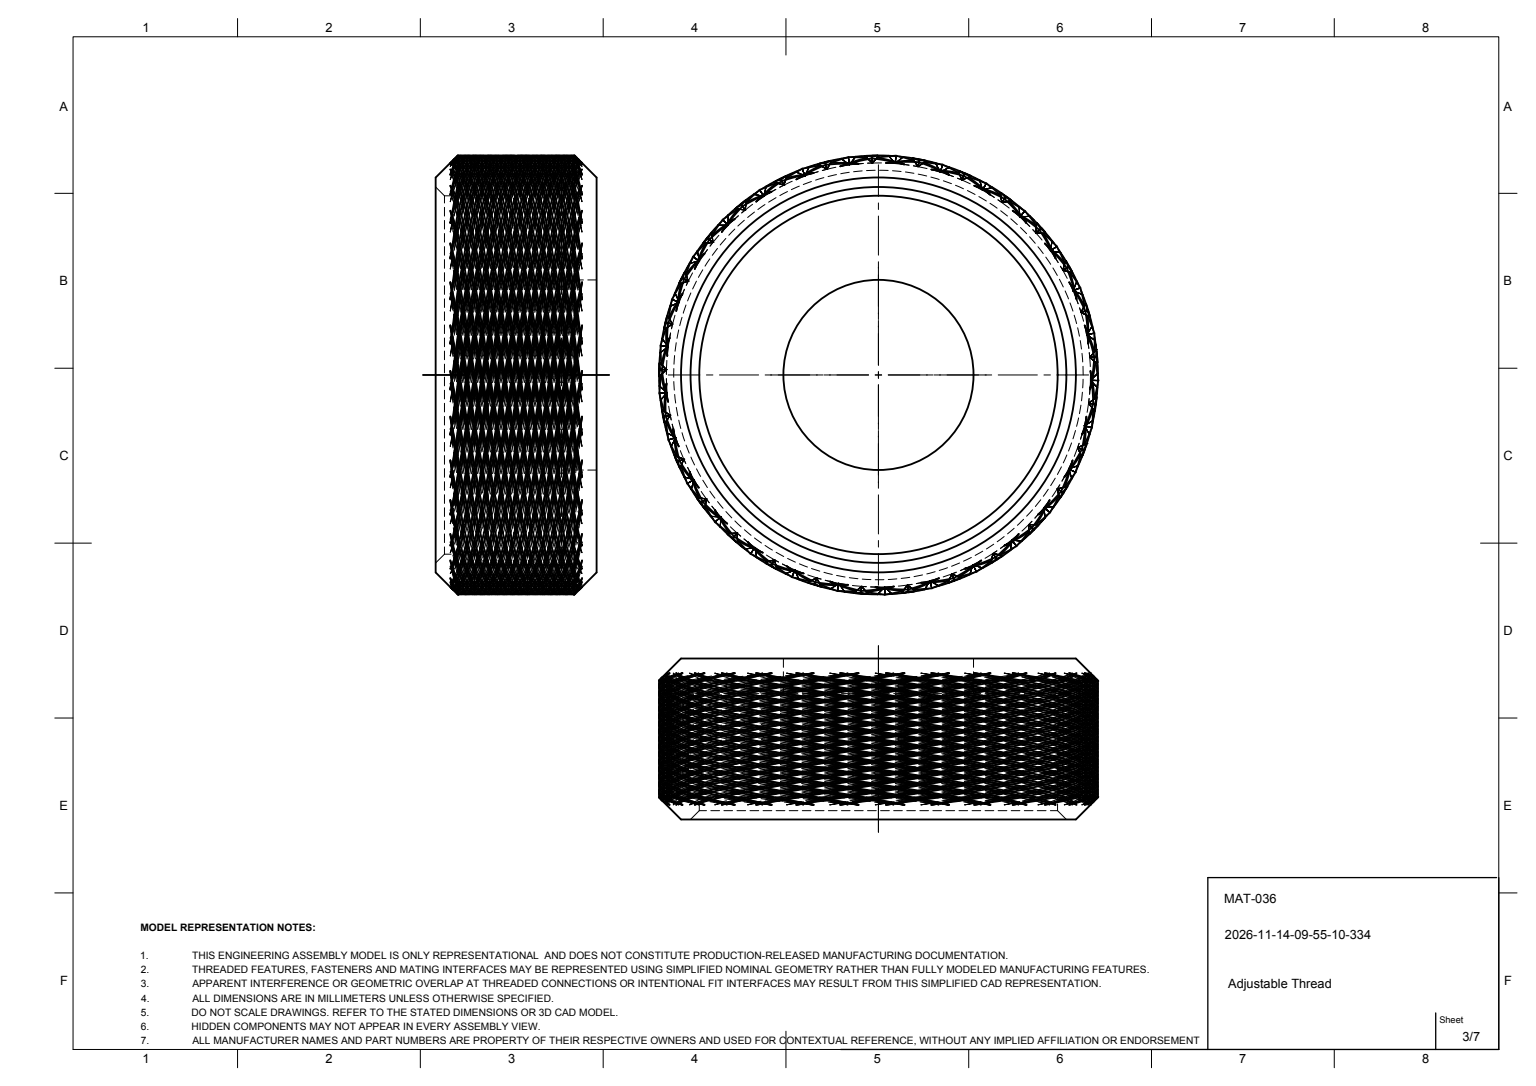
ISO-10303-21;
HEADER;
/* Generated by software containing ST-Developer
 * from STEP Tools, Inc. (www.steptools.com) 
 */

FILE_DESCRIPTION(
/* description */ (''),
/* implementation_level */ '2;1');

FILE_NAME(
/* name */ 'Adjustable Thread.step',
/* time_stamp */ '2026-11-14T09:55:16-08:00',
/* author */ (''),
/* organization */ (''),
/* preprocessor_version */ 'ST-DEVELOPER v20.2',
/* originating_system */ 'Autodesk Translation Framework v15.17.0.0',
/* authorisation */ '');

FILE_SCHEMA (('AUTOMOTIVE_DESIGN { 1 0 10303 214 3 1 1 }'));
ENDSEC;

DATA;
#10=MECHANICAL_DESIGN_GEOMETRIC_PRESENTATION_REPRESENTATION('',(#56),#170250);
#44=SHAPE_REPRESENTATION_RELATIONSHIP('SRR','None',#170276,#50);
#50=ADVANCED_BREP_SHAPE_REPRESENTATION('',(#64),#170244);
#56=STYLED_ITEM('',(#170315),#64);
#64=MANIFOLD_SOLID_BREP('Body1',#71398);
#70=FACE_BOUND('',#15472,.T.);
#71=FACE_BOUND('',#15675,.T.);
#72=FACE_BOUND('',#15851,.T.);
#73=FACE_BOUND('',#15853,.T.);
#86=PLANE('',#77414);
#87=PLANE('',#77609);
#88=PLANE('',#77639);
#89=PLANE('',#77640);
#112=ELLIPSE('',#76563,9.43047305119864,1.30240788908406);
#113=ELLIPSE('',#76566,9.43046793206525,1.30241506001113);
#114=ELLIPSE('',#76569,9.43050328768157,1.3024182004793);
#115=ELLIPSE('',#76572,9.43068708057878,1.30243363570333);
#116=ELLIPSE('',#76575,9.43006152330499,1.30236357371331);
#117=ELLIPSE('',#76578,9.4302777984402,1.30238875446472);
#118=ELLIPSE('',#76581,9.43072787174344,1.30243587534547);
#119=ELLIPSE('',#76584,9.43045773730215,1.30241075091437);
#120=ELLIPSE('',#76587,9.43030510916545,1.30239601642258);
#121=ELLIPSE('',#76590,9.43064494614307,1.30242369243536);
#122=ELLIPSE('',#76593,9.43056062900003,1.30242031583658);
#123=ELLIPSE('',#76596,9.43045585415815,1.30241175558088);
#124=ELLIPSE('',#76599,9.43046939213538,1.30240966255557);
#125=ELLIPSE('',#76602,9.43067088687587,1.30243579801834);
#126=ELLIPSE('',#76605,9.43040719667397,1.30240457641196);
#127=ELLIPSE('',#76608,9.42988108574405,1.30234497490862);
#128=ELLIPSE('',#76611,9.43068064311873,1.30243410507078);
#129=ELLIPSE('',#76614,9.43052303530734,1.30242084912571);
#130=ELLIPSE('',#76617,9.43038125328305,1.30240668645391);
#131=ELLIPSE('',#76620,9.43072128552616,1.30244009783621);
#132=ELLIPSE('',#76623,9.4305707477918,1.30242345770117);
#133=ELLIPSE('',#76626,9.43046465435441,1.30241113143356);
#134=ELLIPSE('',#76629,9.4308407271015,1.30245127577812);
#135=ELLIPSE('',#76632,9.43070104226015,1.30243878786344);
#136=ELLIPSE('',#76635,9.43055049151391,1.30242224667773);
#137=ELLIPSE('',#76638,9.43061695677763,1.30242474192035);
#138=ELLIPSE('',#76641,9.43035235935973,1.30239838521342);
#139=ELLIPSE('',#76644,9.4305559320503,1.30242196321693);
#140=ELLIPSE('',#76647,9.43068952357752,1.30243327777871);
#141=ELLIPSE('',#77415,9.431895379298,1.30254932670111);
#142=ELLIPSE('',#77418,15.3174410154795,1.90661239924035);
#143=ELLIPSE('',#77421,15.3157768747818,1.90647582479234);
#144=ELLIPSE('',#77424,15.3170696122663,1.90658252792732);
#145=ELLIPSE('',#77427,15.3167139940069,1.90655328959697);
#146=ELLIPSE('',#77430,15.3168209377553,1.90657168275161);
#147=ELLIPSE('',#77433,15.3160754936824,1.90650905813206);
#148=ELLIPSE('',#77436,15.3161208425833,1.90650426169268);
#149=ELLIPSE('',#77439,15.3159589603063,1.90649559716548);
#150=ELLIPSE('',#77442,15.3157944590339,1.9064768703695);
#151=ELLIPSE('',#77445,15.3172323469206,1.9066030234614);
#152=ELLIPSE('',#77448,15.3155039380165,1.9064570427492);
#153=ELLIPSE('',#77451,15.3159291529044,1.90649334528717);
#154=ELLIPSE('',#77454,15.3157700330761,1.90647081272421);
#155=ELLIPSE('',#77457,15.3160955154982,1.90650647722667);
#156=ELLIPSE('',#77460,15.3166693144536,1.90656216883429);
#157=ELLIPSE('',#77463,15.3166817133067,1.90655124693864);
#158=ELLIPSE('',#77466,15.31703730362,1.90657833462818);
#159=ELLIPSE('',#77469,15.3160164937855,1.90649874196003);
#160=ELLIPSE('',#77472,15.3158753484009,1.90648217113556);
#161=ELLIPSE('',#77475,15.3162380117898,1.90650822609983);
#162=ELLIPSE('',#77478,15.3156441463648,1.90646585124018);
#163=ELLIPSE('',#77481,15.317005919152,1.90658194664794);
#164=ELLIPSE('',#77484,15.3161739347467,1.90650429978856);
#165=ELLIPSE('',#77487,15.3153630258202,1.90644004375235);
#166=ELLIPSE('',#77490,15.3163094563979,1.90652013375223);
#167=ELLIPSE('',#77493,15.3167561122212,1.90656182181374);
#168=ELLIPSE('',#77496,15.3163730027201,1.90652953147296);
#169=ELLIPSE('',#77499,15.315903684448,1.90649008174056);
#170=ELLIPSE('',#77530,3.69853833711443,0.520053862149324);
#171=ELLIPSE('',#77535,3.6990050944682,0.520121997590068);
#172=ELLIPSE('',#77538,3.69740745136945,0.519884819312743);
#173=ELLIPSE('',#77541,3.6973850577443,0.519871926709589);
#174=ELLIPSE('',#77544,3.69880689749974,0.520100628836089);
#175=ELLIPSE('',#77547,3.69848799508326,0.520043846508826);
#176=ELLIPSE('',#77552,3.6988594244713,0.520105289468088);
#177=ELLIPSE('',#77555,3.6986202776342,0.520065731438254);
#178=ELLIPSE('',#77558,3.69735633553684,0.519872421748739);
#179=ELLIPSE('',#77561,3.69840385438922,0.520042143078421);
#180=ELLIPSE('',#77566,3.69753466975073,0.519893625210943);
#181=ELLIPSE('',#77569,3.69957450398795,0.520227606150056);
#182=ELLIPSE('',#77574,3.69928463265645,0.520166995452598);
#183=ELLIPSE('',#77579,3.69917885823403,0.520148170670083);
#184=ELLIPSE('',#77582,3.69767815300263,0.519919195910691);
#185=ELLIPSE('',#77589,3.69757944713663,0.519903285571644);
#186=ELLIPSE('',#77592,3.69653763812213,0.519733793607226);
#187=ELLIPSE('',#77595,3.69967418134432,0.520228182339355);
#188=ELLIPSE('',#77598,3.69741584633747,0.519874782638118);
#189=ELLIPSE('',#77601,3.69673411928317,0.519776228529677);
#190=ELLIPSE('',#77604,3.69979295210335,0.520255955848595);
#191=ELLIPSE('',#77607,3.69808486598988,0.51998245490985);
#194=(
BOUNDED_SURFACE()
B_SPLINE_SURFACE(1,2,((#95581,#95582,#95583),(#95584,#95585,#95586)),
 .UNSPECIFIED.,.F.,.F.,.F.)
B_SPLINE_SURFACE_WITH_KNOTS((2,2),(3,3),(0.,0.289681084359929),(0.331965345783649,
0.349369696259361),.UNSPECIFIED.)
GEOMETRIC_REPRESENTATION_ITEM()
RATIONAL_B_SPLINE_SURFACE(((0.988555124858681,0.99035748704491,0.99513694090229),
(0.988555124858681,0.99035748704491,0.99513694090229)))
REPRESENTATION_ITEM('')
SURFACE()
);
#195=(
BOUNDED_SURFACE()
B_SPLINE_SURFACE(1,2,((#95600,#95601,#95602,#95603,#95604),(#95605,#95606,
#95607,#95608,#95609),(#95610,#95611,#95612,#95613,#95614)),
 .UNSPECIFIED.,.F.,.F.,.F.)
B_SPLINE_SURFACE_WITH_KNOTS((2,1,2),(3,2,3),(-0.00289807040992861,0.,0.29039955403664),
(0.383340713896693,0.383933227114987,0.401145492974693),.UNSPECIFIED.)
GEOMETRIC_REPRESENTATION_ITEM()
RATIONAL_B_SPLINE_SURFACE(((0.988246641953811,0.988246641953811,0.988246641953811,
0.986737013496293,0.988139125479962),(0.988246641953811,0.988246641953811,
0.988246641953811,0.986737013496293,0.988139125479962),(0.988246641953811,
0.988246641953811,0.988246641953811,0.986737013496293,0.988139125479961)))
REPRESENTATION_ITEM('')
SURFACE()
);
#196=(
BOUNDED_SURFACE()
B_SPLINE_SURFACE(1,2,((#95639,#95640,#95641),(#95642,#95643,#95644)),
 .UNSPECIFIED.,.F.,.F.,.F.)
B_SPLINE_SURFACE_WITH_KNOTS((2,2),(3,3),(0.,0.289681084359919),(0.331965345783649,
0.349369696259361),.UNSPECIFIED.)
GEOMETRIC_REPRESENTATION_ITEM()
RATIONAL_B_SPLINE_SURFACE(((0.988555124858681,0.99035748704491,0.99513694090229),
(0.988555124858682,0.99035748704491,0.99513694090229)))
REPRESENTATION_ITEM('')
SURFACE()
);
#197=(
BOUNDED_SURFACE()
B_SPLINE_SURFACE(1,2,((#95648,#95649,#95650,#95651,#95652),(#95653,#95654,
#95655,#95656,#95657),(#95658,#95659,#95660,#95661,#95662)),
 .UNSPECIFIED.,.F.,.F.,.F.)
B_SPLINE_SURFACE_WITH_KNOTS((2,1,2),(3,2,3),(-0.00289807040992683,0.,0.290399554012505),
(0.38334071392065,0.383933227114987,0.401145492974695),.UNSPECIFIED.)
GEOMETRIC_REPRESENTATION_ITEM()
RATIONAL_B_SPLINE_SURFACE(((0.988246641953811,0.988246641953811,0.988246641953811,
0.986737013496293,0.988139125479962),(0.988246641953811,0.988246641953811,
0.988246641953811,0.986737013496293,0.988139125479962),(0.988246641953811,
0.988246641953811,0.988246641953811,0.986737013496293,0.988139125479962)))
REPRESENTATION_ITEM('')
SURFACE()
);
#198=(
BOUNDED_SURFACE()
B_SPLINE_SURFACE(1,2,((#95687,#95688,#95689),(#95690,#95691,#95692)),
 .UNSPECIFIED.,.F.,.F.,.F.)
B_SPLINE_SURFACE_WITH_KNOTS((2,2),(3,3),(0.,0.289681084359922),(0.331965345783648,
0.349369696259454),.UNSPECIFIED.)
GEOMETRIC_REPRESENTATION_ITEM()
RATIONAL_B_SPLINE_SURFACE(((0.988555124858681,0.99035748704492,0.995136940902341),
(0.988555124858682,0.99035748704492,0.995136940902341)))
REPRESENTATION_ITEM('')
SURFACE()
);
#199=(
BOUNDED_SURFACE()
B_SPLINE_SURFACE(1,2,((#95696,#95697,#95698,#95699,#95700),(#95701,#95702,
#95703,#95704,#95705),(#95706,#95707,#95708,#95709,#95710)),
 .UNSPECIFIED.,.F.,.F.,.F.)
B_SPLINE_SURFACE_WITH_KNOTS((2,1,2),(3,2,3),(-0.00289807040992654,0.,0.290399554026877),
(0.383340713906249,0.383933227114987,0.401145492974697),.UNSPECIFIED.)
GEOMETRIC_REPRESENTATION_ITEM()
RATIONAL_B_SPLINE_SURFACE(((0.988246641953811,0.988246641953811,0.988246641953811,
0.986737013496293,0.988139125479962),(0.988246641953811,0.988246641953811,
0.988246641953811,0.986737013496293,0.988139125479962),(0.988246641953811,
0.988246641953811,0.988246641953811,0.986737013496293,0.988139125479962)))
REPRESENTATION_ITEM('')
SURFACE()
);
#200=(
BOUNDED_SURFACE()
B_SPLINE_SURFACE(1,2,((#95735,#95736,#95737),(#95738,#95739,#95740)),
 .UNSPECIFIED.,.F.,.F.,.F.)
B_SPLINE_SURFACE_WITH_KNOTS((2,2),(3,3),(0.,0.289681084359918),(0.331965345783649,
0.349369696259361),.UNSPECIFIED.)
GEOMETRIC_REPRESENTATION_ITEM()
RATIONAL_B_SPLINE_SURFACE(((0.988555124858682,0.99035748704491,0.99513694090229),
(0.988555124858682,0.99035748704491,0.99513694090229)))
REPRESENTATION_ITEM('')
SURFACE()
);
#201=(
BOUNDED_SURFACE()
B_SPLINE_SURFACE(1,2,((#95744,#95745,#95746,#95747,#95748),(#95749,#95750,
#95751,#95752,#95753),(#95754,#95755,#95756,#95757,#95758)),
 .UNSPECIFIED.,.F.,.F.,.F.)
B_SPLINE_SURFACE_WITH_KNOTS((2,1,2),(3,2,3),(-0.00289807040992802,0.,0.29039955403663),
(0.383340713896644,0.383933227114987,0.401145492974693),.UNSPECIFIED.)
GEOMETRIC_REPRESENTATION_ITEM()
RATIONAL_B_SPLINE_SURFACE(((0.988246641953811,0.988246641953811,0.988246641953811,
0.986737013496293,0.988139125479962),(0.988246641953811,0.988246641953811,
0.988246641953811,0.986737013496293,0.988139125479962),(0.988246641953811,
0.988246641953811,0.988246641953811,0.986737013496293,0.988139125479962)))
REPRESENTATION_ITEM('')
SURFACE()
);
#202=(
BOUNDED_SURFACE()
B_SPLINE_SURFACE(1,2,((#95783,#95784,#95785),(#95786,#95787,#95788)),
 .UNSPECIFIED.,.F.,.F.,.F.)
B_SPLINE_SURFACE_WITH_KNOTS((2,2),(3,3),(0.,0.289681084359923),(0.331965345783649,
0.349369696259361),.UNSPECIFIED.)
GEOMETRIC_REPRESENTATION_ITEM()
RATIONAL_B_SPLINE_SURFACE(((0.988555124858681,0.99035748704491,0.99513694090229),
(0.988555124858682,0.99035748704491,0.99513694090229)))
REPRESENTATION_ITEM('')
SURFACE()
);
#203=(
BOUNDED_SURFACE()
B_SPLINE_SURFACE(1,2,((#95792,#95793,#95794,#95795,#95796),(#95797,#95798,
#95799,#95800,#95801),(#95802,#95803,#95804,#95805,#95806)),
 .UNSPECIFIED.,.F.,.F.,.F.)
B_SPLINE_SURFACE_WITH_KNOTS((2,1,2),(3,2,3),(-0.00289807040992325,0.,0.290399554035561),
(0.383340713897236,0.383933227114987,0.401145492974693),.UNSPECIFIED.)
GEOMETRIC_REPRESENTATION_ITEM()
RATIONAL_B_SPLINE_SURFACE(((0.988246641953811,0.988246641953811,0.988246641953811,
0.986737013496293,0.988139125479962),(0.988246641953811,0.988246641953811,
0.988246641953811,0.986737013496293,0.988139125479962),(0.988246641953811,
0.988246641953811,0.988246641953811,0.986737013496293,0.988139125479961)))
REPRESENTATION_ITEM('')
SURFACE()
);
#204=(
BOUNDED_SURFACE()
B_SPLINE_SURFACE(1,2,((#95831,#95832,#95833),(#95834,#95835,#95836)),
 .UNSPECIFIED.,.F.,.F.,.F.)
B_SPLINE_SURFACE_WITH_KNOTS((2,2),(3,3),(0.,0.289681084359924),(0.331965345783649,
0.349369696259361),.UNSPECIFIED.)
GEOMETRIC_REPRESENTATION_ITEM()
RATIONAL_B_SPLINE_SURFACE(((0.988555124858681,0.99035748704491,0.99513694090229),
(0.988555124858682,0.99035748704491,0.99513694090229)))
REPRESENTATION_ITEM('')
SURFACE()
);
#205=(
BOUNDED_SURFACE()
B_SPLINE_SURFACE(1,2,((#95840,#95841,#95842,#95843,#95844),(#95845,#95846,
#95847,#95848,#95849),(#95850,#95851,#95852,#95853,#95854)),
 .UNSPECIFIED.,.F.,.F.,.F.)
B_SPLINE_SURFACE_WITH_KNOTS((2,1,2),(3,2,3),(-0.00289807040992448,0.,0.290399554023854),
(0.383340713909065,0.383933227114976,0.401145492974693),.UNSPECIFIED.)
GEOMETRIC_REPRESENTATION_ITEM()
RATIONAL_B_SPLINE_SURFACE(((0.988246641953813,0.988246641953813,0.988246641953813,
0.986737013496292,0.988139125479961),(0.988246641953813,0.988246641953813,
0.988246641953813,0.986737013496292,0.988139125479961),(0.988246641953813,
0.988246641953813,0.988246641953813,0.986737013496292,0.988139125479961)))
REPRESENTATION_ITEM('')
SURFACE()
);
#206=(
BOUNDED_SURFACE()
B_SPLINE_SURFACE(1,2,((#95879,#95880,#95881),(#95882,#95883,#95884)),
 .UNSPECIFIED.,.F.,.F.,.F.)
B_SPLINE_SURFACE_WITH_KNOTS((2,2),(3,3),(0.,0.289681084359932),(0.331965345783649,
0.349369696259361),.UNSPECIFIED.)
GEOMETRIC_REPRESENTATION_ITEM()
RATIONAL_B_SPLINE_SURFACE(((0.988555124858682,0.99035748704491,0.99513694090229),
(0.988555124858682,0.99035748704491,0.99513694090229)))
REPRESENTATION_ITEM('')
SURFACE()
);
#207=(
BOUNDED_SURFACE()
B_SPLINE_SURFACE(1,2,((#95888,#95889,#95890,#95891,#95892),(#95893,#95894,
#95895,#95896,#95897),(#95898,#95899,#95900,#95901,#95902)),
 .UNSPECIFIED.,.F.,.F.,.F.)
B_SPLINE_SURFACE_WITH_KNOTS((2,1,2),(3,2,3),(-0.00289807040992691,0.,0.290399554024332),
(0.383340713908832,0.383933227114987,0.401145492974693),.UNSPECIFIED.)
GEOMETRIC_REPRESENTATION_ITEM()
RATIONAL_B_SPLINE_SURFACE(((0.988246641953811,0.988246641953811,0.988246641953811,
0.986737013496293,0.988139125479962),(0.988246641953811,0.988246641953811,
0.988246641953811,0.986737013496293,0.988139125479962),(0.988246641953811,
0.988246641953811,0.988246641953811,0.986737013496293,0.988139125479962)))
REPRESENTATION_ITEM('')
SURFACE()
);
#208=(
BOUNDED_SURFACE()
B_SPLINE_SURFACE(1,2,((#95912,#95913,#95914),(#95915,#95916,#95917)),
 .UNSPECIFIED.,.F.,.F.,.F.)
B_SPLINE_SURFACE_WITH_KNOTS((2,2),(3,3),(0.,0.289681084359925),(0.331965345783649,
0.349369696259361),.UNSPECIFIED.)
GEOMETRIC_REPRESENTATION_ITEM()
RATIONAL_B_SPLINE_SURFACE(((0.988555124858682,0.99035748704491,0.99513694090229),
(0.988555124858682,0.99035748704491,0.99513694090229)))
REPRESENTATION_ITEM('')
SURFACE()
);
#209=(
BOUNDED_SURFACE()
B_SPLINE_SURFACE(1,2,((#95921,#95922,#95923,#95924,#95925),(#95926,#95927,
#95928,#95929,#95930),(#95931,#95932,#95933,#95934,#95935)),
 .UNSPECIFIED.,.F.,.F.,.F.)
B_SPLINE_SURFACE_WITH_KNOTS((2,1,2),(3,2,3),(-0.00289807040992912,0.,0.290399554034495),
(0.383340713898888,0.383933227114987,0.401145492974693),.UNSPECIFIED.)
GEOMETRIC_REPRESENTATION_ITEM()
RATIONAL_B_SPLINE_SURFACE(((0.988246641953811,0.988246641953811,0.988246641953811,
0.986737013496293,0.988139125479962),(0.988246641953811,0.988246641953811,
0.988246641953811,0.986737013496293,0.988139125479962),(0.988246641953811,
0.988246641953811,0.988246641953811,0.986737013496293,0.988139125479962)))
REPRESENTATION_ITEM('')
SURFACE()
);
#210=(
BOUNDED_SURFACE()
B_SPLINE_SURFACE(1,2,((#95960,#95961,#95962),(#95963,#95964,#95965)),
 .UNSPECIFIED.,.F.,.F.,.F.)
B_SPLINE_SURFACE_WITH_KNOTS((2,2),(3,3),(0.,0.28968108435992),(0.331965345783649,
0.349369696259364),.UNSPECIFIED.)
GEOMETRIC_REPRESENTATION_ITEM()
RATIONAL_B_SPLINE_SURFACE(((0.988555124858682,0.990357487044911,0.995136940902291),
(0.988555124858682,0.990357487044911,0.995136940902291)))
REPRESENTATION_ITEM('')
SURFACE()
);
#211=(
BOUNDED_SURFACE()
B_SPLINE_SURFACE(1,2,((#95969,#95970,#95971,#95972,#95973),(#95974,#95975,
#95976,#95977,#95978),(#95979,#95980,#95981,#95982,#95983)),
 .UNSPECIFIED.,.F.,.F.,.F.)
B_SPLINE_SURFACE_WITH_KNOTS((2,1,2),(3,2,3),(-0.0028980704099176,0.,0.290399554034344),
(0.383340713897888,0.383933227114987,0.401145492974693),.UNSPECIFIED.)
GEOMETRIC_REPRESENTATION_ITEM()
RATIONAL_B_SPLINE_SURFACE(((0.988246641953811,0.988246641953811,0.988246641953811,
0.986737013496293,0.988139125479962),(0.988246641953811,0.988246641953811,
0.988246641953811,0.986737013496293,0.988139125479962),(0.988246641953811,
0.988246641953811,0.988246641953811,0.986737013496293,0.988139125479961)))
REPRESENTATION_ITEM('')
SURFACE()
);
#212=(
BOUNDED_SURFACE()
B_SPLINE_SURFACE(1,2,((#96008,#96009,#96010),(#96011,#96012,#96013)),
 .UNSPECIFIED.,.F.,.F.,.F.)
B_SPLINE_SURFACE_WITH_KNOTS((2,2),(3,3),(0.,0.289681084359917),(0.331965345783649,
0.349369696259361),.UNSPECIFIED.)
GEOMETRIC_REPRESENTATION_ITEM()
RATIONAL_B_SPLINE_SURFACE(((0.988555124858681,0.99035748704491,0.99513694090229),
(0.988555124858681,0.99035748704491,0.99513694090229)))
REPRESENTATION_ITEM('')
SURFACE()
);
#213=(
BOUNDED_SURFACE()
B_SPLINE_SURFACE(1,2,((#96017,#96018,#96019,#96020,#96021),(#96022,#96023,
#96024,#96025,#96026),(#96027,#96028,#96029,#96030,#96031)),
 .UNSPECIFIED.,.F.,.F.,.F.)
B_SPLINE_SURFACE_WITH_KNOTS((2,1,2),(3,2,3),(-0.00289807040991716,0.,0.29039955402085),
(0.383340713911338,0.383933227114987,0.401145492974693),.UNSPECIFIED.)
GEOMETRIC_REPRESENTATION_ITEM()
RATIONAL_B_SPLINE_SURFACE(((0.988246641953811,0.988246641953811,0.988246641953811,
0.986737013496293,0.988139125479962),(0.988246641953811,0.988246641953811,
0.988246641953811,0.986737013496293,0.988139125479962),(0.988246641953811,
0.988246641953811,0.988246641953811,0.986737013496293,0.988139125479962)))
REPRESENTATION_ITEM('')
SURFACE()
);
#214=(
BOUNDED_SURFACE()
B_SPLINE_SURFACE(1,2,((#96056,#96057,#96058),(#96059,#96060,#96061)),
 .UNSPECIFIED.,.F.,.F.,.F.)
B_SPLINE_SURFACE_WITH_KNOTS((2,2),(3,3),(0.,0.289681084359927),(0.331965345783649,
0.349369696259361),.UNSPECIFIED.)
GEOMETRIC_REPRESENTATION_ITEM()
RATIONAL_B_SPLINE_SURFACE(((0.988555124858681,0.99035748704491,0.99513694090229),
(0.988555124858682,0.99035748704491,0.99513694090229)))
REPRESENTATION_ITEM('')
SURFACE()
);
#215=(
BOUNDED_SURFACE()
B_SPLINE_SURFACE(1,2,((#96065,#96066,#96067,#96068,#96069),(#96070,#96071,
#96072,#96073,#96074),(#96075,#96076,#96077,#96078,#96079)),
 .UNSPECIFIED.,.F.,.F.,.F.)
B_SPLINE_SURFACE_WITH_KNOTS((2,1,2),(3,2,3),(-0.00289807040991567,0.,0.290399554021739),
(0.3833407139103,0.383933227114987,0.401145492974693),.UNSPECIFIED.)
GEOMETRIC_REPRESENTATION_ITEM()
RATIONAL_B_SPLINE_SURFACE(((0.988246641953811,0.988246641953811,0.988246641953811,
0.986737013496293,0.988139125479962),(0.988246641953811,0.988246641953811,
0.988246641953811,0.986737013496293,0.988139125479962),(0.988246641953811,
0.988246641953811,0.988246641953811,0.986737013496293,0.988139125479962)))
REPRESENTATION_ITEM('')
SURFACE()
);
#216=(
BOUNDED_SURFACE()
B_SPLINE_SURFACE(1,2,((#96104,#96105,#96106),(#96107,#96108,#96109)),
 .UNSPECIFIED.,.F.,.F.,.F.)
B_SPLINE_SURFACE_WITH_KNOTS((2,2),(3,3),(0.,0.289681084359927),(0.331965345783649,
0.349369696259361),.UNSPECIFIED.)
GEOMETRIC_REPRESENTATION_ITEM()
RATIONAL_B_SPLINE_SURFACE(((0.988555124858681,0.99035748704491,0.99513694090229),
(0.988555124858682,0.99035748704491,0.99513694090229)))
REPRESENTATION_ITEM('')
SURFACE()
);
#217=(
BOUNDED_SURFACE()
B_SPLINE_SURFACE(1,2,((#96113,#96114,#96115,#96116,#96117),(#96118,#96119,
#96120,#96121,#96122),(#96123,#96124,#96125,#96126,#96127)),
 .UNSPECIFIED.,.F.,.F.,.F.)
B_SPLINE_SURFACE_WITH_KNOTS((2,1,2),(3,2,3),(-0.00289807040991562,0.,0.290399554030109),
(0.383340713901925,0.383933227114987,0.401145492974693),.UNSPECIFIED.)
GEOMETRIC_REPRESENTATION_ITEM()
RATIONAL_B_SPLINE_SURFACE(((0.988246641953811,0.988246641953811,0.988246641953811,
0.986737013496293,0.988139125479962),(0.988246641953811,0.988246641953811,
0.988246641953811,0.986737013496293,0.988139125479962),(0.988246641953811,
0.988246641953811,0.988246641953811,0.986737013496293,0.988139125479962)))
REPRESENTATION_ITEM('')
SURFACE()
);
#218=(
BOUNDED_SURFACE()
B_SPLINE_SURFACE(1,2,((#96152,#96153,#96154),(#96155,#96156,#96157)),
 .UNSPECIFIED.,.F.,.F.,.F.)
B_SPLINE_SURFACE_WITH_KNOTS((2,2),(3,3),(0.,0.289681084359926),(0.331965345783649,
0.349369696259361),.UNSPECIFIED.)
GEOMETRIC_REPRESENTATION_ITEM()
RATIONAL_B_SPLINE_SURFACE(((0.988555124858682,0.99035748704491,0.99513694090229),
(0.988555124858682,0.99035748704491,0.99513694090229)))
REPRESENTATION_ITEM('')
SURFACE()
);
#219=(
BOUNDED_SURFACE()
B_SPLINE_SURFACE(1,2,((#96161,#96162,#96163,#96164,#96165),(#96166,#96167,
#96168,#96169,#96170),(#96171,#96172,#96173,#96174,#96175)),
 .UNSPECIFIED.,.F.,.F.,.F.)
B_SPLINE_SURFACE_WITH_KNOTS((2,1,2),(3,2,3),(-0.00289807040991561,0.,0.290399554022484),
(0.383340713909549,0.383933227114987,0.401145492974693),.UNSPECIFIED.)
GEOMETRIC_REPRESENTATION_ITEM()
RATIONAL_B_SPLINE_SURFACE(((0.988246641953811,0.988246641953811,0.988246641953811,
0.986737013496293,0.988139125479962),(0.988246641953811,0.988246641953811,
0.988246641953811,0.986737013496293,0.988139125479962),(0.988246641953811,
0.988246641953811,0.988246641953811,0.986737013496293,0.988139125479962)))
REPRESENTATION_ITEM('')
SURFACE()
);
#220=(
BOUNDED_SURFACE()
B_SPLINE_SURFACE(1,2,((#96200,#96201,#96202),(#96203,#96204,#96205)),
 .UNSPECIFIED.,.F.,.F.,.F.)
B_SPLINE_SURFACE_WITH_KNOTS((2,2),(3,3),(0.,0.289681084359927),(0.331965345783649,
0.349369696259361),.UNSPECIFIED.)
GEOMETRIC_REPRESENTATION_ITEM()
RATIONAL_B_SPLINE_SURFACE(((0.988555124858682,0.99035748704491,0.99513694090229),
(0.988555124858682,0.99035748704491,0.99513694090229)))
REPRESENTATION_ITEM('')
SURFACE()
);
#221=(
BOUNDED_SURFACE()
B_SPLINE_SURFACE(1,2,((#96209,#96210,#96211,#96212,#96213),(#96214,#96215,
#96216,#96217,#96218),(#96219,#96220,#96221,#96222,#96223)),
 .UNSPECIFIED.,.F.,.F.,.F.)
B_SPLINE_SURFACE_WITH_KNOTS((2,1,2),(3,2,3),(-0.00289807040991793,0.,0.290399554012505),
(0.38334071391976,0.383933227114987,0.401145492974693),.UNSPECIFIED.)
GEOMETRIC_REPRESENTATION_ITEM()
RATIONAL_B_SPLINE_SURFACE(((0.988246641953811,0.988246641953811,0.988246641953811,
0.986737013496293,0.988139125479962),(0.988246641953811,0.988246641953811,
0.988246641953811,0.986737013496293,0.988139125479962),(0.988246641953811,
0.988246641953811,0.988246641953811,0.986737013496293,0.988139125479962)))
REPRESENTATION_ITEM('')
SURFACE()
);
#222=(
BOUNDED_SURFACE()
B_SPLINE_SURFACE(1,2,((#96248,#96249,#96250),(#96251,#96252,#96253)),
 .UNSPECIFIED.,.F.,.F.,.F.)
B_SPLINE_SURFACE_WITH_KNOTS((2,2),(3,3),(0.,0.289681084359918),(0.331965345783649,
0.349369696259361),.UNSPECIFIED.)
GEOMETRIC_REPRESENTATION_ITEM()
RATIONAL_B_SPLINE_SURFACE(((0.988555124858682,0.99035748704491,0.99513694090229),
(0.988555124858682,0.99035748704491,0.99513694090229)))
REPRESENTATION_ITEM('')
SURFACE()
);
#223=(
BOUNDED_SURFACE()
B_SPLINE_SURFACE(1,2,((#96257,#96258,#96259,#96260,#96261),(#96262,#96263,
#96264,#96265,#96266),(#96267,#96268,#96269,#96270,#96271)),
 .UNSPECIFIED.,.F.,.F.,.F.)
B_SPLINE_SURFACE_WITH_KNOTS((2,1,2),(3,2,3),(-0.00289807040991568,0.,0.290399554034899),
(0.38334071389714,0.383933227114987,0.401145492974693),.UNSPECIFIED.)
GEOMETRIC_REPRESENTATION_ITEM()
RATIONAL_B_SPLINE_SURFACE(((0.988246641953811,0.988246641953811,0.988246641953811,
0.986737013496293,0.988139125479962),(0.988246641953811,0.988246641953811,
0.988246641953811,0.986737013496293,0.988139125479962),(0.988246641953811,
0.988246641953811,0.988246641953811,0.986737013496293,0.988139125479962)))
REPRESENTATION_ITEM('')
SURFACE()
);
#224=(
BOUNDED_SURFACE()
B_SPLINE_SURFACE(1,2,((#96296,#96297,#96298),(#96299,#96300,#96301)),
 .UNSPECIFIED.,.F.,.F.,.F.)
B_SPLINE_SURFACE_WITH_KNOTS((2,2),(3,3),(0.,0.289681084359924),(0.331965345783649,
0.349369696259361),.UNSPECIFIED.)
GEOMETRIC_REPRESENTATION_ITEM()
RATIONAL_B_SPLINE_SURFACE(((0.988555124858681,0.99035748704491,0.99513694090229),
(0.988555124858682,0.99035748704491,0.99513694090229)))
REPRESENTATION_ITEM('')
SURFACE()
);
#225=(
BOUNDED_SURFACE()
B_SPLINE_SURFACE(1,2,((#96305,#96306,#96307,#96308,#96309),(#96310,#96311,
#96312,#96313,#96314),(#96315,#96316,#96317,#96318,#96319)),
 .UNSPECIFIED.,.F.,.F.,.F.)
B_SPLINE_SURFACE_WITH_KNOTS((2,1,2),(3,2,3),(-0.0028980704099169,0.,0.290399554016211),
(0.383340713915951,0.383933227114987,0.401145492974693),.UNSPECIFIED.)
GEOMETRIC_REPRESENTATION_ITEM()
RATIONAL_B_SPLINE_SURFACE(((0.988246641953811,0.988246641953811,0.988246641953811,
0.986737013496293,0.988139125479962),(0.988246641953811,0.988246641953811,
0.988246641953811,0.986737013496293,0.988139125479962),(0.988246641953811,
0.988246641953811,0.988246641953811,0.986737013496293,0.988139125479962)))
REPRESENTATION_ITEM('')
SURFACE()
);
#226=(
BOUNDED_SURFACE()
B_SPLINE_SURFACE(1,2,((#96344,#96345,#96346),(#96347,#96348,#96349)),
 .UNSPECIFIED.,.F.,.F.,.F.)
B_SPLINE_SURFACE_WITH_KNOTS((2,2),(3,3),(0.,0.289681084359922),(0.331965345783649,
0.349369696259361),.UNSPECIFIED.)
GEOMETRIC_REPRESENTATION_ITEM()
RATIONAL_B_SPLINE_SURFACE(((0.988555124858682,0.99035748704491,0.99513694090229),
(0.988555124858682,0.99035748704491,0.99513694090229)))
REPRESENTATION_ITEM('')
SURFACE()
);
#227=(
BOUNDED_SURFACE()
B_SPLINE_SURFACE(1,2,((#96353,#96354,#96355,#96356,#96357),(#96358,#96359,
#96360,#96361,#96362),(#96363,#96364,#96365,#96366,#96367)),
 .UNSPECIFIED.,.F.,.F.,.F.)
B_SPLINE_SURFACE_WITH_KNOTS((2,1,2),(3,2,3),(-0.00289807040992971,0.,0.290399554009193),
(0.38334071392425,0.383933227114987,0.401145492974693),.UNSPECIFIED.)
GEOMETRIC_REPRESENTATION_ITEM()
RATIONAL_B_SPLINE_SURFACE(((0.988246641953811,0.988246641953811,0.988246641953811,
0.986737013496293,0.988139125479962),(0.988246641953811,0.988246641953811,
0.988246641953811,0.986737013496293,0.988139125479962),(0.988246641953811,
0.988246641953811,0.988246641953811,0.986737013496293,0.988139125479962)))
REPRESENTATION_ITEM('')
SURFACE()
);
#228=(
BOUNDED_SURFACE()
B_SPLINE_SURFACE(1,2,((#96392,#96393,#96394),(#96395,#96396,#96397)),
 .UNSPECIFIED.,.F.,.F.,.F.)
B_SPLINE_SURFACE_WITH_KNOTS((2,2),(3,3),(0.,0.28968108435992),(0.331965345783649,
0.349369696259361),.UNSPECIFIED.)
GEOMETRIC_REPRESENTATION_ITEM()
RATIONAL_B_SPLINE_SURFACE(((0.988555124858682,0.99035748704491,0.99513694090229),
(0.988555124858682,0.99035748704491,0.99513694090229)))
REPRESENTATION_ITEM('')
SURFACE()
);
#229=(
BOUNDED_SURFACE()
B_SPLINE_SURFACE(1,2,((#96401,#96402,#96403,#96404,#96405),(#96406,#96407,
#96408,#96409,#96410),(#96411,#96412,#96413,#96414,#96415)),
 .UNSPECIFIED.,.F.,.F.,.F.)
B_SPLINE_SURFACE_WITH_KNOTS((2,1,2),(3,2,3),(-0.00289807040991918,0.,0.290399554039631),
(0.383340713892758,0.383933227114987,0.401145492974693),.UNSPECIFIED.)
GEOMETRIC_REPRESENTATION_ITEM()
RATIONAL_B_SPLINE_SURFACE(((0.988246641953811,0.988246641953811,0.988246641953811,
0.986737013496293,0.988139125479962),(0.988246641953811,0.988246641953811,
0.988246641953811,0.986737013496293,0.988139125479962),(0.988246641953811,
0.988246641953811,0.988246641953811,0.986737013496293,0.988139125479962)))
REPRESENTATION_ITEM('')
SURFACE()
);
#230=(
BOUNDED_SURFACE()
B_SPLINE_SURFACE(1,2,((#96440,#96441,#96442),(#96443,#96444,#96445)),
 .UNSPECIFIED.,.F.,.F.,.F.)
B_SPLINE_SURFACE_WITH_KNOTS((2,2),(3,3),(0.,0.289681084359919),(0.331965345783649,
0.349369696259361),.UNSPECIFIED.)
GEOMETRIC_REPRESENTATION_ITEM()
RATIONAL_B_SPLINE_SURFACE(((0.988555124858682,0.99035748704491,0.99513694090229),
(0.988555124858682,0.99035748704491,0.99513694090229)))
REPRESENTATION_ITEM('')
SURFACE()
);
#231=(
BOUNDED_SURFACE()
B_SPLINE_SURFACE(1,2,((#96449,#96450,#96451,#96452,#96453),(#96454,#96455,
#96456,#96457,#96458),(#96459,#96460,#96461,#96462,#96463)),
 .UNSPECIFIED.,.F.,.F.,.F.)
B_SPLINE_SURFACE_WITH_KNOTS((2,1,2),(3,2,3),(-0.0028980704099156,0.,0.290399554016024),
(0.383340713916008,0.383933227114987,0.401145492974693),.UNSPECIFIED.)
GEOMETRIC_REPRESENTATION_ITEM()
RATIONAL_B_SPLINE_SURFACE(((0.988246641953811,0.988246641953811,0.988246641953811,
0.986737013496293,0.988139125479962),(0.988246641953811,0.988246641953811,
0.988246641953811,0.986737013496293,0.988139125479962),(0.988246641953811,
0.988246641953811,0.988246641953811,0.986737013496293,0.988139125479962)))
REPRESENTATION_ITEM('')
SURFACE()
);
#232=(
BOUNDED_SURFACE()
B_SPLINE_SURFACE(1,2,((#96488,#96489,#96490),(#96491,#96492,#96493)),
 .UNSPECIFIED.,.F.,.F.,.F.)
B_SPLINE_SURFACE_WITH_KNOTS((2,2),(3,3),(0.,0.289681084359922),(0.331965345783649,
0.349369696259361),.UNSPECIFIED.)
GEOMETRIC_REPRESENTATION_ITEM()
RATIONAL_B_SPLINE_SURFACE(((0.988555124858681,0.99035748704491,0.99513694090229),
(0.988555124858682,0.99035748704491,0.99513694090229)))
REPRESENTATION_ITEM('')
SURFACE()
);
#233=(
BOUNDED_SURFACE()
B_SPLINE_SURFACE(1,2,((#96497,#96498,#96499,#96500,#96501),(#96502,#96503,
#96504,#96505,#96506),(#96507,#96508,#96509,#96510,#96511)),
 .UNSPECIFIED.,.F.,.F.,.F.)
B_SPLINE_SURFACE_WITH_KNOTS((2,1,2),(3,2,3),(-0.00289807040991647,0.,0.290399554018306),
(0.383340713913812,0.383933227114987,0.401145492974693),.UNSPECIFIED.)
GEOMETRIC_REPRESENTATION_ITEM()
RATIONAL_B_SPLINE_SURFACE(((0.988246641953811,0.988246641953811,0.988246641953811,
0.986737013496293,0.988139125479962),(0.988246641953811,0.988246641953811,
0.988246641953811,0.986737013496293,0.988139125479962),(0.988246641953811,
0.988246641953811,0.988246641953811,0.986737013496293,0.988139125479962)))
REPRESENTATION_ITEM('')
SURFACE()
);
#234=(
BOUNDED_SURFACE()
B_SPLINE_SURFACE(1,2,((#96536,#96537,#96538),(#96539,#96540,#96541)),
 .UNSPECIFIED.,.F.,.F.,.F.)
B_SPLINE_SURFACE_WITH_KNOTS((2,2),(3,3),(0.,0.289681084359919),(0.331965345783649,
0.349369696259361),.UNSPECIFIED.)
GEOMETRIC_REPRESENTATION_ITEM()
RATIONAL_B_SPLINE_SURFACE(((0.988555124858681,0.99035748704491,0.99513694090229),
(0.988555124858681,0.99035748704491,0.99513694090229)))
REPRESENTATION_ITEM('')
SURFACE()
);
#235=(
BOUNDED_SURFACE()
B_SPLINE_SURFACE(1,2,((#96545,#96546,#96547,#96548,#96549),(#96550,#96551,
#96552,#96553,#96554),(#96555,#96556,#96557,#96558,#96559)),
 .UNSPECIFIED.,.F.,.F.,.F.)
B_SPLINE_SURFACE_WITH_KNOTS((2,1,2),(3,2,3),(-0.00289807040991561,0.,0.29039955400762),
(0.383340713924413,0.383933227114987,0.401145492974693),.UNSPECIFIED.)
GEOMETRIC_REPRESENTATION_ITEM()
RATIONAL_B_SPLINE_SURFACE(((0.988246641953811,0.988246641953811,0.988246641953811,
0.986737013496293,0.988139125479961),(0.988246641953811,0.988246641953811,
0.988246641953811,0.986737013496293,0.988139125479961),(0.988246641953811,
0.988246641953811,0.988246641953811,0.986737013496293,0.988139125479961)))
REPRESENTATION_ITEM('')
SURFACE()
);
#236=(
BOUNDED_SURFACE()
B_SPLINE_SURFACE(1,2,((#96584,#96585,#96586),(#96587,#96588,#96589)),
 .UNSPECIFIED.,.F.,.F.,.F.)
B_SPLINE_SURFACE_WITH_KNOTS((2,2),(3,3),(0.,0.289681084359919),(0.331965345783649,
0.349369696259361),.UNSPECIFIED.)
GEOMETRIC_REPRESENTATION_ITEM()
RATIONAL_B_SPLINE_SURFACE(((0.988555124858682,0.99035748704491,0.99513694090229),
(0.988555124858682,0.99035748704491,0.99513694090229)))
REPRESENTATION_ITEM('')
SURFACE()
);
#237=(
BOUNDED_SURFACE()
B_SPLINE_SURFACE(1,2,((#96593,#96594,#96595,#96596,#96597),(#96598,#96599,
#96600,#96601,#96602),(#96603,#96604,#96605,#96606,#96607)),
 .UNSPECIFIED.,.F.,.F.,.F.)
B_SPLINE_SURFACE_WITH_KNOTS((2,1,2),(3,2,3),(-0.00289807040991639,0.,0.290399554026997),
(0.383340713905114,0.383933227114987,0.401145492974693),.UNSPECIFIED.)
GEOMETRIC_REPRESENTATION_ITEM()
RATIONAL_B_SPLINE_SURFACE(((0.988246641953811,0.988246641953811,0.988246641953811,
0.986737013496293,0.988139125479962),(0.988246641953811,0.988246641953811,
0.988246641953811,0.986737013496293,0.988139125479962),(0.988246641953811,
0.988246641953811,0.988246641953811,0.986737013496293,0.988139125479962)))
REPRESENTATION_ITEM('')
SURFACE()
);
#238=(
BOUNDED_SURFACE()
B_SPLINE_SURFACE(1,2,((#96632,#96633,#96634),(#96635,#96636,#96637)),
 .UNSPECIFIED.,.F.,.F.,.F.)
B_SPLINE_SURFACE_WITH_KNOTS((2,2),(3,3),(0.,0.28968108435992),(0.331965345783649,
0.349369696259361),.UNSPECIFIED.)
GEOMETRIC_REPRESENTATION_ITEM()
RATIONAL_B_SPLINE_SURFACE(((0.988555124858682,0.99035748704491,0.99513694090229),
(0.988555124858682,0.99035748704491,0.99513694090229)))
REPRESENTATION_ITEM('')
SURFACE()
);
#239=(
BOUNDED_SURFACE()
B_SPLINE_SURFACE(1,2,((#96641,#96642,#96643,#96644,#96645),(#96646,#96647,
#96648,#96649,#96650),(#96651,#96652,#96653,#96654,#96655)),
 .UNSPECIFIED.,.F.,.F.,.F.)
B_SPLINE_SURFACE_WITH_KNOTS((2,1,2),(3,2,3),(-0.00289807040991643,0.,0.290399554033924),
(0.383340713898191,0.383933227114987,0.401145492974693),.UNSPECIFIED.)
GEOMETRIC_REPRESENTATION_ITEM()
RATIONAL_B_SPLINE_SURFACE(((0.988246641953811,0.988246641953811,0.988246641953811,
0.986737013496293,0.988139125479961),(0.988246641953811,0.988246641953811,
0.988246641953811,0.986737013496293,0.988139125479961),(0.988246641953811,
0.988246641953811,0.988246641953811,0.986737013496293,0.988139125479961)))
REPRESENTATION_ITEM('')
SURFACE()
);
#240=(
BOUNDED_SURFACE()
B_SPLINE_SURFACE(1,2,((#96680,#96681,#96682),(#96683,#96684,#96685)),
 .UNSPECIFIED.,.F.,.F.,.F.)
B_SPLINE_SURFACE_WITH_KNOTS((2,2),(3,3),(0.,0.289681084359918),(0.331965345783649,
0.349369696259361),.UNSPECIFIED.)
GEOMETRIC_REPRESENTATION_ITEM()
RATIONAL_B_SPLINE_SURFACE(((0.988555124858681,0.99035748704491,0.99513694090229),
(0.988555124858681,0.99035748704491,0.99513694090229)))
REPRESENTATION_ITEM('')
SURFACE()
);
#241=(
BOUNDED_SURFACE()
B_SPLINE_SURFACE(1,2,((#96689,#96690,#96691,#96692,#96693),(#96694,#96695,
#96696,#96697,#96698),(#96699,#96700,#96701,#96702,#96703)),
 .UNSPECIFIED.,.F.,.F.,.F.)
B_SPLINE_SURFACE_WITH_KNOTS((2,1,2),(3,2,3),(-0.00289807040991642,0.,0.290399554026227),
(0.383340713905887,0.383933227114987,0.401145492974693),.UNSPECIFIED.)
GEOMETRIC_REPRESENTATION_ITEM()
RATIONAL_B_SPLINE_SURFACE(((0.988246641953811,0.988246641953811,0.988246641953811,
0.986737013496293,0.988139125479962),(0.988246641953811,0.988246641953811,
0.988246641953811,0.986737013496293,0.988139125479962),(0.988246641953811,
0.988246641953811,0.988246641953811,0.986737013496293,0.988139125479961)))
REPRESENTATION_ITEM('')
SURFACE()
);
#242=(
BOUNDED_SURFACE()
B_SPLINE_SURFACE(1,2,((#96728,#96729,#96730),(#96731,#96732,#96733)),
 .UNSPECIFIED.,.F.,.F.,.F.)
B_SPLINE_SURFACE_WITH_KNOTS((2,2),(3,3),(0.,0.289681084359924),(0.331965345783649,
0.349369696259361),.UNSPECIFIED.)
GEOMETRIC_REPRESENTATION_ITEM()
RATIONAL_B_SPLINE_SURFACE(((0.988555124858681,0.99035748704491,0.99513694090229),
(0.988555124858681,0.99035748704491,0.99513694090229)))
REPRESENTATION_ITEM('')
SURFACE()
);
#243=(
BOUNDED_SURFACE()
B_SPLINE_SURFACE(1,2,((#96737,#96738,#96739,#96740,#96741),(#96742,#96743,
#96744,#96745,#96746),(#96747,#96748,#96749,#96750,#96751)),
 .UNSPECIFIED.,.F.,.F.,.F.)
B_SPLINE_SURFACE_WITH_KNOTS((2,1,2),(3,2,3),(-0.00289807040991638,0.,0.290399554027218),
(0.383340713904892,0.383933227114987,0.401145492974692),.UNSPECIFIED.)
GEOMETRIC_REPRESENTATION_ITEM()
RATIONAL_B_SPLINE_SURFACE(((0.988246641953811,0.988246641953811,0.988246641953811,
0.986737013496293,0.988139125479961),(0.988246641953811,0.988246641953811,
0.988246641953811,0.986737013496293,0.988139125479961),(0.988246641953811,
0.988246641953811,0.988246641953811,0.986737013496293,0.988139125479961)))
REPRESENTATION_ITEM('')
SURFACE()
);
#244=(
BOUNDED_SURFACE()
B_SPLINE_SURFACE(1,2,((#96764,#96765,#96766),(#96767,#96768,#96769)),
 .UNSPECIFIED.,.F.,.F.,.F.)
B_SPLINE_SURFACE_WITH_KNOTS((2,2),(3,3),(0.,0.289681084359914),(0.33196534578365,
0.349369696259362),.UNSPECIFIED.)
GEOMETRIC_REPRESENTATION_ITEM()
RATIONAL_B_SPLINE_SURFACE(((0.988555124858682,0.990357487044911,0.99513694090229),
(0.988555124858682,0.990357487044911,0.99513694090229)))
REPRESENTATION_ITEM('')
SURFACE()
);
#245=(
BOUNDED_SURFACE()
B_SPLINE_SURFACE(1,2,((#96785,#96786,#96787,#96788,#96789),(#96790,#96791,
#96792,#96793,#96794),(#96795,#96796,#96797,#96798,#96799)),
 .UNSPECIFIED.,.F.,.F.,.F.)
B_SPLINE_SURFACE_WITH_KNOTS((2,1,2),(3,2,3),(-0.00289807040991564,0.,0.290399554037147),
(0.383340713894887,0.383933227114985,0.401145492974692),.UNSPECIFIED.)
GEOMETRIC_REPRESENTATION_ITEM()
RATIONAL_B_SPLINE_SURFACE(((0.988246641953811,0.988246641953811,0.988246641953811,
0.986737013496293,0.988139125479961),(0.988246641953811,0.988246641953811,
0.988246641953811,0.986737013496293,0.988139125479961),(0.988246641953811,
0.988246641953811,0.988246641953811,0.986737013496293,0.988139125479961)))
REPRESENTATION_ITEM('')
SURFACE()
);
#246=(
BOUNDED_SURFACE()
B_SPLINE_SURFACE(1,2,((#96824,#96825,#96826),(#96827,#96828,#96829)),
 .UNSPECIFIED.,.F.,.F.,.F.)
B_SPLINE_SURFACE_WITH_KNOTS((2,2),(3,3),(0.,0.289681084359935),(0.33196534578365,
0.349369696259361),.UNSPECIFIED.)
GEOMETRIC_REPRESENTATION_ITEM()
RATIONAL_B_SPLINE_SURFACE(((0.988555124858682,0.990357487044911,0.99513694090229),
(0.988555124858682,0.990357487044911,0.99513694090229)))
REPRESENTATION_ITEM('')
SURFACE()
);
#247=(
BOUNDED_SURFACE()
B_SPLINE_SURFACE(1,2,((#96833,#96834,#96835,#96836,#96837),(#96838,#96839,
#96840,#96841,#96842),(#96843,#96844,#96845,#96846,#96847)),
 .UNSPECIFIED.,.F.,.F.,.F.)
B_SPLINE_SURFACE_WITH_KNOTS((2,1,2),(3,2,3),(-0.00289807040991981,0.,0.29039955402774),
(0.383340713904713,0.383933227114987,0.401145492974693),.UNSPECIFIED.)
GEOMETRIC_REPRESENTATION_ITEM()
RATIONAL_B_SPLINE_SURFACE(((0.988246641953811,0.988246641953811,0.988246641953811,
0.986737013496293,0.988139125479962),(0.988246641953811,0.988246641953811,
0.988246641953811,0.986737013496293,0.988139125479962),(0.988246641953811,
0.988246641953811,0.988246641953811,0.986737013496293,0.988139125479962)))
REPRESENTATION_ITEM('')
SURFACE()
);
#248=(
BOUNDED_SURFACE()
B_SPLINE_SURFACE(1,2,((#96872,#96873,#96874),(#96875,#96876,#96877)),
 .UNSPECIFIED.,.F.,.F.,.F.)
B_SPLINE_SURFACE_WITH_KNOTS((2,2),(3,3),(0.,0.289681084359928),(0.331965345783649,
0.349369696259361),.UNSPECIFIED.)
GEOMETRIC_REPRESENTATION_ITEM()
RATIONAL_B_SPLINE_SURFACE(((0.988555124858681,0.99035748704491,0.99513694090229),
(0.988555124858681,0.99035748704491,0.99513694090229)))
REPRESENTATION_ITEM('')
SURFACE()
);
#249=(
BOUNDED_SURFACE()
B_SPLINE_SURFACE(1,2,((#96881,#96882,#96883,#96884,#96885),(#96886,#96887,
#96888,#96889,#96890),(#96891,#96892,#96893,#96894,#96895)),
 .UNSPECIFIED.,.F.,.F.,.F.)
B_SPLINE_SURFACE_WITH_KNOTS((2,1,2),(3,2,3),(-0.00289807040991899,0.,0.290399554020957),
(0.383340713911414,0.383933227114987,0.401145492974693),.UNSPECIFIED.)
GEOMETRIC_REPRESENTATION_ITEM()
RATIONAL_B_SPLINE_SURFACE(((0.988246641953811,0.988246641953811,0.988246641953811,
0.986737013496293,0.988139125479962),(0.988246641953811,0.988246641953811,
0.988246641953811,0.986737013496293,0.988139125479962),(0.988246641953811,
0.988246641953811,0.988246641953811,0.986737013496293,0.988139125479962)))
REPRESENTATION_ITEM('')
SURFACE()
);
#250=(
BOUNDED_SURFACE()
B_SPLINE_SURFACE(1,2,((#96920,#96921,#96922),(#96923,#96924,#96925)),
 .UNSPECIFIED.,.F.,.F.,.F.)
B_SPLINE_SURFACE_WITH_KNOTS((2,2),(3,3),(0.,0.289681084359927),(0.331965345783649,
0.349369696259361),.UNSPECIFIED.)
GEOMETRIC_REPRESENTATION_ITEM()
RATIONAL_B_SPLINE_SURFACE(((0.988555124858681,0.99035748704491,0.99513694090229),
(0.988555124858681,0.99035748704491,0.99513694090229)))
REPRESENTATION_ITEM('')
SURFACE()
);
#251=(
BOUNDED_SURFACE()
B_SPLINE_SURFACE(1,2,((#96941,#96942,#96943,#96944,#96945),(#96946,#96947,
#96948,#96949,#96950),(#96951,#96952,#96953,#96954,#96955)),
 .UNSPECIFIED.,.F.,.F.,.F.)
B_SPLINE_SURFACE_WITH_KNOTS((2,1,2),(3,2,3),(-0.0028980704099201,0.,0.290399554036522),
(0.383340713895899,0.383933227114987,0.401145492974693),.UNSPECIFIED.)
GEOMETRIC_REPRESENTATION_ITEM()
RATIONAL_B_SPLINE_SURFACE(((0.988246641953811,0.988246641953811,0.988246641953811,
0.986737013496293,0.988139125479962),(0.988246641953811,0.988246641953811,
0.988246641953811,0.986737013496293,0.988139125479962),(0.988246641953811,
0.988246641953811,0.988246641953811,0.986737013496293,0.988139125479962)))
REPRESENTATION_ITEM('')
SURFACE()
);
#252=(
BOUNDED_SURFACE()
B_SPLINE_SURFACE(1,2,((#96958,#96959,#96960,#96961,#96962),(#96963,#96964,
#96965,#96966,#96967)),.UNSPECIFIED.,.F.,.F.,.F.)
B_SPLINE_SURFACE_WITH_KNOTS((2,2),(3,2,3),(0.709593954894314,1.),(0.331470144829386,
0.332069149066804,0.349473499542517),.UNSPECIFIED.)
GEOMETRIC_REPRESENTATION_ITEM()
RATIONAL_B_SPLINE_SURFACE(((0.988576730109495,0.988576730109495,0.988576730109495,
0.990396848309667,0.99519405818099),(0.988576730109495,0.988576730109495,
0.988576730109495,0.990396848309667,0.99519405818099)))
REPRESENTATION_ITEM('')
SURFACE()
);
#253=(
BOUNDED_SURFACE()
B_SPLINE_SURFACE(1,2,((#96978,#96979,#96980),(#96981,#96982,#96983),(#96984,
#96985,#96986)),.UNSPECIFIED.,.F.,.F.,.F.)
B_SPLINE_SURFACE_WITH_KNOTS((2,1,2),(3,3),(0.707422104796139,0.710318915639742,
1.),(0.383830569465724,0.401042835325431),.UNSPECIFIED.)
GEOMETRIC_REPRESENTATION_ITEM()
RATIONAL_B_SPLINE_SURFACE(((0.988264753026337,0.986737758323643,0.988122504062136),
(0.988264753026337,0.986737758323643,0.988122504062136),(0.988264753026337,
0.986737758323643,0.988122504062136)))
REPRESENTATION_ITEM('')
SURFACE()
);
#254=(
BOUNDED_SURFACE()
B_SPLINE_SURFACE(1,2,((#96997,#96998,#96999,#97000,#97001),(#97002,#97003,
#97004,#97005,#97006)),.UNSPECIFIED.,.F.,.F.,.F.)
B_SPLINE_SURFACE_WITH_KNOTS((2,2),(3,2,3),(0.709593954927603,1.),(0.331470144862805,
0.332069149066804,0.349473499542517),.UNSPECIFIED.)
GEOMETRIC_REPRESENTATION_ITEM()
RATIONAL_B_SPLINE_SURFACE(((0.988576730109495,0.988576730109495,0.988576730109495,
0.990396848309667,0.99519405818099),(0.988576730109495,0.988576730109495,
0.988576730109495,0.990396848309667,0.99519405818099)))
REPRESENTATION_ITEM('')
SURFACE()
);
#255=(
BOUNDED_SURFACE()
B_SPLINE_SURFACE(1,2,((#97014,#97015,#97016),(#97017,#97018,#97019),(#97020,
#97021,#97022)),.UNSPECIFIED.,.F.,.F.,.F.)
B_SPLINE_SURFACE_WITH_KNOTS((2,1,2),(3,3),(0.707422104796059,0.710318915639662,
1.),(0.383830569465724,0.401042835325431),.UNSPECIFIED.)
GEOMETRIC_REPRESENTATION_ITEM()
RATIONAL_B_SPLINE_SURFACE(((0.988264753026337,0.986737758323643,0.988122504062136),
(0.988264753026337,0.986737758323643,0.988122504062136),(0.988264753026337,
0.986737758323643,0.988122504062136)))
REPRESENTATION_ITEM('')
SURFACE()
);
#256=(
BOUNDED_SURFACE()
B_SPLINE_SURFACE(1,2,((#97033,#97034,#97035,#97036,#97037),(#97038,#97039,
#97040,#97041,#97042)),.UNSPECIFIED.,.F.,.F.,.F.)
B_SPLINE_SURFACE_WITH_KNOTS((2,2),(3,2,3),(0.70959395491761,1.),(0.33147014485254,
0.332069149066805,0.349473499542517),.UNSPECIFIED.)
GEOMETRIC_REPRESENTATION_ITEM()
RATIONAL_B_SPLINE_SURFACE(((0.988576730109495,0.988576730109495,0.988576730109495,
0.990396848309667,0.99519405818099),(0.988576730109495,0.988576730109495,
0.988576730109495,0.990396848309667,0.99519405818099)))
REPRESENTATION_ITEM('')
SURFACE()
);
#257=(
BOUNDED_SURFACE()
B_SPLINE_SURFACE(1,2,((#97050,#97051,#97052),(#97053,#97054,#97055),(#97056,
#97057,#97058)),.UNSPECIFIED.,.F.,.F.,.F.)
B_SPLINE_SURFACE_WITH_KNOTS((2,1,2),(3,3),(0.707422104796478,0.710318915640077,
1.),(0.383830569465723,0.40104283532543),.UNSPECIFIED.)
GEOMETRIC_REPRESENTATION_ITEM()
RATIONAL_B_SPLINE_SURFACE(((0.988264753026337,0.986737758323643,0.988122504062136),
(0.988264753026337,0.986737758323643,0.988122504062136),(0.988264753026337,
0.986737758323643,0.988122504062136)))
REPRESENTATION_ITEM('')
SURFACE()
);
#258=(
BOUNDED_SURFACE()
B_SPLINE_SURFACE(1,2,((#97069,#97070,#97071,#97072,#97073),(#97074,#97075,
#97076,#97077,#97078)),.UNSPECIFIED.,.F.,.F.,.F.)
B_SPLINE_SURFACE_WITH_KNOTS((2,2),(3,2,3),(0.709593954926867,1.),(0.331470144853475,
0.332069149066805,0.349473499542518),.UNSPECIFIED.)
GEOMETRIC_REPRESENTATION_ITEM()
RATIONAL_B_SPLINE_SURFACE(((0.988576730109495,0.988576730109495,0.988576730109495,
0.990396848309667,0.995194058180991),(0.988576730109495,0.988576730109495,
0.988576730109495,0.990396848309667,0.995194058180991)))
REPRESENTATION_ITEM('')
SURFACE()
);
#259=(
BOUNDED_SURFACE()
B_SPLINE_SURFACE(1,2,((#97086,#97087,#97088),(#97089,#97090,#97091),(#97092,
#97093,#97094)),.UNSPECIFIED.,.F.,.F.,.F.)
B_SPLINE_SURFACE_WITH_KNOTS((2,1,2),(3,3),(0.707422104796401,0.710318915640001,
1.),(0.383830569465724,0.40104283532543),.UNSPECIFIED.)
GEOMETRIC_REPRESENTATION_ITEM()
RATIONAL_B_SPLINE_SURFACE(((0.988264753026337,0.986737758323643,0.988122504062135),
(0.988264753026337,0.986737758323643,0.988122504062135),(0.988264753026337,
0.986737758323643,0.988122504062135)))
REPRESENTATION_ITEM('')
SURFACE()
);
#260=(
BOUNDED_SURFACE()
B_SPLINE_SURFACE(1,2,((#97105,#97106,#97107,#97108,#97109),(#97110,#97111,
#97112,#97113,#97114)),.UNSPECIFIED.,.F.,.F.,.F.)
B_SPLINE_SURFACE_WITH_KNOTS((2,2),(3,2,3),(0.709593954920529,1.),(0.331470144847347,
0.332069149066804,0.349473499542517),.UNSPECIFIED.)
GEOMETRIC_REPRESENTATION_ITEM()
RATIONAL_B_SPLINE_SURFACE(((0.988576730109495,0.988576730109495,0.988576730109495,
0.990396848309667,0.99519405818099),(0.988576730109495,0.988576730109495,
0.988576730109495,0.990396848309667,0.99519405818099)))
REPRESENTATION_ITEM('')
SURFACE()
);
#261=(
BOUNDED_SURFACE()
B_SPLINE_SURFACE(1,2,((#97122,#97123,#97124),(#97125,#97126,#97127),(#97128,
#97129,#97130)),.UNSPECIFIED.,.F.,.F.,.F.)
B_SPLINE_SURFACE_WITH_KNOTS((2,1,2),(3,3),(0.707422104796399,0.710318915639999,
1.),(0.383830569465724,0.401042835325431),.UNSPECIFIED.)
GEOMETRIC_REPRESENTATION_ITEM()
RATIONAL_B_SPLINE_SURFACE(((0.988264753026337,0.986737758323643,0.988122504062135),
(0.988264753026337,0.986737758323643,0.988122504062135),(0.988264753026337,
0.986737758323643,0.988122504062135)))
REPRESENTATION_ITEM('')
SURFACE()
);
#262=(
BOUNDED_SURFACE()
B_SPLINE_SURFACE(1,2,((#97141,#97142,#97143,#97144,#97145),(#97146,#97147,
#97148,#97149,#97150)),.UNSPECIFIED.,.F.,.F.,.F.)
B_SPLINE_SURFACE_WITH_KNOTS((2,2),(3,2,3),(0.709593954913145,1.),(0.331470144839669,
0.332069149066804,0.349473499542517),.UNSPECIFIED.)
GEOMETRIC_REPRESENTATION_ITEM()
RATIONAL_B_SPLINE_SURFACE(((0.988576730109495,0.988576730109495,0.988576730109495,
0.990396848309667,0.99519405818099),(0.988576730109495,0.988576730109495,
0.988576730109495,0.990396848309667,0.99519405818099)))
REPRESENTATION_ITEM('')
SURFACE()
);
#263=(
BOUNDED_SURFACE()
B_SPLINE_SURFACE(1,2,((#97158,#97159,#97160),(#97161,#97162,#97163),(#97164,
#97165,#97166)),.UNSPECIFIED.,.F.,.F.,.F.)
B_SPLINE_SURFACE_WITH_KNOTS((2,1,2),(3,3),(0.707422104796394,0.710318915639994,
1.),(0.383830569465724,0.401042835325431),.UNSPECIFIED.)
GEOMETRIC_REPRESENTATION_ITEM()
RATIONAL_B_SPLINE_SURFACE(((0.988264753026337,0.986737758323643,0.988122504062135),
(0.988264753026337,0.986737758323643,0.988122504062135),(0.988264753026337,
0.986737758323643,0.988122504062135)))
REPRESENTATION_ITEM('')
SURFACE()
);
#264=(
BOUNDED_SURFACE()
B_SPLINE_SURFACE(1,2,((#97177,#97178,#97179,#97180,#97181),(#97182,#97183,
#97184,#97185,#97186)),.UNSPECIFIED.,.F.,.F.,.F.)
B_SPLINE_SURFACE_WITH_KNOTS((2,2),(3,2,3),(0.709593954887389,1.),(0.331470144814559,
0.332069149066804,0.349473499542517),.UNSPECIFIED.)
GEOMETRIC_REPRESENTATION_ITEM()
RATIONAL_B_SPLINE_SURFACE(((0.988576730109495,0.988576730109495,0.988576730109495,
0.990396848309667,0.99519405818099),(0.988576730109495,0.988576730109495,
0.988576730109495,0.990396848309667,0.99519405818099)))
REPRESENTATION_ITEM('')
SURFACE()
);
#265=(
BOUNDED_SURFACE()
B_SPLINE_SURFACE(1,2,((#97194,#97195,#97196),(#97197,#97198,#97199),(#97200,
#97201,#97202)),.UNSPECIFIED.,.F.,.F.,.F.)
B_SPLINE_SURFACE_WITH_KNOTS((2,1,2),(3,3),(0.7074221047964,0.71031891564,
1.),(0.383830569465724,0.401042835325431),.UNSPECIFIED.)
GEOMETRIC_REPRESENTATION_ITEM()
RATIONAL_B_SPLINE_SURFACE(((0.988264753026337,0.986737758323643,0.988122504062136),
(0.988264753026337,0.986737758323643,0.988122504062136),(0.988264753026337,
0.986737758323643,0.988122504062136)))
REPRESENTATION_ITEM('')
SURFACE()
);
#266=(
BOUNDED_SURFACE()
B_SPLINE_SURFACE(1,2,((#97213,#97214,#97215,#97216,#97217),(#97218,#97219,
#97220,#97221,#97222)),.UNSPECIFIED.,.F.,.F.,.F.)
B_SPLINE_SURFACE_WITH_KNOTS((2,2),(3,2,3),(0.709593954900147,1.),(0.331470144834562,
0.332069149066804,0.349473499542517),.UNSPECIFIED.)
GEOMETRIC_REPRESENTATION_ITEM()
RATIONAL_B_SPLINE_SURFACE(((0.988576730109495,0.988576730109495,0.988576730109495,
0.990396848309667,0.99519405818099),(0.988576730109495,0.988576730109495,
0.988576730109495,0.990396848309667,0.99519405818099)))
REPRESENTATION_ITEM('')
SURFACE()
);
#267=(
BOUNDED_SURFACE()
B_SPLINE_SURFACE(1,2,((#97230,#97231,#97232),(#97233,#97234,#97235),(#97236,
#97237,#97238)),.UNSPECIFIED.,.F.,.F.,.F.)
B_SPLINE_SURFACE_WITH_KNOTS((2,1,2),(3,3),(0.70742210479648,0.710318915640079,
1.),(0.383830569465724,0.401042835325431),.UNSPECIFIED.)
GEOMETRIC_REPRESENTATION_ITEM()
RATIONAL_B_SPLINE_SURFACE(((0.988264753026337,0.986737758323643,0.988122504062135),
(0.988264753026337,0.986737758323643,0.988122504062135),(0.988264753026337,
0.986737758323643,0.988122504062135)))
REPRESENTATION_ITEM('')
SURFACE()
);
#268=(
BOUNDED_SURFACE()
B_SPLINE_SURFACE(1,2,((#97249,#97250,#97251,#97252,#97253),(#97254,#97255,
#97256,#97257,#97258)),.UNSPECIFIED.,.F.,.F.,.F.)
B_SPLINE_SURFACE_WITH_KNOTS((2,2),(3,2,3),(0.709593954911915,1.),(0.331470144846543,
0.332069149066804,0.349473499542517),.UNSPECIFIED.)
GEOMETRIC_REPRESENTATION_ITEM()
RATIONAL_B_SPLINE_SURFACE(((0.988576730109495,0.988576730109495,0.988576730109495,
0.990396848309667,0.99519405818099),(0.988576730109495,0.988576730109495,
0.988576730109495,0.990396848309667,0.99519405818099)))
REPRESENTATION_ITEM('')
SURFACE()
);
#269=(
BOUNDED_SURFACE()
B_SPLINE_SURFACE(1,2,((#97266,#97267,#97268),(#97269,#97270,#97271),(#97272,
#97273,#97274)),.UNSPECIFIED.,.F.,.F.,.F.)
B_SPLINE_SURFACE_WITH_KNOTS((2,1,2),(3,3),(0.707422104796394,0.710318915639994,
1.),(0.383830569465724,0.401042835325431),.UNSPECIFIED.)
GEOMETRIC_REPRESENTATION_ITEM()
RATIONAL_B_SPLINE_SURFACE(((0.988264753026337,0.986737758323643,0.988122504062135),
(0.988264753026337,0.986737758323643,0.988122504062135),(0.988264753026337,
0.986737758323643,0.988122504062135)))
REPRESENTATION_ITEM('')
SURFACE()
);
#270=(
BOUNDED_SURFACE()
B_SPLINE_SURFACE(1,2,((#97285,#97286,#97287,#97288,#97289),(#97290,#97291,
#97292,#97293,#97294)),.UNSPECIFIED.,.F.,.F.,.F.)
B_SPLINE_SURFACE_WITH_KNOTS((2,2),(3,2,3),(0.709593954893798,1.),(0.331470144828196,
0.332069149066804,0.349473499542517),.UNSPECIFIED.)
GEOMETRIC_REPRESENTATION_ITEM()
RATIONAL_B_SPLINE_SURFACE(((0.988576730109495,0.988576730109495,0.988576730109495,
0.990396848309667,0.99519405818099),(0.988576730109495,0.988576730109495,
0.988576730109495,0.990396848309667,0.99519405818099)))
REPRESENTATION_ITEM('')
SURFACE()
);
#271=(
BOUNDED_SURFACE()
B_SPLINE_SURFACE(1,2,((#97302,#97303,#97304),(#97305,#97306,#97307),(#97308,
#97309,#97310)),.UNSPECIFIED.,.F.,.F.,.F.)
B_SPLINE_SURFACE_WITH_KNOTS((2,1,2),(3,3),(0.707422104796478,0.710318915640077,
1.),(0.383830569465724,0.401042835325431),.UNSPECIFIED.)
GEOMETRIC_REPRESENTATION_ITEM()
RATIONAL_B_SPLINE_SURFACE(((0.988264753026337,0.986737758323643,0.988122504062136),
(0.988264753026337,0.986737758323643,0.988122504062136),(0.988264753026337,
0.986737758323643,0.988122504062136)))
REPRESENTATION_ITEM('')
SURFACE()
);
#272=(
BOUNDED_SURFACE()
B_SPLINE_SURFACE(1,2,((#97321,#97322,#97323,#97324,#97325),(#97326,#97327,
#97328,#97329,#97330)),.UNSPECIFIED.,.F.,.F.,.F.)
B_SPLINE_SURFACE_WITH_KNOTS((2,2),(3,2,3),(0.709593954913158,1.),(0.331470144847742,
0.332069149066804,0.349473499542517),.UNSPECIFIED.)
GEOMETRIC_REPRESENTATION_ITEM()
RATIONAL_B_SPLINE_SURFACE(((0.988576730109495,0.988576730109495,0.988576730109495,
0.990396848309667,0.99519405818099),(0.988576730109495,0.988576730109495,
0.988576730109495,0.990396848309667,0.99519405818099)))
REPRESENTATION_ITEM('')
SURFACE()
);
#273=(
BOUNDED_SURFACE()
B_SPLINE_SURFACE(1,2,((#97338,#97339,#97340),(#97341,#97342,#97343),(#97344,
#97345,#97346)),.UNSPECIFIED.,.F.,.F.,.F.)
B_SPLINE_SURFACE_WITH_KNOTS((2,1,2),(3,3),(0.707422104796117,0.71031891563972,
1.),(0.383830569465724,0.401042835325431),.UNSPECIFIED.)
GEOMETRIC_REPRESENTATION_ITEM()
RATIONAL_B_SPLINE_SURFACE(((0.988264753026337,0.986737758323643,0.988122504062136),
(0.988264753026337,0.986737758323643,0.988122504062136),(0.988264753026337,
0.986737758323643,0.988122504062136)))
REPRESENTATION_ITEM('')
SURFACE()
);
#274=(
BOUNDED_SURFACE()
B_SPLINE_SURFACE(1,2,((#97357,#97358,#97359,#97360,#97361),(#97362,#97363,
#97364,#97365,#97366)),.UNSPECIFIED.,.F.,.F.,.F.)
B_SPLINE_SURFACE_WITH_KNOTS((2,2),(3,2,3),(0.709593954916007,1.),(0.331470144842851,
0.332069149066804,0.349473499542517),.UNSPECIFIED.)
GEOMETRIC_REPRESENTATION_ITEM()
RATIONAL_B_SPLINE_SURFACE(((0.988576730109495,0.988576730109495,0.988576730109495,
0.990396848309667,0.99519405818099),(0.988576730109495,0.988576730109495,
0.988576730109495,0.990396848309667,0.99519405818099)))
REPRESENTATION_ITEM('')
SURFACE()
);
#275=(
BOUNDED_SURFACE()
B_SPLINE_SURFACE(1,2,((#97374,#97375,#97376),(#97377,#97378,#97379),(#97380,
#97381,#97382)),.UNSPECIFIED.,.F.,.F.,.F.)
B_SPLINE_SURFACE_WITH_KNOTS((2,1,2),(3,3),(0.707422104795055,0.710318915638668,
1.),(0.383830569465724,0.401042835325431),.UNSPECIFIED.)
GEOMETRIC_REPRESENTATION_ITEM()
RATIONAL_B_SPLINE_SURFACE(((0.988264753026337,0.986737758323643,0.988122504062136),
(0.988264753026337,0.986737758323643,0.988122504062136),(0.988264753026337,
0.986737758323643,0.988122504062136)))
REPRESENTATION_ITEM('')
SURFACE()
);
#276=(
BOUNDED_SURFACE()
B_SPLINE_SURFACE(1,2,((#97393,#97394,#97395,#97396,#97397),(#97398,#97399,
#97400,#97401,#97402)),.UNSPECIFIED.,.F.,.F.,.F.)
B_SPLINE_SURFACE_WITH_KNOTS((2,2),(3,2,3),(0.709593954907459,1.),(0.331470144835858,
0.332069149066804,0.349473499542517),.UNSPECIFIED.)
GEOMETRIC_REPRESENTATION_ITEM()
RATIONAL_B_SPLINE_SURFACE(((0.988576730109495,0.988576730109495,0.988576730109495,
0.990396848309667,0.99519405818099),(0.988576730109495,0.988576730109495,
0.988576730109495,0.990396848309667,0.99519405818099)))
REPRESENTATION_ITEM('')
SURFACE()
);
#277=(
BOUNDED_SURFACE()
B_SPLINE_SURFACE(1,2,((#97410,#97411,#97412),(#97413,#97414,#97415),(#97416,
#97417,#97418)),.UNSPECIFIED.,.F.,.F.,.F.)
B_SPLINE_SURFACE_WITH_KNOTS((2,1,2),(3,3),(0.707422104796353,0.710318915639953,
1.),(0.383830569465724,0.401042835325431),.UNSPECIFIED.)
GEOMETRIC_REPRESENTATION_ITEM()
RATIONAL_B_SPLINE_SURFACE(((0.988264753026337,0.986737758323643,0.988122504062136),
(0.988264753026337,0.986737758323643,0.988122504062136),(0.988264753026337,
0.986737758323643,0.988122504062136)))
REPRESENTATION_ITEM('')
SURFACE()
);
#278=(
BOUNDED_SURFACE()
B_SPLINE_SURFACE(1,2,((#97429,#97430,#97431,#97432,#97433),(#97434,#97435,
#97436,#97437,#97438)),.UNSPECIFIED.,.F.,.F.,.F.)
B_SPLINE_SURFACE_WITH_KNOTS((2,2),(3,2,3),(0.709593954923838,1.),(0.331470144850567,
0.332069149066804,0.349473499542517),.UNSPECIFIED.)
GEOMETRIC_REPRESENTATION_ITEM()
RATIONAL_B_SPLINE_SURFACE(((0.988576730109495,0.988576730109495,0.988576730109495,
0.990396848309667,0.99519405818099),(0.988576730109495,0.988576730109495,
0.988576730109495,0.990396848309667,0.99519405818099)))
REPRESENTATION_ITEM('')
SURFACE()
);
#279=(
BOUNDED_SURFACE()
B_SPLINE_SURFACE(1,2,((#97446,#97447,#97448),(#97449,#97450,#97451),(#97452,
#97453,#97454)),.UNSPECIFIED.,.F.,.F.,.F.)
B_SPLINE_SURFACE_WITH_KNOTS((2,1,2),(3,3),(0.707422104796472,0.710318915640071,
1.),(0.383830569465724,0.401042835325431),.UNSPECIFIED.)
GEOMETRIC_REPRESENTATION_ITEM()
RATIONAL_B_SPLINE_SURFACE(((0.988264753026337,0.986737758323643,0.988122504062136),
(0.988264753026337,0.986737758323643,0.988122504062136),(0.988264753026337,
0.986737758323643,0.988122504062136)))
REPRESENTATION_ITEM('')
SURFACE()
);
#280=(
BOUNDED_SURFACE()
B_SPLINE_SURFACE(1,2,((#97462,#97463,#97464,#97465,#97466),(#97467,#97468,
#97469,#97470,#97471)),.UNSPECIFIED.,.F.,.F.,.F.)
B_SPLINE_SURFACE_WITH_KNOTS((2,2),(3,2,3),(0.709961110188848,1.),(0.331837300123762,
0.332069149066804,0.349473499542517),.UNSPECIFIED.)
GEOMETRIC_REPRESENTATION_ITEM()
RATIONAL_B_SPLINE_SURFACE(((0.988576730109495,0.988576730109495,0.988576730109495,
0.990396848309667,0.99519405818099),(0.988576730109495,0.988576730109495,
0.988576730109495,0.990396848309667,0.99519405818099)))
REPRESENTATION_ITEM('')
SURFACE()
);
#281=(
BOUNDED_SURFACE()
B_SPLINE_SURFACE(1,2,((#97473,#97474,#97475),(#97476,#97477,#97478),(#97479,
#97480,#97481)),.UNSPECIFIED.,.F.,.F.,.F.)
B_SPLINE_SURFACE_WITH_KNOTS((2,1,2),(3,3),(0.707422104796241,0.710318915639843,
1.),(0.383830569465724,0.401042835325431),.UNSPECIFIED.)
GEOMETRIC_REPRESENTATION_ITEM()
RATIONAL_B_SPLINE_SURFACE(((0.988264753026337,0.986737758323643,0.988122504062135),
(0.988264753026337,0.986737758323643,0.988122504062135),(0.988264753026337,
0.986737758323643,0.988122504062135)))
REPRESENTATION_ITEM('')
SURFACE()
);
#282=(
BOUNDED_SURFACE()
B_SPLINE_SURFACE(1,2,((#97492,#97493,#97494,#97495,#97496),(#97497,#97498,
#97499,#97500,#97501)),.UNSPECIFIED.,.F.,.F.,.F.)
B_SPLINE_SURFACE_WITH_KNOTS((2,2),(3,2,3),(0.70959395489228,1.),(0.331470144827466,
0.332069149066804,0.349473499542517),.UNSPECIFIED.)
GEOMETRIC_REPRESENTATION_ITEM()
RATIONAL_B_SPLINE_SURFACE(((0.988576730109495,0.988576730109495,0.988576730109495,
0.990396848309667,0.99519405818099),(0.988576730109495,0.988576730109495,
0.988576730109495,0.990396848309667,0.99519405818099)))
REPRESENTATION_ITEM('')
SURFACE()
);
#283=(
BOUNDED_SURFACE()
B_SPLINE_SURFACE(1,2,((#97509,#97510,#97511),(#97512,#97513,#97514),(#97515,
#97516,#97517)),.UNSPECIFIED.,.F.,.F.,.F.)
B_SPLINE_SURFACE_WITH_KNOTS((2,1,2),(3,3),(0.707422104796478,0.710318915640077,
1.),(0.383830569465724,0.401042835325431),.UNSPECIFIED.)
GEOMETRIC_REPRESENTATION_ITEM()
RATIONAL_B_SPLINE_SURFACE(((0.988264753026337,0.986737758323643,0.988122504062136),
(0.988264753026337,0.986737758323643,0.988122504062136),(0.988264753026337,
0.986737758323643,0.988122504062136)))
REPRESENTATION_ITEM('')
SURFACE()
);
#284=(
BOUNDED_SURFACE()
B_SPLINE_SURFACE(1,2,((#97528,#97529,#97530,#97531,#97532),(#97533,#97534,
#97535,#97536,#97537)),.UNSPECIFIED.,.F.,.F.,.F.)
B_SPLINE_SURFACE_WITH_KNOTS((2,2),(3,2,3),(0.709593954915317,1.),(0.33147014485014,
0.332069149066804,0.349473499542517),.UNSPECIFIED.)
GEOMETRIC_REPRESENTATION_ITEM()
RATIONAL_B_SPLINE_SURFACE(((0.988576730109495,0.988576730109495,0.988576730109495,
0.990396848309667,0.99519405818099),(0.988576730109495,0.988576730109495,
0.988576730109495,0.990396848309667,0.99519405818099)))
REPRESENTATION_ITEM('')
SURFACE()
);
#285=(
BOUNDED_SURFACE()
B_SPLINE_SURFACE(1,2,((#97545,#97546,#97547),(#97548,#97549,#97550),(#97551,
#97552,#97553)),.UNSPECIFIED.,.F.,.F.,.F.)
B_SPLINE_SURFACE_WITH_KNOTS((2,1,2),(3,3),(0.707422104796476,0.710318915640075,
1.),(0.383830569465724,0.401042835325431),.UNSPECIFIED.)
GEOMETRIC_REPRESENTATION_ITEM()
RATIONAL_B_SPLINE_SURFACE(((0.988264753026337,0.986737758323643,0.988122504062135),
(0.988264753026337,0.986737758323643,0.988122504062135),(0.988264753026337,
0.986737758323643,0.988122504062135)))
REPRESENTATION_ITEM('')
SURFACE()
);
#286=(
BOUNDED_SURFACE()
B_SPLINE_SURFACE(1,2,((#97564,#97565,#97566,#97567,#97568),(#97569,#97570,
#97571,#97572,#97573)),.UNSPECIFIED.,.F.,.F.,.F.)
B_SPLINE_SURFACE_WITH_KNOTS((2,2),(3,2,3),(0.70959395491621,1.),(0.331470144850383,
0.332069149066804,0.349473499542517),.UNSPECIFIED.)
GEOMETRIC_REPRESENTATION_ITEM()
RATIONAL_B_SPLINE_SURFACE(((0.988576730109495,0.988576730109495,0.988576730109495,
0.990396848309667,0.99519405818099),(0.988576730109495,0.988576730109495,
0.988576730109495,0.990396848309667,0.99519405818099)))
REPRESENTATION_ITEM('')
SURFACE()
);
#287=(
BOUNDED_SURFACE()
B_SPLINE_SURFACE(1,2,((#97581,#97582,#97583),(#97584,#97585,#97586),(#97587,
#97588,#97589)),.UNSPECIFIED.,.F.,.F.,.F.)
B_SPLINE_SURFACE_WITH_KNOTS((2,1,2),(3,3),(0.707422104796473,0.710318915640072,
1.),(0.383830569465724,0.401042835325431),.UNSPECIFIED.)
GEOMETRIC_REPRESENTATION_ITEM()
RATIONAL_B_SPLINE_SURFACE(((0.988264753026337,0.986737758323643,0.988122504062135),
(0.988264753026337,0.986737758323643,0.988122504062135),(0.988264753026337,
0.986737758323643,0.988122504062135)))
REPRESENTATION_ITEM('')
SURFACE()
);
#288=(
BOUNDED_SURFACE()
B_SPLINE_SURFACE(1,2,((#97600,#97601,#97602,#97603,#97604),(#97605,#97606,
#97607,#97608,#97609)),.UNSPECIFIED.,.F.,.F.,.F.)
B_SPLINE_SURFACE_WITH_KNOTS((2,2),(3,2,3),(0.709593954915993,1.),(0.331470144842909,
0.332069149066804,0.349473499542517),.UNSPECIFIED.)
GEOMETRIC_REPRESENTATION_ITEM()
RATIONAL_B_SPLINE_SURFACE(((0.988576730109495,0.988576730109495,0.988576730109495,
0.990396848309667,0.99519405818099),(0.988576730109495,0.988576730109495,
0.988576730109495,0.990396848309667,0.99519405818099)))
REPRESENTATION_ITEM('')
SURFACE()
);
#289=(
BOUNDED_SURFACE()
B_SPLINE_SURFACE(1,2,((#97617,#97618,#97619),(#97620,#97621,#97622),(#97623,
#97624,#97625)),.UNSPECIFIED.,.F.,.F.,.F.)
B_SPLINE_SURFACE_WITH_KNOTS((2,1,2),(3,3),(0.707422104796323,0.710318915639924,
1.),(0.383830569465724,0.401042835325431),.UNSPECIFIED.)
GEOMETRIC_REPRESENTATION_ITEM()
RATIONAL_B_SPLINE_SURFACE(((0.988264753026337,0.986737758323643,0.988122504062136),
(0.988264753026337,0.986737758323643,0.988122504062136),(0.988264753026337,
0.986737758323643,0.988122504062136)))
REPRESENTATION_ITEM('')
SURFACE()
);
#290=(
BOUNDED_SURFACE()
B_SPLINE_SURFACE(1,2,((#97636,#97637,#97638,#97639,#97640),(#97641,#97642,
#97643,#97644,#97645)),.UNSPECIFIED.,.F.,.F.,.F.)
B_SPLINE_SURFACE_WITH_KNOTS((2,2),(3,2,3),(0.7095939549075,1.),(0.331470144834758,
0.332069149066804,0.349473499542517),.UNSPECIFIED.)
GEOMETRIC_REPRESENTATION_ITEM()
RATIONAL_B_SPLINE_SURFACE(((0.988576730109495,0.988576730109495,0.988576730109495,
0.990396848309667,0.99519405818099),(0.988576730109495,0.988576730109495,
0.988576730109495,0.990396848309667,0.99519405818099)))
REPRESENTATION_ITEM('')
SURFACE()
);
#291=(
BOUNDED_SURFACE()
B_SPLINE_SURFACE(1,2,((#97653,#97654,#97655),(#97656,#97657,#97658),(#97659,
#97660,#97661)),.UNSPECIFIED.,.F.,.F.,.F.)
B_SPLINE_SURFACE_WITH_KNOTS((2,1,2),(3,3),(0.707422104796278,0.710318915639879,
1.),(0.383830569465724,0.401042835325431),.UNSPECIFIED.)
GEOMETRIC_REPRESENTATION_ITEM()
RATIONAL_B_SPLINE_SURFACE(((0.988264753026337,0.986737758323643,0.988122504062136),
(0.988264753026337,0.986737758323643,0.988122504062136),(0.988264753026337,
0.986737758323643,0.988122504062136)))
REPRESENTATION_ITEM('')
SURFACE()
);
#292=(
BOUNDED_SURFACE()
B_SPLINE_SURFACE(1,2,((#97672,#97673,#97674,#97675,#97676),(#97677,#97678,
#97679,#97680,#97681)),.UNSPECIFIED.,.F.,.F.,.F.)
B_SPLINE_SURFACE_WITH_KNOTS((2,2),(3,2,3),(0.709593954908083,1.),(0.331470144835444,
0.332069149066804,0.349473499542517),.UNSPECIFIED.)
GEOMETRIC_REPRESENTATION_ITEM()
RATIONAL_B_SPLINE_SURFACE(((0.988576730109495,0.988576730109495,0.988576730109495,
0.990396848309667,0.99519405818099),(0.988576730109495,0.988576730109495,
0.988576730109495,0.990396848309667,0.99519405818099)))
REPRESENTATION_ITEM('')
SURFACE()
);
#293=(
BOUNDED_SURFACE()
B_SPLINE_SURFACE(1,2,((#97689,#97690,#97691),(#97692,#97693,#97694),(#97695,
#97696,#97697)),.UNSPECIFIED.,.F.,.F.,.F.)
B_SPLINE_SURFACE_WITH_KNOTS((2,1,2),(3,3),(0.707422104795113,0.710318915638726,
1.),(0.383830569465724,0.401042835325439),.UNSPECIFIED.)
GEOMETRIC_REPRESENTATION_ITEM()
RATIONAL_B_SPLINE_SURFACE(((0.988264753026337,0.986737758323642,0.988122504062137),
(0.988264753026337,0.986737758323642,0.988122504062137),(0.988264753026337,
0.986737758323642,0.988122504062137)))
REPRESENTATION_ITEM('')
SURFACE()
);
#294=(
BOUNDED_SURFACE()
B_SPLINE_SURFACE(1,2,((#97708,#97709,#97710,#97711,#97712),(#97713,#97714,
#97715,#97716,#97717)),.UNSPECIFIED.,.F.,.F.,.F.)
B_SPLINE_SURFACE_WITH_KNOTS((2,2),(3,2,3),(0.709593954917731,1.),(0.331470144846068,
0.332069149066804,0.349473499542517),.UNSPECIFIED.)
GEOMETRIC_REPRESENTATION_ITEM()
RATIONAL_B_SPLINE_SURFACE(((0.988576730109495,0.988576730109495,0.988576730109495,
0.990396848309667,0.99519405818099),(0.988576730109495,0.988576730109495,
0.988576730109495,0.990396848309667,0.99519405818099)))
REPRESENTATION_ITEM('')
SURFACE()
);
#295=(
BOUNDED_SURFACE()
B_SPLINE_SURFACE(1,2,((#97725,#97726,#97727),(#97728,#97729,#97730),(#97731,
#97732,#97733)),.UNSPECIFIED.,.F.,.F.,.F.)
B_SPLINE_SURFACE_WITH_KNOTS((2,1,2),(3,3),(0.707422104795338,0.710318915638948,
1.),(0.383830569465724,0.401042835325431),.UNSPECIFIED.)
GEOMETRIC_REPRESENTATION_ITEM()
RATIONAL_B_SPLINE_SURFACE(((0.988264753026337,0.986737758323643,0.988122504062136),
(0.988264753026337,0.986737758323643,0.988122504062136),(0.988264753026337,
0.986737758323643,0.988122504062136)))
REPRESENTATION_ITEM('')
SURFACE()
);
#296=(
BOUNDED_SURFACE()
B_SPLINE_SURFACE(1,2,((#97744,#97745,#97746,#97747,#97748),(#97749,#97750,
#97751,#97752,#97753)),.UNSPECIFIED.,.F.,.F.,.F.)
B_SPLINE_SURFACE_WITH_KNOTS((2,2),(3,2,3),(0.709593954917719,1.),(0.331470144853412,
0.332069149066804,0.349473499542517),.UNSPECIFIED.)
GEOMETRIC_REPRESENTATION_ITEM()
RATIONAL_B_SPLINE_SURFACE(((0.988576730109495,0.988576730109495,0.988576730109495,
0.990396848309667,0.99519405818099),(0.988576730109495,0.988576730109495,
0.988576730109495,0.990396848309667,0.99519405818099)))
REPRESENTATION_ITEM('')
SURFACE()
);
#297=(
BOUNDED_SURFACE()
B_SPLINE_SURFACE(1,2,((#97761,#97762,#97763),(#97764,#97765,#97766),(#97767,
#97768,#97769)),.UNSPECIFIED.,.F.,.F.,.F.)
B_SPLINE_SURFACE_WITH_KNOTS((2,1,2),(3,3),(0.707422104795584,0.710318915639192,
1.),(0.383830569465714,0.401042835325431),.UNSPECIFIED.)
GEOMETRIC_REPRESENTATION_ITEM()
RATIONAL_B_SPLINE_SURFACE(((0.988264753026339,0.986737758323642,0.988122504062136),
(0.988264753026339,0.986737758323642,0.988122504062136),(0.988264753026339,
0.986737758323642,0.988122504062136)))
REPRESENTATION_ITEM('')
SURFACE()
);
#298=(
BOUNDED_SURFACE()
B_SPLINE_SURFACE(1,2,((#97780,#97781,#97782,#97783,#97784),(#97785,#97786,
#97787,#97788,#97789)),.UNSPECIFIED.,.F.,.F.,.F.)
B_SPLINE_SURFACE_WITH_KNOTS((2,2),(3,2,3),(0.709593954893256,1.),(0.331470144829105,
0.332069149066804,0.349473499542517),.UNSPECIFIED.)
GEOMETRIC_REPRESENTATION_ITEM()
RATIONAL_B_SPLINE_SURFACE(((0.988576730109495,0.988576730109495,0.988576730109495,
0.990396848309667,0.99519405818099),(0.988576730109495,0.988576730109495,
0.988576730109495,0.990396848309667,0.99519405818099)))
REPRESENTATION_ITEM('')
SURFACE()
);
#299=(
BOUNDED_SURFACE()
B_SPLINE_SURFACE(1,2,((#97797,#97798,#97799),(#97800,#97801,#97802),(#97803,
#97804,#97805)),.UNSPECIFIED.,.F.,.F.,.F.)
B_SPLINE_SURFACE_WITH_KNOTS((2,1,2),(3,3),(0.707422104795713,0.71031891563932,
1.),(0.383830569465724,0.401042835325432),.UNSPECIFIED.)
GEOMETRIC_REPRESENTATION_ITEM()
RATIONAL_B_SPLINE_SURFACE(((0.988264753026337,0.986737758323643,0.988122504062136),
(0.988264753026337,0.986737758323643,0.988122504062136),(0.988264753026337,
0.986737758323643,0.988122504062136)))
REPRESENTATION_ITEM('')
SURFACE()
);
#300=(
BOUNDED_SURFACE()
B_SPLINE_SURFACE(1,2,((#97816,#97817,#97818,#97819,#97820),(#97821,#97822,
#97823,#97824,#97825)),.UNSPECIFIED.,.F.,.F.,.F.)
B_SPLINE_SURFACE_WITH_KNOTS((2,2),(3,2,3),(0.709593954897723,1.),(0.331470144833009,
0.332069149066804,0.349473499542517),.UNSPECIFIED.)
GEOMETRIC_REPRESENTATION_ITEM()
RATIONAL_B_SPLINE_SURFACE(((0.988576730109495,0.988576730109495,0.988576730109495,
0.990396848309667,0.99519405818099),(0.988576730109495,0.988576730109495,
0.988576730109495,0.990396848309667,0.99519405818099)))
REPRESENTATION_ITEM('')
SURFACE()
);
#301=(
BOUNDED_SURFACE()
B_SPLINE_SURFACE(1,2,((#97833,#97834,#97835),(#97836,#97837,#97838),(#97839,
#97840,#97841)),.UNSPECIFIED.,.F.,.F.,.F.)
B_SPLINE_SURFACE_WITH_KNOTS((2,1,2),(3,3),(0.707422104795225,0.710318915638837,
1.),(0.383830569465724,0.401042835325431),.UNSPECIFIED.)
GEOMETRIC_REPRESENTATION_ITEM()
RATIONAL_B_SPLINE_SURFACE(((0.988264753026337,0.986737758323643,0.988122504062136),
(0.988264753026337,0.986737758323643,0.988122504062136),(0.988264753026337,
0.986737758323643,0.988122504062136)))
REPRESENTATION_ITEM('')
SURFACE()
);
#302=(
BOUNDED_SURFACE()
B_SPLINE_SURFACE(1,2,((#97852,#97853,#97854,#97855,#97856),(#97857,#97858,
#97859,#97860,#97861)),.UNSPECIFIED.,.F.,.F.,.F.)
B_SPLINE_SURFACE_WITH_KNOTS((2,2),(3,2,3),(0.709593954907626,1.),(0.331470144835888,
0.332069149066804,0.349473499542517),.UNSPECIFIED.)
GEOMETRIC_REPRESENTATION_ITEM()
RATIONAL_B_SPLINE_SURFACE(((0.988576730109495,0.988576730109495,0.988576730109495,
0.990396848309667,0.99519405818099),(0.988576730109495,0.988576730109495,
0.988576730109495,0.990396848309667,0.99519405818099)))
REPRESENTATION_ITEM('')
SURFACE()
);
#303=(
BOUNDED_SURFACE()
B_SPLINE_SURFACE(1,2,((#97869,#97870,#97871),(#97872,#97873,#97874),(#97875,
#97876,#97877)),.UNSPECIFIED.,.F.,.F.,.F.)
B_SPLINE_SURFACE_WITH_KNOTS((2,1,2),(3,3),(0.707422104795377,0.710318915638987,
1.),(0.383830569465724,0.401042835325434),.UNSPECIFIED.)
GEOMETRIC_REPRESENTATION_ITEM()
RATIONAL_B_SPLINE_SURFACE(((0.988264753026337,0.986737758323643,0.988122504062136),
(0.988264753026337,0.986737758323643,0.988122504062136),(0.988264753026337,
0.986737758323643,0.988122504062136)))
REPRESENTATION_ITEM('')
SURFACE()
);
#304=(
BOUNDED_SURFACE()
B_SPLINE_SURFACE(1,2,((#97888,#97889,#97890,#97891,#97892),(#97893,#97894,
#97895,#97896,#97897)),.UNSPECIFIED.,.F.,.F.,.F.)
B_SPLINE_SURFACE_WITH_KNOTS((2,2),(3,2,3),(0.709593954929305,1.),(0.331470144857018,
0.332069149066804,0.349473499542517),.UNSPECIFIED.)
GEOMETRIC_REPRESENTATION_ITEM()
RATIONAL_B_SPLINE_SURFACE(((0.988576730109495,0.988576730109495,0.988576730109495,
0.990396848309667,0.99519405818099),(0.988576730109495,0.988576730109495,
0.988576730109495,0.990396848309667,0.99519405818099)))
REPRESENTATION_ITEM('')
SURFACE()
);
#305=(
BOUNDED_SURFACE()
B_SPLINE_SURFACE(1,2,((#97905,#97906,#97907),(#97908,#97909,#97910),(#97911,
#97912,#97913)),.UNSPECIFIED.,.F.,.F.,.F.)
B_SPLINE_SURFACE_WITH_KNOTS((2,1,2),(3,3),(0.707422104795348,0.710318915638958,
1.),(0.383830569465724,0.401042835325432),.UNSPECIFIED.)
GEOMETRIC_REPRESENTATION_ITEM()
RATIONAL_B_SPLINE_SURFACE(((0.988264753026337,0.986737758323643,0.988122504062136),
(0.988264753026337,0.986737758323643,0.988122504062136),(0.988264753026337,
0.986737758323643,0.988122504062136)))
REPRESENTATION_ITEM('')
SURFACE()
);
#306=(
BOUNDED_SURFACE()
B_SPLINE_SURFACE(1,2,((#97924,#97925,#97926,#97927,#97928),(#97929,#97930,
#97931,#97932,#97933)),.UNSPECIFIED.,.F.,.F.,.F.)
B_SPLINE_SURFACE_WITH_KNOTS((2,2),(3,2,3),(0.709593954903671,1.),(0.331470144831592,
0.332069149066804,0.349473499542517),.UNSPECIFIED.)
GEOMETRIC_REPRESENTATION_ITEM()
RATIONAL_B_SPLINE_SURFACE(((0.988576730109495,0.988576730109495,0.988576730109495,
0.990396848309667,0.99519405818099),(0.988576730109495,0.988576730109495,
0.988576730109495,0.990396848309667,0.99519405818099)))
REPRESENTATION_ITEM('')
SURFACE()
);
#307=(
BOUNDED_SURFACE()
B_SPLINE_SURFACE(1,2,((#97941,#97942,#97943),(#97944,#97945,#97946),(#97947,
#97948,#97949)),.UNSPECIFIED.,.F.,.F.,.F.)
B_SPLINE_SURFACE_WITH_KNOTS((2,1,2),(3,3),(0.707422104795167,0.710318915638779,
1.),(0.383830569465724,0.401042835325431),.UNSPECIFIED.)
GEOMETRIC_REPRESENTATION_ITEM()
RATIONAL_B_SPLINE_SURFACE(((0.988264753026337,0.986737758323643,0.988122504062136),
(0.988264753026337,0.986737758323643,0.988122504062136),(0.988264753026337,
0.986737758323643,0.988122504062136)))
REPRESENTATION_ITEM('')
SURFACE()
);
#308=(
BOUNDED_SURFACE()
B_SPLINE_SURFACE(1,2,((#97960,#97961,#97962,#97963,#97964),(#97965,#97966,
#97967,#97968,#97969)),.UNSPECIFIED.,.F.,.F.,.F.)
B_SPLINE_SURFACE_WITH_KNOTS((2,2),(3,2,3),(0.709593954891873,1.),(0.33147014482002,
0.332069149066804,0.349473499542517),.UNSPECIFIED.)
GEOMETRIC_REPRESENTATION_ITEM()
RATIONAL_B_SPLINE_SURFACE(((0.988576730109495,0.988576730109495,0.988576730109495,
0.990396848309667,0.99519405818099),(0.988576730109495,0.988576730109495,
0.988576730109495,0.990396848309667,0.99519405818099)))
REPRESENTATION_ITEM('')
SURFACE()
);
#309=(
BOUNDED_SURFACE()
B_SPLINE_SURFACE(1,2,((#97983,#97984,#97985),(#97986,#97987,#97988),(#97989,
#97990,#97991)),.UNSPECIFIED.,.F.,.F.,.F.)
B_SPLINE_SURFACE_WITH_KNOTS((2,1,2),(3,3),(0.707422104796028,0.710318915639632,
1.),(0.383830569465724,0.401042835325431),.UNSPECIFIED.)
GEOMETRIC_REPRESENTATION_ITEM()
RATIONAL_B_SPLINE_SURFACE(((0.988264753026337,0.986737758323643,0.988122504062135),
(0.988264753026337,0.986737758323643,0.988122504062135),(0.988264753026337,
0.986737758323643,0.988122504062135)))
REPRESENTATION_ITEM('')
SURFACE()
);
#310=(
BOUNDED_SURFACE()
B_SPLINE_SURFACE(1,2,((#97993,#97994,#97995),(#97996,#97997,#97998)),
 .UNSPECIFIED.,.F.,.F.,.F.)
B_SPLINE_SURFACE_WITH_KNOTS((2,2),(3,3),(0.710318915639632,1.),(0.366717817351065,
0.383933227114987),.UNSPECIFIED.)
GEOMETRIC_REPRESENTATION_ITEM()
RATIONAL_B_SPLINE_SURFACE(((0.994179254576316,0.989756546152321,0.988246641953811),
(0.994179254576316,0.989756546152321,0.988246641953811)))
REPRESENTATION_ITEM('')
SURFACE()
);
#311=(
BOUNDED_SURFACE()
B_SPLINE_SURFACE(1,2,((#98007,#98008,#98009,#98010,#98011,#98012,#98013),
(#98014,#98015,#98016,#98017,#98018,#98019,#98020)),.UNSPECIFIED.,.F.,.F.,
 .F.)
B_SPLINE_SURFACE_WITH_KNOTS((2,2),(3,2,2,3),(0.710192959007138,1.),(0.349194141236593,
0.349369696259361,0.357142857142857,0.366925198536205),.UNSPECIFIED.)
GEOMETRIC_REPRESENTATION_ITEM()
RATIONAL_B_SPLINE_SURFACE(((0.99513694090229,0.99513694090229,0.99513694090229,
0.997271548787858,1.,0.99656630788526,0.994073123128689),(0.99513694090229,
0.99513694090229,0.99513694090229,0.997271548787858,1.,0.99656630788526,
0.994073123128689)))
REPRESENTATION_ITEM('')
SURFACE()
);
#312=(
BOUNDED_SURFACE()
B_SPLINE_SURFACE(1,2,((#98033,#98034,#98035),(#98036,#98037,#98038)),
 .UNSPECIFIED.,.F.,.F.,.F.)
B_SPLINE_SURFACE_WITH_KNOTS((2,2),(3,3),(0.710318915638778,1.),(0.366717817351071,
0.383933227114987),.UNSPECIFIED.)
GEOMETRIC_REPRESENTATION_ITEM()
RATIONAL_B_SPLINE_SURFACE(((0.994179254576313,0.989756546152321,0.988246641953811),
(0.994179254576313,0.989756546152321,0.988246641953811)))
REPRESENTATION_ITEM('')
SURFACE()
);
#313=(
BOUNDED_SURFACE()
B_SPLINE_SURFACE(1,2,((#98040,#98041,#98042,#98043,#98044,#98045,#98046),
(#98047,#98048,#98049,#98050,#98051,#98052,#98053)),.UNSPECIFIED.,.F.,.F.,
 .F.)
B_SPLINE_SURFACE_WITH_KNOTS((2,2),(3,2,2,3),(0.710192959007322,1.),(0.349194141236593,
0.349369696259361,0.357142857142857,0.366925198536205),.UNSPECIFIED.)
GEOMETRIC_REPRESENTATION_ITEM()
RATIONAL_B_SPLINE_SURFACE(((0.99513694090229,0.99513694090229,0.99513694090229,
0.997271548787858,1.,0.99656630788526,0.99407312312869),(0.99513694090229,
0.99513694090229,0.99513694090229,0.997271548787858,1.,0.99656630788526,
0.99407312312869)))
REPRESENTATION_ITEM('')
SURFACE()
);
#314=(
BOUNDED_SURFACE()
B_SPLINE_SURFACE(1,2,((#98066,#98067,#98068),(#98069,#98070,#98071)),
 .UNSPECIFIED.,.F.,.F.,.F.)
B_SPLINE_SURFACE_WITH_KNOTS((2,2),(3,3),(0.710318915638965,1.),(0.366717817351071,
0.383933227115084),.UNSPECIFIED.)
GEOMETRIC_REPRESENTATION_ITEM()
RATIONAL_B_SPLINE_SURFACE(((0.994179254576314,0.989756546152296,0.988246641953794),
(0.994179254576314,0.989756546152296,0.988246641953794)))
REPRESENTATION_ITEM('')
SURFACE()
);
#315=(
BOUNDED_SURFACE()
B_SPLINE_SURFACE(1,2,((#98073,#98074,#98075,#98076,#98077,#98078,#98079),
(#98080,#98081,#98082,#98083,#98084,#98085,#98086)),.UNSPECIFIED.,.F.,.F.,
 .F.)
B_SPLINE_SURFACE_WITH_KNOTS((2,2),(3,2,2,3),(0.710192959007349,1.),(0.349194141236593,
0.349369696259361,0.357142857142857,0.366925198536205),.UNSPECIFIED.)
GEOMETRIC_REPRESENTATION_ITEM()
RATIONAL_B_SPLINE_SURFACE(((0.99513694090229,0.99513694090229,0.99513694090229,
0.997271548787858,1.,0.99656630788526,0.994073123128689),(0.99513694090229,
0.99513694090229,0.99513694090229,0.997271548787858,1.,0.99656630788526,
0.994073123128689)))
REPRESENTATION_ITEM('')
SURFACE()
);
#316=(
BOUNDED_SURFACE()
B_SPLINE_SURFACE(1,2,((#98099,#98100,#98101),(#98102,#98103,#98104)),
 .UNSPECIFIED.,.F.,.F.,.F.)
B_SPLINE_SURFACE_WITH_KNOTS((2,2),(3,3),(0.710318915638993,1.),(0.366717817351071,
0.383933227114987),.UNSPECIFIED.)
GEOMETRIC_REPRESENTATION_ITEM()
RATIONAL_B_SPLINE_SURFACE(((0.994179254576313,0.989756546152321,0.988246641953811),
(0.994179254576313,0.989756546152321,0.988246641953811)))
REPRESENTATION_ITEM('')
SURFACE()
);
#317=(
BOUNDED_SURFACE()
B_SPLINE_SURFACE(1,2,((#98106,#98107,#98108,#98109,#98110,#98111,#98112),
(#98113,#98114,#98115,#98116,#98117,#98118,#98119)),.UNSPECIFIED.,.F.,.F.,
 .F.)
B_SPLINE_SURFACE_WITH_KNOTS((2,2),(3,2,2,3),(0.710192959007199,1.),(0.349194141236593,
0.349369696259361,0.357142857142857,0.366925198536205),.UNSPECIFIED.)
GEOMETRIC_REPRESENTATION_ITEM()
RATIONAL_B_SPLINE_SURFACE(((0.99513694090229,0.99513694090229,0.99513694090229,
0.997271548787858,1.,0.99656630788526,0.994073123128689),(0.99513694090229,
0.99513694090229,0.99513694090229,0.997271548787858,1.,0.99656630788526,
0.994073123128689)))
REPRESENTATION_ITEM('')
SURFACE()
);
#318=(
BOUNDED_SURFACE()
B_SPLINE_SURFACE(1,2,((#98132,#98133,#98134),(#98135,#98136,#98137)),
 .UNSPECIFIED.,.F.,.F.,.F.)
B_SPLINE_SURFACE_WITH_KNOTS((2,2),(3,3),(0.710318915638838,1.),(0.366717817351071,
0.383933227114987),.UNSPECIFIED.)
GEOMETRIC_REPRESENTATION_ITEM()
RATIONAL_B_SPLINE_SURFACE(((0.994179254576313,0.98975654615232,0.988246641953811),
(0.994179254576313,0.989756546152321,0.988246641953811)))
REPRESENTATION_ITEM('')
SURFACE()
);
#319=(
BOUNDED_SURFACE()
B_SPLINE_SURFACE(1,2,((#98139,#98140,#98141,#98142,#98143,#98144,#98145),
(#98146,#98147,#98148,#98149,#98150,#98151,#98152)),.UNSPECIFIED.,.F.,.F.,
 .F.)
B_SPLINE_SURFACE_WITH_KNOTS((2,2),(3,2,2,3),(0.710192959007675,1.),(0.349194141236593,
0.349369696259361,0.357142857142857,0.366925198536205),.UNSPECIFIED.)
GEOMETRIC_REPRESENTATION_ITEM()
RATIONAL_B_SPLINE_SURFACE(((0.99513694090229,0.99513694090229,0.99513694090229,
0.997271548787858,1.,0.99656630788526,0.99407312312869),(0.99513694090229,
0.99513694090229,0.99513694090229,0.997271548787858,1.,0.99656630788526,
0.99407312312869)))
REPRESENTATION_ITEM('')
SURFACE()
);
#320=(
BOUNDED_SURFACE()
B_SPLINE_SURFACE(1,2,((#98165,#98166,#98167),(#98168,#98169,#98170)),
 .UNSPECIFIED.,.F.,.F.,.F.)
B_SPLINE_SURFACE_WITH_KNOTS((2,2),(3,3),(0.710318915639317,1.),(0.366717817351071,
0.383933227114987),.UNSPECIFIED.)
GEOMETRIC_REPRESENTATION_ITEM()
RATIONAL_B_SPLINE_SURFACE(((0.994179254576314,0.989756546152321,0.988246641953811),
(0.994179254576314,0.989756546152321,0.988246641953811)))
REPRESENTATION_ITEM('')
SURFACE()
);
#321=(
BOUNDED_SURFACE()
B_SPLINE_SURFACE(1,2,((#98172,#98173,#98174,#98175,#98176,#98177,#98178),
(#98179,#98180,#98181,#98182,#98183,#98184,#98185)),.UNSPECIFIED.,.F.,.F.,
 .F.)
B_SPLINE_SURFACE_WITH_KNOTS((2,2),(3,2,2,3),(0.71019295900755,1.),(0.349194141236582,
0.349369696259351,0.357142857142857,0.366925198536205),.UNSPECIFIED.)
GEOMETRIC_REPRESENTATION_ITEM()
RATIONAL_B_SPLINE_SURFACE(((0.995136940902284,0.995136940902284,0.995136940902284,
0.997271548787855,1.,0.99656630788526,0.99407312312869),(0.995136940902284,
0.995136940902284,0.995136940902284,0.997271548787855,1.,0.99656630788526,
0.99407312312869)))
REPRESENTATION_ITEM('')
SURFACE()
);
#322=(
BOUNDED_SURFACE()
B_SPLINE_SURFACE(1,2,((#98198,#98199,#98200),(#98201,#98202,#98203)),
 .UNSPECIFIED.,.F.,.F.,.F.)
B_SPLINE_SURFACE_WITH_KNOTS((2,2),(3,3),(0.710318915639189,1.),(0.366717817351071,
0.383933227114987),.UNSPECIFIED.)
GEOMETRIC_REPRESENTATION_ITEM()
RATIONAL_B_SPLINE_SURFACE(((0.994179254576313,0.98975654615232,0.988246641953811),
(0.994179254576313,0.989756546152321,0.988246641953811)))
REPRESENTATION_ITEM('')
SURFACE()
);
#323=(
BOUNDED_SURFACE()
B_SPLINE_SURFACE(1,2,((#98205,#98206,#98207,#98208,#98209,#98210,#98211),
(#98212,#98213,#98214,#98215,#98216,#98217,#98218)),.UNSPECIFIED.,.F.,.F.,
 .F.)
B_SPLINE_SURFACE_WITH_KNOTS((2,2),(3,2,2,3),(0.71019295900731,1.),(0.349194141236593,
0.349369696259361,0.357142857142857,0.366925198536205),.UNSPECIFIED.)
GEOMETRIC_REPRESENTATION_ITEM()
RATIONAL_B_SPLINE_SURFACE(((0.99513694090229,0.99513694090229,0.99513694090229,
0.997271548787858,1.,0.99656630788526,0.99407312312869),(0.99513694090229,
0.99513694090229,0.99513694090229,0.997271548787858,1.,0.99656630788526,
0.99407312312869)))
REPRESENTATION_ITEM('')
SURFACE()
);
#324=(
BOUNDED_SURFACE()
B_SPLINE_SURFACE(1,2,((#98231,#98232,#98233),(#98234,#98235,#98236)),
 .UNSPECIFIED.,.F.,.F.,.F.)
B_SPLINE_SURFACE_WITH_KNOTS((2,2),(3,3),(0.71031891563895,1.),(0.366717817351071,
0.383933227114987),.UNSPECIFIED.)
GEOMETRIC_REPRESENTATION_ITEM()
RATIONAL_B_SPLINE_SURFACE(((0.994179254576313,0.98975654615232,0.988246641953811),
(0.994179254576313,0.989756546152321,0.988246641953811)))
REPRESENTATION_ITEM('')
SURFACE()
);
#325=(
BOUNDED_SURFACE()
B_SPLINE_SURFACE(1,2,((#98238,#98239,#98240,#98241,#98242,#98243,#98244),
(#98245,#98246,#98247,#98248,#98249,#98250,#98251)),.UNSPECIFIED.,.F.,.F.,
 .F.)
B_SPLINE_SURFACE_WITH_KNOTS((2,2),(3,2,2,3),(0.710192959007093,1.),(0.349194141236593,
0.349369696259361,0.357142857142857,0.366925198536205),.UNSPECIFIED.)
GEOMETRIC_REPRESENTATION_ITEM()
RATIONAL_B_SPLINE_SURFACE(((0.99513694090229,0.99513694090229,0.99513694090229,
0.997271548787859,1.,0.99656630788526,0.994073123128689),(0.99513694090229,
0.99513694090229,0.99513694090229,0.997271548787859,1.,0.99656630788526,
0.994073123128689)))
REPRESENTATION_ITEM('')
SURFACE()
);
#326=(
BOUNDED_SURFACE()
B_SPLINE_SURFACE(1,2,((#98266,#98267,#98268),(#98269,#98270,#98271)),
 .UNSPECIFIED.,.F.,.F.,.F.)
B_SPLINE_SURFACE_WITH_KNOTS((2,2),(3,3),(0.710318915638735,1.),(0.366717817351071,
0.38393322711499),.UNSPECIFIED.)
GEOMETRIC_REPRESENTATION_ITEM()
RATIONAL_B_SPLINE_SURFACE(((0.994179254576314,0.98975654615232,0.988246641953811),
(0.994179254576314,0.98975654615232,0.988246641953811)))
REPRESENTATION_ITEM('')
SURFACE()
);
#327=(
BOUNDED_SURFACE()
B_SPLINE_SURFACE(1,2,((#98273,#98274,#98275,#98276,#98277,#98278,#98279),
(#98280,#98281,#98282,#98283,#98284,#98285,#98286)),.UNSPECIFIED.,.F.,.F.,
 .F.)
B_SPLINE_SURFACE_WITH_KNOTS((2,2),(3,2,2,3),(0.710192959008241,1.),(0.349194141236593,
0.349369696259361,0.357142857142857,0.366925198536205),.UNSPECIFIED.)
GEOMETRIC_REPRESENTATION_ITEM()
RATIONAL_B_SPLINE_SURFACE(((0.99513694090229,0.99513694090229,0.99513694090229,
0.997271548787858,1.,0.99656630788526,0.99407312312869),(0.99513694090229,
0.99513694090229,0.99513694090229,0.997271548787858,1.,0.99656630788526,
0.99407312312869)))
REPRESENTATION_ITEM('')
SURFACE()
);
#328=(
BOUNDED_SURFACE()
B_SPLINE_SURFACE(1,2,((#98299,#98300,#98301),(#98302,#98303,#98304)),
 .UNSPECIFIED.,.F.,.F.,.F.)
B_SPLINE_SURFACE_WITH_KNOTS((2,2),(3,3),(0.710318915639881,1.),(0.366717817351071,
0.383933227114987),.UNSPECIFIED.)
GEOMETRIC_REPRESENTATION_ITEM()
RATIONAL_B_SPLINE_SURFACE(((0.994179254576313,0.989756546152321,0.988246641953811),
(0.994179254576313,0.989756546152321,0.988246641953811)))
REPRESENTATION_ITEM('')
SURFACE()
);
#329=(
BOUNDED_SURFACE()
B_SPLINE_SURFACE(1,2,((#98306,#98307,#98308,#98309,#98310,#98311,#98312),
(#98313,#98314,#98315,#98316,#98317,#98318,#98319)),.UNSPECIFIED.,.F.,.F.,
 .F.)
B_SPLINE_SURFACE_WITH_KNOTS((2,2),(3,2,2,3),(0.710192959008286,1.),(0.349194141236593,
0.349369696259361,0.357142857142857,0.366925198536205),.UNSPECIFIED.)
GEOMETRIC_REPRESENTATION_ITEM()
RATIONAL_B_SPLINE_SURFACE(((0.99513694090229,0.99513694090229,0.99513694090229,
0.997271548787858,1.,0.99656630788526,0.994073123128689),(0.99513694090229,
0.99513694090229,0.99513694090229,0.997271548787858,1.,0.99656630788526,
0.994073123128689)))
REPRESENTATION_ITEM('')
SURFACE()
);
#330=(
BOUNDED_SURFACE()
B_SPLINE_SURFACE(1,2,((#98332,#98333,#98334),(#98335,#98336,#98337)),
 .UNSPECIFIED.,.F.,.F.,.F.)
B_SPLINE_SURFACE_WITH_KNOTS((2,2),(3,3),(0.710318915639926,1.),(0.366717817351071,
0.383933227114987),.UNSPECIFIED.)
GEOMETRIC_REPRESENTATION_ITEM()
RATIONAL_B_SPLINE_SURFACE(((0.994179254576313,0.989756546152321,0.988246641953811),
(0.994179254576313,0.989756546152321,0.988246641953811)))
REPRESENTATION_ITEM('')
SURFACE()
);
#331=(
BOUNDED_SURFACE()
B_SPLINE_SURFACE(1,2,((#98339,#98340,#98341,#98342,#98343,#98344,#98345),
(#98346,#98347,#98348,#98349,#98350,#98351,#98352)),.UNSPECIFIED.,.F.,.F.,
 .F.)
B_SPLINE_SURFACE_WITH_KNOTS((2,2),(3,2,2,3),(0.710192959008439,1.),(0.349194141236593,
0.349369696259361,0.357142857142857,0.366925198536205),.UNSPECIFIED.)
GEOMETRIC_REPRESENTATION_ITEM()
RATIONAL_B_SPLINE_SURFACE(((0.99513694090229,0.99513694090229,0.99513694090229,
0.997271548787858,1.,0.99656630788526,0.994073123128689),(0.99513694090229,
0.99513694090229,0.99513694090229,0.997271548787858,1.,0.99656630788526,
0.994073123128689)))
REPRESENTATION_ITEM('')
SURFACE()
);
#332=(
BOUNDED_SURFACE()
B_SPLINE_SURFACE(1,2,((#98365,#98366,#98367),(#98368,#98369,#98370)),
 .UNSPECIFIED.,.F.,.F.,.F.)
B_SPLINE_SURFACE_WITH_KNOTS((2,2),(3,3),(0.710318915640072,1.),(0.366717817351071,
0.383933227114987),.UNSPECIFIED.)
GEOMETRIC_REPRESENTATION_ITEM()
RATIONAL_B_SPLINE_SURFACE(((0.994179254576314,0.989756546152321,0.988246641953811),
(0.994179254576314,0.989756546152321,0.988246641953811)))
REPRESENTATION_ITEM('')
SURFACE()
);
#333=(
BOUNDED_SURFACE()
B_SPLINE_SURFACE(1,2,((#98372,#98373,#98374,#98375,#98376,#98377,#98378),
(#98379,#98380,#98381,#98382,#98383,#98384,#98385)),.UNSPECIFIED.,.F.,.F.,
 .F.)
B_SPLINE_SURFACE_WITH_KNOTS((2,2),(3,2,2,3),(0.710192959008445,1.),(0.349194141236593,
0.349369696259361,0.357142857142857,0.366925198536205),.UNSPECIFIED.)
GEOMETRIC_REPRESENTATION_ITEM()
RATIONAL_B_SPLINE_SURFACE(((0.99513694090229,0.99513694090229,0.99513694090229,
0.997271548787858,1.,0.99656630788526,0.99407312312869),(0.99513694090229,
0.99513694090229,0.99513694090229,0.997271548787858,1.,0.99656630788526,
0.99407312312869)))
REPRESENTATION_ITEM('')
SURFACE()
);
#334=(
BOUNDED_SURFACE()
B_SPLINE_SURFACE(1,2,((#98398,#98399,#98400),(#98401,#98402,#98403)),
 .UNSPECIFIED.,.F.,.F.,.F.)
B_SPLINE_SURFACE_WITH_KNOTS((2,2),(3,3),(0.710318915640078,1.),(0.36671781735104,
0.383933227114987),.UNSPECIFIED.)
GEOMETRIC_REPRESENTATION_ITEM()
RATIONAL_B_SPLINE_SURFACE(((0.994179254576329,0.989756546152323,0.988246641953811),
(0.994179254576329,0.989756546152323,0.988246641953811)))
REPRESENTATION_ITEM('')
SURFACE()
);
#335=(
BOUNDED_SURFACE()
B_SPLINE_SURFACE(1,2,((#98405,#98406,#98407,#98408,#98409,#98410,#98411),
(#98412,#98413,#98414,#98415,#98416,#98417,#98418)),.UNSPECIFIED.,.F.,.F.,
 .F.)
B_SPLINE_SURFACE_WITH_KNOTS((2,2),(3,2,2,3),(0.710192959008438,1.),(0.349194141236593,
0.349369696259361,0.357142857142857,0.366925198536205),.UNSPECIFIED.)
GEOMETRIC_REPRESENTATION_ITEM()
RATIONAL_B_SPLINE_SURFACE(((0.99513694090229,0.99513694090229,0.99513694090229,
0.997271548787858,1.,0.99656630788526,0.99407312312869),(0.99513694090229,
0.99513694090229,0.99513694090229,0.997271548787858,1.,0.99656630788526,
0.99407312312869)))
REPRESENTATION_ITEM('')
SURFACE()
);
#336=(
BOUNDED_SURFACE()
B_SPLINE_SURFACE(1,2,((#98433,#98434,#98435),(#98436,#98437,#98438)),
 .UNSPECIFIED.,.F.,.F.,.F.)
B_SPLINE_SURFACE_WITH_KNOTS((2,2),(3,3),(0.710318915640075,1.),(0.366717817351071,
0.383933227114987),.UNSPECIFIED.)
GEOMETRIC_REPRESENTATION_ITEM()
RATIONAL_B_SPLINE_SURFACE(((0.994179254576313,0.989756546152321,0.988246641953811),
(0.994179254576313,0.989756546152321,0.988246641953811)))
REPRESENTATION_ITEM('')
SURFACE()
);
#337=(
BOUNDED_SURFACE()
B_SPLINE_SURFACE(1,2,((#98440,#98441,#98442,#98443,#98444,#98445,#98446),
(#98447,#98448,#98449,#98450,#98451,#98452,#98453)),.UNSPECIFIED.,.F.,.F.,
 .F.)
B_SPLINE_SURFACE_WITH_KNOTS((2,2),(3,2,2,3),(0.710192959008205,1.),(0.349194141236593,
0.349369696259361,0.357142857142857,0.366925198536205),.UNSPECIFIED.)
GEOMETRIC_REPRESENTATION_ITEM()
RATIONAL_B_SPLINE_SURFACE(((0.99513694090229,0.99513694090229,0.99513694090229,
0.997271548787858,1.,0.99656630788526,0.99407312312869),(0.99513694090229,
0.99513694090229,0.99513694090229,0.997271548787858,1.,0.99656630788526,
0.99407312312869)))
REPRESENTATION_ITEM('')
SURFACE()
);
#338=(
BOUNDED_SURFACE()
B_SPLINE_SURFACE(1,2,((#98468,#98469,#98470),(#98471,#98472,#98473)),
 .UNSPECIFIED.,.F.,.F.,.F.)
B_SPLINE_SURFACE_WITH_KNOTS((2,2),(3,3),(0.710318915639842,1.),(0.366717817351071,
0.383933227114987),.UNSPECIFIED.)
GEOMETRIC_REPRESENTATION_ITEM()
RATIONAL_B_SPLINE_SURFACE(((0.994179254576314,0.989756546152321,0.988246641953811),
(0.994179254576314,0.989756546152321,0.988246641953811)))
REPRESENTATION_ITEM('')
SURFACE()
);
#339=(
BOUNDED_SURFACE()
B_SPLINE_SURFACE(1,2,((#98475,#98476,#98477,#98478,#98479,#98480,#98481),
(#98482,#98483,#98484,#98485,#98486,#98487,#98488)),.UNSPECIFIED.,.F.,.F.,
 .F.)
B_SPLINE_SURFACE_WITH_KNOTS((2,2),(3,2,2,3),(0.710192959008435,1.),(0.349194141236593,
0.349369696259361,0.357142857142857,0.366925198536205),.UNSPECIFIED.)
GEOMETRIC_REPRESENTATION_ITEM()
RATIONAL_B_SPLINE_SURFACE(((0.99513694090229,0.99513694090229,0.99513694090229,
0.997271548787858,1.,0.99656630788526,0.994073123128689),(0.99513694090229,
0.99513694090229,0.99513694090229,0.997271548787858,1.,0.99656630788526,
0.994073123128689)))
REPRESENTATION_ITEM('')
SURFACE()
);
#340=(
BOUNDED_SURFACE()
B_SPLINE_SURFACE(1,2,((#98501,#98502,#98503),(#98504,#98505,#98506)),
 .UNSPECIFIED.,.F.,.F.,.F.)
B_SPLINE_SURFACE_WITH_KNOTS((2,2),(3,3),(0.710318915640073,1.),(0.366717817351071,
0.383933227114987),.UNSPECIFIED.)
GEOMETRIC_REPRESENTATION_ITEM()
RATIONAL_B_SPLINE_SURFACE(((0.994179254576314,0.989756546152321,0.988246641953811),
(0.994179254576314,0.989756546152321,0.988246641953811)))
REPRESENTATION_ITEM('')
SURFACE()
);
#341=(
BOUNDED_SURFACE()
B_SPLINE_SURFACE(1,2,((#98508,#98509,#98510,#98511,#98512,#98513,#98514),
(#98515,#98516,#98517,#98518,#98519,#98520,#98521)),.UNSPECIFIED.,.F.,.F.,
 .F.)
B_SPLINE_SURFACE_WITH_KNOTS((2,2),(3,2,2,3),(0.71019295900831,1.),(0.349194141236593,
0.349369696259361,0.357142857142857,0.366925198536205),.UNSPECIFIED.)
GEOMETRIC_REPRESENTATION_ITEM()
RATIONAL_B_SPLINE_SURFACE(((0.99513694090229,0.99513694090229,0.99513694090229,
0.997271548787858,1.,0.99656630788526,0.99407312312869),(0.99513694090229,
0.99513694090229,0.99513694090229,0.997271548787858,1.,0.99656630788526,
0.99407312312869)))
REPRESENTATION_ITEM('')
SURFACE()
);
#342=(
BOUNDED_SURFACE()
B_SPLINE_SURFACE(1,2,((#98534,#98535,#98536),(#98537,#98538,#98539)),
 .UNSPECIFIED.,.F.,.F.,.F.)
B_SPLINE_SURFACE_WITH_KNOTS((2,2),(3,3),(0.71031891563995,1.),(0.366717817351071,
0.383933227114987),.UNSPECIFIED.)
GEOMETRIC_REPRESENTATION_ITEM()
RATIONAL_B_SPLINE_SURFACE(((0.994179254576314,0.989756546152321,0.988246641953811),
(0.994179254576314,0.989756546152321,0.988246641953811)))
REPRESENTATION_ITEM('')
SURFACE()
);
#343=(
BOUNDED_SURFACE()
B_SPLINE_SURFACE(1,2,((#98541,#98542,#98543,#98544,#98545,#98546,#98547),
(#98548,#98549,#98550,#98551,#98552,#98553,#98554)),.UNSPECIFIED.,.F.,.F.,
 .F.)
B_SPLINE_SURFACE_WITH_KNOTS((2,2),(3,2,2,3),(0.710192959007032,1.),(0.349194141236593,
0.349369696259361,0.357142857142857,0.366925198536205),.UNSPECIFIED.)
GEOMETRIC_REPRESENTATION_ITEM()
RATIONAL_B_SPLINE_SURFACE(((0.99513694090229,0.99513694090229,0.99513694090229,
0.997271548787858,1.,0.99656630788526,0.994073123128689),(0.99513694090229,
0.99513694090229,0.99513694090229,0.997271548787858,1.,0.99656630788526,
0.994073123128689)))
REPRESENTATION_ITEM('')
SURFACE()
);
#344=(
BOUNDED_SURFACE()
B_SPLINE_SURFACE(1,2,((#98569,#98570,#98571),(#98572,#98573,#98574)),
 .UNSPECIFIED.,.F.,.F.,.F.)
B_SPLINE_SURFACE_WITH_KNOTS((2,2),(3,3),(0.710318915638672,1.),(0.366717817351071,
0.383933227114987),.UNSPECIFIED.)
GEOMETRIC_REPRESENTATION_ITEM()
RATIONAL_B_SPLINE_SURFACE(((0.994179254576314,0.989756546152321,0.988246641953811),
(0.994179254576314,0.989756546152321,0.988246641953811)))
REPRESENTATION_ITEM('')
SURFACE()
);
#345=(
BOUNDED_SURFACE()
B_SPLINE_SURFACE(1,2,((#98576,#98577,#98578,#98579,#98580,#98581,#98582),
(#98583,#98584,#98585,#98586,#98587,#98588,#98589)),.UNSPECIFIED.,.F.,.F.,
 .F.)
B_SPLINE_SURFACE_WITH_KNOTS((2,2),(3,2,2,3),(0.710192959008083,1.),(0.349194141236593,
0.349369696259361,0.357142857142857,0.366925198536205),.UNSPECIFIED.)
GEOMETRIC_REPRESENTATION_ITEM()
RATIONAL_B_SPLINE_SURFACE(((0.99513694090229,0.99513694090229,0.99513694090229,
0.997271548787858,1.,0.99656630788526,0.99407312312869),(0.99513694090229,
0.99513694090229,0.99513694090229,0.997271548787858,1.,0.996566307885261,
0.99407312312869)))
REPRESENTATION_ITEM('')
SURFACE()
);
#346=(
BOUNDED_SURFACE()
B_SPLINE_SURFACE(1,2,((#98602,#98603,#98604),(#98605,#98606,#98607)),
 .UNSPECIFIED.,.F.,.F.,.F.)
B_SPLINE_SURFACE_WITH_KNOTS((2,2),(3,3),(0.71031891563972,1.),(0.36671781735083,
0.383933227114987),.UNSPECIFIED.)
GEOMETRIC_REPRESENTATION_ITEM()
RATIONAL_B_SPLINE_SURFACE(((0.994179254576438,0.989756546152342,0.988246641953811),
(0.994179254576438,0.989756546152342,0.988246641953811)))
REPRESENTATION_ITEM('')
SURFACE()
);
#347=(
BOUNDED_SURFACE()
B_SPLINE_SURFACE(1,2,((#98609,#98610,#98611,#98612,#98613,#98614,#98615),
(#98616,#98617,#98618,#98619,#98620,#98621,#98622)),.UNSPECIFIED.,.F.,.F.,
 .F.)
B_SPLINE_SURFACE_WITH_KNOTS((2,2),(3,2,2,3),(0.710192959008441,1.),(0.349194141236593,
0.349369696259361,0.357142857142857,0.366925198536205),.UNSPECIFIED.)
GEOMETRIC_REPRESENTATION_ITEM()
RATIONAL_B_SPLINE_SURFACE(((0.99513694090229,0.99513694090229,0.99513694090229,
0.997271548787858,1.,0.99656630788526,0.99407312312869),(0.99513694090229,
0.99513694090229,0.99513694090229,0.997271548787858,1.,0.99656630788526,
0.99407312312869)))
REPRESENTATION_ITEM('')
SURFACE()
);
#348=(
BOUNDED_SURFACE()
B_SPLINE_SURFACE(1,2,((#98635,#98636,#98637),(#98638,#98639,#98640)),
 .UNSPECIFIED.,.F.,.F.,.F.)
B_SPLINE_SURFACE_WITH_KNOTS((2,2),(3,3),(0.710318915640079,1.),(0.366717817350746,
0.383933227114987),.UNSPECIFIED.)
GEOMETRIC_REPRESENTATION_ITEM()
RATIONAL_B_SPLINE_SURFACE(((0.99417925457648,0.989756546152349,0.988246641953811),
(0.99417925457648,0.989756546152349,0.988246641953811)))
REPRESENTATION_ITEM('')
SURFACE()
);
#349=(
BOUNDED_SURFACE()
B_SPLINE_SURFACE(1,2,((#98642,#98643,#98644,#98645,#98646,#98647,#98648),
(#98649,#98650,#98651,#98652,#98653,#98654,#98655)),.UNSPECIFIED.,.F.,.F.,
 .F.)
B_SPLINE_SURFACE_WITH_KNOTS((2,2),(3,2,2,3),(0.710192959008353,1.),(0.349194141236593,
0.349369696259361,0.357142857142857,0.366925198536205),.UNSPECIFIED.)
GEOMETRIC_REPRESENTATION_ITEM()
RATIONAL_B_SPLINE_SURFACE(((0.99513694090229,0.99513694090229,0.99513694090229,
0.997271548787858,1.,0.99656630788526,0.994073123128689),(0.99513694090229,
0.99513694090229,0.99513694090229,0.997271548787858,1.,0.99656630788526,
0.994073123128689)))
REPRESENTATION_ITEM('')
SURFACE()
);
#350=(
BOUNDED_SURFACE()
B_SPLINE_SURFACE(1,2,((#98668,#98669,#98670),(#98671,#98672,#98673)),
 .UNSPECIFIED.,.F.,.F.,.F.)
B_SPLINE_SURFACE_WITH_KNOTS((2,2),(3,3),(0.710318915639995,1.),(0.366717817351071,
0.383933227114987),.UNSPECIFIED.)
GEOMETRIC_REPRESENTATION_ITEM()
RATIONAL_B_SPLINE_SURFACE(((0.994179254576314,0.989756546152321,0.988246641953811),
(0.994179254576314,0.989756546152321,0.988246641953811)))
REPRESENTATION_ITEM('')
SURFACE()
);
#351=(
BOUNDED_SURFACE()
B_SPLINE_SURFACE(1,2,((#98675,#98676,#98677,#98678,#98679,#98680,#98681),
(#98682,#98683,#98684,#98685,#98686,#98687,#98688)),.UNSPECIFIED.,.F.,.F.,
 .F.)
B_SPLINE_SURFACE_WITH_KNOTS((2,2),(3,2,2,3),(0.710192959008441,1.),(0.349194141236593,
0.349369696259361,0.357142857142857,0.366925198536205),.UNSPECIFIED.)
GEOMETRIC_REPRESENTATION_ITEM()
RATIONAL_B_SPLINE_SURFACE(((0.99513694090229,0.99513694090229,0.99513694090229,
0.997271548787858,1.,0.99656630788526,0.99407312312869),(0.99513694090229,
0.99513694090229,0.99513694090229,0.997271548787858,1.,0.99656630788526,
0.99407312312869)))
REPRESENTATION_ITEM('')
SURFACE()
);
#352=(
BOUNDED_SURFACE()
B_SPLINE_SURFACE(1,2,((#98701,#98702,#98703),(#98704,#98705,#98706)),
 .UNSPECIFIED.,.F.,.F.,.F.)
B_SPLINE_SURFACE_WITH_KNOTS((2,2),(3,3),(0.71031891564008,1.),(0.366717817351071,
0.383933227114987),.UNSPECIFIED.)
GEOMETRIC_REPRESENTATION_ITEM()
RATIONAL_B_SPLINE_SURFACE(((0.994179254576313,0.989756546152321,0.988246641953811),
(0.994179254576313,0.989756546152321,0.988246641953811)))
REPRESENTATION_ITEM('')
SURFACE()
);
#353=(
BOUNDED_SURFACE()
B_SPLINE_SURFACE(1,2,((#98708,#98709,#98710,#98711,#98712,#98713,#98714),
(#98715,#98716,#98717,#98718,#98719,#98720,#98721)),.UNSPECIFIED.,.F.,.F.,
 .F.)
B_SPLINE_SURFACE_WITH_KNOTS((2,2),(3,2,2,3),(0.710192959008357,1.),(0.349194141236593,
0.349369696259361,0.357142857142857,0.366925198536205),.UNSPECIFIED.)
GEOMETRIC_REPRESENTATION_ITEM()
RATIONAL_B_SPLINE_SURFACE(((0.99513694090229,0.99513694090229,0.99513694090229,
0.997271548787858,1.,0.99656630788526,0.99407312312869),(0.99513694090229,
0.99513694090229,0.99513694090229,0.997271548787858,1.,0.99656630788526,
0.99407312312869)))
REPRESENTATION_ITEM('')
SURFACE()
);
#354=(
BOUNDED_SURFACE()
B_SPLINE_SURFACE(1,2,((#98734,#98735,#98736),(#98737,#98738,#98739)),
 .UNSPECIFIED.,.F.,.F.,.F.)
B_SPLINE_SURFACE_WITH_KNOTS((2,2),(3,3),(0.710318915639997,1.),(0.366717817350691,
0.383933227114987),.UNSPECIFIED.)
GEOMETRIC_REPRESENTATION_ITEM()
RATIONAL_B_SPLINE_SURFACE(((0.994179254576509,0.989756546152354,0.988246641953811),
(0.994179254576509,0.989756546152354,0.988246641953811)))
REPRESENTATION_ITEM('')
SURFACE()
);
#355=(
BOUNDED_SURFACE()
B_SPLINE_SURFACE(1,2,((#98741,#98742,#98743,#98744,#98745,#98746,#98747),
(#98748,#98749,#98750,#98751,#98752,#98753,#98754)),.UNSPECIFIED.,.F.,.F.,
 .F.)
B_SPLINE_SURFACE_WITH_KNOTS((2,2),(3,2,2,3),(0.710192959008355,1.),(0.349194141236593,
0.349369696259361,0.357142857142857,0.366925198536205),.UNSPECIFIED.)
GEOMETRIC_REPRESENTATION_ITEM()
RATIONAL_B_SPLINE_SURFACE(((0.99513694090229,0.99513694090229,0.99513694090229,
0.997271548787858,1.,0.99656630788526,0.994073123128689),(0.99513694090229,
0.99513694090229,0.99513694090229,0.997271548787858,1.,0.99656630788526,
0.994073123128689)))
REPRESENTATION_ITEM('')
SURFACE()
);
#356=(
BOUNDED_SURFACE()
B_SPLINE_SURFACE(1,2,((#98769,#98770,#98771),(#98772,#98773,#98774)),
 .UNSPECIFIED.,.F.,.F.,.F.)
B_SPLINE_SURFACE_WITH_KNOTS((2,2),(3,3),(0.710318915639994,1.),(0.366717817351071,
0.383933227114987),.UNSPECIFIED.)
GEOMETRIC_REPRESENTATION_ITEM()
RATIONAL_B_SPLINE_SURFACE(((0.994179254576314,0.989756546152321,0.988246641953811),
(0.994179254576314,0.989756546152321,0.988246641953811)))
REPRESENTATION_ITEM('')
SURFACE()
);
#357=(
BOUNDED_SURFACE()
B_SPLINE_SURFACE(1,2,((#98776,#98777,#98778,#98779,#98780,#98781,#98782),
(#98783,#98784,#98785,#98786,#98787,#98788,#98789)),.UNSPECIFIED.,.F.,.F.,
 .F.)
B_SPLINE_SURFACE_WITH_KNOTS((2,2),(3,2,2,3),(0.710192959008362,1.),(0.349194141236593,
0.349369696259361,0.357142857142857,0.366925198536205),.UNSPECIFIED.)
GEOMETRIC_REPRESENTATION_ITEM()
RATIONAL_B_SPLINE_SURFACE(((0.99513694090229,0.99513694090229,0.99513694090229,
0.997271548787859,1.,0.99656630788526,0.99407312312869),(0.99513694090229,
0.99513694090229,0.99513694090229,0.997271548787859,1.,0.99656630788526,
0.99407312312869)))
REPRESENTATION_ITEM('')
SURFACE()
);
#358=(
BOUNDED_SURFACE()
B_SPLINE_SURFACE(1,2,((#98804,#98805,#98806),(#98807,#98808,#98809)),
 .UNSPECIFIED.,.F.,.F.,.F.)
B_SPLINE_SURFACE_WITH_KNOTS((2,2),(3,3),(0.710318915640001,1.),(0.366717817351071,
0.383933227114987),.UNSPECIFIED.)
GEOMETRIC_REPRESENTATION_ITEM()
RATIONAL_B_SPLINE_SURFACE(((0.994179254576314,0.989756546152321,0.988246641953811),
(0.994179254576314,0.989756546152321,0.988246641953811)))
REPRESENTATION_ITEM('')
SURFACE()
);
#359=(
BOUNDED_SURFACE()
B_SPLINE_SURFACE(1,2,((#98811,#98812,#98813,#98814,#98815,#98816,#98817),
(#98818,#98819,#98820,#98821,#98822,#98823,#98824)),.UNSPECIFIED.,.F.,.F.,
 .F.)
B_SPLINE_SURFACE_WITH_KNOTS((2,2),(3,2,2,3),(0.710192959008356,1.),(0.349194141236593,
0.349369696259361,0.357142857142857,0.366925198536205),.UNSPECIFIED.)
GEOMETRIC_REPRESENTATION_ITEM()
RATIONAL_B_SPLINE_SURFACE(((0.99513694090229,0.99513694090229,0.99513694090229,
0.997271548787858,1.,0.99656630788526,0.99407312312869),(0.99513694090229,
0.99513694090229,0.99513694090229,0.997271548787858,1.,0.99656630788526,
0.99407312312869)))
REPRESENTATION_ITEM('')
SURFACE()
);
#360=(
BOUNDED_SURFACE()
B_SPLINE_SURFACE(1,2,((#98839,#98840,#98841),(#98842,#98843,#98844)),
 .UNSPECIFIED.,.F.,.F.,.F.)
B_SPLINE_SURFACE_WITH_KNOTS((2,2),(3,3),(0.710318915639994,1.),(0.366717817351071,
0.383933227114986),.UNSPECIFIED.)
GEOMETRIC_REPRESENTATION_ITEM()
RATIONAL_B_SPLINE_SURFACE(((0.994179254576314,0.989756546152321,0.988246641953811),
(0.994179254576314,0.989756546152321,0.988246641953811)))
REPRESENTATION_ITEM('')
SURFACE()
);
#361=(
BOUNDED_SURFACE()
B_SPLINE_SURFACE(1,2,((#98846,#98847,#98848,#98849,#98850,#98851,#98852),
(#98853,#98854,#98855,#98856,#98857,#98858,#98859)),.UNSPECIFIED.,.F.,.F.,
 .F.)
B_SPLINE_SURFACE_WITH_KNOTS((2,2),(3,2,2,3),(0.710192959007468,1.),(0.349194141236594,
0.349369696259362,0.357142857142857,0.366925198536205),.UNSPECIFIED.)
GEOMETRIC_REPRESENTATION_ITEM()
RATIONAL_B_SPLINE_SURFACE(((0.99513694090229,0.99513694090229,0.99513694090229,
0.997271548787859,1.,0.996566307885261,0.99407312312869),(0.99513694090229,
0.99513694090229,0.99513694090229,0.997271548787859,1.,0.996566307885261,
0.99407312312869)))
REPRESENTATION_ITEM('')
SURFACE()
);
#362=(
BOUNDED_SURFACE()
B_SPLINE_SURFACE(1,2,((#98872,#98873,#98874),(#98875,#98876,#98877)),
 .UNSPECIFIED.,.F.,.F.,.F.)
B_SPLINE_SURFACE_WITH_KNOTS((2,2),(3,3),(0.710318915639108,1.),(0.366717817351052,
0.383933227114987),.UNSPECIFIED.)
GEOMETRIC_REPRESENTATION_ITEM()
RATIONAL_B_SPLINE_SURFACE(((0.994179254576324,0.989756546152323,0.988246641953811),
(0.994179254576324,0.989756546152322,0.988246641953811)))
REPRESENTATION_ITEM('')
SURFACE()
);
#363=(
BOUNDED_SURFACE()
B_SPLINE_SURFACE(1,2,((#98879,#98880,#98881,#98882,#98883,#98884,#98885),
(#98886,#98887,#98888,#98889,#98890,#98891,#98892)),.UNSPECIFIED.,.F.,.F.,
 .F.)
B_SPLINE_SURFACE_WITH_KNOTS((2,2),(3,2,2,3),(0.710192959008014,1.),(0.349194141236593,
0.349369696259361,0.357142857142857,0.366925198536205),.UNSPECIFIED.)
GEOMETRIC_REPRESENTATION_ITEM()
RATIONAL_B_SPLINE_SURFACE(((0.99513694090229,0.99513694090229,0.99513694090229,
0.997271548787858,1.,0.99656630788526,0.994073123128689),(0.99513694090229,
0.99513694090229,0.99513694090229,0.997271548787858,1.,0.99656630788526,
0.994073123128689)))
REPRESENTATION_ITEM('')
SURFACE()
);
#364=(
BOUNDED_SURFACE()
B_SPLINE_SURFACE(1,2,((#98905,#98906,#98907),(#98908,#98909,#98910)),
 .UNSPECIFIED.,.F.,.F.,.F.)
B_SPLINE_SURFACE_WITH_KNOTS((2,2),(3,3),(0.710318915639655,1.),(0.366717817351039,
0.383933227114987),.UNSPECIFIED.)
GEOMETRIC_REPRESENTATION_ITEM()
RATIONAL_B_SPLINE_SURFACE(((0.99417925457633,0.989756546152323,0.988246641953811),
(0.99417925457633,0.989756546152323,0.988246641953811)))
REPRESENTATION_ITEM('')
SURFACE()
);
#365=(
BOUNDED_SURFACE()
B_SPLINE_SURFACE(1,2,((#98912,#98913,#98914,#98915,#98916,#98917,#98918),
(#98919,#98920,#98921,#98922,#98923,#98924,#98925)),.UNSPECIFIED.,.F.,.F.,
 .F.)
B_SPLINE_SURFACE_WITH_KNOTS((2,2),(3,2,2,3),(0.710192959008103,1.),(0.349194141236593,
0.349369696259361,0.357142857142857,0.366925198536205),.UNSPECIFIED.)
GEOMETRIC_REPRESENTATION_ITEM()
RATIONAL_B_SPLINE_SURFACE(((0.99513694090229,0.99513694090229,0.99513694090229,
0.997271548787858,1.,0.99656630788526,0.99407312312869),(0.99513694090229,
0.99513694090229,0.99513694090229,0.997271548787858,1.,0.99656630788526,
0.99407312312869)))
REPRESENTATION_ITEM('')
SURFACE()
);
#366=(
BOUNDED_SURFACE()
B_SPLINE_SURFACE(1,2,((#98938,#98939,#98940),(#98941,#98942,#98943)),
 .UNSPECIFIED.,.F.,.F.,.F.)
B_SPLINE_SURFACE_WITH_KNOTS((2,2),(3,3),(0.710318915639745,1.),(0.366717817351071,
0.383933227114987),.UNSPECIFIED.)
GEOMETRIC_REPRESENTATION_ITEM()
RATIONAL_B_SPLINE_SURFACE(((0.994179254576314,0.989756546152321,0.988246641953811),
(0.994179254576314,0.989756546152321,0.988246641953811)))
REPRESENTATION_ITEM('')
SURFACE()
);
#367=(
BOUNDED_SURFACE()
B_SPLINE_SURFACE(1,2,((#98945,#98946,#98947,#98948,#98949,#98950,#98951),
(#98952,#98953,#98954,#98955,#98956,#98957,#98958)),.UNSPECIFIED.,.F.,.F.,
 .F.)
B_SPLINE_SURFACE_WITH_KNOTS((2,2),(3,2,2,3),(0.710192959007991,1.),(0.349194141236593,
0.349369696259361,0.357142857142857,0.366925198536206),.UNSPECIFIED.)
GEOMETRIC_REPRESENTATION_ITEM()
RATIONAL_B_SPLINE_SURFACE(((0.99513694090229,0.99513694090229,0.99513694090229,
0.997271548787859,1.,0.99656630788526,0.994073123128689),(0.99513694090229,
0.99513694090229,0.99513694090229,0.997271548787859,1.,0.99656630788526,
0.994073123128689)))
REPRESENTATION_ITEM('')
SURFACE()
);
#368=(
BOUNDED_SURFACE()
B_SPLINE_SURFACE(1,2,((#98966,#98967,#98968,#98969,#98970),(#98971,#98972,
#98973,#98974,#98975)),.UNSPECIFIED.,.F.,.F.,.F.)
B_SPLINE_SURFACE_WITH_KNOTS((2,2),(3,2,3),(0.,0.29040523113993),(0.40044464504831,
0.401042835325431,0.418415696246123),.UNSPECIFIED.)
GEOMETRIC_REPRESENTATION_ITEM()
RATIONAL_B_SPLINE_SURFACE(((0.988122504062136,0.988122504062136,0.988122504062136,
0.989520169850094,0.993884164197532),(0.988122504062135,0.988122504062135,
0.988122504062135,0.989520169850094,0.993884164197532)))
REPRESENTATION_ITEM('')
SURFACE()
);
#369=(
BOUNDED_SURFACE()
B_SPLINE_SURFACE(1,2,((#98984,#98985,#98986),(#98987,#98988,#98989)),
 .UNSPECIFIED.,.F.,.F.,.F.)
B_SPLINE_SURFACE_WITH_KNOTS((2,2),(3,3),(0.,0.289681084359929),(0.314840108491246,
0.332069149066805),.UNSPECIFIED.)
GEOMETRIC_REPRESENTATION_ITEM()
RATIONAL_B_SPLINE_SURFACE(((0.98789057959819,0.986774945528862,0.988576730109495),
(0.98789057959819,0.986774945528862,0.988576730109495)))
REPRESENTATION_ITEM('')
SURFACE()
);
#370=(
BOUNDED_SURFACE()
B_SPLINE_SURFACE(1,2,((#98998,#98999,#99000,#99001,#99002),(#99003,#99004,
#99005,#99006,#99007)),.UNSPECIFIED.,.F.,.F.,.F.)
B_SPLINE_SURFACE_WITH_KNOTS((2,2),(3,2,3),(0.,0.290405231173627),(0.400444645014739,
0.401042835325431,0.418415696246122),.UNSPECIFIED.)
GEOMETRIC_REPRESENTATION_ITEM()
RATIONAL_B_SPLINE_SURFACE(((0.988122504062135,0.988122504062135,0.988122504062135,
0.989520169850094,0.993884164197532),(0.988122504062135,0.988122504062135,
0.988122504062135,0.989520169850094,0.993884164197532)))
REPRESENTATION_ITEM('')
SURFACE()
);
#371=(
BOUNDED_SURFACE()
B_SPLINE_SURFACE(1,2,((#99009,#99010,#99011),(#99012,#99013,#99014)),
 .UNSPECIFIED.,.F.,.F.,.F.)
B_SPLINE_SURFACE_WITH_KNOTS((2,2),(3,3),(0.,0.28968108435993),(0.314840108491247,
0.332069149066804),.UNSPECIFIED.)
GEOMETRIC_REPRESENTATION_ITEM()
RATIONAL_B_SPLINE_SURFACE(((0.98789057959819,0.986774945528862,0.988576730109495),
(0.98789057959819,0.986774945528862,0.988576730109495)))
REPRESENTATION_ITEM('')
SURFACE()
);
#372=(
BOUNDED_SURFACE()
B_SPLINE_SURFACE(1,2,((#99023,#99024,#99025,#99026,#99027),(#99028,#99029,
#99030,#99031,#99032)),.UNSPECIFIED.,.F.,.F.,.F.)
B_SPLINE_SURFACE_WITH_KNOTS((2,2),(3,2,3),(0.,0.290405231161606),(0.400444645026067,
0.40104283532543,0.418415696246121),.UNSPECIFIED.)
GEOMETRIC_REPRESENTATION_ITEM()
RATIONAL_B_SPLINE_SURFACE(((0.988122504062135,0.988122504062135,0.988122504062135,
0.989520169850093,0.993884164197532),(0.988122504062135,0.988122504062135,
0.988122504062135,0.989520169850093,0.993884164197532)))
REPRESENTATION_ITEM('')
SURFACE()
);
#373=(
BOUNDED_SURFACE()
B_SPLINE_SURFACE(1,2,((#99034,#99035,#99036),(#99037,#99038,#99039)),
 .UNSPECIFIED.,.F.,.F.,.F.)
B_SPLINE_SURFACE_WITH_KNOTS((2,2),(3,3),(0.,0.289681084359922),(0.314840108491247,
0.332069149066805),.UNSPECIFIED.)
GEOMETRIC_REPRESENTATION_ITEM()
RATIONAL_B_SPLINE_SURFACE(((0.98789057959819,0.986774945528862,0.988576730109495),
(0.98789057959819,0.986774945528862,0.988576730109495)))
REPRESENTATION_ITEM('')
SURFACE()
);
#374=(
BOUNDED_SURFACE()
B_SPLINE_SURFACE(1,2,((#99048,#99049,#99050,#99051,#99052),(#99053,#99054,
#99055,#99056,#99057)),.UNSPECIFIED.,.F.,.F.,.F.)
B_SPLINE_SURFACE_WITH_KNOTS((2,2),(3,2,3),(0.,0.290405231142216),(0.400444645037561,
0.40104283532543,0.418415696246121),.UNSPECIFIED.)
GEOMETRIC_REPRESENTATION_ITEM()
RATIONAL_B_SPLINE_SURFACE(((0.988122504062135,0.988122504062135,0.988122504062135,
0.989520169850093,0.993884164197532),(0.988122504062135,0.988122504062135,
0.988122504062135,0.989520169850093,0.993884164197532)))
REPRESENTATION_ITEM('')
SURFACE()
);
#375=(
BOUNDED_SURFACE()
B_SPLINE_SURFACE(1,2,((#99059,#99060,#99061),(#99062,#99063,#99064)),
 .UNSPECIFIED.,.F.,.F.,.F.)
B_SPLINE_SURFACE_WITH_KNOTS((2,2),(3,3),(0.,0.289681084359915),(0.314840108491247,
0.332069149066805),.UNSPECIFIED.)
GEOMETRIC_REPRESENTATION_ITEM()
RATIONAL_B_SPLINE_SURFACE(((0.98789057959819,0.986774945528862,0.988576730109495),
(0.98789057959819,0.986774945528862,0.988576730109495)))
REPRESENTATION_ITEM('')
SURFACE()
);
#376=(
BOUNDED_SURFACE()
B_SPLINE_SURFACE(1,2,((#99073,#99074,#99075,#99076,#99077),(#99078,#99079,
#99080,#99081,#99082)),.UNSPECIFIED.,.F.,.F.,.F.)
B_SPLINE_SURFACE_WITH_KNOTS((2,2),(3,2,3),(0.,0.290405231151886),(0.400444645028098,
0.401042835325431,0.418415696246121),.UNSPECIFIED.)
GEOMETRIC_REPRESENTATION_ITEM()
RATIONAL_B_SPLINE_SURFACE(((0.988122504062136,0.988122504062136,0.988122504062136,
0.989520169850094,0.993884164197532),(0.988122504062136,0.988122504062136,
0.988122504062136,0.989520169850094,0.993884164197532)))
REPRESENTATION_ITEM('')
SURFACE()
);
#377=(
BOUNDED_SURFACE()
B_SPLINE_SURFACE(1,2,((#99084,#99085,#99086),(#99087,#99088,#99089)),
 .UNSPECIFIED.,.F.,.F.,.F.)
B_SPLINE_SURFACE_WITH_KNOTS((2,2),(3,3),(0.,0.289681084359921),(0.314840108491246,
0.332069149066804),.UNSPECIFIED.)
GEOMETRIC_REPRESENTATION_ITEM()
RATIONAL_B_SPLINE_SURFACE(((0.98789057959819,0.986774945528862,0.988576730109495),
(0.98789057959819,0.986774945528862,0.988576730109495)))
REPRESENTATION_ITEM('')
SURFACE()
);
#378=(
BOUNDED_SURFACE()
B_SPLINE_SURFACE(1,2,((#99098,#99099,#99100,#99101,#99102),(#99103,#99104,
#99105,#99106,#99107)),.UNSPECIFIED.,.F.,.F.,.F.)
B_SPLINE_SURFACE_WITH_KNOTS((2,2),(3,2,3),(0.,0.290405231115877),(0.400444645063817,
0.401042835325431,0.418415696246122),.UNSPECIFIED.)
GEOMETRIC_REPRESENTATION_ITEM()
RATIONAL_B_SPLINE_SURFACE(((0.988122504062135,0.988122504062135,0.988122504062135,
0.989520169850094,0.993884164197532),(0.988122504062136,0.988122504062136,
0.988122504062136,0.989520169850094,0.993884164197532)))
REPRESENTATION_ITEM('')
SURFACE()
);
#379=(
BOUNDED_SURFACE()
B_SPLINE_SURFACE(1,2,((#99109,#99110,#99111),(#99112,#99113,#99114)),
 .UNSPECIFIED.,.F.,.F.,.F.)
B_SPLINE_SURFACE_WITH_KNOTS((2,2),(3,3),(0.,0.289681084359917),(0.314840108491246,
0.332069149066804),.UNSPECIFIED.)
GEOMETRIC_REPRESENTATION_ITEM()
RATIONAL_B_SPLINE_SURFACE(((0.98789057959819,0.986774945528862,0.988576730109495),
(0.98789057959819,0.986774945528862,0.988576730109495)))
REPRESENTATION_ITEM('')
SURFACE()
);
#380=(
BOUNDED_SURFACE()
B_SPLINE_SURFACE(1,2,((#99123,#99124,#99125,#99126,#99127),(#99128,#99129,
#99130,#99131,#99132)),.UNSPECIFIED.,.F.,.F.,.F.)
B_SPLINE_SURFACE_WITH_KNOTS((2,2),(3,2,3),(0.,0.290405231151133),(0.400444645029202,
0.401042835325431,0.418415696246122),.UNSPECIFIED.)
GEOMETRIC_REPRESENTATION_ITEM()
RATIONAL_B_SPLINE_SURFACE(((0.988122504062136,0.988122504062136,0.988122504062136,
0.989520169850094,0.993884164197532),(0.988122504062135,0.988122504062135,
0.988122504062135,0.989520169850094,0.993884164197532)))
REPRESENTATION_ITEM('')
SURFACE()
);
#381=(
BOUNDED_SURFACE()
B_SPLINE_SURFACE(1,2,((#99134,#99135,#99136),(#99137,#99138,#99139)),
 .UNSPECIFIED.,.F.,.F.,.F.)
B_SPLINE_SURFACE_WITH_KNOTS((2,2),(3,3),(0.,0.289681084359922),(0.314840108491246,
0.332069149066804),.UNSPECIFIED.)
GEOMETRIC_REPRESENTATION_ITEM()
RATIONAL_B_SPLINE_SURFACE(((0.98789057959819,0.986774945528862,0.988576730109495),
(0.98789057959819,0.986774945528862,0.988576730109495)))
REPRESENTATION_ITEM('')
SURFACE()
);
#382=(
BOUNDED_SURFACE()
B_SPLINE_SURFACE(1,2,((#99148,#99149,#99150,#99151,#99152),(#99153,#99154,
#99155,#99156,#99157)),.UNSPECIFIED.,.F.,.F.,.F.)
B_SPLINE_SURFACE_WITH_KNOTS((2,2),(3,2,3),(0.,0.290405231117896),(0.400444645069685,
0.401042835325431,0.418415696246122),.UNSPECIFIED.)
GEOMETRIC_REPRESENTATION_ITEM()
RATIONAL_B_SPLINE_SURFACE(((0.988122504062136,0.988122504062136,0.988122504062136,
0.989520169850094,0.993884164197532),(0.988122504062135,0.988122504062135,
0.988122504062135,0.989520169850094,0.993884164197532)))
REPRESENTATION_ITEM('')
SURFACE()
);
#383=(
BOUNDED_SURFACE()
B_SPLINE_SURFACE(1,2,((#99159,#99160,#99161),(#99162,#99163,#99164)),
 .UNSPECIFIED.,.F.,.F.,.F.)
B_SPLINE_SURFACE_WITH_KNOTS((2,2),(3,3),(0.,0.289681084359918),(0.314840108491246,
0.332069149066804),.UNSPECIFIED.)
GEOMETRIC_REPRESENTATION_ITEM()
RATIONAL_B_SPLINE_SURFACE(((0.98789057959819,0.986774945528862,0.988576730109495),
(0.98789057959819,0.986774945528862,0.988576730109495)))
REPRESENTATION_ITEM('')
SURFACE()
);
#384=(
BOUNDED_SURFACE()
B_SPLINE_SURFACE(1,2,((#99173,#99174,#99175,#99176,#99177),(#99178,#99179,
#99180,#99181,#99182)),.UNSPECIFIED.,.F.,.F.,.F.)
B_SPLINE_SURFACE_WITH_KNOTS((2,2),(3,2,3),(0.,0.290405231125489),(0.400444645062306,
0.401042835325431,0.418415696246122),.UNSPECIFIED.)
GEOMETRIC_REPRESENTATION_ITEM()
RATIONAL_B_SPLINE_SURFACE(((0.988122504062135,0.988122504062135,0.988122504062135,
0.989520169850094,0.993884164197532),(0.988122504062136,0.988122504062136,
0.988122504062136,0.989520169850094,0.993884164197532)))
REPRESENTATION_ITEM('')
SURFACE()
);
#385=(
BOUNDED_SURFACE()
B_SPLINE_SURFACE(1,2,((#99184,#99185,#99186),(#99187,#99188,#99189)),
 .UNSPECIFIED.,.F.,.F.,.F.)
B_SPLINE_SURFACE_WITH_KNOTS((2,2),(3,3),(0.,0.289681084359918),(0.314840108491246,
0.332069149066804),.UNSPECIFIED.)
GEOMETRIC_REPRESENTATION_ITEM()
RATIONAL_B_SPLINE_SURFACE(((0.98789057959819,0.986774945528862,0.988576730109495),
(0.98789057959819,0.986774945528862,0.988576730109495)))
REPRESENTATION_ITEM('')
SURFACE()
);
#386=(
BOUNDED_SURFACE()
B_SPLINE_SURFACE(1,2,((#99198,#99199,#99200,#99201,#99202),(#99203,#99204,
#99205,#99206,#99207)),.UNSPECIFIED.,.F.,.F.,.F.)
B_SPLINE_SURFACE_WITH_KNOTS((2,2),(3,2,3),(0.,0.290405231155539),(0.400444645032021,
0.401042835325431,0.418415696246122),.UNSPECIFIED.)
GEOMETRIC_REPRESENTATION_ITEM()
RATIONAL_B_SPLINE_SURFACE(((0.988122504062136,0.988122504062136,0.988122504062136,
0.989520169850094,0.993884164197532),(0.988122504062136,0.988122504062136,
0.988122504062136,0.989520169850094,0.993884164197532)))
REPRESENTATION_ITEM('')
SURFACE()
);
#387=(
BOUNDED_SURFACE()
B_SPLINE_SURFACE(1,2,((#99209,#99210,#99211),(#99212,#99213,#99214)),
 .UNSPECIFIED.,.F.,.F.,.F.)
B_SPLINE_SURFACE_WITH_KNOTS((2,2),(3,3),(0.,0.289681084359924),(0.314840108491246,
0.332069149066804),.UNSPECIFIED.)
GEOMETRIC_REPRESENTATION_ITEM()
RATIONAL_B_SPLINE_SURFACE(((0.98789057959819,0.986774945528862,0.988576730109495),
(0.98789057959819,0.986774945528862,0.988576730109495)))
REPRESENTATION_ITEM('')
SURFACE()
);
#388=(
BOUNDED_SURFACE()
B_SPLINE_SURFACE(1,2,((#99223,#99224,#99225,#99226,#99227),(#99228,#99229,
#99230,#99231,#99232)),.UNSPECIFIED.,.F.,.F.,.F.)
B_SPLINE_SURFACE_WITH_KNOTS((2,2),(3,2,3),(0.,0.290405231152987),(0.400444645034762,
0.401042835325431,0.418415696246122),.UNSPECIFIED.)
GEOMETRIC_REPRESENTATION_ITEM()
RATIONAL_B_SPLINE_SURFACE(((0.988122504062136,0.988122504062136,0.988122504062136,
0.989520169850094,0.993884164197532),(0.988122504062136,0.988122504062136,
0.988122504062136,0.989520169850094,0.993884164197532)))
REPRESENTATION_ITEM('')
SURFACE()
);
#389=(
BOUNDED_SURFACE()
B_SPLINE_SURFACE(1,2,((#99234,#99235,#99236),(#99237,#99238,#99239)),
 .UNSPECIFIED.,.F.,.F.,.F.)
B_SPLINE_SURFACE_WITH_KNOTS((2,2),(3,3),(0.,0.289681084359924),(0.314840108491246,
0.332069149066804),.UNSPECIFIED.)
GEOMETRIC_REPRESENTATION_ITEM()
RATIONAL_B_SPLINE_SURFACE(((0.98789057959819,0.986774945528862,0.988576730109495),
(0.98789057959819,0.986774945528862,0.988576730109495)))
REPRESENTATION_ITEM('')
SURFACE()
);
#390=(
BOUNDED_SURFACE()
B_SPLINE_SURFACE(1,2,((#99248,#99249,#99250,#99251,#99252),(#99253,#99254,
#99255,#99256,#99257)),.UNSPECIFIED.,.F.,.F.,.F.)
B_SPLINE_SURFACE_WITH_KNOTS((2,2),(3,2,3),(0.,0.290405231142137),(0.400444645037875,
0.401042835325431,0.418415696246122),.UNSPECIFIED.)
GEOMETRIC_REPRESENTATION_ITEM()
RATIONAL_B_SPLINE_SURFACE(((0.988122504062136,0.988122504062136,0.988122504062136,
0.989520169850094,0.993884164197532),(0.988122504062136,0.988122504062136,
0.988122504062136,0.989520169850094,0.993884164197532)))
REPRESENTATION_ITEM('')
SURFACE()
);
#391=(
BOUNDED_SURFACE()
B_SPLINE_SURFACE(1,2,((#99259,#99260,#99261),(#99262,#99263,#99264)),
 .UNSPECIFIED.,.F.,.F.,.F.)
B_SPLINE_SURFACE_WITH_KNOTS((2,2),(3,3),(0.,0.28968108435992),(0.314840108491246,
0.332069149066804),.UNSPECIFIED.)
GEOMETRIC_REPRESENTATION_ITEM()
RATIONAL_B_SPLINE_SURFACE(((0.98789057959819,0.986774945528862,0.988576730109495),
(0.98789057959819,0.986774945528862,0.988576730109495)))
REPRESENTATION_ITEM('')
SURFACE()
);
#392=(
BOUNDED_SURFACE()
B_SPLINE_SURFACE(1,2,((#99273,#99274,#99275,#99276,#99277),(#99278,#99279,
#99280,#99281,#99282)),.UNSPECIFIED.,.F.,.F.,.F.)
B_SPLINE_SURFACE_WITH_KNOTS((2,2),(3,2,3),(0.,0.290405231138609),(0.400444645042956,
0.401042835325431,0.418415696246122),.UNSPECIFIED.)
GEOMETRIC_REPRESENTATION_ITEM()
RATIONAL_B_SPLINE_SURFACE(((0.988122504062136,0.988122504062136,0.988122504062136,
0.989520169850094,0.993884164197532),(0.988122504062136,0.988122504062136,
0.988122504062136,0.989520169850094,0.993884164197532)))
REPRESENTATION_ITEM('')
SURFACE()
);
#393=(
BOUNDED_SURFACE()
B_SPLINE_SURFACE(1,2,((#99284,#99285,#99286),(#99287,#99288,#99289)),
 .UNSPECIFIED.,.F.,.F.,.F.)
B_SPLINE_SURFACE_WITH_KNOTS((2,2),(3,3),(0.,0.289681084359919),(0.314840108491246,
0.332069149066804),.UNSPECIFIED.)
GEOMETRIC_REPRESENTATION_ITEM()
RATIONAL_B_SPLINE_SURFACE(((0.98789057959819,0.986774945528862,0.988576730109495),
(0.98789057959819,0.986774945528862,0.988576730109495)))
REPRESENTATION_ITEM('')
SURFACE()
);
#394=(
BOUNDED_SURFACE()
B_SPLINE_SURFACE(1,2,((#99298,#99299,#99300,#99301,#99302),(#99303,#99304,
#99305,#99306,#99307)),.UNSPECIFIED.,.F.,.F.,.F.)
B_SPLINE_SURFACE_WITH_KNOTS((2,2),(3,2,3),(0.,0.290405231111565),(0.400444645068332,
0.401042835325431,0.418415696246122),.UNSPECIFIED.)
GEOMETRIC_REPRESENTATION_ITEM()
RATIONAL_B_SPLINE_SURFACE(((0.988122504062136,0.988122504062136,0.988122504062136,
0.989520169850094,0.993884164197532),(0.988122504062135,0.988122504062135,
0.988122504062135,0.989520169850094,0.993884164197532)))
REPRESENTATION_ITEM('')
SURFACE()
);
#395=(
BOUNDED_SURFACE()
B_SPLINE_SURFACE(1,2,((#99309,#99310,#99311),(#99312,#99313,#99314)),
 .UNSPECIFIED.,.F.,.F.,.F.)
B_SPLINE_SURFACE_WITH_KNOTS((2,2),(3,3),(0.,0.289681084359928),(0.314840108491246,
0.332069149066804),.UNSPECIFIED.)
GEOMETRIC_REPRESENTATION_ITEM()
RATIONAL_B_SPLINE_SURFACE(((0.98789057959819,0.986774945528862,0.988576730109495),
(0.98789057959819,0.986774945528862,0.988576730109495)))
REPRESENTATION_ITEM('')
SURFACE()
);
#396=(
BOUNDED_SURFACE()
B_SPLINE_SURFACE(1,2,((#99323,#99324,#99325,#99326,#99327),(#99328,#99329,
#99330,#99331,#99332)),.UNSPECIFIED.,.F.,.F.,.F.)
B_SPLINE_SURFACE_WITH_KNOTS((2,2),(3,2,3),(0.,0.290038987984222),(0.400810888203859,
0.401042835325431,0.418415696246122),.UNSPECIFIED.)
GEOMETRIC_REPRESENTATION_ITEM()
RATIONAL_B_SPLINE_SURFACE(((0.988122504062136,0.988122504062136,0.988122504062136,
0.989520169850094,0.993884164197532),(0.988122504062136,0.988122504062136,
0.988122504062136,0.989520169850094,0.993884164197532)))
REPRESENTATION_ITEM('')
SURFACE()
);
#397=(
BOUNDED_SURFACE()
B_SPLINE_SURFACE(1,2,((#99334,#99335,#99336),(#99337,#99338,#99339)),
 .UNSPECIFIED.,.F.,.F.,.F.)
B_SPLINE_SURFACE_WITH_KNOTS((2,2),(3,3),(0.,0.289681084359918),(0.314840108491245,
0.332069149066804),.UNSPECIFIED.)
GEOMETRIC_REPRESENTATION_ITEM()
RATIONAL_B_SPLINE_SURFACE(((0.98789057959819,0.986774945528862,0.988576730109495),
(0.98789057959819,0.986774945528862,0.988576730109495)))
REPRESENTATION_ITEM('')
SURFACE()
);
#398=(
BOUNDED_SURFACE()
B_SPLINE_SURFACE(1,2,((#99348,#99349,#99350,#99351,#99352),(#99353,#99354,
#99355,#99356,#99357)),.UNSPECIFIED.,.F.,.F.,.F.)
B_SPLINE_SURFACE_WITH_KNOTS((2,2),(3,2,3),(0.,0.290405231165758),(0.400444645022587,
0.401042835325431,0.418415696246122),.UNSPECIFIED.)
GEOMETRIC_REPRESENTATION_ITEM()
RATIONAL_B_SPLINE_SURFACE(((0.988122504062135,0.988122504062135,0.988122504062135,
0.989520169850094,0.993884164197532),(0.988122504062135,0.988122504062135,
0.988122504062135,0.989520169850094,0.993884164197532)))
REPRESENTATION_ITEM('')
SURFACE()
);
#399=(
BOUNDED_SURFACE()
B_SPLINE_SURFACE(1,2,((#99359,#99360,#99361),(#99362,#99363,#99364)),
 .UNSPECIFIED.,.F.,.F.,.F.)
B_SPLINE_SURFACE_WITH_KNOTS((2,2),(3,3),(0.,0.289681084359926),(0.314840108491246,
0.332069149066804),.UNSPECIFIED.)
GEOMETRIC_REPRESENTATION_ITEM()
RATIONAL_B_SPLINE_SURFACE(((0.98789057959819,0.986774945528862,0.988576730109495),
(0.98789057959819,0.986774945528862,0.988576730109495)))
REPRESENTATION_ITEM('')
SURFACE()
);
#400=(
BOUNDED_SURFACE()
B_SPLINE_SURFACE(1,2,((#99373,#99374,#99375,#99376,#99377),(#99378,#99379,
#99380,#99381,#99382)),.UNSPECIFIED.,.F.,.F.,.F.)
B_SPLINE_SURFACE_WITH_KNOTS((2,2),(3,2,3),(0.,0.290405231142974),(0.40044464504501,
0.401042835325431,0.418415696246122),.UNSPECIFIED.)
GEOMETRIC_REPRESENTATION_ITEM()
RATIONAL_B_SPLINE_SURFACE(((0.988122504062136,0.988122504062136,0.988122504062136,
0.989520169850094,0.993884164197532),(0.988122504062136,0.988122504062136,
0.988122504062136,0.989520169850094,0.993884164197532)))
REPRESENTATION_ITEM('')
SURFACE()
);
#401=(
BOUNDED_SURFACE()
B_SPLINE_SURFACE(1,2,((#99384,#99385,#99386),(#99387,#99388,#99389)),
 .UNSPECIFIED.,.F.,.F.,.F.)
B_SPLINE_SURFACE_WITH_KNOTS((2,2),(3,3),(0.,0.289681084359927),(0.314840108491246,
0.332069149066804),.UNSPECIFIED.)
GEOMETRIC_REPRESENTATION_ITEM()
RATIONAL_B_SPLINE_SURFACE(((0.98789057959819,0.986774945528862,0.988576730109495),
(0.98789057959819,0.986774945528862,0.988576730109495)))
REPRESENTATION_ITEM('')
SURFACE()
);
#402=(
BOUNDED_SURFACE()
B_SPLINE_SURFACE(1,2,((#99398,#99399,#99400,#99401,#99402),(#99403,#99404,
#99405,#99406,#99407)),.UNSPECIFIED.,.F.,.F.,.F.)
B_SPLINE_SURFACE_WITH_KNOTS((2,2),(3,2,3),(0.,0.290405231138202),(0.400444645049142,
0.401042835325431,0.418415696246122),.UNSPECIFIED.)
GEOMETRIC_REPRESENTATION_ITEM()
RATIONAL_B_SPLINE_SURFACE(((0.988122504062135,0.988122504062135,0.988122504062135,
0.989520169850094,0.993884164197532),(0.988122504062135,0.988122504062135,
0.988122504062135,0.989520169850094,0.993884164197532)))
REPRESENTATION_ITEM('')
SURFACE()
);
#403=(
BOUNDED_SURFACE()
B_SPLINE_SURFACE(1,2,((#99409,#99410,#99411),(#99412,#99413,#99414)),
 .UNSPECIFIED.,.F.,.F.,.F.)
B_SPLINE_SURFACE_WITH_KNOTS((2,2),(3,3),(0.,0.289681084359929),(0.314840108491246,
0.332069149066804),.UNSPECIFIED.)
GEOMETRIC_REPRESENTATION_ITEM()
RATIONAL_B_SPLINE_SURFACE(((0.98789057959819,0.986774945528862,0.988576730109495),
(0.98789057959819,0.986774945528862,0.988576730109495)))
REPRESENTATION_ITEM('')
SURFACE()
);
#404=(
BOUNDED_SURFACE()
B_SPLINE_SURFACE(1,2,((#99423,#99424,#99425,#99426,#99427),(#99428,#99429,
#99430,#99431,#99432)),.UNSPECIFIED.,.F.,.F.,.F.)
B_SPLINE_SURFACE_WITH_KNOTS((2,2),(3,2,3),(0.,0.290405231155372),(0.400444645024719,
0.401042835325431,0.418415696246122),.UNSPECIFIED.)
GEOMETRIC_REPRESENTATION_ITEM()
RATIONAL_B_SPLINE_SURFACE(((0.988122504062136,0.988122504062136,0.988122504062136,
0.989520169850094,0.993884164197532),(0.988122504062136,0.988122504062136,
0.988122504062136,0.989520169850094,0.993884164197532)))
REPRESENTATION_ITEM('')
SURFACE()
);
#405=(
BOUNDED_SURFACE()
B_SPLINE_SURFACE(1,2,((#99434,#99435,#99436),(#99437,#99438,#99439)),
 .UNSPECIFIED.,.F.,.F.,.F.)
B_SPLINE_SURFACE_WITH_KNOTS((2,2),(3,3),(0.,0.289681084359924),(0.314840108491246,
0.332069149066804),.UNSPECIFIED.)
GEOMETRIC_REPRESENTATION_ITEM()
RATIONAL_B_SPLINE_SURFACE(((0.98789057959819,0.986774945528862,0.988576730109495),
(0.98789057959819,0.986774945528862,0.988576730109495)))
REPRESENTATION_ITEM('')
SURFACE()
);
#406=(
BOUNDED_SURFACE()
B_SPLINE_SURFACE(1,2,((#99448,#99449,#99450,#99451,#99452),(#99453,#99454,
#99455,#99456,#99457)),.UNSPECIFIED.,.F.,.F.,.F.)
B_SPLINE_SURFACE_WITH_KNOTS((2,2),(3,2,3),(0.,0.290405231151189),(0.40044464502924,
0.401042835325431,0.418415696246122),.UNSPECIFIED.)
GEOMETRIC_REPRESENTATION_ITEM()
RATIONAL_B_SPLINE_SURFACE(((0.988122504062136,0.988122504062136,0.988122504062136,
0.989520169850094,0.993884164197532),(0.988122504062136,0.988122504062136,
0.988122504062136,0.989520169850094,0.993884164197532)))
REPRESENTATION_ITEM('')
SURFACE()
);
#407=(
BOUNDED_SURFACE()
B_SPLINE_SURFACE(1,2,((#99459,#99460,#99461),(#99462,#99463,#99464)),
 .UNSPECIFIED.,.F.,.F.,.F.)
B_SPLINE_SURFACE_WITH_KNOTS((2,2),(3,3),(0.,0.289681084359917),(0.314840108491246,
0.332069149066804),.UNSPECIFIED.)
GEOMETRIC_REPRESENTATION_ITEM()
RATIONAL_B_SPLINE_SURFACE(((0.98789057959819,0.986774945528862,0.988576730109495),
(0.98789057959819,0.986774945528862,0.988576730109495)))
REPRESENTATION_ITEM('')
SURFACE()
);
#408=(
BOUNDED_SURFACE()
B_SPLINE_SURFACE(1,2,((#99473,#99474,#99475,#99476,#99477),(#99478,#99479,
#99480,#99481,#99482)),.UNSPECIFIED.,.F.,.F.,.F.)
B_SPLINE_SURFACE_WITH_KNOTS((2,2),(3,2,3),(0.,0.290405231148719),(0.400444645031816,
0.401042835325431,0.418415696246123),.UNSPECIFIED.)
GEOMETRIC_REPRESENTATION_ITEM()
RATIONAL_B_SPLINE_SURFACE(((0.988122504062136,0.988122504062136,0.988122504062136,
0.989520169850094,0.993884164197532),(0.988122504062136,0.988122504062136,
0.988122504062136,0.989520169850094,0.993884164197532)))
REPRESENTATION_ITEM('')
SURFACE()
);
#409=(
BOUNDED_SURFACE()
B_SPLINE_SURFACE(1,2,((#99484,#99485,#99486),(#99487,#99488,#99489)),
 .UNSPECIFIED.,.F.,.F.,.F.)
B_SPLINE_SURFACE_WITH_KNOTS((2,2),(3,3),(0.,0.289681084359925),(0.314840108491246,
0.332069149066812),.UNSPECIFIED.)
GEOMETRIC_REPRESENTATION_ITEM()
RATIONAL_B_SPLINE_SURFACE(((0.98789057959819,0.986774945528861,0.988576730109497),
(0.98789057959819,0.986774945528861,0.988576730109497)))
REPRESENTATION_ITEM('')
SURFACE()
);
#410=(
BOUNDED_SURFACE()
B_SPLINE_SURFACE(1,2,((#99498,#99499,#99500,#99501,#99502),(#99503,#99504,
#99505,#99506,#99507)),.UNSPECIFIED.,.F.,.F.,.F.)
B_SPLINE_SURFACE_WITH_KNOTS((2,2),(3,2,3),(0.,0.290405231137082),(0.400444645044425,
0.401042835325431,0.418415696246122),.UNSPECIFIED.)
GEOMETRIC_REPRESENTATION_ITEM()
RATIONAL_B_SPLINE_SURFACE(((0.988122504062135,0.988122504062135,0.988122504062135,
0.989520169850094,0.993884164197532),(0.988122504062135,0.988122504062135,
0.988122504062135,0.989520169850094,0.993884164197532)))
REPRESENTATION_ITEM('')
SURFACE()
);
#411=(
BOUNDED_SURFACE()
B_SPLINE_SURFACE(1,2,((#99509,#99510,#99511),(#99512,#99513,#99514)),
 .UNSPECIFIED.,.F.,.F.,.F.)
B_SPLINE_SURFACE_WITH_KNOTS((2,2),(3,3),(0.,0.289681084359928),(0.314840108491246,
0.332069149066804),.UNSPECIFIED.)
GEOMETRIC_REPRESENTATION_ITEM()
RATIONAL_B_SPLINE_SURFACE(((0.98789057959819,0.986774945528862,0.988576730109495),
(0.98789057959819,0.986774945528862,0.988576730109495)))
REPRESENTATION_ITEM('')
SURFACE()
);
#412=(
BOUNDED_SURFACE()
B_SPLINE_SURFACE(1,2,((#99523,#99524,#99525,#99526,#99527),(#99528,#99529,
#99530,#99531,#99532)),.UNSPECIFIED.,.F.,.F.,.F.)
B_SPLINE_SURFACE_WITH_KNOTS((2,2),(3,2,3),(0.,0.290405231145953),(0.400444645042899,
0.401042835325431,0.418415696246122),.UNSPECIFIED.)
GEOMETRIC_REPRESENTATION_ITEM()
RATIONAL_B_SPLINE_SURFACE(((0.988122504062136,0.988122504062136,0.988122504062136,
0.989520169850094,0.993884164197532),(0.988122504062135,0.988122504062135,
0.988122504062135,0.989520169850094,0.993884164197532)))
REPRESENTATION_ITEM('')
SURFACE()
);
#413=(
BOUNDED_SURFACE()
B_SPLINE_SURFACE(1,2,((#99534,#99535,#99536),(#99537,#99538,#99539)),
 .UNSPECIFIED.,.F.,.F.,.F.)
B_SPLINE_SURFACE_WITH_KNOTS((2,2),(3,3),(0.,0.289681084359932),(0.314840108491246,
0.332069149066804),.UNSPECIFIED.)
GEOMETRIC_REPRESENTATION_ITEM()
RATIONAL_B_SPLINE_SURFACE(((0.98789057959819,0.986774945528862,0.988576730109495),
(0.98789057959819,0.986774945528862,0.988576730109495)))
REPRESENTATION_ITEM('')
SURFACE()
);
#414=(
BOUNDED_SURFACE()
B_SPLINE_SURFACE(1,2,((#99548,#99549,#99550,#99551,#99552),(#99553,#99554,
#99555,#99556,#99557)),.UNSPECIFIED.,.F.,.F.,.F.)
B_SPLINE_SURFACE_WITH_KNOTS((2,2),(3,2,3),(0.,0.290405231150516),(0.400444645038493,
0.401042835325431,0.418415696246122),.UNSPECIFIED.)
GEOMETRIC_REPRESENTATION_ITEM()
RATIONAL_B_SPLINE_SURFACE(((0.988122504062136,0.988122504062136,0.988122504062136,
0.989520169850094,0.993884164197532),(0.988122504062135,0.988122504062135,
0.988122504062135,0.989520169850094,0.993884164197532)))
REPRESENTATION_ITEM('')
SURFACE()
);
#415=(
BOUNDED_SURFACE()
B_SPLINE_SURFACE(1,2,((#99559,#99560,#99561),(#99562,#99563,#99564)),
 .UNSPECIFIED.,.F.,.F.,.F.)
B_SPLINE_SURFACE_WITH_KNOTS((2,2),(3,3),(0.,0.289681084359926),(0.314840108491246,
0.332069149066806),.UNSPECIFIED.)
GEOMETRIC_REPRESENTATION_ITEM()
RATIONAL_B_SPLINE_SURFACE(((0.98789057959819,0.986774945528862,0.988576730109495),
(0.98789057959819,0.986774945528862,0.988576730109495)))
REPRESENTATION_ITEM('')
SURFACE()
);
#416=(
BOUNDED_SURFACE()
B_SPLINE_SURFACE(1,2,((#99573,#99574,#99575,#99576,#99577),(#99578,#99579,
#99580,#99581,#99582)),.UNSPECIFIED.,.F.,.F.,.F.)
B_SPLINE_SURFACE_WITH_KNOTS((2,2),(3,2,3),(0.,0.290405231145865),(0.400444645042583,
0.401042835325431,0.418415696246123),.UNSPECIFIED.)
GEOMETRIC_REPRESENTATION_ITEM()
RATIONAL_B_SPLINE_SURFACE(((0.988122504062135,0.988122504062135,0.988122504062135,
0.989520169850094,0.993884164197532),(0.988122504062136,0.988122504062136,
0.988122504062136,0.989520169850094,0.993884164197532)))
REPRESENTATION_ITEM('')
SURFACE()
);
#417=(
BOUNDED_SURFACE()
B_SPLINE_SURFACE(1,2,((#99584,#99585,#99586),(#99587,#99588,#99589)),
 .UNSPECIFIED.,.F.,.F.,.F.)
B_SPLINE_SURFACE_WITH_KNOTS((2,2),(3,3),(0.,0.289681084359922),(0.314840108491246,
0.332069149066804),.UNSPECIFIED.)
GEOMETRIC_REPRESENTATION_ITEM()
RATIONAL_B_SPLINE_SURFACE(((0.98789057959819,0.986774945528862,0.988576730109495),
(0.98789057959819,0.986774945528862,0.988576730109495)))
REPRESENTATION_ITEM('')
SURFACE()
);
#418=(
BOUNDED_SURFACE()
B_SPLINE_SURFACE(1,2,((#99598,#99599,#99600,#99601,#99602),(#99603,#99604,
#99605,#99606,#99607)),.UNSPECIFIED.,.F.,.F.,.F.)
B_SPLINE_SURFACE_WITH_KNOTS((2,2),(3,2,3),(0.,0.290405231151855),(0.400444645029575,
0.401042835325431,0.418415696246125),.UNSPECIFIED.)
GEOMETRIC_REPRESENTATION_ITEM()
RATIONAL_B_SPLINE_SURFACE(((0.988122504062136,0.988122504062136,0.988122504062136,
0.989520169850094,0.993884164197534),(0.988122504062136,0.988122504062136,
0.988122504062136,0.989520169850094,0.993884164197534)))
REPRESENTATION_ITEM('')
SURFACE()
);
#419=(
BOUNDED_SURFACE()
B_SPLINE_SURFACE(1,2,((#99609,#99610,#99611),(#99612,#99613,#99614)),
 .UNSPECIFIED.,.F.,.F.,.F.)
B_SPLINE_SURFACE_WITH_KNOTS((2,2),(3,3),(0.,0.289681084359918),(0.314840108491246,
0.332069149066807),.UNSPECIFIED.)
GEOMETRIC_REPRESENTATION_ITEM()
RATIONAL_B_SPLINE_SURFACE(((0.98789057959819,0.986774945528862,0.988576730109496),
(0.98789057959819,0.986774945528862,0.988576730109496)))
REPRESENTATION_ITEM('')
SURFACE()
);
#420=(
BOUNDED_SURFACE()
B_SPLINE_SURFACE(1,2,((#99623,#99624,#99625,#99626,#99627),(#99628,#99629,
#99630,#99631,#99632)),.UNSPECIFIED.,.F.,.F.,.F.)
B_SPLINE_SURFACE_WITH_KNOTS((2,2),(3,2,3),(0.,0.290405231144711),(0.400444645036177,
0.401042835325431,0.418415696246122),.UNSPECIFIED.)
GEOMETRIC_REPRESENTATION_ITEM()
RATIONAL_B_SPLINE_SURFACE(((0.988122504062135,0.988122504062135,0.988122504062135,
0.989520169850094,0.993884164197532),(0.988122504062135,0.988122504062135,
0.988122504062135,0.989520169850094,0.993884164197532)))
REPRESENTATION_ITEM('')
SURFACE()
);
#421=(
BOUNDED_SURFACE()
B_SPLINE_SURFACE(1,2,((#99634,#99635,#99636),(#99637,#99638,#99639)),
 .UNSPECIFIED.,.F.,.F.,.F.)
B_SPLINE_SURFACE_WITH_KNOTS((2,2),(3,3),(0.,0.289681084359923),(0.314840108491246,
0.332069149066806),.UNSPECIFIED.)
GEOMETRIC_REPRESENTATION_ITEM()
RATIONAL_B_SPLINE_SURFACE(((0.98789057959819,0.986774945528862,0.988576730109495),
(0.98789057959819,0.986774945528862,0.988576730109495)))
REPRESENTATION_ITEM('')
SURFACE()
);
#422=(
BOUNDED_SURFACE()
B_SPLINE_SURFACE(1,2,((#99648,#99649,#99650,#99651,#99652),(#99653,#99654,
#99655,#99656,#99657)),.UNSPECIFIED.,.F.,.F.,.F.)
B_SPLINE_SURFACE_WITH_KNOTS((2,2),(3,2,3),(0.,0.29040523112861),(0.400444645052479,
0.401042835325431,0.418415696246122),.UNSPECIFIED.)
GEOMETRIC_REPRESENTATION_ITEM()
RATIONAL_B_SPLINE_SURFACE(((0.988122504062135,0.988122504062135,0.988122504062135,
0.989520169850094,0.993884164197532),(0.988122504062135,0.988122504062135,
0.988122504062135,0.989520169850094,0.993884164197532)))
REPRESENTATION_ITEM('')
SURFACE()
);
#423=(
BOUNDED_SURFACE()
B_SPLINE_SURFACE(1,2,((#99659,#99660,#99661),(#99662,#99663,#99664)),
 .UNSPECIFIED.,.F.,.F.,.F.)
B_SPLINE_SURFACE_WITH_KNOTS((2,2),(3,3),(0.,0.289681084359918),(0.314840108491246,
0.332069149066804),.UNSPECIFIED.)
GEOMETRIC_REPRESENTATION_ITEM()
RATIONAL_B_SPLINE_SURFACE(((0.98789057959819,0.986774945528862,0.988576730109495),
(0.98789057959819,0.986774945528862,0.988576730109495)))
REPRESENTATION_ITEM('')
SURFACE()
);
#424=(
BOUNDED_SURFACE()
B_SPLINE_SURFACE(1,2,((#99673,#99674,#99675,#99676,#99677),(#99678,#99679,
#99680,#99681,#99682)),.UNSPECIFIED.,.F.,.F.,.F.)
B_SPLINE_SURFACE_WITH_KNOTS((2,2),(3,2,3),(0.,0.290405231116345),(0.400444645064969,
0.401042835325431,0.418415696246122),.UNSPECIFIED.)
GEOMETRIC_REPRESENTATION_ITEM()
RATIONAL_B_SPLINE_SURFACE(((0.988122504062136,0.988122504062136,0.988122504062136,
0.989520169850094,0.993884164197532),(0.988122504062136,0.988122504062136,
0.988122504062136,0.989520169850094,0.993884164197532)))
REPRESENTATION_ITEM('')
SURFACE()
);
#425=(
BOUNDED_SURFACE()
B_SPLINE_SURFACE(1,2,((#99684,#99685,#99686),(#99687,#99688,#99689)),
 .UNSPECIFIED.,.F.,.F.,.F.)
B_SPLINE_SURFACE_WITH_KNOTS((2,2),(3,3),(0.,0.289681084359931),(0.314840108491246,
0.332069149066804),.UNSPECIFIED.)
GEOMETRIC_REPRESENTATION_ITEM()
RATIONAL_B_SPLINE_SURFACE(((0.98789057959819,0.986774945528862,0.988576730109495),
(0.98789057959819,0.986774945528862,0.988576730109495)))
REPRESENTATION_ITEM('')
SURFACE()
);
#426=(
BOUNDED_SURFACE()
B_SPLINE_SURFACE(1,2,((#99691,#99692,#99693),(#99694,#99695,#99696)),
 .UNSPECIFIED.,.F.,.F.,.F.)
B_SPLINE_SURFACE_WITH_KNOTS((2,2),(3,3),(0.,0.289807040992008),(0.366820493751253,
0.384035903515169),.UNSPECIFIED.)
GEOMETRIC_REPRESENTATION_ITEM()
RATIONAL_B_SPLINE_SURFACE(((0.994126602224873,0.989721266390694,0.988228734781998),
(0.994126602224873,0.989721266390694,0.988228734781998)))
REPRESENTATION_ITEM('')
SURFACE()
);
#427=(
BOUNDED_SURFACE()
B_SPLINE_SURFACE(1,2,((#99725,#99726,#99727,#99728,#99729,#99730,#99731),
(#99732,#99733,#99734,#99735,#99736,#99737,#99738)),.UNSPECIFIED.,.F.,.F.,
 .F.)
B_SPLINE_SURFACE_WITH_KNOTS((2,2),(3,2,2,3),(0.,0.289681084359932),(0.34926499147441,
0.357142857142857,0.366820493751254,0.366996048774023),.UNSPECIFIED.)
GEOMETRIC_REPRESENTATION_ITEM()
RATIONAL_B_SPLINE_SURFACE(((0.995079542144874,0.997234796441972,1.,0.996603060231146,
0.994126602224873,0.994126602224873,0.994126602224873),(0.995079542144874,
0.997234796441972,1.,0.996603060231146,0.994126602224873,0.994126602224873,
0.994126602224873)))
REPRESENTATION_ITEM('')
SURFACE()
);
#428=(
BOUNDED_SURFACE()
B_SPLINE_SURFACE(1,2,((#99740,#99741,#99742),(#99743,#99744,#99745)),
 .UNSPECIFIED.,.F.,.F.,.F.)
B_SPLINE_SURFACE_WITH_KNOTS((2,2),(3,3),(0.,0.289807040992861),(0.366820493751253,
0.384035903515169),.UNSPECIFIED.)
GEOMETRIC_REPRESENTATION_ITEM()
RATIONAL_B_SPLINE_SURFACE(((0.994126602224873,0.989721266390694,0.988228734781998),
(0.994126602224873,0.989721266390694,0.988228734781998)))
REPRESENTATION_ITEM('')
SURFACE()
);
#429=(
BOUNDED_SURFACE()
B_SPLINE_SURFACE(1,2,((#99774,#99775,#99776,#99777,#99778,#99779,#99780),
(#99781,#99782,#99783,#99784,#99785,#99786,#99787)),.UNSPECIFIED.,.F.,.F.,
 .F.)
B_SPLINE_SURFACE_WITH_KNOTS((2,2),(3,2,2,3),(0.,0.289681084360137),(0.34926499147441,
0.357142857142857,0.366820493751255,0.366996048774024),.UNSPECIFIED.)
GEOMETRIC_REPRESENTATION_ITEM()
RATIONAL_B_SPLINE_SURFACE(((0.995079542144874,0.997234796441972,1.,0.996603060231146,
0.994126602224872,0.994126602224872,0.994126602224872),(0.995079542144874,
0.997234796441972,1.,0.996603060231146,0.994126602224872,0.994126602224872,
0.994126602224872)))
REPRESENTATION_ITEM('')
SURFACE()
);
#430=(
BOUNDED_SURFACE()
B_SPLINE_SURFACE(1,2,((#99789,#99790,#99791),(#99792,#99793,#99794)),
 .UNSPECIFIED.,.F.,.F.,.F.)
B_SPLINE_SURFACE_WITH_KNOTS((2,2),(3,3),(0.,0.289807040992678),(0.366820493751253,
0.384035903515169),.UNSPECIFIED.)
GEOMETRIC_REPRESENTATION_ITEM()
RATIONAL_B_SPLINE_SURFACE(((0.994126602224873,0.989721266390694,0.988228734781998),
(0.994126602224873,0.989721266390694,0.988228734781998)))
REPRESENTATION_ITEM('')
SURFACE()
);
#431=(
BOUNDED_SURFACE()
B_SPLINE_SURFACE(1,2,((#99823,#99824,#99825,#99826,#99827,#99828,#99829),
(#99830,#99831,#99832,#99833,#99834,#99835,#99836)),.UNSPECIFIED.,.F.,.F.,
 .F.)
B_SPLINE_SURFACE_WITH_KNOTS((2,2),(3,2,2,3),(0.,0.289681084360355),(0.34926499147441,
0.357142857142857,0.366820493751254,0.366996048774023),.UNSPECIFIED.)
GEOMETRIC_REPRESENTATION_ITEM()
RATIONAL_B_SPLINE_SURFACE(((0.995079542144874,0.997234796441972,1.,0.996603060231146,
0.994126602224873,0.994126602224873,0.994126602224873),(0.995079542144874,
0.997234796441972,1.,0.996603060231146,0.994126602224873,0.994126602224873,
0.994126602224873)))
REPRESENTATION_ITEM('')
SURFACE()
);
#432=(
BOUNDED_SURFACE()
B_SPLINE_SURFACE(1,2,((#99838,#99839,#99840),(#99841,#99842,#99843)),
 .UNSPECIFIED.,.F.,.F.,.F.)
B_SPLINE_SURFACE_WITH_KNOTS((2,2),(3,3),(0.,0.289807040992652),(0.366820493751253,
0.384035903515169),.UNSPECIFIED.)
GEOMETRIC_REPRESENTATION_ITEM()
RATIONAL_B_SPLINE_SURFACE(((0.994126602224873,0.989721266390694,0.988228734781998),
(0.994126602224873,0.989721266390694,0.988228734781998)))
REPRESENTATION_ITEM('')
SURFACE()
);
#433=(
BOUNDED_SURFACE()
B_SPLINE_SURFACE(1,2,((#99872,#99873,#99874,#99875,#99876,#99877,#99878),
(#99879,#99880,#99881,#99882,#99883,#99884,#99885)),.UNSPECIFIED.,.F.,.F.,
 .F.)
B_SPLINE_SURFACE_WITH_KNOTS((2,2),(3,2,2,3),(0.,0.289681084359916),(0.34926499147441,
0.357142857142857,0.366820493751254,0.366996048774023),.UNSPECIFIED.)
GEOMETRIC_REPRESENTATION_ITEM()
RATIONAL_B_SPLINE_SURFACE(((0.995079542144874,0.997234796441972,1.,0.996603060231146,
0.994126602224873,0.994126602224873,0.994126602224873),(0.995079542144874,
0.997234796441972,1.,0.996603060231146,0.994126602224873,0.994126602224873,
0.994126602224873)))
REPRESENTATION_ITEM('')
SURFACE()
);
#434=(
BOUNDED_SURFACE()
B_SPLINE_SURFACE(1,2,((#99887,#99888,#99889),(#99890,#99891,#99892)),
 .UNSPECIFIED.,.F.,.F.,.F.)
B_SPLINE_SURFACE_WITH_KNOTS((2,2),(3,3),(0.,0.289807040992801),(0.366820493751253,
0.384035903515169),.UNSPECIFIED.)
GEOMETRIC_REPRESENTATION_ITEM()
RATIONAL_B_SPLINE_SURFACE(((0.994126602224873,0.989721266390694,0.988228734781998),
(0.994126602224873,0.989721266390694,0.988228734781998)))
REPRESENTATION_ITEM('')
SURFACE()
);
#435=(
BOUNDED_SURFACE()
B_SPLINE_SURFACE(1,2,((#99921,#99922,#99923,#99924,#99925,#99926,#99927),
(#99928,#99929,#99930,#99931,#99932,#99933,#99934)),.UNSPECIFIED.,.F.,.F.,
 .F.)
B_SPLINE_SURFACE_WITH_KNOTS((2,2),(3,2,2,3),(0.,0.289681084359922),(0.34926499147441,
0.357142857142857,0.366820493751254,0.366996048774023),.UNSPECIFIED.)
GEOMETRIC_REPRESENTATION_ITEM()
RATIONAL_B_SPLINE_SURFACE(((0.995079542144874,0.997234796441972,1.,0.996603060231146,
0.994126602224873,0.994126602224873,0.994126602224873),(0.995079542144874,
0.997234796441972,1.,0.996603060231146,0.994126602224873,0.994126602224873,
0.994126602224873)))
REPRESENTATION_ITEM('')
SURFACE()
);
#436=(
BOUNDED_SURFACE()
B_SPLINE_SURFACE(1,2,((#99936,#99937,#99938),(#99939,#99940,#99941)),
 .UNSPECIFIED.,.F.,.F.,.F.)
B_SPLINE_SURFACE_WITH_KNOTS((2,2),(3,3),(0.,0.289807040992325),(0.366820493751253,
0.384035903515169),.UNSPECIFIED.)
GEOMETRIC_REPRESENTATION_ITEM()
RATIONAL_B_SPLINE_SURFACE(((0.994126602224873,0.989721266390694,0.988228734781998),
(0.994126602224873,0.989721266390694,0.988228734781998)))
REPRESENTATION_ITEM('')
SURFACE()
);
#437=(
BOUNDED_SURFACE()
B_SPLINE_SURFACE(1,2,((#99970,#99971,#99972,#99973,#99974,#99975,#99976),
(#99977,#99978,#99979,#99980,#99981,#99982,#99983)),.UNSPECIFIED.,.F.,.F.,
 .F.)
B_SPLINE_SURFACE_WITH_KNOTS((2,2),(3,2,2,3),(0.,0.289681084360531),(0.3492649914744,
0.357142857142857,0.366820493751254,0.366996048774023),.UNSPECIFIED.)
GEOMETRIC_REPRESENTATION_ITEM()
RATIONAL_B_SPLINE_SURFACE(((0.995079542144869,0.997234796441969,1.,0.996603060231146,
0.994126602224873,0.994126602224873,0.994126602224873),(0.995079542144869,
0.997234796441969,1.,0.996603060231146,0.994126602224873,0.994126602224873,
0.994126602224873)))
REPRESENTATION_ITEM('')
SURFACE()
);
#438=(
BOUNDED_SURFACE()
B_SPLINE_SURFACE(1,2,((#99985,#99986,#99987),(#99988,#99989,#99990)),
 .UNSPECIFIED.,.F.,.F.,.F.)
B_SPLINE_SURFACE_WITH_KNOTS((2,2),(3,3),(0.,0.289807040992452),(0.366820493751253,
0.384035903515169),.UNSPECIFIED.)
GEOMETRIC_REPRESENTATION_ITEM()
RATIONAL_B_SPLINE_SURFACE(((0.994126602224873,0.989721266390694,0.988228734781998),
(0.994126602224873,0.989721266390694,0.988228734781998)))
REPRESENTATION_ITEM('')
SURFACE()
);
#439=(
BOUNDED_SURFACE()
B_SPLINE_SURFACE(1,2,((#100019,#100020,#100021,#100022,#100023,#100024,
#100025),(#100026,#100027,#100028,#100029,#100030,#100031,#100032)),
 .UNSPECIFIED.,.F.,.F.,.F.)
B_SPLINE_SURFACE_WITH_KNOTS((2,2),(3,2,2,3),(0.,0.289681084359929),(0.34926499147441,
0.357142857142857,0.366820493751254,0.366996048774023),.UNSPECIFIED.)
GEOMETRIC_REPRESENTATION_ITEM()
RATIONAL_B_SPLINE_SURFACE(((0.995079542144874,0.997234796441972,1.,0.996603060231146,
0.994126602224873,0.994126602224873,0.994126602224873),(0.995079542144874,
0.997234796441972,1.,0.996603060231146,0.994126602224873,0.994126602224873,
0.994126602224873)))
REPRESENTATION_ITEM('')
SURFACE()
);
#440=(
BOUNDED_SURFACE()
B_SPLINE_SURFACE(1,2,((#100034,#100035,#100036),(#100037,#100038,#100039)),
 .UNSPECIFIED.,.F.,.F.,.F.)
B_SPLINE_SURFACE_WITH_KNOTS((2,2),(3,3),(0.,0.289807040992693),(0.366820493751253,
0.384035903515169),.UNSPECIFIED.)
GEOMETRIC_REPRESENTATION_ITEM()
RATIONAL_B_SPLINE_SURFACE(((0.994126602224873,0.989721266390694,0.988228734781998),
(0.994126602224873,0.989721266390694,0.988228734781998)))
REPRESENTATION_ITEM('')
SURFACE()
);
#441=(
BOUNDED_SURFACE()
B_SPLINE_SURFACE(1,2,((#100068,#100069,#100070,#100071,#100072,#100073,
#100074),(#100075,#100076,#100077,#100078,#100079,#100080,#100081)),
 .UNSPECIFIED.,.F.,.F.,.F.)
B_SPLINE_SURFACE_WITH_KNOTS((2,2),(3,2,2,3),(-0.000247526158567017,0.289681084359924),
(0.349122170180809,0.357142857142857,0.366820493751254,0.367068020353655),
 .UNSPECIFIED.)
GEOMETRIC_REPRESENTATION_ITEM()
RATIONAL_B_SPLINE_SURFACE(((0.995001595513646,0.997184664849756,1.,0.996603060231146,
0.994126602224873,0.994126602224873,0.994126602224873),(0.995001595513646,
0.997184664849755,1.,0.996603060231146,0.994126602224873,0.994126602224873,
0.994126602224873)))
REPRESENTATION_ITEM('')
SURFACE()
);
#442=(
BOUNDED_SURFACE()
B_SPLINE_SURFACE(1,2,((#100083,#100084,#100085),(#100086,#100087,#100088)),
 .UNSPECIFIED.,.F.,.F.,.F.)
B_SPLINE_SURFACE_WITH_KNOTS((2,2),(3,3),(0.,0.289807040992909),(0.366820493751253,
0.384035903515169),.UNSPECIFIED.)
GEOMETRIC_REPRESENTATION_ITEM()
RATIONAL_B_SPLINE_SURFACE(((0.994126602224873,0.989721266390694,0.988228734781998),
(0.994126602224873,0.989721266390694,0.988228734781998)))
REPRESENTATION_ITEM('')
SURFACE()
);
#443=(
BOUNDED_SURFACE()
B_SPLINE_SURFACE(1,2,((#100117,#100118,#100119,#100120,#100121,#100122,
#100123),(#100124,#100125,#100126,#100127,#100128,#100129,#100130)),
 .UNSPECIFIED.,.F.,.F.,.F.)
B_SPLINE_SURFACE_WITH_KNOTS((2,2),(3,2,2,3),(0.,0.28968108435992),(0.34926499147441,
0.357142857142857,0.366820493751254,0.366996048774023),.UNSPECIFIED.)
GEOMETRIC_REPRESENTATION_ITEM()
RATIONAL_B_SPLINE_SURFACE(((0.995079542144874,0.997234796441972,1.,0.996603060231146,
0.994126602224873,0.994126602224873,0.994126602224873),(0.995079542144874,
0.997234796441972,1.,0.996603060231146,0.994126602224873,0.994126602224873,
0.994126602224873)))
REPRESENTATION_ITEM('')
SURFACE()
);
#444=(
BOUNDED_SURFACE()
B_SPLINE_SURFACE(1,2,((#100132,#100133,#100134),(#100135,#100136,#100137)),
 .UNSPECIFIED.,.F.,.F.,.F.)
B_SPLINE_SURFACE_WITH_KNOTS((2,2),(3,3),(0.,0.28980704099176),(0.366820493751253,
0.384035903515169),.UNSPECIFIED.)
GEOMETRIC_REPRESENTATION_ITEM()
RATIONAL_B_SPLINE_SURFACE(((0.994126602224873,0.989721266390694,0.988228734781998),
(0.994126602224873,0.989721266390694,0.988228734781998)))
REPRESENTATION_ITEM('')
SURFACE()
);
#445=(
BOUNDED_SURFACE()
B_SPLINE_SURFACE(1,2,((#100166,#100167,#100168,#100169,#100170,#100171,
#100172),(#100173,#100174,#100175,#100176,#100177,#100178,#100179)),
 .UNSPECIFIED.,.F.,.F.,.F.)
B_SPLINE_SURFACE_WITH_KNOTS((2,2),(3,2,2,3),(0.,0.289681084359916),(0.34926499147441,
0.357142857142857,0.366820493751263,0.366996048774032),.UNSPECIFIED.)
GEOMETRIC_REPRESENTATION_ITEM()
RATIONAL_B_SPLINE_SURFACE(((0.995079542144874,0.997234796441972,1.,0.996603060231143,
0.994126602224868,0.994126602224868,0.994126602224868),(0.995079542144874,
0.997234796441972,1.,0.996603060231143,0.994126602224868,0.994126602224868,
0.994126602224868)))
REPRESENTATION_ITEM('')
SURFACE()
);
#446=(
BOUNDED_SURFACE()
B_SPLINE_SURFACE(1,2,((#100181,#100182,#100183),(#100184,#100185,#100186)),
 .UNSPECIFIED.,.F.,.F.,.F.)
B_SPLINE_SURFACE_WITH_KNOTS((2,2),(3,3),(0.,0.289807040991715),(0.366820493751253,
0.384035903515169),.UNSPECIFIED.)
GEOMETRIC_REPRESENTATION_ITEM()
RATIONAL_B_SPLINE_SURFACE(((0.994126602224873,0.989721266390694,0.988228734781998),
(0.994126602224873,0.989721266390694,0.988228734781998)))
REPRESENTATION_ITEM('')
SURFACE()
);
#447=(
BOUNDED_SURFACE()
B_SPLINE_SURFACE(1,2,((#100215,#100216,#100217,#100218,#100219,#100220,
#100221),(#100222,#100223,#100224,#100225,#100226,#100227,#100228)),
 .UNSPECIFIED.,.F.,.F.,.F.)
B_SPLINE_SURFACE_WITH_KNOTS((2,2),(3,2,2,3),(0.,0.289681084359924),(0.34926499147441,
0.357142857142857,0.366820493751263,0.366996048774032),.UNSPECIFIED.)
GEOMETRIC_REPRESENTATION_ITEM()
RATIONAL_B_SPLINE_SURFACE(((0.995079542144874,0.997234796441972,1.,0.996603060231143,
0.994126602224868,0.994126602224868,0.994126602224868),(0.995079542144874,
0.997234796441972,1.,0.996603060231143,0.994126602224868,0.994126602224868,
0.994126602224868)))
REPRESENTATION_ITEM('')
SURFACE()
);
#448=(
BOUNDED_SURFACE()
B_SPLINE_SURFACE(1,2,((#100230,#100231,#100232),(#100233,#100234,#100235)),
 .UNSPECIFIED.,.F.,.F.,.F.)
B_SPLINE_SURFACE_WITH_KNOTS((2,2),(3,3),(0.,0.289807040991572),(0.366820493751253,
0.384035903515169),.UNSPECIFIED.)
GEOMETRIC_REPRESENTATION_ITEM()
RATIONAL_B_SPLINE_SURFACE(((0.994126602224873,0.989721266390694,0.988228734781998),
(0.994126602224873,0.989721266390694,0.988228734781998)))
REPRESENTATION_ITEM('')
SURFACE()
);
#449=(
BOUNDED_SURFACE()
B_SPLINE_SURFACE(1,2,((#100264,#100265,#100266,#100267,#100268,#100269,
#100270),(#100271,#100272,#100273,#100274,#100275,#100276,#100277)),
 .UNSPECIFIED.,.F.,.F.,.F.)
B_SPLINE_SURFACE_WITH_KNOTS((2,2),(3,2,2,3),(0.,0.289681084360495),(0.34926499147441,
0.357142857142857,0.366820493751263,0.366996048774032),.UNSPECIFIED.)
GEOMETRIC_REPRESENTATION_ITEM()
RATIONAL_B_SPLINE_SURFACE(((0.995079542144874,0.997234796441972,1.,0.996603060231143,
0.994126602224868,0.994126602224868,0.994126602224868),(0.995079542144874,
0.997234796441972,1.,0.996603060231143,0.994126602224868,0.994126602224868,
0.994126602224868)))
REPRESENTATION_ITEM('')
SURFACE()
);
#450=(
BOUNDED_SURFACE()
B_SPLINE_SURFACE(1,2,((#100279,#100280,#100281),(#100282,#100283,#100284)),
 .UNSPECIFIED.,.F.,.F.,.F.)
B_SPLINE_SURFACE_WITH_KNOTS((2,2),(3,3),(0.,0.289807040991562),(0.366820493751253,
0.384035903515169),.UNSPECIFIED.)
GEOMETRIC_REPRESENTATION_ITEM()
RATIONAL_B_SPLINE_SURFACE(((0.994126602224873,0.989721266390694,0.988228734781998),
(0.994126602224873,0.989721266390694,0.988228734781998)))
REPRESENTATION_ITEM('')
SURFACE()
);
#451=(
BOUNDED_SURFACE()
B_SPLINE_SURFACE(1,2,((#100313,#100314,#100315,#100316,#100317,#100318,
#100319),(#100320,#100321,#100322,#100323,#100324,#100325,#100326)),
 .UNSPECIFIED.,.F.,.F.,.F.)
B_SPLINE_SURFACE_WITH_KNOTS((2,2),(3,2,2,3),(-0.000247526265803812,0.289681084359927),
(0.349122170275924,0.357142857142857,0.366820493751263,0.367068020291019),
 .UNSPECIFIED.)
GEOMETRIC_REPRESENTATION_ITEM()
RATIONAL_B_SPLINE_SURFACE(((0.995001595565422,0.997184664883142,1.,0.996603060231143,
0.994126602224868,0.994126602224868,0.994126602224868),(0.995001595565422,
0.997184664883142,1.,0.996603060231143,0.994126602224868,0.994126602224868,
0.994126602224868)))
REPRESENTATION_ITEM('')
SURFACE()
);
#452=(
BOUNDED_SURFACE()
B_SPLINE_SURFACE(1,2,((#100328,#100329,#100330),(#100331,#100332,#100333)),
 .UNSPECIFIED.,.F.,.F.,.F.)
B_SPLINE_SURFACE_WITH_KNOTS((2,2),(3,3),(0.,0.289807040991566),(0.366820493751253,
0.384035903515169),.UNSPECIFIED.)
GEOMETRIC_REPRESENTATION_ITEM()
RATIONAL_B_SPLINE_SURFACE(((0.994126602224873,0.989721266390694,0.988228734781998),
(0.994126602224873,0.989721266390694,0.988228734781998)))
REPRESENTATION_ITEM('')
SURFACE()
);
#453=(
BOUNDED_SURFACE()
B_SPLINE_SURFACE(1,2,((#100362,#100363,#100364,#100365,#100366,#100367,
#100368),(#100369,#100370,#100371,#100372,#100373,#100374,#100375)),
 .UNSPECIFIED.,.F.,.F.,.F.)
B_SPLINE_SURFACE_WITH_KNOTS((2,2),(3,2,2,3),(-0.000247526295446904,0.289681084359932),
(0.349122170227907,0.357142857142857,0.366820493751263,0.367068020309611),
 .UNSPECIFIED.)
GEOMETRIC_REPRESENTATION_ITEM()
RATIONAL_B_SPLINE_SURFACE(((0.995001595539283,0.997184664866287,1.,0.996603060231143,
0.994126602224868,0.994126602224868,0.994126602224868),(0.995001595539283,
0.997184664866287,1.,0.996603060231143,0.994126602224868,0.994126602224868,
0.994126602224868)))
REPRESENTATION_ITEM('')
SURFACE()
);
#454=(
BOUNDED_SURFACE()
B_SPLINE_SURFACE(1,2,((#100377,#100378,#100379),(#100380,#100381,#100382)),
 .UNSPECIFIED.,.F.,.F.,.F.)
B_SPLINE_SURFACE_WITH_KNOTS((2,2),(3,3),(0.,0.289807040991565),(0.366820493751253,
0.384035903515169),.UNSPECIFIED.)
GEOMETRIC_REPRESENTATION_ITEM()
RATIONAL_B_SPLINE_SURFACE(((0.994126602224873,0.989721266390694,0.988228734781998),
(0.994126602224873,0.989721266390694,0.988228734781998)))
REPRESENTATION_ITEM('')
SURFACE()
);
#455=(
BOUNDED_SURFACE()
B_SPLINE_SURFACE(1,2,((#100390,#100391,#100392,#100393,#100394,#100395,
#100396),(#100397,#100398,#100399,#100400,#100401,#100402,#100403)),
 .UNSPECIFIED.,.F.,.F.,.F.)
B_SPLINE_SURFACE_WITH_KNOTS((2,2),(3,2,2,3),(0.,0.289681084359918),(0.34926499147441,
0.357142857142857,0.366820493751263,0.366996048774032),.UNSPECIFIED.)
GEOMETRIC_REPRESENTATION_ITEM()
RATIONAL_B_SPLINE_SURFACE(((0.995079542144874,0.997234796441972,1.,0.996603060231143,
0.994126602224868,0.994126602224868,0.994126602224868),(0.995079542144874,
0.997234796441972,1.,0.996603060231143,0.994126602224868,0.994126602224868,
0.994126602224868)))
REPRESENTATION_ITEM('')
SURFACE()
);
#456=(
BOUNDED_SURFACE()
B_SPLINE_SURFACE(1,2,((#100405,#100406,#100407),(#100408,#100409,#100410)),
 .UNSPECIFIED.,.F.,.F.,.F.)
B_SPLINE_SURFACE_WITH_KNOTS((2,2),(3,3),(0.,0.289807040991565),(0.366820493751253,
0.384035903515169),.UNSPECIFIED.)
GEOMETRIC_REPRESENTATION_ITEM()
RATIONAL_B_SPLINE_SURFACE(((0.994126602224873,0.989721266390694,0.988228734781998),
(0.994126602224873,0.989721266390694,0.988228734781998)))
REPRESENTATION_ITEM('')
SURFACE()
);
#457=(
BOUNDED_SURFACE()
B_SPLINE_SURFACE(1,2,((#100439,#100440,#100441,#100442,#100443,#100444,
#100445),(#100446,#100447,#100448,#100449,#100450,#100451,#100452)),
 .UNSPECIFIED.,.F.,.F.,.F.)
B_SPLINE_SURFACE_WITH_KNOTS((2,2),(3,2,2,3),(0.,0.289681084359923),(0.34926499147441,
0.357142857142857,0.366820493751263,0.366996048774032),.UNSPECIFIED.)
GEOMETRIC_REPRESENTATION_ITEM()
RATIONAL_B_SPLINE_SURFACE(((0.995079542144874,0.997234796441972,1.,0.996603060231143,
0.994126602224868,0.994126602224868,0.994126602224868),(0.995079542144874,
0.997234796441972,1.,0.996603060231143,0.994126602224868,0.994126602224868,
0.994126602224868)))
REPRESENTATION_ITEM('')
SURFACE()
);
#458=(
BOUNDED_SURFACE()
B_SPLINE_SURFACE(1,2,((#100454,#100455,#100456),(#100457,#100458,#100459)),
 .UNSPECIFIED.,.F.,.F.,.F.)
B_SPLINE_SURFACE_WITH_KNOTS((2,2),(3,3),(0.,0.289807040991669),(0.366820493751253,
0.384035903515169),.UNSPECIFIED.)
GEOMETRIC_REPRESENTATION_ITEM()
RATIONAL_B_SPLINE_SURFACE(((0.994126602224873,0.989721266390694,0.988228734781998),
(0.994126602224873,0.989721266390694,0.988228734781998)))
REPRESENTATION_ITEM('')
SURFACE()
);
#459=(
BOUNDED_SURFACE()
B_SPLINE_SURFACE(1,2,((#100488,#100489,#100490,#100491,#100492,#100493,
#100494),(#100495,#100496,#100497,#100498,#100499,#100500,#100501)),
 .UNSPECIFIED.,.F.,.F.,.F.)
B_SPLINE_SURFACE_WITH_KNOTS((2,2),(3,2,2,3),(-0.00024752625948705,0.289681084359921),
(0.349122170220907,0.357142857142857,0.366820493751263,0.367068020290794),
 .UNSPECIFIED.)
GEOMETRIC_REPRESENTATION_ITEM()
RATIONAL_B_SPLINE_SURFACE(((0.995001595535473,0.99718466486383,1.,0.996603060231143,
0.994126602224868,0.994126602224868,0.994126602224868),(0.995001595535473,
0.99718466486383,1.,0.996603060231143,0.994126602224868,0.994126602224868,
0.994126602224868)))
REPRESENTATION_ITEM('')
SURFACE()
);
#460=(
BOUNDED_SURFACE()
B_SPLINE_SURFACE(1,2,((#100503,#100504,#100505),(#100506,#100507,#100508)),
 .UNSPECIFIED.,.F.,.F.,.F.)
B_SPLINE_SURFACE_WITH_KNOTS((2,2),(3,3),(0.,0.289807040992969),(0.366820493751253,
0.384035903515169),.UNSPECIFIED.)
GEOMETRIC_REPRESENTATION_ITEM()
RATIONAL_B_SPLINE_SURFACE(((0.994126602224873,0.989721266390694,0.988228734781998),
(0.994126602224873,0.989721266390694,0.988228734781998)))
REPRESENTATION_ITEM('')
SURFACE()
);
#461=(
BOUNDED_SURFACE()
B_SPLINE_SURFACE(1,2,((#100537,#100538,#100539,#100540,#100541,#100542,
#100543),(#100544,#100545,#100546,#100547,#100548,#100549,#100550)),
 .UNSPECIFIED.,.F.,.F.,.F.)
B_SPLINE_SURFACE_WITH_KNOTS((2,2),(3,2,2,3),(0.,0.28968108435992),(0.34926499147441,
0.357142857142857,0.366820493751263,0.366996048774032),.UNSPECIFIED.)
GEOMETRIC_REPRESENTATION_ITEM()
RATIONAL_B_SPLINE_SURFACE(((0.995079542144874,0.997234796441972,1.,0.996603060231143,
0.994126602224868,0.994126602224868,0.994126602224868),(0.995079542144874,
0.997234796441972,1.,0.996603060231143,0.994126602224868,0.994126602224868,
0.994126602224868)))
REPRESENTATION_ITEM('')
SURFACE()
);
#462=(
BOUNDED_SURFACE()
B_SPLINE_SURFACE(1,2,((#100552,#100553,#100554),(#100555,#100556,#100557)),
 .UNSPECIFIED.,.F.,.F.,.F.)
B_SPLINE_SURFACE_WITH_KNOTS((2,2),(3,3),(0.,0.289807040991813),(0.366820493751013,
0.384035903515171),.UNSPECIFIED.)
GEOMETRIC_REPRESENTATION_ITEM()
RATIONAL_B_SPLINE_SURFACE(((0.994126602224996,0.989721266390715,0.988228734781998),
(0.994126602224996,0.989721266390715,0.988228734781998)))
REPRESENTATION_ITEM('')
SURFACE()
);
#463=(
BOUNDED_SURFACE()
B_SPLINE_SURFACE(1,2,((#100586,#100587,#100588,#100589,#100590,#100591,
#100592),(#100593,#100594,#100595,#100596,#100597,#100598,#100599)),
 .UNSPECIFIED.,.F.,.F.,.F.)
B_SPLINE_SURFACE_WITH_KNOTS((2,2),(3,2,2,3),(0.,0.289681084359919),(0.34926499147441,
0.357142857142857,0.366820493751263,0.366996048774032),.UNSPECIFIED.)
GEOMETRIC_REPRESENTATION_ITEM()
RATIONAL_B_SPLINE_SURFACE(((0.995079542144874,0.997234796441972,1.,0.996603060231143,
0.994126602224868,0.994126602224868,0.994126602224868),(0.995079542144874,
0.997234796441972,1.,0.996603060231143,0.994126602224868,0.994126602224868,
0.994126602224868)))
REPRESENTATION_ITEM('')
SURFACE()
);
#464=(
BOUNDED_SURFACE()
B_SPLINE_SURFACE(1,2,((#100601,#100602,#100603),(#100604,#100605,#100606)),
 .UNSPECIFIED.,.F.,.F.,.F.)
B_SPLINE_SURFACE_WITH_KNOTS((2,2),(3,3),(0.,0.289807040991562),(0.366820493751253,
0.384035903515169),.UNSPECIFIED.)
GEOMETRIC_REPRESENTATION_ITEM()
RATIONAL_B_SPLINE_SURFACE(((0.994126602224873,0.989721266390694,0.988228734781998),
(0.994126602224873,0.989721266390694,0.988228734781998)))
REPRESENTATION_ITEM('')
SURFACE()
);
#465=(
BOUNDED_SURFACE()
B_SPLINE_SURFACE(1,2,((#100635,#100636,#100637,#100638,#100639,#100640,
#100641),(#100642,#100643,#100644,#100645,#100646,#100647,#100648)),
 .UNSPECIFIED.,.F.,.F.,.F.)
B_SPLINE_SURFACE_WITH_KNOTS((2,2),(3,2,2,3),(0.,0.289681084359922),(0.34926499147441,
0.357142857142857,0.366820493751263,0.366996048774032),.UNSPECIFIED.)
GEOMETRIC_REPRESENTATION_ITEM()
RATIONAL_B_SPLINE_SURFACE(((0.995079542144874,0.997234796441972,1.,0.996603060231143,
0.994126602224868,0.994126602224868,0.994126602224868),(0.995079542144874,
0.997234796441972,1.,0.996603060231143,0.994126602224868,0.994126602224868,
0.994126602224868)))
REPRESENTATION_ITEM('')
SURFACE()
);
#466=(
BOUNDED_SURFACE()
B_SPLINE_SURFACE(1,2,((#100650,#100651,#100652),(#100653,#100654,#100655)),
 .UNSPECIFIED.,.F.,.F.,.F.)
B_SPLINE_SURFACE_WITH_KNOTS((2,2),(3,3),(0.,0.289807040991559),(0.366820493751253,
0.384035903515169),.UNSPECIFIED.)
GEOMETRIC_REPRESENTATION_ITEM()
RATIONAL_B_SPLINE_SURFACE(((0.994126602224873,0.989721266390694,0.988228734781998),
(0.994126602224873,0.989721266390694,0.988228734781998)))
REPRESENTATION_ITEM('')
SURFACE()
);
#467=(
BOUNDED_SURFACE()
B_SPLINE_SURFACE(1,2,((#100684,#100685,#100686,#100687,#100688,#100689,
#100690),(#100691,#100692,#100693,#100694,#100695,#100696,#100697)),
 .UNSPECIFIED.,.F.,.F.,.F.)
B_SPLINE_SURFACE_WITH_KNOTS((2,2),(3,2,2,3),(0.,0.289681084359918),(0.34926499147441,
0.357142857142857,0.366820493751263,0.366996048774032),.UNSPECIFIED.)
GEOMETRIC_REPRESENTATION_ITEM()
RATIONAL_B_SPLINE_SURFACE(((0.995079542144874,0.997234796441972,1.,0.996603060231143,
0.994126602224868,0.994126602224868,0.994126602224868),(0.995079542144874,
0.997234796441972,1.,0.996603060231143,0.994126602224868,0.994126602224868,
0.994126602224868)))
REPRESENTATION_ITEM('')
SURFACE()
);
#468=(
BOUNDED_SURFACE()
B_SPLINE_SURFACE(1,2,((#100699,#100700,#100701),(#100702,#100703,#100704)),
 .UNSPECIFIED.,.F.,.F.,.F.)
B_SPLINE_SURFACE_WITH_KNOTS((2,2),(3,3),(0.,0.289807040991558),(0.366820493751253,
0.384035903515169),.UNSPECIFIED.)
GEOMETRIC_REPRESENTATION_ITEM()
RATIONAL_B_SPLINE_SURFACE(((0.994126602224873,0.989721266390694,0.988228734781998),
(0.994126602224873,0.989721266390694,0.988228734781998)))
REPRESENTATION_ITEM('')
SURFACE()
);
#469=(
BOUNDED_SURFACE()
B_SPLINE_SURFACE(1,2,((#100733,#100734,#100735,#100736,#100737,#100738,
#100739),(#100740,#100741,#100742,#100743,#100744,#100745,#100746)),
 .UNSPECIFIED.,.F.,.F.,.F.)
B_SPLINE_SURFACE_WITH_KNOTS((2,2),(3,2,2,3),(0.,0.289681084359919),(0.34926499147441,
0.357142857142857,0.366820493751263,0.366996048774032),.UNSPECIFIED.)
GEOMETRIC_REPRESENTATION_ITEM()
RATIONAL_B_SPLINE_SURFACE(((0.995079542144874,0.997234796441972,1.,0.996603060231143,
0.994126602224868,0.994126602224868,0.994126602224868),(0.995079542144874,
0.997234796441972,1.,0.996603060231143,0.994126602224868,0.994126602224868,
0.994126602224868)))
REPRESENTATION_ITEM('')
SURFACE()
);
#470=(
BOUNDED_SURFACE()
B_SPLINE_SURFACE(1,2,((#100748,#100749,#100750),(#100751,#100752,#100753)),
 .UNSPECIFIED.,.F.,.F.,.F.)
B_SPLINE_SURFACE_WITH_KNOTS((2,2),(3,3),(0.,0.289807040991561),(0.366820493751253,
0.384035903515169),.UNSPECIFIED.)
GEOMETRIC_REPRESENTATION_ITEM()
RATIONAL_B_SPLINE_SURFACE(((0.994126602224873,0.989721266390694,0.988228734781998),
(0.994126602224873,0.989721266390694,0.988228734781998)))
REPRESENTATION_ITEM('')
SURFACE()
);
#471=(
BOUNDED_SURFACE()
B_SPLINE_SURFACE(1,2,((#100782,#100783,#100784,#100785,#100786,#100787,
#100788),(#100789,#100790,#100791,#100792,#100793,#100794,#100795)),
 .UNSPECIFIED.,.F.,.F.,.F.)
B_SPLINE_SURFACE_WITH_KNOTS((2,2),(3,2,2,3),(-0.00024752608979232,0.289681084359921),
(0.349122170468145,0.357142857142857,0.366820493751263,0.367068020114749),
 .UNSPECIFIED.)
GEOMETRIC_REPRESENTATION_ITEM()
RATIONAL_B_SPLINE_SURFACE(((0.99500159567006,0.997184664950614,1.,0.996603060231143,
0.994126602224868,0.994126602224868,0.994126602224868),(0.99500159567006,
0.997184664950614,1.,0.996603060231143,0.994126602224868,0.994126602224868,
0.994126602224868)))
REPRESENTATION_ITEM('')
SURFACE()
);
#472=(
BOUNDED_SURFACE()
B_SPLINE_SURFACE(1,2,((#100797,#100798,#100799),(#100800,#100801,#100802)),
 .UNSPECIFIED.,.F.,.F.,.F.)
B_SPLINE_SURFACE_WITH_KNOTS((2,2),(3,3),(0.,0.289807040991564),(0.366820493751253,
0.384035903515169),.UNSPECIFIED.)
GEOMETRIC_REPRESENTATION_ITEM()
RATIONAL_B_SPLINE_SURFACE(((0.994126602224873,0.989721266390694,0.988228734781998),
(0.994126602224873,0.989721266390694,0.988228734781998)))
REPRESENTATION_ITEM('')
SURFACE()
);
#473=(
BOUNDED_SURFACE()
B_SPLINE_SURFACE(1,2,((#100831,#100832,#100833,#100834,#100835,#100836,
#100837),(#100838,#100839,#100840,#100841,#100842,#100843,#100844)),
 .UNSPECIFIED.,.F.,.F.,.F.)
B_SPLINE_SURFACE_WITH_KNOTS((2,2),(3,2,2,3),(-0.000247526153271754,0.289681084359918),
(0.349122170380219,0.357142857142857,0.366820493751264,0.367068020171335),
 .UNSPECIFIED.)
GEOMETRIC_REPRESENTATION_ITEM()
RATIONAL_B_SPLINE_SURFACE(((0.995001595622196,0.99718466491975,1.,0.996603060231143,
0.994126602224868,0.994126602224868,0.994126602224868),(0.995001595622196,
0.99718466491975,1.,0.996603060231143,0.994126602224868,0.994126602224868,
0.994126602224868)))
REPRESENTATION_ITEM('')
SURFACE()
);
#474=(
BOUNDED_SURFACE()
B_SPLINE_SURFACE(1,2,((#100846,#100847,#100848),(#100849,#100850,#100851)),
 .UNSPECIFIED.,.F.,.F.,.F.)
B_SPLINE_SURFACE_WITH_KNOTS((2,2),(3,3),(0.,0.289807040991555),(0.366820493751253,
0.384035903515169),.UNSPECIFIED.)
GEOMETRIC_REPRESENTATION_ITEM()
RATIONAL_B_SPLINE_SURFACE(((0.994126602224873,0.989721266390694,0.988228734781998),
(0.994126602224873,0.989721266390694,0.988228734781998)))
REPRESENTATION_ITEM('')
SURFACE()
);
#475=(
BOUNDED_SURFACE()
B_SPLINE_SURFACE(1,2,((#100862,#100863,#100864,#100865,#100866,#100867,
#100868),(#100869,#100870,#100871,#100872,#100873,#100874,#100875)),
 .UNSPECIFIED.,.F.,.F.,.F.)
B_SPLINE_SURFACE_WITH_KNOTS((2,2),(3,2,2,3),(-0.000247526181841607,0.289681084359921),
(0.349122170318008,0.357142857142857,0.366820493751254,0.367068020198209),
 .UNSPECIFIED.)
GEOMETRIC_REPRESENTATION_ITEM()
RATIONAL_B_SPLINE_SURFACE(((0.995001595588331,0.997184664897914,1.,0.996603060231146,
0.994126602224873,0.994126602224873,0.994126602224873),(0.995001595588331,
0.997184664897914,1.,0.996603060231146,0.994126602224873,0.994126602224873,
0.994126602224873)))
REPRESENTATION_ITEM('')
SURFACE()
);
#476=(
BOUNDED_SURFACE()
B_SPLINE_SURFACE(1,2,((#100895,#100896,#100897),(#100898,#100899,#100900)),
 .UNSPECIFIED.,.F.,.F.,.F.)
B_SPLINE_SURFACE_WITH_KNOTS((2,2),(3,3),(0.,0.289807040991564),(0.366820493751253,
0.384035903515168),.UNSPECIFIED.)
GEOMETRIC_REPRESENTATION_ITEM()
RATIONAL_B_SPLINE_SURFACE(((0.994126602224873,0.989721266390694,0.988228734781998),
(0.994126602224873,0.989721266390694,0.988228734781998)))
REPRESENTATION_ITEM('')
SURFACE()
);
#477=(
BOUNDED_SURFACE()
B_SPLINE_SURFACE(1,2,((#100929,#100930,#100931,#100932,#100933,#100934,
#100935),(#100936,#100937,#100938,#100939,#100940,#100941,#100942)),
 .UNSPECIFIED.,.F.,.F.,.F.)
B_SPLINE_SURFACE_WITH_KNOTS((2,2),(3,2,2,3),(0.,0.289681084360377),(0.349264991474411,
0.357142857142857,0.366820493751254,0.366996048774023),.UNSPECIFIED.)
GEOMETRIC_REPRESENTATION_ITEM()
RATIONAL_B_SPLINE_SURFACE(((0.995079542144875,0.997234796441973,1.,0.996603060231146,
0.994126602224873,0.994126602224873,0.994126602224873),(0.995079542144875,
0.997234796441973,1.,0.996603060231146,0.994126602224873,0.994126602224873,
0.994126602224873)))
REPRESENTATION_ITEM('')
SURFACE()
);
#478=(
BOUNDED_SURFACE()
B_SPLINE_SURFACE(1,2,((#100944,#100945,#100946),(#100947,#100948,#100949)),
 .UNSPECIFIED.,.F.,.F.,.F.)
B_SPLINE_SURFACE_WITH_KNOTS((2,2),(3,3),(0.,0.289807040992019),(0.366820493751234,
0.384035903515169),.UNSPECIFIED.)
GEOMETRIC_REPRESENTATION_ITEM()
RATIONAL_B_SPLINE_SURFACE(((0.994126602224883,0.989721266390696,0.988228734781998),
(0.994126602224883,0.989721266390696,0.988228734781998)))
REPRESENTATION_ITEM('')
SURFACE()
);
#479=(
BOUNDED_SURFACE()
B_SPLINE_SURFACE(1,2,((#100978,#100979,#100980,#100981,#100982,#100983,
#100984),(#100985,#100986,#100987,#100988,#100989,#100990,#100991)),
 .UNSPECIFIED.,.F.,.F.,.F.)
B_SPLINE_SURFACE_WITH_KNOTS((2,2),(3,2,2,3),(0.,0.289681084359932),(0.34926499147441,
0.357142857142857,0.366820493751254,0.366996048774023),.UNSPECIFIED.)
GEOMETRIC_REPRESENTATION_ITEM()
RATIONAL_B_SPLINE_SURFACE(((0.995079542144874,0.997234796441972,1.,0.996603060231146,
0.994126602224873,0.994126602224873,0.994126602224873),(0.995079542144874,
0.997234796441972,1.,0.996603060231146,0.994126602224873,0.994126602224873,
0.994126602224873)))
REPRESENTATION_ITEM('')
SURFACE()
);
#480=(
BOUNDED_SURFACE()
B_SPLINE_SURFACE(1,2,((#100993,#100994,#100995),(#100996,#100997,#100998)),
 .UNSPECIFIED.,.F.,.F.,.F.)
B_SPLINE_SURFACE_WITH_KNOTS((2,2),(3,3),(0.,0.289807040991983),(0.366820493751253,
0.384035903515169),.UNSPECIFIED.)
GEOMETRIC_REPRESENTATION_ITEM()
RATIONAL_B_SPLINE_SURFACE(((0.994126602224873,0.989721266390694,0.988228734781998),
(0.994126602224873,0.989721266390694,0.988228734781998)))
REPRESENTATION_ITEM('')
SURFACE()
);
#481=(
BOUNDED_SURFACE()
B_SPLINE_SURFACE(1,2,((#101027,#101028,#101029,#101030,#101031,#101032,
#101033),(#101034,#101035,#101036,#101037,#101038,#101039,#101040)),
 .UNSPECIFIED.,.F.,.F.,.F.)
B_SPLINE_SURFACE_WITH_KNOTS((2,2),(3,2,2,3),(0.,0.289681084359986),(0.34926499147441,
0.357142857142857,0.366820493751254,0.366996048774023),.UNSPECIFIED.)
GEOMETRIC_REPRESENTATION_ITEM()
RATIONAL_B_SPLINE_SURFACE(((0.995079542144874,0.997234796441972,1.,0.996603060231146,
0.994126602224873,0.994126602224873,0.994126602224873),(0.995079542144874,
0.997234796441972,1.,0.996603060231146,0.994126602224873,0.994126602224873,
0.994126602224873)))
REPRESENTATION_ITEM('')
SURFACE()
);
#482=(
BOUNDED_SURFACE()
B_SPLINE_SURFACE(1,2,((#101042,#101043,#101044),(#101045,#101046,#101047)),
 .UNSPECIFIED.,.F.,.F.,.F.)
B_SPLINE_SURFACE_WITH_KNOTS((2,2),(3,3),(0.,0.289807040991897),(0.366820493751253,
0.38403590351517),.UNSPECIFIED.)
GEOMETRIC_REPRESENTATION_ITEM()
RATIONAL_B_SPLINE_SURFACE(((0.994126602224873,0.989721266390694,0.988228734781998),
(0.994126602224873,0.989721266390694,0.988228734781998)))
REPRESENTATION_ITEM('')
SURFACE()
);
#483=(
BOUNDED_SURFACE()
B_SPLINE_SURFACE(1,2,((#101076,#101077,#101078,#101079,#101080,#101081,
#101082),(#101083,#101084,#101085,#101086,#101087,#101088,#101089)),
 .UNSPECIFIED.,.F.,.F.,.F.)
B_SPLINE_SURFACE_WITH_KNOTS((2,2),(3,2,2,3),(-0.00024752631999515,0.289681084359929),
(0.349122170227001,0.357142857142857,0.366820493751255,0.367068020367516),
 .UNSPECIFIED.)
GEOMETRIC_REPRESENTATION_ITEM()
RATIONAL_B_SPLINE_SURFACE(((0.995001595538792,0.99718466486597,1.,0.996603060231146,
0.994126602224872,0.994126602224872,0.994126602224872),(0.995001595538792,
0.99718466486597,1.,0.996603060231146,0.994126602224872,0.994126602224872,
0.994126602224872)))
REPRESENTATION_ITEM('')
SURFACE()
);
#484=(
BOUNDED_SURFACE()
B_SPLINE_SURFACE(1,2,((#101091,#101092,#101093,#101094,#101095),(#101096,
#101097,#101098,#101099,#101100)),.UNSPECIFIED.,.F.,.F.,.F.)
B_SPLINE_SURFACE_WITH_KNOTS((2,2),(3,2,3),(0.710318915639635,1.),(0.400939219852743,
0.418312080773435,0.418485809382642),.UNSPECIFIED.)
GEOMETRIC_REPRESENTATION_ITEM()
RATIONAL_B_SPLINE_SURFACE(((0.988105937622242,0.989485911589766,0.99383221411677,
0.99383221411677,0.99383221411677),(0.988105937622242,0.989485911589766,
0.99383221411677,0.99383221411677,0.99383221411677)))
REPRESENTATION_ITEM('')
SURFACE()
);
#485=(
BOUNDED_SURFACE()
B_SPLINE_SURFACE(1,2,((#101111,#101112,#101113,#101114,#101115),(#101116,
#101117,#101118,#101119,#101120)),.UNSPECIFIED.,.F.,.F.,.F.)
B_SPLINE_SURFACE_WITH_KNOTS((2,2),(3,2,3),(0.710192959005959,1.),(0.314770575782735,
0.314942866188491,0.332171906764074),.UNSPECIFIED.)
GEOMETRIC_REPRESENTATION_ITEM()
RATIONAL_B_SPLINE_SURFACE(((0.987877375613935,0.987877375613935,0.987877375613935,
0.986779141655833,0.988598326347701),(0.987877375613935,0.987877375613935,
0.987877375613935,0.986779141655833,0.988598326347701)))
REPRESENTATION_ITEM('')
SURFACE()
);
#486=(
BOUNDED_SURFACE()
B_SPLINE_SURFACE(1,2,((#101132,#101133,#101134,#101135,#101136),(#101137,
#101138,#101139,#101140,#101141)),.UNSPECIFIED.,.F.,.F.,.F.)
B_SPLINE_SURFACE_WITH_KNOTS((2,2),(3,2,3),(0.710318915639749,1.),(0.400939219852741,
0.418312080773612,0.41848580938282),.UNSPECIFIED.)
GEOMETRIC_REPRESENTATION_ITEM()
RATIONAL_B_SPLINE_SURFACE(((0.988105937622242,0.98948591158978,0.993832214116859,
0.993832214116859,0.993832214116859),(0.988105937622242,0.98948591158978,
0.993832214116859,0.993832214116859,0.993832214116859)))
REPRESENTATION_ITEM('')
SURFACE()
);
#487=(
BOUNDED_SURFACE()
B_SPLINE_SURFACE(1,2,((#101152,#101153,#101154,#101155,#101156),(#101157,
#101158,#101159,#101160,#101161)),.UNSPECIFIED.,.F.,.F.,.F.)
B_SPLINE_SURFACE_WITH_KNOTS((2,2),(3,2,3),(0.710192959006404,1.),(0.314770575782736,
0.314942866188492,0.332171906764074),.UNSPECIFIED.)
GEOMETRIC_REPRESENTATION_ITEM()
RATIONAL_B_SPLINE_SURFACE(((0.987877375613934,0.987877375613934,0.987877375613934,
0.986779141655833,0.988598326347701),(0.987877375613934,0.987877375613934,
0.987877375613934,0.986779141655833,0.988598326347701)))
REPRESENTATION_ITEM('')
SURFACE()
);
#488=(
BOUNDED_SURFACE()
B_SPLINE_SURFACE(1,2,((#101173,#101174,#101175,#101176,#101177),(#101178,
#101179,#101180,#101181,#101182)),.UNSPECIFIED.,.F.,.F.,.F.)
B_SPLINE_SURFACE_WITH_KNOTS((2,2),(3,2,3),(0.710318915640079,1.),(0.400939219852742,
0.418312080773433,0.41848580938264),.UNSPECIFIED.)
GEOMETRIC_REPRESENTATION_ITEM()
RATIONAL_B_SPLINE_SURFACE(((0.988105937622242,0.989485911589765,0.99383221411677,
0.99383221411677,0.99383221411677),(0.988105937622242,0.989485911589765,
0.99383221411677,0.99383221411677,0.99383221411677)))
REPRESENTATION_ITEM('')
SURFACE()
);
#489=(
BOUNDED_SURFACE()
B_SPLINE_SURFACE(1,2,((#101193,#101194,#101195,#101196,#101197),(#101198,
#101199,#101200,#101201,#101202)),.UNSPECIFIED.,.F.,.F.,.F.)
B_SPLINE_SURFACE_WITH_KNOTS((2,2),(3,2,3),(0.710192959008441,1.),(0.314770575782762,
0.314942866188517,0.332171906764075),.UNSPECIFIED.)
GEOMETRIC_REPRESENTATION_ITEM()
RATIONAL_B_SPLINE_SURFACE(((0.987877375613931,0.987877375613931,0.987877375613931,
0.986779141655835,0.988598326347701),(0.987877375613931,0.987877375613931,
0.987877375613931,0.986779141655835,0.988598326347701)))
REPRESENTATION_ITEM('')
SURFACE()
);
#490=(
BOUNDED_SURFACE()
B_SPLINE_SURFACE(1,2,((#101214,#101215,#101216,#101217,#101218),(#101219,
#101220,#101221,#101222,#101223)),.UNSPECIFIED.,.F.,.F.,.F.)
B_SPLINE_SURFACE_WITH_KNOTS((2,2),(3,2,3),(0.71031891564008,1.),(0.400939219852742,
0.418312080773433,0.41848580938264),.UNSPECIFIED.)
GEOMETRIC_REPRESENTATION_ITEM()
RATIONAL_B_SPLINE_SURFACE(((0.988105937622242,0.989485911589765,0.99383221411677,
0.99383221411677,0.99383221411677),(0.988105937622242,0.989485911589765,
0.99383221411677,0.99383221411677,0.99383221411677)))
REPRESENTATION_ITEM('')
SURFACE()
);
#491=(
BOUNDED_SURFACE()
B_SPLINE_SURFACE(1,2,((#101234,#101235,#101236,#101237,#101238),(#101239,
#101240,#101241,#101242,#101243)),.UNSPECIFIED.,.F.,.F.,.F.)
B_SPLINE_SURFACE_WITH_KNOTS((2,2),(3,2,3),(0.710192959006408,1.),(0.314770575782736,
0.314942866188492,0.332171906764075),.UNSPECIFIED.)
GEOMETRIC_REPRESENTATION_ITEM()
RATIONAL_B_SPLINE_SURFACE(((0.987877375613934,0.987877375613934,0.987877375613934,
0.986779141655833,0.988598326347701),(0.987877375613934,0.987877375613934,
0.987877375613934,0.986779141655833,0.988598326347701)))
REPRESENTATION_ITEM('')
SURFACE()
);
#492=(
BOUNDED_SURFACE()
B_SPLINE_SURFACE(1,2,((#101255,#101256,#101257,#101258,#101259),(#101260,
#101261,#101262,#101263,#101264)),.UNSPECIFIED.,.F.,.F.,.F.)
B_SPLINE_SURFACE_WITH_KNOTS((2,2),(3,2,3),(0.710318915639995,1.),(0.400939219852743,
0.418312080773433,0.41848580938264),.UNSPECIFIED.)
GEOMETRIC_REPRESENTATION_ITEM()
RATIONAL_B_SPLINE_SURFACE(((0.988105937622242,0.989485911589766,0.99383221411677,
0.99383221411677,0.99383221411677),(0.988105937622242,0.989485911589766,
0.99383221411677,0.99383221411677,0.99383221411677)))
REPRESENTATION_ITEM('')
SURFACE()
);
#493=(
BOUNDED_SURFACE()
B_SPLINE_SURFACE(1,2,((#101275,#101276,#101277,#101278,#101279),(#101280,
#101281,#101282,#101283,#101284)),.UNSPECIFIED.,.F.,.F.,.F.)
B_SPLINE_SURFACE_WITH_KNOTS((2,2),(3,2,3),(0.710192959008355,1.),(0.314770575782761,
0.314942866188516,0.332171906764074),.UNSPECIFIED.)
GEOMETRIC_REPRESENTATION_ITEM()
RATIONAL_B_SPLINE_SURFACE(((0.987877375613931,0.987877375613931,0.987877375613931,
0.986779141655835,0.988598326347701),(0.987877375613931,0.987877375613931,
0.987877375613931,0.986779141655835,0.988598326347701)))
REPRESENTATION_ITEM('')
SURFACE()
);
#494=(
BOUNDED_SURFACE()
B_SPLINE_SURFACE(1,2,((#101296,#101297,#101298,#101299,#101300),(#101301,
#101302,#101303,#101304,#101305)),.UNSPECIFIED.,.F.,.F.,.F.)
B_SPLINE_SURFACE_WITH_KNOTS((2,2),(3,2,3),(0.710318915640001,1.),(0.400939219852743,
0.418312080773434,0.418485809382641),.UNSPECIFIED.)
GEOMETRIC_REPRESENTATION_ITEM()
RATIONAL_B_SPLINE_SURFACE(((0.988105937622242,0.989485911589766,0.99383221411677,
0.99383221411677,0.99383221411677),(0.988105937622242,0.989485911589766,
0.99383221411677,0.99383221411677,0.99383221411677)))
REPRESENTATION_ITEM('')
SURFACE()
);
#495=(
BOUNDED_SURFACE()
B_SPLINE_SURFACE(1,2,((#101316,#101317,#101318,#101319,#101320),(#101321,
#101322,#101323,#101324,#101325)),.UNSPECIFIED.,.F.,.F.,.F.)
B_SPLINE_SURFACE_WITH_KNOTS((2,2),(3,2,3),(0.710192959006325,1.),(0.314770575782735,
0.314942866188491,0.332171906764074),.UNSPECIFIED.)
GEOMETRIC_REPRESENTATION_ITEM()
RATIONAL_B_SPLINE_SURFACE(((0.987877375613935,0.987877375613935,0.987877375613935,
0.986779141655833,0.988598326347701),(0.987877375613935,0.987877375613935,
0.987877375613935,0.986779141655833,0.988598326347701)))
REPRESENTATION_ITEM('')
SURFACE()
);
#496=(
BOUNDED_SURFACE()
B_SPLINE_SURFACE(1,2,((#101337,#101338,#101339,#101340,#101341),(#101342,
#101343,#101344,#101345,#101346)),.UNSPECIFIED.,.F.,.F.,.F.)
B_SPLINE_SURFACE_WITH_KNOTS((2,2),(3,2,3),(0.710318915639997,1.),(0.400939219852743,
0.418312080773434,0.418485809382641),.UNSPECIFIED.)
GEOMETRIC_REPRESENTATION_ITEM()
RATIONAL_B_SPLINE_SURFACE(((0.988105937622242,0.989485911589766,0.99383221411677,
0.99383221411677,0.99383221411677),(0.988105937622242,0.989485911589766,
0.99383221411677,0.99383221411677,0.99383221411677)))
REPRESENTATION_ITEM('')
SURFACE()
);
#497=(
BOUNDED_SURFACE()
B_SPLINE_SURFACE(1,2,((#101357,#101358,#101359,#101360,#101361),(#101362,
#101363,#101364,#101365,#101366)),.UNSPECIFIED.,.F.,.F.,.F.)
B_SPLINE_SURFACE_WITH_KNOTS((2,2),(3,2,3),(0.710192959008357,1.),(0.314770575782761,
0.314942866188516,0.332171906764074),.UNSPECIFIED.)
GEOMETRIC_REPRESENTATION_ITEM()
RATIONAL_B_SPLINE_SURFACE(((0.987877375613931,0.987877375613931,0.987877375613931,
0.986779141655835,0.988598326347701),(0.987877375613931,0.987877375613931,
0.987877375613931,0.986779141655835,0.988598326347701)))
REPRESENTATION_ITEM('')
SURFACE()
);
#498=(
BOUNDED_SURFACE()
B_SPLINE_SURFACE(1,2,((#101378,#101379,#101380,#101381,#101382),(#101383,
#101384,#101385,#101386,#101387)),.UNSPECIFIED.,.F.,.F.,.F.)
B_SPLINE_SURFACE_WITH_KNOTS((2,2),(3,2,3),(0.710318915639995,1.),(0.400939219852743,
0.418312080773434,0.418485809382641),.UNSPECIFIED.)
GEOMETRIC_REPRESENTATION_ITEM()
RATIONAL_B_SPLINE_SURFACE(((0.988105937622242,0.989485911589766,0.99383221411677,
0.99383221411677,0.99383221411677),(0.988105937622242,0.989485911589766,
0.99383221411677,0.99383221411677,0.99383221411677)))
REPRESENTATION_ITEM('')
SURFACE()
);
#499=(
BOUNDED_SURFACE()
B_SPLINE_SURFACE(1,2,((#101398,#101399,#101400,#101401,#101402),(#101403,
#101404,#101405,#101406,#101407)),.UNSPECIFIED.,.F.,.F.,.F.)
B_SPLINE_SURFACE_WITH_KNOTS((2,2),(3,2,3),(0.710192959006321,1.),(0.314770575782735,
0.314942866188491,0.332171906764074),.UNSPECIFIED.)
GEOMETRIC_REPRESENTATION_ITEM()
RATIONAL_B_SPLINE_SURFACE(((0.987877375613935,0.987877375613935,0.987877375613935,
0.986779141655833,0.988598326347701),(0.987877375613935,0.987877375613935,
0.987877375613935,0.986779141655833,0.988598326347701)))
REPRESENTATION_ITEM('')
SURFACE()
);
#500=(
BOUNDED_SURFACE()
B_SPLINE_SURFACE(1,2,((#101419,#101420,#101421,#101422,#101423),(#101424,
#101425,#101426,#101427,#101428)),.UNSPECIFIED.,.F.,.F.,.F.)
B_SPLINE_SURFACE_WITH_KNOTS((2,2),(3,2,3),(0.710318915640079,1.),(0.400939219852743,
0.418312080773434,0.418485809382641),.UNSPECIFIED.)
GEOMETRIC_REPRESENTATION_ITEM()
RATIONAL_B_SPLINE_SURFACE(((0.988105937622242,0.989485911589766,0.99383221411677,
0.99383221411677,0.99383221411677),(0.988105937622242,0.989485911589766,
0.99383221411677,0.99383221411677,0.99383221411677)))
REPRESENTATION_ITEM('')
SURFACE()
);
#501=(
BOUNDED_SURFACE()
B_SPLINE_SURFACE(1,2,((#101439,#101440,#101441,#101442,#101443),(#101444,
#101445,#101446,#101447,#101448)),.UNSPECIFIED.,.F.,.F.,.F.)
B_SPLINE_SURFACE_WITH_KNOTS((2,2),(3,2,3),(0.71019295900844,1.),(0.314770575782761,
0.314942866188516,0.332171906764074),.UNSPECIFIED.)
GEOMETRIC_REPRESENTATION_ITEM()
RATIONAL_B_SPLINE_SURFACE(((0.987877375613931,0.987877375613931,0.987877375613931,
0.986779141655835,0.988598326347701),(0.987877375613931,0.987877375613931,
0.987877375613931,0.986779141655835,0.988598326347701)))
REPRESENTATION_ITEM('')
SURFACE()
);
#502=(
BOUNDED_SURFACE()
B_SPLINE_SURFACE(1,2,((#101460,#101461,#101462,#101463,#101464),(#101465,
#101466,#101467,#101468,#101469)),.UNSPECIFIED.,.F.,.F.,.F.)
B_SPLINE_SURFACE_WITH_KNOTS((2,2),(3,2,3),(0.710318915639987,1.),(0.400939219852743,
0.418312080773434,0.418485809382641),.UNSPECIFIED.)
GEOMETRIC_REPRESENTATION_ITEM()
RATIONAL_B_SPLINE_SURFACE(((0.988105937622242,0.989485911589766,0.99383221411677,
0.99383221411677,0.99383221411677),(0.988105937622242,0.989485911589766,
0.99383221411677,0.99383221411677,0.99383221411677)))
REPRESENTATION_ITEM('')
SURFACE()
);
#503=(
BOUNDED_SURFACE()
B_SPLINE_SURFACE(1,2,((#101480,#101481,#101482,#101483,#101484),(#101485,
#101486,#101487,#101488,#101489)),.UNSPECIFIED.,.F.,.F.,.F.)
B_SPLINE_SURFACE_WITH_KNOTS((2,2),(3,2,3),(0.710192959008348,1.),(0.314770575782761,
0.314942866188516,0.332171906764074),.UNSPECIFIED.)
GEOMETRIC_REPRESENTATION_ITEM()
RATIONAL_B_SPLINE_SURFACE(((0.987877375613931,0.987877375613931,0.987877375613931,
0.986779141655835,0.988598326347701),(0.987877375613931,0.987877375613931,
0.987877375613931,0.986779141655835,0.988598326347701)))
REPRESENTATION_ITEM('')
SURFACE()
);
#504=(
BOUNDED_SURFACE()
B_SPLINE_SURFACE(1,2,((#101501,#101502,#101503,#101504,#101505),(#101506,
#101507,#101508,#101509,#101510)),.UNSPECIFIED.,.F.,.F.,.F.)
B_SPLINE_SURFACE_WITH_KNOTS((2,2),(3,2,3),(0.71031891564008,1.),(0.400939219852743,
0.418312080773434,0.418485809382641),.UNSPECIFIED.)
GEOMETRIC_REPRESENTATION_ITEM()
RATIONAL_B_SPLINE_SURFACE(((0.988105937622242,0.989485911589766,0.99383221411677,
0.99383221411677,0.99383221411677),(0.988105937622242,0.989485911589766,
0.99383221411677,0.99383221411677,0.99383221411677)))
REPRESENTATION_ITEM('')
SURFACE()
);
#505=(
BOUNDED_SURFACE()
B_SPLINE_SURFACE(1,2,((#101521,#101522,#101523,#101524,#101525),(#101526,
#101527,#101528,#101529,#101530)),.UNSPECIFIED.,.F.,.F.,.F.)
B_SPLINE_SURFACE_WITH_KNOTS((2,2),(3,2,3),(0.710192959008438,1.),(0.314770575782761,
0.314942866188516,0.332171906764074),.UNSPECIFIED.)
GEOMETRIC_REPRESENTATION_ITEM()
RATIONAL_B_SPLINE_SURFACE(((0.987877375613931,0.987877375613931,0.987877375613931,
0.986779141655835,0.988598326347701),(0.987877375613931,0.987877375613931,
0.987877375613931,0.986779141655835,0.988598326347701)))
REPRESENTATION_ITEM('')
SURFACE()
);
#506=(
BOUNDED_SURFACE()
B_SPLINE_SURFACE(1,2,((#101542,#101543,#101544,#101545,#101546),(#101547,
#101548,#101549,#101550,#101551)),.UNSPECIFIED.,.F.,.F.,.F.)
B_SPLINE_SURFACE_WITH_KNOTS((2,2),(3,2,3),(0.710318915639721,1.),(0.400939219852743,
0.418312080773435,0.418485809382642),.UNSPECIFIED.)
GEOMETRIC_REPRESENTATION_ITEM()
RATIONAL_B_SPLINE_SURFACE(((0.988105937622242,0.989485911589766,0.99383221411677,
0.99383221411677,0.99383221411677),(0.988105937622242,0.989485911589766,
0.99383221411677,0.99383221411677,0.99383221411677)))
REPRESENTATION_ITEM('')
SURFACE()
);
#507=(
BOUNDED_SURFACE()
B_SPLINE_SURFACE(1,2,((#101562,#101563,#101564,#101565,#101566),(#101567,
#101568,#101569,#101570,#101571)),.UNSPECIFIED.,.F.,.F.,.F.)
B_SPLINE_SURFACE_WITH_KNOTS((2,2),(3,2,3),(0.710192959006046,1.),(0.314770575782735,
0.314942866188491,0.332171906764074),.UNSPECIFIED.)
GEOMETRIC_REPRESENTATION_ITEM()
RATIONAL_B_SPLINE_SURFACE(((0.987877375613935,0.987877375613935,0.987877375613935,
0.986779141655833,0.988598326347701),(0.987877375613935,0.987877375613935,
0.987877375613935,0.986779141655833,0.988598326347701)))
REPRESENTATION_ITEM('')
SURFACE()
);
#508=(
BOUNDED_SURFACE()
B_SPLINE_SURFACE(1,2,((#101583,#101584,#101585,#101586,#101587),(#101588,
#101589,#101590,#101591,#101592)),.UNSPECIFIED.,.F.,.F.,.F.)
B_SPLINE_SURFACE_WITH_KNOTS((2,2),(3,2,3),(0.710318915638673,1.),(0.400939219852743,
0.418312080773434,0.418485809382641),.UNSPECIFIED.)
GEOMETRIC_REPRESENTATION_ITEM()
RATIONAL_B_SPLINE_SURFACE(((0.988105937622242,0.989485911589766,0.99383221411677,
0.99383221411677,0.99383221411677),(0.988105937622242,0.989485911589766,
0.99383221411677,0.99383221411677,0.99383221411677)))
REPRESENTATION_ITEM('')
SURFACE()
);
#509=(
BOUNDED_SURFACE()
B_SPLINE_SURFACE(1,2,((#101603,#101604,#101605,#101606,#101607),(#101608,
#101609,#101610,#101611,#101612)),.UNSPECIFIED.,.F.,.F.,.F.)
B_SPLINE_SURFACE_WITH_KNOTS((2,2),(3,2,3),(0.710192959007032,1.),(0.314770575782761,
0.314942866188516,0.332171906764074),.UNSPECIFIED.)
GEOMETRIC_REPRESENTATION_ITEM()
RATIONAL_B_SPLINE_SURFACE(((0.987877375613931,0.987877375613931,0.987877375613931,
0.986779141655835,0.988598326347701),(0.987877375613931,0.987877375613931,
0.987877375613931,0.986779141655835,0.988598326347701)))
REPRESENTATION_ITEM('')
SURFACE()
);
#510=(
BOUNDED_SURFACE()
B_SPLINE_SURFACE(1,2,((#101624,#101625,#101626,#101627,#101628),(#101629,
#101630,#101631,#101632,#101633)),.UNSPECIFIED.,.F.,.F.,.F.)
B_SPLINE_SURFACE_WITH_KNOTS((2,2),(3,2,3),(0.710318915639952,1.),(0.400939219852743,
0.418312080773434,0.418485809382641),.UNSPECIFIED.)
GEOMETRIC_REPRESENTATION_ITEM()
RATIONAL_B_SPLINE_SURFACE(((0.988105937622242,0.989485911589766,0.99383221411677,
0.99383221411677,0.99383221411677),(0.988105937622242,0.989485911589766,
0.99383221411677,0.99383221411677,0.99383221411677)))
REPRESENTATION_ITEM('')
SURFACE()
);
#511=(
BOUNDED_SURFACE()
B_SPLINE_SURFACE(1,2,((#101644,#101645,#101646,#101647,#101648),(#101649,
#101650,#101651,#101652,#101653)),.UNSPECIFIED.,.F.,.F.,.F.)
B_SPLINE_SURFACE_WITH_KNOTS((2,2),(3,2,3),(0.710192959006276,1.),(0.314770575782735,
0.314942866188491,0.332171906764074),.UNSPECIFIED.)
GEOMETRIC_REPRESENTATION_ITEM()
RATIONAL_B_SPLINE_SURFACE(((0.987877375613934,0.987877375613934,0.987877375613934,
0.986779141655832,0.988598326347701),(0.987877375613935,0.987877375613935,
0.987877375613935,0.986779141655832,0.988598326347701)))
REPRESENTATION_ITEM('')
SURFACE()
);
#512=(
BOUNDED_SURFACE()
B_SPLINE_SURFACE(1,2,((#101665,#101666,#101667,#101668,#101669),(#101670,
#101671,#101672,#101673,#101674)),.UNSPECIFIED.,.F.,.F.,.F.)
B_SPLINE_SURFACE_WITH_KNOTS((2,2),(3,2,3),(0.710318915640067,1.),(0.400939219852743,
0.418312080773434,0.418485809382641),.UNSPECIFIED.)
GEOMETRIC_REPRESENTATION_ITEM()
RATIONAL_B_SPLINE_SURFACE(((0.988105937622242,0.989485911589766,0.99383221411677,
0.99383221411677,0.99383221411677),(0.988105937622242,0.989485911589766,
0.99383221411677,0.99383221411677,0.99383221411677)))
REPRESENTATION_ITEM('')
SURFACE()
);
#513=(
BOUNDED_SURFACE()
B_SPLINE_SURFACE(1,2,((#101685,#101686,#101687,#101688,#101689),(#101690,
#101691,#101692,#101693,#101694)),.UNSPECIFIED.,.F.,.F.,.F.)
B_SPLINE_SURFACE_WITH_KNOTS((2,2),(3,2,3),(0.710192959008432,1.),(0.31477057578276,
0.314942866188515,0.332171906764074),.UNSPECIFIED.)
GEOMETRIC_REPRESENTATION_ITEM()
RATIONAL_B_SPLINE_SURFACE(((0.987877375613931,0.987877375613931,0.987877375613931,
0.986779141655835,0.988598326347701),(0.987877375613931,0.987877375613931,
0.987877375613931,0.986779141655835,0.988598326347701)))
REPRESENTATION_ITEM('')
SURFACE()
);
#514=(
BOUNDED_SURFACE()
B_SPLINE_SURFACE(1,2,((#101706,#101707,#101708,#101709,#101710),(#101711,
#101712,#101713,#101714,#101715)),.UNSPECIFIED.,.F.,.F.,.F.)
B_SPLINE_SURFACE_WITH_KNOTS((2,2),(3,2,3),(0.710318915639847,1.),(0.400939219852743,
0.418312080773434,0.418485809382641),.UNSPECIFIED.)
GEOMETRIC_REPRESENTATION_ITEM()
RATIONAL_B_SPLINE_SURFACE(((0.988105937622242,0.989485911589766,0.99383221411677,
0.99383221411677,0.99383221411677),(0.988105937622242,0.989485911589766,
0.99383221411677,0.99383221411677,0.99383221411677)))
REPRESENTATION_ITEM('')
SURFACE()
);
#515=(
BOUNDED_SURFACE()
B_SPLINE_SURFACE(1,2,((#101726,#101727,#101728,#101729,#101730),(#101731,
#101732,#101733,#101734,#101735)),.UNSPECIFIED.,.F.,.F.,.F.)
B_SPLINE_SURFACE_WITH_KNOTS((2,2),(3,2,3),(0.710192959006166,1.),(0.314770575782735,
0.314942866188491,0.332171906764074),.UNSPECIFIED.)
GEOMETRIC_REPRESENTATION_ITEM()
RATIONAL_B_SPLINE_SURFACE(((0.987877375613935,0.987877375613935,0.987877375613935,
0.986779141655833,0.988598326347701),(0.987877375613935,0.987877375613935,
0.987877375613935,0.986779141655833,0.988598326347701)))
REPRESENTATION_ITEM('')
SURFACE()
);
#516=(
BOUNDED_SURFACE()
B_SPLINE_SURFACE(1,2,((#101747,#101748,#101749,#101750,#101751),(#101752,
#101753,#101754,#101755,#101756)),.UNSPECIFIED.,.F.,.F.,.F.)
B_SPLINE_SURFACE_WITH_KNOTS((2,2),(3,2,3),(0.710318915640079,1.),(0.400939219852743,
0.418312080773434,0.418485809382641),.UNSPECIFIED.)
GEOMETRIC_REPRESENTATION_ITEM()
RATIONAL_B_SPLINE_SURFACE(((0.988105937622242,0.989485911589766,0.99383221411677,
0.99383221411677,0.99383221411677),(0.988105937622242,0.989485911589766,
0.99383221411677,0.99383221411677,0.99383221411677)))
REPRESENTATION_ITEM('')
SURFACE()
);
#517=(
BOUNDED_SURFACE()
B_SPLINE_SURFACE(1,2,((#101767,#101768,#101769,#101770,#101771),(#101772,
#101773,#101774,#101775,#101776)),.UNSPECIFIED.,.F.,.F.,.F.)
B_SPLINE_SURFACE_WITH_KNOTS((2,2),(3,2,3),(0.710192959008438,1.),(0.314770575782761,
0.314942866188516,0.332171906764074),.UNSPECIFIED.)
GEOMETRIC_REPRESENTATION_ITEM()
RATIONAL_B_SPLINE_SURFACE(((0.987877375613931,0.987877375613931,0.987877375613931,
0.986779141655835,0.988598326347701),(0.987877375613931,0.987877375613931,
0.987877375613931,0.986779141655835,0.988598326347701)))
REPRESENTATION_ITEM('')
SURFACE()
);
#518=(
BOUNDED_SURFACE()
B_SPLINE_SURFACE(1,2,((#101788,#101789,#101790,#101791,#101792),(#101793,
#101794,#101795,#101796,#101797)),.UNSPECIFIED.,.F.,.F.,.F.)
B_SPLINE_SURFACE_WITH_KNOTS((2,2),(3,2,3),(0.710318915638946,1.),(0.400939219852743,
0.418312080773434,0.418485809382641),.UNSPECIFIED.)
GEOMETRIC_REPRESENTATION_ITEM()
RATIONAL_B_SPLINE_SURFACE(((0.988105937622242,0.989485911589766,0.99383221411677,
0.99383221411677,0.99383221411677),(0.988105937622242,0.989485911589766,
0.99383221411677,0.99383221411677,0.99383221411677)))
REPRESENTATION_ITEM('')
SURFACE()
);
#519=(
BOUNDED_SURFACE()
B_SPLINE_SURFACE(1,2,((#101808,#101809,#101810,#101811,#101812),(#101813,
#101814,#101815,#101816,#101817)),.UNSPECIFIED.,.F.,.F.,.F.)
B_SPLINE_SURFACE_WITH_KNOTS((2,2),(3,2,3),(0.710192959005266,1.),(0.314770575782735,
0.314942866188491,0.332171906764074),.UNSPECIFIED.)
GEOMETRIC_REPRESENTATION_ITEM()
RATIONAL_B_SPLINE_SURFACE(((0.987877375613935,0.987877375613935,0.987877375613935,
0.986779141655833,0.988598326347701),(0.987877375613935,0.987877375613935,
0.987877375613935,0.986779141655833,0.988598326347701)))
REPRESENTATION_ITEM('')
SURFACE()
);
#520=(
BOUNDED_SURFACE()
B_SPLINE_SURFACE(1,2,((#101829,#101830,#101831,#101832,#101833),(#101834,
#101835,#101836,#101837,#101838)),.UNSPECIFIED.,.F.,.F.,.F.)
B_SPLINE_SURFACE_WITH_KNOTS((2,2),(3,2,3),(0.710318915639109,1.),(0.400939219852743,
0.418312080773434,0.418485809382641),.UNSPECIFIED.)
GEOMETRIC_REPRESENTATION_ITEM()
RATIONAL_B_SPLINE_SURFACE(((0.988105937622242,0.989485911589766,0.99383221411677,
0.99383221411677,0.99383221411677),(0.988105937622242,0.989485911589766,
0.99383221411677,0.99383221411677,0.99383221411677)))
REPRESENTATION_ITEM('')
SURFACE()
);
#521=(
BOUNDED_SURFACE()
B_SPLINE_SURFACE(1,2,((#101849,#101850,#101851,#101852,#101853),(#101854,
#101855,#101856,#101857,#101858)),.UNSPECIFIED.,.F.,.F.,.F.)
B_SPLINE_SURFACE_WITH_KNOTS((2,2),(3,2,3),(0.710192959007463,1.),(0.314770575782761,
0.314942866188516,0.332171906764074),.UNSPECIFIED.)
GEOMETRIC_REPRESENTATION_ITEM()
RATIONAL_B_SPLINE_SURFACE(((0.987877375613931,0.987877375613931,0.987877375613931,
0.986779141655835,0.988598326347701),(0.987877375613931,0.987877375613931,
0.987877375613931,0.986779141655835,0.988598326347701)))
REPRESENTATION_ITEM('')
SURFACE()
);
#522=(
BOUNDED_SURFACE()
B_SPLINE_SURFACE(1,2,((#101870,#101871,#101872,#101873,#101874),(#101875,
#101876,#101877,#101878,#101879)),.UNSPECIFIED.,.F.,.F.,.F.)
B_SPLINE_SURFACE_WITH_KNOTS((2,2),(3,2,3),(0.710318915638975,1.),(0.400939219852743,
0.418312080773434,0.418485809382641),.UNSPECIFIED.)
GEOMETRIC_REPRESENTATION_ITEM()
RATIONAL_B_SPLINE_SURFACE(((0.988105937622242,0.989485911589766,0.99383221411677,
0.99383221411677,0.99383221411677),(0.988105937622242,0.989485911589766,
0.99383221411677,0.99383221411677,0.99383221411677)))
REPRESENTATION_ITEM('')
SURFACE()
);
#523=(
BOUNDED_SURFACE()
B_SPLINE_SURFACE(1,2,((#101890,#101891,#101892,#101893,#101894),(#101895,
#101896,#101897,#101898,#101899)),.UNSPECIFIED.,.F.,.F.,.F.)
B_SPLINE_SURFACE_WITH_KNOTS((2,2),(3,2,3),(0.710192959005298,1.),(0.314770575782735,
0.314942866188491,0.332171906764074),.UNSPECIFIED.)
GEOMETRIC_REPRESENTATION_ITEM()
RATIONAL_B_SPLINE_SURFACE(((0.987877375613935,0.987877375613935,0.987877375613935,
0.986779141655833,0.988598326347701),(0.987877375613935,0.987877375613935,
0.987877375613935,0.986779141655833,0.988598326347701)))
REPRESENTATION_ITEM('')
SURFACE()
);
#524=(
BOUNDED_SURFACE()
B_SPLINE_SURFACE(1,2,((#101911,#101912,#101913,#101914,#101915),(#101916,
#101917,#101918,#101919,#101920)),.UNSPECIFIED.,.F.,.F.,.F.)
B_SPLINE_SURFACE_WITH_KNOTS((2,2),(3,2,3),(0.710318915639871,1.),(0.400939219852743,
0.418312080773435,0.418485809382642),.UNSPECIFIED.)
GEOMETRIC_REPRESENTATION_ITEM()
RATIONAL_B_SPLINE_SURFACE(((0.988105937622242,0.989485911589766,0.99383221411677,
0.99383221411677,0.99383221411677),(0.988105937622242,0.989485911589766,
0.99383221411677,0.99383221411677,0.99383221411677)))
REPRESENTATION_ITEM('')
SURFACE()
);
#525=(
BOUNDED_SURFACE()
B_SPLINE_SURFACE(1,2,((#101931,#101932,#101933,#101934,#101935),(#101936,
#101937,#101938,#101939,#101940)),.UNSPECIFIED.,.F.,.F.,.F.)
B_SPLINE_SURFACE_WITH_KNOTS((2,2),(3,2,3),(0.710192959008236,1.),(0.314770575782761,
0.314942866188516,0.332171906764074),.UNSPECIFIED.)
GEOMETRIC_REPRESENTATION_ITEM()
RATIONAL_B_SPLINE_SURFACE(((0.987877375613931,0.987877375613931,0.987877375613931,
0.986779141655835,0.988598326347701),(0.987877375613931,0.987877375613931,
0.987877375613931,0.986779141655835,0.988598326347701)))
REPRESENTATION_ITEM('')
SURFACE()
);
#526=(
BOUNDED_SURFACE()
B_SPLINE_SURFACE(1,2,((#101952,#101953,#101954,#101955,#101956),(#101957,
#101958,#101959,#101960,#101961)),.UNSPECIFIED.,.F.,.F.,.F.)
B_SPLINE_SURFACE_WITH_KNOTS((2,2),(3,2,3),(0.710318915638728,1.),(0.400939219852742,
0.418312080773556,0.418485809382764),.UNSPECIFIED.)
GEOMETRIC_REPRESENTATION_ITEM()
RATIONAL_B_SPLINE_SURFACE(((0.988105937622242,0.989485911589775,0.993832214116831,
0.993832214116831,0.993832214116831),(0.988105937622242,0.989485911589775,
0.993832214116831,0.993832214116831,0.993832214116831)))
REPRESENTATION_ITEM('')
SURFACE()
);
#527=(
BOUNDED_SURFACE()
B_SPLINE_SURFACE(1,2,((#101969,#101970,#101971,#101972,#101973),(#101974,
#101975,#101976,#101977,#101978)),.UNSPECIFIED.,.F.,.F.,.F.)
B_SPLINE_SURFACE_WITH_KNOTS((2,2),(3,2,3),(0.710192959005056,1.),(0.314770575782735,
0.314942866188491,0.332171906764074),.UNSPECIFIED.)
GEOMETRIC_REPRESENTATION_ITEM()
RATIONAL_B_SPLINE_SURFACE(((0.987877375613935,0.987877375613935,0.987877375613935,
0.986779141655833,0.988598326347701),(0.987877375613935,0.987877375613935,
0.987877375613935,0.986779141655833,0.988598326347701)))
REPRESENTATION_ITEM('')
SURFACE()
);
#528=(
BOUNDED_SURFACE()
B_SPLINE_SURFACE(1,2,((#101980,#101981,#101982,#101983,#101984),(#101985,
#101986,#101987,#101988,#101989)),.UNSPECIFIED.,.F.,.F.,.F.)
B_SPLINE_SURFACE_WITH_KNOTS((2,2),(3,2,3),(0.710318915638947,1.),(0.400939219852743,
0.418312080773435,0.418485809382642),.UNSPECIFIED.)
GEOMETRIC_REPRESENTATION_ITEM()
RATIONAL_B_SPLINE_SURFACE(((0.988105937622242,0.989485911589766,0.99383221411677,
0.99383221411677,0.99383221411677),(0.988105937622242,0.989485911589766,
0.99383221411677,0.99383221411677,0.99383221411677)))
REPRESENTATION_ITEM('')
SURFACE()
);
#529=(
BOUNDED_SURFACE()
B_SPLINE_SURFACE(1,2,((#102000,#102001,#102002,#102003,#102004),(#102005,
#102006,#102007,#102008,#102009)),.UNSPECIFIED.,.F.,.F.,.F.)
B_SPLINE_SURFACE_WITH_KNOTS((2,2),(3,2,3),(0.710192959007303,1.),(0.314770575782761,
0.314942866188516,0.332171906764074),.UNSPECIFIED.)
GEOMETRIC_REPRESENTATION_ITEM()
RATIONAL_B_SPLINE_SURFACE(((0.987877375613931,0.987877375613931,0.987877375613931,
0.986779141655835,0.988598326347701),(0.987877375613931,0.987877375613931,
0.987877375613931,0.986779141655835,0.988598326347701)))
REPRESENTATION_ITEM('')
SURFACE()
);
#530=(
BOUNDED_SURFACE()
B_SPLINE_SURFACE(1,2,((#102021,#102022,#102023,#102024,#102025),(#102026,
#102027,#102028,#102029,#102030)),.UNSPECIFIED.,.F.,.F.,.F.)
B_SPLINE_SURFACE_WITH_KNOTS((2,2),(3,2,3),(0.710318915639195,1.),(0.400939219852743,
0.418312080773434,0.418485809382641),.UNSPECIFIED.)
GEOMETRIC_REPRESENTATION_ITEM()
RATIONAL_B_SPLINE_SURFACE(((0.988105937622242,0.989485911589766,0.99383221411677,
0.99383221411677,0.99383221411677),(0.988105937622242,0.989485911589766,
0.99383221411677,0.99383221411677,0.99383221411677)))
REPRESENTATION_ITEM('')
SURFACE()
);
#531=(
BOUNDED_SURFACE()
B_SPLINE_SURFACE(1,2,((#102041,#102042,#102043,#102044,#102045),(#102046,
#102047,#102048,#102049,#102050)),.UNSPECIFIED.,.F.,.F.,.F.)
B_SPLINE_SURFACE_WITH_KNOTS((2,2),(3,2,3),(0.710192959005512,1.),(0.314770575782735,
0.314942866188491,0.332171906764074),.UNSPECIFIED.)
GEOMETRIC_REPRESENTATION_ITEM()
RATIONAL_B_SPLINE_SURFACE(((0.987877375613935,0.987877375613935,0.987877375613935,
0.986779141655833,0.988598326347701),(0.987877375613935,0.987877375613935,
0.987877375613935,0.986779141655833,0.988598326347701)))
REPRESENTATION_ITEM('')
SURFACE()
);
#532=(
BOUNDED_SURFACE()
B_SPLINE_SURFACE(1,2,((#102062,#102063,#102064,#102065,#102066),(#102067,
#102068,#102069,#102070,#102071)),.UNSPECIFIED.,.F.,.F.,.F.)
B_SPLINE_SURFACE_WITH_KNOTS((2,2),(3,2,3),(0.71031891563932,1.),(0.400939219852743,
0.418312080773435,0.418485809382642),.UNSPECIFIED.)
GEOMETRIC_REPRESENTATION_ITEM()
RATIONAL_B_SPLINE_SURFACE(((0.988105937622242,0.989485911589766,0.99383221411677,
0.99383221411677,0.99383221411677),(0.988105937622242,0.989485911589766,
0.99383221411677,0.99383221411677,0.99383221411677)))
REPRESENTATION_ITEM('')
SURFACE()
);
#533=(
BOUNDED_SURFACE()
B_SPLINE_SURFACE(1,2,((#102082,#102083,#102084,#102085,#102086),(#102087,
#102088,#102089,#102090,#102091)),.UNSPECIFIED.,.F.,.F.,.F.)
B_SPLINE_SURFACE_WITH_KNOTS((2,2),(3,2,3),(0.710192959007678,1.),(0.314770575782761,
0.314942866188516,0.332171906764074),.UNSPECIFIED.)
GEOMETRIC_REPRESENTATION_ITEM()
RATIONAL_B_SPLINE_SURFACE(((0.987877375613931,0.987877375613931,0.987877375613931,
0.986779141655835,0.988598326347701),(0.987877375613931,0.987877375613931,
0.987877375613931,0.986779141655835,0.988598326347701)))
REPRESENTATION_ITEM('')
SURFACE()
);
#534=(
BOUNDED_SURFACE()
B_SPLINE_SURFACE(1,2,((#102103,#102104,#102105,#102106,#102107),(#102108,
#102109,#102110,#102111,#102112)),.UNSPECIFIED.,.F.,.F.,.F.)
B_SPLINE_SURFACE_WITH_KNOTS((2,2),(3,2,3),(0.710318915638836,1.),(0.400939219852743,
0.418312080773437,0.418485809382644),.UNSPECIFIED.)
GEOMETRIC_REPRESENTATION_ITEM()
RATIONAL_B_SPLINE_SURFACE(((0.988105937622242,0.989485911589766,0.993832214116771,
0.993832214116771,0.993832214116771),(0.988105937622242,0.989485911589766,
0.993832214116771,0.993832214116771,0.993832214116771)))
REPRESENTATION_ITEM('')
SURFACE()
);
#535=(
BOUNDED_SURFACE()
B_SPLINE_SURFACE(1,2,((#102123,#102124,#102125,#102126,#102127),(#102128,
#102129,#102130,#102131,#102132)),.UNSPECIFIED.,.F.,.F.,.F.)
B_SPLINE_SURFACE_WITH_KNOTS((2,2),(3,2,3),(0.710192959005161,1.),(0.314770575782735,
0.314942866188491,0.332171906764077),.UNSPECIFIED.)
GEOMETRIC_REPRESENTATION_ITEM()
RATIONAL_B_SPLINE_SURFACE(((0.987877375613935,0.987877375613935,0.987877375613935,
0.986779141655832,0.988598326347702),(0.987877375613935,0.987877375613935,
0.987877375613935,0.986779141655832,0.988598326347702)))
REPRESENTATION_ITEM('')
SURFACE()
);
#536=(
BOUNDED_SURFACE()
B_SPLINE_SURFACE(1,2,((#102144,#102145,#102146,#102147,#102148),(#102149,
#102150,#102151,#102152,#102153)),.UNSPECIFIED.,.F.,.F.,.F.)
B_SPLINE_SURFACE_WITH_KNOTS((2,2),(3,2,3),(0.710318915638982,1.),(0.400939219852743,
0.418312080773434,0.418485809382641),.UNSPECIFIED.)
GEOMETRIC_REPRESENTATION_ITEM()
RATIONAL_B_SPLINE_SURFACE(((0.988105937622242,0.989485911589766,0.99383221411677,
0.99383221411677,0.99383221411677),(0.988105937622242,0.989485911589766,
0.99383221411677,0.99383221411677,0.99383221411677)))
REPRESENTATION_ITEM('')
SURFACE()
);
#537=(
BOUNDED_SURFACE()
B_SPLINE_SURFACE(1,2,((#102164,#102165,#102166,#102167,#102168),(#102169,
#102170,#102171,#102172,#102173)),.UNSPECIFIED.,.F.,.F.,.F.)
B_SPLINE_SURFACE_WITH_KNOTS((2,2),(3,2,3),(0.710192959007347,1.),(0.314770575782761,
0.314942866188516,0.332171906764075),.UNSPECIFIED.)
GEOMETRIC_REPRESENTATION_ITEM()
RATIONAL_B_SPLINE_SURFACE(((0.987877375613931,0.987877375613931,0.987877375613931,
0.986779141655835,0.988598326347701),(0.987877375613931,0.987877375613931,
0.987877375613931,0.986779141655835,0.988598326347701)))
REPRESENTATION_ITEM('')
SURFACE()
);
#538=(
BOUNDED_SURFACE()
B_SPLINE_SURFACE(1,2,((#102185,#102186,#102187,#102188,#102189),(#102190,
#102191,#102192,#102193,#102194)),.UNSPECIFIED.,.F.,.F.,.F.)
B_SPLINE_SURFACE_WITH_KNOTS((2,2),(3,2,3),(0.71031891563896,1.),(0.400939219852743,
0.418312080773435,0.418485809382642),.UNSPECIFIED.)
GEOMETRIC_REPRESENTATION_ITEM()
RATIONAL_B_SPLINE_SURFACE(((0.988105937622242,0.989485911589766,0.99383221411677,
0.99383221411677,0.99383221411677),(0.988105937622242,0.989485911589766,
0.99383221411677,0.99383221411677,0.99383221411677)))
REPRESENTATION_ITEM('')
SURFACE()
);
#539=(
BOUNDED_SURFACE()
B_SPLINE_SURFACE(1,2,((#102205,#102206,#102207,#102208,#102209),(#102210,
#102211,#102212,#102213,#102214)),.UNSPECIFIED.,.F.,.F.,.F.)
B_SPLINE_SURFACE_WITH_KNOTS((2,2),(3,2,3),(0.71019295900529,1.),(0.314770575782735,
0.314942866188491,0.332171906764074),.UNSPECIFIED.)
GEOMETRIC_REPRESENTATION_ITEM()
RATIONAL_B_SPLINE_SURFACE(((0.987877375613935,0.987877375613935,0.987877375613935,
0.986779141655833,0.988598326347701),(0.987877375613935,0.987877375613935,
0.987877375613935,0.986779141655833,0.988598326347701)))
REPRESENTATION_ITEM('')
SURFACE()
);
#540=(
BOUNDED_SURFACE()
B_SPLINE_SURFACE(1,2,((#102226,#102227,#102228,#102229,#102230),(#102231,
#102232,#102233,#102234,#102235)),.UNSPECIFIED.,.F.,.F.,.F.)
B_SPLINE_SURFACE_WITH_KNOTS((2,2),(3,2,3),(0.71031891563878,1.),(0.400939219852743,
0.418312080773434,0.418485809382641),.UNSPECIFIED.)
GEOMETRIC_REPRESENTATION_ITEM()
RATIONAL_B_SPLINE_SURFACE(((0.988105937622242,0.989485911589766,0.99383221411677,
0.99383221411677,0.99383221411677),(0.988105937622242,0.989485911589766,
0.99383221411677,0.99383221411677,0.99383221411677)))
REPRESENTATION_ITEM('')
SURFACE()
);
#541=(
BOUNDED_SURFACE()
B_SPLINE_SURFACE(1,2,((#102246,#102247,#102248,#102249,#102250),(#102251,
#102252,#102253,#102254,#102255)),.UNSPECIFIED.,.F.,.F.,.F.)
B_SPLINE_SURFACE_WITH_KNOTS((2,2),(3,2,3),(0.71019295900714,1.),(0.314770575782761,
0.314942866188516,0.332171906764074),.UNSPECIFIED.)
GEOMETRIC_REPRESENTATION_ITEM()
RATIONAL_B_SPLINE_SURFACE(((0.987877375613931,0.987877375613931,0.987877375613931,
0.986779141655835,0.988598326347701),(0.987877375613931,0.987877375613931,
0.987877375613931,0.986779141655835,0.988598326347701)))
REPRESENTATION_ITEM('')
SURFACE()
);
#542=(
BOUNDED_SURFACE()
B_SPLINE_SURFACE(1,2,((#102267,#102268,#102269),(#102270,#102271,#102272)),
 .UNSPECIFIED.,.F.,.F.,.F.)
B_SPLINE_SURFACE_WITH_KNOTS((2,2),(3,3),(0.710192959007992,1.),(0.366820493751253,
0.384035903515169),.UNSPECIFIED.)
GEOMETRIC_REPRESENTATION_ITEM()
RATIONAL_B_SPLINE_SURFACE(((0.994126602224873,0.989721266390694,0.988228734781998),
(0.994126602224873,0.989721266390694,0.988228734781998)))
REPRESENTATION_ITEM('')
SURFACE()
);
#543=(
BOUNDED_SURFACE()
B_SPLINE_SURFACE(1,2,((#102281,#102282,#102283,#102284,#102285,#102286,
#102287),(#102288,#102289,#102290,#102291,#102292,#102293,#102294)),
 .UNSPECIFIED.,.F.,.F.,.F.)
B_SPLINE_SURFACE_WITH_KNOTS((2,2),(3,2,2,3),(0.71031891563963,1.),(0.349264991474409,
0.357142857142857,0.366820493751254,0.366996048774023),.UNSPECIFIED.)
GEOMETRIC_REPRESENTATION_ITEM()
RATIONAL_B_SPLINE_SURFACE(((0.995079542144874,0.997234796441972,1.,0.996603060231146,
0.994126602224873,0.994126602224873,0.994126602224873),(0.995079542144874,
0.997234796441972,1.,0.996603060231146,0.994126602224873,0.994126602224873,
0.994126602224873)))
REPRESENTATION_ITEM('')
SURFACE()
);
#544=(
BOUNDED_SURFACE()
B_SPLINE_SURFACE(1,2,((#102302,#102303,#102304),(#102305,#102306,#102307)),
 .UNSPECIFIED.,.F.,.F.,.F.)
B_SPLINE_SURFACE_WITH_KNOTS((2,2),(3,3),(0.710192959007136,1.),(0.366820493751253,
0.384035903515172),.UNSPECIFIED.)
GEOMETRIC_REPRESENTATION_ITEM()
RATIONAL_B_SPLINE_SURFACE(((0.994126602224873,0.989721266390694,0.988228734781998),
(0.994126602224873,0.989721266390694,0.988228734781998)))
REPRESENTATION_ITEM('')
SURFACE()
);
#545=(
BOUNDED_SURFACE()
B_SPLINE_SURFACE(1,2,((#102316,#102317,#102318,#102319,#102320,#102321,
#102322),(#102323,#102324,#102325,#102326,#102327,#102328,#102329)),
 .UNSPECIFIED.,.F.,.F.,.F.)
B_SPLINE_SURFACE_WITH_KNOTS((2,2),(3,2,2,3),(0.710318915638783,1.),(0.349264991474413,
0.357142857142857,0.366820493751255,0.366996048774024),.UNSPECIFIED.)
GEOMETRIC_REPRESENTATION_ITEM()
RATIONAL_B_SPLINE_SURFACE(((0.995079542144876,0.997234796441973,1.,0.996603060231146,
0.994126602224872,0.994126602224872,0.994126602224872),(0.995079542144876,
0.997234796441973,1.,0.996603060231146,0.994126602224872,0.994126602224872,
0.994126602224872)))
REPRESENTATION_ITEM('')
SURFACE()
);
#546=(
BOUNDED_SURFACE()
B_SPLINE_SURFACE(1,2,((#102337,#102338,#102339),(#102340,#102341,#102342)),
 .UNSPECIFIED.,.F.,.F.,.F.)
B_SPLINE_SURFACE_WITH_KNOTS((2,2),(3,3),(0.710192959007322,1.),(0.366820493751253,
0.384035903515175),.UNSPECIFIED.)
GEOMETRIC_REPRESENTATION_ITEM()
RATIONAL_B_SPLINE_SURFACE(((0.994126602224873,0.989721266390693,0.988228734781997),
(0.994126602224873,0.989721266390693,0.988228734781997)))
REPRESENTATION_ITEM('')
SURFACE()
);
#547=(
BOUNDED_SURFACE()
B_SPLINE_SURFACE(1,2,((#102351,#102352,#102353,#102354,#102355,#102356,
#102357),(#102358,#102359,#102360,#102361,#102362,#102363,#102364)),
 .UNSPECIFIED.,.F.,.F.,.F.)
B_SPLINE_SURFACE_WITH_KNOTS((2,2),(3,2,2,3),(0.710318915638966,1.),(0.349264991474414,
0.357142857142857,0.366820493751254,0.366996048774023),.UNSPECIFIED.)
GEOMETRIC_REPRESENTATION_ITEM()
RATIONAL_B_SPLINE_SURFACE(((0.995079542144877,0.997234796441974,1.,0.996603060231146,
0.994126602224873,0.994126602224873,0.994126602224873),(0.995079542144877,
0.997234796441974,1.,0.996603060231146,0.994126602224873,0.994126602224873,
0.994126602224873)))
REPRESENTATION_ITEM('')
SURFACE()
);
#548=(
BOUNDED_SURFACE()
B_SPLINE_SURFACE(1,2,((#102372,#102373,#102374),(#102375,#102376,#102377)),
 .UNSPECIFIED.,.F.,.F.,.F.)
B_SPLINE_SURFACE_WITH_KNOTS((2,2),(3,3),(0.710192959007347,1.),(0.366820493751253,
0.384035903515169),.UNSPECIFIED.)
GEOMETRIC_REPRESENTATION_ITEM()
RATIONAL_B_SPLINE_SURFACE(((0.994126602224873,0.989721266390694,0.988228734781998),
(0.994126602224873,0.989721266390694,0.988228734781998)))
REPRESENTATION_ITEM('')
SURFACE()
);
#549=(
BOUNDED_SURFACE()
B_SPLINE_SURFACE(1,2,((#102386,#102387,#102388,#102389,#102390,#102391,
#102392),(#102393,#102394,#102395,#102396,#102397,#102398,#102399)),
 .UNSPECIFIED.,.F.,.F.,.F.)
B_SPLINE_SURFACE_WITH_KNOTS((2,2),(3,2,2,3),(0.710318915638992,1.),(0.349264991474409,
0.357142857142857,0.366820493751254,0.366996048774023),.UNSPECIFIED.)
GEOMETRIC_REPRESENTATION_ITEM()
RATIONAL_B_SPLINE_SURFACE(((0.995079542144874,0.997234796441972,1.,0.996603060231146,
0.994126602224873,0.994126602224873,0.994126602224873),(0.995079542144874,
0.997234796441972,1.,0.996603060231146,0.994126602224873,0.994126602224873,
0.994126602224873)))
REPRESENTATION_ITEM('')
SURFACE()
);
#550=(
BOUNDED_SURFACE()
B_SPLINE_SURFACE(1,2,((#102407,#102408,#102409),(#102410,#102411,#102412)),
 .UNSPECIFIED.,.F.,.F.,.F.)
B_SPLINE_SURFACE_WITH_KNOTS((2,2),(3,3),(0.710192959007198,1.),(0.366820493751253,
0.384035903515169),.UNSPECIFIED.)
GEOMETRIC_REPRESENTATION_ITEM()
RATIONAL_B_SPLINE_SURFACE(((0.994126602224873,0.989721266390694,0.988228734781998),
(0.994126602224873,0.989721266390694,0.988228734781998)))
REPRESENTATION_ITEM('')
SURFACE()
);
#551=(
BOUNDED_SURFACE()
B_SPLINE_SURFACE(1,2,((#102421,#102422,#102423,#102424,#102425,#102426,
#102427),(#102428,#102429,#102430,#102431,#102432,#102433,#102434)),
 .UNSPECIFIED.,.F.,.F.,.F.)
B_SPLINE_SURFACE_WITH_KNOTS((2,2),(3,2,2,3),(0.710318915638841,1.),(0.34926499147441,
0.357142857142857,0.366820493751254,0.366996048774023),.UNSPECIFIED.)
GEOMETRIC_REPRESENTATION_ITEM()
RATIONAL_B_SPLINE_SURFACE(((0.995079542144874,0.997234796441972,1.,0.996603060231146,
0.994126602224873,0.994126602224873,0.994126602224873),(0.995079542144874,
0.997234796441972,1.,0.996603060231146,0.994126602224873,0.994126602224873,
0.994126602224873)))
REPRESENTATION_ITEM('')
SURFACE()
);
#552=(
BOUNDED_SURFACE()
B_SPLINE_SURFACE(1,2,((#102442,#102443,#102444),(#102445,#102446,#102447)),
 .UNSPECIFIED.,.F.,.F.,.F.)
B_SPLINE_SURFACE_WITH_KNOTS((2,2),(3,3),(0.710192959007674,1.),(0.366820493751253,
0.384035903515168),.UNSPECIFIED.)
GEOMETRIC_REPRESENTATION_ITEM()
RATIONAL_B_SPLINE_SURFACE(((0.994126602224873,0.989721266390695,0.988228734781999),
(0.994126602224873,0.989721266390695,0.988228734781999)))
REPRESENTATION_ITEM('')
SURFACE()
);
#553=(
BOUNDED_SURFACE()
B_SPLINE_SURFACE(1,2,((#102456,#102457,#102458,#102459,#102460,#102461,
#102462),(#102463,#102464,#102465,#102466,#102467,#102468,#102469)),
 .UNSPECIFIED.,.F.,.F.,.F.)
B_SPLINE_SURFACE_WITH_KNOTS((2,2),(3,2,2,3),(0.71031891563931,1.),(0.349264991474391,
0.357142857142857,0.366820493751254,0.366996048774023),.UNSPECIFIED.)
GEOMETRIC_REPRESENTATION_ITEM()
RATIONAL_B_SPLINE_SURFACE(((0.995079542144864,0.997234796441966,1.,0.996603060231146,
0.994126602224873,0.994126602224873,0.994126602224873),(0.995079542144864,
0.997234796441966,1.,0.996603060231146,0.994126602224873,0.994126602224873,
0.994126602224873)))
REPRESENTATION_ITEM('')
SURFACE()
);
#554=(
BOUNDED_SURFACE()
B_SPLINE_SURFACE(1,2,((#102477,#102478,#102479),(#102480,#102481,#102482)),
 .UNSPECIFIED.,.F.,.F.,.F.)
B_SPLINE_SURFACE_WITH_KNOTS((2,2),(3,3),(0.710192959007547,1.),(0.366820493751253,
0.384035903515167),.UNSPECIFIED.)
GEOMETRIC_REPRESENTATION_ITEM()
RATIONAL_B_SPLINE_SURFACE(((0.994126602224873,0.989721266390695,0.988228734781999),
(0.994126602224873,0.989721266390695,0.988228734781999)))
REPRESENTATION_ITEM('')
SURFACE()
);
#555=(
BOUNDED_SURFACE()
B_SPLINE_SURFACE(1,2,((#102491,#102492,#102493,#102494,#102495,#102496,
#102497),(#102498,#102499,#102500,#102501,#102502,#102503,#102504)),
 .UNSPECIFIED.,.F.,.F.,.F.)
B_SPLINE_SURFACE_WITH_KNOTS((2,2),(3,2,2,3),(0.71031891563919,1.),(0.349264991474391,
0.357142857142857,0.366820493751254,0.366996048774023),.UNSPECIFIED.)
GEOMETRIC_REPRESENTATION_ITEM()
RATIONAL_B_SPLINE_SURFACE(((0.995079542144864,0.997234796441966,1.,0.996603060231146,
0.994126602224873,0.994126602224873,0.994126602224873),(0.995079542144864,
0.997234796441966,1.,0.996603060231146,0.994126602224873,0.994126602224873,
0.994126602224873)))
REPRESENTATION_ITEM('')
SURFACE()
);
#556=(
BOUNDED_SURFACE()
B_SPLINE_SURFACE(1,2,((#102512,#102513,#102514),(#102515,#102516,#102517)),
 .UNSPECIFIED.,.F.,.F.,.F.)
B_SPLINE_SURFACE_WITH_KNOTS((2,2),(3,3),(0.710192959007307,1.),(0.366820493751253,
0.384035903515168),.UNSPECIFIED.)
GEOMETRIC_REPRESENTATION_ITEM()
RATIONAL_B_SPLINE_SURFACE(((0.994126602224873,0.989721266390695,0.988228734781999),
(0.994126602224873,0.989721266390695,0.988228734781999)))
REPRESENTATION_ITEM('')
SURFACE()
);
#557=(
BOUNDED_SURFACE()
B_SPLINE_SURFACE(1,2,((#102526,#102527,#102528,#102529,#102530,#102531,
#102532),(#102533,#102534,#102535,#102536,#102537,#102538,#102539)),
 .UNSPECIFIED.,.F.,.F.,.F.)
B_SPLINE_SURFACE_WITH_KNOTS((2,2),(3,2,2,3),(0.710318915638953,1.),(0.349264991474392,
0.357142857142857,0.366820493751254,0.366996048774023),.UNSPECIFIED.)
GEOMETRIC_REPRESENTATION_ITEM()
RATIONAL_B_SPLINE_SURFACE(((0.995079542144865,0.997234796441966,1.,0.996603060231146,
0.994126602224873,0.994126602224873,0.994126602224873),(0.995079542144865,
0.997234796441966,1.,0.996603060231146,0.994126602224873,0.994126602224873,
0.994126602224873)))
REPRESENTATION_ITEM('')
SURFACE()
);
#558=(
BOUNDED_SURFACE()
B_SPLINE_SURFACE(1,2,((#102547,#102548,#102549),(#102550,#102551,#102552)),
 .UNSPECIFIED.,.F.,.F.,.F.)
B_SPLINE_SURFACE_WITH_KNOTS((2,2),(3,3),(0.710192959007092,1.),(0.366820493751253,
0.384035903515168),.UNSPECIFIED.)
GEOMETRIC_REPRESENTATION_ITEM()
RATIONAL_B_SPLINE_SURFACE(((0.994126602224873,0.989721266390695,0.988228734781998),
(0.994126602224873,0.989721266390695,0.988228734781998)))
REPRESENTATION_ITEM('')
SURFACE()
);
#559=(
BOUNDED_SURFACE()
B_SPLINE_SURFACE(1,2,((#102561,#102562,#102563,#102564,#102565,#102566,
#102567),(#102568,#102569,#102570,#102571,#102572,#102573,#102574)),
 .UNSPECIFIED.,.F.,.F.,.F.)
B_SPLINE_SURFACE_WITH_KNOTS((2,2),(3,2,2,3),(0.710318915638733,1.),(0.349264991474392,
0.357142857142857,0.366820493751254,0.366996048774023),.UNSPECIFIED.)
GEOMETRIC_REPRESENTATION_ITEM()
RATIONAL_B_SPLINE_SURFACE(((0.995079542144865,0.997234796441966,1.,0.996603060231146,
0.994126602224873,0.994126602224873,0.994126602224873),(0.995079542144865,
0.997234796441966,1.,0.996603060231146,0.994126602224873,0.994126602224873,
0.994126602224873)))
REPRESENTATION_ITEM('')
SURFACE()
);
#560=(
BOUNDED_SURFACE()
B_SPLINE_SURFACE(1,2,((#102582,#102583,#102584),(#102585,#102586,#102587)),
 .UNSPECIFIED.,.F.,.F.,.F.)
B_SPLINE_SURFACE_WITH_KNOTS((2,2),(3,3),(0.71019295900824,1.),(0.366820493751253,
0.384035903515169),.UNSPECIFIED.)
GEOMETRIC_REPRESENTATION_ITEM()
RATIONAL_B_SPLINE_SURFACE(((0.994126602224873,0.989721266390694,0.988228734781998),
(0.994126602224873,0.989721266390694,0.988228734781998)))
REPRESENTATION_ITEM('')
SURFACE()
);
#561=(
BOUNDED_SURFACE()
B_SPLINE_SURFACE(1,2,((#102596,#102597,#102598,#102599,#102600,#102601,
#102602),(#102603,#102604,#102605,#102606,#102607,#102608,#102609)),
 .UNSPECIFIED.,.F.,.F.,.F.)
B_SPLINE_SURFACE_WITH_KNOTS((2,2),(3,2,2,3),(0.710318915639881,1.),(0.349264991474409,
0.357142857142857,0.366820493751264,0.366996048774033),.UNSPECIFIED.)
GEOMETRIC_REPRESENTATION_ITEM()
RATIONAL_B_SPLINE_SURFACE(((0.995079542144874,0.997234796441972,1.,0.996603060231143,
0.994126602224868,0.994126602224868,0.994126602224868),(0.995079542144874,
0.997234796441972,1.,0.996603060231143,0.994126602224868,0.994126602224868,
0.994126602224868)))
REPRESENTATION_ITEM('')
SURFACE()
);
#562=(
BOUNDED_SURFACE()
B_SPLINE_SURFACE(1,2,((#102617,#102618,#102619),(#102620,#102621,#102622)),
 .UNSPECIFIED.,.F.,.F.,.F.)
B_SPLINE_SURFACE_WITH_KNOTS((2,2),(3,3),(0.710192959008287,1.),(0.366820493751253,
0.384035903515169),.UNSPECIFIED.)
GEOMETRIC_REPRESENTATION_ITEM()
RATIONAL_B_SPLINE_SURFACE(((0.994126602224873,0.989721266390694,0.988228734781998),
(0.994126602224873,0.989721266390694,0.988228734781998)))
REPRESENTATION_ITEM('')
SURFACE()
);
#563=(
BOUNDED_SURFACE()
B_SPLINE_SURFACE(1,2,((#102631,#102632,#102633,#102634,#102635,#102636,
#102637),(#102638,#102639,#102640,#102641,#102642,#102643,#102644)),
 .UNSPECIFIED.,.F.,.F.,.F.)
B_SPLINE_SURFACE_WITH_KNOTS((2,2),(3,2,2,3),(0.710318915639928,1.),(0.349264991474409,
0.357142857142857,0.366820493751264,0.366996048774033),.UNSPECIFIED.)
GEOMETRIC_REPRESENTATION_ITEM()
RATIONAL_B_SPLINE_SURFACE(((0.995079542144874,0.997234796441972,1.,0.996603060231143,
0.994126602224868,0.994126602224868,0.994126602224868),(0.995079542144874,
0.997234796441972,1.,0.996603060231143,0.994126602224868,0.994126602224868,
0.994126602224868)))
REPRESENTATION_ITEM('')
SURFACE()
);
#564=(
BOUNDED_SURFACE()
B_SPLINE_SURFACE(1,2,((#102652,#102653,#102654),(#102655,#102656,#102657)),
 .UNSPECIFIED.,.F.,.F.,.F.)
B_SPLINE_SURFACE_WITH_KNOTS((2,2),(3,3),(0.710192959008438,1.),(0.366820493751253,
0.384035903515169),.UNSPECIFIED.)
GEOMETRIC_REPRESENTATION_ITEM()
RATIONAL_B_SPLINE_SURFACE(((0.994126602224873,0.989721266390694,0.988228734781998),
(0.994126602224873,0.989721266390694,0.988228734781998)))
REPRESENTATION_ITEM('')
SURFACE()
);
#565=(
BOUNDED_SURFACE()
B_SPLINE_SURFACE(1,2,((#102666,#102667,#102668,#102669,#102670,#102671,
#102672),(#102673,#102674,#102675,#102676,#102677,#102678,#102679)),
 .UNSPECIFIED.,.F.,.F.,.F.)
B_SPLINE_SURFACE_WITH_KNOTS((2,2),(3,2,2,3),(0.710318915639478,1.),(0.349264991474409,
0.357142857142857,0.366820493751264,0.366996048774033),.UNSPECIFIED.)
GEOMETRIC_REPRESENTATION_ITEM()
RATIONAL_B_SPLINE_SURFACE(((0.995079542144874,0.997234796441972,1.,0.996603060231143,
0.994126602224868,0.994126602224868,0.994126602224868),(0.995079542144874,
0.997234796441972,1.,0.996603060231143,0.994126602224868,0.994126602224868,
0.994126602224868)))
REPRESENTATION_ITEM('')
SURFACE()
);
#566=(
BOUNDED_SURFACE()
B_SPLINE_SURFACE(1,2,((#102687,#102688,#102689),(#102690,#102691,#102692)),
 .UNSPECIFIED.,.F.,.F.,.F.)
B_SPLINE_SURFACE_WITH_KNOTS((2,2),(3,3),(0.710192959008445,1.),(0.366820493751253,
0.384035903515169),.UNSPECIFIED.)
GEOMETRIC_REPRESENTATION_ITEM()
RATIONAL_B_SPLINE_SURFACE(((0.994126602224873,0.989721266390694,0.988228734781998),
(0.994126602224873,0.989721266390694,0.988228734781998)))
REPRESENTATION_ITEM('')
SURFACE()
);
#567=(
BOUNDED_SURFACE()
B_SPLINE_SURFACE(1,2,((#102701,#102702,#102703,#102704,#102705,#102706,
#102707),(#102708,#102709,#102710,#102711,#102712,#102713,#102714)),
 .UNSPECIFIED.,.F.,.F.,.F.)
B_SPLINE_SURFACE_WITH_KNOTS((2,2),(3,2,2,3),(0.710318915640074,1.),(0.34926499147441,
0.357142857142857,0.366820493751264,0.366996048774033),.UNSPECIFIED.)
GEOMETRIC_REPRESENTATION_ITEM()
RATIONAL_B_SPLINE_SURFACE(((0.995079542144874,0.997234796441972,1.,0.996603060231143,
0.994126602224868,0.994126602224868,0.994126602224868),(0.995079542144874,
0.997234796441972,1.,0.996603060231143,0.994126602224868,0.994126602224868,
0.994126602224868)))
REPRESENTATION_ITEM('')
SURFACE()
);
#568=(
BOUNDED_SURFACE()
B_SPLINE_SURFACE(1,2,((#102722,#102723,#102724),(#102725,#102726,#102727)),
 .UNSPECIFIED.,.F.,.F.,.F.)
B_SPLINE_SURFACE_WITH_KNOTS((2,2),(3,3),(0.710192959008436,1.),(0.366820493751253,
0.384035903515169),.UNSPECIFIED.)
GEOMETRIC_REPRESENTATION_ITEM()
RATIONAL_B_SPLINE_SURFACE(((0.994126602224873,0.989721266390694,0.988228734781998),
(0.994126602224873,0.989721266390694,0.988228734781998)))
REPRESENTATION_ITEM('')
SURFACE()
);
#569=(
BOUNDED_SURFACE()
B_SPLINE_SURFACE(1,2,((#102736,#102737,#102738,#102739,#102740,#102741,
#102742),(#102743,#102744,#102745,#102746,#102747,#102748,#102749)),
 .UNSPECIFIED.,.F.,.F.,.F.)
B_SPLINE_SURFACE_WITH_KNOTS((2,2),(3,2,2,3),(0.710318915640068,1.),(0.349264991474409,
0.357142857142857,0.366820493751264,0.366996048774033),.UNSPECIFIED.)
GEOMETRIC_REPRESENTATION_ITEM()
RATIONAL_B_SPLINE_SURFACE(((0.995079542144874,0.997234796441972,1.,0.996603060231143,
0.994126602224868,0.994126602224868,0.994126602224868),(0.995079542144874,
0.997234796441972,1.,0.996603060231143,0.994126602224868,0.994126602224868,
0.994126602224868)))
REPRESENTATION_ITEM('')
SURFACE()
);
#570=(
BOUNDED_SURFACE()
B_SPLINE_SURFACE(1,2,((#102757,#102758,#102759),(#102760,#102761,#102762)),
 .UNSPECIFIED.,.F.,.F.,.F.)
B_SPLINE_SURFACE_WITH_KNOTS((2,2),(3,3),(0.710192959008435,1.),(0.366820493751253,
0.384035903515169),.UNSPECIFIED.)
GEOMETRIC_REPRESENTATION_ITEM()
RATIONAL_B_SPLINE_SURFACE(((0.994126602224873,0.989721266390694,0.988228734781998),
(0.994126602224873,0.989721266390694,0.988228734781998)))
REPRESENTATION_ITEM('')
SURFACE()
);
#571=(
BOUNDED_SURFACE()
B_SPLINE_SURFACE(1,2,((#102771,#102772,#102773,#102774,#102775,#102776,
#102777),(#102778,#102779,#102780,#102781,#102782,#102783,#102784)),
 .UNSPECIFIED.,.F.,.F.,.F.)
B_SPLINE_SURFACE_WITH_KNOTS((2,2),(3,2,2,3),(0.710318915640079,1.),(0.34926499147441,
0.357142857142857,0.366820493751264,0.366996048774033),.UNSPECIFIED.)
GEOMETRIC_REPRESENTATION_ITEM()
RATIONAL_B_SPLINE_SURFACE(((0.995079542144874,0.997234796441972,1.,0.996603060231143,
0.994126602224868,0.994126602224868,0.994126602224868),(0.995079542144874,
0.997234796441972,1.,0.996603060231143,0.994126602224868,0.994126602224868,
0.994126602224868)))
REPRESENTATION_ITEM('')
SURFACE()
);
#572=(
BOUNDED_SURFACE()
B_SPLINE_SURFACE(1,2,((#102792,#102793,#102794),(#102795,#102796,#102797)),
 .UNSPECIFIED.,.F.,.F.,.F.)
B_SPLINE_SURFACE_WITH_KNOTS((2,2),(3,3),(0.710192959008434,1.),(0.366820493751253,
0.384035903515169),.UNSPECIFIED.)
GEOMETRIC_REPRESENTATION_ITEM()
RATIONAL_B_SPLINE_SURFACE(((0.994126602224873,0.989721266390694,0.988228734781998),
(0.994126602224873,0.989721266390694,0.988228734781998)))
REPRESENTATION_ITEM('')
SURFACE()
);
#573=(
BOUNDED_SURFACE()
B_SPLINE_SURFACE(1,2,((#102806,#102807,#102808,#102809,#102810,#102811,
#102812),(#102813,#102814,#102815,#102816,#102817,#102818,#102819)),
 .UNSPECIFIED.,.F.,.F.,.F.)
B_SPLINE_SURFACE_WITH_KNOTS((2,2),(3,2,2,3),(0.710318915640073,1.),(0.349264991474409,
0.357142857142857,0.366820493751264,0.366996048774033),.UNSPECIFIED.)
GEOMETRIC_REPRESENTATION_ITEM()
RATIONAL_B_SPLINE_SURFACE(((0.995079542144874,0.997234796441972,1.,0.996603060231143,
0.994126602224868,0.994126602224868,0.994126602224868),(0.995079542144874,
0.997234796441972,1.,0.996603060231143,0.994126602224868,0.994126602224868,
0.994126602224868)))
REPRESENTATION_ITEM('')
SURFACE()
);
#574=(
BOUNDED_SURFACE()
B_SPLINE_SURFACE(1,2,((#102827,#102828,#102829),(#102830,#102831,#102832)),
 .UNSPECIFIED.,.F.,.F.,.F.)
B_SPLINE_SURFACE_WITH_KNOTS((2,2),(3,3),(0.71019295900833,1.),(0.366820493751253,
0.384035903515169),.UNSPECIFIED.)
GEOMETRIC_REPRESENTATION_ITEM()
RATIONAL_B_SPLINE_SURFACE(((0.994126602224873,0.989721266390694,0.988228734781998),
(0.994126602224873,0.989721266390694,0.988228734781998)))
REPRESENTATION_ITEM('')
SURFACE()
);
#575=(
BOUNDED_SURFACE()
B_SPLINE_SURFACE(1,2,((#102841,#102842,#102843,#102844,#102845,#102846,
#102847),(#102848,#102849,#102850,#102851,#102852,#102853,#102854)),
 .UNSPECIFIED.,.F.,.F.,.F.)
B_SPLINE_SURFACE_WITH_KNOTS((2,2),(3,2,2,3),(0.710318915639974,1.),(0.349264991474409,
0.357142857142857,0.366820493751264,0.366996048774033),.UNSPECIFIED.)
GEOMETRIC_REPRESENTATION_ITEM()
RATIONAL_B_SPLINE_SURFACE(((0.995079542144874,0.997234796441972,1.,0.996603060231143,
0.994126602224868,0.994126602224868,0.994126602224868),(0.995079542144874,
0.997234796441972,1.,0.996603060231143,0.994126602224868,0.994126602224868,
0.994126602224868)))
REPRESENTATION_ITEM('')
SURFACE()
);
#576=(
BOUNDED_SURFACE()
B_SPLINE_SURFACE(1,2,((#102862,#102863,#102864),(#102865,#102866,#102867)),
 .UNSPECIFIED.,.F.,.F.,.F.)
B_SPLINE_SURFACE_WITH_KNOTS((2,2),(3,3),(0.710192959007029,1.),(0.366820493751253,
0.384035903515169),.UNSPECIFIED.)
GEOMETRIC_REPRESENTATION_ITEM()
RATIONAL_B_SPLINE_SURFACE(((0.994126602224873,0.989721266390694,0.988228734781998),
(0.994126602224873,0.989721266390694,0.988228734781998)))
REPRESENTATION_ITEM('')
SURFACE()
);
#577=(
BOUNDED_SURFACE()
B_SPLINE_SURFACE(1,2,((#102876,#102877,#102878,#102879,#102880,#102881,
#102882),(#102883,#102884,#102885,#102886,#102887,#102888,#102889)),
 .UNSPECIFIED.,.F.,.F.,.F.)
B_SPLINE_SURFACE_WITH_KNOTS((2,2),(3,2,2,3),(0.71031891563867,1.),(0.34926499147441,
0.357142857142857,0.366820493751264,0.366996048774033),.UNSPECIFIED.)
GEOMETRIC_REPRESENTATION_ITEM()
RATIONAL_B_SPLINE_SURFACE(((0.995079542144874,0.997234796441972,1.,0.996603060231143,
0.994126602224868,0.994126602224868,0.994126602224868),(0.995079542144874,
0.997234796441972,1.,0.996603060231143,0.994126602224868,0.994126602224868,
0.994126602224868)))
REPRESENTATION_ITEM('')
SURFACE()
);
#578=(
BOUNDED_SURFACE()
B_SPLINE_SURFACE(1,2,((#102897,#102898,#102899),(#102900,#102901,#102902)),
 .UNSPECIFIED.,.F.,.F.,.F.)
B_SPLINE_SURFACE_WITH_KNOTS((2,2),(3,3),(0.710192959008187,1.),(0.366820493751026,
0.38403590351517),.UNSPECIFIED.)
GEOMETRIC_REPRESENTATION_ITEM()
RATIONAL_B_SPLINE_SURFACE(((0.994126602224989,0.989721266390714,0.988228734781998),
(0.994126602224989,0.989721266390714,0.988228734781998)))
REPRESENTATION_ITEM('')
SURFACE()
);
#579=(
BOUNDED_SURFACE()
B_SPLINE_SURFACE(1,2,((#102911,#102912,#102913,#102914,#102915,#102916,
#102917),(#102918,#102919,#102920,#102921,#102922,#102923,#102924)),
 .UNSPECIFIED.,.F.,.F.,.F.)
B_SPLINE_SURFACE_WITH_KNOTS((2,2),(3,2,2,3),(0.710318915639827,1.),(0.349264991474409,
0.357142857142857,0.366820493751264,0.366996048774033),.UNSPECIFIED.)
GEOMETRIC_REPRESENTATION_ITEM()
RATIONAL_B_SPLINE_SURFACE(((0.995079542144874,0.997234796441972,1.,0.996603060231143,
0.994126602224868,0.994126602224868,0.994126602224868),(0.995079542144874,
0.997234796441972,1.,0.996603060231143,0.994126602224868,0.994126602224868,
0.994126602224868)))
REPRESENTATION_ITEM('')
SURFACE()
);
#580=(
BOUNDED_SURFACE()
B_SPLINE_SURFACE(1,2,((#102932,#102933,#102934),(#102935,#102936,#102937)),
 .UNSPECIFIED.,.F.,.F.,.F.)
B_SPLINE_SURFACE_WITH_KNOTS((2,2),(3,3),(0.710192959008439,1.),(0.366820493751253,
0.384035903515169),.UNSPECIFIED.)
GEOMETRIC_REPRESENTATION_ITEM()
RATIONAL_B_SPLINE_SURFACE(((0.994126602224873,0.989721266390694,0.988228734781998),
(0.994126602224873,0.989721266390694,0.988228734781998)))
REPRESENTATION_ITEM('')
SURFACE()
);
#581=(
BOUNDED_SURFACE()
B_SPLINE_SURFACE(1,2,((#102946,#102947,#102948,#102949,#102950,#102951,
#102952),(#102953,#102954,#102955,#102956,#102957,#102958,#102959)),
 .UNSPECIFIED.,.F.,.F.,.F.)
B_SPLINE_SURFACE_WITH_KNOTS((2,2),(3,2,2,3),(0.710318915640079,1.),(0.349264991474409,
0.357142857142857,0.366820493751264,0.366996048774033),.UNSPECIFIED.)
GEOMETRIC_REPRESENTATION_ITEM()
RATIONAL_B_SPLINE_SURFACE(((0.995079542144874,0.997234796441972,1.,0.996603060231143,
0.994126602224868,0.994126602224868,0.994126602224868),(0.995079542144874,
0.997234796441972,1.,0.996603060231143,0.994126602224868,0.994126602224868,
0.994126602224868)))
REPRESENTATION_ITEM('')
SURFACE()
);
#582=(
BOUNDED_SURFACE()
B_SPLINE_SURFACE(1,2,((#102967,#102968,#102969),(#102970,#102971,#102972)),
 .UNSPECIFIED.,.F.,.F.,.F.)
B_SPLINE_SURFACE_WITH_KNOTS((2,2),(3,3),(0.710192959008441,1.),(0.366820493751253,
0.384035903515169),.UNSPECIFIED.)
GEOMETRIC_REPRESENTATION_ITEM()
RATIONAL_B_SPLINE_SURFACE(((0.994126602224873,0.989721266390694,0.988228734781998),
(0.994126602224873,0.989721266390694,0.988228734781998)))
REPRESENTATION_ITEM('')
SURFACE()
);
#583=(
BOUNDED_SURFACE()
B_SPLINE_SURFACE(1,2,((#102981,#102982,#102983,#102984,#102985,#102986,
#102987),(#102988,#102989,#102990,#102991,#102992,#102993,#102994)),
 .UNSPECIFIED.,.F.,.F.,.F.)
B_SPLINE_SURFACE_WITH_KNOTS((2,2),(3,2,2,3),(0.710318915640082,1.),(0.349264991474409,
0.357142857142857,0.366820493751264,0.366996048774033),.UNSPECIFIED.)
GEOMETRIC_REPRESENTATION_ITEM()
RATIONAL_B_SPLINE_SURFACE(((0.995079542144874,0.997234796441972,1.,0.996603060231143,
0.994126602224868,0.994126602224868,0.994126602224868),(0.995079542144874,
0.997234796441972,1.,0.996603060231143,0.994126602224868,0.994126602224868,
0.994126602224868)))
REPRESENTATION_ITEM('')
SURFACE()
);
#584=(
BOUNDED_SURFACE()
B_SPLINE_SURFACE(1,2,((#103002,#103003,#103004),(#103005,#103006,#103007)),
 .UNSPECIFIED.,.F.,.F.,.F.)
B_SPLINE_SURFACE_WITH_KNOTS((2,2),(3,3),(0.710192959008439,1.),(0.366820493751253,
0.384035903515169),.UNSPECIFIED.)
GEOMETRIC_REPRESENTATION_ITEM()
RATIONAL_B_SPLINE_SURFACE(((0.994126602224873,0.989721266390694,0.988228734781998),
(0.994126602224873,0.989721266390694,0.988228734781998)))
REPRESENTATION_ITEM('')
SURFACE()
);
#585=(
BOUNDED_SURFACE()
B_SPLINE_SURFACE(1,2,((#103016,#103017,#103018,#103019,#103020,#103021,
#103022),(#103023,#103024,#103025,#103026,#103027,#103028,#103029)),
 .UNSPECIFIED.,.F.,.F.,.F.)
B_SPLINE_SURFACE_WITH_KNOTS((2,2),(3,2,2,3),(0.710318915640079,1.),(0.349264991474409,
0.357142857142857,0.366820493751264,0.366996048774033),.UNSPECIFIED.)
GEOMETRIC_REPRESENTATION_ITEM()
RATIONAL_B_SPLINE_SURFACE(((0.995079542144874,0.997234796441972,1.,0.996603060231143,
0.994126602224868,0.994126602224868,0.994126602224868),(0.995079542144874,
0.997234796441972,1.,0.996603060231143,0.994126602224868,0.994126602224868,
0.994126602224868)))
REPRESENTATION_ITEM('')
SURFACE()
);
#586=(
BOUNDED_SURFACE()
B_SPLINE_SURFACE(1,2,((#103037,#103038,#103039),(#103040,#103041,#103042)),
 .UNSPECIFIED.,.F.,.F.,.F.)
B_SPLINE_SURFACE_WITH_KNOTS((2,2),(3,3),(0.710192959008439,1.),(0.366820493751253,
0.384035903515169),.UNSPECIFIED.)
GEOMETRIC_REPRESENTATION_ITEM()
RATIONAL_B_SPLINE_SURFACE(((0.994126602224873,0.989721266390694,0.988228734781998),
(0.994126602224873,0.989721266390694,0.988228734781998)))
REPRESENTATION_ITEM('')
SURFACE()
);
#587=(
BOUNDED_SURFACE()
B_SPLINE_SURFACE(1,2,((#103051,#103052,#103053,#103054,#103055,#103056,
#103057),(#103058,#103059,#103060,#103061,#103062,#103063,#103064)),
 .UNSPECIFIED.,.F.,.F.,.F.)
B_SPLINE_SURFACE_WITH_KNOTS((2,2),(3,2,2,3),(0.710318915640081,1.),(0.34926499147441,
0.357142857142857,0.366820493751264,0.366996048774033),.UNSPECIFIED.)
GEOMETRIC_REPRESENTATION_ITEM()
RATIONAL_B_SPLINE_SURFACE(((0.995079542144874,0.997234796441972,1.,0.996603060231143,
0.994126602224868,0.994126602224868,0.994126602224868),(0.995079542144874,
0.997234796441972,1.,0.996603060231143,0.994126602224868,0.994126602224868,
0.994126602224868)))
REPRESENTATION_ITEM('')
SURFACE()
);
#588=(
BOUNDED_SURFACE()
B_SPLINE_SURFACE(1,2,((#103072,#103073,#103074),(#103075,#103076,#103077)),
 .UNSPECIFIED.,.F.,.F.,.F.)
B_SPLINE_SURFACE_WITH_KNOTS((2,2),(3,3),(0.710192959008437,1.),(0.366820493751253,
0.384035903515169),.UNSPECIFIED.)
GEOMETRIC_REPRESENTATION_ITEM()
RATIONAL_B_SPLINE_SURFACE(((0.994126602224873,0.989721266390694,0.988228734781998),
(0.994126602224873,0.989721266390694,0.988228734781998)))
REPRESENTATION_ITEM('')
SURFACE()
);
#589=(
BOUNDED_SURFACE()
B_SPLINE_SURFACE(1,2,((#103086,#103087,#103088,#103089,#103090,#103091,
#103092),(#103093,#103094,#103095,#103096,#103097,#103098,#103099)),
 .UNSPECIFIED.,.F.,.F.,.F.)
B_SPLINE_SURFACE_WITH_KNOTS((2,2),(3,2,2,3),(0.710318915640083,1.),(0.349264991474409,
0.357142857142857,0.366820493751264,0.366996048774033),.UNSPECIFIED.)
GEOMETRIC_REPRESENTATION_ITEM()
RATIONAL_B_SPLINE_SURFACE(((0.995079542144874,0.997234796441972,1.,0.996603060231143,
0.994126602224867,0.994126602224867,0.994126602224867),(0.995079542144874,
0.997234796441972,1.,0.996603060231143,0.994126602224867,0.994126602224867,
0.994126602224867)))
REPRESENTATION_ITEM('')
SURFACE()
);
#590=(
BOUNDED_SURFACE()
B_SPLINE_SURFACE(1,2,((#103107,#103108,#103109),(#103110,#103111,#103112)),
 .UNSPECIFIED.,.F.,.F.,.F.)
B_SPLINE_SURFACE_WITH_KNOTS((2,2),(3,3),(0.710192959008444,1.),(0.366820493751253,
0.384035903515168),.UNSPECIFIED.)
GEOMETRIC_REPRESENTATION_ITEM()
RATIONAL_B_SPLINE_SURFACE(((0.994126602224873,0.989721266390695,0.988228734781999),
(0.994126602224873,0.989721266390695,0.988228734781999)))
REPRESENTATION_ITEM('')
SURFACE()
);
#591=(
BOUNDED_SURFACE()
B_SPLINE_SURFACE(1,2,((#103121,#103122,#103123,#103124,#103125,#103126,
#103127),(#103128,#103129,#103130,#103131,#103132,#103133,#103134)),
 .UNSPECIFIED.,.F.,.F.,.F.)
B_SPLINE_SURFACE_WITH_KNOTS((2,2),(3,2,2,3),(0.710318915640079,1.),(0.349264991474406,
0.357142857142857,0.366820493751254,0.366996048774023),.UNSPECIFIED.)
GEOMETRIC_REPRESENTATION_ITEM()
RATIONAL_B_SPLINE_SURFACE(((0.995079542144872,0.997234796441971,1.,0.996603060231146,
0.994126602224873,0.994126602224873,0.994126602224873),(0.995079542144872,
0.997234796441971,1.,0.996603060231146,0.994126602224873,0.994126602224873,
0.994126602224873)))
REPRESENTATION_ITEM('')
SURFACE()
);
#592=(
BOUNDED_SURFACE()
B_SPLINE_SURFACE(1,2,((#103142,#103143,#103144),(#103145,#103146,#103147)),
 .UNSPECIFIED.,.F.,.F.,.F.)
B_SPLINE_SURFACE_WITH_KNOTS((2,2),(3,3),(0.71019295900816,1.),(0.366820493751253,
0.384035903515168),.UNSPECIFIED.)
GEOMETRIC_REPRESENTATION_ITEM()
RATIONAL_B_SPLINE_SURFACE(((0.994126602224873,0.989721266390694,0.988228734781998),
(0.994126602224873,0.989721266390694,0.988228734781998)))
REPRESENTATION_ITEM('')
SURFACE()
);
#593=(
BOUNDED_SURFACE()
B_SPLINE_SURFACE(1,2,((#103156,#103157,#103158,#103159,#103160,#103161,
#103162),(#103163,#103164,#103165,#103166,#103167,#103168,#103169)),
 .UNSPECIFIED.,.F.,.F.,.F.)
B_SPLINE_SURFACE_WITH_KNOTS((2,2),(3,2,2,3),(0.710318915639601,1.),(0.349264991474411,
0.357142857142857,0.366820493751254,0.366996048774023),.UNSPECIFIED.)
GEOMETRIC_REPRESENTATION_ITEM()
RATIONAL_B_SPLINE_SURFACE(((0.995079542144875,0.997234796441973,1.,0.996603060231146,
0.994126602224873,0.994126602224873,0.994126602224873),(0.995079542144875,
0.997234796441973,1.,0.996603060231146,0.994126602224873,0.994126602224873,
0.994126602224873)))
REPRESENTATION_ITEM('')
SURFACE()
);
#594=(
BOUNDED_SURFACE()
B_SPLINE_SURFACE(1,2,((#103177,#103178,#103179),(#103180,#103181,#103182)),
 .UNSPECIFIED.,.F.,.F.,.F.)
B_SPLINE_SURFACE_WITH_KNOTS((2,2),(3,3),(0.710192959007978,1.),(0.366820493751235,
0.384035903515169),.UNSPECIFIED.)
GEOMETRIC_REPRESENTATION_ITEM()
RATIONAL_B_SPLINE_SURFACE(((0.994126602224882,0.989721266390696,0.988228734781998),
(0.994126602224882,0.989721266390696,0.988228734781998)))
REPRESENTATION_ITEM('')
SURFACE()
);
#595=(
BOUNDED_SURFACE()
B_SPLINE_SURFACE(1,2,((#103191,#103192,#103193,#103194,#103195,#103196,
#103197),(#103198,#103199,#103200,#103201,#103202,#103203,#103204)),
 .UNSPECIFIED.,.F.,.F.,.F.)
B_SPLINE_SURFACE_WITH_KNOTS((2,2),(3,2,2,3),(0.710318915639618,1.),(0.34926499147441,
0.357142857142857,0.366820493751254,0.366996048774023),.UNSPECIFIED.)
GEOMETRIC_REPRESENTATION_ITEM()
RATIONAL_B_SPLINE_SURFACE(((0.995079542144874,0.997234796441972,1.,0.996603060231146,
0.994126602224873,0.994126602224873,0.994126602224873),(0.995079542144874,
0.997234796441972,1.,0.996603060231146,0.994126602224873,0.994126602224873,
0.994126602224873)))
REPRESENTATION_ITEM('')
SURFACE()
);
#596=(
BOUNDED_SURFACE()
B_SPLINE_SURFACE(1,2,((#103212,#103213,#103214),(#103215,#103216,#103217)),
 .UNSPECIFIED.,.F.,.F.,.F.)
B_SPLINE_SURFACE_WITH_KNOTS((2,2),(3,3),(0.710192959008014,1.),(0.366820493751253,
0.384035903515169),.UNSPECIFIED.)
GEOMETRIC_REPRESENTATION_ITEM()
RATIONAL_B_SPLINE_SURFACE(((0.994126602224873,0.989721266390694,0.988228734781998),
(0.994126602224873,0.989721266390694,0.988228734781998)))
REPRESENTATION_ITEM('')
SURFACE()
);
#597=(
BOUNDED_SURFACE()
B_SPLINE_SURFACE(1,2,((#103226,#103227,#103228,#103229,#103230,#103231,
#103232),(#103233,#103234,#103235,#103236,#103237,#103238,#103239)),
 .UNSPECIFIED.,.F.,.F.,.F.)
B_SPLINE_SURFACE_WITH_KNOTS((2,2),(3,2,2,3),(0.710318915639658,1.),(0.34926499147441,
0.357142857142857,0.366820493751254,0.366996048774023),.UNSPECIFIED.)
GEOMETRIC_REPRESENTATION_ITEM()
RATIONAL_B_SPLINE_SURFACE(((0.995079542144874,0.997234796441972,1.,0.996603060231146,
0.994126602224873,0.994126602224873,0.994126602224873),(0.995079542144874,
0.997234796441972,1.,0.996603060231146,0.994126602224873,0.994126602224873,
0.994126602224873)))
REPRESENTATION_ITEM('')
SURFACE()
);
#598=(
BOUNDED_SURFACE()
B_SPLINE_SURFACE(1,2,((#103247,#103248,#103249),(#103250,#103251,#103252)),
 .UNSPECIFIED.,.F.,.F.,.F.)
B_SPLINE_SURFACE_WITH_KNOTS((2,2),(3,3),(0.710192959008105,1.),(0.366820493751253,
0.384035903515169),.UNSPECIFIED.)
GEOMETRIC_REPRESENTATION_ITEM()
RATIONAL_B_SPLINE_SURFACE(((0.994126602224873,0.989721266390694,0.988228734781998),
(0.994126602224873,0.989721266390694,0.988228734781998)))
REPRESENTATION_ITEM('')
SURFACE()
);
#599=(
BOUNDED_SURFACE()
B_SPLINE_SURFACE(1,2,((#103261,#103262,#103263,#103264,#103265,#103266,
#103267),(#103268,#103269,#103270,#103271,#103272,#103273,#103274)),
 .UNSPECIFIED.,.F.,.F.,.F.)
B_SPLINE_SURFACE_WITH_KNOTS((2,2),(3,2,2,3),(0.710318915639747,1.),(0.34926499147441,
0.357142857142857,0.366820493751255,0.366996048774024),.UNSPECIFIED.)
GEOMETRIC_REPRESENTATION_ITEM()
RATIONAL_B_SPLINE_SURFACE(((0.995079542144874,0.997234796441972,1.,0.996603060231146,
0.994126602224872,0.994126602224872,0.994126602224872),(0.995079542144874,
0.997234796441972,1.,0.996603060231146,0.994126602224872,0.994126602224872,
0.994126602224872)))
REPRESENTATION_ITEM('')
SURFACE()
);
#600=(
BOUNDED_SURFACE()
B_SPLINE_SURFACE(1,2,((#103282,#103283,#103284),(#103285,#103286,#103287)),
 .UNSPECIFIED.,.F.,.F.,.F.)
B_SPLINE_SURFACE_WITH_KNOTS((2,2),(3,3),(0.,0.289681084359928),(0.297753987024565,
0.314942866188516),.UNSPECIFIED.)
GEOMETRIC_REPRESENTATION_ITEM()
RATIONAL_B_SPLINE_SURFACE(((0.99297255681853,0.98897304955565,0.987877375613931),
(0.99297255681853,0.98897304955565,0.987877375613931)))
REPRESENTATION_ITEM('')
SURFACE()
);
#601=(
BOUNDED_SURFACE()
B_SPLINE_SURFACE(1,2,((#103296,#103297,#103298,#103299,#103300),(#103301,
#103302,#103303,#103304,#103305)),.UNSPECIFIED.,.F.,.F.,.F.)
B_SPLINE_SURFACE_WITH_KNOTS((2,2),(3,2,3),(0.,0.289807040992001),(0.418312080773434,
0.428571428571429,0.435879799328077),.UNSPECIFIED.)
GEOMETRIC_REPRESENTATION_ITEM()
RATIONAL_B_SPLINE_SURFACE(((0.99383221411677,0.99639887423472,1.,0.997434694412141,
0.995394338545807),(0.99383221411677,0.99639887423472,1.,0.997434694412141,
0.995394338545807)))
REPRESENTATION_ITEM('')
SURFACE()
);
#602=(
BOUNDED_SURFACE()
B_SPLINE_SURFACE(1,2,((#103313,#103314,#103315),(#103316,#103317,#103318)),
 .UNSPECIFIED.,.F.,.F.,.F.)
B_SPLINE_SURFACE_WITH_KNOTS((2,2),(3,3),(0.,0.289681084359927),(0.297753987024626,
0.314942866188684),.UNSPECIFIED.)
GEOMETRIC_REPRESENTATION_ITEM()
RATIONAL_B_SPLINE_SURFACE(((0.992972556818501,0.988973049555607,0.98787737561391),
(0.992972556818501,0.988973049555607,0.98787737561391)))
REPRESENTATION_ITEM('')
SURFACE()
);
#603=(
BOUNDED_SURFACE()
B_SPLINE_SURFACE(1,2,((#103327,#103328,#103329,#103330,#103331),(#103332,
#103333,#103334,#103335,#103336)),.UNSPECIFIED.,.F.,.F.,.F.)
B_SPLINE_SURFACE_WITH_KNOTS((2,2),(3,2,3),(0.,0.289807040991563),(0.418312080773433,
0.428571428571429,0.435879799328076),.UNSPECIFIED.)
GEOMETRIC_REPRESENTATION_ITEM()
RATIONAL_B_SPLINE_SURFACE(((0.993832214116769,0.99639887423472,1.,0.997434694412141,
0.995394338545808),(0.993832214116769,0.99639887423472,1.,0.997434694412141,
0.995394338545808)))
REPRESENTATION_ITEM('')
SURFACE()
);
#604=(
BOUNDED_SURFACE()
B_SPLINE_SURFACE(1,2,((#103344,#103345,#103346),(#103347,#103348,#103349)),
 .UNSPECIFIED.,.F.,.F.,.F.)
B_SPLINE_SURFACE_WITH_KNOTS((2,2),(3,3),(0.,0.289681084359919),(0.297753987024627,
0.314942866188517),.UNSPECIFIED.)
GEOMETRIC_REPRESENTATION_ITEM()
RATIONAL_B_SPLINE_SURFACE(((0.992972556818501,0.988973049555646,0.987877375613931),
(0.992972556818501,0.988973049555646,0.987877375613931)))
REPRESENTATION_ITEM('')
SURFACE()
);
#605=(
BOUNDED_SURFACE()
B_SPLINE_SURFACE(1,2,((#103358,#103359,#103360,#103361,#103362),(#103363,
#103364,#103365,#103366,#103367)),.UNSPECIFIED.,.F.,.F.,.F.)
B_SPLINE_SURFACE_WITH_KNOTS((2,2),(3,2,3),(0.,0.289807040991555),(0.418312080773433,
0.428571428571429,0.435879799328076),.UNSPECIFIED.)
GEOMETRIC_REPRESENTATION_ITEM()
RATIONAL_B_SPLINE_SURFACE(((0.993832214116769,0.99639887423472,1.,0.997434694412141,
0.995394338545808),(0.993832214116769,0.99639887423472,1.,0.997434694412141,
0.995394338545808)))
REPRESENTATION_ITEM('')
SURFACE()
);
#606=(
BOUNDED_SURFACE()
B_SPLINE_SURFACE(1,2,((#103375,#103376,#103377),(#103378,#103379,#103380)),
 .UNSPECIFIED.,.F.,.F.,.F.)
B_SPLINE_SURFACE_WITH_KNOTS((2,2),(3,3),(0.,0.289681084359924),(0.297753987024233,
0.314942866188517),.UNSPECIFIED.)
GEOMETRIC_REPRESENTATION_ITEM()
RATIONAL_B_SPLINE_SURFACE(((0.992972556818685,0.988973049555671,0.987877375613931),
(0.992972556818685,0.988973049555671,0.987877375613931)))
REPRESENTATION_ITEM('')
SURFACE()
);
#607=(
BOUNDED_SURFACE()
B_SPLINE_SURFACE(1,2,((#103389,#103390,#103391,#103392,#103393),(#103394,
#103395,#103396,#103397,#103398)),.UNSPECIFIED.,.F.,.F.,.F.)
B_SPLINE_SURFACE_WITH_KNOTS((2,2),(3,2,3),(0.,0.289807040991561),(0.418312080773433,
0.428571428571429,0.435879799328076),.UNSPECIFIED.)
GEOMETRIC_REPRESENTATION_ITEM()
RATIONAL_B_SPLINE_SURFACE(((0.993832214116769,0.99639887423472,1.,0.997434694412141,
0.995394338545808),(0.993832214116769,0.99639887423472,1.,0.997434694412141,
0.995394338545808)))
REPRESENTATION_ITEM('')
SURFACE()
);
#608=(
BOUNDED_SURFACE()
B_SPLINE_SURFACE(1,2,((#103406,#103407,#103408),(#103409,#103410,#103411)),
 .UNSPECIFIED.,.F.,.F.,.F.)
B_SPLINE_SURFACE_WITH_KNOTS((2,2),(3,3),(0.,0.28968108435992),(0.297753987024627,
0.314942866188517),.UNSPECIFIED.)
GEOMETRIC_REPRESENTATION_ITEM()
RATIONAL_B_SPLINE_SURFACE(((0.992972556818501,0.988973049555646,0.987877375613931),
(0.992972556818501,0.988973049555646,0.987877375613931)))
REPRESENTATION_ITEM('')
SURFACE()
);
#609=(
BOUNDED_SURFACE()
B_SPLINE_SURFACE(1,2,((#103420,#103421,#103422,#103423,#103424),(#103425,
#103426,#103427,#103428,#103429)),.UNSPECIFIED.,.F.,.F.,.F.)
B_SPLINE_SURFACE_WITH_KNOTS((2,2),(3,2,3),(0.,0.289807040991644),(0.418312080773434,
0.428571428571429,0.435879799328076),.UNSPECIFIED.)
GEOMETRIC_REPRESENTATION_ITEM()
RATIONAL_B_SPLINE_SURFACE(((0.99383221411677,0.99639887423472,1.,0.997434694412141,
0.995394338545808),(0.99383221411677,0.99639887423472,1.,0.997434694412141,
0.995394338545808)))
REPRESENTATION_ITEM('')
SURFACE()
);
#610=(
BOUNDED_SURFACE()
B_SPLINE_SURFACE(1,2,((#103437,#103438,#103439),(#103440,#103441,#103442)),
 .UNSPECIFIED.,.F.,.F.,.F.)
B_SPLINE_SURFACE_WITH_KNOTS((2,2),(3,3),(0.,0.289681084359923),(0.297753987024626,
0.314942866188516),.UNSPECIFIED.)
GEOMETRIC_REPRESENTATION_ITEM()
RATIONAL_B_SPLINE_SURFACE(((0.992972556818502,0.988973049555646,0.987877375613931),
(0.992972556818502,0.988973049555646,0.987877375613931)))
REPRESENTATION_ITEM('')
SURFACE()
);
#611=(
BOUNDED_SURFACE()
B_SPLINE_SURFACE(1,2,((#103451,#103452,#103453,#103454,#103455),(#103456,
#103457,#103458,#103459,#103460)),.UNSPECIFIED.,.F.,.F.,.F.)
B_SPLINE_SURFACE_WITH_KNOTS((2,2),(3,2,3),(0.,0.289807040991639),(0.418312080773434,
0.428571428571429,0.435879799328077),.UNSPECIFIED.)
GEOMETRIC_REPRESENTATION_ITEM()
RATIONAL_B_SPLINE_SURFACE(((0.99383221411677,0.996398874234721,1.,0.997434694412141,
0.995394338545807),(0.99383221411677,0.996398874234721,1.,0.997434694412141,
0.995394338545807)))
REPRESENTATION_ITEM('')
SURFACE()
);
#612=(
BOUNDED_SURFACE()
B_SPLINE_SURFACE(1,2,((#103468,#103469,#103470),(#103471,#103472,#103473)),
 .UNSPECIFIED.,.F.,.F.,.F.)
B_SPLINE_SURFACE_WITH_KNOTS((2,2),(3,3),(0.,0.289681084359918),(0.297753987024234,
0.314942866188516),.UNSPECIFIED.)
GEOMETRIC_REPRESENTATION_ITEM()
RATIONAL_B_SPLINE_SURFACE(((0.992972556818684,0.988973049555671,0.987877375613931),
(0.992972556818684,0.988973049555671,0.987877375613931)))
REPRESENTATION_ITEM('')
SURFACE()
);
#613=(
BOUNDED_SURFACE()
B_SPLINE_SURFACE(1,2,((#103482,#103483,#103484,#103485,#103486),(#103487,
#103488,#103489,#103490,#103491)),.UNSPECIFIED.,.F.,.F.,.F.)
B_SPLINE_SURFACE_WITH_KNOTS((2,2),(3,2,3),(0.,0.289807040991643),(0.418312080773434,
0.428571428571429,0.435879799328077),.UNSPECIFIED.)
GEOMETRIC_REPRESENTATION_ITEM()
RATIONAL_B_SPLINE_SURFACE(((0.99383221411677,0.99639887423472,1.,0.997434694412141,
0.995394338545807),(0.99383221411677,0.99639887423472,1.,0.997434694412141,
0.995394338545807)))
REPRESENTATION_ITEM('')
SURFACE()
);
#614=(
BOUNDED_SURFACE()
B_SPLINE_SURFACE(1,2,((#103499,#103500,#103501),(#103502,#103503,#103504)),
 .UNSPECIFIED.,.F.,.F.,.F.)
B_SPLINE_SURFACE_WITH_KNOTS((2,2),(3,3),(0.,0.289681084359921),(0.297753987024234,
0.314942866188516),.UNSPECIFIED.)
GEOMETRIC_REPRESENTATION_ITEM()
RATIONAL_B_SPLINE_SURFACE(((0.992972556818684,0.988973049555671,0.987877375613931),
(0.992972556818684,0.988973049555671,0.987877375613931)))
REPRESENTATION_ITEM('')
SURFACE()
);
#615=(
BOUNDED_SURFACE()
B_SPLINE_SURFACE(1,2,((#103513,#103514,#103515,#103516,#103517),(#103518,
#103519,#103520,#103521,#103522)),.UNSPECIFIED.,.F.,.F.,.F.)
B_SPLINE_SURFACE_WITH_KNOTS((2,2),(3,2,3),(0.,0.289807040991642),(0.418312080773434,
0.428571428571429,0.435879799328077),.UNSPECIFIED.)
GEOMETRIC_REPRESENTATION_ITEM()
RATIONAL_B_SPLINE_SURFACE(((0.99383221411677,0.996398874234721,1.,0.997434694412141,
0.995394338545807),(0.99383221411677,0.996398874234721,1.,0.997434694412141,
0.995394338545807)))
REPRESENTATION_ITEM('')
SURFACE()
);
#616=(
BOUNDED_SURFACE()
B_SPLINE_SURFACE(1,2,((#103530,#103531,#103532),(#103533,#103534,#103535)),
 .UNSPECIFIED.,.F.,.F.,.F.)
B_SPLINE_SURFACE_WITH_KNOTS((2,2),(3,3),(0.,0.289681084359921),(0.297753987024245,
0.314942866188516),.UNSPECIFIED.)
GEOMETRIC_REPRESENTATION_ITEM()
RATIONAL_B_SPLINE_SURFACE(((0.992972556818679,0.988973049555671,0.987877375613931),
(0.992972556818679,0.988973049555671,0.987877375613931)))
REPRESENTATION_ITEM('')
SURFACE()
);
#617=(
BOUNDED_SURFACE()
B_SPLINE_SURFACE(1,2,((#103544,#103545,#103546,#103547,#103548),(#103549,
#103550,#103551,#103552,#103553)),.UNSPECIFIED.,.F.,.F.,.F.)
B_SPLINE_SURFACE_WITH_KNOTS((2,2),(3,2,3),(0.,0.28980704099156),(0.418312080773434,
0.428571428571429,0.435879799328077),.UNSPECIFIED.)
GEOMETRIC_REPRESENTATION_ITEM()
RATIONAL_B_SPLINE_SURFACE(((0.99383221411677,0.996398874234721,1.,0.997434694412141,
0.995394338545807),(0.99383221411677,0.996398874234721,1.,0.997434694412141,
0.995394338545807)))
REPRESENTATION_ITEM('')
SURFACE()
);
#618=(
BOUNDED_SURFACE()
B_SPLINE_SURFACE(1,2,((#103561,#103562,#103563),(#103564,#103565,#103566)),
 .UNSPECIFIED.,.F.,.F.,.F.)
B_SPLINE_SURFACE_WITH_KNOTS((2,2),(3,3),(0.,0.289681084359924),(0.297753987024626,
0.314942866188516),.UNSPECIFIED.)
GEOMETRIC_REPRESENTATION_ITEM()
RATIONAL_B_SPLINE_SURFACE(((0.992972556818502,0.988973049555647,0.987877375613931),
(0.992972556818502,0.988973049555647,0.987877375613931)))
REPRESENTATION_ITEM('')
SURFACE()
);
#619=(
BOUNDED_SURFACE()
B_SPLINE_SURFACE(1,2,((#103575,#103576,#103577,#103578,#103579),(#103580,
#103581,#103582,#103583,#103584)),.UNSPECIFIED.,.F.,.F.,.F.)
B_SPLINE_SURFACE_WITH_KNOTS((2,2),(3,2,3),(0.,0.289807040991648),(0.418312080773434,
0.428571428571429,0.435879799328077),.UNSPECIFIED.)
GEOMETRIC_REPRESENTATION_ITEM()
RATIONAL_B_SPLINE_SURFACE(((0.99383221411677,0.996398874234721,1.,0.997434694412141,
0.995394338545807),(0.99383221411677,0.996398874234721,1.,0.997434694412141,
0.995394338545807)))
REPRESENTATION_ITEM('')
SURFACE()
);
#620=(
BOUNDED_SURFACE()
B_SPLINE_SURFACE(1,2,((#103592,#103593,#103594),(#103595,#103596,#103597)),
 .UNSPECIFIED.,.F.,.F.,.F.)
B_SPLINE_SURFACE_WITH_KNOTS((2,2),(3,3),(0.,0.289681084359922),(0.297753987024626,
0.314942866188516),.UNSPECIFIED.)
GEOMETRIC_REPRESENTATION_ITEM()
RATIONAL_B_SPLINE_SURFACE(((0.992972556818502,0.988973049555646,0.987877375613931),
(0.992972556818502,0.988973049555646,0.987877375613931)))
REPRESENTATION_ITEM('')
SURFACE()
);
#621=(
BOUNDED_SURFACE()
B_SPLINE_SURFACE(1,2,((#103606,#103607,#103608,#103609,#103610),(#103611,
#103612,#103613,#103614,#103615)),.UNSPECIFIED.,.F.,.F.,.F.)
B_SPLINE_SURFACE_WITH_KNOTS((2,2),(3,2,3),(0.,0.289807040991562),(0.418312080773434,
0.428571428571429,0.435879799328077),.UNSPECIFIED.)
GEOMETRIC_REPRESENTATION_ITEM()
RATIONAL_B_SPLINE_SURFACE(((0.99383221411677,0.99639887423472,1.,0.997434694412141,
0.995394338545807),(0.99383221411677,0.99639887423472,1.,0.997434694412141,
0.995394338545807)))
REPRESENTATION_ITEM('')
SURFACE()
);
#622=(
BOUNDED_SURFACE()
B_SPLINE_SURFACE(1,2,((#103623,#103624,#103625),(#103626,#103627,#103628)),
 .UNSPECIFIED.,.F.,.F.,.F.)
B_SPLINE_SURFACE_WITH_KNOTS((2,2),(3,3),(0.,0.289681084359921),(0.297753987024245,
0.314942866188516),.UNSPECIFIED.)
GEOMETRIC_REPRESENTATION_ITEM()
RATIONAL_B_SPLINE_SURFACE(((0.992972556818679,0.988973049555671,0.987877375613931),
(0.992972556818679,0.988973049555671,0.987877375613931)))
REPRESENTATION_ITEM('')
SURFACE()
);
#623=(
BOUNDED_SURFACE()
B_SPLINE_SURFACE(1,2,((#103637,#103638,#103639,#103640,#103641),(#103642,
#103643,#103644,#103645,#103646)),.UNSPECIFIED.,.F.,.F.,.F.)
B_SPLINE_SURFACE_WITH_KNOTS((2,2),(3,2,3),(0.,0.289807040991916),(0.418312080773434,
0.428571428571429,0.435879799328077),.UNSPECIFIED.)
GEOMETRIC_REPRESENTATION_ITEM()
RATIONAL_B_SPLINE_SURFACE(((0.99383221411677,0.996398874234721,1.,0.997434694412141,
0.995394338545807),(0.99383221411677,0.996398874234721,1.,0.997434694412141,
0.995394338545807)))
REPRESENTATION_ITEM('')
SURFACE()
);
#624=(
BOUNDED_SURFACE()
B_SPLINE_SURFACE(1,2,((#103654,#103655,#103656),(#103657,#103658,#103659)),
 .UNSPECIFIED.,.F.,.F.,.F.)
B_SPLINE_SURFACE_WITH_KNOTS((2,2),(3,3),(0.,0.28968108435992),(0.297753987024247,
0.314942866188516),.UNSPECIFIED.)
GEOMETRIC_REPRESENTATION_ITEM()
RATIONAL_B_SPLINE_SURFACE(((0.992972556818678,0.988973049555671,0.987877375613931),
(0.992972556818678,0.98897304955567,0.987877375613931)))
REPRESENTATION_ITEM('')
SURFACE()
);
#625=(
BOUNDED_SURFACE()
B_SPLINE_SURFACE(1,2,((#103668,#103669,#103670,#103671,#103672),(#103673,
#103674,#103675,#103676,#103677)),.UNSPECIFIED.,.F.,.F.,.F.)
B_SPLINE_SURFACE_WITH_KNOTS((2,2),(3,2,3),(0.,0.28980704099297),(0.418312080773434,
0.428571428571429,0.435879799328077),.UNSPECIFIED.)
GEOMETRIC_REPRESENTATION_ITEM()
RATIONAL_B_SPLINE_SURFACE(((0.99383221411677,0.996398874234721,1.,0.997434694412141,
0.995394338545807),(0.99383221411677,0.996398874234721,1.,0.997434694412141,
0.995394338545807)))
REPRESENTATION_ITEM('')
SURFACE()
);
#626=(
BOUNDED_SURFACE()
B_SPLINE_SURFACE(1,2,((#103685,#103686,#103687),(#103688,#103689,#103690)),
 .UNSPECIFIED.,.F.,.F.,.F.)
B_SPLINE_SURFACE_WITH_KNOTS((2,2),(3,3),(0.,0.28968108435992),(0.297753987024626,
0.314942866188516),.UNSPECIFIED.)
GEOMETRIC_REPRESENTATION_ITEM()
RATIONAL_B_SPLINE_SURFACE(((0.992972556818502,0.988973049555647,0.987877375613931),
(0.992972556818502,0.988973049555647,0.987877375613931)))
REPRESENTATION_ITEM('')
SURFACE()
);
#627=(
BOUNDED_SURFACE()
B_SPLINE_SURFACE(1,2,((#103699,#103700,#103701,#103702,#103703),(#103704,
#103705,#103706,#103707,#103708)),.UNSPECIFIED.,.F.,.F.,.F.)
B_SPLINE_SURFACE_WITH_KNOTS((2,2),(3,2,3),(0.,0.289807040991686),(0.418312080773434,
0.428571428571429,0.435879799328077),.UNSPECIFIED.)
GEOMETRIC_REPRESENTATION_ITEM()
RATIONAL_B_SPLINE_SURFACE(((0.99383221411677,0.99639887423472,1.,0.997434694412141,
0.995394338545807),(0.99383221411677,0.99639887423472,1.,0.997434694412141,
0.995394338545807)))
REPRESENTATION_ITEM('')
SURFACE()
);
#628=(
BOUNDED_SURFACE()
B_SPLINE_SURFACE(1,2,((#103716,#103717,#103718),(#103719,#103720,#103721)),
 .UNSPECIFIED.,.F.,.F.,.F.)
B_SPLINE_SURFACE_WITH_KNOTS((2,2),(3,3),(0.,0.289681084359925),(0.297753987024473,
0.314942866188516),.UNSPECIFIED.)
GEOMETRIC_REPRESENTATION_ITEM()
RATIONAL_B_SPLINE_SURFACE(((0.992972556818573,0.988973049555656,0.987877375613931),
(0.992972556818573,0.988973049555656,0.987877375613931)))
REPRESENTATION_ITEM('')
SURFACE()
);
#629=(
BOUNDED_SURFACE()
B_SPLINE_SURFACE(1,2,((#103730,#103731,#103732,#103733,#103734),(#103735,
#103736,#103737,#103738,#103739)),.UNSPECIFIED.,.F.,.F.,.F.)
B_SPLINE_SURFACE_WITH_KNOTS((2,2),(3,2,3),(0.,0.289807040991566),(0.418312080773433,
0.428571428571429,0.435879799328077),.UNSPECIFIED.)
GEOMETRIC_REPRESENTATION_ITEM()
RATIONAL_B_SPLINE_SURFACE(((0.99383221411677,0.99639887423472,1.,0.997434694412141,
0.995394338545807),(0.99383221411677,0.99639887423472,1.,0.997434694412141,
0.995394338545807)))
REPRESENTATION_ITEM('')
SURFACE()
);
#630=(
BOUNDED_SURFACE()
B_SPLINE_SURFACE(1,2,((#103747,#103748,#103749),(#103750,#103751,#103752)),
 .UNSPECIFIED.,.F.,.F.,.F.)
B_SPLINE_SURFACE_WITH_KNOTS((2,2),(3,3),(0.,0.289681084359922),(0.297753987024626,
0.314942866188516),.UNSPECIFIED.)
GEOMETRIC_REPRESENTATION_ITEM()
RATIONAL_B_SPLINE_SURFACE(((0.992972556818502,0.988973049555646,0.987877375613931),
(0.992972556818502,0.988973049555646,0.987877375613931)))
REPRESENTATION_ITEM('')
SURFACE()
);
#631=(
BOUNDED_SURFACE()
B_SPLINE_SURFACE(1,2,((#103761,#103762,#103763,#103764,#103765),(#103766,
#103767,#103768,#103769,#103770)),.UNSPECIFIED.,.F.,.F.,.F.)
B_SPLINE_SURFACE_WITH_KNOTS((2,2),(3,2,3),(0.,0.289807040991795),(0.418312080773434,
0.428571428571429,0.435879799328077),.UNSPECIFIED.)
GEOMETRIC_REPRESENTATION_ITEM()
RATIONAL_B_SPLINE_SURFACE(((0.99383221411677,0.996398874234721,1.,0.997434694412141,
0.995394338545807),(0.99383221411677,0.996398874234721,1.,0.997434694412141,
0.995394338545807)))
REPRESENTATION_ITEM('')
SURFACE()
);
#632=(
BOUNDED_SURFACE()
B_SPLINE_SURFACE(1,2,((#103778,#103779,#103780),(#103781,#103782,#103783)),
 .UNSPECIFIED.,.F.,.F.,.F.)
B_SPLINE_SURFACE_WITH_KNOTS((2,2),(3,3),(0.,0.289681084359927),(0.297753987024626,
0.314942866188516),.UNSPECIFIED.)
GEOMETRIC_REPRESENTATION_ITEM()
RATIONAL_B_SPLINE_SURFACE(((0.992972556818501,0.988973049555646,0.987877375613931),
(0.992972556818501,0.988973049555646,0.987877375613931)))
REPRESENTATION_ITEM('')
SURFACE()
);
#633=(
BOUNDED_SURFACE()
B_SPLINE_SURFACE(1,2,((#103792,#103793,#103794,#103795,#103796),(#103797,
#103798,#103799,#103800,#103801)),.UNSPECIFIED.,.F.,.F.,.F.)
B_SPLINE_SURFACE_WITH_KNOTS((2,2),(3,2,3),(0.,0.28980704099156),(0.418312080773434,
0.428571428571429,0.435879799328077),.UNSPECIFIED.)
GEOMETRIC_REPRESENTATION_ITEM()
RATIONAL_B_SPLINE_SURFACE(((0.99383221411677,0.996398874234721,1.,0.997434694412141,
0.995394338545807),(0.99383221411677,0.996398874234721,1.,0.997434694412141,
0.995394338545807)))
REPRESENTATION_ITEM('')
SURFACE()
);
#634=(
BOUNDED_SURFACE()
B_SPLINE_SURFACE(1,2,((#103809,#103810,#103811),(#103812,#103813,#103814)),
 .UNSPECIFIED.,.F.,.F.,.F.)
B_SPLINE_SURFACE_WITH_KNOTS((2,2),(3,3),(0.,0.289681084359927),(0.297753987024626,
0.314942866188516),.UNSPECIFIED.)
GEOMETRIC_REPRESENTATION_ITEM()
RATIONAL_B_SPLINE_SURFACE(((0.992972556818502,0.988973049555646,0.987877375613931),
(0.992972556818502,0.988973049555646,0.987877375613931)))
REPRESENTATION_ITEM('')
SURFACE()
);
#635=(
BOUNDED_SURFACE()
B_SPLINE_SURFACE(1,2,((#103823,#103824,#103825,#103826,#103827),(#103828,
#103829,#103830,#103831,#103832)),.UNSPECIFIED.,.F.,.F.,.F.)
B_SPLINE_SURFACE_WITH_KNOTS((2,2),(3,2,3),(0.,0.289807040992696),(0.418312080773434,
0.428571428571429,0.435879799328077),.UNSPECIFIED.)
GEOMETRIC_REPRESENTATION_ITEM()
RATIONAL_B_SPLINE_SURFACE(((0.99383221411677,0.996398874234721,1.,0.997434694412141,
0.995394338545807),(0.99383221411677,0.996398874234721,1.,0.997434694412141,
0.995394338545807)))
REPRESENTATION_ITEM('')
SURFACE()
);
#636=(
BOUNDED_SURFACE()
B_SPLINE_SURFACE(1,2,((#103840,#103841,#103842),(#103843,#103844,#103845)),
 .UNSPECIFIED.,.F.,.F.,.F.)
B_SPLINE_SURFACE_WITH_KNOTS((2,2),(3,3),(0.,0.289681084359927),(0.297753987024626,
0.314942866188516),.UNSPECIFIED.)
GEOMETRIC_REPRESENTATION_ITEM()
RATIONAL_B_SPLINE_SURFACE(((0.992972556818502,0.988973049555646,0.987877375613931),
(0.992972556818502,0.988973049555646,0.987877375613931)))
REPRESENTATION_ITEM('')
SURFACE()
);
#637=(
BOUNDED_SURFACE()
B_SPLINE_SURFACE(1,2,((#103854,#103855,#103856,#103857,#103858),(#103859,
#103860,#103861,#103862,#103863)),.UNSPECIFIED.,.F.,.F.,.F.)
B_SPLINE_SURFACE_WITH_KNOTS((2,2),(3,2,3),(0.,0.289807040992534),(0.418312080773434,
0.428571428571429,0.435879799328077),.UNSPECIFIED.)
GEOMETRIC_REPRESENTATION_ITEM()
RATIONAL_B_SPLINE_SURFACE(((0.99383221411677,0.996398874234721,1.,0.997434694412141,
0.995394338545807),(0.99383221411677,0.996398874234721,1.,0.997434694412141,
0.995394338545807)))
REPRESENTATION_ITEM('')
SURFACE()
);
#638=(
BOUNDED_SURFACE()
B_SPLINE_SURFACE(1,2,((#103871,#103872,#103873),(#103874,#103875,#103876)),
 .UNSPECIFIED.,.F.,.F.,.F.)
B_SPLINE_SURFACE_WITH_KNOTS((2,2),(3,3),(0.,0.289681084359924),(0.297753987024145,
0.314942866188516),.UNSPECIFIED.)
GEOMETRIC_REPRESENTATION_ITEM()
RATIONAL_B_SPLINE_SURFACE(((0.992972556818725,0.988973049555677,0.987877375613931),
(0.992972556818725,0.988973049555677,0.987877375613931)))
REPRESENTATION_ITEM('')
SURFACE()
);
#639=(
BOUNDED_SURFACE()
B_SPLINE_SURFACE(1,2,((#103885,#103886,#103887,#103888,#103889),(#103890,
#103891,#103892,#103893,#103894)),.UNSPECIFIED.,.F.,.F.,.F.)
B_SPLINE_SURFACE_WITH_KNOTS((2,2),(3,2,3),(0.,0.289807040992668),(0.418312080773434,
0.428571428571429,0.435879799328077),.UNSPECIFIED.)
GEOMETRIC_REPRESENTATION_ITEM()
RATIONAL_B_SPLINE_SURFACE(((0.99383221411677,0.996398874234721,1.,0.997434694412141,
0.995394338545807),(0.99383221411677,0.996398874234721,1.,0.997434694412141,
0.995394338545807)))
REPRESENTATION_ITEM('')
SURFACE()
);
#640=(
BOUNDED_SURFACE()
B_SPLINE_SURFACE(1,2,((#103902,#103903,#103904),(#103905,#103906,#103907)),
 .UNSPECIFIED.,.F.,.F.,.F.)
B_SPLINE_SURFACE_WITH_KNOTS((2,2),(3,3),(0.,0.28968108435992),(0.297753987024274,
0.314942866188516),.UNSPECIFIED.)
GEOMETRIC_REPRESENTATION_ITEM()
RATIONAL_B_SPLINE_SURFACE(((0.992972556818666,0.988973049555669,0.987877375613931),
(0.992972556818666,0.988973049555669,0.987877375613932)))
REPRESENTATION_ITEM('')
SURFACE()
);
#641=(
BOUNDED_SURFACE()
B_SPLINE_SURFACE(1,2,((#103916,#103917,#103918,#103919,#103920),(#103921,
#103922,#103923,#103924,#103925)),.UNSPECIFIED.,.F.,.F.,.F.)
B_SPLINE_SURFACE_WITH_KNOTS((2,2),(3,2,3),(0.,0.289807040991766),(0.418312080773434,
0.428571428571429,0.435879799328077),.UNSPECIFIED.)
GEOMETRIC_REPRESENTATION_ITEM()
RATIONAL_B_SPLINE_SURFACE(((0.99383221411677,0.996398874234721,1.,0.997434694412141,
0.995394338545807),(0.99383221411677,0.996398874234721,1.,0.997434694412141,
0.995394338545807)))
REPRESENTATION_ITEM('')
SURFACE()
);
#642=(
BOUNDED_SURFACE()
B_SPLINE_SURFACE(1,2,((#103933,#103934,#103935),(#103936,#103937,#103938)),
 .UNSPECIFIED.,.F.,.F.,.F.)
B_SPLINE_SURFACE_WITH_KNOTS((2,2),(3,3),(0.,0.289681084359923),(0.297753987024625,
0.314942866188631),.UNSPECIFIED.)
GEOMETRIC_REPRESENTATION_ITEM()
RATIONAL_B_SPLINE_SURFACE(((0.992972556818502,0.98897304955562,0.987877375613917),
(0.992972556818502,0.98897304955562,0.987877375613917)))
REPRESENTATION_ITEM('')
SURFACE()
);
#643=(
BOUNDED_SURFACE()
B_SPLINE_SURFACE(1,2,((#103947,#103948,#103949,#103950,#103951),(#103952,
#103953,#103954,#103955,#103956)),.UNSPECIFIED.,.F.,.F.,.F.)
B_SPLINE_SURFACE_WITH_KNOTS((2,2),(3,2,3),(0.,0.289807040992909),(0.418312080773434,
0.428571428571429,0.435879799328077),.UNSPECIFIED.)
GEOMETRIC_REPRESENTATION_ITEM()
RATIONAL_B_SPLINE_SURFACE(((0.99383221411677,0.996398874234721,1.,0.997434694412141,
0.995394338545807),(0.99383221411677,0.996398874234721,1.,0.997434694412141,
0.995394338545807)))
REPRESENTATION_ITEM('')
SURFACE()
);
#644=(
BOUNDED_SURFACE()
B_SPLINE_SURFACE(1,2,((#103964,#103965,#103966),(#103967,#103968,#103969)),
 .UNSPECIFIED.,.F.,.F.,.F.)
B_SPLINE_SURFACE_WITH_KNOTS((2,2),(3,3),(0.,0.289681084359929),(0.297753987024626,
0.314942866188516),.UNSPECIFIED.)
GEOMETRIC_REPRESENTATION_ITEM()
RATIONAL_B_SPLINE_SURFACE(((0.992972556818501,0.988973049555646,0.987877375613931),
(0.992972556818501,0.988973049555646,0.987877375613931)))
REPRESENTATION_ITEM('')
SURFACE()
);
#645=(
BOUNDED_SURFACE()
B_SPLINE_SURFACE(1,2,((#103978,#103979,#103980,#103981,#103982),(#103983,
#103984,#103985,#103986,#103987)),.UNSPECIFIED.,.F.,.F.,.F.)
B_SPLINE_SURFACE_WITH_KNOTS((2,2),(3,2,3),(0.,0.28980704099269),(0.418312080773434,
0.428571428571429,0.435879799328077),.UNSPECIFIED.)
GEOMETRIC_REPRESENTATION_ITEM()
RATIONAL_B_SPLINE_SURFACE(((0.99383221411677,0.99639887423472,1.,0.997434694412141,
0.995394338545807),(0.99383221411677,0.99639887423472,1.,0.997434694412141,
0.995394338545807)))
REPRESENTATION_ITEM('')
SURFACE()
);
#646=(
BOUNDED_SURFACE()
B_SPLINE_SURFACE(1,2,((#103995,#103996,#103997),(#103998,#103999,#104000)),
 .UNSPECIFIED.,.F.,.F.,.F.)
B_SPLINE_SURFACE_WITH_KNOTS((2,2),(3,3),(0.,0.289681084359937),(0.297753987024626,
0.314942866188516),.UNSPECIFIED.)
GEOMETRIC_REPRESENTATION_ITEM()
RATIONAL_B_SPLINE_SURFACE(((0.992972556818501,0.988973049555646,0.987877375613931),
(0.992972556818501,0.988973049555646,0.987877375613931)))
REPRESENTATION_ITEM('')
SURFACE()
);
#647=(
BOUNDED_SURFACE()
B_SPLINE_SURFACE(1,2,((#104009,#104010,#104011,#104012,#104013),(#104014,
#104015,#104016,#104017,#104018)),.UNSPECIFIED.,.F.,.F.,.F.)
B_SPLINE_SURFACE_WITH_KNOTS((2,2),(3,2,3),(0.,0.289807040992446),(0.418312080773434,
0.428571428571429,0.435879799328077),.UNSPECIFIED.)
GEOMETRIC_REPRESENTATION_ITEM()
RATIONAL_B_SPLINE_SURFACE(((0.99383221411677,0.996398874234721,1.,0.997434694412141,
0.995394338545807),(0.99383221411677,0.996398874234721,1.,0.997434694412141,
0.995394338545807)))
REPRESENTATION_ITEM('')
SURFACE()
);
#648=(
BOUNDED_SURFACE()
B_SPLINE_SURFACE(1,2,((#104026,#104027,#104028),(#104029,#104030,#104031)),
 .UNSPECIFIED.,.F.,.F.,.F.)
B_SPLINE_SURFACE_WITH_KNOTS((2,2),(3,3),(0.,0.289681084359928),(0.297753987024165,
0.314942866188516),.UNSPECIFIED.)
GEOMETRIC_REPRESENTATION_ITEM()
RATIONAL_B_SPLINE_SURFACE(((0.992972556818716,0.988973049555676,0.987877375613931),
(0.992972556818716,0.988973049555676,0.987877375613931)))
REPRESENTATION_ITEM('')
SURFACE()
);
#649=(
BOUNDED_SURFACE()
B_SPLINE_SURFACE(1,2,((#104040,#104041,#104042,#104043,#104044),(#104045,
#104046,#104047,#104048,#104049)),.UNSPECIFIED.,.F.,.F.,.F.)
B_SPLINE_SURFACE_WITH_KNOTS((2,2),(3,2,3),(0.,0.289807040992323),(0.418312080773434,
0.428571428571429,0.43587979932776),.UNSPECIFIED.)
GEOMETRIC_REPRESENTATION_ITEM()
RATIONAL_B_SPLINE_SURFACE(((0.99383221411677,0.996398874234721,1.,0.997434694412253,
0.995394338545984),(0.99383221411677,0.996398874234721,1.,0.997434694412253,
0.995394338545984)))
REPRESENTATION_ITEM('')
SURFACE()
);
#650=(
BOUNDED_SURFACE()
B_SPLINE_SURFACE(1,2,((#104057,#104058,#104059),(#104060,#104061,#104062)),
 .UNSPECIFIED.,.F.,.F.,.F.)
B_SPLINE_SURFACE_WITH_KNOTS((2,2),(3,3),(0.,0.289681084359923),(0.297753987024626,
0.314942866188518),.UNSPECIFIED.)
GEOMETRIC_REPRESENTATION_ITEM()
RATIONAL_B_SPLINE_SURFACE(((0.992972556818501,0.988973049555646,0.987877375613931),
(0.992972556818501,0.988973049555646,0.987877375613931)))
REPRESENTATION_ITEM('')
SURFACE()
);
#651=(
BOUNDED_SURFACE()
B_SPLINE_SURFACE(1,2,((#104071,#104072,#104073,#104074,#104075),(#104076,
#104077,#104078,#104079,#104080)),.UNSPECIFIED.,.F.,.F.,.F.)
B_SPLINE_SURFACE_WITH_KNOTS((2,2),(3,2,3),(0.,0.289807040992806),(0.418312080773434,
0.428571428571429,0.435879799328077),.UNSPECIFIED.)
GEOMETRIC_REPRESENTATION_ITEM()
RATIONAL_B_SPLINE_SURFACE(((0.99383221411677,0.99639887423472,1.,0.997434694412141,
0.995394338545807),(0.99383221411677,0.99639887423472,1.,0.997434694412141,
0.995394338545807)))
REPRESENTATION_ITEM('')
SURFACE()
);
#652=(
BOUNDED_SURFACE()
B_SPLINE_SURFACE(1,2,((#104088,#104089,#104090),(#104091,#104092,#104093)),
 .UNSPECIFIED.,.F.,.F.,.F.)
B_SPLINE_SURFACE_WITH_KNOTS((2,2),(3,3),(0.,0.289681084359917),(0.297753987024276,
0.314942866188516),.UNSPECIFIED.)
GEOMETRIC_REPRESENTATION_ITEM()
RATIONAL_B_SPLINE_SURFACE(((0.992972556818665,0.988973049555669,0.987877375613931),
(0.992972556818665,0.988973049555669,0.987877375613931)))
REPRESENTATION_ITEM('')
SURFACE()
);
#653=(
BOUNDED_SURFACE()
B_SPLINE_SURFACE(1,2,((#104102,#104103,#104104,#104105,#104106),(#104107,
#104108,#104109,#104110,#104111)),.UNSPECIFIED.,.F.,.F.,.F.)
B_SPLINE_SURFACE_WITH_KNOTS((2,2),(3,2,3),(0.,0.289807040992654),(0.418312080773434,
0.428571428571429,0.435879799328077),.UNSPECIFIED.)
GEOMETRIC_REPRESENTATION_ITEM()
RATIONAL_B_SPLINE_SURFACE(((0.99383221411677,0.996398874234721,1.,0.997434694412141,
0.995394338545807),(0.99383221411677,0.996398874234721,1.,0.997434694412141,
0.995394338545807)))
REPRESENTATION_ITEM('')
SURFACE()
);
#654=(
BOUNDED_SURFACE()
B_SPLINE_SURFACE(1,2,((#104119,#104120,#104121),(#104122,#104123,#104124)),
 .UNSPECIFIED.,.F.,.F.,.F.)
B_SPLINE_SURFACE_WITH_KNOTS((2,2),(3,3),(0.,0.289681084359925),(0.29775398702428,
0.314942866188516),.UNSPECIFIED.)
GEOMETRIC_REPRESENTATION_ITEM()
RATIONAL_B_SPLINE_SURFACE(((0.992972556818663,0.988973049555669,0.987877375613931),
(0.992972556818663,0.988973049555669,0.987877375613931)))
REPRESENTATION_ITEM('')
SURFACE()
);
#655=(
BOUNDED_SURFACE()
B_SPLINE_SURFACE(1,2,((#104133,#104134,#104135,#104136,#104137),(#104138,
#104139,#104140,#104141,#104142)),.UNSPECIFIED.,.F.,.F.,.F.)
B_SPLINE_SURFACE_WITH_KNOTS((2,2),(3,2,3),(0.,0.289807040992678),(0.418312080773434,
0.428571428571429,0.435879799327938),.UNSPECIFIED.)
GEOMETRIC_REPRESENTATION_ITEM()
RATIONAL_B_SPLINE_SURFACE(((0.99383221411677,0.99639887423472,1.,0.99743469441219,
0.995394338545885),(0.99383221411677,0.99639887423472,1.,0.99743469441219,
0.995394338545885)))
REPRESENTATION_ITEM('')
SURFACE()
);
#656=(
BOUNDED_SURFACE()
B_SPLINE_SURFACE(1,2,((#104150,#104151,#104152),(#104153,#104154,#104155)),
 .UNSPECIFIED.,.F.,.F.,.F.)
B_SPLINE_SURFACE_WITH_KNOTS((2,2),(3,3),(0.,0.289681084359921),(0.297753987024197,
0.314942866188516),.UNSPECIFIED.)
GEOMETRIC_REPRESENTATION_ITEM()
RATIONAL_B_SPLINE_SURFACE(((0.992972556818701,0.988973049555674,0.987877375613931),
(0.992972556818701,0.988973049555674,0.987877375613931)))
REPRESENTATION_ITEM('')
SURFACE()
);
#657=(
BOUNDED_SURFACE()
B_SPLINE_SURFACE(1,2,((#104164,#104165,#104166,#104167,#104168),(#104169,
#104170,#104171,#104172,#104173)),.UNSPECIFIED.,.F.,.F.,.F.)
B_SPLINE_SURFACE_WITH_KNOTS((2,2),(3,2,3),(0.,0.28980704099286),(0.418312080773434,
0.428571428571429,0.435879799328077),.UNSPECIFIED.)
GEOMETRIC_REPRESENTATION_ITEM()
RATIONAL_B_SPLINE_SURFACE(((0.99383221411677,0.996398874234721,1.,0.997434694412141,
0.995394338545807),(0.99383221411677,0.99639887423472,1.,0.997434694412141,
0.995394338545807)))
REPRESENTATION_ITEM('')
SURFACE()
);
#658=(
BOUNDED_SURFACE()
B_SPLINE_SURFACE(1,2,((#104181,#104182,#104183),(#104184,#104185,#104186)),
 .UNSPECIFIED.,.F.,.F.,.F.)
B_SPLINE_SURFACE_WITH_KNOTS((2,2),(3,3),(0.,0.289681084359929),(0.366717817351071,
0.383933227114987),.UNSPECIFIED.)
GEOMETRIC_REPRESENTATION_ITEM()
RATIONAL_B_SPLINE_SURFACE(((0.994179254576314,0.989756546152321,0.988246641953811),
(0.994179254576314,0.989756546152321,0.988246641953811)))
REPRESENTATION_ITEM('')
SURFACE()
);
#659=(
BOUNDED_SURFACE()
B_SPLINE_SURFACE(1,2,((#104197,#104198,#104199,#104200,#104201,#104202,
#104203),(#104204,#104205,#104206,#104207,#104208,#104209,#104210)),
 .UNSPECIFIED.,.F.,.F.,.F.)
B_SPLINE_SURFACE_WITH_KNOTS((2,2),(3,2,2,3),(-0.000384471073508479,0.289807040992007),
(0.348985225175754,0.349369696259361,0.357142857142857,0.367204964717613),
 .UNSPECIFIED.)
GEOMETRIC_REPRESENTATION_ITEM()
RATIONAL_B_SPLINE_SURFACE(((0.995136940902289,0.99513694090229,0.99513694090229,
0.997271548787858,1.,0.996468107373496,0.993931286686403),(0.99513694090229,
0.99513694090229,0.99513694090229,0.997271548787858,1.,0.996468107373496,
0.993931286686403)))
REPRESENTATION_ITEM('')
SURFACE()
);
#660=(
BOUNDED_SURFACE()
B_SPLINE_SURFACE(1,2,((#104233,#104234,#104235),(#104236,#104237,#104238)),
 .UNSPECIFIED.,.F.,.F.,.F.)
B_SPLINE_SURFACE_WITH_KNOTS((2,2),(3,3),(0.,0.289681084359933),(0.366717817351071,
0.383933227114989),.UNSPECIFIED.)
GEOMETRIC_REPRESENTATION_ITEM()
RATIONAL_B_SPLINE_SURFACE(((0.994179254576313,0.98975654615232,0.98824664195381),
(0.994179254576313,0.98975654615232,0.98824664195381)))
REPRESENTATION_ITEM('')
SURFACE()
);
#661=(
BOUNDED_SURFACE()
B_SPLINE_SURFACE(1,2,((#104240,#104241,#104242,#104243,#104244,#104245,
#104246),(#104247,#104248,#104249,#104250,#104251,#104252,#104253)),
 .UNSPECIFIED.,.F.,.F.,.F.)
B_SPLINE_SURFACE_WITH_KNOTS((2,2),(3,2,2,3),(-0.000384470876990202,0.289807040992908),
(0.348985225379442,0.349369696259359,0.357142857142857,0.3672049644935),
 .UNSPECIFIED.)
GEOMETRIC_REPRESENTATION_ITEM()
RATIONAL_B_SPLINE_SURFACE(((0.995136940902289,0.995136940902289,0.995136940902289,
0.997271548787858,1.,0.996468107452162,0.993931286799409),(0.995136940902289,
0.995136940902289,0.995136940902289,0.997271548787858,1.,0.996468107452162,
0.993931286799409)))
REPRESENTATION_ITEM('')
SURFACE()
);
#662=(
BOUNDED_SURFACE()
B_SPLINE_SURFACE(1,2,((#104276,#104277,#104278),(#104279,#104280,#104281)),
 .UNSPECIFIED.,.F.,.F.,.F.)
B_SPLINE_SURFACE_WITH_KNOTS((2,2),(3,3),(0.,0.289681084359918),(0.366717817351071,
0.383933227114993),.UNSPECIFIED.)
GEOMETRIC_REPRESENTATION_ITEM()
RATIONAL_B_SPLINE_SURFACE(((0.994179254576314,0.989756546152319,0.98824664195381),
(0.994179254576314,0.989756546152319,0.98824664195381)))
REPRESENTATION_ITEM('')
SURFACE()
);
#663=(
BOUNDED_SURFACE()
B_SPLINE_SURFACE(1,2,((#104283,#104284,#104285,#104286,#104287,#104288,
#104289),(#104290,#104291,#104292,#104293,#104294,#104295,#104296)),
 .UNSPECIFIED.,.F.,.F.,.F.)
B_SPLINE_SURFACE_WITH_KNOTS((2,2),(3,2,2,3),(-0.000384470989622132,0.289807040992866),
(0.348985225264237,0.349369696259357,0.357142857142857,0.367204964620462),
 .UNSPECIFIED.)
GEOMETRIC_REPRESENTATION_ITEM()
RATIONAL_B_SPLINE_SURFACE(((0.995136940902288,0.995136940902288,0.995136940902288,
0.997271548787857,1.,0.996468107407598,0.993931286735391),(0.995136940902287,
0.995136940902288,0.995136940902288,0.997271548787857,1.,0.996468107407597,
0.993931286735391)))
REPRESENTATION_ITEM('')
SURFACE()
);
#664=(
BOUNDED_SURFACE()
B_SPLINE_SURFACE(1,2,((#104319,#104320,#104321),(#104322,#104323,#104324)),
 .UNSPECIFIED.,.F.,.F.,.F.)
B_SPLINE_SURFACE_WITH_KNOTS((2,2),(3,3),(0.,0.289681084359924),(0.366717817351071,
0.383933227114987),.UNSPECIFIED.)
GEOMETRIC_REPRESENTATION_ITEM()
RATIONAL_B_SPLINE_SURFACE(((0.994179254576313,0.989756546152321,0.988246641953811),
(0.994179254576313,0.989756546152321,0.988246641953811)))
REPRESENTATION_ITEM('')
SURFACE()
);
#665=(
BOUNDED_SURFACE()
B_SPLINE_SURFACE(1,2,((#104326,#104327,#104328,#104329,#104330,#104331,
#104332),(#104333,#104334,#104335,#104336,#104337,#104338,#104339)),
 .UNSPECIFIED.,.F.,.F.,.F.)
B_SPLINE_SURFACE_WITH_KNOTS((2,2),(3,2,2,3),(-0.000384470951243084,0.289807040992824),
(0.348985225310178,0.349369696259357,0.357142857142857,0.367204964579277),
 .UNSPECIFIED.)
GEOMETRIC_REPRESENTATION_ITEM()
RATIONAL_B_SPLINE_SURFACE(((0.995136940902288,0.995136940902288,0.995136940902288,
0.997271548787857,1.,0.996468107422053,0.993931286756156),(0.995136940902288,
0.995136940902288,0.995136940902288,0.997271548787857,1.,0.996468107422054,
0.993931286756156)))
REPRESENTATION_ITEM('')
SURFACE()
);
#666=(
BOUNDED_SURFACE()
B_SPLINE_SURFACE(1,2,((#104362,#104363,#104364),(#104365,#104366,#104367)),
 .UNSPECIFIED.,.F.,.F.,.F.)
B_SPLINE_SURFACE_WITH_KNOTS((2,2),(3,3),(0.,0.289681084359916),(0.366717817351071,
0.383933227114987),.UNSPECIFIED.)
GEOMETRIC_REPRESENTATION_ITEM()
RATIONAL_B_SPLINE_SURFACE(((0.994179254576314,0.989756546152321,0.988246641953811),
(0.994179254576314,0.989756546152321,0.988246641953811)))
REPRESENTATION_ITEM('')
SURFACE()
);
#667=(
BOUNDED_SURFACE()
B_SPLINE_SURFACE(1,2,((#104369,#104370,#104371,#104372,#104373,#104374,
#104375),(#104376,#104377,#104378,#104379,#104380,#104381,#104382)),
 .UNSPECIFIED.,.F.,.F.,.F.)
B_SPLINE_SURFACE_WITH_KNOTS((2,2),(3,2,2,3),(-0.000384470777086583,0.289807040992855),
(0.348985225477453,0.349369696259359,0.357142857142857,0.367204964427647),
 .UNSPECIFIED.)
GEOMETRIC_REPRESENTATION_ITEM()
RATIONAL_B_SPLINE_SURFACE(((0.995136940902289,0.995136940902289,0.995136940902289,
0.997271548787858,1.,0.996468107475277,0.993931286832614),(0.995136940902289,
0.995136940902289,0.995136940902289,0.997271548787858,1.,0.996468107475277,
0.993931286832614)))
REPRESENTATION_ITEM('')
SURFACE()
);
#668=(
BOUNDED_SURFACE()
B_SPLINE_SURFACE(1,2,((#104405,#104406,#104407),(#104408,#104409,#104410)),
 .UNSPECIFIED.,.F.,.F.,.F.)
B_SPLINE_SURFACE_WITH_KNOTS((2,2),(3,3),(0.,0.289681084359922),(0.366717817351071,
0.383933227114987),.UNSPECIFIED.)
GEOMETRIC_REPRESENTATION_ITEM()
RATIONAL_B_SPLINE_SURFACE(((0.994179254576313,0.989756546152321,0.988246641953811),
(0.994179254576313,0.989756546152321,0.988246641953811)))
REPRESENTATION_ITEM('')
SURFACE()
);
#669=(
BOUNDED_SURFACE()
B_SPLINE_SURFACE(1,2,((#104412,#104413,#104414,#104415,#104416,#104417,
#104418),(#104419,#104420,#104421,#104422,#104423,#104424,#104425)),
 .UNSPECIFIED.,.F.,.F.,.F.)
B_SPLINE_SURFACE_WITH_KNOTS((2,2),(3,2,2,3),(-0.00038447093632129,0.289807040992328),
(0.348985225303722,0.349369696259343,0.357142857142857,0.367204964575977),
 .UNSPECIFIED.)
GEOMETRIC_REPRESENTATION_ITEM()
RATIONAL_B_SPLINE_SURFACE(((0.99513694090228,0.99513694090228,0.99513694090228,
0.997271548787852,1.,0.996468107423212,0.993931286757821),(0.99513694090228,
0.99513694090228,0.99513694090228,0.997271548787852,1.,0.996468107423212,
0.993931286757821)))
REPRESENTATION_ITEM('')
SURFACE()
);
#670=(
BOUNDED_SURFACE()
B_SPLINE_SURFACE(1,2,((#104448,#104449,#104450),(#104451,#104452,#104453)),
 .UNSPECIFIED.,.F.,.F.,.F.)
B_SPLINE_SURFACE_WITH_KNOTS((2,2),(3,3),(0.,0.28968108435993),(0.366717817351071,
0.383933227114987),.UNSPECIFIED.)
GEOMETRIC_REPRESENTATION_ITEM()
RATIONAL_B_SPLINE_SURFACE(((0.994179254576314,0.989756546152321,0.988246641953811),
(0.994179254576314,0.989756546152321,0.988246641953811)))
REPRESENTATION_ITEM('')
SURFACE()
);
#671=(
BOUNDED_SURFACE()
B_SPLINE_SURFACE(1,2,((#104455,#104456,#104457,#104458,#104459,#104460,
#104461),(#104462,#104463,#104464,#104465,#104466,#104467,#104468)),
 .UNSPECIFIED.,.F.,.F.,.F.)
B_SPLINE_SURFACE_WITH_KNOTS((2,2),(3,2,2,3),(-0.000384470852077006,0.289807040992451),
(0.348985225406444,0.349369696259343,0.357142857142857,0.367204964477797),
 .UNSPECIFIED.)
GEOMETRIC_REPRESENTATION_ITEM()
RATIONAL_B_SPLINE_SURFACE(((0.99513694090228,0.99513694090228,0.99513694090228,
0.997271548787852,1.,0.996468107457674,0.993931286807326),(0.99513694090228,
0.99513694090228,0.99513694090228,0.997271548787852,1.,0.996468107457674,
0.993931286807326)))
REPRESENTATION_ITEM('')
SURFACE()
);
#672=(
BOUNDED_SURFACE()
B_SPLINE_SURFACE(1,2,((#104476,#104477,#104478),(#104479,#104480,#104481)),
 .UNSPECIFIED.,.F.,.F.,.F.)
B_SPLINE_SURFACE_WITH_KNOTS((2,2),(3,3),(0.,0.289681084359928),(0.366717817351071,
0.383933227114987),.UNSPECIFIED.)
GEOMETRIC_REPRESENTATION_ITEM()
RATIONAL_B_SPLINE_SURFACE(((0.994179254576314,0.989756546152321,0.988246641953811),
(0.994179254576314,0.989756546152321,0.988246641953811)))
REPRESENTATION_ITEM('')
SURFACE()
);
#673=(
BOUNDED_SURFACE()
B_SPLINE_SURFACE(1,2,((#104483,#104484,#104485,#104486,#104487,#104488,
#104489),(#104490,#104491,#104492,#104493,#104494,#104495,#104496)),
 .UNSPECIFIED.,.F.,.F.,.F.)
B_SPLINE_SURFACE_WITH_KNOTS((2,2),(3,2,2,3),(-0.000384470769131978,0.289807040992686),
(0.348985225423804,0.349369696259343,0.357142857142857,0.367204964462875),
 .UNSPECIFIED.)
GEOMETRIC_REPRESENTATION_ITEM()
RATIONAL_B_SPLINE_SURFACE(((0.99513694090228,0.99513694090228,0.99513694090228,
0.997271548787852,1.,0.996468107462912,0.993931286814852),(0.99513694090228,
0.99513694090228,0.99513694090228,0.997271548787852,1.,0.996468107462912,
0.993931286814851)))
REPRESENTATION_ITEM('')
SURFACE()
);
#674=(
BOUNDED_SURFACE()
B_SPLINE_SURFACE(1,2,((#104519,#104520,#104521),(#104522,#104523,#104524)),
 .UNSPECIFIED.,.F.,.F.,.F.)
B_SPLINE_SURFACE_WITH_KNOTS((2,2),(3,3),(0.,0.289681084359927),(0.366717817351071,
0.383933227114987),.UNSPECIFIED.)
GEOMETRIC_REPRESENTATION_ITEM()
RATIONAL_B_SPLINE_SURFACE(((0.994179254576313,0.989756546152321,0.988246641953811),
(0.994179254576313,0.989756546152321,0.988246641953811)))
REPRESENTATION_ITEM('')
SURFACE()
);
#675=(
BOUNDED_SURFACE()
B_SPLINE_SURFACE(1,2,((#104526,#104527,#104528,#104529,#104530,#104531,
#104532),(#104533,#104534,#104535,#104536,#104537,#104538,#104539)),
 .UNSPECIFIED.,.F.,.F.,.F.)
B_SPLINE_SURFACE_WITH_KNOTS((2,2),(3,2,2,3),(-0.000384470922438091,0.289807040992906),
(0.348985225331245,0.349369696259343,0.357142857142857,0.367204964547758),
 .UNSPECIFIED.)
GEOMETRIC_REPRESENTATION_ITEM()
RATIONAL_B_SPLINE_SURFACE(((0.995136940902279,0.99513694090228,0.99513694090228,
0.997271548787852,1.,0.996468107433117,0.993931286772051),(0.99513694090228,
0.99513694090228,0.99513694090228,0.997271548787852,1.,0.996468107433117,
0.993931286772051)))
REPRESENTATION_ITEM('')
SURFACE()
);
#676=(
BOUNDED_SURFACE()
B_SPLINE_SURFACE(1,2,((#104562,#104563,#104564),(#104565,#104566,#104567)),
 .UNSPECIFIED.,.F.,.F.,.F.)
B_SPLINE_SURFACE_WITH_KNOTS((2,2),(3,3),(0.,0.28968108435992),(0.366717817350772,
0.383933227114987),.UNSPECIFIED.)
GEOMETRIC_REPRESENTATION_ITEM()
RATIONAL_B_SPLINE_SURFACE(((0.994179254576467,0.989756546152347,0.988246641953811),
(0.994179254576467,0.989756546152347,0.988246641953811)))
REPRESENTATION_ITEM('')
SURFACE()
);
#677=(
BOUNDED_SURFACE()
B_SPLINE_SURFACE(1,2,((#104569,#104570,#104571,#104572,#104573,#104574,
#104575),(#104576,#104577,#104578,#104579,#104580,#104581,#104582)),
 .UNSPECIFIED.,.F.,.F.,.F.)
B_SPLINE_SURFACE_WITH_KNOTS((2,2),(3,2,2,3),(-0.000384470727756695,0.289807040991758),
(0.348985225510703,0.349369696259361,0.357142857142857,0.367204964365651),
 .UNSPECIFIED.)
GEOMETRIC_REPRESENTATION_ITEM()
RATIONAL_B_SPLINE_SURFACE(((0.99513694090229,0.99513694090229,0.99513694090229,
0.997271548787858,1.,0.996468107497038,0.993931286863875),(0.99513694090229,
0.99513694090229,0.99513694090229,0.997271548787858,1.,0.996468107497038,
0.993931286863875)))
REPRESENTATION_ITEM('')
SURFACE()
);
#678=(
BOUNDED_SURFACE()
B_SPLINE_SURFACE(1,2,((#104605,#104606,#104607),(#104608,#104609,#104610)),
 .UNSPECIFIED.,.F.,.F.,.F.)
B_SPLINE_SURFACE_WITH_KNOTS((2,2),(3,3),(0.,0.28968108435992),(0.366717817350851,
0.383933227114987),.UNSPECIFIED.)
GEOMETRIC_REPRESENTATION_ITEM()
RATIONAL_B_SPLINE_SURFACE(((0.994179254576426,0.98975654615234,0.988246641953811),
(0.994179254576426,0.98975654615234,0.988246641953811)))
REPRESENTATION_ITEM('')
SURFACE()
);
#679=(
BOUNDED_SURFACE()
B_SPLINE_SURFACE(1,2,((#104612,#104613,#104614,#104615,#104616,#104617,
#104618),(#104619,#104620,#104621,#104622,#104623,#104624,#104625)),
 .UNSPECIFIED.,.F.,.F.,.F.)
B_SPLINE_SURFACE_WITH_KNOTS((2,2),(3,2,2,3),(-0.000384470761284522,0.289807040991714),
(0.348985225499164,0.349369696259361,0.357142857142857,0.36720496441584),
 .UNSPECIFIED.)
GEOMETRIC_REPRESENTATION_ITEM()
RATIONAL_B_SPLINE_SURFACE(((0.99513694090229,0.99513694090229,0.99513694090229,
0.997271548787858,1.,0.996468107479421,0.993931286838568),(0.99513694090229,
0.99513694090229,0.99513694090229,0.997271548787858,1.,0.996468107479422,
0.993931286838568)))
REPRESENTATION_ITEM('')
SURFACE()
);
#680=(
BOUNDED_SURFACE()
B_SPLINE_SURFACE(1,2,((#104648,#104649,#104650),(#104651,#104652,#104653)),
 .UNSPECIFIED.,.F.,.F.,.F.)
B_SPLINE_SURFACE_WITH_KNOTS((2,2),(3,3),(0.,0.289681084359927),(0.366717817351071,
0.383933227114987),.UNSPECIFIED.)
GEOMETRIC_REPRESENTATION_ITEM()
RATIONAL_B_SPLINE_SURFACE(((0.994179254576314,0.989756546152321,0.988246641953811),
(0.994179254576314,0.989756546152321,0.988246641953811)))
REPRESENTATION_ITEM('')
SURFACE()
);
#681=(
BOUNDED_SURFACE()
B_SPLINE_SURFACE(1,2,((#104655,#104656,#104657,#104658,#104659,#104660,
#104661),(#104662,#104663,#104664,#104665,#104666,#104667,#104668)),
 .UNSPECIFIED.,.F.,.F.,.F.)
B_SPLINE_SURFACE_WITH_KNOTS((2,2),(3,2,2,3),(-0.000384471191006712,0.289807040991564),
(0.348985225048002,0.349369696259361,0.357142857142857,0.367204964836913),
 .UNSPECIFIED.)
GEOMETRIC_REPRESENTATION_ITEM()
RATIONAL_B_SPLINE_SURFACE(((0.99513694090229,0.99513694090229,0.99513694090229,
0.997271548787858,1.,0.996468107331621,0.99393128662625),(0.99513694090229,
0.99513694090229,0.99513694090229,0.997271548787858,1.,0.996468107331621,
0.99393128662625)))
REPRESENTATION_ITEM('')
SURFACE()
);
#682=(
BOUNDED_SURFACE()
B_SPLINE_SURFACE(1,2,((#104691,#104692,#104693),(#104694,#104695,#104696)),
 .UNSPECIFIED.,.F.,.F.,.F.)
B_SPLINE_SURFACE_WITH_KNOTS((2,2),(3,3),(0.,0.289681084359927),(0.366717817351071,
0.383933227114987),.UNSPECIFIED.)
GEOMETRIC_REPRESENTATION_ITEM()
RATIONAL_B_SPLINE_SURFACE(((0.994179254576313,0.989756546152321,0.988246641953811),
(0.994179254576314,0.989756546152321,0.988246641953811)))
REPRESENTATION_ITEM('')
SURFACE()
);
#683=(
BOUNDED_SURFACE()
B_SPLINE_SURFACE(1,2,((#104698,#104699,#104700,#104701,#104702,#104703,
#104704),(#104705,#104706,#104707,#104708,#104709,#104710,#104711)),
 .UNSPECIFIED.,.F.,.F.,.F.)
B_SPLINE_SURFACE_WITH_KNOTS((2,2),(3,2,2,3),(-0.000384470750397015,0.289807040991566),
(0.348985225457864,0.349369696259361,0.357142857142857,0.367204964420445),
 .UNSPECIFIED.)
GEOMETRIC_REPRESENTATION_ITEM()
RATIONAL_B_SPLINE_SURFACE(((0.995136940902291,0.99513694090229,0.99513694090229,
0.997271548787858,1.,0.996468107477805,0.993931286836245),(0.995136940902291,
0.99513694090229,0.99513694090229,0.997271548787858,1.,0.996468107477805,
0.993931286836245)))
REPRESENTATION_ITEM('')
SURFACE()
);
#684=(
BOUNDED_SURFACE()
B_SPLINE_SURFACE(1,2,((#104734,#104735,#104736),(#104737,#104738,#104739)),
 .UNSPECIFIED.,.F.,.F.,.F.)
B_SPLINE_SURFACE_WITH_KNOTS((2,2),(3,3),(0.,0.289681084359929),(0.366717817350786,
0.383933227114987),.UNSPECIFIED.)
GEOMETRIC_REPRESENTATION_ITEM()
RATIONAL_B_SPLINE_SURFACE(((0.99417925457646,0.989756546152346,0.988246641953811),
(0.99417925457646,0.989756546152346,0.988246641953811)))
REPRESENTATION_ITEM('')
SURFACE()
);
#685=(
BOUNDED_SURFACE()
B_SPLINE_SURFACE(1,2,((#104741,#104742,#104743,#104744,#104745,#104746,
#104747),(#104748,#104749,#104750,#104751,#104752,#104753,#104754)),
 .UNSPECIFIED.,.F.,.F.,.F.)
B_SPLINE_SURFACE_WITH_KNOTS((2,2),(3,2,2,3),(-0.000384470913180565,0.289807040991567),
(0.3489852253338,0.349369696259361,0.357142857142857,0.367204964552289),
 .UNSPECIFIED.)
GEOMETRIC_REPRESENTATION_ITEM()
RATIONAL_B_SPLINE_SURFACE(((0.99513694090229,0.99513694090229,0.99513694090229,
0.997271548787858,1.,0.996468107431527,0.993931286769765),(0.99513694090229,
0.99513694090229,0.99513694090229,0.997271548787858,1.,0.996468107431527,
0.993931286769765)))
REPRESENTATION_ITEM('')
SURFACE()
);
#686=(
BOUNDED_SURFACE()
B_SPLINE_SURFACE(1,2,((#104777,#104778,#104779),(#104780,#104781,#104782)),
 .UNSPECIFIED.,.F.,.F.,.F.)
B_SPLINE_SURFACE_WITH_KNOTS((2,2),(3,3),(0.,0.289681084359931),(0.366717817351071,
0.383933227114987),.UNSPECIFIED.)
GEOMETRIC_REPRESENTATION_ITEM()
RATIONAL_B_SPLINE_SURFACE(((0.994179254576313,0.989756546152321,0.988246641953811),
(0.994179254576313,0.989756546152321,0.988246641953811)))
REPRESENTATION_ITEM('')
SURFACE()
);
#687=(
BOUNDED_SURFACE()
B_SPLINE_SURFACE(1,2,((#104784,#104785,#104786,#104787,#104788,#104789,
#104790),(#104791,#104792,#104793,#104794,#104795,#104796,#104797)),
 .UNSPECIFIED.,.F.,.F.,.F.)
B_SPLINE_SURFACE_WITH_KNOTS((2,2),(3,2,2,3),(-0.000384470870558051,0.289807040991559),
(0.348985225349386,0.349369696259361,0.357142857142857,0.367204964535364),
 .UNSPECIFIED.)
GEOMETRIC_REPRESENTATION_ITEM()
RATIONAL_B_SPLINE_SURFACE(((0.99513694090229,0.99513694090229,0.99513694090229,
0.997271548787858,1.,0.996468107437468,0.993931286778301),(0.99513694090229,
0.99513694090229,0.99513694090229,0.997271548787858,1.,0.996468107437468,
0.9939312867783)))
REPRESENTATION_ITEM('')
SURFACE()
);
#688=(
BOUNDED_SURFACE()
B_SPLINE_SURFACE(1,2,((#104820,#104821,#104822),(#104823,#104824,#104825)),
 .UNSPECIFIED.,.F.,.F.,.F.)
B_SPLINE_SURFACE_WITH_KNOTS((2,2),(3,3),(0.,0.28968108435992),(0.366717817351071,
0.383933227114987),.UNSPECIFIED.)
GEOMETRIC_REPRESENTATION_ITEM()
RATIONAL_B_SPLINE_SURFACE(((0.994179254576314,0.989756546152321,0.988246641953811),
(0.994179254576314,0.989756546152321,0.988246641953811)))
REPRESENTATION_ITEM('')
SURFACE()
);
#689=(
BOUNDED_SURFACE()
B_SPLINE_SURFACE(1,2,((#104827,#104828,#104829,#104830,#104831,#104832,
#104833),(#104834,#104835,#104836,#104837,#104838,#104839,#104840)),
 .UNSPECIFIED.,.F.,.F.,.F.)
B_SPLINE_SURFACE_WITH_KNOTS((2,2),(3,2,2,3),(-0.000384470880878568,0.289807040991565),
(0.348985225371886,0.349369696259361,0.357142857142857,0.367204964508579),
 .UNSPECIFIED.)
GEOMETRIC_REPRESENTATION_ITEM()
RATIONAL_B_SPLINE_SURFACE(((0.995136940902291,0.99513694090229,0.99513694090229,
0.997271548787858,1.,0.996468107446869,0.993931286791805),(0.995136940902291,
0.99513694090229,0.99513694090229,0.997271548787858,1.,0.996468107446869,
0.993931286791805)))
REPRESENTATION_ITEM('')
SURFACE()
);
#690=(
BOUNDED_SURFACE()
B_SPLINE_SURFACE(1,2,((#104863,#104864,#104865),(#104866,#104867,#104868)),
 .UNSPECIFIED.,.F.,.F.,.F.)
B_SPLINE_SURFACE_WITH_KNOTS((2,2),(3,3),(0.,0.289681084359924),(0.366717817351071,
0.383933227114987),.UNSPECIFIED.)
GEOMETRIC_REPRESENTATION_ITEM()
RATIONAL_B_SPLINE_SURFACE(((0.994179254576313,0.989756546152321,0.988246641953811),
(0.994179254576313,0.989756546152321,0.988246641953811)))
REPRESENTATION_ITEM('')
SURFACE()
);
#691=(
BOUNDED_SURFACE()
B_SPLINE_SURFACE(1,2,((#104870,#104871,#104872,#104873,#104874,#104875,
#104876),(#104877,#104878,#104879,#104880,#104881,#104882,#104883)),
 .UNSPECIFIED.,.F.,.F.,.F.)
B_SPLINE_SURFACE_WITH_KNOTS((2,2),(3,2,2,3),(-0.000384470963773044,0.289807040991667),
(0.348985225287661,0.349369696259361,0.357142857142857,0.367204964598757),
 .UNSPECIFIED.)
GEOMETRIC_REPRESENTATION_ITEM()
RATIONAL_B_SPLINE_SURFACE(((0.99513694090229,0.99513694090229,0.99513694090229,
0.997271548787858,1.,0.996468107415216,0.993931286746336),(0.99513694090229,
0.99513694090229,0.99513694090229,0.997271548787858,1.,0.996468107415216,
0.993931286746336)))
REPRESENTATION_ITEM('')
SURFACE()
);
#692=(
BOUNDED_SURFACE()
B_SPLINE_SURFACE(1,2,((#104906,#104907,#104908),(#104909,#104910,#104911)),
 .UNSPECIFIED.,.F.,.F.,.F.)
B_SPLINE_SURFACE_WITH_KNOTS((2,2),(3,3),(0.,0.289681084359924),(0.366717817351071,
0.383933227114987),.UNSPECIFIED.)
GEOMETRIC_REPRESENTATION_ITEM()
RATIONAL_B_SPLINE_SURFACE(((0.994179254576313,0.989756546152321,0.988246641953811),
(0.994179254576313,0.989756546152321,0.988246641953811)))
REPRESENTATION_ITEM('')
SURFACE()
);
#693=(
BOUNDED_SURFACE()
B_SPLINE_SURFACE(1,2,((#104913,#104914,#104915,#104916,#104917,#104918,
#104919),(#104920,#104921,#104922,#104923,#104924,#104925,#104926)),
 .UNSPECIFIED.,.F.,.F.,.F.)
B_SPLINE_SURFACE_WITH_KNOTS((2,2),(3,2,2,3),(-0.000384470506086084,0.289807040992968),
(0.348985225660948,0.349369696259361,0.357142857142857,0.367204964215901),
 .UNSPECIFIED.)
GEOMETRIC_REPRESENTATION_ITEM()
RATIONAL_B_SPLINE_SURFACE(((0.995136940902291,0.99513694090229,0.99513694090229,
0.997271548787858,1.,0.996468107549602,0.993931286939384),(0.995136940902291,
0.99513694090229,0.99513694090229,0.997271548787858,1.,0.996468107549602,
0.993931286939384)))
REPRESENTATION_ITEM('')
SURFACE()
);
#694=(
BOUNDED_SURFACE()
B_SPLINE_SURFACE(1,2,((#104949,#104950,#104951),(#104952,#104953,#104954)),
 .UNSPECIFIED.,.F.,.F.,.F.)
B_SPLINE_SURFACE_WITH_KNOTS((2,2),(3,3),(0.,0.289681084359921),(0.366717817350842,
0.383933227114987),.UNSPECIFIED.)
GEOMETRIC_REPRESENTATION_ITEM()
RATIONAL_B_SPLINE_SURFACE(((0.994179254576431,0.989756546152341,0.988246641953811),
(0.994179254576431,0.989756546152341,0.988246641953811)))
REPRESENTATION_ITEM('')
SURFACE()
);
#695=(
BOUNDED_SURFACE()
B_SPLINE_SURFACE(1,2,((#104956,#104957,#104958,#104959,#104960,#104961,
#104962),(#104963,#104964,#104965,#104966,#104967,#104968,#104969)),
 .UNSPECIFIED.,.F.,.F.,.F.)
B_SPLINE_SURFACE_WITH_KNOTS((2,2),(3,2,2,3),(-0.000384470883047098,0.289807040991813),
(0.34898522534491,0.349369696259361,0.357142857142857,0.367204964524695),
 .UNSPECIFIED.)
GEOMETRIC_REPRESENTATION_ITEM()
RATIONAL_B_SPLINE_SURFACE(((0.99513694090229,0.99513694090229,0.99513694090229,
0.997271548787858,1.,0.996468107441213,0.99393128678368),(0.99513694090229,
0.99513694090229,0.99513694090229,0.997271548787858,1.,0.996468107441213,
0.99393128678368)))
REPRESENTATION_ITEM('')
SURFACE()
);
#696=(
BOUNDED_SURFACE()
B_SPLINE_SURFACE(1,2,((#104992,#104993,#104994),(#104995,#104996,#104997)),
 .UNSPECIFIED.,.F.,.F.,.F.)
B_SPLINE_SURFACE_WITH_KNOTS((2,2),(3,3),(0.,0.289681084359923),(0.366717817351071,
0.383933227114987),.UNSPECIFIED.)
GEOMETRIC_REPRESENTATION_ITEM()
RATIONAL_B_SPLINE_SURFACE(((0.994179254576314,0.989756546152321,0.988246641953811),
(0.994179254576314,0.989756546152321,0.988246641953811)))
REPRESENTATION_ITEM('')
SURFACE()
);
#697=(
BOUNDED_SURFACE()
B_SPLINE_SURFACE(1,2,((#104999,#105000,#105001,#105002,#105003,#105004,
#105005),(#105006,#105007,#105008,#105009,#105010,#105011,#105012)),
 .UNSPECIFIED.,.F.,.F.,.F.)
B_SPLINE_SURFACE_WITH_KNOTS((2,2),(3,2,2,3),(-0.000384470884855509,0.289807040991563),
(0.348985225362649,0.349369696259361,0.357142857142857,0.367204964528156),
 .UNSPECIFIED.)
GEOMETRIC_REPRESENTATION_ITEM()
RATIONAL_B_SPLINE_SURFACE(((0.995136940902291,0.995136940902291,0.99513694090229,
0.997271548787858,1.,0.996468107439998,0.993931286781934),(0.995136940902291,
0.99513694090229,0.99513694090229,0.997271548787858,1.,0.996468107439998,
0.993931286781934)))
REPRESENTATION_ITEM('')
SURFACE()
);
#698=(
BOUNDED_SURFACE()
B_SPLINE_SURFACE(1,2,((#105035,#105036,#105037),(#105038,#105039,#105040)),
 .UNSPECIFIED.,.F.,.F.,.F.)
B_SPLINE_SURFACE_WITH_KNOTS((2,2),(3,3),(0.,0.289681084359921),(0.366717817351071,
0.383933227114987),.UNSPECIFIED.)
GEOMETRIC_REPRESENTATION_ITEM()
RATIONAL_B_SPLINE_SURFACE(((0.994179254576313,0.989756546152321,0.988246641953811),
(0.994179254576313,0.989756546152321,0.988246641953811)))
REPRESENTATION_ITEM('')
SURFACE()
);
#699=(
BOUNDED_SURFACE()
B_SPLINE_SURFACE(1,2,((#105042,#105043,#105044,#105045,#105046,#105047,
#105048),(#105049,#105050,#105051,#105052,#105053,#105054,#105055)),
 .UNSPECIFIED.,.F.,.F.,.F.)
B_SPLINE_SURFACE_WITH_KNOTS((2,2),(3,2,2,3),(-0.000384470797821128,0.289807040991558),
(0.348985225443547,0.349369696259361,0.357142857142857,0.367204964439945),
 .UNSPECIFIED.)
GEOMETRIC_REPRESENTATION_ITEM()
RATIONAL_B_SPLINE_SURFACE(((0.995136940902289,0.99513694090229,0.99513694090229,
0.997271548787858,1.,0.996468107470961,0.993931286826414),(0.99513694090229,
0.99513694090229,0.99513694090229,0.997271548787858,1.,0.996468107470961,
0.993931286826414)))
REPRESENTATION_ITEM('')
SURFACE()
);
#700=(
BOUNDED_SURFACE()
B_SPLINE_SURFACE(1,2,((#105078,#105079,#105080),(#105081,#105082,#105083)),
 .UNSPECIFIED.,.F.,.F.,.F.)
B_SPLINE_SURFACE_WITH_KNOTS((2,2),(3,3),(0.,0.289681084359919),(0.366717817351071,
0.383933227114987),.UNSPECIFIED.)
GEOMETRIC_REPRESENTATION_ITEM()
RATIONAL_B_SPLINE_SURFACE(((0.994179254576314,0.989756546152321,0.988246641953811),
(0.994179254576314,0.989756546152321,0.988246641953811)))
REPRESENTATION_ITEM('')
SURFACE()
);
#701=(
BOUNDED_SURFACE()
B_SPLINE_SURFACE(1,2,((#105085,#105086,#105087,#105088,#105089,#105090,
#105091),(#105092,#105093,#105094,#105095,#105096,#105097,#105098)),
 .UNSPECIFIED.,.F.,.F.,.F.)
B_SPLINE_SURFACE_WITH_KNOTS((2,2),(3,2,2,3),(-0.000384470745199549,0.28980704099156),
(0.348985225479933,0.349369696259361,0.357142857142857,0.367204964406885),
 .UNSPECIFIED.)
GEOMETRIC_REPRESENTATION_ITEM()
RATIONAL_B_SPLINE_SURFACE(((0.995136940902291,0.99513694090229,0.99513694090229,
0.997271548787858,1.,0.996468107482565,0.993931286843084),(0.995136940902291,
0.99513694090229,0.99513694090229,0.997271548787858,1.,0.996468107482565,
0.993931286843084)))
REPRESENTATION_ITEM('')
SURFACE()
);
#702=(
BOUNDED_SURFACE()
B_SPLINE_SURFACE(1,2,((#105121,#105122,#105123),(#105124,#105125,#105126)),
 .UNSPECIFIED.,.F.,.F.,.F.)
B_SPLINE_SURFACE_WITH_KNOTS((2,2),(3,3),(0.,0.289681084359919),(0.366717817351071,
0.383933227114987),.UNSPECIFIED.)
GEOMETRIC_REPRESENTATION_ITEM()
RATIONAL_B_SPLINE_SURFACE(((0.994179254576313,0.989756546152321,0.988246641953811),
(0.994179254576313,0.989756546152321,0.988246641953811)))
REPRESENTATION_ITEM('')
SURFACE()
);
#703=(
BOUNDED_SURFACE()
B_SPLINE_SURFACE(1,2,((#105128,#105129,#105130,#105131,#105132,#105133,
#105134),(#105135,#105136,#105137,#105138,#105139,#105140,#105141)),
 .UNSPECIFIED.,.F.,.F.,.F.)
B_SPLINE_SURFACE_WITH_KNOTS((2,2),(3,2,2,3),(-0.000384470876979244,0.289807040991562),
(0.348985225392862,0.349369696259361,0.357142857142857,0.36720496451606),
 .UNSPECIFIED.)
GEOMETRIC_REPRESENTATION_ITEM()
RATIONAL_B_SPLINE_SURFACE(((0.99513694090229,0.99513694090229,0.99513694090229,
0.997271548787858,1.,0.996468107444244,0.993931286788034),(0.99513694090229,
0.99513694090229,0.99513694090229,0.997271548787858,1.,0.996468107444244,
0.993931286788034)))
REPRESENTATION_ITEM('')
SURFACE()
);
#704=(
BOUNDED_SURFACE()
B_SPLINE_SURFACE(1,2,((#105164,#105165,#105166),(#105167,#105168,#105169)),
 .UNSPECIFIED.,.F.,.F.,.F.)
B_SPLINE_SURFACE_WITH_KNOTS((2,2),(3,3),(0.,0.289681084359922),(0.366717817351071,
0.383933227114987),.UNSPECIFIED.)
GEOMETRIC_REPRESENTATION_ITEM()
RATIONAL_B_SPLINE_SURFACE(((0.994179254576314,0.989756546152321,0.988246641953811),
(0.994179254576314,0.989756546152321,0.988246641953811)))
REPRESENTATION_ITEM('')
SURFACE()
);
#705=(
BOUNDED_SURFACE()
B_SPLINE_SURFACE(1,2,((#105171,#105172,#105173,#105174,#105175,#105176,
#105177),(#105178,#105179,#105180,#105181,#105182,#105183,#105184)),
 .UNSPECIFIED.,.F.,.F.,.F.)
B_SPLINE_SURFACE_WITH_KNOTS((2,2),(3,2,2,3),(-0.000384470896032662,0.289807040991558),
(0.348985225362887,0.349369696259361,0.357142857142857,0.367204964522724),
 .UNSPECIFIED.)
GEOMETRIC_REPRESENTATION_ITEM()
RATIONAL_B_SPLINE_SURFACE(((0.99513694090229,0.99513694090229,0.99513694090229,
0.997271548787858,1.,0.996468107441904,0.993931286784672),(0.99513694090229,
0.99513694090229,0.99513694090229,0.997271548787858,1.,0.996468107441904,
0.993931286784672)))
REPRESENTATION_ITEM('')
SURFACE()
);
#706=(
BOUNDED_SURFACE()
B_SPLINE_SURFACE(1,2,((#105201,#105202,#105203),(#105204,#105205,#105206)),
 .UNSPECIFIED.,.F.,.F.,.F.)
B_SPLINE_SURFACE_WITH_KNOTS((2,2),(3,3),(0.,0.289681084359918),(0.366717817351071,
0.383933227114987),.UNSPECIFIED.)
GEOMETRIC_REPRESENTATION_ITEM()
RATIONAL_B_SPLINE_SURFACE(((0.994179254576314,0.989756546152321,0.988246641953811),
(0.994179254576314,0.989756546152321,0.988246641953811)))
REPRESENTATION_ITEM('')
SURFACE()
);
#707=(
BOUNDED_SURFACE()
B_SPLINE_SURFACE(1,2,((#105214,#105215,#105216,#105217,#105218,#105219,
#105220),(#105221,#105222,#105223,#105224,#105225,#105226,#105227)),
 .UNSPECIFIED.,.F.,.F.,.F.)
B_SPLINE_SURFACE_WITH_KNOTS((2,2),(3,2,2,3),(-0.000384470919179307,0.28980704099156),
(0.348985225341793,0.349369696259357,0.357142857142857,0.367204964567339),
 .UNSPECIFIED.)
GEOMETRIC_REPRESENTATION_ITEM()
RATIONAL_B_SPLINE_SURFACE(((0.995136940902287,0.995136940902287,0.995136940902287,
0.997271548787857,1.,0.996468107426244,0.993931286762177),(0.995136940902288,
0.995136940902288,0.995136940902288,0.997271548787857,1.,0.996468107426244,
0.993931286762177)))
REPRESENTATION_ITEM('')
SURFACE()
);
#708=(
BOUNDED_SURFACE()
B_SPLINE_SURFACE(1,2,((#105250,#105251,#105252),(#105253,#105254,#105255)),
 .UNSPECIFIED.,.F.,.F.,.F.)
B_SPLINE_SURFACE_WITH_KNOTS((2,2),(3,3),(0.,0.289681084359925),(0.366717817350596,
0.383933227114986),.UNSPECIFIED.)
GEOMETRIC_REPRESENTATION_ITEM()
RATIONAL_B_SPLINE_SURFACE(((0.994179254576558,0.989756546152363,0.988246641953811),
(0.994179254576558,0.989756546152363,0.988246641953811)))
REPRESENTATION_ITEM('')
SURFACE()
);
#709=(
BOUNDED_SURFACE()
B_SPLINE_SURFACE(1,2,((#105257,#105258,#105259,#105260,#105261,#105262,
#105263),(#105264,#105265,#105266,#105267,#105268,#105269,#105270)),
 .UNSPECIFIED.,.F.,.F.,.F.)
B_SPLINE_SURFACE_WITH_KNOTS((2,2),(3,2,2,3),(-0.000384470951268838,0.289807040991836),
(0.348985225303333,0.349369696259362,0.357142857142857,0.367204964581818),
 .UNSPECIFIED.)
GEOMETRIC_REPRESENTATION_ITEM()
RATIONAL_B_SPLINE_SURFACE(((0.995136940902291,0.99513694090229,0.99513694090229,
0.997271548787859,1.,0.996468107421162,0.993931286754876),(0.995136940902291,
0.99513694090229,0.99513694090229,0.997271548787859,1.,0.996468107421162,
0.993931286754876)))
REPRESENTATION_ITEM('')
SURFACE()
);
#710=(
BOUNDED_SURFACE()
B_SPLINE_SURFACE(1,2,((#105293,#105294,#105295),(#105296,#105297,#105298)),
 .UNSPECIFIED.,.F.,.F.,.F.)
B_SPLINE_SURFACE_WITH_KNOTS((2,2),(3,3),(0.,0.289681084359919),(0.366717817351007,
0.383933227114987),.UNSPECIFIED.)
GEOMETRIC_REPRESENTATION_ITEM()
RATIONAL_B_SPLINE_SURFACE(((0.994179254576346,0.989756546152326,0.988246641953811),
(0.994179254576346,0.989756546152326,0.988246641953811)))
REPRESENTATION_ITEM('')
SURFACE()
);
#711=(
BOUNDED_SURFACE()
B_SPLINE_SURFACE(1,2,((#105300,#105301,#105302,#105303,#105304,#105305,
#105306),(#105307,#105308,#105309,#105310,#105311,#105312,#105313)),
 .UNSPECIFIED.,.F.,.F.,.F.)
B_SPLINE_SURFACE_WITH_KNOTS((2,2),(3,2,2,3),(-0.000384470793921457,0.289807040992022),
(0.348985225456814,0.349369696259361,0.357142857142857,0.367204964438393),
 .UNSPECIFIED.)
GEOMETRIC_REPRESENTATION_ITEM()
RATIONAL_B_SPLINE_SURFACE(((0.99513694090229,0.99513694090229,0.99513694090229,
0.997271548787858,1.,0.996468107471505,0.993931286827196),(0.99513694090229,
0.99513694090229,0.99513694090229,0.997271548787858,1.,0.996468107471505,
0.993931286827196)))
REPRESENTATION_ITEM('')
SURFACE()
);
#712=(
BOUNDED_SURFACE()
B_SPLINE_SURFACE(1,2,((#105336,#105337,#105338),(#105339,#105340,#105341)),
 .UNSPECIFIED.,.F.,.F.,.F.)
B_SPLINE_SURFACE_WITH_KNOTS((2,2),(3,3),(0.,0.289681084359933),(0.366717817351071,
0.383933227114987),.UNSPECIFIED.)
GEOMETRIC_REPRESENTATION_ITEM()
RATIONAL_B_SPLINE_SURFACE(((0.994179254576314,0.989756546152321,0.988246641953811),
(0.994179254576314,0.989756546152321,0.988246641953811)))
REPRESENTATION_ITEM('')
SURFACE()
);
#713=(
BOUNDED_SURFACE()
B_SPLINE_SURFACE(1,2,((#105343,#105344,#105345,#105346,#105347,#105348,
#105349),(#105350,#105351,#105352,#105353,#105354,#105355,#105356)),
 .UNSPECIFIED.,.F.,.F.,.F.)
B_SPLINE_SURFACE_WITH_KNOTS((2,2),(3,2,2,3),(-0.000384470853099693,0.289807040991983),
(0.34898522538828,0.349369696259361,0.357142857142857,0.367204964474479),
 .UNSPECIFIED.)
GEOMETRIC_REPRESENTATION_ITEM()
RATIONAL_B_SPLINE_SURFACE(((0.995136940902289,0.99513694090229,0.99513694090229,
0.997271548787858,1.,0.996468107458839,0.993931286808999),(0.995136940902289,
0.99513694090229,0.99513694090229,0.997271548787858,1.,0.996468107458839,
0.993931286808999)))
REPRESENTATION_ITEM('')
SURFACE()
);
#714=(
BOUNDED_SURFACE()
B_SPLINE_SURFACE(1,2,((#105379,#105380,#105381),(#105382,#105383,#105384)),
 .UNSPECIFIED.,.F.,.F.,.F.)
B_SPLINE_SURFACE_WITH_KNOTS((2,2),(3,3),(0.,0.289681084359926),(0.366717817351071,
0.383933227114987),.UNSPECIFIED.)
GEOMETRIC_REPRESENTATION_ITEM()
RATIONAL_B_SPLINE_SURFACE(((0.994179254576314,0.989756546152321,0.988246641953811),
(0.994179254576314,0.989756546152321,0.988246641953811)))
REPRESENTATION_ITEM('')
SURFACE()
);
#715=(
BOUNDED_SURFACE()
B_SPLINE_SURFACE(1,2,((#105398,#105399,#105400,#105401,#105402,#105403,
#105404),(#105405,#105406,#105407,#105408,#105409,#105410,#105411)),
 .UNSPECIFIED.,.F.,.F.,.F.)
B_SPLINE_SURFACE_WITH_KNOTS((2,2),(3,2,2,3),(-0.000384472577672092,0.289807040991895),
(0.348985223670602,0.349369696259361,0.357142857142857,0.367204966456659),
 .UNSPECIFIED.)
GEOMETRIC_REPRESENTATION_ITEM()
RATIONAL_B_SPLINE_SURFACE(((0.995136940902289,0.99513694090229,0.99513694090229,
0.997271548787858,1.,0.996468106763076,0.99393128580952),(0.99513694090229,
0.99513694090229,0.99513694090229,0.997271548787858,1.,0.996468106763076,
0.993931285809521)))
REPRESENTATION_ITEM('')
SURFACE()
);
#716=(
BOUNDED_SURFACE()
B_SPLINE_SURFACE(1,2,((#105413,#105414,#105415,#105416,#105417),(#105418,
#105419,#105420,#105421,#105422)),.UNSPECIFIED.,.F.,.F.,.F.)
B_SPLINE_SURFACE_WITH_KNOTS((2,2),(3,2,3),(0.710192959007142,1.),(0.297684616398914,
0.297856505190553,0.315045384354504),.UNSPECIFIED.)
GEOMETRIC_REPRESENTATION_ITEM()
RATIONAL_B_SPLINE_SURFACE(((0.99292495227316,0.99292495227316,0.99292495227316,
0.988942764095695,0.98786440923939),(0.99292495227316,0.99292495227316,
0.99292495227316,0.988942764095695,0.98786440923939)))
REPRESENTATION_ITEM('')
SURFACE()
);
#717=(
BOUNDED_SURFACE()
B_SPLINE_SURFACE(1,2,((#105433,#105434,#105435,#105436,#105437,#105438,
#105439),(#105440,#105441,#105442,#105443,#105444,#105445,#105446)),
 .UNSPECIFIED.,.F.,.F.,.F.)
B_SPLINE_SURFACE_WITH_KNOTS((2,2),(3,2,2,3),(0.710318915639639,1.),(0.418207303127979,
0.428571428571429,0.435775021682622,0.435950698868169),.UNSPECIFIED.)
GEOMETRIC_REPRESENTATION_ITEM()
RATIONAL_B_SPLINE_SURFACE(((0.993779895952495,0.996362096314125,1.,0.997471472332736,
0.995452950231063,0.995452950231063,0.995452950231063),(0.993779895952495,
0.996362096314125,1.,0.997471472332736,0.995452950231063,0.995452950231063,
0.995452950231063)))
REPRESENTATION_ITEM('')
SURFACE()
);
#718=(
BOUNDED_SURFACE()
B_SPLINE_SURFACE(1,2,((#105463,#105464,#105465,#105466,#105467),(#105468,
#105469,#105470,#105471,#105472)),.UNSPECIFIED.,.F.,.F.,.F.)
B_SPLINE_SURFACE_WITH_KNOTS((2,2),(3,2,3),(0.710192959007996,1.),(0.297684616398975,
0.297856505190614,0.315045384354503),.UNSPECIFIED.)
GEOMETRIC_REPRESENTATION_ITEM()
RATIONAL_B_SPLINE_SURFACE(((0.992924952273131,0.992924952273131,0.992924952273131,
0.988942764095691,0.98786440923939),(0.992924952273131,0.992924952273131,
0.992924952273131,0.988942764095691,0.98786440923939)))
REPRESENTATION_ITEM('')
SURFACE()
);
#719=(
BOUNDED_SURFACE()
B_SPLINE_SURFACE(1,2,((#105480,#105481,#105482,#105483,#105484,#105485,
#105486),(#105487,#105488,#105489,#105490,#105491,#105492,#105493)),
 .UNSPECIFIED.,.F.,.F.,.F.)
B_SPLINE_SURFACE_WITH_KNOTS((2,2),(3,2,2,3),(0.710318915640079,1.),(0.418207303127978,
0.428571428571429,0.435775021682621,0.435950698868168),.UNSPECIFIED.)
GEOMETRIC_REPRESENTATION_ITEM()
RATIONAL_B_SPLINE_SURFACE(((0.993779895952494,0.996362096314125,1.,0.997471472332737,
0.995452950231064,0.995452950231064,0.995452950231064),(0.993779895952495,
0.996362096314125,1.,0.997471472332737,0.995452950231064,0.995452950231064,
0.995452950231064)))
REPRESENTATION_ITEM('')
SURFACE()
);
#720=(
BOUNDED_SURFACE()
B_SPLINE_SURFACE(1,2,((#105510,#105511,#105512,#105513,#105514),(#105515,
#105516,#105517,#105518,#105519)),.UNSPECIFIED.,.F.,.F.,.F.)
B_SPLINE_SURFACE_WITH_KNOTS((2,2),(3,2,3),(0.710192959008438,1.),(0.297684616398975,
0.297856505190614,0.315045384354504),.UNSPECIFIED.)
GEOMETRIC_REPRESENTATION_ITEM()
RATIONAL_B_SPLINE_SURFACE(((0.992924952273132,0.992924952273132,0.992924952273132,
0.988942764095691,0.98786440923939),(0.992924952273132,0.992924952273132,
0.992924952273132,0.988942764095691,0.98786440923939)))
REPRESENTATION_ITEM('')
SURFACE()
);
#721=(
BOUNDED_SURFACE()
B_SPLINE_SURFACE(1,2,((#105527,#105528,#105529,#105530,#105531,#105532,
#105533),(#105534,#105535,#105536,#105537,#105538,#105539,#105540)),
 .UNSPECIFIED.,.F.,.F.,.F.)
B_SPLINE_SURFACE_WITH_KNOTS((2,2),(3,2,2,3),(0.710318915639646,1.),(0.418207303127977,
0.428571428571429,0.435775021682621,0.435950698868168),.UNSPECIFIED.)
GEOMETRIC_REPRESENTATION_ITEM()
RATIONAL_B_SPLINE_SURFACE(((0.993779895952494,0.996362096314125,1.,0.997471472332737,
0.995452950231064,0.995452950231064,0.995452950231064),(0.993779895952494,
0.996362096314125,1.,0.997471472332737,0.995452950231064,0.995452950231064,
0.995452950231064)))
REPRESENTATION_ITEM('')
SURFACE()
);
#722=(
BOUNDED_SURFACE()
B_SPLINE_SURFACE(1,2,((#105557,#105558,#105559,#105560,#105561),(#105562,
#105563,#105564,#105565,#105566)),.UNSPECIFIED.,.F.,.F.,.F.)
B_SPLINE_SURFACE_WITH_KNOTS((2,2),(3,2,3),(0.71019295900844,1.),(0.297684616398975,
0.297856505190614,0.315045384354504),.UNSPECIFIED.)
GEOMETRIC_REPRESENTATION_ITEM()
RATIONAL_B_SPLINE_SURFACE(((0.992924952273132,0.992924952273132,0.992924952273132,
0.988942764095691,0.98786440923939),(0.992924952273131,0.992924952273131,
0.992924952273131,0.988942764095691,0.98786440923939)))
REPRESENTATION_ITEM('')
SURFACE()
);
#723=(
BOUNDED_SURFACE()
B_SPLINE_SURFACE(1,2,((#105574,#105575,#105576,#105577,#105578,#105579,
#105580),(#105581,#105582,#105583,#105584,#105585,#105586,#105587)),
 .UNSPECIFIED.,.F.,.F.,.F.)
B_SPLINE_SURFACE_WITH_KNOTS((2,2),(3,2,2,3),(0.710318915640077,1.),(0.418207303127978,
0.428571428571429,0.435775021682621,0.435950698868168),.UNSPECIFIED.)
GEOMETRIC_REPRESENTATION_ITEM()
RATIONAL_B_SPLINE_SURFACE(((0.993779895952495,0.996362096314125,1.,0.997471472332737,
0.995452950231063,0.995452950231063,0.995452950231063),(0.993779895952495,
0.996362096314125,1.,0.997471472332737,0.995452950231063,0.995452950231063,
0.995452950231063)))
REPRESENTATION_ITEM('')
SURFACE()
);
#724=(
BOUNDED_SURFACE()
B_SPLINE_SURFACE(1,2,((#105604,#105605,#105606,#105607,#105608),(#105609,
#105610,#105611,#105612,#105613)),.UNSPECIFIED.,.F.,.F.,.F.)
B_SPLINE_SURFACE_WITH_KNOTS((2,2),(3,2,3),(0.710192959008444,1.),(0.297684616398975,
0.297856505190614,0.315045384354504),.UNSPECIFIED.)
GEOMETRIC_REPRESENTATION_ITEM()
RATIONAL_B_SPLINE_SURFACE(((0.992924952273132,0.992924952273132,0.992924952273132,
0.988942764095691,0.98786440923939),(0.992924952273131,0.992924952273131,
0.992924952273131,0.988942764095691,0.98786440923939)))
REPRESENTATION_ITEM('')
SURFACE()
);
#725=(
BOUNDED_SURFACE()
B_SPLINE_SURFACE(1,2,((#105621,#105622,#105623,#105624,#105625,#105626,
#105627),(#105628,#105629,#105630,#105631,#105632,#105633,#105634)),
 .UNSPECIFIED.,.F.,.F.,.F.)
B_SPLINE_SURFACE_WITH_KNOTS((2,2),(3,2,2,3),(0.710318915639999,1.),(0.418207303127979,
0.428571428571429,0.435775021682621,0.435950698868168),.UNSPECIFIED.)
GEOMETRIC_REPRESENTATION_ITEM()
RATIONAL_B_SPLINE_SURFACE(((0.993779895952495,0.996362096314125,1.,0.997471472332737,
0.995452950231064,0.995452950231064,0.995452950231064),(0.993779895952495,
0.996362096314125,1.,0.997471472332737,0.995452950231064,0.995452950231064,
0.995452950231064)))
REPRESENTATION_ITEM('')
SURFACE()
);
#726=(
BOUNDED_SURFACE()
B_SPLINE_SURFACE(1,2,((#105651,#105652,#105653,#105654,#105655),(#105656,
#105657,#105658,#105659,#105660)),.UNSPECIFIED.,.F.,.F.,.F.)
B_SPLINE_SURFACE_WITH_KNOTS((2,2),(3,2,3),(0.710192959008359,1.),(0.297684616398974,
0.297856505190613,0.315045384354503),.UNSPECIFIED.)
GEOMETRIC_REPRESENTATION_ITEM()
RATIONAL_B_SPLINE_SURFACE(((0.992924952273132,0.992924952273132,0.992924952273132,
0.988942764095691,0.98786440923939),(0.992924952273132,0.992924952273132,
0.992924952273132,0.988942764095691,0.98786440923939)))
REPRESENTATION_ITEM('')
SURFACE()
);
#727=(
BOUNDED_SURFACE()
B_SPLINE_SURFACE(1,2,((#105668,#105669,#105670,#105671,#105672,#105673,
#105674),(#105675,#105676,#105677,#105678,#105679,#105680,#105681)),
 .UNSPECIFIED.,.F.,.F.,.F.)
B_SPLINE_SURFACE_WITH_KNOTS((2,2),(3,2,2,3),(0.710318915639655,1.),(0.418207303127979,
0.428571428571429,0.435775021682622,0.435950698868169),.UNSPECIFIED.)
GEOMETRIC_REPRESENTATION_ITEM()
RATIONAL_B_SPLINE_SURFACE(((0.993779895952495,0.996362096314125,1.,0.997471472332736,
0.995452950231063,0.995452950231063,0.995452950231063),(0.993779895952495,
0.996362096314125,1.,0.997471472332736,0.995452950231063,0.995452950231063,
0.995452950231063)))
REPRESENTATION_ITEM('')
SURFACE()
);
#728=(
BOUNDED_SURFACE()
B_SPLINE_SURFACE(1,2,((#105698,#105699,#105700,#105701,#105702),(#105703,
#105704,#105705,#105706,#105707)),.UNSPECIFIED.,.F.,.F.,.F.)
B_SPLINE_SURFACE_WITH_KNOTS((2,2),(3,2,3),(0.710192959008363,1.),(0.297684616398974,
0.297856505190613,0.315045384354503),.UNSPECIFIED.)
GEOMETRIC_REPRESENTATION_ITEM()
RATIONAL_B_SPLINE_SURFACE(((0.992924952273132,0.992924952273132,0.992924952273132,
0.988942764095691,0.98786440923939),(0.992924952273132,0.992924952273132,
0.992924952273132,0.988942764095691,0.98786440923939)))
REPRESENTATION_ITEM('')
SURFACE()
);
#729=(
BOUNDED_SURFACE()
B_SPLINE_SURFACE(1,2,((#105715,#105716,#105717,#105718,#105719,#105720,
#105721),(#105722,#105723,#105724,#105725,#105726,#105727,#105728)),
 .UNSPECIFIED.,.F.,.F.,.F.)
B_SPLINE_SURFACE_WITH_KNOTS((2,2),(3,2,2,3),(0.71031891564,1.),(0.418207303127979,
0.428571428571429,0.435775021682622,0.435950698868169),.UNSPECIFIED.)
GEOMETRIC_REPRESENTATION_ITEM()
RATIONAL_B_SPLINE_SURFACE(((0.993779895952495,0.996362096314125,1.,0.997471472332736,
0.995452950231063,0.995452950231063,0.995452950231063),(0.993779895952495,
0.996362096314125,1.,0.997471472332736,0.995452950231063,0.995452950231063,
0.995452950231063)))
REPRESENTATION_ITEM('')
SURFACE()
);
#730=(
BOUNDED_SURFACE()
B_SPLINE_SURFACE(1,2,((#105745,#105746,#105747,#105748,#105749),(#105750,
#105751,#105752,#105753,#105754)),.UNSPECIFIED.,.F.,.F.,.F.)
B_SPLINE_SURFACE_WITH_KNOTS((2,2),(3,2,3),(0.710192959008359,1.),(0.297684616398974,
0.297856505190613,0.315045384354503),.UNSPECIFIED.)
GEOMETRIC_REPRESENTATION_ITEM()
RATIONAL_B_SPLINE_SURFACE(((0.992924952273132,0.992924952273132,0.992924952273132,
0.988942764095691,0.98786440923939),(0.992924952273132,0.992924952273132,
0.992924952273132,0.988942764095691,0.98786440923939)))
REPRESENTATION_ITEM('')
SURFACE()
);
#731=(
BOUNDED_SURFACE()
B_SPLINE_SURFACE(1,2,((#105762,#105763,#105764,#105765,#105766,#105767,
#105768),(#105769,#105770,#105771,#105772,#105773,#105774,#105775)),
 .UNSPECIFIED.,.F.,.F.,.F.)
B_SPLINE_SURFACE_WITH_KNOTS((2,2),(3,2,2,3),(0.710318915639998,1.),(0.418207303127979,
0.428571428571429,0.435775021682622,0.435950698868169),.UNSPECIFIED.)
GEOMETRIC_REPRESENTATION_ITEM()
RATIONAL_B_SPLINE_SURFACE(((0.993779895952495,0.996362096314125,1.,0.997471472332736,
0.995452950231063,0.995452950231063,0.995452950231063),(0.993779895952495,
0.996362096314125,1.,0.997471472332736,0.995452950231063,0.995452950231063,
0.995452950231063)))
REPRESENTATION_ITEM('')
SURFACE()
);
#732=(
BOUNDED_SURFACE()
B_SPLINE_SURFACE(1,2,((#105792,#105793,#105794,#105795,#105796),(#105797,
#105798,#105799,#105800,#105801)),.UNSPECIFIED.,.F.,.F.,.F.)
B_SPLINE_SURFACE_WITH_KNOTS((2,2),(3,2,3),(0.710192959008358,1.),(0.297684616398974,
0.297856505190613,0.315045384354503),.UNSPECIFIED.)
GEOMETRIC_REPRESENTATION_ITEM()
RATIONAL_B_SPLINE_SURFACE(((0.992924952273132,0.992924952273132,0.992924952273132,
0.988942764095691,0.98786440923939),(0.992924952273132,0.992924952273132,
0.992924952273132,0.988942764095691,0.98786440923939)))
REPRESENTATION_ITEM('')
SURFACE()
);
#733=(
BOUNDED_SURFACE()
B_SPLINE_SURFACE(1,2,((#105809,#105810,#105811,#105812,#105813,#105814,
#105815),(#105816,#105817,#105818,#105819,#105820,#105821,#105822)),
 .UNSPECIFIED.,.F.,.F.,.F.)
B_SPLINE_SURFACE_WITH_KNOTS((2,2),(3,2,2,3),(0.71031891563967,1.),(0.418207303127979,
0.428571428571429,0.435775021682622,0.435950698868169),.UNSPECIFIED.)
GEOMETRIC_REPRESENTATION_ITEM()
RATIONAL_B_SPLINE_SURFACE(((0.993779895952495,0.996362096314125,1.,0.997471472332736,
0.995452950231063,0.995452950231063,0.995452950231063),(0.993779895952495,
0.996362096314125,1.,0.997471472332736,0.995452950231063,0.995452950231063,
0.995452950231063)))
REPRESENTATION_ITEM('')
SURFACE()
);
#734=(
BOUNDED_SURFACE()
B_SPLINE_SURFACE(1,2,((#105839,#105840,#105841,#105842,#105843),(#105844,
#105845,#105846,#105847,#105848)),.UNSPECIFIED.,.F.,.F.,.F.)
B_SPLINE_SURFACE_WITH_KNOTS((2,2),(3,2,3),(0.71019295900844,1.),(0.297684616398974,
0.297856505190613,0.315045384354503),.UNSPECIFIED.)
GEOMETRIC_REPRESENTATION_ITEM()
RATIONAL_B_SPLINE_SURFACE(((0.992924952273132,0.992924952273132,0.992924952273132,
0.988942764095691,0.98786440923939),(0.992924952273132,0.992924952273132,
0.992924952273132,0.988942764095691,0.98786440923939)))
REPRESENTATION_ITEM('')
SURFACE()
);
#735=(
BOUNDED_SURFACE()
B_SPLINE_SURFACE(1,2,((#105856,#105857,#105858,#105859,#105860,#105861,
#105862),(#105863,#105864,#105865,#105866,#105867,#105868,#105869)),
 .UNSPECIFIED.,.F.,.F.,.F.)
B_SPLINE_SURFACE_WITH_KNOTS((2,2),(3,2,2,3),(0.710318915639991,1.),(0.418207303127979,
0.428571428571429,0.435775021682622,0.435950698868169),.UNSPECIFIED.)
GEOMETRIC_REPRESENTATION_ITEM()
RATIONAL_B_SPLINE_SURFACE(((0.993779895952495,0.996362096314125,1.,0.997471472332736,
0.995452950231063,0.995452950231063,0.995452950231063),(0.993779895952495,
0.996362096314125,1.,0.997471472332736,0.995452950231063,0.995452950231063,
0.995452950231063)))
REPRESENTATION_ITEM('')
SURFACE()
);
#736=(
BOUNDED_SURFACE()
B_SPLINE_SURFACE(1,2,((#105886,#105887,#105888,#105889,#105890),(#105891,
#105892,#105893,#105894,#105895)),.UNSPECIFIED.,.F.,.F.,.F.)
B_SPLINE_SURFACE_WITH_KNOTS((2,2),(3,2,3),(0.710192959008349,1.),(0.297684616398974,
0.297856505190613,0.315045384354503),.UNSPECIFIED.)
GEOMETRIC_REPRESENTATION_ITEM()
RATIONAL_B_SPLINE_SURFACE(((0.992924952273132,0.992924952273132,0.992924952273132,
0.988942764095691,0.98786440923939),(0.992924952273132,0.992924952273132,
0.992924952273132,0.988942764095691,0.98786440923939)))
REPRESENTATION_ITEM('')
SURFACE()
);
#737=(
BOUNDED_SURFACE()
B_SPLINE_SURFACE(1,2,((#105903,#105904,#105905,#105906,#105907,#105908,
#105909),(#105910,#105911,#105912,#105913,#105914,#105915,#105916)),
 .UNSPECIFIED.,.F.,.F.,.F.)
B_SPLINE_SURFACE_WITH_KNOTS((2,2),(3,2,2,3),(0.710318915640076,1.),(0.418207303127979,
0.428571428571429,0.435775021682622,0.435950698868169),.UNSPECIFIED.)
GEOMETRIC_REPRESENTATION_ITEM()
RATIONAL_B_SPLINE_SURFACE(((0.993779895952495,0.996362096314125,1.,0.997471472332736,
0.995452950231063,0.995452950231063,0.995452950231063),(0.993779895952495,
0.996362096314125,1.,0.997471472332736,0.995452950231063,0.995452950231063,
0.995452950231063)))
REPRESENTATION_ITEM('')
SURFACE()
);
#738=(
BOUNDED_SURFACE()
B_SPLINE_SURFACE(1,2,((#105933,#105934,#105935,#105936,#105937),(#105938,
#105939,#105940,#105941,#105942)),.UNSPECIFIED.,.F.,.F.,.F.)
B_SPLINE_SURFACE_WITH_KNOTS((2,2),(3,2,3),(0.710192959008437,1.),(0.297684616398974,
0.297856505190613,0.315045384354503),.UNSPECIFIED.)
GEOMETRIC_REPRESENTATION_ITEM()
RATIONAL_B_SPLINE_SURFACE(((0.992924952273132,0.992924952273132,0.992924952273132,
0.988942764095691,0.98786440923939),(0.992924952273132,0.992924952273132,
0.992924952273132,0.988942764095691,0.98786440923939)))
REPRESENTATION_ITEM('')
SURFACE()
);
#739=(
BOUNDED_SURFACE()
B_SPLINE_SURFACE(1,2,((#105950,#105951,#105952,#105953,#105954,#105955,
#105956),(#105957,#105958,#105959,#105960,#105961,#105962,#105963)),
 .UNSPECIFIED.,.F.,.F.,.F.)
B_SPLINE_SURFACE_WITH_KNOTS((2,2),(3,2,2,3),(0.710318915639662,1.),(0.418207303127979,
0.428571428571429,0.435775021682622,0.435950698868169),.UNSPECIFIED.)
GEOMETRIC_REPRESENTATION_ITEM()
RATIONAL_B_SPLINE_SURFACE(((0.993779895952495,0.996362096314125,1.,0.997471472332736,
0.995452950231063,0.995452950231063,0.995452950231063),(0.993779895952495,
0.996362096314125,1.,0.997471472332736,0.995452950231063,0.995452950231063,
0.995452950231063)))
REPRESENTATION_ITEM('')
SURFACE()
);
#740=(
BOUNDED_SURFACE()
B_SPLINE_SURFACE(1,2,((#105980,#105981,#105982,#105983,#105984),(#105985,
#105986,#105987,#105988,#105989)),.UNSPECIFIED.,.F.,.F.,.F.)
B_SPLINE_SURFACE_WITH_KNOTS((2,2),(3,2,3),(0.71019295900808,1.),(0.297684616398974,
0.297856505190613,0.315045384354503),.UNSPECIFIED.)
GEOMETRIC_REPRESENTATION_ITEM()
RATIONAL_B_SPLINE_SURFACE(((0.992924952273132,0.992924952273132,0.992924952273132,
0.988942764095691,0.98786440923939),(0.992924952273132,0.992924952273132,
0.992924952273132,0.988942764095691,0.98786440923939)))
REPRESENTATION_ITEM('')
SURFACE()
);
#741=(
BOUNDED_SURFACE()
B_SPLINE_SURFACE(1,2,((#105997,#105998,#105999,#106000,#106001,#106002,
#106003),(#106004,#106005,#106006,#106007,#106008,#106009,#106010)),
 .UNSPECIFIED.,.F.,.F.,.F.)
B_SPLINE_SURFACE_WITH_KNOTS((2,2),(3,2,2,3),(0.71031891563867,1.),(0.418207303127979,
0.428571428571429,0.435775021682622,0.435950698868169),.UNSPECIFIED.)
GEOMETRIC_REPRESENTATION_ITEM()
RATIONAL_B_SPLINE_SURFACE(((0.993779895952495,0.996362096314125,1.,0.997471472332736,
0.995452950231063,0.995452950231063,0.995452950231063),(0.993779895952495,
0.996362096314125,1.,0.997471472332736,0.995452950231063,0.995452950231063,
0.995452950231063)))
REPRESENTATION_ITEM('')
SURFACE()
);
#742=(
BOUNDED_SURFACE()
B_SPLINE_SURFACE(1,2,((#106027,#106028,#106029,#106030,#106031),(#106032,
#106033,#106034,#106035,#106036)),.UNSPECIFIED.,.F.,.F.,.F.)
B_SPLINE_SURFACE_WITH_KNOTS((2,2),(3,2,3),(0.710192959007034,1.),(0.297684616398974,
0.297856505190613,0.315045384354503),.UNSPECIFIED.)
GEOMETRIC_REPRESENTATION_ITEM()
RATIONAL_B_SPLINE_SURFACE(((0.992924952273132,0.992924952273132,0.992924952273132,
0.988942764095691,0.98786440923939),(0.992924952273132,0.992924952273132,
0.992924952273132,0.988942764095691,0.98786440923939)))
REPRESENTATION_ITEM('')
SURFACE()
);
#743=(
BOUNDED_SURFACE()
B_SPLINE_SURFACE(1,2,((#106044,#106045,#106046,#106047,#106048,#106049,
#106050),(#106051,#106052,#106053,#106054,#106055,#106056,#106057)),
 .UNSPECIFIED.,.F.,.F.,.F.)
B_SPLINE_SURFACE_WITH_KNOTS((2,2),(3,2,2,3),(0.710318915639954,1.),(0.418207303127979,
0.428571428571429,0.435775021682622,0.435950698868169),.UNSPECIFIED.)
GEOMETRIC_REPRESENTATION_ITEM()
RATIONAL_B_SPLINE_SURFACE(((0.993779895952495,0.996362096314125,1.,0.997471472332736,
0.995452950231063,0.995452950231063,0.995452950231063),(0.993779895952495,
0.996362096314125,1.,0.997471472332736,0.995452950231063,0.995452950231063,
0.995452950231063)))
REPRESENTATION_ITEM('')
SURFACE()
);
#744=(
BOUNDED_SURFACE()
B_SPLINE_SURFACE(1,2,((#106065,#106066,#106067,#106068,#106069),(#106070,
#106071,#106072,#106073,#106074)),.UNSPECIFIED.,.F.,.F.,.F.)
B_SPLINE_SURFACE_WITH_KNOTS((2,2),(3,2,3),(0.71019295900831,1.),(0.29768461639882,
0.297856505190461,0.315045384354504),.UNSPECIFIED.)
GEOMETRIC_REPRESENTATION_ITEM()
RATIONAL_B_SPLINE_SURFACE(((0.992924952273203,0.992924952273203,0.992924952273203,
0.988942764095701,0.98786440923939),(0.992924952273203,0.992924952273203,
0.992924952273203,0.988942764095701,0.98786440923939)))
REPRESENTATION_ITEM('')
SURFACE()
);
#745=(
BOUNDED_SURFACE()
B_SPLINE_SURFACE(1,2,((#106076,#106077,#106078,#106079,#106080,#106081,
#106082),(#106083,#106084,#106085,#106086,#106087,#106088,#106089)),
 .UNSPECIFIED.,.F.,.F.,.F.)
B_SPLINE_SURFACE_WITH_KNOTS((2,2),(3,2,2,3),(0.710318915640076,1.),(0.418207303127978,
0.428571428571429,0.435775021682622,0.435950698868169),.UNSPECIFIED.)
GEOMETRIC_REPRESENTATION_ITEM()
RATIONAL_B_SPLINE_SURFACE(((0.993779895952495,0.996362096314125,1.,0.997471472332736,
0.995452950231063,0.995452950231063,0.995452950231063),(0.993779895952495,
0.996362096314125,1.,0.997471472332736,0.995452950231063,0.995452950231063,
0.995452950231063)))
REPRESENTATION_ITEM('')
SURFACE()
);
#746=(
BOUNDED_SURFACE()
B_SPLINE_SURFACE(1,2,((#106106,#106107,#106108,#106109,#106110),(#106111,
#106112,#106113,#106114,#106115)),.UNSPECIFIED.,.F.,.F.,.F.)
B_SPLINE_SURFACE_WITH_KNOTS((2,2),(3,2,3),(0.710192959008433,1.),(0.297684616398974,
0.297856505190613,0.315045384354503),.UNSPECIFIED.)
GEOMETRIC_REPRESENTATION_ITEM()
RATIONAL_B_SPLINE_SURFACE(((0.992924952273132,0.992924952273132,0.992924952273132,
0.988942764095691,0.98786440923939),(0.992924952273132,0.992924952273132,
0.992924952273132,0.988942764095691,0.98786440923939)))
REPRESENTATION_ITEM('')
SURFACE()
);
#747=(
BOUNDED_SURFACE()
B_SPLINE_SURFACE(1,2,((#106123,#106124,#106125,#106126,#106127,#106128,
#106129),(#106130,#106131,#106132,#106133,#106134,#106135,#106136)),
 .UNSPECIFIED.,.F.,.F.,.F.)
B_SPLINE_SURFACE_WITH_KNOTS((2,2),(3,2,2,3),(0.71031891563985,1.),(0.418207303127979,
0.428571428571429,0.435775021682622,0.435950698868169),.UNSPECIFIED.)
GEOMETRIC_REPRESENTATION_ITEM()
RATIONAL_B_SPLINE_SURFACE(((0.993779895952495,0.996362096314125,1.,0.997471472332736,
0.995452950231063,0.995452950231063,0.995452950231063),(0.993779895952495,
0.996362096314125,1.,0.997471472332736,0.995452950231063,0.995452950231063,
0.995452950231063)))
REPRESENTATION_ITEM('')
SURFACE()
);
#748=(
BOUNDED_SURFACE()
B_SPLINE_SURFACE(1,2,((#106153,#106154,#106155,#106156,#106157),(#106158,
#106159,#106160,#106161,#106162)),.UNSPECIFIED.,.F.,.F.,.F.)
B_SPLINE_SURFACE_WITH_KNOTS((2,2),(3,2,3),(0.710192959008205,1.),(0.297684616398974,
0.297856505190613,0.315045384354503),.UNSPECIFIED.)
GEOMETRIC_REPRESENTATION_ITEM()
RATIONAL_B_SPLINE_SURFACE(((0.992924952273132,0.992924952273132,0.992924952273132,
0.988942764095691,0.987864409239391),(0.992924952273132,0.992924952273132,
0.992924952273132,0.988942764095691,0.98786440923939)))
REPRESENTATION_ITEM('')
SURFACE()
);
#749=(
BOUNDED_SURFACE()
B_SPLINE_SURFACE(1,2,((#106170,#106171,#106172,#106173,#106174,#106175,
#106176),(#106177,#106178,#106179,#106180,#106181,#106182,#106183)),
 .UNSPECIFIED.,.F.,.F.,.F.)
B_SPLINE_SURFACE_WITH_KNOTS((2,2),(3,2,2,3),(0.71031891564008,1.),(0.418207303127979,
0.428571428571429,0.435775021682622,0.435950698868169),.UNSPECIFIED.)
GEOMETRIC_REPRESENTATION_ITEM()
RATIONAL_B_SPLINE_SURFACE(((0.993779895952495,0.996362096314125,1.,0.997471472332736,
0.995452950231063,0.995452950231063,0.995452950231063),(0.993779895952495,
0.996362096314125,1.,0.997471472332736,0.995452950231063,0.995452950231063,
0.995452950231063)))
REPRESENTATION_ITEM('')
SURFACE()
);
#750=(
BOUNDED_SURFACE()
B_SPLINE_SURFACE(1,2,((#106200,#106201,#106202,#106203,#106204),(#106205,
#106206,#106207,#106208,#106209)),.UNSPECIFIED.,.F.,.F.,.F.)
B_SPLINE_SURFACE_WITH_KNOTS((2,2),(3,2,3),(0.71019295900844,1.),(0.297684616398974,
0.297856505190613,0.315045384354503),.UNSPECIFIED.)
GEOMETRIC_REPRESENTATION_ITEM()
RATIONAL_B_SPLINE_SURFACE(((0.992924952273132,0.992924952273132,0.992924952273132,
0.988942764095691,0.98786440923939),(0.992924952273132,0.992924952273132,
0.992924952273132,0.988942764095691,0.98786440923939)))
REPRESENTATION_ITEM('')
SURFACE()
);
#751=(
BOUNDED_SURFACE()
B_SPLINE_SURFACE(1,2,((#106217,#106218,#106219,#106220,#106221,#106222,
#106223),(#106224,#106225,#106226,#106227,#106228,#106229,#106230)),
 .UNSPECIFIED.,.F.,.F.,.F.)
B_SPLINE_SURFACE_WITH_KNOTS((2,2),(3,2,2,3),(0.710318915638946,1.),(0.418207303127979,
0.428571428571429,0.435775021682622,0.435950698868169),.UNSPECIFIED.)
GEOMETRIC_REPRESENTATION_ITEM()
RATIONAL_B_SPLINE_SURFACE(((0.993779895952495,0.996362096314125,1.,0.997471472332736,
0.995452950231063,0.995452950231063,0.995452950231063),(0.993779895952495,
0.996362096314125,1.,0.997471472332736,0.995452950231063,0.995452950231063,
0.995452950231063)))
REPRESENTATION_ITEM('')
SURFACE()
);
#752=(
BOUNDED_SURFACE()
B_SPLINE_SURFACE(1,2,((#106247,#106248,#106249,#106250,#106251),(#106252,
#106253,#106254,#106255,#106256)),.UNSPECIFIED.,.F.,.F.,.F.)
B_SPLINE_SURFACE_WITH_KNOTS((2,2),(3,2,3),(0.710192959007305,1.),(0.297684616398974,
0.297856505190613,0.315045384354503),.UNSPECIFIED.)
GEOMETRIC_REPRESENTATION_ITEM()
RATIONAL_B_SPLINE_SURFACE(((0.992924952273132,0.992924952273132,0.992924952273132,
0.988942764095691,0.98786440923939),(0.992924952273132,0.992924952273132,
0.992924952273132,0.988942764095691,0.98786440923939)))
REPRESENTATION_ITEM('')
SURFACE()
);
#753=(
BOUNDED_SURFACE()
B_SPLINE_SURFACE(1,2,((#106264,#106265,#106266,#106267,#106268,#106269,
#106270),(#106271,#106272,#106273,#106274,#106275,#106276,#106277)),
 .UNSPECIFIED.,.F.,.F.,.F.)
B_SPLINE_SURFACE_WITH_KNOTS((2,2),(3,2,2,3),(0.710318915639109,1.),(0.418207303127979,
0.428571428571429,0.435775021682622,0.435950698868169),.UNSPECIFIED.)
GEOMETRIC_REPRESENTATION_ITEM()
RATIONAL_B_SPLINE_SURFACE(((0.993779895952495,0.996362096314125,1.,0.997471472332736,
0.995452950231063,0.995452950231063,0.995452950231063),(0.993779895952495,
0.996362096314125,1.,0.997471472332736,0.995452950231063,0.995452950231063,
0.995452950231063)))
REPRESENTATION_ITEM('')
SURFACE()
);
#754=(
BOUNDED_SURFACE()
B_SPLINE_SURFACE(1,2,((#106294,#106295,#106296,#106297,#106298),(#106299,
#106300,#106301,#106302,#106303)),.UNSPECIFIED.,.F.,.F.,.F.)
B_SPLINE_SURFACE_WITH_KNOTS((2,2),(3,2,3),(0.710192959007464,1.),(0.297684616398492,
0.297856505190135,0.315045384354506),.UNSPECIFIED.)
GEOMETRIC_REPRESENTATION_ITEM()
RATIONAL_B_SPLINE_SURFACE(((0.992924952273353,0.992924952273353,0.992924952273353,
0.98894276409572,0.98786440923939),(0.992924952273353,0.992924952273353,
0.992924952273353,0.98894276409572,0.98786440923939)))
REPRESENTATION_ITEM('')
SURFACE()
);
#755=(
BOUNDED_SURFACE()
B_SPLINE_SURFACE(1,2,((#106311,#106312,#106313,#106314,#106315,#106316,
#106317),(#106318,#106319,#106320,#106321,#106322,#106323,#106324)),
 .UNSPECIFIED.,.F.,.F.,.F.)
B_SPLINE_SURFACE_WITH_KNOTS((2,2),(3,2,2,3),(0.710318915638971,1.),(0.418207303127979,
0.428571428571429,0.435775021682622,0.435950698868169),.UNSPECIFIED.)
GEOMETRIC_REPRESENTATION_ITEM()
RATIONAL_B_SPLINE_SURFACE(((0.993779895952495,0.996362096314125,1.,0.997471472332736,
0.995452950231063,0.995452950231063,0.995452950231063),(0.993779895952495,
0.996362096314125,1.,0.997471472332736,0.995452950231063,0.995452950231063,
0.995452950231063)))
REPRESENTATION_ITEM('')
SURFACE()
);
#756=(
BOUNDED_SURFACE()
B_SPLINE_SURFACE(1,2,((#106341,#106342,#106343,#106344,#106345),(#106346,
#106347,#106348,#106349,#106350)),.UNSPECIFIED.,.F.,.F.,.F.)
B_SPLINE_SURFACE_WITH_KNOTS((2,2),(3,2,3),(0.710192959007334,1.),(0.297684616398621,
0.297856505190263,0.315045384354506),.UNSPECIFIED.)
GEOMETRIC_REPRESENTATION_ITEM()
RATIONAL_B_SPLINE_SURFACE(((0.992924952273294,0.992924952273294,0.992924952273294,
0.988942764095713,0.98786440923939),(0.992924952273294,0.992924952273294,
0.992924952273294,0.988942764095713,0.98786440923939)))
REPRESENTATION_ITEM('')
SURFACE()
);
#757=(
BOUNDED_SURFACE()
B_SPLINE_SURFACE(1,2,((#106358,#106359,#106360,#106361,#106362,#106363,
#106364),(#106365,#106366,#106367,#106368,#106369,#106370,#106371)),
 .UNSPECIFIED.,.F.,.F.,.F.)
B_SPLINE_SURFACE_WITH_KNOTS((2,2),(3,2,2,3),(0.710318915639849,1.),(0.418207303127979,
0.428571428571429,0.435775021682622,0.435950698868169),.UNSPECIFIED.)
GEOMETRIC_REPRESENTATION_ITEM()
RATIONAL_B_SPLINE_SURFACE(((0.993779895952495,0.996362096314125,1.,0.997471472332736,
0.995452950231063,0.995452950231063,0.995452950231063),(0.993779895952495,
0.996362096314125,1.,0.997471472332736,0.995452950231063,0.995452950231063,
0.995452950231063)))
REPRESENTATION_ITEM('')
SURFACE()
);
#758=(
BOUNDED_SURFACE()
B_SPLINE_SURFACE(1,2,((#106388,#106389,#106390,#106391,#106392),(#106393,
#106394,#106395,#106396,#106397)),.UNSPECIFIED.,.F.,.F.,.F.)
B_SPLINE_SURFACE_WITH_KNOTS((2,2),(3,2,3),(0.710192959008238,1.),(0.297684616398974,
0.297856505190613,0.315045384354504),.UNSPECIFIED.)
GEOMETRIC_REPRESENTATION_ITEM()
RATIONAL_B_SPLINE_SURFACE(((0.992924952273132,0.992924952273132,0.992924952273132,
0.988942764095691,0.98786440923939),(0.992924952273132,0.992924952273132,
0.992924952273132,0.988942764095691,0.98786440923939)))
REPRESENTATION_ITEM('')
SURFACE()
);
#759=(
BOUNDED_SURFACE()
B_SPLINE_SURFACE(1,2,((#106405,#106406,#106407,#106408,#106409,#106410,
#106411),(#106412,#106413,#106414,#106415,#106416,#106417,#106418)),
 .UNSPECIFIED.,.F.,.F.,.F.)
B_SPLINE_SURFACE_WITH_KNOTS((2,2),(3,2,2,3),(0.710318915638589,1.),(0.418207303127979,
0.428571428571429,0.435775021682622,0.435950698868169),.UNSPECIFIED.)
GEOMETRIC_REPRESENTATION_ITEM()
RATIONAL_B_SPLINE_SURFACE(((0.993779895952495,0.996362096314125,1.,0.997471472332736,
0.995452950231063,0.995452950231063,0.995452950231063),(0.993779895952495,
0.996362096314125,1.,0.997471472332736,0.995452950231063,0.995452950231063,
0.995452950231063)))
REPRESENTATION_ITEM('')
SURFACE()
);
#760=(
BOUNDED_SURFACE()
B_SPLINE_SURFACE(1,2,((#106435,#106436,#106437,#106438,#106439),(#106440,
#106441,#106442,#106443,#106444)),.UNSPECIFIED.,.F.,.F.,.F.)
B_SPLINE_SURFACE_WITH_KNOTS((2,2),(3,2,3),(0.710192959006948,1.),(0.297684616398974,
0.297856505190613,0.315045384354503),.UNSPECIFIED.)
GEOMETRIC_REPRESENTATION_ITEM()
RATIONAL_B_SPLINE_SURFACE(((0.992924952273132,0.992924952273132,0.992924952273132,
0.988942764095691,0.98786440923939),(0.992924952273132,0.992924952273132,
0.992924952273132,0.988942764095691,0.98786440923939)))
REPRESENTATION_ITEM('')
SURFACE()
);
#761=(
BOUNDED_SURFACE()
B_SPLINE_SURFACE(1,2,((#106452,#106453,#106454,#106455,#106456,#106457,
#106458),(#106459,#106460,#106461,#106462,#106463,#106464,#106465)),
 .UNSPECIFIED.,.F.,.F.,.F.)
B_SPLINE_SURFACE_WITH_KNOTS((2,2),(3,2,2,3),(0.710318915638846,1.),(0.418207303127979,
0.428571428571429,0.435775021682622,0.435950698868169),.UNSPECIFIED.)
GEOMETRIC_REPRESENTATION_ITEM()
RATIONAL_B_SPLINE_SURFACE(((0.993779895952495,0.996362096314125,1.,0.997471472332736,
0.995452950231063,0.995452950231063,0.995452950231063),(0.993779895952495,
0.996362096314125,1.,0.997471472332736,0.995452950231063,0.995452950231063,
0.995452950231063)))
REPRESENTATION_ITEM('')
SURFACE()
);
#762=(
BOUNDED_SURFACE()
B_SPLINE_SURFACE(1,2,((#106482,#106483,#106484,#106485,#106486),(#106487,
#106488,#106489,#106490,#106491)),.UNSPECIFIED.,.F.,.F.,.F.)
B_SPLINE_SURFACE_WITH_KNOTS((2,2),(3,2,3),(0.710192959007198,1.),(0.297684616398974,
0.297856505190613,0.315045384354504),.UNSPECIFIED.)
GEOMETRIC_REPRESENTATION_ITEM()
RATIONAL_B_SPLINE_SURFACE(((0.992924952273132,0.992924952273132,0.992924952273132,
0.988942764095691,0.98786440923939),(0.992924952273132,0.992924952273132,
0.992924952273132,0.988942764095691,0.98786440923939)))
REPRESENTATION_ITEM('')
SURFACE()
);
#763=(
BOUNDED_SURFACE()
B_SPLINE_SURFACE(1,2,((#106499,#106500,#106501,#106502,#106503,#106504,
#106505),(#106506,#106507,#106508,#106509,#106510,#106511,#106512)),
 .UNSPECIFIED.,.F.,.F.,.F.)
B_SPLINE_SURFACE_WITH_KNOTS((2,2),(3,2,2,3),(0.710318915639085,1.),(0.418207303127979,
0.428571428571429,0.435775021682622,0.435950698868169),.UNSPECIFIED.)
GEOMETRIC_REPRESENTATION_ITEM()
RATIONAL_B_SPLINE_SURFACE(((0.993779895952495,0.996362096314125,1.,0.997471472332736,
0.995452950231063,0.995452950231063,0.995452950231063),(0.993779895952495,
0.996362096314125,1.,0.997471472332736,0.995452950231063,0.995452950231063,
0.995452950231063)))
REPRESENTATION_ITEM('')
SURFACE()
);
#764=(
BOUNDED_SURFACE()
B_SPLINE_SURFACE(1,2,((#106529,#106530,#106531,#106532,#106533),(#106534,
#106535,#106536,#106537,#106538)),.UNSPECIFIED.,.F.,.F.,.F.)
B_SPLINE_SURFACE_WITH_KNOTS((2,2),(3,2,3),(0.710192959007439,1.),(0.297684616398674,
0.297856505190316,0.315045384354505),.UNSPECIFIED.)
GEOMETRIC_REPRESENTATION_ITEM()
RATIONAL_B_SPLINE_SURFACE(((0.99292495227327,0.99292495227327,0.99292495227327,
0.98894276409571,0.98786440923939),(0.99292495227327,0.99292495227327,0.99292495227327,
0.988942764095709,0.98786440923939)))
REPRESENTATION_ITEM('')
SURFACE()
);
#765=(
BOUNDED_SURFACE()
B_SPLINE_SURFACE(1,2,((#106546,#106547,#106548,#106549,#106550,#106551,
#106552),(#106553,#106554,#106555,#106556,#106557,#106558,#106559)),
 .UNSPECIFIED.,.F.,.F.,.F.)
B_SPLINE_SURFACE_WITH_KNOTS((2,2),(3,2,2,3),(0.710318915639157,1.),(0.418207303127979,
0.428571428571429,0.435775021682622,0.435950698868169),.UNSPECIFIED.)
GEOMETRIC_REPRESENTATION_ITEM()
RATIONAL_B_SPLINE_SURFACE(((0.993779895952495,0.996362096314125,1.,0.997471472332736,
0.995452950231063,0.995452950231063,0.995452950231063),(0.993779895952495,
0.996362096314125,1.,0.997471472332736,0.995452950231063,0.995452950231063,
0.995452950231063)))
REPRESENTATION_ITEM('')
SURFACE()
);
#766=(
BOUNDED_SURFACE()
B_SPLINE_SURFACE(1,2,((#106576,#106577,#106578,#106579,#106580),(#106581,
#106582,#106583,#106584,#106585)),.UNSPECIFIED.,.F.,.F.,.F.)
B_SPLINE_SURFACE_WITH_KNOTS((2,2),(3,2,3),(0.710192959007517,1.),(0.297684616398974,
0.297856505190613,0.315045384354506),.UNSPECIFIED.)
GEOMETRIC_REPRESENTATION_ITEM()
RATIONAL_B_SPLINE_SURFACE(((0.992924952273132,0.992924952273132,0.992924952273132,
0.98894276409569,0.98786440923939),(0.992924952273132,0.992924952273132,
0.992924952273132,0.98894276409569,0.98786440923939)))
REPRESENTATION_ITEM('')
SURFACE()
);
#767=(
BOUNDED_SURFACE()
B_SPLINE_SURFACE(1,2,((#106593,#106594,#106595,#106596,#106597,#106598,
#106599),(#106600,#106601,#106602,#106603,#106604,#106605,#106606)),
 .UNSPECIFIED.,.F.,.F.,.F.)
B_SPLINE_SURFACE_WITH_KNOTS((2,2),(3,2,2,3),(0.710318915638831,1.),(0.418207303127979,
0.428571428571429,0.435775021682622,0.435950698868169),.UNSPECIFIED.)
GEOMETRIC_REPRESENTATION_ITEM()
RATIONAL_B_SPLINE_SURFACE(((0.993779895952495,0.996362096314125,1.,0.997471472332736,
0.995452950231063,0.995452950231063,0.995452950231063),(0.993779895952495,
0.996362096314125,1.,0.997471472332736,0.995452950231063,0.995452950231063,
0.995452950231063)))
REPRESENTATION_ITEM('')
SURFACE()
);
#768=(
BOUNDED_SURFACE()
B_SPLINE_SURFACE(1,2,((#106623,#106624,#106625,#106626,#106627),(#106628,
#106629,#106630,#106631,#106632)),.UNSPECIFIED.,.F.,.F.,.F.)
B_SPLINE_SURFACE_WITH_KNOTS((2,2),(3,2,3),(0.710192959007199,1.),(0.297684616398623,
0.297856505190265,0.315045384354506),.UNSPECIFIED.)
GEOMETRIC_REPRESENTATION_ITEM()
RATIONAL_B_SPLINE_SURFACE(((0.992924952273293,0.992924952273293,0.992924952273293,
0.988942764095713,0.98786440923939),(0.992924952273293,0.992924952273293,
0.992924952273293,0.988942764095713,0.98786440923939)))
REPRESENTATION_ITEM('')
SURFACE()
);
#769=(
BOUNDED_SURFACE()
B_SPLINE_SURFACE(1,2,((#106640,#106641,#106642,#106643,#106644,#106645,
#106646),(#106647,#106648,#106649,#106650,#106651,#106652,#106653)),
 .UNSPECIFIED.,.F.,.F.,.F.)
B_SPLINE_SURFACE_WITH_KNOTS((2,2),(3,2,2,3),(0.710318915638982,1.),(0.418207303127979,
0.428571428571429,0.435775021682622,0.435950698868169),.UNSPECIFIED.)
GEOMETRIC_REPRESENTATION_ITEM()
RATIONAL_B_SPLINE_SURFACE(((0.993779895952495,0.996362096314125,1.,0.997471472332736,
0.995452950231063,0.995452950231063,0.995452950231063),(0.993779895952495,
0.996362096314125,1.,0.997471472332736,0.995452950231063,0.995452950231063,
0.995452950231063)))
REPRESENTATION_ITEM('')
SURFACE()
);
#770=(
BOUNDED_SURFACE()
B_SPLINE_SURFACE(1,2,((#106670,#106671,#106672,#106673,#106674),(#106675,
#106676,#106677,#106678,#106679)),.UNSPECIFIED.,.F.,.F.,.F.)
B_SPLINE_SURFACE_WITH_KNOTS((2,2),(3,2,3),(0.710192959007344,1.),(0.297684616398843,
0.297856505190483,0.315045384354504),.UNSPECIFIED.)
GEOMETRIC_REPRESENTATION_ITEM()
RATIONAL_B_SPLINE_SURFACE(((0.992924952273192,0.992924952273192,0.992924952273192,
0.988942764095699,0.98786440923939),(0.992924952273192,0.992924952273192,
0.992924952273192,0.988942764095699,0.98786440923939)))
REPRESENTATION_ITEM('')
SURFACE()
);
#771=(
BOUNDED_SURFACE()
B_SPLINE_SURFACE(1,2,((#106687,#106688,#106689,#106690,#106691,#106692,
#106693),(#106694,#106695,#106696,#106697,#106698,#106699,#106700)),
 .UNSPECIFIED.,.F.,.F.,.F.)
B_SPLINE_SURFACE_WITH_KNOTS((2,2),(3,2,2,3),(0.710318915638968,1.),(0.418207303127979,
0.428571428571429,0.435775021682622,0.435950698868169),.UNSPECIFIED.)
GEOMETRIC_REPRESENTATION_ITEM()
RATIONAL_B_SPLINE_SURFACE(((0.993779895952495,0.996362096314125,1.,0.997471472332736,
0.995452950231063,0.995452950231063,0.995452950231063),(0.993779895952495,
0.996362096314125,1.,0.997471472332736,0.995452950231063,0.995452950231063,
0.995452950231063)))
REPRESENTATION_ITEM('')
SURFACE()
);
#772=(
BOUNDED_SURFACE()
B_SPLINE_SURFACE(1,2,((#106717,#106718,#106719,#106720,#106721),(#106722,
#106723,#106724,#106725,#106726)),.UNSPECIFIED.,.F.,.F.,.F.)
B_SPLINE_SURFACE_WITH_KNOTS((2,2),(3,2,3),(0.710192959007328,1.),(0.297684616398544,
0.297856505190187,0.315045384354506),.UNSPECIFIED.)
GEOMETRIC_REPRESENTATION_ITEM()
RATIONAL_B_SPLINE_SURFACE(((0.99292495227333,0.99292495227333,0.99292495227333,
0.988942764095718,0.98786440923939),(0.99292495227333,0.99292495227333,
0.99292495227333,0.988942764095718,0.98786440923939)))
REPRESENTATION_ITEM('')
SURFACE()
);
#773=(
BOUNDED_SURFACE()
B_SPLINE_SURFACE(1,2,((#106746,#106747,#106748,#106749,#106750,#106751,
#106752),(#106753,#106754,#106755,#106756,#106757,#106758,#106759)),
 .UNSPECIFIED.,.F.,.F.,.F.)
B_SPLINE_SURFACE_WITH_KNOTS((2,2),(3,2,2,3),(0.710318915638782,1.),(0.418207303127979,
0.428571428571429,0.435775021682622,0.435950698868169),.UNSPECIFIED.)
GEOMETRIC_REPRESENTATION_ITEM()
RATIONAL_B_SPLINE_SURFACE(((0.993779895952495,0.996362096314125,1.,0.997471472332736,
0.995452950231063,0.995452950231063,0.995452950231063),(0.993779895952495,
0.996362096314125,1.,0.997471472332736,0.995452950231063,0.995452950231063,
0.995452950231063)))
REPRESENTATION_ITEM('')
SURFACE()
);
#774=(
BOUNDED_SURFACE()
B_SPLINE_SURFACE(1,2,((#106761,#106762,#106763),(#106764,#106765,#106766)),
 .UNSPECIFIED.,.F.,.F.,.F.)
B_SPLINE_SURFACE_WITH_KNOTS((2,2),(3,3),(0.710318915639741,1.),(0.331965345783649,
0.349369696259361),.UNSPECIFIED.)
GEOMETRIC_REPRESENTATION_ITEM()
RATIONAL_B_SPLINE_SURFACE(((0.988555124858682,0.99035748704491,0.99513694090229),
(0.988555124858682,0.99035748704491,0.99513694090229)))
REPRESENTATION_ITEM('')
SURFACE()
);
#775=(
BOUNDED_SURFACE()
B_SPLINE_SURFACE(1,2,((#106775,#106776,#106777,#106778,#106779),(#106780,
#106781,#106782,#106783,#106784),(#106785,#106786,#106787,#106788,#106789)),
 .UNSPECIFIED.,.F.,.F.,.F.)
B_SPLINE_SURFACE_WITH_KNOTS((2,1,2),(3,2,3),(0.709600445964224,1.,1.00289807040992),
(0.383340713896642,0.383933227114987,0.401145492974693),.UNSPECIFIED.)
GEOMETRIC_REPRESENTATION_ITEM()
RATIONAL_B_SPLINE_SURFACE(((0.988246641953811,0.988246641953811,0.988246641953811,
0.986737013496293,0.988139125479961),(0.988246641953811,0.988246641953811,
0.988246641953811,0.986737013496293,0.988139125479961),(0.988246641953811,
0.988246641953811,0.988246641953811,0.986737013496293,0.988139125479961)))
REPRESENTATION_ITEM('')
SURFACE()
);
#776=(
BOUNDED_SURFACE()
B_SPLINE_SURFACE(1,2,((#106798,#106799,#106800),(#106801,#106802,#106803)),
 .UNSPECIFIED.,.F.,.F.,.F.)
B_SPLINE_SURFACE_WITH_KNOTS((2,2),(3,3),(0.710318915639637,1.),(0.331965345783649,
0.349369696259364),.UNSPECIFIED.)
GEOMETRIC_REPRESENTATION_ITEM()
RATIONAL_B_SPLINE_SURFACE(((0.988555124858682,0.990357487044911,0.995136940902291),
(0.988555124858682,0.990357487044911,0.995136940902291)))
REPRESENTATION_ITEM('')
SURFACE()
);
#777=(
BOUNDED_SURFACE()
B_SPLINE_SURFACE(1,2,((#106805,#106806,#106807,#106808,#106809),(#106810,
#106811,#106812,#106813,#106814),(#106815,#106816,#106817,#106818,#106819)),
 .UNSPECIFIED.,.F.,.F.,.F.)
B_SPLINE_SURFACE_WITH_KNOTS((2,1,2),(3,2,3),(0.709600445987324,1.,1.00289807040993),
(0.383340713920641,0.383933227114984,0.401145492974693),.UNSPECIFIED.)
GEOMETRIC_REPRESENTATION_ITEM()
RATIONAL_B_SPLINE_SURFACE(((0.988246641953811,0.988246641953811,0.988246641953811,
0.986737013496293,0.988139125479962),(0.988246641953811,0.988246641953811,
0.988246641953811,0.986737013496293,0.988139125479962),(0.988246641953811,
0.988246641953811,0.988246641953811,0.986737013496293,0.988139125479962)))
REPRESENTATION_ITEM('')
SURFACE()
);
#778=(
BOUNDED_SURFACE()
B_SPLINE_SURFACE(1,2,((#106828,#106829,#106830),(#106831,#106832,#106833)),
 .UNSPECIFIED.,.F.,.F.,.F.)
B_SPLINE_SURFACE_WITH_KNOTS((2,2),(3,3),(0.710318915638942,1.),(0.331965345783649,
0.349369696259367),.UNSPECIFIED.)
GEOMETRIC_REPRESENTATION_ITEM()
RATIONAL_B_SPLINE_SURFACE(((0.988555124858681,0.990357487044911,0.995136940902293),
(0.988555124858681,0.990357487044911,0.995136940902293)))
REPRESENTATION_ITEM('')
SURFACE()
);
#779=(
BOUNDED_SURFACE()
B_SPLINE_SURFACE(1,2,((#106835,#106836,#106837,#106838,#106839),(#106840,
#106841,#106842,#106843,#106844),(#106845,#106846,#106847,#106848,#106849)),
 .UNSPECIFIED.,.F.,.F.,.F.)
B_SPLINE_SURFACE_WITH_KNOTS((2,1,2),(3,2,3),(0.709600445972972,1.,1.00289807040993),
(0.383340713906237,0.383933227114983,0.401145492974693),.UNSPECIFIED.)
GEOMETRIC_REPRESENTATION_ITEM()
RATIONAL_B_SPLINE_SURFACE(((0.988246641953811,0.988246641953811,0.988246641953811,
0.986737013496293,0.988139125479961),(0.988246641953811,0.988246641953811,
0.988246641953811,0.986737013496293,0.988139125479961),(0.988246641953811,
0.988246641953811,0.988246641953811,0.986737013496293,0.988139125479961)))
REPRESENTATION_ITEM('')
SURFACE()
);
#780=(
BOUNDED_SURFACE()
B_SPLINE_SURFACE(1,2,((#106858,#106859,#106860),(#106861,#106862,#106863)),
 .UNSPECIFIED.,.F.,.F.,.F.)
B_SPLINE_SURFACE_WITH_KNOTS((2,2),(3,3),(0.710318915639095,1.),(0.331965345783647,
0.349369696259361),.UNSPECIFIED.)
GEOMETRIC_REPRESENTATION_ITEM()
RATIONAL_B_SPLINE_SURFACE(((0.988555124858681,0.99035748704491,0.99513694090229),
(0.988555124858681,0.99035748704491,0.99513694090229)))
REPRESENTATION_ITEM('')
SURFACE()
);
#781=(
BOUNDED_SURFACE()
B_SPLINE_SURFACE(1,2,((#106865,#106866,#106867,#106868,#106869),(#106870,
#106871,#106872,#106873,#106874),(#106875,#106876,#106877,#106878,#106879)),
 .UNSPECIFIED.,.F.,.F.,.F.)
B_SPLINE_SURFACE_WITH_KNOTS((2,1,2),(3,2,3),(0.7096004459634,1.,1.00289807040993),
(0.383340713896623,0.383933227114983,0.401145492974693),.UNSPECIFIED.)
GEOMETRIC_REPRESENTATION_ITEM()
RATIONAL_B_SPLINE_SURFACE(((0.988246641953811,0.988246641953811,0.988246641953811,
0.986737013496292,0.988139125479961),(0.988246641953811,0.988246641953811,
0.988246641953811,0.986737013496293,0.988139125479961),(0.988246641953811,
0.988246641953811,0.988246641953811,0.986737013496293,0.988139125479961)))
REPRESENTATION_ITEM('')
SURFACE()
);
#782=(
BOUNDED_SURFACE()
B_SPLINE_SURFACE(1,2,((#106888,#106889,#106890),(#106891,#106892,#106893)),
 .UNSPECIFIED.,.F.,.F.,.F.)
B_SPLINE_SURFACE_WITH_KNOTS((2,2),(3,3),(0.710318915639123,1.),(0.331965345783649,
0.349369696259361),.UNSPECIFIED.)
GEOMETRIC_REPRESENTATION_ITEM()
RATIONAL_B_SPLINE_SURFACE(((0.988555124858681,0.99035748704491,0.99513694090229),
(0.988555124858681,0.99035748704491,0.99513694090229)))
REPRESENTATION_ITEM('')
SURFACE()
);
#783=(
BOUNDED_SURFACE()
B_SPLINE_SURFACE(1,2,((#106895,#106896,#106897,#106898,#106899),(#106900,
#106901,#106902,#106903,#106904),(#106905,#106906,#106907,#106908,#106909)),
 .UNSPECIFIED.,.F.,.F.,.F.)
B_SPLINE_SURFACE_WITH_KNOTS((2,1,2),(3,2,3),(0.709600445963976,1.,1.00289807040993),
(0.383340713897237,0.383933227114985,0.401145492974693),.UNSPECIFIED.)
GEOMETRIC_REPRESENTATION_ITEM()
RATIONAL_B_SPLINE_SURFACE(((0.988246641953811,0.988246641953811,0.988246641953811,
0.986737013496293,0.988139125479962),(0.988246641953811,0.988246641953811,
0.988246641953811,0.986737013496293,0.988139125479962),(0.988246641953811,
0.988246641953811,0.988246641953811,0.986737013496293,0.988139125479962)))
REPRESENTATION_ITEM('')
SURFACE()
);
#784=(
BOUNDED_SURFACE()
B_SPLINE_SURFACE(1,2,((#106918,#106919,#106920),(#106921,#106922,#106923)),
 .UNSPECIFIED.,.F.,.F.,.F.)
B_SPLINE_SURFACE_WITH_KNOTS((2,2),(3,3),(0.710318915638953,1.),(0.331965345783649,
0.349369696259361),.UNSPECIFIED.)
GEOMETRIC_REPRESENTATION_ITEM()
RATIONAL_B_SPLINE_SURFACE(((0.988555124858682,0.99035748704491,0.99513694090229),
(0.988555124858681,0.99035748704491,0.99513694090229)))
REPRESENTATION_ITEM('')
SURFACE()
);
#785=(
BOUNDED_SURFACE()
B_SPLINE_SURFACE(1,2,((#106925,#106926,#106927,#106928,#106929),(#106930,
#106931,#106932,#106933,#106934),(#106935,#106936,#106937,#106938,#106939)),
 .UNSPECIFIED.,.F.,.F.,.F.)
B_SPLINE_SURFACE_WITH_KNOTS((2,1,2),(3,2,3),(0.709600445977375,1.,1.00289807040992),
(0.383340713910112,0.38393322711497,0.401145492974693),.UNSPECIFIED.)
GEOMETRIC_REPRESENTATION_ITEM()
RATIONAL_B_SPLINE_SURFACE(((0.988246641953814,0.988246641953814,0.988246641953814,
0.986737013496291,0.988139125479961),(0.988246641953814,0.988246641953814,
0.988246641953814,0.986737013496291,0.988139125479961),(0.988246641953814,
0.988246641953814,0.988246641953814,0.986737013496291,0.988139125479961)))
REPRESENTATION_ITEM('')
SURFACE()
);
#786=(
BOUNDED_SURFACE()
B_SPLINE_SURFACE(1,2,((#106948,#106949,#106950),(#106951,#106952,#106953)),
 .UNSPECIFIED.,.F.,.F.,.F.)
B_SPLINE_SURFACE_WITH_KNOTS((2,2),(3,3),(0.710318915639313,1.),(0.331965345783649,
0.349369696259361),.UNSPECIFIED.)
GEOMETRIC_REPRESENTATION_ITEM()
RATIONAL_B_SPLINE_SURFACE(((0.988555124858681,0.99035748704491,0.99513694090229),
(0.988555124858681,0.99035748704491,0.99513694090229)))
REPRESENTATION_ITEM('')
SURFACE()
);
#787=(
BOUNDED_SURFACE()
B_SPLINE_SURFACE(1,2,((#106955,#106956,#106957,#106958,#106959),(#106960,
#106961,#106962,#106963,#106964),(#106965,#106966,#106967,#106968,#106969)),
 .UNSPECIFIED.,.F.,.F.,.F.)
B_SPLINE_SURFACE_WITH_KNOTS((2,1,2),(3,2,3),(0.709600445975744,1.,1.00289807040992),
(0.383340713908609,0.383933227114969,0.401145492974693),.UNSPECIFIED.)
GEOMETRIC_REPRESENTATION_ITEM()
RATIONAL_B_SPLINE_SURFACE(((0.988246641953814,0.988246641953814,0.988246641953814,
0.986737013496292,0.988139125479962),(0.988246641953814,0.988246641953814,
0.988246641953814,0.986737013496292,0.988139125479962),(0.988246641953814,
0.988246641953814,0.988246641953814,0.986737013496292,0.988139125479962)))
REPRESENTATION_ITEM('')
SURFACE()
);
#788=(
BOUNDED_SURFACE()
B_SPLINE_SURFACE(1,2,((#106978,#106979,#106980),(#106981,#106982,#106983)),
 .UNSPECIFIED.,.F.,.F.,.F.)
B_SPLINE_SURFACE_WITH_KNOTS((2,2),(3,3),(0.710318915639192,1.),(0.331965345783646,
0.349369696259361),.UNSPECIFIED.)
GEOMETRIC_REPRESENTATION_ITEM()
RATIONAL_B_SPLINE_SURFACE(((0.988555124858681,0.99035748704491,0.99513694090229),
(0.988555124858681,0.99035748704491,0.99513694090229)))
REPRESENTATION_ITEM('')
SURFACE()
);
#789=(
BOUNDED_SURFACE()
B_SPLINE_SURFACE(1,2,((#106985,#106986,#106987,#106988,#106989),(#106990,
#106991,#106992,#106993,#106994),(#106995,#106996,#106997,#106998,#106999)),
 .UNSPECIFIED.,.F.,.F.,.F.)
B_SPLINE_SURFACE_WITH_KNOTS((2,1,2),(3,2,3),(0.709600445963145,1.,1.00289807040993),
(0.383340713896254,0.38393322711497,0.401145492974693),.UNSPECIFIED.)
GEOMETRIC_REPRESENTATION_ITEM()
RATIONAL_B_SPLINE_SURFACE(((0.988246641953814,0.988246641953814,0.988246641953814,
0.986737013496292,0.988139125479962),(0.988246641953814,0.988246641953814,
0.988246641953814,0.986737013496292,0.988139125479962),(0.988246641953814,
0.988246641953814,0.988246641953814,0.986737013496292,0.988139125479962)))
REPRESENTATION_ITEM('')
SURFACE()
);
#790=(
BOUNDED_SURFACE()
B_SPLINE_SURFACE(1,2,((#107008,#107009,#107010),(#107011,#107012,#107013)),
 .UNSPECIFIED.,.F.,.F.,.F.)
B_SPLINE_SURFACE_WITH_KNOTS((2,2),(3,3),(0.710318915638951,1.),(0.331965345783647,
0.349369696259361),.UNSPECIFIED.)
GEOMETRIC_REPRESENTATION_ITEM()
RATIONAL_B_SPLINE_SURFACE(((0.988555124858681,0.99035748704491,0.99513694090229),
(0.988555124858681,0.99035748704491,0.99513694090229)))
REPRESENTATION_ITEM('')
SURFACE()
);
#791=(
BOUNDED_SURFACE()
B_SPLINE_SURFACE(1,2,((#107015,#107016,#107017,#107018,#107019),(#107020,
#107021,#107022,#107023,#107024),(#107025,#107026,#107027,#107028,#107029)),
 .UNSPECIFIED.,.F.,.F.,.F.)
B_SPLINE_SURFACE_WITH_KNOTS((2,1,2),(3,2,3),(0.709600445963726,1.,1.00289807040993),
(0.383340713897051,0.38393322711497,0.401145492974693),.UNSPECIFIED.)
GEOMETRIC_REPRESENTATION_ITEM()
RATIONAL_B_SPLINE_SURFACE(((0.988246641953814,0.988246641953814,0.988246641953814,
0.986737013496292,0.988139125479961),(0.988246641953814,0.988246641953814,
0.988246641953814,0.986737013496292,0.988139125479961),(0.988246641953814,
0.988246641953814,0.988246641953814,0.986737013496292,0.988139125479961)))
REPRESENTATION_ITEM('')
SURFACE()
);
#792=(
BOUNDED_SURFACE()
B_SPLINE_SURFACE(1,2,((#107038,#107039,#107040),(#107041,#107042,#107043)),
 .UNSPECIFIED.,.F.,.F.,.F.)
B_SPLINE_SURFACE_WITH_KNOTS((2,2),(3,3),(0.710318915638733,1.),(0.331965345783646,
0.349369696259361),.UNSPECIFIED.)
GEOMETRIC_REPRESENTATION_ITEM()
RATIONAL_B_SPLINE_SURFACE(((0.988555124858681,0.99035748704491,0.99513694090229),
(0.988555124858681,0.99035748704491,0.99513694090229)))
REPRESENTATION_ITEM('')
SURFACE()
);
#793=(
BOUNDED_SURFACE()
B_SPLINE_SURFACE(1,2,((#107045,#107046,#107047,#107048,#107049),(#107050,
#107051,#107052,#107053,#107054),(#107055,#107056,#107057,#107058,#107059)),
 .UNSPECIFIED.,.F.,.F.,.F.)
B_SPLINE_SURFACE_WITH_KNOTS((2,1,2),(3,2,3),(0.709600445979167,1.,1.00289807040992),
(0.383340713911332,0.383933227114987,0.401145492974693),.UNSPECIFIED.)
GEOMETRIC_REPRESENTATION_ITEM()
RATIONAL_B_SPLINE_SURFACE(((0.988246641953811,0.988246641953811,0.988246641953811,
0.986737013496293,0.988139125479962),(0.988246641953811,0.988246641953811,
0.988246641953811,0.986737013496293,0.988139125479962),(0.988246641953811,
0.988246641953811,0.988246641953811,0.986737013496293,0.988139125479962)))
REPRESENTATION_ITEM('')
SURFACE()
);
#794=(
BOUNDED_SURFACE()
B_SPLINE_SURFACE(1,2,((#107068,#107069,#107070),(#107071,#107072,#107073)),
 .UNSPECIFIED.,.F.,.F.,.F.)
B_SPLINE_SURFACE_WITH_KNOTS((2,2),(3,3),(0.710318915639885,1.),(0.331965345783647,
0.349369696259361),.UNSPECIFIED.)
GEOMETRIC_REPRESENTATION_ITEM()
RATIONAL_B_SPLINE_SURFACE(((0.988555124858681,0.99035748704491,0.99513694090229),
(0.988555124858681,0.99035748704491,0.99513694090229)))
REPRESENTATION_ITEM('')
SURFACE()
);
#795=(
BOUNDED_SURFACE()
B_SPLINE_SURFACE(1,2,((#107075,#107076,#107077,#107078,#107079),(#107080,
#107081,#107082,#107083,#107084),(#107085,#107086,#107087,#107088,#107089)),
 .UNSPECIFIED.,.F.,.F.,.F.)
B_SPLINE_SURFACE_WITH_KNOTS((2,1,2),(3,2,3),(0.709600445978175,1.,1.00289807040992),
(0.383340713910296,0.383933227114987,0.401145492974693),.UNSPECIFIED.)
GEOMETRIC_REPRESENTATION_ITEM()
RATIONAL_B_SPLINE_SURFACE(((0.988246641953811,0.988246641953811,0.988246641953811,
0.986737013496293,0.988139125479961),(0.988246641953811,0.988246641953811,
0.988246641953811,0.986737013496293,0.988139125479961),(0.988246641953811,
0.988246641953811,0.988246641953811,0.986737013496293,0.988139125479961)))
REPRESENTATION_ITEM('')
SURFACE()
);
#796=(
BOUNDED_SURFACE()
B_SPLINE_SURFACE(1,2,((#107098,#107099,#107100),(#107101,#107102,#107103)),
 .UNSPECIFIED.,.F.,.F.,.F.)
B_SPLINE_SURFACE_WITH_KNOTS((2,2),(3,3),(0.71031891563993,1.),(0.331965345783646,
0.349369696259361),.UNSPECIFIED.)
GEOMETRIC_REPRESENTATION_ITEM()
RATIONAL_B_SPLINE_SURFACE(((0.988555124858681,0.99035748704491,0.99513694090229),
(0.988555124858681,0.99035748704491,0.99513694090229)))
REPRESENTATION_ITEM('')
SURFACE()
);
#797=(
BOUNDED_SURFACE()
B_SPLINE_SURFACE(1,2,((#107105,#107106,#107107,#107108,#107109),(#107110,
#107111,#107112,#107113,#107114),(#107115,#107116,#107117,#107118,#107119)),
 .UNSPECIFIED.,.F.,.F.,.F.)
B_SPLINE_SURFACE_WITH_KNOTS((2,1,2),(3,2,3),(0.709600445969953,1.,1.00289807040992),
(0.383340713901921,0.383933227114987,0.401145492974693),.UNSPECIFIED.)
GEOMETRIC_REPRESENTATION_ITEM()
RATIONAL_B_SPLINE_SURFACE(((0.988246641953811,0.988246641953811,0.988246641953811,
0.986737013496293,0.988139125479962),(0.988246641953811,0.988246641953811,
0.988246641953811,0.986737013496293,0.988139125479962),(0.988246641953811,
0.988246641953811,0.988246641953811,0.986737013496293,0.988139125479962)))
REPRESENTATION_ITEM('')
SURFACE()
);
#798=(
BOUNDED_SURFACE()
B_SPLINE_SURFACE(1,2,((#107128,#107129,#107130),(#107131,#107132,#107133)),
 .UNSPECIFIED.,.F.,.F.,.F.)
B_SPLINE_SURFACE_WITH_KNOTS((2,2),(3,3),(0.710318915640068,1.),(0.331965345783649,
0.349369696259361),.UNSPECIFIED.)
GEOMETRIC_REPRESENTATION_ITEM()
RATIONAL_B_SPLINE_SURFACE(((0.988555124858682,0.99035748704491,0.99513694090229),
(0.988555124858682,0.99035748704491,0.99513694090229)))
REPRESENTATION_ITEM('')
SURFACE()
);
#799=(
BOUNDED_SURFACE()
B_SPLINE_SURFACE(1,2,((#107135,#107136,#107137,#107138,#107139),(#107140,
#107141,#107142,#107143,#107144),(#107145,#107146,#107147,#107148,#107149)),
 .UNSPECIFIED.,.F.,.F.,.F.)
B_SPLINE_SURFACE_WITH_KNOTS((2,1,2),(3,2,3),(0.70960044597758,1.,1.00289807040992),
(0.383340713909544,0.383933227114987,0.401145492974693),.UNSPECIFIED.)
GEOMETRIC_REPRESENTATION_ITEM()
RATIONAL_B_SPLINE_SURFACE(((0.988246641953811,0.988246641953811,0.988246641953811,
0.986737013496293,0.988139125479962),(0.988246641953811,0.988246641953811,
0.988246641953811,0.986737013496293,0.988139125479962),(0.988246641953811,
0.988246641953811,0.988246641953811,0.986737013496293,0.988139125479962)))
REPRESENTATION_ITEM('')
SURFACE()
);
#800=(
BOUNDED_SURFACE()
B_SPLINE_SURFACE(1,2,((#107158,#107159,#107160),(#107161,#107162,#107163)),
 .UNSPECIFIED.,.F.,.F.,.F.)
B_SPLINE_SURFACE_WITH_KNOTS((2,2),(3,3),(0.71031891564007,1.),(0.331965345783649,
0.349369696259361),.UNSPECIFIED.)
GEOMETRIC_REPRESENTATION_ITEM()
RATIONAL_B_SPLINE_SURFACE(((0.988555124858681,0.99035748704491,0.99513694090229),
(0.988555124858681,0.99035748704491,0.99513694090229)))
REPRESENTATION_ITEM('')
SURFACE()
);
#801=(
BOUNDED_SURFACE()
B_SPLINE_SURFACE(1,2,((#107165,#107166,#107167,#107168,#107169),(#107170,
#107171,#107172,#107173,#107174),(#107175,#107176,#107177,#107178,#107179)),
 .UNSPECIFIED.,.F.,.F.,.F.)
B_SPLINE_SURFACE_WITH_KNOTS((2,1,2),(3,2,3),(0.709600445987776,1.,1.00289807040992),
(0.383340713919749,0.383933227114986,0.401145492974693),.UNSPECIFIED.)
GEOMETRIC_REPRESENTATION_ITEM()
RATIONAL_B_SPLINE_SURFACE(((0.988246641953811,0.988246641953811,0.988246641953811,
0.986737013496293,0.988139125479962),(0.988246641953811,0.988246641953811,
0.988246641953811,0.986737013496293,0.988139125479962),(0.988246641953811,
0.988246641953811,0.988246641953811,0.986737013496293,0.988139125479962)))
REPRESENTATION_ITEM('')
SURFACE()
);
#802=(
BOUNDED_SURFACE()
B_SPLINE_SURFACE(1,2,((#107188,#107189,#107190),(#107191,#107192,#107193)),
 .UNSPECIFIED.,.F.,.F.,.F.)
B_SPLINE_SURFACE_WITH_KNOTS((2,2),(3,3),(0.710318915640073,1.),(0.331965345783649,
0.349369696259361),.UNSPECIFIED.)
GEOMETRIC_REPRESENTATION_ITEM()
RATIONAL_B_SPLINE_SURFACE(((0.988555124858682,0.99035748704491,0.99513694090229),
(0.988555124858681,0.99035748704491,0.99513694090229)))
REPRESENTATION_ITEM('')
SURFACE()
);
#803=(
BOUNDED_SURFACE()
B_SPLINE_SURFACE(1,2,((#107195,#107196,#107197,#107198,#107199),(#107200,
#107201,#107202,#107203,#107204),(#107205,#107206,#107207,#107208,#107209)),
 .UNSPECIFIED.,.F.,.F.,.F.)
B_SPLINE_SURFACE_WITH_KNOTS((2,1,2),(3,2,3),(0.709600445965168,1.,1.00289807040992),
(0.383340713897137,0.383933227114987,0.401145492974693),.UNSPECIFIED.)
GEOMETRIC_REPRESENTATION_ITEM()
RATIONAL_B_SPLINE_SURFACE(((0.988246641953811,0.988246641953811,0.988246641953811,
0.986737013496293,0.988139125479962),(0.988246641953811,0.988246641953811,
0.988246641953811,0.986737013496293,0.988139125479962),(0.988246641953811,
0.988246641953811,0.988246641953811,0.986737013496293,0.988139125479962)))
REPRESENTATION_ITEM('')
SURFACE()
);
#804=(
BOUNDED_SURFACE()
B_SPLINE_SURFACE(1,2,((#107218,#107219,#107220),(#107221,#107222,#107223)),
 .UNSPECIFIED.,.F.,.F.,.F.)
B_SPLINE_SURFACE_WITH_KNOTS((2,2),(3,3),(0.71031891564008,1.),(0.331965345783649,
0.349369696259361),.UNSPECIFIED.)
GEOMETRIC_REPRESENTATION_ITEM()
RATIONAL_B_SPLINE_SURFACE(((0.988555124858681,0.99035748704491,0.99513694090229),
(0.988555124858681,0.99035748704491,0.99513694090229)))
REPRESENTATION_ITEM('')
SURFACE()
);
#805=(
BOUNDED_SURFACE()
B_SPLINE_SURFACE(1,2,((#107225,#107226,#107227,#107228,#107229),(#107230,
#107231,#107232,#107233,#107234),(#107235,#107236,#107237,#107238,#107239)),
 .UNSPECIFIED.,.F.,.F.,.F.)
B_SPLINE_SURFACE_WITH_KNOTS((2,1,2),(3,2,3),(0.709600445983969,1.,1.00289807040992),
(0.383340713915941,0.383933227114987,0.401145492974693),.UNSPECIFIED.)
GEOMETRIC_REPRESENTATION_ITEM()
RATIONAL_B_SPLINE_SURFACE(((0.988246641953811,0.988246641953811,0.988246641953811,
0.986737013496293,0.988139125479962),(0.988246641953811,0.988246641953811,
0.988246641953811,0.986737013496293,0.988139125479962),(0.988246641953811,
0.988246641953811,0.988246641953811,0.986737013496293,0.988139125479962)))
REPRESENTATION_ITEM('')
SURFACE()
);
#806=(
BOUNDED_SURFACE()
B_SPLINE_SURFACE(1,2,((#107248,#107249,#107250),(#107251,#107252,#107253)),
 .UNSPECIFIED.,.F.,.F.,.F.)
B_SPLINE_SURFACE_WITH_KNOTS((2,2),(3,3),(0.710318915640075,1.),(0.331965345783649,
0.349369696259361),.UNSPECIFIED.)
GEOMETRIC_REPRESENTATION_ITEM()
RATIONAL_B_SPLINE_SURFACE(((0.988555124858682,0.99035748704491,0.99513694090229),
(0.988555124858682,0.99035748704491,0.99513694090229)))
REPRESENTATION_ITEM('')
SURFACE()
);
#807=(
BOUNDED_SURFACE()
B_SPLINE_SURFACE(1,2,((#107255,#107256,#107257,#107258,#107259),(#107260,
#107261,#107262,#107263,#107264),(#107265,#107266,#107267,#107268,#107269)),
 .UNSPECIFIED.,.F.,.F.,.F.)
B_SPLINE_SURFACE_WITH_KNOTS((2,1,2),(3,2,3),(0.70960044599214,1.,1.00289807040992),
(0.383340713924216,0.383933227114986,0.401145492974693),.UNSPECIFIED.)
GEOMETRIC_REPRESENTATION_ITEM()
RATIONAL_B_SPLINE_SURFACE(((0.988246641953811,0.988246641953811,0.988246641953811,
0.986737013496293,0.988139125479961),(0.988246641953811,0.988246641953811,
0.988246641953811,0.986737013496293,0.988139125479961),(0.988246641953811,
0.988246641953811,0.988246641953811,0.986737013496293,0.988139125479961)))
REPRESENTATION_ITEM('')
SURFACE()
);
#808=(
BOUNDED_SURFACE()
B_SPLINE_SURFACE(1,2,((#107278,#107279,#107280),(#107281,#107282,#107283)),
 .UNSPECIFIED.,.F.,.F.,.F.)
B_SPLINE_SURFACE_WITH_KNOTS((2,2),(3,3),(0.710318915639971,1.),(0.331965345783649,
0.349369696259361),.UNSPECIFIED.)
GEOMETRIC_REPRESENTATION_ITEM()
RATIONAL_B_SPLINE_SURFACE(((0.988555124858682,0.99035748704491,0.99513694090229),
(0.988555124858682,0.99035748704491,0.99513694090229)))
REPRESENTATION_ITEM('')
SURFACE()
);
#809=(
BOUNDED_SURFACE()
B_SPLINE_SURFACE(1,2,((#107285,#107286,#107287,#107288,#107289),(#107290,
#107291,#107292,#107293,#107294),(#107295,#107296,#107297,#107298,#107299)),
 .UNSPECIFIED.,.F.,.F.,.F.)
B_SPLINE_SURFACE_WITH_KNOTS((2,1,2),(3,2,3),(0.709600445959392,1.,1.00289807040993),
(0.38334071389278,0.383933227114987,0.401145492974693),.UNSPECIFIED.)
GEOMETRIC_REPRESENTATION_ITEM()
RATIONAL_B_SPLINE_SURFACE(((0.988246641953811,0.988246641953811,0.988246641953811,
0.986737013496293,0.988139125479962),(0.988246641953811,0.988246641953811,
0.988246641953811,0.986737013496293,0.988139125479962),(0.988246641953811,
0.988246641953811,0.988246641953811,0.986737013496293,0.988139125479962)))
REPRESENTATION_ITEM('')
SURFACE()
);
#810=(
BOUNDED_SURFACE()
B_SPLINE_SURFACE(1,2,((#107308,#107309,#107310),(#107311,#107312,#107313)),
 .UNSPECIFIED.,.F.,.F.,.F.)
B_SPLINE_SURFACE_WITH_KNOTS((2,2),(3,3),(0.710318915638668,1.),(0.331965345783647,
0.349369696259361),.UNSPECIFIED.)
GEOMETRIC_REPRESENTATION_ITEM()
RATIONAL_B_SPLINE_SURFACE(((0.988555124858681,0.99035748704491,0.99513694090229),
(0.988555124858681,0.99035748704491,0.99513694090229)))
REPRESENTATION_ITEM('')
SURFACE()
);
#811=(
BOUNDED_SURFACE()
B_SPLINE_SURFACE(1,2,((#107315,#107316,#107317,#107318,#107319),(#107320,
#107321,#107322,#107323,#107324),(#107325,#107326,#107327,#107328,#107329)),
 .UNSPECIFIED.,.F.,.F.,.F.)
B_SPLINE_SURFACE_WITH_KNOTS((2,1,2),(3,2,3),(0.70960044598379,1.,1.00289807040992),
(0.383340713916011,0.383933227114987,0.401145492974693),.UNSPECIFIED.)
GEOMETRIC_REPRESENTATION_ITEM()
RATIONAL_B_SPLINE_SURFACE(((0.988246641953811,0.988246641953811,0.988246641953811,
0.986737013496293,0.988139125479961),(0.988246641953811,0.988246641953811,
0.988246641953811,0.986737013496293,0.988139125479962),(0.988246641953811,
0.988246641953811,0.988246641953811,0.986737013496293,0.988139125479962)))
REPRESENTATION_ITEM('')
SURFACE()
);
#812=(
BOUNDED_SURFACE()
B_SPLINE_SURFACE(1,2,((#107338,#107339,#107340),(#107341,#107342,#107343)),
 .UNSPECIFIED.,.F.,.F.,.F.)
B_SPLINE_SURFACE_WITH_KNOTS((2,2),(3,3),(0.710318915639827,1.),(0.331965345783647,
0.349369696259361),.UNSPECIFIED.)
GEOMETRIC_REPRESENTATION_ITEM()
RATIONAL_B_SPLINE_SURFACE(((0.988555124858681,0.99035748704491,0.99513694090229),
(0.988555124858681,0.99035748704491,0.99513694090229)))
REPRESENTATION_ITEM('')
SURFACE()
);
#813=(
BOUNDED_SURFACE()
B_SPLINE_SURFACE(1,2,((#107345,#107346,#107347,#107348,#107349),(#107350,
#107351,#107352,#107353,#107354),(#107355,#107356,#107357,#107358,#107359)),
 .UNSPECIFIED.,.F.,.F.,.F.)
B_SPLINE_SURFACE_WITH_KNOTS((2,1,2),(3,2,3),(0.709600445981835,1.,1.00289807040992),
(0.383340713913804,0.383933227114986,0.401145492974693),.UNSPECIFIED.)
GEOMETRIC_REPRESENTATION_ITEM()
RATIONAL_B_SPLINE_SURFACE(((0.988246641953811,0.988246641953811,0.988246641953811,
0.986737013496293,0.988139125479961),(0.988246641953811,0.988246641953811,
0.988246641953811,0.986737013496293,0.988139125479961),(0.988246641953811,
0.988246641953811,0.988246641953811,0.986737013496293,0.988139125479961)))
REPRESENTATION_ITEM('')
SURFACE()
);
#814=(
BOUNDED_SURFACE()
B_SPLINE_SURFACE(1,2,((#107368,#107369,#107370),(#107371,#107372,#107373)),
 .UNSPECIFIED.,.F.,.F.,.F.)
B_SPLINE_SURFACE_WITH_KNOTS((2,2),(3,3),(0.710318915640078,1.),(0.331965345783649,
0.349369696259361),.UNSPECIFIED.)
GEOMETRIC_REPRESENTATION_ITEM()
RATIONAL_B_SPLINE_SURFACE(((0.988555124858682,0.99035748704491,0.99513694090229),
(0.988555124858681,0.99035748704491,0.99513694090229)))
REPRESENTATION_ITEM('')
SURFACE()
);
#815=(
BOUNDED_SURFACE()
B_SPLINE_SURFACE(1,2,((#107375,#107376,#107377,#107378,#107379),(#107380,
#107381,#107382,#107383,#107384),(#107385,#107386,#107387,#107388,#107389)),
 .UNSPECIFIED.,.F.,.F.,.F.)
B_SPLINE_SURFACE_WITH_KNOTS((2,1,2),(3,2,3),(0.70960044599244,1.,1.00289807040992),
(0.383340713924407,0.383933227114987,0.401145492974693),.UNSPECIFIED.)
GEOMETRIC_REPRESENTATION_ITEM()
RATIONAL_B_SPLINE_SURFACE(((0.988246641953811,0.988246641953811,0.988246641953811,
0.986737013496293,0.988139125479962),(0.988246641953811,0.988246641953811,
0.988246641953811,0.986737013496293,0.988139125479962),(0.988246641953811,
0.988246641953811,0.988246641953811,0.986737013496293,0.988139125479962)))
REPRESENTATION_ITEM('')
SURFACE()
);
#816=(
BOUNDED_SURFACE()
B_SPLINE_SURFACE(1,2,((#107398,#107399,#107400),(#107401,#107402,#107403)),
 .UNSPECIFIED.,.F.,.F.,.F.)
B_SPLINE_SURFACE_WITH_KNOTS((2,2),(3,3),(0.71031891564008,1.),(0.331965345783647,
0.349369696259361),.UNSPECIFIED.)
GEOMETRIC_REPRESENTATION_ITEM()
RATIONAL_B_SPLINE_SURFACE(((0.988555124858681,0.99035748704491,0.99513694090229),
(0.988555124858681,0.99035748704491,0.99513694090229)))
REPRESENTATION_ITEM('')
SURFACE()
);
#817=(
BOUNDED_SURFACE()
B_SPLINE_SURFACE(1,2,((#107405,#107406,#107407,#107408,#107409),(#107410,
#107411,#107412,#107413,#107414),(#107415,#107416,#107417,#107418,#107419)),
 .UNSPECIFIED.,.F.,.F.,.F.)
B_SPLINE_SURFACE_WITH_KNOTS((2,1,2),(3,2,3),(0.709600445973141,1.,1.00289807040992),
(0.383340713905106,0.383933227114987,0.401145492974693),.UNSPECIFIED.)
GEOMETRIC_REPRESENTATION_ITEM()
RATIONAL_B_SPLINE_SURFACE(((0.988246641953811,0.988246641953811,0.988246641953811,
0.986737013496293,0.988139125479961),(0.988246641953811,0.988246641953811,
0.988246641953811,0.986737013496293,0.988139125479961),(0.988246641953811,
0.988246641953811,0.988246641953811,0.986737013496293,0.988139125479961)))
REPRESENTATION_ITEM('')
SURFACE()
);
#818=(
BOUNDED_SURFACE()
B_SPLINE_SURFACE(1,2,((#107428,#107429,#107430),(#107431,#107432,#107433)),
 .UNSPECIFIED.,.F.,.F.,.F.)
B_SPLINE_SURFACE_WITH_KNOTS((2,2),(3,3),(0.710318915640081,1.),(0.331965345783647,
0.349369696259361),.UNSPECIFIED.)
GEOMETRIC_REPRESENTATION_ITEM()
RATIONAL_B_SPLINE_SURFACE(((0.988555124858681,0.99035748704491,0.99513694090229),
(0.988555124858681,0.99035748704491,0.99513694090229)))
REPRESENTATION_ITEM('')
SURFACE()
);
#819=(
BOUNDED_SURFACE()
B_SPLINE_SURFACE(1,2,((#107435,#107436,#107437,#107438,#107439),(#107440,
#107441,#107442,#107443,#107444),(#107445,#107446,#107447,#107448,#107449)),
 .UNSPECIFIED.,.F.,.F.,.F.)
B_SPLINE_SURFACE_WITH_KNOTS((2,1,2),(3,2,3),(0.709600445966216,1.,1.00289807040992),
(0.383340713898184,0.383933227114987,0.401145492974693),.UNSPECIFIED.)
GEOMETRIC_REPRESENTATION_ITEM()
RATIONAL_B_SPLINE_SURFACE(((0.988246641953811,0.988246641953811,0.988246641953811,
0.986737013496293,0.988139125479962),(0.988246641953811,0.988246641953811,
0.988246641953811,0.986737013496293,0.988139125479962),(0.988246641953811,
0.988246641953811,0.988246641953811,0.986737013496293,0.988139125479962)))
REPRESENTATION_ITEM('')
SURFACE()
);
#820=(
BOUNDED_SURFACE()
B_SPLINE_SURFACE(1,2,((#107458,#107459,#107460),(#107461,#107462,#107463)),
 .UNSPECIFIED.,.F.,.F.,.F.)
B_SPLINE_SURFACE_WITH_KNOTS((2,2),(3,3),(0.710318915640083,1.),(0.331965345783647,
0.349369696259361),.UNSPECIFIED.)
GEOMETRIC_REPRESENTATION_ITEM()
RATIONAL_B_SPLINE_SURFACE(((0.988555124858681,0.99035748704491,0.99513694090229),
(0.988555124858681,0.99035748704491,0.99513694090229)))
REPRESENTATION_ITEM('')
SURFACE()
);
#821=(
BOUNDED_SURFACE()
B_SPLINE_SURFACE(1,2,((#107465,#107466,#107467,#107468,#107469),(#107470,
#107471,#107472,#107473,#107474),(#107475,#107476,#107477,#107478,#107479)),
 .UNSPECIFIED.,.F.,.F.,.F.)
B_SPLINE_SURFACE_WITH_KNOTS((2,1,2),(3,2,3),(0.70960044597391,1.,1.00289807040992),
(0.383340713905879,0.383933227114987,0.401145492974693),.UNSPECIFIED.)
GEOMETRIC_REPRESENTATION_ITEM()
RATIONAL_B_SPLINE_SURFACE(((0.988246641953811,0.988246641953811,0.988246641953811,
0.986737013496293,0.988139125479962),(0.988246641953811,0.988246641953811,
0.988246641953811,0.986737013496293,0.988139125479962),(0.988246641953811,
0.988246641953811,0.988246641953811,0.986737013496293,0.988139125479962)))
REPRESENTATION_ITEM('')
SURFACE()
);
#822=(
BOUNDED_SURFACE()
B_SPLINE_SURFACE(1,2,((#107488,#107489,#107490),(#107491,#107492,#107493)),
 .UNSPECIFIED.,.F.,.F.,.F.)
B_SPLINE_SURFACE_WITH_KNOTS((2,2),(3,3),(0.710318915640079,1.),(0.331965345783649,
0.349369696259361),.UNSPECIFIED.)
GEOMETRIC_REPRESENTATION_ITEM()
RATIONAL_B_SPLINE_SURFACE(((0.988555124858681,0.99035748704491,0.99513694090229),
(0.988555124858681,0.99035748704491,0.99513694090229)))
REPRESENTATION_ITEM('')
SURFACE()
);
#823=(
BOUNDED_SURFACE()
B_SPLINE_SURFACE(1,2,((#107495,#107496,#107497,#107498,#107499),(#107500,
#107501,#107502,#107503,#107504),(#107505,#107506,#107507,#107508,#107509)),
 .UNSPECIFIED.,.F.,.F.,.F.)
B_SPLINE_SURFACE_WITH_KNOTS((2,1,2),(3,2,3),(0.709600445962162,1.,1.00289807040992),
(0.383340713894442,0.383933227114983,0.401145492974692),.UNSPECIFIED.)
GEOMETRIC_REPRESENTATION_ITEM()
RATIONAL_B_SPLINE_SURFACE(((0.988246641953811,0.988246641953811,0.988246641953811,
0.986737013496293,0.988139125479961),(0.988246641953811,0.988246641953811,
0.988246641953811,0.986737013496293,0.988139125479961),(0.988246641953811,
0.988246641953811,0.988246641953811,0.986737013496293,0.988139125479961)))
REPRESENTATION_ITEM('')
SURFACE()
);
#824=(
BOUNDED_SURFACE()
B_SPLINE_SURFACE(1,2,((#107518,#107519,#107520),(#107521,#107522,#107523)),
 .UNSPECIFIED.,.F.,.F.,.F.)
B_SPLINE_SURFACE_WITH_KNOTS((2,2),(3,3),(0.710318915639765,1.),(0.331965345783648,
0.349369696259362),.UNSPECIFIED.)
GEOMETRIC_REPRESENTATION_ITEM()
RATIONAL_B_SPLINE_SURFACE(((0.988555124858681,0.99035748704491,0.99513694090229),
(0.988555124858681,0.99035748704491,0.995136940902291)))
REPRESENTATION_ITEM('')
SURFACE()
);
#825=(
BOUNDED_SURFACE()
B_SPLINE_SURFACE(1,2,((#107525,#107526,#107527,#107528,#107529),(#107530,
#107531,#107532,#107533,#107534),(#107535,#107536,#107537,#107538,#107539)),
 .UNSPECIFIED.,.F.,.F.,.F.)
B_SPLINE_SURFACE_WITH_KNOTS((2,1,2),(3,2,3),(0.709600445962641,1.,1.00289807040992),
(0.383340713894891,0.383933227114985,0.401145492974692),.UNSPECIFIED.)
GEOMETRIC_REPRESENTATION_ITEM()
RATIONAL_B_SPLINE_SURFACE(((0.988246641953811,0.988246641953811,0.988246641953811,
0.986737013496293,0.988139125479961),(0.988246641953811,0.988246641953811,
0.988246641953811,0.986737013496293,0.988139125479961),(0.988246641953811,
0.988246641953811,0.988246641953811,0.986737013496293,0.988139125479961)))
REPRESENTATION_ITEM('')
SURFACE()
);
#826=(
BOUNDED_SURFACE()
B_SPLINE_SURFACE(1,2,((#107548,#107549,#107550),(#107551,#107552,#107553)),
 .UNSPECIFIED.,.F.,.F.,.F.)
B_SPLINE_SURFACE_WITH_KNOTS((2,2),(3,3),(0.7103189156398,1.),(0.331965345783649,
0.349369696259361),.UNSPECIFIED.)
GEOMETRIC_REPRESENTATION_ITEM()
RATIONAL_B_SPLINE_SURFACE(((0.988555124858681,0.99035748704491,0.99513694090229),
(0.988555124858682,0.990357487044911,0.99513694090229)))
REPRESENTATION_ITEM('')
SURFACE()
);
#827=(
BOUNDED_SURFACE()
B_SPLINE_SURFACE(1,2,((#107555,#107556,#107557,#107558,#107559),(#107560,
#107561,#107562,#107563,#107564),(#107565,#107566,#107567,#107568,#107569)),
 .UNSPECIFIED.,.F.,.F.,.F.)
B_SPLINE_SURFACE_WITH_KNOTS((2,1,2),(3,2,3),(0.709600445972273,1.,1.00289807040992),
(0.383340713904703,0.383933227114987,0.401145492974693),.UNSPECIFIED.)
GEOMETRIC_REPRESENTATION_ITEM()
RATIONAL_B_SPLINE_SURFACE(((0.988246641953811,0.988246641953811,0.988246641953811,
0.986737013496293,0.988139125479962),(0.988246641953811,0.988246641953811,
0.988246641953811,0.986737013496293,0.988139125479962),(0.988246641953811,
0.988246641953811,0.988246641953811,0.986737013496293,0.988139125479962)))
REPRESENTATION_ITEM('')
SURFACE()
);
#828=(
BOUNDED_SURFACE()
B_SPLINE_SURFACE(1,2,((#107578,#107579,#107580),(#107581,#107582,#107583)),
 .UNSPECIFIED.,.F.,.F.,.F.)
B_SPLINE_SURFACE_WITH_KNOTS((2,2),(3,3),(0.710318915639619,1.),(0.331965345783649,
0.349369696259361),.UNSPECIFIED.)
GEOMETRIC_REPRESENTATION_ITEM()
RATIONAL_B_SPLINE_SURFACE(((0.988555124858681,0.99035748704491,0.99513694090229),
(0.988555124858681,0.99035748704491,0.99513694090229)))
REPRESENTATION_ITEM('')
SURFACE()
);
#829=(
BOUNDED_SURFACE()
B_SPLINE_SURFACE(1,2,((#107585,#107586,#107587,#107588,#107589),(#107590,
#107591,#107592,#107593,#107594),(#107595,#107596,#107597,#107598,#107599)),
 .UNSPECIFIED.,.F.,.F.,.F.)
B_SPLINE_SURFACE_WITH_KNOTS((2,1,2),(3,2,3),(0.709600445979013,1.,1.00289807040992),
(0.383340713911408,0.383933227114987,0.401145492974693),.UNSPECIFIED.)
GEOMETRIC_REPRESENTATION_ITEM()
RATIONAL_B_SPLINE_SURFACE(((0.988246641953811,0.988246641953811,0.988246641953811,
0.986737013496293,0.988139125479962),(0.988246641953811,0.988246641953811,
0.988246641953811,0.986737013496293,0.988139125479962),(0.988246641953811,
0.988246641953811,0.988246641953811,0.986737013496293,0.988139125479962)))
REPRESENTATION_ITEM('')
SURFACE()
);
#830=(
BOUNDED_SURFACE()
B_SPLINE_SURFACE(1,2,((#107608,#107609,#107610),(#107611,#107612,#107613)),
 .UNSPECIFIED.,.F.,.F.,.F.)
B_SPLINE_SURFACE_WITH_KNOTS((2,2),(3,3),(0.71031891563966,1.),(0.331965345783649,
0.349369696259361),.UNSPECIFIED.)
GEOMETRIC_REPRESENTATION_ITEM()
RATIONAL_B_SPLINE_SURFACE(((0.988555124858681,0.99035748704491,0.99513694090229),
(0.988555124858681,0.99035748704491,0.99513694090229)))
REPRESENTATION_ITEM('')
SURFACE()
);
#831=(
BOUNDED_SURFACE()
B_SPLINE_SURFACE(1,2,((#107615,#107616,#107617,#107618,#107619),(#107620,
#107621,#107622,#107623,#107624),(#107625,#107626,#107627,#107628,#107629)),
 .UNSPECIFIED.,.F.,.F.,.F.)
B_SPLINE_SURFACE_WITH_KNOTS((2,1,2),(3,2,3),(0.709600445963461,1.,1.00289807040992),
(0.383340713895831,0.383933227114987,0.401145492974693),.UNSPECIFIED.)
GEOMETRIC_REPRESENTATION_ITEM()
RATIONAL_B_SPLINE_SURFACE(((0.988246641953811,0.988246641953811,0.988246641953811,
0.986737013496293,0.988139125479962),(0.988246641953811,0.988246641953811,
0.988246641953811,0.986737013496293,0.988139125479962),(0.988246641953811,
0.988246641953811,0.988246641953811,0.986737013496293,0.988139125479962)))
REPRESENTATION_ITEM('')
SURFACE()
);
#832=(
BOUNDED_SURFACE()
B_SPLINE_SURFACE(1,2,((#107631,#107632,#107633),(#107634,#107635,#107636)),
 .UNSPECIFIED.,.F.,.F.,.F.)
B_SPLINE_SURFACE_WITH_KNOTS((2,2),(3,3),(0.,0.289807040992854),(0.435775021682558,
0.453027768259469),.UNSPECIFIED.)
GEOMETRIC_REPRESENTATION_ITEM()
RATIONAL_B_SPLINE_SURFACE(((0.995452950231099,0.990618550266721,0.988709602819327),
(0.995452950231099,0.990618550266721,0.988709602819327)))
REPRESENTATION_ITEM('')
SURFACE()
);
#833=(
BOUNDED_SURFACE()
B_SPLINE_SURFACE(1,2,((#107645,#107646,#107647,#107648,#107649),(#107650,
#107651,#107652,#107653,#107654)),.UNSPECIFIED.,.F.,.F.,.F.)
B_SPLINE_SURFACE_WITH_KNOTS((2,2),(3,2,3),(0.,0.289681084360052),(0.280328542633766,
0.285714285714286,0.297856505190614),.UNSPECIFIED.)
GEOMETRIC_REPRESENTATION_ITEM()
RATIONAL_B_SPLINE_SURFACE(((0.996504189652447,0.998109554471267,1.,0.995737968897747,
0.992924952273132),(0.996504189652447,0.998109554471267,1.,0.995737968897747,
0.992924952273132)))
REPRESENTATION_ITEM('')
SURFACE()
);
#834=(
BOUNDED_SURFACE()
B_SPLINE_SURFACE(1,2,((#107672,#107673,#107674),(#107675,#107676,#107677)),
 .UNSPECIFIED.,.F.,.F.,.F.)
B_SPLINE_SURFACE_WITH_KNOTS((2,2),(3,3),(0.,0.289807040991561),(0.435775021682621,
0.453027768259468),.UNSPECIFIED.)
GEOMETRIC_REPRESENTATION_ITEM()
RATIONAL_B_SPLINE_SURFACE(((0.995452950231064,0.990618550266715,0.988709602819327),
(0.995452950231064,0.990618550266715,0.988709602819327)))
REPRESENTATION_ITEM('')
SURFACE()
);
#835=(
BOUNDED_SURFACE()
B_SPLINE_SURFACE(1,2,((#107679,#107680,#107681,#107682,#107683),(#107684,
#107685,#107686,#107687,#107688)),.UNSPECIFIED.,.F.,.F.,.F.)
B_SPLINE_SURFACE_WITH_KNOTS((2,2),(3,2,3),(0.,0.289681084359918),(0.280328542633766,
0.285714285714286,0.297856505190615),.UNSPECIFIED.)
GEOMETRIC_REPRESENTATION_ITEM()
RATIONAL_B_SPLINE_SURFACE(((0.996504189652447,0.998109554471267,1.,0.995737968897747,
0.992924952273131),(0.996504189652447,0.998109554471267,1.,0.995737968897747,
0.992924952273131)))
REPRESENTATION_ITEM('')
SURFACE()
);
#836=(
BOUNDED_SURFACE()
B_SPLINE_SURFACE(1,2,((#107706,#107707,#107708),(#107709,#107710,#107711)),
 .UNSPECIFIED.,.F.,.F.,.F.)
B_SPLINE_SURFACE_WITH_KNOTS((2,2),(3,3),(0.,0.289807040991557),(0.435775021682621,
0.453027768259468),.UNSPECIFIED.)
GEOMETRIC_REPRESENTATION_ITEM()
RATIONAL_B_SPLINE_SURFACE(((0.995452950231064,0.990618550266715,0.988709602819327),
(0.995452950231064,0.990618550266715,0.988709602819327)))
REPRESENTATION_ITEM('')
SURFACE()
);
#837=(
BOUNDED_SURFACE()
B_SPLINE_SURFACE(1,2,((#107713,#107714,#107715,#107716,#107717),(#107718,
#107719,#107720,#107721,#107722)),.UNSPECIFIED.,.F.,.F.,.F.)
B_SPLINE_SURFACE_WITH_KNOTS((2,2),(3,2,3),(0.,0.289681084360338),(0.280328542633766,
0.285714285714286,0.297856505190615),.UNSPECIFIED.)
GEOMETRIC_REPRESENTATION_ITEM()
RATIONAL_B_SPLINE_SURFACE(((0.996504189652447,0.998109554471267,1.,0.995737968897747,
0.992924952273132),(0.996504189652447,0.998109554471267,1.,0.995737968897747,
0.992924952273132)))
REPRESENTATION_ITEM('')
SURFACE()
);
#838=(
BOUNDED_SURFACE()
B_SPLINE_SURFACE(1,2,((#107740,#107741,#107742),(#107743,#107744,#107745)),
 .UNSPECIFIED.,.F.,.F.,.F.)
B_SPLINE_SURFACE_WITH_KNOTS((2,2),(3,3),(0.,0.28980704099156),(0.435775021682621,
0.453027768259468),.UNSPECIFIED.)
GEOMETRIC_REPRESENTATION_ITEM()
RATIONAL_B_SPLINE_SURFACE(((0.995452950231064,0.990618550266715,0.988709602819327),
(0.995452950231064,0.990618550266715,0.988709602819327)))
REPRESENTATION_ITEM('')
SURFACE()
);
#839=(
BOUNDED_SURFACE()
B_SPLINE_SURFACE(1,2,((#107747,#107748,#107749,#107750,#107751),(#107752,
#107753,#107754,#107755,#107756)),.UNSPECIFIED.,.F.,.F.,.F.)
B_SPLINE_SURFACE_WITH_KNOTS((2,2),(3,2,3),(0.,0.289681084359927),(0.280328542633766,
0.285714285714286,0.297856505190615),.UNSPECIFIED.)
GEOMETRIC_REPRESENTATION_ITEM()
RATIONAL_B_SPLINE_SURFACE(((0.996504189652447,0.998109554471267,1.,0.995737968897747,
0.992924952273131),(0.996504189652447,0.998109554471267,1.,0.995737968897747,
0.992924952273131)))
REPRESENTATION_ITEM('')
SURFACE()
);
#840=(
BOUNDED_SURFACE()
B_SPLINE_SURFACE(1,2,((#107774,#107775,#107776),(#107777,#107778,#107779)),
 .UNSPECIFIED.,.F.,.F.,.F.)
B_SPLINE_SURFACE_WITH_KNOTS((2,2),(3,3),(0.,0.289807040991564),(0.435775021682621,
0.453027768259468),.UNSPECIFIED.)
GEOMETRIC_REPRESENTATION_ITEM()
RATIONAL_B_SPLINE_SURFACE(((0.995452950231064,0.990618550266715,0.988709602819327),
(0.995452950231064,0.990618550266715,0.988709602819327)))
REPRESENTATION_ITEM('')
SURFACE()
);
#841=(
BOUNDED_SURFACE()
B_SPLINE_SURFACE(1,2,((#107781,#107782,#107783,#107784,#107785),(#107786,
#107787,#107788,#107789,#107790)),.UNSPECIFIED.,.F.,.F.,.F.)
B_SPLINE_SURFACE_WITH_KNOTS((2,2),(3,2,3),(0.,0.289681084359916),(0.280328542633766,
0.285714285714286,0.297856505190615),.UNSPECIFIED.)
GEOMETRIC_REPRESENTATION_ITEM()
RATIONAL_B_SPLINE_SURFACE(((0.996504189652447,0.998109554471267,1.,0.995737968897747,
0.992924952273131),(0.996504189652447,0.998109554471267,1.,0.995737968897747,
0.992924952273131)))
REPRESENTATION_ITEM('')
SURFACE()
);
#842=(
BOUNDED_SURFACE()
B_SPLINE_SURFACE(1,2,((#107808,#107809,#107810),(#107811,#107812,#107813)),
 .UNSPECIFIED.,.F.,.F.,.F.)
B_SPLINE_SURFACE_WITH_KNOTS((2,2),(3,3),(0.,0.289807040991642),(0.435775021682622,
0.453027768259468),.UNSPECIFIED.)
GEOMETRIC_REPRESENTATION_ITEM()
RATIONAL_B_SPLINE_SURFACE(((0.995452950231063,0.990618550266715,0.988709602819327),
(0.995452950231063,0.990618550266715,0.988709602819327)))
REPRESENTATION_ITEM('')
SURFACE()
);
#843=(
BOUNDED_SURFACE()
B_SPLINE_SURFACE(1,2,((#107815,#107816,#107817,#107818,#107819),(#107820,
#107821,#107822,#107823,#107824)),.UNSPECIFIED.,.F.,.F.,.F.)
B_SPLINE_SURFACE_WITH_KNOTS((2,2),(3,2,3),(0.,0.28968108436033),(0.280328542633765,
0.285714285714286,0.297856505190614),.UNSPECIFIED.)
GEOMETRIC_REPRESENTATION_ITEM()
RATIONAL_B_SPLINE_SURFACE(((0.996504189652447,0.998109554471267,1.,0.995737968897747,
0.992924952273132),(0.996504189652447,0.998109554471267,1.,0.995737968897747,
0.992924952273132)))
REPRESENTATION_ITEM('')
SURFACE()
);
#844=(
BOUNDED_SURFACE()
B_SPLINE_SURFACE(1,2,((#107842,#107843,#107844),(#107845,#107846,#107847)),
 .UNSPECIFIED.,.F.,.F.,.F.)
B_SPLINE_SURFACE_WITH_KNOTS((2,2),(3,3),(0.,0.289807040991638),(0.435775021682622,
0.453027768259469),.UNSPECIFIED.)
GEOMETRIC_REPRESENTATION_ITEM()
RATIONAL_B_SPLINE_SURFACE(((0.995452950231063,0.990618550266714,0.988709602819327),
(0.995452950231063,0.990618550266714,0.988709602819327)))
REPRESENTATION_ITEM('')
SURFACE()
);
#845=(
BOUNDED_SURFACE()
B_SPLINE_SURFACE(1,2,((#107849,#107850,#107851,#107852,#107853),(#107854,
#107855,#107856,#107857,#107858)),.UNSPECIFIED.,.F.,.F.,.F.)
B_SPLINE_SURFACE_WITH_KNOTS((2,2),(3,2,3),(0.,0.289681084359919),(0.280328542633765,
0.285714285714286,0.297856505190614),.UNSPECIFIED.)
GEOMETRIC_REPRESENTATION_ITEM()
RATIONAL_B_SPLINE_SURFACE(((0.996504189652447,0.998109554471267,1.,0.995737968897747,
0.992924952273132),(0.996504189652447,0.998109554471267,1.,0.995737968897747,
0.992924952273132)))
REPRESENTATION_ITEM('')
SURFACE()
);
#846=(
BOUNDED_SURFACE()
B_SPLINE_SURFACE(1,2,((#107876,#107877,#107878),(#107879,#107880,#107881)),
 .UNSPECIFIED.,.F.,.F.,.F.)
B_SPLINE_SURFACE_WITH_KNOTS((2,2),(3,3),(0.,0.28980704099164),(0.435775021682622,
0.453027768259469),.UNSPECIFIED.)
GEOMETRIC_REPRESENTATION_ITEM()
RATIONAL_B_SPLINE_SURFACE(((0.995452950231063,0.990618550266714,0.988709602819327),
(0.995452950231063,0.990618550266714,0.988709602819327)))
REPRESENTATION_ITEM('')
SURFACE()
);
#847=(
BOUNDED_SURFACE()
B_SPLINE_SURFACE(1,2,((#107883,#107884,#107885,#107886,#107887),(#107888,
#107889,#107890,#107891,#107892)),.UNSPECIFIED.,.F.,.F.,.F.)
B_SPLINE_SURFACE_WITH_KNOTS((2,2),(3,2,3),(0.,0.289681084359922),(0.280328542633765,
0.285714285714286,0.297856505190614),.UNSPECIFIED.)
GEOMETRIC_REPRESENTATION_ITEM()
RATIONAL_B_SPLINE_SURFACE(((0.996504189652447,0.998109554471267,1.,0.995737968897747,
0.992924952273132),(0.996504189652447,0.998109554471267,1.,0.995737968897747,
0.992924952273132)))
REPRESENTATION_ITEM('')
SURFACE()
);
#848=(
BOUNDED_SURFACE()
B_SPLINE_SURFACE(1,2,((#107910,#107911,#107912),(#107913,#107914,#107915)),
 .UNSPECIFIED.,.F.,.F.,.F.)
B_SPLINE_SURFACE_WITH_KNOTS((2,2),(3,3),(0.,0.289807040991643),(0.435775021682622,
0.453027768259469),.UNSPECIFIED.)
GEOMETRIC_REPRESENTATION_ITEM()
RATIONAL_B_SPLINE_SURFACE(((0.995452950231063,0.990618550266714,0.988709602819327),
(0.995452950231063,0.990618550266714,0.988709602819327)))
REPRESENTATION_ITEM('')
SURFACE()
);
#849=(
BOUNDED_SURFACE()
B_SPLINE_SURFACE(1,2,((#107917,#107918,#107919,#107920,#107921),(#107922,
#107923,#107924,#107925,#107926)),.UNSPECIFIED.,.F.,.F.,.F.)
B_SPLINE_SURFACE_WITH_KNOTS((2,2),(3,2,3),(0.,0.289681084360311),(0.280328542633765,
0.285714285714286,0.297856505190614),.UNSPECIFIED.)
GEOMETRIC_REPRESENTATION_ITEM()
RATIONAL_B_SPLINE_SURFACE(((0.996504189652447,0.998109554471267,1.,0.995737968897747,
0.992924952273132),(0.996504189652447,0.998109554471267,1.,0.995737968897747,
0.992924952273132)))
REPRESENTATION_ITEM('')
SURFACE()
);
#850=(
BOUNDED_SURFACE()
B_SPLINE_SURFACE(1,2,((#107944,#107945,#107946),(#107947,#107948,#107949)),
 .UNSPECIFIED.,.F.,.F.,.F.)
B_SPLINE_SURFACE_WITH_KNOTS((2,2),(3,3),(0.,0.289807040991563),(0.435775021682622,
0.453027768259469),.UNSPECIFIED.)
GEOMETRIC_REPRESENTATION_ITEM()
RATIONAL_B_SPLINE_SURFACE(((0.995452950231063,0.990618550266714,0.988709602819327),
(0.995452950231063,0.990618550266714,0.988709602819327)))
REPRESENTATION_ITEM('')
SURFACE()
);
#851=(
BOUNDED_SURFACE()
B_SPLINE_SURFACE(1,2,((#107951,#107952,#107953,#107954,#107955),(#107956,
#107957,#107958,#107959,#107960)),.UNSPECIFIED.,.F.,.F.,.F.)
B_SPLINE_SURFACE_WITH_KNOTS((2,2),(3,2,3),(0.,0.289681084359919),(0.280328542633765,
0.285714285714286,0.297856505190614),.UNSPECIFIED.)
GEOMETRIC_REPRESENTATION_ITEM()
RATIONAL_B_SPLINE_SURFACE(((0.996504189652447,0.998109554471267,1.,0.995737968897747,
0.992924952273132),(0.996504189652447,0.998109554471267,1.,0.995737968897747,
0.992924952273132)))
REPRESENTATION_ITEM('')
SURFACE()
);
#852=(
BOUNDED_SURFACE()
B_SPLINE_SURFACE(1,2,((#107978,#107979,#107980),(#107981,#107982,#107983)),
 .UNSPECIFIED.,.F.,.F.,.F.)
B_SPLINE_SURFACE_WITH_KNOTS((2,2),(3,3),(0.,0.289807040991651),(0.435775021682622,
0.453027768259469),.UNSPECIFIED.)
GEOMETRIC_REPRESENTATION_ITEM()
RATIONAL_B_SPLINE_SURFACE(((0.995452950231063,0.990618550266714,0.988709602819327),
(0.995452950231063,0.990618550266714,0.988709602819327)))
REPRESENTATION_ITEM('')
SURFACE()
);
#853=(
BOUNDED_SURFACE()
B_SPLINE_SURFACE(1,2,((#107985,#107986,#107987,#107988,#107989),(#107990,
#107991,#107992,#107993,#107994)),.UNSPECIFIED.,.F.,.F.,.F.)
B_SPLINE_SURFACE_WITH_KNOTS((2,2),(3,2,3),(0.,0.289681084359921),(0.280328542633765,
0.285714285714286,0.297856505190614),.UNSPECIFIED.)
GEOMETRIC_REPRESENTATION_ITEM()
RATIONAL_B_SPLINE_SURFACE(((0.996504189652447,0.998109554471267,1.,0.995737968897747,
0.992924952273132),(0.996504189652447,0.998109554471267,1.,0.995737968897747,
0.992924952273132)))
REPRESENTATION_ITEM('')
SURFACE()
);
#854=(
BOUNDED_SURFACE()
B_SPLINE_SURFACE(1,2,((#108012,#108013,#108014),(#108015,#108016,#108017)),
 .UNSPECIFIED.,.F.,.F.,.F.)
B_SPLINE_SURFACE_WITH_KNOTS((2,2),(3,3),(0.,0.28980704099156),(0.435775021682622,
0.453027768259469),.UNSPECIFIED.)
GEOMETRIC_REPRESENTATION_ITEM()
RATIONAL_B_SPLINE_SURFACE(((0.995452950231063,0.990618550266714,0.988709602819327),
(0.995452950231063,0.990618550266714,0.988709602819327)))
REPRESENTATION_ITEM('')
SURFACE()
);
#855=(
BOUNDED_SURFACE()
B_SPLINE_SURFACE(1,2,((#108019,#108020,#108021,#108022,#108023),(#108024,
#108025,#108026,#108027,#108028)),.UNSPECIFIED.,.F.,.F.,.F.)
B_SPLINE_SURFACE_WITH_KNOTS((2,2),(3,2,3),(0.,0.289681084360324),(0.280328542633765,
0.285714285714286,0.297856505190614),.UNSPECIFIED.)
GEOMETRIC_REPRESENTATION_ITEM()
RATIONAL_B_SPLINE_SURFACE(((0.996504189652447,0.998109554471267,1.,0.995737968897747,
0.992924952273132),(0.996504189652447,0.998109554471267,1.,0.995737968897747,
0.992924952273132)))
REPRESENTATION_ITEM('')
SURFACE()
);
#856=(
BOUNDED_SURFACE()
B_SPLINE_SURFACE(1,2,((#108046,#108047,#108048),(#108049,#108050,#108051)),
 .UNSPECIFIED.,.F.,.F.,.F.)
B_SPLINE_SURFACE_WITH_KNOTS((2,2),(3,3),(0.,0.289807040991919),(0.435775021682622,
0.453027768259469),.UNSPECIFIED.)
GEOMETRIC_REPRESENTATION_ITEM()
RATIONAL_B_SPLINE_SURFACE(((0.995452950231063,0.990618550266714,0.988709602819327),
(0.995452950231063,0.990618550266714,0.988709602819327)))
REPRESENTATION_ITEM('')
SURFACE()
);
#857=(
BOUNDED_SURFACE()
B_SPLINE_SURFACE(1,2,((#108053,#108054,#108055,#108056,#108057),(#108058,
#108059,#108060,#108061,#108062)),.UNSPECIFIED.,.F.,.F.,.F.)
B_SPLINE_SURFACE_WITH_KNOTS((2,2),(3,2,3),(0.,0.289681084359923),(0.280328542633765,
0.285714285714286,0.297856505190614),.UNSPECIFIED.)
GEOMETRIC_REPRESENTATION_ITEM()
RATIONAL_B_SPLINE_SURFACE(((0.996504189652447,0.998109554471267,1.,0.995737968897747,
0.992924952273132),(0.996504189652447,0.998109554471267,1.,0.995737968897747,
0.992924952273132)))
REPRESENTATION_ITEM('')
SURFACE()
);
#858=(
BOUNDED_SURFACE()
B_SPLINE_SURFACE(1,2,((#108080,#108081,#108082),(#108083,#108084,#108085)),
 .UNSPECIFIED.,.F.,.F.,.F.)
B_SPLINE_SURFACE_WITH_KNOTS((2,2),(3,3),(0.,0.289807040992968),(0.435775021682622,
0.453027768259469),.UNSPECIFIED.)
GEOMETRIC_REPRESENTATION_ITEM()
RATIONAL_B_SPLINE_SURFACE(((0.995452950231063,0.990618550266714,0.988709602819327),
(0.995452950231063,0.990618550266714,0.988709602819327)))
REPRESENTATION_ITEM('')
SURFACE()
);
#859=(
BOUNDED_SURFACE()
B_SPLINE_SURFACE(1,2,((#108087,#108088,#108089,#108090,#108091),(#108092,
#108093,#108094,#108095,#108096)),.UNSPECIFIED.,.F.,.F.,.F.)
B_SPLINE_SURFACE_WITH_KNOTS((2,2),(3,2,3),(0.,0.289681084359921),(0.280328542633765,
0.285714285714286,0.297856505190614),.UNSPECIFIED.)
GEOMETRIC_REPRESENTATION_ITEM()
RATIONAL_B_SPLINE_SURFACE(((0.996504189652447,0.998109554471267,1.,0.995737968897747,
0.992924952273132),(0.996504189652447,0.998109554471267,1.,0.995737968897747,
0.992924952273132)))
REPRESENTATION_ITEM('')
SURFACE()
);
#860=(
BOUNDED_SURFACE()
B_SPLINE_SURFACE(1,2,((#108114,#108115,#108116),(#108117,#108118,#108119)),
 .UNSPECIFIED.,.F.,.F.,.F.)
B_SPLINE_SURFACE_WITH_KNOTS((2,2),(3,3),(0.,0.289807040991685),(0.435775021682461,
0.45302776825947),.UNSPECIFIED.)
GEOMETRIC_REPRESENTATION_ITEM()
RATIONAL_B_SPLINE_SURFACE(((0.995452950231154,0.990618550266732,0.988709602819327),
(0.995452950231154,0.990618550266732,0.988709602819327)))
REPRESENTATION_ITEM('')
SURFACE()
);
#861=(
BOUNDED_SURFACE()
B_SPLINE_SURFACE(1,2,((#108121,#108122,#108123,#108124,#108125),(#108126,
#108127,#108128,#108129,#108130)),.UNSPECIFIED.,.F.,.F.,.F.)
B_SPLINE_SURFACE_WITH_KNOTS((2,2),(3,2,3),(0.,0.289681084359926),(0.280328542633765,
0.285714285714286,0.297856505190614),.UNSPECIFIED.)
GEOMETRIC_REPRESENTATION_ITEM()
RATIONAL_B_SPLINE_SURFACE(((0.996504189652447,0.998109554471267,1.,0.995737968897747,
0.992924952273132),(0.996504189652447,0.998109554471267,1.,0.995737968897747,
0.992924952273132)))
REPRESENTATION_ITEM('')
SURFACE()
);
#862=(
BOUNDED_SURFACE()
B_SPLINE_SURFACE(1,2,((#108148,#108149,#108150),(#108151,#108152,#108153)),
 .UNSPECIFIED.,.F.,.F.,.F.)
B_SPLINE_SURFACE_WITH_KNOTS((2,2),(3,3),(0.,0.289807040991565),(0.435775021682622,
0.453027768259469),.UNSPECIFIED.)
GEOMETRIC_REPRESENTATION_ITEM()
RATIONAL_B_SPLINE_SURFACE(((0.995452950231063,0.990618550266714,0.988709602819327),
(0.995452950231063,0.990618550266714,0.988709602819327)))
REPRESENTATION_ITEM('')
SURFACE()
);
#863=(
BOUNDED_SURFACE()
B_SPLINE_SURFACE(1,2,((#108155,#108156,#108157,#108158,#108159),(#108160,
#108161,#108162,#108163,#108164)),.UNSPECIFIED.,.F.,.F.,.F.)
B_SPLINE_SURFACE_WITH_KNOTS((2,2),(3,2,3),(0.,0.289681084360124),(0.280328542633765,
0.285714285714286,0.297856505190614),.UNSPECIFIED.)
GEOMETRIC_REPRESENTATION_ITEM()
RATIONAL_B_SPLINE_SURFACE(((0.996504189652447,0.998109554471267,1.,0.995737968897747,
0.992924952273132),(0.996504189652447,0.998109554471267,1.,0.995737968897747,
0.992924952273132)))
REPRESENTATION_ITEM('')
SURFACE()
);
#864=(
BOUNDED_SURFACE()
B_SPLINE_SURFACE(1,2,((#108182,#108183,#108184),(#108185,#108186,#108187)),
 .UNSPECIFIED.,.F.,.F.,.F.)
B_SPLINE_SURFACE_WITH_KNOTS((2,2),(3,3),(0.,0.289807040991792),(0.435775021682622,
0.453027768259469),.UNSPECIFIED.)
GEOMETRIC_REPRESENTATION_ITEM()
RATIONAL_B_SPLINE_SURFACE(((0.995452950231063,0.990618550266714,0.988709602819327),
(0.995452950231063,0.990618550266714,0.988709602819327)))
REPRESENTATION_ITEM('')
SURFACE()
);
#865=(
BOUNDED_SURFACE()
B_SPLINE_SURFACE(1,2,((#108189,#108190,#108191,#108192,#108193),(#108194,
#108195,#108196,#108197,#108198)),.UNSPECIFIED.,.F.,.F.,.F.)
B_SPLINE_SURFACE_WITH_KNOTS((2,2),(3,2,3),(0.,0.289681084359926),(0.280328542633765,
0.285714285714286,0.297856505190614),.UNSPECIFIED.)
GEOMETRIC_REPRESENTATION_ITEM()
RATIONAL_B_SPLINE_SURFACE(((0.996504189652447,0.998109554471267,1.,0.995737968897747,
0.992924952273132),(0.996504189652447,0.998109554471267,1.,0.995737968897747,
0.992924952273132)))
REPRESENTATION_ITEM('')
SURFACE()
);
#866=(
BOUNDED_SURFACE()
B_SPLINE_SURFACE(1,2,((#108216,#108217,#108218),(#108219,#108220,#108221)),
 .UNSPECIFIED.,.F.,.F.,.F.)
B_SPLINE_SURFACE_WITH_KNOTS((2,2),(3,3),(0.,0.289807040991559),(0.435775021682622,
0.453027768259469),.UNSPECIFIED.)
GEOMETRIC_REPRESENTATION_ITEM()
RATIONAL_B_SPLINE_SURFACE(((0.995452950231063,0.990618550266714,0.988709602819327),
(0.995452950231063,0.990618550266714,0.988709602819327)))
REPRESENTATION_ITEM('')
SURFACE()
);
#867=(
BOUNDED_SURFACE()
B_SPLINE_SURFACE(1,2,((#108223,#108224,#108225,#108226,#108227),(#108228,
#108229,#108230,#108231,#108232)),.UNSPECIFIED.,.F.,.F.,.F.)
B_SPLINE_SURFACE_WITH_KNOTS((2,2),(3,2,3),(0.,0.289681084359928),(0.280328542633765,
0.285714285714286,0.297856505190614),.UNSPECIFIED.)
GEOMETRIC_REPRESENTATION_ITEM()
RATIONAL_B_SPLINE_SURFACE(((0.996504189652446,0.998109554471267,1.,0.995737968897747,
0.992924952273132),(0.996504189652446,0.998109554471267,1.,0.995737968897747,
0.992924952273132)))
REPRESENTATION_ITEM('')
SURFACE()
);
#868=(
BOUNDED_SURFACE()
B_SPLINE_SURFACE(1,2,((#108250,#108251,#108252),(#108253,#108254,#108255)),
 .UNSPECIFIED.,.F.,.F.,.F.)
B_SPLINE_SURFACE_WITH_KNOTS((2,2),(3,3),(0.,0.289807040992696),(0.435775021682622,
0.453027768259469),.UNSPECIFIED.)
GEOMETRIC_REPRESENTATION_ITEM()
RATIONAL_B_SPLINE_SURFACE(((0.995452950231063,0.990618550266714,0.988709602819327),
(0.995452950231063,0.990618550266714,0.988709602819327)))
REPRESENTATION_ITEM('')
SURFACE()
);
#869=(
BOUNDED_SURFACE()
B_SPLINE_SURFACE(1,2,((#108257,#108258,#108259,#108260,#108261),(#108262,
#108263,#108264,#108265,#108266)),.UNSPECIFIED.,.F.,.F.,.F.)
B_SPLINE_SURFACE_WITH_KNOTS((2,2),(3,2,3),(0.,0.289681084360402),(0.280328542633765,
0.285714285714286,0.297856505190614),.UNSPECIFIED.)
GEOMETRIC_REPRESENTATION_ITEM()
RATIONAL_B_SPLINE_SURFACE(((0.996504189652447,0.998109554471267,1.,0.995737968897747,
0.992924952273132),(0.996504189652447,0.998109554471267,1.,0.995737968897747,
0.992924952273132)))
REPRESENTATION_ITEM('')
SURFACE()
);
#870=(
BOUNDED_SURFACE()
B_SPLINE_SURFACE(1,2,((#108284,#108285,#108286),(#108287,#108288,#108289)),
 .UNSPECIFIED.,.F.,.F.,.F.)
B_SPLINE_SURFACE_WITH_KNOTS((2,2),(3,3),(0.,0.289807040992538),(0.435775021682116,
0.453027768259472),.UNSPECIFIED.)
GEOMETRIC_REPRESENTATION_ITEM()
RATIONAL_B_SPLINE_SURFACE(((0.995452950231347,0.990618550266769,0.988709602819326),
(0.995452950231347,0.990618550266769,0.988709602819326)))
REPRESENTATION_ITEM('')
SURFACE()
);
#871=(
BOUNDED_SURFACE()
B_SPLINE_SURFACE(1,2,((#108291,#108292,#108293,#108294,#108295),(#108296,
#108297,#108298,#108299,#108300)),.UNSPECIFIED.,.F.,.F.,.F.)
B_SPLINE_SURFACE_WITH_KNOTS((2,2),(3,2,3),(0.,0.289681084359924),(0.280328542633765,
0.285714285714286,0.297856505190614),.UNSPECIFIED.)
GEOMETRIC_REPRESENTATION_ITEM()
RATIONAL_B_SPLINE_SURFACE(((0.996504189652447,0.998109554471267,1.,0.995737968897747,
0.992924952273132),(0.996504189652447,0.998109554471267,1.,0.995737968897747,
0.992924952273132)))
REPRESENTATION_ITEM('')
SURFACE()
);
#872=(
BOUNDED_SURFACE()
B_SPLINE_SURFACE(1,2,((#108318,#108319,#108320),(#108321,#108322,#108323)),
 .UNSPECIFIED.,.F.,.F.,.F.)
B_SPLINE_SURFACE_WITH_KNOTS((2,2),(3,3),(0.,0.289807040992669),(0.435775021682251,
0.453027768259471),.UNSPECIFIED.)
GEOMETRIC_REPRESENTATION_ITEM()
RATIONAL_B_SPLINE_SURFACE(((0.995452950231271,0.990618550266755,0.988709602819326),
(0.995452950231271,0.990618550266755,0.988709602819326)))
REPRESENTATION_ITEM('')
SURFACE()
);
#873=(
BOUNDED_SURFACE()
B_SPLINE_SURFACE(1,2,((#108325,#108326,#108327,#108328,#108329),(#108330,
#108331,#108332,#108333,#108334)),.UNSPECIFIED.,.F.,.F.,.F.)
B_SPLINE_SURFACE_WITH_KNOTS((2,2),(3,2,3),(0.,0.289681084360136),(0.280328542633765,
0.285714285714286,0.297856505190614),.UNSPECIFIED.)
GEOMETRIC_REPRESENTATION_ITEM()
RATIONAL_B_SPLINE_SURFACE(((0.996504189652447,0.998109554471267,1.,0.995737968897747,
0.992924952273132),(0.996504189652447,0.998109554471267,1.,0.995737968897747,
0.992924952273132)))
REPRESENTATION_ITEM('')
SURFACE()
);
#874=(
BOUNDED_SURFACE()
B_SPLINE_SURFACE(1,2,((#108352,#108353,#108354),(#108355,#108356,#108357)),
 .UNSPECIFIED.,.F.,.F.,.F.)
B_SPLINE_SURFACE_WITH_KNOTS((2,2),(3,3),(0.,0.289807040991763),(0.435775021682622,
0.453027768259469),.UNSPECIFIED.)
GEOMETRIC_REPRESENTATION_ITEM()
RATIONAL_B_SPLINE_SURFACE(((0.995452950231063,0.990618550266714,0.988709602819327),
(0.995452950231063,0.990618550266714,0.988709602819327)))
REPRESENTATION_ITEM('')
SURFACE()
);
#875=(
BOUNDED_SURFACE()
B_SPLINE_SURFACE(1,2,((#108359,#108360,#108361,#108362,#108363),(#108364,
#108365,#108366,#108367,#108368)),.UNSPECIFIED.,.F.,.F.,.F.)
B_SPLINE_SURFACE_WITH_KNOTS((2,2),(3,2,3),(0.,0.289681084359923),(0.280328542633765,
0.285714285714286,0.297856505190614),.UNSPECIFIED.)
GEOMETRIC_REPRESENTATION_ITEM()
RATIONAL_B_SPLINE_SURFACE(((0.996504189652446,0.998109554471267,1.,0.995737968897747,
0.992924952273132),(0.996504189652446,0.998109554471267,1.,0.995737968897747,
0.992924952273132)))
REPRESENTATION_ITEM('')
SURFACE()
);
#876=(
BOUNDED_SURFACE()
B_SPLINE_SURFACE(1,2,((#108386,#108387,#108388),(#108389,#108390,#108391)),
 .UNSPECIFIED.,.F.,.F.,.F.)
B_SPLINE_SURFACE_WITH_KNOTS((2,2),(3,3),(0.,0.289807040993048),(0.435775021682622,
0.453027768259469),.UNSPECIFIED.)
GEOMETRIC_REPRESENTATION_ITEM()
RATIONAL_B_SPLINE_SURFACE(((0.995452950231063,0.990618550266714,0.988709602819327),
(0.995452950231063,0.990618550266714,0.988709602819327)))
REPRESENTATION_ITEM('')
SURFACE()
);
#877=(
BOUNDED_SURFACE()
B_SPLINE_SURFACE(1,2,((#108393,#108394,#108395,#108396,#108397),(#108398,
#108399,#108400,#108401,#108402)),.UNSPECIFIED.,.F.,.F.,.F.)
B_SPLINE_SURFACE_WITH_KNOTS((2,2),(3,2,3),(0.,0.289681084359929),(0.280328542633765,
0.285714285714286,0.297856505190614),.UNSPECIFIED.)
GEOMETRIC_REPRESENTATION_ITEM()
RATIONAL_B_SPLINE_SURFACE(((0.996504189652446,0.998109554471267,1.,0.995737968897747,
0.992924952273132),(0.996504189652446,0.998109554471267,1.,0.995737968897747,
0.992924952273132)))
REPRESENTATION_ITEM('')
SURFACE()
);
#878=(
BOUNDED_SURFACE()
B_SPLINE_SURFACE(1,2,((#108420,#108421,#108422),(#108423,#108424,#108425)),
 .UNSPECIFIED.,.F.,.F.,.F.)
B_SPLINE_SURFACE_WITH_KNOTS((2,2),(3,3),(0.,0.289807040992795),(0.435775021682622,
0.453027768259469),.UNSPECIFIED.)
GEOMETRIC_REPRESENTATION_ITEM()
RATIONAL_B_SPLINE_SURFACE(((0.995452950231063,0.990618550266714,0.988709602819327),
(0.995452950231063,0.990618550266714,0.988709602819327)))
REPRESENTATION_ITEM('')
SURFACE()
);
#879=(
BOUNDED_SURFACE()
B_SPLINE_SURFACE(1,2,((#108427,#108428,#108429,#108430,#108431),(#108432,
#108433,#108434,#108435,#108436)),.UNSPECIFIED.,.F.,.F.,.F.)
B_SPLINE_SURFACE_WITH_KNOTS((2,2),(3,2,3),(0.,0.289681084360214),(0.280328542633765,
0.285714285714286,0.297856505190614),.UNSPECIFIED.)
GEOMETRIC_REPRESENTATION_ITEM()
RATIONAL_B_SPLINE_SURFACE(((0.996504189652446,0.998109554471267,1.,0.995737968897747,
0.992924952273132),(0.996504189652446,0.998109554471267,1.,0.995737968897747,
0.992924952273132)))
REPRESENTATION_ITEM('')
SURFACE()
);
#880=(
BOUNDED_SURFACE()
B_SPLINE_SURFACE(1,2,((#108454,#108455,#108456),(#108457,#108458,#108459)),
 .UNSPECIFIED.,.F.,.F.,.F.)
B_SPLINE_SURFACE_WITH_KNOTS((2,2),(3,3),(0.,0.289807040992557),(0.435775021682307,
0.453027768259471),.UNSPECIFIED.)
GEOMETRIC_REPRESENTATION_ITEM()
RATIONAL_B_SPLINE_SURFACE(((0.99545295023124,0.990618550266749,0.988709602819327),
(0.99545295023124,0.990618550266749,0.988709602819327)))
REPRESENTATION_ITEM('')
SURFACE()
);
#881=(
BOUNDED_SURFACE()
B_SPLINE_SURFACE(1,2,((#108461,#108462,#108463,#108464,#108465),(#108466,
#108467,#108468,#108469,#108470)),.UNSPECIFIED.,.F.,.F.,.F.)
B_SPLINE_SURFACE_WITH_KNOTS((2,2),(3,2,3),(0.,0.289681084360026),(0.280328542633765,
0.285714285714286,0.297856505190614),.UNSPECIFIED.)
GEOMETRIC_REPRESENTATION_ITEM()
RATIONAL_B_SPLINE_SURFACE(((0.996504189652447,0.998109554471267,1.,0.995737968897747,
0.992924952273132),(0.996504189652447,0.998109554471267,1.,0.995737968897747,
0.992924952273132)))
REPRESENTATION_ITEM('')
SURFACE()
);
#882=(
BOUNDED_SURFACE()
B_SPLINE_SURFACE(1,2,((#108488,#108489,#108490),(#108491,#108492,#108493)),
 .UNSPECIFIED.,.F.,.F.,.F.)
B_SPLINE_SURFACE_WITH_KNOTS((2,2),(3,3),(0.,0.289807040992487),(0.435775021682621,
0.453027768259469),.UNSPECIFIED.)
GEOMETRIC_REPRESENTATION_ITEM()
RATIONAL_B_SPLINE_SURFACE(((0.995452950231063,0.990618550266714,0.988709602819327),
(0.995452950231063,0.990618550266714,0.988709602819327)))
REPRESENTATION_ITEM('')
SURFACE()
);
#883=(
BOUNDED_SURFACE()
B_SPLINE_SURFACE(1,2,((#108495,#108496,#108497,#108498,#108499),(#108500,
#108501,#108502,#108503,#108504)),.UNSPECIFIED.,.F.,.F.,.F.)
B_SPLINE_SURFACE_WITH_KNOTS((2,2),(3,2,3),(0.,0.28968108436023),(0.280328542633765,
0.285714285714286,0.297856505190614),.UNSPECIFIED.)
GEOMETRIC_REPRESENTATION_ITEM()
RATIONAL_B_SPLINE_SURFACE(((0.996504189652447,0.998109554471267,1.,0.995737968897747,
0.992924952273132),(0.996504189652447,0.998109554471267,1.,0.995737968897747,
0.992924952273132)))
REPRESENTATION_ITEM('')
SURFACE()
);
#884=(
BOUNDED_SURFACE()
B_SPLINE_SURFACE(1,2,((#108522,#108523,#108524),(#108525,#108526,#108527)),
 .UNSPECIFIED.,.F.,.F.,.F.)
B_SPLINE_SURFACE_WITH_KNOTS((2,2),(3,3),(0.,0.289807040992805),(0.435775021682253,
0.453027768259471),.UNSPECIFIED.)
GEOMETRIC_REPRESENTATION_ITEM()
RATIONAL_B_SPLINE_SURFACE(((0.99545295023127,0.990618550266755,0.988709602819327),
(0.99545295023127,0.990618550266755,0.988709602819327)))
REPRESENTATION_ITEM('')
SURFACE()
);
#885=(
BOUNDED_SURFACE()
B_SPLINE_SURFACE(1,2,((#108529,#108530,#108531,#108532,#108533),(#108534,
#108535,#108536,#108537,#108538)),.UNSPECIFIED.,.F.,.F.,.F.)
B_SPLINE_SURFACE_WITH_KNOTS((2,2),(3,2,3),(0.,0.28968108435992),(0.280328542633765,
0.285714285714286,0.297856505190614),.UNSPECIFIED.)
GEOMETRIC_REPRESENTATION_ITEM()
RATIONAL_B_SPLINE_SURFACE(((0.996504189652447,0.998109554471267,1.,0.995737968897747,
0.992924952273132),(0.996504189652447,0.998109554471267,1.,0.995737968897747,
0.992924952273132)))
REPRESENTATION_ITEM('')
SURFACE()
);
#886=(
BOUNDED_SURFACE()
B_SPLINE_SURFACE(1,2,((#108556,#108557,#108558),(#108559,#108560,#108561)),
 .UNSPECIFIED.,.F.,.F.,.F.)
B_SPLINE_SURFACE_WITH_KNOTS((2,2),(3,3),(0.,0.28980704099266),(0.435775021682484,
0.45302776825947),.UNSPECIFIED.)
GEOMETRIC_REPRESENTATION_ITEM()
RATIONAL_B_SPLINE_SURFACE(((0.99545295023114,0.990618550266729,0.988709602819327),
(0.99545295023114,0.990618550266729,0.988709602819327)))
REPRESENTATION_ITEM('')
SURFACE()
);
#887=(
BOUNDED_SURFACE()
B_SPLINE_SURFACE(1,2,((#108563,#108564,#108565,#108566,#108567),(#108568,
#108569,#108570,#108571,#108572)),.UNSPECIFIED.,.F.,.F.,.F.)
B_SPLINE_SURFACE_WITH_KNOTS((2,2),(3,2,3),(0.,0.289681084359924),(0.280328542633765,
0.285714285714286,0.297856505190614),.UNSPECIFIED.)
GEOMETRIC_REPRESENTATION_ITEM()
RATIONAL_B_SPLINE_SURFACE(((0.996504189652446,0.998109554471267,1.,0.995737968897747,
0.992924952273132),(0.996504189652446,0.998109554471267,1.,0.995737968897747,
0.992924952273132)))
REPRESENTATION_ITEM('')
SURFACE()
);
#888=(
BOUNDED_SURFACE()
B_SPLINE_SURFACE(1,2,((#108590,#108591,#108592),(#108593,#108594,#108595)),
 .UNSPECIFIED.,.F.,.F.,.F.)
B_SPLINE_SURFACE_WITH_KNOTS((2,2),(3,3),(0.,0.289807040992677),(0.43577502168217,
0.453027768259471),.UNSPECIFIED.)
GEOMETRIC_REPRESENTATION_ITEM()
RATIONAL_B_SPLINE_SURFACE(((0.995452950231316,0.990618550266764,0.988709602819327),
(0.995452950231316,0.990618550266764,0.988709602819327)))
REPRESENTATION_ITEM('')
SURFACE()
);
#889=(
BOUNDED_SURFACE()
B_SPLINE_SURFACE(1,2,((#108597,#108598,#108599,#108600,#108601),(#108602,
#108603,#108604,#108605,#108606)),.UNSPECIFIED.,.F.,.F.,.F.)
B_SPLINE_SURFACE_WITH_KNOTS((2,2),(3,2,3),(0.,0.289681084359919),(0.280328542633765,
0.285714285714286,0.297856505190614),.UNSPECIFIED.)
GEOMETRIC_REPRESENTATION_ITEM()
RATIONAL_B_SPLINE_SURFACE(((0.996504189652446,0.998109554471267,1.,0.995737968897747,
0.992924952273132),(0.996504189652446,0.998109554471267,1.,0.995737968897747,
0.992924952273132)))
REPRESENTATION_ITEM('')
SURFACE()
);
#890=(
BOUNDED_SURFACE()
B_SPLINE_SURFACE(1,2,((#108612,#108613,#108614,#108615,#108616),(#108617,
#108618,#108619,#108620,#108621)),.UNSPECIFIED.,.F.,.F.,.F.)
B_SPLINE_SURFACE_WITH_KNOTS((2,2),(3,2,3),(0.,0.290406045058907),(0.331470144818563,
0.332069149066804,0.349473499542517),.UNSPECIFIED.)
GEOMETRIC_REPRESENTATION_ITEM()
RATIONAL_B_SPLINE_SURFACE(((0.988576730109495,0.988576730109495,0.988576730109495,
0.990396848309667,0.99519405818099),(0.988576730109495,0.988576730109495,
0.988576730109495,0.990396848309667,0.99519405818099)))
REPRESENTATION_ITEM('')
SURFACE()
);
#891=(
BOUNDED_SURFACE()
B_SPLINE_SURFACE(1,2,((#108638,#108639,#108640),(#108641,#108642,#108643),
(#108644,#108645,#108646)),.UNSPECIFIED.,.F.,.F.,.F.)
B_SPLINE_SURFACE_WITH_KNOTS((2,1,2),(3,3),(0.,0.289681084359929,0.292577895203529),
(0.383830569465723,0.401042835325579),.UNSPECIFIED.)
GEOMETRIC_REPRESENTATION_ITEM()
RATIONAL_B_SPLINE_SURFACE(((0.988264753026337,0.98673775832363,0.988122504062159),
(0.988264753026337,0.98673775832363,0.988122504062159),(0.988264753026337,
0.98673775832363,0.988122504062159)))
REPRESENTATION_ITEM('')
SURFACE()
);
#892=(
BOUNDED_SURFACE()
B_SPLINE_SURFACE(1,2,((#108648,#108649,#108650,#108651,#108652),(#108653,
#108654,#108655,#108656,#108657)),.UNSPECIFIED.,.F.,.F.,.F.)
B_SPLINE_SURFACE_WITH_KNOTS((2,2),(3,2,3),(0.,0.290406045025257),(0.331470144821685,
0.332069149066804,0.349473499542519),.UNSPECIFIED.)
GEOMETRIC_REPRESENTATION_ITEM()
RATIONAL_B_SPLINE_SURFACE(((0.988576730109495,0.988576730109495,0.988576730109495,
0.990396848309667,0.995194058180991),(0.988576730109495,0.988576730109495,
0.988576730109495,0.990396848309667,0.995194058180991)))
REPRESENTATION_ITEM('')
SURFACE()
);
#893=(
BOUNDED_SURFACE()
B_SPLINE_SURFACE(1,2,((#108674,#108675,#108676),(#108677,#108678,#108679),
(#108680,#108681,#108682)),.UNSPECIFIED.,.F.,.F.,.F.)
B_SPLINE_SURFACE_WITH_KNOTS((2,1,2),(3,3),(0.,0.289681084359929,0.292577895203529),
(0.383830569465724,0.401042835325431),.UNSPECIFIED.)
GEOMETRIC_REPRESENTATION_ITEM()
RATIONAL_B_SPLINE_SURFACE(((0.988264753026337,0.986737758323643,0.988122504062135),
(0.988264753026337,0.986737758323643,0.988122504062135),(0.988264753026337,
0.986737758323643,0.988122504062135)))
REPRESENTATION_ITEM('')
SURFACE()
);
#894=(
BOUNDED_SURFACE()
B_SPLINE_SURFACE(1,2,((#108684,#108685,#108686,#108687,#108688),(#108689,
#108690,#108691,#108692,#108693)),.UNSPECIFIED.,.F.,.F.,.F.)
B_SPLINE_SURFACE_WITH_KNOTS((2,2),(3,2,3),(0.,0.290406045000865),(0.331470144846541,
0.332069149066804,0.349473499542523),.UNSPECIFIED.)
GEOMETRIC_REPRESENTATION_ITEM()
RATIONAL_B_SPLINE_SURFACE(((0.988576730109495,0.988576730109495,0.988576730109495,
0.990396848309668,0.995194058180993),(0.988576730109495,0.988576730109495,
0.988576730109495,0.990396848309668,0.995194058180993)))
REPRESENTATION_ITEM('')
SURFACE()
);
#895=(
BOUNDED_SURFACE()
B_SPLINE_SURFACE(1,2,((#108710,#108711,#108712),(#108713,#108714,#108715),
(#108716,#108717,#108718)),.UNSPECIFIED.,.F.,.F.,.F.)
B_SPLINE_SURFACE_WITH_KNOTS((2,1,2),(3,3),(0.,0.289681084359919,0.292577895203518),
(0.383830569465724,0.401042835325431),.UNSPECIFIED.)
GEOMETRIC_REPRESENTATION_ITEM()
RATIONAL_B_SPLINE_SURFACE(((0.988264753026337,0.986737758323643,0.988122504062135),
(0.988264753026337,0.986737758323643,0.988122504062135),(0.988264753026337,
0.986737758323643,0.988122504062135)))
REPRESENTATION_ITEM('')
SURFACE()
);
#896=(
BOUNDED_SURFACE()
B_SPLINE_SURFACE(1,2,((#108720,#108721,#108722,#108723,#108724),(#108725,
#108726,#108727,#108728,#108729)),.UNSPECIFIED.,.F.,.F.,.F.)
B_SPLINE_SURFACE_WITH_KNOTS((2,2),(3,2,3),(0.,0.290406045022049),(0.331470144825657,
0.332069149066802,0.349473499542516),.UNSPECIFIED.)
GEOMETRIC_REPRESENTATION_ITEM()
RATIONAL_B_SPLINE_SURFACE(((0.988576730109495,0.988576730109495,0.988576730109495,
0.990396848309667,0.99519405818099),(0.988576730109495,0.988576730109495,
0.988576730109495,0.990396848309667,0.99519405818099)))
REPRESENTATION_ITEM('')
SURFACE()
);
#897=(
BOUNDED_SURFACE()
B_SPLINE_SURFACE(1,2,((#108746,#108747,#108748),(#108749,#108750,#108751),
(#108752,#108753,#108754)),.UNSPECIFIED.,.F.,.F.,.F.)
B_SPLINE_SURFACE_WITH_KNOTS((2,1,2),(3,3),(0.,0.289681084359923,0.292577895203522),
(0.383830569465724,0.401042835325431),.UNSPECIFIED.)
GEOMETRIC_REPRESENTATION_ITEM()
RATIONAL_B_SPLINE_SURFACE(((0.988264753026337,0.986737758323643,0.988122504062135),
(0.988264753026337,0.986737758323643,0.988122504062135),(0.988264753026337,
0.986737758323643,0.988122504062135)))
REPRESENTATION_ITEM('')
SURFACE()
);
#898=(
BOUNDED_SURFACE()
B_SPLINE_SURFACE(1,2,((#108756,#108757,#108758,#108759,#108760),(#108761,
#108762,#108763,#108764,#108765)),.UNSPECIFIED.,.F.,.F.,.F.)
B_SPLINE_SURFACE_WITH_KNOTS((2,2),(3,2,3),(0.,0.290406045027367),(0.331470144820027,
0.332069149066804,0.349473499542516),.UNSPECIFIED.)
GEOMETRIC_REPRESENTATION_ITEM()
RATIONAL_B_SPLINE_SURFACE(((0.988576730109495,0.988576730109495,0.988576730109495,
0.990396848309667,0.99519405818099),(0.988576730109495,0.988576730109495,
0.988576730109495,0.990396848309667,0.99519405818099)))
REPRESENTATION_ITEM('')
SURFACE()
);
#899=(
BOUNDED_SURFACE()
B_SPLINE_SURFACE(1,2,((#108782,#108783,#108784),(#108785,#108786,#108787),
(#108788,#108789,#108790)),.UNSPECIFIED.,.F.,.F.,.F.)
B_SPLINE_SURFACE_WITH_KNOTS((2,1,2),(3,3),(0.,0.289681084359917,0.292577895203516),
(0.383830569465724,0.401042835325431),.UNSPECIFIED.)
GEOMETRIC_REPRESENTATION_ITEM()
RATIONAL_B_SPLINE_SURFACE(((0.988264753026337,0.986737758323643,0.988122504062135),
(0.988264753026337,0.986737758323643,0.988122504062135),(0.988264753026337,
0.986737758323643,0.988122504062135)))
REPRESENTATION_ITEM('')
SURFACE()
);
#900=(
BOUNDED_SURFACE()
B_SPLINE_SURFACE(1,2,((#108792,#108793,#108794,#108795,#108796),(#108797,
#108798,#108799,#108800,#108801)),.UNSPECIFIED.,.F.,.F.,.F.)
B_SPLINE_SURFACE_WITH_KNOTS((2,2),(3,2,3),(0.,0.290406045052955),(0.331470144825287,
0.332069149066804,0.349473499542498),.UNSPECIFIED.)
GEOMETRIC_REPRESENTATION_ITEM()
RATIONAL_B_SPLINE_SURFACE(((0.988576730109495,0.988576730109495,0.988576730109495,
0.990396848309665,0.99519405818098),(0.988576730109495,0.988576730109495,
0.988576730109495,0.990396848309665,0.99519405818098)))
REPRESENTATION_ITEM('')
SURFACE()
);
#901=(
BOUNDED_SURFACE()
B_SPLINE_SURFACE(1,2,((#108818,#108819,#108820),(#108821,#108822,#108823),
(#108824,#108825,#108826)),.UNSPECIFIED.,.F.,.F.,.F.)
B_SPLINE_SURFACE_WITH_KNOTS((2,1,2),(3,3),(0.,0.289681084359922,0.292577895203521),
(0.383830569465707,0.401042835325431),.UNSPECIFIED.)
GEOMETRIC_REPRESENTATION_ITEM()
RATIONAL_B_SPLINE_SURFACE(((0.98826475302634,0.986737758323642,0.988122504062136),
(0.98826475302634,0.986737758323642,0.988122504062136),(0.98826475302634,
0.986737758323642,0.988122504062136)))
REPRESENTATION_ITEM('')
SURFACE()
);
#902=(
BOUNDED_SURFACE()
B_SPLINE_SURFACE(1,2,((#108828,#108829,#108830,#108831,#108832),(#108833,
#108834,#108835,#108836,#108837)),.UNSPECIFIED.,.F.,.F.,.F.)
B_SPLINE_SURFACE_WITH_KNOTS((2,2),(3,2,3),(0.,0.290406045005485),(0.331470144841198,
0.332069149066804,0.349473499542501),.UNSPECIFIED.)
GEOMETRIC_REPRESENTATION_ITEM()
RATIONAL_B_SPLINE_SURFACE(((0.988576730109495,0.988576730109495,0.988576730109495,
0.990396848309665,0.995194058180981),(0.988576730109495,0.988576730109495,
0.988576730109495,0.990396848309665,0.995194058180981)))
REPRESENTATION_ITEM('')
SURFACE()
);
#903=(
BOUNDED_SURFACE()
B_SPLINE_SURFACE(1,2,((#108854,#108855,#108856),(#108857,#108858,#108859),
(#108860,#108861,#108862)),.UNSPECIFIED.,.F.,.F.,.F.)
B_SPLINE_SURFACE_WITH_KNOTS((2,1,2),(3,3),(0.,0.289681084359922,0.292577895203521),
(0.383830569465707,0.401042835325431),.UNSPECIFIED.)
GEOMETRIC_REPRESENTATION_ITEM()
RATIONAL_B_SPLINE_SURFACE(((0.98826475302634,0.986737758323642,0.988122504062136),
(0.98826475302634,0.986737758323642,0.988122504062136),(0.98826475302634,
0.986737758323642,0.988122504062136)))
REPRESENTATION_ITEM('')
SURFACE()
);
#904=(
BOUNDED_SURFACE()
B_SPLINE_SURFACE(1,2,((#108864,#108865,#108866,#108867,#108868),(#108869,
#108870,#108871,#108872,#108873)),.UNSPECIFIED.,.F.,.F.,.F.)
B_SPLINE_SURFACE_WITH_KNOTS((2,2),(3,2,3),(0.,0.290406045032764),(0.331470144844551,
0.332069149066802,0.349473499542498),.UNSPECIFIED.)
GEOMETRIC_REPRESENTATION_ITEM()
RATIONAL_B_SPLINE_SURFACE(((0.988576730109495,0.988576730109495,0.988576730109495,
0.990396848309664,0.99519405818098),(0.988576730109495,0.988576730109495,
0.988576730109495,0.990396848309664,0.99519405818098)))
REPRESENTATION_ITEM('')
SURFACE()
);
#905=(
BOUNDED_SURFACE()
B_SPLINE_SURFACE(1,2,((#108890,#108891,#108892),(#108893,#108894,#108895),
(#108896,#108897,#108898)),.UNSPECIFIED.,.F.,.F.,.F.)
B_SPLINE_SURFACE_WITH_KNOTS((2,1,2),(3,3),(0.,0.289681084359926,0.292577895203525),
(0.383830569465707,0.401042835325431),.UNSPECIFIED.)
GEOMETRIC_REPRESENTATION_ITEM()
RATIONAL_B_SPLINE_SURFACE(((0.98826475302634,0.986737758323642,0.988122504062136),
(0.98826475302634,0.986737758323642,0.988122504062136),(0.98826475302634,
0.986737758323642,0.988122504062136)))
REPRESENTATION_ITEM('')
SURFACE()
);
#906=(
BOUNDED_SURFACE()
B_SPLINE_SURFACE(1,2,((#108900,#108901,#108902,#108903,#108904),(#108905,
#108906,#108907,#108908,#108909)),.UNSPECIFIED.,.F.,.F.,.F.)
B_SPLINE_SURFACE_WITH_KNOTS((2,2),(3,2,3),(0.,0.290406045042011),(0.331470144835407,
0.332069149066802,0.349473499542498),.UNSPECIFIED.)
GEOMETRIC_REPRESENTATION_ITEM()
RATIONAL_B_SPLINE_SURFACE(((0.988576730109495,0.988576730109495,0.988576730109495,
0.990396848309665,0.99519405818098),(0.988576730109495,0.988576730109495,
0.988576730109495,0.990396848309665,0.99519405818098)))
REPRESENTATION_ITEM('')
SURFACE()
);
#907=(
BOUNDED_SURFACE()
B_SPLINE_SURFACE(1,2,((#108926,#108927,#108928),(#108929,#108930,#108931),
(#108932,#108933,#108934)),.UNSPECIFIED.,.F.,.F.,.F.)
B_SPLINE_SURFACE_WITH_KNOTS((2,1,2),(3,3),(0.,0.289681084359927,0.292577895203526),
(0.383830569465707,0.401042835325431),.UNSPECIFIED.)
GEOMETRIC_REPRESENTATION_ITEM()
RATIONAL_B_SPLINE_SURFACE(((0.98826475302634,0.986737758323642,0.988122504062136),
(0.98826475302634,0.986737758323642,0.988122504062136),(0.98826475302634,
0.986737758323642,0.988122504062136)))
REPRESENTATION_ITEM('')
SURFACE()
);
#908=(
BOUNDED_SURFACE()
B_SPLINE_SURFACE(1,2,((#108936,#108937,#108938,#108939,#108940),(#108941,
#108942,#108943,#108944,#108945)),.UNSPECIFIED.,.F.,.F.,.F.)
B_SPLINE_SURFACE_WITH_KNOTS((2,2),(3,2,3),(0.,0.290406045022594),(0.331470144824454,
0.332069149066802,0.349473499542517),.UNSPECIFIED.)
GEOMETRIC_REPRESENTATION_ITEM()
RATIONAL_B_SPLINE_SURFACE(((0.988576730109495,0.988576730109495,0.988576730109495,
0.990396848309666,0.99519405818099),(0.988576730109495,0.988576730109495,
0.988576730109495,0.990396848309666,0.99519405818099)))
REPRESENTATION_ITEM('')
SURFACE()
);
#909=(
BOUNDED_SURFACE()
B_SPLINE_SURFACE(1,2,((#108962,#108963,#108964),(#108965,#108966,#108967),
(#108968,#108969,#108970)),.UNSPECIFIED.,.F.,.F.,.F.)
B_SPLINE_SURFACE_WITH_KNOTS((2,1,2),(3,3),(0.,0.289681084359921,0.29257789520352),
(0.383830569465723,0.401042835325579),.UNSPECIFIED.)
GEOMETRIC_REPRESENTATION_ITEM()
RATIONAL_B_SPLINE_SURFACE(((0.988264753026337,0.98673775832363,0.98812250406216),
(0.988264753026337,0.98673775832363,0.98812250406216),(0.988264753026337,
0.98673775832363,0.98812250406216)))
REPRESENTATION_ITEM('')
SURFACE()
);
#910=(
BOUNDED_SURFACE()
B_SPLINE_SURFACE(1,2,((#108972,#108973,#108974,#108975,#108976),(#108977,
#108978,#108979,#108980,#108981)),.UNSPECIFIED.,.F.,.F.,.F.)
B_SPLINE_SURFACE_WITH_KNOTS((2,2),(3,2,3),(0.,0.290406045013778),(0.33147014483302,
0.332069149066802,0.349473499542517),.UNSPECIFIED.)
GEOMETRIC_REPRESENTATION_ITEM()
RATIONAL_B_SPLINE_SURFACE(((0.988576730109495,0.988576730109495,0.988576730109495,
0.990396848309666,0.99519405818099),(0.988576730109495,0.988576730109495,
0.988576730109495,0.990396848309666,0.99519405818099)))
REPRESENTATION_ITEM('')
SURFACE()
);
#911=(
BOUNDED_SURFACE()
B_SPLINE_SURFACE(1,2,((#108998,#108999,#109000),(#109001,#109002,#109003),
(#109004,#109005,#109006)),.UNSPECIFIED.,.F.,.F.,.F.)
B_SPLINE_SURFACE_WITH_KNOTS((2,1,2),(3,3),(0.,0.289681084359917,0.292577895203516),
(0.383830569465724,0.401042835325432),.UNSPECIFIED.)
GEOMETRIC_REPRESENTATION_ITEM()
RATIONAL_B_SPLINE_SURFACE(((0.988264753026337,0.986737758323643,0.988122504062136),
(0.988264753026337,0.986737758323643,0.988122504062136),(0.988264753026337,
0.986737758323643,0.988122504062136)))
REPRESENTATION_ITEM('')
SURFACE()
);
#912=(
BOUNDED_SURFACE()
B_SPLINE_SURFACE(1,2,((#109008,#109009,#109010,#109011,#109012),(#109013,
#109014,#109015,#109016,#109017)),.UNSPECIFIED.,.F.,.F.,.F.)
B_SPLINE_SURFACE_WITH_KNOTS((2,2),(3,2,3),(0.,0.290406045030811),(0.33147014484647,
0.332069149066802,0.349473499542517),.UNSPECIFIED.)
GEOMETRIC_REPRESENTATION_ITEM()
RATIONAL_B_SPLINE_SURFACE(((0.988576730109495,0.988576730109495,0.988576730109495,
0.990396848309666,0.99519405818099),(0.988576730109495,0.988576730109495,
0.988576730109495,0.990396848309667,0.99519405818099)))
REPRESENTATION_ITEM('')
SURFACE()
);
#913=(
BOUNDED_SURFACE()
B_SPLINE_SURFACE(1,2,((#109034,#109035,#109036),(#109037,#109038,#109039),
(#109040,#109041,#109042)),.UNSPECIFIED.,.F.,.F.,.F.)
B_SPLINE_SURFACE_WITH_KNOTS((2,1,2),(3,3),(0.,0.289681084359925,0.292577895203524),
(0.383830569465724,0.401042835325431),.UNSPECIFIED.)
GEOMETRIC_REPRESENTATION_ITEM()
RATIONAL_B_SPLINE_SURFACE(((0.988264753026337,0.986737758323643,0.988122504062136),
(0.988264753026337,0.986737758323643,0.988122504062135),(0.988264753026337,
0.986737758323643,0.988122504062135)))
REPRESENTATION_ITEM('')
SURFACE()
);
#914=(
BOUNDED_SURFACE()
B_SPLINE_SURFACE(1,2,((#109044,#109045,#109046,#109047,#109048),(#109049,
#109050,#109051,#109052,#109053)),.UNSPECIFIED.,.F.,.F.,.F.)
B_SPLINE_SURFACE_WITH_KNOTS((2,2),(3,2,3),(0.,0.290406045030277),(0.331470144846858,
0.332069149066804,0.349473499542517),.UNSPECIFIED.)
GEOMETRIC_REPRESENTATION_ITEM()
RATIONAL_B_SPLINE_SURFACE(((0.988576730109495,0.988576730109495,0.988576730109495,
0.990396848309667,0.99519405818099),(0.988576730109495,0.988576730109495,
0.988576730109495,0.990396848309667,0.99519405818099)))
REPRESENTATION_ITEM('')
SURFACE()
);
#915=(
BOUNDED_SURFACE()
B_SPLINE_SURFACE(1,2,((#109070,#109071,#109072),(#109073,#109074,#109075),
(#109076,#109077,#109078)),.UNSPECIFIED.,.F.,.F.,.F.)
B_SPLINE_SURFACE_WITH_KNOTS((2,1,2),(3,3),(0.,0.289681084359927,0.292577895203526),
(0.383830569465724,0.401042835325431),.UNSPECIFIED.)
GEOMETRIC_REPRESENTATION_ITEM()
RATIONAL_B_SPLINE_SURFACE(((0.988264753026337,0.986737758323643,0.988122504062136),
(0.988264753026337,0.986737758323643,0.988122504062136),(0.988264753026337,
0.986737758323643,0.988122504062136)))
REPRESENTATION_ITEM('')
SURFACE()
);
#916=(
BOUNDED_SURFACE()
B_SPLINE_SURFACE(1,2,((#109080,#109081,#109082,#109083,#109084),(#109085,
#109086,#109087,#109088,#109089)),.UNSPECIFIED.,.F.,.F.,.F.)
B_SPLINE_SURFACE_WITH_KNOTS((2,2),(3,2,3),(0.,0.290406045030895),(0.331470144814642,
0.332069149066804,0.349473499542517),.UNSPECIFIED.)
GEOMETRIC_REPRESENTATION_ITEM()
RATIONAL_B_SPLINE_SURFACE(((0.988576730109495,0.988576730109495,0.988576730109495,
0.990396848309667,0.99519405818099),(0.988576730109495,0.988576730109495,
0.988576730109495,0.990396848309667,0.99519405818099)))
REPRESENTATION_ITEM('')
SURFACE()
);
#917=(
BOUNDED_SURFACE()
B_SPLINE_SURFACE(1,2,((#109106,#109107,#109108),(#109109,#109110,#109111),
(#109112,#109113,#109114)),.UNSPECIFIED.,.F.,.F.,.F.)
B_SPLINE_SURFACE_WITH_KNOTS((2,1,2),(3,3),(0.,0.289681084359927,0.292577895203526),
(0.383830569465724,0.401042835325431),.UNSPECIFIED.)
GEOMETRIC_REPRESENTATION_ITEM()
RATIONAL_B_SPLINE_SURFACE(((0.988264753026337,0.986737758323643,0.988122504062136),
(0.988264753026337,0.986737758323643,0.988122504062136),(0.988264753026337,
0.986737758323643,0.988122504062136)))
REPRESENTATION_ITEM('')
SURFACE()
);
#918=(
BOUNDED_SURFACE()
B_SPLINE_SURFACE(1,2,((#109116,#109117,#109118,#109119,#109120),(#109121,
#109122,#109123,#109124,#109125)),.UNSPECIFIED.,.F.,.F.,.F.)
B_SPLINE_SURFACE_WITH_KNOTS((2,2),(3,2,3),(0.,0.290038889744793),(0.331837300100696,
0.332069149066804,0.349473499542517),.UNSPECIFIED.)
GEOMETRIC_REPRESENTATION_ITEM()
RATIONAL_B_SPLINE_SURFACE(((0.988576730109495,0.988576730109495,0.988576730109495,
0.990396848309667,0.99519405818099),(0.988576730109495,0.988576730109495,
0.988576730109495,0.990396848309667,0.99519405818099)))
REPRESENTATION_ITEM('')
SURFACE()
);
#919=(
BOUNDED_SURFACE()
B_SPLINE_SURFACE(1,2,((#109133,#109134,#109135),(#109136,#109137,#109138),
(#109139,#109140,#109141)),.UNSPECIFIED.,.F.,.F.,.F.)
B_SPLINE_SURFACE_WITH_KNOTS((2,1,2),(3,3),(0.,0.289681084359933,0.292577895203533),
(0.383830569465724,0.401042835325431),.UNSPECIFIED.)
GEOMETRIC_REPRESENTATION_ITEM()
RATIONAL_B_SPLINE_SURFACE(((0.988264753026337,0.986737758323643,0.988122504062136),
(0.988264753026337,0.986737758323643,0.988122504062136),(0.988264753026337,
0.986737758323643,0.988122504062136)))
REPRESENTATION_ITEM('')
SURFACE()
);
#920=(
BOUNDED_SURFACE()
B_SPLINE_SURFACE(1,2,((#109143,#109144,#109145,#109146,#109147),(#109148,
#109149,#109150,#109151,#109152)),.UNSPECIFIED.,.F.,.F.,.F.)
B_SPLINE_SURFACE_WITH_KNOTS((2,2),(3,2,3),(0.,0.290406045005544),(0.331470144840714,
0.332069149066804,0.349473499542517),.UNSPECIFIED.)
GEOMETRIC_REPRESENTATION_ITEM()
RATIONAL_B_SPLINE_SURFACE(((0.988576730109495,0.988576730109495,0.988576730109495,
0.990396848309667,0.99519405818099),(0.988576730109495,0.988576730109495,
0.988576730109495,0.990396848309667,0.99519405818099)))
REPRESENTATION_ITEM('')
SURFACE()
);
#921=(
BOUNDED_SURFACE()
B_SPLINE_SURFACE(1,2,((#109169,#109170,#109171),(#109172,#109173,#109174),
(#109175,#109176,#109177)),.UNSPECIFIED.,.F.,.F.,.F.)
B_SPLINE_SURFACE_WITH_KNOTS((2,1,2),(3,3),(0.,0.289681084359918,0.292577895203517),
(0.383830569465724,0.401042835325432),.UNSPECIFIED.)
GEOMETRIC_REPRESENTATION_ITEM()
RATIONAL_B_SPLINE_SURFACE(((0.988264753026337,0.986737758323643,0.988122504062136),
(0.988264753026337,0.986737758323643,0.988122504062136),(0.988264753026337,
0.986737758323643,0.988122504062136)))
REPRESENTATION_ITEM('')
SURFACE()
);
#922=(
BOUNDED_SURFACE()
B_SPLINE_SURFACE(1,2,((#109179,#109180,#109181,#109182,#109183),(#109184,
#109185,#109186,#109187,#109188)),.UNSPECIFIED.,.F.,.F.,.F.)
B_SPLINE_SURFACE_WITH_KNOTS((2,2),(3,2,3),(0.,0.29040604502067),(0.331470144826036,
0.332069149066804,0.349473499542517),.UNSPECIFIED.)
GEOMETRIC_REPRESENTATION_ITEM()
RATIONAL_B_SPLINE_SURFACE(((0.988576730109495,0.988576730109495,0.988576730109495,
0.990396848309667,0.99519405818099),(0.988576730109495,0.988576730109495,
0.988576730109495,0.990396848309667,0.99519405818099)))
REPRESENTATION_ITEM('')
SURFACE()
);
#923=(
BOUNDED_SURFACE()
B_SPLINE_SURFACE(1,2,((#109205,#109206,#109207),(#109208,#109209,#109210),
(#109211,#109212,#109213)),.UNSPECIFIED.,.F.,.F.,.F.)
B_SPLINE_SURFACE_WITH_KNOTS((2,1,2),(3,3),(0.,0.289681084359923,0.292577895203522),
(0.383830569465724,0.401042835325432),.UNSPECIFIED.)
GEOMETRIC_REPRESENTATION_ITEM()
RATIONAL_B_SPLINE_SURFACE(((0.988264753026337,0.986737758323643,0.988122504062136),
(0.988264753026337,0.986737758323643,0.988122504062136),(0.988264753026337,
0.986737758323643,0.988122504062136)))
REPRESENTATION_ITEM('')
SURFACE()
);
#924=(
BOUNDED_SURFACE()
B_SPLINE_SURFACE(1,2,((#109215,#109216,#109217,#109218,#109219),(#109220,
#109221,#109222,#109223,#109224)),.UNSPECIFIED.,.F.,.F.,.F.)
B_SPLINE_SURFACE_WITH_KNOTS((2,2),(3,2,3),(0.,0.290406045013821),(0.331470144832401,
0.332069149066804,0.349473499542517),.UNSPECIFIED.)
GEOMETRIC_REPRESENTATION_ITEM()
RATIONAL_B_SPLINE_SURFACE(((0.988576730109495,0.988576730109495,0.988576730109495,
0.990396848309667,0.99519405818099),(0.988576730109495,0.988576730109495,
0.988576730109495,0.990396848309667,0.99519405818099)))
REPRESENTATION_ITEM('')
SURFACE()
);
#925=(
BOUNDED_SURFACE()
B_SPLINE_SURFACE(1,2,((#109241,#109242,#109243),(#109244,#109245,#109246),
(#109247,#109248,#109249)),.UNSPECIFIED.,.F.,.F.,.F.)
B_SPLINE_SURFACE_WITH_KNOTS((2,1,2),(3,3),(0.,0.289681084359923,0.292577895203522),
(0.383830569465724,0.401042835325432),.UNSPECIFIED.)
GEOMETRIC_REPRESENTATION_ITEM()
RATIONAL_B_SPLINE_SURFACE(((0.988264753026337,0.986737758323643,0.988122504062136),
(0.988264753026337,0.986737758323643,0.988122504062136),(0.988264753026337,
0.986737758323643,0.988122504062136)))
REPRESENTATION_ITEM('')
SURFACE()
);
#926=(
BOUNDED_SURFACE()
B_SPLINE_SURFACE(1,2,((#109251,#109252,#109253,#109254,#109255),(#109256,
#109257,#109258,#109259,#109260)),.UNSPECIFIED.,.F.,.F.,.F.)
B_SPLINE_SURFACE_WITH_KNOTS((2,2),(3,2,3),(0.,0.2904060450347),(0.331470144843839,
0.332069149066802,0.349473499542517),.UNSPECIFIED.)
GEOMETRIC_REPRESENTATION_ITEM()
RATIONAL_B_SPLINE_SURFACE(((0.988576730109495,0.988576730109495,0.988576730109495,
0.990396848309667,0.99519405818099),(0.988576730109495,0.988576730109495,
0.988576730109495,0.990396848309667,0.99519405818099)))
REPRESENTATION_ITEM('')
SURFACE()
);
#927=(
BOUNDED_SURFACE()
B_SPLINE_SURFACE(1,2,((#109277,#109278,#109279),(#109280,#109281,#109282),
(#109283,#109284,#109285)),.UNSPECIFIED.,.F.,.F.,.F.)
B_SPLINE_SURFACE_WITH_KNOTS((2,1,2),(3,3),(0.,0.289681084359922,0.292577895203521),
(0.383830569465724,0.401042835325431),.UNSPECIFIED.)
GEOMETRIC_REPRESENTATION_ITEM()
RATIONAL_B_SPLINE_SURFACE(((0.988264753026337,0.986737758323643,0.988122504062136),
(0.988264753026337,0.986737758323643,0.988122504062136),(0.988264753026337,
0.986737758323643,0.988122504062136)))
REPRESENTATION_ITEM('')
SURFACE()
);
#928=(
BOUNDED_SURFACE()
B_SPLINE_SURFACE(1,2,((#109287,#109288,#109289,#109290,#109291),(#109292,
#109293,#109294,#109295,#109296)),.UNSPECIFIED.,.F.,.F.,.F.)
B_SPLINE_SURFACE_WITH_KNOTS((2,2),(3,2,3),(0.,0.290406045030005),(0.331470144816454,
0.332069149066802,0.349473499542517),.UNSPECIFIED.)
GEOMETRIC_REPRESENTATION_ITEM()
RATIONAL_B_SPLINE_SURFACE(((0.988576730109495,0.988576730109495,0.988576730109495,
0.990396848309667,0.99519405818099),(0.988576730109495,0.988576730109495,
0.988576730109495,0.990396848309667,0.99519405818099)))
REPRESENTATION_ITEM('')
SURFACE()
);
#929=(
BOUNDED_SURFACE()
B_SPLINE_SURFACE(1,2,((#109313,#109314,#109315),(#109316,#109317,#109318),
(#109319,#109320,#109321)),.UNSPECIFIED.,.F.,.F.,.F.)
B_SPLINE_SURFACE_WITH_KNOTS((2,1,2),(3,3),(0.,0.289681084359921,0.29257789520352),
(0.383830569465724,0.401042835325431),.UNSPECIFIED.)
GEOMETRIC_REPRESENTATION_ITEM()
RATIONAL_B_SPLINE_SURFACE(((0.988264753026337,0.986737758323643,0.988122504062136),
(0.988264753026337,0.986737758323643,0.988122504062136),(0.988264753026337,
0.986737758323643,0.988122504062136)))
REPRESENTATION_ITEM('')
SURFACE()
);
#930=(
BOUNDED_SURFACE()
B_SPLINE_SURFACE(1,2,((#109323,#109324,#109325,#109326,#109327),(#109328,
#109329,#109330,#109331,#109332)),.UNSPECIFIED.,.F.,.F.,.F.)
B_SPLINE_SURFACE_WITH_KNOTS((2,2),(3,2,3),(0.,0.290406045012658),(0.331470144833921,
0.332069149066804,0.349473499542517),.UNSPECIFIED.)
GEOMETRIC_REPRESENTATION_ITEM()
RATIONAL_B_SPLINE_SURFACE(((0.988576730109495,0.988576730109495,0.988576730109495,
0.990396848309667,0.99519405818099),(0.988576730109495,0.988576730109495,
0.988576730109495,0.990396848309667,0.99519405818099)))
REPRESENTATION_ITEM('')
SURFACE()
);
#931=(
BOUNDED_SURFACE()
B_SPLINE_SURFACE(1,2,((#109349,#109350,#109351),(#109352,#109353,#109354),
(#109355,#109356,#109357)),.UNSPECIFIED.,.F.,.F.,.F.)
B_SPLINE_SURFACE_WITH_KNOTS((2,1,2),(3,3),(0.,0.289681084359924,0.292577895203523),
(0.383830569465724,0.401042835325431),.UNSPECIFIED.)
GEOMETRIC_REPRESENTATION_ITEM()
RATIONAL_B_SPLINE_SURFACE(((0.988264753026337,0.986737758323643,0.988122504062136),
(0.988264753026337,0.986737758323643,0.988122504062135),(0.988264753026337,
0.986737758323643,0.988122504062135)))
REPRESENTATION_ITEM('')
SURFACE()
);
#932=(
BOUNDED_SURFACE()
B_SPLINE_SURFACE(1,2,((#109359,#109360,#109361,#109362,#109363),(#109364,
#109365,#109366,#109367,#109368)),.UNSPECIFIED.,.F.,.F.,.F.)
B_SPLINE_SURFACE_WITH_KNOTS((2,2),(3,2,3),(0.,0.29040604502366),(0.331470144822577,
0.332069149066802,0.349473499542517),.UNSPECIFIED.)
GEOMETRIC_REPRESENTATION_ITEM()
RATIONAL_B_SPLINE_SURFACE(((0.988576730109495,0.988576730109495,0.988576730109495,
0.990396848309667,0.99519405818099),(0.988576730109495,0.988576730109495,
0.988576730109495,0.990396848309667,0.99519405818099)))
REPRESENTATION_ITEM('')
SURFACE()
);
#933=(
BOUNDED_SURFACE()
B_SPLINE_SURFACE(1,2,((#109385,#109386,#109387),(#109388,#109389,#109390),
(#109391,#109392,#109393)),.UNSPECIFIED.,.F.,.F.,.F.)
B_SPLINE_SURFACE_WITH_KNOTS((2,1,2),(3,3),(0.,0.289681084359919,0.292577895203518),
(0.383830569465724,0.401042835325431),.UNSPECIFIED.)
GEOMETRIC_REPRESENTATION_ITEM()
RATIONAL_B_SPLINE_SURFACE(((0.988264753026337,0.986737758323643,0.988122504062136),
(0.988264753026337,0.986737758323643,0.988122504062135),(0.988264753026337,
0.986737758323643,0.988122504062135)))
REPRESENTATION_ITEM('')
SURFACE()
);
#934=(
BOUNDED_SURFACE()
B_SPLINE_SURFACE(1,2,((#109395,#109396,#109397,#109398,#109399),(#109400,
#109401,#109402,#109403,#109404)),.UNSPECIFIED.,.F.,.F.,.F.)
B_SPLINE_SURFACE_WITH_KNOTS((2,2),(3,2,3),(0.,0.290406045042354),(0.33147014480446,
0.332069149066802,0.349473499542517),.UNSPECIFIED.)
GEOMETRIC_REPRESENTATION_ITEM()
RATIONAL_B_SPLINE_SURFACE(((0.988576730109495,0.988576730109495,0.988576730109495,
0.990396848309667,0.99519405818099),(0.988576730109495,0.988576730109495,
0.988576730109495,0.990396848309666,0.99519405818099)))
REPRESENTATION_ITEM('')
SURFACE()
);
#935=(
BOUNDED_SURFACE()
B_SPLINE_SURFACE(1,2,((#109421,#109422,#109423),(#109424,#109425,#109426),
(#109427,#109428,#109429)),.UNSPECIFIED.,.F.,.F.,.F.)
B_SPLINE_SURFACE_WITH_KNOTS((2,1,2),(3,3),(0.,0.289681084359919,0.292577895203518),
(0.383830569465724,0.401042835325431),.UNSPECIFIED.)
GEOMETRIC_REPRESENTATION_ITEM()
RATIONAL_B_SPLINE_SURFACE(((0.988264753026337,0.986737758323643,0.988122504062136),
(0.988264753026337,0.986737758323643,0.988122504062136),(0.988264753026337,
0.986737758323643,0.988122504062136)))
REPRESENTATION_ITEM('')
SURFACE()
);
#936=(
BOUNDED_SURFACE()
B_SPLINE_SURFACE(1,2,((#109431,#109432,#109433,#109434,#109435),(#109436,
#109437,#109438,#109439,#109440)),.UNSPECIFIED.,.F.,.F.,.F.)
B_SPLINE_SURFACE_WITH_KNOTS((2,2),(3,2,3),(0.,0.290406045004334),(0.331470144841729,
0.332069149066802,0.349473499542517),.UNSPECIFIED.)
GEOMETRIC_REPRESENTATION_ITEM()
RATIONAL_B_SPLINE_SURFACE(((0.988576730109495,0.988576730109495,0.988576730109495,
0.990396848309667,0.99519405818099),(0.988576730109495,0.988576730109495,
0.988576730109495,0.990396848309666,0.99519405818099)))
REPRESENTATION_ITEM('')
SURFACE()
);
#937=(
BOUNDED_SURFACE()
B_SPLINE_SURFACE(1,2,((#109451,#109452,#109453),(#109454,#109455,#109456),
(#109457,#109458,#109459)),.UNSPECIFIED.,.F.,.F.,.F.)
B_SPLINE_SURFACE_WITH_KNOTS((2,1,2),(3,3),(0.,0.289681084359924,0.292577895203523),
(0.383830569465724,0.401042835325431),.UNSPECIFIED.)
GEOMETRIC_REPRESENTATION_ITEM()
RATIONAL_B_SPLINE_SURFACE(((0.988264753026337,0.986737758323643,0.988122504062136),
(0.988264753026337,0.986737758323643,0.988122504062136),(0.988264753026337,
0.986737758323643,0.988122504062136)))
REPRESENTATION_ITEM('')
SURFACE()
);
#938=(
BOUNDED_SURFACE()
B_SPLINE_SURFACE(1,2,((#109467,#109468,#109469,#109470,#109471),(#109472,
#109473,#109474,#109475,#109476)),.UNSPECIFIED.,.F.,.F.,.F.)
B_SPLINE_SURFACE_WITH_KNOTS((2,2),(3,2,3),(0.,0.290406045008831),(0.331470144837565,
0.332069149066804,0.349473499542517),.UNSPECIFIED.)
GEOMETRIC_REPRESENTATION_ITEM()
RATIONAL_B_SPLINE_SURFACE(((0.988576730109495,0.988576730109495,0.988576730109495,
0.990396848309667,0.99519405818099),(0.988576730109495,0.988576730109495,
0.988576730109495,0.990396848309667,0.99519405818099)))
REPRESENTATION_ITEM('')
SURFACE()
);
#939=(
BOUNDED_SURFACE()
B_SPLINE_SURFACE(1,2,((#109493,#109494,#109495),(#109496,#109497,#109498),
(#109499,#109500,#109501)),.UNSPECIFIED.,.F.,.F.,.F.)
B_SPLINE_SURFACE_WITH_KNOTS((2,1,2),(3,3),(0.,0.289681084359917,0.292577895203516),
(0.38383056946572,0.401042835325487),.UNSPECIFIED.)
GEOMETRIC_REPRESENTATION_ITEM()
RATIONAL_B_SPLINE_SURFACE(((0.988264753026338,0.986737758323638,0.988122504062145),
(0.988264753026338,0.986737758323638,0.988122504062145),(0.988264753026338,
0.986737758323638,0.988122504062145)))
REPRESENTATION_ITEM('')
SURFACE()
);
#940=(
BOUNDED_SURFACE()
B_SPLINE_SURFACE(1,2,((#109503,#109504,#109505,#109506,#109507),(#109508,
#109509,#109510,#109511,#109512)),.UNSPECIFIED.,.F.,.F.,.F.)
B_SPLINE_SURFACE_WITH_KNOTS((2,2),(3,2,3),(0.,0.290406045002945),(0.331470144843635,
0.332069149066803,0.349473499542518),.UNSPECIFIED.)
GEOMETRIC_REPRESENTATION_ITEM()
RATIONAL_B_SPLINE_SURFACE(((0.988576730109495,0.988576730109495,0.988576730109495,
0.990396848309667,0.995194058180991),(0.988576730109495,0.988576730109495,
0.988576730109495,0.990396848309667,0.995194058180991)))
REPRESENTATION_ITEM('')
SURFACE()
);
#941=(
BOUNDED_SURFACE()
B_SPLINE_SURFACE(1,2,((#109529,#109530,#109531),(#109532,#109533,#109534),
(#109535,#109536,#109537)),.UNSPECIFIED.,.F.,.F.,.F.)
B_SPLINE_SURFACE_WITH_KNOTS((2,1,2),(3,3),(0.,0.289681084359926,0.292577895203525),
(0.383830569465722,0.40104283532548),.UNSPECIFIED.)
GEOMETRIC_REPRESENTATION_ITEM()
RATIONAL_B_SPLINE_SURFACE(((0.988264753026337,0.986737758323638,0.988122504062143),
(0.988264753026337,0.986737758323638,0.988122504062143),(0.988264753026337,
0.986737758323638,0.988122504062143)))
REPRESENTATION_ITEM('')
SURFACE()
);
#942=(
BOUNDED_SURFACE()
B_SPLINE_SURFACE(1,2,((#109539,#109540,#109541,#109542,#109543),(#109544,
#109545,#109546,#109547,#109548)),.UNSPECIFIED.,.F.,.F.,.F.)
B_SPLINE_SURFACE_WITH_KNOTS((2,2),(3,2,3),(0.,0.290406045028382),(0.331470144849026,
0.332069149066805,0.349473499542517),.UNSPECIFIED.)
GEOMETRIC_REPRESENTATION_ITEM()
RATIONAL_B_SPLINE_SURFACE(((0.988576730109495,0.988576730109495,0.988576730109495,
0.990396848309667,0.99519405818099),(0.988576730109495,0.988576730109495,
0.988576730109495,0.990396848309667,0.99519405818099)))
REPRESENTATION_ITEM('')
SURFACE()
);
#943=(
BOUNDED_SURFACE()
B_SPLINE_SURFACE(1,2,((#109565,#109566,#109567),(#109568,#109569,#109570),
(#109571,#109572,#109573)),.UNSPECIFIED.,.F.,.F.,.F.)
B_SPLINE_SURFACE_WITH_KNOTS((2,1,2),(3,3),(0.,0.289681084359917,0.292577895203516),
(0.383830569465723,0.40104283532558),.UNSPECIFIED.)
GEOMETRIC_REPRESENTATION_ITEM()
RATIONAL_B_SPLINE_SURFACE(((0.988264753026337,0.98673775832363,0.98812250406216),
(0.988264753026337,0.98673775832363,0.98812250406216),(0.988264753026337,
0.98673775832363,0.98812250406216)))
REPRESENTATION_ITEM('')
SURFACE()
);
#944=(
BOUNDED_SURFACE()
B_SPLINE_SURFACE(1,2,((#109575,#109576,#109577,#109578,#109579),(#109580,
#109581,#109582,#109583,#109584)),.UNSPECIFIED.,.F.,.F.,.F.)
B_SPLINE_SURFACE_WITH_KNOTS((2,2),(3,2,3),(0.,0.290406045018038),(0.331470144859553,
0.332069149066804,0.349473499542517),.UNSPECIFIED.)
GEOMETRIC_REPRESENTATION_ITEM()
RATIONAL_B_SPLINE_SURFACE(((0.988576730109495,0.988576730109495,0.988576730109495,
0.990396848309667,0.99519405818099),(0.988576730109495,0.988576730109495,
0.988576730109495,0.990396848309667,0.99519405818099)))
REPRESENTATION_ITEM('')
SURFACE()
);
#945=(
BOUNDED_SURFACE()
B_SPLINE_SURFACE(1,2,((#109601,#109602,#109603),(#109604,#109605,#109606),
(#109607,#109608,#109609)),.UNSPECIFIED.,.F.,.F.,.F.)
B_SPLINE_SURFACE_WITH_KNOTS((2,1,2),(3,3),(0.,0.289681084359936,0.292577895203535),
(0.383830569465723,0.40104283532558),.UNSPECIFIED.)
GEOMETRIC_REPRESENTATION_ITEM()
RATIONAL_B_SPLINE_SURFACE(((0.988264753026337,0.986737758323629,0.988122504062159),
(0.988264753026337,0.986737758323629,0.988122504062159),(0.988264753026337,
0.986737758323629,0.988122504062159)))
REPRESENTATION_ITEM('')
SURFACE()
);
#946=(
BOUNDED_SURFACE()
B_SPLINE_SURFACE(1,2,((#109611,#109612,#109613,#109614,#109615),(#109616,
#109617,#109618,#109619,#109620)),.UNSPECIFIED.,.F.,.F.,.F.)
B_SPLINE_SURFACE_WITH_KNOTS((2,2),(3,2,3),(0.,0.290406045046641),(0.331470144830908,
0.332069149066804,0.349473499542517),.UNSPECIFIED.)
GEOMETRIC_REPRESENTATION_ITEM()
RATIONAL_B_SPLINE_SURFACE(((0.988576730109495,0.988576730109495,0.988576730109495,
0.990396848309667,0.99519405818099),(0.988576730109495,0.988576730109495,
0.988576730109495,0.990396848309667,0.99519405818099)))
REPRESENTATION_ITEM('')
SURFACE()
);
#947=(
BOUNDED_SURFACE()
B_SPLINE_SURFACE(1,2,((#109637,#109638,#109639),(#109640,#109641,#109642),
(#109643,#109644,#109645)),.UNSPECIFIED.,.F.,.F.,.F.)
B_SPLINE_SURFACE_WITH_KNOTS((2,1,2),(3,3),(0.,0.289681084359927,0.292577895203526),
(0.383830569465723,0.401042835325579),.UNSPECIFIED.)
GEOMETRIC_REPRESENTATION_ITEM()
RATIONAL_B_SPLINE_SURFACE(((0.988264753026337,0.98673775832363,0.988122504062159),
(0.988264753026337,0.98673775832363,0.988122504062159),(0.988264753026337,
0.98673775832363,0.988122504062159)))
REPRESENTATION_ITEM('')
SURFACE()
);
#948=(
BOUNDED_SURFACE()
B_SPLINE_SURFACE(1,2,((#109647,#109648,#109649),(#109650,#109651,#109652)),
 .UNSPECIFIED.,.F.,.F.,.F.)
B_SPLINE_SURFACE_WITH_KNOTS((2,2),(3,3),(0.710318915638199,1.),(0.435672122597606,
0.452924869174518),.UNSPECIFIED.)
GEOMETRIC_REPRESENTATION_ITEM()
RATIONAL_B_SPLINE_SURFACE(((0.995510721093658,0.99065887310234,0.988732477628005),
(0.995510721093658,0.99065887310234,0.988732477628005)))
REPRESENTATION_ITEM('')
SURFACE()
);
#949=(
BOUNDED_SURFACE()
B_SPLINE_SURFACE(1,2,((#109663,#109664,#109665,#109666,#109667,#109668,
#109669),(#109670,#109671,#109672,#109673,#109674,#109675,#109676)),
 .UNSPECIFIED.,.F.,.F.,.F.)
B_SPLINE_SURFACE_WITH_KNOTS((2,2),(3,2,2,3),(0.710192959006552,1.),(0.280257803540346,
0.280433083165914,0.285714285714286,0.297961045722742),.UNSPECIFIED.)
GEOMETRIC_REPRESENTATION_ITEM()
RATIONAL_B_SPLINE_SURFACE(((0.996566619267864,0.996566619267864,0.996566619267864,
0.998146249162903,1.,0.995701274206118,0.992876621380151),(0.996566619267864,
0.996566619267864,0.996566619267864,0.998146249162903,1.,0.995701274206118,
0.992876621380151)))
REPRESENTATION_ITEM('')
SURFACE()
);
#950=(
BOUNDED_SURFACE()
B_SPLINE_SURFACE(1,2,((#109690,#109691,#109692),(#109693,#109694,#109695)),
 .UNSPECIFIED.,.F.,.F.,.F.)
B_SPLINE_SURFACE_WITH_KNOTS((2,2),(3,3),(0.710318915640079,1.),(0.43567212259767,
0.452924869174517),.UNSPECIFIED.)
GEOMETRIC_REPRESENTATION_ITEM()
RATIONAL_B_SPLINE_SURFACE(((0.995510721093622,0.990658873102333,0.988732477628005),
(0.995510721093622,0.990658873102333,0.988732477628005)))
REPRESENTATION_ITEM('')
SURFACE()
);
#951=(
BOUNDED_SURFACE()
B_SPLINE_SURFACE(1,2,((#109706,#109707,#109708,#109709,#109710,#109711,
#109712),(#109713,#109714,#109715,#109716,#109717,#109718,#109719)),
 .UNSPECIFIED.,.F.,.F.,.F.)
B_SPLINE_SURFACE_WITH_KNOTS((2,2),(3,2,2,3),(0.710192959008442,1.),(0.280257803540343,
0.280433083165911,0.285714285714286,0.297961045722763),.UNSPECIFIED.)
GEOMETRIC_REPRESENTATION_ITEM()
RATIONAL_B_SPLINE_SURFACE(((0.996566619267862,0.996566619267862,0.996566619267862,
0.998146249162902,1.,0.995701274206111,0.992876621380142),(0.996566619267862,
0.996566619267862,0.996566619267862,0.998146249162902,1.,0.995701274206111,
0.992876621380142)))
REPRESENTATION_ITEM('')
SURFACE()
);
#952=(
BOUNDED_SURFACE()
B_SPLINE_SURFACE(1,2,((#109733,#109734,#109735),(#109736,#109737,#109738)),
 .UNSPECIFIED.,.F.,.F.,.F.)
B_SPLINE_SURFACE_WITH_KNOTS((2,2),(3,3),(0.710318915639502,1.),(0.43567212259767,
0.452924869174517),.UNSPECIFIED.)
GEOMETRIC_REPRESENTATION_ITEM()
RATIONAL_B_SPLINE_SURFACE(((0.995510721093622,0.990658873102333,0.988732477628006),
(0.995510721093622,0.990658873102333,0.988732477628006)))
REPRESENTATION_ITEM('')
SURFACE()
);
#953=(
BOUNDED_SURFACE()
B_SPLINE_SURFACE(1,2,((#109749,#109750,#109751,#109752,#109753,#109754,
#109755),(#109756,#109757,#109758,#109759,#109760,#109761,#109762)),
 .UNSPECIFIED.,.F.,.F.,.F.)
B_SPLINE_SURFACE_WITH_KNOTS((2,2),(3,2,2,3),(0.710192959007859,1.),(0.280257803540345,
0.280433083165913,0.285714285714286,0.297961045722763),.UNSPECIFIED.)
GEOMETRIC_REPRESENTATION_ITEM()
RATIONAL_B_SPLINE_SURFACE(((0.996566619267863,0.996566619267863,0.996566619267863,
0.998146249162903,1.,0.995701274206111,0.992876621380141),(0.996566619267863,
0.996566619267863,0.996566619267863,0.998146249162903,1.,0.995701274206111,
0.992876621380141)))
REPRESENTATION_ITEM('')
SURFACE()
);
#954=(
BOUNDED_SURFACE()
B_SPLINE_SURFACE(1,2,((#109776,#109777,#109778),(#109779,#109780,#109781)),
 .UNSPECIFIED.,.F.,.F.,.F.)
B_SPLINE_SURFACE_WITH_KNOTS((2,2),(3,3),(0.710318915640078,1.),(0.43567212259767,
0.452924869174517),.UNSPECIFIED.)
GEOMETRIC_REPRESENTATION_ITEM()
RATIONAL_B_SPLINE_SURFACE(((0.995510721093622,0.990658873102333,0.988732477628005),
(0.995510721093622,0.990658873102333,0.988732477628005)))
REPRESENTATION_ITEM('')
SURFACE()
);
#955=(
BOUNDED_SURFACE()
B_SPLINE_SURFACE(1,2,((#109792,#109793,#109794,#109795,#109796,#109797,
#109798),(#109799,#109800,#109801,#109802,#109803,#109804,#109805)),
 .UNSPECIFIED.,.F.,.F.,.F.)
B_SPLINE_SURFACE_WITH_KNOTS((2,2),(3,2,2,3),(0.710192959008441,1.),(0.280257803540345,
0.280433083165913,0.285714285714286,0.297961045722763),.UNSPECIFIED.)
GEOMETRIC_REPRESENTATION_ITEM()
RATIONAL_B_SPLINE_SURFACE(((0.996566619267863,0.996566619267863,0.996566619267863,
0.998146249162903,1.,0.995701274206111,0.992876621380142),(0.996566619267863,
0.996566619267863,0.996566619267863,0.998146249162903,1.,0.995701274206111,
0.992876621380142)))
REPRESENTATION_ITEM('')
SURFACE()
);
#956=(
BOUNDED_SURFACE()
B_SPLINE_SURFACE(1,2,((#109819,#109820,#109821),(#109822,#109823,#109824)),
 .UNSPECIFIED.,.F.,.F.,.F.)
B_SPLINE_SURFACE_WITH_KNOTS((2,2),(3,3),(0.710318915639499,1.),(0.43567212259767,
0.452924869174517),.UNSPECIFIED.)
GEOMETRIC_REPRESENTATION_ITEM()
RATIONAL_B_SPLINE_SURFACE(((0.995510721093622,0.990658873102333,0.988732477628005),
(0.995510721093622,0.990658873102333,0.988732477628005)))
REPRESENTATION_ITEM('')
SURFACE()
);
#957=(
BOUNDED_SURFACE()
B_SPLINE_SURFACE(1,2,((#109835,#109836,#109837,#109838,#109839,#109840,
#109841),(#109842,#109843,#109844,#109845,#109846,#109847,#109848)),
 .UNSPECIFIED.,.F.,.F.,.F.)
B_SPLINE_SURFACE_WITH_KNOTS((2,2),(3,2,2,3),(0.710192959007862,1.),(0.280257803540345,
0.280433083165913,0.285714285714286,0.297961045722763),.UNSPECIFIED.)
GEOMETRIC_REPRESENTATION_ITEM()
RATIONAL_B_SPLINE_SURFACE(((0.996566619267863,0.996566619267863,0.996566619267863,
0.998146249162903,1.,0.995701274206111,0.992876621380142),(0.996566619267863,
0.996566619267863,0.996566619267863,0.998146249162903,1.,0.995701274206111,
0.992876621380142)))
REPRESENTATION_ITEM('')
SURFACE()
);
#958=(
BOUNDED_SURFACE()
B_SPLINE_SURFACE(1,2,((#109862,#109863,#109864),(#109865,#109866,#109867)),
 .UNSPECIFIED.,.F.,.F.,.F.)
B_SPLINE_SURFACE_WITH_KNOTS((2,2),(3,3),(0.710318915640002,1.),(0.435672122597671,
0.452924869174517),.UNSPECIFIED.)
GEOMETRIC_REPRESENTATION_ITEM()
RATIONAL_B_SPLINE_SURFACE(((0.995510721093621,0.990658873102333,0.988732477628005),
(0.995510721093621,0.990658873102333,0.988732477628005)))
REPRESENTATION_ITEM('')
SURFACE()
);
#959=(
BOUNDED_SURFACE()
B_SPLINE_SURFACE(1,2,((#109878,#109879,#109880,#109881,#109882,#109883,
#109884),(#109885,#109886,#109887,#109888,#109889,#109890,#109891)),
 .UNSPECIFIED.,.F.,.F.,.F.)
B_SPLINE_SURFACE_WITH_KNOTS((2,2),(3,2,2,3),(0.710192959008361,1.),(0.280257803540343,
0.280433083165911,0.285714285714286,0.297961045722762),.UNSPECIFIED.)
GEOMETRIC_REPRESENTATION_ITEM()
RATIONAL_B_SPLINE_SURFACE(((0.996566619267862,0.996566619267862,0.996566619267862,
0.998146249162902,1.,0.995701274206111,0.992876621380142),(0.996566619267862,
0.996566619267862,0.996566619267862,0.998146249162902,1.,0.995701274206111,
0.992876621380142)))
REPRESENTATION_ITEM('')
SURFACE()
);
#960=(
BOUNDED_SURFACE()
B_SPLINE_SURFACE(1,2,((#109905,#109906,#109907),(#109908,#109909,#109910)),
 .UNSPECIFIED.,.F.,.F.,.F.)
B_SPLINE_SURFACE_WITH_KNOTS((2,2),(3,3),(0.710318915640002,1.),(0.435672122597671,
0.452924869174518),.UNSPECIFIED.)
GEOMETRIC_REPRESENTATION_ITEM()
RATIONAL_B_SPLINE_SURFACE(((0.995510721093621,0.990658873102333,0.988732477628005),
(0.995510721093621,0.990658873102333,0.988732477628005)))
REPRESENTATION_ITEM('')
SURFACE()
);
#961=(
BOUNDED_SURFACE()
B_SPLINE_SURFACE(1,2,((#109921,#109922,#109923,#109924,#109925,#109926,
#109927),(#109928,#109929,#109930,#109931,#109932,#109933,#109934)),
 .UNSPECIFIED.,.F.,.F.,.F.)
B_SPLINE_SURFACE_WITH_KNOTS((2,2),(3,2,2,3),(0.710192959008365,1.),(0.280257803540344,
0.280433083165912,0.285714285714286,0.297961045722762),.UNSPECIFIED.)
GEOMETRIC_REPRESENTATION_ITEM()
RATIONAL_B_SPLINE_SURFACE(((0.996566619267863,0.996566619267863,0.996566619267863,
0.998146249162903,1.,0.995701274206111,0.992876621380142),(0.996566619267863,
0.996566619267863,0.996566619267863,0.998146249162903,1.,0.995701274206111,
0.992876621380142)))
REPRESENTATION_ITEM('')
SURFACE()
);
#962=(
BOUNDED_SURFACE()
B_SPLINE_SURFACE(1,2,((#109948,#109949,#109950),(#109951,#109952,#109953)),
 .UNSPECIFIED.,.F.,.F.,.F.)
B_SPLINE_SURFACE_WITH_KNOTS((2,2),(3,3),(0.71031891563941,1.),(0.435672122597671,
0.452924869174518),.UNSPECIFIED.)
GEOMETRIC_REPRESENTATION_ITEM()
RATIONAL_B_SPLINE_SURFACE(((0.995510721093621,0.990658873102333,0.988732477628005),
(0.995510721093621,0.990658873102333,0.988732477628005)))
REPRESENTATION_ITEM('')
SURFACE()
);
#963=(
BOUNDED_SURFACE()
B_SPLINE_SURFACE(1,2,((#109964,#109965,#109966,#109967,#109968,#109969,
#109970),(#109971,#109972,#109973,#109974,#109975,#109976,#109977)),
 .UNSPECIFIED.,.F.,.F.,.F.)
B_SPLINE_SURFACE_WITH_KNOTS((2,2),(3,2,2,3),(0.71019295900777,1.),(0.280257803540344,
0.280433083165912,0.285714285714286,0.297961045722762),.UNSPECIFIED.)
GEOMETRIC_REPRESENTATION_ITEM()
RATIONAL_B_SPLINE_SURFACE(((0.996566619267863,0.996566619267863,0.996566619267863,
0.998146249162903,1.,0.995701274206111,0.992876621380142),(0.996566619267863,
0.996566619267863,0.996566619267863,0.998146249162903,1.,0.995701274206111,
0.992876621380142)))
REPRESENTATION_ITEM('')
SURFACE()
);
#964=(
BOUNDED_SURFACE()
B_SPLINE_SURFACE(1,2,((#109991,#109992,#109993),(#109994,#109995,#109996)),
 .UNSPECIFIED.,.F.,.F.,.F.)
B_SPLINE_SURFACE_WITH_KNOTS((2,2),(3,3),(0.710318915639997,1.),(0.435672122597671,
0.452924869174518),.UNSPECIFIED.)
GEOMETRIC_REPRESENTATION_ITEM()
RATIONAL_B_SPLINE_SURFACE(((0.995510721093621,0.990658873102333,0.988732477628005),
(0.995510721093621,0.990658873102333,0.988732477628005)))
REPRESENTATION_ITEM('')
SURFACE()
);
#965=(
BOUNDED_SURFACE()
B_SPLINE_SURFACE(1,2,((#110007,#110008,#110009,#110010,#110011,#110012,
#110013),(#110014,#110015,#110016,#110017,#110018,#110019,#110020)),
 .UNSPECIFIED.,.F.,.F.,.F.)
B_SPLINE_SURFACE_WITH_KNOTS((2,2),(3,2,2,3),(0.710192959008358,1.),(0.280257803540343,
0.280433083165911,0.285714285714286,0.297961045722762),.UNSPECIFIED.)
GEOMETRIC_REPRESENTATION_ITEM()
RATIONAL_B_SPLINE_SURFACE(((0.996566619267862,0.996566619267862,0.996566619267862,
0.998146249162902,1.,0.995701274206111,0.992876621380142),(0.996566619267862,
0.996566619267862,0.996566619267862,0.998146249162902,1.,0.995701274206111,
0.992876621380142)))
REPRESENTATION_ITEM('')
SURFACE()
);
#966=(
BOUNDED_SURFACE()
B_SPLINE_SURFACE(1,2,((#110034,#110035,#110036),(#110037,#110038,#110039)),
 .UNSPECIFIED.,.F.,.F.,.F.)
B_SPLINE_SURFACE_WITH_KNOTS((2,2),(3,3),(0.710318915639496,1.),(0.435672122597671,
0.452924869174518),.UNSPECIFIED.)
GEOMETRIC_REPRESENTATION_ITEM()
RATIONAL_B_SPLINE_SURFACE(((0.995510721093621,0.990658873102333,0.988732477628005),
(0.995510721093621,0.990658873102333,0.988732477628005)))
REPRESENTATION_ITEM('')
SURFACE()
);
#967=(
BOUNDED_SURFACE()
B_SPLINE_SURFACE(1,2,((#110050,#110051,#110052,#110053,#110054,#110055,
#110056),(#110057,#110058,#110059,#110060,#110061,#110062,#110063)),
 .UNSPECIFIED.,.F.,.F.,.F.)
B_SPLINE_SURFACE_WITH_KNOTS((2,2),(3,2,2,3),(0.710192959007859,1.),(0.280257803540344,
0.280433083165912,0.285714285714286,0.297961045722762),.UNSPECIFIED.)
GEOMETRIC_REPRESENTATION_ITEM()
RATIONAL_B_SPLINE_SURFACE(((0.996566619267862,0.996566619267862,0.996566619267862,
0.998146249162902,1.,0.995701274206111,0.992876621380142),(0.996566619267862,
0.996566619267862,0.996566619267862,0.998146249162902,1.,0.995701274206111,
0.992876621380142)))
REPRESENTATION_ITEM('')
SURFACE()
);
#968=(
BOUNDED_SURFACE()
B_SPLINE_SURFACE(1,2,((#110077,#110078,#110079),(#110080,#110081,#110082)),
 .UNSPECIFIED.,.F.,.F.,.F.)
B_SPLINE_SURFACE_WITH_KNOTS((2,2),(3,3),(0.71031891563999,1.),(0.435672122597671,
0.452924869174518),.UNSPECIFIED.)
GEOMETRIC_REPRESENTATION_ITEM()
RATIONAL_B_SPLINE_SURFACE(((0.995510721093621,0.990658873102333,0.988732477628005),
(0.995510721093621,0.990658873102333,0.988732477628005)))
REPRESENTATION_ITEM('')
SURFACE()
);
#969=(
BOUNDED_SURFACE()
B_SPLINE_SURFACE(1,2,((#110093,#110094,#110095,#110096,#110097,#110098,
#110099),(#110100,#110101,#110102,#110103,#110104,#110105,#110106)),
 .UNSPECIFIED.,.F.,.F.,.F.)
B_SPLINE_SURFACE_WITH_KNOTS((2,2),(3,2,2,3),(0.710192959008352,1.),(0.280257803540344,
0.280433083165912,0.285714285714286,0.297961045722762),.UNSPECIFIED.)
GEOMETRIC_REPRESENTATION_ITEM()
RATIONAL_B_SPLINE_SURFACE(((0.996566619267863,0.996566619267863,0.996566619267863,
0.998146249162902,1.,0.995701274206111,0.992876621380142),(0.996566619267863,
0.996566619267863,0.996566619267863,0.998146249162902,1.,0.995701274206111,
0.992876621380142)))
REPRESENTATION_ITEM('')
SURFACE()
);
#970=(
BOUNDED_SURFACE()
B_SPLINE_SURFACE(1,2,((#110120,#110121,#110122),(#110123,#110124,#110125)),
 .UNSPECIFIED.,.F.,.F.,.F.)
B_SPLINE_SURFACE_WITH_KNOTS((2,2),(3,3),(0.710318915639497,1.),(0.435672122597671,
0.452924869174518),.UNSPECIFIED.)
GEOMETRIC_REPRESENTATION_ITEM()
RATIONAL_B_SPLINE_SURFACE(((0.995510721093621,0.990658873102333,0.988732477628005),
(0.995510721093621,0.990658873102333,0.988732477628005)))
REPRESENTATION_ITEM('')
SURFACE()
);
#971=(
BOUNDED_SURFACE()
B_SPLINE_SURFACE(1,2,((#110136,#110137,#110138,#110139,#110140,#110141,
#110142),(#110143,#110144,#110145,#110146,#110147,#110148,#110149)),
 .UNSPECIFIED.,.F.,.F.,.F.)
B_SPLINE_SURFACE_WITH_KNOTS((2,2),(3,2,2,3),(0.710192959007853,1.),(0.280257803540344,
0.280433083165912,0.285714285714286,0.297961045722762),.UNSPECIFIED.)
GEOMETRIC_REPRESENTATION_ITEM()
RATIONAL_B_SPLINE_SURFACE(((0.996566619267863,0.996566619267863,0.996566619267863,
0.998146249162902,1.,0.995701274206111,0.992876621380142),(0.996566619267863,
0.996566619267863,0.996566619267863,0.998146249162902,1.,0.995701274206111,
0.992876621380142)))
REPRESENTATION_ITEM('')
SURFACE()
);
#972=(
BOUNDED_SURFACE()
B_SPLINE_SURFACE(1,2,((#110163,#110164,#110165),(#110166,#110167,#110168)),
 .UNSPECIFIED.,.F.,.F.,.F.)
B_SPLINE_SURFACE_WITH_KNOTS((2,2),(3,3),(0.710318915639716,1.),(0.435672122597671,
0.452924869174518),.UNSPECIFIED.)
GEOMETRIC_REPRESENTATION_ITEM()
RATIONAL_B_SPLINE_SURFACE(((0.995510721093621,0.990658873102333,0.988732477628005),
(0.995510721093621,0.990658873102333,0.988732477628005)))
REPRESENTATION_ITEM('')
SURFACE()
);
#973=(
BOUNDED_SURFACE()
B_SPLINE_SURFACE(1,2,((#110179,#110180,#110181,#110182,#110183,#110184,
#110185),(#110186,#110187,#110188,#110189,#110190,#110191,#110192)),
 .UNSPECIFIED.,.F.,.F.,.F.)
B_SPLINE_SURFACE_WITH_KNOTS((2,2),(3,2,2,3),(0.71019295900808,1.),(0.280257803540343,
0.280433083165911,0.285714285714286,0.297961045722762),.UNSPECIFIED.)
GEOMETRIC_REPRESENTATION_ITEM()
RATIONAL_B_SPLINE_SURFACE(((0.996566619267862,0.996566619267862,0.996566619267862,
0.998146249162902,1.,0.995701274206111,0.992876621380142),(0.996566619267862,
0.996566619267862,0.996566619267862,0.998146249162902,1.,0.995701274206111,
0.992876621380142)))
REPRESENTATION_ITEM('')
SURFACE()
);
#974=(
BOUNDED_SURFACE()
B_SPLINE_SURFACE(1,2,((#110206,#110207,#110208),(#110209,#110210,#110211)),
 .UNSPECIFIED.,.F.,.F.,.F.)
B_SPLINE_SURFACE_WITH_KNOTS((2,2),(3,3),(0.710318915638671,1.),(0.435672122597671,
0.452924869174518),.UNSPECIFIED.)
GEOMETRIC_REPRESENTATION_ITEM()
RATIONAL_B_SPLINE_SURFACE(((0.995510721093621,0.990658873102333,0.988732477628005),
(0.995510721093621,0.990658873102333,0.988732477628005)))
REPRESENTATION_ITEM('')
SURFACE()
);
#975=(
BOUNDED_SURFACE()
B_SPLINE_SURFACE(1,2,((#110222,#110223,#110224,#110225,#110226,#110227,
#110228),(#110229,#110230,#110231,#110232,#110233,#110234,#110235)),
 .UNSPECIFIED.,.F.,.F.,.F.)
B_SPLINE_SURFACE_WITH_KNOTS((2,2),(3,2,2,3),(0.710192959007032,1.),(0.280257803540344,
0.280433083165912,0.285714285714286,0.297961045722762),.UNSPECIFIED.)
GEOMETRIC_REPRESENTATION_ITEM()
RATIONAL_B_SPLINE_SURFACE(((0.996566619267863,0.996566619267863,0.996566619267863,
0.998146249162902,1.,0.995701274206111,0.992876621380142),(0.996566619267863,
0.996566619267863,0.996566619267863,0.998146249162902,1.,0.995701274206111,
0.992876621380142)))
REPRESENTATION_ITEM('')
SURFACE()
);
#976=(
BOUNDED_SURFACE()
B_SPLINE_SURFACE(1,2,((#110249,#110250,#110251),(#110252,#110253,#110254)),
 .UNSPECIFIED.,.F.,.F.,.F.)
B_SPLINE_SURFACE_WITH_KNOTS((2,2),(3,3),(0.710318915639955,1.),(0.435672122597508,
0.452924869174518),.UNSPECIFIED.)
GEOMETRIC_REPRESENTATION_ITEM()
RATIONAL_B_SPLINE_SURFACE(((0.995510721093713,0.990658873102351,0.988732477628005),
(0.995510721093713,0.990658873102351,0.988732477628005)))
REPRESENTATION_ITEM('')
SURFACE()
);
#977=(
BOUNDED_SURFACE()
B_SPLINE_SURFACE(1,2,((#110265,#110266,#110267,#110268,#110269,#110270,
#110271),(#110272,#110273,#110274,#110275,#110276,#110277,#110278)),
 .UNSPECIFIED.,.F.,.F.,.F.)
B_SPLINE_SURFACE_WITH_KNOTS((2,2),(3,2,2,3),(0.710192959008314,1.),(0.280257803540344,
0.280433083165912,0.285714285714286,0.29796104572276),.UNSPECIFIED.)
GEOMETRIC_REPRESENTATION_ITEM()
RATIONAL_B_SPLINE_SURFACE(((0.996566619267863,0.996566619267863,0.996566619267863,
0.998146249162903,1.,0.995701274206112,0.992876621380143),(0.996566619267863,
0.996566619267863,0.996566619267863,0.998146249162903,1.,0.995701274206112,
0.992876621380143)))
REPRESENTATION_ITEM('')
SURFACE()
);
#978=(
BOUNDED_SURFACE()
B_SPLINE_SURFACE(1,2,((#110292,#110293,#110294),(#110295,#110296,#110297)),
 .UNSPECIFIED.,.F.,.F.,.F.)
B_SPLINE_SURFACE_WITH_KNOTS((2,2),(3,3),(0.710318915640075,1.),(0.435672122597671,
0.452924869174518),.UNSPECIFIED.)
GEOMETRIC_REPRESENTATION_ITEM()
RATIONAL_B_SPLINE_SURFACE(((0.995510721093621,0.990658873102333,0.988732477628005),
(0.995510721093621,0.990658873102333,0.988732477628005)))
REPRESENTATION_ITEM('')
SURFACE()
);
#979=(
BOUNDED_SURFACE()
B_SPLINE_SURFACE(1,2,((#110308,#110309,#110310,#110311,#110312,#110313,
#110314),(#110315,#110316,#110317,#110318,#110319,#110320,#110321)),
 .UNSPECIFIED.,.F.,.F.,.F.)
B_SPLINE_SURFACE_WITH_KNOTS((2,2),(3,2,2,3),(0.710192959008435,1.),(0.280257803540343,
0.280433083165911,0.285714285714286,0.297961045722762),.UNSPECIFIED.)
GEOMETRIC_REPRESENTATION_ITEM()
RATIONAL_B_SPLINE_SURFACE(((0.996566619267862,0.996566619267862,0.996566619267862,
0.998146249162902,1.,0.995701274206111,0.992876621380142),(0.996566619267862,
0.996566619267862,0.996566619267862,0.998146249162902,1.,0.995701274206111,
0.992876621380142)))
REPRESENTATION_ITEM('')
SURFACE()
);
#980=(
BOUNDED_SURFACE()
B_SPLINE_SURFACE(1,2,((#110335,#110336,#110337),(#110338,#110339,#110340)),
 .UNSPECIFIED.,.F.,.F.,.F.)
B_SPLINE_SURFACE_WITH_KNOTS((2,2),(3,3),(0.710318915639446,1.),(0.4356721225975,
0.452924869174518),.UNSPECIFIED.)
GEOMETRIC_REPRESENTATION_ITEM()
RATIONAL_B_SPLINE_SURFACE(((0.995510721093717,0.990658873102352,0.988732477628005),
(0.995510721093717,0.990658873102352,0.988732477628005)))
REPRESENTATION_ITEM('')
SURFACE()
);
#981=(
BOUNDED_SURFACE()
B_SPLINE_SURFACE(1,2,((#110351,#110352,#110353,#110354,#110355,#110356,
#110357),(#110358,#110359,#110360,#110361,#110362,#110363,#110364)),
 .UNSPECIFIED.,.F.,.F.,.F.)
B_SPLINE_SURFACE_WITH_KNOTS((2,2),(3,2,2,3),(0.710192959007802,1.),(0.280257803540344,
0.280433083165912,0.285714285714286,0.297961045722762),.UNSPECIFIED.)
GEOMETRIC_REPRESENTATION_ITEM()
RATIONAL_B_SPLINE_SURFACE(((0.996566619267863,0.996566619267863,0.996566619267863,
0.998146249162902,1.,0.995701274206111,0.992876621380142),(0.996566619267863,
0.996566619267863,0.996566619267863,0.998146249162902,1.,0.995701274206111,
0.992876621380142)))
REPRESENTATION_ITEM('')
SURFACE()
);
#982=(
BOUNDED_SURFACE()
B_SPLINE_SURFACE(1,2,((#110378,#110379,#110380),(#110381,#110382,#110383)),
 .UNSPECIFIED.,.F.,.F.,.F.)
B_SPLINE_SURFACE_WITH_KNOTS((2,2),(3,3),(0.71031891564008,1.),(0.435672122597573,
0.452924869174518),.UNSPECIFIED.)
GEOMETRIC_REPRESENTATION_ITEM()
RATIONAL_B_SPLINE_SURFACE(((0.995510721093677,0.990658873102344,0.988732477628005),
(0.995510721093677,0.990658873102344,0.988732477628005)))
REPRESENTATION_ITEM('')
SURFACE()
);
#983=(
BOUNDED_SURFACE()
B_SPLINE_SURFACE(1,2,((#110394,#110395,#110396,#110397,#110398,#110399,
#110400),(#110401,#110402,#110403,#110404,#110405,#110406,#110407)),
 .UNSPECIFIED.,.F.,.F.,.F.)
B_SPLINE_SURFACE_WITH_KNOTS((2,2),(3,2,2,3),(0.710192959008442,1.),(0.280257803540345,
0.280433083165913,0.285714285714286,0.297961045722762),.UNSPECIFIED.)
GEOMETRIC_REPRESENTATION_ITEM()
RATIONAL_B_SPLINE_SURFACE(((0.996566619267863,0.996566619267863,0.996566619267863,
0.998146249162903,1.,0.995701274206111,0.992876621380142),(0.996566619267863,
0.996566619267863,0.996566619267863,0.998146249162903,1.,0.995701274206111,
0.992876621380142)))
REPRESENTATION_ITEM('')
SURFACE()
);
#984=(
BOUNDED_SURFACE()
B_SPLINE_SURFACE(1,2,((#110421,#110422,#110423),(#110424,#110425,#110426)),
 .UNSPECIFIED.,.F.,.F.,.F.)
B_SPLINE_SURFACE_WITH_KNOTS((2,2),(3,3),(0.710318915638947,1.),(0.435672122597671,
0.452924869174518),.UNSPECIFIED.)
GEOMETRIC_REPRESENTATION_ITEM()
RATIONAL_B_SPLINE_SURFACE(((0.995510721093621,0.990658873102333,0.988732477628005),
(0.995510721093621,0.990658873102333,0.988732477628005)))
REPRESENTATION_ITEM('')
SURFACE()
);
#985=(
BOUNDED_SURFACE()
B_SPLINE_SURFACE(1,2,((#110437,#110438,#110439,#110440,#110441,#110442,
#110443),(#110444,#110445,#110446,#110447,#110448,#110449,#110450)),
 .UNSPECIFIED.,.F.,.F.,.F.)
B_SPLINE_SURFACE_WITH_KNOTS((2,2),(3,2,2,3),(0.710192959007306,1.),(0.280257803540345,
0.280433083165913,0.285714285714286,0.297961045722762),.UNSPECIFIED.)
GEOMETRIC_REPRESENTATION_ITEM()
RATIONAL_B_SPLINE_SURFACE(((0.996566619267863,0.996566619267863,0.996566619267863,
0.998146249162903,1.,0.995701274206111,0.992876621380142),(0.996566619267863,
0.996566619267863,0.996566619267863,0.998146249162903,1.,0.995701274206111,
0.992876621380142)))
REPRESENTATION_ITEM('')
SURFACE()
);
#986=(
BOUNDED_SURFACE()
B_SPLINE_SURFACE(1,2,((#110464,#110465,#110466),(#110467,#110468,#110469)),
 .UNSPECIFIED.,.F.,.F.,.F.)
B_SPLINE_SURFACE_WITH_KNOTS((2,2),(3,3),(0.710318915639103,1.),(0.435672122597161,
0.452924869174518),.UNSPECIFIED.)
GEOMETRIC_REPRESENTATION_ITEM()
RATIONAL_B_SPLINE_SURFACE(((0.995510721093908,0.99065887310239,0.988732477628006),
(0.995510721093908,0.99065887310239,0.988732477628006)))
REPRESENTATION_ITEM('')
SURFACE()
);
#987=(
BOUNDED_SURFACE()
B_SPLINE_SURFACE(1,2,((#110480,#110481,#110482,#110483,#110484,#110485,
#110486),(#110487,#110488,#110489,#110490,#110491,#110492,#110493)),
 .UNSPECIFIED.,.F.,.F.,.F.)
B_SPLINE_SURFACE_WITH_KNOTS((2,2),(3,2,2,3),(0.710192959007465,1.),(0.280257803540345,
0.280433083165913,0.285714285714286,0.29796104572276),.UNSPECIFIED.)
GEOMETRIC_REPRESENTATION_ITEM()
RATIONAL_B_SPLINE_SURFACE(((0.996566619267863,0.996566619267863,0.996566619267863,
0.998146249162903,1.,0.995701274206112,0.992876621380143),(0.996566619267863,
0.996566619267863,0.996566619267863,0.998146249162903,1.,0.995701274206112,
0.992876621380143)))
REPRESENTATION_ITEM('')
SURFACE()
);
#988=(
BOUNDED_SURFACE()
B_SPLINE_SURFACE(1,2,((#110507,#110508,#110509),(#110510,#110511,#110512)),
 .UNSPECIFIED.,.F.,.F.,.F.)
B_SPLINE_SURFACE_WITH_KNOTS((2,2),(3,3),(0.710318915638374,1.),(0.435672122597297,
0.452924869174625),.UNSPECIFIED.)
GEOMETRIC_REPRESENTATION_ITEM()
RATIONAL_B_SPLINE_SURFACE(((0.995510721093831,0.990658873102344,0.988732477627981),
(0.995510721093832,0.990658873102344,0.988732477627981)))
REPRESENTATION_ITEM('')
SURFACE()
);
#989=(
BOUNDED_SURFACE()
B_SPLINE_SURFACE(1,2,((#110523,#110524,#110525,#110526,#110527,#110528,
#110529),(#110530,#110531,#110532,#110533,#110534,#110535,#110536)),
 .UNSPECIFIED.,.F.,.F.,.F.)
B_SPLINE_SURFACE_WITH_KNOTS((2,2),(3,2,2,3),(0.710192959006739,1.),(0.280257803540345,
0.280433083165913,0.285714285714286,0.29796104572276),.UNSPECIFIED.)
GEOMETRIC_REPRESENTATION_ITEM()
RATIONAL_B_SPLINE_SURFACE(((0.996566619267863,0.996566619267863,0.996566619267863,
0.998146249162903,1.,0.995701274206112,0.992876621380143),(0.996566619267863,
0.996566619267863,0.996566619267863,0.998146249162903,1.,0.995701274206112,
0.992876621380143)))
REPRESENTATION_ITEM('')
SURFACE()
);
#990=(
BOUNDED_SURFACE()
B_SPLINE_SURFACE(1,2,((#110550,#110551,#110552),(#110553,#110554,#110555)),
 .UNSPECIFIED.,.F.,.F.,.F.)
B_SPLINE_SURFACE_WITH_KNOTS((2,2),(3,3),(0.710318915639878,1.),(0.435672122597669,
0.452924869174794),.UNSPECIFIED.)
GEOMETRIC_REPRESENTATION_ITEM()
RATIONAL_B_SPLINE_SURFACE(((0.995510721093622,0.990658873102255,0.988732477627944),
(0.995510721093622,0.990658873102255,0.988732477627944)))
REPRESENTATION_ITEM('')
SURFACE()
);
#991=(
BOUNDED_SURFACE()
B_SPLINE_SURFACE(1,2,((#110566,#110567,#110568,#110569,#110570,#110571,
#110572),(#110573,#110574,#110575,#110576,#110577,#110578,#110579)),
 .UNSPECIFIED.,.F.,.F.,.F.)
B_SPLINE_SURFACE_WITH_KNOTS((2,2),(3,2,2,3),(0.710192959008237,1.),(0.280257803540345,
0.280433083165913,0.285714285714286,0.297961045722762),.UNSPECIFIED.)
GEOMETRIC_REPRESENTATION_ITEM()
RATIONAL_B_SPLINE_SURFACE(((0.996566619267863,0.996566619267863,0.996566619267863,
0.998146249162903,1.,0.995701274206111,0.992876621380142),(0.996566619267863,
0.996566619267863,0.996566619267863,0.998146249162903,1.,0.995701274206111,
0.992876621380142)))
REPRESENTATION_ITEM('')
SURFACE()
);
#992=(
BOUNDED_SURFACE()
B_SPLINE_SURFACE(1,2,((#110593,#110594,#110595),(#110596,#110597,#110598)),
 .UNSPECIFIED.,.F.,.F.,.F.)
B_SPLINE_SURFACE_WITH_KNOTS((2,2),(3,3),(0.710318915638592,1.),(0.435672122597671,
0.452924869174518),.UNSPECIFIED.)
GEOMETRIC_REPRESENTATION_ITEM()
RATIONAL_B_SPLINE_SURFACE(((0.995510721093621,0.990658873102333,0.988732477628005),
(0.995510721093621,0.990658873102333,0.988732477628005)))
REPRESENTATION_ITEM('')
SURFACE()
);
#993=(
BOUNDED_SURFACE()
B_SPLINE_SURFACE(1,2,((#110609,#110610,#110611,#110612,#110613,#110614,
#110615),(#110616,#110617,#110618,#110619,#110620,#110621,#110622)),
 .UNSPECIFIED.,.F.,.F.,.F.)
B_SPLINE_SURFACE_WITH_KNOTS((2,2),(3,2,2,3),(0.710192959006951,1.),(0.280257803540345,
0.280433083165913,0.285714285714286,0.297961045722762),.UNSPECIFIED.)
GEOMETRIC_REPRESENTATION_ITEM()
RATIONAL_B_SPLINE_SURFACE(((0.996566619267863,0.996566619267863,0.996566619267863,
0.998146249162903,1.,0.995701274206111,0.992876621380142),(0.996566619267863,
0.996566619267863,0.996566619267863,0.998146249162903,1.,0.995701274206111,
0.992876621380142)))
REPRESENTATION_ITEM('')
SURFACE()
);
#994=(
BOUNDED_SURFACE()
B_SPLINE_SURFACE(1,2,((#110636,#110637,#110638),(#110639,#110640,#110641)),
 .UNSPECIFIED.,.F.,.F.,.F.)
B_SPLINE_SURFACE_WITH_KNOTS((2,2),(3,3),(0.710318915638846,1.),(0.435672122597539,
0.452924869174518),.UNSPECIFIED.)
GEOMETRIC_REPRESENTATION_ITEM()
RATIONAL_B_SPLINE_SURFACE(((0.995510721093696,0.990658873102347,0.988732477628005),
(0.995510721093696,0.990658873102347,0.988732477628005)))
REPRESENTATION_ITEM('')
SURFACE()
);
#995=(
BOUNDED_SURFACE()
B_SPLINE_SURFACE(1,2,((#110652,#110653,#110654,#110655,#110656,#110657,
#110658),(#110659,#110660,#110661,#110662,#110663,#110664,#110665)),
 .UNSPECIFIED.,.F.,.F.,.F.)
B_SPLINE_SURFACE_WITH_KNOTS((2,2),(3,2,2,3),(0.710192959007199,1.),(0.280257803540345,
0.280433083165913,0.285714285714286,0.297961045722762),.UNSPECIFIED.)
GEOMETRIC_REPRESENTATION_ITEM()
RATIONAL_B_SPLINE_SURFACE(((0.996566619267863,0.996566619267863,0.996566619267863,
0.998146249162903,1.,0.995701274206111,0.992876621380142),(0.996566619267863,
0.996566619267863,0.996566619267863,0.998146249162903,1.,0.995701274206111,
0.992876621380142)))
REPRESENTATION_ITEM('')
SURFACE()
);
#996=(
BOUNDED_SURFACE()
B_SPLINE_SURFACE(1,2,((#110679,#110680,#110681),(#110682,#110683,#110684)),
 .UNSPECIFIED.,.F.,.F.,.F.)
B_SPLINE_SURFACE_WITH_KNOTS((2,2),(3,3),(0.710318915639085,1.),(0.435672122597353,
0.452924869174518),.UNSPECIFIED.)
GEOMETRIC_REPRESENTATION_ITEM()
RATIONAL_B_SPLINE_SURFACE(((0.9955107210938,0.990658873102368,0.988732477628005),
(0.9955107210938,0.990658873102368,0.988732477628005)))
REPRESENTATION_ITEM('')
SURFACE()
);
#997=(
BOUNDED_SURFACE()
B_SPLINE_SURFACE(1,2,((#110695,#110696,#110697,#110698,#110699,#110700,
#110701),(#110702,#110703,#110704,#110705,#110706,#110707,#110708)),
 .UNSPECIFIED.,.F.,.F.,.F.)
B_SPLINE_SURFACE_WITH_KNOTS((2,2),(3,2,2,3),(0.71019295900744,1.),(0.280257803540346,
0.280433083165913,0.285714285714286,0.297961045722604),.UNSPECIFIED.)
GEOMETRIC_REPRESENTATION_ITEM()
RATIONAL_B_SPLINE_SURFACE(((0.996566619267863,0.996566619267863,0.996566619267863,
0.998146249162903,1.,0.995701274206166,0.992876621380215),(0.996566619267863,
0.996566619267863,0.996566619267863,0.998146249162903,1.,0.995701274206166,
0.992876621380215)))
REPRESENTATION_ITEM('')
SURFACE()
);
#998=(
BOUNDED_SURFACE()
B_SPLINE_SURFACE(1,2,((#110722,#110723,#110724),(#110725,#110726,#110727)),
 .UNSPECIFIED.,.F.,.F.,.F.)
B_SPLINE_SURFACE_WITH_KNOTS((2,2),(3,3),(0.710318915639152,1.),(0.435672122597622,
0.452924869174518),.UNSPECIFIED.)
GEOMETRIC_REPRESENTATION_ITEM()
RATIONAL_B_SPLINE_SURFACE(((0.995510721093649,0.990658873102338,0.988732477628005),
(0.995510721093649,0.990658873102338,0.988732477628005)))
REPRESENTATION_ITEM('')
SURFACE()
);
#999=(
BOUNDED_SURFACE()
B_SPLINE_SURFACE(1,2,((#110738,#110739,#110740,#110741,#110742,#110743,
#110744),(#110745,#110746,#110747,#110748,#110749,#110750,#110751)),
 .UNSPECIFIED.,.F.,.F.,.F.)
B_SPLINE_SURFACE_WITH_KNOTS((2,2),(3,2,2,3),(0.710192959007518,1.),(0.280257803540345,
0.280433083165913,0.285714285714286,0.297961045722762),.UNSPECIFIED.)
GEOMETRIC_REPRESENTATION_ITEM()
RATIONAL_B_SPLINE_SURFACE(((0.996566619267863,0.996566619267863,0.996566619267863,
0.998146249162903,1.,0.995701274206111,0.992876621380142),(0.996566619267863,
0.996566619267863,0.996566619267863,0.998146249162903,1.,0.995701274206111,
0.992876621380142)))
REPRESENTATION_ITEM('')
SURFACE()
);
#1000=(
BOUNDED_SURFACE()
B_SPLINE_SURFACE(1,2,((#110765,#110766,#110767),(#110768,#110769,#110770)),
 .UNSPECIFIED.,.F.,.F.,.F.)
B_SPLINE_SURFACE_WITH_KNOTS((2,2),(3,3),(0.710318915638835,1.),(0.4356721225973,
0.452924869174518),.UNSPECIFIED.)
GEOMETRIC_REPRESENTATION_ITEM()
RATIONAL_B_SPLINE_SURFACE(((0.99551072109383,0.990658873102374,0.988732477628005),
(0.99551072109383,0.990658873102374,0.988732477628005)))
REPRESENTATION_ITEM('')
SURFACE()
);
#1001=(
BOUNDED_SURFACE()
B_SPLINE_SURFACE(1,2,((#110781,#110782,#110783,#110784,#110785,#110786,
#110787),(#110788,#110789,#110790,#110791,#110792,#110793,#110794)),
 .UNSPECIFIED.,.F.,.F.,.F.)
B_SPLINE_SURFACE_WITH_KNOTS((2,2),(3,2,2,3),(0.710192959006289,1.),(0.280257803540335,
0.280433083165902,0.285714285714286,0.297961045722673),.UNSPECIFIED.)
GEOMETRIC_REPRESENTATION_ITEM()
RATIONAL_B_SPLINE_SURFACE(((0.996566619267857,0.996566619267857,0.996566619267857,
0.998146249162899,1.,0.995701274206142,0.992876621380183),(0.996566619267857,
0.996566619267857,0.996566619267857,0.998146249162899,1.,0.995701274206142,
0.992876621380183)))
REPRESENTATION_ITEM('')
SURFACE()
);
#1002=(
BOUNDED_SURFACE()
B_SPLINE_SURFACE(1,2,((#110808,#110809,#110810),(#110811,#110812,#110813)),
 .UNSPECIFIED.,.F.,.F.,.F.)
B_SPLINE_SURFACE_WITH_KNOTS((2,2),(3,3),(0.710318915638985,1.),(0.435672122597532,
0.452924869174518),.UNSPECIFIED.)
GEOMETRIC_REPRESENTATION_ITEM()
RATIONAL_B_SPLINE_SURFACE(((0.9955107210937,0.990658873102348,0.988732477628005),
(0.9955107210937,0.990658873102348,0.988732477628005)))
REPRESENTATION_ITEM('')
SURFACE()
);
#1003=(
BOUNDED_SURFACE()
B_SPLINE_SURFACE(1,2,((#110824,#110825,#110826,#110827,#110828,#110829,
#110830),(#110831,#110832,#110833,#110834,#110835,#110836,#110837)),
 .UNSPECIFIED.,.F.,.F.,.F.)
B_SPLINE_SURFACE_WITH_KNOTS((2,2),(3,2,2,3),(0.710192959007348,1.),(0.280257803540345,
0.280433083165913,0.285714285714286,0.29796104572276),.UNSPECIFIED.)
GEOMETRIC_REPRESENTATION_ITEM()
RATIONAL_B_SPLINE_SURFACE(((0.996566619267863,0.996566619267863,0.996566619267863,
0.998146249162903,1.,0.995701274206112,0.992876621380143),(0.996566619267863,
0.996566619267863,0.996566619267863,0.998146249162903,1.,0.995701274206112,
0.992876621380143)))
REPRESENTATION_ITEM('')
SURFACE()
);
#1004=(
BOUNDED_SURFACE()
B_SPLINE_SURFACE(1,2,((#110851,#110852,#110853),(#110854,#110855,#110856)),
 .UNSPECIFIED.,.F.,.F.,.F.)
B_SPLINE_SURFACE_WITH_KNOTS((2,2),(3,3),(0.710318915638962,1.),(0.435672122597216,
0.452924869174518),.UNSPECIFIED.)
GEOMETRIC_REPRESENTATION_ITEM()
RATIONAL_B_SPLINE_SURFACE(((0.995510721093877,0.990658873102383,0.988732477628005),
(0.995510721093877,0.990658873102383,0.988732477628005)))
REPRESENTATION_ITEM('')
SURFACE()
);
#1005=(
BOUNDED_SURFACE()
B_SPLINE_SURFACE(1,2,((#110867,#110868,#110869,#110870,#110871,#110872,
#110873),(#110874,#110875,#110876,#110877,#110878,#110879,#110880)),
 .UNSPECIFIED.,.F.,.F.,.F.)
B_SPLINE_SURFACE_WITH_KNOTS((2,2),(3,2,2,3),(0.710192959007327,1.),(0.280257803540346,
0.280433083165913,0.285714285714286,0.297961045722661),.UNSPECIFIED.)
GEOMETRIC_REPRESENTATION_ITEM()
RATIONAL_B_SPLINE_SURFACE(((0.996566619267863,0.996566619267863,0.996566619267863,
0.998146249162903,1.,0.995701274206146,0.992876621380189),(0.996566619267863,
0.996566619267863,0.996566619267863,0.998146249162903,1.,0.995701274206146,
0.992876621380189)))
REPRESENTATION_ITEM('')
SURFACE()
);
#1006=(
BOUNDED_SURFACE()
B_SPLINE_SURFACE(1,2,((#110894,#110895,#110896,#110897,#110898),(#110899,
#110900,#110901,#110902,#110903)),.UNSPECIFIED.,.F.,.F.,.F.)
B_SPLINE_SURFACE_WITH_KNOTS((2,2),(3,2,3),(0.709594768913623,1.),(0.40044464506204,
0.401042835325431,0.418415696246127),.UNSPECIFIED.)
GEOMETRIC_REPRESENTATION_ITEM()
RATIONAL_B_SPLINE_SURFACE(((0.988122504062136,0.988122504062136,0.988122504062136,
0.989520169850094,0.993884164197535),(0.988122504062136,0.988122504062136,
0.988122504062136,0.989520169850094,0.993884164197535)))
REPRESENTATION_ITEM('')
SURFACE()
);
#1007=(
BOUNDED_SURFACE()
B_SPLINE_SURFACE(1,2,((#110912,#110913,#110914),(#110915,#110916,#110917)),
 .UNSPECIFIED.,.F.,.F.,.F.)
B_SPLINE_SURFACE_WITH_KNOTS((2,2),(3,3),(0.710318915639747,1.),(0.314840108491245,
0.332069149066961),.UNSPECIFIED.)
GEOMETRIC_REPRESENTATION_ITEM()
RATIONAL_B_SPLINE_SURFACE(((0.98789057959819,0.986774945528852,0.988576730109528),
(0.98789057959819,0.986774945528852,0.988576730109528)))
REPRESENTATION_ITEM('')
SURFACE()
);
#1008=(
BOUNDED_SURFACE()
B_SPLINE_SURFACE(1,2,((#110919,#110920,#110921,#110922,#110923),(#110924,
#110925,#110926,#110927,#110928)),.UNSPECIFIED.,.F.,.F.,.F.)
B_SPLINE_SURFACE_WITH_KNOTS((2,2),(3,2,3),(0.709594768940214,1.),(0.400444645034863,
0.401042835325431,0.418415696246122),.UNSPECIFIED.)
GEOMETRIC_REPRESENTATION_ITEM()
RATIONAL_B_SPLINE_SURFACE(((0.988122504062136,0.988122504062136,0.988122504062136,
0.989520169850094,0.993884164197532),(0.988122504062136,0.988122504062136,
0.988122504062136,0.989520169850094,0.993884164197532)))
REPRESENTATION_ITEM('')
SURFACE()
);
#1009=(
BOUNDED_SURFACE()
B_SPLINE_SURFACE(1,2,((#110937,#110938,#110939),(#110940,#110941,#110942)),
 .UNSPECIFIED.,.F.,.F.,.F.)
B_SPLINE_SURFACE_WITH_KNOTS((2,2),(3,3),(0.710318915639637,1.),(0.314840108491246,
0.332069149066804),.UNSPECIFIED.)
GEOMETRIC_REPRESENTATION_ITEM()
RATIONAL_B_SPLINE_SURFACE(((0.98789057959819,0.986774945528862,0.988576730109495),
(0.98789057959819,0.986774945528862,0.988576730109495)))
REPRESENTATION_ITEM('')
SURFACE()
);
#1010=(
BOUNDED_SURFACE()
B_SPLINE_SURFACE(1,2,((#110944,#110945,#110946,#110947,#110948),(#110949,
#110950,#110951,#110952,#110953)),.UNSPECIFIED.,.F.,.F.,.F.)
B_SPLINE_SURFACE_WITH_KNOTS((2,2),(3,2,3),(0.709594768922229,1.),(0.400444645017343,
0.40104283532543,0.418415696246122),.UNSPECIFIED.)
GEOMETRIC_REPRESENTATION_ITEM()
RATIONAL_B_SPLINE_SURFACE(((0.988122504062135,0.988122504062135,0.988122504062135,
0.989520169850094,0.993884164197532),(0.988122504062135,0.988122504062135,
0.988122504062135,0.989520169850094,0.993884164197532)))
REPRESENTATION_ITEM('')
SURFACE()
);
#1011=(
BOUNDED_SURFACE()
B_SPLINE_SURFACE(1,2,((#110962,#110963,#110964),(#110965,#110966,#110967)),
 .UNSPECIFIED.,.F.,.F.,.F.)
B_SPLINE_SURFACE_WITH_KNOTS((2,2),(3,3),(0.710318915638961,1.),(0.314840108491246,
0.332069149066804),.UNSPECIFIED.)
GEOMETRIC_REPRESENTATION_ITEM()
RATIONAL_B_SPLINE_SURFACE(((0.98789057959819,0.986774945528862,0.988576730109495),
(0.98789057959819,0.986774945528862,0.988576730109495)))
REPRESENTATION_ITEM('')
SURFACE()
);
#1012=(
BOUNDED_SURFACE()
B_SPLINE_SURFACE(1,2,((#110969,#110970,#110971,#110972,#110973),(#110974,
#110975,#110976,#110977,#110978)),.UNSPECIFIED.,.F.,.F.,.F.)
B_SPLINE_SURFACE_WITH_KNOTS((2,2),(3,2,3),(0.709594768914856,1.),(0.400444645010268,
0.401042835325429,0.418415696246123),.UNSPECIFIED.)
GEOMETRIC_REPRESENTATION_ITEM()
RATIONAL_B_SPLINE_SURFACE(((0.988122504062135,0.988122504062135,0.988122504062135,
0.989520169850093,0.993884164197532),(0.988122504062135,0.988122504062135,
0.988122504062135,0.989520169850093,0.993884164197532)))
REPRESENTATION_ITEM('')
SURFACE()
);
#1013=(
BOUNDED_SURFACE()
B_SPLINE_SURFACE(1,2,((#110987,#110988,#110989),(#110990,#110991,#110992)),
 .UNSPECIFIED.,.F.,.F.,.F.)
B_SPLINE_SURFACE_WITH_KNOTS((2,2),(3,3),(0.710318915639114,1.),(0.314840108491246,
0.332069149066804),.UNSPECIFIED.)
GEOMETRIC_REPRESENTATION_ITEM()
RATIONAL_B_SPLINE_SURFACE(((0.98789057959819,0.986774945528862,0.988576730109495),
(0.98789057959819,0.986774945528862,0.988576730109495)))
REPRESENTATION_ITEM('')
SURFACE()
);
#1014=(
BOUNDED_SURFACE()
B_SPLINE_SURFACE(1,2,((#110994,#110995,#110996,#110997,#110998),(#110999,
#111000,#111001,#111002,#111003)),.UNSPECIFIED.,.F.,.F.,.F.)
B_SPLINE_SURFACE_WITH_KNOTS((2,2),(3,2,3),(0.70959476892646,1.),(0.40044464502156,
0.40104283532543,0.418415696246148),.UNSPECIFIED.)
GEOMETRIC_REPRESENTATION_ITEM()
RATIONAL_B_SPLINE_SURFACE(((0.988122504062136,0.988122504062136,0.988122504062136,
0.989520169850096,0.993884164197545),(0.988122504062135,0.988122504062135,
0.988122504062135,0.989520169850095,0.993884164197545)))
REPRESENTATION_ITEM('')
SURFACE()
);
#1015=(
BOUNDED_SURFACE()
B_SPLINE_SURFACE(1,2,((#111012,#111013,#111014),(#111015,#111016,#111017)),
 .UNSPECIFIED.,.F.,.F.,.F.)
B_SPLINE_SURFACE_WITH_KNOTS((2,2),(3,3),(0.710318915639138,1.),(0.314840108491246,
0.332069149066804),.UNSPECIFIED.)
GEOMETRIC_REPRESENTATION_ITEM()
RATIONAL_B_SPLINE_SURFACE(((0.98789057959819,0.986774945528862,0.988576730109495),
(0.98789057959819,0.986774945528862,0.988576730109495)))
REPRESENTATION_ITEM('')
SURFACE()
);
#1016=(
BOUNDED_SURFACE()
B_SPLINE_SURFACE(1,2,((#111019,#111020,#111021,#111022,#111023),(#111024,
#111025,#111026,#111027,#111028)),.UNSPECIFIED.,.F.,.F.,.F.)
B_SPLINE_SURFACE_WITH_KNOTS((2,2),(3,2,3),(0.709594768882625,1.),(0.400444645032233,
0.401042835325431,0.418415696246122),.UNSPECIFIED.)
GEOMETRIC_REPRESENTATION_ITEM()
RATIONAL_B_SPLINE_SURFACE(((0.988122504062136,0.988122504062136,0.988122504062136,
0.989520169850094,0.993884164197532),(0.988122504062136,0.988122504062136,
0.988122504062136,0.989520169850094,0.993884164197532)))
REPRESENTATION_ITEM('')
SURFACE()
);
#1017=(
BOUNDED_SURFACE()
B_SPLINE_SURFACE(1,2,((#111037,#111038,#111039),(#111040,#111041,#111042)),
 .UNSPECIFIED.,.F.,.F.,.F.)
B_SPLINE_SURFACE_WITH_KNOTS((2,2),(3,3),(0.710318915638967,1.),(0.314840108491246,
0.332069149066804),.UNSPECIFIED.)
GEOMETRIC_REPRESENTATION_ITEM()
RATIONAL_B_SPLINE_SURFACE(((0.98789057959819,0.986774945528862,0.988576730109495),
(0.98789057959819,0.986774945528862,0.988576730109495)))
REPRESENTATION_ITEM('')
SURFACE()
);
#1018=(
BOUNDED_SURFACE()
B_SPLINE_SURFACE(1,2,((#111044,#111045,#111046,#111047,#111048),(#111049,
#111050,#111051,#111052,#111053)),.UNSPECIFIED.,.F.,.F.,.F.)
B_SPLINE_SURFACE_WITH_KNOTS((2,2),(3,2,3),(0.709594768927658,1.),(0.40044464502204,
0.401042835325431,0.418415696246123),.UNSPECIFIED.)
GEOMETRIC_REPRESENTATION_ITEM()
RATIONAL_B_SPLINE_SURFACE(((0.988122504062135,0.988122504062135,0.988122504062135,
0.989520169850094,0.993884164197532),(0.988122504062136,0.988122504062136,
0.988122504062136,0.989520169850094,0.993884164197532)))
REPRESENTATION_ITEM('')
SURFACE()
);
#1019=(
BOUNDED_SURFACE()
B_SPLINE_SURFACE(1,2,((#111062,#111063,#111064),(#111065,#111066,#111067)),
 .UNSPECIFIED.,.F.,.F.,.F.)
B_SPLINE_SURFACE_WITH_KNOTS((2,2),(3,3),(0.710318915639904,1.),(0.314840108491246,
0.332069149066804),.UNSPECIFIED.)
GEOMETRIC_REPRESENTATION_ITEM()
RATIONAL_B_SPLINE_SURFACE(((0.98789057959819,0.986774945528862,0.988576730109495),
(0.98789057959819,0.986774945528862,0.988576730109495)))
REPRESENTATION_ITEM('')
SURFACE()
);
#1020=(
BOUNDED_SURFACE()
B_SPLINE_SURFACE(1,2,((#111069,#111070,#111071,#111072,#111073),(#111074,
#111075,#111076,#111077,#111078)),.UNSPECIFIED.,.F.,.F.,.F.)
B_SPLINE_SURFACE_WITH_KNOTS((2,2),(3,2,3),(0.709594768892998,1.),(0.400444645041438,
0.401042835325428,0.418415696246122),.UNSPECIFIED.)
GEOMETRIC_REPRESENTATION_ITEM()
RATIONAL_B_SPLINE_SURFACE(((0.988122504062135,0.988122504062135,0.988122504062135,
0.989520169850093,0.993884164197532),(0.988122504062135,0.988122504062135,
0.988122504062135,0.989520169850093,0.993884164197532)))
REPRESENTATION_ITEM('')
SURFACE()
);
#1021=(
BOUNDED_SURFACE()
B_SPLINE_SURFACE(1,2,((#111087,#111088,#111089),(#111090,#111091,#111092)),
 .UNSPECIFIED.,.F.,.F.,.F.)
B_SPLINE_SURFACE_WITH_KNOTS((2,2),(3,3),(0.710318915639899,1.),(0.314840108491246,
0.332069149066804),.UNSPECIFIED.)
GEOMETRIC_REPRESENTATION_ITEM()
RATIONAL_B_SPLINE_SURFACE(((0.98789057959819,0.986774945528862,0.988576730109495),
(0.98789057959819,0.986774945528862,0.988576730109495)))
REPRESENTATION_ITEM('')
SURFACE()
);
#1022=(
BOUNDED_SURFACE()
B_SPLINE_SURFACE(1,2,((#111094,#111095,#111096,#111097,#111098),(#111099,
#111100,#111101,#111102,#111103)),.UNSPECIFIED.,.F.,.F.,.F.)
B_SPLINE_SURFACE_WITH_KNOTS((2,2),(3,2,3),(0.709594768879046,1.),(0.400444645027766,
0.401042835325429,0.418415696246122),.UNSPECIFIED.)
GEOMETRIC_REPRESENTATION_ITEM()
RATIONAL_B_SPLINE_SURFACE(((0.988122504062135,0.988122504062135,0.988122504062135,
0.989520169850093,0.993884164197532),(0.988122504062135,0.988122504062135,
0.988122504062135,0.989520169850093,0.993884164197532)))
REPRESENTATION_ITEM('')
SURFACE()
);
#1023=(
BOUNDED_SURFACE()
B_SPLINE_SURFACE(1,2,((#111112,#111113,#111114),(#111115,#111116,#111117)),
 .UNSPECIFIED.,.F.,.F.,.F.)
B_SPLINE_SURFACE_WITH_KNOTS((2,2),(3,3),(0.710318915639792,1.),(0.314840108491246,
0.332069149066804),.UNSPECIFIED.)
GEOMETRIC_REPRESENTATION_ITEM()
RATIONAL_B_SPLINE_SURFACE(((0.98789057959819,0.986774945528862,0.988576730109495),
(0.98789057959819,0.986774945528862,0.988576730109495)))
REPRESENTATION_ITEM('')
SURFACE()
);
#1024=(
BOUNDED_SURFACE()
B_SPLINE_SURFACE(1,2,((#111119,#111120,#111121,#111122,#111123),(#111124,
#111125,#111126,#111127,#111128)),.UNSPECIFIED.,.F.,.F.,.F.)
B_SPLINE_SURFACE_WITH_KNOTS((2,2),(3,2,3),(0.709594768914364,1.),(0.400444645009116,
0.401042835325428,0.418415696246123),.UNSPECIFIED.)
GEOMETRIC_REPRESENTATION_ITEM()
RATIONAL_B_SPLINE_SURFACE(((0.988122504062135,0.988122504062135,0.988122504062135,
0.989520169850093,0.993884164197532),(0.988122504062135,0.988122504062135,
0.988122504062135,0.989520169850093,0.993884164197532)))
REPRESENTATION_ITEM('')
SURFACE()
);
#1025=(
BOUNDED_SURFACE()
B_SPLINE_SURFACE(1,2,((#111137,#111138,#111139),(#111140,#111141,#111142)),
 .UNSPECIFIED.,.F.,.F.,.F.)
B_SPLINE_SURFACE_WITH_KNOTS((2,2),(3,3),(0.710318915639852,1.),(0.314840108491245,
0.332069149066961),.UNSPECIFIED.)
GEOMETRIC_REPRESENTATION_ITEM()
RATIONAL_B_SPLINE_SURFACE(((0.98789057959819,0.986774945528852,0.988576730109528),
(0.98789057959819,0.986774945528852,0.988576730109528)))
REPRESENTATION_ITEM('')
SURFACE()
);
#1026=(
BOUNDED_SURFACE()
B_SPLINE_SURFACE(1,2,((#111144,#111145,#111146,#111147,#111148),(#111149,
#111150,#111151,#111152,#111153)),.UNSPECIFIED.,.F.,.F.,.F.)
B_SPLINE_SURFACE_WITH_KNOTS((2,2),(3,2,3),(0.709594768913958,1.),(0.40044464500846,
0.401042835325429,0.418415696246123),.UNSPECIFIED.)
GEOMETRIC_REPRESENTATION_ITEM()
RATIONAL_B_SPLINE_SURFACE(((0.988122504062135,0.988122504062135,0.988122504062135,
0.989520169850093,0.993884164197532),(0.988122504062135,0.988122504062135,
0.988122504062135,0.989520169850093,0.993884164197532)))
REPRESENTATION_ITEM('')
SURFACE()
);
#1027=(
BOUNDED_SURFACE()
B_SPLINE_SURFACE(1,2,((#111162,#111163,#111164),(#111165,#111166,#111167)),
 .UNSPECIFIED.,.F.,.F.,.F.)
B_SPLINE_SURFACE_WITH_KNOTS((2,2),(3,3),(0.710318915639882,1.),(0.314840108491246,
0.332069149066805),.UNSPECIFIED.)
GEOMETRIC_REPRESENTATION_ITEM()
RATIONAL_B_SPLINE_SURFACE(((0.98789057959819,0.986774945528862,0.988576730109495),
(0.98789057959819,0.986774945528862,0.988576730109495)))
REPRESENTATION_ITEM('')
SURFACE()
);
#1028=(
BOUNDED_SURFACE()
B_SPLINE_SURFACE(1,2,((#111169,#111170,#111171,#111172,#111173),(#111174,
#111175,#111176,#111177,#111178)),.UNSPECIFIED.,.F.,.F.,.F.)
B_SPLINE_SURFACE_WITH_KNOTS((2,2),(3,2,3),(0.709594768896135,1.),(0.400444645043879,
0.401042835325428,0.418415696246123),.UNSPECIFIED.)
GEOMETRIC_REPRESENTATION_ITEM()
RATIONAL_B_SPLINE_SURFACE(((0.988122504062135,0.988122504062135,0.988122504062135,
0.989520169850093,0.993884164197532),(0.988122504062135,0.988122504062135,
0.988122504062135,0.989520169850093,0.993884164197532)))
REPRESENTATION_ITEM('')
SURFACE()
);
#1029=(
BOUNDED_SURFACE()
B_SPLINE_SURFACE(1,2,((#111187,#111188,#111189),(#111190,#111191,#111192)),
 .UNSPECIFIED.,.F.,.F.,.F.)
B_SPLINE_SURFACE_WITH_KNOTS((2,2),(3,3),(0.710318915639927,1.),(0.314840108491246,
0.332069149066805),.UNSPECIFIED.)
GEOMETRIC_REPRESENTATION_ITEM()
RATIONAL_B_SPLINE_SURFACE(((0.98789057959819,0.986774945528862,0.988576730109495),
(0.98789057959819,0.986774945528862,0.988576730109495)))
REPRESENTATION_ITEM('')
SURFACE()
);
#1030=(
BOUNDED_SURFACE()
B_SPLINE_SURFACE(1,2,((#111194,#111195,#111196,#111197,#111198),(#111199,
#111200,#111201,#111202,#111203)),.UNSPECIFIED.,.F.,.F.,.F.)
B_SPLINE_SURFACE_WITH_KNOTS((2,2),(3,2,3),(0.709594768891415,1.),(0.400444645039748,
0.401042835325431,0.418415696246122),.UNSPECIFIED.)
GEOMETRIC_REPRESENTATION_ITEM()
RATIONAL_B_SPLINE_SURFACE(((0.988122504062136,0.988122504062136,0.988122504062136,
0.989520169850094,0.993884164197532),(0.988122504062136,0.988122504062136,
0.988122504062136,0.989520169850094,0.993884164197532)))
REPRESENTATION_ITEM('')
SURFACE()
);
#1031=(
BOUNDED_SURFACE()
B_SPLINE_SURFACE(1,2,((#111212,#111213,#111214),(#111215,#111216,#111217)),
 .UNSPECIFIED.,.F.,.F.,.F.)
B_SPLINE_SURFACE_WITH_KNOTS((2,2),(3,3),(0.710318915640067,1.),(0.314840108491246,
0.332069149066804),.UNSPECIFIED.)
GEOMETRIC_REPRESENTATION_ITEM()
RATIONAL_B_SPLINE_SURFACE(((0.98789057959819,0.986774945528862,0.988576730109495),
(0.98789057959819,0.986774945528862,0.988576730109495)))
REPRESENTATION_ITEM('')
SURFACE()
);
#1032=(
BOUNDED_SURFACE()
B_SPLINE_SURFACE(1,2,((#111219,#111220,#111221,#111222,#111223),(#111224,
#111225,#111226,#111227,#111228)),.UNSPECIFIED.,.F.,.F.,.F.)
B_SPLINE_SURFACE_WITH_KNOTS((2,2),(3,2,3),(0.709594768879615,1.),(0.400444644973927,
0.40104283532543,0.418415696246122),.UNSPECIFIED.)
GEOMETRIC_REPRESENTATION_ITEM()
RATIONAL_B_SPLINE_SURFACE(((0.988122504062136,0.988122504062136,0.988122504062136,
0.989520169850094,0.993884164197532),(0.988122504062135,0.988122504062135,
0.988122504062135,0.989520169850094,0.993884164197532)))
REPRESENTATION_ITEM('')
SURFACE()
);
#1033=(
BOUNDED_SURFACE()
B_SPLINE_SURFACE(1,2,((#111237,#111238,#111239),(#111240,#111241,#111242)),
 .UNSPECIFIED.,.F.,.F.,.F.)
B_SPLINE_SURFACE_WITH_KNOTS((2,2),(3,3),(0.710318915640078,1.),(0.314840108491246,
0.332069149066804),.UNSPECIFIED.)
GEOMETRIC_REPRESENTATION_ITEM()
RATIONAL_B_SPLINE_SURFACE(((0.98789057959819,0.986774945528862,0.988576730109495),
(0.98789057959819,0.986774945528862,0.988576730109495)))
REPRESENTATION_ITEM('')
SURFACE()
);
#1034=(
BOUNDED_SURFACE()
B_SPLINE_SURFACE(1,2,((#111244,#111245,#111246,#111247,#111248),(#111249,
#111250,#111251,#111252,#111253)),.UNSPECIFIED.,.F.,.F.,.F.)
B_SPLINE_SURFACE_WITH_KNOTS((2,2),(3,2,3),(0.709961012046059,1.),(0.400810888140328,
0.401042835325431,0.418415696246122),.UNSPECIFIED.)
GEOMETRIC_REPRESENTATION_ITEM()
RATIONAL_B_SPLINE_SURFACE(((0.988122504062135,0.988122504062135,0.988122504062135,
0.989520169850094,0.993884164197532),(0.988122504062135,0.988122504062135,
0.988122504062135,0.989520169850094,0.993884164197532)))
REPRESENTATION_ITEM('')
SURFACE()
);
#1035=(
BOUNDED_SURFACE()
B_SPLINE_SURFACE(1,2,((#111262,#111263,#111264),(#111265,#111266,#111267)),
 .UNSPECIFIED.,.F.,.F.,.F.)
B_SPLINE_SURFACE_WITH_KNOTS((2,2),(3,3),(0.710318915640071,1.),(0.314840108491246,
0.332069149066804),.UNSPECIFIED.)
GEOMETRIC_REPRESENTATION_ITEM()
RATIONAL_B_SPLINE_SURFACE(((0.98789057959819,0.986774945528862,0.988576730109495),
(0.98789057959819,0.986774945528862,0.988576730109495)))
REPRESENTATION_ITEM('')
SURFACE()
);
#1036=(
BOUNDED_SURFACE()
B_SPLINE_SURFACE(1,2,((#111269,#111270,#111271,#111272,#111273),(#111274,
#111275,#111276,#111277,#111278)),.UNSPECIFIED.,.F.,.F.,.F.)
B_SPLINE_SURFACE_WITH_KNOTS((2,2),(3,2,3),(0.709594768954711,1.),(0.400444645048674,
0.401042835325431,0.418415696246122),.UNSPECIFIED.)
GEOMETRIC_REPRESENTATION_ITEM()
RATIONAL_B_SPLINE_SURFACE(((0.988122504062136,0.988122504062136,0.988122504062136,
0.989520169850094,0.993884164197532),(0.988122504062135,0.988122504062135,
0.988122504062135,0.989520169850094,0.993884164197532)))
REPRESENTATION_ITEM('')
SURFACE()
);
#1037=(
BOUNDED_SURFACE()
B_SPLINE_SURFACE(1,2,((#111287,#111288,#111289),(#111290,#111291,#111292)),
 .UNSPECIFIED.,.F.,.F.,.F.)
B_SPLINE_SURFACE_WITH_KNOTS((2,2),(3,3),(0.71031891564008,1.),(0.314840108491246,
0.332069149066805),.UNSPECIFIED.)
GEOMETRIC_REPRESENTATION_ITEM()
RATIONAL_B_SPLINE_SURFACE(((0.98789057959819,0.986774945528862,0.988576730109495),
(0.98789057959819,0.986774945528862,0.988576730109495)))
REPRESENTATION_ITEM('')
SURFACE()
);
#1038=(
BOUNDED_SURFACE()
B_SPLINE_SURFACE(1,2,((#111294,#111295,#111296,#111297,#111298),(#111299,
#111300,#111301,#111302,#111303)),.UNSPECIFIED.,.F.,.F.,.F.)
B_SPLINE_SURFACE_WITH_KNOTS((2,2),(3,2,3),(0.709594768929927,1.),(0.400444645024341,
0.401042835325431,0.418415696246123),.UNSPECIFIED.)
GEOMETRIC_REPRESENTATION_ITEM()
RATIONAL_B_SPLINE_SURFACE(((0.988122504062136,0.988122504062136,0.988122504062136,
0.989520169850094,0.993884164197532),(0.988122504062136,0.988122504062136,
0.988122504062136,0.989520169850094,0.993884164197532)))
REPRESENTATION_ITEM('')
SURFACE()
);
#1039=(
BOUNDED_SURFACE()
B_SPLINE_SURFACE(1,2,((#111312,#111313,#111314),(#111315,#111316,#111317)),
 .UNSPECIFIED.,.F.,.F.,.F.)
B_SPLINE_SURFACE_WITH_KNOTS((2,2),(3,3),(0.710318915640074,1.),(0.314840108491246,
0.332069149066805),.UNSPECIFIED.)
GEOMETRIC_REPRESENTATION_ITEM()
RATIONAL_B_SPLINE_SURFACE(((0.98789057959819,0.986774945528862,0.988576730109495),
(0.98789057959819,0.986774945528862,0.988576730109495)))
REPRESENTATION_ITEM('')
SURFACE()
);
#1040=(
BOUNDED_SURFACE()
B_SPLINE_SURFACE(1,2,((#111319,#111320,#111321,#111322,#111323),(#111324,
#111325,#111326,#111327,#111328)),.UNSPECIFIED.,.F.,.F.,.F.)
B_SPLINE_SURFACE_WITH_KNOTS((2,2),(3,2,3),(0.709594768925206,1.),(0.400444645019135,
0.401042835325431,0.418415696246122),.UNSPECIFIED.)
GEOMETRIC_REPRESENTATION_ITEM()
RATIONAL_B_SPLINE_SURFACE(((0.988122504062136,0.988122504062136,0.988122504062136,
0.989520169850094,0.993884164197532),(0.988122504062136,0.988122504062136,
0.988122504062136,0.989520169850094,0.993884164197532)))
REPRESENTATION_ITEM('')
SURFACE()
);
#1041=(
BOUNDED_SURFACE()
B_SPLINE_SURFACE(1,2,((#111337,#111338,#111339),(#111340,#111341,#111342)),
 .UNSPECIFIED.,.F.,.F.,.F.)
B_SPLINE_SURFACE_WITH_KNOTS((2,2),(3,3),(0.71031891563997,1.),(0.314840108491246,
0.332069149066805),.UNSPECIFIED.)
GEOMETRIC_REPRESENTATION_ITEM()
RATIONAL_B_SPLINE_SURFACE(((0.98789057959819,0.986774945528862,0.988576730109495),
(0.98789057959819,0.986774945528862,0.988576730109495)))
REPRESENTATION_ITEM('')
SURFACE()
);
#1042=(
BOUNDED_SURFACE()
B_SPLINE_SURFACE(1,2,((#111344,#111345,#111346,#111347,#111348),(#111349,
#111350,#111351,#111352,#111353)),.UNSPECIFIED.,.F.,.F.,.F.)
B_SPLINE_SURFACE_WITH_KNOTS((2,2),(3,2,3),(0.70959476887014,1.),(0.40044464501961,
0.401042835325428,0.418415696246123),.UNSPECIFIED.)
GEOMETRIC_REPRESENTATION_ITEM()
RATIONAL_B_SPLINE_SURFACE(((0.988122504062135,0.988122504062135,0.988122504062135,
0.989520169850093,0.993884164197532),(0.988122504062135,0.988122504062135,
0.988122504062135,0.989520169850093,0.993884164197532)))
REPRESENTATION_ITEM('')
SURFACE()
);
#1043=(
BOUNDED_SURFACE()
B_SPLINE_SURFACE(1,2,((#111362,#111363,#111364),(#111365,#111366,#111367)),
 .UNSPECIFIED.,.F.,.F.,.F.)
B_SPLINE_SURFACE_WITH_KNOTS((2,2),(3,3),(0.710318915638668,1.),(0.314840108491246,
0.332069149066805),.UNSPECIFIED.)
GEOMETRIC_REPRESENTATION_ITEM()
RATIONAL_B_SPLINE_SURFACE(((0.98789057959819,0.986774945528862,0.988576730109495),
(0.98789057959819,0.986774945528862,0.988576730109495)))
REPRESENTATION_ITEM('')
SURFACE()
);
#1044=(
BOUNDED_SURFACE()
B_SPLINE_SURFACE(1,2,((#111369,#111370,#111371,#111372,#111373),(#111374,
#111375,#111376,#111377,#111378)),.UNSPECIFIED.,.F.,.F.,.F.)
B_SPLINE_SURFACE_WITH_KNOTS((2,2),(3,2,3),(0.709594768915212,1.),(0.400444645009376,
0.401042835325429,0.418415696246122),.UNSPECIFIED.)
GEOMETRIC_REPRESENTATION_ITEM()
RATIONAL_B_SPLINE_SURFACE(((0.988122504062135,0.988122504062135,0.988122504062135,
0.989520169850093,0.993884164197532),(0.988122504062135,0.988122504062135,
0.988122504062135,0.989520169850093,0.993884164197532)))
REPRESENTATION_ITEM('')
SURFACE()
);
#1045=(
BOUNDED_SURFACE()
B_SPLINE_SURFACE(1,2,((#111387,#111388,#111389),(#111390,#111391,#111392)),
 .UNSPECIFIED.,.F.,.F.,.F.)
B_SPLINE_SURFACE_WITH_KNOTS((2,2),(3,3),(0.710318915639828,1.),(0.314840108491246,
0.332069149066805),.UNSPECIFIED.)
GEOMETRIC_REPRESENTATION_ITEM()
RATIONAL_B_SPLINE_SURFACE(((0.98789057959819,0.986774945528862,0.988576730109495),
(0.98789057959819,0.986774945528862,0.988576730109495)))
REPRESENTATION_ITEM('')
SURFACE()
);
#1046=(
BOUNDED_SURFACE()
B_SPLINE_SURFACE(1,2,((#111394,#111395,#111396,#111397,#111398),(#111399,
#111400,#111401,#111402,#111403)),.UNSPECIFIED.,.F.,.F.,.F.)
B_SPLINE_SURFACE_WITH_KNOTS((2,2),(3,2,3),(0.709594768950057,1.),(0.400444645044343,
0.401042835325431,0.418415696246123),.UNSPECIFIED.)
GEOMETRIC_REPRESENTATION_ITEM()
RATIONAL_B_SPLINE_SURFACE(((0.988122504062135,0.988122504062135,0.988122504062135,
0.989520169850094,0.993884164197532),(0.988122504062135,0.988122504062135,
0.988122504062135,0.989520169850094,0.993884164197532)))
REPRESENTATION_ITEM('')
SURFACE()
);
#1047=(
BOUNDED_SURFACE()
B_SPLINE_SURFACE(1,2,((#111412,#111413,#111414),(#111415,#111416,#111417)),
 .UNSPECIFIED.,.F.,.F.,.F.)
B_SPLINE_SURFACE_WITH_KNOTS((2,2),(3,3),(0.710318915640079,1.),(0.314840108491246,
0.332069149066805),.UNSPECIFIED.)
GEOMETRIC_REPRESENTATION_ITEM()
RATIONAL_B_SPLINE_SURFACE(((0.98789057959819,0.986774945528862,0.988576730109495),
(0.98789057959819,0.986774945528862,0.988576730109495)))
REPRESENTATION_ITEM('')
SURFACE()
);
#1048=(
BOUNDED_SURFACE()
B_SPLINE_SURFACE(1,2,((#111419,#111420,#111421,#111422,#111423),(#111424,
#111425,#111426,#111427,#111428)),.UNSPECIFIED.,.F.,.F.,.F.)
B_SPLINE_SURFACE_WITH_KNOTS((2,2),(3,2,3),(0.709594768954782,1.),(0.400444645048726,
0.401042835325429,0.418415696246123),.UNSPECIFIED.)
GEOMETRIC_REPRESENTATION_ITEM()
RATIONAL_B_SPLINE_SURFACE(((0.988122504062135,0.988122504062135,0.988122504062135,
0.989520169850093,0.993884164197532),(0.988122504062135,0.988122504062135,
0.988122504062135,0.989520169850093,0.993884164197532)))
REPRESENTATION_ITEM('')
SURFACE()
);
#1049=(
BOUNDED_SURFACE()
B_SPLINE_SURFACE(1,2,((#111437,#111438,#111439),(#111440,#111441,#111442)),
 .UNSPECIFIED.,.F.,.F.,.F.)
B_SPLINE_SURFACE_WITH_KNOTS((2,2),(3,3),(0.710318915640079,1.),(0.314840108491246,
0.332069149066805),.UNSPECIFIED.)
GEOMETRIC_REPRESENTATION_ITEM()
RATIONAL_B_SPLINE_SURFACE(((0.98789057959819,0.986774945528862,0.988576730109495),
(0.98789057959819,0.986774945528862,0.988576730109495)))
REPRESENTATION_ITEM('')
SURFACE()
);
#1050=(
BOUNDED_SURFACE()
B_SPLINE_SURFACE(1,2,((#111444,#111445,#111446,#111447,#111448),(#111449,
#111450,#111451,#111452,#111453)),.UNSPECIFIED.,.F.,.F.,.F.)
B_SPLINE_SURFACE_WITH_KNOTS((2,2),(3,2,3),(0.709594768915967,1.),(0.400444645010483,
0.401042835325429,0.418415696246123),.UNSPECIFIED.)
GEOMETRIC_REPRESENTATION_ITEM()
RATIONAL_B_SPLINE_SURFACE(((0.988122504062135,0.988122504062135,0.988122504062135,
0.989520169850093,0.993884164197532),(0.988122504062135,0.988122504062135,
0.988122504062135,0.989520169850093,0.993884164197532)))
REPRESENTATION_ITEM('')
SURFACE()
);
#1051=(
BOUNDED_SURFACE()
B_SPLINE_SURFACE(1,2,((#111462,#111463,#111464),(#111465,#111466,#111467)),
 .UNSPECIFIED.,.F.,.F.,.F.)
B_SPLINE_SURFACE_WITH_KNOTS((2,2),(3,3),(0.71031891564008,1.),(0.314840108491246,
0.332069149066805),.UNSPECIFIED.)
GEOMETRIC_REPRESENTATION_ITEM()
RATIONAL_B_SPLINE_SURFACE(((0.98789057959819,0.986774945528862,0.988576730109495),
(0.98789057959819,0.986774945528862,0.988576730109495)))
REPRESENTATION_ITEM('')
SURFACE()
);
#1052=(
BOUNDED_SURFACE()
B_SPLINE_SURFACE(1,2,((#111469,#111470,#111471,#111472,#111473),(#111474,
#111475,#111476,#111477,#111478)),.UNSPECIFIED.,.F.,.F.,.F.)
B_SPLINE_SURFACE_WITH_KNOTS((2,2),(3,2,3),(0.709594768949808,1.),(0.400444645043581,
0.401042835325428,0.418415696246123),.UNSPECIFIED.)
GEOMETRIC_REPRESENTATION_ITEM()
RATIONAL_B_SPLINE_SURFACE(((0.988122504062135,0.988122504062135,0.988122504062135,
0.989520169850093,0.993884164197532),(0.988122504062135,0.988122504062135,
0.988122504062135,0.989520169850093,0.993884164197532)))
REPRESENTATION_ITEM('')
SURFACE()
);
#1053=(
BOUNDED_SURFACE()
B_SPLINE_SURFACE(1,2,((#111487,#111488,#111489),(#111490,#111491,#111492)),
 .UNSPECIFIED.,.F.,.F.,.F.)
B_SPLINE_SURFACE_WITH_KNOTS((2,2),(3,3),(0.710318915640075,1.),(0.314840108491246,
0.332069149066804),.UNSPECIFIED.)
GEOMETRIC_REPRESENTATION_ITEM()
RATIONAL_B_SPLINE_SURFACE(((0.98789057959819,0.986774945528862,0.988576730109495),
(0.98789057959819,0.986774945528862,0.988576730109495)))
REPRESENTATION_ITEM('')
SURFACE()
);
#1054=(
BOUNDED_SURFACE()
B_SPLINE_SURFACE(1,2,((#111494,#111495,#111496,#111497,#111498),(#111499,
#111500,#111501,#111502,#111503)),.UNSPECIFIED.,.F.,.F.,.F.)
B_SPLINE_SURFACE_WITH_KNOTS((2,2),(3,2,3),(0.709594768917399,1.),(0.400444645011763,
0.401042835325431,0.418415696246121),.UNSPECIFIED.)
GEOMETRIC_REPRESENTATION_ITEM()
RATIONAL_B_SPLINE_SURFACE(((0.988122504062135,0.988122504062135,0.988122504062135,
0.989520169850093,0.993884164197532),(0.988122504062135,0.988122504062135,
0.988122504062135,0.989520169850093,0.993884164197532)))
REPRESENTATION_ITEM('')
SURFACE()
);
#1055=(
BOUNDED_SURFACE()
B_SPLINE_SURFACE(1,2,((#111512,#111513,#111514),(#111515,#111516,#111517)),
 .UNSPECIFIED.,.F.,.F.,.F.)
B_SPLINE_SURFACE_WITH_KNOTS((2,2),(3,3),(0.710318915639816,1.),(0.314840108491247,
0.332069149066865),.UNSPECIFIED.)
GEOMETRIC_REPRESENTATION_ITEM()
RATIONAL_B_SPLINE_SURFACE(((0.98789057959819,0.986774945528858,0.988576730109508),
(0.98789057959819,0.986774945528858,0.988576730109508)))
REPRESENTATION_ITEM('')
SURFACE()
);
#1056=(
BOUNDED_SURFACE()
B_SPLINE_SURFACE(1,2,((#111519,#111520,#111521,#111522,#111523),(#111524,
#111525,#111526,#111527,#111528)),.UNSPECIFIED.,.F.,.F.,.F.)
B_SPLINE_SURFACE_WITH_KNOTS((2,2),(3,2,3),(0.709594768924498,1.),(0.400444645018782,
0.401042835325428,0.418415696246121),.UNSPECIFIED.)
GEOMETRIC_REPRESENTATION_ITEM()
RATIONAL_B_SPLINE_SURFACE(((0.988122504062135,0.988122504062135,0.988122504062135,
0.989520169850093,0.993884164197532),(0.988122504062135,0.988122504062135,
0.988122504062135,0.989520169850093,0.993884164197532)))
REPRESENTATION_ITEM('')
SURFACE()
);
#1057=(
BOUNDED_SURFACE()
B_SPLINE_SURFACE(1,2,((#111537,#111538,#111539),(#111540,#111541,#111542)),
 .UNSPECIFIED.,.F.,.F.,.F.)
B_SPLINE_SURFACE_WITH_KNOTS((2,2),(3,3),(0.71031891563976,1.),(0.314840108491247,
0.332069149066858),.UNSPECIFIED.)
GEOMETRIC_REPRESENTATION_ITEM()
RATIONAL_B_SPLINE_SURFACE(((0.98789057959819,0.986774945528858,0.988576730109506),
(0.98789057959819,0.986774945528858,0.988576730109506)))
REPRESENTATION_ITEM('')
SURFACE()
);
#1058=(
BOUNDED_SURFACE()
B_SPLINE_SURFACE(1,2,((#111544,#111545,#111546,#111547,#111548),(#111549,
#111550,#111551,#111552,#111553)),.UNSPECIFIED.,.F.,.F.,.F.)
B_SPLINE_SURFACE_WITH_KNOTS((2,2),(3,2,3),(0.709594768872521,1.),(0.400444645020776,
0.401042835325429,0.418415696246121),.UNSPECIFIED.)
GEOMETRIC_REPRESENTATION_ITEM()
RATIONAL_B_SPLINE_SURFACE(((0.988122504062135,0.988122504062135,0.988122504062135,
0.989520169850093,0.993884164197532),(0.988122504062135,0.988122504062135,
0.988122504062135,0.989520169850093,0.993884164197532)))
REPRESENTATION_ITEM('')
SURFACE()
);
#1059=(
BOUNDED_SURFACE()
B_SPLINE_SURFACE(1,2,((#111562,#111563,#111564),(#111565,#111566,#111567)),
 .UNSPECIFIED.,.F.,.F.,.F.)
B_SPLINE_SURFACE_WITH_KNOTS((2,2),(3,3),(0.710318915639801,1.),(0.314840108491246,
0.332069149066961),.UNSPECIFIED.)
GEOMETRIC_REPRESENTATION_ITEM()
RATIONAL_B_SPLINE_SURFACE(((0.98789057959819,0.986774945528852,0.988576730109528),
(0.98789057959819,0.986774945528852,0.988576730109528)))
REPRESENTATION_ITEM('')
SURFACE()
);
#1060=(
BOUNDED_SURFACE()
B_SPLINE_SURFACE(1,2,((#111569,#111570,#111571,#111572,#111573),(#111574,
#111575,#111576,#111577,#111578)),.UNSPECIFIED.,.F.,.F.,.F.)
B_SPLINE_SURFACE_WITH_KNOTS((2,2),(3,2,3),(0.709594768860568,1.),(0.400444645009416,
0.40104283532543,0.418415696246122),.UNSPECIFIED.)
GEOMETRIC_REPRESENTATION_ITEM()
RATIONAL_B_SPLINE_SURFACE(((0.988122504062135,0.988122504062135,0.988122504062135,
0.989520169850094,0.993884164197532),(0.988122504062135,0.988122504062135,
0.988122504062135,0.989520169850094,0.993884164197532)))
REPRESENTATION_ITEM('')
SURFACE()
);
#1061=(
BOUNDED_SURFACE()
B_SPLINE_SURFACE(1,2,((#111587,#111588,#111589),(#111590,#111591,#111592)),
 .UNSPECIFIED.,.F.,.F.,.F.)
B_SPLINE_SURFACE_WITH_KNOTS((2,2),(3,3),(0.710318915639618,1.),(0.314840108491245,
0.332069149066961),.UNSPECIFIED.)
GEOMETRIC_REPRESENTATION_ITEM()
RATIONAL_B_SPLINE_SURFACE(((0.98789057959819,0.986774945528851,0.988576730109528),
(0.98789057959819,0.986774945528852,0.988576730109528)))
REPRESENTATION_ITEM('')
SURFACE()
);
#1062=(
BOUNDED_SURFACE()
B_SPLINE_SURFACE(1,2,((#111594,#111595,#111596,#111597,#111598),(#111599,
#111600,#111601,#111602,#111603)),.UNSPECIFIED.,.F.,.F.,.F.)
B_SPLINE_SURFACE_WITH_KNOTS((2,2),(3,2,3),(0.709594768894549,1.),(0.400444645043085,
0.401042835325431,0.418415696246122),.UNSPECIFIED.)
GEOMETRIC_REPRESENTATION_ITEM()
RATIONAL_B_SPLINE_SURFACE(((0.988122504062135,0.988122504062135,0.988122504062135,
0.989520169850094,0.993884164197532),(0.988122504062135,0.988122504062135,
0.988122504062135,0.989520169850094,0.993884164197532)))
REPRESENTATION_ITEM('')
SURFACE()
);
#1063=(
BOUNDED_SURFACE()
B_SPLINE_SURFACE(1,2,((#111612,#111613,#111614),(#111615,#111616,#111617)),
 .UNSPECIFIED.,.F.,.F.,.F.)
B_SPLINE_SURFACE_WITH_KNOTS((2,2),(3,3),(0.71031891563966,1.),(0.314840108491245,
0.332069149066961),.UNSPECIFIED.)
GEOMETRIC_REPRESENTATION_ITEM()
RATIONAL_B_SPLINE_SURFACE(((0.98789057959819,0.986774945528852,0.988576730109528),
(0.98789057959819,0.986774945528852,0.988576730109528)))
REPRESENTATION_ITEM('')
SURFACE()
);
#1064=(
BOUNDED_SURFACE()
B_SPLINE_SURFACE(1,2,((#111619,#111620,#111621),(#111622,#111623,#111624)),
 .UNSPECIFIED.,.F.,.F.,.F.)
B_SPLINE_SURFACE_WITH_KNOTS((2,2),(3,3),(0.,0.28968108435992),(0.262994994770444,
0.280433083165913),.UNSPECIFIED.)
GEOMETRIC_REPRESENTATION_ITEM()
RATIONAL_B_SPLINE_SURFACE(((0.989123653000983,0.991350813683904,0.996566619267863),
(0.989123653000983,0.991350813683904,0.996566619267863)))
REPRESENTATION_ITEM('')
SURFACE()
);
#1065=(
BOUNDED_SURFACE()
B_SPLINE_SURFACE(1,2,((#111633,#111634,#111635,#111636,#111637),(#111638,
#111639,#111640,#111641,#111642)),.UNSPECIFIED.,.F.,.F.,.F.)
B_SPLINE_SURFACE_WITH_KNOTS((2,2),(3,2,3),(0.,0.29039866515125),(0.452333244852708,
0.452924869174517,0.470122329512317),.UNSPECIFIED.)
GEOMETRIC_REPRESENTATION_ITEM()
RATIONAL_B_SPLINE_SURFACE(((0.988732477628006,0.988732477628006,0.988732477628006,
0.986812255267055,0.987798766302166),(0.988732477628006,0.988732477628006,
0.988732477628006,0.986812255267055,0.987798766302166)))
REPRESENTATION_ITEM('')
SURFACE()
);
#1066=(
BOUNDED_SURFACE()
B_SPLINE_SURFACE(1,2,((#111644,#111645,#111646),(#111647,#111648,#111649)),
 .UNSPECIFIED.,.F.,.F.,.F.)
B_SPLINE_SURFACE_WITH_KNOTS((2,2),(3,3),(0.,0.289681084359921),(0.262994994770445,
0.280433083165915),.UNSPECIFIED.)
GEOMETRIC_REPRESENTATION_ITEM()
RATIONAL_B_SPLINE_SURFACE(((0.989123653000983,0.991350813683905,0.996566619267864),
(0.989123653000983,0.991350813683905,0.996566619267864)))
REPRESENTATION_ITEM('')
SURFACE()
);
#1067=(
BOUNDED_SURFACE()
B_SPLINE_SURFACE(1,2,((#111658,#111659,#111660,#111661,#111662),(#111663,
#111664,#111665,#111666,#111667)),.UNSPECIFIED.,.F.,.F.,.F.)
B_SPLINE_SURFACE_WITH_KNOTS((2,2),(3,2,3),(0.,0.290398665170194),(0.452333244833745,
0.452924869174514,0.470122329512317),.UNSPECIFIED.)
GEOMETRIC_REPRESENTATION_ITEM()
RATIONAL_B_SPLINE_SURFACE(((0.988732477628006,0.988732477628006,0.988732477628006,
0.986812255267055,0.987798766302166),(0.988732477628006,0.988732477628006,
0.988732477628006,0.986812255267055,0.987798766302166)))
REPRESENTATION_ITEM('')
SURFACE()
);
#1068=(
BOUNDED_SURFACE()
B_SPLINE_SURFACE(1,2,((#111669,#111670,#111671),(#111672,#111673,#111674)),
 .UNSPECIFIED.,.F.,.F.,.F.)
B_SPLINE_SURFACE_WITH_KNOTS((2,2),(3,3),(0.,0.289681084359918),(0.262994994770445,
0.280433083165914),.UNSPECIFIED.)
GEOMETRIC_REPRESENTATION_ITEM()
RATIONAL_B_SPLINE_SURFACE(((0.989123653000983,0.991350813683905,0.996566619267864),
(0.989123653000983,0.991350813683905,0.996566619267864)))
REPRESENTATION_ITEM('')
SURFACE()
);
#1069=(
BOUNDED_SURFACE()
B_SPLINE_SURFACE(1,2,((#111683,#111684,#111685,#111686,#111687),(#111688,
#111689,#111690,#111691,#111692)),.UNSPECIFIED.,.F.,.F.,.F.)
B_SPLINE_SURFACE_WITH_KNOTS((2,2),(3,2,3),(0.,0.290398665162971),(0.452333244841549,
0.452924869174515,0.470122329512317),.UNSPECIFIED.)
GEOMETRIC_REPRESENTATION_ITEM()
RATIONAL_B_SPLINE_SURFACE(((0.988732477628006,0.988732477628006,0.988732477628006,
0.986812255267055,0.987798766302166),(0.988732477628006,0.988732477628006,
0.988732477628006,0.986812255267055,0.987798766302166)))
REPRESENTATION_ITEM('')
SURFACE()
);
#1070=(
BOUNDED_SURFACE()
B_SPLINE_SURFACE(1,2,((#111694,#111695,#111696),(#111697,#111698,#111699)),
 .UNSPECIFIED.,.F.,.F.,.F.)
B_SPLINE_SURFACE_WITH_KNOTS((2,2),(3,3),(0.,0.289681084359921),(0.262994994770445,
0.280433083165914),.UNSPECIFIED.)
GEOMETRIC_REPRESENTATION_ITEM()
RATIONAL_B_SPLINE_SURFACE(((0.989123653000983,0.991350813683905,0.996566619267864),
(0.989123653000983,0.991350813683905,0.996566619267864)))
REPRESENTATION_ITEM('')
SURFACE()
);
#1071=(
BOUNDED_SURFACE()
B_SPLINE_SURFACE(1,2,((#111708,#111709,#111710,#111711,#111712),(#111713,
#111714,#111715,#111716,#111717)),.UNSPECIFIED.,.F.,.F.,.F.)
B_SPLINE_SURFACE_WITH_KNOTS((2,2),(3,2,3),(0.,0.290398665157545),(0.452333244846396,
0.452924869174515,0.470122329512317),.UNSPECIFIED.)
GEOMETRIC_REPRESENTATION_ITEM()
RATIONAL_B_SPLINE_SURFACE(((0.988732477628006,0.988732477628006,0.988732477628006,
0.986812255267055,0.987798766302166),(0.988732477628006,0.988732477628006,
0.988732477628006,0.986812255267055,0.987798766302166)))
REPRESENTATION_ITEM('')
SURFACE()
);
#1072=(
BOUNDED_SURFACE()
B_SPLINE_SURFACE(1,2,((#111719,#111720,#111721),(#111722,#111723,#111724)),
 .UNSPECIFIED.,.F.,.F.,.F.)
B_SPLINE_SURFACE_WITH_KNOTS((2,2),(3,3),(0.,0.289681084359921),(0.262994994770445,
0.280433083165914),.UNSPECIFIED.)
GEOMETRIC_REPRESENTATION_ITEM()
RATIONAL_B_SPLINE_SURFACE(((0.989123653000983,0.991350813683905,0.996566619267864),
(0.989123653000983,0.991350813683905,0.996566619267864)))
REPRESENTATION_ITEM('')
SURFACE()
);
#1073=(
BOUNDED_SURFACE()
B_SPLINE_SURFACE(1,2,((#111733,#111734,#111735,#111736,#111737),(#111738,
#111739,#111740,#111741,#111742)),.UNSPECIFIED.,.F.,.F.,.F.)
B_SPLINE_SURFACE_WITH_KNOTS((2,2),(3,2,3),(0.,0.29039866515236),(0.452333244852162,
0.452924869174515,0.470122329512317),.UNSPECIFIED.)
GEOMETRIC_REPRESENTATION_ITEM()
RATIONAL_B_SPLINE_SURFACE(((0.988732477628006,0.988732477628006,0.988732477628006,
0.986812255267055,0.987798766302166),(0.988732477628006,0.988732477628006,
0.988732477628006,0.986812255267055,0.987798766302166)))
REPRESENTATION_ITEM('')
SURFACE()
);
#1074=(
BOUNDED_SURFACE()
B_SPLINE_SURFACE(1,2,((#111744,#111745,#111746),(#111747,#111748,#111749)),
 .UNSPECIFIED.,.F.,.F.,.F.)
B_SPLINE_SURFACE_WITH_KNOTS((2,2),(3,3),(0.,0.289681084359916),(0.262994994770445,
0.280433083165914),.UNSPECIFIED.)
GEOMETRIC_REPRESENTATION_ITEM()
RATIONAL_B_SPLINE_SURFACE(((0.989123653000983,0.991350813683905,0.996566619267864),
(0.989123653000983,0.991350813683905,0.996566619267864)))
REPRESENTATION_ITEM('')
SURFACE()
);
#1075=(
BOUNDED_SURFACE()
B_SPLINE_SURFACE(1,2,((#111758,#111759,#111760,#111761,#111762),(#111763,
#111764,#111765,#111766,#111767)),.UNSPECIFIED.,.F.,.F.,.F.)
B_SPLINE_SURFACE_WITH_KNOTS((2,2),(3,2,3),(0.,0.290398665167829),(0.452333244836186,
0.452924869174516,0.470122329512317),.UNSPECIFIED.)
GEOMETRIC_REPRESENTATION_ITEM()
RATIONAL_B_SPLINE_SURFACE(((0.988732477628006,0.988732477628006,0.988732477628006,
0.986812255267055,0.987798766302166),(0.988732477628006,0.988732477628006,
0.988732477628006,0.986812255267055,0.987798766302166)))
REPRESENTATION_ITEM('')
SURFACE()
);
#1076=(
BOUNDED_SURFACE()
B_SPLINE_SURFACE(1,2,((#111769,#111770,#111771),(#111772,#111773,#111774)),
 .UNSPECIFIED.,.F.,.F.,.F.)
B_SPLINE_SURFACE_WITH_KNOTS((2,2),(3,3),(0.,0.289681084359922),(0.262994994770443,
0.280433083165913),.UNSPECIFIED.)
GEOMETRIC_REPRESENTATION_ITEM()
RATIONAL_B_SPLINE_SURFACE(((0.989123653000983,0.991350813683904,0.996566619267864),
(0.989123653000983,0.991350813683904,0.996566619267864)))
REPRESENTATION_ITEM('')
SURFACE()
);
#1077=(
BOUNDED_SURFACE()
B_SPLINE_SURFACE(1,2,((#111783,#111784,#111785,#111786,#111787),(#111788,
#111789,#111790,#111791,#111792)),.UNSPECIFIED.,.F.,.F.,.F.)
B_SPLINE_SURFACE_WITH_KNOTS((2,2),(3,2,3),(0.,0.290398665157212),(0.452333244846804,
0.452924869174517,0.470122329512318),.UNSPECIFIED.)
GEOMETRIC_REPRESENTATION_ITEM()
RATIONAL_B_SPLINE_SURFACE(((0.988732477628006,0.988732477628006,0.988732477628006,
0.986812255267055,0.987798766302167),(0.988732477628006,0.988732477628006,
0.988732477628006,0.986812255267055,0.987798766302167)))
REPRESENTATION_ITEM('')
SURFACE()
);
#1078=(
BOUNDED_SURFACE()
B_SPLINE_SURFACE(1,2,((#111794,#111795,#111796),(#111797,#111798,#111799)),
 .UNSPECIFIED.,.F.,.F.,.F.)
B_SPLINE_SURFACE_WITH_KNOTS((2,2),(3,3),(0.,0.289681084359917),(0.262994994770443,
0.280433083165913),.UNSPECIFIED.)
GEOMETRIC_REPRESENTATION_ITEM()
RATIONAL_B_SPLINE_SURFACE(((0.989123653000983,0.991350813683904,0.996566619267863),
(0.989123653000983,0.991350813683904,0.996566619267863)))
REPRESENTATION_ITEM('')
SURFACE()
);
#1079=(
BOUNDED_SURFACE()
B_SPLINE_SURFACE(1,2,((#111808,#111809,#111810,#111811,#111812),(#111813,
#111814,#111815,#111816,#111817)),.UNSPECIFIED.,.F.,.F.,.F.)
B_SPLINE_SURFACE_WITH_KNOTS((2,2),(3,2,3),(0.,0.290398665177456),(0.45233324482716,
0.452924869174517,0.470122329512318),.UNSPECIFIED.)
GEOMETRIC_REPRESENTATION_ITEM()
RATIONAL_B_SPLINE_SURFACE(((0.988732477628005,0.988732477628005,0.988732477628005,
0.986812255267055,0.987798766302166),(0.988732477628005,0.988732477628005,
0.988732477628005,0.986812255267055,0.987798766302166)))
REPRESENTATION_ITEM('')
SURFACE()
);
#1080=(
BOUNDED_SURFACE()
B_SPLINE_SURFACE(1,2,((#111819,#111820,#111821),(#111822,#111823,#111824)),
 .UNSPECIFIED.,.F.,.F.,.F.)
B_SPLINE_SURFACE_WITH_KNOTS((2,2),(3,3),(0.,0.289681084359919),(0.262994994770443,
0.280433083165913),.UNSPECIFIED.)
GEOMETRIC_REPRESENTATION_ITEM()
RATIONAL_B_SPLINE_SURFACE(((0.989123653000983,0.991350813683904,0.996566619267864),
(0.989123653000983,0.991350813683904,0.996566619267864)))
REPRESENTATION_ITEM('')
SURFACE()
);
#1081=(
BOUNDED_SURFACE()
B_SPLINE_SURFACE(1,2,((#111833,#111834,#111835,#111836,#111837),(#111838,
#111839,#111840,#111841,#111842)),.UNSPECIFIED.,.F.,.F.,.F.)
B_SPLINE_SURFACE_WITH_KNOTS((2,2),(3,2,3),(0.,0.290398665175405),(0.452333244828615,
0.452924869174516,0.470122329512318),.UNSPECIFIED.)
GEOMETRIC_REPRESENTATION_ITEM()
RATIONAL_B_SPLINE_SURFACE(((0.988732477628006,0.988732477628006,0.988732477628006,
0.986812255267055,0.987798766302166),(0.988732477628006,0.988732477628006,
0.988732477628006,0.986812255267055,0.987798766302166)))
REPRESENTATION_ITEM('')
SURFACE()
);
#1082=(
BOUNDED_SURFACE()
B_SPLINE_SURFACE(1,2,((#111844,#111845,#111846),(#111847,#111848,#111849)),
 .UNSPECIFIED.,.F.,.F.,.F.)
B_SPLINE_SURFACE_WITH_KNOTS((2,2),(3,3),(0.,0.289681084359922),(0.262994994770443,
0.280433083165913),.UNSPECIFIED.)
GEOMETRIC_REPRESENTATION_ITEM()
RATIONAL_B_SPLINE_SURFACE(((0.989123653000983,0.991350813683904,0.996566619267863),
(0.989123653000983,0.991350813683904,0.996566619267863)))
REPRESENTATION_ITEM('')
SURFACE()
);
#1083=(
BOUNDED_SURFACE()
B_SPLINE_SURFACE(1,2,((#111858,#111859,#111860,#111861,#111862),(#111863,
#111864,#111865,#111866,#111867)),.UNSPECIFIED.,.F.,.F.,.F.)
B_SPLINE_SURFACE_WITH_KNOTS((2,2),(3,2,3),(0.,0.290398665173023),(0.452333244831502,
0.452924869174516,0.470122329512318),.UNSPECIFIED.)
GEOMETRIC_REPRESENTATION_ITEM()
RATIONAL_B_SPLINE_SURFACE(((0.988732477628006,0.988732477628006,0.988732477628006,
0.986812255267055,0.987798766302167),(0.988732477628006,0.988732477628006,
0.988732477628006,0.986812255267055,0.987798766302167)))
REPRESENTATION_ITEM('')
SURFACE()
);
#1084=(
BOUNDED_SURFACE()
B_SPLINE_SURFACE(1,2,((#111869,#111870,#111871),(#111872,#111873,#111874)),
 .UNSPECIFIED.,.F.,.F.,.F.)
B_SPLINE_SURFACE_WITH_KNOTS((2,2),(3,3),(0.,0.289681084359919),(0.262994994770443,
0.280433083165913),.UNSPECIFIED.)
GEOMETRIC_REPRESENTATION_ITEM()
RATIONAL_B_SPLINE_SURFACE(((0.989123653000983,0.991350813683904,0.996566619267864),
(0.989123653000983,0.991350813683904,0.996566619267864)))
REPRESENTATION_ITEM('')
SURFACE()
);
#1085=(
BOUNDED_SURFACE()
B_SPLINE_SURFACE(1,2,((#111883,#111884,#111885,#111886,#111887),(#111888,
#111889,#111890,#111891,#111892)),.UNSPECIFIED.,.F.,.F.,.F.)
B_SPLINE_SURFACE_WITH_KNOTS((2,2),(3,2,3),(0.,0.290398665142381),(0.452333244861645,
0.452924869174517,0.470122329512318),.UNSPECIFIED.)
GEOMETRIC_REPRESENTATION_ITEM()
RATIONAL_B_SPLINE_SURFACE(((0.988732477628006,0.988732477628006,0.988732477628006,
0.986812255267055,0.987798766302167),(0.988732477628006,0.988732477628006,
0.988732477628006,0.986812255267055,0.987798766302167)))
REPRESENTATION_ITEM('')
SURFACE()
);
#1086=(
BOUNDED_SURFACE()
B_SPLINE_SURFACE(1,2,((#111894,#111895,#111896),(#111897,#111898,#111899)),
 .UNSPECIFIED.,.F.,.F.,.F.)
B_SPLINE_SURFACE_WITH_KNOTS((2,2),(3,3),(0.,0.289681084359921),(0.262994994770443,
0.280433083165913),.UNSPECIFIED.)
GEOMETRIC_REPRESENTATION_ITEM()
RATIONAL_B_SPLINE_SURFACE(((0.989123653000983,0.991350813683904,0.996566619267864),
(0.989123653000983,0.991350813683904,0.996566619267864)))
REPRESENTATION_ITEM('')
SURFACE()
);
#1087=(
BOUNDED_SURFACE()
B_SPLINE_SURFACE(1,2,((#111908,#111909,#111910,#111911,#111912),(#111913,
#111914,#111915,#111916,#111917)),.UNSPECIFIED.,.F.,.F.,.F.)
B_SPLINE_SURFACE_WITH_KNOTS((2,2),(3,2,3),(0.,0.290398665147505),(0.452333244857022,
0.452924869174516,0.470122329512318),.UNSPECIFIED.)
GEOMETRIC_REPRESENTATION_ITEM()
RATIONAL_B_SPLINE_SURFACE(((0.988732477628006,0.988732477628006,0.988732477628006,
0.986812255267055,0.987798766302166),(0.988732477628006,0.988732477628006,
0.988732477628006,0.986812255267055,0.987798766302166)))
REPRESENTATION_ITEM('')
SURFACE()
);
#1088=(
BOUNDED_SURFACE()
B_SPLINE_SURFACE(1,2,((#111919,#111920,#111921),(#111922,#111923,#111924)),
 .UNSPECIFIED.,.F.,.F.,.F.)
B_SPLINE_SURFACE_WITH_KNOTS((2,2),(3,3),(0.,0.289681084359921),(0.262994994770444,
0.280433083165913),.UNSPECIFIED.)
GEOMETRIC_REPRESENTATION_ITEM()
RATIONAL_B_SPLINE_SURFACE(((0.989123653000983,0.991350813683904,0.996566619267863),
(0.989123653000983,0.991350813683904,0.996566619267863)))
REPRESENTATION_ITEM('')
SURFACE()
);
#1089=(
BOUNDED_SURFACE()
B_SPLINE_SURFACE(1,2,((#111933,#111934,#111935,#111936,#111937),(#111938,
#111939,#111940,#111941,#111942)),.UNSPECIFIED.,.F.,.F.,.F.)
B_SPLINE_SURFACE_WITH_KNOTS((2,2),(3,2,3),(0.,0.290398665150954),(0.452333244853345,
0.452924869174516,0.470122329512318),.UNSPECIFIED.)
GEOMETRIC_REPRESENTATION_ITEM()
RATIONAL_B_SPLINE_SURFACE(((0.988732477628006,0.988732477628006,0.988732477628006,
0.986812255267055,0.987798766302166),(0.988732477628006,0.988732477628006,
0.988732477628006,0.986812255267055,0.987798766302166)))
REPRESENTATION_ITEM('')
SURFACE()
);
#1090=(
BOUNDED_SURFACE()
B_SPLINE_SURFACE(1,2,((#111944,#111945,#111946),(#111947,#111948,#111949)),
 .UNSPECIFIED.,.F.,.F.,.F.)
B_SPLINE_SURFACE_WITH_KNOTS((2,2),(3,3),(0.,0.289681084359921),(0.262994994770444,
0.280433083165913),.UNSPECIFIED.)
GEOMETRIC_REPRESENTATION_ITEM()
RATIONAL_B_SPLINE_SURFACE(((0.989123653000983,0.991350813683904,0.996566619267864),
(0.989123653000983,0.991350813683904,0.996566619267864)))
REPRESENTATION_ITEM('')
SURFACE()
);
#1091=(
BOUNDED_SURFACE()
B_SPLINE_SURFACE(1,2,((#111958,#111959,#111960,#111961,#111962),(#111963,
#111964,#111965,#111966,#111967)),.UNSPECIFIED.,.F.,.F.,.F.)
B_SPLINE_SURFACE_WITH_KNOTS((2,2),(3,2,3),(0.,0.290398665158173),(0.45233324484718,
0.452924869174516,0.470122329512318),.UNSPECIFIED.)
GEOMETRIC_REPRESENTATION_ITEM()
RATIONAL_B_SPLINE_SURFACE(((0.988732477628006,0.988732477628006,0.988732477628006,
0.986812255267055,0.987798766302167),(0.988732477628006,0.988732477628006,
0.988732477628006,0.986812255267055,0.987798766302166)))
REPRESENTATION_ITEM('')
SURFACE()
);
#1092=(
BOUNDED_SURFACE()
B_SPLINE_SURFACE(1,2,((#111969,#111970,#111971),(#111972,#111973,#111974)),
 .UNSPECIFIED.,.F.,.F.,.F.)
B_SPLINE_SURFACE_WITH_KNOTS((2,2),(3,3),(0.,0.289681084359921),(0.262994994770444,
0.280433083165913),.UNSPECIFIED.)
GEOMETRIC_REPRESENTATION_ITEM()
RATIONAL_B_SPLINE_SURFACE(((0.989123653000983,0.991350813683904,0.996566619267864),
(0.989123653000983,0.991350813683904,0.996566619267864)))
REPRESENTATION_ITEM('')
SURFACE()
);
#1093=(
BOUNDED_SURFACE()
B_SPLINE_SURFACE(1,2,((#111983,#111984,#111985,#111986,#111987),(#111988,
#111989,#111990,#111991,#111992)),.UNSPECIFIED.,.F.,.F.,.F.)
B_SPLINE_SURFACE_WITH_KNOTS((2,2),(3,2,3),(0.,0.290398665174958),(0.452333244829107,
0.452924869174517,0.470122329512318),.UNSPECIFIED.)
GEOMETRIC_REPRESENTATION_ITEM()
RATIONAL_B_SPLINE_SURFACE(((0.988732477628005,0.988732477628005,0.988732477628005,
0.986812255267055,0.987798766302167),(0.988732477628005,0.988732477628005,
0.988732477628005,0.986812255267055,0.987798766302167)))
REPRESENTATION_ITEM('')
SURFACE()
);
#1094=(
BOUNDED_SURFACE()
B_SPLINE_SURFACE(1,2,((#111994,#111995,#111996),(#111997,#111998,#111999)),
 .UNSPECIFIED.,.F.,.F.,.F.)
B_SPLINE_SURFACE_WITH_KNOTS((2,2),(3,3),(0.,0.28968108435993),(0.262994994770444,
0.280433083165913),.UNSPECIFIED.)
GEOMETRIC_REPRESENTATION_ITEM()
RATIONAL_B_SPLINE_SURFACE(((0.989123653000983,0.991350813683904,0.996566619267864),
(0.989123653000983,0.991350813683904,0.996566619267864)))
REPRESENTATION_ITEM('')
SURFACE()
);
#1095=(
BOUNDED_SURFACE()
B_SPLINE_SURFACE(1,2,((#112008,#112009,#112010,#112011,#112012),(#112013,
#112014,#112015,#112016,#112017)),.UNSPECIFIED.,.F.,.F.,.F.)
B_SPLINE_SURFACE_WITH_KNOTS((2,2),(3,2,3),(0.,0.290398665152165),(0.452333244851786,
0.452924869174515,0.470122329512318),.UNSPECIFIED.)
GEOMETRIC_REPRESENTATION_ITEM()
RATIONAL_B_SPLINE_SURFACE(((0.988732477628006,0.988732477628006,0.988732477628006,
0.986812255267055,0.987798766302166),(0.988732477628006,0.988732477628006,
0.988732477628006,0.986812255267055,0.987798766302166)))
REPRESENTATION_ITEM('')
SURFACE()
);
#1096=(
BOUNDED_SURFACE()
B_SPLINE_SURFACE(1,2,((#112019,#112020,#112021),(#112022,#112023,#112024)),
 .UNSPECIFIED.,.F.,.F.,.F.)
B_SPLINE_SURFACE_WITH_KNOTS((2,2),(3,3),(0.,0.289681084359921),(0.262994994770443,
0.280433083165913),.UNSPECIFIED.)
GEOMETRIC_REPRESENTATION_ITEM()
RATIONAL_B_SPLINE_SURFACE(((0.989123653000983,0.991350813683904,0.996566619267863),
(0.989123653000983,0.991350813683904,0.996566619267863)))
REPRESENTATION_ITEM('')
SURFACE()
);
#1097=(
BOUNDED_SURFACE()
B_SPLINE_SURFACE(1,2,((#112033,#112034,#112035,#112036,#112037),(#112038,
#112039,#112040,#112041,#112042)),.UNSPECIFIED.,.F.,.F.,.F.)
B_SPLINE_SURFACE_WITH_KNOTS((2,2),(3,2,3),(0.,0.290398665180164),(0.452333244824412,
0.452924869174517,0.470122329512318),.UNSPECIFIED.)
GEOMETRIC_REPRESENTATION_ITEM()
RATIONAL_B_SPLINE_SURFACE(((0.988732477628006,0.988732477628006,0.988732477628006,
0.986812255267055,0.987798766302167),(0.988732477628006,0.988732477628006,
0.988732477628006,0.986812255267055,0.987798766302167)))
REPRESENTATION_ITEM('')
SURFACE()
);
#1098=(
BOUNDED_SURFACE()
B_SPLINE_SURFACE(1,2,((#112044,#112045,#112046),(#112047,#112048,#112049)),
 .UNSPECIFIED.,.F.,.F.,.F.)
B_SPLINE_SURFACE_WITH_KNOTS((2,2),(3,3),(0.,0.289681084359926),(0.262994994770443,
0.280433083165913),.UNSPECIFIED.)
GEOMETRIC_REPRESENTATION_ITEM()
RATIONAL_B_SPLINE_SURFACE(((0.989123653000983,0.991350813683904,0.996566619267863),
(0.989123653000983,0.991350813683904,0.996566619267863)))
REPRESENTATION_ITEM('')
SURFACE()
);
#1099=(
BOUNDED_SURFACE()
B_SPLINE_SURFACE(1,2,((#112058,#112059,#112060,#112061,#112062),(#112063,
#112064,#112065,#112066,#112067)),.UNSPECIFIED.,.F.,.F.,.F.)
B_SPLINE_SURFACE_WITH_KNOTS((2,2),(3,2,3),(0.,0.290398665174101),(0.45233324482984,
0.452924869174517,0.470122329512318),.UNSPECIFIED.)
GEOMETRIC_REPRESENTATION_ITEM()
RATIONAL_B_SPLINE_SURFACE(((0.988732477628005,0.988732477628005,0.988732477628005,
0.986812255267055,0.987798766302166),(0.988732477628005,0.988732477628005,
0.988732477628005,0.986812255267055,0.987798766302166)))
REPRESENTATION_ITEM('')
SURFACE()
);
#1100=(
BOUNDED_SURFACE()
B_SPLINE_SURFACE(1,2,((#112069,#112070,#112071),(#112072,#112073,#112074)),
 .UNSPECIFIED.,.F.,.F.,.F.)
B_SPLINE_SURFACE_WITH_KNOTS((2,2),(3,3),(0.,0.289681084359926),(0.262994994770443,
0.280433083165913),.UNSPECIFIED.)
GEOMETRIC_REPRESENTATION_ITEM()
RATIONAL_B_SPLINE_SURFACE(((0.989123653000983,0.991350813683904,0.996566619267864),
(0.989123653000983,0.991350813683904,0.996566619267864)))
REPRESENTATION_ITEM('')
SURFACE()
);
#1101=(
BOUNDED_SURFACE()
B_SPLINE_SURFACE(1,2,((#112083,#112084,#112085,#112086,#112087),(#112088,
#112089,#112090,#112091,#112092)),.UNSPECIFIED.,.F.,.F.,.F.)
B_SPLINE_SURFACE_WITH_KNOTS((2,2),(3,2,3),(0.,0.29039866517598),(0.452333244829113,
0.452924869174518,0.470122329512318),.UNSPECIFIED.)
GEOMETRIC_REPRESENTATION_ITEM()
RATIONAL_B_SPLINE_SURFACE(((0.988732477628005,0.988732477628005,0.988732477628005,
0.986812255267055,0.987798766302166),(0.988732477628005,0.988732477628005,
0.988732477628005,0.986812255267055,0.987798766302166)))
REPRESENTATION_ITEM('')
SURFACE()
);
#1102=(
BOUNDED_SURFACE()
B_SPLINE_SURFACE(1,2,((#112094,#112095,#112096),(#112097,#112098,#112099)),
 .UNSPECIFIED.,.F.,.F.,.F.)
B_SPLINE_SURFACE_WITH_KNOTS((2,2),(3,3),(0.,0.289681084359929),(0.262994994770443,
0.280433083165913),.UNSPECIFIED.)
GEOMETRIC_REPRESENTATION_ITEM()
RATIONAL_B_SPLINE_SURFACE(((0.989123653000983,0.991350813683904,0.996566619267863),
(0.989123653000983,0.991350813683904,0.996566619267863)))
REPRESENTATION_ITEM('')
SURFACE()
);
#1103=(
BOUNDED_SURFACE()
B_SPLINE_SURFACE(1,2,((#112108,#112109,#112110,#112111,#112112),(#112113,
#112114,#112115,#112116,#112117)),.UNSPECIFIED.,.F.,.F.,.F.)
B_SPLINE_SURFACE_WITH_KNOTS((2,2),(3,2,3),(0.,0.290398665149643),(0.452333244855286,
0.452924869174518,0.470122329512318),.UNSPECIFIED.)
GEOMETRIC_REPRESENTATION_ITEM()
RATIONAL_B_SPLINE_SURFACE(((0.988732477628005,0.988732477628005,0.988732477628005,
0.986812255267055,0.987798766302167),(0.988732477628005,0.988732477628005,
0.988732477628005,0.986812255267055,0.987798766302167)))
REPRESENTATION_ITEM('')
SURFACE()
);
#1104=(
BOUNDED_SURFACE()
B_SPLINE_SURFACE(1,2,((#112119,#112120,#112121),(#112122,#112123,#112124)),
 .UNSPECIFIED.,.F.,.F.,.F.)
B_SPLINE_SURFACE_WITH_KNOTS((2,2),(3,3),(0.,0.289681084359926),(0.262994994770443,
0.280433083166016),.UNSPECIFIED.)
GEOMETRIC_REPRESENTATION_ITEM()
RATIONAL_B_SPLINE_SURFACE(((0.989123653000982,0.991350813683917,0.996566619267925),
(0.989123653000982,0.991350813683917,0.996566619267925)))
REPRESENTATION_ITEM('')
SURFACE()
);
#1105=(
BOUNDED_SURFACE()
B_SPLINE_SURFACE(1,2,((#112133,#112134,#112135,#112136,#112137),(#112138,
#112139,#112140,#112141,#112142)),.UNSPECIFIED.,.F.,.F.,.F.)
B_SPLINE_SURFACE_WITH_KNOTS((2,2),(3,2,3),(0.,0.290398665156825),(0.452333244848833,
0.452924869174518,0.470122329512318),.UNSPECIFIED.)
GEOMETRIC_REPRESENTATION_ITEM()
RATIONAL_B_SPLINE_SURFACE(((0.988732477628005,0.988732477628005,0.988732477628005,
0.986812255267055,0.987798766302166),(0.988732477628005,0.988732477628005,
0.988732477628005,0.986812255267055,0.987798766302166)))
REPRESENTATION_ITEM('')
SURFACE()
);
#1106=(
BOUNDED_SURFACE()
B_SPLINE_SURFACE(1,2,((#112144,#112145,#112146),(#112147,#112148,#112149)),
 .UNSPECIFIED.,.F.,.F.,.F.)
B_SPLINE_SURFACE_WITH_KNOTS((2,2),(3,3),(0.,0.289681084359918),(0.262994994770442,
0.280433083166178),.UNSPECIFIED.)
GEOMETRIC_REPRESENTATION_ITEM()
RATIONAL_B_SPLINE_SURFACE(((0.989123653000982,0.991350813683937,0.996566619268022),
(0.989123653000982,0.991350813683937,0.996566619268022)))
REPRESENTATION_ITEM('')
SURFACE()
);
#1107=(
BOUNDED_SURFACE()
B_SPLINE_SURFACE(1,2,((#112158,#112159,#112160,#112161,#112162),(#112163,
#112164,#112165,#112166,#112167)),.UNSPECIFIED.,.F.,.F.,.F.)
B_SPLINE_SURFACE_WITH_KNOTS((2,2),(3,2,3),(0.,0.290398665150478),(0.45233324485367,
0.452924869174517,0.470122329512318),.UNSPECIFIED.)
GEOMETRIC_REPRESENTATION_ITEM()
RATIONAL_B_SPLINE_SURFACE(((0.988732477628005,0.988732477628005,0.988732477628005,
0.986812255267055,0.987798766302167),(0.988732477628005,0.988732477628005,
0.988732477628005,0.986812255267055,0.987798766302167)))
REPRESENTATION_ITEM('')
SURFACE()
);
#1108=(
BOUNDED_SURFACE()
B_SPLINE_SURFACE(1,2,((#112169,#112170,#112171),(#112172,#112173,#112174)),
 .UNSPECIFIED.,.F.,.F.,.F.)
B_SPLINE_SURFACE_WITH_KNOTS((2,2),(3,3),(0.,0.289681084359922),(0.262994994770443,
0.280433083165913),.UNSPECIFIED.)
GEOMETRIC_REPRESENTATION_ITEM()
RATIONAL_B_SPLINE_SURFACE(((0.989123653000983,0.991350813683904,0.996566619267863),
(0.989123653000983,0.991350813683904,0.996566619267863)))
REPRESENTATION_ITEM('')
SURFACE()
);
#1109=(
BOUNDED_SURFACE()
B_SPLINE_SURFACE(1,2,((#112183,#112184,#112185,#112186,#112187),(#112188,
#112189,#112190,#112191,#112192)),.UNSPECIFIED.,.F.,.F.,.F.)
B_SPLINE_SURFACE_WITH_KNOTS((2,2),(3,2,3),(0.,0.290398665153931),(0.452333244851512,
0.452924869174518,0.470122329512318),.UNSPECIFIED.)
GEOMETRIC_REPRESENTATION_ITEM()
RATIONAL_B_SPLINE_SURFACE(((0.988732477628005,0.988732477628005,0.988732477628005,
0.986812255267055,0.987798766302167),(0.988732477628005,0.988732477628005,
0.988732477628005,0.986812255267055,0.987798766302167)))
REPRESENTATION_ITEM('')
SURFACE()
);
#1110=(
BOUNDED_SURFACE()
B_SPLINE_SURFACE(1,2,((#112194,#112195,#112196),(#112197,#112198,#112199)),
 .UNSPECIFIED.,.F.,.F.,.F.)
B_SPLINE_SURFACE_WITH_KNOTS((2,2),(3,3),(0.,0.289681084359929),(0.262994994770444,
0.280433083165913),.UNSPECIFIED.)
GEOMETRIC_REPRESENTATION_ITEM()
RATIONAL_B_SPLINE_SURFACE(((0.989123653000983,0.991350813683904,0.996566619267863),
(0.989123653000983,0.991350813683904,0.996566619267863)))
REPRESENTATION_ITEM('')
SURFACE()
);
#1111=(
BOUNDED_SURFACE()
B_SPLINE_SURFACE(1,2,((#112208,#112209,#112210,#112211,#112212),(#112213,
#112214,#112215,#112216,#112217)),.UNSPECIFIED.,.F.,.F.,.F.)
B_SPLINE_SURFACE_WITH_KNOTS((2,2),(3,2,3),(0.,0.290398665157378),(0.452333244847814,
0.452924869174518,0.470122329512321),.UNSPECIFIED.)
GEOMETRIC_REPRESENTATION_ITEM()
RATIONAL_B_SPLINE_SURFACE(((0.988732477628005,0.988732477628005,0.988732477628005,
0.986812255267055,0.987798766302167),(0.988732477628005,0.988732477628005,
0.988732477628005,0.986812255267055,0.987798766302167)))
REPRESENTATION_ITEM('')
SURFACE()
);
#1112=(
BOUNDED_SURFACE()
B_SPLINE_SURFACE(1,2,((#112219,#112220,#112221),(#112222,#112223,#112224)),
 .UNSPECIFIED.,.F.,.F.,.F.)
B_SPLINE_SURFACE_WITH_KNOTS((2,2),(3,3),(0.,0.289681084359937),(0.262994994770443,
0.280433083165913),.UNSPECIFIED.)
GEOMETRIC_REPRESENTATION_ITEM()
RATIONAL_B_SPLINE_SURFACE(((0.989123653000983,0.991350813683904,0.996566619267863),
(0.989123653000983,0.991350813683904,0.996566619267863)))
REPRESENTATION_ITEM('')
SURFACE()
);
#1113=(
BOUNDED_SURFACE()
B_SPLINE_SURFACE(1,2,((#112233,#112234,#112235,#112236,#112237),(#112238,
#112239,#112240,#112241,#112242)),.UNSPECIFIED.,.F.,.F.,.F.)
B_SPLINE_SURFACE_WITH_KNOTS((2,2),(3,2,3),(0.,0.290398665156934),(0.452333244848014,
0.452924869174518,0.470122329512319),.UNSPECIFIED.)
GEOMETRIC_REPRESENTATION_ITEM()
RATIONAL_B_SPLINE_SURFACE(((0.988732477628005,0.988732477628005,0.988732477628005,
0.986812255267055,0.987798766302166),(0.988732477628005,0.988732477628005,
0.988732477628005,0.986812255267055,0.987798766302166)))
REPRESENTATION_ITEM('')
SURFACE()
);
#1114=(
BOUNDED_SURFACE()
B_SPLINE_SURFACE(1,2,((#112244,#112245,#112246),(#112247,#112248,#112249)),
 .UNSPECIFIED.,.F.,.F.,.F.)
B_SPLINE_SURFACE_WITH_KNOTS((2,2),(3,3),(0.,0.289681084359929),(0.262994994770443,
0.280433083165913),.UNSPECIFIED.)
GEOMETRIC_REPRESENTATION_ITEM()
RATIONAL_B_SPLINE_SURFACE(((0.989123653000983,0.991350813683904,0.996566619267863),
(0.989123653000983,0.991350813683904,0.996566619267863)))
REPRESENTATION_ITEM('')
SURFACE()
);
#1115=(
BOUNDED_SURFACE()
B_SPLINE_SURFACE(1,2,((#112258,#112259,#112260,#112261,#112262),(#112263,
#112264,#112265,#112266,#112267)),.UNSPECIFIED.,.F.,.F.,.F.)
B_SPLINE_SURFACE_WITH_KNOTS((2,2),(3,2,3),(0.,0.29039866515975),(0.452333244845127,
0.452924869174518,0.470122329512318),.UNSPECIFIED.)
GEOMETRIC_REPRESENTATION_ITEM()
RATIONAL_B_SPLINE_SURFACE(((0.988732477628005,0.988732477628005,0.988732477628005,
0.986812255267055,0.987798766302166),(0.988732477628005,0.988732477628005,
0.988732477628005,0.986812255267055,0.987798766302167)))
REPRESENTATION_ITEM('')
SURFACE()
);
#1116=(
BOUNDED_SURFACE()
B_SPLINE_SURFACE(1,2,((#112269,#112270,#112271),(#112272,#112273,#112274)),
 .UNSPECIFIED.,.F.,.F.,.F.)
B_SPLINE_SURFACE_WITH_KNOTS((2,2),(3,3),(0.,0.289681084359923),(0.262994994770443,
0.280433083165913),.UNSPECIFIED.)
GEOMETRIC_REPRESENTATION_ITEM()
RATIONAL_B_SPLINE_SURFACE(((0.989123653000983,0.991350813683904,0.996566619267863),
(0.989123653000983,0.991350813683904,0.996566619267863)))
REPRESENTATION_ITEM('')
SURFACE()
);
#1117=(
BOUNDED_SURFACE()
B_SPLINE_SURFACE(1,2,((#112283,#112284,#112285,#112286,#112287),(#112288,
#112289,#112290,#112291,#112292)),.UNSPECIFIED.,.F.,.F.,.F.)
B_SPLINE_SURFACE_WITH_KNOTS((2,2),(3,2,3),(0.,0.29039866518354),(0.452333244822635,
0.452924869174506,0.470122329512318),.UNSPECIFIED.)
GEOMETRIC_REPRESENTATION_ITEM()
RATIONAL_B_SPLINE_SURFACE(((0.988732477628008,0.988732477628008,0.988732477628008,
0.986812255267055,0.987798766302166),(0.988732477628008,0.988732477628008,
0.988732477628008,0.986812255267054,0.987798766302166)))
REPRESENTATION_ITEM('')
SURFACE()
);
#1118=(
BOUNDED_SURFACE()
B_SPLINE_SURFACE(1,2,((#112294,#112295,#112296),(#112297,#112298,#112299)),
 .UNSPECIFIED.,.F.,.F.,.F.)
B_SPLINE_SURFACE_WITH_KNOTS((2,2),(3,3),(0.,0.289681084359921),(0.262994994770443,
0.280433083165913),.UNSPECIFIED.)
GEOMETRIC_REPRESENTATION_ITEM()
RATIONAL_B_SPLINE_SURFACE(((0.989123653000983,0.991350813683904,0.996566619267864),
(0.989123653000983,0.991350813683904,0.996566619267864)))
REPRESENTATION_ITEM('')
SURFACE()
);
#1119=(
BOUNDED_SURFACE()
B_SPLINE_SURFACE(1,2,((#112308,#112309,#112310,#112311,#112312),(#112313,
#112314,#112315,#112316,#112317)),.UNSPECIFIED.,.F.,.F.,.F.)
B_SPLINE_SURFACE_WITH_KNOTS((2,2),(3,2,3),(0.,0.290398665168458),(0.452333244836591,
0.452924869174517,0.470122329512318),.UNSPECIFIED.)
GEOMETRIC_REPRESENTATION_ITEM()
RATIONAL_B_SPLINE_SURFACE(((0.988732477628005,0.988732477628005,0.988732477628005,
0.986812255267055,0.987798766302167),(0.988732477628005,0.988732477628005,
0.988732477628005,0.986812255267055,0.987798766302167)))
REPRESENTATION_ITEM('')
SURFACE()
);
#1120=(
BOUNDED_SURFACE()
B_SPLINE_SURFACE(1,2,((#112319,#112320,#112321),(#112322,#112323,#112324)),
 .UNSPECIFIED.,.F.,.F.,.F.)
B_SPLINE_SURFACE_WITH_KNOTS((2,2),(3,3),(0.,0.289681084359922),(0.262994994770443,
0.280433083165913),.UNSPECIFIED.)
GEOMETRIC_REPRESENTATION_ITEM()
RATIONAL_B_SPLINE_SURFACE(((0.989123653000983,0.991350813683904,0.996566619267863),
(0.989123653000983,0.991350813683904,0.996566619267863)))
REPRESENTATION_ITEM('')
SURFACE()
);
#1121=(
BOUNDED_SURFACE()
B_SPLINE_SURFACE(1,2,((#112333,#112334,#112335,#112336,#112337),(#112338,
#112339,#112340,#112341,#112342)),.UNSPECIFIED.,.F.,.F.,.F.)
B_SPLINE_SURFACE_WITH_KNOTS((2,2),(3,2,3),(0.,0.290398665166776),(0.452333244838288,
0.452924869174517,0.470122329512318),.UNSPECIFIED.)
GEOMETRIC_REPRESENTATION_ITEM()
RATIONAL_B_SPLINE_SURFACE(((0.988732477628005,0.988732477628005,0.988732477628005,
0.986812255267055,0.987798766302166),(0.988732477628005,0.988732477628005,
0.988732477628005,0.986812255267055,0.987798766302166)))
REPRESENTATION_ITEM('')
SURFACE()
);
#1122=(
BOUNDED_SURFACE()
B_SPLINE_SURFACE(1,2,((#112344,#112345,#112346,#112347,#112348),(#112349,
#112350,#112351,#112352,#112353)),.UNSPECIFIED.,.F.,.F.,.F.)
B_SPLINE_SURFACE_WITH_KNOTS((2,2),(3,2,3),(0.,0.289681084359925),(0.400939219852743,
0.418312080773439,0.418485809382646),.UNSPECIFIED.)
GEOMETRIC_REPRESENTATION_ITEM()
RATIONAL_B_SPLINE_SURFACE(((0.988105937622242,0.989485911589766,0.993832214116773,
0.993832214116773,0.993832214116773),(0.988105937622242,0.989485911589766,
0.993832214116773,0.993832214116773,0.993832214116773)))
REPRESENTATION_ITEM('')
SURFACE()
);
#1123=(
BOUNDED_SURFACE()
B_SPLINE_SURFACE(1,2,((#112364,#112365,#112366,#112367,#112368),(#112369,
#112370,#112371,#112372,#112373)),.UNSPECIFIED.,.F.,.F.,.F.)
B_SPLINE_SURFACE_WITH_KNOTS((2,2),(3,2,3),(0.,0.289807040991894),(0.314770575782761,
0.314942866188516,0.332171906764074),.UNSPECIFIED.)
GEOMETRIC_REPRESENTATION_ITEM()
RATIONAL_B_SPLINE_SURFACE(((0.987877375613931,0.987877375613931,0.987877375613931,
0.986779141655835,0.988598326347701),(0.987877375613931,0.987877375613931,
0.987877375613931,0.986779141655835,0.988598326347701)))
REPRESENTATION_ITEM('')
SURFACE()
);
#1124=(
BOUNDED_SURFACE()
B_SPLINE_SURFACE(1,2,((#112399,#112400,#112401,#112402,#112403),(#112404,
#112405,#112406,#112407,#112408)),.UNSPECIFIED.,.F.,.F.,.F.)
B_SPLINE_SURFACE_WITH_KNOTS((2,2),(3,2,3),(0.,0.289681084359929),(0.400939219852743,
0.418312080773434,0.418485809382641),.UNSPECIFIED.)
GEOMETRIC_REPRESENTATION_ITEM()
RATIONAL_B_SPLINE_SURFACE(((0.988105937622242,0.989485911589766,0.99383221411677,
0.99383221411677,0.99383221411677),(0.988105937622242,0.989485911589766,
0.99383221411677,0.99383221411677,0.99383221411677)))
REPRESENTATION_ITEM('')
SURFACE()
);
#1125=(
BOUNDED_SURFACE()
B_SPLINE_SURFACE(1,2,((#112410,#112411,#112412,#112413,#112414),(#112415,
#112416,#112417,#112418,#112419)),.UNSPECIFIED.,.F.,.F.,.F.)
B_SPLINE_SURFACE_WITH_KNOTS((2,2),(3,2,3),(0.,0.289807040992009),(0.314770575782761,
0.314942866188516,0.332171906764074),.UNSPECIFIED.)
GEOMETRIC_REPRESENTATION_ITEM()
RATIONAL_B_SPLINE_SURFACE(((0.987877375613931,0.987877375613931,0.987877375613931,
0.986779141655835,0.988598326347701),(0.987877375613931,0.987877375613931,
0.987877375613931,0.986779141655835,0.988598326347701)))
REPRESENTATION_ITEM('')
SURFACE()
);
#1126=(
BOUNDED_SURFACE()
B_SPLINE_SURFACE(1,2,((#112445,#112446,#112447,#112448,#112449),(#112450,
#112451,#112452,#112453,#112454)),.UNSPECIFIED.,.F.,.F.,.F.)
B_SPLINE_SURFACE_WITH_KNOTS((2,2),(3,2,3),(0.,0.289681084359929),(0.400939219852742,
0.418312080773434,0.418485809382641),.UNSPECIFIED.)
GEOMETRIC_REPRESENTATION_ITEM()
RATIONAL_B_SPLINE_SURFACE(((0.988105937622242,0.989485911589766,0.99383221411677,
0.99383221411677,0.99383221411677),(0.988105937622242,0.989485911589766,
0.99383221411677,0.99383221411677,0.99383221411677)))
REPRESENTATION_ITEM('')
SURFACE()
);
#1127=(
BOUNDED_SURFACE()
B_SPLINE_SURFACE(1,2,((#112456,#112457,#112458,#112459,#112460),(#112461,
#112462,#112463,#112464,#112465)),.UNSPECIFIED.,.F.,.F.,.F.)
B_SPLINE_SURFACE_WITH_KNOTS((2,2),(3,2,3),(0.,0.289807040993042),(0.314770575782756,
0.314942866188511,0.332171906764072),.UNSPECIFIED.)
GEOMETRIC_REPRESENTATION_ITEM()
RATIONAL_B_SPLINE_SURFACE(((0.987877375613932,0.987877375613932,0.987877375613932,
0.986779141655835,0.988598326347701),(0.987877375613932,0.987877375613932,
0.987877375613932,0.986779141655835,0.988598326347701)))
REPRESENTATION_ITEM('')
SURFACE()
);
#1128=(
BOUNDED_SURFACE()
B_SPLINE_SURFACE(1,2,((#112491,#112492,#112493,#112494,#112495),(#112496,
#112497,#112498,#112499,#112500)),.UNSPECIFIED.,.F.,.F.,.F.)
B_SPLINE_SURFACE_WITH_KNOTS((2,2),(3,2,3),(0.,0.289681084359915),(0.40093921985274,
0.418312080773435,0.418485809382642),.UNSPECIFIED.)
GEOMETRIC_REPRESENTATION_ITEM()
RATIONAL_B_SPLINE_SURFACE(((0.988105937622242,0.989485911589765,0.99383221411677,
0.99383221411677,0.99383221411677),(0.988105937622242,0.989485911589765,
0.99383221411677,0.99383221411677,0.99383221411677)))
REPRESENTATION_ITEM('')
SURFACE()
);
#1129=(
BOUNDED_SURFACE()
B_SPLINE_SURFACE(1,2,((#112502,#112503,#112504,#112505,#112506),(#112507,
#112508,#112509,#112510,#112511)),.UNSPECIFIED.,.F.,.F.,.F.)
B_SPLINE_SURFACE_WITH_KNOTS((2,2),(3,2,3),(0.,0.289807040992772),(0.314770575782758,
0.314942866188513,0.332171906764074),.UNSPECIFIED.)
GEOMETRIC_REPRESENTATION_ITEM()
RATIONAL_B_SPLINE_SURFACE(((0.987877375613932,0.987877375613932,0.987877375613932,
0.986779141655835,0.988598326347701),(0.987877375613932,0.987877375613932,
0.987877375613932,0.986779141655835,0.988598326347701)))
REPRESENTATION_ITEM('')
SURFACE()
);
#1130=(
BOUNDED_SURFACE()
B_SPLINE_SURFACE(1,2,((#112537,#112538,#112539,#112540,#112541),(#112542,
#112543,#112544,#112545,#112546)),.UNSPECIFIED.,.F.,.F.,.F.)
B_SPLINE_SURFACE_WITH_KNOTS((2,2),(3,2,3),(0.,0.289681084359922),(0.400939219852742,
0.41831208077346,0.418485809382667),.UNSPECIFIED.)
GEOMETRIC_REPRESENTATION_ITEM()
RATIONAL_B_SPLINE_SURFACE(((0.988105937622242,0.989485911589768,0.993832214116783,
0.993832214116783,0.993832214116783),(0.988105937622242,0.989485911589768,
0.993832214116783,0.993832214116783,0.993832214116783)))
REPRESENTATION_ITEM('')
SURFACE()
);
#1131=(
BOUNDED_SURFACE()
B_SPLINE_SURFACE(1,2,((#112548,#112549,#112550,#112551,#112552),(#112553,
#112554,#112555,#112556,#112557)),.UNSPECIFIED.,.F.,.F.,.F.)
B_SPLINE_SURFACE_WITH_KNOTS((2,2),(3,2,3),(0.,0.2898070409925),(0.314770575782761,
0.314942866188516,0.332171906764074),.UNSPECIFIED.)
GEOMETRIC_REPRESENTATION_ITEM()
RATIONAL_B_SPLINE_SURFACE(((0.987877375613931,0.987877375613931,0.987877375613931,
0.986779141655835,0.988598326347701),(0.987877375613931,0.987877375613931,
0.987877375613931,0.986779141655835,0.988598326347701)))
REPRESENTATION_ITEM('')
SURFACE()
);
#1132=(
BOUNDED_SURFACE()
B_SPLINE_SURFACE(1,2,((#112583,#112584,#112585,#112586,#112587),(#112588,
#112589,#112590,#112591,#112592)),.UNSPECIFIED.,.F.,.F.,.F.)
B_SPLINE_SURFACE_WITH_KNOTS((2,2),(3,2,3),(0.,0.289681084359915),(0.400939219852743,
0.418312080773434,0.418485809382641),.UNSPECIFIED.)
GEOMETRIC_REPRESENTATION_ITEM()
RATIONAL_B_SPLINE_SURFACE(((0.988105937622242,0.989485911589766,0.99383221411677,
0.99383221411677,0.99383221411677),(0.988105937622242,0.989485911589766,
0.99383221411677,0.99383221411677,0.99383221411677)))
REPRESENTATION_ITEM('')
SURFACE()
);
#1133=(
BOUNDED_SURFACE()
B_SPLINE_SURFACE(1,2,((#112594,#112595,#112596,#112597,#112598),(#112599,
#112600,#112601,#112602,#112603)),.UNSPECIFIED.,.F.,.F.,.F.)
B_SPLINE_SURFACE_WITH_KNOTS((2,2),(3,2,3),(0.,0.289807040992675),(0.314770575782761,
0.314942866188516,0.332171906764074),.UNSPECIFIED.)
GEOMETRIC_REPRESENTATION_ITEM()
RATIONAL_B_SPLINE_SURFACE(((0.987877375613931,0.987877375613931,0.987877375613931,
0.986779141655835,0.988598326347701),(0.987877375613931,0.987877375613931,
0.987877375613931,0.986779141655835,0.988598326347701)))
REPRESENTATION_ITEM('')
SURFACE()
);
#1134=(
BOUNDED_SURFACE()
B_SPLINE_SURFACE(1,2,((#112629,#112630,#112631,#112632,#112633),(#112634,
#112635,#112636,#112637,#112638)),.UNSPECIFIED.,.F.,.F.,.F.)
B_SPLINE_SURFACE_WITH_KNOTS((2,2),(3,2,3),(0.,0.289681084359923),(0.400939219852743,
0.418312080773434,0.418485809382641),.UNSPECIFIED.)
GEOMETRIC_REPRESENTATION_ITEM()
RATIONAL_B_SPLINE_SURFACE(((0.988105937622242,0.989485911589766,0.99383221411677,
0.99383221411677,0.99383221411677),(0.988105937622242,0.989485911589766,
0.99383221411677,0.99383221411677,0.99383221411677)))
REPRESENTATION_ITEM('')
SURFACE()
);
#1135=(
BOUNDED_SURFACE()
B_SPLINE_SURFACE(1,2,((#112640,#112641,#112642,#112643,#112644),(#112645,
#112646,#112647,#112648,#112649)),.UNSPECIFIED.,.F.,.F.,.F.)
B_SPLINE_SURFACE_WITH_KNOTS((2,2),(3,2,3),(0.,0.289807040991735),(0.314770575782761,
0.314942866188516,0.332171906764071),.UNSPECIFIED.)
GEOMETRIC_REPRESENTATION_ITEM()
RATIONAL_B_SPLINE_SURFACE(((0.987877375613931,0.987877375613931,0.987877375613931,
0.986779141655835,0.9885983263477),(0.987877375613931,0.987877375613931,
0.987877375613931,0.986779141655835,0.9885983263477)))
REPRESENTATION_ITEM('')
SURFACE()
);
#1136=(
BOUNDED_SURFACE()
B_SPLINE_SURFACE(1,2,((#112657,#112658,#112659,#112660,#112661),(#112662,
#112663,#112664,#112665,#112666)),.UNSPECIFIED.,.F.,.F.,.F.)
B_SPLINE_SURFACE_WITH_KNOTS((2,2),(3,2,3),(0.,0.289681084359923),(0.40093921985274,
0.418312080773434,0.418485809382641),.UNSPECIFIED.)
GEOMETRIC_REPRESENTATION_ITEM()
RATIONAL_B_SPLINE_SURFACE(((0.988105937622241,0.989485911589765,0.99383221411677,
0.99383221411677,0.99383221411677),(0.988105937622241,0.989485911589765,
0.99383221411677,0.99383221411677,0.99383221411677)))
REPRESENTATION_ITEM('')
SURFACE()
);
#1137=(
BOUNDED_SURFACE()
B_SPLINE_SURFACE(1,2,((#112668,#112669,#112670,#112671,#112672),(#112673,
#112674,#112675,#112676,#112677)),.UNSPECIFIED.,.F.,.F.,.F.)
B_SPLINE_SURFACE_WITH_KNOTS((2,2),(3,2,3),(0.,0.289807040991743),(0.314770575782761,
0.314942866188516,0.332171906764072),.UNSPECIFIED.)
GEOMETRIC_REPRESENTATION_ITEM()
RATIONAL_B_SPLINE_SURFACE(((0.987877375613931,0.987877375613931,0.987877375613931,
0.986779141655835,0.9885983263477),(0.987877375613931,0.987877375613931,
0.987877375613931,0.986779141655835,0.9885983263477)))
REPRESENTATION_ITEM('')
SURFACE()
);
#1138=(
BOUNDED_SURFACE()
B_SPLINE_SURFACE(1,2,((#112703,#112704,#112705,#112706,#112707),(#112708,
#112709,#112710,#112711,#112712)),.UNSPECIFIED.,.F.,.F.,.F.)
B_SPLINE_SURFACE_WITH_KNOTS((2,2),(3,2,3),(0.,0.289681084359925),(0.40093921985274,
0.418312080773435,0.418485809382642),.UNSPECIFIED.)
GEOMETRIC_REPRESENTATION_ITEM()
RATIONAL_B_SPLINE_SURFACE(((0.988105937622242,0.989485911589765,0.99383221411677,
0.99383221411677,0.99383221411677),(0.988105937622242,0.989485911589765,
0.99383221411677,0.99383221411677,0.99383221411677)))
REPRESENTATION_ITEM('')
SURFACE()
);
#1139=(
BOUNDED_SURFACE()
B_SPLINE_SURFACE(1,2,((#112714,#112715,#112716,#112717,#112718),(#112719,
#112720,#112721,#112722,#112723)),.UNSPECIFIED.,.F.,.F.,.F.)
B_SPLINE_SURFACE_WITH_KNOTS((2,2),(3,2,3),(0.,0.289807040991848),(0.314770575782761,
0.314942866188516,0.332171906764071),.UNSPECIFIED.)
GEOMETRIC_REPRESENTATION_ITEM()
RATIONAL_B_SPLINE_SURFACE(((0.987877375613931,0.987877375613931,0.987877375613931,
0.986779141655835,0.9885983263477),(0.987877375613931,0.987877375613931,
0.987877375613931,0.986779141655835,0.9885983263477)))
REPRESENTATION_ITEM('')
SURFACE()
);
#1140=(
BOUNDED_SURFACE()
B_SPLINE_SURFACE(1,2,((#112749,#112750,#112751,#112752,#112753),(#112754,
#112755,#112756,#112757,#112758)),.UNSPECIFIED.,.F.,.F.,.F.)
B_SPLINE_SURFACE_WITH_KNOTS((2,2),(3,2,3),(0.,0.28968108435993),(0.40093921985274,
0.418312080773434,0.418485809382641),.UNSPECIFIED.)
GEOMETRIC_REPRESENTATION_ITEM()
RATIONAL_B_SPLINE_SURFACE(((0.988105937622242,0.989485911589765,0.99383221411677,
0.99383221411677,0.99383221411677),(0.988105937622241,0.989485911589765,
0.99383221411677,0.99383221411677,0.99383221411677)))
REPRESENTATION_ITEM('')
SURFACE()
);
#1141=(
BOUNDED_SURFACE()
B_SPLINE_SURFACE(1,2,((#112760,#112761,#112762,#112763,#112764),(#112765,
#112766,#112767,#112768,#112769)),.UNSPECIFIED.,.F.,.F.,.F.)
B_SPLINE_SURFACE_WITH_KNOTS((2,2),(3,2,3),(0.,0.289807040991791),(0.314770575782761,
0.314942866188516,0.332171906764072),.UNSPECIFIED.)
GEOMETRIC_REPRESENTATION_ITEM()
RATIONAL_B_SPLINE_SURFACE(((0.987877375613931,0.987877375613931,0.987877375613931,
0.986779141655835,0.988598326347701),(0.987877375613931,0.987877375613931,
0.987877375613931,0.986779141655836,0.988598326347701)))
REPRESENTATION_ITEM('')
SURFACE()
);
#1142=(
BOUNDED_SURFACE()
B_SPLINE_SURFACE(1,2,((#112795,#112796,#112797,#112798,#112799),(#112800,
#112801,#112802,#112803,#112804)),.UNSPECIFIED.,.F.,.F.,.F.)
B_SPLINE_SURFACE_WITH_KNOTS((2,2),(3,2,3),(0.,0.289681084359921),(0.400939219852741,
0.418312080773434,0.418485809382641),.UNSPECIFIED.)
GEOMETRIC_REPRESENTATION_ITEM()
RATIONAL_B_SPLINE_SURFACE(((0.988105937622242,0.989485911589765,0.99383221411677,
0.99383221411677,0.99383221411677),(0.988105937622242,0.989485911589765,
0.99383221411677,0.99383221411677,0.99383221411677)))
REPRESENTATION_ITEM('')
SURFACE()
);
#1143=(
BOUNDED_SURFACE()
B_SPLINE_SURFACE(1,2,((#112806,#112807,#112808,#112809,#112810),(#112811,
#112812,#112813,#112814,#112815)),.UNSPECIFIED.,.F.,.F.,.F.)
B_SPLINE_SURFACE_WITH_KNOTS((2,2),(3,2,3),(0.,0.289807040991756),(0.314770575782761,
0.314942866188516,0.332171906764071),.UNSPECIFIED.)
GEOMETRIC_REPRESENTATION_ITEM()
RATIONAL_B_SPLINE_SURFACE(((0.987877375613931,0.987877375613931,0.987877375613931,
0.986779141655835,0.9885983263477),(0.987877375613931,0.987877375613931,
0.987877375613931,0.986779141655835,0.9885983263477)))
REPRESENTATION_ITEM('')
SURFACE()
);
#1144=(
BOUNDED_SURFACE()
B_SPLINE_SURFACE(1,2,((#112841,#112842,#112843,#112844,#112845),(#112846,
#112847,#112848,#112849,#112850)),.UNSPECIFIED.,.F.,.F.,.F.)
B_SPLINE_SURFACE_WITH_KNOTS((2,2),(3,2,3),(0.,0.289681084359919),(0.40093921985274,
0.418312080773434,0.418485809382641),.UNSPECIFIED.)
GEOMETRIC_REPRESENTATION_ITEM()
RATIONAL_B_SPLINE_SURFACE(((0.988105937622242,0.989485911589765,0.99383221411677,
0.99383221411677,0.99383221411677),(0.988105937622241,0.989485911589765,
0.99383221411677,0.99383221411677,0.99383221411677)))
REPRESENTATION_ITEM('')
SURFACE()
);
#1145=(
BOUNDED_SURFACE()
B_SPLINE_SURFACE(1,2,((#112852,#112853,#112854,#112855,#112856),(#112857,
#112858,#112859,#112860,#112861)),.UNSPECIFIED.,.F.,.F.,.F.)
B_SPLINE_SURFACE_WITH_KNOTS((2,2),(3,2,3),(0.,0.289807040991712),(0.314770575782761,
0.314942866188516,0.332171906764074),.UNSPECIFIED.)
GEOMETRIC_REPRESENTATION_ITEM()
RATIONAL_B_SPLINE_SURFACE(((0.987877375613931,0.987877375613931,0.987877375613931,
0.986779141655835,0.988598326347701),(0.987877375613931,0.987877375613931,
0.987877375613931,0.986779141655835,0.988598326347701)))
REPRESENTATION_ITEM('')
SURFACE()
);
#1146=(
BOUNDED_SURFACE()
B_SPLINE_SURFACE(1,2,((#112887,#112888,#112889,#112890,#112891),(#112892,
#112893,#112894,#112895,#112896)),.UNSPECIFIED.,.F.,.F.,.F.)
B_SPLINE_SURFACE_WITH_KNOTS((2,2),(3,2,3),(0.,0.289681084359925),(0.400939219852743,
0.418312080773434,0.418485809382641),.UNSPECIFIED.)
GEOMETRIC_REPRESENTATION_ITEM()
RATIONAL_B_SPLINE_SURFACE(((0.988105937622242,0.989485911589766,0.99383221411677,
0.99383221411677,0.99383221411677),(0.988105937622242,0.989485911589766,
0.99383221411677,0.99383221411677,0.99383221411677)))
REPRESENTATION_ITEM('')
SURFACE()
);
#1147=(
BOUNDED_SURFACE()
B_SPLINE_SURFACE(1,2,((#112898,#112899,#112900,#112901,#112902),(#112903,
#112904,#112905,#112906,#112907)),.UNSPECIFIED.,.F.,.F.,.F.)
B_SPLINE_SURFACE_WITH_KNOTS((2,2),(3,2,3),(0.,0.289807040991569),(0.314770575782761,
0.314942866188516,0.332171906764074),.UNSPECIFIED.)
GEOMETRIC_REPRESENTATION_ITEM()
RATIONAL_B_SPLINE_SURFACE(((0.987877375613931,0.987877375613931,0.987877375613931,
0.986779141655835,0.988598326347701),(0.987877375613931,0.987877375613931,
0.987877375613931,0.986779141655835,0.988598326347701)))
REPRESENTATION_ITEM('')
SURFACE()
);
#1148=(
BOUNDED_SURFACE()
B_SPLINE_SURFACE(1,2,((#112933,#112934,#112935,#112936,#112937),(#112938,
#112939,#112940,#112941,#112942)),.UNSPECIFIED.,.F.,.F.,.F.)
B_SPLINE_SURFACE_WITH_KNOTS((2,2),(3,2,3),(0.,0.289681084359925),(0.400939219852742,
0.418312080773434,0.418485809382641),.UNSPECIFIED.)
GEOMETRIC_REPRESENTATION_ITEM()
RATIONAL_B_SPLINE_SURFACE(((0.988105937622242,0.989485911589766,0.99383221411677,
0.99383221411677,0.99383221411677),(0.988105937622242,0.989485911589766,
0.99383221411677,0.99383221411677,0.99383221411677)))
REPRESENTATION_ITEM('')
SURFACE()
);
#1149=(
BOUNDED_SURFACE()
B_SPLINE_SURFACE(1,2,((#112944,#112945,#112946,#112947,#112948),(#112949,
#112950,#112951,#112952,#112953)),.UNSPECIFIED.,.F.,.F.,.F.)
B_SPLINE_SURFACE_WITH_KNOTS((2,2),(3,2,3),(0.,0.289807040991565),(0.314770575782761,
0.314942866188516,0.332171906764074),.UNSPECIFIED.)
GEOMETRIC_REPRESENTATION_ITEM()
RATIONAL_B_SPLINE_SURFACE(((0.987877375613931,0.987877375613931,0.987877375613931,
0.986779141655835,0.988598326347701),(0.987877375613931,0.987877375613931,
0.987877375613931,0.986779141655835,0.988598326347701)))
REPRESENTATION_ITEM('')
SURFACE()
);
#1150=(
BOUNDED_SURFACE()
B_SPLINE_SURFACE(1,2,((#112979,#112980,#112981,#112982,#112983),(#112984,
#112985,#112986,#112987,#112988)),.UNSPECIFIED.,.F.,.F.,.F.)
B_SPLINE_SURFACE_WITH_KNOTS((2,2),(3,2,3),(0.,0.289681084359926),(0.400939219852743,
0.418312080773434,0.418485809382641),.UNSPECIFIED.)
GEOMETRIC_REPRESENTATION_ITEM()
RATIONAL_B_SPLINE_SURFACE(((0.988105937622242,0.989485911589766,0.99383221411677,
0.99383221411677,0.99383221411677),(0.988105937622242,0.989485911589766,
0.99383221411677,0.99383221411677,0.99383221411677)))
REPRESENTATION_ITEM('')
SURFACE()
);
#1151=(
BOUNDED_SURFACE()
B_SPLINE_SURFACE(1,2,((#112990,#112991,#112992,#112993,#112994),(#112995,
#112996,#112997,#112998,#112999)),.UNSPECIFIED.,.F.,.F.,.F.)
B_SPLINE_SURFACE_WITH_KNOTS((2,2),(3,2,3),(0.,0.289807040991566),(0.314770575782761,
0.314942866188516,0.332171906764074),.UNSPECIFIED.)
GEOMETRIC_REPRESENTATION_ITEM()
RATIONAL_B_SPLINE_SURFACE(((0.987877375613931,0.987877375613931,0.987877375613931,
0.986779141655835,0.988598326347701),(0.987877375613931,0.987877375613931,
0.987877375613931,0.986779141655835,0.988598326347701)))
REPRESENTATION_ITEM('')
SURFACE()
);
#1152=(
BOUNDED_SURFACE()
B_SPLINE_SURFACE(1,2,((#113025,#113026,#113027,#113028,#113029),(#113030,
#113031,#113032,#113033,#113034)),.UNSPECIFIED.,.F.,.F.,.F.)
B_SPLINE_SURFACE_WITH_KNOTS((2,2),(3,2,3),(0.,0.289681084359931),(0.400939219852743,
0.418312080773435,0.418485809382642),.UNSPECIFIED.)
GEOMETRIC_REPRESENTATION_ITEM()
RATIONAL_B_SPLINE_SURFACE(((0.988105937622242,0.989485911589766,0.993832214116771,
0.993832214116771,0.993832214116771),(0.988105937622242,0.989485911589766,
0.993832214116771,0.993832214116771,0.993832214116771)))
REPRESENTATION_ITEM('')
SURFACE()
);
#1153=(
BOUNDED_SURFACE()
B_SPLINE_SURFACE(1,2,((#113036,#113037,#113038,#113039,#113040),(#113041,
#113042,#113043,#113044,#113045)),.UNSPECIFIED.,.F.,.F.,.F.)
B_SPLINE_SURFACE_WITH_KNOTS((2,2),(3,2,3),(0.,0.289807040991562),(0.314770575782761,
0.314942866188516,0.332171906764074),.UNSPECIFIED.)
GEOMETRIC_REPRESENTATION_ITEM()
RATIONAL_B_SPLINE_SURFACE(((0.987877375613931,0.987877375613931,0.987877375613931,
0.986779141655835,0.988598326347701),(0.987877375613931,0.987877375613931,
0.987877375613931,0.986779141655835,0.988598326347701)))
REPRESENTATION_ITEM('')
SURFACE()
);
#1154=(
BOUNDED_SURFACE()
B_SPLINE_SURFACE(1,2,((#113071,#113072,#113073,#113074,#113075),(#113076,
#113077,#113078,#113079,#113080)),.UNSPECIFIED.,.F.,.F.,.F.)
B_SPLINE_SURFACE_WITH_KNOTS((2,2),(3,2,3),(0.,0.289681084359919),(0.400939219852743,
0.418312080773434,0.418485809382641),.UNSPECIFIED.)
GEOMETRIC_REPRESENTATION_ITEM()
RATIONAL_B_SPLINE_SURFACE(((0.988105937622242,0.989485911589766,0.99383221411677,
0.99383221411677,0.99383221411677),(0.988105937622242,0.989485911589766,
0.99383221411677,0.99383221411677,0.99383221411677)))
REPRESENTATION_ITEM('')
SURFACE()
);
#1155=(
BOUNDED_SURFACE()
B_SPLINE_SURFACE(1,2,((#113082,#113083,#113084,#113085,#113086),(#113087,
#113088,#113089,#113090,#113091)),.UNSPECIFIED.,.F.,.F.,.F.)
B_SPLINE_SURFACE_WITH_KNOTS((2,2),(3,2,3),(0.,0.289807040991562),(0.314770575782761,
0.314942866188516,0.332171906764074),.UNSPECIFIED.)
GEOMETRIC_REPRESENTATION_ITEM()
RATIONAL_B_SPLINE_SURFACE(((0.987877375613931,0.987877375613931,0.987877375613931,
0.986779141655835,0.988598326347701),(0.987877375613931,0.987877375613931,
0.987877375613931,0.986779141655835,0.988598326347701)))
REPRESENTATION_ITEM('')
SURFACE()
);
#1156=(
BOUNDED_SURFACE()
B_SPLINE_SURFACE(1,2,((#113117,#113118,#113119,#113120,#113121),(#113122,
#113123,#113124,#113125,#113126)),.UNSPECIFIED.,.F.,.F.,.F.)
B_SPLINE_SURFACE_WITH_KNOTS((2,2),(3,2,3),(0.,0.28968108435992),(0.400939219852743,
0.418312080773434,0.418485809382641),.UNSPECIFIED.)
GEOMETRIC_REPRESENTATION_ITEM()
RATIONAL_B_SPLINE_SURFACE(((0.988105937622242,0.989485911589766,0.99383221411677,
0.99383221411677,0.99383221411677),(0.988105937622242,0.989485911589766,
0.99383221411677,0.99383221411677,0.99383221411677)))
REPRESENTATION_ITEM('')
SURFACE()
);
#1157=(
BOUNDED_SURFACE()
B_SPLINE_SURFACE(1,2,((#113128,#113129,#113130,#113131,#113132),(#113133,
#113134,#113135,#113136,#113137)),.UNSPECIFIED.,.F.,.F.,.F.)
B_SPLINE_SURFACE_WITH_KNOTS((2,2),(3,2,3),(0.,0.289807040991671),(0.314770575782761,
0.314942866188516,0.332171906764072),.UNSPECIFIED.)
GEOMETRIC_REPRESENTATION_ITEM()
RATIONAL_B_SPLINE_SURFACE(((0.987877375613931,0.987877375613931,0.987877375613931,
0.986779141655835,0.9885983263477),(0.987877375613931,0.987877375613931,
0.987877375613931,0.986779141655836,0.988598326347701)))
REPRESENTATION_ITEM('')
SURFACE()
);
#1158=(
BOUNDED_SURFACE()
B_SPLINE_SURFACE(1,2,((#113163,#113164,#113165,#113166,#113167),(#113168,
#113169,#113170,#113171,#113172)),.UNSPECIFIED.,.F.,.F.,.F.)
B_SPLINE_SURFACE_WITH_KNOTS((2,2),(3,2,3),(0.,0.289681084359922),(0.40093921985274,
0.418312080773434,0.418485809382641),.UNSPECIFIED.)
GEOMETRIC_REPRESENTATION_ITEM()
RATIONAL_B_SPLINE_SURFACE(((0.988105937622242,0.989485911589765,0.99383221411677,
0.99383221411677,0.99383221411677),(0.988105937622242,0.989485911589765,
0.99383221411677,0.99383221411677,0.99383221411677)))
REPRESENTATION_ITEM('')
SURFACE()
);
#1159=(
BOUNDED_SURFACE()
B_SPLINE_SURFACE(1,2,((#113174,#113175,#113176,#113177,#113178),(#113179,
#113180,#113181,#113182,#113183)),.UNSPECIFIED.,.F.,.F.,.F.)
B_SPLINE_SURFACE_WITH_KNOTS((2,2),(3,2,3),(0.,0.289807040992971),(0.314770575782761,
0.314942866188516,0.332171906764072),.UNSPECIFIED.)
GEOMETRIC_REPRESENTATION_ITEM()
RATIONAL_B_SPLINE_SURFACE(((0.987877375613931,0.987877375613931,0.987877375613931,
0.986779141655835,0.9885983263477),(0.987877375613931,0.987877375613931,
0.987877375613931,0.986779141655835,0.9885983263477)))
REPRESENTATION_ITEM('')
SURFACE()
);
#1160=(
BOUNDED_SURFACE()
B_SPLINE_SURFACE(1,2,((#113209,#113210,#113211,#113212,#113213),(#113214,
#113215,#113216,#113217,#113218)),.UNSPECIFIED.,.F.,.F.,.F.)
B_SPLINE_SURFACE_WITH_KNOTS((2,2),(3,2,3),(0.,0.28968108435992),(0.40093921985274,
0.418312080773434,0.418485809382641),.UNSPECIFIED.)
GEOMETRIC_REPRESENTATION_ITEM()
RATIONAL_B_SPLINE_SURFACE(((0.988105937622242,0.989485911589765,0.99383221411677,
0.99383221411677,0.99383221411677),(0.988105937622242,0.989485911589765,
0.99383221411677,0.99383221411677,0.99383221411677)))
REPRESENTATION_ITEM('')
SURFACE()
);
#1161=(
BOUNDED_SURFACE()
B_SPLINE_SURFACE(1,2,((#113220,#113221,#113222,#113223,#113224),(#113225,
#113226,#113227,#113228,#113229)),.UNSPECIFIED.,.F.,.F.,.F.)
B_SPLINE_SURFACE_WITH_KNOTS((2,2),(3,2,3),(0.,0.289807040991813),(0.314770575782761,
0.314942866188516,0.332171906764074),.UNSPECIFIED.)
GEOMETRIC_REPRESENTATION_ITEM()
RATIONAL_B_SPLINE_SURFACE(((0.987877375613931,0.987877375613931,0.987877375613931,
0.986779141655835,0.988598326347701),(0.987877375613931,0.987877375613931,
0.987877375613931,0.986779141655835,0.988598326347701)))
REPRESENTATION_ITEM('')
SURFACE()
);
#1162=(
BOUNDED_SURFACE()
B_SPLINE_SURFACE(1,2,((#113255,#113256,#113257,#113258,#113259),(#113260,
#113261,#113262,#113263,#113264)),.UNSPECIFIED.,.F.,.F.,.F.)
B_SPLINE_SURFACE_WITH_KNOTS((2,2),(3,2,3),(0.,0.289681084359921),(0.400939219852743,
0.418312080773434,0.418485809382641),.UNSPECIFIED.)
GEOMETRIC_REPRESENTATION_ITEM()
RATIONAL_B_SPLINE_SURFACE(((0.988105937622242,0.989485911589766,0.99383221411677,
0.99383221411677,0.99383221411677),(0.988105937622242,0.989485911589766,
0.99383221411677,0.99383221411677,0.99383221411677)))
REPRESENTATION_ITEM('')
SURFACE()
);
#1163=(
BOUNDED_SURFACE()
B_SPLINE_SURFACE(1,2,((#113266,#113267,#113268,#113269,#113270),(#113271,
#113272,#113273,#113274,#113275)),.UNSPECIFIED.,.F.,.F.,.F.)
B_SPLINE_SURFACE_WITH_KNOTS((2,2),(3,2,3),(0.,0.28980704099156),(0.314770575782761,
0.314942866188516,0.332171906764072),.UNSPECIFIED.)
GEOMETRIC_REPRESENTATION_ITEM()
RATIONAL_B_SPLINE_SURFACE(((0.987877375613931,0.987877375613931,0.987877375613931,
0.986779141655835,0.9885983263477),(0.987877375613931,0.987877375613931,
0.987877375613931,0.986779141655835,0.9885983263477)))
REPRESENTATION_ITEM('')
SURFACE()
);
#1164=(
BOUNDED_SURFACE()
B_SPLINE_SURFACE(1,2,((#113301,#113302,#113303,#113304,#113305),(#113306,
#113307,#113308,#113309,#113310)),.UNSPECIFIED.,.F.,.F.,.F.)
B_SPLINE_SURFACE_WITH_KNOTS((2,2),(3,2,3),(0.,0.289681084359923),(0.400939219852741,
0.418312080773434,0.418485809382641),.UNSPECIFIED.)
GEOMETRIC_REPRESENTATION_ITEM()
RATIONAL_B_SPLINE_SURFACE(((0.988105937622242,0.989485911589765,0.99383221411677,
0.99383221411677,0.99383221411677),(0.988105937622242,0.989485911589765,
0.99383221411677,0.99383221411677,0.99383221411677)))
REPRESENTATION_ITEM('')
SURFACE()
);
#1165=(
BOUNDED_SURFACE()
B_SPLINE_SURFACE(1,2,((#113312,#113313,#113314,#113315,#113316),(#113317,
#113318,#113319,#113320,#113321)),.UNSPECIFIED.,.F.,.F.,.F.)
B_SPLINE_SURFACE_WITH_KNOTS((2,2),(3,2,3),(0.,0.28980704099156),(0.314770575782761,
0.314942866188516,0.332171906764072),.UNSPECIFIED.)
GEOMETRIC_REPRESENTATION_ITEM()
RATIONAL_B_SPLINE_SURFACE(((0.987877375613931,0.987877375613931,0.987877375613931,
0.986779141655835,0.988598326347701),(0.987877375613931,0.987877375613931,
0.987877375613931,0.986779141655836,0.988598326347701)))
REPRESENTATION_ITEM('')
SURFACE()
);
#1166=(
BOUNDED_SURFACE()
B_SPLINE_SURFACE(1,2,((#113347,#113348,#113349,#113350,#113351),(#113352,
#113353,#113354,#113355,#113356)),.UNSPECIFIED.,.F.,.F.,.F.)
B_SPLINE_SURFACE_WITH_KNOTS((2,2),(3,2,3),(0.,0.289681084359917),(0.40093921985274,
0.418312080773434,0.418485809382641),.UNSPECIFIED.)
GEOMETRIC_REPRESENTATION_ITEM()
RATIONAL_B_SPLINE_SURFACE(((0.988105937622242,0.989485911589765,0.99383221411677,
0.99383221411677,0.99383221411677),(0.988105937622242,0.989485911589765,
0.99383221411677,0.99383221411677,0.99383221411677)))
REPRESENTATION_ITEM('')
SURFACE()
);
#1167=(
BOUNDED_SURFACE()
B_SPLINE_SURFACE(1,2,((#113358,#113359,#113360,#113361,#113362),(#113363,
#113364,#113365,#113366,#113367)),.UNSPECIFIED.,.F.,.F.,.F.)
B_SPLINE_SURFACE_WITH_KNOTS((2,2),(3,2,3),(0.,0.289807040991559),(0.314770575782761,
0.314942866188516,0.332171906764072),.UNSPECIFIED.)
GEOMETRIC_REPRESENTATION_ITEM()
RATIONAL_B_SPLINE_SURFACE(((0.987877375613931,0.987877375613931,0.987877375613931,
0.986779141655835,0.9885983263477),(0.987877375613931,0.987877375613931,
0.987877375613931,0.986779141655835,0.9885983263477)))
REPRESENTATION_ITEM('')
SURFACE()
);
#1168=(
BOUNDED_SURFACE()
B_SPLINE_SURFACE(1,2,((#113378,#113379,#113380,#113381,#113382),(#113383,
#113384,#113385,#113386,#113387)),.UNSPECIFIED.,.F.,.F.,.F.)
B_SPLINE_SURFACE_WITH_KNOTS((2,2),(3,2,3),(0.,0.289681084359918),(0.40093921985274,
0.418312080773435,0.418485809382642),.UNSPECIFIED.)
GEOMETRIC_REPRESENTATION_ITEM()
RATIONAL_B_SPLINE_SURFACE(((0.988105937622242,0.989485911589765,0.99383221411677,
0.99383221411677,0.99383221411677),(0.988105937622242,0.989485911589765,
0.99383221411677,0.99383221411677,0.99383221411677)))
REPRESENTATION_ITEM('')
SURFACE()
);
#1169=(
BOUNDED_SURFACE()
B_SPLINE_SURFACE(1,2,((#113404,#113405,#113406,#113407,#113408),(#113409,
#113410,#113411,#113412,#113413)),.UNSPECIFIED.,.F.,.F.,.F.)
B_SPLINE_SURFACE_WITH_KNOTS((2,2),(3,2,3),(0.,0.28980704099156),(0.314770575782761,
0.314942866188516,0.332171906764074),.UNSPECIFIED.)
GEOMETRIC_REPRESENTATION_ITEM()
RATIONAL_B_SPLINE_SURFACE(((0.987877375613931,0.987877375613931,0.987877375613931,
0.986779141655835,0.988598326347701),(0.987877375613931,0.987877375613931,
0.987877375613931,0.986779141655835,0.988598326347701)))
REPRESENTATION_ITEM('')
SURFACE()
);
#1170=(
BOUNDED_SURFACE()
B_SPLINE_SURFACE(1,2,((#113439,#113440,#113441,#113442,#113443),(#113444,
#113445,#113446,#113447,#113448)),.UNSPECIFIED.,.F.,.F.,.F.)
B_SPLINE_SURFACE_WITH_KNOTS((2,2),(3,2,3),(0.,0.289681084359927),(0.400939219852743,
0.418312080773433,0.41848580938264),.UNSPECIFIED.)
GEOMETRIC_REPRESENTATION_ITEM()
RATIONAL_B_SPLINE_SURFACE(((0.988105937622242,0.989485911589766,0.99383221411677,
0.99383221411677,0.99383221411677),(0.988105937622242,0.989485911589766,
0.99383221411677,0.99383221411677,0.99383221411677)))
REPRESENTATION_ITEM('')
SURFACE()
);
#1171=(
BOUNDED_SURFACE()
B_SPLINE_SURFACE(1,2,((#113450,#113451,#113452,#113453,#113454),(#113455,
#113456,#113457,#113458,#113459)),.UNSPECIFIED.,.F.,.F.,.F.)
B_SPLINE_SURFACE_WITH_KNOTS((2,2),(3,2,3),(0.,0.289807040991823),(0.314770575782762,
0.314942866188517,0.332171906764075),.UNSPECIFIED.)
GEOMETRIC_REPRESENTATION_ITEM()
RATIONAL_B_SPLINE_SURFACE(((0.987877375613931,0.987877375613931,0.987877375613931,
0.986779141655835,0.988598326347701),(0.987877375613931,0.987877375613931,
0.987877375613931,0.986779141655835,0.988598326347701)))
REPRESENTATION_ITEM('')
SURFACE()
);
#1172=(
BOUNDED_SURFACE()
B_SPLINE_SURFACE(1,2,((#113485,#113486,#113487,#113488,#113489),(#113490,
#113491,#113492,#113493,#113494)),.UNSPECIFIED.,.F.,.F.,.F.)
B_SPLINE_SURFACE_WITH_KNOTS((2,2),(3,2,3),(0.,0.289681084359918),(0.400939219852739,
0.418312080773433,0.41848580938264),.UNSPECIFIED.)
GEOMETRIC_REPRESENTATION_ITEM()
RATIONAL_B_SPLINE_SURFACE(((0.988105937622241,0.989485911589765,0.99383221411677,
0.99383221411677,0.99383221411677),(0.988105937622241,0.989485911589765,
0.99383221411677,0.99383221411677,0.99383221411677)))
REPRESENTATION_ITEM('')
SURFACE()
);
#1173=(
BOUNDED_SURFACE()
B_SPLINE_SURFACE(1,2,((#113496,#113497,#113498,#113499,#113500),(#113501,
#113502,#113503,#113504,#113505)),.UNSPECIFIED.,.F.,.F.,.F.)
B_SPLINE_SURFACE_WITH_KNOTS((2,2),(3,2,3),(0.,0.289807040991884),(0.314770575782762,
0.314942866188517,0.332171906764075),.UNSPECIFIED.)
GEOMETRIC_REPRESENTATION_ITEM()
RATIONAL_B_SPLINE_SURFACE(((0.987877375613931,0.987877375613931,0.987877375613931,
0.986779141655835,0.988598326347701),(0.987877375613931,0.987877375613931,
0.987877375613931,0.986779141655835,0.988598326347701)))
REPRESENTATION_ITEM('')
SURFACE()
);
#1174=(
BOUNDED_SURFACE()
B_SPLINE_SURFACE(1,2,((#113531,#113532,#113533,#113534,#113535),(#113536,
#113537,#113538,#113539,#113540)),.UNSPECIFIED.,.F.,.F.,.F.)
B_SPLINE_SURFACE_WITH_KNOTS((2,2),(3,2,3),(0.,0.289681084359927),(0.400939219852741,
0.418312080773433,0.41848580938264),.UNSPECIFIED.)
GEOMETRIC_REPRESENTATION_ITEM()
RATIONAL_B_SPLINE_SURFACE(((0.988105937622242,0.989485911589765,0.99383221411677,
0.99383221411677,0.99383221411677),(0.988105937622242,0.989485911589765,
0.99383221411677,0.99383221411677,0.99383221411677)))
REPRESENTATION_ITEM('')
SURFACE()
);
#1175=(
BOUNDED_SURFACE()
B_SPLINE_SURFACE(1,2,((#113542,#113543,#113544,#113545,#113546),(#113547,
#113548,#113549,#113550,#113551)),.UNSPECIFIED.,.F.,.F.,.F.)
B_SPLINE_SURFACE_WITH_KNOTS((2,2),(3,2,3),(0.,0.289807040991838),(0.314770575782762,
0.314942866188517,0.332171906764074),.UNSPECIFIED.)
GEOMETRIC_REPRESENTATION_ITEM()
RATIONAL_B_SPLINE_SURFACE(((0.987877375613931,0.987877375613931,0.987877375613931,
0.986779141655835,0.988598326347701),(0.987877375613931,0.987877375613931,
0.987877375613931,0.986779141655835,0.988598326347701)))
REPRESENTATION_ITEM('')
SURFACE()
);
#1176=(
BOUNDED_SURFACE()
B_SPLINE_SURFACE(1,2,((#113577,#113578,#113579,#113580,#113581),(#113582,
#113583,#113584,#113585,#113586)),.UNSPECIFIED.,.F.,.F.,.F.)
B_SPLINE_SURFACE_WITH_KNOTS((2,2),(3,2,3),(0.,0.289681084359916),(0.400939219852742,
0.418312080773434,0.418485809382641),.UNSPECIFIED.)
GEOMETRIC_REPRESENTATION_ITEM()
RATIONAL_B_SPLINE_SURFACE(((0.988105937622242,0.989485911589766,0.99383221411677,
0.99383221411677,0.99383221411677),(0.988105937622242,0.989485911589766,
0.99383221411677,0.99383221411677,0.99383221411677)))
REPRESENTATION_ITEM('')
SURFACE()
);
#1177=(
BOUNDED_SURFACE()
B_SPLINE_SURFACE(1,2,((#113588,#113589,#113590,#113591,#113592),(#113593,
#113594,#113595,#113596,#113597)),.UNSPECIFIED.,.F.,.F.,.F.)
B_SPLINE_SURFACE_WITH_KNOTS((2,2),(3,2,3),(0.,0.289807040992021),(0.314770575782761,
0.314942866188516,0.332171906764074),.UNSPECIFIED.)
GEOMETRIC_REPRESENTATION_ITEM()
RATIONAL_B_SPLINE_SURFACE(((0.987877375613931,0.987877375613931,0.987877375613931,
0.986779141655835,0.988598326347701),(0.987877375613931,0.987877375613931,
0.987877375613931,0.986779141655835,0.988598326347701)))
REPRESENTATION_ITEM('')
SURFACE()
);
#1178=(
BOUNDED_SURFACE()
B_SPLINE_SURFACE(1,2,((#113623,#113624,#113625,#113626,#113627),(#113628,
#113629,#113630,#113631,#113632)),.UNSPECIFIED.,.F.,.F.,.F.)
B_SPLINE_SURFACE_WITH_KNOTS((2,2),(3,2,3),(0.,0.289681084359935),(0.400939219852743,
0.418312080773434,0.418485809382641),.UNSPECIFIED.)
GEOMETRIC_REPRESENTATION_ITEM()
RATIONAL_B_SPLINE_SURFACE(((0.988105937622242,0.989485911589766,0.99383221411677,
0.99383221411677,0.99383221411677),(0.988105937622242,0.989485911589766,
0.99383221411677,0.99383221411677,0.99383221411677)))
REPRESENTATION_ITEM('')
SURFACE()
);
#1179=(
BOUNDED_SURFACE()
B_SPLINE_SURFACE(1,2,((#113649,#113650,#113651,#113652,#113653),(#113654,
#113655,#113656,#113657,#113658)),.UNSPECIFIED.,.F.,.F.,.F.)
B_SPLINE_SURFACE_WITH_KNOTS((2,2),(3,2,3),(0.,0.289807040991979),(0.314770575782761,
0.314942866188516,0.332171906764074),.UNSPECIFIED.)
GEOMETRIC_REPRESENTATION_ITEM()
RATIONAL_B_SPLINE_SURFACE(((0.987877375613931,0.987877375613931,0.987877375613931,
0.986779141655835,0.988598326347701),(0.987877375613931,0.987877375613931,
0.987877375613931,0.986779141655835,0.988598326347701)))
REPRESENTATION_ITEM('')
SURFACE()
);
#1180=(
BOUNDED_SURFACE()
B_SPLINE_SURFACE(1,2,((#113660,#113661,#113662,#113663,#113664),(#113665,
#113666,#113667,#113668,#113669)),.UNSPECIFIED.,.F.,.F.,.F.)
B_SPLINE_SURFACE_WITH_KNOTS((2,2),(3,2,3),(0.710192959007329,1.),(0.262924618389842,
0.263098999273797,0.280537087669266),.UNSPECIFIED.)
GEOMETRIC_REPRESENTATION_ITEM()
RATIONAL_B_SPLINE_SURFACE(((0.989150325841653,0.989150325841653,0.989150325841653,
0.991395311444462,0.996628941948308),(0.989150325841653,0.989150325841653,
0.989150325841653,0.991395311444462,0.996628941948308)))
REPRESENTATION_ITEM('')
SURFACE()
);
#1181=(
BOUNDED_SURFACE()
B_SPLINE_SURFACE(1,2,((#113680,#113681,#113682),(#113683,#113684,#113685)),
 .UNSPECIFIED.,.F.,.F.,.F.)
B_SPLINE_SURFACE_WITH_KNOTS((2,2),(3,3),(0.710318915640079,1.),(0.452822299828563,
0.470019760166384),.UNSPECIFIED.)
GEOMETRIC_REPRESENTATION_ITEM()
RATIONAL_B_SPLINE_SURFACE(((0.988755486262821,0.986817927519784,0.987787102172816),
(0.988755486262821,0.986817927519784,0.987787102172816)))
REPRESENTATION_ITEM('')
SURFACE()
);
#1182=(
BOUNDED_SURFACE()
B_SPLINE_SURFACE(1,2,((#113696,#113697,#113698,#113699,#113700),(#113701,
#113702,#113703,#113704,#113705)),.UNSPECIFIED.,.F.,.F.,.F.)
B_SPLINE_SURFACE_WITH_KNOTS((2,2),(3,2,3),(0.710192959008441,1.),(0.262924618389842,
0.263098999273797,0.280537087669267),.UNSPECIFIED.)
GEOMETRIC_REPRESENTATION_ITEM()
RATIONAL_B_SPLINE_SURFACE(((0.989150325841653,0.989150325841653,0.989150325841653,
0.991395311444462,0.996628941948308),(0.989150325841653,0.989150325841653,
0.989150325841653,0.991395311444462,0.996628941948308)))
REPRESENTATION_ITEM('')
SURFACE()
);
#1183=(
BOUNDED_SURFACE()
B_SPLINE_SURFACE(1,2,((#113713,#113714,#113715),(#113716,#113717,#113718)),
 .UNSPECIFIED.,.F.,.F.,.F.)
B_SPLINE_SURFACE_WITH_KNOTS((2,2),(3,3),(0.710318915640082,1.),(0.452822299828565,
0.470019760166366),.UNSPECIFIED.)
GEOMETRIC_REPRESENTATION_ITEM()
RATIONAL_B_SPLINE_SURFACE(((0.988755486262821,0.986817927519786,0.987787102172814),
(0.988755486262821,0.986817927519786,0.987787102172814)))
REPRESENTATION_ITEM('')
SURFACE()
);
#1184=(
BOUNDED_SURFACE()
B_SPLINE_SURFACE(1,2,((#113729,#113730,#113731,#113732,#113733),(#113734,
#113735,#113736,#113737,#113738)),.UNSPECIFIED.,.F.,.F.,.F.)
B_SPLINE_SURFACE_WITH_KNOTS((2,2),(3,2,3),(0.710192959008439,1.),(0.262924618389842,
0.263098999273797,0.280537087669267),.UNSPECIFIED.)
GEOMETRIC_REPRESENTATION_ITEM()
RATIONAL_B_SPLINE_SURFACE(((0.989150325841653,0.989150325841653,0.989150325841653,
0.991395311444462,0.996628941948308),(0.989150325841653,0.989150325841653,
0.989150325841653,0.991395311444462,0.996628941948308)))
REPRESENTATION_ITEM('')
SURFACE()
);
#1185=(
BOUNDED_SURFACE()
B_SPLINE_SURFACE(1,2,((#113746,#113747,#113748),(#113749,#113750,#113751)),
 .UNSPECIFIED.,.F.,.F.,.F.)
B_SPLINE_SURFACE_WITH_KNOTS((2,2),(3,3),(0.710318915639499,1.),(0.452822299828566,
0.470019760166366),.UNSPECIFIED.)
GEOMETRIC_REPRESENTATION_ITEM()
RATIONAL_B_SPLINE_SURFACE(((0.98875548626282,0.986817927519786,0.987787102172814),
(0.98875548626282,0.986817927519786,0.987787102172814)))
REPRESENTATION_ITEM('')
SURFACE()
);
#1186=(
BOUNDED_SURFACE()
B_SPLINE_SURFACE(1,2,((#113762,#113763,#113764,#113765,#113766),(#113767,
#113768,#113769,#113770,#113771)),.UNSPECIFIED.,.F.,.F.,.F.)
B_SPLINE_SURFACE_WITH_KNOTS((2,2),(3,2,3),(0.709593130080989,1.),(0.26249917015916,
0.263098999273797,0.280537087669267),.UNSPECIFIED.)
GEOMETRIC_REPRESENTATION_ITEM()
RATIONAL_B_SPLINE_SURFACE(((0.989150325841653,0.989150325841653,0.989150325841653,
0.991395311444462,0.996628941948308),(0.989150325841653,0.989150325841653,
0.989150325841653,0.991395311444462,0.996628941948308)))
REPRESENTATION_ITEM('')
SURFACE()
);
#1187=(
BOUNDED_SURFACE()
B_SPLINE_SURFACE(1,2,((#113779,#113780,#113781),(#113782,#113783,#113784)),
 .UNSPECIFIED.,.F.,.F.,.F.)
B_SPLINE_SURFACE_WITH_KNOTS((2,2),(3,3),(0.710318915640079,1.),(0.452822299828565,
0.470019760166366),.UNSPECIFIED.)
GEOMETRIC_REPRESENTATION_ITEM()
RATIONAL_B_SPLINE_SURFACE(((0.98875548626282,0.986817927519786,0.987787102172814),
(0.988755486262821,0.986817927519786,0.987787102172814)))
REPRESENTATION_ITEM('')
SURFACE()
);
#1188=(
BOUNDED_SURFACE()
B_SPLINE_SURFACE(1,2,((#113795,#113796,#113797,#113798,#113799),(#113800,
#113801,#113802,#113803,#113804)),.UNSPECIFIED.,.F.,.F.,.F.)
B_SPLINE_SURFACE_WITH_KNOTS((2,2),(3,2,3),(0.709593130109806,1.),(0.262499170175398,
0.263098999273797,0.280537087669267),.UNSPECIFIED.)
GEOMETRIC_REPRESENTATION_ITEM()
RATIONAL_B_SPLINE_SURFACE(((0.989150325841653,0.989150325841653,0.989150325841653,
0.991395311444462,0.996628941948309),(0.989150325841653,0.989150325841653,
0.989150325841653,0.991395311444462,0.996628941948308)))
REPRESENTATION_ITEM('')
SURFACE()
);
#1189=(
BOUNDED_SURFACE()
B_SPLINE_SURFACE(1,2,((#113812,#113813,#113814),(#113815,#113816,#113817)),
 .UNSPECIFIED.,.F.,.F.,.F.)
B_SPLINE_SURFACE_WITH_KNOTS((2,2),(3,3),(0.710318915639495,1.),(0.452822299828565,
0.470019760166366),.UNSPECIFIED.)
GEOMETRIC_REPRESENTATION_ITEM()
RATIONAL_B_SPLINE_SURFACE(((0.98875548626282,0.986817927519786,0.987787102172814),
(0.988755486262821,0.986817927519786,0.987787102172814)))
REPRESENTATION_ITEM('')
SURFACE()
);
#1190=(
BOUNDED_SURFACE()
B_SPLINE_SURFACE(1,2,((#113828,#113829,#113830,#113831,#113832),(#113833,
#113834,#113835,#113836,#113837)),.UNSPECIFIED.,.F.,.F.,.F.)
B_SPLINE_SURFACE_WITH_KNOTS((2,2),(3,2,3),(0.709593130090909,1.),(0.262499170157079,
0.263098999273797,0.280537087669267),.UNSPECIFIED.)
GEOMETRIC_REPRESENTATION_ITEM()
RATIONAL_B_SPLINE_SURFACE(((0.989150325841653,0.989150325841653,0.989150325841653,
0.991395311444462,0.996628941948308),(0.989150325841653,0.989150325841653,
0.989150325841653,0.991395311444462,0.996628941948308)))
REPRESENTATION_ITEM('')
SURFACE()
);
#1191=(
BOUNDED_SURFACE()
B_SPLINE_SURFACE(1,2,((#113845,#113846,#113847),(#113848,#113849,#113850)),
 .UNSPECIFIED.,.F.,.F.,.F.)
B_SPLINE_SURFACE_WITH_KNOTS((2,2),(3,3),(0.710318915639997,1.),(0.452822299828567,
0.470019760166366),.UNSPECIFIED.)
GEOMETRIC_REPRESENTATION_ITEM()
RATIONAL_B_SPLINE_SURFACE(((0.98875548626282,0.986817927519786,0.987787102172814),
(0.98875548626282,0.986817927519786,0.987787102172814)))
REPRESENTATION_ITEM('')
SURFACE()
);
#1192=(
BOUNDED_SURFACE()
B_SPLINE_SURFACE(1,2,((#113861,#113862,#113863,#113864,#113865),(#113866,
#113867,#113868,#113869,#113870)),.UNSPECIFIED.,.F.,.F.,.F.)
B_SPLINE_SURFACE_WITH_KNOTS((2,2),(3,2,3),(0.709593130119578,1.),(0.262499170185248,
0.263098999273796,0.280537087669266),.UNSPECIFIED.)
GEOMETRIC_REPRESENTATION_ITEM()
RATIONAL_B_SPLINE_SURFACE(((0.989150325841653,0.989150325841653,0.989150325841653,
0.991395311444461,0.996628941948308),(0.989150325841653,0.989150325841653,
0.989150325841653,0.991395311444461,0.996628941948308)))
REPRESENTATION_ITEM('')
SURFACE()
);
#1193=(
BOUNDED_SURFACE()
B_SPLINE_SURFACE(1,2,((#113878,#113879,#113880),(#113881,#113882,#113883)),
 .UNSPECIFIED.,.F.,.F.,.F.)
B_SPLINE_SURFACE_WITH_KNOTS((2,2),(3,3),(0.710318915640003,1.),(0.452822299828567,
0.470019760166367),.UNSPECIFIED.)
GEOMETRIC_REPRESENTATION_ITEM()
RATIONAL_B_SPLINE_SURFACE(((0.98875548626282,0.986817927519786,0.987787102172814),
(0.98875548626282,0.986817927519786,0.987787102172814)))
REPRESENTATION_ITEM('')
SURFACE()
);
#1194=(
BOUNDED_SURFACE()
B_SPLINE_SURFACE(1,2,((#113894,#113895,#113896,#113897,#113898),(#113899,
#113900,#113901,#113902,#113903)),.UNSPECIFIED.,.F.,.F.,.F.)
B_SPLINE_SURFACE_WITH_KNOTS((2,2),(3,2,3),(0.710192959008368,1.),(0.262924618389841,
0.263098999273796,0.280537087669266),.UNSPECIFIED.)
GEOMETRIC_REPRESENTATION_ITEM()
RATIONAL_B_SPLINE_SURFACE(((0.989150325841653,0.989150325841653,0.989150325841653,
0.991395311444461,0.996628941948308),(0.989150325841653,0.989150325841653,
0.989150325841653,0.991395311444461,0.996628941948308)))
REPRESENTATION_ITEM('')
SURFACE()
);
#1195=(
BOUNDED_SURFACE()
B_SPLINE_SURFACE(1,2,((#113911,#113912,#113913),(#113914,#113915,#113916)),
 .UNSPECIFIED.,.F.,.F.,.F.)
B_SPLINE_SURFACE_WITH_KNOTS((2,2),(3,3),(0.710318915639408,1.),(0.452822299828567,
0.470019760166367),.UNSPECIFIED.)
GEOMETRIC_REPRESENTATION_ITEM()
RATIONAL_B_SPLINE_SURFACE(((0.98875548626282,0.986817927519786,0.987787102172814),
(0.98875548626282,0.986817927519786,0.987787102172814)))
REPRESENTATION_ITEM('')
SURFACE()
);
#1196=(
BOUNDED_SURFACE()
B_SPLINE_SURFACE(1,2,((#113927,#113928,#113929,#113930,#113931),(#113932,
#113933,#113934,#113935,#113936)),.UNSPECIFIED.,.F.,.F.,.F.)
B_SPLINE_SURFACE_WITH_KNOTS((2,2),(3,2,3),(0.710192959007765,1.),(0.262924618389841,
0.263098999273796,0.280537087669266),.UNSPECIFIED.)
GEOMETRIC_REPRESENTATION_ITEM()
RATIONAL_B_SPLINE_SURFACE(((0.989150325841653,0.989150325841653,0.989150325841653,
0.991395311444461,0.996628941948308),(0.989150325841653,0.989150325841653,
0.989150325841653,0.991395311444461,0.996628941948308)))
REPRESENTATION_ITEM('')
SURFACE()
);
#1197=(
BOUNDED_SURFACE()
B_SPLINE_SURFACE(1,2,((#113944,#113945,#113946),(#113947,#113948,#113949)),
 .UNSPECIFIED.,.F.,.F.,.F.)
B_SPLINE_SURFACE_WITH_KNOTS((2,2),(3,3),(0.710318915639996,1.),(0.452822299828567,
0.470019760166367),.UNSPECIFIED.)
GEOMETRIC_REPRESENTATION_ITEM()
RATIONAL_B_SPLINE_SURFACE(((0.98875548626282,0.986817927519786,0.987787102172814),
(0.98875548626282,0.986817927519786,0.987787102172814)))
REPRESENTATION_ITEM('')
SURFACE()
);
#1198=(
BOUNDED_SURFACE()
B_SPLINE_SURFACE(1,2,((#113960,#113961,#113962,#113963,#113964),(#113965,
#113966,#113967,#113968,#113969)),.UNSPECIFIED.,.F.,.F.,.F.)
B_SPLINE_SURFACE_WITH_KNOTS((2,2),(3,2,3),(0.710192959008356,1.),(0.262924618389841,
0.263098999273796,0.280537087669266),.UNSPECIFIED.)
GEOMETRIC_REPRESENTATION_ITEM()
RATIONAL_B_SPLINE_SURFACE(((0.989150325841653,0.989150325841653,0.989150325841653,
0.991395311444461,0.996628941948308),(0.989150325841653,0.989150325841653,
0.989150325841653,0.991395311444461,0.996628941948308)))
REPRESENTATION_ITEM('')
SURFACE()
);
#1199=(
BOUNDED_SURFACE()
B_SPLINE_SURFACE(1,2,((#113977,#113978,#113979),(#113980,#113981,#113982)),
 .UNSPECIFIED.,.F.,.F.,.F.)
B_SPLINE_SURFACE_WITH_KNOTS((2,2),(3,3),(0.710318915639494,1.),(0.452822299828567,
0.470019760166367),.UNSPECIFIED.)
GEOMETRIC_REPRESENTATION_ITEM()
RATIONAL_B_SPLINE_SURFACE(((0.98875548626282,0.986817927519786,0.987787102172814),
(0.98875548626282,0.986817927519786,0.987787102172814)))
REPRESENTATION_ITEM('')
SURFACE()
);
#1200=(
BOUNDED_SURFACE()
B_SPLINE_SURFACE(1,2,((#113993,#113994,#113995,#113996,#113997),(#113998,
#113999,#114000,#114001,#114002)),.UNSPECIFIED.,.F.,.F.,.F.)
B_SPLINE_SURFACE_WITH_KNOTS((2,2),(3,2,3),(0.710192959007858,1.),(0.262924618389841,
0.263098999273796,0.280537087669266),.UNSPECIFIED.)
GEOMETRIC_REPRESENTATION_ITEM()
RATIONAL_B_SPLINE_SURFACE(((0.989150325841653,0.989150325841653,0.989150325841653,
0.991395311444461,0.996628941948308),(0.989150325841653,0.989150325841653,
0.989150325841653,0.991395311444461,0.996628941948308)))
REPRESENTATION_ITEM('')
SURFACE()
);
#1201=(
BOUNDED_SURFACE()
B_SPLINE_SURFACE(1,2,((#114010,#114011,#114012),(#114013,#114014,#114015)),
 .UNSPECIFIED.,.F.,.F.,.F.)
B_SPLINE_SURFACE_WITH_KNOTS((2,2),(3,3),(0.710318915639993,1.),(0.452822299828567,
0.470019760166367),.UNSPECIFIED.)
GEOMETRIC_REPRESENTATION_ITEM()
RATIONAL_B_SPLINE_SURFACE(((0.98875548626282,0.986817927519786,0.987787102172814),
(0.98875548626282,0.986817927519786,0.987787102172814)))
REPRESENTATION_ITEM('')
SURFACE()
);
#1202=(
BOUNDED_SURFACE()
B_SPLINE_SURFACE(1,2,((#114026,#114027,#114028,#114029,#114030),(#114031,
#114032,#114033,#114034,#114035)),.UNSPECIFIED.,.F.,.F.,.F.)
B_SPLINE_SURFACE_WITH_KNOTS((2,2),(3,2,3),(0.709593130089926,1.),(0.262499170167511,
0.263098999273796,0.280537087669266),.UNSPECIFIED.)
GEOMETRIC_REPRESENTATION_ITEM()
RATIONAL_B_SPLINE_SURFACE(((0.989150325841653,0.989150325841653,0.989150325841653,
0.991395311444461,0.996628941948308),(0.989150325841653,0.989150325841653,
0.989150325841653,0.991395311444461,0.996628941948308)))
REPRESENTATION_ITEM('')
SURFACE()
);
#1203=(
BOUNDED_SURFACE()
B_SPLINE_SURFACE(1,2,((#114043,#114044,#114045),(#114046,#114047,#114048)),
 .UNSPECIFIED.,.F.,.F.,.F.)
B_SPLINE_SURFACE_WITH_KNOTS((2,2),(3,3),(0.710318915639495,1.),(0.452822299828567,
0.470019760166367),.UNSPECIFIED.)
GEOMETRIC_REPRESENTATION_ITEM()
RATIONAL_B_SPLINE_SURFACE(((0.98875548626282,0.986817927519786,0.987787102172814),
(0.98875548626282,0.986817927519786,0.987787102172814)))
REPRESENTATION_ITEM('')
SURFACE()
);
#1204=(
BOUNDED_SURFACE()
B_SPLINE_SURFACE(1,2,((#114059,#114060,#114061,#114062,#114063),(#114064,
#114065,#114066,#114067,#114068)),.UNSPECIFIED.,.F.,.F.,.F.)
B_SPLINE_SURFACE_WITH_KNOTS((2,2),(3,2,3),(0.709593130096317,1.),(0.262499170174355,
0.263098999273796,0.280537087669266),.UNSPECIFIED.)
GEOMETRIC_REPRESENTATION_ITEM()
RATIONAL_B_SPLINE_SURFACE(((0.989150325841653,0.989150325841653,0.989150325841653,
0.991395311444461,0.996628941948308),(0.989150325841653,0.989150325841653,
0.989150325841653,0.991395311444461,0.996628941948308)))
REPRESENTATION_ITEM('')
SURFACE()
);
#1205=(
BOUNDED_SURFACE()
B_SPLINE_SURFACE(1,2,((#114076,#114077,#114078),(#114079,#114080,#114081)),
 .UNSPECIFIED.,.F.,.F.,.F.)
B_SPLINE_SURFACE_WITH_KNOTS((2,2),(3,3),(0.710318915639721,1.),(0.452822299828567,
0.470019760166367),.UNSPECIFIED.)
GEOMETRIC_REPRESENTATION_ITEM()
RATIONAL_B_SPLINE_SURFACE(((0.98875548626282,0.986817927519786,0.987787102172814),
(0.98875548626282,0.986817927519786,0.987787102172814)))
REPRESENTATION_ITEM('')
SURFACE()
);
#1206=(
BOUNDED_SURFACE()
B_SPLINE_SURFACE(1,2,((#114092,#114093,#114094,#114095,#114096),(#114097,
#114098,#114099,#114100,#114101)),.UNSPECIFIED.,.F.,.F.,.F.)
B_SPLINE_SURFACE_WITH_KNOTS((2,2),(3,2,3),(0.709593130099464,1.),(0.262499170165416,
0.263098999273796,0.280537087669266),.UNSPECIFIED.)
GEOMETRIC_REPRESENTATION_ITEM()
RATIONAL_B_SPLINE_SURFACE(((0.989150325841653,0.989150325841653,0.989150325841653,
0.991395311444461,0.996628941948308),(0.989150325841653,0.989150325841653,
0.989150325841653,0.991395311444461,0.996628941948308)))
REPRESENTATION_ITEM('')
SURFACE()
);
#1207=(
BOUNDED_SURFACE()
B_SPLINE_SURFACE(1,2,((#114109,#114110,#114111),(#114112,#114113,#114114)),
 .UNSPECIFIED.,.F.,.F.,.F.)
B_SPLINE_SURFACE_WITH_KNOTS((2,2),(3,3),(0.710318915638678,1.),(0.452822299828567,
0.470019760166367),.UNSPECIFIED.)
GEOMETRIC_REPRESENTATION_ITEM()
RATIONAL_B_SPLINE_SURFACE(((0.98875548626282,0.986817927519786,0.987787102172814),
(0.98875548626282,0.986817927519786,0.987787102172814)))
REPRESENTATION_ITEM('')
SURFACE()
);
#1208=(
BOUNDED_SURFACE()
B_SPLINE_SURFACE(1,2,((#114122,#114123,#114124,#114125,#114126),(#114127,
#114128,#114129,#114130,#114131)),.UNSPECIFIED.,.F.,.F.,.F.)
B_SPLINE_SURFACE_WITH_KNOTS((2,2),(3,2,3),(0.71019295900703,1.),(0.262924618389841,
0.263098999273796,0.280537087669266),.UNSPECIFIED.)
GEOMETRIC_REPRESENTATION_ITEM()
RATIONAL_B_SPLINE_SURFACE(((0.989150325841653,0.989150325841653,0.989150325841653,
0.991395311444461,0.996628941948308),(0.989150325841653,0.989150325841653,
0.989150325841653,0.991395311444461,0.996628941948308)))
REPRESENTATION_ITEM('')
SURFACE()
);
#1209=(
BOUNDED_SURFACE()
B_SPLINE_SURFACE(1,2,((#114133,#114134,#114135),(#114136,#114137,#114138)),
 .UNSPECIFIED.,.F.,.F.,.F.)
B_SPLINE_SURFACE_WITH_KNOTS((2,2),(3,3),(0.710318915639959,1.),(0.452822299828567,
0.470019760166367),.UNSPECIFIED.)
GEOMETRIC_REPRESENTATION_ITEM()
RATIONAL_B_SPLINE_SURFACE(((0.98875548626282,0.986817927519786,0.987787102172814),
(0.98875548626282,0.986817927519786,0.987787102172814)))
REPRESENTATION_ITEM('')
SURFACE()
);
#1210=(
BOUNDED_SURFACE()
B_SPLINE_SURFACE(1,2,((#114149,#114150,#114151,#114152,#114153),(#114154,
#114155,#114156,#114157,#114158)),.UNSPECIFIED.,.F.,.F.,.F.)
B_SPLINE_SURFACE_WITH_KNOTS((2,2),(3,2,3),(0.710192959008315,1.),(0.262924618389841,
0.263098999273796,0.280537087669266),.UNSPECIFIED.)
GEOMETRIC_REPRESENTATION_ITEM()
RATIONAL_B_SPLINE_SURFACE(((0.989150325841653,0.989150325841653,0.989150325841653,
0.991395311444461,0.996628941948308),(0.989150325841653,0.989150325841653,
0.989150325841653,0.991395311444461,0.996628941948308)))
REPRESENTATION_ITEM('')
SURFACE()
);
#1211=(
BOUNDED_SURFACE()
B_SPLINE_SURFACE(1,2,((#114166,#114167,#114168),(#114169,#114170,#114171)),
 .UNSPECIFIED.,.F.,.F.,.F.)
B_SPLINE_SURFACE_WITH_KNOTS((2,2),(3,3),(0.710318915640075,1.),(0.452822299828567,
0.470019760166367),.UNSPECIFIED.)
GEOMETRIC_REPRESENTATION_ITEM()
RATIONAL_B_SPLINE_SURFACE(((0.98875548626282,0.986817927519786,0.987787102172814),
(0.98875548626282,0.986817927519786,0.987787102172814)))
REPRESENTATION_ITEM('')
SURFACE()
);
#1212=(
BOUNDED_SURFACE()
B_SPLINE_SURFACE(1,2,((#114182,#114183,#114184,#114185,#114186),(#114187,
#114188,#114189,#114190,#114191)),.UNSPECIFIED.,.F.,.F.,.F.)
B_SPLINE_SURFACE_WITH_KNOTS((2,2),(3,2,3),(0.710192959008434,1.),(0.262924618389841,
0.263098999273796,0.280537087669266),.UNSPECIFIED.)
GEOMETRIC_REPRESENTATION_ITEM()
RATIONAL_B_SPLINE_SURFACE(((0.989150325841653,0.989150325841653,0.989150325841653,
0.991395311444461,0.996628941948308),(0.989150325841653,0.989150325841653,
0.989150325841653,0.991395311444461,0.996628941948308)))
REPRESENTATION_ITEM('')
SURFACE()
);
#1213=(
BOUNDED_SURFACE()
B_SPLINE_SURFACE(1,2,((#114199,#114200,#114201),(#114202,#114203,#114204)),
 .UNSPECIFIED.,.F.,.F.,.F.)
B_SPLINE_SURFACE_WITH_KNOTS((2,2),(3,3),(0.710318915639447,1.),(0.452822299828566,
0.470019760166367),.UNSPECIFIED.)
GEOMETRIC_REPRESENTATION_ITEM()
RATIONAL_B_SPLINE_SURFACE(((0.98875548626282,0.986817927519786,0.987787102172814),
(0.98875548626282,0.986817927519786,0.987787102172814)))
REPRESENTATION_ITEM('')
SURFACE()
);
#1214=(
BOUNDED_SURFACE()
B_SPLINE_SURFACE(1,2,((#114215,#114216,#114217,#114218,#114219),(#114220,
#114221,#114222,#114223,#114224)),.UNSPECIFIED.,.F.,.F.,.F.)
B_SPLINE_SURFACE_WITH_KNOTS((2,2),(3,2,3),(0.710192959007799,1.),(0.262924618389841,
0.263098999273796,0.280537087669266),.UNSPECIFIED.)
GEOMETRIC_REPRESENTATION_ITEM()
RATIONAL_B_SPLINE_SURFACE(((0.989150325841653,0.989150325841653,0.989150325841653,
0.991395311444461,0.996628941948308),(0.989150325841653,0.989150325841653,
0.989150325841653,0.991395311444461,0.996628941948308)))
REPRESENTATION_ITEM('')
SURFACE()
);
#1215=(
BOUNDED_SURFACE()
B_SPLINE_SURFACE(1,2,((#114232,#114233,#114234),(#114235,#114236,#114237)),
 .UNSPECIFIED.,.F.,.F.,.F.)
B_SPLINE_SURFACE_WITH_KNOTS((2,2),(3,3),(0.71031891564008,1.),(0.452822299828566,
0.470019760166367),.UNSPECIFIED.)
GEOMETRIC_REPRESENTATION_ITEM()
RATIONAL_B_SPLINE_SURFACE(((0.98875548626282,0.986817927519786,0.987787102172814),
(0.98875548626282,0.986817927519786,0.987787102172814)))
REPRESENTATION_ITEM('')
SURFACE()
);
#1216=(
BOUNDED_SURFACE()
B_SPLINE_SURFACE(1,2,((#114248,#114249,#114250,#114251,#114252),(#114253,
#114254,#114255,#114256,#114257)),.UNSPECIFIED.,.F.,.F.,.F.)
B_SPLINE_SURFACE_WITH_KNOTS((2,2),(3,2,3),(0.709593130092405,1.),(0.262499170169975,
0.263098999273796,0.280537087669266),.UNSPECIFIED.)
GEOMETRIC_REPRESENTATION_ITEM()
RATIONAL_B_SPLINE_SURFACE(((0.989150325841653,0.989150325841653,0.989150325841653,
0.991395311444461,0.996628941948308),(0.989150325841653,0.989150325841653,
0.989150325841653,0.991395311444461,0.996628941948308)))
REPRESENTATION_ITEM('')
SURFACE()
);
#1217=(
BOUNDED_SURFACE()
B_SPLINE_SURFACE(1,2,((#114265,#114266,#114267),(#114268,#114269,#114270)),
 .UNSPECIFIED.,.F.,.F.,.F.)
B_SPLINE_SURFACE_WITH_KNOTS((2,2),(3,3),(0.710318915638944,1.),(0.452822299828567,
0.470019760166367),.UNSPECIFIED.)
GEOMETRIC_REPRESENTATION_ITEM()
RATIONAL_B_SPLINE_SURFACE(((0.98875548626282,0.986817927519786,0.987787102172814),
(0.98875548626282,0.986817927519786,0.987787102172814)))
REPRESENTATION_ITEM('')
SURFACE()
);
#1218=(
BOUNDED_SURFACE()
B_SPLINE_SURFACE(1,2,((#114281,#114282,#114283,#114284,#114285),(#114286,
#114287,#114288,#114289,#114290)),.UNSPECIFIED.,.F.,.F.,.F.)
B_SPLINE_SURFACE_WITH_KNOTS((2,2),(3,2,3),(0.70959313010765,1.),(0.262499170174373,
0.263098999273796,0.280537087669266),.UNSPECIFIED.)
GEOMETRIC_REPRESENTATION_ITEM()
RATIONAL_B_SPLINE_SURFACE(((0.989150325841653,0.989150325841653,0.989150325841653,
0.991395311444461,0.996628941948308),(0.989150325841653,0.989150325841653,
0.989150325841653,0.991395311444461,0.996628941948308)))
REPRESENTATION_ITEM('')
SURFACE()
);
#1219=(
BOUNDED_SURFACE()
B_SPLINE_SURFACE(1,2,((#114298,#114299,#114300),(#114301,#114302,#114303)),
 .UNSPECIFIED.,.F.,.F.,.F.)
B_SPLINE_SURFACE_WITH_KNOTS((2,2),(3,3),(0.710318915639103,1.),(0.452822299828567,
0.470019760166367),.UNSPECIFIED.)
GEOMETRIC_REPRESENTATION_ITEM()
RATIONAL_B_SPLINE_SURFACE(((0.98875548626282,0.986817927519786,0.987787102172814),
(0.98875548626282,0.986817927519786,0.987787102172814)))
REPRESENTATION_ITEM('')
SURFACE()
);
#1220=(
BOUNDED_SURFACE()
B_SPLINE_SURFACE(1,2,((#114314,#114315,#114316,#114317,#114318),(#114319,
#114320,#114321,#114322,#114323)),.UNSPECIFIED.,.F.,.F.,.F.)
B_SPLINE_SURFACE_WITH_KNOTS((2,2),(3,2,3),(0.709593130086774,1.),(0.262499170165146,
0.263098999273796,0.280537087669266),.UNSPECIFIED.)
GEOMETRIC_REPRESENTATION_ITEM()
RATIONAL_B_SPLINE_SURFACE(((0.989150325841653,0.989150325841653,0.989150325841653,
0.991395311444461,0.996628941948308),(0.989150325841653,0.989150325841653,
0.989150325841653,0.991395311444461,0.996628941948308)))
REPRESENTATION_ITEM('')
SURFACE()
);
#1221=(
BOUNDED_SURFACE()
B_SPLINE_SURFACE(1,2,((#114331,#114332,#114333),(#114334,#114335,#114336)),
 .UNSPECIFIED.,.F.,.F.,.F.)
B_SPLINE_SURFACE_WITH_KNOTS((2,2),(3,3),(0.710318915638382,1.),(0.452822299828567,
0.470019760166367),.UNSPECIFIED.)
GEOMETRIC_REPRESENTATION_ITEM()
RATIONAL_B_SPLINE_SURFACE(((0.98875548626282,0.986817927519786,0.987787102172814),
(0.98875548626282,0.986817927519786,0.987787102172814)))
REPRESENTATION_ITEM('')
SURFACE()
);
#1222=(
BOUNDED_SURFACE()
B_SPLINE_SURFACE(1,2,((#114347,#114348,#114349,#114350,#114351),(#114352,
#114353,#114354,#114355,#114356)),.UNSPECIFIED.,.F.,.F.,.F.)
B_SPLINE_SURFACE_WITH_KNOTS((2,2),(3,2,3),(0.709593130097478,1.),(0.262499170176673,
0.263098999273796,0.280537087669266),.UNSPECIFIED.)
GEOMETRIC_REPRESENTATION_ITEM()
RATIONAL_B_SPLINE_SURFACE(((0.989150325841653,0.989150325841653,0.989150325841653,
0.991395311444461,0.996628941948308),(0.989150325841653,0.989150325841653,
0.989150325841653,0.991395311444461,0.996628941948308)))
REPRESENTATION_ITEM('')
SURFACE()
);
#1223=(
BOUNDED_SURFACE()
B_SPLINE_SURFACE(1,2,((#114364,#114365,#114366),(#114367,#114368,#114369)),
 .UNSPECIFIED.,.F.,.F.,.F.)
B_SPLINE_SURFACE_WITH_KNOTS((2,2),(3,3),(0.71031891563988,1.),(0.452822299828566,
0.470019760166367),.UNSPECIFIED.)
GEOMETRIC_REPRESENTATION_ITEM()
RATIONAL_B_SPLINE_SURFACE(((0.98875548626282,0.986817927519786,0.987787102172814),
(0.98875548626282,0.986817927519786,0.987787102172814)))
REPRESENTATION_ITEM('')
SURFACE()
);
#1224=(
BOUNDED_SURFACE()
B_SPLINE_SURFACE(1,2,((#114380,#114381,#114382,#114383,#114384),(#114385,
#114386,#114387,#114388,#114389)),.UNSPECIFIED.,.F.,.F.,.F.)
B_SPLINE_SURFACE_WITH_KNOTS((2,2),(3,2,3),(0.710192959008239,1.),(0.262924618389841,
0.263098999273796,0.280537087669266),.UNSPECIFIED.)
GEOMETRIC_REPRESENTATION_ITEM()
RATIONAL_B_SPLINE_SURFACE(((0.989150325841653,0.989150325841653,0.989150325841653,
0.991395311444461,0.996628941948308),(0.989150325841653,0.989150325841653,
0.989150325841653,0.991395311444461,0.996628941948308)))
REPRESENTATION_ITEM('')
SURFACE()
);
#1225=(
BOUNDED_SURFACE()
B_SPLINE_SURFACE(1,2,((#114397,#114398,#114399),(#114400,#114401,#114402)),
 .UNSPECIFIED.,.F.,.F.,.F.)
B_SPLINE_SURFACE_WITH_KNOTS((2,2),(3,3),(0.710318915638594,1.),(0.452822299828566,
0.470019760166367),.UNSPECIFIED.)
GEOMETRIC_REPRESENTATION_ITEM()
RATIONAL_B_SPLINE_SURFACE(((0.98875548626282,0.986817927519787,0.987787102172814),
(0.98875548626282,0.986817927519786,0.987787102172814)))
REPRESENTATION_ITEM('')
SURFACE()
);
#1226=(
BOUNDED_SURFACE()
B_SPLINE_SURFACE(1,2,((#114413,#114414,#114415,#114416,#114417),(#114418,
#114419,#114420,#114421,#114422)),.UNSPECIFIED.,.F.,.F.,.F.)
B_SPLINE_SURFACE_WITH_KNOTS((2,2),(3,2,3),(0.710192959006949,1.),(0.262924618389841,
0.263098999273796,0.280537087669266),.UNSPECIFIED.)
GEOMETRIC_REPRESENTATION_ITEM()
RATIONAL_B_SPLINE_SURFACE(((0.989150325841653,0.989150325841653,0.989150325841653,
0.991395311444461,0.996628941948308),(0.989150325841653,0.989150325841653,
0.989150325841653,0.991395311444461,0.996628941948308)))
REPRESENTATION_ITEM('')
SURFACE()
);
#1227=(
BOUNDED_SURFACE()
B_SPLINE_SURFACE(1,2,((#114430,#114431,#114432),(#114433,#114434,#114435)),
 .UNSPECIFIED.,.F.,.F.,.F.)
B_SPLINE_SURFACE_WITH_KNOTS((2,2),(3,3),(0.710318915638842,1.),(0.452822299828566,
0.47001976016637),.UNSPECIFIED.)
GEOMETRIC_REPRESENTATION_ITEM()
RATIONAL_B_SPLINE_SURFACE(((0.98875548626282,0.986817927519786,0.987787102172814),
(0.98875548626282,0.986817927519786,0.987787102172814)))
REPRESENTATION_ITEM('')
SURFACE()
);
#1228=(
BOUNDED_SURFACE()
B_SPLINE_SURFACE(1,2,((#114446,#114447,#114448,#114449,#114450),(#114451,
#114452,#114453,#114454,#114455)),.UNSPECIFIED.,.F.,.F.,.F.)
B_SPLINE_SURFACE_WITH_KNOTS((2,2),(3,2,3),(0.710192959007197,1.),(0.262924618389841,
0.263098999273796,0.280537087669266),.UNSPECIFIED.)
GEOMETRIC_REPRESENTATION_ITEM()
RATIONAL_B_SPLINE_SURFACE(((0.989150325841653,0.989150325841653,0.989150325841653,
0.991395311444461,0.996628941948308),(0.989150325841653,0.989150325841653,
0.989150325841653,0.991395311444461,0.996628941948308)))
REPRESENTATION_ITEM('')
SURFACE()
);
#1229=(
BOUNDED_SURFACE()
B_SPLINE_SURFACE(1,2,((#114463,#114464,#114465),(#114466,#114467,#114468)),
 .UNSPECIFIED.,.F.,.F.,.F.)
B_SPLINE_SURFACE_WITH_KNOTS((2,2),(3,3),(0.71031891563908,1.),(0.452822299828567,
0.470019760166368),.UNSPECIFIED.)
GEOMETRIC_REPRESENTATION_ITEM()
RATIONAL_B_SPLINE_SURFACE(((0.98875548626282,0.986817927519786,0.987787102172814),
(0.98875548626282,0.986817927519786,0.987787102172814)))
REPRESENTATION_ITEM('')
SURFACE()
);
#1230=(
BOUNDED_SURFACE()
B_SPLINE_SURFACE(1,2,((#114479,#114480,#114481,#114482,#114483),(#114484,
#114485,#114486,#114487,#114488)),.UNSPECIFIED.,.F.,.F.,.F.)
B_SPLINE_SURFACE_WITH_KNOTS((2,2),(3,2,3),(0.709593130094452,1.),(0.262499170161042,
0.263098999273796,0.280537087669266),.UNSPECIFIED.)
GEOMETRIC_REPRESENTATION_ITEM()
RATIONAL_B_SPLINE_SURFACE(((0.989150325841653,0.989150325841653,0.989150325841653,
0.991395311444461,0.996628941948308),(0.989150325841653,0.989150325841653,
0.989150325841653,0.991395311444461,0.996628941948308)))
REPRESENTATION_ITEM('')
SURFACE()
);
#1231=(
BOUNDED_SURFACE()
B_SPLINE_SURFACE(1,2,((#114496,#114497,#114498),(#114499,#114500,#114501)),
 .UNSPECIFIED.,.F.,.F.,.F.)
B_SPLINE_SURFACE_WITH_KNOTS((2,2),(3,3),(0.710318915639153,1.),(0.452822299828566,
0.470019760166367),.UNSPECIFIED.)
GEOMETRIC_REPRESENTATION_ITEM()
RATIONAL_B_SPLINE_SURFACE(((0.98875548626282,0.986817927519786,0.987787102172814),
(0.98875548626282,0.986817927519786,0.987787102172814)))
REPRESENTATION_ITEM('')
SURFACE()
);
#1232=(
BOUNDED_SURFACE()
B_SPLINE_SURFACE(1,2,((#114512,#114513,#114514,#114515,#114516),(#114517,
#114518,#114519,#114520,#114521)),.UNSPECIFIED.,.F.,.F.,.F.)
B_SPLINE_SURFACE_WITH_KNOTS((2,2),(3,2,3),(0.70959313010617,1.),(0.262499170172683,
0.263098999273796,0.280537087669266),.UNSPECIFIED.)
GEOMETRIC_REPRESENTATION_ITEM()
RATIONAL_B_SPLINE_SURFACE(((0.989150325841653,0.989150325841653,0.989150325841653,
0.991395311444461,0.996628941948308),(0.989150325841653,0.989150325841653,
0.989150325841653,0.991395311444461,0.996628941948308)))
REPRESENTATION_ITEM('')
SURFACE()
);
#1233=(
BOUNDED_SURFACE()
B_SPLINE_SURFACE(1,2,((#114529,#114530,#114531),(#114532,#114533,#114534)),
 .UNSPECIFIED.,.F.,.F.,.F.)
B_SPLINE_SURFACE_WITH_KNOTS((2,2),(3,3),(0.710318915638837,1.),(0.452822299828566,
0.470019760166367),.UNSPECIFIED.)
GEOMETRIC_REPRESENTATION_ITEM()
RATIONAL_B_SPLINE_SURFACE(((0.98875548626282,0.986817927519786,0.987787102172814),
(0.98875548626282,0.986817927519786,0.987787102172814)))
REPRESENTATION_ITEM('')
SURFACE()
);
#1234=(
BOUNDED_SURFACE()
B_SPLINE_SURFACE(1,2,((#114545,#114546,#114547,#114548,#114549),(#114550,
#114551,#114552,#114553,#114554)),.UNSPECIFIED.,.F.,.F.,.F.)
B_SPLINE_SURFACE_WITH_KNOTS((2,2),(3,2,3),(0.709593130114102,1.),(0.262499170180933,
0.263098999273796,0.280537087669266),.UNSPECIFIED.)
GEOMETRIC_REPRESENTATION_ITEM()
RATIONAL_B_SPLINE_SURFACE(((0.989150325841653,0.989150325841653,0.989150325841653,
0.991395311444461,0.996628941948308),(0.989150325841653,0.989150325841653,
0.989150325841653,0.991395311444461,0.996628941948308)))
REPRESENTATION_ITEM('')
SURFACE()
);
#1235=(
BOUNDED_SURFACE()
B_SPLINE_SURFACE(1,2,((#114562,#114563,#114564),(#114565,#114566,#114567)),
 .UNSPECIFIED.,.F.,.F.,.F.)
B_SPLINE_SURFACE_WITH_KNOTS((2,2),(3,3),(0.710318915638982,1.),(0.452822299828566,
0.470019760166367),.UNSPECIFIED.)
GEOMETRIC_REPRESENTATION_ITEM()
RATIONAL_B_SPLINE_SURFACE(((0.98875548626282,0.986817927519786,0.987787102172814),
(0.98875548626282,0.986817927519786,0.987787102172814)))
REPRESENTATION_ITEM('')
SURFACE()
);
#1236=(
BOUNDED_SURFACE()
B_SPLINE_SURFACE(1,2,((#114578,#114579,#114580,#114581,#114582),(#114583,
#114584,#114585,#114586,#114587)),.UNSPECIFIED.,.F.,.F.,.F.)
B_SPLINE_SURFACE_WITH_KNOTS((2,2),(3,2,3),(0.709593130112758,1.),(0.262499170191214,
0.263098999273796,0.280537087669266),.UNSPECIFIED.)
GEOMETRIC_REPRESENTATION_ITEM()
RATIONAL_B_SPLINE_SURFACE(((0.989150325841653,0.989150325841653,0.989150325841653,
0.991395311444461,0.996628941948308),(0.989150325841653,0.989150325841653,
0.989150325841653,0.991395311444461,0.996628941948308)))
REPRESENTATION_ITEM('')
SURFACE()
);
#1237=(
BOUNDED_SURFACE()
B_SPLINE_SURFACE(1,2,((#114601,#114602,#114603),(#114604,#114605,#114606)),
 .UNSPECIFIED.,.F.,.F.,.F.)
B_SPLINE_SURFACE_WITH_KNOTS((2,2),(3,3),(0.710318915638967,1.),(0.452822299828566,
0.470019760166367),.UNSPECIFIED.)
GEOMETRIC_REPRESENTATION_ITEM()
RATIONAL_B_SPLINE_SURFACE(((0.98875548626282,0.986817927519786,0.987787102172814),
(0.98875548626282,0.986817927519786,0.987787102172814)))
REPRESENTATION_ITEM('')
SURFACE()
);
#1238=(
BOUNDED_SURFACE()
B_SPLINE_SURFACE(1,2,((#114608,#114609,#114610),(#114611,#114612,#114613)),
 .UNSPECIFIED.,.F.,.F.,.F.)
B_SPLINE_SURFACE_WITH_KNOTS((2,2),(3,3),(0.710318915639666,1.),(0.297753987024626,
0.314942866188521),.UNSPECIFIED.)
GEOMETRIC_REPRESENTATION_ITEM()
RATIONAL_B_SPLINE_SURFACE(((0.992972556818501,0.988973049555645,0.987877375613931),
(0.992972556818501,0.988973049555645,0.987877375613931)))
REPRESENTATION_ITEM('')
SURFACE()
);
#1239=(
BOUNDED_SURFACE()
B_SPLINE_SURFACE(1,2,((#114622,#114623,#114624,#114625,#114626),(#114627,
#114628,#114629,#114630,#114631)),.UNSPECIFIED.,.F.,.F.,.F.)
B_SPLINE_SURFACE_WITH_KNOTS((2,2),(3,2,3),(0.710192959008103,1.),(0.418312080773434,
0.428571428571429,0.435879799328077),.UNSPECIFIED.)
GEOMETRIC_REPRESENTATION_ITEM()
RATIONAL_B_SPLINE_SURFACE(((0.99383221411677,0.996398874234721,1.,0.997434694412141,
0.995394338545807),(0.99383221411677,0.996398874234721,1.,0.997434694412141,
0.995394338545807)))
REPRESENTATION_ITEM('')
SURFACE()
);
#1240=(
BOUNDED_SURFACE()
B_SPLINE_SURFACE(1,2,((#114646,#114647,#114648),(#114649,#114650,#114651)),
 .UNSPECIFIED.,.F.,.F.,.F.)
B_SPLINE_SURFACE_WITH_KNOTS((2,2),(3,3),(0.710318915639748,1.),(0.297753987024626,
0.314942866188516),.UNSPECIFIED.)
GEOMETRIC_REPRESENTATION_ITEM()
RATIONAL_B_SPLINE_SURFACE(((0.992972556818501,0.988973049555646,0.987877375613931),
(0.992972556818501,0.988973049555646,0.987877375613931)))
REPRESENTATION_ITEM('')
SURFACE()
);
#1241=(
BOUNDED_SURFACE()
B_SPLINE_SURFACE(1,2,((#114653,#114654,#114655,#114656,#114657),(#114658,
#114659,#114660,#114661,#114662)),.UNSPECIFIED.,.F.,.F.,.F.)
B_SPLINE_SURFACE_WITH_KNOTS((2,2),(3,2,3),(0.710192959007989,1.),(0.418312080773434,
0.428571428571429,0.435879799327622),.UNSPECIFIED.)
GEOMETRIC_REPRESENTATION_ITEM()
RATIONAL_B_SPLINE_SURFACE(((0.99383221411677,0.996398874234721,1.,0.997434694412301,
0.995394338546061),(0.99383221411677,0.996398874234721,1.,0.997434694412301,
0.995394338546061)))
REPRESENTATION_ITEM('')
SURFACE()
);
#1242=(
BOUNDED_SURFACE()
B_SPLINE_SURFACE(1,2,((#114677,#114678,#114679),(#114680,#114681,#114682)),
 .UNSPECIFIED.,.F.,.F.,.F.)
B_SPLINE_SURFACE_WITH_KNOTS((2,2),(3,3),(0.710318915639632,1.),(0.297753987024127,
0.314942866188516),.UNSPECIFIED.)
GEOMETRIC_REPRESENTATION_ITEM()
RATIONAL_B_SPLINE_SURFACE(((0.992972556818734,0.988973049555678,0.987877375613931),
(0.992972556818734,0.988973049555678,0.987877375613931)))
REPRESENTATION_ITEM('')
SURFACE()
);
#1243=(
BOUNDED_SURFACE()
B_SPLINE_SURFACE(1,2,((#114684,#114685,#114686,#114687,#114688),(#114689,
#114690,#114691,#114692,#114693)),.UNSPECIFIED.,.F.,.F.,.F.)
B_SPLINE_SURFACE_WITH_KNOTS((2,2),(3,2,3),(0.710192959006973,1.),(0.41831208077343,
0.428571428571429,0.435879799328077),.UNSPECIFIED.)
GEOMETRIC_REPRESENTATION_ITEM()
RATIONAL_B_SPLINE_SURFACE(((0.993832214116768,0.996398874234719,1.,0.997434694412141,
0.995394338545807),(0.993832214116768,0.996398874234719,1.,0.997434694412141,
0.995394338545807)))
REPRESENTATION_ITEM('')
SURFACE()
);
#1244=(
BOUNDED_SURFACE()
B_SPLINE_SURFACE(1,2,((#114708,#114709,#114710),(#114711,#114712,#114713)),
 .UNSPECIFIED.,.F.,.F.,.F.)
B_SPLINE_SURFACE_WITH_KNOTS((2,2),(3,3),(0.71031891563896,1.),(0.297753987024626,
0.314942866188516),.UNSPECIFIED.)
GEOMETRIC_REPRESENTATION_ITEM()
RATIONAL_B_SPLINE_SURFACE(((0.992972556818501,0.988973049555646,0.987877375613931),
(0.992972556818501,0.988973049555646,0.987877375613931)))
REPRESENTATION_ITEM('')
SURFACE()
);
#1245=(
BOUNDED_SURFACE()
B_SPLINE_SURFACE(1,2,((#114715,#114716,#114717,#114718,#114719),(#114720,
#114721,#114722,#114723,#114724)),.UNSPECIFIED.,.F.,.F.,.F.)
B_SPLINE_SURFACE_WITH_KNOTS((2,2),(3,2,3),(0.710192959007242,1.),(0.418312080773432,
0.428571428571429,0.435879799328077),.UNSPECIFIED.)
GEOMETRIC_REPRESENTATION_ITEM()
RATIONAL_B_SPLINE_SURFACE(((0.993832214116769,0.99639887423472,1.,0.997434694412141,
0.995394338545807),(0.993832214116769,0.99639887423472,1.,0.997434694412141,
0.995394338545807)))
REPRESENTATION_ITEM('')
SURFACE()
);
#1246=(
BOUNDED_SURFACE()
B_SPLINE_SURFACE(1,2,((#114739,#114740,#114741),(#114742,#114743,#114744)),
 .UNSPECIFIED.,.F.,.F.,.F.)
B_SPLINE_SURFACE_WITH_KNOTS((2,2),(3,3),(0.710318915639108,1.),(0.297753987024626,
0.314942866188543),.UNSPECIFIED.)
GEOMETRIC_REPRESENTATION_ITEM()
RATIONAL_B_SPLINE_SURFACE(((0.992972556818502,0.98897304955564,0.987877375613928),
(0.992972556818501,0.98897304955564,0.987877375613928)))
REPRESENTATION_ITEM('')
SURFACE()
);
#1247=(
BOUNDED_SURFACE()
B_SPLINE_SURFACE(1,2,((#114746,#114747,#114748,#114749,#114750),(#114751,
#114752,#114753,#114754,#114755)),.UNSPECIFIED.,.F.,.F.,.F.)
B_SPLINE_SURFACE_WITH_KNOTS((2,2),(3,2,3),(0.710192959007502,1.),(0.418312080773435,
0.428571428571429,0.435879799328077),.UNSPECIFIED.)
GEOMETRIC_REPRESENTATION_ITEM()
RATIONAL_B_SPLINE_SURFACE(((0.99383221411677,0.996398874234721,1.,0.997434694412141,
0.995394338545807),(0.99383221411677,0.996398874234721,1.,0.997434694412141,
0.995394338545807)))
REPRESENTATION_ITEM('')
SURFACE()
);
#1248=(
BOUNDED_SURFACE()
B_SPLINE_SURFACE(1,2,((#114770,#114771,#114772),(#114773,#114774,#114775)),
 .UNSPECIFIED.,.F.,.F.,.F.)
B_SPLINE_SURFACE_WITH_KNOTS((2,2),(3,3),(0.710318915639139,1.),(0.297753987024626,
0.314942866188516),.UNSPECIFIED.)
GEOMETRIC_REPRESENTATION_ITEM()
RATIONAL_B_SPLINE_SURFACE(((0.992972556818501,0.988973049555646,0.987877375613931),
(0.992972556818501,0.988973049555646,0.987877375613931)))
REPRESENTATION_ITEM('')
SURFACE()
);
#1249=(
BOUNDED_SURFACE()
B_SPLINE_SURFACE(1,2,((#114777,#114778,#114779,#114780,#114781),(#114782,
#114783,#114784,#114785,#114786)),.UNSPECIFIED.,.F.,.F.,.F.)
B_SPLINE_SURFACE_WITH_KNOTS((2,2),(3,2,3),(0.710192959007329,1.),(0.418312080773434,
0.428571428571429,0.435879799328077),.UNSPECIFIED.)
GEOMETRIC_REPRESENTATION_ITEM()
RATIONAL_B_SPLINE_SURFACE(((0.99383221411677,0.996398874234721,1.,0.997434694412141,
0.995394338545807),(0.99383221411677,0.996398874234721,1.,0.997434694412141,
0.995394338545807)))
REPRESENTATION_ITEM('')
SURFACE()
);
#1250=(
BOUNDED_SURFACE()
B_SPLINE_SURFACE(1,2,((#114801,#114802,#114803),(#114804,#114805,#114806)),
 .UNSPECIFIED.,.F.,.F.,.F.)
B_SPLINE_SURFACE_WITH_KNOTS((2,2),(3,3),(0.710318915638972,1.),(0.297753987024626,
0.314942866188516),.UNSPECIFIED.)
GEOMETRIC_REPRESENTATION_ITEM()
RATIONAL_B_SPLINE_SURFACE(((0.992972556818502,0.988973049555647,0.987877375613931),
(0.992972556818502,0.988973049555647,0.987877375613931)))
REPRESENTATION_ITEM('')
SURFACE()
);
#1251=(
BOUNDED_SURFACE()
B_SPLINE_SURFACE(1,2,((#114808,#114809,#114810,#114811,#114812),(#114813,
#114814,#114815,#114816,#114817)),.UNSPECIFIED.,.F.,.F.,.F.)
B_SPLINE_SURFACE_WITH_KNOTS((2,2),(3,2,3),(0.710192959008261,1.),(0.418312080773434,
0.428571428571429,0.435879799328077),.UNSPECIFIED.)
GEOMETRIC_REPRESENTATION_ITEM()
RATIONAL_B_SPLINE_SURFACE(((0.99383221411677,0.996398874234721,1.,0.997434694412141,
0.995394338545807),(0.99383221411677,0.996398874234721,1.,0.997434694412141,
0.995394338545807)))
REPRESENTATION_ITEM('')
SURFACE()
);
#1252=(
BOUNDED_SURFACE()
B_SPLINE_SURFACE(1,2,((#114832,#114833,#114834),(#114835,#114836,#114837)),
 .UNSPECIFIED.,.F.,.F.,.F.)
B_SPLINE_SURFACE_WITH_KNOTS((2,2),(3,3),(0.710318915639903,1.),(0.297753987024626,
0.314942866188516),.UNSPECIFIED.)
GEOMETRIC_REPRESENTATION_ITEM()
RATIONAL_B_SPLINE_SURFACE(((0.992972556818501,0.988973049555646,0.987877375613931),
(0.992972556818501,0.988973049555646,0.987877375613931)))
REPRESENTATION_ITEM('')
SURFACE()
);
#1253=(
BOUNDED_SURFACE()
B_SPLINE_SURFACE(1,2,((#114839,#114840,#114841,#114842,#114843),(#114844,
#114845,#114846,#114847,#114848)),.UNSPECIFIED.,.F.,.F.,.F.)
B_SPLINE_SURFACE_WITH_KNOTS((2,2),(3,2,3),(0.71019295900825,1.),(0.418312080773434,
0.428571428571429,0.435879799328077),.UNSPECIFIED.)
GEOMETRIC_REPRESENTATION_ITEM()
RATIONAL_B_SPLINE_SURFACE(((0.99383221411677,0.996398874234721,1.,0.997434694412141,
0.995394338545807),(0.99383221411677,0.996398874234721,1.,0.997434694412141,
0.995394338545807)))
REPRESENTATION_ITEM('')
SURFACE()
);
#1254=(
BOUNDED_SURFACE()
B_SPLINE_SURFACE(1,2,((#114863,#114864,#114865),(#114866,#114867,#114868)),
 .UNSPECIFIED.,.F.,.F.,.F.)
B_SPLINE_SURFACE_WITH_KNOTS((2,2),(3,3),(0.710318915639894,1.),(0.297753987024626,
0.314942866188516),.UNSPECIFIED.)
GEOMETRIC_REPRESENTATION_ITEM()
RATIONAL_B_SPLINE_SURFACE(((0.992972556818502,0.988973049555647,0.987877375613931),
(0.992972556818502,0.988973049555647,0.987877375613931)))
REPRESENTATION_ITEM('')
SURFACE()
);
#1255=(
BOUNDED_SURFACE()
B_SPLINE_SURFACE(1,2,((#114870,#114871,#114872,#114873,#114874),(#114875,
#114876,#114877,#114878,#114879)),.UNSPECIFIED.,.F.,.F.,.F.)
B_SPLINE_SURFACE_WITH_KNOTS((2,2),(3,2,3),(0.710192959008146,1.),(0.418312080773434,
0.428571428571429,0.435879799328077),.UNSPECIFIED.)
GEOMETRIC_REPRESENTATION_ITEM()
RATIONAL_B_SPLINE_SURFACE(((0.99383221411677,0.996398874234721,1.,0.997434694412141,
0.995394338545807),(0.99383221411677,0.996398874234721,1.,0.997434694412141,
0.995394338545807)))
REPRESENTATION_ITEM('')
SURFACE()
);
#1256=(
BOUNDED_SURFACE()
B_SPLINE_SURFACE(1,2,((#114894,#114895,#114896),(#114897,#114898,#114899)),
 .UNSPECIFIED.,.F.,.F.,.F.)
B_SPLINE_SURFACE_WITH_KNOTS((2,2),(3,3),(0.710318915639792,1.),(0.29775398702454,
0.314942866188516),.UNSPECIFIED.)
GEOMETRIC_REPRESENTATION_ITEM()
RATIONAL_B_SPLINE_SURFACE(((0.992972556818541,0.988973049555652,0.987877375613931),
(0.992972556818541,0.988973049555652,0.987877375613931)))
REPRESENTATION_ITEM('')
SURFACE()
);
#1257=(
BOUNDED_SURFACE()
B_SPLINE_SURFACE(1,2,((#114901,#114902,#114903,#114904,#114905),(#114906,
#114907,#114908,#114909,#114910)),.UNSPECIFIED.,.F.,.F.,.F.)
B_SPLINE_SURFACE_WITH_KNOTS((2,2),(3,2,3),(0.710192959008211,1.),(0.418312080773434,
0.428571428571429,0.435879799328077),.UNSPECIFIED.)
GEOMETRIC_REPRESENTATION_ITEM()
RATIONAL_B_SPLINE_SURFACE(((0.99383221411677,0.996398874234721,1.,0.997434694412141,
0.995394338545807),(0.99383221411677,0.996398874234721,1.,0.997434694412141,
0.995394338545807)))
REPRESENTATION_ITEM('')
SURFACE()
);
#1258=(
BOUNDED_SURFACE()
B_SPLINE_SURFACE(1,2,((#114925,#114926,#114927),(#114928,#114929,#114930)),
 .UNSPECIFIED.,.F.,.F.,.F.)
B_SPLINE_SURFACE_WITH_KNOTS((2,2),(3,3),(0.710318915639852,1.),(0.297753987024605,
0.314942866188516),.UNSPECIFIED.)
GEOMETRIC_REPRESENTATION_ITEM()
RATIONAL_B_SPLINE_SURFACE(((0.992972556818511,0.988973049555648,0.987877375613931),
(0.992972556818511,0.988973049555648,0.987877375613931)))
REPRESENTATION_ITEM('')
SURFACE()
);
#1259=(
BOUNDED_SURFACE()
B_SPLINE_SURFACE(1,2,((#114932,#114933,#114934,#114935,#114936),(#114937,
#114938,#114939,#114940,#114941)),.UNSPECIFIED.,.F.,.F.,.F.)
B_SPLINE_SURFACE_WITH_KNOTS((2,2),(3,2,3),(0.710192959008243,1.),(0.418312080773434,
0.428571428571429,0.435879799328077),.UNSPECIFIED.)
GEOMETRIC_REPRESENTATION_ITEM()
RATIONAL_B_SPLINE_SURFACE(((0.99383221411677,0.996398874234721,1.,0.997434694412141,
0.995394338545807),(0.99383221411677,0.996398874234721,1.,0.997434694412141,
0.995394338545807)))
REPRESENTATION_ITEM('')
SURFACE()
);
#1260=(
BOUNDED_SURFACE()
B_SPLINE_SURFACE(1,2,((#114956,#114957,#114958),(#114959,#114960,#114961)),
 .UNSPECIFIED.,.F.,.F.,.F.)
B_SPLINE_SURFACE_WITH_KNOTS((2,2),(3,3),(0.71031891563988,1.),(0.297753987024518,
0.314942866188516),.UNSPECIFIED.)
GEOMETRIC_REPRESENTATION_ITEM()
RATIONAL_B_SPLINE_SURFACE(((0.992972556818552,0.988973049555653,0.987877375613931),
(0.992972556818552,0.988973049555653,0.987877375613931)))
REPRESENTATION_ITEM('')
SURFACE()
);
#1261=(
BOUNDED_SURFACE()
B_SPLINE_SURFACE(1,2,((#114963,#114964,#114965,#114966,#114967),(#114968,
#114969,#114970,#114971,#114972)),.UNSPECIFIED.,.F.,.F.,.F.)
B_SPLINE_SURFACE_WITH_KNOTS((2,2),(3,2,3),(0.71019295900829,1.),(0.418312080773434,
0.428571428571429,0.435879799328077),.UNSPECIFIED.)
GEOMETRIC_REPRESENTATION_ITEM()
RATIONAL_B_SPLINE_SURFACE(((0.99383221411677,0.996398874234721,1.,0.997434694412141,
0.995394338545807),(0.99383221411677,0.996398874234721,1.,0.997434694412141,
0.995394338545807)))
REPRESENTATION_ITEM('')
SURFACE()
);
#1262=(
BOUNDED_SURFACE()
B_SPLINE_SURFACE(1,2,((#114987,#114988,#114989),(#114990,#114991,#114992)),
 .UNSPECIFIED.,.F.,.F.,.F.)
B_SPLINE_SURFACE_WITH_KNOTS((2,2),(3,3),(0.710318915639924,1.),(0.297753987024626,
0.314942866188516),.UNSPECIFIED.)
GEOMETRIC_REPRESENTATION_ITEM()
RATIONAL_B_SPLINE_SURFACE(((0.992972556818502,0.988973049555646,0.987877375613931),
(0.992972556818502,0.988973049555646,0.987877375613931)))
REPRESENTATION_ITEM('')
SURFACE()
);
#1263=(
BOUNDED_SURFACE()
B_SPLINE_SURFACE(1,2,((#114994,#114995,#114996,#114997,#114998),(#114999,
#115000,#115001,#115002,#115003)),.UNSPECIFIED.,.F.,.F.,.F.)
B_SPLINE_SURFACE_WITH_KNOTS((2,2),(3,2,3),(0.710192959008442,1.),(0.418312080773434,
0.428571428571429,0.435879799328077),.UNSPECIFIED.)
GEOMETRIC_REPRESENTATION_ITEM()
RATIONAL_B_SPLINE_SURFACE(((0.99383221411677,0.996398874234721,1.,0.997434694412141,
0.995394338545807),(0.99383221411677,0.996398874234721,1.,0.997434694412141,
0.995394338545807)))
REPRESENTATION_ITEM('')
SURFACE()
);
#1264=(
BOUNDED_SURFACE()
B_SPLINE_SURFACE(1,2,((#115018,#115019,#115020),(#115021,#115022,#115023)),
 .UNSPECIFIED.,.F.,.F.,.F.)
B_SPLINE_SURFACE_WITH_KNOTS((2,2),(3,3),(0.710318915640075,1.),(0.297753987024626,
0.314942866188516),.UNSPECIFIED.)
GEOMETRIC_REPRESENTATION_ITEM()
RATIONAL_B_SPLINE_SURFACE(((0.992972556818502,0.988973049555646,0.987877375613931),
(0.992972556818502,0.988973049555646,0.987877375613931)))
REPRESENTATION_ITEM('')
SURFACE()
);
#1265=(
BOUNDED_SURFACE()
B_SPLINE_SURFACE(1,2,((#115025,#115026,#115027,#115028,#115029),(#115030,
#115031,#115032,#115033,#115034)),.UNSPECIFIED.,.F.,.F.,.F.)
B_SPLINE_SURFACE_WITH_KNOTS((2,2),(3,2,3),(0.710192959008442,1.),(0.418312080773434,
0.428571428571429,0.435879799328077),.UNSPECIFIED.)
GEOMETRIC_REPRESENTATION_ITEM()
RATIONAL_B_SPLINE_SURFACE(((0.99383221411677,0.996398874234721,1.,0.997434694412141,
0.995394338545807),(0.99383221411677,0.996398874234721,1.,0.997434694412141,
0.995394338545807)))
REPRESENTATION_ITEM('')
SURFACE()
);
#1266=(
BOUNDED_SURFACE()
B_SPLINE_SURFACE(1,2,((#115049,#115050,#115051),(#115052,#115053,#115054)),
 .UNSPECIFIED.,.F.,.F.,.F.)
B_SPLINE_SURFACE_WITH_KNOTS((2,2),(3,3),(0.710318915640075,1.),(0.297753987024626,
0.314942866188516),.UNSPECIFIED.)
GEOMETRIC_REPRESENTATION_ITEM()
RATIONAL_B_SPLINE_SURFACE(((0.992972556818501,0.988973049555646,0.987877375613931),
(0.992972556818501,0.988973049555646,0.987877375613931)))
REPRESENTATION_ITEM('')
SURFACE()
);
#1267=(
BOUNDED_SURFACE()
B_SPLINE_SURFACE(1,2,((#115056,#115057,#115058,#115059,#115060),(#115061,
#115062,#115063,#115064,#115065)),.UNSPECIFIED.,.F.,.F.,.F.)
B_SPLINE_SURFACE_WITH_KNOTS((2,2),(3,2,3),(0.710192959008435,1.),(0.418312080773434,
0.428571428571429,0.435879799328077),.UNSPECIFIED.)
GEOMETRIC_REPRESENTATION_ITEM()
RATIONAL_B_SPLINE_SURFACE(((0.99383221411677,0.996398874234721,1.,0.997434694412141,
0.995394338545807),(0.99383221411677,0.996398874234721,1.,0.997434694412141,
0.995394338545807)))
REPRESENTATION_ITEM('')
SURFACE()
);
#1268=(
BOUNDED_SURFACE()
B_SPLINE_SURFACE(1,2,((#115080,#115081,#115082),(#115083,#115084,#115085)),
 .UNSPECIFIED.,.F.,.F.,.F.)
B_SPLINE_SURFACE_WITH_KNOTS((2,2),(3,3),(0.710318915640074,1.),(0.297753987024626,
0.314942866188517),.UNSPECIFIED.)
GEOMETRIC_REPRESENTATION_ITEM()
RATIONAL_B_SPLINE_SURFACE(((0.992972556818502,0.988973049555646,0.987877375613931),
(0.992972556818502,0.988973049555646,0.987877375613931)))
REPRESENTATION_ITEM('')
SURFACE()
);
#1269=(
BOUNDED_SURFACE()
B_SPLINE_SURFACE(1,2,((#115087,#115088,#115089,#115090,#115091),(#115092,
#115093,#115094,#115095,#115096)),.UNSPECIFIED.,.F.,.F.,.F.)
B_SPLINE_SURFACE_WITH_KNOTS((2,2),(3,2,3),(0.710192959008438,1.),(0.418312080773434,
0.428571428571429,0.435879799328077),.UNSPECIFIED.)
GEOMETRIC_REPRESENTATION_ITEM()
RATIONAL_B_SPLINE_SURFACE(((0.99383221411677,0.996398874234721,1.,0.997434694412141,
0.995394338545807),(0.99383221411677,0.996398874234721,1.,0.997434694412141,
0.995394338545807)))
REPRESENTATION_ITEM('')
SURFACE()
);
#1270=(
BOUNDED_SURFACE()
B_SPLINE_SURFACE(1,2,((#115111,#115112,#115113),(#115114,#115115,#115116)),
 .UNSPECIFIED.,.F.,.F.,.F.)
B_SPLINE_SURFACE_WITH_KNOTS((2,2),(3,3),(0.710318915640078,1.),(0.297753987024626,
0.314942866188516),.UNSPECIFIED.)
GEOMETRIC_REPRESENTATION_ITEM()
RATIONAL_B_SPLINE_SURFACE(((0.992972556818502,0.988973049555647,0.987877375613931),
(0.992972556818502,0.988973049555646,0.987877375613931)))
REPRESENTATION_ITEM('')
SURFACE()
);
#1271=(
BOUNDED_SURFACE()
B_SPLINE_SURFACE(1,2,((#115118,#115119,#115120,#115121,#115122),(#115123,
#115124,#115125,#115126,#115127)),.UNSPECIFIED.,.F.,.F.,.F.)
B_SPLINE_SURFACE_WITH_KNOTS((2,2),(3,2,3),(0.710192959008439,1.),(0.418312080773434,
0.428571428571429,0.435879799328077),.UNSPECIFIED.)
GEOMETRIC_REPRESENTATION_ITEM()
RATIONAL_B_SPLINE_SURFACE(((0.99383221411677,0.996398874234721,1.,0.997434694412141,
0.995394338545807),(0.99383221411677,0.996398874234721,1.,0.997434694412141,
0.995394338545807)))
REPRESENTATION_ITEM('')
SURFACE()
);
#1272=(
BOUNDED_SURFACE()
B_SPLINE_SURFACE(1,2,((#115142,#115143,#115144),(#115145,#115146,#115147)),
 .UNSPECIFIED.,.F.,.F.,.F.)
B_SPLINE_SURFACE_WITH_KNOTS((2,2),(3,3),(0.710318915640077,1.),(0.297753987024626,
0.314942866188516),.UNSPECIFIED.)
GEOMETRIC_REPRESENTATION_ITEM()
RATIONAL_B_SPLINE_SURFACE(((0.992972556818502,0.988973049555646,0.987877375613931),
(0.992972556818502,0.988973049555646,0.987877375613931)))
REPRESENTATION_ITEM('')
SURFACE()
);
#1273=(
BOUNDED_SURFACE()
B_SPLINE_SURFACE(1,2,((#115149,#115150,#115151,#115152,#115153),(#115154,
#115155,#115156,#115157,#115158)),.UNSPECIFIED.,.F.,.F.,.F.)
B_SPLINE_SURFACE_WITH_KNOTS((2,2),(3,2,3),(0.710192959008327,1.),(0.418312080773434,
0.428571428571429,0.435879799328077),.UNSPECIFIED.)
GEOMETRIC_REPRESENTATION_ITEM()
RATIONAL_B_SPLINE_SURFACE(((0.99383221411677,0.996398874234721,1.,0.997434694412141,
0.995394338545807),(0.99383221411677,0.996398874234721,1.,0.997434694412141,
0.995394338545807)))
REPRESENTATION_ITEM('')
SURFACE()
);
#1274=(
BOUNDED_SURFACE()
B_SPLINE_SURFACE(1,2,((#115173,#115174,#115175),(#115176,#115177,#115178)),
 .UNSPECIFIED.,.F.,.F.,.F.)
B_SPLINE_SURFACE_WITH_KNOTS((2,2),(3,3),(0.710318915639967,1.),(0.297753987024626,
0.314942866188516),.UNSPECIFIED.)
GEOMETRIC_REPRESENTATION_ITEM()
RATIONAL_B_SPLINE_SURFACE(((0.992972556818502,0.988973049555646,0.987877375613931),
(0.992972556818502,0.988973049555646,0.987877375613931)))
REPRESENTATION_ITEM('')
SURFACE()
);
#1275=(
BOUNDED_SURFACE()
B_SPLINE_SURFACE(1,2,((#115180,#115181,#115182,#115183,#115184),(#115185,
#115186,#115187,#115188,#115189)),.UNSPECIFIED.,.F.,.F.,.F.)
B_SPLINE_SURFACE_WITH_KNOTS((2,2),(3,2,3),(0.71019295900703,1.),(0.418312080773434,
0.428571428571429,0.435879799328077),.UNSPECIFIED.)
GEOMETRIC_REPRESENTATION_ITEM()
RATIONAL_B_SPLINE_SURFACE(((0.99383221411677,0.996398874234721,1.,0.997434694412141,
0.995394338545807),(0.99383221411677,0.996398874234721,1.,0.997434694412141,
0.995394338545807)))
REPRESENTATION_ITEM('')
SURFACE()
);
#1276=(
BOUNDED_SURFACE()
B_SPLINE_SURFACE(1,2,((#115204,#115205,#115206),(#115207,#115208,#115209)),
 .UNSPECIFIED.,.F.,.F.,.F.)
B_SPLINE_SURFACE_WITH_KNOTS((2,2),(3,3),(0.71031891563867,1.),(0.297753987024626,
0.314942866188516),.UNSPECIFIED.)
GEOMETRIC_REPRESENTATION_ITEM()
RATIONAL_B_SPLINE_SURFACE(((0.992972556818502,0.988973049555647,0.987877375613931),
(0.992972556818502,0.988973049555647,0.987877375613931)))
REPRESENTATION_ITEM('')
SURFACE()
);
#1277=(
BOUNDED_SURFACE()
B_SPLINE_SURFACE(1,2,((#115211,#115212,#115213,#115214,#115215),(#115216,
#115217,#115218,#115219,#115220)),.UNSPECIFIED.,.F.,.F.,.F.)
B_SPLINE_SURFACE_WITH_KNOTS((2,2),(3,2,3),(0.710192959008186,1.),(0.418312080773434,
0.428571428571429,0.435879799328077),.UNSPECIFIED.)
GEOMETRIC_REPRESENTATION_ITEM()
RATIONAL_B_SPLINE_SURFACE(((0.99383221411677,0.996398874234721,1.,0.997434694412141,
0.995394338545807),(0.99383221411677,0.996398874234721,1.,0.997434694412141,
0.995394338545807)))
REPRESENTATION_ITEM('')
SURFACE()
);
#1278=(
BOUNDED_SURFACE()
B_SPLINE_SURFACE(1,2,((#115235,#115236,#115237),(#115238,#115239,#115240)),
 .UNSPECIFIED.,.F.,.F.,.F.)
B_SPLINE_SURFACE_WITH_KNOTS((2,2),(3,3),(0.710318915639825,1.),(0.297753987024626,
0.314942866188516),.UNSPECIFIED.)
GEOMETRIC_REPRESENTATION_ITEM()
RATIONAL_B_SPLINE_SURFACE(((0.992972556818502,0.988973049555647,0.987877375613931),
(0.992972556818502,0.988973049555647,0.987877375613931)))
REPRESENTATION_ITEM('')
SURFACE()
);
#1279=(
BOUNDED_SURFACE()
B_SPLINE_SURFACE(1,2,((#115242,#115243,#115244,#115245,#115246),(#115247,
#115248,#115249,#115250,#115251)),.UNSPECIFIED.,.F.,.F.,.F.)
B_SPLINE_SURFACE_WITH_KNOTS((2,2),(3,2,3),(0.710192959008442,1.),(0.418312080773434,
0.428571428571429,0.435879799328077),.UNSPECIFIED.)
GEOMETRIC_REPRESENTATION_ITEM()
RATIONAL_B_SPLINE_SURFACE(((0.99383221411677,0.996398874234721,1.,0.997434694412141,
0.995394338545807),(0.99383221411677,0.996398874234721,1.,0.997434694412141,
0.995394338545807)))
REPRESENTATION_ITEM('')
SURFACE()
);
#1280=(
BOUNDED_SURFACE()
B_SPLINE_SURFACE(1,2,((#115266,#115267,#115268),(#115269,#115270,#115271)),
 .UNSPECIFIED.,.F.,.F.,.F.)
B_SPLINE_SURFACE_WITH_KNOTS((2,2),(3,3),(0.710318915640081,1.),(0.297753987024626,
0.314942866188516),.UNSPECIFIED.)
GEOMETRIC_REPRESENTATION_ITEM()
RATIONAL_B_SPLINE_SURFACE(((0.992972556818501,0.988973049555646,0.987877375613931),
(0.992972556818501,0.988973049555646,0.987877375613931)))
REPRESENTATION_ITEM('')
SURFACE()
);
#1281=(
BOUNDED_SURFACE()
B_SPLINE_SURFACE(1,2,((#115273,#115274,#115275,#115276,#115277),(#115278,
#115279,#115280,#115281,#115282)),.UNSPECIFIED.,.F.,.F.,.F.)
B_SPLINE_SURFACE_WITH_KNOTS((2,2),(3,2,3),(0.71019295900844,1.),(0.418312080773434,
0.428571428571429,0.435879799328077),.UNSPECIFIED.)
GEOMETRIC_REPRESENTATION_ITEM()
RATIONAL_B_SPLINE_SURFACE(((0.99383221411677,0.996398874234721,1.,0.997434694412141,
0.995394338545807),(0.99383221411677,0.996398874234721,1.,0.997434694412141,
0.995394338545807)))
REPRESENTATION_ITEM('')
SURFACE()
);
#1282=(
BOUNDED_SURFACE()
B_SPLINE_SURFACE(1,2,((#115297,#115298,#115299),(#115300,#115301,#115302)),
 .UNSPECIFIED.,.F.,.F.,.F.)
B_SPLINE_SURFACE_WITH_KNOTS((2,2),(3,3),(0.710318915640086,1.),(0.297753987024626,
0.314942866188516),.UNSPECIFIED.)
GEOMETRIC_REPRESENTATION_ITEM()
RATIONAL_B_SPLINE_SURFACE(((0.992972556818502,0.988973049555646,0.987877375613931),
(0.992972556818502,0.988973049555646,0.987877375613931)))
REPRESENTATION_ITEM('')
SURFACE()
);
#1283=(
BOUNDED_SURFACE()
B_SPLINE_SURFACE(1,2,((#115304,#115305,#115306,#115307,#115308),(#115309,
#115310,#115311,#115312,#115313)),.UNSPECIFIED.,.F.,.F.,.F.)
B_SPLINE_SURFACE_WITH_KNOTS((2,2),(3,2,3),(0.710192959008441,1.),(0.418312080773434,
0.428571428571429,0.435879799328077),.UNSPECIFIED.)
GEOMETRIC_REPRESENTATION_ITEM()
RATIONAL_B_SPLINE_SURFACE(((0.99383221411677,0.996398874234721,1.,0.997434694412141,
0.995394338545807),(0.99383221411677,0.996398874234721,1.,0.997434694412141,
0.995394338545807)))
REPRESENTATION_ITEM('')
SURFACE()
);
#1284=(
BOUNDED_SURFACE()
B_SPLINE_SURFACE(1,2,((#115328,#115329,#115330),(#115331,#115332,#115333)),
 .UNSPECIFIED.,.F.,.F.,.F.)
B_SPLINE_SURFACE_WITH_KNOTS((2,2),(3,3),(0.710318915640077,1.),(0.297753987024626,
0.314942866188516),.UNSPECIFIED.)
GEOMETRIC_REPRESENTATION_ITEM()
RATIONAL_B_SPLINE_SURFACE(((0.992972556818502,0.988973049555646,0.987877375613931),
(0.992972556818502,0.988973049555646,0.987877375613931)))
REPRESENTATION_ITEM('')
SURFACE()
);
#1285=(
BOUNDED_SURFACE()
B_SPLINE_SURFACE(1,2,((#115335,#115336,#115337,#115338,#115339),(#115340,
#115341,#115342,#115343,#115344)),.UNSPECIFIED.,.F.,.F.,.F.)
B_SPLINE_SURFACE_WITH_KNOTS((2,2),(3,2,3),(0.71019295900772,1.),(0.418312080773434,
0.428571428571429,0.435879799328076),.UNSPECIFIED.)
GEOMETRIC_REPRESENTATION_ITEM()
RATIONAL_B_SPLINE_SURFACE(((0.99383221411677,0.996398874234721,1.,0.997434694412141,
0.995394338545808),(0.99383221411677,0.996398874234721,1.,0.997434694412141,
0.995394338545808)))
REPRESENTATION_ITEM('')
SURFACE()
);
#1286=(
BOUNDED_SURFACE()
B_SPLINE_SURFACE(1,2,((#115359,#115360,#115361),(#115362,#115363,#115364)),
 .UNSPECIFIED.,.F.,.F.,.F.)
B_SPLINE_SURFACE_WITH_KNOTS((2,2),(3,3),(0.710318915639364,1.),(0.297753987024627,
0.314942866188517),.UNSPECIFIED.)
GEOMETRIC_REPRESENTATION_ITEM()
RATIONAL_B_SPLINE_SURFACE(((0.992972556818501,0.988973049555646,0.987877375613931),
(0.992972556818501,0.988973049555646,0.987877375613931)))
REPRESENTATION_ITEM('')
SURFACE()
);
#1287=(
BOUNDED_SURFACE()
B_SPLINE_SURFACE(1,2,((#115366,#115367,#115368,#115369,#115370),(#115371,
#115372,#115373,#115374,#115375)),.UNSPECIFIED.,.F.,.F.,.F.)
B_SPLINE_SURFACE_WITH_KNOTS((2,2),(3,2,3),(0.710192959008172,1.),(0.418312080773433,
0.428571428571429,0.435879799328076),.UNSPECIFIED.)
GEOMETRIC_REPRESENTATION_ITEM()
RATIONAL_B_SPLINE_SURFACE(((0.993832214116769,0.99639887423472,1.,0.997434694412141,
0.995394338545808),(0.993832214116769,0.99639887423472,1.,0.997434694412141,
0.995394338545808)))
REPRESENTATION_ITEM('')
SURFACE()
);
#1288=(
BOUNDED_SURFACE()
B_SPLINE_SURFACE(1,2,((#115390,#115391,#115392),(#115393,#115394,#115395)),
 .UNSPECIFIED.,.F.,.F.,.F.)
B_SPLINE_SURFACE_WITH_KNOTS((2,2),(3,3),(0.710318915639813,1.),(0.297753987024418,
0.314942866188517),.UNSPECIFIED.)
GEOMETRIC_REPRESENTATION_ITEM()
RATIONAL_B_SPLINE_SURFACE(((0.992972556818598,0.988973049555659,0.987877375613931),
(0.992972556818598,0.988973049555659,0.987877375613931)))
REPRESENTATION_ITEM('')
SURFACE()
);
#1289=(
BOUNDED_SURFACE()
B_SPLINE_SURFACE(1,2,((#115397,#115398,#115399,#115400,#115401),(#115402,
#115403,#115404,#115405,#115406)),.UNSPECIFIED.,.F.,.F.,.F.)
B_SPLINE_SURFACE_WITH_KNOTS((2,2),(3,2,3),(0.710192959008117,1.),(0.418312080773433,
0.428571428571429,0.435879799328042),.UNSPECIFIED.)
GEOMETRIC_REPRESENTATION_ITEM()
RATIONAL_B_SPLINE_SURFACE(((0.99383221411677,0.99639887423472,1.,0.997434694412154,
0.995394338545827),(0.99383221411677,0.99639887423472,1.,0.997434694412154,
0.995394338545827)))
REPRESENTATION_ITEM('')
SURFACE()
);
#1290=(
BOUNDED_SURFACE()
B_SPLINE_SURFACE(1,2,((#115421,#115422,#115423),(#115424,#115425,#115426)),
 .UNSPECIFIED.,.F.,.F.,.F.)
B_SPLINE_SURFACE_WITH_KNOTS((2,2),(3,3),(0.710318915639757,1.),(0.297753987024401,
0.314942866188517),.UNSPECIFIED.)
GEOMETRIC_REPRESENTATION_ITEM()
RATIONAL_B_SPLINE_SURFACE(((0.992972556818606,0.98897304955566,0.987877375613931),
(0.992972556818606,0.98897304955566,0.987877375613931)))
REPRESENTATION_ITEM('')
SURFACE()
);
#1291=(
BOUNDED_SURFACE()
B_SPLINE_SURFACE(1,2,((#115428,#115429,#115430,#115431,#115432),(#115433,
#115434,#115435,#115436,#115437)),.UNSPECIFIED.,.F.,.F.,.F.)
B_SPLINE_SURFACE_WITH_KNOTS((2,2),(3,2,3),(0.710192959008159,1.),(0.418312080773433,
0.428571428571429,0.435879799328077),.UNSPECIFIED.)
GEOMETRIC_REPRESENTATION_ITEM()
RATIONAL_B_SPLINE_SURFACE(((0.993832214116769,0.99639887423472,1.,0.997434694412141,
0.995394338545807),(0.993832214116769,0.99639887423472,1.,0.997434694412141,
0.995394338545807)))
REPRESENTATION_ITEM('')
SURFACE()
);
#1292=(
BOUNDED_SURFACE()
B_SPLINE_SURFACE(1,2,((#115452,#115453,#115454),(#115455,#115456,#115457)),
 .UNSPECIFIED.,.F.,.F.,.F.)
B_SPLINE_SURFACE_WITH_KNOTS((2,2),(3,3),(0.710318915639801,1.),(0.297753987024479,
0.314942866188516),.UNSPECIFIED.)
GEOMETRIC_REPRESENTATION_ITEM()
RATIONAL_B_SPLINE_SURFACE(((0.99297255681857,0.988973049555656,0.987877375613931),
(0.99297255681857,0.988973049555656,0.987877375613931)))
REPRESENTATION_ITEM('')
SURFACE()
);
#1293=(
BOUNDED_SURFACE()
B_SPLINE_SURFACE(1,2,((#115459,#115460,#115461,#115462,#115463),(#115464,
#115465,#115466,#115467,#115468)),.UNSPECIFIED.,.F.,.F.,.F.)
B_SPLINE_SURFACE_WITH_KNOTS((2,2),(3,2,3),(0.71019295900798,1.),(0.418312080773434,
0.428571428571429,0.435879799328079),.UNSPECIFIED.)
GEOMETRIC_REPRESENTATION_ITEM()
RATIONAL_B_SPLINE_SURFACE(((0.99383221411677,0.996398874234721,1.,0.997434694412141,
0.995394338545806),(0.99383221411677,0.996398874234721,1.,0.997434694412141,
0.995394338545806)))
REPRESENTATION_ITEM('')
SURFACE()
);
#1294=(
BOUNDED_SURFACE()
B_SPLINE_SURFACE(1,2,((#115483,#115484,#115485),(#115486,#115487,#115488)),
 .UNSPECIFIED.,.F.,.F.,.F.)
B_SPLINE_SURFACE_WITH_KNOTS((2,2),(3,3),(0.710318915639618,1.),(0.297753987024626,
0.314942866188516),.UNSPECIFIED.)
GEOMETRIC_REPRESENTATION_ITEM()
RATIONAL_B_SPLINE_SURFACE(((0.992972556818502,0.988973049555647,0.987877375613931),
(0.992972556818502,0.988973049555647,0.987877375613931)))
REPRESENTATION_ITEM('')
SURFACE()
);
#1295=(
BOUNDED_SURFACE()
B_SPLINE_SURFACE(1,2,((#115490,#115491,#115492,#115493,#115494),(#115495,
#115496,#115497,#115498,#115499)),.UNSPECIFIED.,.F.,.F.,.F.)
B_SPLINE_SURFACE_WITH_KNOTS((2,2),(3,2,3),(0.710192959008018,1.),(0.418312080773434,
0.428571428571429,0.435879799328077),.UNSPECIFIED.)
GEOMETRIC_REPRESENTATION_ITEM()
RATIONAL_B_SPLINE_SURFACE(((0.99383221411677,0.996398874234721,1.,0.997434694412141,
0.995394338545807),(0.99383221411677,0.996398874234721,1.,0.997434694412141,
0.995394338545807)))
REPRESENTATION_ITEM('')
SURFACE()
);
#1296=(
BOUNDED_SURFACE()
B_SPLINE_SURFACE(1,2,((#115507,#115508,#115509,#115510,#115511),(#115512,
#115513,#115514,#115515,#115516)),.UNSPECIFIED.,.F.,.F.,.F.)
B_SPLINE_SURFACE_WITH_KNOTS((2,2),(3,2,3),(0.,0.28980704099156),(0.469846324360764,
0.470019760166365,0.487363340726489),.UNSPECIFIED.)
GEOMETRIC_REPRESENTATION_ITEM()
RATIONAL_B_SPLINE_SURFACE(((0.987787102172814,0.987787102172814,0.987787102172814,
0.988764511531024,0.992698258926487),(0.987787102172814,0.987787102172814,
0.987787102172814,0.988764511531024,0.992698258926487)))
REPRESENTATION_ITEM('')
SURFACE()
);
#1297=(
BOUNDED_SURFACE()
B_SPLINE_SURFACE(1,2,((#115525,#115526,#115527),(#115528,#115529,#115530)),
 .UNSPECIFIED.,.F.,.F.,.F.)
B_SPLINE_SURFACE_WITH_KNOTS((2,2),(3,3),(0.,0.289681084359914),(0.245851183393691,
0.263098999273814),.UNSPECIFIED.)
GEOMETRIC_REPRESENTATION_ITEM()
RATIONAL_B_SPLINE_SURFACE(((0.987633126750593,0.986929835989061,0.989150325841658),
(0.987633126750593,0.986929835989061,0.989150325841658)))
REPRESENTATION_ITEM('')
SURFACE()
);
#1298=(
BOUNDED_SURFACE()
B_SPLINE_SURFACE(1,2,((#115539,#115540,#115541,#115542,#115543),(#115544,
#115545,#115546,#115547,#115548)),.UNSPECIFIED.,.F.,.F.,.F.)
B_SPLINE_SURFACE_WITH_KNOTS((2,2),(3,2,3),(0.,0.289807040991555),(0.469846324360765,
0.470019760166366,0.487363340726489),.UNSPECIFIED.)
GEOMETRIC_REPRESENTATION_ITEM()
RATIONAL_B_SPLINE_SURFACE(((0.987787102172814,0.987787102172814,0.987787102172814,
0.988764511531023,0.992698258926487),(0.987787102172814,0.987787102172814,
0.987787102172814,0.988764511531023,0.992698258926487)))
REPRESENTATION_ITEM('')
SURFACE()
);
#1299=(
BOUNDED_SURFACE()
B_SPLINE_SURFACE(1,2,((#115550,#115551,#115552),(#115553,#115554,#115555)),
 .UNSPECIFIED.,.F.,.F.,.F.)
B_SPLINE_SURFACE_WITH_KNOTS((2,2),(3,3),(0.,0.289681084359923),(0.245851183393691,
0.263098999273798),.UNSPECIFIED.)
GEOMETRIC_REPRESENTATION_ITEM()
RATIONAL_B_SPLINE_SURFACE(((0.987633126750593,0.986929835989062,0.989150325841653),
(0.987633126750593,0.986929835989062,0.989150325841653)))
REPRESENTATION_ITEM('')
SURFACE()
);
#1300=(
BOUNDED_SURFACE()
B_SPLINE_SURFACE(1,2,((#115564,#115565,#115566,#115567,#115568),(#115569,
#115570,#115571,#115572,#115573)),.UNSPECIFIED.,.F.,.F.,.F.)
B_SPLINE_SURFACE_WITH_KNOTS((2,2),(3,2,3),(0.,0.289807040991561),(0.469846324360764,
0.470019760166365,0.487363340726489),.UNSPECIFIED.)
GEOMETRIC_REPRESENTATION_ITEM()
RATIONAL_B_SPLINE_SURFACE(((0.987787102172814,0.987787102172814,0.987787102172814,
0.988764511531024,0.992698258926487),(0.987787102172814,0.987787102172814,
0.987787102172814,0.988764511531024,0.992698258926487)))
REPRESENTATION_ITEM('')
SURFACE()
);
#1301=(
BOUNDED_SURFACE()
B_SPLINE_SURFACE(1,2,((#115575,#115576,#115577),(#115578,#115579,#115580)),
 .UNSPECIFIED.,.F.,.F.,.F.)
B_SPLINE_SURFACE_WITH_KNOTS((2,2),(3,3),(0.,0.289681084359918),(0.245851183393691,
0.263098999273798),.UNSPECIFIED.)
GEOMETRIC_REPRESENTATION_ITEM()
RATIONAL_B_SPLINE_SURFACE(((0.987633126750594,0.986929835989062,0.989150325841653),
(0.987633126750594,0.986929835989062,0.989150325841653)))
REPRESENTATION_ITEM('')
SURFACE()
);
#1302=(
BOUNDED_SURFACE()
B_SPLINE_SURFACE(1,2,((#115589,#115590,#115591,#115592,#115593),(#115594,
#115595,#115596,#115597,#115598)),.UNSPECIFIED.,.F.,.F.,.F.)
B_SPLINE_SURFACE_WITH_KNOTS((2,2),(3,2,3),(0.,0.290404426476257),(0.469422374491981,
0.470019760166365,0.487363340726489),.UNSPECIFIED.)
GEOMETRIC_REPRESENTATION_ITEM()
RATIONAL_B_SPLINE_SURFACE(((0.987787102172814,0.987787102172814,0.987787102172814,
0.988764511531023,0.992698258926487),(0.987787102172814,0.987787102172814,
0.987787102172814,0.988764511531023,0.992698258926487)))
REPRESENTATION_ITEM('')
SURFACE()
);
#1303=(
BOUNDED_SURFACE()
B_SPLINE_SURFACE(1,2,((#115600,#115601,#115602),(#115603,#115604,#115605)),
 .UNSPECIFIED.,.F.,.F.,.F.)
B_SPLINE_SURFACE_WITH_KNOTS((2,2),(3,3),(0.,0.289681084359921),(0.245851183393691,
0.263098999273798),.UNSPECIFIED.)
GEOMETRIC_REPRESENTATION_ITEM()
RATIONAL_B_SPLINE_SURFACE(((0.987633126750593,0.986929835989062,0.989150325841653),
(0.987633126750593,0.986929835989062,0.989150325841653)))
REPRESENTATION_ITEM('')
SURFACE()
);
#1304=(
BOUNDED_SURFACE()
B_SPLINE_SURFACE(1,2,((#115614,#115615,#115616,#115617,#115618),(#115619,
#115620,#115621,#115622,#115623)),.UNSPECIFIED.,.F.,.F.,.F.)
B_SPLINE_SURFACE_WITH_KNOTS((2,2),(3,2,3),(0.,0.290404426466868),(0.469422374491797,
0.470019760166365,0.487363340726489),.UNSPECIFIED.)
GEOMETRIC_REPRESENTATION_ITEM()
RATIONAL_B_SPLINE_SURFACE(((0.987787102172814,0.987787102172814,0.987787102172814,
0.988764511531023,0.992698258926487),(0.987787102172814,0.987787102172814,
0.987787102172814,0.988764511531023,0.992698258926487)))
REPRESENTATION_ITEM('')
SURFACE()
);
#1305=(
BOUNDED_SURFACE()
B_SPLINE_SURFACE(1,2,((#115625,#115626,#115627),(#115628,#115629,#115630)),
 .UNSPECIFIED.,.F.,.F.,.F.)
B_SPLINE_SURFACE_WITH_KNOTS((2,2),(3,3),(0.,0.289681084359923),(0.245851183393691,
0.263098999273798),.UNSPECIFIED.)
GEOMETRIC_REPRESENTATION_ITEM()
RATIONAL_B_SPLINE_SURFACE(((0.987633126750594,0.986929835989062,0.989150325841653),
(0.987633126750594,0.986929835989062,0.989150325841653)))
REPRESENTATION_ITEM('')
SURFACE()
);
#1306=(
BOUNDED_SURFACE()
B_SPLINE_SURFACE(1,2,((#115639,#115640,#115641,#115642,#115643),(#115644,
#115645,#115646,#115647,#115648)),.UNSPECIFIED.,.F.,.F.,.F.)
B_SPLINE_SURFACE_WITH_KNOTS((2,2),(3,2,3),(0.,0.290404426468995),(0.469422374490255,
0.470019760166365,0.487363340726489),.UNSPECIFIED.)
GEOMETRIC_REPRESENTATION_ITEM()
RATIONAL_B_SPLINE_SURFACE(((0.987787102172814,0.987787102172814,0.987787102172814,
0.988764511531023,0.992698258926487),(0.987787102172814,0.987787102172814,
0.987787102172814,0.988764511531023,0.992698258926487)))
REPRESENTATION_ITEM('')
SURFACE()
);
#1307=(
BOUNDED_SURFACE()
B_SPLINE_SURFACE(1,2,((#115650,#115651,#115652),(#115653,#115654,#115655)),
 .UNSPECIFIED.,.F.,.F.,.F.)
B_SPLINE_SURFACE_WITH_KNOTS((2,2),(3,3),(0.,0.289681084359914),(0.245851183393691,
0.263098999273798),.UNSPECIFIED.)
GEOMETRIC_REPRESENTATION_ITEM()
RATIONAL_B_SPLINE_SURFACE(((0.987633126750593,0.986929835989062,0.989150325841653),
(0.987633126750593,0.986929835989062,0.989150325841653)))
REPRESENTATION_ITEM('')
SURFACE()
);
#1308=(
BOUNDED_SURFACE()
B_SPLINE_SURFACE(1,2,((#115664,#115665,#115666,#115667,#115668),(#115669,
#115670,#115671,#115672,#115673)),.UNSPECIFIED.,.F.,.F.,.F.)
B_SPLINE_SURFACE_WITH_KNOTS((2,2),(3,2,3),(0.,0.290404426439913),(0.469422374518831,
0.470019760166367,0.487363340726489),.UNSPECIFIED.)
GEOMETRIC_REPRESENTATION_ITEM()
RATIONAL_B_SPLINE_SURFACE(((0.987787102172814,0.987787102172814,0.987787102172814,
0.988764511531024,0.992698258926487),(0.987787102172814,0.987787102172814,
0.987787102172814,0.988764511531024,0.992698258926487)))
REPRESENTATION_ITEM('')
SURFACE()
);
#1309=(
BOUNDED_SURFACE()
B_SPLINE_SURFACE(1,2,((#115675,#115676,#115677),(#115678,#115679,#115680)),
 .UNSPECIFIED.,.F.,.F.,.F.)
B_SPLINE_SURFACE_WITH_KNOTS((2,2),(3,3),(0.,0.289681084359922),(0.24585118339369,
0.263098999273797),.UNSPECIFIED.)
GEOMETRIC_REPRESENTATION_ITEM()
RATIONAL_B_SPLINE_SURFACE(((0.987633126750593,0.986929835989062,0.989150325841653),
(0.987633126750593,0.986929835989062,0.989150325841653)))
REPRESENTATION_ITEM('')
SURFACE()
);
#1310=(
BOUNDED_SURFACE()
B_SPLINE_SURFACE(1,2,((#115689,#115690,#115691,#115692,#115693),(#115694,
#115695,#115696,#115697,#115698)),.UNSPECIFIED.,.F.,.F.,.F.)
B_SPLINE_SURFACE_WITH_KNOTS((2,2),(3,2,3),(0.,0.289807040991635),(0.469846324360766,
0.470019760166367,0.48736334072649),.UNSPECIFIED.)
GEOMETRIC_REPRESENTATION_ITEM()
RATIONAL_B_SPLINE_SURFACE(((0.987787102172814,0.987787102172814,0.987787102172814,
0.988764511531024,0.992698258926488),(0.987787102172814,0.987787102172814,
0.987787102172814,0.988764511531024,0.992698258926488)))
REPRESENTATION_ITEM('')
SURFACE()
);
#1311=(
BOUNDED_SURFACE()
B_SPLINE_SURFACE(1,2,((#115700,#115701,#115702),(#115703,#115704,#115705)),
 .UNSPECIFIED.,.F.,.F.,.F.)
B_SPLINE_SURFACE_WITH_KNOTS((2,2),(3,3),(0.,0.289681084359916),(0.24585118339369,
0.263098999273797),.UNSPECIFIED.)
GEOMETRIC_REPRESENTATION_ITEM()
RATIONAL_B_SPLINE_SURFACE(((0.987633126750594,0.986929835989062,0.989150325841653),
(0.987633126750594,0.986929835989062,0.989150325841653)))
REPRESENTATION_ITEM('')
SURFACE()
);
#1312=(
BOUNDED_SURFACE()
B_SPLINE_SURFACE(1,2,((#115714,#115715,#115716,#115717,#115718),(#115719,
#115720,#115721,#115722,#115723)),.UNSPECIFIED.,.F.,.F.,.F.)
B_SPLINE_SURFACE_WITH_KNOTS((2,2),(3,2,3),(0.,0.289807040992233),(0.469846324360766,
0.470019760166367,0.48736334072649),.UNSPECIFIED.)
GEOMETRIC_REPRESENTATION_ITEM()
RATIONAL_B_SPLINE_SURFACE(((0.987787102172814,0.987787102172814,0.987787102172814,
0.988764511531024,0.992698258926488),(0.987787102172814,0.987787102172814,
0.987787102172814,0.988764511531024,0.992698258926488)))
REPRESENTATION_ITEM('')
SURFACE()
);
#1313=(
BOUNDED_SURFACE()
B_SPLINE_SURFACE(1,2,((#115725,#115726,#115727),(#115728,#115729,#115730)),
 .UNSPECIFIED.,.F.,.F.,.F.)
B_SPLINE_SURFACE_WITH_KNOTS((2,2),(3,3),(0.,0.289681084359921),(0.24585118339369,
0.263098999273797),.UNSPECIFIED.)
GEOMETRIC_REPRESENTATION_ITEM()
RATIONAL_B_SPLINE_SURFACE(((0.987633126750594,0.986929835989062,0.989150325841653),
(0.987633126750594,0.986929835989062,0.989150325841653)))
REPRESENTATION_ITEM('')
SURFACE()
);
#1314=(
BOUNDED_SURFACE()
B_SPLINE_SURFACE(1,2,((#115739,#115740,#115741,#115742,#115743),(#115744,
#115745,#115746,#115747,#115748)),.UNSPECIFIED.,.F.,.F.,.F.)
B_SPLINE_SURFACE_WITH_KNOTS((2,2),(3,2,3),(0.,0.289807040991645),(0.469846324360766,
0.470019760166367,0.48736334072649),.UNSPECIFIED.)
GEOMETRIC_REPRESENTATION_ITEM()
RATIONAL_B_SPLINE_SURFACE(((0.987787102172814,0.987787102172814,0.987787102172814,
0.988764511531024,0.992698258926488),(0.987787102172814,0.987787102172814,
0.987787102172814,0.988764511531024,0.992698258926488)))
REPRESENTATION_ITEM('')
SURFACE()
);
#1315=(
BOUNDED_SURFACE()
B_SPLINE_SURFACE(1,2,((#115750,#115751,#115752),(#115753,#115754,#115755)),
 .UNSPECIFIED.,.F.,.F.,.F.)
B_SPLINE_SURFACE_WITH_KNOTS((2,2),(3,3),(0.,0.28968108435992),(0.24585118339369,
0.263098999273797),.UNSPECIFIED.)
GEOMETRIC_REPRESENTATION_ITEM()
RATIONAL_B_SPLINE_SURFACE(((0.987633126750594,0.986929835989062,0.989150325841653),
(0.987633126750594,0.986929835989062,0.989150325841653)))
REPRESENTATION_ITEM('')
SURFACE()
);
#1316=(
BOUNDED_SURFACE()
B_SPLINE_SURFACE(1,2,((#115764,#115765,#115766,#115767,#115768),(#115769,
#115770,#115771,#115772,#115773)),.UNSPECIFIED.,.F.,.F.,.F.)
B_SPLINE_SURFACE_WITH_KNOTS((2,2),(3,2,3),(0.,0.289807040992142),(0.469846324360766,
0.470019760166367,0.48736334072649),.UNSPECIFIED.)
GEOMETRIC_REPRESENTATION_ITEM()
RATIONAL_B_SPLINE_SURFACE(((0.987787102172814,0.987787102172814,0.987787102172814,
0.988764511531024,0.992698258926488),(0.987787102172814,0.987787102172814,
0.987787102172814,0.988764511531024,0.992698258926488)))
REPRESENTATION_ITEM('')
SURFACE()
);
#1317=(
BOUNDED_SURFACE()
B_SPLINE_SURFACE(1,2,((#115775,#115776,#115777),(#115778,#115779,#115780)),
 .UNSPECIFIED.,.F.,.F.,.F.)
B_SPLINE_SURFACE_WITH_KNOTS((2,2),(3,3),(0.,0.28968108435992),(0.24585118339369,
0.263098999273797),.UNSPECIFIED.)
GEOMETRIC_REPRESENTATION_ITEM()
RATIONAL_B_SPLINE_SURFACE(((0.987633126750594,0.986929835989062,0.989150325841653),
(0.987633126750594,0.986929835989062,0.989150325841653)))
REPRESENTATION_ITEM('')
SURFACE()
);
#1318=(
BOUNDED_SURFACE()
B_SPLINE_SURFACE(1,2,((#115789,#115790,#115791,#115792,#115793),(#115794,
#115795,#115796,#115797,#115798)),.UNSPECIFIED.,.F.,.F.,.F.)
B_SPLINE_SURFACE_WITH_KNOTS((2,2),(3,2,3),(0.,0.290404426498244),(0.469422374469413,
0.470019760166367,0.48736334072649),.UNSPECIFIED.)
GEOMETRIC_REPRESENTATION_ITEM()
RATIONAL_B_SPLINE_SURFACE(((0.987787102172814,0.987787102172814,0.987787102172814,
0.988764511531024,0.992698258926488),(0.987787102172814,0.987787102172814,
0.987787102172814,0.988764511531024,0.992698258926488)))
REPRESENTATION_ITEM('')
SURFACE()
);
#1319=(
BOUNDED_SURFACE()
B_SPLINE_SURFACE(1,2,((#115800,#115801,#115802),(#115803,#115804,#115805)),
 .UNSPECIFIED.,.F.,.F.,.F.)
B_SPLINE_SURFACE_WITH_KNOTS((2,2),(3,3),(0.,0.289681084359923),(0.24585118339369,
0.263098999273797),.UNSPECIFIED.)
GEOMETRIC_REPRESENTATION_ITEM()
RATIONAL_B_SPLINE_SURFACE(((0.987633126750594,0.986929835989062,0.989150325841653),
(0.987633126750594,0.986929835989062,0.989150325841653)))
REPRESENTATION_ITEM('')
SURFACE()
);
#1320=(
BOUNDED_SURFACE()
B_SPLINE_SURFACE(1,2,((#115814,#115815,#115816,#115817,#115818),(#115819,
#115820,#115821,#115822,#115823)),.UNSPECIFIED.,.F.,.F.,.F.)
B_SPLINE_SURFACE_WITH_KNOTS((2,2),(3,2,3),(0.,0.290404426464598),(0.469422374503515,
0.470019760166367,0.48736334072649),.UNSPECIFIED.)
GEOMETRIC_REPRESENTATION_ITEM()
RATIONAL_B_SPLINE_SURFACE(((0.987787102172814,0.987787102172814,0.987787102172814,
0.988764511531024,0.992698258926488),(0.987787102172814,0.987787102172814,
0.987787102172814,0.988764511531024,0.992698258926488)))
REPRESENTATION_ITEM('')
SURFACE()
);
#1321=(
BOUNDED_SURFACE()
B_SPLINE_SURFACE(1,2,((#115825,#115826,#115827),(#115828,#115829,#115830)),
 .UNSPECIFIED.,.F.,.F.,.F.)
B_SPLINE_SURFACE_WITH_KNOTS((2,2),(3,3),(0.,0.289681084359922),(0.24585118339369,
0.263098999273797),.UNSPECIFIED.)
GEOMETRIC_REPRESENTATION_ITEM()
RATIONAL_B_SPLINE_SURFACE(((0.987633126750594,0.986929835989062,0.989150325841653),
(0.987633126750594,0.986929835989062,0.989150325841653)))
REPRESENTATION_ITEM('')
SURFACE()
);
#1322=(
BOUNDED_SURFACE()
B_SPLINE_SURFACE(1,2,((#115839,#115840,#115841,#115842,#115843),(#115844,
#115845,#115846,#115847,#115848)),.UNSPECIFIED.,.F.,.F.,.F.)
B_SPLINE_SURFACE_WITH_KNOTS((2,2),(3,2,3),(0.,0.290404426443499),(0.469422374515526,
0.470019760166367,0.48736334072649),.UNSPECIFIED.)
GEOMETRIC_REPRESENTATION_ITEM()
RATIONAL_B_SPLINE_SURFACE(((0.987787102172814,0.987787102172814,0.987787102172814,
0.988764511531024,0.992698258926488),(0.987787102172814,0.987787102172814,
0.987787102172814,0.988764511531024,0.992698258926488)))
REPRESENTATION_ITEM('')
SURFACE()
);
#1323=(
BOUNDED_SURFACE()
B_SPLINE_SURFACE(1,2,((#115850,#115851,#115852),(#115853,#115854,#115855)),
 .UNSPECIFIED.,.F.,.F.,.F.)
B_SPLINE_SURFACE_WITH_KNOTS((2,2),(3,3),(0.,0.289681084359924),(0.24585118339369,
0.263098999273797),.UNSPECIFIED.)
GEOMETRIC_REPRESENTATION_ITEM()
RATIONAL_B_SPLINE_SURFACE(((0.987633126750593,0.986929835989062,0.989150325841653),
(0.987633126750593,0.986929835989062,0.989150325841653)))
REPRESENTATION_ITEM('')
SURFACE()
);
#1324=(
BOUNDED_SURFACE()
B_SPLINE_SURFACE(1,2,((#115864,#115865,#115866,#115867,#115868),(#115869,
#115870,#115871,#115872,#115873)),.UNSPECIFIED.,.F.,.F.,.F.)
B_SPLINE_SURFACE_WITH_KNOTS((2,2),(3,2,3),(0.,0.289807040992967),(0.469846324360766,
0.470019760166367,0.48736334072649),.UNSPECIFIED.)
GEOMETRIC_REPRESENTATION_ITEM()
RATIONAL_B_SPLINE_SURFACE(((0.987787102172814,0.987787102172814,0.987787102172814,
0.988764511531024,0.992698258926488),(0.987787102172814,0.987787102172814,
0.987787102172814,0.988764511531024,0.992698258926488)))
REPRESENTATION_ITEM('')
SURFACE()
);
#1325=(
BOUNDED_SURFACE()
B_SPLINE_SURFACE(1,2,((#115875,#115876,#115877),(#115878,#115879,#115880)),
 .UNSPECIFIED.,.F.,.F.,.F.)
B_SPLINE_SURFACE_WITH_KNOTS((2,2),(3,3),(0.,0.289681084359922),(0.24585118339369,
0.263098999273797),.UNSPECIFIED.)
GEOMETRIC_REPRESENTATION_ITEM()
RATIONAL_B_SPLINE_SURFACE(((0.987633126750594,0.986929835989062,0.989150325841653),
(0.987633126750594,0.986929835989062,0.989150325841653)))
REPRESENTATION_ITEM('')
SURFACE()
);
#1326=(
BOUNDED_SURFACE()
B_SPLINE_SURFACE(1,2,((#115889,#115890,#115891,#115892,#115893),(#115894,
#115895,#115896,#115897,#115898)),.UNSPECIFIED.,.F.,.F.,.F.)
B_SPLINE_SURFACE_WITH_KNOTS((2,2),(3,2,3),(0.,0.289807040991681),(0.469846324360766,
0.470019760166367,0.48736334072649),.UNSPECIFIED.)
GEOMETRIC_REPRESENTATION_ITEM()
RATIONAL_B_SPLINE_SURFACE(((0.987787102172814,0.987787102172814,0.987787102172814,
0.988764511531024,0.992698258926488),(0.987787102172814,0.987787102172814,
0.987787102172814,0.988764511531024,0.992698258926488)))
REPRESENTATION_ITEM('')
SURFACE()
);
#1327=(
BOUNDED_SURFACE()
B_SPLINE_SURFACE(1,2,((#115900,#115901,#115902),(#115903,#115904,#115905)),
 .UNSPECIFIED.,.F.,.F.,.F.)
B_SPLINE_SURFACE_WITH_KNOTS((2,2),(3,3),(0.,0.289681084359928),(0.24585118339369,
0.263098999273797),.UNSPECIFIED.)
GEOMETRIC_REPRESENTATION_ITEM()
RATIONAL_B_SPLINE_SURFACE(((0.987633126750594,0.986929835989062,0.989150325841653),
(0.987633126750594,0.986929835989062,0.989150325841653)))
REPRESENTATION_ITEM('')
SURFACE()
);
#1328=(
BOUNDED_SURFACE()
B_SPLINE_SURFACE(1,2,((#115914,#115915,#115916,#115917,#115918),(#115919,
#115920,#115921,#115922,#115923)),.UNSPECIFIED.,.F.,.F.,.F.)
B_SPLINE_SURFACE_WITH_KNOTS((2,2),(3,2,3),(0.,0.289807040991564),(0.469846324360766,
0.470019760166367,0.48736334072649),.UNSPECIFIED.)
GEOMETRIC_REPRESENTATION_ITEM()
RATIONAL_B_SPLINE_SURFACE(((0.987787102172814,0.987787102172814,0.987787102172814,
0.988764511531024,0.992698258926488),(0.987787102172814,0.987787102172814,
0.987787102172814,0.988764511531024,0.992698258926488)))
REPRESENTATION_ITEM('')
SURFACE()
);
#1329=(
BOUNDED_SURFACE()
B_SPLINE_SURFACE(1,2,((#115925,#115926,#115927),(#115928,#115929,#115930)),
 .UNSPECIFIED.,.F.,.F.,.F.)
B_SPLINE_SURFACE_WITH_KNOTS((2,2),(3,3),(0.,0.289681084359921),(0.24585118339369,
0.263098999273796),.UNSPECIFIED.)
GEOMETRIC_REPRESENTATION_ITEM()
RATIONAL_B_SPLINE_SURFACE(((0.987633126750594,0.986929835989062,0.989150325841653),
(0.987633126750594,0.986929835989062,0.989150325841653)))
REPRESENTATION_ITEM('')
SURFACE()
);
#1330=(
BOUNDED_SURFACE()
B_SPLINE_SURFACE(1,2,((#115939,#115940,#115941,#115942,#115943),(#115944,
#115945,#115946,#115947,#115948)),.UNSPECIFIED.,.F.,.F.,.F.)
B_SPLINE_SURFACE_WITH_KNOTS((2,2),(3,2,3),(0.,0.289807040992195),(0.469846324360765,
0.470019760166366,0.48736334072649),.UNSPECIFIED.)
GEOMETRIC_REPRESENTATION_ITEM()
RATIONAL_B_SPLINE_SURFACE(((0.987787102172814,0.987787102172814,0.987787102172814,
0.988764511531024,0.992698258926488),(0.987787102172814,0.987787102172814,
0.987787102172814,0.988764511531024,0.992698258926488)))
REPRESENTATION_ITEM('')
SURFACE()
);
#1331=(
BOUNDED_SURFACE()
B_SPLINE_SURFACE(1,2,((#115950,#115951,#115952),(#115953,#115954,#115955)),
 .UNSPECIFIED.,.F.,.F.,.F.)
B_SPLINE_SURFACE_WITH_KNOTS((2,2),(3,3),(0.,0.289681084359926),(0.24585118339369,
0.263098999273796),.UNSPECIFIED.)
GEOMETRIC_REPRESENTATION_ITEM()
RATIONAL_B_SPLINE_SURFACE(((0.987633126750594,0.986929835989062,0.989150325841653),
(0.987633126750594,0.986929835989062,0.989150325841653)))
REPRESENTATION_ITEM('')
SURFACE()
);
#1332=(
BOUNDED_SURFACE()
B_SPLINE_SURFACE(1,2,((#115964,#115965,#115966,#115967,#115968),(#115969,
#115970,#115971,#115972,#115973)),.UNSPECIFIED.,.F.,.F.,.F.)
B_SPLINE_SURFACE_WITH_KNOTS((2,2),(3,2,3),(0.,0.290404426475224),(0.469422374492427,
0.470019760166367,0.48736334072649),.UNSPECIFIED.)
GEOMETRIC_REPRESENTATION_ITEM()
RATIONAL_B_SPLINE_SURFACE(((0.987787102172814,0.987787102172814,0.987787102172814,
0.988764511531024,0.992698258926488),(0.987787102172814,0.987787102172814,
0.987787102172814,0.988764511531024,0.992698258926488)))
REPRESENTATION_ITEM('')
SURFACE()
);
#1333=(
BOUNDED_SURFACE()
B_SPLINE_SURFACE(1,2,((#115975,#115976,#115977),(#115978,#115979,#115980)),
 .UNSPECIFIED.,.F.,.F.,.F.)
B_SPLINE_SURFACE_WITH_KNOTS((2,2),(3,3),(0.,0.289681084359927),(0.24585118339369,
0.263098999273796),.UNSPECIFIED.)
GEOMETRIC_REPRESENTATION_ITEM()
RATIONAL_B_SPLINE_SURFACE(((0.987633126750594,0.986929835989062,0.989150325841653),
(0.987633126750594,0.986929835989062,0.989150325841653)))
REPRESENTATION_ITEM('')
SURFACE()
);
#1334=(
BOUNDED_SURFACE()
B_SPLINE_SURFACE(1,2,((#115989,#115990,#115991,#115992,#115993),(#115994,
#115995,#115996,#115997,#115998)),.UNSPECIFIED.,.F.,.F.,.F.)
B_SPLINE_SURFACE_WITH_KNOTS((2,2),(3,2,3),(0.,0.290404426435714),(0.469422374524091,
0.470019760166367,0.48736334072649),.UNSPECIFIED.)
GEOMETRIC_REPRESENTATION_ITEM()
RATIONAL_B_SPLINE_SURFACE(((0.987787102172814,0.987787102172814,0.987787102172814,
0.988764511531024,0.992698258926488),(0.987787102172814,0.987787102172814,
0.987787102172814,0.988764511531024,0.992698258926488)))
REPRESENTATION_ITEM('')
SURFACE()
);
#1335=(
BOUNDED_SURFACE()
B_SPLINE_SURFACE(1,2,((#116000,#116001,#116002),(#116003,#116004,#116005)),
 .UNSPECIFIED.,.F.,.F.,.F.)
B_SPLINE_SURFACE_WITH_KNOTS((2,2),(3,3),(0.,0.289681084359928),(0.24585118339369,
0.263098999273796),.UNSPECIFIED.)
GEOMETRIC_REPRESENTATION_ITEM()
RATIONAL_B_SPLINE_SURFACE(((0.987633126750594,0.986929835989062,0.989150325841653),
(0.987633126750594,0.986929835989062,0.989150325841653)))
REPRESENTATION_ITEM('')
SURFACE()
);
#1336=(
BOUNDED_SURFACE()
B_SPLINE_SURFACE(1,2,((#116014,#116015,#116016,#116017,#116018),(#116019,
#116020,#116021,#116022,#116023)),.UNSPECIFIED.,.F.,.F.,.F.)
B_SPLINE_SURFACE_WITH_KNOTS((2,2),(3,2,3),(0.,0.290404426476923),(0.469422374491519,
0.470019760166367,0.48736334072649),.UNSPECIFIED.)
GEOMETRIC_REPRESENTATION_ITEM()
RATIONAL_B_SPLINE_SURFACE(((0.987787102172814,0.987787102172814,0.987787102172814,
0.988764511531024,0.992698258926488),(0.987787102172814,0.987787102172814,
0.987787102172814,0.988764511531024,0.992698258926488)))
REPRESENTATION_ITEM('')
SURFACE()
);
#1337=(
BOUNDED_SURFACE()
B_SPLINE_SURFACE(1,2,((#116025,#116026,#116027),(#116028,#116029,#116030)),
 .UNSPECIFIED.,.F.,.F.,.F.)
B_SPLINE_SURFACE_WITH_KNOTS((2,2),(3,3),(0.,0.289681084359926),(0.24585118339369,
0.263098999273796),.UNSPECIFIED.)
GEOMETRIC_REPRESENTATION_ITEM()
RATIONAL_B_SPLINE_SURFACE(((0.987633126750594,0.986929835989062,0.989150325841653),
(0.987633126750594,0.986929835989062,0.989150325841653)))
REPRESENTATION_ITEM('')
SURFACE()
);
#1338=(
BOUNDED_SURFACE()
B_SPLINE_SURFACE(1,2,((#116039,#116040,#116041,#116042,#116043),(#116044,
#116045,#116046,#116047,#116048)),.UNSPECIFIED.,.F.,.F.,.F.)
B_SPLINE_SURFACE_WITH_KNOTS((2,2),(3,2,3),(0.,0.290404426447106),(0.469422374522161,
0.470019760166367,0.48736334072649),.UNSPECIFIED.)
GEOMETRIC_REPRESENTATION_ITEM()
RATIONAL_B_SPLINE_SURFACE(((0.987787102172814,0.987787102172814,0.987787102172814,
0.988764511531024,0.992698258926488),(0.987787102172814,0.987787102172814,
0.987787102172814,0.988764511531024,0.992698258926488)))
REPRESENTATION_ITEM('')
SURFACE()
);
#1339=(
BOUNDED_SURFACE()
B_SPLINE_SURFACE(1,2,((#116050,#116051,#116052),(#116053,#116054,#116055)),
 .UNSPECIFIED.,.F.,.F.,.F.)
B_SPLINE_SURFACE_WITH_KNOTS((2,2),(3,3),(0.,0.28968108435992),(0.24585118339369,
0.263098999273796),.UNSPECIFIED.)
GEOMETRIC_REPRESENTATION_ITEM()
RATIONAL_B_SPLINE_SURFACE(((0.987633126750594,0.986929835989062,0.989150325841653),
(0.987633126750594,0.986929835989062,0.989150325841653)))
REPRESENTATION_ITEM('')
SURFACE()
);
#1340=(
BOUNDED_SURFACE()
B_SPLINE_SURFACE(1,2,((#116064,#116065,#116066,#116067,#116068),(#116069,
#116070,#116071,#116072,#116073)),.UNSPECIFIED.,.F.,.F.,.F.)
B_SPLINE_SURFACE_WITH_KNOTS((2,2),(3,2,3),(0.,0.28980704099176),(0.469846324360766,
0.470019760166367,0.48736334072649),.UNSPECIFIED.)
GEOMETRIC_REPRESENTATION_ITEM()
RATIONAL_B_SPLINE_SURFACE(((0.987787102172814,0.987787102172814,0.987787102172814,
0.988764511531024,0.992698258926488),(0.987787102172814,0.987787102172814,
0.987787102172814,0.988764511531024,0.992698258926488)))
REPRESENTATION_ITEM('')
SURFACE()
);
#1341=(
BOUNDED_SURFACE()
B_SPLINE_SURFACE(1,2,((#116075,#116076,#116077),(#116078,#116079,#116080)),
 .UNSPECIFIED.,.F.,.F.,.F.)
B_SPLINE_SURFACE_WITH_KNOTS((2,2),(3,3),(0.,0.289681084359922),(0.24585118339369,
0.263098999273796),.UNSPECIFIED.)
GEOMETRIC_REPRESENTATION_ITEM()
RATIONAL_B_SPLINE_SURFACE(((0.987633126750594,0.986929835989062,0.989150325841653),
(0.987633126750594,0.986929835989062,0.989150325841653)))
REPRESENTATION_ITEM('')
SURFACE()
);
#1342=(
BOUNDED_SURFACE()
B_SPLINE_SURFACE(1,2,((#116089,#116090,#116091,#116092,#116093),(#116094,
#116095,#116096,#116097,#116098)),.UNSPECIFIED.,.F.,.F.,.F.)
B_SPLINE_SURFACE_WITH_KNOTS((2,2),(3,2,3),(0.,0.289807040993049),(0.469846324360766,
0.470019760166367,0.48736334072649),.UNSPECIFIED.)
GEOMETRIC_REPRESENTATION_ITEM()
RATIONAL_B_SPLINE_SURFACE(((0.987787102172814,0.987787102172814,0.987787102172814,
0.988764511531024,0.992698258926488),(0.987787102172814,0.987787102172814,
0.987787102172814,0.988764511531024,0.992698258926488)))
REPRESENTATION_ITEM('')
SURFACE()
);
#1343=(
BOUNDED_SURFACE()
B_SPLINE_SURFACE(1,2,((#116100,#116101,#116102),(#116103,#116104,#116105)),
 .UNSPECIFIED.,.F.,.F.,.F.)
B_SPLINE_SURFACE_WITH_KNOTS((2,2),(3,3),(0.,0.289681084359929),(0.24585118339369,
0.2630989992738),.UNSPECIFIED.)
GEOMETRIC_REPRESENTATION_ITEM()
RATIONAL_B_SPLINE_SURFACE(((0.987633126750594,0.986929835989062,0.989150325841654),
(0.987633126750594,0.986929835989062,0.989150325841654)))
REPRESENTATION_ITEM('')
SURFACE()
);
#1344=(
BOUNDED_SURFACE()
B_SPLINE_SURFACE(1,2,((#116114,#116115,#116116,#116117,#116118),(#116119,
#116120,#116121,#116122,#116123)),.UNSPECIFIED.,.F.,.F.,.F.)
B_SPLINE_SURFACE_WITH_KNOTS((2,2),(3,2,3),(0.,0.289807040992803),(0.469846324360765,
0.470019760166366,0.48736334072649),.UNSPECIFIED.)
GEOMETRIC_REPRESENTATION_ITEM()
RATIONAL_B_SPLINE_SURFACE(((0.987787102172814,0.987787102172814,0.987787102172814,
0.988764511531024,0.992698258926488),(0.987787102172814,0.987787102172814,
0.987787102172814,0.988764511531024,0.992698258926488)))
REPRESENTATION_ITEM('')
SURFACE()
);
#1345=(
BOUNDED_SURFACE()
B_SPLINE_SURFACE(1,2,((#116125,#116126,#116127),(#116128,#116129,#116130)),
 .UNSPECIFIED.,.F.,.F.,.F.)
B_SPLINE_SURFACE_WITH_KNOTS((2,2),(3,3),(0.,0.289681084359935),(0.24585118339369,
0.263098999273798),.UNSPECIFIED.)
GEOMETRIC_REPRESENTATION_ITEM()
RATIONAL_B_SPLINE_SURFACE(((0.987633126750594,0.986929835989062,0.989150325841653),
(0.987633126750594,0.986929835989062,0.989150325841653)))
REPRESENTATION_ITEM('')
SURFACE()
);
#1346=(
BOUNDED_SURFACE()
B_SPLINE_SURFACE(1,2,((#116139,#116140,#116141,#116142,#116143),(#116144,
#116145,#116146,#116147,#116148)),.UNSPECIFIED.,.F.,.F.,.F.)
B_SPLINE_SURFACE_WITH_KNOTS((2,2),(3,2,3),(0.,0.290404426453367),(0.469422374506297,
0.470019760166367,0.48736334072649),.UNSPECIFIED.)
GEOMETRIC_REPRESENTATION_ITEM()
RATIONAL_B_SPLINE_SURFACE(((0.987787102172814,0.987787102172814,0.987787102172814,
0.988764511531024,0.992698258926488),(0.987787102172814,0.987787102172814,
0.987787102172814,0.988764511531024,0.992698258926488)))
REPRESENTATION_ITEM('')
SURFACE()
);
#1347=(
BOUNDED_SURFACE()
B_SPLINE_SURFACE(1,2,((#116150,#116151,#116152),(#116153,#116154,#116155)),
 .UNSPECIFIED.,.F.,.F.,.F.)
B_SPLINE_SURFACE_WITH_KNOTS((2,2),(3,3),(0.,0.289681084359929),(0.24585118339369,
0.263098999273796),.UNSPECIFIED.)
GEOMETRIC_REPRESENTATION_ITEM()
RATIONAL_B_SPLINE_SURFACE(((0.987633126750594,0.986929835989062,0.989150325841653),
(0.987633126750594,0.986929835989062,0.989150325841653)))
REPRESENTATION_ITEM('')
SURFACE()
);
#1348=(
BOUNDED_SURFACE()
B_SPLINE_SURFACE(1,2,((#116164,#116165,#116166,#116167,#116168),(#116169,
#116170,#116171,#116172,#116173)),.UNSPECIFIED.,.F.,.F.,.F.)
B_SPLINE_SURFACE_WITH_KNOTS((2,2),(3,2,3),(0.,0.290404426459532),(0.46942237450006,
0.470019760166366,0.48736334072649),.UNSPECIFIED.)
GEOMETRIC_REPRESENTATION_ITEM()
RATIONAL_B_SPLINE_SURFACE(((0.987787102172814,0.987787102172814,0.987787102172814,
0.988764511531024,0.992698258926488),(0.987787102172814,0.987787102172814,
0.987787102172814,0.988764511531024,0.992698258926488)))
REPRESENTATION_ITEM('')
SURFACE()
);
#1349=(
BOUNDED_SURFACE()
B_SPLINE_SURFACE(1,2,((#116175,#116176,#116177),(#116178,#116179,#116180)),
 .UNSPECIFIED.,.F.,.F.,.F.)
B_SPLINE_SURFACE_WITH_KNOTS((2,2),(3,3),(0.,0.289681084359924),(0.24585118339369,
0.263098999273796),.UNSPECIFIED.)
GEOMETRIC_REPRESENTATION_ITEM()
RATIONAL_B_SPLINE_SURFACE(((0.987633126750594,0.986929835989062,0.989150325841653),
(0.987633126750594,0.986929835989062,0.989150325841653)))
REPRESENTATION_ITEM('')
SURFACE()
);
#1350=(
BOUNDED_SURFACE()
B_SPLINE_SURFACE(1,2,((#116189,#116190,#116191,#116192,#116193),(#116194,
#116195,#116196,#116197,#116198)),.UNSPECIFIED.,.F.,.F.,.F.)
B_SPLINE_SURFACE_WITH_KNOTS((2,2),(3,2,3),(0.,0.290404426466932),(0.469422374492982,
0.470019760166367,0.487363340726492),.UNSPECIFIED.)
GEOMETRIC_REPRESENTATION_ITEM()
RATIONAL_B_SPLINE_SURFACE(((0.987787102172814,0.987787102172814,0.987787102172814,
0.988764511531024,0.992698258926488),(0.987787102172814,0.987787102172814,
0.987787102172814,0.988764511531024,0.992698258926488)))
REPRESENTATION_ITEM('')
SURFACE()
);
#1351=(
BOUNDED_SURFACE()
B_SPLINE_SURFACE(1,2,((#116200,#116201,#116202),(#116203,#116204,#116205)),
 .UNSPECIFIED.,.F.,.F.,.F.)
B_SPLINE_SURFACE_WITH_KNOTS((2,2),(3,3),(0.,0.289681084359922),(0.245851183393682,
0.263098999273796),.UNSPECIFIED.)
GEOMETRIC_REPRESENTATION_ITEM()
RATIONAL_B_SPLINE_SURFACE(((0.987633126750594,0.986929835989061,0.989150325841653),
(0.987633126750594,0.986929835989061,0.989150325841653)))
REPRESENTATION_ITEM('')
SURFACE()
);
#1352=(
BOUNDED_SURFACE()
B_SPLINE_SURFACE(1,2,((#116214,#116215,#116216,#116217,#116218),(#116219,
#116220,#116221,#116222,#116223)),.UNSPECIFIED.,.F.,.F.,.F.)
B_SPLINE_SURFACE_WITH_KNOTS((2,2),(3,2,3),(0.,0.290404426475473),(0.469422374493052,
0.470019760166366,0.48736334072649),.UNSPECIFIED.)
GEOMETRIC_REPRESENTATION_ITEM()
RATIONAL_B_SPLINE_SURFACE(((0.987787102172814,0.987787102172814,0.987787102172814,
0.988764511531024,0.992698258926488),(0.987787102172814,0.987787102172814,
0.987787102172814,0.988764511531024,0.992698258926488)))
REPRESENTATION_ITEM('')
SURFACE()
);
#1353=(
BOUNDED_SURFACE()
B_SPLINE_SURFACE(1,2,((#116225,#116226,#116227),(#116228,#116229,#116230)),
 .UNSPECIFIED.,.F.,.F.,.F.)
B_SPLINE_SURFACE_WITH_KNOTS((2,2),(3,3),(0.,0.289681084359924),(0.245851183393691,
0.263098999273796),.UNSPECIFIED.)
GEOMETRIC_REPRESENTATION_ITEM()
RATIONAL_B_SPLINE_SURFACE(((0.987633126750594,0.986929835989062,0.989150325841653),
(0.987633126750594,0.986929835989062,0.989150325841653)))
REPRESENTATION_ITEM('')
SURFACE()
);
#1354=(
BOUNDED_SURFACE()
B_SPLINE_SURFACE(1,2,((#116232,#116233,#116234,#116235,#116236),(#116237,
#116238,#116239,#116240,#116241)),.UNSPECIFIED.,.F.,.F.,.F.)
B_SPLINE_SURFACE_WITH_KNOTS((2,2),(3,2,3),(0.,0.289807040991971),(0.297684616398974,
0.297856505190613,0.315045384354509),.UNSPECIFIED.)
GEOMETRIC_REPRESENTATION_ITEM()
RATIONAL_B_SPLINE_SURFACE(((0.992924952273132,0.992924952273132,0.992924952273132,
0.98894276409569,0.98786440923939),(0.992924952273132,0.992924952273132,
0.992924952273132,0.98894276409569,0.98786440923939)))
REPRESENTATION_ITEM('')
SURFACE()
);
#1355=(
BOUNDED_SURFACE()
B_SPLINE_SURFACE(1,2,((#116264,#116265,#116266,#116267,#116268,#116269,
#116270),(#116271,#116272,#116273,#116274,#116275,#116276,#116277)),
 .UNSPECIFIED.,.F.,.F.,.F.)
B_SPLINE_SURFACE_WITH_KNOTS((2,2),(3,2,2,3),(0.,0.289681084359924),(0.418207303127979,
0.428571428571429,0.435775021682622,0.435950698868169),.UNSPECIFIED.)
GEOMETRIC_REPRESENTATION_ITEM()
RATIONAL_B_SPLINE_SURFACE(((0.993779895952495,0.996362096314125,1.,0.997471472332736,
0.995452950231063,0.995452950231063,0.995452950231063),(0.993779895952495,
0.996362096314125,1.,0.997471472332736,0.995452950231063,0.995452950231063,
0.995452950231063)))
REPRESENTATION_ITEM('')
SURFACE()
);
#1356=(
BOUNDED_SURFACE()
B_SPLINE_SURFACE(1,2,((#116279,#116280,#116281,#116282,#116283),(#116284,
#116285,#116286,#116287,#116288)),.UNSPECIFIED.,.F.,.F.,.F.)
B_SPLINE_SURFACE_WITH_KNOTS((2,2),(3,2,3),(0.,0.289807040991893),(0.297684616398974,
0.297856505190613,0.315045384354503),.UNSPECIFIED.)
GEOMETRIC_REPRESENTATION_ITEM()
RATIONAL_B_SPLINE_SURFACE(((0.992924952273132,0.992924952273132,0.992924952273132,
0.988942764095691,0.987864409239391),(0.992924952273132,0.992924952273132,
0.992924952273132,0.988942764095691,0.987864409239391)))
REPRESENTATION_ITEM('')
SURFACE()
);
#1357=(
BOUNDED_SURFACE()
B_SPLINE_SURFACE(1,2,((#116311,#116312,#116313,#116314,#116315,#116316,
#116317),(#116318,#116319,#116320,#116321,#116322,#116323,#116324)),
 .UNSPECIFIED.,.F.,.F.,.F.)
B_SPLINE_SURFACE_WITH_KNOTS((2,2),(3,2,2,3),(0.,0.289681084359928),(0.418207303127979,
0.428571428571429,0.435775021682622,0.435950698868169),.UNSPECIFIED.)
GEOMETRIC_REPRESENTATION_ITEM()
RATIONAL_B_SPLINE_SURFACE(((0.993779895952495,0.996362096314125,1.,0.997471472332736,
0.995452950231063,0.995452950231063,0.995452950231063),(0.993779895952495,
0.996362096314125,1.,0.997471472332736,0.995452950231063,0.995452950231063,
0.995452950231063)))
REPRESENTATION_ITEM('')
SURFACE()
);
#1358=(
BOUNDED_SURFACE()
B_SPLINE_SURFACE(1,2,((#116326,#116327,#116328,#116329,#116330),(#116331,
#116332,#116333,#116334,#116335)),.UNSPECIFIED.,.F.,.F.,.F.)
B_SPLINE_SURFACE_WITH_KNOTS((2,2),(3,2,3),(0.,0.289807040992008),(0.297684616398473,
0.297856505190117,0.315045384354506),.UNSPECIFIED.)
GEOMETRIC_REPRESENTATION_ITEM()
RATIONAL_B_SPLINE_SURFACE(((0.992924952273362,0.992924952273362,0.992924952273362,
0.988942764095722,0.98786440923939),(0.992924952273362,0.992924952273362,
0.992924952273362,0.988942764095722,0.98786440923939)))
REPRESENTATION_ITEM('')
SURFACE()
);
#1359=(
BOUNDED_SURFACE()
B_SPLINE_SURFACE(1,2,((#116358,#116359,#116360,#116361,#116362,#116363,
#116364),(#116365,#116366,#116367,#116368,#116369,#116370,#116371)),
 .UNSPECIFIED.,.F.,.F.,.F.)
B_SPLINE_SURFACE_WITH_KNOTS((2,2),(3,2,2,3),(0.,0.289681084359928),(0.418207303127979,
0.428571428571429,0.435775021682622,0.435950698868169),.UNSPECIFIED.)
GEOMETRIC_REPRESENTATION_ITEM()
RATIONAL_B_SPLINE_SURFACE(((0.993779895952495,0.996362096314125,1.,0.997471472332736,
0.995452950231063,0.995452950231063,0.995452950231063),(0.993779895952495,
0.996362096314125,1.,0.997471472332736,0.995452950231063,0.995452950231063,
0.995452950231063)))
REPRESENTATION_ITEM('')
SURFACE()
);
#1360=(
BOUNDED_SURFACE()
B_SPLINE_SURFACE(1,2,((#116373,#116374,#116375,#116376,#116377),(#116378,
#116379,#116380,#116381,#116382)),.UNSPECIFIED.,.F.,.F.,.F.)
B_SPLINE_SURFACE_WITH_KNOTS((2,2),(3,2,3),(0.,0.289807040992683),(0.297684616398974,
0.297856505190613,0.315045384354503),.UNSPECIFIED.)
GEOMETRIC_REPRESENTATION_ITEM()
RATIONAL_B_SPLINE_SURFACE(((0.992924952273132,0.992924952273132,0.992924952273132,
0.988942764095691,0.98786440923939),(0.992924952273132,0.992924952273132,
0.992924952273132,0.988942764095691,0.98786440923939)))
REPRESENTATION_ITEM('')
SURFACE()
);
#1361=(
BOUNDED_SURFACE()
B_SPLINE_SURFACE(1,2,((#116405,#116406,#116407,#116408,#116409,#116410,
#116411),(#116412,#116413,#116414,#116415,#116416,#116417,#116418)),
 .UNSPECIFIED.,.F.,.F.,.F.)
B_SPLINE_SURFACE_WITH_KNOTS((2,2),(3,2,2,3),(0.,0.289681084360555),(0.418207303127979,
0.428571428571429,0.435775021682622,0.435950698868169),.UNSPECIFIED.)
GEOMETRIC_REPRESENTATION_ITEM()
RATIONAL_B_SPLINE_SURFACE(((0.993779895952495,0.996362096314125,1.,0.997471472332736,
0.995452950231063,0.995452950231063,0.995452950231063),(0.993779895952495,
0.996362096314125,1.,0.997471472332736,0.995452950231063,0.995452950231063,
0.995452950231063)))
REPRESENTATION_ITEM('')
SURFACE()
);
#1362=(
BOUNDED_SURFACE()
B_SPLINE_SURFACE(1,2,((#116420,#116421,#116422,#116423,#116424),(#116425,
#116426,#116427,#116428,#116429)),.UNSPECIFIED.,.F.,.F.,.F.)
B_SPLINE_SURFACE_WITH_KNOTS((2,2),(3,2,3),(0.,0.289807040992536),(0.297684616398974,
0.297856505190613,0.31504538435453),.UNSPECIFIED.)
GEOMETRIC_REPRESENTATION_ITEM()
RATIONAL_B_SPLINE_SURFACE(((0.992924952273132,0.992924952273132,0.992924952273132,
0.988942764095685,0.987864409239387),(0.992924952273132,0.992924952273132,
0.992924952273132,0.988942764095685,0.987864409239387)))
REPRESENTATION_ITEM('')
SURFACE()
);
#1363=(
BOUNDED_SURFACE()
B_SPLINE_SURFACE(1,2,((#116452,#116453,#116454,#116455,#116456,#116457,
#116458),(#116459,#116460,#116461,#116462,#116463,#116464,#116465)),
 .UNSPECIFIED.,.F.,.F.,.F.)
B_SPLINE_SURFACE_WITH_KNOTS((2,2),(3,2,2,3),(0.,0.289681084360345),(0.41820730312798,
0.428571428571429,0.435775021682622,0.435950698868169),.UNSPECIFIED.)
GEOMETRIC_REPRESENTATION_ITEM()
RATIONAL_B_SPLINE_SURFACE(((0.993779895952495,0.996362096314126,1.,0.997471472332736,
0.995452950231063,0.995452950231063,0.995452950231063),(0.993779895952495,
0.996362096314126,1.,0.997471472332736,0.995452950231063,0.995452950231063,
0.995452950231063)))
REPRESENTATION_ITEM('')
SURFACE()
);
#1364=(
BOUNDED_SURFACE()
B_SPLINE_SURFACE(1,2,((#116467,#116468,#116469,#116470,#116471),(#116472,
#116473,#116474,#116475,#116476)),.UNSPECIFIED.,.F.,.F.,.F.)
B_SPLINE_SURFACE_WITH_KNOTS((2,2),(3,2,3),(0.,0.289807040992501),(0.297684616398974,
0.297856505190613,0.315045384354503),.UNSPECIFIED.)
GEOMETRIC_REPRESENTATION_ITEM()
RATIONAL_B_SPLINE_SURFACE(((0.992924952273132,0.992924952273132,0.992924952273132,
0.988942764095691,0.98786440923939),(0.992924952273132,0.992924952273132,
0.992924952273132,0.988942764095691,0.987864409239391)))
REPRESENTATION_ITEM('')
SURFACE()
);
#1365=(
BOUNDED_SURFACE()
B_SPLINE_SURFACE(1,2,((#116499,#116500,#116501,#116502,#116503,#116504,
#116505),(#116506,#116507,#116508,#116509,#116510,#116511,#116512)),
 .UNSPECIFIED.,.F.,.F.,.F.)
B_SPLINE_SURFACE_WITH_KNOTS((2,2),(3,2,2,3),(0.,0.289681084359914),(0.418207303127979,
0.428571428571429,0.435775021682622,0.435950698868169),.UNSPECIFIED.)
GEOMETRIC_REPRESENTATION_ITEM()
RATIONAL_B_SPLINE_SURFACE(((0.993779895952495,0.996362096314125,1.,0.997471472332736,
0.995452950231063,0.995452950231063,0.995452950231063),(0.993779895952495,
0.996362096314125,1.,0.997471472332736,0.995452950231063,0.995452950231063,
0.995452950231063)))
REPRESENTATION_ITEM('')
SURFACE()
);
#1366=(
BOUNDED_SURFACE()
B_SPLINE_SURFACE(1,2,((#116514,#116515,#116516,#116517,#116518),(#116519,
#116520,#116521,#116522,#116523)),.UNSPECIFIED.,.F.,.F.,.F.)
B_SPLINE_SURFACE_WITH_KNOTS((2,2),(3,2,3),(0.,0.289807040992673),(0.297684616398974,
0.297856505190613,0.315045384354503),.UNSPECIFIED.)
GEOMETRIC_REPRESENTATION_ITEM()
RATIONAL_B_SPLINE_SURFACE(((0.992924952273132,0.992924952273132,0.992924952273132,
0.988942764095691,0.98786440923939),(0.992924952273132,0.992924952273132,
0.992924952273132,0.988942764095691,0.98786440923939)))
REPRESENTATION_ITEM('')
SURFACE()
);
#1367=(
BOUNDED_SURFACE()
B_SPLINE_SURFACE(1,2,((#116546,#116547,#116548,#116549,#116550,#116551,
#116552),(#116553,#116554,#116555,#116556,#116557,#116558,#116559)),
 .UNSPECIFIED.,.F.,.F.,.F.)
B_SPLINE_SURFACE_WITH_KNOTS((2,2),(3,2,2,3),(0.,0.28968108435992),(0.418207303127979,
0.428571428571429,0.435775021682622,0.435950698868169),.UNSPECIFIED.)
GEOMETRIC_REPRESENTATION_ITEM()
RATIONAL_B_SPLINE_SURFACE(((0.993779895952495,0.996362096314125,1.,0.997471472332736,
0.995452950231063,0.995452950231063,0.995452950231063),(0.993779895952495,
0.996362096314125,1.,0.997471472332736,0.995452950231063,0.995452950231063,
0.995452950231063)))
REPRESENTATION_ITEM('')
SURFACE()
);
#1368=(
BOUNDED_SURFACE()
B_SPLINE_SURFACE(1,2,((#116561,#116562,#116563,#116564,#116565),(#116566,
#116567,#116568,#116569,#116570)),.UNSPECIFIED.,.F.,.F.,.F.)
B_SPLINE_SURFACE_WITH_KNOTS((2,2),(3,2,3),(0.,0.289807040991738),(0.297684616398974,
0.297856505190613,0.315045384354503),.UNSPECIFIED.)
GEOMETRIC_REPRESENTATION_ITEM()
RATIONAL_B_SPLINE_SURFACE(((0.992924952273132,0.992924952273132,0.992924952273132,
0.988942764095691,0.98786440923939),(0.992924952273132,0.992924952273132,
0.992924952273132,0.988942764095691,0.98786440923939)))
REPRESENTATION_ITEM('')
SURFACE()
);
#1369=(
BOUNDED_SURFACE()
B_SPLINE_SURFACE(1,2,((#116593,#116594,#116595,#116596,#116597,#116598,
#116599),(#116600,#116601,#116602,#116603,#116604,#116605,#116606)),
 .UNSPECIFIED.,.F.,.F.,.F.)
B_SPLINE_SURFACE_WITH_KNOTS((2,2),(3,2,2,3),(0.,0.289681084359925),(0.418207303127979,
0.428571428571429,0.435775021682622,0.435950698868169),.UNSPECIFIED.)
GEOMETRIC_REPRESENTATION_ITEM()
RATIONAL_B_SPLINE_SURFACE(((0.993779895952495,0.996362096314125,1.,0.997471472332736,
0.995452950231063,0.995452950231063,0.995452950231063),(0.993779895952495,
0.996362096314125,1.,0.997471472332736,0.995452950231063,0.995452950231063,
0.995452950231063)))
REPRESENTATION_ITEM('')
SURFACE()
);
#1370=(
BOUNDED_SURFACE()
B_SPLINE_SURFACE(1,2,((#116608,#116609,#116610,#116611,#116612),(#116613,
#116614,#116615,#116616,#116617)),.UNSPECIFIED.,.F.,.F.,.F.)
B_SPLINE_SURFACE_WITH_KNOTS((2,2),(3,2,3),(0.,0.289807040991744),(0.297684616398974,
0.297856505190613,0.315045384354503),.UNSPECIFIED.)
GEOMETRIC_REPRESENTATION_ITEM()
RATIONAL_B_SPLINE_SURFACE(((0.992924952273132,0.992924952273132,0.992924952273132,
0.988942764095691,0.98786440923939),(0.992924952273132,0.992924952273132,
0.992924952273132,0.988942764095691,0.98786440923939)))
REPRESENTATION_ITEM('')
SURFACE()
);
#1371=(
BOUNDED_SURFACE()
B_SPLINE_SURFACE(1,2,((#116640,#116641,#116642,#116643,#116644,#116645,
#116646),(#116647,#116648,#116649,#116650,#116651,#116652,#116653)),
 .UNSPECIFIED.,.F.,.F.,.F.)
B_SPLINE_SURFACE_WITH_KNOTS((2,2),(3,2,2,3),(0.,0.289681084359988),(0.418207303127979,
0.428571428571429,0.435775021682622,0.435950698868169),.UNSPECIFIED.)
GEOMETRIC_REPRESENTATION_ITEM()
RATIONAL_B_SPLINE_SURFACE(((0.993779895952495,0.996362096314125,1.,0.997471472332736,
0.995452950231063,0.995452950231063,0.995452950231063),(0.993779895952495,
0.996362096314125,1.,0.997471472332736,0.995452950231063,0.995452950231063,
0.995452950231063)))
REPRESENTATION_ITEM('')
SURFACE()
);
#1372=(
BOUNDED_SURFACE()
B_SPLINE_SURFACE(1,2,((#116655,#116656,#116657,#116658,#116659),(#116660,
#116661,#116662,#116663,#116664)),.UNSPECIFIED.,.F.,.F.,.F.)
B_SPLINE_SURFACE_WITH_KNOTS((2,2),(3,2,3),(0.,0.289807040991851),(0.297684616398974,
0.297856505190613,0.315045384354503),.UNSPECIFIED.)
GEOMETRIC_REPRESENTATION_ITEM()
RATIONAL_B_SPLINE_SURFACE(((0.992924952273132,0.992924952273132,0.992924952273132,
0.988942764095691,0.98786440923939),(0.992924952273132,0.992924952273132,
0.992924952273132,0.988942764095691,0.98786440923939)))
REPRESENTATION_ITEM('')
SURFACE()
);
#1373=(
BOUNDED_SURFACE()
B_SPLINE_SURFACE(1,2,((#116687,#116688,#116689,#116690,#116691,#116692,
#116693),(#116694,#116695,#116696,#116697,#116698,#116699,#116700)),
 .UNSPECIFIED.,.F.,.F.,.F.)
B_SPLINE_SURFACE_WITH_KNOTS((2,2),(3,2,2,3),(0.,0.289681084360646),(0.418207303127979,
0.428571428571429,0.435775021682622,0.435950698868169),.UNSPECIFIED.)
GEOMETRIC_REPRESENTATION_ITEM()
RATIONAL_B_SPLINE_SURFACE(((0.993779895952495,0.996362096314125,1.,0.997471472332736,
0.995452950231063,0.995452950231063,0.995452950231063),(0.993779895952495,
0.996362096314125,1.,0.997471472332736,0.995452950231063,0.995452950231063,
0.995452950231063)))
REPRESENTATION_ITEM('')
SURFACE()
);
#1374=(
BOUNDED_SURFACE()
B_SPLINE_SURFACE(1,2,((#116702,#116703,#116704,#116705,#116706),(#116707,
#116708,#116709,#116710,#116711)),.UNSPECIFIED.,.F.,.F.,.F.)
B_SPLINE_SURFACE_WITH_KNOTS((2,2),(3,2,3),(0.,0.289807040991787),(0.297684616398974,
0.297856505190613,0.315045384354503),.UNSPECIFIED.)
GEOMETRIC_REPRESENTATION_ITEM()
RATIONAL_B_SPLINE_SURFACE(((0.992924952273132,0.992924952273132,0.992924952273132,
0.988942764095691,0.98786440923939),(0.992924952273132,0.992924952273132,
0.992924952273132,0.988942764095691,0.98786440923939)))
REPRESENTATION_ITEM('')
SURFACE()
);
#1375=(
BOUNDED_SURFACE()
B_SPLINE_SURFACE(1,2,((#116734,#116735,#116736,#116737,#116738,#116739,
#116740),(#116741,#116742,#116743,#116744,#116745,#116746,#116747)),
 .UNSPECIFIED.,.F.,.F.,.F.)
B_SPLINE_SURFACE_WITH_KNOTS((2,2),(3,2,2,3),(0.,0.289681084359924),(0.418207303127979,
0.428571428571429,0.435775021682622,0.435950698868169),.UNSPECIFIED.)
GEOMETRIC_REPRESENTATION_ITEM()
RATIONAL_B_SPLINE_SURFACE(((0.993779895952495,0.996362096314125,1.,0.997471472332736,
0.995452950231063,0.995452950231063,0.995452950231063),(0.993779895952495,
0.996362096314125,1.,0.997471472332736,0.995452950231063,0.995452950231063,
0.995452950231063)))
REPRESENTATION_ITEM('')
SURFACE()
);
#1376=(
BOUNDED_SURFACE()
B_SPLINE_SURFACE(1,2,((#116749,#116750,#116751,#116752,#116753),(#116754,
#116755,#116756,#116757,#116758)),.UNSPECIFIED.,.F.,.F.,.F.)
B_SPLINE_SURFACE_WITH_KNOTS((2,2),(3,2,3),(0.,0.289807040991759),(0.297684616398974,
0.297856505190613,0.315045384354503),.UNSPECIFIED.)
GEOMETRIC_REPRESENTATION_ITEM()
RATIONAL_B_SPLINE_SURFACE(((0.992924952273132,0.992924952273132,0.992924952273132,
0.988942764095691,0.98786440923939),(0.992924952273132,0.992924952273132,
0.992924952273132,0.988942764095691,0.98786440923939)))
REPRESENTATION_ITEM('')
SURFACE()
);
#1377=(
BOUNDED_SURFACE()
B_SPLINE_SURFACE(1,2,((#116781,#116782,#116783,#116784,#116785,#116786,
#116787),(#116788,#116789,#116790,#116791,#116792,#116793,#116794)),
 .UNSPECIFIED.,.F.,.F.,.F.)
B_SPLINE_SURFACE_WITH_KNOTS((2,2),(3,2,2,3),(0.,0.289681084359918),(0.418207303127979,
0.428571428571429,0.435775021682622,0.435950698868169),.UNSPECIFIED.)
GEOMETRIC_REPRESENTATION_ITEM()
RATIONAL_B_SPLINE_SURFACE(((0.993779895952495,0.996362096314125,1.,0.997471472332736,
0.995452950231063,0.995452950231063,0.995452950231063),(0.993779895952495,
0.996362096314125,1.,0.997471472332736,0.995452950231063,0.995452950231063,
0.995452950231063)))
REPRESENTATION_ITEM('')
SURFACE()
);
#1378=(
BOUNDED_SURFACE()
B_SPLINE_SURFACE(1,2,((#116796,#116797,#116798,#116799,#116800),(#116801,
#116802,#116803,#116804,#116805)),.UNSPECIFIED.,.F.,.F.,.F.)
B_SPLINE_SURFACE_WITH_KNOTS((2,2),(3,2,3),(0.,0.289807040991714),(0.297684616398974,
0.297856505190613,0.315045384354503),.UNSPECIFIED.)
GEOMETRIC_REPRESENTATION_ITEM()
RATIONAL_B_SPLINE_SURFACE(((0.992924952273132,0.992924952273132,0.992924952273132,
0.988942764095691,0.98786440923939),(0.992924952273132,0.992924952273132,
0.992924952273132,0.988942764095691,0.98786440923939)))
REPRESENTATION_ITEM('')
SURFACE()
);
#1379=(
BOUNDED_SURFACE()
B_SPLINE_SURFACE(1,2,((#116828,#116829,#116830,#116831,#116832,#116833,
#116834),(#116835,#116836,#116837,#116838,#116839,#116840,#116841)),
 .UNSPECIFIED.,.F.,.F.,.F.)
B_SPLINE_SURFACE_WITH_KNOTS((2,2),(3,2,2,3),(0.,0.289681084359924),(0.418207303127979,
0.428571428571429,0.435775021682622,0.435950698868169),.UNSPECIFIED.)
GEOMETRIC_REPRESENTATION_ITEM()
RATIONAL_B_SPLINE_SURFACE(((0.993779895952495,0.996362096314125,1.,0.997471472332736,
0.995452950231063,0.995452950231063,0.995452950231063),(0.993779895952495,
0.996362096314125,1.,0.997471472332736,0.995452950231063,0.995452950231063,
0.995452950231063)))
REPRESENTATION_ITEM('')
SURFACE()
);
#1380=(
BOUNDED_SURFACE()
B_SPLINE_SURFACE(1,2,((#116843,#116844,#116845,#116846,#116847),(#116848,
#116849,#116850,#116851,#116852)),.UNSPECIFIED.,.F.,.F.,.F.)
B_SPLINE_SURFACE_WITH_KNOTS((2,2),(3,2,3),(0.,0.289807040991564),(0.297684616398974,
0.297856505190613,0.315045384354503),.UNSPECIFIED.)
GEOMETRIC_REPRESENTATION_ITEM()
RATIONAL_B_SPLINE_SURFACE(((0.992924952273132,0.992924952273132,0.992924952273132,
0.988942764095691,0.98786440923939),(0.992924952273132,0.992924952273132,
0.992924952273132,0.988942764095691,0.98786440923939)))
REPRESENTATION_ITEM('')
SURFACE()
);
#1381=(
BOUNDED_SURFACE()
B_SPLINE_SURFACE(1,2,((#116875,#116876,#116877,#116878,#116879,#116880,
#116881),(#116882,#116883,#116884,#116885,#116886,#116887,#116888)),
 .UNSPECIFIED.,.F.,.F.,.F.)
B_SPLINE_SURFACE_WITH_KNOTS((2,2),(3,2,2,3),(0.,0.289681084359924),(0.418207303127979,
0.428571428571429,0.435775021682622,0.435950698868169),.UNSPECIFIED.)
GEOMETRIC_REPRESENTATION_ITEM()
RATIONAL_B_SPLINE_SURFACE(((0.993779895952495,0.996362096314125,1.,0.997471472332736,
0.995452950231063,0.995452950231063,0.995452950231063),(0.993779895952495,
0.996362096314125,1.,0.997471472332736,0.995452950231063,0.995452950231063,
0.995452950231063)))
REPRESENTATION_ITEM('')
SURFACE()
);
#1382=(
BOUNDED_SURFACE()
B_SPLINE_SURFACE(1,2,((#116890,#116891,#116892,#116893,#116894),(#116895,
#116896,#116897,#116898,#116899)),.UNSPECIFIED.,.F.,.F.,.F.)
B_SPLINE_SURFACE_WITH_KNOTS((2,2),(3,2,3),(0.,0.289807040991565),(0.297684616398974,
0.297856505190613,0.315045384354503),.UNSPECIFIED.)
GEOMETRIC_REPRESENTATION_ITEM()
RATIONAL_B_SPLINE_SURFACE(((0.992924952273132,0.992924952273132,0.992924952273132,
0.988942764095691,0.98786440923939),(0.992924952273132,0.992924952273132,
0.992924952273132,0.988942764095691,0.98786440923939)))
REPRESENTATION_ITEM('')
SURFACE()
);
#1383=(
BOUNDED_SURFACE()
B_SPLINE_SURFACE(1,2,((#116907,#116908,#116909,#116910,#116911,#116912,
#116913),(#116914,#116915,#116916,#116917,#116918,#116919,#116920)),
 .UNSPECIFIED.,.F.,.F.,.F.)
B_SPLINE_SURFACE_WITH_KNOTS((2,2),(3,2,2,3),(0.,0.289681084359926),(0.418207303127979,
0.428571428571429,0.435775021682622,0.435950698868169),.UNSPECIFIED.)
GEOMETRIC_REPRESENTATION_ITEM()
RATIONAL_B_SPLINE_SURFACE(((0.993779895952495,0.996362096314125,1.,0.997471472332736,
0.995452950231063,0.995452950231063,0.995452950231063),(0.993779895952495,
0.996362096314125,1.,0.997471472332736,0.995452950231063,0.995452950231063,
0.995452950231063)))
REPRESENTATION_ITEM('')
SURFACE()
);
#1384=(
BOUNDED_SURFACE()
B_SPLINE_SURFACE(1,2,((#116922,#116923,#116924,#116925,#116926),(#116927,
#116928,#116929,#116930,#116931)),.UNSPECIFIED.,.F.,.F.,.F.)
B_SPLINE_SURFACE_WITH_KNOTS((2,2),(3,2,3),(0.,0.289807040991568),(0.297684616398974,
0.297856505190613,0.315045384354503),.UNSPECIFIED.)
GEOMETRIC_REPRESENTATION_ITEM()
RATIONAL_B_SPLINE_SURFACE(((0.992924952273132,0.992924952273132,0.992924952273132,
0.988942764095691,0.98786440923939),(0.992924952273132,0.992924952273132,
0.992924952273132,0.988942764095691,0.98786440923939)))
REPRESENTATION_ITEM('')
SURFACE()
);
#1385=(
BOUNDED_SURFACE()
B_SPLINE_SURFACE(1,2,((#116954,#116955,#116956,#116957,#116958,#116959,
#116960),(#116961,#116962,#116963,#116964,#116965,#116966,#116967)),
 .UNSPECIFIED.,.F.,.F.,.F.)
B_SPLINE_SURFACE_WITH_KNOTS((2,2),(3,2,2,3),(0.,0.289681084359931),(0.418207303127979,
0.428571428571429,0.435775021682622,0.435950698868169),.UNSPECIFIED.)
GEOMETRIC_REPRESENTATION_ITEM()
RATIONAL_B_SPLINE_SURFACE(((0.993779895952495,0.996362096314125,1.,0.997471472332736,
0.995452950231063,0.995452950231063,0.995452950231063),(0.993779895952495,
0.996362096314125,1.,0.997471472332736,0.995452950231063,0.995452950231063,
0.995452950231063)))
REPRESENTATION_ITEM('')
SURFACE()
);
#1386=(
BOUNDED_SURFACE()
B_SPLINE_SURFACE(1,2,((#116969,#116970,#116971,#116972,#116973),(#116974,
#116975,#116976,#116977,#116978)),.UNSPECIFIED.,.F.,.F.,.F.)
B_SPLINE_SURFACE_WITH_KNOTS((2,2),(3,2,3),(0.,0.289807040991561),(0.297684616398974,
0.297856505190613,0.315045384354503),.UNSPECIFIED.)
GEOMETRIC_REPRESENTATION_ITEM()
RATIONAL_B_SPLINE_SURFACE(((0.992924952273132,0.992924952273132,0.992924952273132,
0.988942764095691,0.98786440923939),(0.992924952273132,0.992924952273132,
0.992924952273132,0.988942764095691,0.98786440923939)))
REPRESENTATION_ITEM('')
SURFACE()
);
#1387=(
BOUNDED_SURFACE()
B_SPLINE_SURFACE(1,2,((#117001,#117002,#117003,#117004,#117005,#117006,
#117007),(#117008,#117009,#117010,#117011,#117012,#117013,#117014)),
 .UNSPECIFIED.,.F.,.F.,.F.)
B_SPLINE_SURFACE_WITH_KNOTS((2,2),(3,2,2,3),(0.,0.289681084359919),(0.418207303127979,
0.428571428571429,0.435775021682622,0.435950698868169),.UNSPECIFIED.)
GEOMETRIC_REPRESENTATION_ITEM()
RATIONAL_B_SPLINE_SURFACE(((0.993779895952495,0.996362096314125,1.,0.997471472332736,
0.995452950231063,0.995452950231063,0.995452950231063),(0.993779895952495,
0.996362096314125,1.,0.997471472332736,0.995452950231063,0.995452950231063,
0.995452950231063)))
REPRESENTATION_ITEM('')
SURFACE()
);
#1388=(
BOUNDED_SURFACE()
B_SPLINE_SURFACE(1,2,((#117016,#117017,#117018,#117019,#117020),(#117021,
#117022,#117023,#117024,#117025)),.UNSPECIFIED.,.F.,.F.,.F.)
B_SPLINE_SURFACE_WITH_KNOTS((2,2),(3,2,3),(0.,0.289807040991558),(0.297684616398974,
0.297856505190613,0.315045384354503),.UNSPECIFIED.)
GEOMETRIC_REPRESENTATION_ITEM()
RATIONAL_B_SPLINE_SURFACE(((0.992924952273132,0.992924952273132,0.992924952273132,
0.988942764095691,0.98786440923939),(0.992924952273132,0.992924952273132,
0.992924952273132,0.988942764095691,0.98786440923939)))
REPRESENTATION_ITEM('')
SURFACE()
);
#1389=(
BOUNDED_SURFACE()
B_SPLINE_SURFACE(1,2,((#117048,#117049,#117050,#117051,#117052,#117053,
#117054),(#117055,#117056,#117057,#117058,#117059,#117060,#117061)),
 .UNSPECIFIED.,.F.,.F.,.F.)
B_SPLINE_SURFACE_WITH_KNOTS((2,2),(3,2,2,3),(0.,0.289681084359921),(0.418207303127979,
0.428571428571429,0.435775021682622,0.435950698868169),.UNSPECIFIED.)
GEOMETRIC_REPRESENTATION_ITEM()
RATIONAL_B_SPLINE_SURFACE(((0.993779895952495,0.996362096314125,1.,0.997471472332736,
0.995452950231063,0.995452950231063,0.995452950231063),(0.993779895952495,
0.996362096314125,1.,0.997471472332736,0.995452950231063,0.995452950231063,
0.995452950231063)))
REPRESENTATION_ITEM('')
SURFACE()
);
#1390=(
BOUNDED_SURFACE()
B_SPLINE_SURFACE(1,2,((#117063,#117064,#117065,#117066,#117067),(#117068,
#117069,#117070,#117071,#117072)),.UNSPECIFIED.,.F.,.F.,.F.)
B_SPLINE_SURFACE_WITH_KNOTS((2,2),(3,2,3),(0.,0.289807040991672),(0.297684616398974,
0.297856505190613,0.315045384354503),.UNSPECIFIED.)
GEOMETRIC_REPRESENTATION_ITEM()
RATIONAL_B_SPLINE_SURFACE(((0.992924952273132,0.992924952273132,0.992924952273132,
0.988942764095691,0.98786440923939),(0.992924952273132,0.992924952273132,
0.992924952273132,0.988942764095691,0.98786440923939)))
REPRESENTATION_ITEM('')
SURFACE()
);
#1391=(
BOUNDED_SURFACE()
B_SPLINE_SURFACE(1,2,((#117095,#117096,#117097,#117098,#117099,#117100,
#117101),(#117102,#117103,#117104,#117105,#117106,#117107,#117108)),
 .UNSPECIFIED.,.F.,.F.,.F.)
B_SPLINE_SURFACE_WITH_KNOTS((2,2),(3,2,2,3),(0.,0.289681084359923),(0.418207303127979,
0.428571428571429,0.435775021682622,0.435950698868169),.UNSPECIFIED.)
GEOMETRIC_REPRESENTATION_ITEM()
RATIONAL_B_SPLINE_SURFACE(((0.993779895952495,0.996362096314125,1.,0.997471472332736,
0.995452950231063,0.995452950231063,0.995452950231063),(0.993779895952495,
0.996362096314125,1.,0.997471472332736,0.995452950231063,0.995452950231063,
0.995452950231063)))
REPRESENTATION_ITEM('')
SURFACE()
);
#1392=(
BOUNDED_SURFACE()
B_SPLINE_SURFACE(1,2,((#117110,#117111,#117112,#117113,#117114),(#117115,
#117116,#117117,#117118,#117119)),.UNSPECIFIED.,.F.,.F.,.F.)
B_SPLINE_SURFACE_WITH_KNOTS((2,2),(3,2,3),(0.,0.289807040992966),(0.297684616398974,
0.297856505190613,0.315045384354503),.UNSPECIFIED.)
GEOMETRIC_REPRESENTATION_ITEM()
RATIONAL_B_SPLINE_SURFACE(((0.992924952273132,0.992924952273132,0.992924952273132,
0.988942764095691,0.98786440923939),(0.992924952273132,0.992924952273132,
0.992924952273132,0.988942764095691,0.98786440923939)))
REPRESENTATION_ITEM('')
SURFACE()
);
#1393=(
BOUNDED_SURFACE()
B_SPLINE_SURFACE(1,2,((#117142,#117143,#117144,#117145,#117146,#117147,
#117148),(#117149,#117150,#117151,#117152,#117153,#117154,#117155)),
 .UNSPECIFIED.,.F.,.F.,.F.)
B_SPLINE_SURFACE_WITH_KNOTS((2,2),(3,2,2,3),(0.,0.28968108435992),(0.418207303127979,
0.428571428571429,0.435775021682622,0.435950698868169),.UNSPECIFIED.)
GEOMETRIC_REPRESENTATION_ITEM()
RATIONAL_B_SPLINE_SURFACE(((0.993779895952495,0.996362096314125,1.,0.997471472332736,
0.995452950231063,0.995452950231063,0.995452950231063),(0.993779895952495,
0.996362096314125,1.,0.997471472332736,0.995452950231063,0.995452950231063,
0.995452950231063)))
REPRESENTATION_ITEM('')
SURFACE()
);
#1394=(
BOUNDED_SURFACE()
B_SPLINE_SURFACE(1,2,((#117157,#117158,#117159,#117160,#117161),(#117162,
#117163,#117164,#117165,#117166)),.UNSPECIFIED.,.F.,.F.,.F.)
B_SPLINE_SURFACE_WITH_KNOTS((2,2),(3,2,3),(0.,0.289807040991817),(0.297684616398974,
0.297856505190613,0.315045384354503),.UNSPECIFIED.)
GEOMETRIC_REPRESENTATION_ITEM()
RATIONAL_B_SPLINE_SURFACE(((0.992924952273132,0.992924952273132,0.992924952273132,
0.988942764095691,0.98786440923939),(0.992924952273132,0.992924952273132,
0.992924952273132,0.988942764095691,0.987864409239391)))
REPRESENTATION_ITEM('')
SURFACE()
);
#1395=(
BOUNDED_SURFACE()
B_SPLINE_SURFACE(1,2,((#117189,#117190,#117191,#117192,#117193,#117194,
#117195),(#117196,#117197,#117198,#117199,#117200,#117201,#117202)),
 .UNSPECIFIED.,.F.,.F.,.F.)
B_SPLINE_SURFACE_WITH_KNOTS((2,2),(3,2,2,3),(0.,0.28968108435992),(0.418207303127979,
0.428571428571429,0.435775021682622,0.435950698868169),.UNSPECIFIED.)
GEOMETRIC_REPRESENTATION_ITEM()
RATIONAL_B_SPLINE_SURFACE(((0.993779895952495,0.996362096314125,1.,0.997471472332736,
0.995452950231063,0.995452950231063,0.995452950231063),(0.993779895952495,
0.996362096314125,1.,0.997471472332736,0.995452950231063,0.995452950231063,
0.995452950231063)))
REPRESENTATION_ITEM('')
SURFACE()
);
#1396=(
BOUNDED_SURFACE()
B_SPLINE_SURFACE(1,2,((#117204,#117205,#117206,#117207,#117208),(#117209,
#117210,#117211,#117212,#117213)),.UNSPECIFIED.,.F.,.F.,.F.)
B_SPLINE_SURFACE_WITH_KNOTS((2,2),(3,2,3),(0.,0.28980704099156),(0.297684616398974,
0.297856505190613,0.315045384354503),.UNSPECIFIED.)
GEOMETRIC_REPRESENTATION_ITEM()
RATIONAL_B_SPLINE_SURFACE(((0.992924952273132,0.992924952273132,0.992924952273132,
0.988942764095691,0.98786440923939),(0.992924952273132,0.992924952273132,
0.992924952273132,0.988942764095691,0.98786440923939)))
REPRESENTATION_ITEM('')
SURFACE()
);
#1397=(
BOUNDED_SURFACE()
B_SPLINE_SURFACE(1,2,((#117236,#117237,#117238,#117239,#117240,#117241,
#117242),(#117243,#117244,#117245,#117246,#117247,#117248,#117249)),
 .UNSPECIFIED.,.F.,.F.,.F.)
B_SPLINE_SURFACE_WITH_KNOTS((2,2),(3,2,2,3),(0.,0.28968108435992),(0.418207303127979,
0.428571428571429,0.435775021682622,0.435950698868169),.UNSPECIFIED.)
GEOMETRIC_REPRESENTATION_ITEM()
RATIONAL_B_SPLINE_SURFACE(((0.993779895952495,0.996362096314125,1.,0.997471472332736,
0.995452950231063,0.995452950231063,0.995452950231063),(0.993779895952495,
0.996362096314125,1.,0.997471472332736,0.995452950231063,0.995452950231063,
0.995452950231063)))
REPRESENTATION_ITEM('')
SURFACE()
);
#1398=(
BOUNDED_SURFACE()
B_SPLINE_SURFACE(1,2,((#117251,#117252,#117253,#117254,#117255),(#117256,
#117257,#117258,#117259,#117260)),.UNSPECIFIED.,.F.,.F.,.F.)
B_SPLINE_SURFACE_WITH_KNOTS((2,2),(3,2,3),(0.,0.289807040991555),(0.297684616398974,
0.297856505190613,0.315045384354503),.UNSPECIFIED.)
GEOMETRIC_REPRESENTATION_ITEM()
RATIONAL_B_SPLINE_SURFACE(((0.992924952273132,0.992924952273132,0.992924952273132,
0.988942764095691,0.98786440923939),(0.992924952273132,0.992924952273132,
0.992924952273132,0.988942764095691,0.98786440923939)))
REPRESENTATION_ITEM('')
SURFACE()
);
#1399=(
BOUNDED_SURFACE()
B_SPLINE_SURFACE(1,2,((#117271,#117272,#117273,#117274,#117275,#117276,
#117277),(#117278,#117279,#117280,#117281,#117282,#117283,#117284)),
 .UNSPECIFIED.,.F.,.F.,.F.)
B_SPLINE_SURFACE_WITH_KNOTS((2,2),(3,2,2,3),(0.,0.289681084359917),(0.418207303127979,
0.428571428571429,0.435775021682622,0.435950698868169),.UNSPECIFIED.)
GEOMETRIC_REPRESENTATION_ITEM()
RATIONAL_B_SPLINE_SURFACE(((0.993779895952495,0.996362096314125,1.,0.997471472332736,
0.995452950231063,0.995452950231063,0.995452950231063),(0.993779895952495,
0.996362096314125,1.,0.997471472332736,0.995452950231063,0.995452950231063,
0.995452950231063)))
REPRESENTATION_ITEM('')
SURFACE()
);
#1400=(
BOUNDED_SURFACE()
B_SPLINE_SURFACE(1,2,((#117298,#117299,#117300,#117301,#117302),(#117303,
#117304,#117305,#117306,#117307)),.UNSPECIFIED.,.F.,.F.,.F.)
B_SPLINE_SURFACE_WITH_KNOTS((2,2),(3,2,3),(0.,0.289807040991562),(0.297684616398974,
0.297856505190613,0.315045384354503),.UNSPECIFIED.)
GEOMETRIC_REPRESENTATION_ITEM()
RATIONAL_B_SPLINE_SURFACE(((0.992924952273132,0.992924952273132,0.992924952273132,
0.988942764095691,0.98786440923939),(0.992924952273132,0.992924952273132,
0.992924952273132,0.988942764095691,0.98786440923939)))
REPRESENTATION_ITEM('')
SURFACE()
);
#1401=(
BOUNDED_SURFACE()
B_SPLINE_SURFACE(1,2,((#117330,#117331,#117332,#117333,#117334,#117335,
#117336),(#117337,#117338,#117339,#117340,#117341,#117342,#117343)),
 .UNSPECIFIED.,.F.,.F.,.F.)
B_SPLINE_SURFACE_WITH_KNOTS((2,2),(3,2,2,3),(0.,0.289681084359921),(0.418207303127979,
0.428571428571429,0.435775021682621,0.435950698868168),.UNSPECIFIED.)
GEOMETRIC_REPRESENTATION_ITEM()
RATIONAL_B_SPLINE_SURFACE(((0.993779895952495,0.996362096314125,1.,0.997471472332737,
0.995452950231064,0.995452950231064,0.995452950231064),(0.993779895952495,
0.996362096314125,1.,0.997471472332737,0.995452950231063,0.995452950231063,
0.995452950231063)))
REPRESENTATION_ITEM('')
SURFACE()
);
#1402=(
BOUNDED_SURFACE()
B_SPLINE_SURFACE(1,2,((#117345,#117346,#117347,#117348,#117349),(#117350,
#117351,#117352,#117353,#117354)),.UNSPECIFIED.,.F.,.F.,.F.)
B_SPLINE_SURFACE_WITH_KNOTS((2,2),(3,2,3),(0.,0.289807040991634),(0.297684616398489,
0.297856505190132,0.315045384354507),.UNSPECIFIED.)
GEOMETRIC_REPRESENTATION_ITEM()
RATIONAL_B_SPLINE_SURFACE(((0.992924952273355,0.992924952273355,0.992924952273355,
0.988942764095721,0.98786440923939),(0.992924952273355,0.992924952273355,
0.992924952273355,0.988942764095721,0.98786440923939)))
REPRESENTATION_ITEM('')
SURFACE()
);
#1403=(
BOUNDED_SURFACE()
B_SPLINE_SURFACE(1,2,((#117377,#117378,#117379,#117380,#117381,#117382,
#117383),(#117384,#117385,#117386,#117387,#117388,#117389,#117390)),
 .UNSPECIFIED.,.F.,.F.,.F.)
B_SPLINE_SURFACE_WITH_KNOTS((2,2),(3,2,2,3),(0.,0.289681084359999),(0.418207303127978,
0.428571428571429,0.435775021682621,0.435950698868168),.UNSPECIFIED.)
GEOMETRIC_REPRESENTATION_ITEM()
RATIONAL_B_SPLINE_SURFACE(((0.993779895952495,0.996362096314125,1.,0.997471472332737,
0.995452950231063,0.995452950231063,0.995452950231063),(0.993779895952495,
0.996362096314125,1.,0.997471472332737,0.995452950231063,0.995452950231063,
0.995452950231063)))
REPRESENTATION_ITEM('')
SURFACE()
);
#1404=(
BOUNDED_SURFACE()
B_SPLINE_SURFACE(1,2,((#117392,#117393,#117394,#117395,#117396),(#117397,
#117398,#117399,#117400,#117401)),.UNSPECIFIED.,.F.,.F.,.F.)
B_SPLINE_SURFACE_WITH_KNOTS((2,2),(3,2,3),(0.,0.289807040991643),(0.297684616398975,
0.297856505190614,0.315045384354505),.UNSPECIFIED.)
GEOMETRIC_REPRESENTATION_ITEM()
RATIONAL_B_SPLINE_SURFACE(((0.992924952273132,0.992924952273132,0.992924952273132,
0.988942764095691,0.98786440923939),(0.992924952273132,0.992924952273132,
0.992924952273132,0.988942764095691,0.98786440923939)))
REPRESENTATION_ITEM('')
SURFACE()
);
#1405=(
BOUNDED_SURFACE()
B_SPLINE_SURFACE(1,2,((#117424,#117425,#117426,#117427,#117428,#117429,
#117430),(#117431,#117432,#117433,#117434,#117435,#117436,#117437)),
 .UNSPECIFIED.,.F.,.F.,.F.)
B_SPLINE_SURFACE_WITH_KNOTS((2,2),(3,2,2,3),(0.,0.28968108436),(0.418207303127978,
0.428571428571429,0.435775021682621,0.435950698868168),.UNSPECIFIED.)
GEOMETRIC_REPRESENTATION_ITEM()
RATIONAL_B_SPLINE_SURFACE(((0.993779895952495,0.996362096314125,1.,0.997471472332737,
0.995452950231063,0.995452950231063,0.995452950231063),(0.993779895952495,
0.996362096314125,1.,0.997471472332737,0.995452950231063,0.995452950231063,
0.995452950231063)))
REPRESENTATION_ITEM('')
SURFACE()
);
#1406=(
BOUNDED_SURFACE()
B_SPLINE_SURFACE(1,2,((#117439,#117440,#117441,#117442,#117443),(#117444,
#117445,#117446,#117447,#117448)),.UNSPECIFIED.,.F.,.F.,.F.)
B_SPLINE_SURFACE_WITH_KNOTS((2,2),(3,2,3),(0.,0.289807040991662),(0.29768461639894,
0.297856505190579,0.315045384354505),.UNSPECIFIED.)
GEOMETRIC_REPRESENTATION_ITEM()
RATIONAL_B_SPLINE_SURFACE(((0.992924952273148,0.992924952273148,0.992924952273148,
0.988942764095693,0.98786440923939),(0.992924952273148,0.992924952273148,
0.992924952273148,0.988942764095693,0.98786440923939)))
REPRESENTATION_ITEM('')
SURFACE()
);
#1407=(
BOUNDED_SURFACE()
B_SPLINE_SURFACE(1,2,((#117471,#117472,#117473,#117474,#117475,#117476,
#117477),(#117478,#117479,#117480,#117481,#117482,#117483,#117484)),
 .UNSPECIFIED.,.F.,.F.,.F.)
B_SPLINE_SURFACE_WITH_KNOTS((2,2),(3,2,2,3),(0.,0.289681084360011),(0.418207303127978,
0.428571428571429,0.435775021682622,0.435950698868169),.UNSPECIFIED.)
GEOMETRIC_REPRESENTATION_ITEM()
RATIONAL_B_SPLINE_SURFACE(((0.993779895952495,0.996362096314125,1.,0.997471472332736,
0.995452950231063,0.995452950231063,0.995452950231063),(0.993779895952495,
0.996362096314125,1.,0.997471472332736,0.995452950231063,0.995452950231063,
0.995452950231063)))
REPRESENTATION_ITEM('')
SURFACE()
);
#1408=(
BOUNDED_SURFACE()
B_SPLINE_SURFACE(1,2,((#117486,#117487,#117488,#117489,#117490),(#117491,
#117492,#117493,#117494,#117495)),.UNSPECIFIED.,.F.,.F.,.F.)
B_SPLINE_SURFACE_WITH_KNOTS((2,2),(3,2,3),(0.,0.289807040991655),(0.297684616398975,
0.297856505190614,0.315045384354503),.UNSPECIFIED.)
GEOMETRIC_REPRESENTATION_ITEM()
RATIONAL_B_SPLINE_SURFACE(((0.992924952273132,0.992924952273132,0.992924952273132,
0.988942764095691,0.98786440923939),(0.992924952273132,0.992924952273132,
0.992924952273132,0.988942764095691,0.98786440923939)))
REPRESENTATION_ITEM('')
SURFACE()
);
#1409=(
BOUNDED_SURFACE()
B_SPLINE_SURFACE(1,2,((#117518,#117519,#117520,#117521,#117522,#117523,
#117524),(#117525,#117526,#117527,#117528,#117529,#117530,#117531)),
 .UNSPECIFIED.,.F.,.F.,.F.)
B_SPLINE_SURFACE_WITH_KNOTS((2,2),(3,2,2,3),(0.,0.289681084359918),(0.418207303127979,
0.428571428571429,0.435775021682624,0.435950698868171),.UNSPECIFIED.)
GEOMETRIC_REPRESENTATION_ITEM()
RATIONAL_B_SPLINE_SURFACE(((0.993779895952495,0.996362096314125,1.,0.997471472332736,
0.995452950231062,0.995452950231062,0.995452950231062),(0.993779895952495,
0.996362096314125,1.,0.997471472332736,0.995452950231062,0.995452950231062,
0.995452950231062)))
REPRESENTATION_ITEM('')
SURFACE()
);
#1410=(
BOUNDED_SURFACE()
B_SPLINE_SURFACE(1,2,((#117533,#117534,#117535,#117536,#117537),(#117538,
#117539,#117540,#117541,#117542)),.UNSPECIFIED.,.F.,.F.,.F.)
B_SPLINE_SURFACE_WITH_KNOTS((2,2),(3,2,3),(0.,0.289807040992022),(0.297684616398974,
0.297856505190613,0.315045384354503),.UNSPECIFIED.)
GEOMETRIC_REPRESENTATION_ITEM()
RATIONAL_B_SPLINE_SURFACE(((0.992924952273132,0.992924952273132,0.992924952273132,
0.988942764095691,0.98786440923939),(0.992924952273132,0.992924952273132,
0.992924952273132,0.988942764095691,0.98786440923939)))
REPRESENTATION_ITEM('')
SURFACE()
);
#1411=(
BOUNDED_SURFACE()
B_SPLINE_SURFACE(1,2,((#117565,#117566,#117567,#117568,#117569,#117570,
#117571),(#117572,#117573,#117574,#117575,#117576,#117577,#117578)),
 .UNSPECIFIED.,.F.,.F.,.F.)
B_SPLINE_SURFACE_WITH_KNOTS((2,2),(3,2,2,3),(0.,0.289681084359936),(0.418207303127979,
0.428571428571429,0.435775021682622,0.435950698868169),.UNSPECIFIED.)
GEOMETRIC_REPRESENTATION_ITEM()
RATIONAL_B_SPLINE_SURFACE(((0.993779895952495,0.996362096314125,1.,0.997471472332736,
0.995452950231063,0.995452950231063,0.995452950231063),(0.993779895952495,
0.996362096314125,1.,0.997471472332736,0.995452950231063,0.995452950231063,
0.995452950231063)))
REPRESENTATION_ITEM('')
SURFACE()
);
#1412=(
BOUNDED_SURFACE()
B_SPLINE_SURFACE(1,2,((#117580,#117581,#117582,#117583,#117584),(#117585,
#117586,#117587,#117588,#117589)),.UNSPECIFIED.,.F.,.F.,.F.)
B_SPLINE_SURFACE_WITH_KNOTS((2,2),(3,2,3),(0.710318915640079,1.),(0.469916319328035,
0.487259899888158,0.487433335693759),.UNSPECIFIED.)
GEOMETRIC_REPRESENTATION_ITEM()
RATIONAL_B_SPLINE_SURFACE(((0.987775548376701,0.988735325500096,0.992651440660745,
0.992651440660745,0.992651440660745),(0.987775548376701,0.988735325500096,
0.992651440660745,0.992651440660745,0.992651440660745)))
REPRESENTATION_ITEM('')
SURFACE()
);
#1413=(
BOUNDED_SURFACE()
B_SPLINE_SURFACE(1,2,((#117600,#117601,#117602,#117603,#117604),(#117605,
#117606,#117607,#117608,#117609)),.UNSPECIFIED.,.F.,.F.,.F.)
B_SPLINE_SURFACE_WITH_KNOTS((2,2),(3,2,3),(0.709598828809336,1.),(0.245359920965979,
0.245954053070908,0.263201868951015),.UNSPECIFIED.)
GEOMETRIC_REPRESENTATION_ITEM()
RATIONAL_B_SPLINE_SURFACE(((0.987624841600687,0.987624841600687,0.987624841600687,
0.986938988894507,0.989176916802452),(0.987624841600687,0.987624841600687,
0.987624841600687,0.986938988894507,0.989176916802452)))
REPRESENTATION_ITEM('')
SURFACE()
);
#1414=(
BOUNDED_SURFACE()
B_SPLINE_SURFACE(1,2,((#117617,#117618,#117619,#117620,#117621),(#117622,
#117623,#117624,#117625,#117626)),.UNSPECIFIED.,.F.,.F.,.F.)
B_SPLINE_SURFACE_WITH_KNOTS((2,2),(3,2,3),(0.710318915640086,1.),(0.469916319328035,
0.487259899888158,0.487433335693759),.UNSPECIFIED.)
GEOMETRIC_REPRESENTATION_ITEM()
RATIONAL_B_SPLINE_SURFACE(((0.987775548376701,0.988735325500096,0.992651440660745,
0.992651440660745,0.992651440660745),(0.987775548376701,0.988735325500096,
0.992651440660745,0.992651440660745,0.992651440660745)))
REPRESENTATION_ITEM('')
SURFACE()
);
#1415=(
BOUNDED_SURFACE()
B_SPLINE_SURFACE(1,2,((#117637,#117638,#117639,#117640,#117641),(#117642,
#117643,#117644,#117645,#117646)),.UNSPECIFIED.,.F.,.F.,.F.)
B_SPLINE_SURFACE_WITH_KNOTS((2,2),(3,2,3),(0.709598828760674,1.),(0.245359920917525,
0.245954053070909,0.263201868951015),.UNSPECIFIED.)
GEOMETRIC_REPRESENTATION_ITEM()
RATIONAL_B_SPLINE_SURFACE(((0.987624841600687,0.987624841600687,0.987624841600687,
0.986938988894508,0.989176916802452),(0.987624841600687,0.987624841600687,
0.987624841600687,0.986938988894508,0.989176916802452)))
REPRESENTATION_ITEM('')
SURFACE()
);
#1416=(
BOUNDED_SURFACE()
B_SPLINE_SURFACE(1,2,((#117654,#117655,#117656,#117657,#117658),(#117659,
#117660,#117661,#117662,#117663)),.UNSPECIFIED.,.F.,.F.,.F.)
B_SPLINE_SURFACE_WITH_KNOTS((2,2),(3,2,3),(0.710318915640078,1.),(0.469916319328035,
0.487259899888158,0.487433335693759),.UNSPECIFIED.)
GEOMETRIC_REPRESENTATION_ITEM()
RATIONAL_B_SPLINE_SURFACE(((0.987775548376701,0.988735325500096,0.992651440660745,
0.992651440660745,0.992651440660745),(0.987775548376701,0.988735325500096,
0.992651440660745,0.992651440660745,0.992651440660745)))
REPRESENTATION_ITEM('')
SURFACE()
);
#1417=(
BOUNDED_SURFACE()
B_SPLINE_SURFACE(1,2,((#117674,#117675,#117676,#117677,#117678),(#117679,
#117680,#117681,#117682,#117683)),.UNSPECIFIED.,.F.,.F.,.F.)
B_SPLINE_SURFACE_WITH_KNOTS((2,2),(3,2,3),(0.709598828789182,1.),(0.245359920945796,
0.245954053070908,0.263201868951015),.UNSPECIFIED.)
GEOMETRIC_REPRESENTATION_ITEM()
RATIONAL_B_SPLINE_SURFACE(((0.987624841600687,0.987624841600687,0.987624841600687,
0.986938988894507,0.989176916802452),(0.987624841600687,0.987624841600687,
0.987624841600687,0.986938988894508,0.989176916802452)))
REPRESENTATION_ITEM('')
SURFACE()
);
#1418=(
BOUNDED_SURFACE()
B_SPLINE_SURFACE(1,2,((#117691,#117692,#117693,#117694,#117695),(#117696,
#117697,#117698,#117699,#117700)),.UNSPECIFIED.,.F.,.F.,.F.)
B_SPLINE_SURFACE_WITH_KNOTS((2,2),(3,2,3),(0.710318915639496,1.),(0.469916319328035,
0.487259899888158,0.487433335693759),.UNSPECIFIED.)
GEOMETRIC_REPRESENTATION_ITEM()
RATIONAL_B_SPLINE_SURFACE(((0.987775548376701,0.988735325500096,0.992651440660745,
0.992651440660745,0.992651440660745),(0.987775548376701,0.988735325500096,
0.992651440660745,0.992651440660745,0.992651440660745)))
REPRESENTATION_ITEM('')
SURFACE()
);
#1419=(
BOUNDED_SURFACE()
B_SPLINE_SURFACE(1,2,((#117711,#117712,#117713,#117714,#117715),(#117716,
#117717,#117718,#117719,#117720)),.UNSPECIFIED.,.F.,.F.,.F.)
B_SPLINE_SURFACE_WITH_KNOTS((2,2),(3,2,3),(0.709598828802843,1.),(0.245359920959965,
0.245954053070909,0.263201868951015),.UNSPECIFIED.)
GEOMETRIC_REPRESENTATION_ITEM()
RATIONAL_B_SPLINE_SURFACE(((0.987624841600687,0.987624841600687,0.987624841600687,
0.986938988894508,0.989176916802452),(0.987624841600687,0.987624841600687,
0.987624841600687,0.986938988894508,0.989176916802452)))
REPRESENTATION_ITEM('')
SURFACE()
);
#1420=(
BOUNDED_SURFACE()
B_SPLINE_SURFACE(1,2,((#117728,#117729,#117730,#117731,#117732),(#117733,
#117734,#117735,#117736,#117737)),.UNSPECIFIED.,.F.,.F.,.F.)
B_SPLINE_SURFACE_WITH_KNOTS((2,2),(3,2,3),(0.710318915640075,1.),(0.469916319328035,
0.487259899888158,0.487433335693759),.UNSPECIFIED.)
GEOMETRIC_REPRESENTATION_ITEM()
RATIONAL_B_SPLINE_SURFACE(((0.987775548376701,0.988735325500096,0.992651440660745,
0.992651440660745,0.992651440660745),(0.987775548376701,0.988735325500096,
0.992651440660745,0.992651440660745,0.992651440660745)))
REPRESENTATION_ITEM('')
SURFACE()
);
#1421=(
BOUNDED_SURFACE()
B_SPLINE_SURFACE(1,2,((#117748,#117749,#117750,#117751,#117752),(#117753,
#117754,#117755,#117756,#117757)),.UNSPECIFIED.,.F.,.F.,.F.)
B_SPLINE_SURFACE_WITH_KNOTS((2,2),(3,2,3),(0.709598828791051,1.),(0.245359920947667,
0.245954053070909,0.263201868951015),.UNSPECIFIED.)
GEOMETRIC_REPRESENTATION_ITEM()
RATIONAL_B_SPLINE_SURFACE(((0.987624841600687,0.987624841600687,0.987624841600687,
0.986938988894508,0.989176916802452),(0.987624841600687,0.987624841600687,
0.987624841600687,0.986938988894508,0.989176916802452)))
REPRESENTATION_ITEM('')
SURFACE()
);
#1422=(
BOUNDED_SURFACE()
B_SPLINE_SURFACE(1,2,((#117765,#117766,#117767,#117768,#117769),(#117770,
#117771,#117772,#117773,#117774)),.UNSPECIFIED.,.F.,.F.,.F.)
B_SPLINE_SURFACE_WITH_KNOTS((2,2),(3,2,3),(0.710318915639492,1.),(0.469916319328035,
0.487259899888158,0.487433335693759),.UNSPECIFIED.)
GEOMETRIC_REPRESENTATION_ITEM()
RATIONAL_B_SPLINE_SURFACE(((0.987775548376701,0.988735325500096,0.992651440660745,
0.992651440660745,0.992651440660745),(0.987775548376701,0.988735325500096,
0.992651440660745,0.992651440660745,0.992651440660745)))
REPRESENTATION_ITEM('')
SURFACE()
);
#1423=(
BOUNDED_SURFACE()
B_SPLINE_SURFACE(1,2,((#117785,#117786,#117787,#117788,#117789),(#117790,
#117791,#117792,#117793,#117794)),.UNSPECIFIED.,.F.,.F.,.F.)
B_SPLINE_SURFACE_WITH_KNOTS((2,2),(3,2,3),(0.709598828800151,1.),(0.245359920957343,
0.245954053070909,0.263201868951015),.UNSPECIFIED.)
GEOMETRIC_REPRESENTATION_ITEM()
RATIONAL_B_SPLINE_SURFACE(((0.987624841600687,0.987624841600687,0.987624841600687,
0.986938988894508,0.989176916802452),(0.987624841600687,0.987624841600687,
0.987624841600687,0.986938988894508,0.989176916802452)))
REPRESENTATION_ITEM('')
SURFACE()
);
#1424=(
BOUNDED_SURFACE()
B_SPLINE_SURFACE(1,2,((#117802,#117803,#117804,#117805,#117806),(#117807,
#117808,#117809,#117810,#117811)),.UNSPECIFIED.,.F.,.F.,.F.)
B_SPLINE_SURFACE_WITH_KNOTS((2,2),(3,2,3),(0.710318915640001,1.),(0.469916319328036,
0.487259899888158,0.487433335693759),.UNSPECIFIED.)
GEOMETRIC_REPRESENTATION_ITEM()
RATIONAL_B_SPLINE_SURFACE(((0.987775548376701,0.988735325500096,0.992651440660745,
0.992651440660745,0.992651440660745),(0.987775548376701,0.988735325500096,
0.992651440660745,0.992651440660745,0.992651440660745)))
REPRESENTATION_ITEM('')
SURFACE()
);
#1425=(
BOUNDED_SURFACE()
B_SPLINE_SURFACE(1,2,((#117822,#117823,#117824,#117825,#117826),(#117827,
#117828,#117829,#117830,#117831)),.UNSPECIFIED.,.F.,.F.,.F.)
B_SPLINE_SURFACE_WITH_KNOTS((2,2),(3,2,3),(0.709598828766692,1.),(0.245359920923563,
0.245954053070907,0.263201868951014),.UNSPECIFIED.)
GEOMETRIC_REPRESENTATION_ITEM()
RATIONAL_B_SPLINE_SURFACE(((0.987624841600687,0.987624841600687,0.987624841600687,
0.986938988894508,0.989176916802452),(0.987624841600687,0.987624841600687,
0.987624841600687,0.986938988894508,0.989176916802452)))
REPRESENTATION_ITEM('')
SURFACE()
);
#1426=(
BOUNDED_SURFACE()
B_SPLINE_SURFACE(1,2,((#117839,#117840,#117841,#117842,#117843),(#117844,
#117845,#117846,#117847,#117848)),.UNSPECIFIED.,.F.,.F.,.F.)
B_SPLINE_SURFACE_WITH_KNOTS((2,2),(3,2,3),(0.710318915640006,1.),(0.469916319328036,
0.487259899888159,0.48743333569376),.UNSPECIFIED.)
GEOMETRIC_REPRESENTATION_ITEM()
RATIONAL_B_SPLINE_SURFACE(((0.987775548376701,0.988735325500096,0.992651440660746,
0.992651440660746,0.992651440660746),(0.987775548376701,0.988735325500096,
0.992651440660746,0.992651440660746,0.992651440660746)))
REPRESENTATION_ITEM('')
SURFACE()
);
#1427=(
BOUNDED_SURFACE()
B_SPLINE_SURFACE(1,2,((#117859,#117860,#117861,#117862,#117863),(#117864,
#117865,#117866,#117867,#117868)),.UNSPECIFIED.,.F.,.F.,.F.)
B_SPLINE_SURFACE_WITH_KNOTS((2,2),(3,2,3),(0.70959882880507,1.),(0.245359920961868,
0.245954053070908,0.263201868951014),.UNSPECIFIED.)
GEOMETRIC_REPRESENTATION_ITEM()
RATIONAL_B_SPLINE_SURFACE(((0.987624841600687,0.987624841600687,0.987624841600687,
0.986938988894508,0.989176916802451),(0.987624841600687,0.987624841600687,
0.987624841600687,0.986938988894508,0.989176916802451)))
REPRESENTATION_ITEM('')
SURFACE()
);
#1428=(
BOUNDED_SURFACE()
B_SPLINE_SURFACE(1,2,((#117876,#117877,#117878,#117879,#117880),(#117881,
#117882,#117883,#117884,#117885)),.UNSPECIFIED.,.F.,.F.,.F.)
B_SPLINE_SURFACE_WITH_KNOTS((2,2),(3,2,3),(0.710318915639408,1.),(0.469916319328036,
0.487259899888159,0.48743333569376),.UNSPECIFIED.)
GEOMETRIC_REPRESENTATION_ITEM()
RATIONAL_B_SPLINE_SURFACE(((0.987775548376701,0.988735325500096,0.992651440660746,
0.992651440660746,0.992651440660746),(0.987775548376701,0.988735325500096,
0.992651440660746,0.992651440660746,0.992651440660746)))
REPRESENTATION_ITEM('')
SURFACE()
);
#1429=(
BOUNDED_SURFACE()
B_SPLINE_SURFACE(1,2,((#117896,#117897,#117898,#117899,#117900),(#117901,
#117902,#117903,#117904,#117905)),.UNSPECIFIED.,.F.,.F.,.F.)
B_SPLINE_SURFACE_WITH_KNOTS((2,2),(3,2,3),(0.709598828765639,1.),(0.245359920923153,
0.245954053070907,0.263201868951014),.UNSPECIFIED.)
GEOMETRIC_REPRESENTATION_ITEM()
RATIONAL_B_SPLINE_SURFACE(((0.987624841600687,0.987624841600687,0.987624841600687,
0.986938988894508,0.989176916802452),(0.987624841600687,0.987624841600687,
0.987624841600687,0.986938988894508,0.989176916802452)))
REPRESENTATION_ITEM('')
SURFACE()
);
#1430=(
BOUNDED_SURFACE()
B_SPLINE_SURFACE(1,2,((#117913,#117914,#117915,#117916,#117917),(#117918,
#117919,#117920,#117921,#117922)),.UNSPECIFIED.,.F.,.F.,.F.)
B_SPLINE_SURFACE_WITH_KNOTS((2,2),(3,2,3),(0.710318915639994,1.),(0.469916319328036,
0.487259899888159,0.48743333569376),.UNSPECIFIED.)
GEOMETRIC_REPRESENTATION_ITEM()
RATIONAL_B_SPLINE_SURFACE(((0.987775548376701,0.988735325500096,0.992651440660746,
0.992651440660746,0.992651440660746),(0.987775548376701,0.988735325500096,
0.992651440660746,0.992651440660746,0.992651440660746)))
REPRESENTATION_ITEM('')
SURFACE()
);
#1431=(
BOUNDED_SURFACE()
B_SPLINE_SURFACE(1,2,((#117933,#117934,#117935,#117936,#117937),(#117938,
#117939,#117940,#117941,#117942)),.UNSPECIFIED.,.F.,.F.,.F.)
B_SPLINE_SURFACE_WITH_KNOTS((2,2),(3,2,3),(0.709598828795369,1.),(0.245359920952099,
0.245954053070907,0.263201868951014),.UNSPECIFIED.)
GEOMETRIC_REPRESENTATION_ITEM()
RATIONAL_B_SPLINE_SURFACE(((0.987624841600687,0.987624841600687,0.987624841600687,
0.986938988894507,0.989176916802451),(0.987624841600687,0.987624841600687,
0.987624841600687,0.986938988894507,0.989176916802451)))
REPRESENTATION_ITEM('')
SURFACE()
);
#1432=(
BOUNDED_SURFACE()
B_SPLINE_SURFACE(1,2,((#117950,#117951,#117952,#117953,#117954),(#117955,
#117956,#117957,#117958,#117959)),.UNSPECIFIED.,.F.,.F.,.F.)
B_SPLINE_SURFACE_WITH_KNOTS((2,2),(3,2,3),(0.710318915639496,1.),(0.469916319328036,
0.487259899888159,0.48743333569376),.UNSPECIFIED.)
GEOMETRIC_REPRESENTATION_ITEM()
RATIONAL_B_SPLINE_SURFACE(((0.987775548376701,0.988735325500096,0.992651440660745,
0.992651440660745,0.992651440660745),(0.987775548376701,0.988735325500096,
0.992651440660745,0.992651440660745,0.992651440660745)))
REPRESENTATION_ITEM('')
SURFACE()
);
#1433=(
BOUNDED_SURFACE()
B_SPLINE_SURFACE(1,2,((#117970,#117971,#117972,#117973,#117974),(#117975,
#117976,#117977,#117978,#117979)),.UNSPECIFIED.,.F.,.F.,.F.)
B_SPLINE_SURFACE_WITH_KNOTS((2,2),(3,2,3),(0.709598828793834,1.),(0.245359920950977,
0.245954053070907,0.263201868951014),.UNSPECIFIED.)
GEOMETRIC_REPRESENTATION_ITEM()
RATIONAL_B_SPLINE_SURFACE(((0.987624841600687,0.987624841600687,0.987624841600687,
0.986938988894507,0.989176916802451),(0.987624841600687,0.987624841600687,
0.987624841600687,0.986938988894507,0.989176916802451)))
REPRESENTATION_ITEM('')
SURFACE()
);
#1434=(
BOUNDED_SURFACE()
B_SPLINE_SURFACE(1,2,((#117987,#117988,#117989,#117990,#117991),(#117992,
#117993,#117994,#117995,#117996)),.UNSPECIFIED.,.F.,.F.,.F.)
B_SPLINE_SURFACE_WITH_KNOTS((2,2),(3,2,3),(0.71031891563999,1.),(0.469916319328036,
0.48725989988816,0.487433335693761),.UNSPECIFIED.)
GEOMETRIC_REPRESENTATION_ITEM()
RATIONAL_B_SPLINE_SURFACE(((0.987775548376701,0.988735325500096,0.992651440660746,
0.992651440660746,0.992651440660746),(0.987775548376701,0.988735325500096,
0.992651440660746,0.992651440660746,0.992651440660746)))
REPRESENTATION_ITEM('')
SURFACE()
);
#1435=(
BOUNDED_SURFACE()
B_SPLINE_SURFACE(1,2,((#118007,#118008,#118009,#118010,#118011),(#118012,
#118013,#118014,#118015,#118016)),.UNSPECIFIED.,.F.,.F.,.F.)
B_SPLINE_SURFACE_WITH_KNOTS((2,2),(3,2,3),(0.709598828771055,1.),(0.245359920927963,
0.245954053070907,0.263201868951014),.UNSPECIFIED.)
GEOMETRIC_REPRESENTATION_ITEM()
RATIONAL_B_SPLINE_SURFACE(((0.987624841600687,0.987624841600687,0.987624841600687,
0.986938988894508,0.989176916802452),(0.987624841600687,0.987624841600687,
0.987624841600687,0.986938988894508,0.989176916802452)))
REPRESENTATION_ITEM('')
SURFACE()
);
#1436=(
BOUNDED_SURFACE()
B_SPLINE_SURFACE(1,2,((#118024,#118025,#118026,#118027,#118028),(#118029,
#118030,#118031,#118032,#118033)),.UNSPECIFIED.,.F.,.F.,.F.)
B_SPLINE_SURFACE_WITH_KNOTS((2,2),(3,2,3),(0.710318915639492,1.),(0.469916319328036,
0.487259899888159,0.48743333569376),.UNSPECIFIED.)
GEOMETRIC_REPRESENTATION_ITEM()
RATIONAL_B_SPLINE_SURFACE(((0.987775548376701,0.988735325500096,0.992651440660745,
0.992651440660745,0.992651440660745),(0.987775548376701,0.988735325500096,
0.992651440660745,0.992651440660745,0.992651440660745)))
REPRESENTATION_ITEM('')
SURFACE()
);
#1437=(
BOUNDED_SURFACE()
B_SPLINE_SURFACE(1,2,((#118044,#118045,#118046,#118047,#118048),(#118049,
#118050,#118051,#118052,#118053)),.UNSPECIFIED.,.F.,.F.,.F.)
B_SPLINE_SURFACE_WITH_KNOTS((2,2),(3,2,3),(0.709598828793346,1.),(0.2453599209506,
0.245954053070908,0.263201868951014),.UNSPECIFIED.)
GEOMETRIC_REPRESENTATION_ITEM()
RATIONAL_B_SPLINE_SURFACE(((0.987624841600687,0.987624841600687,0.987624841600687,
0.986938988894507,0.989176916802451),(0.987624841600687,0.987624841600687,
0.987624841600687,0.986938988894507,0.989176916802451)))
REPRESENTATION_ITEM('')
SURFACE()
);
#1438=(
BOUNDED_SURFACE()
B_SPLINE_SURFACE(1,2,((#118061,#118062,#118063,#118064,#118065),(#118066,
#118067,#118068,#118069,#118070)),.UNSPECIFIED.,.F.,.F.,.F.)
B_SPLINE_SURFACE_WITH_KNOTS((2,2),(3,2,3),(0.71031891563972,1.),(0.469916319328036,
0.487259899888159,0.48743333569376),.UNSPECIFIED.)
GEOMETRIC_REPRESENTATION_ITEM()
RATIONAL_B_SPLINE_SURFACE(((0.987775548376701,0.988735325500096,0.992651440660746,
0.992651440660746,0.992651440660746),(0.987775548376701,0.988735325500096,
0.992651440660746,0.992651440660746,0.992651440660746)))
REPRESENTATION_ITEM('')
SURFACE()
);
#1439=(
BOUNDED_SURFACE()
B_SPLINE_SURFACE(1,2,((#118081,#118082,#118083,#118084,#118085),(#118086,
#118087,#118088,#118089,#118090)),.UNSPECIFIED.,.F.,.F.,.F.)
B_SPLINE_SURFACE_WITH_KNOTS((2,2),(3,2,3),(0.709598828778751,1.),(0.24535992093593,
0.245954053070907,0.263201868951014),.UNSPECIFIED.)
GEOMETRIC_REPRESENTATION_ITEM()
RATIONAL_B_SPLINE_SURFACE(((0.987624841600687,0.987624841600687,0.987624841600687,
0.986938988894508,0.989176916802452),(0.987624841600687,0.987624841600687,
0.987624841600687,0.986938988894508,0.989176916802452)))
REPRESENTATION_ITEM('')
SURFACE()
);
#1440=(
BOUNDED_SURFACE()
B_SPLINE_SURFACE(1,2,((#118098,#118099,#118100,#118101,#118102),(#118103,
#118104,#118105,#118106,#118107)),.UNSPECIFIED.,.F.,.F.,.F.)
B_SPLINE_SURFACE_WITH_KNOTS((2,2),(3,2,3),(0.710318915638677,1.),(0.469916319328036,
0.487259899888159,0.48743333569376),.UNSPECIFIED.)
GEOMETRIC_REPRESENTATION_ITEM()
RATIONAL_B_SPLINE_SURFACE(((0.987775548376701,0.988735325500096,0.992651440660746,
0.992651440660746,0.992651440660746),(0.987775548376701,0.988735325500096,
0.992651440660746,0.992651440660746,0.992651440660746)))
REPRESENTATION_ITEM('')
SURFACE()
);
#1441=(
BOUNDED_SURFACE()
B_SPLINE_SURFACE(1,2,((#118118,#118119,#118120,#118121,#118122),(#118123,
#118124,#118125,#118126,#118127)),.UNSPECIFIED.,.F.,.F.,.F.)
B_SPLINE_SURFACE_WITH_KNOTS((2,2),(3,2,3),(0.709598828786485,1.),(0.245359920944462,
0.245954053070907,0.263201868951014),.UNSPECIFIED.)
GEOMETRIC_REPRESENTATION_ITEM()
RATIONAL_B_SPLINE_SURFACE(((0.987624841600687,0.987624841600687,0.987624841600687,
0.986938988894508,0.989176916802452),(0.987624841600687,0.987624841600687,
0.987624841600687,0.986938988894507,0.989176916802451)))
REPRESENTATION_ITEM('')
SURFACE()
);
#1442=(
BOUNDED_SURFACE()
B_SPLINE_SURFACE(1,2,((#118135,#118136,#118137,#118138,#118139),(#118140,
#118141,#118142,#118143,#118144)),.UNSPECIFIED.,.F.,.F.,.F.)
B_SPLINE_SURFACE_WITH_KNOTS((2,2),(3,2,3),(0.710318915639962,1.),(0.469916319328036,
0.487259899888159,0.48743333569376),.UNSPECIFIED.)
GEOMETRIC_REPRESENTATION_ITEM()
RATIONAL_B_SPLINE_SURFACE(((0.987775548376701,0.988735325500096,0.992651440660746,
0.992651440660746,0.992651440660746),(0.987775548376701,0.988735325500096,
0.992651440660746,0.992651440660746,0.992651440660746)))
REPRESENTATION_ITEM('')
SURFACE()
);
#1443=(
BOUNDED_SURFACE()
B_SPLINE_SURFACE(1,2,((#118155,#118156,#118157,#118158,#118159),(#118160,
#118161,#118162,#118163,#118164)),.UNSPECIFIED.,.F.,.F.,.F.)
B_SPLINE_SURFACE_WITH_KNOTS((2,2),(3,2,3),(0.709598828781523,1.),(0.245359920938325,
0.245954053070907,0.263201868951014),.UNSPECIFIED.)
GEOMETRIC_REPRESENTATION_ITEM()
RATIONAL_B_SPLINE_SURFACE(((0.987624841600687,0.987624841600687,0.987624841600687,
0.986938988894508,0.989176916802452),(0.987624841600687,0.987624841600687,
0.987624841600687,0.986938988894508,0.989176916802452)))
REPRESENTATION_ITEM('')
SURFACE()
);
#1444=(
BOUNDED_SURFACE()
B_SPLINE_SURFACE(1,2,((#118172,#118173,#118174,#118175,#118176),(#118177,
#118178,#118179,#118180,#118181)),.UNSPECIFIED.,.F.,.F.,.F.)
B_SPLINE_SURFACE_WITH_KNOTS((2,2),(3,2,3),(0.710318915640078,1.),(0.469916319328036,
0.487259899888159,0.48743333569376),.UNSPECIFIED.)
GEOMETRIC_REPRESENTATION_ITEM()
RATIONAL_B_SPLINE_SURFACE(((0.987775548376701,0.988735325500096,0.992651440660746,
0.992651440660746,0.992651440660746),(0.987775548376701,0.988735325500096,
0.992651440660746,0.992651440660746,0.992651440660746)))
REPRESENTATION_ITEM('')
SURFACE()
);
#1445=(
BOUNDED_SURFACE()
B_SPLINE_SURFACE(1,2,((#118192,#118193,#118194,#118195,#118196),(#118197,
#118198,#118199,#118200,#118201)),.UNSPECIFIED.,.F.,.F.,.F.)
B_SPLINE_SURFACE_WITH_KNOTS((2,2),(3,2,3),(0.70959882878374,1.),(0.245359920940315,
0.245954053070907,0.263201868951014),.UNSPECIFIED.)
GEOMETRIC_REPRESENTATION_ITEM()
RATIONAL_B_SPLINE_SURFACE(((0.987624841600687,0.987624841600687,0.987624841600687,
0.986938988894507,0.989176916802451),(0.987624841600687,0.987624841600687,
0.987624841600687,0.986938988894507,0.989176916802451)))
REPRESENTATION_ITEM('')
SURFACE()
);
#1446=(
BOUNDED_SURFACE()
B_SPLINE_SURFACE(1,2,((#118209,#118210,#118211,#118212,#118213),(#118214,
#118215,#118216,#118217,#118218)),.UNSPECIFIED.,.F.,.F.,.F.)
B_SPLINE_SURFACE_WITH_KNOTS((2,2),(3,2,3),(0.710318915639442,1.),(0.469916319328036,
0.487259899888159,0.48743333569376),.UNSPECIFIED.)
GEOMETRIC_REPRESENTATION_ITEM()
RATIONAL_B_SPLINE_SURFACE(((0.987775548376701,0.988735325500096,0.992651440660746,
0.992651440660746,0.992651440660746),(0.987775548376701,0.988735325500096,
0.992651440660746,0.992651440660746,0.992651440660746)))
REPRESENTATION_ITEM('')
SURFACE()
);
#1447=(
BOUNDED_SURFACE()
B_SPLINE_SURFACE(1,2,((#118229,#118230,#118231,#118232,#118233),(#118234,
#118235,#118236,#118237,#118238)),.UNSPECIFIED.,.F.,.F.,.F.)
B_SPLINE_SURFACE_WITH_KNOTS((2,2),(3,2,3),(0.70959882881485,1.),(0.245359920972021,
0.245954053070907,0.263201868951014),.UNSPECIFIED.)
GEOMETRIC_REPRESENTATION_ITEM()
RATIONAL_B_SPLINE_SURFACE(((0.987624841600687,0.987624841600687,0.987624841600687,
0.986938988894507,0.989176916802451),(0.987624841600687,0.987624841600687,
0.987624841600687,0.986938988894507,0.989176916802451)))
REPRESENTATION_ITEM('')
SURFACE()
);
#1448=(
BOUNDED_SURFACE()
B_SPLINE_SURFACE(1,2,((#118246,#118247,#118248,#118249,#118250),(#118251,
#118252,#118253,#118254,#118255)),.UNSPECIFIED.,.F.,.F.,.F.)
B_SPLINE_SURFACE_WITH_KNOTS((2,2),(3,2,3),(0.710318915640074,1.),(0.469916319328036,
0.487259899888159,0.48743333569376),.UNSPECIFIED.)
GEOMETRIC_REPRESENTATION_ITEM()
RATIONAL_B_SPLINE_SURFACE(((0.987775548376701,0.988735325500096,0.992651440660746,
0.992651440660746,0.992651440660746),(0.987775548376701,0.988735325500096,
0.992651440660746,0.992651440660746,0.992651440660746)))
REPRESENTATION_ITEM('')
SURFACE()
);
#1449=(
BOUNDED_SURFACE()
B_SPLINE_SURFACE(1,2,((#118266,#118267,#118268,#118269,#118270),(#118271,
#118272,#118273,#118274,#118275)),.UNSPECIFIED.,.F.,.F.,.F.)
B_SPLINE_SURFACE_WITH_KNOTS((2,2),(3,2,3),(0.709598828775925,1.),(0.245359920932689,
0.245954053070907,0.263201868951013),.UNSPECIFIED.)
GEOMETRIC_REPRESENTATION_ITEM()
RATIONAL_B_SPLINE_SURFACE(((0.987624841600687,0.987624841600687,0.987624841600687,
0.986938988894507,0.989176916802451),(0.987624841600687,0.987624841600687,
0.987624841600687,0.986938988894507,0.989176916802451)))
REPRESENTATION_ITEM('')
SURFACE()
);
#1450=(
BOUNDED_SURFACE()
B_SPLINE_SURFACE(1,2,((#118283,#118284,#118285,#118286,#118287),(#118288,
#118289,#118290,#118291,#118292)),.UNSPECIFIED.,.F.,.F.,.F.)
B_SPLINE_SURFACE_WITH_KNOTS((2,2),(3,2,3),(0.710318915638945,1.),(0.469916319328036,
0.487259899888159,0.48743333569376),.UNSPECIFIED.)
GEOMETRIC_REPRESENTATION_ITEM()
RATIONAL_B_SPLINE_SURFACE(((0.987775548376701,0.988735325500096,0.992651440660746,
0.992651440660746,0.992651440660746),(0.987775548376701,0.988735325500096,
0.992651440660746,0.992651440660746,0.992651440660746)))
REPRESENTATION_ITEM('')
SURFACE()
);
#1451=(
BOUNDED_SURFACE()
B_SPLINE_SURFACE(1,2,((#118303,#118304,#118305,#118306,#118307),(#118308,
#118309,#118310,#118311,#118312)),.UNSPECIFIED.,.F.,.F.,.F.)
B_SPLINE_SURFACE_WITH_KNOTS((2,2),(3,2,3),(0.709598828783652,1.),(0.245359920941388,
0.245954053070907,0.263201868951014),.UNSPECIFIED.)
GEOMETRIC_REPRESENTATION_ITEM()
RATIONAL_B_SPLINE_SURFACE(((0.987624841600687,0.987624841600687,0.987624841600687,
0.986938988894507,0.989176916802451),(0.987624841600687,0.987624841600687,
0.987624841600687,0.986938988894507,0.989176916802451)))
REPRESENTATION_ITEM('')
SURFACE()
);
#1452=(
BOUNDED_SURFACE()
B_SPLINE_SURFACE(1,2,((#118320,#118321,#118322,#118323,#118324),(#118325,
#118326,#118327,#118328,#118329)),.UNSPECIFIED.,.F.,.F.,.F.)
B_SPLINE_SURFACE_WITH_KNOTS((2,2),(3,2,3),(0.710318915639109,1.),(0.469916319328036,
0.487259899888159,0.48743333569376),.UNSPECIFIED.)
GEOMETRIC_REPRESENTATION_ITEM()
RATIONAL_B_SPLINE_SURFACE(((0.987775548376701,0.988735325500096,0.992651440660746,
0.992651440660746,0.992651440660746),(0.987775548376701,0.988735325500096,
0.992651440660746,0.992651440660746,0.992651440660746)))
REPRESENTATION_ITEM('')
SURFACE()
);
#1453=(
BOUNDED_SURFACE()
B_SPLINE_SURFACE(1,2,((#118340,#118341,#118342,#118343,#118344),(#118345,
#118346,#118347,#118348,#118349)),.UNSPECIFIED.,.F.,.F.,.F.)
B_SPLINE_SURFACE_WITH_KNOTS((2,2),(3,2,3),(0.709598828772429,1.),(0.245359920930035,
0.245954053070907,0.263201868951013),.UNSPECIFIED.)
GEOMETRIC_REPRESENTATION_ITEM()
RATIONAL_B_SPLINE_SURFACE(((0.987624841600687,0.987624841600687,0.987624841600687,
0.986938988894508,0.989176916802452),(0.987624841600687,0.987624841600687,
0.987624841600687,0.986938988894508,0.989176916802452)))
REPRESENTATION_ITEM('')
SURFACE()
);
#1454=(
BOUNDED_SURFACE()
B_SPLINE_SURFACE(1,2,((#118357,#118358,#118359,#118360,#118361),(#118362,
#118363,#118364,#118365,#118366)),.UNSPECIFIED.,.F.,.F.,.F.)
B_SPLINE_SURFACE_WITH_KNOTS((2,2),(3,2,3),(0.710318915638385,1.),(0.469916319328036,
0.487259899888159,0.48743333569376),.UNSPECIFIED.)
GEOMETRIC_REPRESENTATION_ITEM()
RATIONAL_B_SPLINE_SURFACE(((0.987775548376701,0.988735325500096,0.992651440660746,
0.992651440660746,0.992651440660746),(0.987775548376701,0.988735325500096,
0.992651440660746,0.992651440660746,0.992651440660746)))
REPRESENTATION_ITEM('')
SURFACE()
);
#1455=(
BOUNDED_SURFACE()
B_SPLINE_SURFACE(1,2,((#118374,#118375,#118376,#118377,#118378),(#118379,
#118380,#118381,#118382,#118383)),.UNSPECIFIED.,.F.,.F.,.F.)
B_SPLINE_SURFACE_WITH_KNOTS((2,2),(3,2,3),(0.709598828798267,1.),(0.245359920956622,
0.245954053070907,0.263201868951013),.UNSPECIFIED.)
GEOMETRIC_REPRESENTATION_ITEM()
RATIONAL_B_SPLINE_SURFACE(((0.987624841600687,0.987624841600687,0.987624841600687,
0.986938988894507,0.989176916802451),(0.987624841600687,0.987624841600687,
0.987624841600687,0.986938988894507,0.989176916802451)))
REPRESENTATION_ITEM('')
SURFACE()
);
#1456=(
BOUNDED_SURFACE()
B_SPLINE_SURFACE(1,2,((#118385,#118386,#118387,#118388,#118389),(#118390,
#118391,#118392,#118393,#118394)),.UNSPECIFIED.,.F.,.F.,.F.)
B_SPLINE_SURFACE_WITH_KNOTS((2,2),(3,2,3),(0.71031891563988,1.),(0.469916319328036,
0.487259899888159,0.48743333569376),.UNSPECIFIED.)
GEOMETRIC_REPRESENTATION_ITEM()
RATIONAL_B_SPLINE_SURFACE(((0.987775548376701,0.988735325500096,0.992651440660746,
0.992651440660746,0.992651440660746),(0.987775548376701,0.988735325500096,
0.992651440660746,0.992651440660746,0.992651440660746)))
REPRESENTATION_ITEM('')
SURFACE()
);
#1457=(
BOUNDED_SURFACE()
B_SPLINE_SURFACE(1,2,((#118405,#118406,#118407,#118408,#118409),(#118410,
#118411,#118412,#118413,#118414)),.UNSPECIFIED.,.F.,.F.,.F.)
B_SPLINE_SURFACE_WITH_KNOTS((2,2),(3,2,3),(0.70959882880242,1.),(0.245359920959295,
0.245954053070907,0.263201868951013),.UNSPECIFIED.)
GEOMETRIC_REPRESENTATION_ITEM()
RATIONAL_B_SPLINE_SURFACE(((0.987624841600687,0.987624841600687,0.987624841600687,
0.986938988894507,0.989176916802451),(0.987624841600687,0.987624841600687,
0.987624841600687,0.986938988894507,0.989176916802451)))
REPRESENTATION_ITEM('')
SURFACE()
);
#1458=(
BOUNDED_SURFACE()
B_SPLINE_SURFACE(1,2,((#118422,#118423,#118424,#118425,#118426),(#118427,
#118428,#118429,#118430,#118431)),.UNSPECIFIED.,.F.,.F.,.F.)
B_SPLINE_SURFACE_WITH_KNOTS((2,2),(3,2,3),(0.710318915638591,1.),(0.469916319328036,
0.487259899888159,0.48743333569376),.UNSPECIFIED.)
GEOMETRIC_REPRESENTATION_ITEM()
RATIONAL_B_SPLINE_SURFACE(((0.987775548376701,0.988735325500096,0.992651440660746,
0.992651440660746,0.992651440660746),(0.987775548376701,0.988735325500096,
0.992651440660746,0.992651440660746,0.992651440660746)))
REPRESENTATION_ITEM('')
SURFACE()
);
#1459=(
BOUNDED_SURFACE()
B_SPLINE_SURFACE(1,2,((#118442,#118443,#118444,#118445,#118446),(#118447,
#118448,#118449,#118450,#118451)),.UNSPECIFIED.,.F.,.F.,.F.)
B_SPLINE_SURFACE_WITH_KNOTS((2,2),(3,2,3),(0.709598828781214,1.),(0.245359920939413,
0.245954053070907,0.263201868951017),.UNSPECIFIED.)
GEOMETRIC_REPRESENTATION_ITEM()
RATIONAL_B_SPLINE_SURFACE(((0.987624841600687,0.987624841600687,0.987624841600687,
0.986938988894507,0.989176916802452),(0.987624841600687,0.987624841600687,
0.987624841600687,0.986938988894507,0.989176916802452)))
REPRESENTATION_ITEM('')
SURFACE()
);
#1460=(
BOUNDED_SURFACE()
B_SPLINE_SURFACE(1,2,((#118459,#118460,#118461,#118462,#118463),(#118464,
#118465,#118466,#118467,#118468)),.UNSPECIFIED.,.F.,.F.,.F.)
B_SPLINE_SURFACE_WITH_KNOTS((2,2),(3,2,3),(0.710318915638836,1.),(0.469916319328036,
0.487259899888159,0.48743333569376),.UNSPECIFIED.)
GEOMETRIC_REPRESENTATION_ITEM()
RATIONAL_B_SPLINE_SURFACE(((0.987775548376701,0.988735325500096,0.992651440660746,
0.992651440660746,0.992651440660746),(0.987775548376701,0.988735325500096,
0.992651440660746,0.992651440660746,0.992651440660746)))
REPRESENTATION_ITEM('')
SURFACE()
);
#1461=(
BOUNDED_SURFACE()
B_SPLINE_SURFACE(1,2,((#118479,#118480,#118481,#118482,#118483),(#118484,
#118485,#118486,#118487,#118488)),.UNSPECIFIED.,.F.,.F.,.F.)
B_SPLINE_SURFACE_WITH_KNOTS((2,2),(3,2,3),(0.709598828784904,1.),(0.245359920942991,
0.245954053070907,0.263201868951015),.UNSPECIFIED.)
GEOMETRIC_REPRESENTATION_ITEM()
RATIONAL_B_SPLINE_SURFACE(((0.987624841600687,0.987624841600687,0.987624841600687,
0.986938988894507,0.989176916802452),(0.987624841600687,0.987624841600687,
0.987624841600687,0.986938988894507,0.989176916802452)))
REPRESENTATION_ITEM('')
SURFACE()
);
#1462=(
BOUNDED_SURFACE()
B_SPLINE_SURFACE(1,2,((#118496,#118497,#118498,#118499,#118500),(#118501,
#118502,#118503,#118504,#118505)),.UNSPECIFIED.,.F.,.F.,.F.)
B_SPLINE_SURFACE_WITH_KNOTS((2,2),(3,2,3),(0.710318915639086,1.),(0.469916319328036,
0.487259899888159,0.48743333569376),.UNSPECIFIED.)
GEOMETRIC_REPRESENTATION_ITEM()
RATIONAL_B_SPLINE_SURFACE(((0.987775548376701,0.988735325500096,0.992651440660746,
0.992651440660746,0.992651440660746),(0.987775548376701,0.988735325500096,
0.992651440660746,0.992651440660746,0.992651440660746)))
REPRESENTATION_ITEM('')
SURFACE()
);
#1463=(
BOUNDED_SURFACE()
B_SPLINE_SURFACE(1,2,((#118516,#118517,#118518,#118519,#118520),(#118521,
#118522,#118523,#118524,#118525)),.UNSPECIFIED.,.F.,.F.,.F.)
B_SPLINE_SURFACE_WITH_KNOTS((2,2),(3,2,3),(0.709598828779162,1.),(0.245359920936906,
0.245954053070907,0.263201868951013),.UNSPECIFIED.)
GEOMETRIC_REPRESENTATION_ITEM()
RATIONAL_B_SPLINE_SURFACE(((0.987624841600687,0.987624841600687,0.987624841600687,
0.986938988894507,0.989176916802451),(0.987624841600687,0.987624841600687,
0.987624841600687,0.986938988894507,0.989176916802451)))
REPRESENTATION_ITEM('')
SURFACE()
);
#1464=(
BOUNDED_SURFACE()
B_SPLINE_SURFACE(1,2,((#118533,#118534,#118535,#118536,#118537),(#118538,
#118539,#118540,#118541,#118542)),.UNSPECIFIED.,.F.,.F.,.F.)
B_SPLINE_SURFACE_WITH_KNOTS((2,2),(3,2,3),(0.710318915639156,1.),(0.469916319328036,
0.487259899888159,0.48743333569376),.UNSPECIFIED.)
GEOMETRIC_REPRESENTATION_ITEM()
RATIONAL_B_SPLINE_SURFACE(((0.987775548376701,0.988735325500096,0.992651440660746,
0.992651440660746,0.992651440660746),(0.987775548376701,0.988735325500096,
0.992651440660746,0.992651440660746,0.992651440660746)))
REPRESENTATION_ITEM('')
SURFACE()
);
#1465=(
BOUNDED_SURFACE()
B_SPLINE_SURFACE(1,2,((#118553,#118554,#118555,#118556,#118557),(#118558,
#118559,#118560,#118561,#118562)),.UNSPECIFIED.,.F.,.F.,.F.)
B_SPLINE_SURFACE_WITH_KNOTS((2,2),(3,2,3),(0.709598828805424,1.),(0.245359920963013,
0.245954053070908,0.263201868951014),.UNSPECIFIED.)
GEOMETRIC_REPRESENTATION_ITEM()
RATIONAL_B_SPLINE_SURFACE(((0.987624841600687,0.987624841600687,0.987624841600687,
0.986938988894508,0.989176916802451),(0.987624841600687,0.987624841600687,
0.987624841600687,0.986938988894508,0.989176916802451)))
REPRESENTATION_ITEM('')
SURFACE()
);
#1466=(
BOUNDED_SURFACE()
B_SPLINE_SURFACE(1,2,((#118570,#118571,#118572,#118573,#118574),(#118575,
#118576,#118577,#118578,#118579)),.UNSPECIFIED.,.F.,.F.,.F.)
B_SPLINE_SURFACE_WITH_KNOTS((2,2),(3,2,3),(0.71031891563883,1.),(0.469916319328036,
0.487259899888161,0.487433335693762),.UNSPECIFIED.)
GEOMETRIC_REPRESENTATION_ITEM()
RATIONAL_B_SPLINE_SURFACE(((0.987775548376701,0.988735325500096,0.992651440660746,
0.992651440660746,0.992651440660746),(0.987775548376701,0.988735325500096,
0.992651440660746,0.992651440660746,0.992651440660746)))
REPRESENTATION_ITEM('')
SURFACE()
);
#1467=(
BOUNDED_SURFACE()
B_SPLINE_SURFACE(1,2,((#118590,#118591,#118592,#118593,#118594),(#118595,
#118596,#118597,#118598,#118599)),.UNSPECIFIED.,.F.,.F.,.F.)
B_SPLINE_SURFACE_WITH_KNOTS((2,2),(3,2,3),(0.709598828788555,1.),(0.24535992094641,
0.245954053070899,0.263201868951014),.UNSPECIFIED.)
GEOMETRIC_REPRESENTATION_ITEM()
RATIONAL_B_SPLINE_SURFACE(((0.987624841600687,0.987624841600687,0.987624841600687,
0.986938988894506,0.989176916802451),(0.987624841600687,0.987624841600687,
0.987624841600687,0.986938988894506,0.989176916802451)))
REPRESENTATION_ITEM('')
SURFACE()
);
#1468=(
BOUNDED_SURFACE()
B_SPLINE_SURFACE(1,2,((#118607,#118608,#118609,#118610,#118611),(#118612,
#118613,#118614,#118615,#118616)),.UNSPECIFIED.,.F.,.F.,.F.)
B_SPLINE_SURFACE_WITH_KNOTS((2,2),(3,2,3),(0.710318915638989,1.),(0.469916319328036,
0.487259899888159,0.48743333569376),.UNSPECIFIED.)
GEOMETRIC_REPRESENTATION_ITEM()
RATIONAL_B_SPLINE_SURFACE(((0.987775548376701,0.988735325500096,0.992651440660746,
0.992651440660746,0.992651440660746),(0.987775548376701,0.988735325500096,
0.992651440660746,0.992651440660746,0.992651440660746)))
REPRESENTATION_ITEM('')
SURFACE()
);
#1469=(
BOUNDED_SURFACE()
B_SPLINE_SURFACE(1,2,((#118627,#118628,#118629,#118630,#118631),(#118632,
#118633,#118634,#118635,#118636)),.UNSPECIFIED.,.F.,.F.,.F.)
B_SPLINE_SURFACE_WITH_KNOTS((2,2),(3,2,3),(0.709598828800189,1.),(0.24535992095796,
0.245954053070909,0.263201868951013),.UNSPECIFIED.)
GEOMETRIC_REPRESENTATION_ITEM()
RATIONAL_B_SPLINE_SURFACE(((0.987624841600687,0.987624841600687,0.987624841600687,
0.986938988894508,0.989176916802452),(0.987624841600687,0.987624841600687,
0.987624841600687,0.986938988894508,0.989176916802452)))
REPRESENTATION_ITEM('')
SURFACE()
);
#1470=(
BOUNDED_SURFACE()
B_SPLINE_SURFACE(1,2,((#118644,#118645,#118646),(#118647,#118648,#118649)),
 .UNSPECIFIED.,.F.,.F.,.F.)
B_SPLINE_SURFACE_WITH_KNOTS((2,2),(3,3),(0.710192959008021,1.),(0.435775021682622,
0.453027768259469),.UNSPECIFIED.)
GEOMETRIC_REPRESENTATION_ITEM()
RATIONAL_B_SPLINE_SURFACE(((0.995452950231063,0.990618550266714,0.988709602819327),
(0.995452950231063,0.990618550266714,0.988709602819327)))
REPRESENTATION_ITEM('')
SURFACE()
);
#1471=(
BOUNDED_SURFACE()
B_SPLINE_SURFACE(1,2,((#118658,#118659,#118660,#118661,#118662),(#118663,
#118664,#118665,#118666,#118667)),.UNSPECIFIED.,.F.,.F.,.F.)
B_SPLINE_SURFACE_WITH_KNOTS((2,2),(3,2,3),(0.710318915639671,1.),(0.280328542633765,
0.285714285714286,0.297856505190614),.UNSPECIFIED.)
GEOMETRIC_REPRESENTATION_ITEM()
RATIONAL_B_SPLINE_SURFACE(((0.996504189652446,0.998109554471267,1.,0.995737968897747,
0.992924952273132),(0.996504189652447,0.998109554471267,1.,0.995737968897747,
0.992924952273132)))
REPRESENTATION_ITEM('')
SURFACE()
);
#1472=(
BOUNDED_SURFACE()
B_SPLINE_SURFACE(1,2,((#118678,#118679,#118680),(#118681,#118682,#118683)),
 .UNSPECIFIED.,.F.,.F.,.F.)
B_SPLINE_SURFACE_WITH_KNOTS((2,2),(3,3),(0.710192959008101,1.),(0.435775021682622,
0.453027768259469),.UNSPECIFIED.)
GEOMETRIC_REPRESENTATION_ITEM()
RATIONAL_B_SPLINE_SURFACE(((0.995452950231063,0.990618550266714,0.988709602819327),
(0.995452950231063,0.990618550266714,0.988709602819327)))
REPRESENTATION_ITEM('')
SURFACE()
);
#1473=(
BOUNDED_SURFACE()
B_SPLINE_SURFACE(1,2,((#118692,#118693,#118694,#118695,#118696),(#118697,
#118698,#118699,#118700,#118701)),.UNSPECIFIED.,.F.,.F.,.F.)
B_SPLINE_SURFACE_WITH_KNOTS((2,2),(3,2,3),(0.710318915639747,1.),(0.280328542633765,
0.285714285714286,0.297856505190613),.UNSPECIFIED.)
GEOMETRIC_REPRESENTATION_ITEM()
RATIONAL_B_SPLINE_SURFACE(((0.996504189652446,0.998109554471267,1.,0.995737968897747,
0.992924952273132),(0.996504189652447,0.998109554471267,1.,0.995737968897747,
0.992924952273132)))
REPRESENTATION_ITEM('')
SURFACE()
);
#1474=(
BOUNDED_SURFACE()
B_SPLINE_SURFACE(1,2,((#118712,#118713,#118714),(#118715,#118716,#118717)),
 .UNSPECIFIED.,.F.,.F.,.F.)
B_SPLINE_SURFACE_WITH_KNOTS((2,2),(3,3),(0.71019295900799,1.),(0.43577502168215,
0.453027768259472),.UNSPECIFIED.)
GEOMETRIC_REPRESENTATION_ITEM()
RATIONAL_B_SPLINE_SURFACE(((0.995452950231328,0.990618550266766,0.988709602819326),
(0.995452950231328,0.990618550266766,0.988709602819326)))
REPRESENTATION_ITEM('')
SURFACE()
);
#1475=(
BOUNDED_SURFACE()
B_SPLINE_SURFACE(1,2,((#118726,#118727,#118728,#118729,#118730),(#118731,
#118732,#118733,#118734,#118735)),.UNSPECIFIED.,.F.,.F.,.F.)
B_SPLINE_SURFACE_WITH_KNOTS((2,2),(3,2,3),(0.710318915639631,1.),(0.280328542633765,
0.285714285714286,0.297856505190614),.UNSPECIFIED.)
GEOMETRIC_REPRESENTATION_ITEM()
RATIONAL_B_SPLINE_SURFACE(((0.996504189652446,0.998109554471267,1.,0.995737968897747,
0.992924952273132),(0.996504189652446,0.998109554471267,1.,0.995737968897747,
0.992924952273132)))
REPRESENTATION_ITEM('')
SURFACE()
);
#1476=(
BOUNDED_SURFACE()
B_SPLINE_SURFACE(1,2,((#118746,#118747,#118748),(#118749,#118750,#118751)),
 .UNSPECIFIED.,.F.,.F.,.F.)
B_SPLINE_SURFACE_WITH_KNOTS((2,2),(3,3),(0.710192959007314,1.),(0.435775021682621,
0.453027768259469),.UNSPECIFIED.)
GEOMETRIC_REPRESENTATION_ITEM()
RATIONAL_B_SPLINE_SURFACE(((0.995452950231063,0.990618550266714,0.988709602819327),
(0.995452950231063,0.990618550266714,0.988709602819327)))
REPRESENTATION_ITEM('')
SURFACE()
);
#1477=(
BOUNDED_SURFACE()
B_SPLINE_SURFACE(1,2,((#118760,#118761,#118762,#118763,#118764),(#118765,
#118766,#118767,#118768,#118769)),.UNSPECIFIED.,.F.,.F.,.F.)
B_SPLINE_SURFACE_WITH_KNOTS((2,2),(3,2,3),(0.710318915638957,1.),(0.280328542633765,
0.285714285714286,0.297856505190614),.UNSPECIFIED.)
GEOMETRIC_REPRESENTATION_ITEM()
RATIONAL_B_SPLINE_SURFACE(((0.996504189652447,0.998109554471267,1.,0.995737968897747,
0.992924952273132),(0.996504189652447,0.998109554471267,1.,0.995737968897747,
0.992924952273132)))
REPRESENTATION_ITEM('')
SURFACE()
);
#1478=(
BOUNDED_SURFACE()
B_SPLINE_SURFACE(1,2,((#118780,#118781,#118782),(#118783,#118784,#118785)),
 .UNSPECIFIED.,.F.,.F.,.F.)
B_SPLINE_SURFACE_WITH_KNOTS((2,2),(3,3),(0.710192959007467,1.),(0.435775021682622,
0.453027768259469),.UNSPECIFIED.)
GEOMETRIC_REPRESENTATION_ITEM()
RATIONAL_B_SPLINE_SURFACE(((0.995452950231063,0.990618550266714,0.988709602819327),
(0.995452950231063,0.990618550266714,0.988709602819327)))
REPRESENTATION_ITEM('')
SURFACE()
);
#1479=(
BOUNDED_SURFACE()
B_SPLINE_SURFACE(1,2,((#118794,#118795,#118796,#118797,#118798),(#118799,
#118800,#118801,#118802,#118803)),.UNSPECIFIED.,.F.,.F.,.F.)
B_SPLINE_SURFACE_WITH_KNOTS((2,2),(3,2,3),(0.710318915639107,1.),(0.280328542633765,
0.285714285714286,0.297856505190614),.UNSPECIFIED.)
GEOMETRIC_REPRESENTATION_ITEM()
RATIONAL_B_SPLINE_SURFACE(((0.996504189652447,0.998109554471267,1.,0.995737968897747,
0.992924952273132),(0.996504189652447,0.998109554471267,1.,0.995737968897747,
0.992924952273132)))
REPRESENTATION_ITEM('')
SURFACE()
);
#1480=(
BOUNDED_SURFACE()
B_SPLINE_SURFACE(1,2,((#118814,#118815,#118816),(#118817,#118818,#118819)),
 .UNSPECIFIED.,.F.,.F.,.F.)
B_SPLINE_SURFACE_WITH_KNOTS((2,2),(3,3),(0.710192959007502,1.),(0.435775021682622,
0.453027768259469),.UNSPECIFIED.)
GEOMETRIC_REPRESENTATION_ITEM()
RATIONAL_B_SPLINE_SURFACE(((0.995452950231063,0.990618550266714,0.988709602819327),
(0.995452950231063,0.990618550266714,0.988709602819327)))
REPRESENTATION_ITEM('')
SURFACE()
);
#1481=(
BOUNDED_SURFACE()
B_SPLINE_SURFACE(1,2,((#118828,#118829,#118830,#118831,#118832),(#118833,
#118834,#118835,#118836,#118837)),.UNSPECIFIED.,.F.,.F.,.F.)
B_SPLINE_SURFACE_WITH_KNOTS((2,2),(3,2,3),(0.710318915639146,1.),(0.280328542633765,
0.285714285714286,0.297856505190614),.UNSPECIFIED.)
GEOMETRIC_REPRESENTATION_ITEM()
RATIONAL_B_SPLINE_SURFACE(((0.996504189652446,0.998109554471267,1.,0.995737968897747,
0.992924952273132),(0.996504189652446,0.998109554471267,1.,0.995737968897747,
0.992924952273132)))
REPRESENTATION_ITEM('')
SURFACE()
);
#1482=(
BOUNDED_SURFACE()
B_SPLINE_SURFACE(1,2,((#118848,#118849,#118850),(#118851,#118852,#118853)),
 .UNSPECIFIED.,.F.,.F.,.F.)
B_SPLINE_SURFACE_WITH_KNOTS((2,2),(3,3),(0.710192959007325,1.),(0.435775021682622,
0.453027768259469),.UNSPECIFIED.)
GEOMETRIC_REPRESENTATION_ITEM()
RATIONAL_B_SPLINE_SURFACE(((0.995452950231063,0.990618550266714,0.988709602819327),
(0.995452950231063,0.990618550266714,0.988709602819327)))
REPRESENTATION_ITEM('')
SURFACE()
);
#1483=(
BOUNDED_SURFACE()
B_SPLINE_SURFACE(1,2,((#118862,#118863,#118864,#118865,#118866),(#118867,
#118868,#118869,#118870,#118871)),.UNSPECIFIED.,.F.,.F.,.F.)
B_SPLINE_SURFACE_WITH_KNOTS((2,2),(3,2,3),(0.710318915638968,1.),(0.280328542633765,
0.285714285714286,0.297856505190614),.UNSPECIFIED.)
GEOMETRIC_REPRESENTATION_ITEM()
RATIONAL_B_SPLINE_SURFACE(((0.996504189652446,0.998109554471267,1.,0.995737968897747,
0.992924952273132),(0.996504189652446,0.998109554471267,1.,0.995737968897747,
0.992924952273132)))
REPRESENTATION_ITEM('')
SURFACE()
);
#1484=(
BOUNDED_SURFACE()
B_SPLINE_SURFACE(1,2,((#118882,#118883,#118884),(#118885,#118886,#118887)),
 .UNSPECIFIED.,.F.,.F.,.F.)
B_SPLINE_SURFACE_WITH_KNOTS((2,2),(3,3),(0.710192959008261,1.),(0.435775021682622,
0.453027768259469),.UNSPECIFIED.)
GEOMETRIC_REPRESENTATION_ITEM()
RATIONAL_B_SPLINE_SURFACE(((0.995452950231063,0.990618550266714,0.988709602819327),
(0.995452950231063,0.990618550266714,0.988709602819327)))
REPRESENTATION_ITEM('')
SURFACE()
);
#1485=(
BOUNDED_SURFACE()
B_SPLINE_SURFACE(1,2,((#118896,#118897,#118898,#118899,#118900),(#118901,
#118902,#118903,#118904,#118905)),.UNSPECIFIED.,.F.,.F.,.F.)
B_SPLINE_SURFACE_WITH_KNOTS((2,2),(3,2,3),(0.7103189156399,1.),(0.280328542633765,
0.285714285714286,0.297856505190614),.UNSPECIFIED.)
GEOMETRIC_REPRESENTATION_ITEM()
RATIONAL_B_SPLINE_SURFACE(((0.996504189652446,0.998109554471267,1.,0.995737968897747,
0.992924952273132),(0.996504189652446,0.998109554471267,1.,0.995737968897747,
0.992924952273132)))
REPRESENTATION_ITEM('')
SURFACE()
);
#1486=(
BOUNDED_SURFACE()
B_SPLINE_SURFACE(1,2,((#118916,#118917,#118918),(#118919,#118920,#118921)),
 .UNSPECIFIED.,.F.,.F.,.F.)
B_SPLINE_SURFACE_WITH_KNOTS((2,2),(3,3),(0.710192959008251,1.),(0.435775021682622,
0.453027768259469),.UNSPECIFIED.)
GEOMETRIC_REPRESENTATION_ITEM()
RATIONAL_B_SPLINE_SURFACE(((0.995452950231063,0.990618550266714,0.988709602819327),
(0.995452950231063,0.990618550266714,0.988709602819327)))
REPRESENTATION_ITEM('')
SURFACE()
);
#1487=(
BOUNDED_SURFACE()
B_SPLINE_SURFACE(1,2,((#118930,#118931,#118932,#118933,#118934),(#118935,
#118936,#118937,#118938,#118939)),.UNSPECIFIED.,.F.,.F.,.F.)
B_SPLINE_SURFACE_WITH_KNOTS((2,2),(3,2,3),(0.710318915639895,1.),(0.280328542633765,
0.285714285714286,0.297856505190614),.UNSPECIFIED.)
GEOMETRIC_REPRESENTATION_ITEM()
RATIONAL_B_SPLINE_SURFACE(((0.996504189652446,0.998109554471267,1.,0.995737968897747,
0.992924952273132),(0.996504189652446,0.998109554471267,1.,0.995737968897747,
0.992924952273132)))
REPRESENTATION_ITEM('')
SURFACE()
);
#1488=(
BOUNDED_SURFACE()
B_SPLINE_SURFACE(1,2,((#118950,#118951,#118952),(#118953,#118954,#118955)),
 .UNSPECIFIED.,.F.,.F.,.F.)
B_SPLINE_SURFACE_WITH_KNOTS((2,2),(3,3),(0.710192959008144,1.),(0.435775021682622,
0.453027768259469),.UNSPECIFIED.)
GEOMETRIC_REPRESENTATION_ITEM()
RATIONAL_B_SPLINE_SURFACE(((0.995452950231063,0.990618550266714,0.988709602819327),
(0.995452950231063,0.990618550266714,0.988709602819327)))
REPRESENTATION_ITEM('')
SURFACE()
);
#1489=(
BOUNDED_SURFACE()
B_SPLINE_SURFACE(1,2,((#118964,#118965,#118966,#118967,#118968),(#118969,
#118970,#118971,#118972,#118973)),.UNSPECIFIED.,.F.,.F.,.F.)
B_SPLINE_SURFACE_WITH_KNOTS((2,2),(3,2,3),(0.710318915639317,1.),(0.280328542633765,
0.285714285714286,0.297856505190614),.UNSPECIFIED.)
GEOMETRIC_REPRESENTATION_ITEM()
RATIONAL_B_SPLINE_SURFACE(((0.996504189652446,0.998109554471267,1.,0.995737968897747,
0.992924952273132),(0.996504189652446,0.998109554471267,1.,0.995737968897747,
0.992924952273132)))
REPRESENTATION_ITEM('')
SURFACE()
);
#1490=(
BOUNDED_SURFACE()
B_SPLINE_SURFACE(1,2,((#118984,#118985,#118986),(#118987,#118988,#118989)),
 .UNSPECIFIED.,.F.,.F.,.F.)
B_SPLINE_SURFACE_WITH_KNOTS((2,2),(3,3),(0.710192959008211,1.),(0.435775021682622,
0.453027768259469),.UNSPECIFIED.)
GEOMETRIC_REPRESENTATION_ITEM()
RATIONAL_B_SPLINE_SURFACE(((0.995452950231063,0.990618550266714,0.988709602819327),
(0.995452950231063,0.990618550266714,0.988709602819327)))
REPRESENTATION_ITEM('')
SURFACE()
);
#1491=(
BOUNDED_SURFACE()
B_SPLINE_SURFACE(1,2,((#118998,#118999,#119000,#119001,#119002),(#119003,
#119004,#119005,#119006,#119007)),.UNSPECIFIED.,.F.,.F.,.F.)
B_SPLINE_SURFACE_WITH_KNOTS((2,2),(3,2,3),(0.710318915639847,1.),(0.280328542633765,
0.285714285714286,0.297856505190614),.UNSPECIFIED.)
GEOMETRIC_REPRESENTATION_ITEM()
RATIONAL_B_SPLINE_SURFACE(((0.996504189652446,0.998109554471267,1.,0.995737968897747,
0.992924952273132),(0.996504189652446,0.998109554471267,1.,0.995737968897747,
0.992924952273132)))
REPRESENTATION_ITEM('')
SURFACE()
);
#1492=(
BOUNDED_SURFACE()
B_SPLINE_SURFACE(1,2,((#119018,#119019,#119020),(#119021,#119022,#119023)),
 .UNSPECIFIED.,.F.,.F.,.F.)
B_SPLINE_SURFACE_WITH_KNOTS((2,2),(3,3),(0.710192959008243,1.),(0.435775021682622,
0.453027768259469),.UNSPECIFIED.)
GEOMETRIC_REPRESENTATION_ITEM()
RATIONAL_B_SPLINE_SURFACE(((0.995452950231063,0.990618550266714,0.988709602819327),
(0.995452950231063,0.990618550266714,0.988709602819327)))
REPRESENTATION_ITEM('')
SURFACE()
);
#1493=(
BOUNDED_SURFACE()
B_SPLINE_SURFACE(1,2,((#119032,#119033,#119034,#119035,#119036),(#119037,
#119038,#119039,#119040,#119041)),.UNSPECIFIED.,.F.,.F.,.F.)
B_SPLINE_SURFACE_WITH_KNOTS((2,2),(3,2,3),(0.710318915639875,1.),(0.280328542633765,
0.285714285714286,0.297856505190614),.UNSPECIFIED.)
GEOMETRIC_REPRESENTATION_ITEM()
RATIONAL_B_SPLINE_SURFACE(((0.996504189652446,0.998109554471267,1.,0.995737968897747,
0.992924952273132),(0.996504189652446,0.998109554471267,1.,0.995737968897747,
0.992924952273132)))
REPRESENTATION_ITEM('')
SURFACE()
);
#1494=(
BOUNDED_SURFACE()
B_SPLINE_SURFACE(1,2,((#119052,#119053,#119054),(#119055,#119056,#119057)),
 .UNSPECIFIED.,.F.,.F.,.F.)
B_SPLINE_SURFACE_WITH_KNOTS((2,2),(3,3),(0.71019295900829,1.),(0.435775021682622,
0.453027768259469),.UNSPECIFIED.)
GEOMETRIC_REPRESENTATION_ITEM()
RATIONAL_B_SPLINE_SURFACE(((0.995452950231063,0.990618550266714,0.988709602819327),
(0.995452950231063,0.990618550266714,0.988709602819327)))
REPRESENTATION_ITEM('')
SURFACE()
);
#1495=(
BOUNDED_SURFACE()
B_SPLINE_SURFACE(1,2,((#119066,#119067,#119068,#119069,#119070),(#119071,
#119072,#119073,#119074,#119075)),.UNSPECIFIED.,.F.,.F.,.F.)
B_SPLINE_SURFACE_WITH_KNOTS((2,2),(3,2,3),(0.710318915639929,1.),(0.280328542633765,
0.285714285714286,0.297856505190614),.UNSPECIFIED.)
GEOMETRIC_REPRESENTATION_ITEM()
RATIONAL_B_SPLINE_SURFACE(((0.996504189652446,0.998109554471267,1.,0.995737968897747,
0.992924952273132),(0.996504189652447,0.998109554471267,1.,0.995737968897747,
0.992924952273132)))
REPRESENTATION_ITEM('')
SURFACE()
);
#1496=(
BOUNDED_SURFACE()
B_SPLINE_SURFACE(1,2,((#119086,#119087,#119088),(#119089,#119090,#119091)),
 .UNSPECIFIED.,.F.,.F.,.F.)
B_SPLINE_SURFACE_WITH_KNOTS((2,2),(3,3),(0.710192959008439,1.),(0.435775021682622,
0.453027768259469),.UNSPECIFIED.)
GEOMETRIC_REPRESENTATION_ITEM()
RATIONAL_B_SPLINE_SURFACE(((0.995452950231063,0.990618550266714,0.988709602819327),
(0.995452950231063,0.990618550266714,0.988709602819327)))
REPRESENTATION_ITEM('')
SURFACE()
);
#1497=(
BOUNDED_SURFACE()
B_SPLINE_SURFACE(1,2,((#119100,#119101,#119102,#119103,#119104),(#119105,
#119106,#119107,#119108,#119109)),.UNSPECIFIED.,.F.,.F.,.F.)
B_SPLINE_SURFACE_WITH_KNOTS((2,2),(3,2,3),(0.710318915640072,1.),(0.280328542633765,
0.285714285714286,0.297856505190614),.UNSPECIFIED.)
GEOMETRIC_REPRESENTATION_ITEM()
RATIONAL_B_SPLINE_SURFACE(((0.996504189652447,0.998109554471267,1.,0.995737968897747,
0.992924952273132),(0.996504189652447,0.998109554471267,1.,0.995737968897747,
0.992924952273132)))
REPRESENTATION_ITEM('')
SURFACE()
);
#1498=(
BOUNDED_SURFACE()
B_SPLINE_SURFACE(1,2,((#119120,#119121,#119122),(#119123,#119124,#119125)),
 .UNSPECIFIED.,.F.,.F.,.F.)
B_SPLINE_SURFACE_WITH_KNOTS((2,2),(3,3),(0.710192959008441,1.),(0.435775021682622,
0.453027768259469),.UNSPECIFIED.)
GEOMETRIC_REPRESENTATION_ITEM()
RATIONAL_B_SPLINE_SURFACE(((0.995452950231063,0.990618550266714,0.988709602819327),
(0.995452950231063,0.990618550266714,0.988709602819327)))
REPRESENTATION_ITEM('')
SURFACE()
);
#1499=(
BOUNDED_SURFACE()
B_SPLINE_SURFACE(1,2,((#119134,#119135,#119136,#119137,#119138),(#119139,
#119140,#119141,#119142,#119143)),.UNSPECIFIED.,.F.,.F.,.F.)
B_SPLINE_SURFACE_WITH_KNOTS((2,2),(3,2,3),(0.710318915640079,1.),(0.280328542633765,
0.285714285714286,0.297856505190614),.UNSPECIFIED.)
GEOMETRIC_REPRESENTATION_ITEM()
RATIONAL_B_SPLINE_SURFACE(((0.996504189652446,0.998109554471267,1.,0.995737968897747,
0.992924952273132),(0.996504189652447,0.998109554471267,1.,0.995737968897747,
0.992924952273132)))
REPRESENTATION_ITEM('')
SURFACE()
);
#1500=(
BOUNDED_SURFACE()
B_SPLINE_SURFACE(1,2,((#119154,#119155,#119156),(#119157,#119158,#119159)),
 .UNSPECIFIED.,.F.,.F.,.F.)
B_SPLINE_SURFACE_WITH_KNOTS((2,2),(3,3),(0.710192959008438,1.),(0.435775021682622,
0.453027768259469),.UNSPECIFIED.)
GEOMETRIC_REPRESENTATION_ITEM()
RATIONAL_B_SPLINE_SURFACE(((0.995452950231063,0.990618550266714,0.988709602819327),
(0.995452950231063,0.990618550266714,0.988709602819327)))
REPRESENTATION_ITEM('')
SURFACE()
);
#1501=(
BOUNDED_SURFACE()
B_SPLINE_SURFACE(1,2,((#119168,#119169,#119170,#119171,#119172),(#119173,
#119174,#119175,#119176,#119177)),.UNSPECIFIED.,.F.,.F.,.F.)
B_SPLINE_SURFACE_WITH_KNOTS((2,2),(3,2,3),(0.710318915640069,1.),(0.280328542633765,
0.285714285714286,0.297856505190614),.UNSPECIFIED.)
GEOMETRIC_REPRESENTATION_ITEM()
RATIONAL_B_SPLINE_SURFACE(((0.996504189652446,0.998109554471267,1.,0.995737968897747,
0.992924952273132),(0.996504189652446,0.998109554471267,1.,0.995737968897747,
0.992924952273132)))
REPRESENTATION_ITEM('')
SURFACE()
);
#1502=(
BOUNDED_SURFACE()
B_SPLINE_SURFACE(1,2,((#119188,#119189,#119190),(#119191,#119192,#119193)),
 .UNSPECIFIED.,.F.,.F.,.F.)
B_SPLINE_SURFACE_WITH_KNOTS((2,2),(3,3),(0.710192959008439,1.),(0.435775021682622,
0.453027768259469),.UNSPECIFIED.)
GEOMETRIC_REPRESENTATION_ITEM()
RATIONAL_B_SPLINE_SURFACE(((0.995452950231063,0.990618550266714,0.988709602819327),
(0.995452950231063,0.990618550266714,0.988709602819327)))
REPRESENTATION_ITEM('')
SURFACE()
);
#1503=(
BOUNDED_SURFACE()
B_SPLINE_SURFACE(1,2,((#119202,#119203,#119204,#119205,#119206),(#119207,
#119208,#119209,#119210,#119211)),.UNSPECIFIED.,.F.,.F.,.F.)
B_SPLINE_SURFACE_WITH_KNOTS((2,2),(3,2,3),(0.710318915640078,1.),(0.280328542633765,
0.285714285714286,0.297856505190614),.UNSPECIFIED.)
GEOMETRIC_REPRESENTATION_ITEM()
RATIONAL_B_SPLINE_SURFACE(((0.996504189652446,0.998109554471267,1.,0.995737968897747,
0.992924952273132),(0.996504189652446,0.998109554471267,1.,0.995737968897747,
0.992924952273132)))
REPRESENTATION_ITEM('')
SURFACE()
);
#1504=(
BOUNDED_SURFACE()
B_SPLINE_SURFACE(1,2,((#119222,#119223,#119224),(#119225,#119226,#119227)),
 .UNSPECIFIED.,.F.,.F.,.F.)
B_SPLINE_SURFACE_WITH_KNOTS((2,2),(3,3),(0.710192959008441,1.),(0.435775021682622,
0.453027768259469),.UNSPECIFIED.)
GEOMETRIC_REPRESENTATION_ITEM()
RATIONAL_B_SPLINE_SURFACE(((0.995452950231063,0.990618550266714,0.988709602819327),
(0.995452950231063,0.990618550266714,0.988709602819327)))
REPRESENTATION_ITEM('')
SURFACE()
);
#1505=(
BOUNDED_SURFACE()
B_SPLINE_SURFACE(1,2,((#119236,#119237,#119238,#119239,#119240),(#119241,
#119242,#119243,#119244,#119245)),.UNSPECIFIED.,.F.,.F.,.F.)
B_SPLINE_SURFACE_WITH_KNOTS((2,2),(3,2,3),(0.710318915640079,1.),(0.280328542633765,
0.285714285714286,0.297856505190614),.UNSPECIFIED.)
GEOMETRIC_REPRESENTATION_ITEM()
RATIONAL_B_SPLINE_SURFACE(((0.996504189652446,0.998109554471267,1.,0.995737968897747,
0.992924952273132),(0.996504189652447,0.998109554471267,1.,0.995737968897747,
0.992924952273132)))
REPRESENTATION_ITEM('')
SURFACE()
);
#1506=(
BOUNDED_SURFACE()
B_SPLINE_SURFACE(1,2,((#119256,#119257,#119258),(#119259,#119260,#119261)),
 .UNSPECIFIED.,.F.,.F.,.F.)
B_SPLINE_SURFACE_WITH_KNOTS((2,2),(3,3),(0.710192959008329,1.),(0.435775021682622,
0.453027768259469),.UNSPECIFIED.)
GEOMETRIC_REPRESENTATION_ITEM()
RATIONAL_B_SPLINE_SURFACE(((0.995452950231063,0.990618550266714,0.988709602819327),
(0.995452950231063,0.990618550266714,0.988709602819327)))
REPRESENTATION_ITEM('')
SURFACE()
);
#1507=(
BOUNDED_SURFACE()
B_SPLINE_SURFACE(1,2,((#119270,#119271,#119272,#119273,#119274),(#119275,
#119276,#119277,#119278,#119279)),.UNSPECIFIED.,.F.,.F.,.F.)
B_SPLINE_SURFACE_WITH_KNOTS((2,2),(3,2,3),(0.710318915639972,1.),(0.280328542633765,
0.285714285714286,0.297856505190614),.UNSPECIFIED.)
GEOMETRIC_REPRESENTATION_ITEM()
RATIONAL_B_SPLINE_SURFACE(((0.996504189652447,0.998109554471267,1.,0.995737968897747,
0.992924952273132),(0.996504189652447,0.998109554471267,1.,0.995737968897747,
0.992924952273132)))
REPRESENTATION_ITEM('')
SURFACE()
);
#1508=(
BOUNDED_SURFACE()
B_SPLINE_SURFACE(1,2,((#119290,#119291,#119292),(#119293,#119294,#119295)),
 .UNSPECIFIED.,.F.,.F.,.F.)
B_SPLINE_SURFACE_WITH_KNOTS((2,2),(3,3),(0.710192959007031,1.),(0.435775021682622,
0.453027768259469),.UNSPECIFIED.)
GEOMETRIC_REPRESENTATION_ITEM()
RATIONAL_B_SPLINE_SURFACE(((0.995452950231063,0.990618550266714,0.988709602819327),
(0.995452950231063,0.990618550266714,0.988709602819327)))
REPRESENTATION_ITEM('')
SURFACE()
);
#1509=(
BOUNDED_SURFACE()
B_SPLINE_SURFACE(1,2,((#119304,#119305,#119306,#119307,#119308),(#119309,
#119310,#119311,#119312,#119313)),.UNSPECIFIED.,.F.,.F.,.F.)
B_SPLINE_SURFACE_WITH_KNOTS((2,2),(3,2,3),(0.710318915638671,1.),(0.280328542633765,
0.285714285714286,0.297856505190614),.UNSPECIFIED.)
GEOMETRIC_REPRESENTATION_ITEM()
RATIONAL_B_SPLINE_SURFACE(((0.996504189652446,0.998109554471267,1.,0.995737968897747,
0.992924952273132),(0.996504189652446,0.998109554471267,1.,0.995737968897747,
0.992924952273132)))
REPRESENTATION_ITEM('')
SURFACE()
);
#1510=(
BOUNDED_SURFACE()
B_SPLINE_SURFACE(1,2,((#119324,#119325,#119326),(#119327,#119328,#119329)),
 .UNSPECIFIED.,.F.,.F.,.F.)
B_SPLINE_SURFACE_WITH_KNOTS((2,2),(3,3),(0.710192959008183,1.),(0.435775021682622,
0.453027768259469),.UNSPECIFIED.)
GEOMETRIC_REPRESENTATION_ITEM()
RATIONAL_B_SPLINE_SURFACE(((0.995452950231063,0.990618550266714,0.988709602819327),
(0.995452950231063,0.990618550266714,0.988709602819327)))
REPRESENTATION_ITEM('')
SURFACE()
);
#1511=(
BOUNDED_SURFACE()
B_SPLINE_SURFACE(1,2,((#119338,#119339,#119340,#119341,#119342),(#119343,
#119344,#119345,#119346,#119347)),.UNSPECIFIED.,.F.,.F.,.F.)
B_SPLINE_SURFACE_WITH_KNOTS((2,2),(3,2,3),(0.710318915639824,1.),(0.280328542633765,
0.285714285714286,0.297856505190614),.UNSPECIFIED.)
GEOMETRIC_REPRESENTATION_ITEM()
RATIONAL_B_SPLINE_SURFACE(((0.996504189652447,0.998109554471267,1.,0.995737968897747,
0.992924952273132),(0.996504189652447,0.998109554471267,1.,0.995737968897747,
0.992924952273132)))
REPRESENTATION_ITEM('')
SURFACE()
);
#1512=(
BOUNDED_SURFACE()
B_SPLINE_SURFACE(1,2,((#119358,#119359,#119360),(#119361,#119362,#119363)),
 .UNSPECIFIED.,.F.,.F.,.F.)
B_SPLINE_SURFACE_WITH_KNOTS((2,2),(3,3),(0.710192959008437,1.),(0.435775021682622,
0.453027768259469),.UNSPECIFIED.)
GEOMETRIC_REPRESENTATION_ITEM()
RATIONAL_B_SPLINE_SURFACE(((0.995452950231063,0.990618550266714,0.988709602819327),
(0.995452950231063,0.990618550266714,0.988709602819327)))
REPRESENTATION_ITEM('')
SURFACE()
);
#1513=(
BOUNDED_SURFACE()
B_SPLINE_SURFACE(1,2,((#119372,#119373,#119374,#119375,#119376),(#119377,
#119378,#119379,#119380,#119381)),.UNSPECIFIED.,.F.,.F.,.F.)
B_SPLINE_SURFACE_WITH_KNOTS((2,2),(3,2,3),(0.710318915640082,1.),(0.280328542633765,
0.285714285714286,0.297856505190614),.UNSPECIFIED.)
GEOMETRIC_REPRESENTATION_ITEM()
RATIONAL_B_SPLINE_SURFACE(((0.996504189652447,0.998109554471267,1.,0.995737968897747,
0.992924952273132),(0.996504189652447,0.998109554471267,1.,0.995737968897747,
0.992924952273132)))
REPRESENTATION_ITEM('')
SURFACE()
);
#1514=(
BOUNDED_SURFACE()
B_SPLINE_SURFACE(1,2,((#119392,#119393,#119394),(#119395,#119396,#119397)),
 .UNSPECIFIED.,.F.,.F.,.F.)
B_SPLINE_SURFACE_WITH_KNOTS((2,2),(3,3),(0.71019295900844,1.),(0.435775021682622,
0.453027768259469),.UNSPECIFIED.)
GEOMETRIC_REPRESENTATION_ITEM()
RATIONAL_B_SPLINE_SURFACE(((0.995452950231063,0.990618550266714,0.988709602819327),
(0.995452950231063,0.990618550266714,0.988709602819327)))
REPRESENTATION_ITEM('')
SURFACE()
);
#1515=(
BOUNDED_SURFACE()
B_SPLINE_SURFACE(1,2,((#119406,#119407,#119408,#119409,#119410),(#119411,
#119412,#119413,#119414,#119415)),.UNSPECIFIED.,.F.,.F.,.F.)
B_SPLINE_SURFACE_WITH_KNOTS((2,2),(3,2,3),(0.710318915640079,1.),(0.280328542633765,
0.285714285714286,0.297856505190614),.UNSPECIFIED.)
GEOMETRIC_REPRESENTATION_ITEM()
RATIONAL_B_SPLINE_SURFACE(((0.996504189652446,0.998109554471267,1.,0.995737968897747,
0.992924952273132),(0.996504189652447,0.998109554471267,1.,0.995737968897747,
0.992924952273132)))
REPRESENTATION_ITEM('')
SURFACE()
);
#1516=(
BOUNDED_SURFACE()
B_SPLINE_SURFACE(1,2,((#119426,#119427,#119428),(#119429,#119430,#119431)),
 .UNSPECIFIED.,.F.,.F.,.F.)
B_SPLINE_SURFACE_WITH_KNOTS((2,2),(3,3),(0.710192959008364,1.),(0.435775021682622,
0.453027768259468),.UNSPECIFIED.)
GEOMETRIC_REPRESENTATION_ITEM()
RATIONAL_B_SPLINE_SURFACE(((0.995452950231063,0.990618550266715,0.988709602819327),
(0.995452950231063,0.990618550266715,0.988709602819327)))
REPRESENTATION_ITEM('')
SURFACE()
);
#1517=(
BOUNDED_SURFACE()
B_SPLINE_SURFACE(1,2,((#119440,#119441,#119442,#119443,#119444),(#119445,
#119446,#119447,#119448,#119449)),.UNSPECIFIED.,.F.,.F.,.F.)
B_SPLINE_SURFACE_WITH_KNOTS((2,2),(3,2,3),(0.710318915640008,1.),(0.280328542633766,
0.285714285714286,0.297856505190615),.UNSPECIFIED.)
GEOMETRIC_REPRESENTATION_ITEM()
RATIONAL_B_SPLINE_SURFACE(((0.996504189652447,0.998109554471267,1.,0.995737968897747,
0.992924952273131),(0.996504189652447,0.998109554471267,1.,0.995737968897747,
0.992924952273131)))
REPRESENTATION_ITEM('')
SURFACE()
);
#1518=(
BOUNDED_SURFACE()
B_SPLINE_SURFACE(1,2,((#119460,#119461,#119462),(#119463,#119464,#119465)),
 .UNSPECIFIED.,.F.,.F.,.F.)
B_SPLINE_SURFACE_WITH_KNOTS((2,2),(3,3),(0.710192959007759,1.),(0.435775021682136,
0.453027768259471),.UNSPECIFIED.)
GEOMETRIC_REPRESENTATION_ITEM()
RATIONAL_B_SPLINE_SURFACE(((0.995452950231336,0.990618550266768,0.988709602819327),
(0.995452950231336,0.990618550266768,0.988709602819327)))
REPRESENTATION_ITEM('')
SURFACE()
);
#1519=(
BOUNDED_SURFACE()
B_SPLINE_SURFACE(1,2,((#119474,#119475,#119476,#119477,#119478),(#119479,
#119480,#119481,#119482,#119483)),.UNSPECIFIED.,.F.,.F.,.F.)
B_SPLINE_SURFACE_WITH_KNOTS((2,2),(3,2,3),(0.710318915639399,1.),(0.280328542633766,
0.285714285714286,0.297856505190615),.UNSPECIFIED.)
GEOMETRIC_REPRESENTATION_ITEM()
RATIONAL_B_SPLINE_SURFACE(((0.996504189652447,0.998109554471267,1.,0.995737968897747,
0.992924952273131),(0.996504189652447,0.998109554471267,1.,0.995737968897747,
0.992924952273131)))
REPRESENTATION_ITEM('')
SURFACE()
);
#1520=(
BOUNDED_SURFACE()
B_SPLINE_SURFACE(1,2,((#119494,#119495,#119496),(#119497,#119498,#119499)),
 .UNSPECIFIED.,.F.,.F.,.F.)
B_SPLINE_SURFACE_WITH_KNOTS((2,2),(3,3),(0.710192959008366,1.),(0.435775021682621,
0.453027768259468),.UNSPECIFIED.)
GEOMETRIC_REPRESENTATION_ITEM()
RATIONAL_B_SPLINE_SURFACE(((0.995452950231064,0.990618550266715,0.988709602819327),
(0.995452950231064,0.990618550266715,0.988709602819327)))
REPRESENTATION_ITEM('')
SURFACE()
);
#1521=(
BOUNDED_SURFACE()
B_SPLINE_SURFACE(1,2,((#119508,#119509,#119510,#119511,#119512),(#119513,
#119514,#119515,#119516,#119517)),.UNSPECIFIED.,.F.,.F.,.F.)
B_SPLINE_SURFACE_WITH_KNOTS((2,2),(3,2,3),(0.710318915640004,1.),(0.280328542633766,
0.285714285714286,0.297856505190615),.UNSPECIFIED.)
GEOMETRIC_REPRESENTATION_ITEM()
RATIONAL_B_SPLINE_SURFACE(((0.996504189652447,0.998109554471267,1.,0.995737968897746,
0.992924952273131),(0.996504189652447,0.998109554471267,1.,0.995737968897746,
0.992924952273131)))
REPRESENTATION_ITEM('')
SURFACE()
);
#1522=(
BOUNDED_SURFACE()
B_SPLINE_SURFACE(1,2,((#119528,#119529,#119530),(#119531,#119532,#119533)),
 .UNSPECIFIED.,.F.,.F.,.F.)
B_SPLINE_SURFACE_WITH_KNOTS((2,2),(3,3),(0.710192959008342,1.),(0.435775021682587,
0.453027768259468),.UNSPECIFIED.)
GEOMETRIC_REPRESENTATION_ITEM()
RATIONAL_B_SPLINE_SURFACE(((0.995452950231083,0.990618550266718,0.988709602819327),
(0.995452950231083,0.990618550266718,0.988709602819327)))
REPRESENTATION_ITEM('')
SURFACE()
);
#1523=(
BOUNDED_SURFACE()
B_SPLINE_SURFACE(1,2,((#119542,#119543,#119544,#119545,#119546),(#119547,
#119548,#119549,#119550,#119551)),.UNSPECIFIED.,.F.,.F.,.F.)
B_SPLINE_SURFACE_WITH_KNOTS((2,2),(3,2,3),(0.710318915639979,1.),(0.280328542633766,
0.285714285714286,0.297856505190616),.UNSPECIFIED.)
GEOMETRIC_REPRESENTATION_ITEM()
RATIONAL_B_SPLINE_SURFACE(((0.996504189652447,0.998109554471267,1.,0.995737968897746,
0.992924952273131),(0.996504189652447,0.998109554471267,1.,0.995737968897746,
0.992924952273131)))
REPRESENTATION_ITEM('')
SURFACE()
);
#1524=(
BOUNDED_SURFACE()
B_SPLINE_SURFACE(1,2,((#119562,#119563,#119564),(#119565,#119566,#119567)),
 .UNSPECIFIED.,.F.,.F.,.F.)
B_SPLINE_SURFACE_WITH_KNOTS((2,2),(3,3),(0.710192959008342,1.),(0.435775021682621,
0.453027768259468),.UNSPECIFIED.)
GEOMETRIC_REPRESENTATION_ITEM()
RATIONAL_B_SPLINE_SURFACE(((0.995452950231064,0.990618550266715,0.988709602819327),
(0.995452950231064,0.990618550266715,0.988709602819327)))
REPRESENTATION_ITEM('')
SURFACE()
);
#1525=(
BOUNDED_SURFACE()
B_SPLINE_SURFACE(1,2,((#119576,#119577,#119578,#119579,#119580),(#119581,
#119582,#119583,#119584,#119585)),.UNSPECIFIED.,.F.,.F.,.F.)
B_SPLINE_SURFACE_WITH_KNOTS((2,2),(3,2,3),(0.710318915639981,1.),(0.280328542633766,
0.285714285714286,0.297856505190615),.UNSPECIFIED.)
GEOMETRIC_REPRESENTATION_ITEM()
RATIONAL_B_SPLINE_SURFACE(((0.996504189652447,0.998109554471267,1.,0.995737968897746,
0.992924952273131),(0.996504189652447,0.998109554471267,1.,0.995737968897746,
0.992924952273131)))
REPRESENTATION_ITEM('')
SURFACE()
);
#1526=(
BOUNDED_SURFACE()
B_SPLINE_SURFACE(1,2,((#119596,#119597,#119598),(#119599,#119600,#119601)),
 .UNSPECIFIED.,.F.,.F.,.F.)
B_SPLINE_SURFACE_WITH_KNOTS((2,2),(3,3),(0.710192959007979,1.),(0.435775021682622,
0.453027768259469),.UNSPECIFIED.)
GEOMETRIC_REPRESENTATION_ITEM()
RATIONAL_B_SPLINE_SURFACE(((0.995452950231063,0.990618550266714,0.988709602819327),
(0.995452950231063,0.990618550266714,0.988709602819327)))
REPRESENTATION_ITEM('')
SURFACE()
);
#1527=(
BOUNDED_SURFACE()
B_SPLINE_SURFACE(1,2,((#119610,#119611,#119612,#119613,#119614),(#119615,
#119616,#119617,#119618,#119619)),.UNSPECIFIED.,.F.,.F.,.F.)
B_SPLINE_SURFACE_WITH_KNOTS((2,2),(3,2,3),(0.710318915639623,1.),(0.280328542633765,
0.285714285714286,0.297856505190614),.UNSPECIFIED.)
GEOMETRIC_REPRESENTATION_ITEM()
RATIONAL_B_SPLINE_SURFACE(((0.996504189652446,0.998109554471267,1.,0.995737968897747,
0.992924952273132),(0.996504189652446,0.998109554471267,1.,0.995737968897747,
0.992924952273132)))
REPRESENTATION_ITEM('')
SURFACE()
);
#1528=(
BOUNDED_SURFACE()
B_SPLINE_SURFACE(1,2,((#119630,#119631,#119632),(#119633,#119634,#119635)),
 .UNSPECIFIED.,.F.,.F.,.F.)
B_SPLINE_SURFACE_WITH_KNOTS((2,2),(3,3),(0.,0.289681084359915),(0.228780950825311,
0.245954053070909),.UNSPECIFIED.)
GEOMETRIC_REPRESENTATION_ITEM()
RATIONAL_B_SPLINE_SURFACE(((0.991889110260683,0.988307723348179,0.987624841600687),
(0.991889110260683,0.988307723348179,0.987624841600687)))
REPRESENTATION_ITEM('')
SURFACE()
);
#1529=(
BOUNDED_SURFACE()
B_SPLINE_SURFACE(1,2,((#119648,#119649,#119650,#119651,#119652),(#119653,
#119654,#119655,#119656,#119657)),.UNSPECIFIED.,.F.,.F.,.F.)
B_SPLINE_SURFACE_WITH_KNOTS((2,2),(3,2,3),(0.,0.289807040991556),(0.487259899888157,
0.5,0.504824515313955),.UNSPECIFIED.)
GEOMETRIC_REPRESENTATION_ITEM()
RATIONAL_B_SPLINE_SURFACE(((0.992651440660745,0.995528107276569,1.,0.998306550597157,
0.996841863226483),(0.992651440660745,0.995528107276569,1.,0.998306550597157,
0.996841863226483)))
REPRESENTATION_ITEM('')
SURFACE()
);
#1530=(
BOUNDED_SURFACE()
B_SPLINE_SURFACE(1,2,((#119668,#119669,#119670),(#119671,#119672,#119673)),
 .UNSPECIFIED.,.F.,.F.,.F.)
B_SPLINE_SURFACE_WITH_KNOTS((2,2),(3,3),(0.,0.289681084359919),(0.228780950825311,
0.245954053070909),.UNSPECIFIED.)
GEOMETRIC_REPRESENTATION_ITEM()
RATIONAL_B_SPLINE_SURFACE(((0.991889110260684,0.988307723348179,0.987624841600686),
(0.991889110260683,0.988307723348179,0.987624841600686)))
REPRESENTATION_ITEM('')
SURFACE()
);
#1531=(
BOUNDED_SURFACE()
B_SPLINE_SURFACE(1,2,((#119686,#119687,#119688,#119689,#119690),(#119691,
#119692,#119693,#119694,#119695)),.UNSPECIFIED.,.F.,.F.,.F.)
B_SPLINE_SURFACE_WITH_KNOTS((2,2),(3,2,3),(0.,0.289807040991562),(0.487259899888158,
0.5,0.504824515313955),.UNSPECIFIED.)
GEOMETRIC_REPRESENTATION_ITEM()
RATIONAL_B_SPLINE_SURFACE(((0.992651440660745,0.995528107276569,1.,0.998306550597157,
0.996841863226483),(0.992651440660745,0.995528107276569,1.,0.998306550597157,
0.996841863226483)))
REPRESENTATION_ITEM('')
SURFACE()
);
#1532=(
BOUNDED_SURFACE()
B_SPLINE_SURFACE(1,2,((#119706,#119707,#119708),(#119709,#119710,#119711)),
 .UNSPECIFIED.,.F.,.F.,.F.)
B_SPLINE_SURFACE_WITH_KNOTS((2,2),(3,3),(0.,0.289681084359922),(0.228780950825753,
0.245954053070909),.UNSPECIFIED.)
GEOMETRIC_REPRESENTATION_ITEM()
RATIONAL_B_SPLINE_SURFACE(((0.991889110260499,0.988307723348161,0.987624841600687),
(0.991889110260499,0.988307723348161,0.987624841600687)))
REPRESENTATION_ITEM('')
SURFACE()
);
#1533=(
BOUNDED_SURFACE()
B_SPLINE_SURFACE(1,2,((#119724,#119725,#119726,#119727,#119728),(#119729,
#119730,#119731,#119732,#119733)),.UNSPECIFIED.,.F.,.F.,.F.)
B_SPLINE_SURFACE_WITH_KNOTS((2,2),(3,2,3),(0.,0.289807040991561),(0.487259899888157,
0.5,0.504824515313955),.UNSPECIFIED.)
GEOMETRIC_REPRESENTATION_ITEM()
RATIONAL_B_SPLINE_SURFACE(((0.992651440660745,0.995528107276569,1.,0.998306550597157,
0.996841863226483),(0.992651440660745,0.995528107276569,1.,0.998306550597157,
0.996841863226483)))
REPRESENTATION_ITEM('')
SURFACE()
);
#1534=(
BOUNDED_SURFACE()
B_SPLINE_SURFACE(1,2,((#119744,#119745,#119746),(#119747,#119748,#119749)),
 .UNSPECIFIED.,.F.,.F.,.F.)
B_SPLINE_SURFACE_WITH_KNOTS((2,2),(3,3),(0.,0.289681084359919),(0.228780950825753,
0.245954053070909),.UNSPECIFIED.)
GEOMETRIC_REPRESENTATION_ITEM()
RATIONAL_B_SPLINE_SURFACE(((0.991889110260499,0.988307723348161,0.987624841600687),
(0.991889110260499,0.988307723348161,0.987624841600687)))
REPRESENTATION_ITEM('')
SURFACE()
);
#1535=(
BOUNDED_SURFACE()
B_SPLINE_SURFACE(1,2,((#119762,#119763,#119764,#119765,#119766),(#119767,
#119768,#119769,#119770,#119771)),.UNSPECIFIED.,.F.,.F.,.F.)
B_SPLINE_SURFACE_WITH_KNOTS((2,2),(3,2,3),(0.,0.289807040992138),(0.487259899888158,
0.5,0.504824515313955),.UNSPECIFIED.)
GEOMETRIC_REPRESENTATION_ITEM()
RATIONAL_B_SPLINE_SURFACE(((0.992651440660745,0.995528107276569,1.,0.998306550597157,
0.996841863226483),(0.992651440660745,0.995528107276569,1.,0.998306550597157,
0.996841863226483)))
REPRESENTATION_ITEM('')
SURFACE()
);
#1536=(
BOUNDED_SURFACE()
B_SPLINE_SURFACE(1,2,((#119782,#119783,#119784),(#119785,#119786,#119787)),
 .UNSPECIFIED.,.F.,.F.,.F.)
B_SPLINE_SURFACE_WITH_KNOTS((2,2),(3,3),(0.,0.289681084359922),(0.228780950825753,
0.245954053070909),.UNSPECIFIED.)
GEOMETRIC_REPRESENTATION_ITEM()
RATIONAL_B_SPLINE_SURFACE(((0.991889110260499,0.988307723348161,0.987624841600687),
(0.991889110260499,0.988307723348161,0.987624841600687)))
REPRESENTATION_ITEM('')
SURFACE()
);
#1537=(
BOUNDED_SURFACE()
B_SPLINE_SURFACE(1,2,((#119800,#119801,#119802,#119803,#119804),(#119805,
#119806,#119807,#119808,#119809)),.UNSPECIFIED.,.F.,.F.,.F.)
B_SPLINE_SURFACE_WITH_KNOTS((2,2),(3,2,3),(0.,0.28980704099156),(0.487259899888158,
0.5,0.504824515313955),.UNSPECIFIED.)
GEOMETRIC_REPRESENTATION_ITEM()
RATIONAL_B_SPLINE_SURFACE(((0.992651440660745,0.995528107276569,1.,0.998306550597157,
0.996841863226483),(0.992651440660745,0.995528107276569,1.,0.998306550597157,
0.996841863226483)))
REPRESENTATION_ITEM('')
SURFACE()
);
#1538=(
BOUNDED_SURFACE()
B_SPLINE_SURFACE(1,2,((#119820,#119821,#119822),(#119823,#119824,#119825)),
 .UNSPECIFIED.,.F.,.F.,.F.)
B_SPLINE_SURFACE_WITH_KNOTS((2,2),(3,3),(0.,0.289681084359924),(0.228780950825753,
0.245954053070909),.UNSPECIFIED.)
GEOMETRIC_REPRESENTATION_ITEM()
RATIONAL_B_SPLINE_SURFACE(((0.991889110260499,0.988307723348161,0.987624841600687),
(0.991889110260499,0.988307723348161,0.987624841600687)))
REPRESENTATION_ITEM('')
SURFACE()
);
#1539=(
BOUNDED_SURFACE()
B_SPLINE_SURFACE(1,2,((#119838,#119839,#119840,#119841,#119842),(#119843,
#119844,#119845,#119846,#119847)),.UNSPECIFIED.,.F.,.F.,.F.)
B_SPLINE_SURFACE_WITH_KNOTS((2,2),(3,2,3),(0.,0.289807040992146),(0.487259899888158,
0.5,0.504824515313955),.UNSPECIFIED.)
GEOMETRIC_REPRESENTATION_ITEM()
RATIONAL_B_SPLINE_SURFACE(((0.992651440660745,0.995528107276569,1.,0.998306550597157,
0.996841863226483),(0.992651440660745,0.995528107276569,1.,0.998306550597157,
0.996841863226483)))
REPRESENTATION_ITEM('')
SURFACE()
);
#1540=(
BOUNDED_SURFACE()
B_SPLINE_SURFACE(1,2,((#119858,#119859,#119860),(#119861,#119862,#119863)),
 .UNSPECIFIED.,.F.,.F.,.F.)
B_SPLINE_SURFACE_WITH_KNOTS((2,2),(3,3),(0.,0.289681084359919),(0.228780950825753,
0.245954053070909),.UNSPECIFIED.)
GEOMETRIC_REPRESENTATION_ITEM()
RATIONAL_B_SPLINE_SURFACE(((0.991889110260499,0.988307723348161,0.987624841600687),
(0.991889110260499,0.988307723348161,0.987624841600687)))
REPRESENTATION_ITEM('')
SURFACE()
);
#1541=(
BOUNDED_SURFACE()
B_SPLINE_SURFACE(1,2,((#119876,#119877,#119878,#119879,#119880),(#119881,
#119882,#119883,#119884,#119885)),.UNSPECIFIED.,.F.,.F.,.F.)
B_SPLINE_SURFACE_WITH_KNOTS((2,2),(3,2,3),(0.,0.28980704099164),(0.487259899888159,
0.5,0.504824515313955),.UNSPECIFIED.)
GEOMETRIC_REPRESENTATION_ITEM()
RATIONAL_B_SPLINE_SURFACE(((0.992651440660745,0.99552810727657,1.,0.998306550597157,
0.996841863226483),(0.992651440660745,0.99552810727657,1.,0.998306550597157,
0.996841863226483)))
REPRESENTATION_ITEM('')
SURFACE()
);
#1542=(
BOUNDED_SURFACE()
B_SPLINE_SURFACE(1,2,((#119896,#119897,#119898),(#119899,#119900,#119901)),
 .UNSPECIFIED.,.F.,.F.,.F.)
B_SPLINE_SURFACE_WITH_KNOTS((2,2),(3,3),(0.,0.289681084359925),(0.228780950825752,
0.245954053070908),.UNSPECIFIED.)
GEOMETRIC_REPRESENTATION_ITEM()
RATIONAL_B_SPLINE_SURFACE(((0.991889110260499,0.988307723348161,0.987624841600687),
(0.991889110260499,0.988307723348161,0.987624841600687)))
REPRESENTATION_ITEM('')
SURFACE()
);
#1543=(
BOUNDED_SURFACE()
B_SPLINE_SURFACE(1,2,((#119914,#119915,#119916,#119917,#119918),(#119919,
#119920,#119921,#119922,#119923)),.UNSPECIFIED.,.F.,.F.,.F.)
B_SPLINE_SURFACE_WITH_KNOTS((2,2),(3,2,3),(0.,0.289807040991634),(0.487259899888159,
0.5,0.504824515313956),.UNSPECIFIED.)
GEOMETRIC_REPRESENTATION_ITEM()
RATIONAL_B_SPLINE_SURFACE(((0.992651440660745,0.99552810727657,1.,0.998306550597157,
0.996841863226482),(0.992651440660745,0.99552810727657,1.,0.998306550597157,
0.996841863226482)))
REPRESENTATION_ITEM('')
SURFACE()
);
#1544=(
BOUNDED_SURFACE()
B_SPLINE_SURFACE(1,2,((#119934,#119935,#119936),(#119937,#119938,#119939)),
 .UNSPECIFIED.,.F.,.F.,.F.)
B_SPLINE_SURFACE_WITH_KNOTS((2,2),(3,3),(0.,0.289681084361937),(0.22878095082531,
0.245954053070933),.UNSPECIFIED.)
GEOMETRIC_REPRESENTATION_ITEM()
RATIONAL_B_SPLINE_SURFACE(((0.991889110260684,0.988307723348174,0.987624841600685),
(0.991889110260684,0.988307723348174,0.987624841600685)))
REPRESENTATION_ITEM('')
SURFACE()
);
#1545=(
BOUNDED_SURFACE()
B_SPLINE_SURFACE(1,2,((#119952,#119953,#119954,#119955,#119956),(#119957,
#119958,#119959,#119960,#119961)),.UNSPECIFIED.,.F.,.F.,.F.)
B_SPLINE_SURFACE_WITH_KNOTS((2,2),(3,2,3),(0.,0.289807040992233),(0.487259899888159,
0.5,0.504824515313956),.UNSPECIFIED.)
GEOMETRIC_REPRESENTATION_ITEM()
RATIONAL_B_SPLINE_SURFACE(((0.992651440660745,0.99552810727657,1.,0.998306550597157,
0.996841863226482),(0.992651440660745,0.99552810727657,1.,0.998306550597157,
0.996841863226482)))
REPRESENTATION_ITEM('')
SURFACE()
);
#1546=(
BOUNDED_SURFACE()
B_SPLINE_SURFACE(1,2,((#119972,#119973,#119974),(#119975,#119976,#119977)),
 .UNSPECIFIED.,.F.,.F.,.F.)
B_SPLINE_SURFACE_WITH_KNOTS((2,2),(3,3),(0.,0.289681084359923),(0.228780950825308,
0.245954053070908),.UNSPECIFIED.)
GEOMETRIC_REPRESENTATION_ITEM()
RATIONAL_B_SPLINE_SURFACE(((0.991889110260685,0.988307723348179,0.987624841600687),
(0.991889110260685,0.988307723348179,0.987624841600687)))
REPRESENTATION_ITEM('')
SURFACE()
);
#1547=(
BOUNDED_SURFACE()
B_SPLINE_SURFACE(1,2,((#119990,#119991,#119992,#119993,#119994),(#119995,
#119996,#119997,#119998,#119999)),.UNSPECIFIED.,.F.,.F.,.F.)
B_SPLINE_SURFACE_WITH_KNOTS((2,2),(3,2,3),(0.,0.289807040991645),(0.487259899888159,
0.5,0.504824515313956),.UNSPECIFIED.)
GEOMETRIC_REPRESENTATION_ITEM()
RATIONAL_B_SPLINE_SURFACE(((0.992651440660745,0.99552810727657,1.,0.998306550597157,
0.996841863226482),(0.992651440660745,0.99552810727657,1.,0.998306550597157,
0.996841863226482)))
REPRESENTATION_ITEM('')
SURFACE()
);
#1548=(
BOUNDED_SURFACE()
B_SPLINE_SURFACE(1,2,((#120010,#120011,#120012),(#120013,#120014,#120015)),
 .UNSPECIFIED.,.F.,.F.,.F.)
B_SPLINE_SURFACE_WITH_KNOTS((2,2),(3,3),(0.,0.289681084359923),(0.228780950825302,
0.245954053070908),.UNSPECIFIED.)
GEOMETRIC_REPRESENTATION_ITEM()
RATIONAL_B_SPLINE_SURFACE(((0.991889110260687,0.98830772334818,0.987624841600687),
(0.991889110260687,0.98830772334818,0.987624841600687)))
REPRESENTATION_ITEM('')
SURFACE()
);
#1549=(
BOUNDED_SURFACE()
B_SPLINE_SURFACE(1,2,((#120028,#120029,#120030,#120031,#120032),(#120033,
#120034,#120035,#120036,#120037)),.UNSPECIFIED.,.F.,.F.,.F.)
B_SPLINE_SURFACE_WITH_KNOTS((2,2),(3,2,3),(0.,0.289807040992145),(0.487259899888159,
0.5,0.504824515313956),.UNSPECIFIED.)
GEOMETRIC_REPRESENTATION_ITEM()
RATIONAL_B_SPLINE_SURFACE(((0.992651440660745,0.99552810727657,1.,0.998306550597157,
0.996841863226482),(0.992651440660745,0.99552810727657,1.,0.998306550597157,
0.996841863226482)))
REPRESENTATION_ITEM('')
SURFACE()
);
#1550=(
BOUNDED_SURFACE()
B_SPLINE_SURFACE(1,2,((#120048,#120049,#120050),(#120051,#120052,#120053)),
 .UNSPECIFIED.,.F.,.F.,.F.)
B_SPLINE_SURFACE_WITH_KNOTS((2,2),(3,3),(0.,0.289681084359918),(0.228780950825752,
0.245954053070908),.UNSPECIFIED.)
GEOMETRIC_REPRESENTATION_ITEM()
RATIONAL_B_SPLINE_SURFACE(((0.991889110260499,0.988307723348161,0.987624841600687),
(0.991889110260499,0.988307723348162,0.987624841600687)))
REPRESENTATION_ITEM('')
SURFACE()
);
#1551=(
BOUNDED_SURFACE()
B_SPLINE_SURFACE(1,2,((#120066,#120067,#120068,#120069,#120070),(#120071,
#120072,#120073,#120074,#120075)),.UNSPECIFIED.,.F.,.F.,.F.)
B_SPLINE_SURFACE_WITH_KNOTS((2,2),(3,2,3),(0.,0.289807040991646),(0.487259899888158,
0.5,0.504824515313956),.UNSPECIFIED.)
GEOMETRIC_REPRESENTATION_ITEM()
RATIONAL_B_SPLINE_SURFACE(((0.992651440660745,0.99552810727657,1.,0.998306550597157,
0.996841863226482),(0.992651440660745,0.99552810727657,1.,0.998306550597157,
0.996841863226482)))
REPRESENTATION_ITEM('')
SURFACE()
);
#1552=(
BOUNDED_SURFACE()
B_SPLINE_SURFACE(1,2,((#120086,#120087,#120088),(#120089,#120090,#120091)),
 .UNSPECIFIED.,.F.,.F.,.F.)
B_SPLINE_SURFACE_WITH_KNOTS((2,2),(3,3),(0.,0.289681084359922),(0.228780950825302,
0.245954053070908),.UNSPECIFIED.)
GEOMETRIC_REPRESENTATION_ITEM()
RATIONAL_B_SPLINE_SURFACE(((0.991889110260687,0.98830772334818,0.987624841600687),
(0.991889110260687,0.98830772334818,0.987624841600687)))
REPRESENTATION_ITEM('')
SURFACE()
);
#1553=(
BOUNDED_SURFACE()
B_SPLINE_SURFACE(1,2,((#120104,#120105,#120106,#120107,#120108),(#120109,
#120110,#120111,#120112,#120113)),.UNSPECIFIED.,.F.,.F.,.F.)
B_SPLINE_SURFACE_WITH_KNOTS((2,2),(3,2,3),(0.,0.289807040992144),(0.487259899888159,
0.5,0.504824515313956),.UNSPECIFIED.)
GEOMETRIC_REPRESENTATION_ITEM()
RATIONAL_B_SPLINE_SURFACE(((0.992651440660745,0.99552810727657,1.,0.998306550597157,
0.996841863226482),(0.992651440660745,0.99552810727657,1.,0.998306550597157,
0.996841863226482)))
REPRESENTATION_ITEM('')
SURFACE()
);
#1554=(
BOUNDED_SURFACE()
B_SPLINE_SURFACE(1,2,((#120124,#120125,#120126),(#120127,#120128,#120129)),
 .UNSPECIFIED.,.F.,.F.,.F.)
B_SPLINE_SURFACE_WITH_KNOTS((2,2),(3,3),(0.,0.289681084359919),(0.228780950825305,
0.245954053070908),.UNSPECIFIED.)
GEOMETRIC_REPRESENTATION_ITEM()
RATIONAL_B_SPLINE_SURFACE(((0.991889110260686,0.988307723348179,0.987624841600687),
(0.991889110260686,0.988307723348179,0.987624841600687)))
REPRESENTATION_ITEM('')
SURFACE()
);
#1555=(
BOUNDED_SURFACE()
B_SPLINE_SURFACE(1,2,((#120142,#120143,#120144,#120145,#120146),(#120147,
#120148,#120149,#120150,#120151)),.UNSPECIFIED.,.F.,.F.,.F.)
B_SPLINE_SURFACE_WITH_KNOTS((2,2),(3,2,3),(0.,0.289807040991922),(0.487259899888159,
0.5,0.504824515313956),.UNSPECIFIED.)
GEOMETRIC_REPRESENTATION_ITEM()
RATIONAL_B_SPLINE_SURFACE(((0.992651440660745,0.99552810727657,1.,0.998306550597157,
0.996841863226482),(0.992651440660745,0.99552810727657,1.,0.998306550597157,
0.996841863226482)))
REPRESENTATION_ITEM('')
SURFACE()
);
#1556=(
BOUNDED_SURFACE()
B_SPLINE_SURFACE(1,2,((#120162,#120163,#120164),(#120165,#120166,#120167)),
 .UNSPECIFIED.,.F.,.F.,.F.)
B_SPLINE_SURFACE_WITH_KNOTS((2,2),(3,3),(0.,0.28968108435992),(0.228780950825309,
0.245954053070908),.UNSPECIFIED.)
GEOMETRIC_REPRESENTATION_ITEM()
RATIONAL_B_SPLINE_SURFACE(((0.991889110260684,0.988307723348179,0.987624841600687),
(0.991889110260684,0.988307723348179,0.987624841600687)))
REPRESENTATION_ITEM('')
SURFACE()
);
#1557=(
BOUNDED_SURFACE()
B_SPLINE_SURFACE(1,2,((#120180,#120181,#120182,#120183,#120184),(#120185,
#120186,#120187,#120188,#120189)),.UNSPECIFIED.,.F.,.F.,.F.)
B_SPLINE_SURFACE_WITH_KNOTS((2,2),(3,2,3),(0.,0.289807040992964),(0.487259899888159,
0.5,0.504824515313956),.UNSPECIFIED.)
GEOMETRIC_REPRESENTATION_ITEM()
RATIONAL_B_SPLINE_SURFACE(((0.992651440660745,0.99552810727657,1.,0.998306550597157,
0.996841863226482),(0.992651440660745,0.99552810727657,1.,0.998306550597157,
0.996841863226482)))
REPRESENTATION_ITEM('')
SURFACE()
);
#1558=(
BOUNDED_SURFACE()
B_SPLINE_SURFACE(1,2,((#120200,#120201,#120202),(#120203,#120204,#120205)),
 .UNSPECIFIED.,.F.,.F.,.F.)
B_SPLINE_SURFACE_WITH_KNOTS((2,2),(3,3),(0.,0.289681084359923),(0.228780950825313,
0.245954053070908),.UNSPECIFIED.)
GEOMETRIC_REPRESENTATION_ITEM()
RATIONAL_B_SPLINE_SURFACE(((0.991889110260683,0.988307723348179,0.987624841600687),
(0.991889110260683,0.988307723348179,0.987624841600687)))
REPRESENTATION_ITEM('')
SURFACE()
);
#1559=(
BOUNDED_SURFACE()
B_SPLINE_SURFACE(1,2,((#120218,#120219,#120220,#120221,#120222),(#120223,
#120224,#120225,#120226,#120227)),.UNSPECIFIED.,.F.,.F.,.F.)
B_SPLINE_SURFACE_WITH_KNOTS((2,2),(3,2,3),(0.,0.289807040991679),(0.487259899888159,
0.5,0.504824515313956),.UNSPECIFIED.)
GEOMETRIC_REPRESENTATION_ITEM()
RATIONAL_B_SPLINE_SURFACE(((0.992651440660745,0.99552810727657,1.,0.998306550597157,
0.996841863226482),(0.992651440660745,0.99552810727657,1.,0.998306550597157,
0.996841863226482)))
REPRESENTATION_ITEM('')
SURFACE()
);
#1560=(
BOUNDED_SURFACE()
B_SPLINE_SURFACE(1,2,((#120238,#120239,#120240),(#120241,#120242,#120243)),
 .UNSPECIFIED.,.F.,.F.,.F.)
B_SPLINE_SURFACE_WITH_KNOTS((2,2),(3,3),(0.,0.289681084359926),(0.228780950825752,
0.245954053070908),.UNSPECIFIED.)
GEOMETRIC_REPRESENTATION_ITEM()
RATIONAL_B_SPLINE_SURFACE(((0.991889110260499,0.988307723348161,0.987624841600687),
(0.991889110260499,0.988307723348161,0.987624841600687)))
REPRESENTATION_ITEM('')
SURFACE()
);
#1561=(
BOUNDED_SURFACE()
B_SPLINE_SURFACE(1,2,((#120256,#120257,#120258,#120259,#120260),(#120261,
#120262,#120263,#120264,#120265)),.UNSPECIFIED.,.F.,.F.,.F.)
B_SPLINE_SURFACE_WITH_KNOTS((2,2),(3,2,3),(0.,0.289807040991562),(0.487259899888159,
0.5,0.504824515313956),.UNSPECIFIED.)
GEOMETRIC_REPRESENTATION_ITEM()
RATIONAL_B_SPLINE_SURFACE(((0.992651440660745,0.99552810727657,1.,0.998306550597157,
0.996841863226482),(0.992651440660745,0.99552810727657,1.,0.998306550597157,
0.996841863226482)))
REPRESENTATION_ITEM('')
SURFACE()
);
#1562=(
BOUNDED_SURFACE()
B_SPLINE_SURFACE(1,2,((#120276,#120277,#120278),(#120279,#120280,#120281)),
 .UNSPECIFIED.,.F.,.F.,.F.)
B_SPLINE_SURFACE_WITH_KNOTS((2,2),(3,3),(0.,0.289681084359922),(0.22878095082551,
0.245954053070908),.UNSPECIFIED.)
GEOMETRIC_REPRESENTATION_ITEM()
RATIONAL_B_SPLINE_SURFACE(((0.9918891102606,0.988307723348171,0.987624841600687),
(0.9918891102606,0.988307723348171,0.987624841600687)))
REPRESENTATION_ITEM('')
SURFACE()
);
#1563=(
BOUNDED_SURFACE()
B_SPLINE_SURFACE(1,2,((#120294,#120295,#120296,#120297,#120298),(#120299,
#120300,#120301,#120302,#120303)),.UNSPECIFIED.,.F.,.F.,.F.)
B_SPLINE_SURFACE_WITH_KNOTS((2,2),(3,2,3),(0.,0.289807040992201),(0.487259899888159,
0.5,0.504824515313956),.UNSPECIFIED.)
GEOMETRIC_REPRESENTATION_ITEM()
RATIONAL_B_SPLINE_SURFACE(((0.992651440660745,0.99552810727657,1.,0.998306550597157,
0.996841863226482),(0.992651440660745,0.99552810727657,1.,0.998306550597157,
0.996841863226482)))
REPRESENTATION_ITEM('')
SURFACE()
);
#1564=(
BOUNDED_SURFACE()
B_SPLINE_SURFACE(1,2,((#120314,#120315,#120316),(#120317,#120318,#120319)),
 .UNSPECIFIED.,.F.,.F.,.F.)
B_SPLINE_SURFACE_WITH_KNOTS((2,2),(3,3),(0.,0.289681084359927),(0.22878095082532,
0.245954053070908),.UNSPECIFIED.)
GEOMETRIC_REPRESENTATION_ITEM()
RATIONAL_B_SPLINE_SURFACE(((0.99188911026068,0.988307723348179,0.987624841600687),
(0.99188911026068,0.988307723348179,0.987624841600687)))
REPRESENTATION_ITEM('')
SURFACE()
);
#1565=(
BOUNDED_SURFACE()
B_SPLINE_SURFACE(1,2,((#120332,#120333,#120334,#120335,#120336),(#120337,
#120338,#120339,#120340,#120341)),.UNSPECIFIED.,.F.,.F.,.F.)
B_SPLINE_SURFACE_WITH_KNOTS((2,2),(3,2,3),(0.,0.289807040991564),(0.487259899888159,
0.5,0.504824515313681),.UNSPECIFIED.)
GEOMETRIC_REPRESENTATION_ITEM()
RATIONAL_B_SPLINE_SURFACE(((0.992651440660745,0.99552810727657,1.,0.998306550597253,
0.996841863226649),(0.992651440660745,0.99552810727657,1.,0.998306550597253,
0.996841863226649)))
REPRESENTATION_ITEM('')
SURFACE()
);
#1566=(
BOUNDED_SURFACE()
B_SPLINE_SURFACE(1,2,((#120352,#120353,#120354),(#120355,#120356,#120357)),
 .UNSPECIFIED.,.F.,.F.,.F.)
B_SPLINE_SURFACE_WITH_KNOTS((2,2),(3,3),(0.,0.289681084359927),(0.228780950825606,
0.245954053070908),.UNSPECIFIED.)
GEOMETRIC_REPRESENTATION_ITEM()
RATIONAL_B_SPLINE_SURFACE(((0.991889110260561,0.988307723348167,0.987624841600687),
(0.991889110260561,0.988307723348168,0.987624841600687)))
REPRESENTATION_ITEM('')
SURFACE()
);
#1567=(
BOUNDED_SURFACE()
B_SPLINE_SURFACE(1,2,((#120370,#120371,#120372,#120373,#120374),(#120375,
#120376,#120377,#120378,#120379)),.UNSPECIFIED.,.F.,.F.,.F.)
B_SPLINE_SURFACE_WITH_KNOTS((2,2),(3,2,3),(0.,0.289807040992693),(0.487259899888159,
0.5,0.504824515313956),.UNSPECIFIED.)
GEOMETRIC_REPRESENTATION_ITEM()
RATIONAL_B_SPLINE_SURFACE(((0.992651440660745,0.99552810727657,1.,0.998306550597157,
0.996841863226482),(0.992651440660745,0.99552810727657,1.,0.998306550597157,
0.996841863226482)))
REPRESENTATION_ITEM('')
SURFACE()
);
#1568=(
BOUNDED_SURFACE()
B_SPLINE_SURFACE(1,2,((#120390,#120391,#120392),(#120393,#120394,#120395)),
 .UNSPECIFIED.,.F.,.F.,.F.)
B_SPLINE_SURFACE_WITH_KNOTS((2,2),(3,3),(0.,0.289681084359929),(0.228780950825752,
0.245954053070908),.UNSPECIFIED.)
GEOMETRIC_REPRESENTATION_ITEM()
RATIONAL_B_SPLINE_SURFACE(((0.991889110260499,0.988307723348162,0.987624841600687),
(0.991889110260499,0.988307723348162,0.987624841600687)))
REPRESENTATION_ITEM('')
SURFACE()
);
#1569=(
BOUNDED_SURFACE()
B_SPLINE_SURFACE(1,2,((#120408,#120409,#120410,#120411,#120412),(#120413,
#120414,#120415,#120416,#120417)),.UNSPECIFIED.,.F.,.F.,.F.)
B_SPLINE_SURFACE_WITH_KNOTS((2,2),(3,2,3),(0.,0.289807040992531),(0.487259899888159,
0.5,0.504824515313956),.UNSPECIFIED.)
GEOMETRIC_REPRESENTATION_ITEM()
RATIONAL_B_SPLINE_SURFACE(((0.992651440660745,0.99552810727657,1.,0.998306550597157,
0.996841863226482),(0.992651440660745,0.99552810727657,1.,0.998306550597157,
0.996841863226482)))
REPRESENTATION_ITEM('')
SURFACE()
);
#1570=(
BOUNDED_SURFACE()
B_SPLINE_SURFACE(1,2,((#120428,#120429,#120430),(#120431,#120432,#120433)),
 .UNSPECIFIED.,.F.,.F.,.F.)
B_SPLINE_SURFACE_WITH_KNOTS((2,2),(3,3),(0.,0.289681084359926),(0.228780950825465,
0.245954053070908),.UNSPECIFIED.)
GEOMETRIC_REPRESENTATION_ITEM()
RATIONAL_B_SPLINE_SURFACE(((0.991889110260619,0.988307723348173,0.987624841600687),
(0.991889110260619,0.988307723348173,0.987624841600687)))
REPRESENTATION_ITEM('')
SURFACE()
);
#1571=(
BOUNDED_SURFACE()
B_SPLINE_SURFACE(1,2,((#120446,#120447,#120448,#120449,#120450),(#120451,
#120452,#120453,#120454,#120455)),.UNSPECIFIED.,.F.,.F.,.F.)
B_SPLINE_SURFACE_WITH_KNOTS((2,2),(3,2,3),(0.,0.289807040993255),(0.487259899888159,
0.5,0.504824515313827),.UNSPECIFIED.)
GEOMETRIC_REPRESENTATION_ITEM()
RATIONAL_B_SPLINE_SURFACE(((0.992651440660745,0.99552810727657,1.,0.998306550597202,
0.99684186322656),(0.992651440660745,0.99552810727657,1.,0.998306550597202,
0.99684186322656)))
REPRESENTATION_ITEM('')
SURFACE()
);
#1572=(
BOUNDED_SURFACE()
B_SPLINE_SURFACE(1,2,((#120466,#120467,#120468),(#120469,#120470,#120471)),
 .UNSPECIFIED.,.F.,.F.,.F.)
B_SPLINE_SURFACE_WITH_KNOTS((2,2),(3,3),(0.,0.289681084359919),(0.228780950825422,
0.245954053070908),.UNSPECIFIED.)
GEOMETRIC_REPRESENTATION_ITEM()
RATIONAL_B_SPLINE_SURFACE(((0.991889110260637,0.988307723348175,0.987624841600687),
(0.991889110260637,0.988307723348175,0.987624841600687)))
REPRESENTATION_ITEM('')
SURFACE()
);
#1573=(
BOUNDED_SURFACE()
B_SPLINE_SURFACE(1,2,((#120484,#120485,#120486,#120487,#120488),(#120489,
#120490,#120491,#120492,#120493)),.UNSPECIFIED.,.F.,.F.,.F.)
B_SPLINE_SURFACE_WITH_KNOTS((2,2),(3,2,3),(0.,0.289807040991761),(0.487259899888159,
0.5,0.504824515313794),.UNSPECIFIED.)
GEOMETRIC_REPRESENTATION_ITEM()
RATIONAL_B_SPLINE_SURFACE(((0.992651440660745,0.99552810727657,1.,0.998306550597214,
0.99684186322658),(0.992651440660745,0.99552810727657,1.,0.998306550597214,
0.99684186322658)))
REPRESENTATION_ITEM('')
SURFACE()
);
#1574=(
BOUNDED_SURFACE()
B_SPLINE_SURFACE(1,2,((#120504,#120505,#120506),(#120507,#120508,#120509)),
 .UNSPECIFIED.,.F.,.F.,.F.)
B_SPLINE_SURFACE_WITH_KNOTS((2,2),(3,3),(0.,0.28968108435992),(0.228780950825549,
0.245954053070908),.UNSPECIFIED.)
GEOMETRIC_REPRESENTATION_ITEM()
RATIONAL_B_SPLINE_SURFACE(((0.991889110260584,0.98830772334817,0.987624841600687),
(0.991889110260584,0.98830772334817,0.987624841600687)))
REPRESENTATION_ITEM('')
SURFACE()
);
#1575=(
BOUNDED_SURFACE()
B_SPLINE_SURFACE(1,2,((#120522,#120523,#120524,#120525,#120526),(#120527,
#120528,#120529,#120530,#120531)),.UNSPECIFIED.,.F.,.F.,.F.)
B_SPLINE_SURFACE_WITH_KNOTS((2,2),(3,2,3),(0.,0.289807040993054),(0.487259899888159,
0.5,0.504824515313847),.UNSPECIFIED.)
GEOMETRIC_REPRESENTATION_ITEM()
RATIONAL_B_SPLINE_SURFACE(((0.992651440660745,0.99552810727657,1.,0.998306550597195,
0.996841863226548),(0.992651440660745,0.99552810727657,1.,0.998306550597195,
0.996841863226548)))
REPRESENTATION_ITEM('')
SURFACE()
);
#1576=(
BOUNDED_SURFACE()
B_SPLINE_SURFACE(1,2,((#120542,#120543,#120544),(#120545,#120546,#120547)),
 .UNSPECIFIED.,.F.,.F.,.F.)
B_SPLINE_SURFACE_WITH_KNOTS((2,2),(3,3),(0.,0.289681084359929),(0.228780950825689,
0.245954053070908),.UNSPECIFIED.)
GEOMETRIC_REPRESENTATION_ITEM()
RATIONAL_B_SPLINE_SURFACE(((0.991889110260526,0.988307723348164,0.987624841600687),
(0.991889110260526,0.988307723348164,0.987624841600687)))
REPRESENTATION_ITEM('')
SURFACE()
);
#1577=(
BOUNDED_SURFACE()
B_SPLINE_SURFACE(1,2,((#120560,#120561,#120562,#120563,#120564),(#120565,
#120566,#120567,#120568,#120569)),.UNSPECIFIED.,.F.,.F.,.F.)
B_SPLINE_SURFACE_WITH_KNOTS((2,2),(3,2,3),(0.,0.289807040992802),(0.487259899888159,
0.5,0.504824515313924),.UNSPECIFIED.)
GEOMETRIC_REPRESENTATION_ITEM()
RATIONAL_B_SPLINE_SURFACE(((0.992651440660745,0.99552810727657,1.,0.998306550597168,
0.996841863226501),(0.992651440660745,0.99552810727657,1.,0.998306550597168,
0.996841863226501)))
REPRESENTATION_ITEM('')
SURFACE()
);
#1578=(
BOUNDED_SURFACE()
B_SPLINE_SURFACE(1,2,((#120580,#120581,#120582),(#120583,#120584,#120585)),
 .UNSPECIFIED.,.F.,.F.,.F.)
B_SPLINE_SURFACE_WITH_KNOTS((2,2),(3,3),(0.,0.289681084359935),(0.228780950825721,
0.245954053070908),.UNSPECIFIED.)
GEOMETRIC_REPRESENTATION_ITEM()
RATIONAL_B_SPLINE_SURFACE(((0.991889110260513,0.988307723348163,0.987624841600687),
(0.991889110260513,0.988307723348163,0.987624841600687)))
REPRESENTATION_ITEM('')
SURFACE()
);
#1579=(
BOUNDED_SURFACE()
B_SPLINE_SURFACE(1,2,((#120598,#120599,#120600,#120601,#120602),(#120603,
#120604,#120605,#120606,#120607)),.UNSPECIFIED.,.F.,.F.,.F.)
B_SPLINE_SURFACE_WITH_KNOTS((2,2),(3,2,3),(0.,0.289807040992555),(0.487259899888159,
0.5,0.50482451531395),.UNSPECIFIED.)
GEOMETRIC_REPRESENTATION_ITEM()
RATIONAL_B_SPLINE_SURFACE(((0.992651440660745,0.99552810727657,1.,0.998306550597159,
0.996841863226485),(0.992651440660745,0.99552810727657,1.,0.998306550597159,
0.996841863226485)))
REPRESENTATION_ITEM('')
SURFACE()
);
#1580=(
BOUNDED_SURFACE()
B_SPLINE_SURFACE(1,2,((#120618,#120619,#120620),(#120621,#120622,#120623)),
 .UNSPECIFIED.,.F.,.F.,.F.)
B_SPLINE_SURFACE_WITH_KNOTS((2,2),(3,3),(0.,0.289681084359928),(0.228780950825752,
0.245954053070908),.UNSPECIFIED.)
GEOMETRIC_REPRESENTATION_ITEM()
RATIONAL_B_SPLINE_SURFACE(((0.9918891102605,0.988307723348162,0.987624841600687),
(0.9918891102605,0.988307723348162,0.987624841600687)))
REPRESENTATION_ITEM('')
SURFACE()
);
#1581=(
BOUNDED_SURFACE()
B_SPLINE_SURFACE(1,2,((#120636,#120637,#120638,#120639,#120640),(#120641,
#120642,#120643,#120644,#120645)),.UNSPECIFIED.,.F.,.F.,.F.)
B_SPLINE_SURFACE_WITH_KNOTS((2,2),(3,2,3),(0.,0.289807040992489),(0.487259899888159,
0.5,0.504824515313956),.UNSPECIFIED.)
GEOMETRIC_REPRESENTATION_ITEM()
RATIONAL_B_SPLINE_SURFACE(((0.992651440660745,0.99552810727657,1.,0.998306550597157,
0.996841863226482),(0.992651440660745,0.99552810727657,1.,0.998306550597157,
0.996841863226482)))
REPRESENTATION_ITEM('')
SURFACE()
);
#1582=(
BOUNDED_SURFACE()
B_SPLINE_SURFACE(1,2,((#120656,#120657,#120658),(#120659,#120660,#120661)),
 .UNSPECIFIED.,.F.,.F.,.F.)
B_SPLINE_SURFACE_WITH_KNOTS((2,2),(3,3),(0.,0.289681084359923),(0.228780950825752,
0.245954053070909),.UNSPECIFIED.)
GEOMETRIC_REPRESENTATION_ITEM()
RATIONAL_B_SPLINE_SURFACE(((0.9918891102605,0.988307723348161,0.987624841600687),
(0.9918891102605,0.988307723348161,0.987624841600687)))
REPRESENTATION_ITEM('')
SURFACE()
);
#1583=(
BOUNDED_SURFACE()
B_SPLINE_SURFACE(1,2,((#120674,#120675,#120676,#120677,#120678),(#120679,
#120680,#120681,#120682,#120683)),.UNSPECIFIED.,.F.,.F.,.F.)
B_SPLINE_SURFACE_WITH_KNOTS((2,2),(3,2,3),(0.,0.289807040992803),(0.48725989988815,
0.5,0.504824515313956),.UNSPECIFIED.)
GEOMETRIC_REPRESENTATION_ITEM()
RATIONAL_B_SPLINE_SURFACE(((0.992651440660741,0.995528107276567,1.,0.998306550597157,
0.996841863226482),(0.992651440660741,0.995528107276567,1.,0.998306550597157,
0.996841863226482)))
REPRESENTATION_ITEM('')
SURFACE()
);
#1584=(
BOUNDED_SURFACE()
B_SPLINE_SURFACE(1,2,((#120694,#120695,#120696),(#120697,#120698,#120699)),
 .UNSPECIFIED.,.F.,.F.,.F.)
B_SPLINE_SURFACE_WITH_KNOTS((2,2),(3,3),(0.,0.289681084359922),(0.228780950825753,
0.245954053070908),.UNSPECIFIED.)
GEOMETRIC_REPRESENTATION_ITEM()
RATIONAL_B_SPLINE_SURFACE(((0.991889110260499,0.988307723348161,0.987624841600687),
(0.991889110260499,0.988307723348161,0.987624841600687)))
REPRESENTATION_ITEM('')
SURFACE()
);
#1585=(
BOUNDED_SURFACE()
B_SPLINE_SURFACE(1,2,((#120712,#120713,#120714,#120715,#120716),(#120717,
#120718,#120719,#120720,#120721)),.UNSPECIFIED.,.F.,.F.,.F.)
B_SPLINE_SURFACE_WITH_KNOTS((2,2),(3,2,3),(0.,0.28980704099156),(0.487259899888158,
0.5,0.504824515313955),.UNSPECIFIED.)
GEOMETRIC_REPRESENTATION_ITEM()
RATIONAL_B_SPLINE_SURFACE(((0.992651440660745,0.995528107276569,1.,0.998306550597157,
0.996841863226483),(0.992651440660745,0.995528107276569,1.,0.998306550597157,
0.996841863226483)))
REPRESENTATION_ITEM('')
SURFACE()
);
#1586=(
BOUNDED_SURFACE()
B_SPLINE_SURFACE(1,2,((#120732,#120733,#120734),(#120735,#120736,#120737)),
 .UNSPECIFIED.,.F.,.F.,.F.)
B_SPLINE_SURFACE_WITH_KNOTS((2,2),(3,3),(0.,0.289681084359934),(0.43567212259767,
0.452924869174518),.UNSPECIFIED.)
GEOMETRIC_REPRESENTATION_ITEM()
RATIONAL_B_SPLINE_SURFACE(((0.995510721093622,0.990658873102333,0.988732477628005),
(0.995510721093622,0.990658873102333,0.988732477628005)))
REPRESENTATION_ITEM('')
SURFACE()
);
#1587=(
BOUNDED_SURFACE()
B_SPLINE_SURFACE(1,2,((#120748,#120749,#120750,#120751,#120752,#120753,
#120754),(#120755,#120756,#120757,#120758,#120759,#120760,#120761)),
 .UNSPECIFIED.,.F.,.F.,.F.)
B_SPLINE_SURFACE_WITH_KNOTS((2,2),(3,2,2,3),(0.,0.289807040991593),(0.280257803540345,
0.280433083165913,0.285714285714286,0.297961045722762),.UNSPECIFIED.)
GEOMETRIC_REPRESENTATION_ITEM()
RATIONAL_B_SPLINE_SURFACE(((0.996566619267863,0.996566619267863,0.996566619267863,
0.998146249162903,1.,0.995701274206111,0.992876621380142),(0.996566619267863,
0.996566619267863,0.996566619267863,0.998146249162903,1.,0.995701274206111,
0.992876621380142)))
REPRESENTATION_ITEM('')
SURFACE()
);
#1588=(
BOUNDED_SURFACE()
B_SPLINE_SURFACE(1,2,((#120784,#120785,#120786),(#120787,#120788,#120789)),
 .UNSPECIFIED.,.F.,.F.,.F.)
B_SPLINE_SURFACE_WITH_KNOTS((2,2),(3,3),(0.,0.289681084359924),(0.43567212259767,
0.452924869174518),.UNSPECIFIED.)
GEOMETRIC_REPRESENTATION_ITEM()
RATIONAL_B_SPLINE_SURFACE(((0.995510721093622,0.990658873102333,0.988732477628005),
(0.995510721093622,0.990658873102333,0.988732477628005)))
REPRESENTATION_ITEM('')
SURFACE()
);
#1589=(
BOUNDED_SURFACE()
B_SPLINE_SURFACE(1,2,((#120791,#120792,#120793,#120794,#120795,#120796,
#120797),(#120798,#120799,#120800,#120801,#120802,#120803,#120804)),
 .UNSPECIFIED.,.F.,.F.,.F.)
B_SPLINE_SURFACE_WITH_KNOTS((2,2),(3,2,2,3),(0.,0.289807040991598),(0.280257803540345,
0.280433083165913,0.285714285714286,0.297961045722761),.UNSPECIFIED.)
GEOMETRIC_REPRESENTATION_ITEM()
RATIONAL_B_SPLINE_SURFACE(((0.996566619267863,0.996566619267863,0.996566619267863,
0.998146249162903,1.,0.995701274206111,0.992876621380142),(0.996566619267863,
0.996566619267863,0.996566619267863,0.998146249162903,1.,0.995701274206111,
0.992876621380142)))
REPRESENTATION_ITEM('')
SURFACE()
);
#1590=(
BOUNDED_SURFACE()
B_SPLINE_SURFACE(1,2,((#120827,#120828,#120829),(#120830,#120831,#120832)),
 .UNSPECIFIED.,.F.,.F.,.F.)
B_SPLINE_SURFACE_WITH_KNOTS((2,2),(3,3),(0.,0.289681084359926),(0.435672122597196,
0.452924869174518),.UNSPECIFIED.)
GEOMETRIC_REPRESENTATION_ITEM()
RATIONAL_B_SPLINE_SURFACE(((0.995510721093888,0.990658873102386,0.988732477628005),
(0.995510721093888,0.990658873102386,0.988732477628005)))
REPRESENTATION_ITEM('')
SURFACE()
);
#1591=(
BOUNDED_SURFACE()
B_SPLINE_SURFACE(1,2,((#120834,#120835,#120836,#120837,#120838,#120839,
#120840),(#120841,#120842,#120843,#120844,#120845,#120846,#120847)),
 .UNSPECIFIED.,.F.,.F.,.F.)
B_SPLINE_SURFACE_WITH_KNOTS((2,2),(3,2,2,3),(0.,0.289807040991589),(0.280257803540345,
0.280433083165913,0.285714285714286,0.297961045722762),.UNSPECIFIED.)
GEOMETRIC_REPRESENTATION_ITEM()
RATIONAL_B_SPLINE_SURFACE(((0.996566619267863,0.996566619267863,0.996566619267863,
0.998146249162903,1.,0.995701274206111,0.992876621380142),(0.996566619267863,
0.996566619267863,0.996566619267863,0.998146249162903,1.,0.995701274206111,
0.992876621380142)))
REPRESENTATION_ITEM('')
SURFACE()
);
#1592=(
BOUNDED_SURFACE()
B_SPLINE_SURFACE(1,2,((#120870,#120871,#120872),(#120873,#120874,#120875)),
 .UNSPECIFIED.,.F.,.F.,.F.)
B_SPLINE_SURFACE_WITH_KNOTS((2,2),(3,3),(0.,0.289681084359925),(0.43567212259767,
0.452924869174518),.UNSPECIFIED.)
GEOMETRIC_REPRESENTATION_ITEM()
RATIONAL_B_SPLINE_SURFACE(((0.995510721093622,0.990658873102333,0.988732477628005),
(0.995510721093622,0.990658873102333,0.988732477628005)))
REPRESENTATION_ITEM('')
SURFACE()
);
#1593=(
BOUNDED_SURFACE()
B_SPLINE_SURFACE(1,2,((#120877,#120878,#120879,#120880,#120881,#120882,
#120883),(#120884,#120885,#120886,#120887,#120888,#120889,#120890)),
 .UNSPECIFIED.,.F.,.F.,.F.)
B_SPLINE_SURFACE_WITH_KNOTS((2,2),(3,2,2,3),(0.,0.289807040992543),(0.280257803540345,
0.280433083165913,0.285714285714286,0.297961045722762),.UNSPECIFIED.)
GEOMETRIC_REPRESENTATION_ITEM()
RATIONAL_B_SPLINE_SURFACE(((0.996566619267863,0.996566619267863,0.996566619267863,
0.998146249162903,1.,0.995701274206111,0.992876621380142),(0.996566619267863,
0.996566619267863,0.996566619267863,0.998146249162903,1.,0.995701274206111,
0.992876621380142)))
REPRESENTATION_ITEM('')
SURFACE()
);
#1594=(
BOUNDED_SURFACE()
B_SPLINE_SURFACE(1,2,((#120913,#120914,#120915),(#120916,#120917,#120918)),
 .UNSPECIFIED.,.F.,.F.,.F.)
B_SPLINE_SURFACE_WITH_KNOTS((2,2),(3,3),(0.,0.289681084359917),(0.43567212259767,
0.452924869174518),.UNSPECIFIED.)
GEOMETRIC_REPRESENTATION_ITEM()
RATIONAL_B_SPLINE_SURFACE(((0.995510721093622,0.990658873102333,0.988732477628005),
(0.995510721093622,0.990658873102333,0.988732477628005)))
REPRESENTATION_ITEM('')
SURFACE()
);
#1595=(
BOUNDED_SURFACE()
B_SPLINE_SURFACE(1,2,((#120920,#120921,#120922,#120923,#120924,#120925,
#120926),(#120927,#120928,#120929,#120930,#120931,#120932,#120933)),
 .UNSPECIFIED.,.F.,.F.,.F.)
B_SPLINE_SURFACE_WITH_KNOTS((2,2),(3,2,2,3),(0.,0.289807040992539),(0.280257803540345,
0.280433083165913,0.285714285714286,0.297961045722762),.UNSPECIFIED.)
GEOMETRIC_REPRESENTATION_ITEM()
RATIONAL_B_SPLINE_SURFACE(((0.996566619267863,0.996566619267863,0.996566619267863,
0.998146249162903,1.,0.995701274206111,0.992876621380142),(0.996566619267863,
0.996566619267863,0.996566619267863,0.998146249162903,1.,0.995701274206111,
0.992876621380142)))
REPRESENTATION_ITEM('')
SURFACE()
);
#1596=(
BOUNDED_SURFACE()
B_SPLINE_SURFACE(1,2,((#120956,#120957,#120958),(#120959,#120960,#120961)),
 .UNSPECIFIED.,.F.,.F.,.F.)
B_SPLINE_SURFACE_WITH_KNOTS((2,2),(3,3),(0.,0.289681084359922),(0.435672122597671,
0.452924869174518),.UNSPECIFIED.)
GEOMETRIC_REPRESENTATION_ITEM()
RATIONAL_B_SPLINE_SURFACE(((0.995510721093621,0.990658873102333,0.988732477628005),
(0.995510721093622,0.990658873102333,0.988732477628005)))
REPRESENTATION_ITEM('')
SURFACE()
);
#1597=(
BOUNDED_SURFACE()
B_SPLINE_SURFACE(1,2,((#120963,#120964,#120965,#120966,#120967,#120968,
#120969),(#120970,#120971,#120972,#120973,#120974,#120975,#120976)),
 .UNSPECIFIED.,.F.,.F.,.F.)
B_SPLINE_SURFACE_WITH_KNOTS((2,2),(3,2,2,3),(0.,0.289807040992498),(0.280257803540345,
0.280433083165913,0.285714285714286,0.297961045722762),.UNSPECIFIED.)
GEOMETRIC_REPRESENTATION_ITEM()
RATIONAL_B_SPLINE_SURFACE(((0.996566619267863,0.996566619267863,0.996566619267863,
0.998146249162903,1.,0.995701274206111,0.992876621380142),(0.996566619267863,
0.996566619267863,0.996566619267863,0.998146249162903,1.,0.995701274206111,
0.992876621380142)))
REPRESENTATION_ITEM('')
SURFACE()
);
#1598=(
BOUNDED_SURFACE()
B_SPLINE_SURFACE(1,2,((#120999,#121000,#121001),(#121002,#121003,#121004)),
 .UNSPECIFIED.,.F.,.F.,.F.)
B_SPLINE_SURFACE_WITH_KNOTS((2,2),(3,3),(0.,0.289681084359914),(0.43567212259767,
0.452924869174518),.UNSPECIFIED.)
GEOMETRIC_REPRESENTATION_ITEM()
RATIONAL_B_SPLINE_SURFACE(((0.995510721093622,0.990658873102333,0.988732477628005),
(0.995510721093622,0.990658873102333,0.988732477628005)))
REPRESENTATION_ITEM('')
SURFACE()
);
#1599=(
BOUNDED_SURFACE()
B_SPLINE_SURFACE(1,2,((#121006,#121007,#121008,#121009,#121010,#121011,
#121012),(#121013,#121014,#121015,#121016,#121017,#121018,#121019)),
 .UNSPECIFIED.,.F.,.F.,.F.)
B_SPLINE_SURFACE_WITH_KNOTS((2,2),(3,2,2,3),(0.,0.289807040992513),(0.280257803540345,
0.280433083165913,0.285714285714286,0.297961045722762),.UNSPECIFIED.)
GEOMETRIC_REPRESENTATION_ITEM()
RATIONAL_B_SPLINE_SURFACE(((0.996566619267863,0.996566619267863,0.996566619267863,
0.998146249162903,1.,0.995701274206111,0.992876621380142),(0.996566619267863,
0.996566619267863,0.996566619267863,0.998146249162903,1.,0.995701274206111,
0.992876621380142)))
REPRESENTATION_ITEM('')
SURFACE()
);
#1600=(
BOUNDED_SURFACE()
B_SPLINE_SURFACE(1,2,((#121027,#121028,#121029),(#121030,#121031,#121032)),
 .UNSPECIFIED.,.F.,.F.,.F.)
B_SPLINE_SURFACE_WITH_KNOTS((2,2),(3,3),(0.,0.289681084359923),(0.43567212259767,
0.452924869174518),.UNSPECIFIED.)
GEOMETRIC_REPRESENTATION_ITEM()
RATIONAL_B_SPLINE_SURFACE(((0.995510721093622,0.990658873102333,0.988732477628005),
(0.995510721093622,0.990658873102333,0.988732477628005)))
REPRESENTATION_ITEM('')
SURFACE()
);
#1601=(
BOUNDED_SURFACE()
B_SPLINE_SURFACE(1,2,((#121034,#121035,#121036,#121037,#121038,#121039,
#121040),(#121041,#121042,#121043,#121044,#121045,#121046,#121047)),
 .UNSPECIFIED.,.F.,.F.,.F.)
B_SPLINE_SURFACE_WITH_KNOTS((2,2),(3,2,2,3),(0.,0.289807040991561),(0.280257803540345,
0.280433083165913,0.285714285714286,0.297961045722762),.UNSPECIFIED.)
GEOMETRIC_REPRESENTATION_ITEM()
RATIONAL_B_SPLINE_SURFACE(((0.996566619267863,0.996566619267863,0.996566619267863,
0.998146249162903,1.,0.995701274206111,0.992876621380142),(0.996566619267863,
0.996566619267863,0.996566619267863,0.998146249162903,1.,0.995701274206111,
0.992876621380142)))
REPRESENTATION_ITEM('')
SURFACE()
);
#1602=(
BOUNDED_SURFACE()
B_SPLINE_SURFACE(1,2,((#121070,#121071,#121072),(#121073,#121074,#121075)),
 .UNSPECIFIED.,.F.,.F.,.F.)
B_SPLINE_SURFACE_WITH_KNOTS((2,2),(3,3),(0.,0.289681084359924),(0.43567212259767,
0.452924869174518),.UNSPECIFIED.)
GEOMETRIC_REPRESENTATION_ITEM()
RATIONAL_B_SPLINE_SURFACE(((0.995510721093622,0.990658873102333,0.988732477628005),
(0.995510721093622,0.990658873102333,0.988732477628005)))
REPRESENTATION_ITEM('')
SURFACE()
);
#1603=(
BOUNDED_SURFACE()
B_SPLINE_SURFACE(1,2,((#121077,#121078,#121079,#121080,#121081,#121082,
#121083),(#121084,#121085,#121086,#121087,#121088,#121089,#121090)),
 .UNSPECIFIED.,.F.,.F.,.F.)
B_SPLINE_SURFACE_WITH_KNOTS((2,2),(3,2,2,3),(0.,0.289807040991563),(0.280257803540345,
0.280433083165913,0.285714285714286,0.297961045722762),.UNSPECIFIED.)
GEOMETRIC_REPRESENTATION_ITEM()
RATIONAL_B_SPLINE_SURFACE(((0.996566619267863,0.996566619267863,0.996566619267863,
0.998146249162903,1.,0.995701274206111,0.992876621380142),(0.996566619267863,
0.996566619267863,0.996566619267863,0.998146249162903,1.,0.995701274206111,
0.992876621380142)))
REPRESENTATION_ITEM('')
SURFACE()
);
#1604=(
BOUNDED_SURFACE()
B_SPLINE_SURFACE(1,2,((#121113,#121114,#121115),(#121116,#121117,#121118)),
 .UNSPECIFIED.,.F.,.F.,.F.)
B_SPLINE_SURFACE_WITH_KNOTS((2,2),(3,3),(0.,0.289681084359924),(0.43567212259767,
0.452924869174518),.UNSPECIFIED.)
GEOMETRIC_REPRESENTATION_ITEM()
RATIONAL_B_SPLINE_SURFACE(((0.995510721093622,0.990658873102333,0.988732477628005),
(0.995510721093622,0.990658873102333,0.988732477628005)))
REPRESENTATION_ITEM('')
SURFACE()
);
#1605=(
BOUNDED_SURFACE()
B_SPLINE_SURFACE(1,2,((#121120,#121121,#121122,#121123,#121124,#121125,
#121126),(#121127,#121128,#121129,#121130,#121131,#121132,#121133)),
 .UNSPECIFIED.,.F.,.F.,.F.)
B_SPLINE_SURFACE_WITH_KNOTS((2,2),(3,2,2,3),(0.,0.289807040991564),(0.280257803540345,
0.280433083165913,0.285714285714286,0.297961045722762),.UNSPECIFIED.)
GEOMETRIC_REPRESENTATION_ITEM()
RATIONAL_B_SPLINE_SURFACE(((0.996566619267863,0.996566619267863,0.996566619267863,
0.998146249162903,1.,0.995701274206111,0.992876621380142),(0.996566619267863,
0.996566619267863,0.996566619267863,0.998146249162903,1.,0.995701274206111,
0.992876621380142)))
REPRESENTATION_ITEM('')
SURFACE()
);
#1606=(
BOUNDED_SURFACE()
B_SPLINE_SURFACE(1,2,((#121156,#121157,#121158),(#121159,#121160,#121161)),
 .UNSPECIFIED.,.F.,.F.,.F.)
B_SPLINE_SURFACE_WITH_KNOTS((2,2),(3,3),(0.,0.289681084359998),(0.43567212259767,
0.452924869174518),.UNSPECIFIED.)
GEOMETRIC_REPRESENTATION_ITEM()
RATIONAL_B_SPLINE_SURFACE(((0.995510721093622,0.990658873102333,0.988732477628005),
(0.995510721093622,0.990658873102333,0.988732477628005)))
REPRESENTATION_ITEM('')
SURFACE()
);
#1607=(
BOUNDED_SURFACE()
B_SPLINE_SURFACE(1,2,((#121163,#121164,#121165,#121166,#121167,#121168,
#121169),(#121170,#121171,#121172,#121173,#121174,#121175,#121176)),
 .UNSPECIFIED.,.F.,.F.,.F.)
B_SPLINE_SURFACE_WITH_KNOTS((2,2),(3,2,2,3),(0.,0.289807040991565),(0.280257803540345,
0.280433083165913,0.285714285714286,0.297961045722762),.UNSPECIFIED.)
GEOMETRIC_REPRESENTATION_ITEM()
RATIONAL_B_SPLINE_SURFACE(((0.996566619267863,0.996566619267863,0.996566619267863,
0.998146249162903,1.,0.995701274206111,0.992876621380142),(0.996566619267863,
0.996566619267863,0.996566619267863,0.998146249162903,1.,0.995701274206111,
0.992876621380142)))
REPRESENTATION_ITEM('')
SURFACE()
);
#1608=(
BOUNDED_SURFACE()
B_SPLINE_SURFACE(1,2,((#121199,#121200,#121201),(#121202,#121203,#121204)),
 .UNSPECIFIED.,.F.,.F.,.F.)
B_SPLINE_SURFACE_WITH_KNOTS((2,2),(3,3),(0.,0.28968108435992),(0.43567212259767,
0.452924869174518),.UNSPECIFIED.)
GEOMETRIC_REPRESENTATION_ITEM()
RATIONAL_B_SPLINE_SURFACE(((0.995510721093622,0.990658873102333,0.988732477628006),
(0.995510721093622,0.990658873102333,0.988732477628006)))
REPRESENTATION_ITEM('')
SURFACE()
);
#1609=(
BOUNDED_SURFACE()
B_SPLINE_SURFACE(1,2,((#121206,#121207,#121208,#121209,#121210,#121211,
#121212),(#121213,#121214,#121215,#121216,#121217,#121218,#121219)),
 .UNSPECIFIED.,.F.,.F.,.F.)
B_SPLINE_SURFACE_WITH_KNOTS((2,2),(3,2,2,3),(0.,0.289807040991563),(0.280257803540345,
0.280433083165913,0.285714285714286,0.297961045722762),.UNSPECIFIED.)
GEOMETRIC_REPRESENTATION_ITEM()
RATIONAL_B_SPLINE_SURFACE(((0.996566619267863,0.996566619267863,0.996566619267863,
0.998146249162903,1.,0.995701274206111,0.992876621380142),(0.996566619267863,
0.996566619267863,0.996566619267863,0.998146249162903,1.,0.995701274206111,
0.992876621380142)))
REPRESENTATION_ITEM('')
SURFACE()
);
#1610=(
BOUNDED_SURFACE()
B_SPLINE_SURFACE(1,2,((#121242,#121243,#121244),(#121245,#121246,#121247)),
 .UNSPECIFIED.,.F.,.F.,.F.)
B_SPLINE_SURFACE_WITH_KNOTS((2,2),(3,3),(0.,0.289681084359918),(0.43567212259767,
0.452924869174518),.UNSPECIFIED.)
GEOMETRIC_REPRESENTATION_ITEM()
RATIONAL_B_SPLINE_SURFACE(((0.995510721093622,0.990658873102333,0.988732477628005),
(0.995510721093622,0.990658873102333,0.988732477628005)))
REPRESENTATION_ITEM('')
SURFACE()
);
#1611=(
BOUNDED_SURFACE()
B_SPLINE_SURFACE(1,2,((#121249,#121250,#121251,#121252,#121253,#121254,
#121255),(#121256,#121257,#121258,#121259,#121260,#121261,#121262)),
 .UNSPECIFIED.,.F.,.F.,.F.)
B_SPLINE_SURFACE_WITH_KNOTS((2,2),(3,2,2,3),(0.,0.289807040991569),(0.280257803540345,
0.280433083165913,0.285714285714286,0.297961045722762),.UNSPECIFIED.)
GEOMETRIC_REPRESENTATION_ITEM()
RATIONAL_B_SPLINE_SURFACE(((0.996566619267863,0.996566619267863,0.996566619267863,
0.998146249162903,1.,0.995701274206111,0.992876621380142),(0.996566619267863,
0.996566619267863,0.996566619267863,0.998146249162903,1.,0.995701274206111,
0.992876621380142)))
REPRESENTATION_ITEM('')
SURFACE()
);
#1612=(
BOUNDED_SURFACE()
B_SPLINE_SURFACE(1,2,((#121285,#121286,#121287),(#121288,#121289,#121290)),
 .UNSPECIFIED.,.F.,.F.,.F.)
B_SPLINE_SURFACE_WITH_KNOTS((2,2),(3,3),(0.,0.289681084359925),(0.43567212259767,
0.452924869174518),.UNSPECIFIED.)
GEOMETRIC_REPRESENTATION_ITEM()
RATIONAL_B_SPLINE_SURFACE(((0.995510721093622,0.990658873102333,0.988732477628005),
(0.995510721093622,0.990658873102333,0.988732477628005)))
REPRESENTATION_ITEM('')
SURFACE()
);
#1613=(
BOUNDED_SURFACE()
B_SPLINE_SURFACE(1,2,((#121292,#121293,#121294,#121295,#121296,#121297,
#121298),(#121299,#121300,#121301,#121302,#121303,#121304,#121305)),
 .UNSPECIFIED.,.F.,.F.,.F.)
B_SPLINE_SURFACE_WITH_KNOTS((2,2),(3,2,2,3),(0.,0.289807040991567),(0.280257803540345,
0.280433083165913,0.285714285714286,0.297961045722762),.UNSPECIFIED.)
GEOMETRIC_REPRESENTATION_ITEM()
RATIONAL_B_SPLINE_SURFACE(((0.996566619267863,0.996566619267863,0.996566619267863,
0.998146249162903,1.,0.995701274206111,0.992876621380142),(0.996566619267863,
0.996566619267863,0.996566619267863,0.998146249162903,1.,0.995701274206111,
0.992876621380142)))
REPRESENTATION_ITEM('')
SURFACE()
);
#1614=(
BOUNDED_SURFACE()
B_SPLINE_SURFACE(1,2,((#121328,#121329,#121330),(#121331,#121332,#121333)),
 .UNSPECIFIED.,.F.,.F.,.F.)
B_SPLINE_SURFACE_WITH_KNOTS((2,2),(3,3),(0.,0.289681084359924),(0.43567212259767,
0.452924869174518),.UNSPECIFIED.)
GEOMETRIC_REPRESENTATION_ITEM()
RATIONAL_B_SPLINE_SURFACE(((0.995510721093622,0.990658873102333,0.988732477628005),
(0.995510721093622,0.990658873102333,0.988732477628005)))
REPRESENTATION_ITEM('')
SURFACE()
);
#1615=(
BOUNDED_SURFACE()
B_SPLINE_SURFACE(1,2,((#121335,#121336,#121337,#121338,#121339,#121340,
#121341),(#121342,#121343,#121344,#121345,#121346,#121347,#121348)),
 .UNSPECIFIED.,.F.,.F.,.F.)
B_SPLINE_SURFACE_WITH_KNOTS((2,2),(3,2,2,3),(0.,0.289807040991561),(0.280257803540345,
0.280433083165913,0.285714285714286,0.297961045722762),.UNSPECIFIED.)
GEOMETRIC_REPRESENTATION_ITEM()
RATIONAL_B_SPLINE_SURFACE(((0.996566619267863,0.996566619267863,0.996566619267863,
0.998146249162903,1.,0.995701274206111,0.992876621380142),(0.996566619267863,
0.996566619267863,0.996566619267863,0.998146249162903,1.,0.995701274206111,
0.992876621380142)))
REPRESENTATION_ITEM('')
SURFACE()
);
#1616=(
BOUNDED_SURFACE()
B_SPLINE_SURFACE(1,2,((#121371,#121372,#121373),(#121374,#121375,#121376)),
 .UNSPECIFIED.,.F.,.F.,.F.)
B_SPLINE_SURFACE_WITH_KNOTS((2,2),(3,3),(0.,0.289681084359921),(0.43567212259767,
0.452924869174518),.UNSPECIFIED.)
GEOMETRIC_REPRESENTATION_ITEM()
RATIONAL_B_SPLINE_SURFACE(((0.995510721093622,0.990658873102333,0.988732477628005),
(0.995510721093622,0.990658873102333,0.988732477628005)))
REPRESENTATION_ITEM('')
SURFACE()
);
#1617=(
BOUNDED_SURFACE()
B_SPLINE_SURFACE(1,2,((#121378,#121379,#121380,#121381,#121382,#121383,
#121384),(#121385,#121386,#121387,#121388,#121389,#121390,#121391)),
 .UNSPECIFIED.,.F.,.F.,.F.)
B_SPLINE_SURFACE_WITH_KNOTS((2,2),(3,2,2,3),(0.,0.289807040991566),(0.280257803540345,
0.280433083165913,0.285714285714286,0.297961045722762),.UNSPECIFIED.)
GEOMETRIC_REPRESENTATION_ITEM()
RATIONAL_B_SPLINE_SURFACE(((0.996566619267863,0.996566619267863,0.996566619267863,
0.998146249162903,1.,0.995701274206111,0.992876621380142),(0.996566619267863,
0.996566619267863,0.996566619267863,0.998146249162903,1.,0.995701274206111,
0.992876621380142)))
REPRESENTATION_ITEM('')
SURFACE()
);
#1618=(
BOUNDED_SURFACE()
B_SPLINE_SURFACE(1,2,((#121414,#121415,#121416),(#121417,#121418,#121419)),
 .UNSPECIFIED.,.F.,.F.,.F.)
B_SPLINE_SURFACE_WITH_KNOTS((2,2),(3,3),(0.,0.289681084359929),(0.43567212259767,
0.452924869174518),.UNSPECIFIED.)
GEOMETRIC_REPRESENTATION_ITEM()
RATIONAL_B_SPLINE_SURFACE(((0.995510721093622,0.990658873102333,0.988732477628005),
(0.995510721093622,0.990658873102333,0.988732477628005)))
REPRESENTATION_ITEM('')
SURFACE()
);
#1619=(
BOUNDED_SURFACE()
B_SPLINE_SURFACE(1,2,((#121421,#121422,#121423,#121424,#121425,#121426,
#121427),(#121428,#121429,#121430,#121431,#121432,#121433,#121434)),
 .UNSPECIFIED.,.F.,.F.,.F.)
B_SPLINE_SURFACE_WITH_KNOTS((2,2),(3,2,2,3),(0.,0.289807040991562),(0.280257803540345,
0.280433083165913,0.285714285714286,0.297961045722762),.UNSPECIFIED.)
GEOMETRIC_REPRESENTATION_ITEM()
RATIONAL_B_SPLINE_SURFACE(((0.996566619267863,0.996566619267863,0.996566619267863,
0.998146249162903,1.,0.995701274206111,0.992876621380142),(0.996566619267863,
0.996566619267863,0.996566619267863,0.998146249162903,1.,0.995701274206111,
0.992876621380142)))
REPRESENTATION_ITEM('')
SURFACE()
);
#1620=(
BOUNDED_SURFACE()
B_SPLINE_SURFACE(1,2,((#121457,#121458,#121459),(#121460,#121461,#121462)),
 .UNSPECIFIED.,.F.,.F.,.F.)
B_SPLINE_SURFACE_WITH_KNOTS((2,2),(3,3),(0.,0.289681084359919),(0.43567212259767,
0.452924869174518),.UNSPECIFIED.)
GEOMETRIC_REPRESENTATION_ITEM()
RATIONAL_B_SPLINE_SURFACE(((0.995510721093622,0.990658873102333,0.988732477628005),
(0.995510721093622,0.990658873102333,0.988732477628005)))
REPRESENTATION_ITEM('')
SURFACE()
);
#1621=(
BOUNDED_SURFACE()
B_SPLINE_SURFACE(1,2,((#121464,#121465,#121466,#121467,#121468,#121469,
#121470),(#121471,#121472,#121473,#121474,#121475,#121476,#121477)),
 .UNSPECIFIED.,.F.,.F.,.F.)
B_SPLINE_SURFACE_WITH_KNOTS((2,2),(3,2,2,3),(0.,0.289807040991561),(0.280257803540345,
0.280433083165913,0.285714285714286,0.297961045722762),.UNSPECIFIED.)
GEOMETRIC_REPRESENTATION_ITEM()
RATIONAL_B_SPLINE_SURFACE(((0.996566619267863,0.996566619267863,0.996566619267863,
0.998146249162903,1.,0.995701274206111,0.992876621380142),(0.996566619267863,
0.996566619267863,0.996566619267863,0.998146249162903,1.,0.995701274206111,
0.992876621380142)))
REPRESENTATION_ITEM('')
SURFACE()
);
#1622=(
BOUNDED_SURFACE()
B_SPLINE_SURFACE(1,2,((#121500,#121501,#121502),(#121503,#121504,#121505)),
 .UNSPECIFIED.,.F.,.F.,.F.)
B_SPLINE_SURFACE_WITH_KNOTS((2,2),(3,3),(0.,0.289681084359921),(0.43567212259767,
0.452924869174518),.UNSPECIFIED.)
GEOMETRIC_REPRESENTATION_ITEM()
RATIONAL_B_SPLINE_SURFACE(((0.995510721093622,0.990658873102333,0.988732477628005),
(0.995510721093622,0.990658873102333,0.988732477628005)))
REPRESENTATION_ITEM('')
SURFACE()
);
#1623=(
BOUNDED_SURFACE()
B_SPLINE_SURFACE(1,2,((#121507,#121508,#121509,#121510,#121511,#121512,
#121513),(#121514,#121515,#121516,#121517,#121518,#121519,#121520)),
 .UNSPECIFIED.,.F.,.F.,.F.)
B_SPLINE_SURFACE_WITH_KNOTS((2,2),(3,2,2,3),(0.,0.28980704099156),(0.280257803540345,
0.280433083165913,0.285714285714286,0.297961045722762),.UNSPECIFIED.)
GEOMETRIC_REPRESENTATION_ITEM()
RATIONAL_B_SPLINE_SURFACE(((0.996566619267863,0.996566619267863,0.996566619267863,
0.998146249162903,1.,0.995701274206111,0.992876621380142),(0.996566619267863,
0.996566619267863,0.996566619267863,0.998146249162903,1.,0.995701274206111,
0.992876621380142)))
REPRESENTATION_ITEM('')
SURFACE()
);
#1624=(
BOUNDED_SURFACE()
B_SPLINE_SURFACE(1,2,((#121543,#121544,#121545),(#121546,#121547,#121548)),
 .UNSPECIFIED.,.F.,.F.,.F.)
B_SPLINE_SURFACE_WITH_KNOTS((2,2),(3,3),(0.,0.289681084359922),(0.43567212259767,
0.452924869174518),.UNSPECIFIED.)
GEOMETRIC_REPRESENTATION_ITEM()
RATIONAL_B_SPLINE_SURFACE(((0.995510721093622,0.990658873102333,0.988732477628005),
(0.995510721093622,0.990658873102333,0.988732477628005)))
REPRESENTATION_ITEM('')
SURFACE()
);
#1625=(
BOUNDED_SURFACE()
B_SPLINE_SURFACE(1,2,((#121550,#121551,#121552,#121553,#121554,#121555,
#121556),(#121557,#121558,#121559,#121560,#121561,#121562,#121563)),
 .UNSPECIFIED.,.F.,.F.,.F.)
B_SPLINE_SURFACE_WITH_KNOTS((2,2),(3,2,2,3),(0.,0.289807040992967),(0.280257803540345,
0.280433083165913,0.285714285714286,0.297961045722762),.UNSPECIFIED.)
GEOMETRIC_REPRESENTATION_ITEM()
RATIONAL_B_SPLINE_SURFACE(((0.996566619267863,0.996566619267863,0.996566619267863,
0.998146249162903,1.,0.995701274206111,0.992876621380142),(0.996566619267863,
0.996566619267863,0.996566619267863,0.998146249162903,1.,0.995701274206111,
0.992876621380142)))
REPRESENTATION_ITEM('')
SURFACE()
);
#1626=(
BOUNDED_SURFACE()
B_SPLINE_SURFACE(1,2,((#121586,#121587,#121588),(#121589,#121590,#121591)),
 .UNSPECIFIED.,.F.,.F.,.F.)
B_SPLINE_SURFACE_WITH_KNOTS((2,2),(3,3),(0.,0.289681084359923),(0.43567212259767,
0.452924869174518),.UNSPECIFIED.)
GEOMETRIC_REPRESENTATION_ITEM()
RATIONAL_B_SPLINE_SURFACE(((0.995510721093622,0.990658873102333,0.988732477628005),
(0.995510721093622,0.990658873102333,0.988732477628005)))
REPRESENTATION_ITEM('')
SURFACE()
);
#1627=(
BOUNDED_SURFACE()
B_SPLINE_SURFACE(1,2,((#121593,#121594,#121595,#121596,#121597,#121598,
#121599),(#121600,#121601,#121602,#121603,#121604,#121605,#121606)),
 .UNSPECIFIED.,.F.,.F.,.F.)
B_SPLINE_SURFACE_WITH_KNOTS((2,2),(3,2,2,3),(0.,0.289807040991561),(0.280257803540345,
0.280433083165913,0.285714285714286,0.297961045722762),.UNSPECIFIED.)
GEOMETRIC_REPRESENTATION_ITEM()
RATIONAL_B_SPLINE_SURFACE(((0.996566619267863,0.996566619267863,0.996566619267863,
0.998146249162903,1.,0.995701274206111,0.992876621380142),(0.996566619267863,
0.996566619267863,0.996566619267863,0.998146249162903,1.,0.995701274206111,
0.992876621380142)))
REPRESENTATION_ITEM('')
SURFACE()
);
#1628=(
BOUNDED_SURFACE()
B_SPLINE_SURFACE(1,2,((#121629,#121630,#121631),(#121632,#121633,#121634)),
 .UNSPECIFIED.,.F.,.F.,.F.)
B_SPLINE_SURFACE_WITH_KNOTS((2,2),(3,3),(0.,0.289681084359924),(0.43567212259767,
0.452924869174518),.UNSPECIFIED.)
GEOMETRIC_REPRESENTATION_ITEM()
RATIONAL_B_SPLINE_SURFACE(((0.995510721093622,0.990658873102333,0.988732477628005),
(0.995510721093622,0.990658873102333,0.988732477628005)))
REPRESENTATION_ITEM('')
SURFACE()
);
#1629=(
BOUNDED_SURFACE()
B_SPLINE_SURFACE(1,2,((#121636,#121637,#121638,#121639,#121640,#121641,
#121642),(#121643,#121644,#121645,#121646,#121647,#121648,#121649)),
 .UNSPECIFIED.,.F.,.F.,.F.)
B_SPLINE_SURFACE_WITH_KNOTS((2,2),(3,2,2,3),(0.,0.289807040991556),(0.280257803540345,
0.280433083165913,0.285714285714286,0.297961045722762),.UNSPECIFIED.)
GEOMETRIC_REPRESENTATION_ITEM()
RATIONAL_B_SPLINE_SURFACE(((0.996566619267863,0.996566619267863,0.996566619267863,
0.998146249162903,1.,0.995701274206111,0.992876621380142),(0.996566619267863,
0.996566619267863,0.996566619267863,0.998146249162903,1.,0.995701274206111,
0.992876621380142)))
REPRESENTATION_ITEM('')
SURFACE()
);
#1630=(
BOUNDED_SURFACE()
B_SPLINE_SURFACE(1,2,((#121666,#121667,#121668),(#121669,#121670,#121671)),
 .UNSPECIFIED.,.F.,.F.,.F.)
B_SPLINE_SURFACE_WITH_KNOTS((2,2),(3,3),(0.,0.28968108435992),(0.43567212259767,
0.452924869174518),.UNSPECIFIED.)
GEOMETRIC_REPRESENTATION_ITEM()
RATIONAL_B_SPLINE_SURFACE(((0.995510721093622,0.990658873102333,0.988732477628005),
(0.995510721093622,0.990658873102333,0.988732477628005)))
REPRESENTATION_ITEM('')
SURFACE()
);
#1631=(
BOUNDED_SURFACE()
B_SPLINE_SURFACE(1,2,((#121679,#121680,#121681,#121682,#121683,#121684,
#121685),(#121686,#121687,#121688,#121689,#121690,#121691,#121692)),
 .UNSPECIFIED.,.F.,.F.,.F.)
B_SPLINE_SURFACE_WITH_KNOTS((2,2),(3,2,2,3),(0.,0.28980704099156),(0.280257803540344,
0.280433083165912,0.285714285714286,0.297961045722762),.UNSPECIFIED.)
GEOMETRIC_REPRESENTATION_ITEM()
RATIONAL_B_SPLINE_SURFACE(((0.996566619267863,0.996566619267863,0.996566619267863,
0.998146249162903,1.,0.995701274206111,0.992876621380142),(0.996566619267863,
0.996566619267863,0.996566619267863,0.998146249162903,1.,0.995701274206111,
0.992876621380142)))
REPRESENTATION_ITEM('')
SURFACE()
);
#1632=(
BOUNDED_SURFACE()
B_SPLINE_SURFACE(1,2,((#121715,#121716,#121717),(#121718,#121719,#121720)),
 .UNSPECIFIED.,.F.,.F.,.F.)
B_SPLINE_SURFACE_WITH_KNOTS((2,2),(3,3),(0.,0.289681084359921),(0.43567212259767,
0.452924869174517),.UNSPECIFIED.)
GEOMETRIC_REPRESENTATION_ITEM()
RATIONAL_B_SPLINE_SURFACE(((0.995510721093622,0.990658873102333,0.988732477628006),
(0.995510721093622,0.990658873102333,0.988732477628006)))
REPRESENTATION_ITEM('')
SURFACE()
);
#1633=(
BOUNDED_SURFACE()
B_SPLINE_SURFACE(1,2,((#121722,#121723,#121724,#121725,#121726,#121727,
#121728),(#121729,#121730,#121731,#121732,#121733,#121734,#121735)),
 .UNSPECIFIED.,.F.,.F.,.F.)
B_SPLINE_SURFACE_WITH_KNOTS((2,2),(3,2,2,3),(0.,0.289807040991633),(0.280257803540346,
0.280433083165914,0.285714285714286,0.297961045722763),.UNSPECIFIED.)
GEOMETRIC_REPRESENTATION_ITEM()
RATIONAL_B_SPLINE_SURFACE(((0.996566619267864,0.996566619267864,0.996566619267864,
0.998146249162903,1.,0.99570127420611,0.992876621380141),(0.996566619267864,
0.996566619267864,0.996566619267864,0.998146249162903,1.,0.995701274206111,
0.992876621380141)))
REPRESENTATION_ITEM('')
SURFACE()
);
#1634=(
BOUNDED_SURFACE()
B_SPLINE_SURFACE(1,2,((#121758,#121759,#121760),(#121761,#121762,#121763)),
 .UNSPECIFIED.,.F.,.F.,.F.)
B_SPLINE_SURFACE_WITH_KNOTS((2,2),(3,3),(0.,0.28968108435992),(0.435672122597669,
0.452924869174531),.UNSPECIFIED.)
GEOMETRIC_REPRESENTATION_ITEM()
RATIONAL_B_SPLINE_SURFACE(((0.995510721093622,0.990658873102329,0.988732477628002),
(0.995510721093622,0.990658873102329,0.988732477628002)))
REPRESENTATION_ITEM('')
SURFACE()
);
#1635=(
BOUNDED_SURFACE()
B_SPLINE_SURFACE(1,2,((#121765,#121766,#121767,#121768,#121769,#121770,
#121771),(#121772,#121773,#121774,#121775,#121776,#121777,#121778)),
 .UNSPECIFIED.,.F.,.F.,.F.)
B_SPLINE_SURFACE_WITH_KNOTS((2,2),(3,2,2,3),(0.,0.289807040992762),(0.28025780354034,
0.280433083165908,0.285714285714286,0.297961045722763),.UNSPECIFIED.)
GEOMETRIC_REPRESENTATION_ITEM()
RATIONAL_B_SPLINE_SURFACE(((0.99656661926786,0.99656661926786,0.99656661926786,
0.998146249162901,1.,0.995701274206111,0.992876621380141),(0.99656661926786,
0.99656661926786,0.99656661926786,0.998146249162901,1.,0.995701274206111,
0.992876621380141)))
REPRESENTATION_ITEM('')
SURFACE()
);
#1636=(
BOUNDED_SURFACE()
B_SPLINE_SURFACE(1,2,((#121801,#121802,#121803),(#121804,#121805,#121806)),
 .UNSPECIFIED.,.F.,.F.,.F.)
B_SPLINE_SURFACE_WITH_KNOTS((2,2),(3,3),(0.,0.289681084359927),(0.435672122597218,
0.452924869174574),.UNSPECIFIED.)
GEOMETRIC_REPRESENTATION_ITEM()
RATIONAL_B_SPLINE_SURFACE(((0.995510721093876,0.990658873102367,0.988732477627993),
(0.995510721093876,0.990658873102368,0.988732477627993)))
REPRESENTATION_ITEM('')
SURFACE()
);
#1637=(
BOUNDED_SURFACE()
B_SPLINE_SURFACE(1,2,((#121808,#121809,#121810,#121811,#121812,#121813,
#121814),(#121815,#121816,#121817,#121818,#121819,#121820,#121821)),
 .UNSPECIFIED.,.F.,.F.,.F.)
B_SPLINE_SURFACE_WITH_KNOTS((2,2),(3,2,2,3),(0.,0.289807040992469),(0.280257803540335,
0.280433083165903,0.285714285714286,0.297961045722763),.UNSPECIFIED.)
GEOMETRIC_REPRESENTATION_ITEM()
RATIONAL_B_SPLINE_SURFACE(((0.996566619267858,0.996566619267858,0.996566619267858,
0.998146249162899,1.,0.995701274206111,0.992876621380142),(0.996566619267858,
0.996566619267858,0.996566619267858,0.998146249162899,1.,0.995701274206111,
0.992876621380142)))
REPRESENTATION_ITEM('')
SURFACE()
);
#1638=(
BOUNDED_SURFACE()
B_SPLINE_SURFACE(1,2,((#121844,#121845,#121846),(#121847,#121848,#121849)),
 .UNSPECIFIED.,.F.,.F.,.F.)
B_SPLINE_SURFACE_WITH_KNOTS((2,2),(3,3),(0.,0.289681084359916),(0.435672122597635,
0.452924869174517),.UNSPECIFIED.)
GEOMETRIC_REPRESENTATION_ITEM()
RATIONAL_B_SPLINE_SURFACE(((0.995510721093642,0.990658873102337,0.988732477628006),
(0.995510721093642,0.990658873102337,0.988732477628006)))
REPRESENTATION_ITEM('')
SURFACE()
);
#1639=(
BOUNDED_SURFACE()
B_SPLINE_SURFACE(1,2,((#121851,#121852,#121853,#121854,#121855,#121856,
#121857),(#121858,#121859,#121860,#121861,#121862,#121863,#121864)),
 .UNSPECIFIED.,.F.,.F.,.F.)
B_SPLINE_SURFACE_WITH_KNOTS((2,2),(3,2,2,3),(0.,0.289807040992393),(0.280257803540336,
0.280433083165904,0.285714285714286,0.297961045722764),.UNSPECIFIED.)
GEOMETRIC_REPRESENTATION_ITEM()
RATIONAL_B_SPLINE_SURFACE(((0.996566619267858,0.996566619267858,0.996566619267858,
0.9981462491629,1.,0.99570127420611,0.992876621380141),(0.996566619267858,
0.996566619267858,0.996566619267858,0.9981462491629,1.,0.99570127420611,
0.992876621380141)))
REPRESENTATION_ITEM('')
SURFACE()
);
#1640=(
BOUNDED_SURFACE()
B_SPLINE_SURFACE(1,2,((#121887,#121888,#121889),(#121890,#121891,#121892)),
 .UNSPECIFIED.,.F.,.F.,.F.)
B_SPLINE_SURFACE_WITH_KNOTS((2,2),(3,3),(0.,0.289681084359926),(0.435672122597471,
0.452924869174526),.UNSPECIFIED.)
GEOMETRIC_REPRESENTATION_ITEM()
RATIONAL_B_SPLINE_SURFACE(((0.995510721093734,0.990658873102352,0.988732477628003),
(0.995510721093734,0.990658873102352,0.988732477628003)))
REPRESENTATION_ITEM('')
SURFACE()
);
#1641=(
BOUNDED_SURFACE()
B_SPLINE_SURFACE(1,2,((#121894,#121895,#121896,#121897,#121898,#121899,
#121900),(#121901,#121902,#121903,#121904,#121905,#121906,#121907)),
 .UNSPECIFIED.,.F.,.F.,.F.)
B_SPLINE_SURFACE_WITH_KNOTS((2,2),(3,2,2,3),(0.,0.289807040992293),(0.280257803540338,
0.280433083165906,0.285714285714286,0.297961045722764),.UNSPECIFIED.)
GEOMETRIC_REPRESENTATION_ITEM()
RATIONAL_B_SPLINE_SURFACE(((0.996566619267859,0.996566619267859,0.996566619267859,
0.9981462491629,1.,0.99570127420611,0.992876621380141),(0.996566619267859,
0.996566619267859,0.996566619267859,0.9981462491629,1.,0.99570127420611,
0.992876621380141)))
REPRESENTATION_ITEM('')
SURFACE()
);
#1642=(
BOUNDED_SURFACE()
B_SPLINE_SURFACE(1,2,((#121930,#121931,#121932),(#121933,#121934,#121935)),
 .UNSPECIFIED.,.F.,.F.,.F.)
B_SPLINE_SURFACE_WITH_KNOTS((2,2),(3,3),(0.,0.289681084359918),(0.43567212259767,
0.452924869174518),.UNSPECIFIED.)
GEOMETRIC_REPRESENTATION_ITEM()
RATIONAL_B_SPLINE_SURFACE(((0.995510721093622,0.990658873102333,0.988732477628005),
(0.995510721093622,0.990658873102333,0.988732477628005)))
REPRESENTATION_ITEM('')
SURFACE()
);
#1643=(
BOUNDED_SURFACE()
B_SPLINE_SURFACE(1,2,((#121949,#121950,#121951,#121952,#121953,#121954,
#121955),(#121956,#121957,#121958,#121959,#121960,#121961,#121962)),
 .UNSPECIFIED.,.F.,.F.,.F.)
B_SPLINE_SURFACE_WITH_KNOTS((2,2),(3,2,2,3),(0.,0.289807040991589),(0.280257803540345,
0.280433083165913,0.285714285714286,0.297961045722762),.UNSPECIFIED.)
GEOMETRIC_REPRESENTATION_ITEM()
RATIONAL_B_SPLINE_SURFACE(((0.996566619267863,0.996566619267863,0.996566619267863,
0.998146249162903,1.,0.995701274206111,0.992876621380142),(0.996566619267863,
0.996566619267863,0.996566619267863,0.998146249162903,1.,0.995701274206111,
0.992876621380142)))
REPRESENTATION_ITEM('')
SURFACE()
);
#1644=(
BOUNDED_SURFACE()
B_SPLINE_SURFACE(1,2,((#121964,#121965,#121966),(#121967,#121968,#121969)),
 .UNSPECIFIED.,.F.,.F.,.F.)
B_SPLINE_SURFACE_WITH_KNOTS((2,2),(3,3),(0.710192959008446,1.),(0.22888337489481,
0.246056477139965),.UNSPECIFIED.)
GEOMETRIC_REPRESENTATION_ITEM()
RATIONAL_B_SPLINE_SURFACE(((0.991846493044689,0.988282393439497,0.987616798999169),
(0.991846493044689,0.988282393439497,0.987616798999169)))
REPRESENTATION_ITEM('')
SURFACE()
);
#1645=(
BOUNDED_SURFACE()
B_SPLINE_SURFACE(1,2,((#121980,#121981,#121982,#121983,#121984),(#121985,
#121986,#121987,#121988,#121989)),.UNSPECIFIED.,.F.,.F.,.F.)
B_SPLINE_SURFACE_WITH_KNOTS((2,2),(3,2,3),(0.710318915639153,1.),(0.487155140750429,
0.5,0.504719756176226),.UNSPECIFIED.)
GEOMETRIC_REPRESENTATION_ITEM()
RATIONAL_B_SPLINE_SURFACE(((0.992604240083356,0.995491335852357,1.,0.99834332202137,
0.996905579294146),(0.992604240083356,0.995491335852357,1.,0.99834332202137,
0.996905579294146)))
REPRESENTATION_ITEM('')
SURFACE()
);
#1646=(
BOUNDED_SURFACE()
B_SPLINE_SURFACE(1,2,((#122006,#122007,#122008),(#122009,#122010,#122011)),
 .UNSPECIFIED.,.F.,.F.,.F.)
B_SPLINE_SURFACE_WITH_KNOTS((2,2),(3,3),(0.710192959007513,1.),(0.22888337489481,
0.246056477139965),.UNSPECIFIED.)
GEOMETRIC_REPRESENTATION_ITEM()
RATIONAL_B_SPLINE_SURFACE(((0.991846493044689,0.988282393439497,0.987616798999169),
(0.991846493044689,0.988282393439497,0.987616798999169)))
REPRESENTATION_ITEM('')
SURFACE()
);
#1647=(
BOUNDED_SURFACE()
B_SPLINE_SURFACE(1,2,((#122019,#122020,#122021,#122022,#122023),(#122024,
#122025,#122026,#122027,#122028)),.UNSPECIFIED.,.F.,.F.,.F.)
B_SPLINE_SURFACE_WITH_KNOTS((2,2),(3,2,3),(0.710318915639152,1.),(0.487155140750429,
0.5,0.504719756176227),.UNSPECIFIED.)
GEOMETRIC_REPRESENTATION_ITEM()
RATIONAL_B_SPLINE_SURFACE(((0.992604240083356,0.995491335852357,1.,0.99834332202137,
0.996905579294146),(0.992604240083356,0.995491335852357,1.,0.99834332202137,
0.996905579294146)))
REPRESENTATION_ITEM('')
SURFACE()
);
#1648=(
BOUNDED_SURFACE()
B_SPLINE_SURFACE(1,2,((#122045,#122046,#122047),(#122048,#122049,#122050)),
 .UNSPECIFIED.,.F.,.F.,.F.)
B_SPLINE_SURFACE_WITH_KNOTS((2,2),(3,3),(0.710192959007511,1.),(0.22888337489481,
0.246056477139965),.UNSPECIFIED.)
GEOMETRIC_REPRESENTATION_ITEM()
RATIONAL_B_SPLINE_SURFACE(((0.991846493044689,0.988282393439497,0.987616798999169),
(0.991846493044689,0.988282393439497,0.987616798999169)))
REPRESENTATION_ITEM('')
SURFACE()
);
#1649=(
BOUNDED_SURFACE()
B_SPLINE_SURFACE(1,2,((#122058,#122059,#122060,#122061,#122062),(#122063,
#122064,#122065,#122066,#122067)),.UNSPECIFIED.,.F.,.F.,.F.)
B_SPLINE_SURFACE_WITH_KNOTS((2,2),(3,2,3),(0.710318915639148,1.),(0.487155140750429,
0.5,0.504719756176227),.UNSPECIFIED.)
GEOMETRIC_REPRESENTATION_ITEM()
RATIONAL_B_SPLINE_SURFACE(((0.992604240083356,0.995491335852357,1.,0.99834332202137,
0.996905579294146),(0.992604240083356,0.995491335852357,1.,0.99834332202137,
0.996905579294146)))
REPRESENTATION_ITEM('')
SURFACE()
);
#1650=(
BOUNDED_SURFACE()
B_SPLINE_SURFACE(1,2,((#122084,#122085,#122086),(#122087,#122088,#122089)),
 .UNSPECIFIED.,.F.,.F.,.F.)
B_SPLINE_SURFACE_WITH_KNOTS((2,2),(3,3),(0.71019295900751,1.),(0.22888337489481,
0.246056477139966),.UNSPECIFIED.)
GEOMETRIC_REPRESENTATION_ITEM()
RATIONAL_B_SPLINE_SURFACE(((0.991846493044689,0.988282393439497,0.987616798999169),
(0.991846493044689,0.988282393439497,0.987616798999169)))
REPRESENTATION_ITEM('')
SURFACE()
);
#1651=(
BOUNDED_SURFACE()
B_SPLINE_SURFACE(1,2,((#122097,#122098,#122099,#122100,#122101),(#122102,
#122103,#122104,#122105,#122106)),.UNSPECIFIED.,.F.,.F.,.F.)
B_SPLINE_SURFACE_WITH_KNOTS((2,2),(3,2,3),(0.710318915638565,1.),(0.487155140750429,
0.5,0.504719756176227),.UNSPECIFIED.)
GEOMETRIC_REPRESENTATION_ITEM()
RATIONAL_B_SPLINE_SURFACE(((0.992604240083356,0.995491335852357,1.,0.99834332202137,
0.996905579294146),(0.992604240083356,0.995491335852357,1.,0.99834332202137,
0.996905579294146)))
REPRESENTATION_ITEM('')
SURFACE()
);
#1652=(
BOUNDED_SURFACE()
B_SPLINE_SURFACE(1,2,((#122123,#122124,#122125),(#122126,#122127,#122128)),
 .UNSPECIFIED.,.F.,.F.,.F.)
B_SPLINE_SURFACE_WITH_KNOTS((2,2),(3,3),(0.710192959006924,1.),(0.22888337489481,
0.246056477139965),.UNSPECIFIED.)
GEOMETRIC_REPRESENTATION_ITEM()
RATIONAL_B_SPLINE_SURFACE(((0.991846493044689,0.988282393439497,0.987616798999169),
(0.991846493044689,0.988282393439497,0.987616798999169)))
REPRESENTATION_ITEM('')
SURFACE()
);
#1653=(
BOUNDED_SURFACE()
B_SPLINE_SURFACE(1,2,((#122136,#122137,#122138,#122139,#122140),(#122141,
#122142,#122143,#122144,#122145)),.UNSPECIFIED.,.F.,.F.,.F.)
B_SPLINE_SURFACE_WITH_KNOTS((2,2),(3,2,3),(0.710318915639151,1.),(0.487155140750429,
0.5,0.504719756176227),.UNSPECIFIED.)
GEOMETRIC_REPRESENTATION_ITEM()
RATIONAL_B_SPLINE_SURFACE(((0.992604240083356,0.995491335852357,1.,0.99834332202137,
0.996905579294146),(0.992604240083356,0.995491335852357,1.,0.99834332202137,
0.996905579294146)))
REPRESENTATION_ITEM('')
SURFACE()
);
#1654=(
BOUNDED_SURFACE()
B_SPLINE_SURFACE(1,2,((#122162,#122163,#122164),(#122165,#122166,#122167)),
 .UNSPECIFIED.,.F.,.F.,.F.)
B_SPLINE_SURFACE_WITH_KNOTS((2,2),(3,3),(0.710192959007512,1.),(0.22888337489481,
0.246056477139966),.UNSPECIFIED.)
GEOMETRIC_REPRESENTATION_ITEM()
RATIONAL_B_SPLINE_SURFACE(((0.991846493044689,0.988282393439497,0.987616798999169),
(0.991846493044689,0.988282393439497,0.987616798999169)))
REPRESENTATION_ITEM('')
SURFACE()
);
#1655=(
BOUNDED_SURFACE()
B_SPLINE_SURFACE(1,2,((#122175,#122176,#122177,#122178,#122179),(#122180,
#122181,#122182,#122183,#122184)),.UNSPECIFIED.,.F.,.F.,.F.)
B_SPLINE_SURFACE_WITH_KNOTS((2,2),(3,2,3),(0.710318915638566,1.),(0.487155140750429,
0.5,0.504719756176226),.UNSPECIFIED.)
GEOMETRIC_REPRESENTATION_ITEM()
RATIONAL_B_SPLINE_SURFACE(((0.992604240083356,0.995491335852357,1.,0.99834332202137,
0.996905579294146),(0.992604240083356,0.995491335852357,1.,0.99834332202137,
0.996905579294146)))
REPRESENTATION_ITEM('')
SURFACE()
);
#1656=(
BOUNDED_SURFACE()
B_SPLINE_SURFACE(1,2,((#122201,#122202,#122203),(#122204,#122205,#122206)),
 .UNSPECIFIED.,.F.,.F.,.F.)
B_SPLINE_SURFACE_WITH_KNOTS((2,2),(3,3),(0.710192959006926,1.),(0.22888337489481,
0.246056477139965),.UNSPECIFIED.)
GEOMETRIC_REPRESENTATION_ITEM()
RATIONAL_B_SPLINE_SURFACE(((0.991846493044689,0.988282393439497,0.987616798999169),
(0.991846493044689,0.988282393439497,0.987616798999169)))
REPRESENTATION_ITEM('')
SURFACE()
);
#1657=(
BOUNDED_SURFACE()
B_SPLINE_SURFACE(1,2,((#122214,#122215,#122216,#122217,#122218),(#122219,
#122220,#122221,#122222,#122223)),.UNSPECIFIED.,.F.,.F.,.F.)
B_SPLINE_SURFACE_WITH_KNOTS((2,2),(3,2,3),(0.710318915639068,1.),(0.48715514075043,
0.5,0.504719756176227),.UNSPECIFIED.)
GEOMETRIC_REPRESENTATION_ITEM()
RATIONAL_B_SPLINE_SURFACE(((0.992604240083356,0.995491335852357,1.,0.99834332202137,
0.996905579294146),(0.992604240083356,0.995491335852357,1.,0.99834332202137,
0.996905579294146)))
REPRESENTATION_ITEM('')
SURFACE()
);
#1658=(
BOUNDED_SURFACE()
B_SPLINE_SURFACE(1,2,((#122240,#122241,#122242),(#122243,#122244,#122245)),
 .UNSPECIFIED.,.F.,.F.,.F.)
B_SPLINE_SURFACE_WITH_KNOTS((2,2),(3,3),(0.71019295900743,1.),(0.228883374894809,
0.246056477139964),.UNSPECIFIED.)
GEOMETRIC_REPRESENTATION_ITEM()
RATIONAL_B_SPLINE_SURFACE(((0.991846493044689,0.988282393439498,0.987616798999169),
(0.991846493044689,0.988282393439498,0.987616798999169)))
REPRESENTATION_ITEM('')
SURFACE()
);
#1659=(
BOUNDED_SURFACE()
B_SPLINE_SURFACE(1,2,((#122253,#122254,#122255,#122256,#122257),(#122258,
#122259,#122260,#122261,#122262)),.UNSPECIFIED.,.F.,.F.,.F.)
B_SPLINE_SURFACE_WITH_KNOTS((2,2),(3,2,3),(0.710318915639073,1.),(0.48715514075043,
0.5,0.504719756176228),.UNSPECIFIED.)
GEOMETRIC_REPRESENTATION_ITEM()
RATIONAL_B_SPLINE_SURFACE(((0.992604240083356,0.995491335852357,1.,0.998343322021369,
0.996905579294145),(0.992604240083356,0.995491335852357,1.,0.998343322021369,
0.996905579294145)))
REPRESENTATION_ITEM('')
SURFACE()
);
#1660=(
BOUNDED_SURFACE()
B_SPLINE_SURFACE(1,2,((#122279,#122280,#122281),(#122282,#122283,#122284)),
 .UNSPECIFIED.,.F.,.F.,.F.)
B_SPLINE_SURFACE_WITH_KNOTS((2,2),(3,3),(0.710192959007434,1.),(0.228883374894809,
0.246056477139964),.UNSPECIFIED.)
GEOMETRIC_REPRESENTATION_ITEM()
RATIONAL_B_SPLINE_SURFACE(((0.991846493044689,0.988282393439498,0.987616798999169),
(0.991846493044689,0.988282393439498,0.987616798999169)))
REPRESENTATION_ITEM('')
SURFACE()
);
#1661=(
BOUNDED_SURFACE()
B_SPLINE_SURFACE(1,2,((#122292,#122293,#122294,#122295,#122296),(#122297,
#122298,#122299,#122300,#122301)),.UNSPECIFIED.,.F.,.F.,.F.)
B_SPLINE_SURFACE_WITH_KNOTS((2,2),(3,2,3),(0.710318915638474,1.),(0.48715514075043,
0.5,0.504719756176228),.UNSPECIFIED.)
GEOMETRIC_REPRESENTATION_ITEM()
RATIONAL_B_SPLINE_SURFACE(((0.992604240083356,0.995491335852357,1.,0.998343322021369,
0.996905579294145),(0.992604240083356,0.995491335852357,1.,0.998343322021369,
0.996905579294145)))
REPRESENTATION_ITEM('')
SURFACE()
);
#1662=(
BOUNDED_SURFACE()
B_SPLINE_SURFACE(1,2,((#122318,#122319,#122320),(#122321,#122322,#122323)),
 .UNSPECIFIED.,.F.,.F.,.F.)
B_SPLINE_SURFACE_WITH_KNOTS((2,2),(3,3),(0.710192959006835,1.),(0.228883374894809,
0.246056477139964),.UNSPECIFIED.)
GEOMETRIC_REPRESENTATION_ITEM()
RATIONAL_B_SPLINE_SURFACE(((0.991846493044689,0.988282393439498,0.987616798999169),
(0.991846493044689,0.988282393439498,0.987616798999169)))
REPRESENTATION_ITEM('')
SURFACE()
);
#1663=(
BOUNDED_SURFACE()
B_SPLINE_SURFACE(1,2,((#122331,#122332,#122333,#122334,#122335),(#122336,
#122337,#122338,#122339,#122340)),.UNSPECIFIED.,.F.,.F.,.F.)
B_SPLINE_SURFACE_WITH_KNOTS((2,2),(3,2,3),(0.710318915639067,1.),(0.48715514075043,
0.5,0.504719756176228),.UNSPECIFIED.)
GEOMETRIC_REPRESENTATION_ITEM()
RATIONAL_B_SPLINE_SURFACE(((0.992604240083356,0.995491335852357,1.,0.998343322021369,
0.996905579294145),(0.992604240083356,0.995491335852357,1.,0.998343322021369,
0.996905579294145)))
REPRESENTATION_ITEM('')
SURFACE()
);
#1664=(
BOUNDED_SURFACE()
B_SPLINE_SURFACE(1,2,((#122357,#122358,#122359),(#122360,#122361,#122362)),
 .UNSPECIFIED.,.F.,.F.,.F.)
B_SPLINE_SURFACE_WITH_KNOTS((2,2),(3,3),(0.710192959007425,1.),(0.228883374894809,
0.246056477139964),.UNSPECIFIED.)
GEOMETRIC_REPRESENTATION_ITEM()
RATIONAL_B_SPLINE_SURFACE(((0.991846493044689,0.988282393439498,0.987616798999169),
(0.991846493044689,0.988282393439498,0.987616798999169)))
REPRESENTATION_ITEM('')
SURFACE()
);
#1665=(
BOUNDED_SURFACE()
B_SPLINE_SURFACE(1,2,((#122370,#122371,#122372,#122373,#122374),(#122375,
#122376,#122377,#122378,#122379)),.UNSPECIFIED.,.F.,.F.,.F.)
B_SPLINE_SURFACE_WITH_KNOTS((2,2),(3,2,3),(0.710318915638563,1.),(0.48715514075043,
0.5,0.504719756176228),.UNSPECIFIED.)
GEOMETRIC_REPRESENTATION_ITEM()
RATIONAL_B_SPLINE_SURFACE(((0.992604240083356,0.995491335852357,1.,0.998343322021369,
0.996905579294145),(0.992604240083356,0.995491335852357,1.,0.998343322021369,
0.996905579294145)))
REPRESENTATION_ITEM('')
SURFACE()
);
#1666=(
BOUNDED_SURFACE()
B_SPLINE_SURFACE(1,2,((#122396,#122397,#122398),(#122399,#122400,#122401)),
 .UNSPECIFIED.,.F.,.F.,.F.)
B_SPLINE_SURFACE_WITH_KNOTS((2,2),(3,3),(0.710192959006925,1.),(0.228883374894809,
0.246056477139964),.UNSPECIFIED.)
GEOMETRIC_REPRESENTATION_ITEM()
RATIONAL_B_SPLINE_SURFACE(((0.991846493044689,0.988282393439498,0.987616798999169),
(0.991846493044689,0.988282393439498,0.987616798999169)))
REPRESENTATION_ITEM('')
SURFACE()
);
#1667=(
BOUNDED_SURFACE()
B_SPLINE_SURFACE(1,2,((#122409,#122410,#122411,#122412,#122413),(#122414,
#122415,#122416,#122417,#122418)),.UNSPECIFIED.,.F.,.F.,.F.)
B_SPLINE_SURFACE_WITH_KNOTS((2,2),(3,2,3),(0.71031891563906,1.),(0.48715514075043,
0.5,0.504719756176228),.UNSPECIFIED.)
GEOMETRIC_REPRESENTATION_ITEM()
RATIONAL_B_SPLINE_SURFACE(((0.992604240083356,0.995491335852357,1.,0.998343322021369,
0.996905579294145),(0.992604240083356,0.995491335852357,1.,0.998343322021369,
0.996905579294145)))
REPRESENTATION_ITEM('')
SURFACE()
);
#1668=(
BOUNDED_SURFACE()
B_SPLINE_SURFACE(1,2,((#122435,#122436,#122437),(#122438,#122439,#122440)),
 .UNSPECIFIED.,.F.,.F.,.F.)
B_SPLINE_SURFACE_WITH_KNOTS((2,2),(3,3),(0.710192959007421,1.),(0.228883374894809,
0.246056477139964),.UNSPECIFIED.)
GEOMETRIC_REPRESENTATION_ITEM()
RATIONAL_B_SPLINE_SURFACE(((0.991846493044689,0.988282393439498,0.987616798999169),
(0.991846493044689,0.988282393439498,0.987616798999169)))
REPRESENTATION_ITEM('')
SURFACE()
);
#1669=(
BOUNDED_SURFACE()
B_SPLINE_SURFACE(1,2,((#122448,#122449,#122450,#122451,#122452),(#122453,
#122454,#122455,#122456,#122457)),.UNSPECIFIED.,.F.,.F.,.F.)
B_SPLINE_SURFACE_WITH_KNOTS((2,2),(3,2,3),(0.710318915638562,1.),(0.48715514075043,
0.5,0.504719756176228),.UNSPECIFIED.)
GEOMETRIC_REPRESENTATION_ITEM()
RATIONAL_B_SPLINE_SURFACE(((0.992604240083356,0.995491335852357,1.,0.998343322021369,
0.996905579294145),(0.992604240083356,0.995491335852357,1.,0.998343322021369,
0.996905579294145)))
REPRESENTATION_ITEM('')
SURFACE()
);
#1670=(
BOUNDED_SURFACE()
B_SPLINE_SURFACE(1,2,((#122474,#122475,#122476),(#122477,#122478,#122479)),
 .UNSPECIFIED.,.F.,.F.,.F.)
B_SPLINE_SURFACE_WITH_KNOTS((2,2),(3,3),(0.710192959006918,1.),(0.228883374894809,
0.246056477139964),.UNSPECIFIED.)
GEOMETRIC_REPRESENTATION_ITEM()
RATIONAL_B_SPLINE_SURFACE(((0.991846493044689,0.988282393439498,0.987616798999169),
(0.991846493044689,0.988282393439498,0.987616798999169)))
REPRESENTATION_ITEM('')
SURFACE()
);
#1671=(
BOUNDED_SURFACE()
B_SPLINE_SURFACE(1,2,((#122487,#122488,#122489,#122490,#122491),(#122492,
#122493,#122494,#122495,#122496)),.UNSPECIFIED.,.F.,.F.,.F.)
B_SPLINE_SURFACE_WITH_KNOTS((2,2),(3,2,3),(0.710318915638789,1.),(0.48715514075043,
0.5,0.504719756176228),.UNSPECIFIED.)
GEOMETRIC_REPRESENTATION_ITEM()
RATIONAL_B_SPLINE_SURFACE(((0.992604240083356,0.995491335852357,1.,0.998343322021369,
0.996905579294145),(0.992604240083356,0.995491335852357,1.,0.998343322021369,
0.996905579294145)))
REPRESENTATION_ITEM('')
SURFACE()
);
#1672=(
BOUNDED_SURFACE()
B_SPLINE_SURFACE(1,2,((#122504,#122505,#122506),(#122507,#122508,#122509)),
 .UNSPECIFIED.,.F.,.F.,.F.)
B_SPLINE_SURFACE_WITH_KNOTS((2,2),(3,3),(0.710192959007146,1.),(0.228883374894809,
0.246056477139964),.UNSPECIFIED.)
GEOMETRIC_REPRESENTATION_ITEM()
RATIONAL_B_SPLINE_SURFACE(((0.991846493044689,0.988282393439498,0.987616798999169),
(0.991846493044689,0.988282393439498,0.987616798999169)))
REPRESENTATION_ITEM('')
SURFACE()
);
#1673=(
BOUNDED_SURFACE()
B_SPLINE_SURFACE(1,2,((#122511,#122512,#122513,#122514,#122515),(#122516,
#122517,#122518,#122519,#122520)),.UNSPECIFIED.,.F.,.F.,.F.)
B_SPLINE_SURFACE_WITH_KNOTS((2,2),(3,2,3),(0.710318915637747,1.),(0.48715514075043,
0.5,0.504719756176228),.UNSPECIFIED.)
GEOMETRIC_REPRESENTATION_ITEM()
RATIONAL_B_SPLINE_SURFACE(((0.992604240083356,0.995491335852357,1.,0.998343322021369,
0.996905579294145),(0.992604240083356,0.995491335852357,1.,0.998343322021369,
0.996905579294145)))
REPRESENTATION_ITEM('')
SURFACE()
);
#1674=(
BOUNDED_SURFACE()
B_SPLINE_SURFACE(1,2,((#122537,#122538,#122539),(#122540,#122541,#122542)),
 .UNSPECIFIED.,.F.,.F.,.F.)
B_SPLINE_SURFACE_WITH_KNOTS((2,2),(3,3),(0.710192959006102,1.),(0.228883374894809,
0.246056477139964),.UNSPECIFIED.)
GEOMETRIC_REPRESENTATION_ITEM()
RATIONAL_B_SPLINE_SURFACE(((0.991846493044689,0.988282393439498,0.987616798999169),
(0.991846493044689,0.988282393439498,0.987616798999169)))
REPRESENTATION_ITEM('')
SURFACE()
);
#1675=(
BOUNDED_SURFACE()
B_SPLINE_SURFACE(1,2,((#122550,#122551,#122552,#122553,#122554),(#122555,
#122556,#122557,#122558,#122559)),.UNSPECIFIED.,.F.,.F.,.F.)
B_SPLINE_SURFACE_WITH_KNOTS((2,2),(3,2,3),(0.710318915639029,1.),(0.48715514075043,
0.5,0.50471975617623),.UNSPECIFIED.)
GEOMETRIC_REPRESENTATION_ITEM()
RATIONAL_B_SPLINE_SURFACE(((0.992604240083356,0.995491335852357,1.,0.998343322021369,
0.996905579294144),(0.992604240083356,0.995491335852357,1.,0.998343322021369,
0.996905579294144)))
REPRESENTATION_ITEM('')
SURFACE()
);
#1676=(
BOUNDED_SURFACE()
B_SPLINE_SURFACE(1,2,((#122576,#122577,#122578),(#122579,#122580,#122581)),
 .UNSPECIFIED.,.F.,.F.,.F.)
B_SPLINE_SURFACE_WITH_KNOTS((2,2),(3,3),(0.710192959007385,1.),(0.228883374894809,
0.246056477139964),.UNSPECIFIED.)
GEOMETRIC_REPRESENTATION_ITEM()
RATIONAL_B_SPLINE_SURFACE(((0.991846493044689,0.988282393439498,0.987616798999169),
(0.991846493044689,0.988282393439498,0.987616798999169)))
REPRESENTATION_ITEM('')
SURFACE()
);
#1677=(
BOUNDED_SURFACE()
B_SPLINE_SURFACE(1,2,((#122589,#122590,#122591,#122592,#122593),(#122594,
#122595,#122596,#122597,#122598)),.UNSPECIFIED.,.F.,.F.,.F.)
B_SPLINE_SURFACE_WITH_KNOTS((2,2),(3,2,3),(0.710318915639146,1.),(0.48715514075043,
0.5,0.504719756176228),.UNSPECIFIED.)
GEOMETRIC_REPRESENTATION_ITEM()
RATIONAL_B_SPLINE_SURFACE(((0.992604240083356,0.995491335852357,1.,0.998343322021369,
0.996905579294145),(0.992604240083356,0.995491335852357,1.,0.998343322021369,
0.996905579294145)))
REPRESENTATION_ITEM('')
SURFACE()
);
#1678=(
BOUNDED_SURFACE()
B_SPLINE_SURFACE(1,2,((#122615,#122616,#122617),(#122618,#122619,#122620)),
 .UNSPECIFIED.,.F.,.F.,.F.)
B_SPLINE_SURFACE_WITH_KNOTS((2,2),(3,3),(0.710192959007501,1.),(0.228883374894809,
0.246056477139964),.UNSPECIFIED.)
GEOMETRIC_REPRESENTATION_ITEM()
RATIONAL_B_SPLINE_SURFACE(((0.991846493044689,0.988282393439498,0.987616798999169),
(0.991846493044689,0.988282393439498,0.987616798999169)))
REPRESENTATION_ITEM('')
SURFACE()
);
#1679=(
BOUNDED_SURFACE()
B_SPLINE_SURFACE(1,2,((#122628,#122629,#122630,#122631,#122632),(#122633,
#122634,#122635,#122636,#122637)),.UNSPECIFIED.,.F.,.F.,.F.)
B_SPLINE_SURFACE_WITH_KNOTS((2,2),(3,2,3),(0.710318915638505,1.),(0.48715514075043,
0.5,0.504719756176228),.UNSPECIFIED.)
GEOMETRIC_REPRESENTATION_ITEM()
RATIONAL_B_SPLINE_SURFACE(((0.992604240083356,0.995491335852357,1.,0.998343322021369,
0.996905579294145),(0.992604240083356,0.995491335852357,1.,0.998343322021369,
0.996905579294145)))
REPRESENTATION_ITEM('')
SURFACE()
);
#1680=(
BOUNDED_SURFACE()
B_SPLINE_SURFACE(1,2,((#122654,#122655,#122656),(#122657,#122658,#122659)),
 .UNSPECIFIED.,.F.,.F.,.F.)
B_SPLINE_SURFACE_WITH_KNOTS((2,2),(3,3),(0.710192959006866,1.),(0.228883374894552,
0.246056477139966),.UNSPECIFIED.)
GEOMETRIC_REPRESENTATION_ITEM()
RATIONAL_B_SPLINE_SURFACE(((0.991846493044796,0.988282393439507,0.987616798999169),
(0.991846493044796,0.988282393439507,0.987616798999169)))
REPRESENTATION_ITEM('')
SURFACE()
);
#1681=(
BOUNDED_SURFACE()
B_SPLINE_SURFACE(1,2,((#122667,#122668,#122669,#122670,#122671),(#122672,
#122673,#122674,#122675,#122676)),.UNSPECIFIED.,.F.,.F.,.F.)
B_SPLINE_SURFACE_WITH_KNOTS((2,2),(3,2,3),(0.710318915639913,1.),(0.48715514075043,
0.5,0.504719756176227),.UNSPECIFIED.)
GEOMETRIC_REPRESENTATION_ITEM()
RATIONAL_B_SPLINE_SURFACE(((0.992604240083356,0.995491335852357,1.,0.998343322021369,
0.996905579294145),(0.992604240083356,0.995491335852357,1.,0.998343322021369,
0.996905579294145)))
REPRESENTATION_ITEM('')
SURFACE()
);
#1682=(
BOUNDED_SURFACE()
B_SPLINE_SURFACE(1,2,((#122693,#122694,#122695),(#122696,#122697,#122698)),
 .UNSPECIFIED.,.F.,.F.,.F.)
B_SPLINE_SURFACE_WITH_KNOTS((2,2),(3,3),(0.710192959008272,1.),(0.228883374894663,
0.246056477139965),.UNSPECIFIED.)
GEOMETRIC_REPRESENTATION_ITEM()
RATIONAL_B_SPLINE_SURFACE(((0.99184649304475,0.988282393439503,0.987616798999169),
(0.99184649304475,0.988282393439503,0.987616798999169)))
REPRESENTATION_ITEM('')
SURFACE()
);
#1683=(
BOUNDED_SURFACE()
B_SPLINE_SURFACE(1,2,((#122706,#122707,#122708,#122709,#122710),(#122711,
#122712,#122713,#122714,#122715)),.UNSPECIFIED.,.F.,.F.,.F.)
B_SPLINE_SURFACE_WITH_KNOTS((2,2),(3,2,3),(0.710318915638763,1.),(0.48715514075043,
0.5,0.504719756176228),.UNSPECIFIED.)
GEOMETRIC_REPRESENTATION_ITEM()
RATIONAL_B_SPLINE_SURFACE(((0.992604240083356,0.995491335852357,1.,0.998343322021369,
0.996905579294145),(0.992604240083356,0.995491335852357,1.,0.998343322021369,
0.996905579294145)))
REPRESENTATION_ITEM('')
SURFACE()
);
#1684=(
BOUNDED_SURFACE()
B_SPLINE_SURFACE(1,2,((#122732,#122733,#122734),(#122735,#122736,#122737)),
 .UNSPECIFIED.,.F.,.F.,.F.)
B_SPLINE_SURFACE_WITH_KNOTS((2,2),(3,3),(0.710192959007122,1.),(0.228883374894809,
0.246056477139964),.UNSPECIFIED.)
GEOMETRIC_REPRESENTATION_ITEM()
RATIONAL_B_SPLINE_SURFACE(((0.991846493044689,0.988282393439497,0.987616798999169),
(0.991846493044689,0.988282393439497,0.987616798999169)))
REPRESENTATION_ITEM('')
SURFACE()
);
#1685=(
BOUNDED_SURFACE()
B_SPLINE_SURFACE(1,2,((#122745,#122746,#122747,#122748,#122749),(#122750,
#122751,#122752,#122753,#122754)),.UNSPECIFIED.,.F.,.F.,.F.)
B_SPLINE_SURFACE_WITH_KNOTS((2,2),(3,2,3),(0.710318915638795,1.),(0.48715514075043,
0.5,0.504719756176228),.UNSPECIFIED.)
GEOMETRIC_REPRESENTATION_ITEM()
RATIONAL_B_SPLINE_SURFACE(((0.992604240083356,0.995491335852357,1.,0.998343322021369,
0.996905579294145),(0.992604240083356,0.995491335852357,1.,0.998343322021369,
0.996905579294145)))
REPRESENTATION_ITEM('')
SURFACE()
);
#1686=(
BOUNDED_SURFACE()
B_SPLINE_SURFACE(1,2,((#122771,#122772,#122773),(#122774,#122775,#122776)),
 .UNSPECIFIED.,.F.,.F.,.F.)
B_SPLINE_SURFACE_WITH_KNOTS((2,2),(3,3),(0.710192959007302,1.),(0.228883374894523,
0.246056477139966),.UNSPECIFIED.)
GEOMETRIC_REPRESENTATION_ITEM()
RATIONAL_B_SPLINE_SURFACE(((0.991846493044808,0.988282393439508,0.987616798999169),
(0.991846493044808,0.988282393439508,0.987616798999169)))
REPRESENTATION_ITEM('')
SURFACE()
);
#1687=(
BOUNDED_SURFACE()
B_SPLINE_SURFACE(1,2,((#122784,#122785,#122786,#122787,#122788),(#122789,
#122790,#122791,#122792,#122793)),.UNSPECIFIED.,.F.,.F.,.F.)
B_SPLINE_SURFACE_WITH_KNOTS((2,2),(3,2,3),(0.710318915638241,1.),(0.48715514075043,
0.5,0.504719756176228),.UNSPECIFIED.)
GEOMETRIC_REPRESENTATION_ITEM()
RATIONAL_B_SPLINE_SURFACE(((0.992604240083356,0.995491335852357,1.,0.998343322021369,
0.996905579294145),(0.992604240083356,0.995491335852357,1.,0.998343322021369,
0.996905579294145)))
REPRESENTATION_ITEM('')
SURFACE()
);
#1688=(
BOUNDED_SURFACE()
B_SPLINE_SURFACE(1,2,((#122810,#122811,#122812),(#122813,#122814,#122815)),
 .UNSPECIFIED.,.F.,.F.,.F.)
B_SPLINE_SURFACE_WITH_KNOTS((2,2),(3,3),(0.710192959006596,1.),(0.228883374894657,
0.246056477139965),.UNSPECIFIED.)
GEOMETRIC_REPRESENTATION_ITEM()
RATIONAL_B_SPLINE_SURFACE(((0.991846493044752,0.988282393439503,0.987616798999169),
(0.991846493044752,0.988282393439503,0.987616798999169)))
REPRESENTATION_ITEM('')
SURFACE()
);
#1689=(
BOUNDED_SURFACE()
B_SPLINE_SURFACE(1,2,((#122823,#122824,#122825,#122826,#122827),(#122828,
#122829,#122830,#122831,#122832)),.UNSPECIFIED.,.F.,.F.,.F.)
B_SPLINE_SURFACE_WITH_KNOTS((2,2),(3,2,3),(0.710318915639737,1.),(0.48715514075043,
0.5,0.504719756176228),.UNSPECIFIED.)
GEOMETRIC_REPRESENTATION_ITEM()
RATIONAL_B_SPLINE_SURFACE(((0.992604240083356,0.995491335852357,1.,0.998343322021369,
0.996905579294145),(0.992604240083356,0.995491335852357,1.,0.998343322021369,
0.996905579294145)))
REPRESENTATION_ITEM('')
SURFACE()
);
#1690=(
BOUNDED_SURFACE()
B_SPLINE_SURFACE(1,2,((#122849,#122850,#122851),(#122852,#122853,#122854)),
 .UNSPECIFIED.,.F.,.F.,.F.)
B_SPLINE_SURFACE_WITH_KNOTS((2,2),(3,3),(0.710192959008097,1.),(0.228883374894707,
0.246056477139965),.UNSPECIFIED.)
GEOMETRIC_REPRESENTATION_ITEM()
RATIONAL_B_SPLINE_SURFACE(((0.991846493044731,0.988282393439501,0.987616798999169),
(0.991846493044731,0.988282393439501,0.987616798999169)))
REPRESENTATION_ITEM('')
SURFACE()
);
#1691=(
BOUNDED_SURFACE()
B_SPLINE_SURFACE(1,2,((#122862,#122863,#122864,#122865,#122866),(#122867,
#122868,#122869,#122870,#122871)),.UNSPECIFIED.,.F.,.F.,.F.)
B_SPLINE_SURFACE_WITH_KNOTS((2,2),(3,2,3),(0.710318915638587,1.),(0.48715514075043,
0.5,0.50471975617627),.UNSPECIFIED.)
GEOMETRIC_REPRESENTATION_ITEM()
RATIONAL_B_SPLINE_SURFACE(((0.992604240083356,0.995491335852357,1.,0.998343322021354,
0.996905579294119),(0.992604240083356,0.995491335852357,1.,0.998343322021354,
0.996905579294119)))
REPRESENTATION_ITEM('')
SURFACE()
);
#1692=(
BOUNDED_SURFACE()
B_SPLINE_SURFACE(1,2,((#122888,#122889,#122890),(#122891,#122892,#122893)),
 .UNSPECIFIED.,.F.,.F.,.F.)
B_SPLINE_SURFACE_WITH_KNOTS((2,2),(3,3),(0.710192959006951,1.),(0.22888337489478,
0.246056477139965),.UNSPECIFIED.)
GEOMETRIC_REPRESENTATION_ITEM()
RATIONAL_B_SPLINE_SURFACE(((0.991846493044701,0.988282393439499,0.987616798999169),
(0.991846493044701,0.988282393439499,0.987616798999169)))
REPRESENTATION_ITEM('')
SURFACE()
);
#1693=(
BOUNDED_SURFACE()
B_SPLINE_SURFACE(1,2,((#122901,#122902,#122903,#122904,#122905),(#122906,
#122907,#122908,#122909,#122910)),.UNSPECIFIED.,.F.,.F.,.F.)
B_SPLINE_SURFACE_WITH_KNOTS((2,2),(3,2,3),(0.710318915638838,1.),(0.48715514075043,
0.5,0.504719756176235),.UNSPECIFIED.)
GEOMETRIC_REPRESENTATION_ITEM()
RATIONAL_B_SPLINE_SURFACE(((0.992604240083356,0.995491335852357,1.,0.998343322021367,
0.996905579294141),(0.992604240083356,0.995491335852357,1.,0.998343322021367,
0.996905579294141)))
REPRESENTATION_ITEM('')
SURFACE()
);
#1694=(
BOUNDED_SURFACE()
B_SPLINE_SURFACE(1,2,((#122927,#122928,#122929),(#122930,#122931,#122932)),
 .UNSPECIFIED.,.F.,.F.,.F.)
B_SPLINE_SURFACE_WITH_KNOTS((2,2),(3,3),(0.710192959007197,1.),(0.228883374894804,
0.246056477139964),.UNSPECIFIED.)
GEOMETRIC_REPRESENTATION_ITEM()
RATIONAL_B_SPLINE_SURFACE(((0.991846493044691,0.988282393439498,0.987616798999169),
(0.991846493044691,0.988282393439498,0.987616798999169)))
REPRESENTATION_ITEM('')
SURFACE()
);
#1695=(
BOUNDED_SURFACE()
B_SPLINE_SURFACE(1,2,((#122940,#122941,#122942,#122943,#122944),(#122945,
#122946,#122947,#122948,#122949)),.UNSPECIFIED.,.F.,.F.,.F.)
B_SPLINE_SURFACE_WITH_KNOTS((2,2),(3,2,3),(0.710318915639088,1.),(0.48715514075043,
0.5,0.504719756176228),.UNSPECIFIED.)
GEOMETRIC_REPRESENTATION_ITEM()
RATIONAL_B_SPLINE_SURFACE(((0.992604240083356,0.995491335852357,1.,0.998343322021369,
0.996905579294145),(0.992604240083356,0.995491335852357,1.,0.998343322021369,
0.996905579294145)))
REPRESENTATION_ITEM('')
SURFACE()
);
#1696=(
BOUNDED_SURFACE()
B_SPLINE_SURFACE(1,2,((#122966,#122967,#122968),(#122969,#122970,#122971)),
 .UNSPECIFIED.,.F.,.F.,.F.)
B_SPLINE_SURFACE_WITH_KNOTS((2,2),(3,3),(0.710192959007447,1.),(0.228883374894809,
0.246056477139964),.UNSPECIFIED.)
GEOMETRIC_REPRESENTATION_ITEM()
RATIONAL_B_SPLINE_SURFACE(((0.991846493044689,0.988282393439498,0.987616798999169),
(0.991846493044689,0.988282393439498,0.987616798999169)))
REPRESENTATION_ITEM('')
SURFACE()
);
#1697=(
BOUNDED_SURFACE()
B_SPLINE_SURFACE(1,2,((#122979,#122980,#122981,#122982,#122983),(#122984,
#122985,#122986,#122987,#122988)),.UNSPECIFIED.,.F.,.F.,.F.)
B_SPLINE_SURFACE_WITH_KNOTS((2,2),(3,2,3),(0.710318915639149,1.),(0.48715514075043,
0.5,0.504719756176302),.UNSPECIFIED.)
GEOMETRIC_REPRESENTATION_ITEM()
RATIONAL_B_SPLINE_SURFACE(((0.992604240083356,0.995491335852357,1.,0.998343322021343,
0.9969055792941),(0.992604240083356,0.995491335852357,1.,0.998343322021343,
0.9969055792941)))
REPRESENTATION_ITEM('')
SURFACE()
);
#1698=(
BOUNDED_SURFACE()
B_SPLINE_SURFACE(1,2,((#123005,#123006,#123007),(#123008,#123009,#123010)),
 .UNSPECIFIED.,.F.,.F.,.F.)
B_SPLINE_SURFACE_WITH_KNOTS((2,2),(3,3),(0.710192959007517,1.),(0.228883374894809,
0.246056477139966),.UNSPECIFIED.)
GEOMETRIC_REPRESENTATION_ITEM()
RATIONAL_B_SPLINE_SURFACE(((0.991846493044689,0.988282393439497,0.987616798999169),
(0.991846493044689,0.988282393439497,0.987616798999169)))
REPRESENTATION_ITEM('')
SURFACE()
);
#1699=(
BOUNDED_SURFACE()
B_SPLINE_SURFACE(1,2,((#123018,#123019,#123020,#123021,#123022),(#123023,
#123024,#123025,#123026,#123027)),.UNSPECIFIED.,.F.,.F.,.F.)
B_SPLINE_SURFACE_WITH_KNOTS((2,2),(3,2,3),(0.710318915637906,1.),(0.487155140750422,
0.5,0.504719756176228),.UNSPECIFIED.)
GEOMETRIC_REPRESENTATION_ITEM()
RATIONAL_B_SPLINE_SURFACE(((0.992604240083352,0.995491335852354,1.,0.998343322021369,
0.996905579294145),(0.992604240083352,0.995491335852354,1.,0.998343322021369,
0.996905579294145)))
REPRESENTATION_ITEM('')
SURFACE()
);
#1700=(
BOUNDED_SURFACE()
B_SPLINE_SURFACE(1,2,((#123044,#123045,#123046),(#123047,#123048,#123049)),
 .UNSPECIFIED.,.F.,.F.,.F.)
B_SPLINE_SURFACE_WITH_KNOTS((2,2),(3,3),(0.710192959006267,1.),(0.22888337489481,
0.246056477139964),.UNSPECIFIED.)
GEOMETRIC_REPRESENTATION_ITEM()
RATIONAL_B_SPLINE_SURFACE(((0.991846493044689,0.988282393439498,0.987616798999169),
(0.991846493044689,0.988282393439498,0.987616798999169)))
REPRESENTATION_ITEM('')
SURFACE()
);
#1701=(
BOUNDED_SURFACE()
B_SPLINE_SURFACE(1,2,((#123069,#123070,#123071,#123072,#123073),(#123074,
#123075,#123076,#123077,#123078)),.UNSPECIFIED.,.F.,.F.,.F.)
B_SPLINE_SURFACE_WITH_KNOTS((2,2),(3,2,3),(0.710318915640079,1.),(0.487155140750429,
0.5,0.504719756176227),.UNSPECIFIED.)
GEOMETRIC_REPRESENTATION_ITEM()
RATIONAL_B_SPLINE_SURFACE(((0.992604240083356,0.995491335852357,1.,0.99834332202137,
0.996905579294146),(0.992604240083356,0.995491335852357,1.,0.99834332202137,
0.996905579294146)))
REPRESENTATION_ITEM('')
SURFACE()
);
#1702=(
BOUNDED_SURFACE()
B_SPLINE_SURFACE(1,2,((#123080,#123081,#123082),(#123083,#123084,#123085)),
 .UNSPECIFIED.,.F.,.F.,.F.)
B_SPLINE_SURFACE_WITH_KNOTS((2,2),(3,3),(0.710318915640052,1.),(0.262994994770441,
0.280433083165913),.UNSPECIFIED.)
GEOMETRIC_REPRESENTATION_ITEM()
RATIONAL_B_SPLINE_SURFACE(((0.989123653000982,0.991350813683903,0.996566619267863),
(0.989123653000982,0.991350813683903,0.996566619267863)))
REPRESENTATION_ITEM('')
SURFACE()
);
#1703=(
BOUNDED_SURFACE()
B_SPLINE_SURFACE(1,2,((#123094,#123095,#123096,#123097,#123098),(#123099,
#123100,#123101,#123102,#123103)),.UNSPECIFIED.,.F.,.F.,.F.)
B_SPLINE_SURFACE_WITH_KNOTS((2,2),(3,2,3),(0.709601334832402,1.),(0.452333244836385,
0.452924869174518,0.470122329512318),.UNSPECIFIED.)
GEOMETRIC_REPRESENTATION_ITEM()
RATIONAL_B_SPLINE_SURFACE(((0.988732477628005,0.988732477628005,0.988732477628005,
0.986812255267055,0.987798766302166),(0.988732477628005,0.988732477628005,
0.988732477628005,0.986812255267055,0.987798766302166)))
REPRESENTATION_ITEM('')
SURFACE()
);
#1704=(
BOUNDED_SURFACE()
B_SPLINE_SURFACE(1,2,((#123112,#123113,#123114),(#123115,#123116,#123117)),
 .UNSPECIFIED.,.F.,.F.,.F.)
B_SPLINE_SURFACE_WITH_KNOTS((2,2),(3,3),(0.710318915640047,1.),(0.262994994770441,
0.280433083165913),.UNSPECIFIED.)
GEOMETRIC_REPRESENTATION_ITEM()
RATIONAL_B_SPLINE_SURFACE(((0.989123653000982,0.991350813683903,0.996566619267863),
(0.989123653000982,0.991350813683903,0.996566619267863)))
REPRESENTATION_ITEM('')
SURFACE()
);
#1705=(
BOUNDED_SURFACE()
B_SPLINE_SURFACE(1,2,((#123119,#123120,#123121,#123122,#123123),(#123124,
#123125,#123126,#123127,#123128)),.UNSPECIFIED.,.F.,.F.,.F.)
B_SPLINE_SURFACE_WITH_KNOTS((2,2),(3,2,3),(0.709601334818244,1.),(0.452333244822231,
0.452924869174517,0.470122329512318),.UNSPECIFIED.)
GEOMETRIC_REPRESENTATION_ITEM()
RATIONAL_B_SPLINE_SURFACE(((0.988732477628005,0.988732477628005,0.988732477628005,
0.986812255267055,0.987798766302166),(0.988732477628005,0.988732477628005,
0.988732477628005,0.986812255267055,0.987798766302167)))
REPRESENTATION_ITEM('')
SURFACE()
);
#1706=(
BOUNDED_SURFACE()
B_SPLINE_SURFACE(1,2,((#123137,#123138,#123139),(#123140,#123141,#123142)),
 .UNSPECIFIED.,.F.,.F.,.F.)
B_SPLINE_SURFACE_WITH_KNOTS((2,2),(3,3),(0.71031891564004,1.),(0.262994994770441,
0.280433083165913),.UNSPECIFIED.)
GEOMETRIC_REPRESENTATION_ITEM()
RATIONAL_B_SPLINE_SURFACE(((0.989123653000982,0.991350813683903,0.996566619267863),
(0.989123653000982,0.991350813683903,0.996566619267863)))
REPRESENTATION_ITEM('')
SURFACE()
);
#1707=(
BOUNDED_SURFACE()
B_SPLINE_SURFACE(1,2,((#123144,#123145,#123146,#123147,#123148),(#123149,
#123150,#123151,#123152,#123153)),.UNSPECIFIED.,.F.,.F.,.F.)
B_SPLINE_SURFACE_WITH_KNOTS((2,2),(3,2,3),(0.70960133484095,1.),(0.452333244844927,
0.452924869174518,0.470122329512318),.UNSPECIFIED.)
GEOMETRIC_REPRESENTATION_ITEM()
RATIONAL_B_SPLINE_SURFACE(((0.988732477628005,0.988732477628005,0.988732477628005,
0.986812255267055,0.987798766302166),(0.988732477628005,0.988732477628005,
0.988732477628005,0.986812255267055,0.987798766302166)))
REPRESENTATION_ITEM('')
SURFACE()
);
#1708=(
BOUNDED_SURFACE()
B_SPLINE_SURFACE(1,2,((#123162,#123163,#123164),(#123165,#123166,#123167)),
 .UNSPECIFIED.,.F.,.F.,.F.)
B_SPLINE_SURFACE_WITH_KNOTS((2,2),(3,3),(0.710318915640049,1.),(0.262994994770441,
0.280433083165913),.UNSPECIFIED.)
GEOMETRIC_REPRESENTATION_ITEM()
RATIONAL_B_SPLINE_SURFACE(((0.989123653000982,0.991350813683903,0.996566619267863),
(0.989123653000982,0.991350813683903,0.996566619267863)))
REPRESENTATION_ITEM('')
SURFACE()
);
#1709=(
BOUNDED_SURFACE()
B_SPLINE_SURFACE(1,2,((#123169,#123170,#123171,#123172,#123173),(#123174,
#123175,#123176,#123177,#123178)),.UNSPECIFIED.,.F.,.F.,.F.)
B_SPLINE_SURFACE_WITH_KNOTS((2,2),(3,2,3),(0.709601334842905,1.),(0.452333244847841,
0.452924869174518,0.470122329512318),.UNSPECIFIED.)
GEOMETRIC_REPRESENTATION_ITEM()
RATIONAL_B_SPLINE_SURFACE(((0.988732477628005,0.988732477628005,0.988732477628005,
0.986812255267055,0.987798766302166),(0.988732477628005,0.988732477628005,
0.988732477628005,0.986812255267055,0.987798766302166)))
REPRESENTATION_ITEM('')
SURFACE()
);
#1710=(
BOUNDED_SURFACE()
B_SPLINE_SURFACE(1,2,((#123187,#123188,#123189),(#123190,#123191,#123192)),
 .UNSPECIFIED.,.F.,.F.,.F.)
B_SPLINE_SURFACE_WITH_KNOTS((2,2),(3,3),(0.710318915639097,1.),(0.262994994770441,
0.280433083165913),.UNSPECIFIED.)
GEOMETRIC_REPRESENTATION_ITEM()
RATIONAL_B_SPLINE_SURFACE(((0.989123653000982,0.991350813683903,0.996566619267863),
(0.989123653000982,0.991350813683903,0.996566619267863)))
REPRESENTATION_ITEM('')
SURFACE()
);
#1711=(
BOUNDED_SURFACE()
B_SPLINE_SURFACE(1,2,((#123194,#123195,#123196,#123197,#123198),(#123199,
#123200,#123201,#123202,#123203)),.UNSPECIFIED.,.F.,.F.,.F.)
B_SPLINE_SURFACE_WITH_KNOTS((2,2),(3,2,3),(0.709601334842701,1.),(0.452333244847627,
0.452924869174518,0.470122329512318),.UNSPECIFIED.)
GEOMETRIC_REPRESENTATION_ITEM()
RATIONAL_B_SPLINE_SURFACE(((0.988732477628005,0.988732477628005,0.988732477628005,
0.986812255267055,0.987798766302167),(0.988732477628005,0.988732477628005,
0.988732477628005,0.986812255267055,0.987798766302166)))
REPRESENTATION_ITEM('')
SURFACE()
);
#1712=(
BOUNDED_SURFACE()
B_SPLINE_SURFACE(1,2,((#123212,#123213,#123214),(#123215,#123216,#123217)),
 .UNSPECIFIED.,.F.,.F.,.F.)
B_SPLINE_SURFACE_WITH_KNOTS((2,2),(3,3),(0.710318915639107,1.),(0.262994994770441,
0.280433083165913),.UNSPECIFIED.)
GEOMETRIC_REPRESENTATION_ITEM()
RATIONAL_B_SPLINE_SURFACE(((0.989123653000982,0.991350813683903,0.996566619267863),
(0.989123653000982,0.991350813683903,0.996566619267863)))
REPRESENTATION_ITEM('')
SURFACE()
);
#1713=(
BOUNDED_SURFACE()
B_SPLINE_SURFACE(1,2,((#123219,#123220,#123221,#123222,#123223),(#123224,
#123225,#123226,#123227,#123228)),.UNSPECIFIED.,.F.,.F.,.F.)
B_SPLINE_SURFACE_WITH_KNOTS((2,2),(3,2,3),(0.709601334846431,1.),(0.45233324485132,
0.452924869174518,0.470122329512318),.UNSPECIFIED.)
GEOMETRIC_REPRESENTATION_ITEM()
RATIONAL_B_SPLINE_SURFACE(((0.988732477628005,0.988732477628005,0.988732477628005,
0.986812255267055,0.987798766302166),(0.988732477628005,0.988732477628005,
0.988732477628005,0.986812255267055,0.987798766302166)))
REPRESENTATION_ITEM('')
SURFACE()
);
#1714=(
BOUNDED_SURFACE()
B_SPLINE_SURFACE(1,2,((#123237,#123238,#123239),(#123240,#123241,#123242)),
 .UNSPECIFIED.,.F.,.F.,.F.)
B_SPLINE_SURFACE_WITH_KNOTS((2,2),(3,3),(0.710318915639146,1.),(0.262994994770441,
0.280433083165913),.UNSPECIFIED.)
GEOMETRIC_REPRESENTATION_ITEM()
RATIONAL_B_SPLINE_SURFACE(((0.989123653000982,0.991350813683903,0.996566619267863),
(0.989123653000982,0.991350813683903,0.996566619267863)))
REPRESENTATION_ITEM('')
SURFACE()
);
#1715=(
BOUNDED_SURFACE()
B_SPLINE_SURFACE(1,2,((#123244,#123245,#123246,#123247,#123248),(#123249,
#123250,#123251,#123252,#123253)),.UNSPECIFIED.,.F.,.F.,.F.)
B_SPLINE_SURFACE_WITH_KNOTS((2,2),(3,2,3),(0.70960133484861,1.),(0.452333244853516,
0.452924869174518,0.470122329512318),.UNSPECIFIED.)
GEOMETRIC_REPRESENTATION_ITEM()
RATIONAL_B_SPLINE_SURFACE(((0.988732477628005,0.988732477628005,0.988732477628005,
0.986812255267055,0.987798766302166),(0.988732477628005,0.988732477628005,
0.988732477628005,0.986812255267055,0.987798766302166)))
REPRESENTATION_ITEM('')
SURFACE()
);
#1716=(
BOUNDED_SURFACE()
B_SPLINE_SURFACE(1,2,((#123262,#123263,#123264),(#123265,#123266,#123267)),
 .UNSPECIFIED.,.F.,.F.,.F.)
B_SPLINE_SURFACE_WITH_KNOTS((2,2),(3,3),(0.710318915639129,1.),(0.262994994770441,
0.280433083165913),.UNSPECIFIED.)
GEOMETRIC_REPRESENTATION_ITEM()
RATIONAL_B_SPLINE_SURFACE(((0.989123653000982,0.991350813683903,0.996566619267863),
(0.989123653000982,0.991350813683903,0.996566619267863)))
REPRESENTATION_ITEM('')
SURFACE()
);
#1717=(
BOUNDED_SURFACE()
B_SPLINE_SURFACE(1,2,((#123269,#123270,#123271,#123272,#123273),(#123274,
#123275,#123276,#123277,#123278)),.UNSPECIFIED.,.F.,.F.,.F.)
B_SPLINE_SURFACE_WITH_KNOTS((2,2),(3,2,3),(0.709601334844663,1.),(0.452333244848607,
0.452924869174518,0.470122329512318),.UNSPECIFIED.)
GEOMETRIC_REPRESENTATION_ITEM()
RATIONAL_B_SPLINE_SURFACE(((0.988732477628005,0.988732477628005,0.988732477628005,
0.986812255267055,0.987798766302166),(0.988732477628005,0.988732477628005,
0.988732477628005,0.986812255267055,0.987798766302166)))
REPRESENTATION_ITEM('')
SURFACE()
);
#1718=(
BOUNDED_SURFACE()
B_SPLINE_SURFACE(1,2,((#123287,#123288,#123289),(#123290,#123291,#123292)),
 .UNSPECIFIED.,.F.,.F.,.F.)
B_SPLINE_SURFACE_WITH_KNOTS((2,2),(3,3),(0.710318915640079,1.),(0.262994994770441,
0.280433083165913),.UNSPECIFIED.)
GEOMETRIC_REPRESENTATION_ITEM()
RATIONAL_B_SPLINE_SURFACE(((0.989123653000982,0.991350813683903,0.996566619267863),
(0.989123653000982,0.991350813683903,0.996566619267863)))
REPRESENTATION_ITEM('')
SURFACE()
);
#1719=(
BOUNDED_SURFACE()
B_SPLINE_SURFACE(1,2,((#123294,#123295,#123296,#123297,#123298),(#123299,
#123300,#123301,#123302,#123303)),.UNSPECIFIED.,.F.,.F.,.F.)
B_SPLINE_SURFACE_WITH_KNOTS((2,2),(3,2,3),(0.709601334851136,1.),(0.452333244855082,
0.452924869174517,0.470122329512318),.UNSPECIFIED.)
GEOMETRIC_REPRESENTATION_ITEM()
RATIONAL_B_SPLINE_SURFACE(((0.988732477628005,0.988732477628005,0.988732477628005,
0.986812255267055,0.987798766302167),(0.988732477628005,0.988732477628005,
0.988732477628005,0.986812255267055,0.987798766302167)))
REPRESENTATION_ITEM('')
SURFACE()
);
#1720=(
BOUNDED_SURFACE()
B_SPLINE_SURFACE(1,2,((#123312,#123313,#123314),(#123315,#123316,#123317)),
 .UNSPECIFIED.,.F.,.F.,.F.)
B_SPLINE_SURFACE_WITH_KNOTS((2,2),(3,3),(0.71031891564008,1.),(0.262994994770441,
0.280433083165913),.UNSPECIFIED.)
GEOMETRIC_REPRESENTATION_ITEM()
RATIONAL_B_SPLINE_SURFACE(((0.989123653000982,0.991350813683903,0.996566619267863),
(0.989123653000982,0.991350813683903,0.996566619267863)))
REPRESENTATION_ITEM('')
SURFACE()
);
#1721=(
BOUNDED_SURFACE()
B_SPLINE_SURFACE(1,2,((#123319,#123320,#123321,#123322,#123323),(#123324,
#123325,#123326,#123327,#123328)),.UNSPECIFIED.,.F.,.F.,.F.)
B_SPLINE_SURFACE_WITH_KNOTS((2,2),(3,2,3),(0.709601334824955,1.),(0.452333244828901,
0.452924869174518,0.47012232951232),.UNSPECIFIED.)
GEOMETRIC_REPRESENTATION_ITEM()
RATIONAL_B_SPLINE_SURFACE(((0.988732477628005,0.988732477628005,0.988732477628005,
0.986812255267055,0.987798766302167),(0.988732477628005,0.988732477628005,
0.988732477628005,0.986812255267055,0.987798766302167)))
REPRESENTATION_ITEM('')
SURFACE()
);
#1722=(
BOUNDED_SURFACE()
B_SPLINE_SURFACE(1,2,((#123337,#123338,#123339),(#123340,#123341,#123342)),
 .UNSPECIFIED.,.F.,.F.,.F.)
B_SPLINE_SURFACE_WITH_KNOTS((2,2),(3,3),(0.710318915639993,1.),(0.262994994770443,
0.280433083165914),.UNSPECIFIED.)
GEOMETRIC_REPRESENTATION_ITEM()
RATIONAL_B_SPLINE_SURFACE(((0.989123653000983,0.991350813683904,0.996566619267864),
(0.989123653000983,0.991350813683904,0.996566619267864)))
REPRESENTATION_ITEM('')
SURFACE()
);
#1723=(
BOUNDED_SURFACE()
B_SPLINE_SURFACE(1,2,((#123344,#123345,#123346,#123347,#123348),(#123349,
#123350,#123351,#123352,#123353)),.UNSPECIFIED.,.F.,.F.,.F.)
B_SPLINE_SURFACE_WITH_KNOTS((2,2),(3,2,3),(0.709601334825716,1.),(0.452333244829658,
0.452924869174518,0.470122329512318),.UNSPECIFIED.)
GEOMETRIC_REPRESENTATION_ITEM()
RATIONAL_B_SPLINE_SURFACE(((0.988732477628005,0.988732477628005,0.988732477628005,
0.986812255267055,0.987798766302166),(0.988732477628005,0.988732477628005,
0.988732477628005,0.986812255267055,0.987798766302166)))
REPRESENTATION_ITEM('')
SURFACE()
);
#1724=(
BOUNDED_SURFACE()
B_SPLINE_SURFACE(1,2,((#123362,#123363,#123364),(#123365,#123366,#123367)),
 .UNSPECIFIED.,.F.,.F.,.F.)
B_SPLINE_SURFACE_WITH_KNOTS((2,2),(3,3),(0.710318915640073,1.),(0.262994994770443,
0.280433083165913),.UNSPECIFIED.)
GEOMETRIC_REPRESENTATION_ITEM()
RATIONAL_B_SPLINE_SURFACE(((0.989123653000983,0.991350813683904,0.996566619267863),
(0.989123653000983,0.991350813683904,0.996566619267863)))
REPRESENTATION_ITEM('')
SURFACE()
);
#1725=(
BOUNDED_SURFACE()
B_SPLINE_SURFACE(1,2,((#123369,#123370,#123371,#123372,#123373),(#123374,
#123375,#123376,#123377,#123378)),.UNSPECIFIED.,.F.,.F.,.F.)
B_SPLINE_SURFACE_WITH_KNOTS((2,2),(3,2,3),(0.709601334819264,1.),(0.452333244823207,
0.452924869174518,0.470122329512318),.UNSPECIFIED.)
GEOMETRIC_REPRESENTATION_ITEM()
RATIONAL_B_SPLINE_SURFACE(((0.988732477628005,0.988732477628005,0.988732477628005,
0.986812255267055,0.987798766302166),(0.988732477628005,0.988732477628005,
0.988732477628005,0.986812255267055,0.987798766302166)))
REPRESENTATION_ITEM('')
SURFACE()
);
#1726=(
BOUNDED_SURFACE()
B_SPLINE_SURFACE(1,2,((#123387,#123388,#123389),(#123390,#123391,#123392)),
 .UNSPECIFIED.,.F.,.F.,.F.)
B_SPLINE_SURFACE_WITH_KNOTS((2,2),(3,3),(0.710318915640082,1.),(0.262994994770441,
0.280433083165913),.UNSPECIFIED.)
GEOMETRIC_REPRESENTATION_ITEM()
RATIONAL_B_SPLINE_SURFACE(((0.989123653000982,0.991350813683903,0.996566619267863),
(0.989123653000982,0.991350813683903,0.996566619267863)))
REPRESENTATION_ITEM('')
SURFACE()
);
#1727=(
BOUNDED_SURFACE()
B_SPLINE_SURFACE(1,2,((#123394,#123395,#123396,#123397,#123398),(#123399,
#123400,#123401,#123402,#123403)),.UNSPECIFIED.,.F.,.F.,.F.)
B_SPLINE_SURFACE_WITH_KNOTS((2,2),(3,2,3),(0.709601334846308,1.),(0.452333244850251,
0.452924869174518,0.470122329512318),.UNSPECIFIED.)
GEOMETRIC_REPRESENTATION_ITEM()
RATIONAL_B_SPLINE_SURFACE(((0.988732477628005,0.988732477628005,0.988732477628005,
0.986812255267055,0.987798766302166),(0.988732477628005,0.988732477628005,
0.988732477628005,0.986812255267055,0.987798766302166)))
REPRESENTATION_ITEM('')
SURFACE()
);
#1728=(
BOUNDED_SURFACE()
B_SPLINE_SURFACE(1,2,((#123412,#123413,#123414),(#123415,#123416,#123417)),
 .UNSPECIFIED.,.F.,.F.,.F.)
B_SPLINE_SURFACE_WITH_KNOTS((2,2),(3,3),(0.710318915640072,1.),(0.262994994770441,
0.280433083165913),.UNSPECIFIED.)
GEOMETRIC_REPRESENTATION_ITEM()
RATIONAL_B_SPLINE_SURFACE(((0.989123653000982,0.991350813683903,0.996566619267863),
(0.989123653000982,0.991350813683903,0.996566619267863)))
REPRESENTATION_ITEM('')
SURFACE()
);
#1729=(
BOUNDED_SURFACE()
B_SPLINE_SURFACE(1,2,((#123419,#123420,#123421,#123422,#123423),(#123424,
#123425,#123426,#123427,#123428)),.UNSPECIFIED.,.F.,.F.,.F.)
B_SPLINE_SURFACE_WITH_KNOTS((2,2),(3,2,3),(0.70960133482498,1.),(0.452333244828929,
0.452924869174518,0.470122329512318),.UNSPECIFIED.)
GEOMETRIC_REPRESENTATION_ITEM()
RATIONAL_B_SPLINE_SURFACE(((0.988732477628005,0.988732477628005,0.988732477628005,
0.986812255267055,0.987798766302166),(0.988732477628005,0.988732477628005,
0.988732477628005,0.986812255267055,0.987798766302166)))
REPRESENTATION_ITEM('')
SURFACE()
);
#1730=(
BOUNDED_SURFACE()
B_SPLINE_SURFACE(1,2,((#123437,#123438,#123439),(#123440,#123441,#123442)),
 .UNSPECIFIED.,.F.,.F.,.F.)
B_SPLINE_SURFACE_WITH_KNOTS((2,2),(3,3),(0.710318915640073,1.),(0.262994994770441,
0.280433083165913),.UNSPECIFIED.)
GEOMETRIC_REPRESENTATION_ITEM()
RATIONAL_B_SPLINE_SURFACE(((0.989123653000982,0.991350813683903,0.996566619267864),
(0.989123653000982,0.991350813683903,0.996566619267864)))
REPRESENTATION_ITEM('')
SURFACE()
);
#1731=(
BOUNDED_SURFACE()
B_SPLINE_SURFACE(1,2,((#123444,#123445,#123446,#123447,#123448),(#123449,
#123450,#123451,#123452,#123453)),.UNSPECIFIED.,.F.,.F.,.F.)
B_SPLINE_SURFACE_WITH_KNOTS((2,2),(3,2,3),(0.709601334843721,1.),(0.452333244847661,
0.452924869174518,0.470122329512318),.UNSPECIFIED.)
GEOMETRIC_REPRESENTATION_ITEM()
RATIONAL_B_SPLINE_SURFACE(((0.988732477628005,0.988732477628005,0.988732477628005,
0.986812255267055,0.987798766302166),(0.988732477628005,0.988732477628005,
0.988732477628005,0.986812255267055,0.987798766302166)))
REPRESENTATION_ITEM('')
SURFACE()
);
#1732=(
BOUNDED_SURFACE()
B_SPLINE_SURFACE(1,2,((#123462,#123463,#123464),(#123465,#123466,#123467)),
 .UNSPECIFIED.,.F.,.F.,.F.)
B_SPLINE_SURFACE_WITH_KNOTS((2,2),(3,3),(0.710318915640077,1.),(0.262994994770441,
0.280433083165913),.UNSPECIFIED.)
GEOMETRIC_REPRESENTATION_ITEM()
RATIONAL_B_SPLINE_SURFACE(((0.989123653000982,0.991350813683903,0.996566619267863),
(0.989123653000982,0.991350813683903,0.996566619267863)))
REPRESENTATION_ITEM('')
SURFACE()
);
#1733=(
BOUNDED_SURFACE()
B_SPLINE_SURFACE(1,2,((#123469,#123470,#123471,#123472,#123473),(#123474,
#123475,#123476,#123477,#123478)),.UNSPECIFIED.,.F.,.F.,.F.)
B_SPLINE_SURFACE_WITH_KNOTS((2,2),(3,2,3),(0.709601334848688,1.),(0.452333244852634,
0.452924869174518,0.470122329512318),.UNSPECIFIED.)
GEOMETRIC_REPRESENTATION_ITEM()
RATIONAL_B_SPLINE_SURFACE(((0.988732477628005,0.988732477628005,0.988732477628005,
0.986812255267055,0.987798766302167),(0.988732477628005,0.988732477628005,
0.988732477628005,0.986812255267055,0.987798766302167)))
REPRESENTATION_ITEM('')
SURFACE()
);
#1734=(
BOUNDED_SURFACE()
B_SPLINE_SURFACE(1,2,((#123487,#123488,#123489),(#123490,#123491,#123492)),
 .UNSPECIFIED.,.F.,.F.,.F.)
B_SPLINE_SURFACE_WITH_KNOTS((2,2),(3,3),(0.710318915640071,1.),(0.262994994770441,
0.280433083165913),.UNSPECIFIED.)
GEOMETRIC_REPRESENTATION_ITEM()
RATIONAL_B_SPLINE_SURFACE(((0.989123653000982,0.991350813683903,0.996566619267863),
(0.989123653000982,0.991350813683903,0.996566619267863)))
REPRESENTATION_ITEM('')
SURFACE()
);
#1735=(
BOUNDED_SURFACE()
B_SPLINE_SURFACE(1,2,((#123494,#123495,#123496,#123497,#123498),(#123499,
#123500,#123501,#123502,#123503)),.UNSPECIFIED.,.F.,.F.,.F.)
B_SPLINE_SURFACE_WITH_KNOTS((2,2),(3,2,3),(0.709601334852901,1.),(0.452333244856846,
0.452924869174518,0.470122329512318),.UNSPECIFIED.)
GEOMETRIC_REPRESENTATION_ITEM()
RATIONAL_B_SPLINE_SURFACE(((0.988732477628005,0.988732477628005,0.988732477628005,
0.986812255267055,0.987798766302167),(0.988732477628005,0.988732477628005,
0.988732477628005,0.986812255267055,0.987798766302167)))
REPRESENTATION_ITEM('')
SURFACE()
);
#1736=(
BOUNDED_SURFACE()
B_SPLINE_SURFACE(1,2,((#123512,#123513,#123514),(#123515,#123516,#123517)),
 .UNSPECIFIED.,.F.,.F.,.F.)
B_SPLINE_SURFACE_WITH_KNOTS((2,2),(3,3),(0.710318915640077,1.),(0.262994994770441,
0.280433083165913),.UNSPECIFIED.)
GEOMETRIC_REPRESENTATION_ITEM()
RATIONAL_B_SPLINE_SURFACE(((0.989123653000982,0.991350813683903,0.996566619267863),
(0.989123653000982,0.991350813683903,0.996566619267863)))
REPRESENTATION_ITEM('')
SURFACE()
);
#1737=(
BOUNDED_SURFACE()
B_SPLINE_SURFACE(1,2,((#123519,#123520,#123521,#123522,#123523),(#123524,
#123525,#123526,#123527,#123528)),.UNSPECIFIED.,.F.,.F.,.F.)
B_SPLINE_SURFACE_WITH_KNOTS((2,2),(3,2,3),(0.70960133485792,1.),(0.452333244861864,
0.452924869174518,0.470122329512318),.UNSPECIFIED.)
GEOMETRIC_REPRESENTATION_ITEM()
RATIONAL_B_SPLINE_SURFACE(((0.988732477628005,0.988732477628005,0.988732477628005,
0.986812255267055,0.987798766302166),(0.988732477628005,0.988732477628005,
0.988732477628005,0.986812255267055,0.987798766302166)))
REPRESENTATION_ITEM('')
SURFACE()
);
#1738=(
BOUNDED_SURFACE()
B_SPLINE_SURFACE(1,2,((#123537,#123538,#123539),(#123540,#123541,#123542)),
 .UNSPECIFIED.,.F.,.F.,.F.)
B_SPLINE_SURFACE_WITH_KNOTS((2,2),(3,3),(0.710318915640081,1.),(0.262994994770441,
0.280433083165913),.UNSPECIFIED.)
GEOMETRIC_REPRESENTATION_ITEM()
RATIONAL_B_SPLINE_SURFACE(((0.989123653000982,0.991350813683903,0.996566619267863),
(0.989123653000982,0.991350813683903,0.996566619267863)))
REPRESENTATION_ITEM('')
SURFACE()
);
#1739=(
BOUNDED_SURFACE()
B_SPLINE_SURFACE(1,2,((#123544,#123545,#123546,#123547,#123548),(#123549,
#123550,#123551,#123552,#123553)),.UNSPECIFIED.,.F.,.F.,.F.)
B_SPLINE_SURFACE_WITH_KNOTS((2,2),(3,2,3),(0.709601334827665,1.),(0.45233324483161,
0.452924869174518,0.470122329512318),.UNSPECIFIED.)
GEOMETRIC_REPRESENTATION_ITEM()
RATIONAL_B_SPLINE_SURFACE(((0.988732477628005,0.988732477628005,0.988732477628005,
0.986812255267055,0.987798766302166),(0.988732477628005,0.988732477628005,
0.988732477628005,0.986812255267055,0.987798766302166)))
REPRESENTATION_ITEM('')
SURFACE()
);
#1740=(
BOUNDED_SURFACE()
B_SPLINE_SURFACE(1,2,((#123562,#123563,#123564),(#123565,#123566,#123567)),
 .UNSPECIFIED.,.F.,.F.,.F.)
B_SPLINE_SURFACE_WITH_KNOTS((2,2),(3,3),(0.710318915640078,1.),(0.262994994770441,
0.280433083165913),.UNSPECIFIED.)
GEOMETRIC_REPRESENTATION_ITEM()
RATIONAL_B_SPLINE_SURFACE(((0.989123653000982,0.991350813683903,0.996566619267863),
(0.989123653000982,0.991350813683903,0.996566619267863)))
REPRESENTATION_ITEM('')
SURFACE()
);
#1741=(
BOUNDED_SURFACE()
B_SPLINE_SURFACE(1,2,((#123569,#123570,#123571,#123572,#123573),(#123574,
#123575,#123576,#123577,#123578)),.UNSPECIFIED.,.F.,.F.,.F.)
B_SPLINE_SURFACE_WITH_KNOTS((2,2),(3,2,3),(0.70960133482239,1.),(0.452333244827756,
0.452924869174518,0.470122329512318),.UNSPECIFIED.)
GEOMETRIC_REPRESENTATION_ITEM()
RATIONAL_B_SPLINE_SURFACE(((0.988732477628005,0.988732477628005,0.988732477628005,
0.986812255267055,0.987798766302166),(0.988732477628005,0.988732477628005,
0.988732477628005,0.986812255267055,0.987798766302166)))
REPRESENTATION_ITEM('')
SURFACE()
);
#1742=(
BOUNDED_SURFACE()
B_SPLINE_SURFACE(1,2,((#123587,#123588,#123589),(#123590,#123591,#123592)),
 .UNSPECIFIED.,.F.,.F.,.F.)
B_SPLINE_SURFACE_WITH_KNOTS((2,2),(3,3),(0.710318915638669,1.),(0.262994994770441,
0.280433083165913),.UNSPECIFIED.)
GEOMETRIC_REPRESENTATION_ITEM()
RATIONAL_B_SPLINE_SURFACE(((0.989123653000982,0.991350813683903,0.996566619267863),
(0.989123653000982,0.991350813683903,0.996566619267863)))
REPRESENTATION_ITEM('')
SURFACE()
);
#1743=(
BOUNDED_SURFACE()
B_SPLINE_SURFACE(1,2,((#123594,#123595,#123596,#123597,#123598),(#123599,
#123600,#123601,#123602,#123603)),.UNSPECIFIED.,.F.,.F.,.F.)
B_SPLINE_SURFACE_WITH_KNOTS((2,2),(3,2,3),(0.709601334823023,1.),(0.452333244826969,
0.452924869174518,0.470122329512318),.UNSPECIFIED.)
GEOMETRIC_REPRESENTATION_ITEM()
RATIONAL_B_SPLINE_SURFACE(((0.988732477628005,0.988732477628005,0.988732477628005,
0.986812255267055,0.987798766302166),(0.988732477628005,0.988732477628005,
0.988732477628005,0.986812255267055,0.987798766302166)))
REPRESENTATION_ITEM('')
SURFACE()
);
#1744=(
BOUNDED_SURFACE()
B_SPLINE_SURFACE(1,2,((#123612,#123613,#123614),(#123615,#123616,#123617)),
 .UNSPECIFIED.,.F.,.F.,.F.)
B_SPLINE_SURFACE_WITH_KNOTS((2,2),(3,3),(0.710318915640086,1.),(0.262994994770441,
0.280433083165913),.UNSPECIFIED.)
GEOMETRIC_REPRESENTATION_ITEM()
RATIONAL_B_SPLINE_SURFACE(((0.989123653000982,0.991350813683903,0.996566619267863),
(0.989123653000982,0.991350813683903,0.996566619267863)))
REPRESENTATION_ITEM('')
SURFACE()
);
#1745=(
BOUNDED_SURFACE()
B_SPLINE_SURFACE(1,2,((#123619,#123620,#123621,#123622,#123623),(#123624,
#123625,#123626,#123627,#123628)),.UNSPECIFIED.,.F.,.F.,.F.)
B_SPLINE_SURFACE_WITH_KNOTS((2,2),(3,2,3),(0.709601334842211,1.),(0.452333244846155,
0.452924869174518,0.47012232951232),.UNSPECIFIED.)
GEOMETRIC_REPRESENTATION_ITEM()
RATIONAL_B_SPLINE_SURFACE(((0.988732477628005,0.988732477628005,0.988732477628005,
0.986812255267055,0.987798766302167),(0.988732477628005,0.988732477628005,
0.988732477628005,0.986812255267055,0.987798766302167)))
REPRESENTATION_ITEM('')
SURFACE()
);
#1746=(
BOUNDED_SURFACE()
B_SPLINE_SURFACE(1,2,((#123637,#123638,#123639),(#123640,#123641,#123642)),
 .UNSPECIFIED.,.F.,.F.,.F.)
B_SPLINE_SURFACE_WITH_KNOTS((2,2),(3,3),(0.710318915640079,1.),(0.262994994770444,
0.280433083165913),.UNSPECIFIED.)
GEOMETRIC_REPRESENTATION_ITEM()
RATIONAL_B_SPLINE_SURFACE(((0.989123653000983,0.991350813683904,0.996566619267863),
(0.989123653000983,0.991350813683904,0.996566619267863)))
REPRESENTATION_ITEM('')
SURFACE()
);
#1747=(
BOUNDED_SURFACE()
B_SPLINE_SURFACE(1,2,((#123644,#123645,#123646,#123647,#123648),(#123649,
#123650,#123651,#123652,#123653)),.UNSPECIFIED.,.F.,.F.,.F.)
B_SPLINE_SURFACE_WITH_KNOTS((2,2),(3,2,3),(0.709601334832975,1.),(0.452333244836997,
0.452924869174517,0.470122329512317),.UNSPECIFIED.)
GEOMETRIC_REPRESENTATION_ITEM()
RATIONAL_B_SPLINE_SURFACE(((0.988732477628005,0.988732477628005,0.988732477628005,
0.986812255267055,0.987798766302166),(0.988732477628005,0.988732477628005,
0.988732477628005,0.986812255267055,0.987798766302166)))
REPRESENTATION_ITEM('')
SURFACE()
);
#1748=(
BOUNDED_SURFACE()
B_SPLINE_SURFACE(1,2,((#123662,#123663,#123664),(#123665,#123666,#123667)),
 .UNSPECIFIED.,.F.,.F.,.F.)
B_SPLINE_SURFACE_WITH_KNOTS((2,2),(3,3),(0.710318915640007,1.),(0.262994994770442,
0.280433083165914),.UNSPECIFIED.)
GEOMETRIC_REPRESENTATION_ITEM()
RATIONAL_B_SPLINE_SURFACE(((0.989123653000982,0.991350813683904,0.996566619267864),
(0.989123653000982,0.991350813683904,0.996566619267864)))
REPRESENTATION_ITEM('')
SURFACE()
);
#1749=(
BOUNDED_SURFACE()
B_SPLINE_SURFACE(1,2,((#123669,#123670,#123671,#123672,#123673),(#123674,
#123675,#123676,#123677,#123678)),.UNSPECIFIED.,.F.,.F.,.F.)
B_SPLINE_SURFACE_WITH_KNOTS((2,2),(3,2,3),(0.709601334848041,1.),(0.452333244852061,
0.452924869174517,0.470122329512317),.UNSPECIFIED.)
GEOMETRIC_REPRESENTATION_ITEM()
RATIONAL_B_SPLINE_SURFACE(((0.988732477628006,0.988732477628006,0.988732477628006,
0.986812255267055,0.987798766302166),(0.988732477628006,0.988732477628006,
0.988732477628006,0.986812255267055,0.987798766302166)))
REPRESENTATION_ITEM('')
SURFACE()
);
#1750=(
BOUNDED_SURFACE()
B_SPLINE_SURFACE(1,2,((#123687,#123688,#123689),(#123690,#123691,#123692)),
 .UNSPECIFIED.,.F.,.F.,.F.)
B_SPLINE_SURFACE_WITH_KNOTS((2,2),(3,3),(0.710318915640003,1.),(0.262994994770442,
0.280433083165929),.UNSPECIFIED.)
GEOMETRIC_REPRESENTATION_ITEM()
RATIONAL_B_SPLINE_SURFACE(((0.989123653000982,0.991350813683906,0.996566619267873),
(0.989123653000982,0.991350813683906,0.996566619267873)))
REPRESENTATION_ITEM('')
SURFACE()
);
#1751=(
BOUNDED_SURFACE()
B_SPLINE_SURFACE(1,2,((#123694,#123695,#123696,#123697,#123698),(#123699,
#123700,#123701,#123702,#123703)),.UNSPECIFIED.,.F.,.F.,.F.)
B_SPLINE_SURFACE_WITH_KNOTS((2,2),(3,2,3),(0.709601334840422,1.),(0.452333244845542,
0.45292486917451,0.470122329512317),.UNSPECIFIED.)
GEOMETRIC_REPRESENTATION_ITEM()
RATIONAL_B_SPLINE_SURFACE(((0.988732477628007,0.988732477628007,0.988732477628007,
0.986812255267055,0.987798766302166),(0.988732477628007,0.988732477628007,
0.988732477628007,0.986812255267055,0.987798766302166)))
REPRESENTATION_ITEM('')
SURFACE()
);
#1752=(
BOUNDED_SURFACE()
B_SPLINE_SURFACE(1,2,((#123712,#123713,#123714),(#123715,#123716,#123717)),
 .UNSPECIFIED.,.F.,.F.,.F.)
B_SPLINE_SURFACE_WITH_KNOTS((2,2),(3,3),(0.710318915639402,1.),(0.262994994770442,
0.280433083165975),.UNSPECIFIED.)
GEOMETRIC_REPRESENTATION_ITEM()
RATIONAL_B_SPLINE_SURFACE(((0.989123653000982,0.991350813683911,0.9965666192679),
(0.989123653000982,0.991350813683911,0.9965666192679)))
REPRESENTATION_ITEM('')
SURFACE()
);
#1753=(
BOUNDED_SURFACE()
B_SPLINE_SURFACE(1,2,((#123719,#123720,#123721,#123722,#123723),(#123724,
#123725,#123726,#123727,#123728)),.UNSPECIFIED.,.F.,.F.,.F.)
B_SPLINE_SURFACE_WITH_KNOTS((2,2),(3,2,3),(0.709601334835961,1.),(0.452333244840766,
0.452924869174507,0.470122329512317),.UNSPECIFIED.)
GEOMETRIC_REPRESENTATION_ITEM()
RATIONAL_B_SPLINE_SURFACE(((0.988732477628008,0.988732477628008,0.988732477628008,
0.986812255267055,0.987798766302166),(0.988732477628008,0.988732477628008,
0.988732477628008,0.986812255267055,0.987798766302166)))
REPRESENTATION_ITEM('')
SURFACE()
);
#1754=(
BOUNDED_SURFACE()
B_SPLINE_SURFACE(1,2,((#123737,#123738,#123739),(#123740,#123741,#123742)),
 .UNSPECIFIED.,.F.,.F.,.F.)
B_SPLINE_SURFACE_WITH_KNOTS((2,2),(3,3),(0.710318915640031,1.),(0.262994994770442,
0.280433083165914),.UNSPECIFIED.)
GEOMETRIC_REPRESENTATION_ITEM()
RATIONAL_B_SPLINE_SURFACE(((0.989123653000982,0.991350813683904,0.996566619267864),
(0.989123653000982,0.991350813683904,0.996566619267864)))
REPRESENTATION_ITEM('')
SURFACE()
);
#1755=(
BOUNDED_SURFACE()
B_SPLINE_SURFACE(1,2,((#123744,#123745,#123746,#123747,#123748),(#123749,
#123750,#123751,#123752,#123753)),.UNSPECIFIED.,.F.,.F.,.F.)
B_SPLINE_SURFACE_WITH_KNOTS((2,2),(3,2,3),(0.7096013348319,1.),(0.452333244836634,
0.452924869174508,0.470122329512317),.UNSPECIFIED.)
GEOMETRIC_REPRESENTATION_ITEM()
RATIONAL_B_SPLINE_SURFACE(((0.988732477628008,0.988732477628008,0.988732477628008,
0.986812255267055,0.987798766302166),(0.988732477628008,0.988732477628008,
0.988732477628008,0.986812255267055,0.987798766302166)))
REPRESENTATION_ITEM('')
SURFACE()
);
#1756=(
BOUNDED_SURFACE()
B_SPLINE_SURFACE(1,2,((#123762,#123763,#123764),(#123765,#123766,#123767)),
 .UNSPECIFIED.,.F.,.F.,.F.)
B_SPLINE_SURFACE_WITH_KNOTS((2,2),(3,3),(0.710318915640007,1.),(0.262994994770442,
0.280433083165924),.UNSPECIFIED.)
GEOMETRIC_REPRESENTATION_ITEM()
RATIONAL_B_SPLINE_SURFACE(((0.989123653000982,0.991350813683905,0.99656661926787),
(0.989123653000982,0.991350813683905,0.99656661926787)))
REPRESENTATION_ITEM('')
SURFACE()
);
#1757=(
BOUNDED_SURFACE()
B_SPLINE_SURFACE(1,2,((#123769,#123770,#123771,#123772,#123773),(#123774,
#123775,#123776,#123777,#123778)),.UNSPECIFIED.,.F.,.F.,.F.)
B_SPLINE_SURFACE_WITH_KNOTS((2,2),(3,2,3),(0.709601334846721,1.),(0.45233324485136,
0.452924869174509,0.470122329512317),.UNSPECIFIED.)
GEOMETRIC_REPRESENTATION_ITEM()
RATIONAL_B_SPLINE_SURFACE(((0.988732477628007,0.988732477628007,0.988732477628007,
0.986812255267055,0.987798766302166),(0.988732477628007,0.988732477628007,
0.988732477628007,0.986812255267055,0.987798766302166)))
REPRESENTATION_ITEM('')
SURFACE()
);
#1758=(
BOUNDED_SURFACE()
B_SPLINE_SURFACE(1,2,((#123787,#123788,#123789),(#123790,#123791,#123792)),
 .UNSPECIFIED.,.F.,.F.,.F.)
B_SPLINE_SURFACE_WITH_KNOTS((2,2),(3,3),(0.710318915640024,1.),(0.262994994770442,
0.280433083165913),.UNSPECIFIED.)
GEOMETRIC_REPRESENTATION_ITEM()
RATIONAL_B_SPLINE_SURFACE(((0.989123653000982,0.991350813683904,0.996566619267864),
(0.989123653000982,0.991350813683904,0.996566619267863)))
REPRESENTATION_ITEM('')
SURFACE()
);
#1759=(
BOUNDED_SURFACE()
B_SPLINE_SURFACE(1,2,((#123794,#123795,#123796,#123797,#123798),(#123799,
#123800,#123801,#123802,#123803)),.UNSPECIFIED.,.F.,.F.,.F.)
B_SPLINE_SURFACE_WITH_KNOTS((2,2),(3,2,3),(0.709601334834013,1.),(0.452333244838054,
0.452924869174518,0.470122329512318),.UNSPECIFIED.)
GEOMETRIC_REPRESENTATION_ITEM()
RATIONAL_B_SPLINE_SURFACE(((0.988732477628005,0.988732477628005,0.988732477628005,
0.986812255267055,0.987798766302166),(0.988732477628005,0.988732477628005,
0.988732477628005,0.986812255267055,0.987798766302166)))
REPRESENTATION_ITEM('')
SURFACE()
);
#1760=(
BOUNDED_SURFACE()
B_SPLINE_SURFACE(1,2,((#123805,#123806,#123807,#123808,#123809),(#123810,
#123811,#123812,#123813,#123814)),.UNSPECIFIED.,.F.,.F.,.F.)
B_SPLINE_SURFACE_WITH_KNOTS((2,2),(3,2,3),(0.,0.289807040992964),(0.504546746573287,
0.504719756176205,0.52202071646804),.UNSPECIFIED.)
GEOMETRIC_REPRESENTATION_ITEM()
RATIONAL_B_SPLINE_SURFACE(((0.996905579294159,0.996905579294159,0.996905579294159,
0.991635321911186,0.989306890555884),(0.996905579294159,0.996905579294159,
0.996905579294159,0.991635321911186,0.989306890555885)))
REPRESENTATION_ITEM('')
SURFACE()
);
#1761=(
BOUNDED_SURFACE()
B_SPLINE_SURFACE(1,2,((#123827,#123828,#123829,#123830,#123831,#123832,
#123833),(#123834,#123835,#123836,#123837,#123838,#123839,#123840)),
 .UNSPECIFIED.,.F.,.F.,.F.)
B_SPLINE_SURFACE_WITH_KNOTS((2,2),(3,2,2,3),(0.,0.289681084359915),(0.211398300093701,
0.214285714285714,0.22888337489481,0.229058225642821),.UNSPECIFIED.)
GEOMETRIC_REPRESENTATION_ITEM()
RATIONAL_B_SPLINE_SURFACE(((0.998054921708739,0.998986490969345,1.,0.994876086397763,
0.991846493044689,0.991846493044689,0.991846493044689),(0.998054921708739,
0.998986490969345,1.,0.994876086397763,0.991846493044689,0.991846493044689,
0.991846493044689)))
REPRESENTATION_ITEM('')
SURFACE()
);
#1762=(
BOUNDED_SURFACE()
B_SPLINE_SURFACE(1,2,((#123862,#123863,#123864,#123865,#123866),(#123867,
#123868,#123869,#123870,#123871)),.UNSPECIFIED.,.F.,.F.,.F.)
B_SPLINE_SURFACE_WITH_KNOTS((2,2),(3,2,3),(0.,0.2898070409939),(0.504546746573287,
0.504719756176205,0.52202071646804),.UNSPECIFIED.)
GEOMETRIC_REPRESENTATION_ITEM()
RATIONAL_B_SPLINE_SURFACE(((0.996905579294159,0.996905579294159,0.996905579294159,
0.991635321911186,0.989306890555885),(0.996905579294159,0.996905579294159,
0.996905579294159,0.991635321911186,0.989306890555885)))
REPRESENTATION_ITEM('')
SURFACE()
);
#1763=(
BOUNDED_SURFACE()
B_SPLINE_SURFACE(1,2,((#123873,#123874,#123875,#123876,#123877,#123878,
#123879),(#123880,#123881,#123882,#123883,#123884,#123885,#123886)),
 .UNSPECIFIED.,.F.,.F.,.F.)
B_SPLINE_SURFACE_WITH_KNOTS((2,2),(3,2,2,3),(0.,0.289681084359916),(0.211398300093701,
0.214285714285714,0.22888337489481,0.229058225642821),.UNSPECIFIED.)
GEOMETRIC_REPRESENTATION_ITEM()
RATIONAL_B_SPLINE_SURFACE(((0.998054921708739,0.998986490969345,1.,0.994876086397763,
0.991846493044689,0.991846493044689,0.991846493044689),(0.998054921708739,
0.998986490969345,1.,0.994876086397763,0.991846493044689,0.991846493044689,
0.991846493044689)))
REPRESENTATION_ITEM('')
SURFACE()
);
#1764=(
BOUNDED_SURFACE()
B_SPLINE_SURFACE(1,2,((#123903,#123904,#123905,#123906,#123907),(#123908,
#123909,#123910,#123911,#123912)),.UNSPECIFIED.,.F.,.F.,.F.)
B_SPLINE_SURFACE_WITH_KNOTS((2,2),(3,2,3),(0.,0.289807040993896),(0.504546746573287,
0.504719756176205,0.52202071646804),.UNSPECIFIED.)
GEOMETRIC_REPRESENTATION_ITEM()
RATIONAL_B_SPLINE_SURFACE(((0.996905579294159,0.996905579294159,0.996905579294159,
0.991635321911186,0.989306890555885),(0.996905579294159,0.996905579294159,
0.996905579294159,0.991635321911186,0.989306890555885)))
REPRESENTATION_ITEM('')
SURFACE()
);
#1765=(
BOUNDED_SURFACE()
B_SPLINE_SURFACE(1,2,((#123914,#123915,#123916,#123917,#123918,#123919,
#123920),(#123921,#123922,#123923,#123924,#123925,#123926,#123927)),
 .UNSPECIFIED.,.F.,.F.,.F.)
B_SPLINE_SURFACE_WITH_KNOTS((2,2),(3,2,2,3),(0.,0.289681084359925),(0.211398300093701,
0.214285714285714,0.22888337489481,0.229058225642821),.UNSPECIFIED.)
GEOMETRIC_REPRESENTATION_ITEM()
RATIONAL_B_SPLINE_SURFACE(((0.998054921708739,0.998986490969345,1.,0.994876086397763,
0.991846493044689,0.991846493044689,0.991846493044689),(0.998054921708739,
0.998986490969345,1.,0.994876086397763,0.991846493044689,0.991846493044689,
0.991846493044689)))
REPRESENTATION_ITEM('')
SURFACE()
);
#1766=(
BOUNDED_SURFACE()
B_SPLINE_SURFACE(1,2,((#123944,#123945,#123946,#123947,#123948),(#123949,
#123950,#123951,#123952,#123953)),.UNSPECIFIED.,.F.,.F.,.F.)
B_SPLINE_SURFACE_WITH_KNOTS((2,2),(3,2,3),(0.,0.289807040993898),(0.504546746573287,
0.504719756176205,0.52202071646804),.UNSPECIFIED.)
GEOMETRIC_REPRESENTATION_ITEM()
RATIONAL_B_SPLINE_SURFACE(((0.996905579294159,0.996905579294159,0.996905579294159,
0.991635321911186,0.989306890555885),(0.996905579294159,0.996905579294159,
0.996905579294159,0.991635321911186,0.989306890555885)))
REPRESENTATION_ITEM('')
SURFACE()
);
#1767=(
BOUNDED_SURFACE()
B_SPLINE_SURFACE(1,2,((#123955,#123956,#123957,#123958,#123959,#123960,
#123961),(#123962,#123963,#123964,#123965,#123966,#123967,#123968)),
 .UNSPECIFIED.,.F.,.F.,.F.)
B_SPLINE_SURFACE_WITH_KNOTS((2,2),(3,2,2,3),(0.,0.28968108435992),(0.211398300093701,
0.214285714285714,0.22888337489481,0.229058225642821),.UNSPECIFIED.)
GEOMETRIC_REPRESENTATION_ITEM()
RATIONAL_B_SPLINE_SURFACE(((0.998054921708739,0.998986490969345,1.,0.994876086397763,
0.991846493044689,0.991846493044689,0.991846493044689),(0.998054921708739,
0.998986490969345,1.,0.994876086397763,0.991846493044689,0.991846493044689,
0.991846493044689)))
REPRESENTATION_ITEM('')
SURFACE()
);
#1768=(
BOUNDED_SURFACE()
B_SPLINE_SURFACE(1,2,((#123990,#123991,#123992,#123993,#123994),(#123995,
#123996,#123997,#123998,#123999)),.UNSPECIFIED.,.F.,.F.,.F.)
B_SPLINE_SURFACE_WITH_KNOTS((2,2),(3,2,3),(0.,0.289807040994484),(0.504546746573287,
0.504719756176205,0.52202071646804),.UNSPECIFIED.)
GEOMETRIC_REPRESENTATION_ITEM()
RATIONAL_B_SPLINE_SURFACE(((0.996905579294159,0.996905579294159,0.996905579294159,
0.991635321911186,0.989306890555885),(0.996905579294159,0.996905579294159,
0.996905579294159,0.991635321911186,0.989306890555885)))
REPRESENTATION_ITEM('')
SURFACE()
);
#1769=(
BOUNDED_SURFACE()
B_SPLINE_SURFACE(1,2,((#124001,#124002,#124003,#124004,#124005,#124006,
#124007),(#124008,#124009,#124010,#124011,#124012,#124013,#124014)),
 .UNSPECIFIED.,.F.,.F.,.F.)
B_SPLINE_SURFACE_WITH_KNOTS((2,2),(3,2,2,3),(0.,0.289681084359918),(0.211398300093701,
0.214285714285714,0.22888337489481,0.229058225642821),.UNSPECIFIED.)
GEOMETRIC_REPRESENTATION_ITEM()
RATIONAL_B_SPLINE_SURFACE(((0.998054921708739,0.998986490969345,1.,0.994876086397763,
0.991846493044689,0.991846493044689,0.991846493044689),(0.998054921708739,
0.998986490969345,1.,0.994876086397763,0.991846493044689,0.991846493044689,
0.991846493044689)))
REPRESENTATION_ITEM('')
SURFACE()
);
#1770=(
BOUNDED_SURFACE()
B_SPLINE_SURFACE(1,2,((#124036,#124037,#124038,#124039,#124040),(#124041,
#124042,#124043,#124044,#124045)),.UNSPECIFIED.,.F.,.F.,.F.)
B_SPLINE_SURFACE_WITH_KNOTS((2,2),(3,2,3),(0.,0.289807040993898),(0.504546746573287,
0.504719756176205,0.52202071646804),.UNSPECIFIED.)
GEOMETRIC_REPRESENTATION_ITEM()
RATIONAL_B_SPLINE_SURFACE(((0.996905579294159,0.996905579294159,0.996905579294159,
0.991635321911186,0.989306890555885),(0.996905579294159,0.996905579294159,
0.996905579294159,0.991635321911186,0.989306890555885)))
REPRESENTATION_ITEM('')
SURFACE()
);
#1771=(
BOUNDED_SURFACE()
B_SPLINE_SURFACE(1,2,((#124047,#124048,#124049,#124050,#124051,#124052,
#124053),(#124054,#124055,#124056,#124057,#124058,#124059,#124060)),
 .UNSPECIFIED.,.F.,.F.,.F.)
B_SPLINE_SURFACE_WITH_KNOTS((2,2),(3,2,2,3),(0.,0.289681084359926),(0.211398300093701,
0.214285714285714,0.22888337489481,0.229058225642821),.UNSPECIFIED.)
GEOMETRIC_REPRESENTATION_ITEM()
RATIONAL_B_SPLINE_SURFACE(((0.998054921708739,0.998986490969345,1.,0.994876086397763,
0.991846493044689,0.991846493044689,0.991846493044689),(0.998054921708739,
0.998986490969345,1.,0.994876086397763,0.991846493044689,0.991846493044689,
0.991846493044689)))
REPRESENTATION_ITEM('')
SURFACE()
);
#1772=(
BOUNDED_SURFACE()
B_SPLINE_SURFACE(1,2,((#124077,#124078,#124079,#124080,#124081),(#124082,
#124083,#124084,#124085,#124086)),.UNSPECIFIED.,.F.,.F.,.F.)
B_SPLINE_SURFACE_WITH_KNOTS((2,2),(3,2,3),(0.,0.289807040994487),(0.504546746573287,
0.504719756176205,0.52202071646804),.UNSPECIFIED.)
GEOMETRIC_REPRESENTATION_ITEM()
RATIONAL_B_SPLINE_SURFACE(((0.996905579294159,0.996905579294159,0.996905579294159,
0.991635321911186,0.989306890555885),(0.996905579294159,0.996905579294159,
0.996905579294159,0.991635321911186,0.989306890555885)))
REPRESENTATION_ITEM('')
SURFACE()
);
#1773=(
BOUNDED_SURFACE()
B_SPLINE_SURFACE(1,2,((#124088,#124089,#124090,#124091,#124092,#124093,
#124094),(#124095,#124096,#124097,#124098,#124099,#124100,#124101)),
 .UNSPECIFIED.,.F.,.F.,.F.)
B_SPLINE_SURFACE_WITH_KNOTS((2,2),(3,2,2,3),(0.,0.289681084359916),(0.211398300093701,
0.214285714285714,0.22888337489481,0.229058225642821),.UNSPECIFIED.)
GEOMETRIC_REPRESENTATION_ITEM()
RATIONAL_B_SPLINE_SURFACE(((0.998054921708739,0.998986490969345,1.,0.994876086397763,
0.991846493044689,0.991846493044689,0.991846493044689),(0.998054921708739,
0.998986490969345,1.,0.994876086397763,0.991846493044689,0.991846493044689,
0.991846493044689)))
REPRESENTATION_ITEM('')
SURFACE()
);
#1774=(
BOUNDED_SURFACE()
B_SPLINE_SURFACE(1,2,((#124118,#124119,#124120,#124121,#124122),(#124123,
#124124,#124125,#124126,#124127)),.UNSPECIFIED.,.F.,.F.,.F.)
B_SPLINE_SURFACE_WITH_KNOTS((2,2),(3,2,3),(0.,0.289807040993979),(0.504546746573288,
0.504719756176206,0.52202071646804),.UNSPECIFIED.)
GEOMETRIC_REPRESENTATION_ITEM()
RATIONAL_B_SPLINE_SURFACE(((0.996905579294159,0.996905579294159,0.996905579294159,
0.991635321911186,0.989306890555885),(0.996905579294159,0.996905579294159,
0.996905579294159,0.991635321911186,0.989306890555885)))
REPRESENTATION_ITEM('')
SURFACE()
);
#1775=(
BOUNDED_SURFACE()
B_SPLINE_SURFACE(1,2,((#124129,#124130,#124131,#124132,#124133,#124134,
#124135),(#124136,#124137,#124138,#124139,#124140,#124141,#124142)),
 .UNSPECIFIED.,.F.,.F.,.F.)
B_SPLINE_SURFACE_WITH_KNOTS((2,2),(3,2,2,3),(0.,0.289681084359922),(0.2113983000937,
0.214285714285714,0.228883374894809,0.22905822564282),.UNSPECIFIED.)
GEOMETRIC_REPRESENTATION_ITEM()
RATIONAL_B_SPLINE_SURFACE(((0.998054921708738,0.998986490969345,1.,0.994876086397764,
0.991846493044689,0.991846493044689,0.991846493044689),(0.998054921708738,
0.998986490969345,1.,0.994876086397764,0.991846493044689,0.991846493044689,
0.991846493044689)))
REPRESENTATION_ITEM('')
SURFACE()
);
#1776=(
BOUNDED_SURFACE()
B_SPLINE_SURFACE(1,2,((#124159,#124160,#124161,#124162,#124163),(#124164,
#124165,#124166,#124167,#124168)),.UNSPECIFIED.,.F.,.F.,.F.)
B_SPLINE_SURFACE_WITH_KNOTS((2,2),(3,2,3),(0.,0.289807040993979),(0.504546746573288,
0.504719756176206,0.522020716468041),.UNSPECIFIED.)
GEOMETRIC_REPRESENTATION_ITEM()
RATIONAL_B_SPLINE_SURFACE(((0.996905579294159,0.996905579294159,0.996905579294159,
0.991635321911186,0.989306890555884),(0.996905579294159,0.996905579294159,
0.996905579294159,0.991635321911186,0.989306890555884)))
REPRESENTATION_ITEM('')
SURFACE()
);
#1777=(
BOUNDED_SURFACE()
B_SPLINE_SURFACE(1,2,((#124170,#124171,#124172,#124173,#124174,#124175,
#124176),(#124177,#124178,#124179,#124180,#124181,#124182,#124183)),
 .UNSPECIFIED.,.F.,.F.,.F.)
B_SPLINE_SURFACE_WITH_KNOTS((2,2),(3,2,2,3),(0.,0.289681084359917),(0.2113983000937,
0.214285714285714,0.228883374894809,0.22905822564282),.UNSPECIFIED.)
GEOMETRIC_REPRESENTATION_ITEM()
RATIONAL_B_SPLINE_SURFACE(((0.998054921708738,0.998986490969345,1.,0.994876086397764,
0.991846493044689,0.991846493044689,0.991846493044689),(0.998054921708738,
0.998986490969345,1.,0.994876086397764,0.991846493044689,0.991846493044689,
0.991846493044689)))
REPRESENTATION_ITEM('')
SURFACE()
);
#1778=(
BOUNDED_SURFACE()
B_SPLINE_SURFACE(1,2,((#124200,#124201,#124202,#124203,#124204),(#124205,
#124206,#124207,#124208,#124209)),.UNSPECIFIED.,.F.,.F.,.F.)
B_SPLINE_SURFACE_WITH_KNOTS((2,2),(3,2,3),(0.,0.289807040994574),(0.504546746573288,
0.504719756176206,0.522020716468041),.UNSPECIFIED.)
GEOMETRIC_REPRESENTATION_ITEM()
RATIONAL_B_SPLINE_SURFACE(((0.996905579294158,0.996905579294158,0.996905579294158,
0.991635321911186,0.989306890555884),(0.996905579294158,0.996905579294158,
0.996905579294158,0.991635321911185,0.989306890555884)))
REPRESENTATION_ITEM('')
SURFACE()
);
#1779=(
BOUNDED_SURFACE()
B_SPLINE_SURFACE(1,2,((#124211,#124212,#124213,#124214,#124215,#124216,
#124217),(#124218,#124219,#124220,#124221,#124222,#124223,#124224)),
 .UNSPECIFIED.,.F.,.F.,.F.)
B_SPLINE_SURFACE_WITH_KNOTS((2,2),(3,2,2,3),(0.,0.289681084359919),(0.2113983000937,
0.214285714285714,0.228883374894809,0.22905822564282),.UNSPECIFIED.)
GEOMETRIC_REPRESENTATION_ITEM()
RATIONAL_B_SPLINE_SURFACE(((0.998054921708738,0.998986490969345,1.,0.994876086397764,
0.991846493044689,0.991846493044689,0.991846493044689),(0.998054921708738,
0.998986490969345,1.,0.994876086397764,0.991846493044689,0.991846493044689,
0.991846493044689)))
REPRESENTATION_ITEM('')
SURFACE()
);
#1780=(
BOUNDED_SURFACE()
B_SPLINE_SURFACE(1,2,((#124246,#124247,#124248,#124249,#124250),(#124251,
#124252,#124253,#124254,#124255)),.UNSPECIFIED.,.F.,.F.,.F.)
B_SPLINE_SURFACE_WITH_KNOTS((2,2),(3,2,3),(0.,0.289807040993985),(0.504546746573288,
0.504719756176206,0.522020716468041),.UNSPECIFIED.)
GEOMETRIC_REPRESENTATION_ITEM()
RATIONAL_B_SPLINE_SURFACE(((0.996905579294158,0.996905579294158,0.996905579294158,
0.991635321911186,0.989306890555884),(0.996905579294158,0.996905579294158,
0.996905579294158,0.991635321911186,0.989306890555884)))
REPRESENTATION_ITEM('')
SURFACE()
);
#1781=(
BOUNDED_SURFACE()
B_SPLINE_SURFACE(1,2,((#124257,#124258,#124259,#124260,#124261,#124262,
#124263),(#124264,#124265,#124266,#124267,#124268,#124269,#124270)),
 .UNSPECIFIED.,.F.,.F.,.F.)
B_SPLINE_SURFACE_WITH_KNOTS((2,2),(3,2,2,3),(0.,0.289681084359918),(0.2113983000937,
0.214285714285714,0.228883374894809,0.22905822564282),.UNSPECIFIED.)
GEOMETRIC_REPRESENTATION_ITEM()
RATIONAL_B_SPLINE_SURFACE(((0.998054921708738,0.998986490969345,1.,0.994876086397764,
0.991846493044689,0.991846493044689,0.991846493044689),(0.998054921708738,
0.998986490969345,1.,0.994876086397764,0.991846493044689,0.991846493044689,
0.991846493044689)))
REPRESENTATION_ITEM('')
SURFACE()
);
#1782=(
BOUNDED_SURFACE()
B_SPLINE_SURFACE(1,2,((#124287,#124288,#124289,#124290,#124291),(#124292,
#124293,#124294,#124295,#124296)),.UNSPECIFIED.,.F.,.F.,.F.)
B_SPLINE_SURFACE_WITH_KNOTS((2,2),(3,2,3),(0.,0.289807040994485),(0.504546746573288,
0.504719756176206,0.522020716468041),.UNSPECIFIED.)
GEOMETRIC_REPRESENTATION_ITEM()
RATIONAL_B_SPLINE_SURFACE(((0.996905579294158,0.996905579294158,0.996905579294158,
0.991635321911186,0.989306890555884),(0.996905579294158,0.996905579294158,
0.996905579294158,0.991635321911185,0.989306890555884)))
REPRESENTATION_ITEM('')
SURFACE()
);
#1783=(
BOUNDED_SURFACE()
B_SPLINE_SURFACE(1,2,((#124298,#124299,#124300,#124301,#124302,#124303,
#124304),(#124305,#124306,#124307,#124308,#124309,#124310,#124311)),
 .UNSPECIFIED.,.F.,.F.,.F.)
B_SPLINE_SURFACE_WITH_KNOTS((2,2),(3,2,2,3),(0.,0.289681084359917),(0.2113983000937,
0.214285714285714,0.228883374894809,0.22905822564282),.UNSPECIFIED.)
GEOMETRIC_REPRESENTATION_ITEM()
RATIONAL_B_SPLINE_SURFACE(((0.998054921708738,0.998986490969345,1.,0.994876086397764,
0.991846493044689,0.991846493044689,0.991846493044689),(0.998054921708738,
0.998986490969345,1.,0.994876086397764,0.991846493044689,0.991846493044689,
0.991846493044689)))
REPRESENTATION_ITEM('')
SURFACE()
);
#1784=(
BOUNDED_SURFACE()
B_SPLINE_SURFACE(1,2,((#124328,#124329,#124330,#124331,#124332),(#124333,
#124334,#124335,#124336,#124337)),.UNSPECIFIED.,.F.,.F.,.F.)
B_SPLINE_SURFACE_WITH_KNOTS((2,2),(3,2,3),(0.,0.289807040993984),(0.504546746573288,
0.504719756176206,0.522020716468041),.UNSPECIFIED.)
GEOMETRIC_REPRESENTATION_ITEM()
RATIONAL_B_SPLINE_SURFACE(((0.996905579294158,0.996905579294158,0.996905579294158,
0.991635321911185,0.989306890555884),(0.996905579294158,0.996905579294158,
0.996905579294158,0.991635321911186,0.989306890555884)))
REPRESENTATION_ITEM('')
SURFACE()
);
#1785=(
BOUNDED_SURFACE()
B_SPLINE_SURFACE(1,2,((#124339,#124340,#124341,#124342,#124343,#124344,
#124345),(#124346,#124347,#124348,#124349,#124350,#124351,#124352)),
 .UNSPECIFIED.,.F.,.F.,.F.)
B_SPLINE_SURFACE_WITH_KNOTS((2,2),(3,2,2,3),(0.,0.28968108435992),(0.2113983000937,
0.214285714285714,0.228883374894809,0.22905822564282),.UNSPECIFIED.)
GEOMETRIC_REPRESENTATION_ITEM()
RATIONAL_B_SPLINE_SURFACE(((0.998054921708738,0.998986490969345,1.,0.994876086397764,
0.991846493044689,0.991846493044689,0.991846493044689),(0.998054921708738,
0.998986490969345,1.,0.994876086397764,0.991846493044689,0.991846493044689,
0.991846493044689)))
REPRESENTATION_ITEM('')
SURFACE()
);
#1786=(
BOUNDED_SURFACE()
B_SPLINE_SURFACE(1,2,((#124369,#124370,#124371,#124372,#124373),(#124374,
#124375,#124376,#124377,#124378)),.UNSPECIFIED.,.F.,.F.,.F.)
B_SPLINE_SURFACE_WITH_KNOTS((2,2),(3,2,3),(0.,0.28980704099449),(0.504546746573288,
0.504719756176206,0.522020716468041),.UNSPECIFIED.)
GEOMETRIC_REPRESENTATION_ITEM()
RATIONAL_B_SPLINE_SURFACE(((0.996905579294158,0.996905579294158,0.996905579294158,
0.991635321911186,0.989306890555884),(0.996905579294158,0.996905579294158,
0.996905579294158,0.991635321911185,0.989306890555884)))
REPRESENTATION_ITEM('')
SURFACE()
);
#1787=(
BOUNDED_SURFACE()
B_SPLINE_SURFACE(1,2,((#124380,#124381,#124382,#124383,#124384,#124385,
#124386),(#124387,#124388,#124389,#124390,#124391,#124392,#124393)),
 .UNSPECIFIED.,.F.,.F.,.F.)
B_SPLINE_SURFACE_WITH_KNOTS((2,2),(3,2,2,3),(0.,0.289681084359921),(0.2113983000937,
0.214285714285714,0.228883374894809,0.22905822564282),.UNSPECIFIED.)
GEOMETRIC_REPRESENTATION_ITEM()
RATIONAL_B_SPLINE_SURFACE(((0.998054921708738,0.998986490969345,1.,0.994876086397764,
0.991846493044689,0.991846493044689,0.991846493044689),(0.998054921708738,
0.998986490969345,1.,0.994876086397764,0.991846493044689,0.991846493044689,
0.991846493044689)))
REPRESENTATION_ITEM('')
SURFACE()
);
#1788=(
BOUNDED_SURFACE()
B_SPLINE_SURFACE(1,2,((#124419,#124420,#124421,#124422,#124423),(#124424,
#124425,#124426,#124427,#124428)),.UNSPECIFIED.,.F.,.F.,.F.)
B_SPLINE_SURFACE_WITH_KNOTS((2,2),(3,2,3),(0.,0.289807040994261),(0.504546746573288,
0.504719756176206,0.522020716468041),.UNSPECIFIED.)
GEOMETRIC_REPRESENTATION_ITEM()
RATIONAL_B_SPLINE_SURFACE(((0.996905579294158,0.996905579294158,0.996905579294158,
0.991635321911186,0.989306890555884),(0.996905579294159,0.996905579294159,
0.996905579294159,0.991635321911186,0.989306890555884)))
REPRESENTATION_ITEM('')
SURFACE()
);
#1789=(
BOUNDED_SURFACE()
B_SPLINE_SURFACE(1,2,((#124430,#124431,#124432,#124433,#124434,#124435,
#124436),(#124437,#124438,#124439,#124440,#124441,#124442,#124443)),
 .UNSPECIFIED.,.F.,.F.,.F.)
B_SPLINE_SURFACE_WITH_KNOTS((2,2),(3,2,2,3),(0.,0.28968108435992),(0.2113983000937,
0.214285714285714,0.228883374894809,0.22905822564282),.UNSPECIFIED.)
GEOMETRIC_REPRESENTATION_ITEM()
RATIONAL_B_SPLINE_SURFACE(((0.998054921708738,0.998986490969345,1.,0.994876086397764,
0.991846493044689,0.991846493044689,0.991846493044689),(0.998054921708738,
0.998986490969345,1.,0.994876086397764,0.991846493044689,0.991846493044689,
0.991846493044689)))
REPRESENTATION_ITEM('')
SURFACE()
);
#1790=(
BOUNDED_SURFACE()
B_SPLINE_SURFACE(1,2,((#124469,#124470,#124471,#124472,#124473),(#124474,
#124475,#124476,#124477,#124478)),.UNSPECIFIED.,.F.,.F.,.F.)
B_SPLINE_SURFACE_WITH_KNOTS((2,2),(3,2,3),(0.,0.289807040995303),(0.504546746573288,
0.504719756176206,0.522020716468041),.UNSPECIFIED.)
GEOMETRIC_REPRESENTATION_ITEM()
RATIONAL_B_SPLINE_SURFACE(((0.996905579294158,0.996905579294158,0.996905579294158,
0.991635321911185,0.989306890555884),(0.996905579294158,0.996905579294158,
0.996905579294158,0.991635321911186,0.989306890555884)))
REPRESENTATION_ITEM('')
SURFACE()
);
#1791=(
BOUNDED_SURFACE()
B_SPLINE_SURFACE(1,2,((#124480,#124481,#124482,#124483,#124484,#124485,
#124486),(#124487,#124488,#124489,#124490,#124491,#124492,#124493)),
 .UNSPECIFIED.,.F.,.F.,.F.)
B_SPLINE_SURFACE_WITH_KNOTS((2,2),(3,2,2,3),(0.,0.289681084359921),(0.2113983000937,
0.214285714285714,0.228883374894811,0.229058225642822),.UNSPECIFIED.)
GEOMETRIC_REPRESENTATION_ITEM()
RATIONAL_B_SPLINE_SURFACE(((0.998054921708738,0.998986490969345,1.,0.994876086397763,
0.991846493044688,0.991846493044688,0.991846493044688),(0.998054921708738,
0.998986490969345,1.,0.994876086397763,0.991846493044688,0.991846493044688,
0.991846493044688)))
REPRESENTATION_ITEM('')
SURFACE()
);
#1792=(
BOUNDED_SURFACE()
B_SPLINE_SURFACE(1,2,((#124519,#124520,#124521,#124522,#124523),(#124524,
#124525,#124526,#124527,#124528)),.UNSPECIFIED.,.F.,.F.,.F.)
B_SPLINE_SURFACE_WITH_KNOTS((2,2),(3,2,3),(0.,0.28980704099402),(0.504546746573288,
0.504719756176206,0.522020716468041),.UNSPECIFIED.)
GEOMETRIC_REPRESENTATION_ITEM()
RATIONAL_B_SPLINE_SURFACE(((0.996905579294158,0.996905579294158,0.996905579294158,
0.991635321911185,0.989306890555884),(0.996905579294158,0.996905579294158,
0.996905579294158,0.991635321911185,0.989306890555884)))
REPRESENTATION_ITEM('')
SURFACE()
);
#1793=(
BOUNDED_SURFACE()
B_SPLINE_SURFACE(1,2,((#124530,#124531,#124532,#124533,#124534,#124535,
#124536),(#124537,#124538,#124539,#124540,#124541,#124542,#124543)),
 .UNSPECIFIED.,.F.,.F.,.F.)
B_SPLINE_SURFACE_WITH_KNOTS((2,2),(3,2,2,3),(0.,0.289681084359926),(0.211398300093698,
0.214285714285714,0.228883374894809,0.22905822564282),.UNSPECIFIED.)
GEOMETRIC_REPRESENTATION_ITEM()
RATIONAL_B_SPLINE_SURFACE(((0.998054921708736,0.998986490969344,1.,0.994876086397764,
0.991846493044689,0.991846493044689,0.991846493044689),(0.998054921708736,
0.998986490969344,1.,0.994876086397764,0.991846493044689,0.991846493044689,
0.991846493044689)))
REPRESENTATION_ITEM('')
SURFACE()
);
#1794=(
BOUNDED_SURFACE()
B_SPLINE_SURFACE(1,2,((#124560,#124561,#124562,#124563,#124564),(#124565,
#124566,#124567,#124568,#124569)),.UNSPECIFIED.,.F.,.F.,.F.)
B_SPLINE_SURFACE_WITH_KNOTS((2,2),(3,2,3),(0.,0.28980704099391),(0.504546746573288,
0.504719756176206,0.522020716468041),.UNSPECIFIED.)
GEOMETRIC_REPRESENTATION_ITEM()
RATIONAL_B_SPLINE_SURFACE(((0.996905579294158,0.996905579294158,0.996905579294158,
0.991635321911186,0.989306890555884),(0.996905579294158,0.996905579294158,
0.996905579294158,0.991635321911186,0.989306890555884)))
REPRESENTATION_ITEM('')
SURFACE()
);
#1795=(
BOUNDED_SURFACE()
B_SPLINE_SURFACE(1,2,((#124571,#124572,#124573,#124574,#124575,#124576,
#124577),(#124578,#124579,#124580,#124581,#124582,#124583,#124584)),
 .UNSPECIFIED.,.F.,.F.,.F.)
B_SPLINE_SURFACE_WITH_KNOTS((2,2),(3,2,2,3),(0.,0.289681084360126),(0.2113983000937,
0.214285714285714,0.228883374894809,0.22905822564282),.UNSPECIFIED.)
GEOMETRIC_REPRESENTATION_ITEM()
RATIONAL_B_SPLINE_SURFACE(((0.998054921708738,0.998986490969345,1.,0.994876086397764,
0.991846493044689,0.991846493044689,0.991846493044689),(0.998054921708738,
0.998986490969345,1.,0.994876086397764,0.991846493044689,0.991846493044689,
0.991846493044689)))
REPRESENTATION_ITEM('')
SURFACE()
);
#1796=(
BOUNDED_SURFACE()
B_SPLINE_SURFACE(1,2,((#124601,#124602,#124603,#124604,#124605),(#124606,
#124607,#124608,#124609,#124610)),.UNSPECIFIED.,.F.,.F.,.F.)
B_SPLINE_SURFACE_WITH_KNOTS((2,2),(3,2,3),(0.,0.289807040994542),(0.504546746573034,
0.504719756175955,0.522020716468043),.UNSPECIFIED.)
GEOMETRIC_REPRESENTATION_ITEM()
RATIONAL_B_SPLINE_SURFACE(((0.996905579294312,0.996905579294312,0.996905579294312,
0.991635321911219,0.989306890555884),(0.996905579294312,0.996905579294312,
0.996905579294312,0.991635321911219,0.989306890555884)))
REPRESENTATION_ITEM('')
SURFACE()
);
#1797=(
BOUNDED_SURFACE()
B_SPLINE_SURFACE(1,2,((#124612,#124613,#124614,#124615,#124616,#124617,
#124618),(#124619,#124620,#124621,#124622,#124623,#124624,#124625)),
 .UNSPECIFIED.,.F.,.F.,.F.)
B_SPLINE_SURFACE_WITH_KNOTS((2,2),(3,2,2,3),(0.,0.289681084359927),(0.2113983000937,
0.214285714285714,0.228883374894809,0.22905822564282),.UNSPECIFIED.)
GEOMETRIC_REPRESENTATION_ITEM()
RATIONAL_B_SPLINE_SURFACE(((0.998054921708738,0.998986490969345,1.,0.994876086397764,
0.991846493044689,0.991846493044689,0.991846493044689),(0.998054921708738,
0.998986490969345,1.,0.994876086397764,0.991846493044689,0.991846493044689,
0.991846493044689)))
REPRESENTATION_ITEM('')
SURFACE()
);
#1798=(
BOUNDED_SURFACE()
B_SPLINE_SURFACE(1,2,((#124647,#124648,#124649,#124650,#124651),(#124652,
#124653,#124654,#124655,#124656)),.UNSPECIFIED.,.F.,.F.,.F.)
B_SPLINE_SURFACE_WITH_KNOTS((2,2),(3,2,3),(0.,0.289807040993132),(0.504546746573153,
0.504719756176073,0.522020716468042),.UNSPECIFIED.)
GEOMETRIC_REPRESENTATION_ITEM()
RATIONAL_B_SPLINE_SURFACE(((0.99690557929424,0.99690557929424,0.99690557929424,
0.991635321911203,0.989306890555884),(0.99690557929424,0.99690557929424,
0.99690557929424,0.991635321911203,0.989306890555884)))
REPRESENTATION_ITEM('')
SURFACE()
);
#1799=(
BOUNDED_SURFACE()
B_SPLINE_SURFACE(1,2,((#124658,#124659,#124660,#124661,#124662,#124663,
#124664),(#124665,#124666,#124667,#124668,#124669,#124670,#124671)),
 .UNSPECIFIED.,.F.,.F.,.F.)
B_SPLINE_SURFACE_WITH_KNOTS((2,2),(3,2,2,3),(0.,0.289681084360278),(0.211398300093698,
0.214285714285714,0.228883374894809,0.22905822564282),.UNSPECIFIED.)
GEOMETRIC_REPRESENTATION_ITEM()
RATIONAL_B_SPLINE_SURFACE(((0.998054921708737,0.998986490969345,1.,0.994876086397764,
0.991846493044689,0.991846493044689,0.991846493044689),(0.998054921708737,
0.998986490969345,1.,0.994876086397764,0.991846493044689,0.991846493044689,
0.991846493044689)))
REPRESENTATION_ITEM('')
SURFACE()
);
#1800=(
BOUNDED_SURFACE()
B_SPLINE_SURFACE(1,2,((#124688,#124689,#124690,#124691,#124692),(#124693,
#124694,#124695,#124696,#124697)),.UNSPECIFIED.,.F.,.F.,.F.)
B_SPLINE_SURFACE_WITH_KNOTS((2,2),(3,2,3),(0.,0.289807040994288),(0.504546746573288,
0.504719756176206,0.522020716468042),.UNSPECIFIED.)
GEOMETRIC_REPRESENTATION_ITEM()
RATIONAL_B_SPLINE_SURFACE(((0.996905579294158,0.996905579294158,0.996905579294158,
0.991635321911185,0.989306890555884),(0.996905579294158,0.996905579294158,
0.996905579294158,0.991635321911185,0.989306890555884)))
REPRESENTATION_ITEM('')
SURFACE()
);
#1801=(
BOUNDED_SURFACE()
B_SPLINE_SURFACE(1,2,((#124699,#124700,#124701,#124702,#124703,#124704,
#124705),(#124706,#124707,#124708,#124709,#124710,#124711,#124712)),
 .UNSPECIFIED.,.F.,.F.,.F.)
B_SPLINE_SURFACE_WITH_KNOTS((2,2),(3,2,2,3),(0.,0.289681084361153),(0.211398300093696,
0.214285714285714,0.228883374894809,0.22905822564282),.UNSPECIFIED.)
GEOMETRIC_REPRESENTATION_ITEM()
RATIONAL_B_SPLINE_SURFACE(((0.998054921708735,0.998986490969344,1.,0.994876086397764,
0.991846493044689,0.991846493044689,0.991846493044689),(0.998054921708735,
0.998986490969344,1.,0.994876086397764,0.991846493044689,0.991846493044689,
0.991846493044689)))
REPRESENTATION_ITEM('')
SURFACE()
);
#1802=(
BOUNDED_SURFACE()
B_SPLINE_SURFACE(1,2,((#124729,#124730,#124731,#124732,#124733),(#124734,
#124735,#124736,#124737,#124738)),.UNSPECIFIED.,.F.,.F.,.F.)
B_SPLINE_SURFACE_WITH_KNOTS((2,2),(3,2,3),(0.,0.289807040994107),(0.504546746573004,
0.504719756175925,0.522020716468042),.UNSPECIFIED.)
GEOMETRIC_REPRESENTATION_ITEM()
RATIONAL_B_SPLINE_SURFACE(((0.99690557929433,0.99690557929433,0.99690557929433,
0.991635321911223,0.989306890555884),(0.99690557929433,0.99690557929433,
0.99690557929433,0.991635321911223,0.989306890555884)))
REPRESENTATION_ITEM('')
SURFACE()
);
#1803=(
BOUNDED_SURFACE()
B_SPLINE_SURFACE(1,2,((#124740,#124741,#124742,#124743,#124744,#124745,
#124746),(#124747,#124748,#124749,#124750,#124751,#124752,#124753)),
 .UNSPECIFIED.,.F.,.F.,.F.)
B_SPLINE_SURFACE_WITH_KNOTS((2,2),(3,2,2,3),(0.,0.289681084359926),(0.2113983000937,
0.214285714285714,0.22888337489481,0.229058225642821),.UNSPECIFIED.)
GEOMETRIC_REPRESENTATION_ITEM()
RATIONAL_B_SPLINE_SURFACE(((0.998054921708738,0.998986490969345,1.,0.994876086397764,
0.991846493044689,0.991846493044689,0.991846493044689),(0.998054921708738,
0.998986490969345,1.,0.994876086397763,0.991846493044689,0.991846493044689,
0.991846493044689)))
REPRESENTATION_ITEM('')
SURFACE()
);
#1804=(
BOUNDED_SURFACE()
B_SPLINE_SURFACE(1,2,((#124775,#124776,#124777,#124778,#124779),(#124780,
#124781,#124782,#124783,#124784)),.UNSPECIFIED.,.F.,.F.,.F.)
B_SPLINE_SURFACE_WITH_KNOTS((2,2),(3,2,3),(0.,0.289807040994811),(0.504546746573147,
0.504719756176067,0.522020716468042),.UNSPECIFIED.)
GEOMETRIC_REPRESENTATION_ITEM()
RATIONAL_B_SPLINE_SURFACE(((0.996905579294243,0.996905579294243,0.996905579294243,
0.991635321911204,0.989306890555884),(0.996905579294243,0.996905579294243,
0.996905579294243,0.991635321911204,0.989306890555884)))
REPRESENTATION_ITEM('')
SURFACE()
);
#1805=(
BOUNDED_SURFACE()
B_SPLINE_SURFACE(1,2,((#124786,#124787,#124788,#124789,#124790,#124791,
#124792),(#124793,#124794,#124795,#124796,#124797,#124798,#124799)),
 .UNSPECIFIED.,.F.,.F.,.F.)
B_SPLINE_SURFACE_WITH_KNOTS((2,2),(3,2,2,3),(0.,0.28968108435992),(0.2113983000937,
0.214285714285714,0.228883374894809,0.22905822564282),.UNSPECIFIED.)
GEOMETRIC_REPRESENTATION_ITEM()
RATIONAL_B_SPLINE_SURFACE(((0.998054921708738,0.998986490969345,1.,0.994876086397764,
0.991846493044689,0.991846493044689,0.991846493044689),(0.998054921708738,
0.998986490969345,1.,0.994876086397764,0.991846493044689,0.991846493044689,
0.991846493044689)))
REPRESENTATION_ITEM('')
SURFACE()
);
#1806=(
BOUNDED_SURFACE()
B_SPLINE_SURFACE(1,2,((#124825,#124826,#124827,#124828,#124829),(#124830,
#124831,#124832,#124833,#124834)),.UNSPECIFIED.,.F.,.F.,.F.)
B_SPLINE_SURFACE_WITH_KNOTS((2,2),(3,2,3),(0.,0.289807040993315),(0.5045467465732,
0.504719756176119,0.522020716468042),.UNSPECIFIED.)
GEOMETRIC_REPRESENTATION_ITEM()
RATIONAL_B_SPLINE_SURFACE(((0.996905579294211,0.996905579294211,0.996905579294211,
0.991635321911197,0.989306890555884),(0.996905579294211,0.996905579294211,
0.996905579294211,0.991635321911197,0.989306890555884)))
REPRESENTATION_ITEM('')
SURFACE()
);
#1807=(
BOUNDED_SURFACE()
B_SPLINE_SURFACE(1,2,((#124836,#124837,#124838,#124839,#124840,#124841,
#124842),(#124843,#124844,#124845,#124846,#124847,#124848,#124849)),
 .UNSPECIFIED.,.F.,.F.,.F.)
B_SPLINE_SURFACE_WITH_KNOTS((2,2),(3,2,2,3),(0.,0.289681084359922),(0.211398300093699,
0.214285714285714,0.22888337489485,0.229058225642861),.UNSPECIFIED.)
GEOMETRIC_REPRESENTATION_ITEM()
RATIONAL_B_SPLINE_SURFACE(((0.998054921708738,0.998986490969345,1.,0.994876086397749,
0.991846493044672,0.991846493044672,0.991846493044672),(0.998054921708738,
0.998986490969345,1.,0.994876086397749,0.991846493044672,0.991846493044672,
0.991846493044672)))
REPRESENTATION_ITEM('')
SURFACE()
);
#1808=(
BOUNDED_SURFACE()
B_SPLINE_SURFACE(1,2,((#124866,#124867,#124868,#124869,#124870),(#124871,
#124872,#124873,#124874,#124875)),.UNSPECIFIED.,.F.,.F.,.F.)
B_SPLINE_SURFACE_WITH_KNOTS((2,2),(3,2,3),(0.,0.289807040994463),(0.504546746573278,
0.504719756176196,0.522020716468041),.UNSPECIFIED.)
GEOMETRIC_REPRESENTATION_ITEM()
RATIONAL_B_SPLINE_SURFACE(((0.996905579294165,0.996905579294165,0.996905579294165,
0.991635321911187,0.989306890555884),(0.996905579294165,0.996905579294165,
0.996905579294165,0.991635321911187,0.989306890555884)))
REPRESENTATION_ITEM('')
SURFACE()
);
#1809=(
BOUNDED_SURFACE()
B_SPLINE_SURFACE(1,2,((#124877,#124878,#124879,#124880,#124881,#124882,
#124883),(#124884,#124885,#124886,#124887,#124888,#124889,#124890)),
 .UNSPECIFIED.,.F.,.F.,.F.)
B_SPLINE_SURFACE_WITH_KNOTS((2,2),(3,2,2,3),(0.,0.289681084360176),(0.2113983000937,
0.214285714285714,0.228883374894816,0.229058225642827),.UNSPECIFIED.)
GEOMETRIC_REPRESENTATION_ITEM()
RATIONAL_B_SPLINE_SURFACE(((0.998054921708738,0.998986490969345,1.,0.994876086397761,
0.991846493044686,0.991846493044686,0.991846493044686),(0.998054921708738,
0.998986490969345,1.,0.994876086397761,0.991846493044686,0.991846493044686,
0.991846493044686)))
REPRESENTATION_ITEM('')
SURFACE()
);
#1810=(
BOUNDED_SURFACE()
B_SPLINE_SURFACE(1,2,((#124907,#124908,#124909,#124910,#124911),(#124912,
#124913,#124914,#124915,#124916)),.UNSPECIFIED.,.F.,.F.,.F.)
B_SPLINE_SURFACE_WITH_KNOTS((2,2),(3,2,3),(0.,0.289807040994211),(0.504546746573288,
0.504719756176206,0.522020716468041),.UNSPECIFIED.)
GEOMETRIC_REPRESENTATION_ITEM()
RATIONAL_B_SPLINE_SURFACE(((0.996905579294158,0.996905579294158,0.996905579294158,
0.991635321911186,0.989306890555885),(0.996905579294158,0.996905579294158,
0.996905579294158,0.991635321911186,0.989306890555884)))
REPRESENTATION_ITEM('')
SURFACE()
);
#1811=(
BOUNDED_SURFACE()
B_SPLINE_SURFACE(1,2,((#124918,#124919,#124920,#124921,#124922,#124923,
#124924),(#124925,#124926,#124927,#124928,#124929,#124930,#124931)),
 .UNSPECIFIED.,.F.,.F.,.F.)
B_SPLINE_SURFACE_WITH_KNOTS((2,2),(3,2,2,3),(0.,0.289681084359936),(0.2113983000937,
0.214285714285714,0.228883374894809,0.22905822564282),.UNSPECIFIED.)
GEOMETRIC_REPRESENTATION_ITEM()
RATIONAL_B_SPLINE_SURFACE(((0.998054921708738,0.998986490969345,1.,0.994876086397764,
0.991846493044689,0.991846493044689,0.991846493044689),(0.998054921708738,
0.998986490969345,1.,0.994876086397764,0.991846493044689,0.991846493044689,
0.991846493044689)))
REPRESENTATION_ITEM('')
SURFACE()
);
#1812=(
BOUNDED_SURFACE()
B_SPLINE_SURFACE(1,2,((#124948,#124949,#124950,#124951,#124952),(#124953,
#124954,#124955,#124956,#124957)),.UNSPECIFIED.,.F.,.F.,.F.)
B_SPLINE_SURFACE_WITH_KNOTS((2,2),(3,2,3),(0.,0.289807040993962),(0.504546746573288,
0.504719756176206,0.522020716468041),.UNSPECIFIED.)
GEOMETRIC_REPRESENTATION_ITEM()
RATIONAL_B_SPLINE_SURFACE(((0.996905579294158,0.996905579294158,0.996905579294158,
0.991635321911186,0.989306890555884),(0.996905579294158,0.996905579294158,
0.996905579294158,0.991635321911186,0.989306890555884)))
REPRESENTATION_ITEM('')
SURFACE()
);
#1813=(
BOUNDED_SURFACE()
B_SPLINE_SURFACE(1,2,((#124959,#124960,#124961,#124962,#124963,#124964,
#124965),(#124966,#124967,#124968,#124969,#124970,#124971,#124972)),
 .UNSPECIFIED.,.F.,.F.,.F.)
B_SPLINE_SURFACE_WITH_KNOTS((2,2),(3,2,2,3),(0.,0.289681084359929),(0.211398300093699,
0.214285714285714,0.228883374894879,0.229058225642891),.UNSPECIFIED.)
GEOMETRIC_REPRESENTATION_ITEM()
RATIONAL_B_SPLINE_SURFACE(((0.998054921708738,0.998986490969345,1.,0.994876086397739,
0.99184649304466,0.99184649304466,0.99184649304466),(0.998054921708738,
0.998986490969345,1.,0.994876086397739,0.99184649304466,0.99184649304466,
0.99184649304466)))
REPRESENTATION_ITEM('')
SURFACE()
);
#1814=(
BOUNDED_SURFACE()
B_SPLINE_SURFACE(1,2,((#124994,#124995,#124996,#124997,#124998),(#124999,
#125000,#125001,#125002,#125003)),.UNSPECIFIED.,.F.,.F.,.F.)
B_SPLINE_SURFACE_WITH_KNOTS((2,2),(3,2,3),(0.,0.289807040993889),(0.504546746573288,
0.504719756176206,0.522020716468041),.UNSPECIFIED.)
GEOMETRIC_REPRESENTATION_ITEM()
RATIONAL_B_SPLINE_SURFACE(((0.996905579294158,0.996905579294158,0.996905579294158,
0.991635321911186,0.989306890555884),(0.996905579294158,0.996905579294158,
0.996905579294158,0.991635321911186,0.989306890555884)))
REPRESENTATION_ITEM('')
SURFACE()
);
#1815=(
BOUNDED_SURFACE()
B_SPLINE_SURFACE(1,2,((#125005,#125006,#125007,#125008,#125009,#125010,
#125011),(#125012,#125013,#125014,#125015,#125016,#125017,#125018)),
 .UNSPECIFIED.,.F.,.F.,.F.)
B_SPLINE_SURFACE_WITH_KNOTS((2,2),(3,2,2,3),(0.,0.289681084359923),(0.211398300093701,
0.214285714285714,0.228883374894809,0.22905822564282),.UNSPECIFIED.)
GEOMETRIC_REPRESENTATION_ITEM()
RATIONAL_B_SPLINE_SURFACE(((0.998054921708739,0.998986490969345,1.,0.994876086397764,
0.991846493044689,0.991846493044689,0.991846493044689),(0.998054921708739,
0.998986490969345,1.,0.994876086397764,0.991846493044689,0.991846493044689,
0.991846493044689)))
REPRESENTATION_ITEM('')
SURFACE()
);
#1816=(
BOUNDED_SURFACE()
B_SPLINE_SURFACE(1,2,((#125040,#125041,#125042,#125043,#125044),(#125045,
#125046,#125047,#125048,#125049)),.UNSPECIFIED.,.F.,.F.,.F.)
B_SPLINE_SURFACE_WITH_KNOTS((2,2),(3,2,3),(0.,0.28980704099297),(0.504546746573287,
0.504719756176205,0.52202071646804),.UNSPECIFIED.)
GEOMETRIC_REPRESENTATION_ITEM()
RATIONAL_B_SPLINE_SURFACE(((0.996905579294159,0.996905579294159,0.996905579294159,
0.991635321911186,0.989306890555885),(0.996905579294159,0.996905579294159,
0.996905579294159,0.991635321911186,0.989306890555885)))
REPRESENTATION_ITEM('')
SURFACE()
);
#1817=(
BOUNDED_SURFACE()
B_SPLINE_SURFACE(1,2,((#125051,#125052,#125053,#125054,#125055,#125056,
#125057),(#125058,#125059,#125060,#125061,#125062,#125063,#125064)),
 .UNSPECIFIED.,.F.,.F.,.F.)
B_SPLINE_SURFACE_WITH_KNOTS((2,2),(3,2,2,3),(0.,0.289681084359914),(0.211398300093701,
0.214285714285714,0.22888337489481,0.229058225642821),.UNSPECIFIED.)
GEOMETRIC_REPRESENTATION_ITEM()
RATIONAL_B_SPLINE_SURFACE(((0.998054921708739,0.998986490969346,1.,0.994876086397763,
0.991846493044689,0.991846493044689,0.991846493044689),(0.998054921708739,
0.998986490969346,1.,0.994876086397763,0.991846493044689,0.991846493044689,
0.991846493044689)))
REPRESENTATION_ITEM('')
SURFACE()
);
#1818=(
BOUNDED_SURFACE()
B_SPLINE_SURFACE(1,2,((#125079,#125080,#125081,#125082,#125083),(#125084,
#125085,#125086,#125087,#125088)),.UNSPECIFIED.,.F.,.F.,.F.)
B_SPLINE_SURFACE_WITH_KNOTS((2,2),(3,2,3),(0.,0.290406869879303),(0.262499170173511,
0.263098999273794,0.280537087669266),.UNSPECIFIED.)
GEOMETRIC_REPRESENTATION_ITEM()
RATIONAL_B_SPLINE_SURFACE(((0.989150325841652,0.989150325841652,0.989150325841652,
0.991395311444461,0.996628941948308),(0.989150325841652,0.989150325841652,
0.989150325841652,0.991395311444461,0.996628941948308)))
REPRESENTATION_ITEM('')
SURFACE()
);
#1819=(
BOUNDED_SURFACE()
B_SPLINE_SURFACE(1,2,((#125105,#125106,#125107),(#125108,#125109,#125110)),
 .UNSPECIFIED.,.F.,.F.,.F.)
B_SPLINE_SURFACE_WITH_KNOTS((2,2),(3,3),(0.,0.289681084359935),(0.452822299828566,
0.470019760166367),.UNSPECIFIED.)
GEOMETRIC_REPRESENTATION_ITEM()
RATIONAL_B_SPLINE_SURFACE(((0.98875548626282,0.986817927519786,0.987787102172814),
(0.98875548626282,0.986817927519786,0.987787102172814)))
REPRESENTATION_ITEM('')
SURFACE()
);
#1820=(
BOUNDED_SURFACE()
B_SPLINE_SURFACE(1,2,((#125112,#125113,#125114,#125115,#125116),(#125117,
#125118,#125119,#125120,#125121)),.UNSPECIFIED.,.F.,.F.,.F.)
B_SPLINE_SURFACE_WITH_KNOTS((2,2),(3,2,3),(0.,0.290406869885275),(0.262499170167527,
0.263098999273794,0.280537087669266),.UNSPECIFIED.)
GEOMETRIC_REPRESENTATION_ITEM()
RATIONAL_B_SPLINE_SURFACE(((0.989150325841652,0.989150325841652,0.989150325841652,
0.991395311444461,0.996628941948308),(0.989150325841652,0.989150325841652,
0.989150325841652,0.991395311444461,0.996628941948308)))
REPRESENTATION_ITEM('')
SURFACE()
);
#1821=(
BOUNDED_SURFACE()
B_SPLINE_SURFACE(1,2,((#125138,#125139,#125140),(#125141,#125142,#125143)),
 .UNSPECIFIED.,.F.,.F.,.F.)
B_SPLINE_SURFACE_WITH_KNOTS((2,2),(3,3),(0.,0.289681084359924),(0.452822299828566,
0.470019760166367),.UNSPECIFIED.)
GEOMETRIC_REPRESENTATION_ITEM()
RATIONAL_B_SPLINE_SURFACE(((0.98875548626282,0.986817927519786,0.987787102172814),
(0.98875548626282,0.986817927519786,0.987787102172814)))
REPRESENTATION_ITEM('')
SURFACE()
);
#1822=(
BOUNDED_SURFACE()
B_SPLINE_SURFACE(1,2,((#125145,#125146,#125147,#125148,#125149),(#125150,
#125151,#125152,#125153,#125154)),.UNSPECIFIED.,.F.,.F.,.F.)
B_SPLINE_SURFACE_WITH_KNOTS((2,2),(3,2,3),(0.,0.290406869890717),(0.262499170162089,
0.263098999273794,0.280537087669266),.UNSPECIFIED.)
GEOMETRIC_REPRESENTATION_ITEM()
RATIONAL_B_SPLINE_SURFACE(((0.989150325841652,0.989150325841652,0.989150325841652,
0.991395311444461,0.996628941948308),(0.989150325841652,0.989150325841652,
0.989150325841652,0.991395311444461,0.996628941948308)))
REPRESENTATION_ITEM('')
SURFACE()
);
#1823=(
BOUNDED_SURFACE()
B_SPLINE_SURFACE(1,2,((#125171,#125172,#125173),(#125174,#125175,#125176)),
 .UNSPECIFIED.,.F.,.F.,.F.)
B_SPLINE_SURFACE_WITH_KNOTS((2,2),(3,3),(0.,0.289681084359928),(0.452822299828566,
0.470019760166367),.UNSPECIFIED.)
GEOMETRIC_REPRESENTATION_ITEM()
RATIONAL_B_SPLINE_SURFACE(((0.98875548626282,0.986817927519786,0.987787102172814),
(0.98875548626282,0.986817927519786,0.987787102172814)))
REPRESENTATION_ITEM('')
SURFACE()
);
#1824=(
BOUNDED_SURFACE()
B_SPLINE_SURFACE(1,2,((#125178,#125179,#125180,#125181,#125182),(#125183,
#125184,#125185,#125186,#125187)),.UNSPECIFIED.,.F.,.F.,.F.)
B_SPLINE_SURFACE_WITH_KNOTS((2,2),(3,2,3),(0.,0.290406869901633),(0.262499170151171,
0.263098999273794,0.280537087669266),.UNSPECIFIED.)
GEOMETRIC_REPRESENTATION_ITEM()
RATIONAL_B_SPLINE_SURFACE(((0.989150325841652,0.989150325841652,0.989150325841652,
0.991395311444461,0.996628941948308),(0.989150325841652,0.989150325841652,
0.989150325841652,0.991395311444461,0.996628941948308)))
REPRESENTATION_ITEM('')
SURFACE()
);
#1825=(
BOUNDED_SURFACE()
B_SPLINE_SURFACE(1,2,((#125204,#125205,#125206),(#125207,#125208,#125209)),
 .UNSPECIFIED.,.F.,.F.,.F.)
B_SPLINE_SURFACE_WITH_KNOTS((2,2),(3,3),(0.,0.289681084359924),(0.452822299828566,
0.470019760166366),.UNSPECIFIED.)
GEOMETRIC_REPRESENTATION_ITEM()
RATIONAL_B_SPLINE_SURFACE(((0.98875548626282,0.986817927519786,0.987787102172814),
(0.98875548626282,0.986817927519786,0.987787102172814)))
REPRESENTATION_ITEM('')
SURFACE()
);
#1826=(
BOUNDED_SURFACE()
B_SPLINE_SURFACE(1,2,((#125211,#125212,#125213,#125214,#125215),(#125216,
#125217,#125218,#125219,#125220)),.UNSPECIFIED.,.F.,.F.,.F.)
B_SPLINE_SURFACE_WITH_KNOTS((2,2),(3,2,3),(0.,0.290406869898682),(0.262499170154123,
0.263098999273794,0.280537087669266),.UNSPECIFIED.)
GEOMETRIC_REPRESENTATION_ITEM()
RATIONAL_B_SPLINE_SURFACE(((0.989150325841652,0.989150325841652,0.989150325841652,
0.991395311444461,0.996628941948308),(0.989150325841652,0.989150325841652,
0.989150325841652,0.991395311444461,0.996628941948308)))
REPRESENTATION_ITEM('')
SURFACE()
);
#1827=(
BOUNDED_SURFACE()
B_SPLINE_SURFACE(1,2,((#125237,#125238,#125239),(#125240,#125241,#125242)),
 .UNSPECIFIED.,.F.,.F.,.F.)
B_SPLINE_SURFACE_WITH_KNOTS((2,2),(3,3),(0.,0.289681084359916),(0.452822299828566,
0.470019760166367),.UNSPECIFIED.)
GEOMETRIC_REPRESENTATION_ITEM()
RATIONAL_B_SPLINE_SURFACE(((0.98875548626282,0.986817927519786,0.987787102172814),
(0.98875548626282,0.986817927519786,0.987787102172814)))
REPRESENTATION_ITEM('')
SURFACE()
);
#1828=(
BOUNDED_SURFACE()
B_SPLINE_SURFACE(1,2,((#125244,#125245,#125246,#125247,#125248),(#125249,
#125250,#125251,#125252,#125253)),.UNSPECIFIED.,.F.,.F.,.F.)
B_SPLINE_SURFACE_WITH_KNOTS((2,2),(3,2,3),(0.,0.290406869896393),(0.262499170156412,
0.263098999273794,0.280537087669266),.UNSPECIFIED.)
GEOMETRIC_REPRESENTATION_ITEM()
RATIONAL_B_SPLINE_SURFACE(((0.989150325841652,0.989150325841652,0.989150325841652,
0.991395311444461,0.996628941948308),(0.989150325841652,0.989150325841652,
0.989150325841652,0.991395311444461,0.996628941948308)))
REPRESENTATION_ITEM('')
SURFACE()
);
#1829=(
BOUNDED_SURFACE()
B_SPLINE_SURFACE(1,2,((#125270,#125271,#125272),(#125273,#125274,#125275)),
 .UNSPECIFIED.,.F.,.F.,.F.)
B_SPLINE_SURFACE_WITH_KNOTS((2,2),(3,3),(0.,0.289681084359921),(0.452822299828566,
0.470019760166367),.UNSPECIFIED.)
GEOMETRIC_REPRESENTATION_ITEM()
RATIONAL_B_SPLINE_SURFACE(((0.98875548626282,0.986817927519786,0.987787102172814),
(0.98875548626282,0.986817927519786,0.987787102172814)))
REPRESENTATION_ITEM('')
SURFACE()
);
#1830=(
BOUNDED_SURFACE()
B_SPLINE_SURFACE(1,2,((#125277,#125278,#125279,#125280,#125281),(#125282,
#125283,#125284,#125285,#125286)),.UNSPECIFIED.,.F.,.F.,.F.)
B_SPLINE_SURFACE_WITH_KNOTS((2,2),(3,2,3),(0.,0.290406869895255),(0.262499170157545,
0.263098999273794,0.280537087669266),.UNSPECIFIED.)
GEOMETRIC_REPRESENTATION_ITEM()
RATIONAL_B_SPLINE_SURFACE(((0.989150325841652,0.989150325841652,0.989150325841652,
0.991395311444461,0.996628941948308),(0.989150325841652,0.989150325841652,
0.989150325841652,0.991395311444461,0.996628941948308)))
REPRESENTATION_ITEM('')
SURFACE()
);
#1831=(
BOUNDED_SURFACE()
B_SPLINE_SURFACE(1,2,((#125303,#125304,#125305),(#125306,#125307,#125308)),
 .UNSPECIFIED.,.F.,.F.,.F.)
B_SPLINE_SURFACE_WITH_KNOTS((2,2),(3,3),(0.,0.289681084359914),(0.452822299828566,
0.470019760166366),.UNSPECIFIED.)
GEOMETRIC_REPRESENTATION_ITEM()
RATIONAL_B_SPLINE_SURFACE(((0.98875548626282,0.986817927519786,0.987787102172814),
(0.98875548626282,0.986817927519786,0.987787102172814)))
REPRESENTATION_ITEM('')
SURFACE()
);
#1832=(
BOUNDED_SURFACE()
B_SPLINE_SURFACE(1,2,((#125310,#125311,#125312,#125313,#125314),(#125315,
#125316,#125317,#125318,#125319)),.UNSPECIFIED.,.F.,.F.,.F.)
B_SPLINE_SURFACE_WITH_KNOTS((2,2),(3,2,3),(0.,0.290406869893768),(0.262499170159038,
0.263098999273794,0.280537087669266),.UNSPECIFIED.)
GEOMETRIC_REPRESENTATION_ITEM()
RATIONAL_B_SPLINE_SURFACE(((0.989150325841652,0.989150325841652,0.989150325841652,
0.991395311444461,0.996628941948308),(0.989150325841652,0.989150325841652,
0.989150325841652,0.991395311444461,0.996628941948308)))
REPRESENTATION_ITEM('')
SURFACE()
);
#1833=(
BOUNDED_SURFACE()
B_SPLINE_SURFACE(1,2,((#125336,#125337,#125338),(#125339,#125340,#125341)),
 .UNSPECIFIED.,.F.,.F.,.F.)
B_SPLINE_SURFACE_WITH_KNOTS((2,2),(3,3),(0.,0.289681084359924),(0.452822299828566,
0.470019760166367),.UNSPECIFIED.)
GEOMETRIC_REPRESENTATION_ITEM()
RATIONAL_B_SPLINE_SURFACE(((0.98875548626282,0.986817927519786,0.987787102172814),
(0.98875548626282,0.986817927519786,0.987787102172814)))
REPRESENTATION_ITEM('')
SURFACE()
);
#1834=(
BOUNDED_SURFACE()
B_SPLINE_SURFACE(1,2,((#125343,#125344,#125345,#125346,#125347),(#125348,
#125349,#125350,#125351,#125352)),.UNSPECIFIED.,.F.,.F.,.F.)
B_SPLINE_SURFACE_WITH_KNOTS((2,2),(3,2,3),(0.,0.290406869888898),(0.262499170163906,
0.263098999273794,0.280537087669266),.UNSPECIFIED.)
GEOMETRIC_REPRESENTATION_ITEM()
RATIONAL_B_SPLINE_SURFACE(((0.989150325841652,0.989150325841652,0.989150325841652,
0.991395311444461,0.996628941948308),(0.989150325841652,0.989150325841652,
0.989150325841652,0.991395311444461,0.996628941948308)))
REPRESENTATION_ITEM('')
SURFACE()
);
#1835=(
BOUNDED_SURFACE()
B_SPLINE_SURFACE(1,2,((#125369,#125370,#125371),(#125372,#125373,#125374)),
 .UNSPECIFIED.,.F.,.F.,.F.)
B_SPLINE_SURFACE_WITH_KNOTS((2,2),(3,3),(0.,0.289681084359924),(0.452822299828566,
0.470019760166367),.UNSPECIFIED.)
GEOMETRIC_REPRESENTATION_ITEM()
RATIONAL_B_SPLINE_SURFACE(((0.98875548626282,0.986817927519786,0.987787102172814),
(0.98875548626282,0.986817927519786,0.987787102172814)))
REPRESENTATION_ITEM('')
SURFACE()
);
#1836=(
BOUNDED_SURFACE()
B_SPLINE_SURFACE(1,2,((#125376,#125377,#125378,#125379,#125380),(#125381,
#125382,#125383,#125384,#125385)),.UNSPECIFIED.,.F.,.F.,.F.)
B_SPLINE_SURFACE_WITH_KNOTS((2,2),(3,2,3),(0.,0.290406869893245),(0.262499170159558,
0.263098999273794,0.280537087669266),.UNSPECIFIED.)
GEOMETRIC_REPRESENTATION_ITEM()
RATIONAL_B_SPLINE_SURFACE(((0.989150325841652,0.989150325841652,0.989150325841652,
0.991395311444461,0.996628941948308),(0.989150325841652,0.989150325841652,
0.989150325841652,0.991395311444461,0.996628941948308)))
REPRESENTATION_ITEM('')
SURFACE()
);
#1837=(
BOUNDED_SURFACE()
B_SPLINE_SURFACE(1,2,((#125402,#125403,#125404),(#125405,#125406,#125407)),
 .UNSPECIFIED.,.F.,.F.,.F.)
B_SPLINE_SURFACE_WITH_KNOTS((2,2),(3,3),(0.,0.289681084359924),(0.452822299828566,
0.470019760166501),.UNSPECIFIED.)
GEOMETRIC_REPRESENTATION_ITEM()
RATIONAL_B_SPLINE_SURFACE(((0.988755486262821,0.986817927519771,0.987787102172829),
(0.988755486262821,0.986817927519771,0.987787102172829)))
REPRESENTATION_ITEM('')
SURFACE()
);
#1838=(
BOUNDED_SURFACE()
B_SPLINE_SURFACE(1,2,((#125409,#125410,#125411,#125412,#125413),(#125414,
#125415,#125416,#125417,#125418)),.UNSPECIFIED.,.F.,.F.,.F.)
B_SPLINE_SURFACE_WITH_KNOTS((2,2),(3,2,3),(0.,0.290406869899846),(0.262499170152963,
0.263098999273796,0.280537087669266),.UNSPECIFIED.)
GEOMETRIC_REPRESENTATION_ITEM()
RATIONAL_B_SPLINE_SURFACE(((0.989150325841653,0.989150325841653,0.989150325841653,
0.991395311444461,0.996628941948308),(0.989150325841653,0.989150325841653,
0.989150325841653,0.991395311444461,0.996628941948308)))
REPRESENTATION_ITEM('')
SURFACE()
);
#1839=(
BOUNDED_SURFACE()
B_SPLINE_SURFACE(1,2,((#125435,#125436,#125437),(#125438,#125439,#125440)),
 .UNSPECIFIED.,.F.,.F.,.F.)
B_SPLINE_SURFACE_WITH_KNOTS((2,2),(3,3),(0.,0.289681084359926),(0.452822299828566,
0.470019760166501),.UNSPECIFIED.)
GEOMETRIC_REPRESENTATION_ITEM()
RATIONAL_B_SPLINE_SURFACE(((0.988755486262821,0.986817927519771,0.987787102172829),
(0.988755486262821,0.986817927519771,0.987787102172829)))
REPRESENTATION_ITEM('')
SURFACE()
);
#1840=(
BOUNDED_SURFACE()
B_SPLINE_SURFACE(1,2,((#125442,#125443,#125444,#125445,#125446),(#125447,
#125448,#125449,#125450,#125451)),.UNSPECIFIED.,.F.,.F.,.F.)
B_SPLINE_SURFACE_WITH_KNOTS((2,2),(3,2,3),(0.,0.29040686990032),(0.262499170152489,
0.263098999273796,0.280537087669266),.UNSPECIFIED.)
GEOMETRIC_REPRESENTATION_ITEM()
RATIONAL_B_SPLINE_SURFACE(((0.989150325841653,0.989150325841653,0.989150325841653,
0.991395311444461,0.996628941948308),(0.989150325841653,0.989150325841653,
0.989150325841653,0.991395311444461,0.996628941948308)))
REPRESENTATION_ITEM('')
SURFACE()
);
#1841=(
BOUNDED_SURFACE()
B_SPLINE_SURFACE(1,2,((#125468,#125469,#125470),(#125471,#125472,#125473)),
 .UNSPECIFIED.,.F.,.F.,.F.)
B_SPLINE_SURFACE_WITH_KNOTS((2,2),(3,3),(0.,0.289681084359922),(0.452822299828566,
0.470019760166501),.UNSPECIFIED.)
GEOMETRIC_REPRESENTATION_ITEM()
RATIONAL_B_SPLINE_SURFACE(((0.988755486262821,0.986817927519771,0.987787102172829),
(0.988755486262821,0.986817927519771,0.987787102172829)))
REPRESENTATION_ITEM('')
SURFACE()
);
#1842=(
BOUNDED_SURFACE()
B_SPLINE_SURFACE(1,2,((#125475,#125476,#125477,#125478,#125479),(#125480,
#125481,#125482,#125483,#125484)),.UNSPECIFIED.,.F.,.F.,.F.)
B_SPLINE_SURFACE_WITH_KNOTS((2,2),(3,2,3),(0.,0.290406869901643),(0.262499170151161,
0.263098999273794,0.280537087669266),.UNSPECIFIED.)
GEOMETRIC_REPRESENTATION_ITEM()
RATIONAL_B_SPLINE_SURFACE(((0.989150325841652,0.989150325841652,0.989150325841652,
0.991395311444461,0.996628941948308),(0.989150325841653,0.989150325841653,
0.989150325841653,0.991395311444461,0.996628941948308)))
REPRESENTATION_ITEM('')
SURFACE()
);
#1843=(
BOUNDED_SURFACE()
B_SPLINE_SURFACE(1,2,((#125501,#125502,#125503),(#125504,#125505,#125506)),
 .UNSPECIFIED.,.F.,.F.,.F.)
B_SPLINE_SURFACE_WITH_KNOTS((2,2),(3,3),(0.,0.289681084359917),(0.452822299828566,
0.470019760166501),.UNSPECIFIED.)
GEOMETRIC_REPRESENTATION_ITEM()
RATIONAL_B_SPLINE_SURFACE(((0.988755486262821,0.986817927519771,0.987787102172829),
(0.988755486262821,0.986817927519771,0.987787102172829)))
REPRESENTATION_ITEM('')
SURFACE()
);
#1844=(
BOUNDED_SURFACE()
B_SPLINE_SURFACE(1,2,((#125508,#125509,#125510,#125511,#125512),(#125513,
#125514,#125515,#125516,#125517)),.UNSPECIFIED.,.F.,.F.,.F.)
B_SPLINE_SURFACE_WITH_KNOTS((2,2),(3,2,3),(0.,0.290406869900499),(0.262499170152311,
0.263098999273794,0.280537087669266),.UNSPECIFIED.)
GEOMETRIC_REPRESENTATION_ITEM()
RATIONAL_B_SPLINE_SURFACE(((0.989150325841652,0.989150325841652,0.989150325841652,
0.991395311444461,0.996628941948308),(0.989150325841652,0.989150325841652,
0.989150325841652,0.991395311444461,0.996628941948308)))
REPRESENTATION_ITEM('')
SURFACE()
);
#1845=(
BOUNDED_SURFACE()
B_SPLINE_SURFACE(1,2,((#125534,#125535,#125536),(#125537,#125538,#125539)),
 .UNSPECIFIED.,.F.,.F.,.F.)
B_SPLINE_SURFACE_WITH_KNOTS((2,2),(3,3),(0.,0.289681084359924),(0.452822299828566,
0.470019760166501),.UNSPECIFIED.)
GEOMETRIC_REPRESENTATION_ITEM()
RATIONAL_B_SPLINE_SURFACE(((0.988755486262821,0.986817927519771,0.987787102172829),
(0.98875548626282,0.986817927519771,0.987787102172829)))
REPRESENTATION_ITEM('')
SURFACE()
);
#1846=(
BOUNDED_SURFACE()
B_SPLINE_SURFACE(1,2,((#125541,#125542,#125543,#125544,#125545),(#125546,
#125547,#125548,#125549,#125550)),.UNSPECIFIED.,.F.,.F.,.F.)
B_SPLINE_SURFACE_WITH_KNOTS((2,2),(3,2,3),(0.,0.290038654277662),(0.262867385775147,
0.263098999273794,0.280537087669266),.UNSPECIFIED.)
GEOMETRIC_REPRESENTATION_ITEM()
RATIONAL_B_SPLINE_SURFACE(((0.989150325841652,0.989150325841652,0.989150325841652,
0.991395311444461,0.996628941948308),(0.989150325841652,0.989150325841652,
0.989150325841652,0.991395311444461,0.996628941948308)))
REPRESENTATION_ITEM('')
SURFACE()
);
#1847=(
BOUNDED_SURFACE()
B_SPLINE_SURFACE(1,2,((#125558,#125559,#125560),(#125561,#125562,#125563)),
 .UNSPECIFIED.,.F.,.F.,.F.)
B_SPLINE_SURFACE_WITH_KNOTS((2,2),(3,3),(0.,0.289681084359922),(0.452822299828566,
0.470019760166501),.UNSPECIFIED.)
GEOMETRIC_REPRESENTATION_ITEM()
RATIONAL_B_SPLINE_SURFACE(((0.988755486262821,0.986817927519771,0.987787102172829),
(0.988755486262821,0.986817927519771,0.987787102172829)))
REPRESENTATION_ITEM('')
SURFACE()
);
#1848=(
BOUNDED_SURFACE()
B_SPLINE_SURFACE(1,2,((#125565,#125566,#125567,#125568,#125569),(#125570,
#125571,#125572,#125573,#125574)),.UNSPECIFIED.,.F.,.F.,.F.)
B_SPLINE_SURFACE_WITH_KNOTS((2,2),(3,2,3),(0.,0.290406869901189),(0.262499170151615,
0.263098999273794,0.280537087669266),.UNSPECIFIED.)
GEOMETRIC_REPRESENTATION_ITEM()
RATIONAL_B_SPLINE_SURFACE(((0.989150325841652,0.989150325841652,0.989150325841652,
0.991395311444461,0.996628941948308),(0.989150325841652,0.989150325841652,
0.989150325841652,0.991395311444461,0.996628941948308)))
REPRESENTATION_ITEM('')
SURFACE()
);
#1849=(
BOUNDED_SURFACE()
B_SPLINE_SURFACE(1,2,((#125591,#125592,#125593),(#125594,#125595,#125596)),
 .UNSPECIFIED.,.F.,.F.,.F.)
B_SPLINE_SURFACE_WITH_KNOTS((2,2),(3,3),(0.,0.289681084359921),(0.452822299828566,
0.470019760166501),.UNSPECIFIED.)
GEOMETRIC_REPRESENTATION_ITEM()
RATIONAL_B_SPLINE_SURFACE(((0.98875548626282,0.986817927519771,0.987787102172829),
(0.98875548626282,0.986817927519771,0.987787102172829)))
REPRESENTATION_ITEM('')
SURFACE()
);
#1850=(
BOUNDED_SURFACE()
B_SPLINE_SURFACE(1,2,((#125598,#125599,#125600,#125601,#125602),(#125603,
#125604,#125605,#125606,#125607)),.UNSPECIFIED.,.F.,.F.,.F.)
B_SPLINE_SURFACE_WITH_KNOTS((2,2),(3,2,3),(0.,0.290406869898487),(0.26249917015432,
0.263098999273794,0.280537087669266),.UNSPECIFIED.)
GEOMETRIC_REPRESENTATION_ITEM()
RATIONAL_B_SPLINE_SURFACE(((0.989150325841652,0.989150325841652,0.989150325841652,
0.991395311444461,0.996628941948308),(0.989150325841652,0.989150325841652,
0.989150325841652,0.991395311444461,0.996628941948308)))
REPRESENTATION_ITEM('')
SURFACE()
);
#1851=(
BOUNDED_SURFACE()
B_SPLINE_SURFACE(1,2,((#125624,#125625,#125626),(#125627,#125628,#125629)),
 .UNSPECIFIED.,.F.,.F.,.F.)
B_SPLINE_SURFACE_WITH_KNOTS((2,2),(3,3),(0.,0.289681084359928),(0.452822299828566,
0.470019760166367),.UNSPECIFIED.)
GEOMETRIC_REPRESENTATION_ITEM()
RATIONAL_B_SPLINE_SURFACE(((0.98875548626282,0.986817927519786,0.987787102172814),
(0.98875548626282,0.986817927519786,0.987787102172814)))
REPRESENTATION_ITEM('')
SURFACE()
);
#1852=(
BOUNDED_SURFACE()
B_SPLINE_SURFACE(1,2,((#125631,#125632,#125633,#125634,#125635),(#125636,
#125637,#125638,#125639,#125640)),.UNSPECIFIED.,.F.,.F.,.F.)
B_SPLINE_SURFACE_WITH_KNOTS((2,2),(3,2,3),(0.,0.290406869899282),(0.262499170153521,
0.263098999273794,0.280537087669266),.UNSPECIFIED.)
GEOMETRIC_REPRESENTATION_ITEM()
RATIONAL_B_SPLINE_SURFACE(((0.989150325841652,0.989150325841652,0.989150325841652,
0.991395311444461,0.996628941948308),(0.989150325841652,0.989150325841652,
0.989150325841652,0.991395311444461,0.996628941948308)))
REPRESENTATION_ITEM('')
SURFACE()
);
#1853=(
BOUNDED_SURFACE()
B_SPLINE_SURFACE(1,2,((#125657,#125658,#125659),(#125660,#125661,#125662)),
 .UNSPECIFIED.,.F.,.F.,.F.)
B_SPLINE_SURFACE_WITH_KNOTS((2,2),(3,3),(0.,0.289681084359918),(0.452822299828566,
0.470019760166367),.UNSPECIFIED.)
GEOMETRIC_REPRESENTATION_ITEM()
RATIONAL_B_SPLINE_SURFACE(((0.98875548626282,0.986817927519786,0.987787102172814),
(0.98875548626282,0.986817927519786,0.987787102172814)))
REPRESENTATION_ITEM('')
SURFACE()
);
#1854=(
BOUNDED_SURFACE()
B_SPLINE_SURFACE(1,2,((#125664,#125665,#125666,#125667,#125668),(#125669,
#125670,#125671,#125672,#125673)),.UNSPECIFIED.,.F.,.F.,.F.)
B_SPLINE_SURFACE_WITH_KNOTS((2,2),(3,2,3),(0.,0.290406869910884),(0.262499170141919,
0.263098999273794,0.280537087669266),.UNSPECIFIED.)
GEOMETRIC_REPRESENTATION_ITEM()
RATIONAL_B_SPLINE_SURFACE(((0.989150325841652,0.989150325841652,0.989150325841652,
0.991395311444461,0.996628941948308),(0.989150325841652,0.989150325841652,
0.989150325841652,0.991395311444461,0.996628941948308)))
REPRESENTATION_ITEM('')
SURFACE()
);
#1855=(
BOUNDED_SURFACE()
B_SPLINE_SURFACE(1,2,((#125690,#125691,#125692),(#125693,#125694,#125695)),
 .UNSPECIFIED.,.F.,.F.,.F.)
B_SPLINE_SURFACE_WITH_KNOTS((2,2),(3,3),(0.,0.289681084359921),(0.452822299828567,
0.470019760166367),.UNSPECIFIED.)
GEOMETRIC_REPRESENTATION_ITEM()
RATIONAL_B_SPLINE_SURFACE(((0.98875548626282,0.986817927519786,0.987787102172814),
(0.98875548626282,0.986817927519786,0.987787102172814)))
REPRESENTATION_ITEM('')
SURFACE()
);
#1856=(
BOUNDED_SURFACE()
B_SPLINE_SURFACE(1,2,((#125697,#125698,#125699,#125700,#125701),(#125702,
#125703,#125704,#125705,#125706)),.UNSPECIFIED.,.F.,.F.,.F.)
B_SPLINE_SURFACE_WITH_KNOTS((2,2),(3,2,3),(0.,0.290406869918552),(0.262499170134253,
0.263098999273794,0.280537087669266),.UNSPECIFIED.)
GEOMETRIC_REPRESENTATION_ITEM()
RATIONAL_B_SPLINE_SURFACE(((0.989150325841652,0.989150325841652,0.989150325841652,
0.991395311444461,0.996628941948308),(0.989150325841652,0.989150325841652,
0.989150325841652,0.991395311444461,0.996628941948308)))
REPRESENTATION_ITEM('')
SURFACE()
);
#1857=(
BOUNDED_SURFACE()
B_SPLINE_SURFACE(1,2,((#125723,#125724,#125725),(#125726,#125727,#125728)),
 .UNSPECIFIED.,.F.,.F.,.F.)
B_SPLINE_SURFACE_WITH_KNOTS((2,2),(3,3),(0.,0.28968108435992),(0.452822299828566,
0.470019760166367),.UNSPECIFIED.)
GEOMETRIC_REPRESENTATION_ITEM()
RATIONAL_B_SPLINE_SURFACE(((0.98875548626282,0.986817927519786,0.987787102172814),
(0.98875548626282,0.986817927519786,0.987787102172814)))
REPRESENTATION_ITEM('')
SURFACE()
);
#1858=(
BOUNDED_SURFACE()
B_SPLINE_SURFACE(1,2,((#125730,#125731,#125732,#125733,#125734),(#125735,
#125736,#125737,#125738,#125739)),.UNSPECIFIED.,.F.,.F.,.F.)
B_SPLINE_SURFACE_WITH_KNOTS((2,2),(3,2,3),(0.,0.290406869903407),(0.262499170150806,
0.263098999273794,0.280537087669266),.UNSPECIFIED.)
GEOMETRIC_REPRESENTATION_ITEM()
RATIONAL_B_SPLINE_SURFACE(((0.989150325841652,0.989150325841652,0.989150325841652,
0.991395311444461,0.996628941948308),(0.989150325841652,0.989150325841652,
0.989150325841652,0.991395311444461,0.996628941948308)))
REPRESENTATION_ITEM('')
SURFACE()
);
#1859=(
BOUNDED_SURFACE()
B_SPLINE_SURFACE(1,2,((#125756,#125757,#125758),(#125759,#125760,#125761)),
 .UNSPECIFIED.,.F.,.F.,.F.)
B_SPLINE_SURFACE_WITH_KNOTS((2,2),(3,3),(0.,0.289681084359922),(0.452822299828566,
0.470019760166367),.UNSPECIFIED.)
GEOMETRIC_REPRESENTATION_ITEM()
RATIONAL_B_SPLINE_SURFACE(((0.98875548626282,0.986817927519786,0.987787102172814),
(0.98875548626282,0.986817927519786,0.987787102172814)))
REPRESENTATION_ITEM('')
SURFACE()
);
#1860=(
BOUNDED_SURFACE()
B_SPLINE_SURFACE(1,2,((#125763,#125764,#125765,#125766,#125767),(#125768,
#125769,#125770,#125771,#125772)),.UNSPECIFIED.,.F.,.F.,.F.)
B_SPLINE_SURFACE_WITH_KNOTS((2,2),(3,2,3),(0.,0.290406869880632),(0.26249917017217,
0.263098999273794,0.280537087669266),.UNSPECIFIED.)
GEOMETRIC_REPRESENTATION_ITEM()
RATIONAL_B_SPLINE_SURFACE(((0.989150325841652,0.989150325841652,0.989150325841652,
0.991395311444461,0.996628941948308),(0.989150325841652,0.989150325841652,
0.989150325841652,0.991395311444461,0.996628941948308)))
REPRESENTATION_ITEM('')
SURFACE()
);
#1861=(
BOUNDED_SURFACE()
B_SPLINE_SURFACE(1,2,((#125783,#125784,#125785),(#125786,#125787,#125788)),
 .UNSPECIFIED.,.F.,.F.,.F.)
B_SPLINE_SURFACE_WITH_KNOTS((2,2),(3,3),(0.,0.289681084359921),(0.452822299828567,
0.470019760166369),.UNSPECIFIED.)
GEOMETRIC_REPRESENTATION_ITEM()
RATIONAL_B_SPLINE_SURFACE(((0.98875548626282,0.986817927519786,0.987787102172814),
(0.98875548626282,0.986817927519786,0.987787102172814)))
REPRESENTATION_ITEM('')
SURFACE()
);
#1862=(
BOUNDED_SURFACE()
B_SPLINE_SURFACE(1,2,((#125796,#125797,#125798,#125799,#125800),(#125801,
#125802,#125803,#125804,#125805)),.UNSPECIFIED.,.F.,.F.,.F.)
B_SPLINE_SURFACE_WITH_KNOTS((2,2),(3,2,3),(0.,0.290406869877571),(0.262499170175233,
0.263098999273796,0.280537087669266),.UNSPECIFIED.)
GEOMETRIC_REPRESENTATION_ITEM()
RATIONAL_B_SPLINE_SURFACE(((0.989150325841653,0.989150325841653,0.989150325841653,
0.991395311444461,0.996628941948308),(0.989150325841653,0.989150325841653,
0.989150325841653,0.991395311444461,0.996628941948308)))
REPRESENTATION_ITEM('')
SURFACE()
);
#1863=(
BOUNDED_SURFACE()
B_SPLINE_SURFACE(1,2,((#125822,#125823,#125824),(#125825,#125826,#125827)),
 .UNSPECIFIED.,.F.,.F.,.F.)
B_SPLINE_SURFACE_WITH_KNOTS((2,2),(3,3),(0.,0.289681084359925),(0.452822299828567,
0.470019760166366),.UNSPECIFIED.)
GEOMETRIC_REPRESENTATION_ITEM()
RATIONAL_B_SPLINE_SURFACE(((0.98875548626282,0.986817927519786,0.987787102172814),
(0.98875548626282,0.986817927519787,0.987787102172814)))
REPRESENTATION_ITEM('')
SURFACE()
);
#1864=(
BOUNDED_SURFACE()
B_SPLINE_SURFACE(1,2,((#125829,#125830,#125831,#125832,#125833),(#125834,
#125835,#125836,#125837,#125838)),.UNSPECIFIED.,.F.,.F.,.F.)
B_SPLINE_SURFACE_WITH_KNOTS((2,2),(3,2,3),(0.,0.290406869909595),(0.262499170143283,
0.263098999273795,0.280537087669267),.UNSPECIFIED.)
GEOMETRIC_REPRESENTATION_ITEM()
RATIONAL_B_SPLINE_SURFACE(((0.989150325841653,0.989150325841653,0.989150325841653,
0.991395311444461,0.996628941948308),(0.989150325841653,0.989150325841653,
0.989150325841653,0.991395311444461,0.996628941948308)))
REPRESENTATION_ITEM('')
SURFACE()
);
#1865=(
BOUNDED_SURFACE()
B_SPLINE_SURFACE(1,2,((#125855,#125856,#125857),(#125858,#125859,#125860)),
 .UNSPECIFIED.,.F.,.F.,.F.)
B_SPLINE_SURFACE_WITH_KNOTS((2,2),(3,3),(0.,0.289681084359917),(0.452822299828565,
0.470019760166369),.UNSPECIFIED.)
GEOMETRIC_REPRESENTATION_ITEM()
RATIONAL_B_SPLINE_SURFACE(((0.988755486262821,0.986817927519786,0.987787102172814),
(0.988755486262821,0.986817927519786,0.987787102172814)))
REPRESENTATION_ITEM('')
SURFACE()
);
#1866=(
BOUNDED_SURFACE()
B_SPLINE_SURFACE(1,2,((#125862,#125863,#125864,#125865,#125866),(#125867,
#125868,#125869,#125870,#125871)),.UNSPECIFIED.,.F.,.F.,.F.)
B_SPLINE_SURFACE_WITH_KNOTS((2,2),(3,2,3),(0.,0.290406869891073),(0.262499170161812,
0.263098999273795,0.280537087669267),.UNSPECIFIED.)
GEOMETRIC_REPRESENTATION_ITEM()
RATIONAL_B_SPLINE_SURFACE(((0.989150325841653,0.989150325841653,0.989150325841653,
0.991395311444461,0.996628941948308),(0.989150325841653,0.989150325841653,
0.989150325841653,0.991395311444461,0.996628941948308)))
REPRESENTATION_ITEM('')
SURFACE()
);
#1867=(
BOUNDED_SURFACE()
B_SPLINE_SURFACE(1,2,((#125888,#125889,#125890),(#125891,#125892,#125893)),
 .UNSPECIFIED.,.F.,.F.,.F.)
B_SPLINE_SURFACE_WITH_KNOTS((2,2),(3,3),(0.,0.289681084359919),(0.452822299828565,
0.470019760166396),.UNSPECIFIED.)
GEOMETRIC_REPRESENTATION_ITEM()
RATIONAL_B_SPLINE_SURFACE(((0.988755486262821,0.986817927519783,0.987787102172817),
(0.988755486262821,0.986817927519783,0.987787102172817)))
REPRESENTATION_ITEM('')
SURFACE()
);
#1868=(
BOUNDED_SURFACE()
B_SPLINE_SURFACE(1,2,((#125895,#125896,#125897,#125898,#125899),(#125900,
#125901,#125902,#125903,#125904)),.UNSPECIFIED.,.F.,.F.,.F.)
B_SPLINE_SURFACE_WITH_KNOTS((2,2),(3,2,3),(0.,0.290406869911321),(0.262499170142164,
0.263098999273795,0.280537087669267),.UNSPECIFIED.)
GEOMETRIC_REPRESENTATION_ITEM()
RATIONAL_B_SPLINE_SURFACE(((0.989150325841653,0.989150325841653,0.989150325841653,
0.991395311444461,0.996628941948308),(0.989150325841653,0.989150325841653,
0.989150325841653,0.991395311444461,0.996628941948308)))
REPRESENTATION_ITEM('')
SURFACE()
);
#1869=(
BOUNDED_SURFACE()
B_SPLINE_SURFACE(1,2,((#125921,#125922,#125923),(#125924,#125925,#125926)),
 .UNSPECIFIED.,.F.,.F.,.F.)
B_SPLINE_SURFACE_WITH_KNOTS((2,2),(3,3),(0.,0.289681084359927),(0.452822299828565,
0.470019760166366),.UNSPECIFIED.)
GEOMETRIC_REPRESENTATION_ITEM()
RATIONAL_B_SPLINE_SURFACE(((0.988755486262821,0.986817927519786,0.987787102172814),
(0.988755486262821,0.986817927519787,0.987787102172814)))
REPRESENTATION_ITEM('')
SURFACE()
);
#1870=(
BOUNDED_SURFACE()
B_SPLINE_SURFACE(1,2,((#125928,#125929,#125930,#125931,#125932),(#125933,
#125934,#125935,#125936,#125937)),.UNSPECIFIED.,.F.,.F.,.F.)
B_SPLINE_SURFACE_WITH_KNOTS((2,2),(3,2,3),(0.,0.29040686991619),(0.262499170136658,
0.263098999273795,0.280537087669267),.UNSPECIFIED.)
GEOMETRIC_REPRESENTATION_ITEM()
RATIONAL_B_SPLINE_SURFACE(((0.989150325841653,0.989150325841653,0.989150325841653,
0.991395311444461,0.996628941948308),(0.989150325841653,0.989150325841653,
0.989150325841653,0.991395311444461,0.996628941948308)))
REPRESENTATION_ITEM('')
SURFACE()
);
#1871=(
BOUNDED_SURFACE()
B_SPLINE_SURFACE(1,2,((#125954,#125955,#125956),(#125957,#125958,#125959)),
 .UNSPECIFIED.,.F.,.F.,.F.)
B_SPLINE_SURFACE_WITH_KNOTS((2,2),(3,3),(0.,0.289681084359918),(0.452822299828565,
0.470019760166365),.UNSPECIFIED.)
GEOMETRIC_REPRESENTATION_ITEM()
RATIONAL_B_SPLINE_SURFACE(((0.988755486262821,0.986817927519786,0.987787102172814),
(0.988755486262821,0.986817927519787,0.987787102172814)))
REPRESENTATION_ITEM('')
SURFACE()
);
#1872=(
BOUNDED_SURFACE()
B_SPLINE_SURFACE(1,2,((#125961,#125962,#125963,#125964,#125965),(#125966,
#125967,#125968,#125969,#125970)),.UNSPECIFIED.,.F.,.F.,.F.)
B_SPLINE_SURFACE_WITH_KNOTS((2,2),(3,2,3),(0.,0.290406869902415),(0.262499170150461,
0.263098999273795,0.280537087669267),.UNSPECIFIED.)
GEOMETRIC_REPRESENTATION_ITEM()
RATIONAL_B_SPLINE_SURFACE(((0.989150325841653,0.989150325841653,0.989150325841653,
0.991395311444461,0.996628941948308),(0.989150325841653,0.989150325841653,
0.989150325841653,0.991395311444461,0.996628941948308)))
REPRESENTATION_ITEM('')
SURFACE()
);
#1873=(
BOUNDED_SURFACE()
B_SPLINE_SURFACE(1,2,((#125987,#125988,#125989),(#125990,#125991,#125992)),
 .UNSPECIFIED.,.F.,.F.,.F.)
B_SPLINE_SURFACE_WITH_KNOTS((2,2),(3,3),(0.,0.289681084359927),(0.452822299828565,
0.470019760166365),.UNSPECIFIED.)
GEOMETRIC_REPRESENTATION_ITEM()
RATIONAL_B_SPLINE_SURFACE(((0.988755486262821,0.986817927519786,0.987787102172814),
(0.988755486262821,0.986817927519787,0.987787102172814)))
REPRESENTATION_ITEM('')
SURFACE()
);
#1874=(
BOUNDED_SURFACE()
B_SPLINE_SURFACE(1,2,((#125994,#125995,#125996,#125997,#125998),(#125999,
#126000,#126001,#126002,#126003)),.UNSPECIFIED.,.F.,.F.,.F.)
B_SPLINE_SURFACE_WITH_KNOTS((2,2),(3,2,3),(0.,0.290406869886822),(0.262499170166043,
0.263098999273795,0.280537087669266),.UNSPECIFIED.)
GEOMETRIC_REPRESENTATION_ITEM()
RATIONAL_B_SPLINE_SURFACE(((0.989150325841653,0.989150325841653,0.989150325841653,
0.991395311444461,0.996628941948308),(0.989150325841653,0.989150325841653,
0.989150325841653,0.991395311444461,0.996628941948308)))
REPRESENTATION_ITEM('')
SURFACE()
);
#1875=(
BOUNDED_SURFACE()
B_SPLINE_SURFACE(1,2,((#126020,#126021,#126022),(#126023,#126024,#126025)),
 .UNSPECIFIED.,.F.,.F.,.F.)
B_SPLINE_SURFACE_WITH_KNOTS((2,2),(3,3),(0.,0.289681084359919),(0.452822299828566,
0.470019760166367),.UNSPECIFIED.)
GEOMETRIC_REPRESENTATION_ITEM()
RATIONAL_B_SPLINE_SURFACE(((0.98875548626282,0.986817927519786,0.987787102172814),
(0.98875548626282,0.986817927519786,0.987787102172814)))
REPRESENTATION_ITEM('')
SURFACE()
);
#1876=(
BOUNDED_SURFACE()
B_SPLINE_SURFACE(1,2,((#126027,#126028,#126029,#126030,#126031),(#126032,
#126033,#126034,#126035,#126036)),.UNSPECIFIED.,.F.,.F.,.F.)
B_SPLINE_SURFACE_WITH_KNOTS((2,2),(3,2,3),(0.710318915640084,1.),(0.504616569534327,
0.52191752982614,0.522090539429058),.UNSPECIFIED.)
GEOMETRIC_REPRESENTATION_ITEM()
RATIONAL_B_SPLINE_SURFACE(((0.996968549833597,0.991680746768561,0.989334769731189,
0.989334769731189,0.989334769731189),(0.996968549833597,0.991680746768561,
0.989334769731189,0.989334769731189,0.989334769731189)))
REPRESENTATION_ITEM('')
SURFACE()
);
#1877=(
BOUNDED_SURFACE()
B_SPLINE_SURFACE(1,2,((#126047,#126048,#126049,#126050,#126051),(#126052,
#126053,#126054,#126055,#126056)),.UNSPECIFIED.,.F.,.F.,.F.)
B_SPLINE_SURFACE_WITH_KNOTS((2,2),(3,2,3),(0.710192959008446,1.),(0.211502584834065,
0.214285714285714,0.228987659635175),.UNSPECIFIED.)
GEOMETRIC_REPRESENTATION_ITEM()
RATIONAL_B_SPLINE_SURFACE(((0.998122319569323,0.999023095875705,1.,0.994839481491404,
0.99180331349328),(0.998122319569323,0.999023095875705,1.,0.994839481491404,
0.99180331349328)))
REPRESENTATION_ITEM('')
SURFACE()
);
#1878=(
BOUNDED_SURFACE()
B_SPLINE_SURFACE(1,2,((#126070,#126071,#126072,#126073,#126074),(#126075,
#126076,#126077,#126078,#126079)),.UNSPECIFIED.,.F.,.F.,.F.)
B_SPLINE_SURFACE_WITH_KNOTS((2,2),(3,2,3),(0.709731017409647,1.),(0.504616569534327,
0.52191752982614,0.522505428214631),.UNSPECIFIED.)
GEOMETRIC_REPRESENTATION_ITEM()
RATIONAL_B_SPLINE_SURFACE(((0.996968549833597,0.991680746768561,0.989334769731189,
0.989334769731189,0.989334769731189),(0.996968549833597,0.991680746768561,
0.989334769731189,0.989334769731189,0.989334769731189)))
REPRESENTATION_ITEM('')
SURFACE()
);
#1879=(
BOUNDED_SURFACE()
B_SPLINE_SURFACE(1,2,((#126090,#126091,#126092,#126093,#126094),(#126095,
#126096,#126097,#126098,#126099)),.UNSPECIFIED.,.F.,.F.,.F.)
B_SPLINE_SURFACE_WITH_KNOTS((2,2),(3,2,3),(0.710192959007514,1.),(0.211502584834065,
0.214285714285714,0.228987659635175),.UNSPECIFIED.)
GEOMETRIC_REPRESENTATION_ITEM()
RATIONAL_B_SPLINE_SURFACE(((0.998122319569323,0.999023095875705,1.,0.994839481491404,
0.99180331349328),(0.998122319569323,0.999023095875705,1.,0.994839481491404,
0.99180331349328)))
REPRESENTATION_ITEM('')
SURFACE()
);
#1880=(
BOUNDED_SURFACE()
B_SPLINE_SURFACE(1,2,((#126113,#126114,#126115,#126116,#126117),(#126118,
#126119,#126120,#126121,#126122)),.UNSPECIFIED.,.F.,.F.,.F.)
B_SPLINE_SURFACE_WITH_KNOTS((2,2),(3,2,3),(0.709731017450111,1.),(0.504616569534327,
0.52191752982614,0.522505428174168),.UNSPECIFIED.)
GEOMETRIC_REPRESENTATION_ITEM()
RATIONAL_B_SPLINE_SURFACE(((0.996968549833597,0.991680746768561,0.989334769731189,
0.989334769731189,0.989334769731189),(0.996968549833597,0.991680746768561,
0.989334769731189,0.989334769731189,0.989334769731189)))
REPRESENTATION_ITEM('')
SURFACE()
);
#1881=(
BOUNDED_SURFACE()
B_SPLINE_SURFACE(1,2,((#126133,#126134,#126135,#126136,#126137),(#126138,
#126139,#126140,#126141,#126142)),.UNSPECIFIED.,.F.,.F.,.F.)
B_SPLINE_SURFACE_WITH_KNOTS((2,2),(3,2,3),(0.710192959007509,1.),(0.211502584834065,
0.214285714285714,0.228987659635175),.UNSPECIFIED.)
GEOMETRIC_REPRESENTATION_ITEM()
RATIONAL_B_SPLINE_SURFACE(((0.998122319569323,0.999023095875705,1.,0.994839481491404,
0.99180331349328),(0.998122319569323,0.999023095875705,1.,0.994839481491404,
0.99180331349328)))
REPRESENTATION_ITEM('')
SURFACE()
);
#1882=(
BOUNDED_SURFACE()
B_SPLINE_SURFACE(1,2,((#126156,#126157,#126158,#126159,#126160),(#126161,
#126162,#126163,#126164,#126165)),.UNSPECIFIED.,.F.,.F.,.F.)
B_SPLINE_SURFACE_WITH_KNOTS((2,2),(3,2,3),(0.709731017378141,1.),(0.504616569534327,
0.52191752982614,0.522505428246138),.UNSPECIFIED.)
GEOMETRIC_REPRESENTATION_ITEM()
RATIONAL_B_SPLINE_SURFACE(((0.996968549833598,0.991680746768561,0.989334769731189,
0.989334769731189,0.989334769731189),(0.996968549833598,0.991680746768561,
0.989334769731189,0.989334769731189,0.989334769731189)))
REPRESENTATION_ITEM('')
SURFACE()
);
#1883=(
BOUNDED_SURFACE()
B_SPLINE_SURFACE(1,2,((#126176,#126177,#126178,#126179,#126180),(#126181,
#126182,#126183,#126184,#126185)),.UNSPECIFIED.,.F.,.F.,.F.)
B_SPLINE_SURFACE_WITH_KNOTS((2,2),(3,2,3),(0.710192959007511,1.),(0.211502584834065,
0.214285714285714,0.228987659635175),.UNSPECIFIED.)
GEOMETRIC_REPRESENTATION_ITEM()
RATIONAL_B_SPLINE_SURFACE(((0.998122319569323,0.999023095875705,1.,0.994839481491404,
0.99180331349328),(0.998122319569323,0.999023095875705,1.,0.994839481491404,
0.99180331349328)))
REPRESENTATION_ITEM('')
SURFACE()
);
#1884=(
BOUNDED_SURFACE()
B_SPLINE_SURFACE(1,2,((#126199,#126200,#126201,#126202,#126203),(#126204,
#126205,#126206,#126207,#126208)),.UNSPECIFIED.,.F.,.F.,.F.)
B_SPLINE_SURFACE_WITH_KNOTS((2,2),(3,2,3),(0.709731017387927,1.),(0.504616569534327,
0.52191752982614,0.522505428181681),.UNSPECIFIED.)
GEOMETRIC_REPRESENTATION_ITEM()
RATIONAL_B_SPLINE_SURFACE(((0.996968549833597,0.991680746768561,0.989334769731189,
0.989334769731189,0.989334769731189),(0.996968549833597,0.991680746768561,
0.989334769731189,0.989334769731189,0.989334769731189)))
REPRESENTATION_ITEM('')
SURFACE()
);
#1885=(
BOUNDED_SURFACE()
B_SPLINE_SURFACE(1,2,((#126219,#126220,#126221,#126222,#126223),(#126224,
#126225,#126226,#126227,#126228)),.UNSPECIFIED.,.F.,.F.,.F.)
B_SPLINE_SURFACE_WITH_KNOTS((2,2),(3,2,3),(0.710192959006926,1.),(0.211502584834065,
0.214285714285714,0.228987659635175),.UNSPECIFIED.)
GEOMETRIC_REPRESENTATION_ITEM()
RATIONAL_B_SPLINE_SURFACE(((0.998122319569323,0.999023095875705,1.,0.994839481491404,
0.991803313493279),(0.998122319569323,0.999023095875705,1.,0.994839481491404,
0.991803313493279)))
REPRESENTATION_ITEM('')
SURFACE()
);
#1886=(
BOUNDED_SURFACE()
B_SPLINE_SURFACE(1,2,((#126242,#126243,#126244,#126245,#126246),(#126247,
#126248,#126249,#126250,#126251)),.UNSPECIFIED.,.F.,.F.,.F.)
B_SPLINE_SURFACE_WITH_KNOTS((2,2),(3,2,3),(0.710318915639154,1.),(0.504616569534327,
0.52191752982614,0.522090539429058),.UNSPECIFIED.)
GEOMETRIC_REPRESENTATION_ITEM()
RATIONAL_B_SPLINE_SURFACE(((0.996968549833597,0.991680746768561,0.989334769731189,
0.989334769731189,0.989334769731189),(0.996968549833597,0.991680746768561,
0.989334769731189,0.989334769731189,0.989334769731189)))
REPRESENTATION_ITEM('')
SURFACE()
);
#1887=(
BOUNDED_SURFACE()
B_SPLINE_SURFACE(1,2,((#126262,#126263,#126264,#126265,#126266),(#126267,
#126268,#126269,#126270,#126271)),.UNSPECIFIED.,.F.,.F.,.F.)
B_SPLINE_SURFACE_WITH_KNOTS((2,2),(3,2,3),(0.710192959007513,1.),(0.211502584834065,
0.214285714285714,0.228987659635175),.UNSPECIFIED.)
GEOMETRIC_REPRESENTATION_ITEM()
RATIONAL_B_SPLINE_SURFACE(((0.998122319569323,0.999023095875705,1.,0.994839481491404,
0.991803313493279),(0.998122319569323,0.999023095875705,1.,0.994839481491404,
0.991803313493279)))
REPRESENTATION_ITEM('')
SURFACE()
);
#1888=(
BOUNDED_SURFACE()
B_SPLINE_SURFACE(1,2,((#126285,#126286,#126287,#126288,#126289),(#126290,
#126291,#126292,#126293,#126294)),.UNSPECIFIED.,.F.,.F.,.F.)
B_SPLINE_SURFACE_WITH_KNOTS((2,2),(3,2,3),(0.709731017354647,1.),(0.504616569534327,
0.52191752982614,0.522505428214449),.UNSPECIFIED.)
GEOMETRIC_REPRESENTATION_ITEM()
RATIONAL_B_SPLINE_SURFACE(((0.996968549833597,0.991680746768561,0.989334769731189,
0.989334769731189,0.989334769731189),(0.996968549833597,0.991680746768561,
0.989334769731189,0.989334769731189,0.989334769731189)))
REPRESENTATION_ITEM('')
SURFACE()
);
#1889=(
BOUNDED_SURFACE()
B_SPLINE_SURFACE(1,2,((#126305,#126306,#126307,#126308,#126309),(#126310,
#126311,#126312,#126313,#126314)),.UNSPECIFIED.,.F.,.F.,.F.)
B_SPLINE_SURFACE_WITH_KNOTS((2,2),(3,2,3),(0.710192959006931,1.),(0.211502584834065,
0.214285714285714,0.228987659635175),.UNSPECIFIED.)
GEOMETRIC_REPRESENTATION_ITEM()
RATIONAL_B_SPLINE_SURFACE(((0.998122319569323,0.999023095875705,1.,0.994839481491404,
0.99180331349328),(0.998122319569323,0.999023095875705,1.,0.994839481491404,
0.99180331349328)))
REPRESENTATION_ITEM('')
SURFACE()
);
#1890=(
BOUNDED_SURFACE()
B_SPLINE_SURFACE(1,2,((#126328,#126329,#126330,#126331,#126332),(#126333,
#126334,#126335,#126336,#126337)),.UNSPECIFIED.,.F.,.F.,.F.)
B_SPLINE_SURFACE_WITH_KNOTS((2,2),(3,2,3),(0.710318915639071,1.),(0.504616569534328,
0.52191752982614,0.522090539429058),.UNSPECIFIED.)
GEOMETRIC_REPRESENTATION_ITEM()
RATIONAL_B_SPLINE_SURFACE(((0.996968549833597,0.991680746768561,0.989334769731189,
0.989334769731189,0.989334769731189),(0.996968549833597,0.991680746768561,
0.989334769731189,0.989334769731189,0.989334769731189)))
REPRESENTATION_ITEM('')
SURFACE()
);
#1891=(
BOUNDED_SURFACE()
B_SPLINE_SURFACE(1,2,((#126348,#126349,#126350,#126351,#126352),(#126353,
#126354,#126355,#126356,#126357)),.UNSPECIFIED.,.F.,.F.,.F.)
B_SPLINE_SURFACE_WITH_KNOTS((2,2),(3,2,3),(0.710192959007428,1.),(0.211502584834064,
0.214285714285714,0.228987659635174),.UNSPECIFIED.)
GEOMETRIC_REPRESENTATION_ITEM()
RATIONAL_B_SPLINE_SURFACE(((0.998122319569322,0.999023095875704,1.,0.994839481491404,
0.99180331349328),(0.998122319569322,0.999023095875704,1.,0.994839481491405,
0.99180331349328)))
REPRESENTATION_ITEM('')
SURFACE()
);
#1892=(
BOUNDED_SURFACE()
B_SPLINE_SURFACE(1,2,((#126371,#126372,#126373,#126374,#126375),(#126376,
#126377,#126378,#126379,#126380)),.UNSPECIFIED.,.F.,.F.,.F.)
B_SPLINE_SURFACE_WITH_KNOTS((2,2),(3,2,3),(0.709731017404435,1.),(0.504616569534328,
0.521917529826141,0.522505428219767),.UNSPECIFIED.)
GEOMETRIC_REPRESENTATION_ITEM()
RATIONAL_B_SPLINE_SURFACE(((0.996968549833597,0.991680746768561,0.989334769731189,
0.989334769731189,0.989334769731189),(0.996968549833597,0.991680746768561,
0.989334769731189,0.989334769731189,0.989334769731189)))
REPRESENTATION_ITEM('')
SURFACE()
);
#1893=(
BOUNDED_SURFACE()
B_SPLINE_SURFACE(1,2,((#126391,#126392,#126393,#126394,#126395),(#126396,
#126397,#126398,#126399,#126400)),.UNSPECIFIED.,.F.,.F.,.F.)
B_SPLINE_SURFACE_WITH_KNOTS((2,2),(3,2,3),(0.710192959007438,1.),(0.211502584834064,
0.214285714285714,0.228987659635174),.UNSPECIFIED.)
GEOMETRIC_REPRESENTATION_ITEM()
RATIONAL_B_SPLINE_SURFACE(((0.998122319569322,0.999023095875704,1.,0.994839481491405,
0.99180331349328),(0.998122319569322,0.999023095875704,1.,0.994839481491405,
0.99180331349328)))
REPRESENTATION_ITEM('')
SURFACE()
);
#1894=(
BOUNDED_SURFACE()
B_SPLINE_SURFACE(1,2,((#126414,#126415,#126416,#126417,#126418),(#126419,
#126420,#126421,#126422,#126423)),.UNSPECIFIED.,.F.,.F.,.F.)
B_SPLINE_SURFACE_WITH_KNOTS((2,2),(3,2,3),(0.709731017441998,1.),(0.504616569534328,
0.521917529826141,0.522505428181611),.UNSPECIFIED.)
GEOMETRIC_REPRESENTATION_ITEM()
RATIONAL_B_SPLINE_SURFACE(((0.996968549833597,0.99168074676856,0.989334769731189,
0.989334769731189,0.989334769731189),(0.996968549833597,0.99168074676856,
0.989334769731189,0.989334769731189,0.989334769731189)))
REPRESENTATION_ITEM('')
SURFACE()
);
#1895=(
BOUNDED_SURFACE()
B_SPLINE_SURFACE(1,2,((#126434,#126435,#126436,#126437,#126438),(#126439,
#126440,#126441,#126442,#126443)),.UNSPECIFIED.,.F.,.F.,.F.)
B_SPLINE_SURFACE_WITH_KNOTS((2,2),(3,2,3),(0.710192959006837,1.),(0.211502584834064,
0.214285714285714,0.228987659635174),.UNSPECIFIED.)
GEOMETRIC_REPRESENTATION_ITEM()
RATIONAL_B_SPLINE_SURFACE(((0.998122319569322,0.999023095875704,1.,0.994839481491405,
0.99180331349328),(0.998122319569322,0.999023095875704,1.,0.994839481491405,
0.99180331349328)))
REPRESENTATION_ITEM('')
SURFACE()
);
#1896=(
BOUNDED_SURFACE()
B_SPLINE_SURFACE(1,2,((#126457,#126458,#126459,#126460,#126461),(#126462,
#126463,#126464,#126465,#126466)),.UNSPECIFIED.,.F.,.F.,.F.)
B_SPLINE_SURFACE_WITH_KNOTS((2,2),(3,2,3),(0.709731017396997,1.),(0.504616569534328,
0.521917529826141,0.522505428227195),.UNSPECIFIED.)
GEOMETRIC_REPRESENTATION_ITEM()
RATIONAL_B_SPLINE_SURFACE(((0.996968549833597,0.991680746768561,0.989334769731189,
0.989334769731189,0.989334769731189),(0.996968549833597,0.991680746768561,
0.989334769731189,0.989334769731189,0.989334769731189)))
REPRESENTATION_ITEM('')
SURFACE()
);
#1897=(
BOUNDED_SURFACE()
B_SPLINE_SURFACE(1,2,((#126477,#126478,#126479,#126480,#126481),(#126482,
#126483,#126484,#126485,#126486)),.UNSPECIFIED.,.F.,.F.,.F.)
B_SPLINE_SURFACE_WITH_KNOTS((2,2),(3,2,3),(0.710192959007424,1.),(0.211502584834064,
0.214285714285714,0.228987659635174),.UNSPECIFIED.)
GEOMETRIC_REPRESENTATION_ITEM()
RATIONAL_B_SPLINE_SURFACE(((0.998122319569322,0.999023095875704,1.,0.994839481491405,
0.99180331349328),(0.998122319569322,0.999023095875704,1.,0.994839481491405,
0.99180331349328)))
REPRESENTATION_ITEM('')
SURFACE()
);
#1898=(
BOUNDED_SURFACE()
B_SPLINE_SURFACE(1,2,((#126500,#126501,#126502,#126503,#126504),(#126505,
#126506,#126507,#126508,#126509)),.UNSPECIFIED.,.F.,.F.,.F.)
B_SPLINE_SURFACE_WITH_KNOTS((2,2),(3,2,3),(0.709731017376469,1.),(0.504616569534328,
0.521917529826141,0.522505428193485),.UNSPECIFIED.)
GEOMETRIC_REPRESENTATION_ITEM()
RATIONAL_B_SPLINE_SURFACE(((0.996968549833597,0.99168074676856,0.989334769731189,
0.989334769731189,0.989334769731189),(0.996968549833597,0.99168074676856,
0.989334769731189,0.989334769731189,0.989334769731189)))
REPRESENTATION_ITEM('')
SURFACE()
);
#1899=(
BOUNDED_SURFACE()
B_SPLINE_SURFACE(1,2,((#126520,#126521,#126522,#126523,#126524),(#126525,
#126526,#126527,#126528,#126529)),.UNSPECIFIED.,.F.,.F.,.F.)
B_SPLINE_SURFACE_WITH_KNOTS((2,2),(3,2,3),(0.710192959006924,1.),(0.211502584834064,
0.214285714285714,0.228987659635174),.UNSPECIFIED.)
GEOMETRIC_REPRESENTATION_ITEM()
RATIONAL_B_SPLINE_SURFACE(((0.998122319569322,0.999023095875704,1.,0.994839481491405,
0.99180331349328),(0.998122319569322,0.999023095875704,1.,0.994839481491405,
0.99180331349328)))
REPRESENTATION_ITEM('')
SURFACE()
);
#1900=(
BOUNDED_SURFACE()
B_SPLINE_SURFACE(1,2,((#126543,#126544,#126545,#126546,#126547),(#126548,
#126549,#126550,#126551,#126552)),.UNSPECIFIED.,.F.,.F.,.F.)
B_SPLINE_SURFACE_WITH_KNOTS((2,2),(3,2,3),(0.709731017436248,1.),(0.504616569534328,
0.521917529826141,0.522505428187947),.UNSPECIFIED.)
GEOMETRIC_REPRESENTATION_ITEM()
RATIONAL_B_SPLINE_SURFACE(((0.996968549833597,0.99168074676856,0.989334769731189,
0.989334769731189,0.989334769731189),(0.996968549833597,0.99168074676856,
0.989334769731189,0.989334769731189,0.989334769731189)))
REPRESENTATION_ITEM('')
SURFACE()
);
#1901=(
BOUNDED_SURFACE()
B_SPLINE_SURFACE(1,2,((#126563,#126564,#126565,#126566,#126567),(#126568,
#126569,#126570,#126571,#126572)),.UNSPECIFIED.,.F.,.F.,.F.)
B_SPLINE_SURFACE_WITH_KNOTS((2,2),(3,2,3),(0.710192959007417,1.),(0.211502584834064,
0.214285714285714,0.228987659635174),.UNSPECIFIED.)
GEOMETRIC_REPRESENTATION_ITEM()
RATIONAL_B_SPLINE_SURFACE(((0.998122319569322,0.999023095875704,1.,0.994839481491405,
0.99180331349328),(0.998122319569322,0.999023095875704,1.,0.994839481491405,
0.99180331349328)))
REPRESENTATION_ITEM('')
SURFACE()
);
#1902=(
BOUNDED_SURFACE()
B_SPLINE_SURFACE(1,2,((#126586,#126587,#126588,#126589,#126590),(#126591,
#126592,#126593,#126594,#126595)),.UNSPECIFIED.,.F.,.F.,.F.)
B_SPLINE_SURFACE_WITH_KNOTS((2,2),(3,2,3),(0.710318915638563,1.),(0.504616569534328,
0.521917529826141,0.522090539429059),.UNSPECIFIED.)
GEOMETRIC_REPRESENTATION_ITEM()
RATIONAL_B_SPLINE_SURFACE(((0.996968549833597,0.991680746768561,0.989334769731189,
0.989334769731189,0.989334769731189),(0.996968549833597,0.991680746768561,
0.989334769731189,0.989334769731189,0.989334769731189)))
REPRESENTATION_ITEM('')
SURFACE()
);
#1903=(
BOUNDED_SURFACE()
B_SPLINE_SURFACE(1,2,((#126606,#126607,#126608,#126609,#126610),(#126611,
#126612,#126613,#126614,#126615)),.UNSPECIFIED.,.F.,.F.,.F.)
B_SPLINE_SURFACE_WITH_KNOTS((2,2),(3,2,3),(0.710192959006919,1.),(0.211502584834064,
0.214285714285714,0.228987659635174),.UNSPECIFIED.)
GEOMETRIC_REPRESENTATION_ITEM()
RATIONAL_B_SPLINE_SURFACE(((0.998122319569322,0.999023095875704,1.,0.994839481491405,
0.99180331349328),(0.998122319569322,0.999023095875704,1.,0.994839481491405,
0.99180331349328)))
REPRESENTATION_ITEM('')
SURFACE()
);
#1904=(
BOUNDED_SURFACE()
B_SPLINE_SURFACE(1,2,((#126629,#126630,#126631,#126632,#126633),(#126634,
#126635,#126636,#126637,#126638)),.UNSPECIFIED.,.F.,.F.,.F.)
B_SPLINE_SURFACE_WITH_KNOTS((2,2),(3,2,3),(0.710318915638789,1.),(0.504616569534328,
0.521917529826141,0.522090539429059),.UNSPECIFIED.)
GEOMETRIC_REPRESENTATION_ITEM()
RATIONAL_B_SPLINE_SURFACE(((0.996968549833597,0.991680746768561,0.989334769731189,
0.989334769731189,0.989334769731189),(0.996968549833597,0.991680746768561,
0.989334769731189,0.989334769731189,0.989334769731189)))
REPRESENTATION_ITEM('')
SURFACE()
);
#1905=(
BOUNDED_SURFACE()
B_SPLINE_SURFACE(1,2,((#126649,#126650,#126651,#126652,#126653),(#126654,
#126655,#126656,#126657,#126658)),.UNSPECIFIED.,.F.,.F.,.F.)
B_SPLINE_SURFACE_WITH_KNOTS((2,2),(3,2,3),(0.710192959007146,1.),(0.211502584834064,
0.214285714285714,0.228987659635174),.UNSPECIFIED.)
GEOMETRIC_REPRESENTATION_ITEM()
RATIONAL_B_SPLINE_SURFACE(((0.998122319569322,0.999023095875704,1.,0.994839481491405,
0.99180331349328),(0.998122319569322,0.999023095875704,1.,0.994839481491405,
0.99180331349328)))
REPRESENTATION_ITEM('')
SURFACE()
);
#1906=(
BOUNDED_SURFACE()
B_SPLINE_SURFACE(1,2,((#126672,#126673,#126674,#126675,#126676),(#126677,
#126678,#126679,#126680,#126681)),.UNSPECIFIED.,.F.,.F.,.F.)
B_SPLINE_SURFACE_WITH_KNOTS((2,2),(3,2,3),(0.709731017416746,1.),(0.504616569534328,
0.521917529826141,0.522505428206132),.UNSPECIFIED.)
GEOMETRIC_REPRESENTATION_ITEM()
RATIONAL_B_SPLINE_SURFACE(((0.996968549833597,0.99168074676856,0.989334769731189,
0.989334769731189,0.989334769731189),(0.996968549833597,0.99168074676856,
0.989334769731189,0.989334769731189,0.989334769731189)))
REPRESENTATION_ITEM('')
SURFACE()
);
#1907=(
BOUNDED_SURFACE()
B_SPLINE_SURFACE(1,2,((#126692,#126693,#126694,#126695,#126696),(#126697,
#126698,#126699,#126700,#126701)),.UNSPECIFIED.,.F.,.F.,.F.)
B_SPLINE_SURFACE_WITH_KNOTS((2,2),(3,2,3),(0.710192959006101,1.),(0.211502584834064,
0.214285714285714,0.228987659635174),.UNSPECIFIED.)
GEOMETRIC_REPRESENTATION_ITEM()
RATIONAL_B_SPLINE_SURFACE(((0.998122319569322,0.999023095875704,1.,0.994839481491405,
0.99180331349328),(0.998122319569322,0.999023095875704,1.,0.994839481491405,
0.99180331349328)))
REPRESENTATION_ITEM('')
SURFACE()
);
#1908=(
BOUNDED_SURFACE()
B_SPLINE_SURFACE(1,2,((#126715,#126716,#126717,#126718,#126719),(#126720,
#126721,#126722,#126723,#126724)),.UNSPECIFIED.,.F.,.F.,.F.)
B_SPLINE_SURFACE_WITH_KNOTS((2,2),(3,2,3),(0.709731017422478,1.),(0.504616569534328,
0.521917529826141,0.522505428201685),.UNSPECIFIED.)
GEOMETRIC_REPRESENTATION_ITEM()
RATIONAL_B_SPLINE_SURFACE(((0.996968549833597,0.991680746768561,0.989334769731189,
0.989334769731189,0.989334769731189),(0.996968549833597,0.99168074676856,
0.989334769731189,0.989334769731189,0.989334769731189)))
REPRESENTATION_ITEM('')
SURFACE()
);
#1909=(
BOUNDED_SURFACE()
B_SPLINE_SURFACE(1,2,((#126735,#126736,#126737,#126738,#126739),(#126740,
#126741,#126742,#126743,#126744)),.UNSPECIFIED.,.F.,.F.,.F.)
B_SPLINE_SURFACE_WITH_KNOTS((2,2),(3,2,3),(0.710192959007388,1.),(0.211502584834062,
0.214285714285714,0.228987659635174),.UNSPECIFIED.)
GEOMETRIC_REPRESENTATION_ITEM()
RATIONAL_B_SPLINE_SURFACE(((0.998122319569321,0.999023095875703,1.,0.994839481491405,
0.99180331349328),(0.998122319569321,0.999023095875703,1.,0.994839481491405,
0.99180331349328)))
REPRESENTATION_ITEM('')
SURFACE()
);
#1910=(
BOUNDED_SURFACE()
B_SPLINE_SURFACE(1,2,((#126758,#126759,#126760,#126761,#126762),(#126763,
#126764,#126765,#126766,#126767)),.UNSPECIFIED.,.F.,.F.,.F.)
B_SPLINE_SURFACE_WITH_KNOTS((2,2),(3,2,3),(0.709731017390974,1.),(0.504616569534328,
0.521917529826141,0.522505428233296),.UNSPECIFIED.)
GEOMETRIC_REPRESENTATION_ITEM()
RATIONAL_B_SPLINE_SURFACE(((0.996968549833597,0.991680746768561,0.989334769731189,
0.989334769731189,0.989334769731189),(0.996968549833597,0.991680746768561,
0.989334769731189,0.989334769731189,0.989334769731189)))
REPRESENTATION_ITEM('')
SURFACE()
);
#1911=(
BOUNDED_SURFACE()
B_SPLINE_SURFACE(1,2,((#126778,#126779,#126780,#126781,#126782),(#126783,
#126784,#126785,#126786,#126787)),.UNSPECIFIED.,.F.,.F.,.F.)
B_SPLINE_SURFACE_WITH_KNOTS((2,2),(3,2,3),(0.710192959007501,1.),(0.211502584834064,
0.214285714285714,0.228987659635174),.UNSPECIFIED.)
GEOMETRIC_REPRESENTATION_ITEM()
RATIONAL_B_SPLINE_SURFACE(((0.998122319569322,0.999023095875704,1.,0.994839481491405,
0.99180331349328),(0.998122319569322,0.999023095875704,1.,0.994839481491405,
0.99180331349328)))
REPRESENTATION_ITEM('')
SURFACE()
);
#1912=(
BOUNDED_SURFACE()
B_SPLINE_SURFACE(1,2,((#126801,#126802,#126803,#126804,#126805),(#126806,
#126807,#126808,#126809,#126810)),.UNSPECIFIED.,.F.,.F.,.F.)
B_SPLINE_SURFACE_WITH_KNOTS((2,2),(3,2,3),(0.710318915638503,1.),(0.504616569534054,
0.521917529826142,0.522090539429063),.UNSPECIFIED.)
GEOMETRIC_REPRESENTATION_ITEM()
RATIONAL_B_SPLINE_SURFACE(((0.996968549833764,0.991680746768598,0.989334769731189,
0.989334769731189,0.989334769731189),(0.996968549833764,0.991680746768598,
0.989334769731189,0.989334769731189,0.989334769731189)))
REPRESENTATION_ITEM('')
SURFACE()
);
#1913=(
BOUNDED_SURFACE()
B_SPLINE_SURFACE(1,2,((#126821,#126822,#126823,#126824,#126825),(#126826,
#126827,#126828,#126829,#126830)),.UNSPECIFIED.,.F.,.F.,.F.)
B_SPLINE_SURFACE_WITH_KNOTS((2,2),(3,2,3),(0.710192959006864,1.),(0.211502584834064,
0.214285714285714,0.228987659635173),.UNSPECIFIED.)
GEOMETRIC_REPRESENTATION_ITEM()
RATIONAL_B_SPLINE_SURFACE(((0.998122319569322,0.999023095875704,1.,0.994839481491405,
0.99180331349328),(0.998122319569322,0.999023095875704,1.,0.994839481491405,
0.99180331349328)))
REPRESENTATION_ITEM('')
SURFACE()
);
#1914=(
BOUNDED_SURFACE()
B_SPLINE_SURFACE(1,2,((#126844,#126845,#126846,#126847,#126848),(#126849,
#126850,#126851,#126852,#126853)),.UNSPECIFIED.,.F.,.F.,.F.)
B_SPLINE_SURFACE_WITH_KNOTS((2,2),(3,2,3),(0.709731017406796,1.),(0.504616569534173,
0.521917529826141,0.522505428218247),.UNSPECIFIED.)
GEOMETRIC_REPRESENTATION_ITEM()
RATIONAL_B_SPLINE_SURFACE(((0.996968549833692,0.991680746768582,0.989334769731189,
0.989334769731189,0.989334769731189),(0.996968549833692,0.991680746768582,
0.989334769731189,0.989334769731189,0.989334769731189)))
REPRESENTATION_ITEM('')
SURFACE()
);
#1915=(
BOUNDED_SURFACE()
B_SPLINE_SURFACE(1,2,((#126864,#126865,#126866,#126867,#126868),(#126869,
#126870,#126871,#126872,#126873)),.UNSPECIFIED.,.F.,.F.,.F.)
B_SPLINE_SURFACE_WITH_KNOTS((2,2),(3,2,3),(0.710192959008269,1.),(0.211502584834063,
0.214285714285714,0.228987659635173),.UNSPECIFIED.)
GEOMETRIC_REPRESENTATION_ITEM()
RATIONAL_B_SPLINE_SURFACE(((0.998122319569321,0.999023095875704,1.,0.994839481491405,
0.99180331349328),(0.998122319569321,0.999023095875704,1.,0.994839481491405,
0.99180331349328)))
REPRESENTATION_ITEM('')
SURFACE()
);
#1916=(
BOUNDED_SURFACE()
B_SPLINE_SURFACE(1,2,((#126887,#126888,#126889,#126890,#126891),(#126892,
#126893,#126894,#126895,#126896)),.UNSPECIFIED.,.F.,.F.,.F.)
B_SPLINE_SURFACE_WITH_KNOTS((2,2),(3,2,3),(0.710318915638758,1.),(0.504616569533916,
0.521917529826141,0.522090539429063),.UNSPECIFIED.)
GEOMETRIC_REPRESENTATION_ITEM()
RATIONAL_B_SPLINE_SURFACE(((0.996968549833849,0.991680746768616,0.989334769731189,
0.989334769731189,0.989334769731189),(0.996968549833849,0.991680746768616,
0.989334769731189,0.989334769731189,0.989334769731189)))
REPRESENTATION_ITEM('')
SURFACE()
);
#1917=(
BOUNDED_SURFACE()
B_SPLINE_SURFACE(1,2,((#126907,#126908,#126909,#126910,#126911),(#126912,
#126913,#126914,#126915,#126916)),.UNSPECIFIED.,.F.,.F.,.F.)
B_SPLINE_SURFACE_WITH_KNOTS((2,2),(3,2,3),(0.710192959007119,1.),(0.21150258483406,
0.214285714285714,0.228987659635174),.UNSPECIFIED.)
GEOMETRIC_REPRESENTATION_ITEM()
RATIONAL_B_SPLINE_SURFACE(((0.998122319569319,0.999023095875703,1.,0.994839481491405,
0.99180331349328),(0.998122319569319,0.999023095875703,1.,0.994839481491405,
0.99180331349328)))
REPRESENTATION_ITEM('')
SURFACE()
);
#1918=(
BOUNDED_SURFACE()
B_SPLINE_SURFACE(1,2,((#126930,#126931,#126932,#126933,#126934),(#126935,
#126936,#126937,#126938,#126939)),.UNSPECIFIED.,.F.,.F.,.F.)
B_SPLINE_SURFACE_WITH_KNOTS((2,2),(3,2,3),(0.710053410952874,1.),(0.504616569534023,
0.521917529826142,0.522183034673918),.UNSPECIFIED.)
GEOMETRIC_REPRESENTATION_ITEM()
RATIONAL_B_SPLINE_SURFACE(((0.996968549833783,0.991680746768602,0.989334769731188,
0.989334769731188,0.989334769731188),(0.996968549833783,0.991680746768602,
0.989334769731188,0.989334769731188,0.989334769731188)))
REPRESENTATION_ITEM('')
SURFACE()
);
#1919=(
BOUNDED_SURFACE()
B_SPLINE_SURFACE(1,2,((#126947,#126948,#126949,#126950,#126951),(#126952,
#126953,#126954,#126955,#126956)),.UNSPECIFIED.,.F.,.F.,.F.)
B_SPLINE_SURFACE_WITH_KNOTS((2,2),(3,2,3),(0.710192959007306,1.),(0.211502584834064,
0.214285714285714,0.228987659635173),.UNSPECIFIED.)
GEOMETRIC_REPRESENTATION_ITEM()
RATIONAL_B_SPLINE_SURFACE(((0.998122319569322,0.999023095875704,1.,0.994839481491405,
0.99180331349328),(0.998122319569322,0.999023095875704,1.,0.994839481491405,
0.99180331349328)))
REPRESENTATION_ITEM('')
SURFACE()
);
#1920=(
BOUNDED_SURFACE()
B_SPLINE_SURFACE(1,2,((#126958,#126959,#126960,#126961,#126962),(#126963,
#126964,#126965,#126966,#126967)),.UNSPECIFIED.,.F.,.F.,.F.)
B_SPLINE_SURFACE_WITH_KNOTS((2,2),(3,2,3),(0.709731017417456,1.),(0.504616569533889,
0.521917529826142,0.522505428205581),.UNSPECIFIED.)
GEOMETRIC_REPRESENTATION_ITEM()
RATIONAL_B_SPLINE_SURFACE(((0.996968549833865,0.99168074676862,0.989334769731189,
0.989334769731189,0.989334769731189),(0.996968549833865,0.99168074676862,
0.989334769731189,0.989334769731189,0.989334769731189)))
REPRESENTATION_ITEM('')
SURFACE()
);
#1921=(
BOUNDED_SURFACE()
B_SPLINE_SURFACE(1,2,((#126978,#126979,#126980,#126981,#126982),(#126983,
#126984,#126985,#126986,#126987)),.UNSPECIFIED.,.F.,.F.,.F.)
B_SPLINE_SURFACE_WITH_KNOTS((2,2),(3,2,3),(0.710192959006265,1.),(0.211502584834064,
0.214285714285714,0.228987659635021),.UNSPECIFIED.)
GEOMETRIC_REPRESENTATION_ITEM()
RATIONAL_B_SPLINE_SURFACE(((0.998122319569322,0.999023095875704,1.,0.994839481491458,
0.991803313493343),(0.998122319569322,0.999023095875704,1.,0.994839481491458,
0.991803313493343)))
REPRESENTATION_ITEM('')
SURFACE()
);
#1922=(
BOUNDED_SURFACE()
B_SPLINE_SURFACE(1,2,((#127001,#127002,#127003,#127004,#127005),(#127006,
#127007,#127008,#127009,#127010)),.UNSPECIFIED.,.F.,.F.,.F.)
B_SPLINE_SURFACE_WITH_KNOTS((2,2),(3,2,3),(0.709731017421646,1.),(0.504616569534085,
0.521917529826141,0.522505428203218),.UNSPECIFIED.)
GEOMETRIC_REPRESENTATION_ITEM()
RATIONAL_B_SPLINE_SURFACE(((0.996968549833745,0.991680746768594,0.989334769731189,
0.989334769731189,0.989334769731189),(0.996968549833745,0.991680746768594,
0.989334769731189,0.989334769731189,0.989334769731189)))
REPRESENTATION_ITEM('')
SURFACE()
);
#1923=(
BOUNDED_SURFACE()
B_SPLINE_SURFACE(1,2,((#127021,#127022,#127023,#127024,#127025),(#127026,
#127027,#127028,#127029,#127030)),.UNSPECIFIED.,.F.,.F.,.F.)
B_SPLINE_SURFACE_WITH_KNOTS((2,2),(3,2,3),(0.710192959008099,1.),(0.211502584834064,
0.214285714285714,0.228987659635071),.UNSPECIFIED.)
GEOMETRIC_REPRESENTATION_ITEM()
RATIONAL_B_SPLINE_SURFACE(((0.998122319569322,0.999023095875704,1.,0.994839481491441,
0.991803313493322),(0.998122319569322,0.999023095875704,1.,0.994839481491441,
0.991803313493322)))
REPRESENTATION_ITEM('')
SURFACE()
);
#1924=(
BOUNDED_SURFACE()
B_SPLINE_SURFACE(1,2,((#127044,#127045,#127046,#127047,#127048),(#127049,
#127050,#127051,#127052,#127053)),.UNSPECIFIED.,.F.,.F.,.F.)
B_SPLINE_SURFACE_WITH_KNOTS((2,2),(3,2,3),(0.709731017417918,1.),(0.504616569534229,
0.521917529826141,0.522505428205796),.UNSPECIFIED.)
GEOMETRIC_REPRESENTATION_ITEM()
RATIONAL_B_SPLINE_SURFACE(((0.996968549833657,0.991680746768574,0.989334769731189,
0.989334769731189,0.989334769731189),(0.996968549833657,0.991680746768574,
0.989334769731189,0.989334769731189,0.989334769731189)))
REPRESENTATION_ITEM('')
SURFACE()
);
#1925=(
BOUNDED_SURFACE()
B_SPLINE_SURFACE(1,2,((#127064,#127065,#127066,#127067,#127068),(#127069,
#127070,#127071,#127072,#127073)),.UNSPECIFIED.,.F.,.F.,.F.)
B_SPLINE_SURFACE_WITH_KNOTS((2,2),(3,2,3),(0.710192959006948,1.),(0.211502584834064,
0.214285714285714,0.228987659635144),.UNSPECIFIED.)
GEOMETRIC_REPRESENTATION_ITEM()
RATIONAL_B_SPLINE_SURFACE(((0.998122319569322,0.999023095875704,1.,0.994839481491415,
0.991803313493292),(0.998122319569322,0.999023095875704,1.,0.994839481491415,
0.991803313493292)))
REPRESENTATION_ITEM('')
SURFACE()
);
#1926=(
BOUNDED_SURFACE()
B_SPLINE_SURFACE(1,2,((#127087,#127088,#127089,#127090,#127091),(#127092,
#127093,#127094,#127095,#127096)),.UNSPECIFIED.,.F.,.F.,.F.)
B_SPLINE_SURFACE_WITH_KNOTS((2,2),(3,2,3),(0.709731017397925,1.),(0.504616569534201,
0.521917529826141,0.522505428226044),.UNSPECIFIED.)
GEOMETRIC_REPRESENTATION_ITEM()
RATIONAL_B_SPLINE_SURFACE(((0.996968549833674,0.991680746768578,0.989334769731189,
0.989334769731189,0.989334769731189),(0.996968549833674,0.991680746768578,
0.989334769731189,0.989334769731189,0.989334769731189)))
REPRESENTATION_ITEM('')
SURFACE()
);
#1927=(
BOUNDED_SURFACE()
B_SPLINE_SURFACE(1,2,((#127107,#127108,#127109,#127110,#127111),(#127112,
#127113,#127114,#127115,#127116)),.UNSPECIFIED.,.F.,.F.,.F.)
B_SPLINE_SURFACE_WITH_KNOTS((2,2),(3,2,3),(0.710192959007196,1.),(0.211502584834064,
0.214285714285714,0.228987659635168),.UNSPECIFIED.)
GEOMETRIC_REPRESENTATION_ITEM()
RATIONAL_B_SPLINE_SURFACE(((0.998122319569322,0.999023095875704,1.,0.994839481491406,
0.991803313493282),(0.998122319569322,0.999023095875704,1.,0.994839481491406,
0.991803313493282)))
REPRESENTATION_ITEM('')
SURFACE()
);
#1928=(
BOUNDED_SURFACE()
B_SPLINE_SURFACE(1,2,((#127130,#127131,#127132,#127133,#127134),(#127135,
#127136,#127137,#127138,#127139)),.UNSPECIFIED.,.F.,.F.,.F.)
B_SPLINE_SURFACE_WITH_KNOTS((2,2),(3,2,3),(0.709731017432417,1.),(0.504616569534328,
0.521917529826141,0.522505428191805),.UNSPECIFIED.)
GEOMETRIC_REPRESENTATION_ITEM()
RATIONAL_B_SPLINE_SURFACE(((0.996968549833597,0.99168074676856,0.989334769731189,
0.989334769731189,0.989334769731189),(0.996968549833597,0.99168074676856,
0.989334769731189,0.989334769731189,0.989334769731189)))
REPRESENTATION_ITEM('')
SURFACE()
);
#1929=(
BOUNDED_SURFACE()
B_SPLINE_SURFACE(1,2,((#127150,#127151,#127152,#127153,#127154),(#127155,
#127156,#127157,#127158,#127159)),.UNSPECIFIED.,.F.,.F.,.F.)
B_SPLINE_SURFACE_WITH_KNOTS((2,2),(3,2,3),(0.710192959006417,1.),(0.211502584834052,
0.214285714285714,0.228987659635174),.UNSPECIFIED.)
GEOMETRIC_REPRESENTATION_ITEM()
RATIONAL_B_SPLINE_SURFACE(((0.998122319569314,0.9990230958757,1.,0.994839481491405,
0.99180331349328),(0.998122319569314,0.9990230958757,1.,0.994839481491405,
0.99180331349328)))
REPRESENTATION_ITEM('')
SURFACE()
);
#1930=(
BOUNDED_SURFACE()
B_SPLINE_SURFACE(1,2,((#127173,#127174,#127175,#127176,#127177),(#127178,
#127179,#127180,#127181,#127182)),.UNSPECIFIED.,.F.,.F.,.F.)
B_SPLINE_SURFACE_WITH_KNOTS((2,2),(3,2,3),(0.710318915639158,1.),(0.504616569534302,
0.521917529826141,0.52209053942906),.UNSPECIFIED.)
GEOMETRIC_REPRESENTATION_ITEM()
RATIONAL_B_SPLINE_SURFACE(((0.996968549833613,0.991680746768564,0.989334769731189,
0.989334769731189,0.989334769731189),(0.996968549833613,0.991680746768564,
0.989334769731189,0.989334769731189,0.989334769731189)))
REPRESENTATION_ITEM('')
SURFACE()
);
#1931=(
BOUNDED_SURFACE()
B_SPLINE_SURFACE(1,2,((#127193,#127194,#127195,#127196,#127197),(#127198,
#127199,#127200,#127201,#127202)),.UNSPECIFIED.,.F.,.F.,.F.)
B_SPLINE_SURFACE_WITH_KNOTS((2,2),(3,2,3),(0.710192959007516,1.),(0.211502584834065,
0.214285714285714,0.228987659635173),.UNSPECIFIED.)
GEOMETRIC_REPRESENTATION_ITEM()
RATIONAL_B_SPLINE_SURFACE(((0.998122319569323,0.999023095875705,1.,0.994839481491405,
0.99180331349328),(0.998122319569323,0.999023095875705,1.,0.994839481491405,
0.99180331349328)))
REPRESENTATION_ITEM('')
SURFACE()
);
#1932=(
BOUNDED_SURFACE()
B_SPLINE_SURFACE(1,2,((#127216,#127217,#127218,#127219,#127220),(#127221,
#127222,#127223,#127224,#127225)),.UNSPECIFIED.,.F.,.F.,.F.)
B_SPLINE_SURFACE_WITH_KNOTS((2,2),(3,2,3),(0.710318915640079,1.),(0.504616569534327,
0.52191752982614,0.522090539429058),.UNSPECIFIED.)
GEOMETRIC_REPRESENTATION_ITEM()
RATIONAL_B_SPLINE_SURFACE(((0.996968549833597,0.991680746768561,0.989334769731189,
0.989334769731189,0.989334769731189),(0.996968549833597,0.991680746768561,
0.989334769731189,0.989334769731189,0.989334769731189)))
REPRESENTATION_ITEM('')
SURFACE()
);
#1933=(
BOUNDED_SURFACE()
B_SPLINE_SURFACE(1,2,((#127236,#127237,#127238,#127239,#127240),(#127241,
#127242,#127243,#127244,#127245)),.UNSPECIFIED.,.F.,.F.,.F.)
B_SPLINE_SURFACE_WITH_KNOTS((2,2),(3,2,3),(0.710192959008445,1.),(0.211502584834065,
0.214285714285714,0.228987659635175),.UNSPECIFIED.)
GEOMETRIC_REPRESENTATION_ITEM()
RATIONAL_B_SPLINE_SURFACE(((0.998122319569323,0.999023095875705,1.,0.994839481491404,
0.99180331349328),(0.998122319569323,0.999023095875705,1.,0.994839481491404,
0.99180331349328)))
REPRESENTATION_ITEM('')
SURFACE()
);
#1934=(
BOUNDED_SURFACE()
B_SPLINE_SURFACE(1,2,((#127259,#127260,#127261,#127262,#127263),(#127264,
#127265,#127266,#127267,#127268)),.UNSPECIFIED.,.F.,.F.,.F.)
B_SPLINE_SURFACE_WITH_KNOTS((2,2),(3,2,3),(0.709595573560721,1.),(0.469422374511333,
0.470019760166364,0.48736334072649),.UNSPECIFIED.)
GEOMETRIC_REPRESENTATION_ITEM()
RATIONAL_B_SPLINE_SURFACE(((0.987787102172814,0.987787102172814,0.987787102172814,
0.988764511531023,0.992698258926488),(0.987787102172814,0.987787102172814,
0.987787102172814,0.988764511531023,0.992698258926488)))
REPRESENTATION_ITEM('')
SURFACE()
);
#1935=(
BOUNDED_SURFACE()
B_SPLINE_SURFACE(1,2,((#127277,#127278,#127279),(#127280,#127281,#127282)),
 .UNSPECIFIED.,.F.,.F.,.F.)
B_SPLINE_SURFACE_WITH_KNOTS((2,2),(3,3),(0.710318915640071,1.),(0.24585118339369,
0.263098999273796),.UNSPECIFIED.)
GEOMETRIC_REPRESENTATION_ITEM()
RATIONAL_B_SPLINE_SURFACE(((0.987633126750594,0.986929835989062,0.989150325841653),
(0.987633126750594,0.986929835989062,0.989150325841653)))
REPRESENTATION_ITEM('')
SURFACE()
);
#1936=(
BOUNDED_SURFACE()
B_SPLINE_SURFACE(1,2,((#127284,#127285,#127286,#127287,#127288),(#127289,
#127290,#127291,#127292,#127293)),.UNSPECIFIED.,.F.,.F.,.F.)
B_SPLINE_SURFACE_WITH_KNOTS((2,2),(3,2,3),(0.709595573563224,1.),(0.469422374513835,
0.470019760166364,0.48736334072649),.UNSPECIFIED.)
GEOMETRIC_REPRESENTATION_ITEM()
RATIONAL_B_SPLINE_SURFACE(((0.987787102172814,0.987787102172814,0.987787102172814,
0.988764511531023,0.992698258926488),(0.987787102172814,0.987787102172814,
0.987787102172814,0.988764511531023,0.992698258926488)))
REPRESENTATION_ITEM('')
SURFACE()
);
#1937=(
BOUNDED_SURFACE()
B_SPLINE_SURFACE(1,2,((#127302,#127303,#127304),(#127305,#127306,#127307)),
 .UNSPECIFIED.,.F.,.F.,.F.)
B_SPLINE_SURFACE_WITH_KNOTS((2,2),(3,3),(0.710318915640084,1.),(0.24585118339369,
0.263098999273796),.UNSPECIFIED.)
GEOMETRIC_REPRESENTATION_ITEM()
RATIONAL_B_SPLINE_SURFACE(((0.987633126750594,0.986929835989062,0.989150325841653),
(0.987633126750594,0.986929835989062,0.989150325841653)))
REPRESENTATION_ITEM('')
SURFACE()
);
#1938=(
BOUNDED_SURFACE()
B_SPLINE_SURFACE(1,2,((#127309,#127310,#127311,#127312,#127313),(#127314,
#127315,#127316,#127317,#127318)),.UNSPECIFIED.,.F.,.F.,.F.)
B_SPLINE_SURFACE_WITH_KNOTS((2,2),(3,2,3),(0.709595573570259,1.),(0.46942237452087,
0.470019760166364,0.48736334072649),.UNSPECIFIED.)
GEOMETRIC_REPRESENTATION_ITEM()
RATIONAL_B_SPLINE_SURFACE(((0.987787102172814,0.987787102172814,0.987787102172814,
0.988764511531023,0.992698258926488),(0.987787102172814,0.987787102172814,
0.987787102172814,0.988764511531023,0.992698258926488)))
REPRESENTATION_ITEM('')
SURFACE()
);
#1939=(
BOUNDED_SURFACE()
B_SPLINE_SURFACE(1,2,((#127327,#127328,#127329),(#127330,#127331,#127332)),
 .UNSPECIFIED.,.F.,.F.,.F.)
B_SPLINE_SURFACE_WITH_KNOTS((2,2),(3,3),(0.710318915640074,1.),(0.24585118339369,
0.263098999273796),.UNSPECIFIED.)
GEOMETRIC_REPRESENTATION_ITEM()
RATIONAL_B_SPLINE_SURFACE(((0.987633126750594,0.986929835989062,0.989150325841653),
(0.987633126750594,0.986929835989062,0.989150325841653)))
REPRESENTATION_ITEM('')
SURFACE()
);
#1940=(
BOUNDED_SURFACE()
B_SPLINE_SURFACE(1,2,((#127334,#127335,#127336,#127337,#127338),(#127339,
#127340,#127341,#127342,#127343)),.UNSPECIFIED.,.F.,.F.,.F.)
B_SPLINE_SURFACE_WITH_KNOTS((2,2),(3,2,3),(0.709595573576442,1.),(0.469422374527051,
0.470019760166364,0.48736334072649),.UNSPECIFIED.)
GEOMETRIC_REPRESENTATION_ITEM()
RATIONAL_B_SPLINE_SURFACE(((0.987787102172814,0.987787102172814,0.987787102172814,
0.988764511531023,0.992698258926488),(0.987787102172814,0.987787102172814,
0.987787102172814,0.988764511531023,0.992698258926488)))
REPRESENTATION_ITEM('')
SURFACE()
);
#1941=(
BOUNDED_SURFACE()
B_SPLINE_SURFACE(1,2,((#127352,#127353,#127354),(#127355,#127356,#127357)),
 .UNSPECIFIED.,.F.,.F.,.F.)
B_SPLINE_SURFACE_WITH_KNOTS((2,2),(3,3),(0.710318915640077,1.),(0.24585118339369,
0.263098999273796),.UNSPECIFIED.)
GEOMETRIC_REPRESENTATION_ITEM()
RATIONAL_B_SPLINE_SURFACE(((0.987633126750594,0.986929835989062,0.989150325841653),
(0.987633126750594,0.986929835989062,0.989150325841653)))
REPRESENTATION_ITEM('')
SURFACE()
);
#1942=(
BOUNDED_SURFACE()
B_SPLINE_SURFACE(1,2,((#127359,#127360,#127361,#127362,#127363),(#127364,
#127365,#127366,#127367,#127368)),.UNSPECIFIED.,.F.,.F.,.F.)
B_SPLINE_SURFACE_WITH_KNOTS((2,2),(3,2,3),(0.709595573604623,1.),(0.469422374555238,
0.470019760166364,0.48736334072649),.UNSPECIFIED.)
GEOMETRIC_REPRESENTATION_ITEM()
RATIONAL_B_SPLINE_SURFACE(((0.987787102172814,0.987787102172814,0.987787102172814,
0.988764511531023,0.992698258926488),(0.987787102172814,0.987787102172814,
0.987787102172814,0.988764511531023,0.992698258926488)))
REPRESENTATION_ITEM('')
SURFACE()
);
#1943=(
BOUNDED_SURFACE()
B_SPLINE_SURFACE(1,2,((#127377,#127378,#127379),(#127380,#127381,#127382)),
 .UNSPECIFIED.,.F.,.F.,.F.)
B_SPLINE_SURFACE_WITH_KNOTS((2,2),(3,3),(0.710318915640083,1.),(0.24585118339369,
0.263098999273796),.UNSPECIFIED.)
GEOMETRIC_REPRESENTATION_ITEM()
RATIONAL_B_SPLINE_SURFACE(((0.987633126750594,0.986929835989062,0.989150325841653),
(0.987633126750594,0.986929835989062,0.989150325841653)))
REPRESENTATION_ITEM('')
SURFACE()
);
#1944=(
BOUNDED_SURFACE()
B_SPLINE_SURFACE(1,2,((#127384,#127385,#127386,#127387,#127388),(#127389,
#127390,#127391,#127392,#127393)),.UNSPECIFIED.,.F.,.F.,.F.)
B_SPLINE_SURFACE_WITH_KNOTS((2,2),(3,2,3),(0.709595573593217,1.),(0.469422374543823,
0.470019760166364,0.48736334072649),.UNSPECIFIED.)
GEOMETRIC_REPRESENTATION_ITEM()
RATIONAL_B_SPLINE_SURFACE(((0.987787102172814,0.987787102172814,0.987787102172814,
0.988764511531023,0.992698258926488),(0.987787102172814,0.987787102172814,
0.987787102172814,0.988764511531023,0.992698258926488)))
REPRESENTATION_ITEM('')
SURFACE()
);
#1945=(
BOUNDED_SURFACE()
B_SPLINE_SURFACE(1,2,((#127402,#127403,#127404),(#127405,#127406,#127407)),
 .UNSPECIFIED.,.F.,.F.,.F.)
B_SPLINE_SURFACE_WITH_KNOTS((2,2),(3,3),(0.710318915640078,1.),(0.24585118339369,
0.263098999273796),.UNSPECIFIED.)
GEOMETRIC_REPRESENTATION_ITEM()
RATIONAL_B_SPLINE_SURFACE(((0.987633126750594,0.986929835989062,0.989150325841653),
(0.987633126750594,0.986929835989062,0.989150325841653)))
REPRESENTATION_ITEM('')
SURFACE()
);
#1946=(
BOUNDED_SURFACE()
B_SPLINE_SURFACE(1,2,((#127409,#127410,#127411,#127412,#127413),(#127414,
#127415,#127416,#127417,#127418)),.UNSPECIFIED.,.F.,.F.,.F.)
B_SPLINE_SURFACE_WITH_KNOTS((2,2),(3,2,3),(0.70959557358438,1.),(0.469422374534986,
0.470019760166364,0.48736334072649),.UNSPECIFIED.)
GEOMETRIC_REPRESENTATION_ITEM()
RATIONAL_B_SPLINE_SURFACE(((0.987787102172814,0.987787102172814,0.987787102172814,
0.988764511531023,0.992698258926488),(0.987787102172814,0.987787102172814,
0.987787102172814,0.988764511531023,0.992698258926488)))
REPRESENTATION_ITEM('')
SURFACE()
);
#1947=(
BOUNDED_SURFACE()
B_SPLINE_SURFACE(1,2,((#127427,#127428,#127429),(#127430,#127431,#127432)),
 .UNSPECIFIED.,.F.,.F.,.F.)
B_SPLINE_SURFACE_WITH_KNOTS((2,2),(3,3),(0.710318915640084,1.),(0.24585118339369,
0.263098999273796),.UNSPECIFIED.)
GEOMETRIC_REPRESENTATION_ITEM()
RATIONAL_B_SPLINE_SURFACE(((0.987633126750594,0.986929835989062,0.989150325841653),
(0.987633126750594,0.986929835989062,0.989150325841653)))
REPRESENTATION_ITEM('')
SURFACE()
);
#1948=(
BOUNDED_SURFACE()
B_SPLINE_SURFACE(1,2,((#127434,#127435,#127436,#127437,#127438),(#127439,
#127440,#127441,#127442,#127443)),.UNSPECIFIED.,.F.,.F.,.F.)
B_SPLINE_SURFACE_WITH_KNOTS((2,2),(3,2,3),(0.709595573589852,1.),(0.469422374540461,
0.470019760166364,0.48736334072649),.UNSPECIFIED.)
GEOMETRIC_REPRESENTATION_ITEM()
RATIONAL_B_SPLINE_SURFACE(((0.987787102172814,0.987787102172814,0.987787102172814,
0.988764511531023,0.992698258926488),(0.987787102172814,0.987787102172814,
0.987787102172814,0.988764511531023,0.992698258926488)))
REPRESENTATION_ITEM('')
SURFACE()
);
#1949=(
BOUNDED_SURFACE()
B_SPLINE_SURFACE(1,2,((#127452,#127453,#127454),(#127455,#127456,#127457)),
 .UNSPECIFIED.,.F.,.F.,.F.)
B_SPLINE_SURFACE_WITH_KNOTS((2,2),(3,3),(0.710318915640076,1.),(0.24585118339369,
0.263098999273796),.UNSPECIFIED.)
GEOMETRIC_REPRESENTATION_ITEM()
RATIONAL_B_SPLINE_SURFACE(((0.987633126750594,0.986929835989062,0.989150325841653),
(0.987633126750594,0.986929835989062,0.989150325841653)))
REPRESENTATION_ITEM('')
SURFACE()
);
#1950=(
BOUNDED_SURFACE()
B_SPLINE_SURFACE(1,2,((#127459,#127460,#127461,#127462,#127463),(#127464,
#127465,#127466,#127467,#127468)),.UNSPECIFIED.,.F.,.F.,.F.)
B_SPLINE_SURFACE_WITH_KNOTS((2,2),(3,2,3),(0.709595573559204,1.),(0.469422374509813,
0.470019760166364,0.48736334072649),.UNSPECIFIED.)
GEOMETRIC_REPRESENTATION_ITEM()
RATIONAL_B_SPLINE_SURFACE(((0.987787102172814,0.987787102172814,0.987787102172814,
0.988764511531023,0.992698258926488),(0.987787102172814,0.987787102172814,
0.987787102172814,0.988764511531023,0.992698258926488)))
REPRESENTATION_ITEM('')
SURFACE()
);
#1951=(
BOUNDED_SURFACE()
B_SPLINE_SURFACE(1,2,((#127477,#127478,#127479),(#127480,#127481,#127482)),
 .UNSPECIFIED.,.F.,.F.,.F.)
B_SPLINE_SURFACE_WITH_KNOTS((2,2),(3,3),(0.710318915640081,1.),(0.24585118339369,
0.263098999273796),.UNSPECIFIED.)
GEOMETRIC_REPRESENTATION_ITEM()
RATIONAL_B_SPLINE_SURFACE(((0.987633126750594,0.986929835989062,0.989150325841653),
(0.987633126750594,0.986929835989062,0.989150325841653)))
REPRESENTATION_ITEM('')
SURFACE()
);
#1952=(
BOUNDED_SURFACE()
B_SPLINE_SURFACE(1,2,((#127484,#127485,#127486,#127487,#127488),(#127489,
#127490,#127491,#127492,#127493)),.UNSPECIFIED.,.F.,.F.,.F.)
B_SPLINE_SURFACE_WITH_KNOTS((2,2),(3,2,3),(0.709595573594376,1.),(0.469422374544989,
0.470019760166364,0.48736334072649),.UNSPECIFIED.)
GEOMETRIC_REPRESENTATION_ITEM()
RATIONAL_B_SPLINE_SURFACE(((0.987787102172814,0.987787102172814,0.987787102172814,
0.988764511531023,0.992698258926488),(0.987787102172814,0.987787102172814,
0.987787102172814,0.988764511531023,0.992698258926488)))
REPRESENTATION_ITEM('')
SURFACE()
);
#1953=(
BOUNDED_SURFACE()
B_SPLINE_SURFACE(1,2,((#127502,#127503,#127504),(#127505,#127506,#127507)),
 .UNSPECIFIED.,.F.,.F.,.F.)
B_SPLINE_SURFACE_WITH_KNOTS((2,2),(3,3),(0.710318915640075,1.),(0.24585118339369,
0.263098999273938),.UNSPECIFIED.)
GEOMETRIC_REPRESENTATION_ITEM()
RATIONAL_B_SPLINE_SURFACE(((0.987633126750594,0.986929835989056,0.989150325841689),
(0.987633126750594,0.986929835989056,0.989150325841689)))
REPRESENTATION_ITEM('')
SURFACE()
);
#1954=(
BOUNDED_SURFACE()
B_SPLINE_SURFACE(1,2,((#127509,#127510,#127511,#127512,#127513),(#127514,
#127515,#127516,#127517,#127518)),.UNSPECIFIED.,.F.,.F.,.F.)
B_SPLINE_SURFACE_WITH_KNOTS((2,2),(3,2,3),(0.709595573559938,1.),(0.469422374510549,
0.470019760166367,0.48736334072649),.UNSPECIFIED.)
GEOMETRIC_REPRESENTATION_ITEM()
RATIONAL_B_SPLINE_SURFACE(((0.987787102172814,0.987787102172814,0.987787102172814,
0.988764511531024,0.992698258926488),(0.987787102172814,0.987787102172814,
0.987787102172814,0.988764511531024,0.992698258926488)))
REPRESENTATION_ITEM('')
SURFACE()
);
#1955=(
BOUNDED_SURFACE()
B_SPLINE_SURFACE(1,2,((#127527,#127528,#127529),(#127530,#127531,#127532)),
 .UNSPECIFIED.,.F.,.F.,.F.)
B_SPLINE_SURFACE_WITH_KNOTS((2,2),(3,3),(0.710318915640069,1.),(0.24585118339369,
0.263098999273938),.UNSPECIFIED.)
GEOMETRIC_REPRESENTATION_ITEM()
RATIONAL_B_SPLINE_SURFACE(((0.987633126750594,0.986929835989056,0.98915032584169),
(0.987633126750594,0.986929835989056,0.98915032584169)))
REPRESENTATION_ITEM('')
SURFACE()
);
#1956=(
BOUNDED_SURFACE()
B_SPLINE_SURFACE(1,2,((#127534,#127535,#127536,#127537,#127538),(#127539,
#127540,#127541,#127542,#127543)),.UNSPECIFIED.,.F.,.F.,.F.)
B_SPLINE_SURFACE_WITH_KNOTS((2,2),(3,2,3),(0.70959557357981,1.),(0.469422374530418,
0.470019760166367,0.48736334072649),.UNSPECIFIED.)
GEOMETRIC_REPRESENTATION_ITEM()
RATIONAL_B_SPLINE_SURFACE(((0.987787102172814,0.987787102172814,0.987787102172814,
0.988764511531024,0.992698258926488),(0.987787102172814,0.987787102172814,
0.987787102172814,0.988764511531024,0.992698258926488)))
REPRESENTATION_ITEM('')
SURFACE()
);
#1957=(
BOUNDED_SURFACE()
B_SPLINE_SURFACE(1,2,((#127552,#127553,#127554),(#127555,#127556,#127557)),
 .UNSPECIFIED.,.F.,.F.,.F.)
B_SPLINE_SURFACE_WITH_KNOTS((2,2),(3,3),(0.710318915640074,1.),(0.24585118339369,
0.263098999273937),.UNSPECIFIED.)
GEOMETRIC_REPRESENTATION_ITEM()
RATIONAL_B_SPLINE_SURFACE(((0.987633126750594,0.986929835989056,0.989150325841689),
(0.987633126750594,0.986929835989056,0.989150325841689)))
REPRESENTATION_ITEM('')
SURFACE()
);
#1958=(
BOUNDED_SURFACE()
B_SPLINE_SURFACE(1,2,((#127559,#127560,#127561,#127562,#127563),(#127564,
#127565,#127566,#127567,#127568)),.UNSPECIFIED.,.F.,.F.,.F.)
B_SPLINE_SURFACE_WITH_KNOTS((2,2),(3,2,3),(0.709595573595216,1.),(0.469422374545822,
0.470019760166364,0.48736334072649),.UNSPECIFIED.)
GEOMETRIC_REPRESENTATION_ITEM()
RATIONAL_B_SPLINE_SURFACE(((0.987787102172814,0.987787102172814,0.987787102172814,
0.988764511531023,0.992698258926488),(0.987787102172814,0.987787102172814,
0.987787102172814,0.988764511531023,0.992698258926488)))
REPRESENTATION_ITEM('')
SURFACE()
);
#1959=(
BOUNDED_SURFACE()
B_SPLINE_SURFACE(1,2,((#127577,#127578,#127579),(#127580,#127581,#127582)),
 .UNSPECIFIED.,.F.,.F.,.F.)
B_SPLINE_SURFACE_WITH_KNOTS((2,2),(3,3),(0.710318915640078,1.),(0.24585118339369,
0.263098999273938),.UNSPECIFIED.)
GEOMETRIC_REPRESENTATION_ITEM()
RATIONAL_B_SPLINE_SURFACE(((0.987633126750594,0.986929835989056,0.98915032584169),
(0.987633126750594,0.986929835989056,0.98915032584169)))
REPRESENTATION_ITEM('')
SURFACE()
);
#1960=(
BOUNDED_SURFACE()
B_SPLINE_SURFACE(1,2,((#127584,#127585,#127586,#127587,#127588),(#127589,
#127590,#127591,#127592,#127593)),.UNSPECIFIED.,.F.,.F.,.F.)
B_SPLINE_SURFACE_WITH_KNOTS((2,2),(3,2,3),(0.709595573583186,1.),(0.469422374533795,
0.470019760166364,0.48736334072649),.UNSPECIFIED.)
GEOMETRIC_REPRESENTATION_ITEM()
RATIONAL_B_SPLINE_SURFACE(((0.987787102172814,0.987787102172814,0.987787102172814,
0.988764511531023,0.992698258926488),(0.987787102172814,0.987787102172814,
0.987787102172814,0.988764511531023,0.992698258926488)))
REPRESENTATION_ITEM('')
SURFACE()
);
#1961=(
BOUNDED_SURFACE()
B_SPLINE_SURFACE(1,2,((#127602,#127603,#127604),(#127605,#127606,#127607)),
 .UNSPECIFIED.,.F.,.F.,.F.)
B_SPLINE_SURFACE_WITH_KNOTS((2,2),(3,3),(0.710318915640077,1.),(0.24585118339369,
0.263098999273938),.UNSPECIFIED.)
GEOMETRIC_REPRESENTATION_ITEM()
RATIONAL_B_SPLINE_SURFACE(((0.987633126750594,0.986929835989056,0.989150325841689),
(0.987633126750594,0.986929835989056,0.989150325841689)))
REPRESENTATION_ITEM('')
SURFACE()
);
#1962=(
BOUNDED_SURFACE()
B_SPLINE_SURFACE(1,2,((#127609,#127610,#127611,#127612,#127613),(#127614,
#127615,#127616,#127617,#127618)),.UNSPECIFIED.,.F.,.F.,.F.)
B_SPLINE_SURFACE_WITH_KNOTS((2,2),(3,2,3),(0.709961051579736,1.),(0.469787852530351,
0.470019760166364,0.48736334072649),.UNSPECIFIED.)
GEOMETRIC_REPRESENTATION_ITEM()
RATIONAL_B_SPLINE_SURFACE(((0.987787102172814,0.987787102172814,0.987787102172814,
0.988764511531023,0.992698258926488),(0.987787102172814,0.987787102172814,
0.987787102172814,0.988764511531023,0.992698258926488)))
REPRESENTATION_ITEM('')
SURFACE()
);
#1963=(
BOUNDED_SURFACE()
B_SPLINE_SURFACE(1,2,((#127627,#127628,#127629),(#127630,#127631,#127632)),
 .UNSPECIFIED.,.F.,.F.,.F.)
B_SPLINE_SURFACE_WITH_KNOTS((2,2),(3,3),(0.710318915640071,1.),(0.24585118339369,
0.263098999273938),.UNSPECIFIED.)
GEOMETRIC_REPRESENTATION_ITEM()
RATIONAL_B_SPLINE_SURFACE(((0.987633126750594,0.986929835989056,0.98915032584169),
(0.987633126750594,0.986929835989056,0.98915032584169)))
REPRESENTATION_ITEM('')
SURFACE()
);
#1964=(
BOUNDED_SURFACE()
B_SPLINE_SURFACE(1,2,((#127634,#127635,#127636,#127637,#127638),(#127639,
#127640,#127641,#127642,#127643)),.UNSPECIFIED.,.F.,.F.,.F.)
B_SPLINE_SURFACE_WITH_KNOTS((2,2),(3,2,3),(0.709595573585733,1.),(0.469422374536338,
0.470019760166364,0.48736334072649),.UNSPECIFIED.)
GEOMETRIC_REPRESENTATION_ITEM()
RATIONAL_B_SPLINE_SURFACE(((0.987787102172814,0.987787102172814,0.987787102172814,
0.988764511531023,0.992698258926488),(0.987787102172814,0.987787102172814,
0.987787102172814,0.988764511531023,0.992698258926488)))
REPRESENTATION_ITEM('')
SURFACE()
);
#1965=(
BOUNDED_SURFACE()
B_SPLINE_SURFACE(1,2,((#127652,#127653,#127654),(#127655,#127656,#127657)),
 .UNSPECIFIED.,.F.,.F.,.F.)
B_SPLINE_SURFACE_WITH_KNOTS((2,2),(3,3),(0.710318915640081,1.),(0.245851183393689,
0.263098999273938),.UNSPECIFIED.)
GEOMETRIC_REPRESENTATION_ITEM()
RATIONAL_B_SPLINE_SURFACE(((0.987633126750594,0.986929835989056,0.989150325841689),
(0.987633126750594,0.986929835989056,0.989150325841689)))
REPRESENTATION_ITEM('')
SURFACE()
);
#1966=(
BOUNDED_SURFACE()
B_SPLINE_SURFACE(1,2,((#127659,#127660,#127661,#127662,#127663),(#127664,
#127665,#127666,#127667,#127668)),.UNSPECIFIED.,.F.,.F.,.F.)
B_SPLINE_SURFACE_WITH_KNOTS((2,2),(3,2,3),(0.709595573571102,1.),(0.469422374521711,
0.470019760166364,0.48736334072649),.UNSPECIFIED.)
GEOMETRIC_REPRESENTATION_ITEM()
RATIONAL_B_SPLINE_SURFACE(((0.987787102172814,0.987787102172814,0.987787102172814,
0.988764511531023,0.992698258926488),(0.987787102172814,0.987787102172814,
0.987787102172814,0.988764511531023,0.992698258926488)))
REPRESENTATION_ITEM('')
SURFACE()
);
#1967=(
BOUNDED_SURFACE()
B_SPLINE_SURFACE(1,2,((#127677,#127678,#127679),(#127680,#127681,#127682)),
 .UNSPECIFIED.,.F.,.F.,.F.)
B_SPLINE_SURFACE_WITH_KNOTS((2,2),(3,3),(0.710318915640074,1.),(0.24585118339369,
0.263098999273796),.UNSPECIFIED.)
GEOMETRIC_REPRESENTATION_ITEM()
RATIONAL_B_SPLINE_SURFACE(((0.987633126750594,0.986929835989062,0.989150325841653),
(0.987633126750594,0.986929835989062,0.989150325841653)))
REPRESENTATION_ITEM('')
SURFACE()
);
#1968=(
BOUNDED_SURFACE()
B_SPLINE_SURFACE(1,2,((#127684,#127685,#127686,#127687,#127688),(#127689,
#127690,#127691,#127692,#127693)),.UNSPECIFIED.,.F.,.F.,.F.)
B_SPLINE_SURFACE_WITH_KNOTS((2,2),(3,2,3),(0.709595573536973,1.),(0.469422374487583,
0.470019760166364,0.48736334072649),.UNSPECIFIED.)
GEOMETRIC_REPRESENTATION_ITEM()
RATIONAL_B_SPLINE_SURFACE(((0.987787102172814,0.987787102172814,0.987787102172814,
0.988764511531023,0.992698258926488),(0.987787102172814,0.987787102172814,
0.987787102172814,0.988764511531023,0.992698258926488)))
REPRESENTATION_ITEM('')
SURFACE()
);
#1969=(
BOUNDED_SURFACE()
B_SPLINE_SURFACE(1,2,((#127702,#127703,#127704),(#127705,#127706,#127707)),
 .UNSPECIFIED.,.F.,.F.,.F.)
B_SPLINE_SURFACE_WITH_KNOTS((2,2),(3,3),(0.71031891564008,1.),(0.24585118339369,
0.263098999273796),.UNSPECIFIED.)
GEOMETRIC_REPRESENTATION_ITEM()
RATIONAL_B_SPLINE_SURFACE(((0.987633126750594,0.986929835989062,0.989150325841653),
(0.987633126750594,0.986929835989062,0.989150325841653)))
REPRESENTATION_ITEM('')
SURFACE()
);
#1970=(
BOUNDED_SURFACE()
B_SPLINE_SURFACE(1,2,((#127709,#127710,#127711,#127712,#127713),(#127714,
#127715,#127716,#127717,#127718)),.UNSPECIFIED.,.F.,.F.,.F.)
B_SPLINE_SURFACE_WITH_KNOTS((2,2),(3,2,3),(0.709595573578629,1.),(0.469422374529239,
0.470019760166364,0.48736334072649),.UNSPECIFIED.)
GEOMETRIC_REPRESENTATION_ITEM()
RATIONAL_B_SPLINE_SURFACE(((0.987787102172814,0.987787102172814,0.987787102172814,
0.988764511531023,0.992698258926488),(0.987787102172814,0.987787102172814,
0.987787102172814,0.988764511531023,0.992698258926488)))
REPRESENTATION_ITEM('')
SURFACE()
);
#1971=(
BOUNDED_SURFACE()
B_SPLINE_SURFACE(1,2,((#127727,#127728,#127729),(#127730,#127731,#127732)),
 .UNSPECIFIED.,.F.,.F.,.F.)
B_SPLINE_SURFACE_WITH_KNOTS((2,2),(3,3),(0.710318915640078,1.),(0.24585118339369,
0.263098999273796),.UNSPECIFIED.)
GEOMETRIC_REPRESENTATION_ITEM()
RATIONAL_B_SPLINE_SURFACE(((0.987633126750594,0.986929835989062,0.989150325841653),
(0.987633126750594,0.986929835989062,0.989150325841653)))
REPRESENTATION_ITEM('')
SURFACE()
);
#1972=(
BOUNDED_SURFACE()
B_SPLINE_SURFACE(1,2,((#127734,#127735,#127736,#127737,#127738),(#127739,
#127740,#127741,#127742,#127743)),.UNSPECIFIED.,.F.,.F.,.F.)
B_SPLINE_SURFACE_WITH_KNOTS((2,2),(3,2,3),(0.709595573584959,1.),(0.469422374535573,
0.470019760166364,0.48736334072649),.UNSPECIFIED.)
GEOMETRIC_REPRESENTATION_ITEM()
RATIONAL_B_SPLINE_SURFACE(((0.987787102172814,0.987787102172814,0.987787102172814,
0.988764511531023,0.992698258926488),(0.987787102172814,0.987787102172814,
0.987787102172814,0.988764511531023,0.992698258926488)))
REPRESENTATION_ITEM('')
SURFACE()
);
#1973=(
BOUNDED_SURFACE()
B_SPLINE_SURFACE(1,2,((#127752,#127753,#127754),(#127755,#127756,#127757)),
 .UNSPECIFIED.,.F.,.F.,.F.)
B_SPLINE_SURFACE_WITH_KNOTS((2,2),(3,3),(0.71031891564008,1.),(0.24585118339369,
0.263098999273796),.UNSPECIFIED.)
GEOMETRIC_REPRESENTATION_ITEM()
RATIONAL_B_SPLINE_SURFACE(((0.987633126750594,0.986929835989062,0.989150325841653),
(0.987633126750594,0.986929835989062,0.989150325841653)))
REPRESENTATION_ITEM('')
SURFACE()
);
#1974=(
BOUNDED_SURFACE()
B_SPLINE_SURFACE(1,2,((#127759,#127760,#127761,#127762,#127763),(#127764,
#127765,#127766,#127767,#127768)),.UNSPECIFIED.,.F.,.F.,.F.)
B_SPLINE_SURFACE_WITH_KNOTS((2,2),(3,2,3),(0.709595573563293,1.),(0.469422374515312,
0.470019760166364,0.48736334072649),.UNSPECIFIED.)
GEOMETRIC_REPRESENTATION_ITEM()
RATIONAL_B_SPLINE_SURFACE(((0.987787102172814,0.987787102172814,0.987787102172814,
0.988764511531023,0.992698258926488),(0.987787102172814,0.987787102172814,
0.987787102172814,0.988764511531023,0.992698258926488)))
REPRESENTATION_ITEM('')
SURFACE()
);
#1975=(
BOUNDED_SURFACE()
B_SPLINE_SURFACE(1,2,((#127777,#127778,#127779),(#127780,#127781,#127782)),
 .UNSPECIFIED.,.F.,.F.,.F.)
B_SPLINE_SURFACE_WITH_KNOTS((2,2),(3,3),(0.710318915638679,1.),(0.24585118339369,
0.263098999273796),.UNSPECIFIED.)
GEOMETRIC_REPRESENTATION_ITEM()
RATIONAL_B_SPLINE_SURFACE(((0.987633126750594,0.986929835989062,0.989150325841653),
(0.987633126750594,0.986929835989062,0.989150325841653)))
REPRESENTATION_ITEM('')
SURFACE()
);
#1976=(
BOUNDED_SURFACE()
B_SPLINE_SURFACE(1,2,((#127784,#127785,#127786,#127787,#127788),(#127789,
#127790,#127791,#127792,#127793)),.UNSPECIFIED.,.F.,.F.,.F.)
B_SPLINE_SURFACE_WITH_KNOTS((2,2),(3,2,3),(0.709595573585933,1.),(0.469422374536543,
0.470019760166364,0.48736334072649),.UNSPECIFIED.)
GEOMETRIC_REPRESENTATION_ITEM()
RATIONAL_B_SPLINE_SURFACE(((0.987787102172814,0.987787102172814,0.987787102172814,
0.988764511531023,0.992698258926488),(0.987787102172814,0.987787102172814,
0.987787102172814,0.988764511531023,0.992698258926488)))
REPRESENTATION_ITEM('')
SURFACE()
);
#1977=(
BOUNDED_SURFACE()
B_SPLINE_SURFACE(1,2,((#127802,#127803,#127804),(#127805,#127806,#127807)),
 .UNSPECIFIED.,.F.,.F.,.F.)
B_SPLINE_SURFACE_WITH_KNOTS((2,2),(3,3),(0.710318915640079,1.),(0.24585118339369,
0.263098999273799),.UNSPECIFIED.)
GEOMETRIC_REPRESENTATION_ITEM()
RATIONAL_B_SPLINE_SURFACE(((0.987633126750594,0.986929835989062,0.989150325841654),
(0.987633126750594,0.986929835989062,0.989150325841654)))
REPRESENTATION_ITEM('')
SURFACE()
);
#1978=(
BOUNDED_SURFACE()
B_SPLINE_SURFACE(1,2,((#127809,#127810,#127811,#127812,#127813),(#127814,
#127815,#127816,#127817,#127818)),.UNSPECIFIED.,.F.,.F.,.F.)
B_SPLINE_SURFACE_WITH_KNOTS((2,2),(3,2,3),(0.709595573588909,1.),(0.469422374539605,
0.470019760166367,0.487363340726489),.UNSPECIFIED.)
GEOMETRIC_REPRESENTATION_ITEM()
RATIONAL_B_SPLINE_SURFACE(((0.987787102172814,0.987787102172814,0.987787102172814,
0.988764511531024,0.992698258926487),(0.987787102172814,0.987787102172814,
0.987787102172814,0.988764511531024,0.992698258926487)))
REPRESENTATION_ITEM('')
SURFACE()
);
#1979=(
BOUNDED_SURFACE()
B_SPLINE_SURFACE(1,2,((#127827,#127828,#127829),(#127830,#127831,#127832)),
 .UNSPECIFIED.,.F.,.F.,.F.)
B_SPLINE_SURFACE_WITH_KNOTS((2,2),(3,3),(0.710318915640001,1.),(0.245851183393691,
0.263098999273797),.UNSPECIFIED.)
GEOMETRIC_REPRESENTATION_ITEM()
RATIONAL_B_SPLINE_SURFACE(((0.987633126750594,0.986929835989062,0.989150325841653),
(0.987633126750594,0.986929835989062,0.989150325841653)))
REPRESENTATION_ITEM('')
SURFACE()
);
#1980=(
BOUNDED_SURFACE()
B_SPLINE_SURFACE(1,2,((#127834,#127835,#127836,#127837,#127838),(#127839,
#127840,#127841,#127842,#127843)),.UNSPECIFIED.,.F.,.F.,.F.)
B_SPLINE_SURFACE_WITH_KNOTS((2,2),(3,2,3),(0.709595573560027,1.),(0.469422374510715,
0.470019760166363,0.487363340726489),.UNSPECIFIED.)
GEOMETRIC_REPRESENTATION_ITEM()
RATIONAL_B_SPLINE_SURFACE(((0.987787102172813,0.987787102172813,0.987787102172813,
0.988764511531023,0.992698258926487),(0.987787102172814,0.987787102172814,
0.987787102172814,0.988764511531023,0.992698258926487)))
REPRESENTATION_ITEM('')
SURFACE()
);
#1981=(
BOUNDED_SURFACE()
B_SPLINE_SURFACE(1,2,((#127852,#127853,#127854),(#127855,#127856,#127857)),
 .UNSPECIFIED.,.F.,.F.,.F.)
B_SPLINE_SURFACE_WITH_KNOTS((2,2),(3,3),(0.71031891564,1.),(0.245851183393691,
0.2630989992738),.UNSPECIFIED.)
GEOMETRIC_REPRESENTATION_ITEM()
RATIONAL_B_SPLINE_SURFACE(((0.987633126750594,0.986929835989062,0.989150325841654),
(0.987633126750594,0.986929835989062,0.989150325841654)))
REPRESENTATION_ITEM('')
SURFACE()
);
#1982=(
BOUNDED_SURFACE()
B_SPLINE_SURFACE(1,2,((#127859,#127860,#127861,#127862,#127863),(#127864,
#127865,#127866,#127867,#127868)),.UNSPECIFIED.,.F.,.F.,.F.)
B_SPLINE_SURFACE_WITH_KNOTS((2,2),(3,2,3),(0.70959557356092,1.),(0.469422374511607,
0.470019760166363,0.487363340726489),.UNSPECIFIED.)
GEOMETRIC_REPRESENTATION_ITEM()
RATIONAL_B_SPLINE_SURFACE(((0.987787102172813,0.987787102172813,0.987787102172813,
0.988764511531023,0.992698258926487),(0.987787102172813,0.987787102172813,
0.987787102172813,0.988764511531023,0.992698258926487)))
REPRESENTATION_ITEM('')
SURFACE()
);
#1983=(
BOUNDED_SURFACE()
B_SPLINE_SURFACE(1,2,((#127877,#127878,#127879),(#127880,#127881,#127882)),
 .UNSPECIFIED.,.F.,.F.,.F.)
B_SPLINE_SURFACE_WITH_KNOTS((2,2),(3,3),(0.710318915640003,1.),(0.245851183393691,
0.26309899927383),.UNSPECIFIED.)
GEOMETRIC_REPRESENTATION_ITEM()
RATIONAL_B_SPLINE_SURFACE(((0.987633126750594,0.98692983598906,0.989150325841661),
(0.987633126750594,0.98692983598906,0.989150325841662)))
REPRESENTATION_ITEM('')
SURFACE()
);
#1984=(
BOUNDED_SURFACE()
B_SPLINE_SURFACE(1,2,((#127884,#127885,#127886,#127887,#127888),(#127889,
#127890,#127891,#127892,#127893)),.UNSPECIFIED.,.F.,.F.,.F.)
B_SPLINE_SURFACE_WITH_KNOTS((2,2),(3,2,3),(0.709595573558224,1.),(0.469422374509515,
0.470019760166363,0.487363340726489),.UNSPECIFIED.)
GEOMETRIC_REPRESENTATION_ITEM()
RATIONAL_B_SPLINE_SURFACE(((0.987787102172813,0.987787102172813,0.987787102172813,
0.988764511531023,0.992698258926487),(0.987787102172813,0.987787102172813,
0.987787102172813,0.988764511531023,0.992698258926487)))
REPRESENTATION_ITEM('')
SURFACE()
);
#1985=(
BOUNDED_SURFACE()
B_SPLINE_SURFACE(1,2,((#127902,#127903,#127904),(#127905,#127906,#127907)),
 .UNSPECIFIED.,.F.,.F.,.F.)
B_SPLINE_SURFACE_WITH_KNOTS((2,2),(3,3),(0.7103189156394,1.),(0.245851183393691,
0.263098999273797),.UNSPECIFIED.)
GEOMETRIC_REPRESENTATION_ITEM()
RATIONAL_B_SPLINE_SURFACE(((0.987633126750594,0.986929835989062,0.989150325841653),
(0.987633126750594,0.986929835989062,0.989150325841653)))
REPRESENTATION_ITEM('')
SURFACE()
);
#1986=(
BOUNDED_SURFACE()
B_SPLINE_SURFACE(1,2,((#127909,#127910,#127911,#127912,#127913),(#127914,
#127915,#127916,#127917,#127918)),.UNSPECIFIED.,.F.,.F.,.F.)
B_SPLINE_SURFACE_WITH_KNOTS((2,2),(3,2,3),(0.709595573582174,1.),(0.46942237453283,
0.470019760166363,0.487363340726489),.UNSPECIFIED.)
GEOMETRIC_REPRESENTATION_ITEM()
RATIONAL_B_SPLINE_SURFACE(((0.987787102172814,0.987787102172814,0.987787102172814,
0.988764511531023,0.992698258926487),(0.987787102172814,0.987787102172814,
0.987787102172814,0.988764511531023,0.992698258926487)))
REPRESENTATION_ITEM('')
SURFACE()
);
#1987=(
BOUNDED_SURFACE()
B_SPLINE_SURFACE(1,2,((#127927,#127928,#127929),(#127930,#127931,#127932)),
 .UNSPECIFIED.,.F.,.F.,.F.)
B_SPLINE_SURFACE_WITH_KNOTS((2,2),(3,3),(0.710318915640033,1.),(0.245851183393691,
0.263098999273797),.UNSPECIFIED.)
GEOMETRIC_REPRESENTATION_ITEM()
RATIONAL_B_SPLINE_SURFACE(((0.987633126750594,0.986929835989062,0.989150325841653),
(0.987633126750594,0.986929835989062,0.989150325841653)))
REPRESENTATION_ITEM('')
SURFACE()
);
#1988=(
BOUNDED_SURFACE()
B_SPLINE_SURFACE(1,2,((#127934,#127935,#127936,#127937,#127938),(#127939,
#127940,#127941,#127942,#127943)),.UNSPECIFIED.,.F.,.F.,.F.)
B_SPLINE_SURFACE_WITH_KNOTS((2,2),(3,2,3),(0.709595573563331,1.),(0.469422374514008,
0.470019760166363,0.487363340726489),.UNSPECIFIED.)
GEOMETRIC_REPRESENTATION_ITEM()
RATIONAL_B_SPLINE_SURFACE(((0.987787102172813,0.987787102172813,0.987787102172813,
0.988764511531023,0.992698258926487),(0.987787102172813,0.987787102172813,
0.987787102172813,0.988764511531023,0.992698258926487)))
REPRESENTATION_ITEM('')
SURFACE()
);
#1989=(
BOUNDED_SURFACE()
B_SPLINE_SURFACE(1,2,((#127952,#127953,#127954),(#127955,#127956,#127957)),
 .UNSPECIFIED.,.F.,.F.,.F.)
B_SPLINE_SURFACE_WITH_KNOTS((2,2),(3,3),(0.710318915640017,1.),(0.245851183393691,
0.263098999273797),.UNSPECIFIED.)
GEOMETRIC_REPRESENTATION_ITEM()
RATIONAL_B_SPLINE_SURFACE(((0.987633126750594,0.986929835989062,0.989150325841653),
(0.987633126750594,0.986929835989062,0.989150325841653)))
REPRESENTATION_ITEM('')
SURFACE()
);
#1990=(
BOUNDED_SURFACE()
B_SPLINE_SURFACE(1,2,((#127959,#127960,#127961,#127962,#127963),(#127964,
#127965,#127966,#127967,#127968)),.UNSPECIFIED.,.F.,.F.,.F.)
B_SPLINE_SURFACE_WITH_KNOTS((2,2),(3,2,3),(0.709595573612439,1.),(0.46942237456311,
0.470019760166363,0.487363340726489),.UNSPECIFIED.)
GEOMETRIC_REPRESENTATION_ITEM()
RATIONAL_B_SPLINE_SURFACE(((0.987787102172814,0.987787102172814,0.987787102172814,
0.988764511531023,0.992698258926487),(0.987787102172813,0.987787102172813,
0.987787102172813,0.988764511531023,0.992698258926487)))
REPRESENTATION_ITEM('')
SURFACE()
);
#1991=(
BOUNDED_SURFACE()
B_SPLINE_SURFACE(1,2,((#127977,#127978,#127979),(#127980,#127981,#127982)),
 .UNSPECIFIED.,.F.,.F.,.F.)
B_SPLINE_SURFACE_WITH_KNOTS((2,2),(3,3),(0.710318915640028,1.),(0.245851183393691,
0.263098999273796),.UNSPECIFIED.)
GEOMETRIC_REPRESENTATION_ITEM()
RATIONAL_B_SPLINE_SURFACE(((0.987633126750594,0.986929835989062,0.989150325841653),
(0.987633126750594,0.986929835989062,0.989150325841653)))
REPRESENTATION_ITEM('')
SURFACE()
);
#1992=(
BOUNDED_SURFACE()
B_SPLINE_SURFACE(1,2,((#127984,#127985,#127986,#127987,#127988),(#127989,
#127990,#127991,#127992,#127993)),.UNSPECIFIED.,.F.,.F.,.F.)
B_SPLINE_SURFACE_WITH_KNOTS((2,2),(3,2,3),(0.,0.290289290029958),(0.194028469417326,
0.211502584834065,0.212110790666945),.UNSPECIFIED.)
GEOMETRIC_REPRESENTATION_ITEM()
RATIONAL_B_SPLINE_SURFACE(((0.989812124691679,0.992466718773227,0.998122319569323,
0.998122319569323,0.998122319569323),(0.989812124691679,0.992466718773227,
0.998122319569323,0.998122319569323,0.998122319569323)))
REPRESENTATION_ITEM('')
SURFACE()
);
#1993=(
BOUNDED_SURFACE()
B_SPLINE_SURFACE(1,2,((#128002,#128003,#128004),(#128005,#128006,#128007)),
 .UNSPECIFIED.,.F.,.F.,.F.)
B_SPLINE_SURFACE_WITH_KNOTS((2,2),(3,3),(0.,0.289807040991561),(0.52191752982614,
0.539102123117534),.UNSPECIFIED.)
GEOMETRIC_REPRESENTATION_ITEM()
RATIONAL_B_SPLINE_SURFACE(((0.989334769731189,0.987004571835916,0.987576759359605),
(0.989334769731189,0.987004571835916,0.987576759359605)))
REPRESENTATION_ITEM('')
SURFACE()
);
#1994=(
BOUNDED_SURFACE()
B_SPLINE_SURFACE(1,2,((#128009,#128010,#128011,#128012,#128013),(#128014,
#128015,#128016,#128017,#128018)),.UNSPECIFIED.,.F.,.F.,.F.)
B_SPLINE_SURFACE_WITH_KNOTS((2,2),(3,2,3),(0.,0.290289290020155),(0.194028469417326,
0.211502584834065,0.212110790657142),.UNSPECIFIED.)
GEOMETRIC_REPRESENTATION_ITEM()
RATIONAL_B_SPLINE_SURFACE(((0.989812124691679,0.992466718773227,0.998122319569323,
0.998122319569323,0.998122319569323),(0.989812124691679,0.992466718773227,
0.998122319569323,0.998122319569323,0.998122319569323)))
REPRESENTATION_ITEM('')
SURFACE()
);
#1995=(
BOUNDED_SURFACE()
B_SPLINE_SURFACE(1,2,((#128027,#128028,#128029),(#128030,#128031,#128032)),
 .UNSPECIFIED.,.F.,.F.,.F.)
B_SPLINE_SURFACE_WITH_KNOTS((2,2),(3,3),(0.,0.289807040992492),(0.52191752982614,
0.539102123117534),.UNSPECIFIED.)
GEOMETRIC_REPRESENTATION_ITEM()
RATIONAL_B_SPLINE_SURFACE(((0.989334769731189,0.987004571835916,0.987576759359605),
(0.989334769731189,0.987004571835916,0.987576759359605)))
REPRESENTATION_ITEM('')
SURFACE()
);
#1996=(
BOUNDED_SURFACE()
B_SPLINE_SURFACE(1,2,((#128034,#128035,#128036,#128037,#128038),(#128039,
#128040,#128041,#128042,#128043)),.UNSPECIFIED.,.F.,.F.,.F.)
B_SPLINE_SURFACE_WITH_KNOTS((2,2),(3,2,3),(0.,0.290289290029112),(0.194028469417326,
0.211502584834065,0.212110790666098),.UNSPECIFIED.)
GEOMETRIC_REPRESENTATION_ITEM()
RATIONAL_B_SPLINE_SURFACE(((0.989812124691679,0.992466718773227,0.998122319569323,
0.998122319569323,0.998122319569323),(0.989812124691679,0.992466718773227,
0.998122319569323,0.998122319569323,0.998122319569323)))
REPRESENTATION_ITEM('')
SURFACE()
);
#1997=(
BOUNDED_SURFACE()
B_SPLINE_SURFACE(1,2,((#128052,#128053,#128054),(#128055,#128056,#128057)),
 .UNSPECIFIED.,.F.,.F.,.F.)
B_SPLINE_SURFACE_WITH_KNOTS((2,2),(3,3),(0.,0.289807040992486),(0.52191752982614,
0.539102123117534),.UNSPECIFIED.)
GEOMETRIC_REPRESENTATION_ITEM()
RATIONAL_B_SPLINE_SURFACE(((0.989334769731189,0.987004571835916,0.987576759359605),
(0.989334769731189,0.987004571835916,0.987576759359605)))
REPRESENTATION_ITEM('')
SURFACE()
);
#1998=(
BOUNDED_SURFACE()
B_SPLINE_SURFACE(1,2,((#128059,#128060,#128061,#128062,#128063),(#128064,
#128065,#128066,#128067,#128068)),.UNSPECIFIED.,.F.,.F.,.F.)
B_SPLINE_SURFACE_WITH_KNOTS((2,2),(3,2,3),(0.,0.290289290026752),(0.194028469417326,
0.211502584834065,0.212110790663731),.UNSPECIFIED.)
GEOMETRIC_REPRESENTATION_ITEM()
RATIONAL_B_SPLINE_SURFACE(((0.989812124691679,0.992466718773227,0.998122319569323,
0.998122319569323,0.998122319569323),(0.989812124691679,0.992466718773227,
0.998122319569323,0.998122319569323,0.998122319569323)))
REPRESENTATION_ITEM('')
SURFACE()
);
#1999=(
BOUNDED_SURFACE()
B_SPLINE_SURFACE(1,2,((#128077,#128078,#128079),(#128080,#128081,#128082)),
 .UNSPECIFIED.,.F.,.F.,.F.)
B_SPLINE_SURFACE_WITH_KNOTS((2,2),(3,3),(0.,0.289807040992493),(0.52191752982614,
0.539102123117534),.UNSPECIFIED.)
GEOMETRIC_REPRESENTATION_ITEM()
RATIONAL_B_SPLINE_SURFACE(((0.989334769731189,0.987004571835916,0.987576759359605),
(0.989334769731189,0.987004571835916,0.987576759359604)))
REPRESENTATION_ITEM('')
SURFACE()
);
#2000=(
BOUNDED_SURFACE()
B_SPLINE_SURFACE(1,2,((#128084,#128085,#128086,#128087,#128088),(#128089,
#128090,#128091,#128092,#128093)),.UNSPECIFIED.,.F.,.F.,.F.)
B_SPLINE_SURFACE_WITH_KNOTS((2,2),(3,2,3),(0.,0.290289290015737),(0.194028469417326,
0.211502584834065,0.21211079065272),.UNSPECIFIED.)
GEOMETRIC_REPRESENTATION_ITEM()
RATIONAL_B_SPLINE_SURFACE(((0.989812124691679,0.992466718773227,0.998122319569323,
0.998122319569323,0.998122319569323),(0.989812124691679,0.992466718773227,
0.998122319569323,0.998122319569323,0.998122319569323)))
REPRESENTATION_ITEM('')
SURFACE()
);
#2001=(
BOUNDED_SURFACE()
B_SPLINE_SURFACE(1,2,((#128102,#128103,#128104),(#128105,#128106,#128107)),
 .UNSPECIFIED.,.F.,.F.,.F.)
B_SPLINE_SURFACE_WITH_KNOTS((2,2),(3,3),(0.,0.289807040993074),(0.52191752982614,
0.539102123117534),.UNSPECIFIED.)
GEOMETRIC_REPRESENTATION_ITEM()
RATIONAL_B_SPLINE_SURFACE(((0.989334769731189,0.987004571835916,0.987576759359605),
(0.989334769731189,0.987004571835916,0.987576759359605)))
REPRESENTATION_ITEM('')
SURFACE()
);
#2002=(
BOUNDED_SURFACE()
B_SPLINE_SURFACE(1,2,((#128109,#128110,#128111,#128112,#128113),(#128114,
#128115,#128116,#128117,#128118)),.UNSPECIFIED.,.F.,.F.,.F.)
B_SPLINE_SURFACE_WITH_KNOTS((2,2),(3,2,3),(0.,0.290289290022082),(0.194028469417326,
0.211502584834065,0.212110790659061),.UNSPECIFIED.)
GEOMETRIC_REPRESENTATION_ITEM()
RATIONAL_B_SPLINE_SURFACE(((0.989812124691679,0.992466718773227,0.998122319569323,
0.998122319569323,0.998122319569323),(0.989812124691679,0.992466718773227,
0.998122319569323,0.998122319569323,0.998122319569323)))
REPRESENTATION_ITEM('')
SURFACE()
);
#2003=(
BOUNDED_SURFACE()
B_SPLINE_SURFACE(1,2,((#128127,#128128,#128129),(#128130,#128131,#128132)),
 .UNSPECIFIED.,.F.,.F.,.F.)
B_SPLINE_SURFACE_WITH_KNOTS((2,2),(3,3),(0.,0.289807040992486),(0.52191752982614,
0.539102123117534),.UNSPECIFIED.)
GEOMETRIC_REPRESENTATION_ITEM()
RATIONAL_B_SPLINE_SURFACE(((0.989334769731189,0.987004571835916,0.987576759359605),
(0.989334769731189,0.987004571835916,0.987576759359605)))
REPRESENTATION_ITEM('')
SURFACE()
);
#2004=(
BOUNDED_SURFACE()
B_SPLINE_SURFACE(1,2,((#128134,#128135,#128136,#128137,#128138),(#128139,
#128140,#128141,#128142,#128143)),.UNSPECIFIED.,.F.,.F.,.F.)
B_SPLINE_SURFACE_WITH_KNOTS((2,2),(3,2,3),(0.,0.290289290016757),(0.194028469417326,
0.211502584834065,0.212110790653736),.UNSPECIFIED.)
GEOMETRIC_REPRESENTATION_ITEM()
RATIONAL_B_SPLINE_SURFACE(((0.989812124691679,0.992466718773227,0.998122319569323,
0.998122319569323,0.998122319569323),(0.989812124691679,0.992466718773227,
0.998122319569323,0.998122319569323,0.998122319569323)))
REPRESENTATION_ITEM('')
SURFACE()
);
#2005=(
BOUNDED_SURFACE()
B_SPLINE_SURFACE(1,2,((#128152,#128153,#128154),(#128155,#128156,#128157)),
 .UNSPECIFIED.,.F.,.F.,.F.)
B_SPLINE_SURFACE_WITH_KNOTS((2,2),(3,3),(0.,0.289807040993074),(0.52191752982614,
0.539102123117534),.UNSPECIFIED.)
GEOMETRIC_REPRESENTATION_ITEM()
RATIONAL_B_SPLINE_SURFACE(((0.989334769731189,0.987004571835916,0.987576759359605),
(0.989334769731189,0.987004571835916,0.987576759359605)))
REPRESENTATION_ITEM('')
SURFACE()
);
#2006=(
BOUNDED_SURFACE()
B_SPLINE_SURFACE(1,2,((#128159,#128160,#128161,#128162,#128163),(#128164,
#128165,#128166,#128167,#128168)),.UNSPECIFIED.,.F.,.F.,.F.)
B_SPLINE_SURFACE_WITH_KNOTS((2,2),(3,2,3),(0.,0.290289290019312),(0.194028469417326,
0.211502584834065,0.212110790656298),.UNSPECIFIED.)
GEOMETRIC_REPRESENTATION_ITEM()
RATIONAL_B_SPLINE_SURFACE(((0.989812124691679,0.992466718773227,0.998122319569323,
0.998122319569323,0.998122319569323),(0.989812124691679,0.992466718773227,
0.998122319569323,0.998122319569323,0.998122319569323)))
REPRESENTATION_ITEM('')
SURFACE()
);
#2007=(
BOUNDED_SURFACE()
B_SPLINE_SURFACE(1,2,((#128177,#128178,#128179),(#128180,#128181,#128182)),
 .UNSPECIFIED.,.F.,.F.,.F.)
B_SPLINE_SURFACE_WITH_KNOTS((2,2),(3,3),(0.,0.289807040992569),(0.521917529826141,
0.539102123117534),.UNSPECIFIED.)
GEOMETRIC_REPRESENTATION_ITEM()
RATIONAL_B_SPLINE_SURFACE(((0.989334769731189,0.987004571835916,0.987576759359605),
(0.989334769731189,0.987004571835916,0.987576759359605)))
REPRESENTATION_ITEM('')
SURFACE()
);
#2008=(
BOUNDED_SURFACE()
B_SPLINE_SURFACE(1,2,((#128184,#128185,#128186,#128187,#128188),(#128189,
#128190,#128191,#128192,#128193)),.UNSPECIFIED.,.F.,.F.,.F.)
B_SPLINE_SURFACE_WITH_KNOTS((2,2),(3,2,3),(0.,0.290289290020932),(0.194028469417325,
0.211502584834064,0.212110790657912),.UNSPECIFIED.)
GEOMETRIC_REPRESENTATION_ITEM()
RATIONAL_B_SPLINE_SURFACE(((0.989812124691679,0.992466718773227,0.998122319569322,
0.998122319569322,0.998122319569322),(0.989812124691679,0.992466718773227,
0.998122319569322,0.998122319569323,0.998122319569323)))
REPRESENTATION_ITEM('')
SURFACE()
);
#2009=(
BOUNDED_SURFACE()
B_SPLINE_SURFACE(1,2,((#128202,#128203,#128204),(#128205,#128206,#128207)),
 .UNSPECIFIED.,.F.,.F.,.F.)
B_SPLINE_SURFACE_WITH_KNOTS((2,2),(3,3),(0.,0.289807040992568),(0.521917529826141,
0.539102123117535),.UNSPECIFIED.)
GEOMETRIC_REPRESENTATION_ITEM()
RATIONAL_B_SPLINE_SURFACE(((0.989334769731189,0.987004571835916,0.987576759359605),
(0.989334769731189,0.987004571835916,0.987576759359605)))
REPRESENTATION_ITEM('')
SURFACE()
);
#2010=(
BOUNDED_SURFACE()
B_SPLINE_SURFACE(1,2,((#128209,#128210,#128211,#128212,#128213),(#128214,
#128215,#128216,#128217,#128218)),.UNSPECIFIED.,.F.,.F.,.F.)
B_SPLINE_SURFACE_WITH_KNOTS((2,2),(3,2,3),(0.,0.290289290013028),(0.194028469417325,
0.211502584834064,0.21211079065001),.UNSPECIFIED.)
GEOMETRIC_REPRESENTATION_ITEM()
RATIONAL_B_SPLINE_SURFACE(((0.989812124691679,0.992466718773227,0.998122319569322,
0.998122319569322,0.998122319569322),(0.989812124691679,0.992466718773227,
0.998122319569322,0.998122319569322,0.998122319569322)))
REPRESENTATION_ITEM('')
SURFACE()
);
#2011=(
BOUNDED_SURFACE()
B_SPLINE_SURFACE(1,2,((#128227,#128228,#128229),(#128230,#128231,#128232)),
 .UNSPECIFIED.,.F.,.F.,.F.)
B_SPLINE_SURFACE_WITH_KNOTS((2,2),(3,3),(0.,0.289807040993163),(0.521917529826141,
0.539102123117535),.UNSPECIFIED.)
GEOMETRIC_REPRESENTATION_ITEM()
RATIONAL_B_SPLINE_SURFACE(((0.989334769731189,0.987004571835916,0.987576759359605),
(0.989334769731189,0.987004571835916,0.987576759359605)))
REPRESENTATION_ITEM('')
SURFACE()
);
#2012=(
BOUNDED_SURFACE()
B_SPLINE_SURFACE(1,2,((#128234,#128235,#128236,#128237,#128238),(#128239,
#128240,#128241,#128242,#128243)),.UNSPECIFIED.,.F.,.F.,.F.)
B_SPLINE_SURFACE_WITH_KNOTS((2,2),(3,2,3),(0.,0.290289290016891),(0.194028469417325,
0.211502584834064,0.212110790653872),.UNSPECIFIED.)
GEOMETRIC_REPRESENTATION_ITEM()
RATIONAL_B_SPLINE_SURFACE(((0.989812124691679,0.992466718773227,0.998122319569322,
0.998122319569322,0.998122319569322),(0.989812124691679,0.992466718773227,
0.998122319569322,0.998122319569322,0.998122319569322)))
REPRESENTATION_ITEM('')
SURFACE()
);
#2013=(
BOUNDED_SURFACE()
B_SPLINE_SURFACE(1,2,((#128252,#128253,#128254),(#128255,#128256,#128257)),
 .UNSPECIFIED.,.F.,.F.,.F.)
B_SPLINE_SURFACE_WITH_KNOTS((2,2),(3,3),(0.,0.289807040992575),(0.521917529826141,
0.539102123117535),.UNSPECIFIED.)
GEOMETRIC_REPRESENTATION_ITEM()
RATIONAL_B_SPLINE_SURFACE(((0.989334769731189,0.987004571835916,0.987576759359605),
(0.989334769731189,0.987004571835916,0.987576759359605)))
REPRESENTATION_ITEM('')
SURFACE()
);
#2014=(
BOUNDED_SURFACE()
B_SPLINE_SURFACE(1,2,((#128259,#128260,#128261,#128262,#128263),(#128264,
#128265,#128266,#128267,#128268)),.UNSPECIFIED.,.F.,.F.,.F.)
B_SPLINE_SURFACE_WITH_KNOTS((2,2),(3,2,3),(0.,0.290289290007279),(0.194028469417325,
0.211502584834064,0.21211079064426),.UNSPECIFIED.)
GEOMETRIC_REPRESENTATION_ITEM()
RATIONAL_B_SPLINE_SURFACE(((0.989812124691679,0.992466718773227,0.998122319569322,
0.998122319569322,0.998122319569322),(0.989812124691679,0.992466718773227,
0.998122319569322,0.998122319569322,0.998122319569322)))
REPRESENTATION_ITEM('')
SURFACE()
);
#2015=(
BOUNDED_SURFACE()
B_SPLINE_SURFACE(1,2,((#128277,#128278,#128279),(#128280,#128281,#128282)),
 .UNSPECIFIED.,.F.,.F.,.F.)
B_SPLINE_SURFACE_WITH_KNOTS((2,2),(3,3),(0.,0.289807040993073),(0.521917529826141,
0.539102123117535),.UNSPECIFIED.)
GEOMETRIC_REPRESENTATION_ITEM()
RATIONAL_B_SPLINE_SURFACE(((0.989334769731189,0.987004571835916,0.987576759359605),
(0.989334769731189,0.987004571835916,0.987576759359605)))
REPRESENTATION_ITEM('')
SURFACE()
);
#2016=(
BOUNDED_SURFACE()
B_SPLINE_SURFACE(1,2,((#128284,#128285,#128286,#128287,#128288),(#128289,
#128290,#128291,#128292,#128293)),.UNSPECIFIED.,.F.,.F.,.F.)
B_SPLINE_SURFACE_WITH_KNOTS((2,2),(3,2,3),(0.,0.290289290012074),(0.194028469417325,
0.211502584834064,0.212110790649057),.UNSPECIFIED.)
GEOMETRIC_REPRESENTATION_ITEM()
RATIONAL_B_SPLINE_SURFACE(((0.989812124691679,0.992466718773227,0.998122319569322,
0.998122319569322,0.998122319569322),(0.989812124691679,0.992466718773227,
0.998122319569322,0.998122319569322,0.998122319569322)))
REPRESENTATION_ITEM('')
SURFACE()
);
#2017=(
BOUNDED_SURFACE()
B_SPLINE_SURFACE(1,2,((#128302,#128303,#128304),(#128305,#128306,#128307)),
 .UNSPECIFIED.,.F.,.F.,.F.)
B_SPLINE_SURFACE_WITH_KNOTS((2,2),(3,3),(0.,0.289807040992579),(0.521917529826141,
0.539102123117535),.UNSPECIFIED.)
GEOMETRIC_REPRESENTATION_ITEM()
RATIONAL_B_SPLINE_SURFACE(((0.989334769731189,0.987004571835916,0.987576759359605),
(0.989334769731189,0.987004571835916,0.987576759359605)))
REPRESENTATION_ITEM('')
SURFACE()
);
#2018=(
BOUNDED_SURFACE()
B_SPLINE_SURFACE(1,2,((#128309,#128310,#128311,#128312,#128313),(#128314,
#128315,#128316,#128317,#128318)),.UNSPECIFIED.,.F.,.F.,.F.)
B_SPLINE_SURFACE_WITH_KNOTS((2,2),(3,2,3),(0.,0.290289290013357),(0.194028469417325,
0.211502584834064,0.212110790650338),.UNSPECIFIED.)
GEOMETRIC_REPRESENTATION_ITEM()
RATIONAL_B_SPLINE_SURFACE(((0.989812124691679,0.992466718773227,0.998122319569322,
0.998122319569322,0.998122319569322),(0.989812124691679,0.992466718773227,
0.998122319569322,0.998122319569322,0.998122319569322)))
REPRESENTATION_ITEM('')
SURFACE()
);
#2019=(
BOUNDED_SURFACE()
B_SPLINE_SURFACE(1,2,((#128327,#128328,#128329),(#128330,#128331,#128332)),
 .UNSPECIFIED.,.F.,.F.,.F.)
B_SPLINE_SURFACE_WITH_KNOTS((2,2),(3,3),(0.,0.289807040993077),(0.521917529826141,
0.539102123117535),.UNSPECIFIED.)
GEOMETRIC_REPRESENTATION_ITEM()
RATIONAL_B_SPLINE_SURFACE(((0.989334769731189,0.987004571835916,0.987576759359605),
(0.989334769731189,0.987004571835916,0.987576759359605)))
REPRESENTATION_ITEM('')
SURFACE()
);
#2020=(
BOUNDED_SURFACE()
B_SPLINE_SURFACE(1,2,((#128334,#128335,#128336,#128337,#128338),(#128339,
#128340,#128341,#128342,#128343)),.UNSPECIFIED.,.F.,.F.,.F.)
B_SPLINE_SURFACE_WITH_KNOTS((2,2),(3,2,3),(0.,0.290289290017703),(0.194028469417325,
0.211502584834064,0.212110790654683),.UNSPECIFIED.)
GEOMETRIC_REPRESENTATION_ITEM()
RATIONAL_B_SPLINE_SURFACE(((0.989812124691679,0.992466718773227,0.998122319569322,
0.998122319569322,0.998122319569322),(0.989812124691679,0.992466718773227,
0.998122319569322,0.998122319569322,0.998122319569322)))
REPRESENTATION_ITEM('')
SURFACE()
);
#2021=(
BOUNDED_SURFACE()
B_SPLINE_SURFACE(1,2,((#128352,#128353,#128354),(#128355,#128356,#128357)),
 .UNSPECIFIED.,.F.,.F.,.F.)
B_SPLINE_SURFACE_WITH_KNOTS((2,2),(3,3),(0.,0.289807040992847),(0.521917529826141,
0.539102123117535),.UNSPECIFIED.)
GEOMETRIC_REPRESENTATION_ITEM()
RATIONAL_B_SPLINE_SURFACE(((0.989334769731189,0.987004571835916,0.987576759359605),
(0.989334769731189,0.987004571835916,0.987576759359605)))
REPRESENTATION_ITEM('')
SURFACE()
);
#2022=(
BOUNDED_SURFACE()
B_SPLINE_SURFACE(1,2,((#128359,#128360,#128361,#128362,#128363),(#128364,
#128365,#128366,#128367,#128368)),.UNSPECIFIED.,.F.,.F.,.F.)
B_SPLINE_SURFACE_WITH_KNOTS((2,2),(3,2,3),(0.,0.290289290035709),(0.194028469417325,
0.211502584834064,0.212110790672689),.UNSPECIFIED.)
GEOMETRIC_REPRESENTATION_ITEM()
RATIONAL_B_SPLINE_SURFACE(((0.989812124691679,0.992466718773227,0.998122319569322,
0.998122319569322,0.998122319569322),(0.989812124691679,0.992466718773227,
0.998122319569322,0.998122319569322,0.998122319569322)))
REPRESENTATION_ITEM('')
SURFACE()
);
#2023=(
BOUNDED_SURFACE()
B_SPLINE_SURFACE(1,2,((#128377,#128378,#128379),(#128380,#128381,#128382)),
 .UNSPECIFIED.,.F.,.F.,.F.)
B_SPLINE_SURFACE_WITH_KNOTS((2,2),(3,3),(0.,0.289807040993896),(0.521917529826141,
0.539102123117535),.UNSPECIFIED.)
GEOMETRIC_REPRESENTATION_ITEM()
RATIONAL_B_SPLINE_SURFACE(((0.989334769731189,0.987004571835916,0.987576759359605),
(0.989334769731189,0.987004571835916,0.987576759359605)))
REPRESENTATION_ITEM('')
SURFACE()
);
#2024=(
BOUNDED_SURFACE()
B_SPLINE_SURFACE(1,2,((#128384,#128385,#128386,#128387,#128388),(#128389,
#128390,#128391,#128392,#128393)),.UNSPECIFIED.,.F.,.F.,.F.)
B_SPLINE_SURFACE_WITH_KNOTS((2,2),(3,2,3),(0.,0.290289290042823),(0.194028469417325,
0.211502584834064,0.212110790679806),.UNSPECIFIED.)
GEOMETRIC_REPRESENTATION_ITEM()
RATIONAL_B_SPLINE_SURFACE(((0.989812124691679,0.992466718773227,0.998122319569322,
0.998122319569322,0.998122319569322),(0.989812124691679,0.992466718773227,
0.998122319569322,0.998122319569322,0.998122319569322)))
REPRESENTATION_ITEM('')
SURFACE()
);
#2025=(
BOUNDED_SURFACE()
B_SPLINE_SURFACE(1,2,((#128402,#128403,#128404),(#128405,#128406,#128407)),
 .UNSPECIFIED.,.F.,.F.,.F.)
B_SPLINE_SURFACE_WITH_KNOTS((2,2),(3,3),(0.,0.289807040992612),(0.521917529826139,
0.539102123117535),.UNSPECIFIED.)
GEOMETRIC_REPRESENTATION_ITEM()
RATIONAL_B_SPLINE_SURFACE(((0.989334769731189,0.987004571835916,0.987576759359605),
(0.989334769731189,0.987004571835916,0.987576759359605)))
REPRESENTATION_ITEM('')
SURFACE()
);
#2026=(
BOUNDED_SURFACE()
B_SPLINE_SURFACE(1,2,((#128409,#128410,#128411,#128412,#128413),(#128414,
#128415,#128416,#128417,#128418)),.UNSPECIFIED.,.F.,.F.,.F.)
B_SPLINE_SURFACE_WITH_KNOTS((2,2),(3,2,3),(0.,0.290289290028364),(0.194028469417325,
0.211502584834064,0.212110790665341),.UNSPECIFIED.)
GEOMETRIC_REPRESENTATION_ITEM()
RATIONAL_B_SPLINE_SURFACE(((0.989812124691679,0.992466718773227,0.998122319569322,
0.998122319569322,0.998122319569322),(0.989812124691679,0.992466718773227,
0.998122319569322,0.998122319569322,0.998122319569322)))
REPRESENTATION_ITEM('')
SURFACE()
);
#2027=(
BOUNDED_SURFACE()
B_SPLINE_SURFACE(1,2,((#128427,#128428,#128429),(#128430,#128431,#128432)),
 .UNSPECIFIED.,.F.,.F.,.F.)
B_SPLINE_SURFACE_WITH_KNOTS((2,2),(3,3),(0.,0.289807040992501),(0.521917529826141,
0.539102123117535),.UNSPECIFIED.)
GEOMETRIC_REPRESENTATION_ITEM()
RATIONAL_B_SPLINE_SURFACE(((0.989334769731189,0.987004571835916,0.987576759359605),
(0.989334769731189,0.987004571835916,0.987576759359605)))
REPRESENTATION_ITEM('')
SURFACE()
);
#2028=(
BOUNDED_SURFACE()
B_SPLINE_SURFACE(1,2,((#128434,#128435,#128436,#128437,#128438),(#128439,
#128440,#128441,#128442,#128443)),.UNSPECIFIED.,.F.,.F.,.F.)
B_SPLINE_SURFACE_WITH_KNOTS((2,2),(3,2,3),(0.,0.290289290031972),(0.194028469417325,
0.211502584834065,0.212110790668951),.UNSPECIFIED.)
GEOMETRIC_REPRESENTATION_ITEM()
RATIONAL_B_SPLINE_SURFACE(((0.989812124691679,0.992466718773227,0.998122319569322,
0.998122319569322,0.998122319569322),(0.989812124691679,0.992466718773227,
0.998122319569322,0.998122319569322,0.998122319569322)))
REPRESENTATION_ITEM('')
SURFACE()
);
#2029=(
BOUNDED_SURFACE()
B_SPLINE_SURFACE(1,2,((#128452,#128453,#128454),(#128455,#128456,#128457)),
 .UNSPECIFIED.,.F.,.F.,.F.)
B_SPLINE_SURFACE_WITH_KNOTS((2,2),(3,3),(0.,0.289807040993131),(0.521917529826141,
0.539102123117535),.UNSPECIFIED.)
GEOMETRIC_REPRESENTATION_ITEM()
RATIONAL_B_SPLINE_SURFACE(((0.989334769731189,0.987004571835916,0.987576759359605),
(0.989334769731189,0.987004571835916,0.987576759359605)))
REPRESENTATION_ITEM('')
SURFACE()
);
#2030=(
BOUNDED_SURFACE()
B_SPLINE_SURFACE(1,2,((#128459,#128460,#128461,#128462,#128463),(#128464,
#128465,#128466,#128467,#128468)),.UNSPECIFIED.,.F.,.F.,.F.)
B_SPLINE_SURFACE_WITH_KNOTS((2,2),(3,2,3),(0.,0.290289290001602),(0.194028469417325,
0.211502584834064,0.212110790638577),.UNSPECIFIED.)
GEOMETRIC_REPRESENTATION_ITEM()
RATIONAL_B_SPLINE_SURFACE(((0.989812124691679,0.992466718773227,0.998122319569322,
0.998122319569322,0.998122319569322),(0.989812124691679,0.992466718773227,
0.998122319569322,0.998122319569322,0.998122319569322)))
REPRESENTATION_ITEM('')
SURFACE()
);
#2031=(
BOUNDED_SURFACE()
B_SPLINE_SURFACE(1,2,((#128477,#128478,#128479),(#128480,#128481,#128482)),
 .UNSPECIFIED.,.F.,.F.,.F.)
B_SPLINE_SURFACE_WITH_KNOTS((2,2),(3,3),(0.,0.289807040991728),(0.52191752982614,
0.539102123117535),.UNSPECIFIED.)
GEOMETRIC_REPRESENTATION_ITEM()
RATIONAL_B_SPLINE_SURFACE(((0.989334769731189,0.987004571835916,0.987576759359605),
(0.989334769731189,0.987004571835916,0.987576759359605)))
REPRESENTATION_ITEM('')
SURFACE()
);
#2032=(
BOUNDED_SURFACE()
B_SPLINE_SURFACE(1,2,((#128484,#128485,#128486,#128487,#128488),(#128489,
#128490,#128491,#128492,#128493)),.UNSPECIFIED.,.F.,.F.,.F.)
B_SPLINE_SURFACE_WITH_KNOTS((2,2),(3,2,3),(0.,0.290289290017461),(0.194028469417325,
0.211502584834064,0.212110790654441),.UNSPECIFIED.)
GEOMETRIC_REPRESENTATION_ITEM()
RATIONAL_B_SPLINE_SURFACE(((0.989812124691679,0.992466718773227,0.998122319569322,
0.998122319569322,0.998122319569322),(0.989812124691679,0.992466718773227,
0.998122319569322,0.998122319569323,0.998122319569323)))
REPRESENTATION_ITEM('')
SURFACE()
);
#2033=(
BOUNDED_SURFACE()
B_SPLINE_SURFACE(1,2,((#128502,#128503,#128504),(#128505,#128506,#128507)),
 .UNSPECIFIED.,.F.,.F.,.F.)
B_SPLINE_SURFACE_WITH_KNOTS((2,2),(3,3),(0.,0.289807040992881),(0.521917529826137,
0.539102123117536),.UNSPECIFIED.)
GEOMETRIC_REPRESENTATION_ITEM()
RATIONAL_B_SPLINE_SURFACE(((0.98933476973119,0.987004571835915,0.987576759359605),
(0.98933476973119,0.987004571835915,0.987576759359605)))
REPRESENTATION_ITEM('')
SURFACE()
);
#2034=(
BOUNDED_SURFACE()
B_SPLINE_SURFACE(1,2,((#128509,#128510,#128511,#128512,#128513),(#128514,
#128515,#128516,#128517,#128518)),.UNSPECIFIED.,.F.,.F.,.F.)
B_SPLINE_SURFACE_WITH_KNOTS((2,2),(3,2,3),(0.,0.289948761105454),(0.194028469417325,
0.211502584834065,0.211770261742427),.UNSPECIFIED.)
GEOMETRIC_REPRESENTATION_ITEM()
RATIONAL_B_SPLINE_SURFACE(((0.989812124691679,0.992466718773227,0.998122319569323,
0.998122319569323,0.998122319569323),(0.989812124691679,0.992466718773227,
0.998122319569323,0.998122319569323,0.998122319569323)))
REPRESENTATION_ITEM('')
SURFACE()
);
#2035=(
BOUNDED_SURFACE()
B_SPLINE_SURFACE(1,2,((#128527,#128528,#128529),(#128530,#128531,#128532)),
 .UNSPECIFIED.,.F.,.F.,.F.)
B_SPLINE_SURFACE_WITH_KNOTS((2,2),(3,3),(0.,0.289807040992693),(0.521917529826141,
0.539102123117535),.UNSPECIFIED.)
GEOMETRIC_REPRESENTATION_ITEM()
RATIONAL_B_SPLINE_SURFACE(((0.989334769731189,0.987004571835916,0.987576759359605),
(0.989334769731189,0.987004571835916,0.987576759359605)))
REPRESENTATION_ITEM('')
SURFACE()
);
#2036=(
BOUNDED_SURFACE()
B_SPLINE_SURFACE(1,2,((#128534,#128535,#128536,#128537,#128538),(#128539,
#128540,#128541,#128542,#128543)),.UNSPECIFIED.,.F.,.F.,.F.)
B_SPLINE_SURFACE_WITH_KNOTS((2,2),(3,2,3),(0.,0.290289290033966),(0.194028469417325,
0.211502584834065,0.212110790670942),.UNSPECIFIED.)
GEOMETRIC_REPRESENTATION_ITEM()
RATIONAL_B_SPLINE_SURFACE(((0.989812124691679,0.992466718773227,0.998122319569322,
0.998122319569322,0.998122319569322),(0.989812124691679,0.992466718773227,
0.998122319569322,0.998122319569322,0.998122319569322)))
REPRESENTATION_ITEM('')
SURFACE()
);
#2037=(
BOUNDED_SURFACE()
B_SPLINE_SURFACE(1,2,((#128552,#128553,#128554),(#128555,#128556,#128557)),
 .UNSPECIFIED.,.F.,.F.,.F.)
B_SPLINE_SURFACE_WITH_KNOTS((2,2),(3,3),(0.,0.289807040993739),(0.521917529826141,
0.539102123117535),.UNSPECIFIED.)
GEOMETRIC_REPRESENTATION_ITEM()
RATIONAL_B_SPLINE_SURFACE(((0.989334769731189,0.987004571835916,0.987576759359605),
(0.989334769731189,0.987004571835916,0.987576759359605)))
REPRESENTATION_ITEM('')
SURFACE()
);
#2038=(
BOUNDED_SURFACE()
B_SPLINE_SURFACE(1,2,((#128559,#128560,#128561,#128562,#128563),(#128564,
#128565,#128566,#128567,#128568)),.UNSPECIFIED.,.F.,.F.,.F.)
B_SPLINE_SURFACE_WITH_KNOTS((2,2),(3,2,3),(0.,0.290289290019958),(0.194028469417325,
0.211502584834064,0.212110790656939),.UNSPECIFIED.)
GEOMETRIC_REPRESENTATION_ITEM()
RATIONAL_B_SPLINE_SURFACE(((0.989812124691679,0.992466718773227,0.998122319569322,
0.998122319569322,0.998122319569322),(0.989812124691679,0.992466718773227,
0.998122319569322,0.998122319569323,0.998122319569323)))
REPRESENTATION_ITEM('')
SURFACE()
);
#2039=(
BOUNDED_SURFACE()
B_SPLINE_SURFACE(1,2,((#128577,#128578,#128579),(#128580,#128581,#128582)),
 .UNSPECIFIED.,.F.,.F.,.F.)
B_SPLINE_SURFACE_WITH_KNOTS((2,2),(3,3),(0.,0.289807040991906),(0.521917529826141,
0.539102123117535),.UNSPECIFIED.)
GEOMETRIC_REPRESENTATION_ITEM()
RATIONAL_B_SPLINE_SURFACE(((0.989334769731189,0.987004571835916,0.987576759359605),
(0.989334769731189,0.987004571835916,0.987576759359605)))
REPRESENTATION_ITEM('')
SURFACE()
);
#2040=(
BOUNDED_SURFACE()
B_SPLINE_SURFACE(1,2,((#128584,#128585,#128586,#128587,#128588),(#128589,
#128590,#128591,#128592,#128593)),.UNSPECIFIED.,.F.,.F.,.F.)
B_SPLINE_SURFACE_WITH_KNOTS((2,2),(3,2,3),(0.,0.290289290009697),(0.194028469417325,
0.211502584834064,0.212110790646677),.UNSPECIFIED.)
GEOMETRIC_REPRESENTATION_ITEM()
RATIONAL_B_SPLINE_SURFACE(((0.989812124691679,0.992466718773227,0.998122319569322,
0.998122319569322,0.998122319569322),(0.989812124691679,0.992466718773227,
0.998122319569322,0.998122319569322,0.998122319569322)))
REPRESENTATION_ITEM('')
SURFACE()
);
#2041=(
BOUNDED_SURFACE()
B_SPLINE_SURFACE(1,2,((#128602,#128603,#128604),(#128605,#128606,#128607)),
 .UNSPECIFIED.,.F.,.F.,.F.)
B_SPLINE_SURFACE_WITH_KNOTS((2,2),(3,3),(0.,0.289807040993054),(0.521917529826141,
0.539102123117535),.UNSPECIFIED.)
GEOMETRIC_REPRESENTATION_ITEM()
RATIONAL_B_SPLINE_SURFACE(((0.989334769731189,0.987004571835916,0.987576759359605),
(0.989334769731189,0.987004571835916,0.987576759359605)))
REPRESENTATION_ITEM('')
SURFACE()
);
#2042=(
BOUNDED_SURFACE()
B_SPLINE_SURFACE(1,2,((#128609,#128610,#128611,#128612,#128613),(#128614,
#128615,#128616,#128617,#128618)),.UNSPECIFIED.,.F.,.F.,.F.)
B_SPLINE_SURFACE_WITH_KNOTS((2,2),(3,2,3),(0.,0.29028929002793),(0.194028469417325,
0.211502584834064,0.212110790664903),.UNSPECIFIED.)
GEOMETRIC_REPRESENTATION_ITEM()
RATIONAL_B_SPLINE_SURFACE(((0.989812124691679,0.992466718773227,0.998122319569322,
0.998122319569322,0.998122319569322),(0.989812124691679,0.992466718773227,
0.998122319569322,0.998122319569323,0.998122319569323)))
REPRESENTATION_ITEM('')
SURFACE()
);
#2043=(
BOUNDED_SURFACE()
B_SPLINE_SURFACE(1,2,((#128627,#128628,#128629),(#128630,#128631,#128632)),
 .UNSPECIFIED.,.F.,.F.,.F.)
B_SPLINE_SURFACE_WITH_KNOTS((2,2),(3,3),(0.,0.289807040992803),(0.521917529826141,
0.539102123117535),.UNSPECIFIED.)
GEOMETRIC_REPRESENTATION_ITEM()
RATIONAL_B_SPLINE_SURFACE(((0.989334769731189,0.987004571835916,0.987576759359605),
(0.989334769731189,0.987004571835916,0.987576759359605)))
REPRESENTATION_ITEM('')
SURFACE()
);
#2044=(
BOUNDED_SURFACE()
B_SPLINE_SURFACE(1,2,((#128634,#128635,#128636,#128637,#128638),(#128639,
#128640,#128641,#128642,#128643)),.UNSPECIFIED.,.F.,.F.,.F.)
B_SPLINE_SURFACE_WITH_KNOTS((2,2),(3,2,3),(0.,0.290289290034783),(0.194028469417325,
0.211502584834064,0.212110790671746),.UNSPECIFIED.)
GEOMETRIC_REPRESENTATION_ITEM()
RATIONAL_B_SPLINE_SURFACE(((0.989812124691679,0.992466718773227,0.998122319569322,
0.998122319569322,0.998122319569322),(0.989812124691679,0.992466718773227,
0.998122319569322,0.998122319569322,0.998122319569322)))
REPRESENTATION_ITEM('')
SURFACE()
);
#2045=(
BOUNDED_SURFACE()
B_SPLINE_SURFACE(1,2,((#128652,#128653,#128654),(#128655,#128656,#128657)),
 .UNSPECIFIED.,.F.,.F.,.F.)
B_SPLINE_SURFACE_WITH_KNOTS((2,2),(3,3),(0.,0.289807040993645),(0.521917529826128,
0.539102123117535),.UNSPECIFIED.)
GEOMETRIC_REPRESENTATION_ITEM()
RATIONAL_B_SPLINE_SURFACE(((0.989334769731192,0.987004571835915,0.987576759359605),
(0.989334769731192,0.987004571835915,0.987576759359605)))
REPRESENTATION_ITEM('')
SURFACE()
);
#2046=(
BOUNDED_SURFACE()
B_SPLINE_SURFACE(1,2,((#128659,#128660,#128661,#128662,#128663),(#128664,
#128665,#128666,#128667,#128668)),.UNSPECIFIED.,.F.,.F.,.F.)
B_SPLINE_SURFACE_WITH_KNOTS((2,2),(3,2,3),(0.,0.290289290037585),(0.194028469417326,
0.211502584834064,0.212110790674559),.UNSPECIFIED.)
GEOMETRIC_REPRESENTATION_ITEM()
RATIONAL_B_SPLINE_SURFACE(((0.989812124691679,0.992466718773227,0.998122319569322,
0.998122319569322,0.998122319569322),(0.989812124691679,0.992466718773227,
0.998122319569322,0.998122319569322,0.998122319569322)))
REPRESENTATION_ITEM('')
SURFACE()
);
#2047=(
BOUNDED_SURFACE()
B_SPLINE_SURFACE(1,2,((#128677,#128678,#128679),(#128680,#128681,#128682)),
 .UNSPECIFIED.,.F.,.F.,.F.)
B_SPLINE_SURFACE_WITH_KNOTS((2,2),(3,3),(0.,0.28980704099156),(0.52191752982614,
0.539102123117534),.UNSPECIFIED.)
GEOMETRIC_REPRESENTATION_ITEM()
RATIONAL_B_SPLINE_SURFACE(((0.989334769731189,0.987004571835916,0.987576759359605),
(0.989334769731189,0.987004571835916,0.987576759359605)))
REPRESENTATION_ITEM('')
SURFACE()
);
#2048=(
BOUNDED_SURFACE()
B_SPLINE_SURFACE(1,2,((#128684,#128685,#128686,#128687,#128688),(#128689,
#128690,#128691,#128692,#128693)),.UNSPECIFIED.,.F.,.F.,.F.)
B_SPLINE_SURFACE_WITH_KNOTS((2,2),(3,2,3),(0.,0.290289290026043),(0.194028469417326,
0.211502584834066,0.21211079066303),.UNSPECIFIED.)
GEOMETRIC_REPRESENTATION_ITEM()
RATIONAL_B_SPLINE_SURFACE(((0.989812124691679,0.992466718773227,0.998122319569323,
0.998122319569323,0.998122319569323),(0.989812124691679,0.992466718773227,
0.998122319569323,0.998122319569323,0.998122319569323)))
REPRESENTATION_ITEM('')
SURFACE()
);
#2049=(
BOUNDED_SURFACE()
B_SPLINE_SURFACE(1,2,((#128702,#128703,#128704),(#128705,#128706,#128707)),
 .UNSPECIFIED.,.F.,.F.,.F.)
B_SPLINE_SURFACE_WITH_KNOTS((2,2),(3,3),(0.,0.289807040991556),(0.52191752982614,
0.539102123117534),.UNSPECIFIED.)
GEOMETRIC_REPRESENTATION_ITEM()
RATIONAL_B_SPLINE_SURFACE(((0.989334769731189,0.987004571835916,0.987576759359605),
(0.989334769731189,0.987004571835916,0.987576759359605)))
REPRESENTATION_ITEM('')
SURFACE()
);
#2050=(
BOUNDED_SURFACE()
B_SPLINE_SURFACE(1,2,((#128709,#128710,#128711,#128712,#128713),(#128714,
#128715,#128716,#128717,#128718)),.UNSPECIFIED.,.F.,.F.,.F.)
B_SPLINE_SURFACE_WITH_KNOTS((2,2),(3,2,3),(0.,0.289681084359917),(0.469916319328034,
0.487259899888159,0.48743333569376),.UNSPECIFIED.)
GEOMETRIC_REPRESENTATION_ITEM()
RATIONAL_B_SPLINE_SURFACE(((0.987775548376701,0.988735325500096,0.992651440660746,
0.992651440660746,0.992651440660746),(0.987775548376701,0.988735325500096,
0.992651440660745,0.992651440660745,0.992651440660745)))
REPRESENTATION_ITEM('')
SURFACE()
);
#2051=(
BOUNDED_SURFACE()
B_SPLINE_SURFACE(1,2,((#128729,#128730,#128731,#128732,#128733),(#128734,
#128735,#128736,#128737,#128738)),.UNSPECIFIED.,.F.,.F.,.F.)
B_SPLINE_SURFACE_WITH_KNOTS((2,2),(3,2,3),(0.,0.290401167136834),(0.245359924934102,
0.245954053070908,0.263201868951011),.UNSPECIFIED.)
GEOMETRIC_REPRESENTATION_ITEM()
RATIONAL_B_SPLINE_SURFACE(((0.987624841600687,0.987624841600687,0.987624841600687,
0.986938988894508,0.989176916802451),(0.987624841600687,0.987624841600687,
0.987624841600687,0.986938988894508,0.989176916802451)))
REPRESENTATION_ITEM('')
SURFACE()
);
#2052=(
BOUNDED_SURFACE()
B_SPLINE_SURFACE(1,2,((#128755,#128756,#128757,#128758,#128759),(#128760,
#128761,#128762,#128763,#128764)),.UNSPECIFIED.,.F.,.F.,.F.)
B_SPLINE_SURFACE_WITH_KNOTS((2,2),(3,2,3),(0.,0.289681084359941),(0.469916319328034,
0.487259899888159,0.48743333569376),.UNSPECIFIED.)
GEOMETRIC_REPRESENTATION_ITEM()
RATIONAL_B_SPLINE_SURFACE(((0.987775548376701,0.988735325500096,0.992651440660746,
0.992651440660746,0.992651440660746),(0.987775548376701,0.988735325500096,
0.992651440660746,0.992651440660746,0.992651440660746)))
REPRESENTATION_ITEM('')
SURFACE()
);
#2053=(
BOUNDED_SURFACE()
B_SPLINE_SURFACE(1,2,((#128766,#128767,#128768,#128769,#128770),(#128771,
#128772,#128773,#128774,#128775)),.UNSPECIFIED.,.F.,.F.,.F.)
B_SPLINE_SURFACE_WITH_KNOTS((2,2),(3,2,3),(0.,0.290401167093823),(0.245359924977154,
0.245954053070908,0.263201868951011),.UNSPECIFIED.)
GEOMETRIC_REPRESENTATION_ITEM()
RATIONAL_B_SPLINE_SURFACE(((0.987624841600687,0.987624841600687,0.987624841600687,
0.986938988894508,0.989176916802451),(0.987624841600687,0.987624841600687,
0.987624841600687,0.986938988894508,0.989176916802451)))
REPRESENTATION_ITEM('')
SURFACE()
);
#2054=(
BOUNDED_SURFACE()
B_SPLINE_SURFACE(1,2,((#128792,#128793,#128794,#128795,#128796),(#128797,
#128798,#128799,#128800,#128801)),.UNSPECIFIED.,.F.,.F.,.F.)
B_SPLINE_SURFACE_WITH_KNOTS((2,2),(3,2,3),(0.,0.289681084359923),(0.469916319328034,
0.487259899888159,0.48743333569376),.UNSPECIFIED.)
GEOMETRIC_REPRESENTATION_ITEM()
RATIONAL_B_SPLINE_SURFACE(((0.987775548376701,0.988735325500096,0.992651440660746,
0.992651440660746,0.992651440660746),(0.987775548376701,0.988735325500096,
0.992651440660746,0.992651440660746,0.992651440660746)))
REPRESENTATION_ITEM('')
SURFACE()
);
#2055=(
BOUNDED_SURFACE()
B_SPLINE_SURFACE(1,2,((#128803,#128804,#128805,#128806,#128807),(#128808,
#128809,#128810,#128811,#128812)),.UNSPECIFIED.,.F.,.F.,.F.)
B_SPLINE_SURFACE_WITH_KNOTS((2,2),(3,2,3),(0.,0.290401167129692),(0.245359924941374,
0.245954053070908,0.263201868951011),.UNSPECIFIED.)
GEOMETRIC_REPRESENTATION_ITEM()
RATIONAL_B_SPLINE_SURFACE(((0.987624841600687,0.987624841600687,0.987624841600687,
0.986938988894508,0.989176916802451),(0.987624841600687,0.987624841600687,
0.987624841600687,0.986938988894508,0.989176916802451)))
REPRESENTATION_ITEM('')
SURFACE()
);
#2056=(
BOUNDED_SURFACE()
B_SPLINE_SURFACE(1,2,((#128829,#128830,#128831,#128832,#128833),(#128834,
#128835,#128836,#128837,#128838)),.UNSPECIFIED.,.F.,.F.,.F.)
B_SPLINE_SURFACE_WITH_KNOTS((2,2),(3,2,3),(0.,0.289681084359927),(0.469916319328034,
0.487259899888159,0.48743333569376),.UNSPECIFIED.)
GEOMETRIC_REPRESENTATION_ITEM()
RATIONAL_B_SPLINE_SURFACE(((0.987775548376701,0.988735325500096,0.992651440660745,
0.992651440660745,0.992651440660745),(0.987775548376701,0.988735325500096,
0.992651440660745,0.992651440660745,0.992651440660745)))
REPRESENTATION_ITEM('')
SURFACE()
);
#2057=(
BOUNDED_SURFACE()
B_SPLINE_SURFACE(1,2,((#128840,#128841,#128842,#128843,#128844),(#128845,
#128846,#128847,#128848,#128849)),.UNSPECIFIED.,.F.,.F.,.F.)
B_SPLINE_SURFACE_WITH_KNOTS((2,2),(3,2,3),(0.,0.290401167115997),(0.245359924955159,
0.245954053070908,0.263201868951011),.UNSPECIFIED.)
GEOMETRIC_REPRESENTATION_ITEM()
RATIONAL_B_SPLINE_SURFACE(((0.987624841600687,0.987624841600687,0.987624841600687,
0.986938988894508,0.989176916802451),(0.987624841600687,0.987624841600687,
0.987624841600687,0.986938988894507,0.989176916802451)))
REPRESENTATION_ITEM('')
SURFACE()
);
#2058=(
BOUNDED_SURFACE()
B_SPLINE_SURFACE(1,2,((#128866,#128867,#128868,#128869,#128870),(#128871,
#128872,#128873,#128874,#128875)),.UNSPECIFIED.,.F.,.F.,.F.)
B_SPLINE_SURFACE_WITH_KNOTS((2,2),(3,2,3),(0.,0.289681084359927),(0.469916319328034,
0.487259899888159,0.48743333569376),.UNSPECIFIED.)
GEOMETRIC_REPRESENTATION_ITEM()
RATIONAL_B_SPLINE_SURFACE(((0.987775548376701,0.988735325500096,0.992651440660746,
0.992651440660746,0.992651440660746),(0.987775548376701,0.988735325500096,
0.992651440660746,0.992651440660746,0.992651440660746)))
REPRESENTATION_ITEM('')
SURFACE()
);
#2059=(
BOUNDED_SURFACE()
B_SPLINE_SURFACE(1,2,((#128877,#128878,#128879,#128880,#128881),(#128882,
#128883,#128884,#128885,#128886)),.UNSPECIFIED.,.F.,.F.,.F.)
B_SPLINE_SURFACE_WITH_KNOTS((2,2),(3,2,3),(0.,0.290401167122636),(0.245359924948379,
0.245954053070908,0.263201868951011),.UNSPECIFIED.)
GEOMETRIC_REPRESENTATION_ITEM()
RATIONAL_B_SPLINE_SURFACE(((0.987624841600687,0.987624841600687,0.987624841600687,
0.986938988894508,0.989176916802451),(0.987624841600687,0.987624841600687,
0.987624841600687,0.986938988894508,0.989176916802451)))
REPRESENTATION_ITEM('')
SURFACE()
);
#2060=(
BOUNDED_SURFACE()
B_SPLINE_SURFACE(1,2,((#128903,#128904,#128905,#128906,#128907),(#128908,
#128909,#128910,#128911,#128912)),.UNSPECIFIED.,.F.,.F.,.F.)
B_SPLINE_SURFACE_WITH_KNOTS((2,2),(3,2,3),(0.,0.289681084359917),(0.469916319328034,
0.487259899888159,0.48743333569376),.UNSPECIFIED.)
GEOMETRIC_REPRESENTATION_ITEM()
RATIONAL_B_SPLINE_SURFACE(((0.987775548376701,0.988735325500096,0.992651440660746,
0.992651440660746,0.992651440660746),(0.987775548376701,0.988735325500096,
0.992651440660746,0.992651440660746,0.992651440660746)))
REPRESENTATION_ITEM('')
SURFACE()
);
#2061=(
BOUNDED_SURFACE()
B_SPLINE_SURFACE(1,2,((#128914,#128915,#128916,#128917,#128918),(#128919,
#128920,#128921,#128922,#128923)),.UNSPECIFIED.,.F.,.F.,.F.)
B_SPLINE_SURFACE_WITH_KNOTS((2,2),(3,2,3),(0.,0.290401167100094),(0.245359924970891,
0.245954053070908,0.263201868951011),.UNSPECIFIED.)
GEOMETRIC_REPRESENTATION_ITEM()
RATIONAL_B_SPLINE_SURFACE(((0.987624841600687,0.987624841600687,0.987624841600687,
0.986938988894508,0.989176916802451),(0.987624841600687,0.987624841600687,
0.987624841600687,0.986938988894508,0.989176916802451)))
REPRESENTATION_ITEM('')
SURFACE()
);
#2062=(
BOUNDED_SURFACE()
B_SPLINE_SURFACE(1,2,((#128940,#128941,#128942,#128943,#128944),(#128945,
#128946,#128947,#128948,#128949)),.UNSPECIFIED.,.F.,.F.,.F.)
B_SPLINE_SURFACE_WITH_KNOTS((2,2),(3,2,3),(0.,0.289681084359919),(0.469916319328034,
0.487259899888159,0.48743333569376),.UNSPECIFIED.)
GEOMETRIC_REPRESENTATION_ITEM()
RATIONAL_B_SPLINE_SURFACE(((0.987775548376701,0.988735325500096,0.992651440660746,
0.992651440660746,0.992651440660746),(0.987775548376701,0.988735325500096,
0.992651440660746,0.992651440660746,0.992651440660746)))
REPRESENTATION_ITEM('')
SURFACE()
);
#2063=(
BOUNDED_SURFACE()
B_SPLINE_SURFACE(1,2,((#128951,#128952,#128953,#128954,#128955),(#128956,
#128957,#128958,#128959,#128960)),.UNSPECIFIED.,.F.,.F.,.F.)
B_SPLINE_SURFACE_WITH_KNOTS((2,2),(3,2,3),(0.,0.290401167107786),(0.245359924963182,
0.245954053070908,0.263201868951011),.UNSPECIFIED.)
GEOMETRIC_REPRESENTATION_ITEM()
RATIONAL_B_SPLINE_SURFACE(((0.987624841600687,0.987624841600687,0.987624841600687,
0.986938988894508,0.989176916802451),(0.987624841600687,0.987624841600687,
0.987624841600687,0.986938988894508,0.989176916802451)))
REPRESENTATION_ITEM('')
SURFACE()
);
#2064=(
BOUNDED_SURFACE()
B_SPLINE_SURFACE(1,2,((#128968,#128969,#128970,#128971,#128972),(#128973,
#128974,#128975,#128976,#128977)),.UNSPECIFIED.,.F.,.F.,.F.)
B_SPLINE_SURFACE_WITH_KNOTS((2,2),(3,2,3),(0.,0.289681084359914),(0.469916319328034,
0.487259899888159,0.48743333569376),.UNSPECIFIED.)
GEOMETRIC_REPRESENTATION_ITEM()
RATIONAL_B_SPLINE_SURFACE(((0.987775548376701,0.988735325500096,0.992651440660746,
0.992651440660746,0.992651440660746),(0.987775548376701,0.988735325500096,
0.992651440660745,0.992651440660745,0.992651440660745)))
REPRESENTATION_ITEM('')
SURFACE()
);
#2065=(
BOUNDED_SURFACE()
B_SPLINE_SURFACE(1,2,((#128979,#128980,#128981,#128982,#128983),(#128984,
#128985,#128986,#128987,#128988)),.UNSPECIFIED.,.F.,.F.,.F.)
B_SPLINE_SURFACE_WITH_KNOTS((2,2),(3,2,3),(0.,0.290401167130326),(0.245359924940621,
0.245954053070908,0.263201868951011),.UNSPECIFIED.)
GEOMETRIC_REPRESENTATION_ITEM()
RATIONAL_B_SPLINE_SURFACE(((0.987624841600687,0.987624841600687,0.987624841600687,
0.986938988894507,0.989176916802451),(0.987624841600687,0.987624841600687,
0.987624841600687,0.986938988894507,0.989176916802451)))
REPRESENTATION_ITEM('')
SURFACE()
);
#2066=(
BOUNDED_SURFACE()
B_SPLINE_SURFACE(1,2,((#129005,#129006,#129007,#129008,#129009),(#129010,
#129011,#129012,#129013,#129014)),.UNSPECIFIED.,.F.,.F.,.F.)
B_SPLINE_SURFACE_WITH_KNOTS((2,2),(3,2,3),(0.,0.289681084359921),(0.469916319328034,
0.487259899888159,0.48743333569376),.UNSPECIFIED.)
GEOMETRIC_REPRESENTATION_ITEM()
RATIONAL_B_SPLINE_SURFACE(((0.987775548376701,0.988735325500096,0.992651440660746,
0.992651440660746,0.992651440660746),(0.987775548376701,0.988735325500096,
0.992651440660746,0.992651440660746,0.992651440660746)))
REPRESENTATION_ITEM('')
SURFACE()
);
#2067=(
BOUNDED_SURFACE()
B_SPLINE_SURFACE(1,2,((#129016,#129017,#129018,#129019,#129020),(#129021,
#129022,#129023,#129024,#129025)),.UNSPECIFIED.,.F.,.F.,.F.)
B_SPLINE_SURFACE_WITH_KNOTS((2,2),(3,2,3),(0.,0.290401167111664),(0.245359924959248,
0.245954053070908,0.263201868951011),.UNSPECIFIED.)
GEOMETRIC_REPRESENTATION_ITEM()
RATIONAL_B_SPLINE_SURFACE(((0.987624841600687,0.987624841600687,0.987624841600687,
0.986938988894507,0.989176916802451),(0.987624841600687,0.987624841600687,
0.987624841600687,0.986938988894508,0.989176916802451)))
REPRESENTATION_ITEM('')
SURFACE()
);
#2068=(
BOUNDED_SURFACE()
B_SPLINE_SURFACE(1,2,((#129042,#129043,#129044,#129045,#129046),(#129047,
#129048,#129049,#129050,#129051)),.UNSPECIFIED.,.F.,.F.,.F.)
B_SPLINE_SURFACE_WITH_KNOTS((2,2),(3,2,3),(0.,0.289681084359923),(0.469916319328034,
0.487259899888159,0.48743333569376),.UNSPECIFIED.)
GEOMETRIC_REPRESENTATION_ITEM()
RATIONAL_B_SPLINE_SURFACE(((0.987775548376701,0.988735325500096,0.992651440660746,
0.992651440660746,0.992651440660746),(0.987775548376701,0.988735325500096,
0.992651440660746,0.992651440660746,0.992651440660746)))
REPRESENTATION_ITEM('')
SURFACE()
);
#2069=(
BOUNDED_SURFACE()
B_SPLINE_SURFACE(1,2,((#129053,#129054,#129055,#129056,#129057),(#129058,
#129059,#129060,#129061,#129062)),.UNSPECIFIED.,.F.,.F.,.F.)
B_SPLINE_SURFACE_WITH_KNOTS((2,2),(3,2,3),(0.,0.290401167139708),(0.245359924931369,
0.245954053070908,0.263201868951016),.UNSPECIFIED.)
GEOMETRIC_REPRESENTATION_ITEM()
RATIONAL_B_SPLINE_SURFACE(((0.987624841600687,0.987624841600687,0.987624841600687,
0.986938988894507,0.989176916802452),(0.987624841600687,0.987624841600687,
0.987624841600687,0.986938988894507,0.989176916802452)))
REPRESENTATION_ITEM('')
SURFACE()
);
#2070=(
BOUNDED_SURFACE()
B_SPLINE_SURFACE(1,2,((#129079,#129080,#129081,#129082,#129083),(#129084,
#129085,#129086,#129087,#129088)),.UNSPECIFIED.,.F.,.F.,.F.)
B_SPLINE_SURFACE_WITH_KNOTS((2,2),(3,2,3),(0.,0.289681084359925),(0.469916319328038,
0.487259899888159,0.48743333569376),.UNSPECIFIED.)
GEOMETRIC_REPRESENTATION_ITEM()
RATIONAL_B_SPLINE_SURFACE(((0.987775548376701,0.988735325500097,0.992651440660745,
0.992651440660745,0.992651440660745),(0.987775548376701,0.988735325500097,
0.992651440660745,0.992651440660745,0.992651440660745)))
REPRESENTATION_ITEM('')
SURFACE()
);
#2071=(
BOUNDED_SURFACE()
B_SPLINE_SURFACE(1,2,((#129090,#129091,#129092,#129093,#129094),(#129095,
#129096,#129097,#129098,#129099)),.UNSPECIFIED.,.F.,.F.,.F.)
B_SPLINE_SURFACE_WITH_KNOTS((2,2),(3,2,3),(0.,0.290401167093765),(0.245359924977085,
0.245954053070908,0.263201868951013),.UNSPECIFIED.)
GEOMETRIC_REPRESENTATION_ITEM()
RATIONAL_B_SPLINE_SURFACE(((0.987624841600687,0.987624841600687,0.987624841600687,
0.986938988894508,0.989176916802451),(0.987624841600687,0.987624841600687,
0.987624841600687,0.986938988894508,0.989176916802451)))
REPRESENTATION_ITEM('')
SURFACE()
);
#2072=(
BOUNDED_SURFACE()
B_SPLINE_SURFACE(1,2,((#129116,#129117,#129118,#129119,#129120),(#129121,
#129122,#129123,#129124,#129125)),.UNSPECIFIED.,.F.,.F.,.F.)
B_SPLINE_SURFACE_WITH_KNOTS((2,2),(3,2,3),(0.,0.289681084359923),(0.469916319328036,
0.487259899888159,0.48743333569376),.UNSPECIFIED.)
GEOMETRIC_REPRESENTATION_ITEM()
RATIONAL_B_SPLINE_SURFACE(((0.987775548376701,0.988735325500096,0.992651440660745,
0.992651440660745,0.992651440660745),(0.987775548376701,0.988735325500096,
0.992651440660745,0.992651440660745,0.992651440660745)))
REPRESENTATION_ITEM('')
SURFACE()
);
#2073=(
BOUNDED_SURFACE()
B_SPLINE_SURFACE(1,2,((#129127,#129128,#129129,#129130,#129131),(#129132,
#129133,#129134,#129135,#129136)),.UNSPECIFIED.,.F.,.F.,.F.)
B_SPLINE_SURFACE_WITH_KNOTS((2,2),(3,2,3),(0.,0.290401167125862),(0.245359924945024,
0.245954053070908,0.263201868951011),.UNSPECIFIED.)
GEOMETRIC_REPRESENTATION_ITEM()
RATIONAL_B_SPLINE_SURFACE(((0.987624841600687,0.987624841600687,0.987624841600687,
0.986938988894508,0.989176916802451),(0.987624841600687,0.987624841600687,
0.987624841600687,0.986938988894508,0.989176916802451)))
REPRESENTATION_ITEM('')
SURFACE()
);
#2074=(
BOUNDED_SURFACE()
B_SPLINE_SURFACE(1,2,((#129153,#129154,#129155,#129156,#129157),(#129158,
#129159,#129160,#129161,#129162)),.UNSPECIFIED.,.F.,.F.,.F.)
B_SPLINE_SURFACE_WITH_KNOTS((2,2),(3,2,3),(0.,0.289681084359923),(0.469916319328034,
0.48725989988816,0.487433335693761),.UNSPECIFIED.)
GEOMETRIC_REPRESENTATION_ITEM()
RATIONAL_B_SPLINE_SURFACE(((0.987775548376701,0.988735325500096,0.992651440660746,
0.992651440660746,0.992651440660746),(0.987775548376701,0.988735325500096,
0.992651440660746,0.992651440660746,0.992651440660746)))
REPRESENTATION_ITEM('')
SURFACE()
);
#2075=(
BOUNDED_SURFACE()
B_SPLINE_SURFACE(1,2,((#129164,#129165,#129166,#129167,#129168),(#129169,
#129170,#129171,#129172,#129173)),.UNSPECIFIED.,.F.,.F.,.F.)
B_SPLINE_SURFACE_WITH_KNOTS((2,2),(3,2,3),(0.,0.290401167139431),(0.245359924931563,
0.245954053070908,0.263201868951011),.UNSPECIFIED.)
GEOMETRIC_REPRESENTATION_ITEM()
RATIONAL_B_SPLINE_SURFACE(((0.987624841600687,0.987624841600687,0.987624841600687,
0.986938988894508,0.989176916802451),(0.987624841600687,0.987624841600687,
0.987624841600687,0.986938988894508,0.989176916802451)))
REPRESENTATION_ITEM('')
SURFACE()
);
#2076=(
BOUNDED_SURFACE()
B_SPLINE_SURFACE(1,2,((#129190,#129191,#129192,#129193,#129194),(#129195,
#129196,#129197,#129198,#129199)),.UNSPECIFIED.,.F.,.F.,.F.)
B_SPLINE_SURFACE_WITH_KNOTS((2,2),(3,2,3),(0.,0.289681084359921),(0.469916319328034,
0.487259899888159,0.48743333569376),.UNSPECIFIED.)
GEOMETRIC_REPRESENTATION_ITEM()
RATIONAL_B_SPLINE_SURFACE(((0.987775548376701,0.988735325500096,0.992651440660745,
0.992651440660745,0.992651440660745),(0.987775548376701,0.988735325500096,
0.992651440660745,0.992651440660745,0.992651440660745)))
REPRESENTATION_ITEM('')
SURFACE()
);
#2077=(
BOUNDED_SURFACE()
B_SPLINE_SURFACE(1,2,((#129201,#129202,#129203,#129204,#129205),(#129206,
#129207,#129208,#129209,#129210)),.UNSPECIFIED.,.F.,.F.,.F.)
B_SPLINE_SURFACE_WITH_KNOTS((2,2),(3,2,3),(0.,0.290401167098445),(0.245359924972439,
0.245954053070908,0.263201868951011),.UNSPECIFIED.)
GEOMETRIC_REPRESENTATION_ITEM()
RATIONAL_B_SPLINE_SURFACE(((0.987624841600687,0.987624841600687,0.987624841600687,
0.986938988894508,0.989176916802451),(0.987624841600687,0.987624841600687,
0.987624841600687,0.986938988894508,0.989176916802451)))
REPRESENTATION_ITEM('')
SURFACE()
);
#2078=(
BOUNDED_SURFACE()
B_SPLINE_SURFACE(1,2,((#129227,#129228,#129229,#129230,#129231),(#129232,
#129233,#129234,#129235,#129236)),.UNSPECIFIED.,.F.,.F.,.F.)
B_SPLINE_SURFACE_WITH_KNOTS((2,2),(3,2,3),(0.,0.289681084359924),(0.469916319328034,
0.487259899888159,0.48743333569376),.UNSPECIFIED.)
GEOMETRIC_REPRESENTATION_ITEM()
RATIONAL_B_SPLINE_SURFACE(((0.987775548376701,0.988735325500096,0.992651440660746,
0.992651440660746,0.992651440660746),(0.987775548376701,0.988735325500096,
0.992651440660746,0.992651440660746,0.992651440660746)))
REPRESENTATION_ITEM('')
SURFACE()
);
#2079=(
BOUNDED_SURFACE()
B_SPLINE_SURFACE(1,2,((#129238,#129239,#129240,#129241,#129242),(#129243,
#129244,#129245,#129246,#129247)),.UNSPECIFIED.,.F.,.F.,.F.)
B_SPLINE_SURFACE_WITH_KNOTS((2,2),(3,2,3),(0.,0.290401167125722),(0.245359924945411,
0.245954053070908,0.263201868951011),.UNSPECIFIED.)
GEOMETRIC_REPRESENTATION_ITEM()
RATIONAL_B_SPLINE_SURFACE(((0.987624841600687,0.987624841600687,0.987624841600687,
0.986938988894508,0.989176916802451),(0.987624841600687,0.987624841600687,
0.987624841600687,0.986938988894508,0.989176916802451)))
REPRESENTATION_ITEM('')
SURFACE()
);
#2080=(
BOUNDED_SURFACE()
B_SPLINE_SURFACE(1,2,((#129264,#129265,#129266,#129267,#129268),(#129269,
#129270,#129271,#129272,#129273)),.UNSPECIFIED.,.F.,.F.,.F.)
B_SPLINE_SURFACE_WITH_KNOTS((2,2),(3,2,3),(0.,0.289681084359924),(0.469916319328034,
0.48725989988816,0.487433335693761),.UNSPECIFIED.)
GEOMETRIC_REPRESENTATION_ITEM()
RATIONAL_B_SPLINE_SURFACE(((0.987775548376701,0.988735325500096,0.992651440660746,
0.992651440660746,0.992651440660746),(0.987775548376701,0.988735325500096,
0.992651440660746,0.992651440660746,0.992651440660746)))
REPRESENTATION_ITEM('')
SURFACE()
);
#2081=(
BOUNDED_SURFACE()
B_SPLINE_SURFACE(1,2,((#129275,#129276,#129277,#129278,#129279),(#129280,
#129281,#129282,#129283,#129284)),.UNSPECIFIED.,.F.,.F.,.F.)
B_SPLINE_SURFACE_WITH_KNOTS((2,2),(3,2,3),(0.,0.290401167113126),(0.24535992495785,
0.245954053070908,0.263201868951011),.UNSPECIFIED.)
GEOMETRIC_REPRESENTATION_ITEM()
RATIONAL_B_SPLINE_SURFACE(((0.987624841600687,0.987624841600687,0.987624841600687,
0.986938988894508,0.989176916802451),(0.987624841600687,0.987624841600687,
0.987624841600687,0.986938988894508,0.989176916802451)))
REPRESENTATION_ITEM('')
SURFACE()
);
#2082=(
BOUNDED_SURFACE()
B_SPLINE_SURFACE(1,2,((#129301,#129302,#129303,#129304,#129305),(#129306,
#129307,#129308,#129309,#129310)),.UNSPECIFIED.,.F.,.F.,.F.)
B_SPLINE_SURFACE_WITH_KNOTS((2,2),(3,2,3),(0.,0.289681084359923),(0.469916319328034,
0.487259899888159,0.48743333569376),.UNSPECIFIED.)
GEOMETRIC_REPRESENTATION_ITEM()
RATIONAL_B_SPLINE_SURFACE(((0.987775548376701,0.988735325500096,0.992651440660746,
0.992651440660746,0.992651440660746),(0.987775548376701,0.988735325500096,
0.992651440660746,0.992651440660746,0.992651440660746)))
REPRESENTATION_ITEM('')
SURFACE()
);
#2083=(
BOUNDED_SURFACE()
B_SPLINE_SURFACE(1,2,((#129312,#129313,#129314,#129315,#129316),(#129317,
#129318,#129319,#129320,#129321)),.UNSPECIFIED.,.F.,.F.,.F.)
B_SPLINE_SURFACE_WITH_KNOTS((2,2),(3,2,3),(0.,0.290401167145354),(0.245359924925784,
0.245954053070908,0.263201868951011),.UNSPECIFIED.)
GEOMETRIC_REPRESENTATION_ITEM()
RATIONAL_B_SPLINE_SURFACE(((0.987624841600687,0.987624841600687,0.987624841600687,
0.986938988894508,0.989176916802451),(0.987624841600687,0.987624841600687,
0.987624841600687,0.986938988894508,0.989176916802451)))
REPRESENTATION_ITEM('')
SURFACE()
);
#2084=(
BOUNDED_SURFACE()
B_SPLINE_SURFACE(1,2,((#129338,#129339,#129340,#129341,#129342),(#129343,
#129344,#129345,#129346,#129347)),.UNSPECIFIED.,.F.,.F.,.F.)
B_SPLINE_SURFACE_WITH_KNOTS((2,2),(3,2,3),(0.,0.289681084359931),(0.469916319328034,
0.487259899888159,0.48743333569376),.UNSPECIFIED.)
GEOMETRIC_REPRESENTATION_ITEM()
RATIONAL_B_SPLINE_SURFACE(((0.987775548376701,0.988735325500096,0.992651440660746,
0.992651440660746,0.992651440660746),(0.987775548376701,0.988735325500096,
0.992651440660746,0.992651440660746,0.992651440660746)))
REPRESENTATION_ITEM('')
SURFACE()
);
#2085=(
BOUNDED_SURFACE()
B_SPLINE_SURFACE(1,2,((#129349,#129350,#129351,#129352,#129353),(#129354,
#129355,#129356,#129357,#129358)),.UNSPECIFIED.,.F.,.F.,.F.)
B_SPLINE_SURFACE_WITH_KNOTS((2,2),(3,2,3),(0.,0.290401167104879),(0.245359924965993,
0.245954053070908,0.263201868951011),.UNSPECIFIED.)
GEOMETRIC_REPRESENTATION_ITEM()
RATIONAL_B_SPLINE_SURFACE(((0.987624841600687,0.987624841600687,0.987624841600687,
0.986938988894508,0.989176916802451),(0.987624841600687,0.987624841600687,
0.987624841600687,0.986938988894508,0.989176916802451)))
REPRESENTATION_ITEM('')
SURFACE()
);
#2086=(
BOUNDED_SURFACE()
B_SPLINE_SURFACE(1,2,((#129375,#129376,#129377,#129378,#129379),(#129380,
#129381,#129382,#129383,#129384)),.UNSPECIFIED.,.F.,.F.,.F.)
B_SPLINE_SURFACE_WITH_KNOTS((2,2),(3,2,3),(0.,0.289681084359923),(0.469916319328034,
0.487259899888159,0.48743333569376),.UNSPECIFIED.)
GEOMETRIC_REPRESENTATION_ITEM()
RATIONAL_B_SPLINE_SURFACE(((0.987775548376701,0.988735325500096,0.992651440660746,
0.992651440660746,0.992651440660746),(0.987775548376701,0.988735325500096,
0.992651440660746,0.992651440660746,0.992651440660746)))
REPRESENTATION_ITEM('')
SURFACE()
);
#2087=(
BOUNDED_SURFACE()
B_SPLINE_SURFACE(1,2,((#129386,#129387,#129388,#129389,#129390),(#129391,
#129392,#129393,#129394,#129395)),.UNSPECIFIED.,.F.,.F.,.F.)
B_SPLINE_SURFACE_WITH_KNOTS((2,2),(3,2,3),(0.,0.290401167103061),(0.245359924967892,
0.245954053070908,0.263201868951011),.UNSPECIFIED.)
GEOMETRIC_REPRESENTATION_ITEM()
RATIONAL_B_SPLINE_SURFACE(((0.987624841600687,0.987624841600687,0.987624841600687,
0.986938988894507,0.989176916802451),(0.987624841600687,0.987624841600687,
0.987624841600687,0.986938988894508,0.989176916802451)))
REPRESENTATION_ITEM('')
SURFACE()
);
#2088=(
BOUNDED_SURFACE()
B_SPLINE_SURFACE(1,2,((#129412,#129413,#129414,#129415,#129416),(#129417,
#129418,#129419,#129420,#129421)),.UNSPECIFIED.,.F.,.F.,.F.)
B_SPLINE_SURFACE_WITH_KNOTS((2,2),(3,2,3),(0.,0.28968108435992),(0.469916319328034,
0.487259899888159,0.48743333569376),.UNSPECIFIED.)
GEOMETRIC_REPRESENTATION_ITEM()
RATIONAL_B_SPLINE_SURFACE(((0.987775548376701,0.988735325500096,0.992651440660746,
0.992651440660746,0.992651440660746),(0.987775548376701,0.988735325500096,
0.992651440660746,0.992651440660746,0.992651440660746)))
REPRESENTATION_ITEM('')
SURFACE()
);
#2089=(
BOUNDED_SURFACE()
B_SPLINE_SURFACE(1,2,((#129423,#129424,#129425,#129426,#129427),(#129428,
#129429,#129430,#129431,#129432)),.UNSPECIFIED.,.F.,.F.,.F.)
B_SPLINE_SURFACE_WITH_KNOTS((2,2),(3,2,3),(0.,0.290401167141549),(0.245359924929602,
0.245954053070908,0.263201868951011),.UNSPECIFIED.)
GEOMETRIC_REPRESENTATION_ITEM()
RATIONAL_B_SPLINE_SURFACE(((0.987624841600687,0.987624841600687,0.987624841600687,
0.986938988894508,0.989176916802451),(0.987624841600687,0.987624841600687,
0.987624841600687,0.986938988894508,0.989176916802451)))
REPRESENTATION_ITEM('')
SURFACE()
);
#2090=(
BOUNDED_SURFACE()
B_SPLINE_SURFACE(1,2,((#129449,#129450,#129451,#129452,#129453),(#129454,
#129455,#129456,#129457,#129458)),.UNSPECIFIED.,.F.,.F.,.F.)
B_SPLINE_SURFACE_WITH_KNOTS((2,2),(3,2,3),(0.,0.289681084359919),(0.469916319328034,
0.487259899888159,0.48743333569376),.UNSPECIFIED.)
GEOMETRIC_REPRESENTATION_ITEM()
RATIONAL_B_SPLINE_SURFACE(((0.987775548376701,0.988735325500096,0.992651440660746,
0.992651440660746,0.992651440660746),(0.987775548376701,0.988735325500096,
0.992651440660746,0.992651440660746,0.992651440660746)))
REPRESENTATION_ITEM('')
SURFACE()
);
#2091=(
BOUNDED_SURFACE()
B_SPLINE_SURFACE(1,2,((#129460,#129461,#129462,#129463,#129464),(#129465,
#129466,#129467,#129468,#129469)),.UNSPECIFIED.,.F.,.F.,.F.)
B_SPLINE_SURFACE_WITH_KNOTS((2,2),(3,2,3),(0.,0.290401167496561),(0.245359925137882,
0.245954053070908,0.263201868951011),.UNSPECIFIED.)
GEOMETRIC_REPRESENTATION_ITEM()
RATIONAL_B_SPLINE_SURFACE(((0.987624841600687,0.987624841600687,0.987624841600687,
0.986938988894508,0.989176916802451),(0.987624841600687,0.987624841600687,
0.987624841600687,0.986938988894508,0.989176916802451)))
REPRESENTATION_ITEM('')
SURFACE()
);
#2092=(
BOUNDED_SURFACE()
B_SPLINE_SURFACE(1,2,((#129480,#129481,#129482,#129483,#129484),(#129485,
#129486,#129487,#129488,#129489)),.UNSPECIFIED.,.F.,.F.,.F.)
B_SPLINE_SURFACE_WITH_KNOTS((2,2),(3,2,3),(0.,0.289681084359921),(0.469916319328034,
0.487259899888159,0.48743333569376),.UNSPECIFIED.)
GEOMETRIC_REPRESENTATION_ITEM()
RATIONAL_B_SPLINE_SURFACE(((0.987775548376701,0.988735325500096,0.992651440660746,
0.992651440660746,0.992651440660746),(0.987775548376701,0.988735325500096,
0.992651440660746,0.992651440660746,0.992651440660746)))
REPRESENTATION_ITEM('')
SURFACE()
);
#2093=(
BOUNDED_SURFACE()
B_SPLINE_SURFACE(1,2,((#129497,#129498,#129499,#129500,#129501),(#129502,
#129503,#129504,#129505,#129506)),.UNSPECIFIED.,.F.,.F.,.F.)
B_SPLINE_SURFACE_WITH_KNOTS((2,2),(3,2,3),(0.,0.290401167141741),(0.245359924929359,
0.245954053070908,0.263201868951016),.UNSPECIFIED.)
GEOMETRIC_REPRESENTATION_ITEM()
RATIONAL_B_SPLINE_SURFACE(((0.987624841600687,0.987624841600687,0.987624841600687,
0.986938988894508,0.989176916802452),(0.987624841600687,0.987624841600687,
0.987624841600687,0.986938988894508,0.989176916802452)))
REPRESENTATION_ITEM('')
SURFACE()
);
#2094=(
BOUNDED_SURFACE()
B_SPLINE_SURFACE(1,2,((#129523,#129524,#129525,#129526,#129527),(#129528,
#129529,#129530,#129531,#129532)),.UNSPECIFIED.,.F.,.F.,.F.)
B_SPLINE_SURFACE_WITH_KNOTS((2,2),(3,2,3),(0.,0.289681084359923),(0.469916319328038,
0.487259899888158,0.487433335693759),.UNSPECIFIED.)
GEOMETRIC_REPRESENTATION_ITEM()
RATIONAL_B_SPLINE_SURFACE(((0.987775548376701,0.988735325500097,0.992651440660745,
0.992651440660745,0.992651440660745),(0.987775548376701,0.988735325500097,
0.992651440660745,0.992651440660745,0.992651440660745)))
REPRESENTATION_ITEM('')
SURFACE()
);
#2095=(
BOUNDED_SURFACE()
B_SPLINE_SURFACE(1,2,((#129534,#129535,#129536,#129537,#129538),(#129539,
#129540,#129541,#129542,#129543)),.UNSPECIFIED.,.F.,.F.,.F.)
B_SPLINE_SURFACE_WITH_KNOTS((2,2),(3,2,3),(0.,0.290401167126936),(0.245359924944069,
0.245954053070909,0.263201868951012),.UNSPECIFIED.)
GEOMETRIC_REPRESENTATION_ITEM()
RATIONAL_B_SPLINE_SURFACE(((0.987624841600687,0.987624841600687,0.987624841600687,
0.986938988894508,0.989176916802451),(0.987624841600687,0.987624841600687,
0.987624841600687,0.986938988894508,0.989176916802451)))
REPRESENTATION_ITEM('')
SURFACE()
);
#2096=(
BOUNDED_SURFACE()
B_SPLINE_SURFACE(1,2,((#129560,#129561,#129562,#129563,#129564),(#129565,
#129566,#129567,#129568,#129569)),.UNSPECIFIED.,.F.,.F.,.F.)
B_SPLINE_SURFACE_WITH_KNOTS((2,2),(3,2,3),(0.,0.289681084359924),(0.469916319328033,
0.487259899888158,0.487433335693759),.UNSPECIFIED.)
GEOMETRIC_REPRESENTATION_ITEM()
RATIONAL_B_SPLINE_SURFACE(((0.9877755483767,0.988735325500095,0.992651440660745,
0.992651440660745,0.992651440660745),(0.9877755483767,0.988735325500095,
0.992651440660745,0.992651440660745,0.992651440660745)))
REPRESENTATION_ITEM('')
SURFACE()
);
#2097=(
BOUNDED_SURFACE()
B_SPLINE_SURFACE(1,2,((#129571,#129572,#129573,#129574,#129575),(#129576,
#129577,#129578,#129579,#129580)),.UNSPECIFIED.,.F.,.F.,.F.)
B_SPLINE_SURFACE_WITH_KNOTS((2,2),(3,2,3),(0.,0.290401167114357),(0.245359924956648,
0.245954053070909,0.263201868951012),.UNSPECIFIED.)
GEOMETRIC_REPRESENTATION_ITEM()
RATIONAL_B_SPLINE_SURFACE(((0.987624841600687,0.987624841600687,0.987624841600687,
0.986938988894508,0.989176916802451),(0.987624841600687,0.987624841600687,
0.987624841600687,0.986938988894508,0.989176916802451)))
REPRESENTATION_ITEM('')
SURFACE()
);
#2098=(
BOUNDED_SURFACE()
B_SPLINE_SURFACE(1,2,((#129597,#129598,#129599,#129600,#129601),(#129602,
#129603,#129604,#129605,#129606)),.UNSPECIFIED.,.F.,.F.,.F.)
B_SPLINE_SURFACE_WITH_KNOTS((2,2),(3,2,3),(0.,0.289681084359919),(0.469916319328033,
0.487259899888158,0.487433335693759),.UNSPECIFIED.)
GEOMETRIC_REPRESENTATION_ITEM()
RATIONAL_B_SPLINE_SURFACE(((0.9877755483767,0.988735325500095,0.992651440660745,
0.992651440660745,0.992651440660745),(0.9877755483767,0.988735325500095,
0.992651440660745,0.992651440660745,0.992651440660745)))
REPRESENTATION_ITEM('')
SURFACE()
);
#2099=(
BOUNDED_SURFACE()
B_SPLINE_SURFACE(1,2,((#129608,#129609,#129610,#129611,#129612),(#129613,
#129614,#129615,#129616,#129617)),.UNSPECIFIED.,.F.,.F.,.F.)
B_SPLINE_SURFACE_WITH_KNOTS((2,2),(3,2,3),(0.,0.290401167111398),(0.245359924959528,
0.245954053070909,0.263201868951012),.UNSPECIFIED.)
GEOMETRIC_REPRESENTATION_ITEM()
RATIONAL_B_SPLINE_SURFACE(((0.987624841600687,0.987624841600687,0.987624841600687,
0.986938988894508,0.989176916802451),(0.987624841600687,0.987624841600687,
0.987624841600687,0.986938988894508,0.989176916802451)))
REPRESENTATION_ITEM('')
SURFACE()
);
#2100=(
BOUNDED_SURFACE()
B_SPLINE_SURFACE(1,2,((#129634,#129635,#129636,#129637,#129638),(#129639,
#129640,#129641,#129642,#129643)),.UNSPECIFIED.,.F.,.F.,.F.)
B_SPLINE_SURFACE_WITH_KNOTS((2,2),(3,2,3),(0.,0.289681084359919),(0.469916319328033,
0.487259899888158,0.487433335693759),.UNSPECIFIED.)
GEOMETRIC_REPRESENTATION_ITEM()
RATIONAL_B_SPLINE_SURFACE(((0.9877755483767,0.988735325500095,0.992651440660745,
0.992651440660745,0.992651440660745),(0.9877755483767,0.988735325500095,
0.992651440660745,0.992651440660745,0.992651440660745)))
REPRESENTATION_ITEM('')
SURFACE()
);
#2101=(
BOUNDED_SURFACE()
B_SPLINE_SURFACE(1,2,((#129645,#129646,#129647,#129648,#129649),(#129650,
#129651,#129652,#129653,#129654)),.UNSPECIFIED.,.F.,.F.,.F.)
B_SPLINE_SURFACE_WITH_KNOTS((2,2),(3,2,3),(0.,0.290401167112765),(0.24535992495884,
0.245954053070909,0.263201868951012),.UNSPECIFIED.)
GEOMETRIC_REPRESENTATION_ITEM()
RATIONAL_B_SPLINE_SURFACE(((0.987624841600687,0.987624841600687,0.987624841600687,
0.986938988894508,0.989176916802451),(0.987624841600687,0.987624841600687,
0.987624841600687,0.986938988894508,0.989176916802451)))
REPRESENTATION_ITEM('')
SURFACE()
);
#2102=(
BOUNDED_SURFACE()
B_SPLINE_SURFACE(1,2,((#129671,#129672,#129673,#129674,#129675),(#129676,
#129677,#129678,#129679,#129680)),.UNSPECIFIED.,.F.,.F.,.F.)
B_SPLINE_SURFACE_WITH_KNOTS((2,2),(3,2,3),(0.,0.289681084359927),(0.469916319328033,
0.487259899888158,0.487433335693759),.UNSPECIFIED.)
GEOMETRIC_REPRESENTATION_ITEM()
RATIONAL_B_SPLINE_SURFACE(((0.9877755483767,0.988735325500095,0.992651440660745,
0.992651440660745,0.992651440660745),(0.9877755483767,0.988735325500095,
0.992651440660745,0.992651440660745,0.992651440660745)))
REPRESENTATION_ITEM('')
SURFACE()
);
#2103=(
BOUNDED_SURFACE()
B_SPLINE_SURFACE(1,2,((#129682,#129683,#129684,#129685,#129686),(#129687,
#129688,#129689,#129690,#129691)),.UNSPECIFIED.,.F.,.F.,.F.)
B_SPLINE_SURFACE_WITH_KNOTS((2,2),(3,2,3),(0.,0.290401167150003),(0.245359924921204,
0.245954053070909,0.263201868951012),.UNSPECIFIED.)
GEOMETRIC_REPRESENTATION_ITEM()
RATIONAL_B_SPLINE_SURFACE(((0.987624841600687,0.987624841600687,0.987624841600687,
0.986938988894508,0.989176916802451),(0.987624841600687,0.987624841600687,
0.987624841600687,0.986938988894508,0.989176916802451)))
REPRESENTATION_ITEM('')
SURFACE()
);
#2104=(
BOUNDED_SURFACE()
B_SPLINE_SURFACE(1,2,((#129708,#129709,#129710,#129711,#129712),(#129713,
#129714,#129715,#129716,#129717)),.UNSPECIFIED.,.F.,.F.,.F.)
B_SPLINE_SURFACE_WITH_KNOTS((2,2),(3,2,3),(0.,0.289681084359916),(0.469916319328029,
0.487259899888781,0.487433335694389),.UNSPECIFIED.)
GEOMETRIC_REPRESENTATION_ITEM()
RATIONAL_B_SPLINE_SURFACE(((0.9877755483767,0.988735325500129,0.992651440661026,
0.992651440661026,0.992651440661026),(0.9877755483767,0.988735325500129,
0.992651440661026,0.992651440661026,0.992651440661026)))
REPRESENTATION_ITEM('')
SURFACE()
);
#2105=(
BOUNDED_SURFACE()
B_SPLINE_SURFACE(1,2,((#129719,#129720,#129721,#129722,#129723),(#129724,
#129725,#129726,#129727,#129728)),.UNSPECIFIED.,.F.,.F.,.F.)
B_SPLINE_SURFACE_WITH_KNOTS((2,2),(3,2,3),(0.,0.290401167096493),(0.245359924974528,
0.245954053070909,0.263201868951012),.UNSPECIFIED.)
GEOMETRIC_REPRESENTATION_ITEM()
RATIONAL_B_SPLINE_SURFACE(((0.987624841600687,0.987624841600687,0.987624841600687,
0.986938988894508,0.989176916802451),(0.987624841600687,0.987624841600687,
0.987624841600687,0.986938988894508,0.989176916802451)))
REPRESENTATION_ITEM('')
SURFACE()
);
#2106=(
BOUNDED_SURFACE()
B_SPLINE_SURFACE(1,2,((#129745,#129746,#129747,#129748,#129749),(#129750,
#129751,#129752,#129753,#129754)),.UNSPECIFIED.,.F.,.F.,.F.)
B_SPLINE_SURFACE_WITH_KNOTS((2,2),(3,2,3),(0.,0.289681084359929),(0.469916319328032,
0.487259899888158,0.487433335693759),.UNSPECIFIED.)
GEOMETRIC_REPRESENTATION_ITEM()
RATIONAL_B_SPLINE_SURFACE(((0.9877755483767,0.988735325500095,0.992651440660745,
0.992651440660745,0.992651440660745),(0.9877755483767,0.988735325500095,
0.992651440660745,0.992651440660745,0.992651440660745)))
REPRESENTATION_ITEM('')
SURFACE()
);
#2107=(
BOUNDED_SURFACE()
B_SPLINE_SURFACE(1,2,((#129762,#129763,#129764,#129765,#129766),(#129767,
#129768,#129769,#129770,#129771)),.UNSPECIFIED.,.F.,.F.,.F.)
B_SPLINE_SURFACE_WITH_KNOTS((2,2),(3,2,3),(0.,0.290401167109339),(0.245359924961707,
0.245954053070909,0.263201868951011),.UNSPECIFIED.)
GEOMETRIC_REPRESENTATION_ITEM()
RATIONAL_B_SPLINE_SURFACE(((0.987624841600687,0.987624841600687,0.987624841600687,
0.986938988894508,0.989176916802451),(0.987624841600687,0.987624841600687,
0.987624841600687,0.986938988894508,0.989176916802451)))
REPRESENTATION_ITEM('')
SURFACE()
);
#2108=(
BOUNDED_SURFACE()
B_SPLINE_SURFACE(1,2,((#129773,#129774,#129775),(#129776,#129777,#129778)),
 .UNSPECIFIED.,.F.,.F.,.F.)
B_SPLINE_SURFACE_WITH_KNOTS((2,2),(3,3),(0.710192959008444,1.),(0.194132688793569,
0.211606804210308),.UNSPECIFIED.)
GEOMETRIC_REPRESENTATION_ITEM()
RATIONAL_B_SPLINE_SURFACE(((0.989843896581211,0.992516389311156,0.998189888755648),
(0.989843896581211,0.992516389311156,0.998189888755648)))
REPRESENTATION_ITEM('')
SURFACE()
);
#2109=(
BOUNDED_SURFACE()
B_SPLINE_SURFACE(1,2,((#129789,#129790,#129791,#129792,#129793),(#129794,
#129795,#129796,#129797,#129798)),.UNSPECIFIED.,.F.,.F.,.F.)
B_SPLINE_SURFACE_WITH_KNOTS((2,2),(3,2,3),(0.709727264421552,1.),(0.521815037222016,
0.53899963051341,0.539591283949508),.UNSPECIFIED.)
GEOMETRIC_REPRESENTATION_ITEM()
RATIONAL_B_SPLINE_SURFACE(((0.989362668575565,0.987015160230477,0.987570037304351,
0.987570037304351,0.987570037304351),(0.989362668575565,0.987015160230477,
0.987570037304351,0.987570037304351,0.987570037304351)))
REPRESENTATION_ITEM('')
SURFACE()
);
#2110=(
BOUNDED_SURFACE()
B_SPLINE_SURFACE(1,2,((#129809,#129810,#129811),(#129812,#129813,#129814)),
 .UNSPECIFIED.,.F.,.F.,.F.)
B_SPLINE_SURFACE_WITH_KNOTS((2,2),(3,3),(0.710192959008445,1.),(0.194132688793569,
0.211606804210308),.UNSPECIFIED.)
GEOMETRIC_REPRESENTATION_ITEM()
RATIONAL_B_SPLINE_SURFACE(((0.989843896581211,0.992516389311156,0.998189888755648),
(0.989843896581211,0.992516389311156,0.998189888755648)))
REPRESENTATION_ITEM('')
SURFACE()
);
#2111=(
BOUNDED_SURFACE()
B_SPLINE_SURFACE(1,2,((#129822,#129823,#129824,#129825,#129826),(#129827,
#129828,#129829,#129830,#129831)),.UNSPECIFIED.,.F.,.F.,.F.)
B_SPLINE_SURFACE_WITH_KNOTS((2,2),(3,2,3),(0.709727264434569,1.),(0.521815037222016,
0.53899963051341,0.539591283935433),.UNSPECIFIED.)
GEOMETRIC_REPRESENTATION_ITEM()
RATIONAL_B_SPLINE_SURFACE(((0.989362668575565,0.987015160230477,0.987570037304351,
0.987570037304351,0.987570037304351),(0.989362668575565,0.987015160230477,
0.987570037304351,0.987570037304351,0.987570037304351)))
REPRESENTATION_ITEM('')
SURFACE()
);
#2112=(
BOUNDED_SURFACE()
B_SPLINE_SURFACE(1,2,((#129842,#129843,#129844),(#129845,#129846,#129847)),
 .UNSPECIFIED.,.F.,.F.,.F.)
B_SPLINE_SURFACE_WITH_KNOTS((2,2),(3,3),(0.71019295900751,1.),(0.194132688793569,
0.211606804210308),.UNSPECIFIED.)
GEOMETRIC_REPRESENTATION_ITEM()
RATIONAL_B_SPLINE_SURFACE(((0.989843896581211,0.992516389311156,0.998189888755648),
(0.989843896581211,0.992516389311156,0.998189888755648)))
REPRESENTATION_ITEM('')
SURFACE()
);
#2113=(
BOUNDED_SURFACE()
B_SPLINE_SURFACE(1,2,((#129855,#129856,#129857,#129858,#129859),(#129860,
#129861,#129862,#129863,#129864)),.UNSPECIFIED.,.F.,.F.,.F.)
B_SPLINE_SURFACE_WITH_KNOTS((2,2),(3,2,3),(0.709727264435488,1.),(0.521815037222016,
0.53899963051341,0.539591283934722),.UNSPECIFIED.)
GEOMETRIC_REPRESENTATION_ITEM()
RATIONAL_B_SPLINE_SURFACE(((0.989362668575565,0.987015160230477,0.987570037304351,
0.987570037304351,0.987570037304351),(0.989362668575565,0.987015160230477,
0.987570037304351,0.987570037304351,0.987570037304351)))
REPRESENTATION_ITEM('')
SURFACE()
);
#2114=(
BOUNDED_SURFACE()
B_SPLINE_SURFACE(1,2,((#129875,#129876,#129877),(#129878,#129879,#129880)),
 .UNSPECIFIED.,.F.,.F.,.F.)
B_SPLINE_SURFACE_WITH_KNOTS((2,2),(3,3),(0.710192959007511,1.),(0.194132688793569,
0.211606804210308),.UNSPECIFIED.)
GEOMETRIC_REPRESENTATION_ITEM()
RATIONAL_B_SPLINE_SURFACE(((0.989843896581211,0.992516389311156,0.998189888755648),
(0.989843896581211,0.992516389311156,0.998189888755648)))
REPRESENTATION_ITEM('')
SURFACE()
);
#2115=(
BOUNDED_SURFACE()
B_SPLINE_SURFACE(1,2,((#129888,#129889,#129890,#129891,#129892),(#129893,
#129894,#129895,#129896,#129897)),.UNSPECIFIED.,.F.,.F.,.F.)
B_SPLINE_SURFACE_WITH_KNOTS((2,2),(3,2,3),(0.709727264431373,1.),(0.521815037222016,
0.53899963051341,0.539591283938545),.UNSPECIFIED.)
GEOMETRIC_REPRESENTATION_ITEM()
RATIONAL_B_SPLINE_SURFACE(((0.989362668575565,0.987015160230477,0.987570037304351,
0.987570037304351,0.987570037304351),(0.989362668575565,0.987015160230477,
0.987570037304351,0.987570037304351,0.987570037304351)))
REPRESENTATION_ITEM('')
SURFACE()
);
#2116=(
BOUNDED_SURFACE()
B_SPLINE_SURFACE(1,2,((#129908,#129909,#129910),(#129911,#129912,#129913)),
 .UNSPECIFIED.,.F.,.F.,.F.)
B_SPLINE_SURFACE_WITH_KNOTS((2,2),(3,3),(0.710192959007508,1.),(0.194132688793569,
0.211606804210308),.UNSPECIFIED.)
GEOMETRIC_REPRESENTATION_ITEM()
RATIONAL_B_SPLINE_SURFACE(((0.989843896581211,0.992516389311156,0.998189888755648),
(0.989843896581211,0.992516389311156,0.998189888755648)))
REPRESENTATION_ITEM('')
SURFACE()
);
#2117=(
BOUNDED_SURFACE()
B_SPLINE_SURFACE(1,2,((#129921,#129922,#129923,#129924,#129925),(#129926,
#129927,#129928,#129929,#129930)),.UNSPECIFIED.,.F.,.F.,.F.)
B_SPLINE_SURFACE_WITH_KNOTS((2,2),(3,2,3),(0.709727264444556,1.),(0.521815037222016,
0.53899963051341,0.53959128392486),.UNSPECIFIED.)
GEOMETRIC_REPRESENTATION_ITEM()
RATIONAL_B_SPLINE_SURFACE(((0.989362668575565,0.987015160230477,0.987570037304351,
0.987570037304351,0.987570037304351),(0.989362668575565,0.987015160230477,
0.987570037304351,0.987570037304351,0.987570037304351)))
REPRESENTATION_ITEM('')
SURFACE()
);
#2118=(
BOUNDED_SURFACE()
B_SPLINE_SURFACE(1,2,((#129941,#129942,#129943),(#129944,#129945,#129946)),
 .UNSPECIFIED.,.F.,.F.,.F.)
B_SPLINE_SURFACE_WITH_KNOTS((2,2),(3,3),(0.710192959006928,1.),(0.194132688793569,
0.211606804210308),.UNSPECIFIED.)
GEOMETRIC_REPRESENTATION_ITEM()
RATIONAL_B_SPLINE_SURFACE(((0.989843896581211,0.992516389311156,0.998189888755648),
(0.989843896581211,0.992516389311156,0.998189888755648)))
REPRESENTATION_ITEM('')
SURFACE()
);
#2119=(
BOUNDED_SURFACE()
B_SPLINE_SURFACE(1,2,((#129954,#129955,#129956,#129957,#129958),(#129959,
#129960,#129961,#129962,#129963)),.UNSPECIFIED.,.F.,.F.,.F.)
B_SPLINE_SURFACE_WITH_KNOTS((2,2),(3,2,3),(0.709727264376017,1.),(0.521815037222016,
0.53899963051341,0.539591283993824),.UNSPECIFIED.)
GEOMETRIC_REPRESENTATION_ITEM()
RATIONAL_B_SPLINE_SURFACE(((0.989362668575565,0.987015160230477,0.987570037304351,
0.987570037304351,0.987570037304351),(0.989362668575565,0.987015160230477,
0.987570037304351,0.987570037304351,0.987570037304351)))
REPRESENTATION_ITEM('')
SURFACE()
);
#2120=(
BOUNDED_SURFACE()
B_SPLINE_SURFACE(1,2,((#129974,#129975,#129976),(#129977,#129978,#129979)),
 .UNSPECIFIED.,.F.,.F.,.F.)
B_SPLINE_SURFACE_WITH_KNOTS((2,2),(3,3),(0.710192959007512,1.),(0.194132688793569,
0.211606804210308),.UNSPECIFIED.)
GEOMETRIC_REPRESENTATION_ITEM()
RATIONAL_B_SPLINE_SURFACE(((0.989843896581211,0.992516389311156,0.998189888755648),
(0.989843896581211,0.992516389311156,0.998189888755648)))
REPRESENTATION_ITEM('')
SURFACE()
);
#2121=(
BOUNDED_SURFACE()
B_SPLINE_SURFACE(1,2,((#129987,#129988,#129989,#129990,#129991),(#129992,
#129993,#129994,#129995,#129996)),.UNSPECIFIED.,.F.,.F.,.F.)
B_SPLINE_SURFACE_WITH_KNOTS((2,2),(3,2,3),(0.709727264422407,1.),(0.521815037222016,
0.53899963051341,0.539591283947025),.UNSPECIFIED.)
GEOMETRIC_REPRESENTATION_ITEM()
RATIONAL_B_SPLINE_SURFACE(((0.989362668575565,0.987015160230477,0.987570037304351,
0.987570037304351,0.987570037304351),(0.989362668575565,0.987015160230477,
0.987570037304351,0.987570037304351,0.987570037304351)))
REPRESENTATION_ITEM('')
SURFACE()
);
#2122=(
BOUNDED_SURFACE()
B_SPLINE_SURFACE(1,2,((#130007,#130008,#130009),(#130010,#130011,#130012)),
 .UNSPECIFIED.,.F.,.F.,.F.)
B_SPLINE_SURFACE_WITH_KNOTS((2,2),(3,3),(0.710192959006932,1.),(0.194132688793569,
0.211606804210308),.UNSPECIFIED.)
GEOMETRIC_REPRESENTATION_ITEM()
RATIONAL_B_SPLINE_SURFACE(((0.989843896581211,0.992516389311156,0.998189888755648),
(0.989843896581211,0.992516389311156,0.998189888755648)))
REPRESENTATION_ITEM('')
SURFACE()
);
#2123=(
BOUNDED_SURFACE()
B_SPLINE_SURFACE(1,2,((#130020,#130021,#130022,#130023,#130024),(#130025,
#130026,#130027,#130028,#130029)),.UNSPECIFIED.,.F.,.F.,.F.)
B_SPLINE_SURFACE_WITH_KNOTS((2,2),(3,2,3),(0.709727264379074,1.),(0.521815037222017,
0.53899963051341,0.539591283990695),.UNSPECIFIED.)
GEOMETRIC_REPRESENTATION_ITEM()
RATIONAL_B_SPLINE_SURFACE(((0.989362668575565,0.987015160230477,0.987570037304351,
0.987570037304351,0.987570037304351),(0.989362668575565,0.987015160230477,
0.987570037304351,0.987570037304351,0.987570037304351)))
REPRESENTATION_ITEM('')
SURFACE()
);
#2124=(
BOUNDED_SURFACE()
B_SPLINE_SURFACE(1,2,((#130040,#130041,#130042),(#130043,#130044,#130045)),
 .UNSPECIFIED.,.F.,.F.,.F.)
B_SPLINE_SURFACE_WITH_KNOTS((2,2),(3,3),(0.710192959007428,1.),(0.194132688793568,
0.211606804210307),.UNSPECIFIED.)
GEOMETRIC_REPRESENTATION_ITEM()
RATIONAL_B_SPLINE_SURFACE(((0.989843896581211,0.992516389311155,0.998189888755648),
(0.989843896581211,0.992516389311155,0.998189888755648)))
REPRESENTATION_ITEM('')
SURFACE()
);
#2125=(
BOUNDED_SURFACE()
B_SPLINE_SURFACE(1,2,((#130053,#130054,#130055,#130056,#130057),(#130058,
#130059,#130060,#130061,#130062)),.UNSPECIFIED.,.F.,.F.,.F.)
B_SPLINE_SURFACE_WITH_KNOTS((2,2),(3,2,3),(0.709727264425964,1.),(0.521815037222018,
0.538999630513411,0.539591283943759),.UNSPECIFIED.)
GEOMETRIC_REPRESENTATION_ITEM()
RATIONAL_B_SPLINE_SURFACE(((0.989362668575565,0.987015160230477,0.987570037304351,
0.987570037304351,0.987570037304351),(0.989362668575565,0.987015160230477,
0.987570037304351,0.987570037304351,0.987570037304351)))
REPRESENTATION_ITEM('')
SURFACE()
);
#2126=(
BOUNDED_SURFACE()
B_SPLINE_SURFACE(1,2,((#130073,#130074,#130075),(#130076,#130077,#130078)),
 .UNSPECIFIED.,.F.,.F.,.F.)
B_SPLINE_SURFACE_WITH_KNOTS((2,2),(3,3),(0.710192959007435,1.),(0.194132688793568,
0.211606804210307),.UNSPECIFIED.)
GEOMETRIC_REPRESENTATION_ITEM()
RATIONAL_B_SPLINE_SURFACE(((0.989843896581211,0.992516389311156,0.998189888755648),
(0.989843896581211,0.992516389311156,0.998189888755648)))
REPRESENTATION_ITEM('')
SURFACE()
);
#2127=(
BOUNDED_SURFACE()
B_SPLINE_SURFACE(1,2,((#130086,#130087,#130088,#130089,#130090),(#130091,
#130092,#130093,#130094,#130095)),.UNSPECIFIED.,.F.,.F.,.F.)
B_SPLINE_SURFACE_WITH_KNOTS((2,2),(3,2,3),(0.709727264418055,1.),(0.521815037222017,
0.538999630513411,0.539591283951268),.UNSPECIFIED.)
GEOMETRIC_REPRESENTATION_ITEM()
RATIONAL_B_SPLINE_SURFACE(((0.989362668575565,0.987015160230477,0.987570037304351,
0.987570037304351,0.987570037304351),(0.989362668575565,0.987015160230477,
0.987570037304351,0.987570037304351,0.987570037304351)))
REPRESENTATION_ITEM('')
SURFACE()
);
#2128=(
BOUNDED_SURFACE()
B_SPLINE_SURFACE(1,2,((#130106,#130107,#130108),(#130109,#130110,#130111)),
 .UNSPECIFIED.,.F.,.F.,.F.)
B_SPLINE_SURFACE_WITH_KNOTS((2,2),(3,3),(0.710192959006835,1.),(0.194132688793568,
0.211606804210307),.UNSPECIFIED.)
GEOMETRIC_REPRESENTATION_ITEM()
RATIONAL_B_SPLINE_SURFACE(((0.989843896581211,0.992516389311155,0.998189888755648),
(0.989843896581211,0.992516389311155,0.998189888755648)))
REPRESENTATION_ITEM('')
SURFACE()
);
#2129=(
BOUNDED_SURFACE()
B_SPLINE_SURFACE(1,2,((#130119,#130120,#130121,#130122,#130123),(#130124,
#130125,#130126,#130127,#130128)),.UNSPECIFIED.,.F.,.F.,.F.)
B_SPLINE_SURFACE_WITH_KNOTS((2,2),(3,2,3),(0.709727264402715,1.),(0.521815037222018,
0.538999630513411,0.539591283967167),.UNSPECIFIED.)
GEOMETRIC_REPRESENTATION_ITEM()
RATIONAL_B_SPLINE_SURFACE(((0.989362668575565,0.987015160230477,0.987570037304351,
0.987570037304351,0.987570037304351),(0.989362668575565,0.987015160230477,
0.987570037304351,0.987570037304351,0.987570037304351)))
REPRESENTATION_ITEM('')
SURFACE()
);
#2130=(
BOUNDED_SURFACE()
B_SPLINE_SURFACE(1,2,((#130139,#130140,#130141),(#130142,#130143,#130144)),
 .UNSPECIFIED.,.F.,.F.,.F.)
B_SPLINE_SURFACE_WITH_KNOTS((2,2),(3,3),(0.710192959007424,1.),(0.194132688793568,
0.211606804210307),.UNSPECIFIED.)
GEOMETRIC_REPRESENTATION_ITEM()
RATIONAL_B_SPLINE_SURFACE(((0.989843896581211,0.992516389311155,0.998189888755648),
(0.989843896581211,0.992516389311155,0.998189888755648)))
REPRESENTATION_ITEM('')
SURFACE()
);
#2131=(
BOUNDED_SURFACE()
B_SPLINE_SURFACE(1,2,((#130152,#130153,#130154,#130155,#130156),(#130157,
#130158,#130159,#130160,#130161)),.UNSPECIFIED.,.F.,.F.,.F.)
B_SPLINE_SURFACE_WITH_KNOTS((2,2),(3,2,3),(0.709727264418693,1.),(0.521815037222018,
0.538999630513411,0.539591283950436),.UNSPECIFIED.)
GEOMETRIC_REPRESENTATION_ITEM()
RATIONAL_B_SPLINE_SURFACE(((0.989362668575565,0.987015160230477,0.987570037304351,
0.987570037304351,0.987570037304351),(0.989362668575565,0.987015160230477,
0.987570037304351,0.987570037304351,0.987570037304351)))
REPRESENTATION_ITEM('')
SURFACE()
);
#2132=(
BOUNDED_SURFACE()
B_SPLINE_SURFACE(1,2,((#130172,#130173,#130174),(#130175,#130176,#130177)),
 .UNSPECIFIED.,.F.,.F.,.F.)
B_SPLINE_SURFACE_WITH_KNOTS((2,2),(3,3),(0.710192959006924,1.),(0.194132688793568,
0.211606804210307),.UNSPECIFIED.)
GEOMETRIC_REPRESENTATION_ITEM()
RATIONAL_B_SPLINE_SURFACE(((0.989843896581211,0.992516389311155,0.998189888755648),
(0.989843896581211,0.992516389311155,0.998189888755648)))
REPRESENTATION_ITEM('')
SURFACE()
);
#2133=(
BOUNDED_SURFACE()
B_SPLINE_SURFACE(1,2,((#130185,#130186,#130187,#130188,#130189),(#130190,
#130191,#130192,#130193,#130194)),.UNSPECIFIED.,.F.,.F.,.F.)
B_SPLINE_SURFACE_WITH_KNOTS((2,2),(3,2,3),(0.709727264417126,1.),(0.521815037222017,
0.538999630513412,0.53959128395279),.UNSPECIFIED.)
GEOMETRIC_REPRESENTATION_ITEM()
RATIONAL_B_SPLINE_SURFACE(((0.989362668575565,0.987015160230477,0.987570037304351,
0.987570037304351,0.987570037304351),(0.989362668575565,0.987015160230477,
0.987570037304351,0.987570037304351,0.987570037304351)))
REPRESENTATION_ITEM('')
SURFACE()
);
#2134=(
BOUNDED_SURFACE()
B_SPLINE_SURFACE(1,2,((#130205,#130206,#130207),(#130208,#130209,#130210)),
 .UNSPECIFIED.,.F.,.F.,.F.)
B_SPLINE_SURFACE_WITH_KNOTS((2,2),(3,3),(0.710192959007418,1.),(0.194132688793568,
0.211606804210307),.UNSPECIFIED.)
GEOMETRIC_REPRESENTATION_ITEM()
RATIONAL_B_SPLINE_SURFACE(((0.989843896581211,0.992516389311156,0.998189888755648),
(0.989843896581211,0.992516389311156,0.998189888755648)))
REPRESENTATION_ITEM('')
SURFACE()
);
#2135=(
BOUNDED_SURFACE()
B_SPLINE_SURFACE(1,2,((#130218,#130219,#130220,#130221,#130222),(#130223,
#130224,#130225,#130226,#130227)),.UNSPECIFIED.,.F.,.F.,.F.)
B_SPLINE_SURFACE_WITH_KNOTS((2,2),(3,2,3),(0.709727265139864,1.),(0.521815037222017,
0.538999630513411,0.539591284245209),.UNSPECIFIED.)
GEOMETRIC_REPRESENTATION_ITEM()
RATIONAL_B_SPLINE_SURFACE(((0.989362668575565,0.987015160230477,0.987570037304351,
0.987570037304351,0.987570037304351),(0.989362668575565,0.987015160230477,
0.987570037304351,0.987570037304351,0.987570037304351)))
REPRESENTATION_ITEM('')
SURFACE()
);
#2136=(
BOUNDED_SURFACE()
B_SPLINE_SURFACE(1,2,((#130235,#130236,#130237),(#130238,#130239,#130240)),
 .UNSPECIFIED.,.F.,.F.,.F.)
B_SPLINE_SURFACE_WITH_KNOTS((2,2),(3,3),(0.710192959006919,1.),(0.194132688793568,
0.211606804210307),.UNSPECIFIED.)
GEOMETRIC_REPRESENTATION_ITEM()
RATIONAL_B_SPLINE_SURFACE(((0.989843896581211,0.992516389311155,0.998189888755648),
(0.989843896581211,0.992516389311155,0.998189888755648)))
REPRESENTATION_ITEM('')
SURFACE()
);
#2137=(
BOUNDED_SURFACE()
B_SPLINE_SURFACE(1,2,((#130242,#130243,#130244,#130245,#130246),(#130247,
#130248,#130249,#130250,#130251)),.UNSPECIFIED.,.F.,.F.,.F.)
B_SPLINE_SURFACE_WITH_KNOTS((2,2),(3,2,3),(0.709727264430238,1.),(0.521815037222018,
0.538999630513411,0.539591283939394),.UNSPECIFIED.)
GEOMETRIC_REPRESENTATION_ITEM()
RATIONAL_B_SPLINE_SURFACE(((0.989362668575565,0.987015160230477,0.987570037304351,
0.987570037304351,0.987570037304351),(0.989362668575565,0.987015160230477,
0.987570037304351,0.987570037304351,0.987570037304351)))
REPRESENTATION_ITEM('')
SURFACE()
);
#2138=(
BOUNDED_SURFACE()
B_SPLINE_SURFACE(1,2,((#130262,#130263,#130264),(#130265,#130266,#130267)),
 .UNSPECIFIED.,.F.,.F.,.F.)
B_SPLINE_SURFACE_WITH_KNOTS((2,2),(3,3),(0.710192959007147,1.),(0.194132688793568,
0.211606804210307),.UNSPECIFIED.)
GEOMETRIC_REPRESENTATION_ITEM()
RATIONAL_B_SPLINE_SURFACE(((0.989843896581211,0.992516389311156,0.998189888755648),
(0.989843896581211,0.992516389311156,0.998189888755648)))
REPRESENTATION_ITEM('')
SURFACE()
);
#2139=(
BOUNDED_SURFACE()
B_SPLINE_SURFACE(1,2,((#130275,#130276,#130277,#130278,#130279),(#130280,
#130281,#130282,#130283,#130284)),.UNSPECIFIED.,.F.,.F.,.F.)
B_SPLINE_SURFACE_WITH_KNOTS((2,2),(3,2,3),(0.709727264407736,1.),(0.521815037222018,
0.538999630513411,0.539591283960815),.UNSPECIFIED.)
GEOMETRIC_REPRESENTATION_ITEM()
RATIONAL_B_SPLINE_SURFACE(((0.989362668575565,0.987015160230477,0.987570037304351,
0.987570037304351,0.987570037304351),(0.989362668575565,0.987015160230477,
0.987570037304351,0.987570037304351,0.987570037304351)))
REPRESENTATION_ITEM('')
SURFACE()
);
#2140=(
BOUNDED_SURFACE()
B_SPLINE_SURFACE(1,2,((#130295,#130296,#130297),(#130298,#130299,#130300)),
 .UNSPECIFIED.,.F.,.F.,.F.)
B_SPLINE_SURFACE_WITH_KNOTS((2,2),(3,3),(0.710192959006099,1.),(0.194132688793568,
0.211606804210307),.UNSPECIFIED.)
GEOMETRIC_REPRESENTATION_ITEM()
RATIONAL_B_SPLINE_SURFACE(((0.989843896581211,0.992516389311156,0.998189888755648),
(0.989843896581211,0.992516389311156,0.998189888755648)))
REPRESENTATION_ITEM('')
SURFACE()
);
#2141=(
BOUNDED_SURFACE()
B_SPLINE_SURFACE(1,2,((#130308,#130309,#130310,#130311,#130312),(#130313,
#130314,#130315,#130316,#130317)),.UNSPECIFIED.,.F.,.F.,.F.)
B_SPLINE_SURFACE_WITH_KNOTS((2,2),(3,2,3),(0.709727264416509,1.),(0.521815037222015,
0.538999630513412,0.539591283953501),.UNSPECIFIED.)
GEOMETRIC_REPRESENTATION_ITEM()
RATIONAL_B_SPLINE_SURFACE(((0.989362668575565,0.987015160230477,0.987570037304351,
0.987570037304351,0.987570037304351),(0.989362668575565,0.987015160230477,
0.987570037304351,0.987570037304351,0.987570037304351)))
REPRESENTATION_ITEM('')
SURFACE()
);
#2142=(
BOUNDED_SURFACE()
B_SPLINE_SURFACE(1,2,((#130328,#130329,#130330),(#130331,#130332,#130333)),
 .UNSPECIFIED.,.F.,.F.,.F.)
B_SPLINE_SURFACE_WITH_KNOTS((2,2),(3,3),(0.710192959007386,1.),(0.194132688793568,
0.211606804210307),.UNSPECIFIED.)
GEOMETRIC_REPRESENTATION_ITEM()
RATIONAL_B_SPLINE_SURFACE(((0.989843896581211,0.992516389311155,0.998189888755647),
(0.989843896581211,0.992516389311155,0.998189888755647)))
REPRESENTATION_ITEM('')
SURFACE()
);
#2143=(
BOUNDED_SURFACE()
B_SPLINE_SURFACE(1,2,((#130341,#130342,#130343,#130344,#130345),(#130346,
#130347,#130348,#130349,#130350)),.UNSPECIFIED.,.F.,.F.,.F.)
B_SPLINE_SURFACE_WITH_KNOTS((2,2),(3,2,3),(0.709727264462459,1.),(0.521815037222018,
0.538999630513411,0.539591283907463),.UNSPECIFIED.)
GEOMETRIC_REPRESENTATION_ITEM()
RATIONAL_B_SPLINE_SURFACE(((0.989362668575565,0.987015160230477,0.987570037304351,
0.987570037304351,0.987570037304351),(0.989362668575565,0.987015160230477,
0.987570037304351,0.987570037304351,0.987570037304351)))
REPRESENTATION_ITEM('')
SURFACE()
);
#2144=(
BOUNDED_SURFACE()
B_SPLINE_SURFACE(1,2,((#130361,#130362,#130363),(#130364,#130365,#130366)),
 .UNSPECIFIED.,.F.,.F.,.F.)
B_SPLINE_SURFACE_WITH_KNOTS((2,2),(3,3),(0.710192959007503,1.),(0.194132688793568,
0.211606804210308),.UNSPECIFIED.)
GEOMETRIC_REPRESENTATION_ITEM()
RATIONAL_B_SPLINE_SURFACE(((0.98984389658121,0.992516389311155,0.998189888755648),
(0.989843896581211,0.992516389311156,0.998189888755648)))
REPRESENTATION_ITEM('')
SURFACE()
);
#2145=(
BOUNDED_SURFACE()
B_SPLINE_SURFACE(1,2,((#130374,#130375,#130376,#130377,#130378),(#130379,
#130380,#130381,#130382,#130383)),.UNSPECIFIED.,.F.,.F.,.F.)
B_SPLINE_SURFACE_WITH_KNOTS((2,2),(3,2,3),(0.709727264412533,1.),(0.521815037222017,
0.538999630513411,0.539591283956678),.UNSPECIFIED.)
GEOMETRIC_REPRESENTATION_ITEM()
RATIONAL_B_SPLINE_SURFACE(((0.989362668575565,0.987015160230477,0.987570037304351,
0.987570037304351,0.987570037304351),(0.989362668575565,0.987015160230477,
0.987570037304351,0.987570037304351,0.987570037304351)))
REPRESENTATION_ITEM('')
SURFACE()
);
#2146=(
BOUNDED_SURFACE()
B_SPLINE_SURFACE(1,2,((#130394,#130395,#130396),(#130397,#130398,#130399)),
 .UNSPECIFIED.,.F.,.F.,.F.)
B_SPLINE_SURFACE_WITH_KNOTS((2,2),(3,3),(0.710192959006866,1.),(0.194132688793568,
0.211606804210307),.UNSPECIFIED.)
GEOMETRIC_REPRESENTATION_ITEM()
RATIONAL_B_SPLINE_SURFACE(((0.989843896581211,0.992516389311155,0.998189888755648),
(0.989843896581211,0.992516389311155,0.998189888755648)))
REPRESENTATION_ITEM('')
SURFACE()
);
#2147=(
BOUNDED_SURFACE()
B_SPLINE_SURFACE(1,2,((#130407,#130408,#130409,#130410,#130411),(#130412,
#130413,#130414,#130415,#130416)),.UNSPECIFIED.,.F.,.F.,.F.)
B_SPLINE_SURFACE_WITH_KNOTS((2,2),(3,2,3),(0.709727264424186,1.),(0.521815037222016,
0.538999630513411,0.539591283946352),.UNSPECIFIED.)
GEOMETRIC_REPRESENTATION_ITEM()
RATIONAL_B_SPLINE_SURFACE(((0.989362668575565,0.987015160230477,0.987570037304351,
0.987570037304351,0.987570037304351),(0.989362668575565,0.987015160230477,
0.987570037304351,0.987570037304351,0.987570037304351)))
REPRESENTATION_ITEM('')
SURFACE()
);
#2148=(
BOUNDED_SURFACE()
B_SPLINE_SURFACE(1,2,((#130427,#130428,#130429),(#130430,#130431,#130432)),
 .UNSPECIFIED.,.F.,.F.,.F.)
B_SPLINE_SURFACE_WITH_KNOTS((2,2),(3,3),(0.710192959008264,1.),(0.194132688793568,
0.211606804210306),.UNSPECIFIED.)
GEOMETRIC_REPRESENTATION_ITEM()
RATIONAL_B_SPLINE_SURFACE(((0.989843896581211,0.992516389311155,0.998189888755647),
(0.989843896581211,0.992516389311155,0.998189888755647)))
REPRESENTATION_ITEM('')
SURFACE()
);
#2149=(
BOUNDED_SURFACE()
B_SPLINE_SURFACE(1,2,((#130440,#130441,#130442,#130443,#130444),(#130445,
#130446,#130447,#130448,#130449)),.UNSPECIFIED.,.F.,.F.,.F.)
B_SPLINE_SURFACE_WITH_KNOTS((2,2),(3,2,3),(0.709727264436057,1.),(0.521815037222013,
0.538999630513413,0.539591283933454),.UNSPECIFIED.)
GEOMETRIC_REPRESENTATION_ITEM()
RATIONAL_B_SPLINE_SURFACE(((0.989362668575566,0.987015160230477,0.987570037304351,
0.987570037304351,0.987570037304351),(0.989362668575566,0.987015160230477,
0.987570037304351,0.987570037304351,0.987570037304351)))
REPRESENTATION_ITEM('')
SURFACE()
);
#2150=(
BOUNDED_SURFACE()
B_SPLINE_SURFACE(1,2,((#130460,#130461,#130462),(#130463,#130464,#130465)),
 .UNSPECIFIED.,.F.,.F.,.F.)
B_SPLINE_SURFACE_WITH_KNOTS((2,2),(3,3),(0.710192959007117,1.),(0.194132688793568,
0.211606804210307),.UNSPECIFIED.)
GEOMETRIC_REPRESENTATION_ITEM()
RATIONAL_B_SPLINE_SURFACE(((0.98984389658121,0.992516389311155,0.998189888755647),
(0.989843896581211,0.992516389311155,0.998189888755647)))
REPRESENTATION_ITEM('')
SURFACE()
);
#2151=(
BOUNDED_SURFACE()
B_SPLINE_SURFACE(1,2,((#130473,#130474,#130475,#130476,#130477),(#130478,
#130479,#130480,#130481,#130482)),.UNSPECIFIED.,.F.,.F.,.F.)
B_SPLINE_SURFACE_WITH_KNOTS((2,2),(3,2,3),(0.709727264437685,1.),(0.521815037222018,
0.538999630513411,0.539591283931768),.UNSPECIFIED.)
GEOMETRIC_REPRESENTATION_ITEM()
RATIONAL_B_SPLINE_SURFACE(((0.989362668575564,0.987015160230477,0.987570037304351,
0.987570037304351,0.987570037304351),(0.989362668575564,0.987015160230477,
0.987570037304351,0.987570037304351,0.987570037304351)))
REPRESENTATION_ITEM('')
SURFACE()
);
#2152=(
BOUNDED_SURFACE()
B_SPLINE_SURFACE(1,2,((#130493,#130494,#130495),(#130496,#130497,#130498)),
 .UNSPECIFIED.,.F.,.F.,.F.)
B_SPLINE_SURFACE_WITH_KNOTS((2,2),(3,3),(0.710192959007304,1.),(0.194132688793568,
0.211606804210308),.UNSPECIFIED.)
GEOMETRIC_REPRESENTATION_ITEM()
RATIONAL_B_SPLINE_SURFACE(((0.989843896581211,0.992516389311156,0.998189888755648),
(0.989843896581211,0.992516389311156,0.998189888755648)))
REPRESENTATION_ITEM('')
SURFACE()
);
#2153=(
BOUNDED_SURFACE()
B_SPLINE_SURFACE(1,2,((#130506,#130507,#130508,#130509,#130510),(#130511,
#130512,#130513,#130514,#130515)),.UNSPECIFIED.,.F.,.F.,.F.)
B_SPLINE_SURFACE_WITH_KNOTS((2,2),(3,2,3),(0.709727264371731,1.),(0.521815037222015,
0.538999630513411,0.539591283996905),.UNSPECIFIED.)
GEOMETRIC_REPRESENTATION_ITEM()
RATIONAL_B_SPLINE_SURFACE(((0.989362668575565,0.987015160230477,0.987570037304351,
0.987570037304351,0.987570037304351),(0.989362668575565,0.987015160230477,
0.987570037304351,0.987570037304351,0.987570037304351)))
REPRESENTATION_ITEM('')
SURFACE()
);
#2154=(
BOUNDED_SURFACE()
B_SPLINE_SURFACE(1,2,((#130526,#130527,#130528),(#130529,#130530,#130531)),
 .UNSPECIFIED.,.F.,.F.,.F.)
B_SPLINE_SURFACE_WITH_KNOTS((2,2),(3,3),(0.710192959006264,1.),(0.194132688793568,
0.211606804210307),.UNSPECIFIED.)
GEOMETRIC_REPRESENTATION_ITEM()
RATIONAL_B_SPLINE_SURFACE(((0.989843896581211,0.992516389311155,0.998189888755648),
(0.989843896581211,0.992516389311155,0.998189888755648)))
REPRESENTATION_ITEM('')
SURFACE()
);
#2155=(
BOUNDED_SURFACE()
B_SPLINE_SURFACE(1,2,((#130539,#130540,#130541,#130542,#130543),(#130544,
#130545,#130546,#130547,#130548)),.UNSPECIFIED.,.F.,.F.,.F.)
B_SPLINE_SURFACE_WITH_KNOTS((2,2),(3,2,3),(0.709727264448413,1.),(0.521815037222016,
0.538999630513412,0.539591283922137),.UNSPECIFIED.)
GEOMETRIC_REPRESENTATION_ITEM()
RATIONAL_B_SPLINE_SURFACE(((0.989362668575565,0.987015160230477,0.987570037304351,
0.987570037304351,0.987570037304351),(0.989362668575565,0.987015160230477,
0.987570037304351,0.987570037304351,0.987570037304351)))
REPRESENTATION_ITEM('')
SURFACE()
);
#2156=(
BOUNDED_SURFACE()
B_SPLINE_SURFACE(1,2,((#130559,#130560,#130561),(#130562,#130563,#130564)),
 .UNSPECIFIED.,.F.,.F.,.F.)
B_SPLINE_SURFACE_WITH_KNOTS((2,2),(3,3),(0.710192959008098,1.),(0.194132688793568,
0.211606804210307),.UNSPECIFIED.)
GEOMETRIC_REPRESENTATION_ITEM()
RATIONAL_B_SPLINE_SURFACE(((0.989843896581211,0.992516389311156,0.998189888755648),
(0.989843896581211,0.992516389311156,0.998189888755648)))
REPRESENTATION_ITEM('')
SURFACE()
);
#2157=(
BOUNDED_SURFACE()
B_SPLINE_SURFACE(1,2,((#130572,#130573,#130574,#130575,#130576),(#130577,
#130578,#130579,#130580,#130581)),.UNSPECIFIED.,.F.,.F.,.F.)
B_SPLINE_SURFACE_WITH_KNOTS((2,2),(3,2,3),(0.709727264440069,1.),(0.521815037222017,
0.538999630513412,0.539591283929231),.UNSPECIFIED.)
GEOMETRIC_REPRESENTATION_ITEM()
RATIONAL_B_SPLINE_SURFACE(((0.989362668575565,0.987015160230477,0.987570037304351,
0.987570037304351,0.987570037304351),(0.989362668575565,0.987015160230477,
0.987570037304351,0.987570037304351,0.987570037304351)))
REPRESENTATION_ITEM('')
SURFACE()
);
#2158=(
BOUNDED_SURFACE()
B_SPLINE_SURFACE(1,2,((#130592,#130593,#130594),(#130595,#130596,#130597)),
 .UNSPECIFIED.,.F.,.F.,.F.)
B_SPLINE_SURFACE_WITH_KNOTS((2,2),(3,3),(0.710192959006946,1.),(0.194132688793568,
0.211606804210307),.UNSPECIFIED.)
GEOMETRIC_REPRESENTATION_ITEM()
RATIONAL_B_SPLINE_SURFACE(((0.989843896581211,0.992516389311155,0.998189888755648),
(0.989843896581211,0.992516389311155,0.998189888755648)))
REPRESENTATION_ITEM('')
SURFACE()
);
#2159=(
BOUNDED_SURFACE()
B_SPLINE_SURFACE(1,2,((#130605,#130606,#130607,#130608,#130609),(#130610,
#130611,#130612,#130613,#130614)),.UNSPECIFIED.,.F.,.F.,.F.)
B_SPLINE_SURFACE_WITH_KNOTS((2,2),(3,2,3),(0.709727264416401,1.),(0.521815037222017,
0.538999630513411,0.539591283953233),.UNSPECIFIED.)
GEOMETRIC_REPRESENTATION_ITEM()
RATIONAL_B_SPLINE_SURFACE(((0.989362668575565,0.987015160230477,0.987570037304351,
0.987570037304351,0.987570037304351),(0.989362668575565,0.987015160230477,
0.987570037304351,0.987570037304351,0.987570037304351)))
REPRESENTATION_ITEM('')
SURFACE()
);
#2160=(
BOUNDED_SURFACE()
B_SPLINE_SURFACE(1,2,((#130625,#130626,#130627),(#130628,#130629,#130630)),
 .UNSPECIFIED.,.F.,.F.,.F.)
B_SPLINE_SURFACE_WITH_KNOTS((2,2),(3,3),(0.710192959007193,1.),(0.194132688793568,
0.211606804210307),.UNSPECIFIED.)
GEOMETRIC_REPRESENTATION_ITEM()
RATIONAL_B_SPLINE_SURFACE(((0.989843896581211,0.992516389311155,0.998189888755648),
(0.989843896581211,0.992516389311155,0.998189888755648)))
REPRESENTATION_ITEM('')
SURFACE()
);
#2161=(
BOUNDED_SURFACE()
B_SPLINE_SURFACE(1,2,((#130638,#130639,#130640,#130641,#130642),(#130643,
#130644,#130645,#130646,#130647)),.UNSPECIFIED.,.F.,.F.,.F.)
B_SPLINE_SURFACE_WITH_KNOTS((2,2),(3,2,3),(0.709727264443144,1.),(0.521815037222018,
0.538999630513411,0.539591283926624),.UNSPECIFIED.)
GEOMETRIC_REPRESENTATION_ITEM()
RATIONAL_B_SPLINE_SURFACE(((0.989362668575565,0.987015160230477,0.987570037304351,
0.987570037304351,0.987570037304351),(0.989362668575565,0.987015160230477,
0.987570037304351,0.987570037304351,0.987570037304351)))
REPRESENTATION_ITEM('')
SURFACE()
);
#2162=(
BOUNDED_SURFACE()
B_SPLINE_SURFACE(1,2,((#130658,#130659,#130660),(#130661,#130662,#130663)),
 .UNSPECIFIED.,.F.,.F.,.F.)
B_SPLINE_SURFACE_WITH_KNOTS((2,2),(3,3),(0.71019295900745,1.),(0.194132688793569,
0.211606804210307),.UNSPECIFIED.)
GEOMETRIC_REPRESENTATION_ITEM()
RATIONAL_B_SPLINE_SURFACE(((0.989843896581211,0.992516389311156,0.998189888755648),
(0.989843896581211,0.992516389311156,0.998189888755648)))
REPRESENTATION_ITEM('')
SURFACE()
);
#2163=(
BOUNDED_SURFACE()
B_SPLINE_SURFACE(1,2,((#130671,#130672,#130673,#130674,#130675),(#130676,
#130677,#130678,#130679,#130680)),.UNSPECIFIED.,.F.,.F.,.F.)
B_SPLINE_SURFACE_WITH_KNOTS((2,2),(3,2,3),(0.709727264402816,1.),(0.521815037222017,
0.53899963051341,0.539591283968033),.UNSPECIFIED.)
GEOMETRIC_REPRESENTATION_ITEM()
RATIONAL_B_SPLINE_SURFACE(((0.989362668575565,0.987015160230477,0.987570037304351,
0.987570037304351,0.987570037304351),(0.989362668575565,0.987015160230477,
0.987570037304351,0.987570037304351,0.987570037304351)))
REPRESENTATION_ITEM('')
SURFACE()
);
#2164=(
BOUNDED_SURFACE()
B_SPLINE_SURFACE(1,2,((#130691,#130692,#130693),(#130694,#130695,#130696)),
 .UNSPECIFIED.,.F.,.F.,.F.)
B_SPLINE_SURFACE_WITH_KNOTS((2,2),(3,3),(0.710192959008445,1.),(0.194132688793569,
0.211606804210309),.UNSPECIFIED.)
GEOMETRIC_REPRESENTATION_ITEM()
RATIONAL_B_SPLINE_SURFACE(((0.989843896581211,0.992516389311156,0.998189888755648),
(0.989843896581211,0.992516389311156,0.998189888755648)))
REPRESENTATION_ITEM('')
SURFACE()
);
#2165=(
BOUNDED_SURFACE()
B_SPLINE_SURFACE(1,2,((#130710,#130711,#130712,#130713,#130714),(#130715,
#130716,#130717,#130718,#130719)),.UNSPECIFIED.,.F.,.F.,.F.)
B_SPLINE_SURFACE_WITH_KNOTS((2,2),(3,2,3),(0.709727265150677,1.),(0.521815037222016,
0.53899963051341,0.539591284235917),.UNSPECIFIED.)
GEOMETRIC_REPRESENTATION_ITEM()
RATIONAL_B_SPLINE_SURFACE(((0.989362668575565,0.987015160230477,0.987570037304351,
0.987570037304351,0.987570037304351),(0.989362668575565,0.987015160230477,
0.987570037304351,0.987570037304351,0.987570037304351)))
REPRESENTATION_ITEM('')
SURFACE()
);
#2166=(
BOUNDED_SURFACE()
B_SPLINE_SURFACE(1,2,((#130721,#130722,#130723),(#130724,#130725,#130726)),
 .UNSPECIFIED.,.F.,.F.,.F.)
B_SPLINE_SURFACE_WITH_KNOTS((2,2),(3,3),(0.710318915638064,1.),(0.228780950825331,
0.245954053070933),.UNSPECIFIED.)
GEOMETRIC_REPRESENTATION_ITEM()
RATIONAL_B_SPLINE_SURFACE(((0.991889110260675,0.988307723348173,0.987624841600685),
(0.991889110260675,0.988307723348173,0.987624841600685)))
REPRESENTATION_ITEM('')
SURFACE()
);
#2167=(
BOUNDED_SURFACE()
B_SPLINE_SURFACE(1,2,((#130739,#130740,#130741,#130742,#130743),(#130744,
#130745,#130746,#130747,#130748)),.UNSPECIFIED.,.F.,.F.,.F.)
B_SPLINE_SURFACE_WITH_KNOTS((2,2),(3,2,3),(0.710192959008441,1.),(0.487259899888159,
0.5,0.504824515313956),.UNSPECIFIED.)
GEOMETRIC_REPRESENTATION_ITEM()
RATIONAL_B_SPLINE_SURFACE(((0.992651440660745,0.99552810727657,1.,0.998306550597157,
0.996841863226482),(0.992651440660745,0.99552810727657,1.,0.998306550597157,
0.996841863226482)))
REPRESENTATION_ITEM('')
SURFACE()
);
#2168=(
BOUNDED_SURFACE()
B_SPLINE_SURFACE(1,2,((#130770,#130771,#130772),(#130773,#130774,#130775)),
 .UNSPECIFIED.,.F.,.F.,.F.)
B_SPLINE_SURFACE_WITH_KNOTS((2,2),(3,3),(0.710318915638051,1.),(0.228780950825644,
0.245954053070933),.UNSPECIFIED.)
GEOMETRIC_REPRESENTATION_ITEM()
RATIONAL_B_SPLINE_SURFACE(((0.991889110260545,0.988307723348161,0.987624841600685),
(0.991889110260545,0.988307723348161,0.987624841600685)))
REPRESENTATION_ITEM('')
SURFACE()
);
#2169=(
BOUNDED_SURFACE()
B_SPLINE_SURFACE(1,2,((#130777,#130778,#130779,#130780,#130781),(#130782,
#130783,#130784,#130785,#130786)),.UNSPECIFIED.,.F.,.F.,.F.)
B_SPLINE_SURFACE_WITH_KNOTS((2,2),(3,2,3),(0.710192959008439,1.),(0.487259899888159,
0.5,0.504824515313956),.UNSPECIFIED.)
GEOMETRIC_REPRESENTATION_ITEM()
RATIONAL_B_SPLINE_SURFACE(((0.992651440660745,0.99552810727657,1.,0.998306550597157,
0.996841863226482),(0.992651440660745,0.99552810727657,1.,0.998306550597157,
0.996841863226482)))
REPRESENTATION_ITEM('')
SURFACE()
);
#2170=(
BOUNDED_SURFACE()
B_SPLINE_SURFACE(1,2,((#130808,#130809,#130810),(#130811,#130812,#130813)),
 .UNSPECIFIED.,.F.,.F.,.F.)
B_SPLINE_SURFACE_WITH_KNOTS((2,2),(3,3),(0.710318915638056,1.),(0.228780950825752,
0.245954053070933),.UNSPECIFIED.)
GEOMETRIC_REPRESENTATION_ITEM()
RATIONAL_B_SPLINE_SURFACE(((0.9918891102605,0.988307723348156,0.987624841600685),
(0.9918891102605,0.988307723348156,0.987624841600685)))
REPRESENTATION_ITEM('')
SURFACE()
);
#2171=(
BOUNDED_SURFACE()
B_SPLINE_SURFACE(1,2,((#130815,#130816,#130817,#130818,#130819),(#130820,
#130821,#130822,#130823,#130824)),.UNSPECIFIED.,.F.,.F.,.F.)
B_SPLINE_SURFACE_WITH_KNOTS((2,2),(3,2,3),(0.71019295900844,1.),(0.487259899888159,
0.5,0.504824515313956),.UNSPECIFIED.)
GEOMETRIC_REPRESENTATION_ITEM()
RATIONAL_B_SPLINE_SURFACE(((0.992651440660745,0.99552810727657,1.,0.998306550597157,
0.996841863226482),(0.992651440660745,0.99552810727657,1.,0.998306550597157,
0.996841863226482)))
REPRESENTATION_ITEM('')
SURFACE()
);
#2172=(
BOUNDED_SURFACE()
B_SPLINE_SURFACE(1,2,((#130846,#130847,#130848),(#130849,#130850,#130851)),
 .UNSPECIFIED.,.F.,.F.,.F.)
B_SPLINE_SURFACE_WITH_KNOTS((2,2),(3,3),(0.710318915638053,1.),(0.228780950825752,
0.245954053070933),.UNSPECIFIED.)
GEOMETRIC_REPRESENTATION_ITEM()
RATIONAL_B_SPLINE_SURFACE(((0.9918891102605,0.988307723348156,0.987624841600685),
(0.9918891102605,0.988307723348156,0.987624841600685)))
REPRESENTATION_ITEM('')
SURFACE()
);
#2173=(
BOUNDED_SURFACE()
B_SPLINE_SURFACE(1,2,((#130853,#130854,#130855,#130856,#130857),(#130858,
#130859,#130860,#130861,#130862)),.UNSPECIFIED.,.F.,.F.,.F.)
B_SPLINE_SURFACE_WITH_KNOTS((2,2),(3,2,3),(0.710192959008442,1.),(0.487259899888159,
0.5,0.504824515313956),.UNSPECIFIED.)
GEOMETRIC_REPRESENTATION_ITEM()
RATIONAL_B_SPLINE_SURFACE(((0.992651440660745,0.99552810727657,1.,0.998306550597157,
0.996841863226482),(0.992651440660745,0.99552810727657,1.,0.998306550597157,
0.996841863226482)))
REPRESENTATION_ITEM('')
SURFACE()
);
#2174=(
BOUNDED_SURFACE()
B_SPLINE_SURFACE(1,2,((#130884,#130885,#130886),(#130887,#130888,#130889)),
 .UNSPECIFIED.,.F.,.F.,.F.)
B_SPLINE_SURFACE_WITH_KNOTS((2,2),(3,3),(0.71031891563806,1.),(0.228780950825244,
0.245954053070933),.UNSPECIFIED.)
GEOMETRIC_REPRESENTATION_ITEM()
RATIONAL_B_SPLINE_SURFACE(((0.991889110260711,0.988307723348176,0.987624841600685),
(0.991889110260711,0.988307723348176,0.987624841600685)))
REPRESENTATION_ITEM('')
SURFACE()
);
#2175=(
BOUNDED_SURFACE()
B_SPLINE_SURFACE(1,2,((#130891,#130892,#130893,#130894,#130895),(#130896,
#130897,#130898,#130899,#130900)),.UNSPECIFIED.,.F.,.F.,.F.)
B_SPLINE_SURFACE_WITH_KNOTS((2,2),(3,2,3),(0.71019295900844,1.),(0.487259899888159,
0.5,0.504824515313956),.UNSPECIFIED.)
GEOMETRIC_REPRESENTATION_ITEM()
RATIONAL_B_SPLINE_SURFACE(((0.992651440660745,0.99552810727657,1.,0.998306550597157,
0.996841863226482),(0.992651440660745,0.99552810727657,1.,0.998306550597157,
0.996841863226482)))
REPRESENTATION_ITEM('')
SURFACE()
);
#2176=(
BOUNDED_SURFACE()
B_SPLINE_SURFACE(1,2,((#130922,#130923,#130924),(#130925,#130926,#130927)),
 .UNSPECIFIED.,.F.,.F.,.F.)
B_SPLINE_SURFACE_WITH_KNOTS((2,2),(3,3),(0.710318915638065,1.),(0.228780950825394,
0.245954053070933),.UNSPECIFIED.)
GEOMETRIC_REPRESENTATION_ITEM()
RATIONAL_B_SPLINE_SURFACE(((0.991889110260649,0.988307723348171,0.987624841600685),
(0.991889110260649,0.988307723348171,0.987624841600685)))
REPRESENTATION_ITEM('')
SURFACE()
);
#2177=(
BOUNDED_SURFACE()
B_SPLINE_SURFACE(1,2,((#130929,#130930,#130931,#130932,#130933),(#130934,
#130935,#130936,#130937,#130938)),.UNSPECIFIED.,.F.,.F.,.F.)
B_SPLINE_SURFACE_WITH_KNOTS((2,2),(3,2,3),(0.710192959008443,1.),(0.487259899888159,
0.5,0.504824515313788),.UNSPECIFIED.)
GEOMETRIC_REPRESENTATION_ITEM()
RATIONAL_B_SPLINE_SURFACE(((0.992651440660745,0.99552810727657,1.,0.998306550597216,
0.996841863226584),(0.992651440660745,0.99552810727657,1.,0.998306550597216,
0.996841863226584)))
REPRESENTATION_ITEM('')
SURFACE()
);
#2178=(
BOUNDED_SURFACE()
B_SPLINE_SURFACE(1,2,((#130960,#130961,#130962),(#130963,#130964,#130965)),
 .UNSPECIFIED.,.F.,.F.,.F.)
B_SPLINE_SURFACE_WITH_KNOTS((2,2),(3,3),(0.71031891563806,1.),(0.228780950825462,
0.245954053070933),.UNSPECIFIED.)
GEOMETRIC_REPRESENTATION_ITEM()
RATIONAL_B_SPLINE_SURFACE(((0.99188911026062,0.988307723348168,0.987624841600685),
(0.99188911026062,0.988307723348168,0.987624841600685)))
REPRESENTATION_ITEM('')
SURFACE()
);
#2179=(
BOUNDED_SURFACE()
B_SPLINE_SURFACE(1,2,((#130967,#130968,#130969,#130970,#130971),(#130972,
#130973,#130974,#130975,#130976)),.UNSPECIFIED.,.F.,.F.,.F.)
B_SPLINE_SURFACE_WITH_KNOTS((2,2),(3,2,3),(0.710192959008441,1.),(0.487259899888159,
0.5,0.504824515313956),.UNSPECIFIED.)
GEOMETRIC_REPRESENTATION_ITEM()
RATIONAL_B_SPLINE_SURFACE(((0.992651440660745,0.99552810727657,1.,0.998306550597157,
0.996841863226482),(0.992651440660745,0.99552810727657,1.,0.998306550597157,
0.996841863226482)))
REPRESENTATION_ITEM('')
SURFACE()
);
#2180=(
BOUNDED_SURFACE()
B_SPLINE_SURFACE(1,2,((#130998,#130999,#131000),(#131001,#131002,#131003)),
 .UNSPECIFIED.,.F.,.F.,.F.)
B_SPLINE_SURFACE_WITH_KNOTS((2,2),(3,3),(0.710318915638069,1.),(0.228780950825752,
0.245954053070933),.UNSPECIFIED.)
GEOMETRIC_REPRESENTATION_ITEM()
RATIONAL_B_SPLINE_SURFACE(((0.991889110260499,0.988307723348156,0.987624841600685),
(0.9918891102605,0.988307723348156,0.987624841600685)))
REPRESENTATION_ITEM('')
SURFACE()
);
#2181=(
BOUNDED_SURFACE()
B_SPLINE_SURFACE(1,2,((#131005,#131006,#131007,#131008,#131009),(#131010,
#131011,#131012,#131013,#131014)),.UNSPECIFIED.,.F.,.F.,.F.)
B_SPLINE_SURFACE_WITH_KNOTS((2,2),(3,2,3),(0.710192959008442,1.),(0.487259899888159,
0.5,0.504824515313956),.UNSPECIFIED.)
GEOMETRIC_REPRESENTATION_ITEM()
RATIONAL_B_SPLINE_SURFACE(((0.992651440660745,0.99552810727657,1.,0.998306550597157,
0.996841863226482),(0.992651440660745,0.99552810727657,1.,0.998306550597157,
0.996841863226482)))
REPRESENTATION_ITEM('')
SURFACE()
);
#2182=(
BOUNDED_SURFACE()
B_SPLINE_SURFACE(1,2,((#131036,#131037,#131038),(#131039,#131040,#131041)),
 .UNSPECIFIED.,.F.,.F.,.F.)
B_SPLINE_SURFACE_WITH_KNOTS((2,2),(3,3),(0.710318915638061,1.),(0.228780950825752,
0.245954053070933),.UNSPECIFIED.)
GEOMETRIC_REPRESENTATION_ITEM()
RATIONAL_B_SPLINE_SURFACE(((0.9918891102605,0.988307723348156,0.987624841600685),
(0.9918891102605,0.988307723348156,0.987624841600685)))
REPRESENTATION_ITEM('')
SURFACE()
);
#2183=(
BOUNDED_SURFACE()
B_SPLINE_SURFACE(1,2,((#131043,#131044,#131045,#131046,#131047),(#131048,
#131049,#131050,#131051,#131052)),.UNSPECIFIED.,.F.,.F.,.F.)
B_SPLINE_SURFACE_WITH_KNOTS((2,2),(3,2,3),(0.710192959008441,1.),(0.487259899888159,
0.5,0.504824515313956),.UNSPECIFIED.)
GEOMETRIC_REPRESENTATION_ITEM()
RATIONAL_B_SPLINE_SURFACE(((0.992651440660745,0.99552810727657,1.,0.998306550597157,
0.996841863226482),(0.992651440660745,0.99552810727657,1.,0.998306550597157,
0.996841863226482)))
REPRESENTATION_ITEM('')
SURFACE()
);
#2184=(
BOUNDED_SURFACE()
B_SPLINE_SURFACE(1,2,((#131074,#131075,#131076),(#131077,#131078,#131079)),
 .UNSPECIFIED.,.F.,.F.,.F.)
B_SPLINE_SURFACE_WITH_KNOTS((2,2),(3,3),(0.710318915638057,1.),(0.228780950825722,
0.245954053070933),.UNSPECIFIED.)
GEOMETRIC_REPRESENTATION_ITEM()
RATIONAL_B_SPLINE_SURFACE(((0.991889110260512,0.988307723348158,0.987624841600685),
(0.991889110260512,0.988307723348158,0.987624841600685)))
REPRESENTATION_ITEM('')
SURFACE()
);
#2185=(
BOUNDED_SURFACE()
B_SPLINE_SURFACE(1,2,((#131081,#131082,#131083,#131084,#131085),(#131086,
#131087,#131088,#131089,#131090)),.UNSPECIFIED.,.F.,.F.,.F.)
B_SPLINE_SURFACE_WITH_KNOTS((2,2),(3,2,3),(0.71019295900844,1.),(0.487259899888159,
0.5,0.504824515313956),.UNSPECIFIED.)
GEOMETRIC_REPRESENTATION_ITEM()
RATIONAL_B_SPLINE_SURFACE(((0.992651440660745,0.99552810727657,1.,0.998306550597157,
0.996841863226482),(0.992651440660745,0.99552810727657,1.,0.998306550597157,
0.996841863226482)))
REPRESENTATION_ITEM('')
SURFACE()
);
#2186=(
BOUNDED_SURFACE()
B_SPLINE_SURFACE(1,2,((#131112,#131113,#131114),(#131115,#131116,#131117)),
 .UNSPECIFIED.,.F.,.F.,.F.)
B_SPLINE_SURFACE_WITH_KNOTS((2,2),(3,3),(0.710318915638055,1.),(0.228780950825752,
0.245954053070933),.UNSPECIFIED.)
GEOMETRIC_REPRESENTATION_ITEM()
RATIONAL_B_SPLINE_SURFACE(((0.991889110260499,0.988307723348156,0.987624841600685),
(0.991889110260499,0.988307723348156,0.987624841600685)))
REPRESENTATION_ITEM('')
SURFACE()
);
#2187=(
BOUNDED_SURFACE()
B_SPLINE_SURFACE(1,2,((#131119,#131120,#131121,#131122,#131123),(#131124,
#131125,#131126,#131127,#131128)),.UNSPECIFIED.,.F.,.F.,.F.)
B_SPLINE_SURFACE_WITH_KNOTS((2,2),(3,2,3),(0.710192959008438,1.),(0.487259899888159,
0.5,0.504824515313956),.UNSPECIFIED.)
GEOMETRIC_REPRESENTATION_ITEM()
RATIONAL_B_SPLINE_SURFACE(((0.992651440660745,0.99552810727657,1.,0.998306550597157,
0.996841863226482),(0.992651440660745,0.99552810727657,1.,0.998306550597157,
0.996841863226482)))
REPRESENTATION_ITEM('')
SURFACE()
);
#2188=(
BOUNDED_SURFACE()
B_SPLINE_SURFACE(1,2,((#131150,#131151,#131152),(#131153,#131154,#131155)),
 .UNSPECIFIED.,.F.,.F.,.F.)
B_SPLINE_SURFACE_WITH_KNOTS((2,2),(3,3),(0.710318915638057,1.),(0.228780950825752,
0.245954053070933),.UNSPECIFIED.)
GEOMETRIC_REPRESENTATION_ITEM()
RATIONAL_B_SPLINE_SURFACE(((0.9918891102605,0.988307723348156,0.987624841600685),
(0.9918891102605,0.988307723348156,0.987624841600685)))
REPRESENTATION_ITEM('')
SURFACE()
);
#2189=(
BOUNDED_SURFACE()
B_SPLINE_SURFACE(1,2,((#131157,#131158,#131159,#131160,#131161),(#131162,
#131163,#131164,#131165,#131166)),.UNSPECIFIED.,.F.,.F.,.F.)
B_SPLINE_SURFACE_WITH_KNOTS((2,2),(3,2,3),(0.710192959008445,1.),(0.487259899888159,
0.5,0.504824515313956),.UNSPECIFIED.)
GEOMETRIC_REPRESENTATION_ITEM()
RATIONAL_B_SPLINE_SURFACE(((0.992651440660745,0.99552810727657,1.,0.998306550597157,
0.996841863226482),(0.992651440660745,0.99552810727657,1.,0.998306550597157,
0.996841863226482)))
REPRESENTATION_ITEM('')
SURFACE()
);
#2190=(
BOUNDED_SURFACE()
B_SPLINE_SURFACE(1,2,((#131188,#131189,#131190),(#131191,#131192,#131193)),
 .UNSPECIFIED.,.F.,.F.,.F.)
B_SPLINE_SURFACE_WITH_KNOTS((2,2),(3,3),(0.710318915638057,1.),(0.228780950825522,
0.245954053070933),.UNSPECIFIED.)
GEOMETRIC_REPRESENTATION_ITEM()
RATIONAL_B_SPLINE_SURFACE(((0.991889110260596,0.988307723348166,0.987624841600685),
(0.991889110260596,0.988307723348166,0.987624841600685)))
REPRESENTATION_ITEM('')
SURFACE()
);
#2191=(
BOUNDED_SURFACE()
B_SPLINE_SURFACE(1,2,((#131195,#131196,#131197,#131198,#131199),(#131200,
#131201,#131202,#131203,#131204)),.UNSPECIFIED.,.F.,.F.,.F.)
B_SPLINE_SURFACE_WITH_KNOTS((2,2),(3,2,3),(0.710192959008444,1.),(0.487259899888159,
0.5,0.504824515313956),.UNSPECIFIED.)
GEOMETRIC_REPRESENTATION_ITEM()
RATIONAL_B_SPLINE_SURFACE(((0.992651440660745,0.99552810727657,1.,0.998306550597157,
0.996841863226482),(0.992651440660745,0.99552810727657,1.,0.998306550597157,
0.996841863226482)))
REPRESENTATION_ITEM('')
SURFACE()
);
#2192=(
BOUNDED_SURFACE()
B_SPLINE_SURFACE(1,2,((#131226,#131227,#131228),(#131229,#131230,#131231)),
 .UNSPECIFIED.,.F.,.F.,.F.)
B_SPLINE_SURFACE_WITH_KNOTS((2,2),(3,3),(0.71031891563806,1.),(0.22878095082566,
0.245954053070933),.UNSPECIFIED.)
GEOMETRIC_REPRESENTATION_ITEM()
RATIONAL_B_SPLINE_SURFACE(((0.991889110260538,0.98830772334816,0.987624841600685),
(0.991889110260538,0.98830772334816,0.987624841600685)))
REPRESENTATION_ITEM('')
SURFACE()
);
#2193=(
BOUNDED_SURFACE()
B_SPLINE_SURFACE(1,2,((#131233,#131234,#131235,#131236,#131237),(#131238,
#131239,#131240,#131241,#131242)),.UNSPECIFIED.,.F.,.F.,.F.)
B_SPLINE_SURFACE_WITH_KNOTS((2,2),(3,2,3),(0.710192959008441,1.),(0.487259899888159,
0.5,0.504824515313956),.UNSPECIFIED.)
GEOMETRIC_REPRESENTATION_ITEM()
RATIONAL_B_SPLINE_SURFACE(((0.992651440660745,0.99552810727657,1.,0.998306550597157,
0.996841863226482),(0.992651440660745,0.99552810727657,1.,0.998306550597157,
0.996841863226482)))
REPRESENTATION_ITEM('')
SURFACE()
);
#2194=(
BOUNDED_SURFACE()
B_SPLINE_SURFACE(1,2,((#131264,#131265,#131266),(#131267,#131268,#131269)),
 .UNSPECIFIED.,.F.,.F.,.F.)
B_SPLINE_SURFACE_WITH_KNOTS((2,2),(3,3),(0.710318915638052,1.),(0.228780950825752,
0.245954053070933),.UNSPECIFIED.)
GEOMETRIC_REPRESENTATION_ITEM()
RATIONAL_B_SPLINE_SURFACE(((0.991889110260499,0.988307723348156,0.987624841600685),
(0.991889110260499,0.988307723348156,0.987624841600685)))
REPRESENTATION_ITEM('')
SURFACE()
);
#2195=(
BOUNDED_SURFACE()
B_SPLINE_SURFACE(1,2,((#131271,#131272,#131273,#131274,#131275),(#131276,
#131277,#131278,#131279,#131280)),.UNSPECIFIED.,.F.,.F.,.F.)
B_SPLINE_SURFACE_WITH_KNOTS((2,2),(3,2,3),(0.710192959008436,1.),(0.487259899888159,
0.5,0.504824515313956),.UNSPECIFIED.)
GEOMETRIC_REPRESENTATION_ITEM()
RATIONAL_B_SPLINE_SURFACE(((0.992651440660745,0.99552810727657,1.,0.998306550597157,
0.996841863226482),(0.992651440660745,0.99552810727657,1.,0.998306550597157,
0.996841863226482)))
REPRESENTATION_ITEM('')
SURFACE()
);
#2196=(
BOUNDED_SURFACE()
B_SPLINE_SURFACE(1,2,((#131302,#131303,#131304),(#131305,#131306,#131307)),
 .UNSPECIFIED.,.F.,.F.,.F.)
B_SPLINE_SURFACE_WITH_KNOTS((2,2),(3,3),(0.710318915638056,1.),(0.228780950825752,
0.245954053070933),.UNSPECIFIED.)
GEOMETRIC_REPRESENTATION_ITEM()
RATIONAL_B_SPLINE_SURFACE(((0.991889110260499,0.988307723348156,0.987624841600685),
(0.991889110260499,0.988307723348156,0.987624841600685)))
REPRESENTATION_ITEM('')
SURFACE()
);
#2197=(
BOUNDED_SURFACE()
B_SPLINE_SURFACE(1,2,((#131309,#131310,#131311,#131312,#131313),(#131314,
#131315,#131316,#131317,#131318)),.UNSPECIFIED.,.F.,.F.,.F.)
B_SPLINE_SURFACE_WITH_KNOTS((2,2),(3,2,3),(0.710192959008442,1.),(0.487259899888159,
0.5,0.504824515313956),.UNSPECIFIED.)
GEOMETRIC_REPRESENTATION_ITEM()
RATIONAL_B_SPLINE_SURFACE(((0.992651440660745,0.99552810727657,1.,0.998306550597157,
0.996841863226482),(0.992651440660745,0.99552810727657,1.,0.998306550597157,
0.996841863226482)))
REPRESENTATION_ITEM('')
SURFACE()
);
#2198=(
BOUNDED_SURFACE()
B_SPLINE_SURFACE(1,2,((#131340,#131341,#131342),(#131343,#131344,#131345)),
 .UNSPECIFIED.,.F.,.F.,.F.)
B_SPLINE_SURFACE_WITH_KNOTS((2,2),(3,3),(0.710318915638057,1.),(0.228780950825752,
0.245954053070933),.UNSPECIFIED.)
GEOMETRIC_REPRESENTATION_ITEM()
RATIONAL_B_SPLINE_SURFACE(((0.991889110260499,0.988307723348156,0.987624841600685),
(0.991889110260499,0.988307723348156,0.987624841600685)))
REPRESENTATION_ITEM('')
SURFACE()
);
#2199=(
BOUNDED_SURFACE()
B_SPLINE_SURFACE(1,2,((#131347,#131348,#131349,#131350,#131351),(#131352,
#131353,#131354,#131355,#131356)),.UNSPECIFIED.,.F.,.F.,.F.)
B_SPLINE_SURFACE_WITH_KNOTS((2,2),(3,2,3),(0.710192959008438,1.),(0.487259899888159,
0.5,0.504824515313956),.UNSPECIFIED.)
GEOMETRIC_REPRESENTATION_ITEM()
RATIONAL_B_SPLINE_SURFACE(((0.992651440660745,0.99552810727657,1.,0.998306550597157,
0.996841863226482),(0.992651440660745,0.99552810727657,1.,0.998306550597157,
0.996841863226482)))
REPRESENTATION_ITEM('')
SURFACE()
);
#2200=(
BOUNDED_SURFACE()
B_SPLINE_SURFACE(1,2,((#131378,#131379,#131380),(#131381,#131382,#131383)),
 .UNSPECIFIED.,.F.,.F.,.F.)
B_SPLINE_SURFACE_WITH_KNOTS((2,2),(3,3),(0.710318915638058,1.),(0.228780950825752,
0.245954053070933),.UNSPECIFIED.)
GEOMETRIC_REPRESENTATION_ITEM()
RATIONAL_B_SPLINE_SURFACE(((0.9918891102605,0.988307723348156,0.987624841600685),
(0.9918891102605,0.988307723348156,0.987624841600685)))
REPRESENTATION_ITEM('')
SURFACE()
);
#2201=(
BOUNDED_SURFACE()
B_SPLINE_SURFACE(1,2,((#131385,#131386,#131387,#131388,#131389),(#131390,
#131391,#131392,#131393,#131394)),.UNSPECIFIED.,.F.,.F.,.F.)
B_SPLINE_SURFACE_WITH_KNOTS((2,2),(3,2,3),(0.710192959008441,1.),(0.487259899888159,
0.5,0.504824515313956),.UNSPECIFIED.)
GEOMETRIC_REPRESENTATION_ITEM()
RATIONAL_B_SPLINE_SURFACE(((0.992651440660745,0.99552810727657,1.,0.998306550597157,
0.996841863226482),(0.992651440660745,0.99552810727657,1.,0.998306550597157,
0.996841863226482)))
REPRESENTATION_ITEM('')
SURFACE()
);
#2202=(
BOUNDED_SURFACE()
B_SPLINE_SURFACE(1,2,((#131416,#131417,#131418),(#131419,#131420,#131421)),
 .UNSPECIFIED.,.F.,.F.,.F.)
B_SPLINE_SURFACE_WITH_KNOTS((2,2),(3,3),(0.710318915638058,1.),(0.228780950825752,
0.245954053070933),.UNSPECIFIED.)
GEOMETRIC_REPRESENTATION_ITEM()
RATIONAL_B_SPLINE_SURFACE(((0.9918891102605,0.988307723348156,0.987624841600685),
(0.9918891102605,0.988307723348156,0.987624841600685)))
REPRESENTATION_ITEM('')
SURFACE()
);
#2203=(
BOUNDED_SURFACE()
B_SPLINE_SURFACE(1,2,((#131423,#131424,#131425,#131426,#131427),(#131428,
#131429,#131430,#131431,#131432)),.UNSPECIFIED.,.F.,.F.,.F.)
B_SPLINE_SURFACE_WITH_KNOTS((2,2),(3,2,3),(0.710192959008441,1.),(0.487259899888159,
0.5,0.504824515313956),.UNSPECIFIED.)
GEOMETRIC_REPRESENTATION_ITEM()
RATIONAL_B_SPLINE_SURFACE(((0.992651440660745,0.99552810727657,1.,0.998306550597157,
0.996841863226482),(0.992651440660745,0.99552810727657,1.,0.998306550597157,
0.996841863226482)))
REPRESENTATION_ITEM('')
SURFACE()
);
#2204=(
BOUNDED_SURFACE()
B_SPLINE_SURFACE(1,2,((#131454,#131455,#131456),(#131457,#131458,#131459)),
 .UNSPECIFIED.,.F.,.F.,.F.)
B_SPLINE_SURFACE_WITH_KNOTS((2,2),(3,3),(0.710318915638061,1.),(0.228780950825752,
0.245954053070933),.UNSPECIFIED.)
GEOMETRIC_REPRESENTATION_ITEM()
RATIONAL_B_SPLINE_SURFACE(((0.991889110260499,0.988307723348156,0.987624841600685),
(0.991889110260499,0.988307723348156,0.987624841600685)))
REPRESENTATION_ITEM('')
SURFACE()
);
#2205=(
BOUNDED_SURFACE()
B_SPLINE_SURFACE(1,2,((#131461,#131462,#131463,#131464,#131465),(#131466,
#131467,#131468,#131469,#131470)),.UNSPECIFIED.,.F.,.F.,.F.)
B_SPLINE_SURFACE_WITH_KNOTS((2,2),(3,2,3),(0.710192959008439,1.),(0.487259899888159,
0.5,0.504824515313956),.UNSPECIFIED.)
GEOMETRIC_REPRESENTATION_ITEM()
RATIONAL_B_SPLINE_SURFACE(((0.992651440660745,0.99552810727657,1.,0.998306550597157,
0.996841863226482),(0.992651440660745,0.99552810727657,1.,0.998306550597157,
0.996841863226482)))
REPRESENTATION_ITEM('')
SURFACE()
);
#2206=(
BOUNDED_SURFACE()
B_SPLINE_SURFACE(1,2,((#131492,#131493,#131494),(#131495,#131496,#131497)),
 .UNSPECIFIED.,.F.,.F.,.F.)
B_SPLINE_SURFACE_WITH_KNOTS((2,2),(3,3),(0.710318915638065,1.),(0.228780950825752,
0.245954053070933),.UNSPECIFIED.)
GEOMETRIC_REPRESENTATION_ITEM()
RATIONAL_B_SPLINE_SURFACE(((0.9918891102605,0.988307723348156,0.987624841600685),
(0.9918891102605,0.988307723348156,0.987624841600685)))
REPRESENTATION_ITEM('')
SURFACE()
);
#2207=(
BOUNDED_SURFACE()
B_SPLINE_SURFACE(1,2,((#131499,#131500,#131501,#131502,#131503),(#131504,
#131505,#131506,#131507,#131508)),.UNSPECIFIED.,.F.,.F.,.F.)
B_SPLINE_SURFACE_WITH_KNOTS((2,2),(3,2,3),(0.710192959007031,1.),(0.487259899888159,
0.5,0.504824515313956),.UNSPECIFIED.)
GEOMETRIC_REPRESENTATION_ITEM()
RATIONAL_B_SPLINE_SURFACE(((0.992651440660745,0.99552810727657,1.,0.998306550597157,
0.996841863226482),(0.992651440660745,0.99552810727657,1.,0.998306550597157,
0.996841863226482)))
REPRESENTATION_ITEM('')
SURFACE()
);
#2208=(
BOUNDED_SURFACE()
B_SPLINE_SURFACE(1,2,((#131530,#131531,#131532),(#131533,#131534,#131535)),
 .UNSPECIFIED.,.F.,.F.,.F.)
B_SPLINE_SURFACE_WITH_KNOTS((2,2),(3,3),(0.710318915640078,1.),(0.228780950825752,
0.245954053070908),.UNSPECIFIED.)
GEOMETRIC_REPRESENTATION_ITEM()
RATIONAL_B_SPLINE_SURFACE(((0.991889110260499,0.988307723348161,0.987624841600687),
(0.991889110260499,0.988307723348161,0.987624841600687)))
REPRESENTATION_ITEM('')
SURFACE()
);
#2209=(
BOUNDED_SURFACE()
B_SPLINE_SURFACE(1,2,((#131537,#131538,#131539,#131540,#131541),(#131542,
#131543,#131544,#131545,#131546)),.UNSPECIFIED.,.F.,.F.,.F.)
B_SPLINE_SURFACE_WITH_KNOTS((2,2),(3,2,3),(0.710192959007785,1.),(0.487259899888159,
0.5,0.504824515313955),.UNSPECIFIED.)
GEOMETRIC_REPRESENTATION_ITEM()
RATIONAL_B_SPLINE_SURFACE(((0.992651440660745,0.99552810727657,1.,0.998306550597157,
0.996841863226483),(0.992651440660745,0.99552810727657,1.,0.998306550597157,
0.996841863226483)))
REPRESENTATION_ITEM('')
SURFACE()
);
#2210=(
BOUNDED_SURFACE()
B_SPLINE_SURFACE(1,2,((#131568,#131569,#131570),(#131571,#131572,#131573)),
 .UNSPECIFIED.,.F.,.F.,.F.)
B_SPLINE_SURFACE_WITH_KNOTS((2,2),(3,3),(0.710318915638065,1.),(0.228780950825753,
0.245954053070934),.UNSPECIFIED.)
GEOMETRIC_REPRESENTATION_ITEM()
RATIONAL_B_SPLINE_SURFACE(((0.991889110260499,0.988307723348156,0.987624841600685),
(0.991889110260499,0.988307723348156,0.987624841600685)))
REPRESENTATION_ITEM('')
SURFACE()
);
#2211=(
BOUNDED_SURFACE()
B_SPLINE_SURFACE(1,2,((#131575,#131576,#131577,#131578,#131579),(#131580,
#131581,#131582,#131583,#131584)),.UNSPECIFIED.,.F.,.F.,.F.)
B_SPLINE_SURFACE_WITH_KNOTS((2,2),(3,2,3),(0.710192959008349,1.),(0.487259899888158,
0.5,0.504824515313955),.UNSPECIFIED.)
GEOMETRIC_REPRESENTATION_ITEM()
RATIONAL_B_SPLINE_SURFACE(((0.992651440660745,0.995528107276569,1.,0.998306550597157,
0.996841863226483),(0.992651440660745,0.995528107276569,1.,0.998306550597157,
0.996841863226483)))
REPRESENTATION_ITEM('')
SURFACE()
);
#2212=(
BOUNDED_SURFACE()
B_SPLINE_SURFACE(1,2,((#131606,#131607,#131608),(#131609,#131610,#131611)),
 .UNSPECIFIED.,.F.,.F.,.F.)
B_SPLINE_SURFACE_WITH_KNOTS((2,2),(3,3),(0.710318915638056,1.),(0.228780950825753,
0.245954053070934),.UNSPECIFIED.)
GEOMETRIC_REPRESENTATION_ITEM()
RATIONAL_B_SPLINE_SURFACE(((0.991889110260499,0.988307723348156,0.987624841600685),
(0.991889110260499,0.988307723348156,0.987624841600685)))
REPRESENTATION_ITEM('')
SURFACE()
);
#2213=(
BOUNDED_SURFACE()
B_SPLINE_SURFACE(1,2,((#131613,#131614,#131615,#131616,#131617),(#131618,
#131619,#131620,#131621,#131622)),.UNSPECIFIED.,.F.,.F.,.F.)
B_SPLINE_SURFACE_WITH_KNOTS((2,2),(3,2,3),(0.710192959008359,1.),(0.487259899888158,
0.5,0.504824515313955),.UNSPECIFIED.)
GEOMETRIC_REPRESENTATION_ITEM()
RATIONAL_B_SPLINE_SURFACE(((0.992651440660745,0.995528107276569,1.,0.998306550597157,
0.996841863226483),(0.992651440660745,0.995528107276569,1.,0.998306550597157,
0.996841863226483)))
REPRESENTATION_ITEM('')
SURFACE()
);
#2214=(
BOUNDED_SURFACE()
B_SPLINE_SURFACE(1,2,((#131644,#131645,#131646),(#131647,#131648,#131649)),
 .UNSPECIFIED.,.F.,.F.,.F.)
B_SPLINE_SURFACE_WITH_KNOTS((2,2),(3,3),(0.710318915638063,1.),(0.228780950825753,
0.245954053070934),.UNSPECIFIED.)
GEOMETRIC_REPRESENTATION_ITEM()
RATIONAL_B_SPLINE_SURFACE(((0.991889110260499,0.988307723348156,0.987624841600685),
(0.991889110260499,0.988307723348156,0.987624841600685)))
REPRESENTATION_ITEM('')
SURFACE()
);
#2215=(
BOUNDED_SURFACE()
B_SPLINE_SURFACE(1,2,((#131651,#131652,#131653,#131654,#131655),(#131656,
#131657,#131658,#131659,#131660)),.UNSPECIFIED.,.F.,.F.,.F.)
B_SPLINE_SURFACE_WITH_KNOTS((2,2),(3,2,3),(0.710192959008363,1.),(0.487259899888158,
0.5,0.504824515313955),.UNSPECIFIED.)
GEOMETRIC_REPRESENTATION_ITEM()
RATIONAL_B_SPLINE_SURFACE(((0.992651440660745,0.995528107276569,1.,0.998306550597157,
0.996841863226482),(0.992651440660745,0.995528107276569,1.,0.998306550597157,
0.996841863226482)))
REPRESENTATION_ITEM('')
SURFACE()
);
#2216=(
BOUNDED_SURFACE()
B_SPLINE_SURFACE(1,2,((#131682,#131683,#131684),(#131685,#131686,#131687)),
 .UNSPECIFIED.,.F.,.F.,.F.)
B_SPLINE_SURFACE_WITH_KNOTS((2,2),(3,3),(0.710318915638062,1.),(0.228780950825753,
0.245954053070934),.UNSPECIFIED.)
GEOMETRIC_REPRESENTATION_ITEM()
RATIONAL_B_SPLINE_SURFACE(((0.991889110260499,0.988307723348156,0.987624841600685),
(0.991889110260499,0.988307723348156,0.987624841600685)))
REPRESENTATION_ITEM('')
SURFACE()
);
#2217=(
BOUNDED_SURFACE()
B_SPLINE_SURFACE(1,2,((#131689,#131690,#131691,#131692,#131693),(#131694,
#131695,#131696,#131697,#131698)),.UNSPECIFIED.,.F.,.F.,.F.)
B_SPLINE_SURFACE_WITH_KNOTS((2,2),(3,2,3),(0.710192959007758,1.),(0.487259899888158,
0.5,0.504824515313955),.UNSPECIFIED.)
GEOMETRIC_REPRESENTATION_ITEM()
RATIONAL_B_SPLINE_SURFACE(((0.992651440660745,0.995528107276569,1.,0.998306550597157,
0.996841863226483),(0.992651440660745,0.995528107276569,1.,0.998306550597157,
0.996841863226483)))
REPRESENTATION_ITEM('')
SURFACE()
);
#2218=(
BOUNDED_SURFACE()
B_SPLINE_SURFACE(1,2,((#131720,#131721,#131722),(#131723,#131724,#131725)),
 .UNSPECIFIED.,.F.,.F.,.F.)
B_SPLINE_SURFACE_WITH_KNOTS((2,2),(3,3),(0.710318915638052,1.),(0.228780950825681,
0.245954053070934),.UNSPECIFIED.)
GEOMETRIC_REPRESENTATION_ITEM()
RATIONAL_B_SPLINE_SURFACE(((0.991889110260529,0.988307723348159,0.987624841600685),
(0.991889110260529,0.988307723348159,0.987624841600685)))
REPRESENTATION_ITEM('')
SURFACE()
);
#2219=(
BOUNDED_SURFACE()
B_SPLINE_SURFACE(1,2,((#131727,#131728,#131729,#131730,#131731),(#131732,
#131733,#131734,#131735,#131736)),.UNSPECIFIED.,.F.,.F.,.F.)
B_SPLINE_SURFACE_WITH_KNOTS((2,2),(3,2,3),(0.710192959008391,1.),(0.487259899888158,
0.5,0.504824515313955),.UNSPECIFIED.)
GEOMETRIC_REPRESENTATION_ITEM()
RATIONAL_B_SPLINE_SURFACE(((0.992651440660745,0.99552810727657,1.,0.998306550597158,
0.996841863226483),(0.992651440660745,0.99552810727657,1.,0.998306550597158,
0.996841863226483)))
REPRESENTATION_ITEM('')
SURFACE()
);
#2220=(
BOUNDED_SURFACE()
B_SPLINE_SURFACE(1,2,((#131758,#131759,#131760),(#131761,#131762,#131763)),
 .UNSPECIFIED.,.F.,.F.,.F.)
B_SPLINE_SURFACE_WITH_KNOTS((2,2),(3,3),(0.710318915638062,1.),(0.22878095082552,
0.245954053071561),.UNSPECIFIED.)
GEOMETRIC_REPRESENTATION_ITEM()
RATIONAL_B_SPLINE_SURFACE(((0.991889110260596,0.988307723348035,0.987624841600635),
(0.991889110260596,0.988307723348035,0.987624841600635)))
REPRESENTATION_ITEM('')
SURFACE()
);
#2221=(
BOUNDED_SURFACE()
B_SPLINE_SURFACE(1,2,((#131765,#131766,#131767,#131768,#131769),(#131770,
#131771,#131772,#131773,#131774)),.UNSPECIFIED.,.F.,.F.,.F.)
B_SPLINE_SURFACE_WITH_KNOTS((2,2),(3,2,3),(0.710192959008374,1.),(0.487259899888158,
0.5,0.504824515313955),.UNSPECIFIED.)
GEOMETRIC_REPRESENTATION_ITEM()
RATIONAL_B_SPLINE_SURFACE(((0.992651440660745,0.995528107276569,1.,0.998306550597157,
0.996841863226483),(0.992651440660745,0.995528107276569,1.,0.998306550597157,
0.996841863226483)))
REPRESENTATION_ITEM('')
SURFACE()
);
#2222=(
BOUNDED_SURFACE()
B_SPLINE_SURFACE(1,2,((#131796,#131797,#131798),(#131799,#131800,#131801)),
 .UNSPECIFIED.,.F.,.F.,.F.)
B_SPLINE_SURFACE_WITH_KNOTS((2,2),(3,3),(0.710318915638058,1.),(0.228780950825311,
0.245954053070934),.UNSPECIFIED.)
GEOMETRIC_REPRESENTATION_ITEM()
RATIONAL_B_SPLINE_SURFACE(((0.991889110260684,0.988307723348174,0.987624841600685),
(0.991889110260683,0.988307723348174,0.987624841600685)))
REPRESENTATION_ITEM('')
SURFACE()
);
#2223=(
BOUNDED_SURFACE()
B_SPLINE_SURFACE(1,2,((#131803,#131804,#131805,#131806,#131807),(#131808,
#131809,#131810,#131811,#131812)),.UNSPECIFIED.,.F.,.F.,.F.)
B_SPLINE_SURFACE_WITH_KNOTS((2,2),(3,2,3),(0.710192959008376,1.),(0.487259899888158,
0.5,0.504824515313552),.UNSPECIFIED.)
GEOMETRIC_REPRESENTATION_ITEM()
RATIONAL_B_SPLINE_SURFACE(((0.992651440660745,0.995528107276569,1.,0.998306550597299,
0.996841863226727),(0.992651440660745,0.995528107276569,1.,0.998306550597299,
0.996841863226727)))
REPRESENTATION_ITEM('')
SURFACE()
);
#2224=(
BOUNDED_SURFACE()
B_SPLINE_SURFACE(1,2,((#131823,#131824,#131825),(#131826,#131827,#131828)),
 .UNSPECIFIED.,.F.,.F.,.F.)
B_SPLINE_SURFACE_WITH_KNOTS((2,2),(3,3),(0.,0.289807040991559),(0.53899963051341,
0.556316102183953),.UNSPECIFIED.)
GEOMETRIC_REPRESENTATION_ITEM()
RATIONAL_B_SPLINE_SURFACE(((0.987570037304351,0.988129172627919,0.99163541140107),
(0.987570037304351,0.988129172627919,0.99163541140107)))
REPRESENTATION_ITEM('')
SURFACE()
);
#2225=(
BOUNDED_SURFACE()
B_SPLINE_SURFACE(1,2,((#131837,#131838,#131839,#131840,#131841),(#131842,
#131843,#131844,#131845,#131846)),.UNSPECIFIED.,.F.,.F.,.F.)
B_SPLINE_SURFACE_WITH_KNOTS((2,2),(3,2,3),(0.,0.290279631762495),(0.176864064841898,
0.194132688793569,0.194731236520879),.UNSPECIFIED.)
GEOMETRIC_REPRESENTATION_ITEM()
RATIONAL_B_SPLINE_SURFACE(((0.987492606357657,0.987202831733786,0.989843896581211,
0.989843896581211,0.989843896581211),(0.987492606357657,0.987202831733786,
0.989843896581211,0.989843896581211,0.989843896581211)))
REPRESENTATION_ITEM('')
SURFACE()
);
#2226=(
BOUNDED_SURFACE()
B_SPLINE_SURFACE(1,2,((#131855,#131856,#131857),(#131858,#131859,#131860),
(#131861,#131862,#131863)),.UNSPECIFIED.,.F.,.F.,.F.)
B_SPLINE_SURFACE_WITH_KNOTS((2,1,2),(3,3),(-0.0028980704099156,0.,0.28980704099156),
(0.53899963051341,0.556316102183953),.UNSPECIFIED.)
GEOMETRIC_REPRESENTATION_ITEM()
RATIONAL_B_SPLINE_SURFACE(((0.987570037304351,0.988129172627919,0.99163541140107),
(0.987570037304351,0.988129172627919,0.99163541140107),(0.987570037304351,
0.988129172627919,0.99163541140107)))
REPRESENTATION_ITEM('')
SURFACE()
);
#2227=(
BOUNDED_SURFACE()
B_SPLINE_SURFACE(1,2,((#131865,#131866,#131867,#131868,#131869),(#131870,
#131871,#131872,#131873,#131874)),.UNSPECIFIED.,.F.,.F.,.F.)
B_SPLINE_SURFACE_WITH_KNOTS((2,2),(3,2,3),(0.,0.290279631761532),(0.176864064841898,
0.194132688793569,0.194731236519916),.UNSPECIFIED.)
GEOMETRIC_REPRESENTATION_ITEM()
RATIONAL_B_SPLINE_SURFACE(((0.987492606357657,0.987202831733786,0.989843896581211,
0.989843896581211,0.989843896581211),(0.987492606357657,0.987202831733786,
0.989843896581211,0.989843896581211,0.989843896581211)))
REPRESENTATION_ITEM('')
SURFACE()
);
#2228=(
BOUNDED_SURFACE()
B_SPLINE_SURFACE(1,2,((#131883,#131884,#131885),(#131886,#131887,#131888),
(#131889,#131890,#131891)),.UNSPECIFIED.,.F.,.F.,.F.)
B_SPLINE_SURFACE_WITH_KNOTS((2,1,2),(3,3),(-0.00289807040992491,0.,0.289807040992491),
(0.53899963051341,0.556316102183953),.UNSPECIFIED.)
GEOMETRIC_REPRESENTATION_ITEM()
RATIONAL_B_SPLINE_SURFACE(((0.987570037304351,0.988129172627919,0.99163541140107),
(0.987570037304351,0.988129172627919,0.99163541140107),(0.987570037304351,
0.988129172627919,0.99163541140107)))
REPRESENTATION_ITEM('')
SURFACE()
);
#2229=(
BOUNDED_SURFACE()
B_SPLINE_SURFACE(1,2,((#131893,#131894,#131895,#131896,#131897),(#131898,
#131899,#131900,#131901,#131902)),.UNSPECIFIED.,.F.,.F.,.F.)
B_SPLINE_SURFACE_WITH_KNOTS((2,2),(3,2,3),(0.,0.290279631742111),(0.176864064841898,
0.194132688793569,0.194731236500496),.UNSPECIFIED.)
GEOMETRIC_REPRESENTATION_ITEM()
RATIONAL_B_SPLINE_SURFACE(((0.987492606357657,0.987202831733786,0.989843896581211,
0.989843896581211,0.989843896581211),(0.987492606357657,0.987202831733785,
0.989843896581211,0.989843896581211,0.989843896581211)))
REPRESENTATION_ITEM('')
SURFACE()
);
#2230=(
BOUNDED_SURFACE()
B_SPLINE_SURFACE(1,2,((#131911,#131912,#131913),(#131914,#131915,#131916),
(#131917,#131918,#131919)),.UNSPECIFIED.,.F.,.F.,.F.)
B_SPLINE_SURFACE_WITH_KNOTS((2,1,2),(3,3),(-0.00289807040992489,0.,0.289807040992489),
(0.53899963051341,0.556316102183953),.UNSPECIFIED.)
GEOMETRIC_REPRESENTATION_ITEM()
RATIONAL_B_SPLINE_SURFACE(((0.987570037304351,0.988129172627919,0.99163541140107),
(0.987570037304351,0.988129172627919,0.99163541140107),(0.987570037304351,
0.988129172627919,0.99163541140107)))
REPRESENTATION_ITEM('')
SURFACE()
);
#2231=(
BOUNDED_SURFACE()
B_SPLINE_SURFACE(1,2,((#131921,#131922,#131923,#131924,#131925),(#131926,
#131927,#131928,#131929,#131930)),.UNSPECIFIED.,.F.,.F.,.F.)
B_SPLINE_SURFACE_WITH_KNOTS((2,2),(3,2,3),(0.,0.290279631766158),(0.176864064841898,
0.194132688793569,0.194731236524534),.UNSPECIFIED.)
GEOMETRIC_REPRESENTATION_ITEM()
RATIONAL_B_SPLINE_SURFACE(((0.987492606357657,0.987202831733786,0.989843896581211,
0.989843896581211,0.989843896581211),(0.987492606357657,0.987202831733786,
0.989843896581211,0.989843896581211,0.989843896581211)))
REPRESENTATION_ITEM('')
SURFACE()
);
#2232=(
BOUNDED_SURFACE()
B_SPLINE_SURFACE(1,2,((#131939,#131940,#131941),(#131942,#131943,#131944),
(#131945,#131946,#131947)),.UNSPECIFIED.,.F.,.F.,.F.)
B_SPLINE_SURFACE_WITH_KNOTS((2,1,2),(3,3),(-0.00289807040992489,0.,0.289807040992489),
(0.53899963051341,0.556316102183953),.UNSPECIFIED.)
GEOMETRIC_REPRESENTATION_ITEM()
RATIONAL_B_SPLINE_SURFACE(((0.987570037304351,0.988129172627919,0.99163541140107),
(0.987570037304351,0.988129172627919,0.99163541140107),(0.987570037304351,
0.988129172627919,0.99163541140107)))
REPRESENTATION_ITEM('')
SURFACE()
);
#2233=(
BOUNDED_SURFACE()
B_SPLINE_SURFACE(1,2,((#131949,#131950,#131951,#131952,#131953),(#131954,
#131955,#131956,#131957,#131958)),.UNSPECIFIED.,.F.,.F.,.F.)
B_SPLINE_SURFACE_WITH_KNOTS((2,2),(3,2,3),(0.,0.290279631775689),(0.176864064841898,
0.194132688793569,0.194731236534068),.UNSPECIFIED.)
GEOMETRIC_REPRESENTATION_ITEM()
RATIONAL_B_SPLINE_SURFACE(((0.987492606357657,0.987202831733786,0.989843896581211,
0.989843896581211,0.989843896581211),(0.987492606357657,0.987202831733786,
0.989843896581211,0.989843896581211,0.989843896581211)))
REPRESENTATION_ITEM('')
SURFACE()
);
#2234=(
BOUNDED_SURFACE()
B_SPLINE_SURFACE(1,2,((#131967,#131968,#131969),(#131970,#131971,#131972),
(#131973,#131974,#131975)),.UNSPECIFIED.,.F.,.F.,.F.)
B_SPLINE_SURFACE_WITH_KNOTS((2,1,2),(3,3),(-0.0028980704099307,0.,0.28980704099307),
(0.53899963051341,0.556316102183953),.UNSPECIFIED.)
GEOMETRIC_REPRESENTATION_ITEM()
RATIONAL_B_SPLINE_SURFACE(((0.987570037304351,0.988129172627919,0.99163541140107),
(0.987570037304351,0.988129172627919,0.99163541140107),(0.987570037304351,
0.988129172627919,0.99163541140107)))
REPRESENTATION_ITEM('')
SURFACE()
);
#2235=(
BOUNDED_SURFACE()
B_SPLINE_SURFACE(1,2,((#131977,#131978,#131979,#131980,#131981),(#131982,
#131983,#131984,#131985,#131986)),.UNSPECIFIED.,.F.,.F.,.F.)
B_SPLINE_SURFACE_WITH_KNOTS((2,2),(3,2,3),(0.,0.290279631757529),(0.176864064841898,
0.194132688793569,0.194731236515912),.UNSPECIFIED.)
GEOMETRIC_REPRESENTATION_ITEM()
RATIONAL_B_SPLINE_SURFACE(((0.987492606357657,0.987202831733786,0.989843896581211,
0.989843896581211,0.989843896581211),(0.987492606357657,0.987202831733786,
0.989843896581211,0.989843896581211,0.989843896581211)))
REPRESENTATION_ITEM('')
SURFACE()
);
#2236=(
BOUNDED_SURFACE()
B_SPLINE_SURFACE(1,2,((#131995,#131996,#131997),(#131998,#131999,#132000),
(#132001,#132002,#132003)),.UNSPECIFIED.,.F.,.F.,.F.)
B_SPLINE_SURFACE_WITH_KNOTS((2,1,2),(3,3),(-0.00289807040992488,0.,0.289807040992488),
(0.53899963051341,0.556316102183954),.UNSPECIFIED.)
GEOMETRIC_REPRESENTATION_ITEM()
RATIONAL_B_SPLINE_SURFACE(((0.987570037304351,0.988129172627919,0.99163541140107),
(0.987570037304351,0.988129172627919,0.99163541140107),(0.987570037304351,
0.988129172627919,0.99163541140107)))
REPRESENTATION_ITEM('')
SURFACE()
);
#2237=(
BOUNDED_SURFACE()
B_SPLINE_SURFACE(1,2,((#132005,#132006,#132007,#132008,#132009),(#132010,
#132011,#132012,#132013,#132014)),.UNSPECIFIED.,.F.,.F.,.F.)
B_SPLINE_SURFACE_WITH_KNOTS((2,2),(3,2,3),(0.,0.290279631749781),(0.176864064841898,
0.194132688793569,0.19473123650816),.UNSPECIFIED.)
GEOMETRIC_REPRESENTATION_ITEM()
RATIONAL_B_SPLINE_SURFACE(((0.987492606357657,0.987202831733786,0.989843896581211,
0.989843896581211,0.989843896581211),(0.987492606357657,0.987202831733786,
0.989843896581211,0.989843896581211,0.989843896581211)))
REPRESENTATION_ITEM('')
SURFACE()
);
#2238=(
BOUNDED_SURFACE()
B_SPLINE_SURFACE(1,2,((#132023,#132024,#132025),(#132026,#132027,#132028),
(#132029,#132030,#132031)),.UNSPECIFIED.,.F.,.F.,.F.)
B_SPLINE_SURFACE_WITH_KNOTS((2,1,2),(3,3),(-0.0028980704099307,0.,0.28980704099307),
(0.53899963051341,0.556316102183953),.UNSPECIFIED.)
GEOMETRIC_REPRESENTATION_ITEM()
RATIONAL_B_SPLINE_SURFACE(((0.987570037304351,0.988129172627919,0.99163541140107),
(0.987570037304351,0.988129172627919,0.99163541140107),(0.987570037304351,
0.988129172627919,0.99163541140107)))
REPRESENTATION_ITEM('')
SURFACE()
);
#2239=(
BOUNDED_SURFACE()
B_SPLINE_SURFACE(1,2,((#132033,#132034,#132035,#132036,#132037),(#132038,
#132039,#132040,#132041,#132042)),.UNSPECIFIED.,.F.,.F.,.F.)
B_SPLINE_SURFACE_WITH_KNOTS((2,2),(3,2,3),(0.,0.29027963174592),(0.176864064841898,
0.194132688793569,0.194731236504307),.UNSPECIFIED.)
GEOMETRIC_REPRESENTATION_ITEM()
RATIONAL_B_SPLINE_SURFACE(((0.987492606357657,0.987202831733786,0.989843896581211,
0.989843896581211,0.989843896581211),(0.987492606357657,0.987202831733786,
0.989843896581211,0.989843896581211,0.989843896581211)))
REPRESENTATION_ITEM('')
SURFACE()
);
#2240=(
BOUNDED_SURFACE()
B_SPLINE_SURFACE(1,2,((#132051,#132052,#132053),(#132054,#132055,#132056),
(#132057,#132058,#132059)),.UNSPECIFIED.,.F.,.F.,.F.)
B_SPLINE_SURFACE_WITH_KNOTS((2,1,2),(3,3),(-0.00289807040992572,0.,0.289807040992572),
(0.538999630513411,0.556316102183953),.UNSPECIFIED.)
GEOMETRIC_REPRESENTATION_ITEM()
RATIONAL_B_SPLINE_SURFACE(((0.987570037304351,0.988129172627919,0.99163541140107),
(0.987570037304351,0.988129172627919,0.99163541140107),(0.987570037304351,
0.988129172627919,0.99163541140107)))
REPRESENTATION_ITEM('')
SURFACE()
);
#2241=(
BOUNDED_SURFACE()
B_SPLINE_SURFACE(1,2,((#132061,#132062,#132063,#132064,#132065),(#132066,
#132067,#132068,#132069,#132070)),.UNSPECIFIED.,.F.,.F.,.F.)
B_SPLINE_SURFACE_WITH_KNOTS((2,2),(3,2,3),(0.,0.290279631772035),(0.176864064841897,
0.194132688793568,0.194731236530414),.UNSPECIFIED.)
GEOMETRIC_REPRESENTATION_ITEM()
RATIONAL_B_SPLINE_SURFACE(((0.987492606357657,0.987202831733786,0.989843896581211,
0.989843896581211,0.989843896581211),(0.987492606357657,0.987202831733786,
0.989843896581211,0.989843896581211,0.989843896581211)))
REPRESENTATION_ITEM('')
SURFACE()
);
#2242=(
BOUNDED_SURFACE()
B_SPLINE_SURFACE(1,2,((#132079,#132080,#132081),(#132082,#132083,#132084),
(#132085,#132086,#132087)),.UNSPECIFIED.,.F.,.F.,.F.)
B_SPLINE_SURFACE_WITH_KNOTS((2,1,2),(3,3),(-0.00289807040992567,0.,0.289807040992567),
(0.538999630513411,0.556316102183955),.UNSPECIFIED.)
GEOMETRIC_REPRESENTATION_ITEM()
RATIONAL_B_SPLINE_SURFACE(((0.987570037304351,0.988129172627919,0.99163541140107),
(0.987570037304351,0.988129172627919,0.99163541140107),(0.987570037304351,
0.988129172627919,0.99163541140107)))
REPRESENTATION_ITEM('')
SURFACE()
);
#2243=(
BOUNDED_SURFACE()
B_SPLINE_SURFACE(1,2,((#132089,#132090,#132091,#132092,#132093),(#132094,
#132095,#132096,#132097,#132098)),.UNSPECIFIED.,.F.,.F.,.F.)
B_SPLINE_SURFACE_WITH_KNOTS((2,2),(3,2,3),(0.,0.290279631748006),(0.176864064841897,
0.194132688793568,0.194731236506389),.UNSPECIFIED.)
GEOMETRIC_REPRESENTATION_ITEM()
RATIONAL_B_SPLINE_SURFACE(((0.987492606357657,0.987202831733786,0.989843896581211,
0.989843896581211,0.989843896581211),(0.987492606357657,0.987202831733786,
0.989843896581211,0.989843896581211,0.989843896581211)))
REPRESENTATION_ITEM('')
SURFACE()
);
#2244=(
BOUNDED_SURFACE()
B_SPLINE_SURFACE(1,2,((#132107,#132108,#132109),(#132110,#132111,#132112),
(#132113,#132114,#132115)),.UNSPECIFIED.,.F.,.F.,.F.)
B_SPLINE_SURFACE_WITH_KNOTS((2,1,2),(3,3),(-0.00289807040993166,0.,0.289807040993166),
(0.538999630513411,0.556316102183954),.UNSPECIFIED.)
GEOMETRIC_REPRESENTATION_ITEM()
RATIONAL_B_SPLINE_SURFACE(((0.987570037304351,0.988129172627919,0.99163541140107),
(0.987570037304351,0.988129172627919,0.99163541140107),(0.987570037304351,
0.988129172627919,0.99163541140107)))
REPRESENTATION_ITEM('')
SURFACE()
);
#2245=(
BOUNDED_SURFACE()
B_SPLINE_SURFACE(1,2,((#132117,#132118,#132119,#132120,#132121),(#132122,
#132123,#132124,#132125,#132126)),.UNSPECIFIED.,.F.,.F.,.F.)
B_SPLINE_SURFACE_WITH_KNOTS((2,2),(3,2,3),(0.,0.290279631752551),(0.176864064841897,
0.194132688793568,0.194731236510931),.UNSPECIFIED.)
GEOMETRIC_REPRESENTATION_ITEM()
RATIONAL_B_SPLINE_SURFACE(((0.987492606357657,0.987202831733785,0.98984389658121,
0.98984389658121,0.98984389658121),(0.987492606357657,0.987202831733785,
0.98984389658121,0.98984389658121,0.98984389658121)))
REPRESENTATION_ITEM('')
SURFACE()
);
#2246=(
BOUNDED_SURFACE()
B_SPLINE_SURFACE(1,2,((#132135,#132136,#132137),(#132138,#132139,#132140),
(#132141,#132142,#132143)),.UNSPECIFIED.,.F.,.F.,.F.)
B_SPLINE_SURFACE_WITH_KNOTS((2,1,2),(3,3),(-0.00289807040992572,0.,0.289807040992572),
(0.538999630513411,0.556316102183955),.UNSPECIFIED.)
GEOMETRIC_REPRESENTATION_ITEM()
RATIONAL_B_SPLINE_SURFACE(((0.987570037304351,0.988129172627919,0.99163541140107),
(0.987570037304351,0.988129172627919,0.99163541140107),(0.987570037304351,
0.988129172627919,0.99163541140107)))
REPRESENTATION_ITEM('')
SURFACE()
);
#2247=(
BOUNDED_SURFACE()
B_SPLINE_SURFACE(1,2,((#132145,#132146,#132147,#132148,#132149),(#132150,
#132151,#132152,#132153,#132154)),.UNSPECIFIED.,.F.,.F.,.F.)
B_SPLINE_SURFACE_WITH_KNOTS((2,2),(3,2,3),(0.,0.290279631773371),(0.176864064841897,
0.194132688793568,0.194731236531752),.UNSPECIFIED.)
GEOMETRIC_REPRESENTATION_ITEM()
RATIONAL_B_SPLINE_SURFACE(((0.987492606357657,0.987202831733786,0.989843896581211,
0.989843896581211,0.989843896581211),(0.987492606357657,0.987202831733786,
0.989843896581211,0.989843896581211,0.989843896581211)))
REPRESENTATION_ITEM('')
SURFACE()
);
#2248=(
BOUNDED_SURFACE()
B_SPLINE_SURFACE(1,2,((#132163,#132164,#132165),(#132166,#132167,#132168),
(#132169,#132170,#132171)),.UNSPECIFIED.,.F.,.F.,.F.)
B_SPLINE_SURFACE_WITH_KNOTS((2,1,2),(3,3),(-0.00289807040993075,0.,0.289807040993075),
(0.538999630513411,0.556316102183955),.UNSPECIFIED.)
GEOMETRIC_REPRESENTATION_ITEM()
RATIONAL_B_SPLINE_SURFACE(((0.987570037304351,0.988129172627919,0.99163541140107),
(0.987570037304351,0.988129172627919,0.99163541140107),(0.987570037304351,
0.988129172627919,0.99163541140107)))
REPRESENTATION_ITEM('')
SURFACE()
);
#2249=(
BOUNDED_SURFACE()
B_SPLINE_SURFACE(1,2,((#132173,#132174,#132175,#132176,#132177),(#132178,
#132179,#132180,#132181,#132182)),.UNSPECIFIED.,.F.,.F.,.F.)
B_SPLINE_SURFACE_WITH_KNOTS((2,2),(3,2,3),(0.,0.2902796317778),(0.176864064841897,
0.194132688793568,0.194731236536179),.UNSPECIFIED.)
GEOMETRIC_REPRESENTATION_ITEM()
RATIONAL_B_SPLINE_SURFACE(((0.987492606357657,0.987202831733786,0.989843896581211,
0.989843896581211,0.989843896581211),(0.987492606357657,0.987202831733786,
0.989843896581211,0.989843896581211,0.989843896581211)))
REPRESENTATION_ITEM('')
SURFACE()
);
#2250=(
BOUNDED_SURFACE()
B_SPLINE_SURFACE(1,2,((#132191,#132192,#132193),(#132194,#132195,#132196),
(#132197,#132198,#132199)),.UNSPECIFIED.,.F.,.F.,.F.)
B_SPLINE_SURFACE_WITH_KNOTS((2,1,2),(3,3),(-0.00289807040992579,0.,0.289807040992579),
(0.538999630513411,0.556316102183955),.UNSPECIFIED.)
GEOMETRIC_REPRESENTATION_ITEM()
RATIONAL_B_SPLINE_SURFACE(((0.987570037304351,0.988129172627919,0.99163541140107),
(0.987570037304351,0.988129172627919,0.99163541140107),(0.987570037304351,
0.988129172627919,0.99163541140107)))
REPRESENTATION_ITEM('')
SURFACE()
);
#2251=(
BOUNDED_SURFACE()
B_SPLINE_SURFACE(1,2,((#132201,#132202,#132203,#132204,#132205),(#132206,
#132207,#132208,#132209,#132210)),.UNSPECIFIED.,.F.,.F.,.F.)
B_SPLINE_SURFACE_WITH_KNOTS((2,2),(3,2,3),(0.,0.290279631762204),(0.176864064841897,
0.194132688793568,0.194731236520584),.UNSPECIFIED.)
GEOMETRIC_REPRESENTATION_ITEM()
RATIONAL_B_SPLINE_SURFACE(((0.987492606357657,0.987202831733786,0.989843896581211,
0.989843896581211,0.989843896581211),(0.987492606357657,0.987202831733786,
0.989843896581211,0.989843896581211,0.989843896581211)))
REPRESENTATION_ITEM('')
SURFACE()
);
#2252=(
BOUNDED_SURFACE()
B_SPLINE_SURFACE(1,2,((#132219,#132220,#132221),(#132222,#132223,#132224),
(#132225,#132226,#132227)),.UNSPECIFIED.,.F.,.F.,.F.)
B_SPLINE_SURFACE_WITH_KNOTS((2,1,2),(3,3),(-0.00289807040993075,0.,0.289807040993075),
(0.538999630513411,0.556316102183955),.UNSPECIFIED.)
GEOMETRIC_REPRESENTATION_ITEM()
RATIONAL_B_SPLINE_SURFACE(((0.987570037304351,0.988129172627919,0.99163541140107),
(0.987570037304351,0.988129172627919,0.99163541140107),(0.987570037304351,
0.988129172627919,0.99163541140107)))
REPRESENTATION_ITEM('')
SURFACE()
);
#2253=(
BOUNDED_SURFACE()
B_SPLINE_SURFACE(1,2,((#132229,#132230,#132231,#132232,#132233),(#132234,
#132235,#132236,#132237,#132238)),.UNSPECIFIED.,.F.,.F.,.F.)
B_SPLINE_SURFACE_WITH_KNOTS((2,2),(3,2,3),(0.,0.290279631773358),(0.176864064841897,
0.194132688793568,0.194731236531739),.UNSPECIFIED.)
GEOMETRIC_REPRESENTATION_ITEM()
RATIONAL_B_SPLINE_SURFACE(((0.987492606357657,0.987202831733786,0.989843896581211,
0.989843896581211,0.989843896581211),(0.987492606357657,0.987202831733786,
0.989843896581211,0.989843896581211,0.989843896581211)))
REPRESENTATION_ITEM('')
SURFACE()
);
#2254=(
BOUNDED_SURFACE()
B_SPLINE_SURFACE(1,2,((#132247,#132248,#132249),(#132250,#132251,#132252),
(#132253,#132254,#132255)),.UNSPECIFIED.,.F.,.F.,.F.)
B_SPLINE_SURFACE_WITH_KNOTS((2,1,2),(3,3),(-0.00289807040992848,0.,0.289807040992848),
(0.538999630513411,0.556316102183955),.UNSPECIFIED.)
GEOMETRIC_REPRESENTATION_ITEM()
RATIONAL_B_SPLINE_SURFACE(((0.987570037304351,0.988129172627919,0.99163541140107),
(0.987570037304351,0.988129172627919,0.99163541140107),(0.987570037304351,
0.988129172627919,0.99163541140107)))
REPRESENTATION_ITEM('')
SURFACE()
);
#2255=(
BOUNDED_SURFACE()
B_SPLINE_SURFACE(1,2,((#132257,#132258,#132259,#132260,#132261),(#132262,
#132263,#132264,#132265,#132266)),.UNSPECIFIED.,.F.,.F.,.F.)
B_SPLINE_SURFACE_WITH_KNOTS((2,2),(3,2,3),(0.,0.290279631764032),(0.176864064841897,
0.194132688793568,0.194731236522411),.UNSPECIFIED.)
GEOMETRIC_REPRESENTATION_ITEM()
RATIONAL_B_SPLINE_SURFACE(((0.987492606357657,0.987202831733786,0.989843896581211,
0.989843896581211,0.989843896581211),(0.987492606357657,0.987202831733786,
0.989843896581211,0.989843896581211,0.989843896581211)))
REPRESENTATION_ITEM('')
SURFACE()
);
#2256=(
BOUNDED_SURFACE()
B_SPLINE_SURFACE(1,2,((#132275,#132276,#132277),(#132278,#132279,#132280),
(#132281,#132282,#132283)),.UNSPECIFIED.,.F.,.F.,.F.)
B_SPLINE_SURFACE_WITH_KNOTS((2,1,2),(3,3),(-0.00289807040993903,0.,0.289807040993903),
(0.538999630513411,0.556316102183955),.UNSPECIFIED.)
GEOMETRIC_REPRESENTATION_ITEM()
RATIONAL_B_SPLINE_SURFACE(((0.987570037304351,0.988129172627919,0.99163541140107),
(0.987570037304351,0.988129172627919,0.99163541140107),(0.987570037304351,
0.988129172627919,0.99163541140107)))
REPRESENTATION_ITEM('')
SURFACE()
);
#2257=(
BOUNDED_SURFACE()
B_SPLINE_SURFACE(1,2,((#132285,#132286,#132287,#132288,#132289),(#132290,
#132291,#132292,#132293,#132294)),.UNSPECIFIED.,.F.,.F.,.F.)
B_SPLINE_SURFACE_WITH_KNOTS((2,2),(3,2,3),(0.,0.290279631752155),(0.176864064841897,
0.194132688793568,0.194731236510534),.UNSPECIFIED.)
GEOMETRIC_REPRESENTATION_ITEM()
RATIONAL_B_SPLINE_SURFACE(((0.987492606357657,0.987202831733786,0.98984389658121,
0.98984389658121,0.98984389658121),(0.987492606357657,0.987202831733786,
0.989843896581211,0.989843896581211,0.989843896581211)))
REPRESENTATION_ITEM('')
SURFACE()
);
#2258=(
BOUNDED_SURFACE()
B_SPLINE_SURFACE(1,2,((#132303,#132304,#132305),(#132306,#132307,#132308),
(#132309,#132310,#132311)),.UNSPECIFIED.,.F.,.F.,.F.)
B_SPLINE_SURFACE_WITH_KNOTS((2,1,2),(3,3),(-0.00289807040992612,0.,0.289807040992612),
(0.538999630513411,0.556316102183954),.UNSPECIFIED.)
GEOMETRIC_REPRESENTATION_ITEM()
RATIONAL_B_SPLINE_SURFACE(((0.987570037304351,0.988129172627919,0.99163541140107),
(0.987570037304351,0.988129172627919,0.99163541140107),(0.987570037304351,
0.988129172627919,0.99163541140107)))
REPRESENTATION_ITEM('')
SURFACE()
);
#2259=(
BOUNDED_SURFACE()
B_SPLINE_SURFACE(1,2,((#132313,#132314,#132315,#132316,#132317),(#132318,
#132319,#132320,#132321,#132322)),.UNSPECIFIED.,.F.,.F.,.F.)
B_SPLINE_SURFACE_WITH_KNOTS((2,2),(3,2,3),(0.,0.290279631748086),(0.176864064841897,
0.194132688793568,0.194731236506461),.UNSPECIFIED.)
GEOMETRIC_REPRESENTATION_ITEM()
RATIONAL_B_SPLINE_SURFACE(((0.987492606357657,0.987202831733786,0.98984389658121,
0.98984389658121,0.98984389658121),(0.987492606357657,0.987202831733786,
0.989843896581211,0.989843896581211,0.989843896581211)))
REPRESENTATION_ITEM('')
SURFACE()
);
#2260=(
BOUNDED_SURFACE()
B_SPLINE_SURFACE(1,2,((#132331,#132332,#132333),(#132334,#132335,#132336),
(#132337,#132338,#132339)),.UNSPECIFIED.,.F.,.F.,.F.)
B_SPLINE_SURFACE_WITH_KNOTS((2,1,2),(3,3),(-0.00289807040992496,0.,0.289807040992496),
(0.538999630513411,0.556316102183955),.UNSPECIFIED.)
GEOMETRIC_REPRESENTATION_ITEM()
RATIONAL_B_SPLINE_SURFACE(((0.987570037304351,0.988129172627919,0.99163541140107),
(0.987570037304351,0.988129172627919,0.99163541140107),(0.987570037304351,
0.988129172627919,0.99163541140107)))
REPRESENTATION_ITEM('')
SURFACE()
);
#2261=(
BOUNDED_SURFACE()
B_SPLINE_SURFACE(1,2,((#132341,#132342,#132343,#132344,#132345),(#132346,
#132347,#132348,#132349,#132350)),.UNSPECIFIED.,.F.,.F.,.F.)
B_SPLINE_SURFACE_WITH_KNOTS((2,2),(3,2,3),(0.,0.290279631782441),(0.176864064841897,
0.194132688793568,0.194731236540818),.UNSPECIFIED.)
GEOMETRIC_REPRESENTATION_ITEM()
RATIONAL_B_SPLINE_SURFACE(((0.987492606357657,0.987202831733786,0.989843896581211,
0.989843896581211,0.989843896581211),(0.987492606357657,0.987202831733786,
0.989843896581211,0.989843896581211,0.989843896581211)))
REPRESENTATION_ITEM('')
SURFACE()
);
#2262=(
BOUNDED_SURFACE()
B_SPLINE_SURFACE(1,2,((#132359,#132360,#132361),(#132362,#132363,#132364),
(#132365,#132366,#132367)),.UNSPECIFIED.,.F.,.F.,.F.)
B_SPLINE_SURFACE_WITH_KNOTS((2,1,2),(3,3),(-0.00289807040993131,0.,0.289807040993131),
(0.538999630513411,0.556316102183955),.UNSPECIFIED.)
GEOMETRIC_REPRESENTATION_ITEM()
RATIONAL_B_SPLINE_SURFACE(((0.987570037304351,0.988129172627919,0.99163541140107),
(0.987570037304351,0.988129172627919,0.99163541140107),(0.987570037304351,
0.988129172627919,0.99163541140107)))
REPRESENTATION_ITEM('')
SURFACE()
);
#2263=(
BOUNDED_SURFACE()
B_SPLINE_SURFACE(1,2,((#132369,#132370,#132371,#132372,#132373),(#132374,
#132375,#132376,#132377,#132378)),.UNSPECIFIED.,.F.,.F.,.F.)
B_SPLINE_SURFACE_WITH_KNOTS((2,2),(3,2,3),(0.,0.290279631760911),(0.176864064841897,
0.194132688793568,0.194731236519285),.UNSPECIFIED.)
GEOMETRIC_REPRESENTATION_ITEM()
RATIONAL_B_SPLINE_SURFACE(((0.987492606357657,0.987202831733786,0.989843896581211,
0.989843896581211,0.989843896581211),(0.987492606357657,0.987202831733786,
0.989843896581211,0.989843896581211,0.989843896581211)))
REPRESENTATION_ITEM('')
SURFACE()
);
#2264=(
BOUNDED_SURFACE()
B_SPLINE_SURFACE(1,2,((#132387,#132388,#132389),(#132390,#132391,#132392),
(#132393,#132394,#132395)),.UNSPECIFIED.,.F.,.F.,.F.)
B_SPLINE_SURFACE_WITH_KNOTS((2,1,2),(3,3),(-0.00289807040991731,0.,0.289807040991731),
(0.538999630513411,0.556316102183955),.UNSPECIFIED.)
GEOMETRIC_REPRESENTATION_ITEM()
RATIONAL_B_SPLINE_SURFACE(((0.987570037304351,0.988129172627919,0.99163541140107),
(0.987570037304351,0.988129172627919,0.99163541140107),(0.987570037304351,
0.988129172627919,0.99163541140107)))
REPRESENTATION_ITEM('')
SURFACE()
);
#2265=(
BOUNDED_SURFACE()
B_SPLINE_SURFACE(1,2,((#132397,#132398,#132399,#132400,#132401),(#132402,
#132403,#132404,#132405,#132406)),.UNSPECIFIED.,.F.,.F.,.F.)
B_SPLINE_SURFACE_WITH_KNOTS((2,2),(3,2,3),(0.,0.290279631775496),(0.176864064841897,
0.194132688793569,0.194731236533875),.UNSPECIFIED.)
GEOMETRIC_REPRESENTATION_ITEM()
RATIONAL_B_SPLINE_SURFACE(((0.987492606357657,0.987202831733786,0.989843896581211,
0.989843896581211,0.989843896581211),(0.987492606357657,0.987202831733786,
0.989843896581211,0.989843896581211,0.989843896581211)))
REPRESENTATION_ITEM('')
SURFACE()
);
#2266=(
BOUNDED_SURFACE()
B_SPLINE_SURFACE(1,2,((#132415,#132416,#132417),(#132418,#132419,#132420),
(#132421,#132422,#132423)),.UNSPECIFIED.,.F.,.F.,.F.)
B_SPLINE_SURFACE_WITH_KNOTS((2,1,2),(3,3),(-0.00289807040992881,0.,0.289807040992881),
(0.538999630513411,0.556316102183955),.UNSPECIFIED.)
GEOMETRIC_REPRESENTATION_ITEM()
RATIONAL_B_SPLINE_SURFACE(((0.987570037304351,0.988129172627919,0.99163541140107),
(0.987570037304351,0.988129172627919,0.99163541140107),(0.987570037304351,
0.988129172627919,0.99163541140107)))
REPRESENTATION_ITEM('')
SURFACE()
);
#2267=(
BOUNDED_SURFACE()
B_SPLINE_SURFACE(1,2,((#132425,#132426,#132427,#132428,#132429),(#132430,
#132431,#132432,#132433,#132434)),.UNSPECIFIED.,.F.,.F.,.F.)
B_SPLINE_SURFACE_WITH_KNOTS((2,2),(3,2,3),(0.,0.290279631758543),(0.176864064841897,
0.194132688793568,0.194731236516916),.UNSPECIFIED.)
GEOMETRIC_REPRESENTATION_ITEM()
RATIONAL_B_SPLINE_SURFACE(((0.987492606357657,0.987202831733786,0.989843896581211,
0.989843896581211,0.989843896581211),(0.987492606357657,0.987202831733786,
0.989843896581211,0.989843896581211,0.989843896581211)))
REPRESENTATION_ITEM('')
SURFACE()
);
#2268=(
BOUNDED_SURFACE()
B_SPLINE_SURFACE(1,2,((#132443,#132444,#132445),(#132446,#132447,#132448),
(#132449,#132450,#132451)),.UNSPECIFIED.,.F.,.F.,.F.)
B_SPLINE_SURFACE_WITH_KNOTS((2,1,2),(3,3),(-0.00289807040992695,0.,0.289807040992695),
(0.538999630513411,0.556316102183954),.UNSPECIFIED.)
GEOMETRIC_REPRESENTATION_ITEM()
RATIONAL_B_SPLINE_SURFACE(((0.987570037304351,0.988129172627919,0.99163541140107),
(0.987570037304351,0.988129172627919,0.99163541140107),(0.987570037304351,
0.988129172627919,0.99163541140107)))
REPRESENTATION_ITEM('')
SURFACE()
);
#2269=(
BOUNDED_SURFACE()
B_SPLINE_SURFACE(1,2,((#132453,#132454,#132455,#132456,#132457),(#132458,
#132459,#132460,#132461,#132462)),.UNSPECIFIED.,.F.,.F.,.F.)
B_SPLINE_SURFACE_WITH_KNOTS((2,2),(3,2,3),(0.,0.290279631770573),(0.176864064841897,
0.194132688793568,0.194731236528949),.UNSPECIFIED.)
GEOMETRIC_REPRESENTATION_ITEM()
RATIONAL_B_SPLINE_SURFACE(((0.987492606357657,0.987202831733786,0.989843896581211,
0.989843896581211,0.989843896581211),(0.987492606357657,0.987202831733786,
0.989843896581211,0.989843896581211,0.989843896581211)))
REPRESENTATION_ITEM('')
SURFACE()
);
#2270=(
BOUNDED_SURFACE()
B_SPLINE_SURFACE(1,2,((#132471,#132472,#132473),(#132474,#132475,#132476),
(#132477,#132478,#132479)),.UNSPECIFIED.,.F.,.F.,.F.)
B_SPLINE_SURFACE_WITH_KNOTS((2,1,2),(3,3),(-0.00289807040993738,0.,0.289807040993738),
(0.538999630513411,0.556316102183954),.UNSPECIFIED.)
GEOMETRIC_REPRESENTATION_ITEM()
RATIONAL_B_SPLINE_SURFACE(((0.987570037304351,0.988129172627919,0.99163541140107),
(0.987570037304351,0.988129172627919,0.99163541140107),(0.987570037304351,
0.988129172627919,0.99163541140107)))
REPRESENTATION_ITEM('')
SURFACE()
);
#2271=(
BOUNDED_SURFACE()
B_SPLINE_SURFACE(1,2,((#132481,#132482,#132483,#132484,#132485),(#132486,
#132487,#132488,#132489,#132490)),.UNSPECIFIED.,.F.,.F.,.F.)
B_SPLINE_SURFACE_WITH_KNOTS((2,2),(3,2,3),(0.,0.290279631757276),(0.176864064841897,
0.194132688793568,0.194731236515657),.UNSPECIFIED.)
GEOMETRIC_REPRESENTATION_ITEM()
RATIONAL_B_SPLINE_SURFACE(((0.987492606357657,0.987202831733786,0.98984389658121,
0.98984389658121,0.98984389658121),(0.987492606357657,0.987202831733786,
0.98984389658121,0.98984389658121,0.98984389658121)))
REPRESENTATION_ITEM('')
SURFACE()
);
#2272=(
BOUNDED_SURFACE()
B_SPLINE_SURFACE(1,2,((#132499,#132500,#132501),(#132502,#132503,#132504),
(#132505,#132506,#132507)),.UNSPECIFIED.,.F.,.F.,.F.)
B_SPLINE_SURFACE_WITH_KNOTS((2,1,2),(3,3),(-0.00289807040991906,0.,0.289807040991906),
(0.538999630513411,0.556316102183956),.UNSPECIFIED.)
GEOMETRIC_REPRESENTATION_ITEM()
RATIONAL_B_SPLINE_SURFACE(((0.987570037304351,0.988129172627919,0.99163541140107),
(0.987570037304351,0.988129172627919,0.99163541140107),(0.987570037304351,
0.988129172627919,0.99163541140107)))
REPRESENTATION_ITEM('')
SURFACE()
);
#2273=(
BOUNDED_SURFACE()
B_SPLINE_SURFACE(1,2,((#132509,#132510,#132511,#132512,#132513),(#132514,
#132515,#132516,#132517,#132518)),.UNSPECIFIED.,.F.,.F.,.F.)
B_SPLINE_SURFACE_WITH_KNOTS((2,2),(3,2,3),(0.,0.290279631753777),(0.176864064841897,
0.194132688793568,0.194731236512156),.UNSPECIFIED.)
GEOMETRIC_REPRESENTATION_ITEM()
RATIONAL_B_SPLINE_SURFACE(((0.987492606357657,0.987202831733786,0.989843896581211,
0.989843896581211,0.989843896581211),(0.987492606357657,0.987202831733786,
0.989843896581211,0.989843896581211,0.989843896581211)))
REPRESENTATION_ITEM('')
SURFACE()
);
#2274=(
BOUNDED_SURFACE()
B_SPLINE_SURFACE(1,2,((#132527,#132528,#132529),(#132530,#132531,#132532),
(#132533,#132534,#132535)),.UNSPECIFIED.,.F.,.F.,.F.)
B_SPLINE_SURFACE_WITH_KNOTS((2,1,2),(3,3),(-0.00289807040993058,0.,0.289807040993058),
(0.538999630513411,0.556316102183954),.UNSPECIFIED.)
GEOMETRIC_REPRESENTATION_ITEM()
RATIONAL_B_SPLINE_SURFACE(((0.987570037304351,0.988129172627919,0.99163541140107),
(0.987570037304351,0.988129172627919,0.99163541140107),(0.987570037304351,
0.988129172627919,0.99163541140107)))
REPRESENTATION_ITEM('')
SURFACE()
);
#2275=(
BOUNDED_SURFACE()
B_SPLINE_SURFACE(1,2,((#132537,#132538,#132539,#132540,#132541),(#132542,
#132543,#132544,#132545,#132546)),.UNSPECIFIED.,.F.,.F.,.F.)
B_SPLINE_SURFACE_WITH_KNOTS((2,2),(3,2,3),(0.,0.290279631751751),(0.176864064841897,
0.194132688793568,0.194731236510121),.UNSPECIFIED.)
GEOMETRIC_REPRESENTATION_ITEM()
RATIONAL_B_SPLINE_SURFACE(((0.987492606357657,0.987202831733785,0.98984389658121,
0.98984389658121,0.98984389658121),(0.987492606357657,0.987202831733785,
0.98984389658121,0.98984389658121,0.98984389658121)))
REPRESENTATION_ITEM('')
SURFACE()
);
#2276=(
BOUNDED_SURFACE()
B_SPLINE_SURFACE(1,2,((#132555,#132556,#132557),(#132558,#132559,#132560),
(#132561,#132562,#132563)),.UNSPECIFIED.,.F.,.F.,.F.)
B_SPLINE_SURFACE_WITH_KNOTS((2,1,2),(3,3),(-0.00289807040992803,0.,0.289807040992803),
(0.538999630513411,0.556316102183955),.UNSPECIFIED.)
GEOMETRIC_REPRESENTATION_ITEM()
RATIONAL_B_SPLINE_SURFACE(((0.987570037304351,0.988129172627919,0.99163541140107),
(0.987570037304351,0.988129172627919,0.99163541140107),(0.987570037304351,
0.988129172627919,0.99163541140107)))
REPRESENTATION_ITEM('')
SURFACE()
);
#2277=(
BOUNDED_SURFACE()
B_SPLINE_SURFACE(1,2,((#132565,#132566,#132567,#132568,#132569),(#132570,
#132571,#132572,#132573,#132574)),.UNSPECIFIED.,.F.,.F.,.F.)
B_SPLINE_SURFACE_WITH_KNOTS((2,2),(3,2,3),(0.,0.290279631762918),(0.176864064841898,
0.194132688793568,0.194731236521282),.UNSPECIFIED.)
GEOMETRIC_REPRESENTATION_ITEM()
RATIONAL_B_SPLINE_SURFACE(((0.987492606357657,0.987202831733786,0.98984389658121,
0.98984389658121,0.98984389658121),(0.987492606357657,0.987202831733786,
0.98984389658121,0.98984389658121,0.98984389658121)))
REPRESENTATION_ITEM('')
SURFACE()
);
#2278=(
BOUNDED_SURFACE()
B_SPLINE_SURFACE(1,2,((#132583,#132584,#132585),(#132586,#132587,#132588),
(#132589,#132590,#132591)),.UNSPECIFIED.,.F.,.F.,.F.)
B_SPLINE_SURFACE_WITH_KNOTS((2,1,2),(3,3),(-0.0028980704099156,0.,0.28980704099156),
(0.53899963051341,0.556316102183953),.UNSPECIFIED.)
GEOMETRIC_REPRESENTATION_ITEM()
RATIONAL_B_SPLINE_SURFACE(((0.987570037304351,0.988129172627919,0.99163541140107),
(0.987570037304351,0.988129172627919,0.99163541140107),(0.987570037304351,
0.988129172627919,0.99163541140107)))
REPRESENTATION_ITEM('')
SURFACE()
);
#2279=(
BOUNDED_SURFACE()
B_SPLINE_SURFACE(1,2,((#132593,#132594,#132595,#132596,#132597),(#132598,
#132599,#132600,#132601,#132602)),.UNSPECIFIED.,.F.,.F.,.F.)
B_SPLINE_SURFACE_WITH_KNOTS((2,2),(3,2,3),(0.,0.290279631766922),(0.176864064841898,
0.194132688793569,0.194731236525302),.UNSPECIFIED.)
GEOMETRIC_REPRESENTATION_ITEM()
RATIONAL_B_SPLINE_SURFACE(((0.987492606357657,0.987202831733786,0.989843896581211,
0.989843896581211,0.989843896581211),(0.987492606357657,0.987202831733786,
0.989843896581211,0.989843896581211,0.989843896581211)))
REPRESENTATION_ITEM('')
SURFACE()
);
#2280=(
BOUNDED_SURFACE()
B_SPLINE_SURFACE(1,2,((#132611,#132612,#132613),(#132614,#132615,#132616),
(#132617,#132618,#132619)),.UNSPECIFIED.,.F.,.F.,.F.)
B_SPLINE_SURFACE_WITH_KNOTS((2,1,2),(3,3),(-0.00289807040991558,0.,0.289807040991558),
(0.53899963051341,0.556316102183954),.UNSPECIFIED.)
GEOMETRIC_REPRESENTATION_ITEM()
RATIONAL_B_SPLINE_SURFACE(((0.987570037304351,0.988129172627919,0.99163541140107),
(0.987570037304351,0.988129172627919,0.99163541140107),(0.987570037304351,
0.988129172627919,0.99163541140107)))
REPRESENTATION_ITEM('')
SURFACE()
);
#2281=(
BOUNDED_SURFACE()
B_SPLINE_SURFACE(1,2,((#132621,#132622,#132623,#132624,#132625),(#132626,
#132627,#132628,#132629,#132630),(#132631,#132632,#132633,#132634,#132635)),
 .UNSPECIFIED.,.F.,.F.,.F.)
B_SPLINE_SURFACE_WITH_KNOTS((2,1,2),(3,2,3),(-0.00289681084359915,0.,0.290279631760325),
(0.176864064841898,0.194132688793569,0.194731236518711),.UNSPECIFIED.)
GEOMETRIC_REPRESENTATION_ITEM()
RATIONAL_B_SPLINE_SURFACE(((0.987492606357657,0.987202831733786,0.989843896581211,
0.989843896581211,0.989843896581211),(0.987492606357657,0.987202831733786,
0.989843896581211,0.989843896581211,0.989843896581211),(0.987492606357657,
0.987202831733786,0.989843896581211,0.989843896581211,0.989843896581211)))
REPRESENTATION_ITEM('')
SURFACE()
);
#2282=(
BOUNDED_SURFACE()
B_SPLINE_SURFACE(1,2,((#132637,#132638,#132639),(#132640,#132641,#132642)),
 .UNSPECIFIED.,.F.,.F.,.F.)
B_SPLINE_SURFACE_WITH_KNOTS((2,2),(3,3),(0.,0.289807040991619),(0.22888337489439,
0.246056477139967),.UNSPECIFIED.)
GEOMETRIC_REPRESENTATION_ITEM()
RATIONAL_B_SPLINE_SURFACE(((0.991846493044863,0.988282393439513,0.987616798999169),
(0.991846493044863,0.988282393439513,0.987616798999169)))
REPRESENTATION_ITEM('')
SURFACE()
);
#2283=(
BOUNDED_SURFACE()
B_SPLINE_SURFACE(1,2,((#132665,#132666,#132667,#132668,#132669),(#132670,
#132671,#132672,#132673,#132674)),.UNSPECIFIED.,.F.,.F.,.F.)
B_SPLINE_SURFACE_WITH_KNOTS((2,2),(3,2,3),(0.,0.289681084359922),(0.487155140750431,
0.5,0.504719756176227),.UNSPECIFIED.)
GEOMETRIC_REPRESENTATION_ITEM()
RATIONAL_B_SPLINE_SURFACE(((0.992604240083356,0.995491335852357,1.,0.998343322021369,
0.996905579294145),(0.992604240083356,0.995491335852357,1.,0.998343322021369,
0.996905579294145)))
REPRESENTATION_ITEM('')
SURFACE()
);
#2284=(
BOUNDED_SURFACE()
B_SPLINE_SURFACE(1,2,((#132676,#132677,#132678),(#132679,#132680,#132681)),
 .UNSPECIFIED.,.F.,.F.,.F.)
B_SPLINE_SURFACE_WITH_KNOTS((2,2),(3,3),(0.,0.289807040991568),(0.228883374894701,
0.246056477139965),.UNSPECIFIED.)
GEOMETRIC_REPRESENTATION_ITEM()
RATIONAL_B_SPLINE_SURFACE(((0.991846493044734,0.988282393439502,0.987616798999169),
(0.991846493044734,0.988282393439502,0.987616798999169)))
REPRESENTATION_ITEM('')
SURFACE()
);
#2285=(
BOUNDED_SURFACE()
B_SPLINE_SURFACE(1,2,((#132704,#132705,#132706,#132707,#132708),(#132709,
#132710,#132711,#132712,#132713)),.UNSPECIFIED.,.F.,.F.,.F.)
B_SPLINE_SURFACE_WITH_KNOTS((2,2),(3,2,3),(0.,0.289681084359935),(0.487155140750431,
0.5,0.504719756176228),.UNSPECIFIED.)
GEOMETRIC_REPRESENTATION_ITEM()
RATIONAL_B_SPLINE_SURFACE(((0.992604240083356,0.995491335852357,1.,0.998343322021369,
0.996905579294145),(0.992604240083356,0.995491335852357,1.,0.998343322021369,
0.996905579294145)))
REPRESENTATION_ITEM('')
SURFACE()
);
#2286=(
BOUNDED_SURFACE()
B_SPLINE_SURFACE(1,2,((#132715,#132716,#132717),(#132718,#132719,#132720)),
 .UNSPECIFIED.,.F.,.F.,.F.)
B_SPLINE_SURFACE_WITH_KNOTS((2,2),(3,3),(0.,0.289807040991561),(0.228883374894809,
0.246056477139964),.UNSPECIFIED.)
GEOMETRIC_REPRESENTATION_ITEM()
RATIONAL_B_SPLINE_SURFACE(((0.991846493044689,0.988282393439498,0.987616798999169),
(0.991846493044689,0.988282393439498,0.987616798999169)))
REPRESENTATION_ITEM('')
SURFACE()
);
#2287=(
BOUNDED_SURFACE()
B_SPLINE_SURFACE(1,2,((#132743,#132744,#132745,#132746,#132747),(#132748,
#132749,#132750,#132751,#132752)),.UNSPECIFIED.,.F.,.F.,.F.)
B_SPLINE_SURFACE_WITH_KNOTS((2,2),(3,2,3),(0.,0.289681084360113),(0.48715514075043,
0.5,0.504719756176228),.UNSPECIFIED.)
GEOMETRIC_REPRESENTATION_ITEM()
RATIONAL_B_SPLINE_SURFACE(((0.992604240083356,0.995491335852357,1.,0.998343322021369,
0.996905579294145),(0.992604240083356,0.995491335852357,1.,0.998343322021369,
0.996905579294145)))
REPRESENTATION_ITEM('')
SURFACE()
);
#2288=(
BOUNDED_SURFACE()
B_SPLINE_SURFACE(1,2,((#132754,#132755,#132756),(#132757,#132758,#132759)),
 .UNSPECIFIED.,.F.,.F.,.F.)
B_SPLINE_SURFACE_WITH_KNOTS((2,2),(3,3),(0.,0.289807040991569),(0.228883374894809,
0.246056477139964),.UNSPECIFIED.)
GEOMETRIC_REPRESENTATION_ITEM()
RATIONAL_B_SPLINE_SURFACE(((0.991846493044689,0.988282393439498,0.987616798999169),
(0.991846493044689,0.988282393439498,0.987616798999169)))
REPRESENTATION_ITEM('')
SURFACE()
);
#2289=(
BOUNDED_SURFACE()
B_SPLINE_SURFACE(1,2,((#132782,#132783,#132784,#132785,#132786),(#132787,
#132788,#132789,#132790,#132791)),.UNSPECIFIED.,.F.,.F.,.F.)
B_SPLINE_SURFACE_WITH_KNOTS((2,2),(3,2,3),(0.,0.289681084359931),(0.48715514075043,
0.5,0.504719756176228),.UNSPECIFIED.)
GEOMETRIC_REPRESENTATION_ITEM()
RATIONAL_B_SPLINE_SURFACE(((0.992604240083356,0.995491335852357,1.,0.998343322021369,
0.996905579294145),(0.992604240083356,0.995491335852357,1.,0.998343322021369,
0.996905579294145)))
REPRESENTATION_ITEM('')
SURFACE()
);
#2290=(
BOUNDED_SURFACE()
B_SPLINE_SURFACE(1,2,((#132793,#132794,#132795),(#132796,#132797,#132798)),
 .UNSPECIFIED.,.F.,.F.,.F.)
B_SPLINE_SURFACE_WITH_KNOTS((2,2),(3,3),(0.,0.289807040991559),(0.228883374894304,
0.246056477139967),.UNSPECIFIED.)
GEOMETRIC_REPRESENTATION_ITEM()
RATIONAL_B_SPLINE_SURFACE(((0.991846493044899,0.988282393439517,0.987616798999169),
(0.991846493044899,0.988282393439516,0.987616798999169)))
REPRESENTATION_ITEM('')
SURFACE()
);
#2291=(
BOUNDED_SURFACE()
B_SPLINE_SURFACE(1,2,((#132821,#132822,#132823,#132824,#132825),(#132826,
#132827,#132828,#132829,#132830)),.UNSPECIFIED.,.F.,.F.,.F.)
B_SPLINE_SURFACE_WITH_KNOTS((2,2),(3,2,3),(0.,0.289681084360006),(0.487155140750431,
0.5,0.504719756176228),.UNSPECIFIED.)
GEOMETRIC_REPRESENTATION_ITEM()
RATIONAL_B_SPLINE_SURFACE(((0.992604240083356,0.995491335852357,1.,0.998343322021369,
0.996905579294145),(0.992604240083356,0.995491335852357,1.,0.998343322021369,
0.996905579294145)))
REPRESENTATION_ITEM('')
SURFACE()
);
#2292=(
BOUNDED_SURFACE()
B_SPLINE_SURFACE(1,2,((#132832,#132833,#132834),(#132835,#132836,#132837)),
 .UNSPECIFIED.,.F.,.F.,.F.)
B_SPLINE_SURFACE_WITH_KNOTS((2,2),(3,3),(0.,0.289807040991556),(0.228883374894453,
0.246056477139966),.UNSPECIFIED.)
GEOMETRIC_REPRESENTATION_ITEM()
RATIONAL_B_SPLINE_SURFACE(((0.991846493044837,0.988282393439511,0.987616798999169),
(0.991846493044837,0.988282393439511,0.987616798999169)))
REPRESENTATION_ITEM('')
SURFACE()
);
#2293=(
BOUNDED_SURFACE()
B_SPLINE_SURFACE(1,2,((#132860,#132861,#132862,#132863,#132864),(#132865,
#132866,#132867,#132868,#132869)),.UNSPECIFIED.,.F.,.F.,.F.)
B_SPLINE_SURFACE_WITH_KNOTS((2,2),(3,2,3),(0.,0.289681084359969),(0.48715514075043,
0.5,0.504719756176227),.UNSPECIFIED.)
GEOMETRIC_REPRESENTATION_ITEM()
RATIONAL_B_SPLINE_SURFACE(((0.992604240083356,0.995491335852357,1.,0.99834332202137,
0.996905579294146),(0.992604240083356,0.995491335852357,1.,0.99834332202137,
0.996905579294146)))
REPRESENTATION_ITEM('')
SURFACE()
);
#2294=(
BOUNDED_SURFACE()
B_SPLINE_SURFACE(1,2,((#132871,#132872,#132873),(#132874,#132875,#132876)),
 .UNSPECIFIED.,.F.,.F.,.F.)
B_SPLINE_SURFACE_WITH_KNOTS((2,2),(3,3),(0.,0.289807040991562),(0.228883374894634,
0.246056477139965),.UNSPECIFIED.)
GEOMETRIC_REPRESENTATION_ITEM()
RATIONAL_B_SPLINE_SURFACE(((0.991846493044762,0.988282393439504,0.987616798999169),
(0.991846493044762,0.988282393439504,0.987616798999169)))
REPRESENTATION_ITEM('')
SURFACE()
);
#2295=(
BOUNDED_SURFACE()
B_SPLINE_SURFACE(1,2,((#132899,#132900,#132901,#132902,#132903),(#132904,
#132905,#132906,#132907,#132908)),.UNSPECIFIED.,.F.,.F.,.F.)
B_SPLINE_SURFACE_WITH_KNOTS((2,2),(3,2,3),(0.,0.289681084360211),(0.487155140750431,
0.5,0.504719756176228),.UNSPECIFIED.)
GEOMETRIC_REPRESENTATION_ITEM()
RATIONAL_B_SPLINE_SURFACE(((0.992604240083356,0.995491335852357,1.,0.998343322021369,
0.996905579294145),(0.992604240083356,0.995491335852358,1.,0.998343322021369,
0.996905579294145)))
REPRESENTATION_ITEM('')
SURFACE()
);
#2296=(
BOUNDED_SURFACE()
B_SPLINE_SURFACE(1,2,((#132910,#132911,#132912),(#132913,#132914,#132915)),
 .UNSPECIFIED.,.F.,.F.,.F.)
B_SPLINE_SURFACE_WITH_KNOTS((2,2),(3,3),(0.,0.289807040991558),(0.228883374894809,
0.246056477139964),.UNSPECIFIED.)
GEOMETRIC_REPRESENTATION_ITEM()
RATIONAL_B_SPLINE_SURFACE(((0.991846493044689,0.988282393439498,0.987616798999169),
(0.991846493044689,0.988282393439498,0.987616798999169)))
REPRESENTATION_ITEM('')
SURFACE()
);
#2297=(
BOUNDED_SURFACE()
B_SPLINE_SURFACE(1,2,((#132938,#132939,#132940,#132941,#132942),(#132943,
#132944,#132945,#132946,#132947)),.UNSPECIFIED.,.F.,.F.,.F.)
B_SPLINE_SURFACE_WITH_KNOTS((2,2),(3,2,3),(0.,0.289681084360285),(0.487155140750431,
0.5,0.504719756176228),.UNSPECIFIED.)
GEOMETRIC_REPRESENTATION_ITEM()
RATIONAL_B_SPLINE_SURFACE(((0.992604240083356,0.995491335852358,1.,0.998343322021369,
0.996905579294145),(0.992604240083356,0.995491335852357,1.,0.998343322021369,
0.996905579294145)))
REPRESENTATION_ITEM('')
SURFACE()
);
#2298=(
BOUNDED_SURFACE()
B_SPLINE_SURFACE(1,2,((#132949,#132950,#132951),(#132952,#132953,#132954)),
 .UNSPECIFIED.,.F.,.F.,.F.)
B_SPLINE_SURFACE_WITH_KNOTS((2,2),(3,3),(0.,0.289807040991562),(0.228883374894809,
0.246056477139964),.UNSPECIFIED.)
GEOMETRIC_REPRESENTATION_ITEM()
RATIONAL_B_SPLINE_SURFACE(((0.991846493044689,0.988282393439498,0.987616798999169),
(0.991846493044689,0.988282393439498,0.987616798999169)))
REPRESENTATION_ITEM('')
SURFACE()
);
#2299=(
BOUNDED_SURFACE()
B_SPLINE_SURFACE(1,2,((#132975,#132976,#132977,#132978,#132979),(#132980,
#132981,#132982,#132983,#132984)),.UNSPECIFIED.,.F.,.F.,.F.)
B_SPLINE_SURFACE_WITH_KNOTS((2,2),(3,2,3),(0.,0.289681084359921),(0.487155140750431,
0.5,0.504719756176228),.UNSPECIFIED.)
GEOMETRIC_REPRESENTATION_ITEM()
RATIONAL_B_SPLINE_SURFACE(((0.992604240083356,0.995491335852357,1.,0.998343322021369,
0.996905579294145),(0.992604240083356,0.995491335852357,1.,0.998343322021369,
0.996905579294145)))
REPRESENTATION_ITEM('')
SURFACE()
);
#2300=(
BOUNDED_SURFACE()
B_SPLINE_SURFACE(1,2,((#132986,#132987,#132988),(#132989,#132990,#132991)),
 .UNSPECIFIED.,.F.,.F.,.F.)
B_SPLINE_SURFACE_WITH_KNOTS((2,2),(3,3),(0.,0.289807040991563),(0.228883374894809,
0.246056477139964),.UNSPECIFIED.)
GEOMETRIC_REPRESENTATION_ITEM()
RATIONAL_B_SPLINE_SURFACE(((0.991846493044689,0.988282393439498,0.987616798999169),
(0.991846493044689,0.988282393439498,0.987616798999169)))
REPRESENTATION_ITEM('')
SURFACE()
);
#2301=(
BOUNDED_SURFACE()
B_SPLINE_SURFACE(1,2,((#133014,#133015,#133016,#133017,#133018),(#133019,
#133020,#133021,#133022,#133023)),.UNSPECIFIED.,.F.,.F.,.F.)
B_SPLINE_SURFACE_WITH_KNOTS((2,2),(3,2,3),(0.,0.289681084359926),(0.487155140750431,
0.5,0.504719756176228),.UNSPECIFIED.)
GEOMETRIC_REPRESENTATION_ITEM()
RATIONAL_B_SPLINE_SURFACE(((0.992604240083356,0.995491335852357,1.,0.998343322021369,
0.996905579294145),(0.992604240083356,0.995491335852357,1.,0.998343322021369,
0.996905579294145)))
REPRESENTATION_ITEM('')
SURFACE()
);
#2302=(
BOUNDED_SURFACE()
B_SPLINE_SURFACE(1,2,((#133025,#133026,#133027),(#133028,#133029,#133030)),
 .UNSPECIFIED.,.F.,.F.,.F.)
B_SPLINE_SURFACE_WITH_KNOTS((2,2),(3,3),(0.,0.289807040991564),(0.228883374894809,
0.246056477139964),.UNSPECIFIED.)
GEOMETRIC_REPRESENTATION_ITEM()
RATIONAL_B_SPLINE_SURFACE(((0.991846493044689,0.988282393439498,0.987616798999169),
(0.991846493044689,0.988282393439498,0.987616798999169)))
REPRESENTATION_ITEM('')
SURFACE()
);
#2303=(
BOUNDED_SURFACE()
B_SPLINE_SURFACE(1,2,((#133053,#133054,#133055,#133056,#133057),(#133058,
#133059,#133060,#133061,#133062)),.UNSPECIFIED.,.F.,.F.,.F.)
B_SPLINE_SURFACE_WITH_KNOTS((2,2),(3,2,3),(0.,0.289681084359927),(0.487155140750431,
0.5,0.504719756176228),.UNSPECIFIED.)
GEOMETRIC_REPRESENTATION_ITEM()
RATIONAL_B_SPLINE_SURFACE(((0.992604240083356,0.995491335852357,1.,0.998343322021369,
0.996905579294145),(0.992604240083356,0.995491335852357,1.,0.998343322021369,
0.996905579294145)))
REPRESENTATION_ITEM('')
SURFACE()
);
#2304=(
BOUNDED_SURFACE()
B_SPLINE_SURFACE(1,2,((#133064,#133065,#133066),(#133067,#133068,#133069)),
 .UNSPECIFIED.,.F.,.F.,.F.)
B_SPLINE_SURFACE_WITH_KNOTS((2,2),(3,3),(0.,0.289807040991562),(0.228883374894809,
0.246056477139964),.UNSPECIFIED.)
GEOMETRIC_REPRESENTATION_ITEM()
RATIONAL_B_SPLINE_SURFACE(((0.991846493044689,0.988282393439498,0.987616798999169),
(0.991846493044689,0.988282393439498,0.987616798999169)))
REPRESENTATION_ITEM('')
SURFACE()
);
#2305=(
BOUNDED_SURFACE()
B_SPLINE_SURFACE(1,2,((#133092,#133093,#133094,#133095,#133096),(#133097,
#133098,#133099,#133100,#133101)),.UNSPECIFIED.,.F.,.F.,.F.)
B_SPLINE_SURFACE_WITH_KNOTS((2,2),(3,2,3),(0.,0.289681084359921),(0.487155140750431,
0.5,0.504719756176228),.UNSPECIFIED.)
GEOMETRIC_REPRESENTATION_ITEM()
RATIONAL_B_SPLINE_SURFACE(((0.992604240083356,0.995491335852357,1.,0.998343322021369,
0.996905579294145),(0.992604240083356,0.995491335852357,1.,0.998343322021369,
0.996905579294145)))
REPRESENTATION_ITEM('')
SURFACE()
);
#2306=(
BOUNDED_SURFACE()
B_SPLINE_SURFACE(1,2,((#133103,#133104,#133105),(#133106,#133107,#133108)),
 .UNSPECIFIED.,.F.,.F.,.F.)
B_SPLINE_SURFACE_WITH_KNOTS((2,2),(3,3),(0.,0.289807040991567),(0.228883374894809,
0.246056477139964),.UNSPECIFIED.)
GEOMETRIC_REPRESENTATION_ITEM()
RATIONAL_B_SPLINE_SURFACE(((0.991846493044689,0.988282393439498,0.987616798999169),
(0.991846493044689,0.988282393439498,0.987616798999169)))
REPRESENTATION_ITEM('')
SURFACE()
);
#2307=(
BOUNDED_SURFACE()
B_SPLINE_SURFACE(1,2,((#133131,#133132,#133133,#133134,#133135),(#133136,
#133137,#133138,#133139,#133140)),.UNSPECIFIED.,.F.,.F.,.F.)
B_SPLINE_SURFACE_WITH_KNOTS((2,2),(3,2,3),(0.,0.289681084359922),(0.487155140750431,
0.5,0.504719756176228),.UNSPECIFIED.)
GEOMETRIC_REPRESENTATION_ITEM()
RATIONAL_B_SPLINE_SURFACE(((0.992604240083356,0.995491335852357,1.,0.998343322021369,
0.996905579294145),(0.992604240083356,0.995491335852357,1.,0.998343322021369,
0.996905579294145)))
REPRESENTATION_ITEM('')
SURFACE()
);
#2308=(
BOUNDED_SURFACE()
B_SPLINE_SURFACE(1,2,((#133142,#133143,#133144),(#133145,#133146,#133147)),
 .UNSPECIFIED.,.F.,.F.,.F.)
B_SPLINE_SURFACE_WITH_KNOTS((2,2),(3,3),(0.,0.289807040991561),(0.228883374894809,
0.246056477139964),.UNSPECIFIED.)
GEOMETRIC_REPRESENTATION_ITEM()
RATIONAL_B_SPLINE_SURFACE(((0.991846493044689,0.988282393439498,0.987616798999169),
(0.991846493044689,0.988282393439498,0.987616798999169)))
REPRESENTATION_ITEM('')
SURFACE()
);
#2309=(
BOUNDED_SURFACE()
B_SPLINE_SURFACE(1,2,((#133170,#133171,#133172,#133173,#133174),(#133175,
#133176,#133177,#133178,#133179)),.UNSPECIFIED.,.F.,.F.,.F.)
B_SPLINE_SURFACE_WITH_KNOTS((2,2),(3,2,3),(0.,0.289681084359917),(0.487155140750431,
0.5,0.504719756176228),.UNSPECIFIED.)
GEOMETRIC_REPRESENTATION_ITEM()
RATIONAL_B_SPLINE_SURFACE(((0.992604240083356,0.995491335852357,1.,0.998343322021369,
0.996905579294145),(0.992604240083356,0.995491335852357,1.,0.998343322021369,
0.996905579294145)))
REPRESENTATION_ITEM('')
SURFACE()
);
#2310=(
BOUNDED_SURFACE()
B_SPLINE_SURFACE(1,2,((#133181,#133182,#133183),(#133184,#133185,#133186)),
 .UNSPECIFIED.,.F.,.F.,.F.)
B_SPLINE_SURFACE_WITH_KNOTS((2,2),(3,3),(0.,0.289807040991563),(0.228883374894809,
0.246056477139964),.UNSPECIFIED.)
GEOMETRIC_REPRESENTATION_ITEM()
RATIONAL_B_SPLINE_SURFACE(((0.991846493044689,0.988282393439498,0.987616798999169),
(0.991846493044689,0.988282393439497,0.987616798999169)))
REPRESENTATION_ITEM('')
SURFACE()
);
#2311=(
BOUNDED_SURFACE()
B_SPLINE_SURFACE(1,2,((#133194,#133195,#133196,#133197,#133198),(#133199,
#133200,#133201,#133202,#133203)),.UNSPECIFIED.,.F.,.F.,.F.)
B_SPLINE_SURFACE_WITH_KNOTS((2,2),(3,2,3),(0.,0.28968108435992),(0.487155140750431,
0.5,0.504719756176228),.UNSPECIFIED.)
GEOMETRIC_REPRESENTATION_ITEM()
RATIONAL_B_SPLINE_SURFACE(((0.992604240083356,0.995491335852357,1.,0.998343322021369,
0.996905579294145),(0.992604240083356,0.995491335852357,1.,0.998343322021369,
0.996905579294145)))
REPRESENTATION_ITEM('')
SURFACE()
);
#2312=(
BOUNDED_SURFACE()
B_SPLINE_SURFACE(1,2,((#133205,#133206,#133207),(#133208,#133209,#133210)),
 .UNSPECIFIED.,.F.,.F.,.F.)
B_SPLINE_SURFACE_WITH_KNOTS((2,2),(3,3),(0.,0.289807040991567),(0.228883374894809,
0.246056477139964),.UNSPECIFIED.)
GEOMETRIC_REPRESENTATION_ITEM()
RATIONAL_B_SPLINE_SURFACE(((0.991846493044689,0.988282393439498,0.987616798999169),
(0.991846493044689,0.988282393439498,0.987616798999169)))
REPRESENTATION_ITEM('')
SURFACE()
);
#2313=(
BOUNDED_SURFACE()
B_SPLINE_SURFACE(1,2,((#133233,#133234,#133235,#133236,#133237),(#133238,
#133239,#133240,#133241,#133242)),.UNSPECIFIED.,.F.,.F.,.F.)
B_SPLINE_SURFACE_WITH_KNOTS((2,2),(3,2,3),(0.,0.289681084359922),(0.487155140750431,
0.5,0.504719756176228),.UNSPECIFIED.)
GEOMETRIC_REPRESENTATION_ITEM()
RATIONAL_B_SPLINE_SURFACE(((0.992604240083356,0.995491335852357,1.,0.998343322021369,
0.996905579294145),(0.992604240083356,0.995491335852357,1.,0.998343322021369,
0.996905579294145)))
REPRESENTATION_ITEM('')
SURFACE()
);
#2314=(
BOUNDED_SURFACE()
B_SPLINE_SURFACE(1,2,((#133244,#133245,#133246),(#133247,#133248,#133249)),
 .UNSPECIFIED.,.F.,.F.,.F.)
B_SPLINE_SURFACE_WITH_KNOTS((2,2),(3,3),(0.,0.28980704099156),(0.228883374894809,
0.246056477139964),.UNSPECIFIED.)
GEOMETRIC_REPRESENTATION_ITEM()
RATIONAL_B_SPLINE_SURFACE(((0.991846493044689,0.988282393439498,0.987616798999169),
(0.991846493044689,0.988282393439498,0.987616798999169)))
REPRESENTATION_ITEM('')
SURFACE()
);
#2315=(
BOUNDED_SURFACE()
B_SPLINE_SURFACE(1,2,((#133272,#133273,#133274,#133275,#133276),(#133277,
#133278,#133279,#133280,#133281)),.UNSPECIFIED.,.F.,.F.,.F.)
B_SPLINE_SURFACE_WITH_KNOTS((2,2),(3,2,3),(0.,0.289681084359922),(0.487155140750431,
0.5,0.504719756176228),.UNSPECIFIED.)
GEOMETRIC_REPRESENTATION_ITEM()
RATIONAL_B_SPLINE_SURFACE(((0.992604240083356,0.995491335852357,1.,0.998343322021369,
0.996905579294145),(0.992604240083356,0.995491335852357,1.,0.998343322021369,
0.996905579294145)))
REPRESENTATION_ITEM('')
SURFACE()
);
#2316=(
BOUNDED_SURFACE()
B_SPLINE_SURFACE(1,2,((#133283,#133284,#133285),(#133286,#133287,#133288)),
 .UNSPECIFIED.,.F.,.F.,.F.)
B_SPLINE_SURFACE_WITH_KNOTS((2,2),(3,3),(0.,0.289807040991562),(0.228883374894809,
0.246056477139964),.UNSPECIFIED.)
GEOMETRIC_REPRESENTATION_ITEM()
RATIONAL_B_SPLINE_SURFACE(((0.991846493044689,0.988282393439498,0.987616798999169),
(0.991846493044689,0.988282393439498,0.987616798999169)))
REPRESENTATION_ITEM('')
SURFACE()
);
#2317=(
BOUNDED_SURFACE()
B_SPLINE_SURFACE(1,2,((#133311,#133312,#133313,#133314,#133315),(#133316,
#133317,#133318,#133319,#133320)),.UNSPECIFIED.,.F.,.F.,.F.)
B_SPLINE_SURFACE_WITH_KNOTS((2,2),(3,2,3),(0.,0.289681084359926),(0.487155140750431,
0.5,0.504719756176228),.UNSPECIFIED.)
GEOMETRIC_REPRESENTATION_ITEM()
RATIONAL_B_SPLINE_SURFACE(((0.992604240083356,0.995491335852357,1.,0.998343322021369,
0.996905579294145),(0.992604240083356,0.995491335852357,1.,0.998343322021369,
0.996905579294145)))
REPRESENTATION_ITEM('')
SURFACE()
);
#2318=(
BOUNDED_SURFACE()
B_SPLINE_SURFACE(1,2,((#133322,#133323,#133324),(#133325,#133326,#133327)),
 .UNSPECIFIED.,.F.,.F.,.F.)
B_SPLINE_SURFACE_WITH_KNOTS((2,2),(3,3),(0.,0.289807040991563),(0.228883374894809,
0.246056477139964),.UNSPECIFIED.)
GEOMETRIC_REPRESENTATION_ITEM()
RATIONAL_B_SPLINE_SURFACE(((0.991846493044689,0.988282393439498,0.987616798999169),
(0.991846493044689,0.988282393439498,0.987616798999169)))
REPRESENTATION_ITEM('')
SURFACE()
);
#2319=(
BOUNDED_SURFACE()
B_SPLINE_SURFACE(1,2,((#133350,#133351,#133352,#133353,#133354),(#133355,
#133356,#133357,#133358,#133359)),.UNSPECIFIED.,.F.,.F.,.F.)
B_SPLINE_SURFACE_WITH_KNOTS((2,2),(3,2,3),(0.,0.289681084359923),(0.487155140750431,
0.5,0.504719756176228),.UNSPECIFIED.)
GEOMETRIC_REPRESENTATION_ITEM()
RATIONAL_B_SPLINE_SURFACE(((0.992604240083356,0.995491335852357,1.,0.998343322021369,
0.996905579294145),(0.992604240083356,0.995491335852358,1.,0.998343322021369,
0.996905579294145)))
REPRESENTATION_ITEM('')
SURFACE()
);
#2320=(
BOUNDED_SURFACE()
B_SPLINE_SURFACE(1,2,((#133361,#133362,#133363),(#133364,#133365,#133366)),
 .UNSPECIFIED.,.F.,.F.,.F.)
B_SPLINE_SURFACE_WITH_KNOTS((2,2),(3,3),(0.,0.289807040991562),(0.228883374894809,
0.246056477139964),.UNSPECIFIED.)
GEOMETRIC_REPRESENTATION_ITEM()
RATIONAL_B_SPLINE_SURFACE(((0.991846493044689,0.988282393439498,0.987616798999169),
(0.991846493044689,0.988282393439498,0.987616798999169)))
REPRESENTATION_ITEM('')
SURFACE()
);
#2321=(
BOUNDED_SURFACE()
B_SPLINE_SURFACE(1,2,((#133389,#133390,#133391,#133392,#133393),(#133394,
#133395,#133396,#133397,#133398)),.UNSPECIFIED.,.F.,.F.,.F.)
B_SPLINE_SURFACE_WITH_KNOTS((2,2),(3,2,3),(0.,0.289681084359926),(0.487155140750431,
0.5,0.504719756176228),.UNSPECIFIED.)
GEOMETRIC_REPRESENTATION_ITEM()
RATIONAL_B_SPLINE_SURFACE(((0.992604240083356,0.995491335852358,1.,0.998343322021369,
0.996905579294145),(0.992604240083356,0.995491335852357,1.,0.998343322021369,
0.996905579294145)))
REPRESENTATION_ITEM('')
SURFACE()
);
#2322=(
BOUNDED_SURFACE()
B_SPLINE_SURFACE(1,2,((#133400,#133401,#133402),(#133403,#133404,#133405)),
 .UNSPECIFIED.,.F.,.F.,.F.)
B_SPLINE_SURFACE_WITH_KNOTS((2,2),(3,3),(0.,0.289807040991556),(0.228883374894809,
0.246056477139964),.UNSPECIFIED.)
GEOMETRIC_REPRESENTATION_ITEM()
RATIONAL_B_SPLINE_SURFACE(((0.991846493044689,0.988282393439498,0.987616798999169),
(0.991846493044689,0.988282393439498,0.987616798999169)))
REPRESENTATION_ITEM('')
SURFACE()
);
#2323=(
BOUNDED_SURFACE()
B_SPLINE_SURFACE(1,2,((#133416,#133417,#133418,#133419,#133420),(#133421,
#133422,#133423,#133424,#133425)),.UNSPECIFIED.,.F.,.F.,.F.)
B_SPLINE_SURFACE_WITH_KNOTS((2,2),(3,2,3),(0.,0.289681084360264),(0.487155140750431,
0.5,0.504719756176228),.UNSPECIFIED.)
GEOMETRIC_REPRESENTATION_ITEM()
RATIONAL_B_SPLINE_SURFACE(((0.992604240083356,0.995491335852357,1.,0.998343322021369,
0.996905579294145),(0.992604240083356,0.995491335852357,1.,0.998343322021369,
0.996905579294145)))
REPRESENTATION_ITEM('')
SURFACE()
);
#2324=(
BOUNDED_SURFACE()
B_SPLINE_SURFACE(1,2,((#133439,#133440,#133441),(#133442,#133443,#133444)),
 .UNSPECIFIED.,.F.,.F.,.F.)
B_SPLINE_SURFACE_WITH_KNOTS((2,2),(3,3),(0.,0.289807040991758),(0.228883374894809,
0.246056477139964),.UNSPECIFIED.)
GEOMETRIC_REPRESENTATION_ITEM()
RATIONAL_B_SPLINE_SURFACE(((0.991846493044689,0.988282393439498,0.987616798999169),
(0.991846493044689,0.988282393439498,0.987616798999169)))
REPRESENTATION_ITEM('')
SURFACE()
);
#2325=(
BOUNDED_SURFACE()
B_SPLINE_SURFACE(1,2,((#133467,#133468,#133469,#133470,#133471),(#133472,
#133473,#133474,#133475,#133476)),.UNSPECIFIED.,.F.,.F.,.F.)
B_SPLINE_SURFACE_WITH_KNOTS((2,2),(3,2,3),(0.,0.289681084360126),(0.487155140750322,
0.5,0.504719756194363),.UNSPECIFIED.)
GEOMETRIC_REPRESENTATION_ITEM()
RATIONAL_B_SPLINE_SURFACE(((0.992604240083307,0.995491335852319,1.,0.998343322015004,
0.996905579283096),(0.992604240083307,0.995491335852319,1.,0.998343322015004,
0.996905579283096)))
REPRESENTATION_ITEM('')
SURFACE()
);
#2326=(
BOUNDED_SURFACE()
B_SPLINE_SURFACE(1,2,((#133478,#133479,#133480),(#133481,#133482,#133483)),
 .UNSPECIFIED.,.F.,.F.,.F.)
B_SPLINE_SURFACE_WITH_KNOTS((2,2),(3,3),(0.,0.289807040992207),(0.22888337489481,
0.246056477139965),.UNSPECIFIED.)
GEOMETRIC_REPRESENTATION_ITEM()
RATIONAL_B_SPLINE_SURFACE(((0.991846493044689,0.988282393439497,0.987616798999169),
(0.991846493044689,0.988282393439497,0.987616798999169)))
REPRESENTATION_ITEM('')
SURFACE()
);
#2327=(
BOUNDED_SURFACE()
B_SPLINE_SURFACE(1,2,((#133506,#133507,#133508,#133509,#133510),(#133511,
#133512,#133513,#133514,#133515)),.UNSPECIFIED.,.F.,.F.,.F.)
B_SPLINE_SURFACE_WITH_KNOTS((2,2),(3,2,3),(0.,0.289681084359926),(0.48715514075043,
0.5,0.504719756176227),.UNSPECIFIED.)
GEOMETRIC_REPRESENTATION_ITEM()
RATIONAL_B_SPLINE_SURFACE(((0.992604240083356,0.995491335852357,1.,0.99834332202137,
0.996905579294146),(0.992604240083356,0.995491335852357,1.,0.99834332202137,
0.996905579294146)))
REPRESENTATION_ITEM('')
SURFACE()
);
#2328=(
BOUNDED_SURFACE()
B_SPLINE_SURFACE(1,2,((#133517,#133518,#133519),(#133520,#133521,#133522)),
 .UNSPECIFIED.,.F.,.F.,.F.)
B_SPLINE_SURFACE_WITH_KNOTS((2,2),(3,3),(0.,0.289807040991645),(0.22888337489481,
0.246056477139965),.UNSPECIFIED.)
GEOMETRIC_REPRESENTATION_ITEM()
RATIONAL_B_SPLINE_SURFACE(((0.991846493044689,0.988282393439497,0.987616798999169),
(0.991846493044689,0.988282393439497,0.987616798999169)))
REPRESENTATION_ITEM('')
SURFACE()
);
#2329=(
BOUNDED_SURFACE()
B_SPLINE_SURFACE(1,2,((#133545,#133546,#133547,#133548,#133549),(#133550,
#133551,#133552,#133553,#133554)),.UNSPECIFIED.,.F.,.F.,.F.)
B_SPLINE_SURFACE_WITH_KNOTS((2,2),(3,2,3),(0.,0.289681084359923),(0.487155140750429,
0.5,0.504719756176227),.UNSPECIFIED.)
GEOMETRIC_REPRESENTATION_ITEM()
RATIONAL_B_SPLINE_SURFACE(((0.992604240083356,0.995491335852357,1.,0.99834332202137,
0.996905579294146),(0.992604240083356,0.995491335852357,1.,0.99834332202137,
0.996905579294146)))
REPRESENTATION_ITEM('')
SURFACE()
);
#2330=(
BOUNDED_SURFACE()
B_SPLINE_SURFACE(1,2,((#133556,#133557,#133558),(#133559,#133560,#133561)),
 .UNSPECIFIED.,.F.,.F.,.F.)
B_SPLINE_SURFACE_WITH_KNOTS((2,2),(3,3),(0.,0.289807040991643),(0.22888337489481,
0.246056477139965),.UNSPECIFIED.)
GEOMETRIC_REPRESENTATION_ITEM()
RATIONAL_B_SPLINE_SURFACE(((0.991846493044689,0.988282393439497,0.987616798999169),
(0.991846493044689,0.988282393439497,0.987616798999169)))
REPRESENTATION_ITEM('')
SURFACE()
);
#2331=(
BOUNDED_SURFACE()
B_SPLINE_SURFACE(1,2,((#133584,#133585,#133586,#133587,#133588),(#133589,
#133590,#133591,#133592,#133593)),.UNSPECIFIED.,.F.,.F.,.F.)
B_SPLINE_SURFACE_WITH_KNOTS((2,2),(3,2,3),(0.,0.289681084359917),(0.487155140750429,
0.5,0.504719756176227),.UNSPECIFIED.)
GEOMETRIC_REPRESENTATION_ITEM()
RATIONAL_B_SPLINE_SURFACE(((0.992604240083356,0.995491335852357,1.,0.99834332202137,
0.996905579294146),(0.992604240083356,0.995491335852357,1.,0.99834332202137,
0.996905579294146)))
REPRESENTATION_ITEM('')
SURFACE()
);
#2332=(
BOUNDED_SURFACE()
B_SPLINE_SURFACE(1,2,((#133595,#133596,#133597),(#133598,#133599,#133600)),
 .UNSPECIFIED.,.F.,.F.,.F.)
B_SPLINE_SURFACE_WITH_KNOTS((2,2),(3,3),(0.,0.289807040991633),(0.22888337489481,
0.246056477139965),.UNSPECIFIED.)
GEOMETRIC_REPRESENTATION_ITEM()
RATIONAL_B_SPLINE_SURFACE(((0.991846493044689,0.988282393439497,0.987616798999169),
(0.991846493044689,0.988282393439497,0.987616798999169)))
REPRESENTATION_ITEM('')
SURFACE()
);
#2333=(
BOUNDED_SURFACE()
B_SPLINE_SURFACE(1,2,((#133623,#133624,#133625,#133626,#133627),(#133628,
#133629,#133630,#133631,#133632)),.UNSPECIFIED.,.F.,.F.,.F.)
B_SPLINE_SURFACE_WITH_KNOTS((2,2),(3,2,3),(0.,0.289681084359922),(0.487155140750429,
0.5,0.504719756176227),.UNSPECIFIED.)
GEOMETRIC_REPRESENTATION_ITEM()
RATIONAL_B_SPLINE_SURFACE(((0.992604240083356,0.995491335852357,1.,0.99834332202137,
0.996905579294146),(0.992604240083356,0.995491335852357,1.,0.99834332202137,
0.996905579294146)))
REPRESENTATION_ITEM('')
SURFACE()
);
#2334=(
BOUNDED_SURFACE()
B_SPLINE_SURFACE(1,2,((#133634,#133635,#133636),(#133637,#133638,#133639)),
 .UNSPECIFIED.,.F.,.F.,.F.)
B_SPLINE_SURFACE_WITH_KNOTS((2,2),(3,3),(0.,0.289807040992241),(0.228883374894738,
0.246056477139966),.UNSPECIFIED.)
GEOMETRIC_REPRESENTATION_ITEM()
RATIONAL_B_SPLINE_SURFACE(((0.991846493044719,0.9882823934395,0.987616798999169),
(0.991846493044719,0.9882823934395,0.987616798999169)))
REPRESENTATION_ITEM('')
SURFACE()
);
#2335=(
BOUNDED_SURFACE()
B_SPLINE_SURFACE(1,2,((#133662,#133663,#133664,#133665,#133666),(#133667,
#133668,#133669,#133670,#133671)),.UNSPECIFIED.,.F.,.F.,.F.)
B_SPLINE_SURFACE_WITH_KNOTS((2,2),(3,2,3),(0.,0.289681084360918),(0.48715514075043,
0.5,0.504719756176227),.UNSPECIFIED.)
GEOMETRIC_REPRESENTATION_ITEM()
RATIONAL_B_SPLINE_SURFACE(((0.992604240083356,0.995491335852357,1.,0.99834332202137,
0.996905579294146),(0.992604240083356,0.995491335852357,1.,0.99834332202137,
0.996905579294146)))
REPRESENTATION_ITEM('')
SURFACE()
);
#2336=(
BOUNDED_SURFACE()
B_SPLINE_SURFACE(1,2,((#133673,#133674,#133675),(#133676,#133677,#133678)),
 .UNSPECIFIED.,.F.,.F.,.F.)
B_SPLINE_SURFACE_WITH_KNOTS((2,2),(3,3),(0.,0.289807040991604),(0.228883374894582,
0.246056477139967),.UNSPECIFIED.)
GEOMETRIC_REPRESENTATION_ITEM()
RATIONAL_B_SPLINE_SURFACE(((0.991846493044783,0.988282393439506,0.987616798999169),
(0.991846493044784,0.988282393439506,0.987616798999169)))
REPRESENTATION_ITEM('')
SURFACE()
);
#2337=(
BOUNDED_SURFACE()
B_SPLINE_SURFACE(1,2,((#133701,#133702,#133703,#133704,#133705),(#133706,
#133707,#133708,#133709,#133710)),.UNSPECIFIED.,.F.,.F.,.F.)
B_SPLINE_SURFACE_WITH_KNOTS((2,2),(3,2,3),(0.,0.289681084359918),(0.487155140750429,
0.5,0.504719756176226),.UNSPECIFIED.)
GEOMETRIC_REPRESENTATION_ITEM()
RATIONAL_B_SPLINE_SURFACE(((0.992604240083356,0.995491335852357,1.,0.99834332202137,
0.996905579294146),(0.992604240083356,0.995491335852357,1.,0.99834332202137,
0.996905579294146)))
REPRESENTATION_ITEM('')
SURFACE()
);
#2338=(
BOUNDED_SURFACE()
B_SPLINE_SURFACE(1,2,((#133712,#133713,#133714),(#133715,#133716,#133717)),
 .UNSPECIFIED.,.F.,.F.,.F.)
B_SPLINE_SURFACE_WITH_KNOTS((2,2),(3,3),(0.,0.289807040991624),(0.22888337489437,
0.246056477139968),.UNSPECIFIED.)
GEOMETRIC_REPRESENTATION_ITEM()
RATIONAL_B_SPLINE_SURFACE(((0.991846493044871,0.988282393439514,0.987616798999169),
(0.991846493044871,0.988282393439514,0.987616798999169)))
REPRESENTATION_ITEM('')
SURFACE()
);
#2339=(
BOUNDED_SURFACE()
B_SPLINE_SURFACE(1,2,((#133740,#133741,#133742,#133743,#133744),(#133745,
#133746,#133747,#133748,#133749)),.UNSPECIFIED.,.F.,.F.,.F.)
B_SPLINE_SURFACE_WITH_KNOTS((2,2),(3,2,3),(0.,0.289681084359928),(0.487155140750429,
0.5,0.504719756176226),.UNSPECIFIED.)
GEOMETRIC_REPRESENTATION_ITEM()
RATIONAL_B_SPLINE_SURFACE(((0.992604240083356,0.995491335852357,1.,0.99834332202137,
0.996905579294146),(0.992604240083356,0.995491335852357,1.,0.99834332202137,
0.996905579294146)))
REPRESENTATION_ITEM('')
SURFACE()
);
#2340=(
BOUNDED_SURFACE()
B_SPLINE_SURFACE(1,2,((#133751,#133752,#133753),(#133754,#133755,#133756)),
 .UNSPECIFIED.,.F.,.F.,.F.)
B_SPLINE_SURFACE_WITH_KNOTS((2,2),(3,3),(0.71031891564008,1.),(0.538896351358318,
0.556212823028861),.UNSPECIFIED.)
GEOMETRIC_REPRESENTATION_ITEM()
RATIONAL_B_SPLINE_SURFACE(((0.987563472532048,0.988105030697865,0.991593692313265),
(0.987563472532048,0.988105030697865,0.991593692313265)))
REPRESENTATION_ITEM('')
SURFACE()
);
#2341=(
BOUNDED_SURFACE()
B_SPLINE_SURFACE(1,2,((#133767,#133768,#133769),(#133770,#133771,#133772)),
 .UNSPECIFIED.,.F.,.F.,.F.)
B_SPLINE_SURFACE_WITH_KNOTS((2,2),(3,3),(0.710192959008443,1.),(0.176967058622922,
0.194235682574593),.UNSPECIFIED.)
GEOMETRIC_REPRESENTATION_ITEM()
RATIONAL_B_SPLINE_SURFACE(((0.98748925405691,0.987216959588932,0.989875504592249),
(0.98748925405691,0.987216959588932,0.989875504592249)))
REPRESENTATION_ITEM('')
SURFACE()
);
#2342=(
BOUNDED_SURFACE()
B_SPLINE_SURFACE(1,2,((#133780,#133781,#133782),(#133783,#133784,#133785)),
 .UNSPECIFIED.,.F.,.F.,.F.)
B_SPLINE_SURFACE_WITH_KNOTS((2,2),(3,3),(0.71031891564008,1.),(0.538896351358318,
0.556212823028861),.UNSPECIFIED.)
GEOMETRIC_REPRESENTATION_ITEM()
RATIONAL_B_SPLINE_SURFACE(((0.987563472532048,0.988105030697865,0.991593692313265),
(0.987563472532048,0.988105030697865,0.991593692313265)))
REPRESENTATION_ITEM('')
SURFACE()
);
#2343=(
BOUNDED_SURFACE()
B_SPLINE_SURFACE(1,2,((#133796,#133797,#133798),(#133799,#133800,#133801)),
 .UNSPECIFIED.,.F.,.F.,.F.)
B_SPLINE_SURFACE_WITH_KNOTS((2,2),(3,3),(0.710192959008445,1.),(0.176967058622922,
0.194235682574593),.UNSPECIFIED.)
GEOMETRIC_REPRESENTATION_ITEM()
RATIONAL_B_SPLINE_SURFACE(((0.98748925405691,0.987216959588932,0.989875504592249),
(0.98748925405691,0.987216959588932,0.989875504592249)))
REPRESENTATION_ITEM('')
SURFACE()
);
#2344=(
BOUNDED_SURFACE()
B_SPLINE_SURFACE(1,2,((#133809,#133810,#133811),(#133812,#133813,#133814)),
 .UNSPECIFIED.,.F.,.F.,.F.)
B_SPLINE_SURFACE_WITH_KNOTS((2,2),(3,3),(0.710318915639147,1.),(0.538896351358318,
0.556212823028861),.UNSPECIFIED.)
GEOMETRIC_REPRESENTATION_ITEM()
RATIONAL_B_SPLINE_SURFACE(((0.987563472532048,0.988105030697866,0.991593692313265),
(0.987563472532048,0.988105030697865,0.991593692313265)))
REPRESENTATION_ITEM('')
SURFACE()
);
#2345=(
BOUNDED_SURFACE()
B_SPLINE_SURFACE(1,2,((#133825,#133826,#133827),(#133828,#133829,#133830)),
 .UNSPECIFIED.,.F.,.F.,.F.)
B_SPLINE_SURFACE_WITH_KNOTS((2,2),(3,3),(0.71019295900751,1.),(0.176967058622922,
0.194235682574593),.UNSPECIFIED.)
GEOMETRIC_REPRESENTATION_ITEM()
RATIONAL_B_SPLINE_SURFACE(((0.98748925405691,0.987216959588932,0.989875504592249),
(0.98748925405691,0.987216959588932,0.989875504592249)))
REPRESENTATION_ITEM('')
SURFACE()
);
#2346=(
BOUNDED_SURFACE()
B_SPLINE_SURFACE(1,2,((#133838,#133839,#133840),(#133841,#133842,#133843)),
 .UNSPECIFIED.,.F.,.F.,.F.)
B_SPLINE_SURFACE_WITH_KNOTS((2,2),(3,3),(0.710318915639151,1.),(0.538896351358318,
0.556212823028861),.UNSPECIFIED.)
GEOMETRIC_REPRESENTATION_ITEM()
RATIONAL_B_SPLINE_SURFACE(((0.987563472532048,0.988105030697865,0.991593692313265),
(0.987563472532048,0.988105030697865,0.991593692313265)))
REPRESENTATION_ITEM('')
SURFACE()
);
#2347=(
BOUNDED_SURFACE()
B_SPLINE_SURFACE(1,2,((#133854,#133855,#133856),(#133857,#133858,#133859)),
 .UNSPECIFIED.,.F.,.F.,.F.)
B_SPLINE_SURFACE_WITH_KNOTS((2,2),(3,3),(0.71019295900751,1.),(0.176967058622922,
0.194235682574593),.UNSPECIFIED.)
GEOMETRIC_REPRESENTATION_ITEM()
RATIONAL_B_SPLINE_SURFACE(((0.98748925405691,0.987216959588932,0.989875504592249),
(0.98748925405691,0.987216959588932,0.989875504592249)))
REPRESENTATION_ITEM('')
SURFACE()
);
#2348=(
BOUNDED_SURFACE()
B_SPLINE_SURFACE(1,2,((#133867,#133868,#133869),(#133870,#133871,#133872)),
 .UNSPECIFIED.,.F.,.F.,.F.)
B_SPLINE_SURFACE_WITH_KNOTS((2,2),(3,3),(0.710318915639144,1.),(0.538896351358318,
0.556212823028861),.UNSPECIFIED.)
GEOMETRIC_REPRESENTATION_ITEM()
RATIONAL_B_SPLINE_SURFACE(((0.987563472532048,0.988105030697865,0.991593692313265),
(0.987563472532048,0.988105030697865,0.991593692313265)))
REPRESENTATION_ITEM('')
SURFACE()
);
#2349=(
BOUNDED_SURFACE()
B_SPLINE_SURFACE(1,2,((#133883,#133884,#133885),(#133886,#133887,#133888)),
 .UNSPECIFIED.,.F.,.F.,.F.)
B_SPLINE_SURFACE_WITH_KNOTS((2,2),(3,3),(0.710192959007507,1.),(0.176967058622922,
0.194235682574593),.UNSPECIFIED.)
GEOMETRIC_REPRESENTATION_ITEM()
RATIONAL_B_SPLINE_SURFACE(((0.98748925405691,0.987216959588931,0.989875504592249),
(0.98748925405691,0.987216959588932,0.989875504592249)))
REPRESENTATION_ITEM('')
SURFACE()
);
#2350=(
BOUNDED_SURFACE()
B_SPLINE_SURFACE(1,2,((#133896,#133897,#133898),(#133899,#133900,#133901)),
 .UNSPECIFIED.,.F.,.F.,.F.)
B_SPLINE_SURFACE_WITH_KNOTS((2,2),(3,3),(0.710318915638568,1.),(0.538896351358318,
0.556212823028861),.UNSPECIFIED.)
GEOMETRIC_REPRESENTATION_ITEM()
RATIONAL_B_SPLINE_SURFACE(((0.987563472532048,0.988105030697866,0.991593692313265),
(0.987563472532048,0.988105030697865,0.991593692313265)))
REPRESENTATION_ITEM('')
SURFACE()
);
#2351=(
BOUNDED_SURFACE()
B_SPLINE_SURFACE(1,2,((#133912,#133913,#133914),(#133915,#133916,#133917)),
 .UNSPECIFIED.,.F.,.F.,.F.)
B_SPLINE_SURFACE_WITH_KNOTS((2,2),(3,3),(0.710192959006925,1.),(0.176967058622922,
0.194235682574593),.UNSPECIFIED.)
GEOMETRIC_REPRESENTATION_ITEM()
RATIONAL_B_SPLINE_SURFACE(((0.98748925405691,0.987216959588932,0.989875504592249),
(0.98748925405691,0.987216959588932,0.989875504592249)))
REPRESENTATION_ITEM('')
SURFACE()
);
#2352=(
BOUNDED_SURFACE()
B_SPLINE_SURFACE(1,2,((#133925,#133926,#133927),(#133928,#133929,#133930)),
 .UNSPECIFIED.,.F.,.F.,.F.)
B_SPLINE_SURFACE_WITH_KNOTS((2,2),(3,3),(0.710318915639155,1.),(0.538896351358318,
0.556212823028861),.UNSPECIFIED.)
GEOMETRIC_REPRESENTATION_ITEM()
RATIONAL_B_SPLINE_SURFACE(((0.987563472532048,0.988105030697865,0.991593692313265),
(0.987563472532048,0.988105030697865,0.991593692313265)))
REPRESENTATION_ITEM('')
SURFACE()
);
#2353=(
BOUNDED_SURFACE()
B_SPLINE_SURFACE(1,2,((#133941,#133942,#133943),(#133944,#133945,#133946)),
 .UNSPECIFIED.,.F.,.F.,.F.)
B_SPLINE_SURFACE_WITH_KNOTS((2,2),(3,3),(0.710192959007512,1.),(0.176967058622922,
0.194235682574593),.UNSPECIFIED.)
GEOMETRIC_REPRESENTATION_ITEM()
RATIONAL_B_SPLINE_SURFACE(((0.98748925405691,0.987216959588931,0.989875504592249),
(0.98748925405691,0.987216959588931,0.989875504592249)))
REPRESENTATION_ITEM('')
SURFACE()
);
#2354=(
BOUNDED_SURFACE()
B_SPLINE_SURFACE(1,2,((#133954,#133955,#133956),(#133957,#133958,#133959)),
 .UNSPECIFIED.,.F.,.F.,.F.)
B_SPLINE_SURFACE_WITH_KNOTS((2,2),(3,3),(0.710318915638571,1.),(0.538896351358318,
0.556212823028861),.UNSPECIFIED.)
GEOMETRIC_REPRESENTATION_ITEM()
RATIONAL_B_SPLINE_SURFACE(((0.987563472532048,0.988105030697865,0.991593692313265),
(0.987563472532048,0.988105030697865,0.991593692313265)))
REPRESENTATION_ITEM('')
SURFACE()
);
#2355=(
BOUNDED_SURFACE()
B_SPLINE_SURFACE(1,2,((#133970,#133971,#133972),(#133973,#133974,#133975)),
 .UNSPECIFIED.,.F.,.F.,.F.)
B_SPLINE_SURFACE_WITH_KNOTS((2,2),(3,3),(0.710192959006933,1.),(0.176967058622922,
0.194235682574593),.UNSPECIFIED.)
GEOMETRIC_REPRESENTATION_ITEM()
RATIONAL_B_SPLINE_SURFACE(((0.98748925405691,0.987216959588931,0.989875504592249),
(0.98748925405691,0.987216959588931,0.989875504592249)))
REPRESENTATION_ITEM('')
SURFACE()
);
#2356=(
BOUNDED_SURFACE()
B_SPLINE_SURFACE(1,2,((#133983,#133984,#133985),(#133986,#133987,#133988)),
 .UNSPECIFIED.,.F.,.F.,.F.)
B_SPLINE_SURFACE_WITH_KNOTS((2,2),(3,3),(0.71031891563907,1.),(0.538896351358319,
0.556212823028861),.UNSPECIFIED.)
GEOMETRIC_REPRESENTATION_ITEM()
RATIONAL_B_SPLINE_SURFACE(((0.987563472532048,0.988105030697866,0.991593692313265),
(0.987563472532048,0.988105030697866,0.991593692313265)))
REPRESENTATION_ITEM('')
SURFACE()
);
#2357=(
BOUNDED_SURFACE()
B_SPLINE_SURFACE(1,2,((#133999,#134000,#134001),(#134002,#134003,#134004)),
 .UNSPECIFIED.,.F.,.F.,.F.)
B_SPLINE_SURFACE_WITH_KNOTS((2,2),(3,3),(0.710192959007426,1.),(0.176967058622921,
0.194235682574592),.UNSPECIFIED.)
GEOMETRIC_REPRESENTATION_ITEM()
RATIONAL_B_SPLINE_SURFACE(((0.98748925405691,0.987216959588932,0.989875504592249),
(0.98748925405691,0.987216959588932,0.989875504592249)))
REPRESENTATION_ITEM('')
SURFACE()
);
#2358=(
BOUNDED_SURFACE()
B_SPLINE_SURFACE(1,2,((#134012,#134013,#134014),(#134015,#134016,#134017)),
 .UNSPECIFIED.,.F.,.F.,.F.)
B_SPLINE_SURFACE_WITH_KNOTS((2,2),(3,3),(0.710318915639068,1.),(0.538896351358319,
0.556212823028862),.UNSPECIFIED.)
GEOMETRIC_REPRESENTATION_ITEM()
RATIONAL_B_SPLINE_SURFACE(((0.987563472532048,0.988105030697866,0.991593692313266),
(0.987563472532048,0.988105030697866,0.991593692313266)))
REPRESENTATION_ITEM('')
SURFACE()
);
#2359=(
BOUNDED_SURFACE()
B_SPLINE_SURFACE(1,2,((#134028,#134029,#134030),(#134031,#134032,#134033)),
 .UNSPECIFIED.,.F.,.F.,.F.)
B_SPLINE_SURFACE_WITH_KNOTS((2,2),(3,3),(0.710192959007431,1.),(0.176967058622921,
0.194235682574592),.UNSPECIFIED.)
GEOMETRIC_REPRESENTATION_ITEM()
RATIONAL_B_SPLINE_SURFACE(((0.98748925405691,0.987216959588931,0.989875504592249),
(0.98748925405691,0.987216959588931,0.989875504592249)))
REPRESENTATION_ITEM('')
SURFACE()
);
#2360=(
BOUNDED_SURFACE()
B_SPLINE_SURFACE(1,2,((#134041,#134042,#134043),(#134044,#134045,#134046)),
 .UNSPECIFIED.,.F.,.F.,.F.)
B_SPLINE_SURFACE_WITH_KNOTS((2,2),(3,3),(0.710318915638475,1.),(0.538896351358319,
0.556212823028862),.UNSPECIFIED.)
GEOMETRIC_REPRESENTATION_ITEM()
RATIONAL_B_SPLINE_SURFACE(((0.987563472532048,0.988105030697866,0.991593692313266),
(0.987563472532048,0.988105030697866,0.991593692313266)))
REPRESENTATION_ITEM('')
SURFACE()
);
#2361=(
BOUNDED_SURFACE()
B_SPLINE_SURFACE(1,2,((#134057,#134058,#134059),(#134060,#134061,#134062)),
 .UNSPECIFIED.,.F.,.F.,.F.)
B_SPLINE_SURFACE_WITH_KNOTS((2,2),(3,3),(0.710192959006835,1.),(0.176967058622921,
0.194235682574592),.UNSPECIFIED.)
GEOMETRIC_REPRESENTATION_ITEM()
RATIONAL_B_SPLINE_SURFACE(((0.98748925405691,0.987216959588931,0.989875504592249),
(0.98748925405691,0.987216959588931,0.989875504592249)))
REPRESENTATION_ITEM('')
SURFACE()
);
#2362=(
BOUNDED_SURFACE()
B_SPLINE_SURFACE(1,2,((#134070,#134071,#134072),(#134073,#134074,#134075)),
 .UNSPECIFIED.,.F.,.F.,.F.)
B_SPLINE_SURFACE_WITH_KNOTS((2,2),(3,3),(0.710318915639071,1.),(0.538896351358319,
0.556212823028862),.UNSPECIFIED.)
GEOMETRIC_REPRESENTATION_ITEM()
RATIONAL_B_SPLINE_SURFACE(((0.987563472532048,0.988105030697866,0.991593692313266),
(0.987563472532048,0.988105030697866,0.991593692313266)))
REPRESENTATION_ITEM('')
SURFACE()
);
#2363=(
BOUNDED_SURFACE()
B_SPLINE_SURFACE(1,2,((#134086,#134087,#134088),(#134089,#134090,#134091)),
 .UNSPECIFIED.,.F.,.F.,.F.)
B_SPLINE_SURFACE_WITH_KNOTS((2,2),(3,3),(0.710192959007428,1.),(0.176967058622921,
0.194235682574592),.UNSPECIFIED.)
GEOMETRIC_REPRESENTATION_ITEM()
RATIONAL_B_SPLINE_SURFACE(((0.98748925405691,0.987216959588932,0.989875504592249),
(0.98748925405691,0.987216959588932,0.989875504592249)))
REPRESENTATION_ITEM('')
SURFACE()
);
#2364=(
BOUNDED_SURFACE()
B_SPLINE_SURFACE(1,2,((#134099,#134100,#134101),(#134102,#134103,#134104)),
 .UNSPECIFIED.,.F.,.F.,.F.)
B_SPLINE_SURFACE_WITH_KNOTS((2,2),(3,3),(0.71031891563857,1.),(0.538896351358319,
0.556212823028862),.UNSPECIFIED.)
GEOMETRIC_REPRESENTATION_ITEM()
RATIONAL_B_SPLINE_SURFACE(((0.987563472532048,0.988105030697866,0.991593692313266),
(0.987563472532048,0.988105030697866,0.991593692313266)))
REPRESENTATION_ITEM('')
SURFACE()
);
#2365=(
BOUNDED_SURFACE()
B_SPLINE_SURFACE(1,2,((#134115,#134116,#134117),(#134118,#134119,#134120)),
 .UNSPECIFIED.,.F.,.F.,.F.)
B_SPLINE_SURFACE_WITH_KNOTS((2,2),(3,3),(0.710192959006926,1.),(0.176967058622921,
0.194235682574592),.UNSPECIFIED.)
GEOMETRIC_REPRESENTATION_ITEM()
RATIONAL_B_SPLINE_SURFACE(((0.98748925405691,0.987216959588932,0.989875504592249),
(0.98748925405691,0.987216959588932,0.989875504592249)))
REPRESENTATION_ITEM('')
SURFACE()
);
#2366=(
BOUNDED_SURFACE()
B_SPLINE_SURFACE(1,2,((#134128,#134129,#134130),(#134131,#134132,#134133)),
 .UNSPECIFIED.,.F.,.F.,.F.)
B_SPLINE_SURFACE_WITH_KNOTS((2,2),(3,3),(0.710318915639063,1.),(0.538896351358319,
0.556212823028862),.UNSPECIFIED.)
GEOMETRIC_REPRESENTATION_ITEM()
RATIONAL_B_SPLINE_SURFACE(((0.987563472532048,0.988105030697866,0.991593692313266),
(0.987563472532048,0.988105030697866,0.991593692313266)))
REPRESENTATION_ITEM('')
SURFACE()
);
#2367=(
BOUNDED_SURFACE()
B_SPLINE_SURFACE(1,2,((#134144,#134145,#134146),(#134147,#134148,#134149)),
 .UNSPECIFIED.,.F.,.F.,.F.)
B_SPLINE_SURFACE_WITH_KNOTS((2,2),(3,3),(0.710192959007417,1.),(0.176967058622921,
0.194235682574592),.UNSPECIFIED.)
GEOMETRIC_REPRESENTATION_ITEM()
RATIONAL_B_SPLINE_SURFACE(((0.98748925405691,0.987216959588931,0.989875504592249),
(0.98748925405691,0.987216959588931,0.989875504592249)))
REPRESENTATION_ITEM('')
SURFACE()
);
#2368=(
BOUNDED_SURFACE()
B_SPLINE_SURFACE(1,2,((#134157,#134158,#134159),(#134160,#134161,#134162)),
 .UNSPECIFIED.,.F.,.F.,.F.)
B_SPLINE_SURFACE_WITH_KNOTS((2,2),(3,3),(0.710318915638562,1.),(0.538896351358319,
0.556212823028862),.UNSPECIFIED.)
GEOMETRIC_REPRESENTATION_ITEM()
RATIONAL_B_SPLINE_SURFACE(((0.987563472532048,0.988105030697866,0.991593692313266),
(0.987563472532048,0.988105030697866,0.991593692313266)))
REPRESENTATION_ITEM('')
SURFACE()
);
#2369=(
BOUNDED_SURFACE()
B_SPLINE_SURFACE(1,2,((#134173,#134174,#134175),(#134176,#134177,#134178)),
 .UNSPECIFIED.,.F.,.F.,.F.)
B_SPLINE_SURFACE_WITH_KNOTS((2,2),(3,3),(0.710192959006918,1.),(0.176967058622921,
0.194235682574592),.UNSPECIFIED.)
GEOMETRIC_REPRESENTATION_ITEM()
RATIONAL_B_SPLINE_SURFACE(((0.98748925405691,0.987216959588931,0.989875504592249),
(0.98748925405691,0.987216959588931,0.989875504592249)))
REPRESENTATION_ITEM('')
SURFACE()
);
#2370=(
BOUNDED_SURFACE()
B_SPLINE_SURFACE(1,2,((#134186,#134187,#134188),(#134189,#134190,#134191)),
 .UNSPECIFIED.,.F.,.F.,.F.)
B_SPLINE_SURFACE_WITH_KNOTS((2,2),(3,3),(0.71031891563879,1.),(0.538896351358319,
0.556212823028862),.UNSPECIFIED.)
GEOMETRIC_REPRESENTATION_ITEM()
RATIONAL_B_SPLINE_SURFACE(((0.987563472532048,0.988105030697866,0.991593692313266),
(0.987563472532048,0.988105030697866,0.991593692313266)))
REPRESENTATION_ITEM('')
SURFACE()
);
#2371=(
BOUNDED_SURFACE()
B_SPLINE_SURFACE(1,2,((#134202,#134203,#134204),(#134205,#134206,#134207)),
 .UNSPECIFIED.,.F.,.F.,.F.)
B_SPLINE_SURFACE_WITH_KNOTS((2,2),(3,3),(0.710192959007143,1.),(0.176967058622921,
0.194235682574592),.UNSPECIFIED.)
GEOMETRIC_REPRESENTATION_ITEM()
RATIONAL_B_SPLINE_SURFACE(((0.98748925405691,0.987216959588932,0.989875504592249),
(0.98748925405691,0.987216959588932,0.989875504592249)))
REPRESENTATION_ITEM('')
SURFACE()
);
#2372=(
BOUNDED_SURFACE()
B_SPLINE_SURFACE(1,2,((#134215,#134216,#134217),(#134218,#134219,#134220)),
 .UNSPECIFIED.,.F.,.F.,.F.)
B_SPLINE_SURFACE_WITH_KNOTS((2,2),(3,3),(0.71031891563774,1.),(0.538896351358319,
0.556212823028862),.UNSPECIFIED.)
GEOMETRIC_REPRESENTATION_ITEM()
RATIONAL_B_SPLINE_SURFACE(((0.987563472532048,0.988105030697866,0.991593692313266),
(0.987563472532048,0.988105030697866,0.991593692313266)))
REPRESENTATION_ITEM('')
SURFACE()
);
#2373=(
BOUNDED_SURFACE()
B_SPLINE_SURFACE(1,2,((#134231,#134232,#134233),(#134234,#134235,#134236)),
 .UNSPECIFIED.,.F.,.F.,.F.)
B_SPLINE_SURFACE_WITH_KNOTS((2,2),(3,3),(0.710192959006099,1.),(0.176967058622921,
0.194235682574592),.UNSPECIFIED.)
GEOMETRIC_REPRESENTATION_ITEM()
RATIONAL_B_SPLINE_SURFACE(((0.98748925405691,0.987216959588931,0.989875504592249),
(0.98748925405691,0.987216959588932,0.989875504592249)))
REPRESENTATION_ITEM('')
SURFACE()
);
#2374=(
BOUNDED_SURFACE()
B_SPLINE_SURFACE(1,2,((#134244,#134245,#134246),(#134247,#134248,#134249)),
 .UNSPECIFIED.,.F.,.F.,.F.)
B_SPLINE_SURFACE_WITH_KNOTS((2,2),(3,3),(0.710318915639028,1.),(0.538896351358319,
0.556212823028862),.UNSPECIFIED.)
GEOMETRIC_REPRESENTATION_ITEM()
RATIONAL_B_SPLINE_SURFACE(((0.987563472532048,0.988105030697866,0.991593692313266),
(0.987563472532048,0.988105030697866,0.991593692313266)))
REPRESENTATION_ITEM('')
SURFACE()
);
#2375=(
BOUNDED_SURFACE()
B_SPLINE_SURFACE(1,2,((#134260,#134261,#134262),(#134263,#134264,#134265)),
 .UNSPECIFIED.,.F.,.F.,.F.)
B_SPLINE_SURFACE_WITH_KNOTS((2,2),(3,3),(0.710192959007385,1.),(0.176967058622921,
0.194235682574592),.UNSPECIFIED.)
GEOMETRIC_REPRESENTATION_ITEM()
RATIONAL_B_SPLINE_SURFACE(((0.98748925405691,0.987216959588932,0.989875504592249),
(0.98748925405691,0.987216959588932,0.989875504592249)))
REPRESENTATION_ITEM('')
SURFACE()
);
#2376=(
BOUNDED_SURFACE()
B_SPLINE_SURFACE(1,2,((#134273,#134274,#134275),(#134276,#134277,#134278)),
 .UNSPECIFIED.,.F.,.F.,.F.)
B_SPLINE_SURFACE_WITH_KNOTS((2,2),(3,3),(0.710318915639144,1.),(0.538896351358319,
0.556212823028862),.UNSPECIFIED.)
GEOMETRIC_REPRESENTATION_ITEM()
RATIONAL_B_SPLINE_SURFACE(((0.987563472532048,0.988105030697866,0.991593692313266),
(0.987563472532048,0.988105030697866,0.991593692313266)))
REPRESENTATION_ITEM('')
SURFACE()
);
#2377=(
BOUNDED_SURFACE()
B_SPLINE_SURFACE(1,2,((#134289,#134290,#134291),(#134292,#134293,#134294)),
 .UNSPECIFIED.,.F.,.F.,.F.)
B_SPLINE_SURFACE_WITH_KNOTS((2,2),(3,3),(0.710192959007499,1.),(0.176967058622921,
0.194235682574596),.UNSPECIFIED.)
GEOMETRIC_REPRESENTATION_ITEM()
RATIONAL_B_SPLINE_SURFACE(((0.98748925405691,0.987216959588931,0.98987550459225),
(0.98748925405691,0.987216959588931,0.98987550459225)))
REPRESENTATION_ITEM('')
SURFACE()
);
#2378=(
BOUNDED_SURFACE()
B_SPLINE_SURFACE(1,2,((#134302,#134303,#134304),(#134305,#134306,#134307)),
 .UNSPECIFIED.,.F.,.F.,.F.)
B_SPLINE_SURFACE_WITH_KNOTS((2,2),(3,3),(0.710318915638508,1.),(0.538896351358319,
0.556212823028862),.UNSPECIFIED.)
GEOMETRIC_REPRESENTATION_ITEM()
RATIONAL_B_SPLINE_SURFACE(((0.987563472532048,0.988105030697866,0.991593692313266),
(0.987563472532048,0.988105030697866,0.991593692313266)))
REPRESENTATION_ITEM('')
SURFACE()
);
#2379=(
BOUNDED_SURFACE()
B_SPLINE_SURFACE(1,2,((#134318,#134319,#134320),(#134321,#134322,#134323)),
 .UNSPECIFIED.,.F.,.F.,.F.)
B_SPLINE_SURFACE_WITH_KNOTS((2,2),(3,3),(0.710192959006863,1.),(0.176967058622921,
0.194235682574592),.UNSPECIFIED.)
GEOMETRIC_REPRESENTATION_ITEM()
RATIONAL_B_SPLINE_SURFACE(((0.98748925405691,0.987216959588931,0.989875504592249),
(0.98748925405691,0.987216959588931,0.989875504592249)))
REPRESENTATION_ITEM('')
SURFACE()
);
#2380=(
BOUNDED_SURFACE()
B_SPLINE_SURFACE(1,2,((#134331,#134332,#134333),(#134334,#134335,#134336)),
 .UNSPECIFIED.,.F.,.F.,.F.)
B_SPLINE_SURFACE_WITH_KNOTS((2,2),(3,3),(0.71031891563991,1.),(0.538896351358319,
0.556212823028862),.UNSPECIFIED.)
GEOMETRIC_REPRESENTATION_ITEM()
RATIONAL_B_SPLINE_SURFACE(((0.987563472532048,0.988105030697866,0.991593692313266),
(0.987563472532048,0.988105030697866,0.991593692313266)))
REPRESENTATION_ITEM('')
SURFACE()
);
#2381=(
BOUNDED_SURFACE()
B_SPLINE_SURFACE(1,2,((#134347,#134348,#134349),(#134350,#134351,#134352)),
 .UNSPECIFIED.,.F.,.F.,.F.)
B_SPLINE_SURFACE_WITH_KNOTS((2,2),(3,3),(0.710192959008264,1.),(0.176967058622921,
0.194235682574593),.UNSPECIFIED.)
GEOMETRIC_REPRESENTATION_ITEM()
RATIONAL_B_SPLINE_SURFACE(((0.98748925405691,0.987216959588931,0.989875504592249),
(0.98748925405691,0.987216959588932,0.989875504592249)))
REPRESENTATION_ITEM('')
SURFACE()
);
#2382=(
BOUNDED_SURFACE()
B_SPLINE_SURFACE(1,2,((#134360,#134361,#134362),(#134363,#134364,#134365)),
 .UNSPECIFIED.,.F.,.F.,.F.)
B_SPLINE_SURFACE_WITH_KNOTS((2,2),(3,3),(0.710318915638761,1.),(0.538896351358319,
0.556212823028862),.UNSPECIFIED.)
GEOMETRIC_REPRESENTATION_ITEM()
RATIONAL_B_SPLINE_SURFACE(((0.987563472532048,0.988105030697866,0.991593692313266),
(0.987563472532048,0.988105030697866,0.991593692313266)))
REPRESENTATION_ITEM('')
SURFACE()
);
#2383=(
BOUNDED_SURFACE()
B_SPLINE_SURFACE(1,2,((#134376,#134377,#134378),(#134379,#134380,#134381)),
 .UNSPECIFIED.,.F.,.F.,.F.)
B_SPLINE_SURFACE_WITH_KNOTS((2,2),(3,3),(0.710192959007121,1.),(0.176967058622921,
0.194235682574592),.UNSPECIFIED.)
GEOMETRIC_REPRESENTATION_ITEM()
RATIONAL_B_SPLINE_SURFACE(((0.98748925405691,0.987216959588932,0.989875504592249),
(0.98748925405691,0.987216959588932,0.989875504592249)))
REPRESENTATION_ITEM('')
SURFACE()
);
#2384=(
BOUNDED_SURFACE()
B_SPLINE_SURFACE(1,2,((#134389,#134390,#134391),(#134392,#134393,#134394)),
 .UNSPECIFIED.,.F.,.F.,.F.)
B_SPLINE_SURFACE_WITH_KNOTS((2,2),(3,3),(0.710318915638945,1.),(0.538896351358319,
0.556212823028862),.UNSPECIFIED.)
GEOMETRIC_REPRESENTATION_ITEM()
RATIONAL_B_SPLINE_SURFACE(((0.987563472532048,0.988105030697866,0.991593692313266),
(0.987563472532048,0.988105030697866,0.991593692313266)))
REPRESENTATION_ITEM('')
SURFACE()
);
#2385=(
BOUNDED_SURFACE()
B_SPLINE_SURFACE(1,2,((#134405,#134406,#134407),(#134408,#134409,#134410)),
 .UNSPECIFIED.,.F.,.F.,.F.)
B_SPLINE_SURFACE_WITH_KNOTS((2,2),(3,3),(0.710192959007306,1.),(0.176967058622921,
0.194235682574592),.UNSPECIFIED.)
GEOMETRIC_REPRESENTATION_ITEM()
RATIONAL_B_SPLINE_SURFACE(((0.98748925405691,0.987216959588932,0.989875504592249),
(0.98748925405691,0.987216959588932,0.989875504592249)))
REPRESENTATION_ITEM('')
SURFACE()
);
#2386=(
BOUNDED_SURFACE()
B_SPLINE_SURFACE(1,2,((#134418,#134419,#134420),(#134421,#134422,#134423)),
 .UNSPECIFIED.,.F.,.F.,.F.)
B_SPLINE_SURFACE_WITH_KNOTS((2,2),(3,3),(0.710318915637902,1.),(0.538896351358319,
0.556212823028862),.UNSPECIFIED.)
GEOMETRIC_REPRESENTATION_ITEM()
RATIONAL_B_SPLINE_SURFACE(((0.987563472532048,0.988105030697866,0.991593692313266),
(0.987563472532048,0.988105030697866,0.991593692313266)))
REPRESENTATION_ITEM('')
SURFACE()
);
#2387=(
BOUNDED_SURFACE()
B_SPLINE_SURFACE(1,2,((#134434,#134435,#134436),(#134437,#134438,#134439)),
 .UNSPECIFIED.,.F.,.F.,.F.)
B_SPLINE_SURFACE_WITH_KNOTS((2,2),(3,3),(0.710192959006265,1.),(0.176967058622921,
0.194235682574592),.UNSPECIFIED.)
GEOMETRIC_REPRESENTATION_ITEM()
RATIONAL_B_SPLINE_SURFACE(((0.98748925405691,0.987216959588932,0.989875504592249),
(0.98748925405691,0.987216959588932,0.989875504592249)))
REPRESENTATION_ITEM('')
SURFACE()
);
#2388=(
BOUNDED_SURFACE()
B_SPLINE_SURFACE(1,2,((#134447,#134448,#134449),(#134450,#134451,#134452)),
 .UNSPECIFIED.,.F.,.F.,.F.)
B_SPLINE_SURFACE_WITH_KNOTS((2,2),(3,3),(0.710318915639735,1.),(0.538896351358319,
0.556212823028863),.UNSPECIFIED.)
GEOMETRIC_REPRESENTATION_ITEM()
RATIONAL_B_SPLINE_SURFACE(((0.987563472532048,0.988105030697866,0.991593692313266),
(0.987563472532048,0.988105030697866,0.991593692313266)))
REPRESENTATION_ITEM('')
SURFACE()
);
#2389=(
BOUNDED_SURFACE()
B_SPLINE_SURFACE(1,2,((#134463,#134464,#134465),(#134466,#134467,#134468)),
 .UNSPECIFIED.,.F.,.F.,.F.)
B_SPLINE_SURFACE_WITH_KNOTS((2,2),(3,3),(0.710192959008098,1.),(0.176967058622921,
0.194235682574592),.UNSPECIFIED.)
GEOMETRIC_REPRESENTATION_ITEM()
RATIONAL_B_SPLINE_SURFACE(((0.98748925405691,0.987216959588931,0.989875504592249),
(0.98748925405691,0.987216959588931,0.989875504592249)))
REPRESENTATION_ITEM('')
SURFACE()
);
#2390=(
BOUNDED_SURFACE()
B_SPLINE_SURFACE(1,2,((#134476,#134477,#134478),(#134479,#134480,#134481)),
 .UNSPECIFIED.,.F.,.F.,.F.)
B_SPLINE_SURFACE_WITH_KNOTS((2,2),(3,3),(0.710318915638586,1.),(0.538896351358319,
0.556212823028862),.UNSPECIFIED.)
GEOMETRIC_REPRESENTATION_ITEM()
RATIONAL_B_SPLINE_SURFACE(((0.987563472532048,0.988105030697866,0.991593692313266),
(0.987563472532048,0.988105030697866,0.991593692313266)))
REPRESENTATION_ITEM('')
SURFACE()
);
#2391=(
BOUNDED_SURFACE()
B_SPLINE_SURFACE(1,2,((#134492,#134493,#134494),(#134495,#134496,#134497)),
 .UNSPECIFIED.,.F.,.F.,.F.)
B_SPLINE_SURFACE_WITH_KNOTS((2,2),(3,3),(0.710192959006949,1.),(0.176967058622921,
0.194235682574592),.UNSPECIFIED.)
GEOMETRIC_REPRESENTATION_ITEM()
RATIONAL_B_SPLINE_SURFACE(((0.98748925405691,0.987216959588931,0.989875504592249),
(0.98748925405691,0.987216959588931,0.989875504592249)))
REPRESENTATION_ITEM('')
SURFACE()
);
#2392=(
BOUNDED_SURFACE()
B_SPLINE_SURFACE(1,2,((#134505,#134506,#134507),(#134508,#134509,#134510)),
 .UNSPECIFIED.,.F.,.F.,.F.)
B_SPLINE_SURFACE_WITH_KNOTS((2,2),(3,3),(0.710318915638841,1.),(0.538896351358319,
0.556212823028862),.UNSPECIFIED.)
GEOMETRIC_REPRESENTATION_ITEM()
RATIONAL_B_SPLINE_SURFACE(((0.987563472532048,0.988105030697866,0.991593692313266),
(0.987563472532048,0.988105030697866,0.991593692313266)))
REPRESENTATION_ITEM('')
SURFACE()
);
#2393=(
BOUNDED_SURFACE()
B_SPLINE_SURFACE(1,2,((#134521,#134522,#134523),(#134524,#134525,#134526)),
 .UNSPECIFIED.,.F.,.F.,.F.)
B_SPLINE_SURFACE_WITH_KNOTS((2,2),(3,3),(0.710192959007194,1.),(0.176967058622922,
0.194235682574592),.UNSPECIFIED.)
GEOMETRIC_REPRESENTATION_ITEM()
RATIONAL_B_SPLINE_SURFACE(((0.98748925405691,0.987216959588932,0.989875504592249),
(0.98748925405691,0.987216959588932,0.989875504592249)))
REPRESENTATION_ITEM('')
SURFACE()
);
#2394=(
BOUNDED_SURFACE()
B_SPLINE_SURFACE(1,2,((#134534,#134535,#134536),(#134537,#134538,#134539)),
 .UNSPECIFIED.,.F.,.F.,.F.)
B_SPLINE_SURFACE_WITH_KNOTS((2,2),(3,3),(0.710318915640079,1.),(0.538896351358318,
0.556212823028861),.UNSPECIFIED.)
GEOMETRIC_REPRESENTATION_ITEM()
RATIONAL_B_SPLINE_SURFACE(((0.987563472532048,0.988105030697865,0.991593692313265),
(0.987563472532048,0.988105030697865,0.991593692313265)))
REPRESENTATION_ITEM('')
SURFACE()
);
#2395=(
BOUNDED_SURFACE()
B_SPLINE_SURFACE(1,2,((#134550,#134551,#134552),(#134553,#134554,#134555)),
 .UNSPECIFIED.,.F.,.F.,.F.)
B_SPLINE_SURFACE_WITH_KNOTS((2,2),(3,3),(0.71019295900844,1.),(0.176967058622922,
0.194235682574593),.UNSPECIFIED.)
GEOMETRIC_REPRESENTATION_ITEM()
RATIONAL_B_SPLINE_SURFACE(((0.98748925405691,0.987216959588932,0.989875504592249),
(0.98748925405691,0.987216959588932,0.989875504592249)))
REPRESENTATION_ITEM('')
SURFACE()
);
#2396=(
BOUNDED_SURFACE()
B_SPLINE_SURFACE(1,2,((#134563,#134564,#134565),(#134566,#134567,#134568)),
 .UNSPECIFIED.,.F.,.F.,.F.)
B_SPLINE_SURFACE_WITH_KNOTS((2,2),(3,3),(0.710318915640083,1.),(0.538896351358318,
0.556212823028861),.UNSPECIFIED.)
GEOMETRIC_REPRESENTATION_ITEM()
RATIONAL_B_SPLINE_SURFACE(((0.987563472532048,0.988105030697865,0.991593692313265),
(0.987563472532048,0.988105030697865,0.991593692313265)))
REPRESENTATION_ITEM('')
SURFACE()
);
#2397=(
BOUNDED_SURFACE()
B_SPLINE_SURFACE(1,2,((#134579,#134580,#134581),(#134582,#134583,#134584)),
 .UNSPECIFIED.,.F.,.F.,.F.)
B_SPLINE_SURFACE_WITH_KNOTS((2,2),(3,3),(0.710192959008441,1.),(0.176967058622922,
0.194235682574593),.UNSPECIFIED.)
GEOMETRIC_REPRESENTATION_ITEM()
RATIONAL_B_SPLINE_SURFACE(((0.98748925405691,0.987216959588932,0.989875504592249),
(0.98748925405691,0.987216959588932,0.989875504592249)))
REPRESENTATION_ITEM('')
SURFACE()
);
#2398=(
BOUNDED_SURFACE()
B_SPLINE_SURFACE(1,2,((#134592,#134593,#134594,#134595,#134596),(#134597,
#134598,#134599,#134600,#134601)),.UNSPECIFIED.,.F.,.F.,.F.)
B_SPLINE_SURFACE_WITH_KNOTS((2,2),(3,2,3),(0.710192959006966,1.),(0.504546746572904,
0.504719756175826,0.522020716468042),.UNSPECIFIED.)
GEOMETRIC_REPRESENTATION_ITEM()
RATIONAL_B_SPLINE_SURFACE(((0.99690557929439,0.99690557929439,0.99690557929439,
0.991635321911236,0.989306890555884),(0.99690557929439,0.99690557929439,
0.99690557929439,0.991635321911236,0.989306890555884)))
REPRESENTATION_ITEM('')
SURFACE()
);
#2399=(
BOUNDED_SURFACE()
B_SPLINE_SURFACE(1,2,((#134614,#134615,#134616,#134617,#134618,#134619,
#134620),(#134621,#134622,#134623,#134624,#134625,#134626,#134627)),
 .UNSPECIFIED.,.F.,.F.,.F.)
B_SPLINE_SURFACE_WITH_KNOTS((2,2),(3,2,2,3),(0.710318915640022,1.),(0.211398300093701,
0.214285714285714,0.228883374894809,0.22905822564282),.UNSPECIFIED.)
GEOMETRIC_REPRESENTATION_ITEM()
RATIONAL_B_SPLINE_SURFACE(((0.998054921708739,0.998986490969345,1.,0.994876086397764,
0.991846493044689,0.991846493044689,0.991846493044689),(0.998054921708739,
0.998986490969345,1.,0.994876086397764,0.991846493044689,0.991846493044689,
0.991846493044689)))
REPRESENTATION_ITEM('')
SURFACE()
);
#2400=(
BOUNDED_SURFACE()
B_SPLINE_SURFACE(1,2,((#134638,#134639,#134640,#134641,#134642),(#134643,
#134644,#134645,#134646,#134647)),.UNSPECIFIED.,.F.,.F.,.F.)
B_SPLINE_SURFACE_WITH_KNOTS((2,2),(3,2,3),(0.710192959007032,1.),(0.504546746573206,
0.504719756176125,0.522020716468041),.UNSPECIFIED.)
GEOMETRIC_REPRESENTATION_ITEM()
RATIONAL_B_SPLINE_SURFACE(((0.996905579294208,0.996905579294208,0.996905579294208,
0.991635321911196,0.989306890555884),(0.996905579294208,0.996905579294208,
0.996905579294208,0.991635321911196,0.989306890555884)))
REPRESENTATION_ITEM('')
SURFACE()
);
#2401=(
BOUNDED_SURFACE()
B_SPLINE_SURFACE(1,2,((#134660,#134661,#134662,#134663,#134664,#134665,
#134666),(#134667,#134668,#134669,#134670,#134671,#134672,#134673)),
 .UNSPECIFIED.,.F.,.F.,.F.)
B_SPLINE_SURFACE_WITH_KNOTS((2,2),(3,2,2,3),(0.710318915640066,1.),(0.2113983000937,
0.214285714285714,0.228883374894809,0.22905822564282),.UNSPECIFIED.)
GEOMETRIC_REPRESENTATION_ITEM()
RATIONAL_B_SPLINE_SURFACE(((0.998054921708738,0.998986490969345,1.,0.994876086397764,
0.991846493044689,0.991846493044689,0.991846493044689),(0.998054921708738,
0.998986490969345,1.,0.994876086397764,0.991846493044689,0.991846493044689,
0.991846493044689)))
REPRESENTATION_ITEM('')
SURFACE()
);
#2402=(
BOUNDED_SURFACE()
B_SPLINE_SURFACE(1,2,((#134684,#134685,#134686,#134687,#134688),(#134689,
#134690,#134691,#134692,#134693)),.UNSPECIFIED.,.F.,.F.,.F.)
B_SPLINE_SURFACE_WITH_KNOTS((2,2),(3,2,3),(0.710192959007032,1.),(0.504546746573288,
0.504719756176206,0.522020716468041),.UNSPECIFIED.)
GEOMETRIC_REPRESENTATION_ITEM()
RATIONAL_B_SPLINE_SURFACE(((0.996905579294158,0.996905579294158,0.996905579294158,
0.991635321911186,0.989306890555884),(0.996905579294158,0.996905579294158,
0.996905579294158,0.991635321911186,0.989306890555884)))
REPRESENTATION_ITEM('')
SURFACE()
);
#2403=(
BOUNDED_SURFACE()
B_SPLINE_SURFACE(1,2,((#134706,#134707,#134708,#134709,#134710,#134711,
#134712),(#134713,#134714,#134715,#134716,#134717,#134718,#134719)),
 .UNSPECIFIED.,.F.,.F.,.F.)
B_SPLINE_SURFACE_WITH_KNOTS((2,2),(3,2,2,3),(0.710318915639876,1.),(0.2113983000937,
0.214285714285714,0.228883374894809,0.22905822564282),.UNSPECIFIED.)
GEOMETRIC_REPRESENTATION_ITEM()
RATIONAL_B_SPLINE_SURFACE(((0.998054921708738,0.998986490969345,1.,0.994876086397764,
0.991846493044689,0.991846493044689,0.991846493044689),(0.998054921708738,
0.998986490969345,1.,0.994876086397764,0.991846493044689,0.991846493044689,
0.991846493044689)))
REPRESENTATION_ITEM('')
SURFACE()
);
#2404=(
BOUNDED_SURFACE()
B_SPLINE_SURFACE(1,2,((#134730,#134731,#134732,#134733,#134734),(#134735,
#134736,#134737,#134738,#134739)),.UNSPECIFIED.,.F.,.F.,.F.)
B_SPLINE_SURFACE_WITH_KNOTS((2,2),(3,2,3),(0.710192959007029,1.),(0.504546746573288,
0.504719756176206,0.522020716468041),.UNSPECIFIED.)
GEOMETRIC_REPRESENTATION_ITEM()
RATIONAL_B_SPLINE_SURFACE(((0.996905579294158,0.996905579294158,0.996905579294158,
0.991635321911186,0.989306890555884),(0.996905579294158,0.996905579294158,
0.996905579294158,0.991635321911186,0.989306890555885)))
REPRESENTATION_ITEM('')
SURFACE()
);
#2405=(
BOUNDED_SURFACE()
B_SPLINE_SURFACE(1,2,((#134752,#134753,#134754,#134755,#134756,#134757,
#134758),(#134759,#134760,#134761,#134762,#134763,#134764,#134765)),
 .UNSPECIFIED.,.F.,.F.,.F.)
B_SPLINE_SURFACE_WITH_KNOTS((2,2),(3,2,2,3),(0.71031891564008,1.),(0.2113983000937,
0.214285714285714,0.228883374894809,0.22905822564282),.UNSPECIFIED.)
GEOMETRIC_REPRESENTATION_ITEM()
RATIONAL_B_SPLINE_SURFACE(((0.998054921708738,0.998986490969345,1.,0.994876086397764,
0.991846493044689,0.991846493044689,0.991846493044689),(0.998054921708738,
0.998986490969345,1.,0.994876086397764,0.991846493044689,0.991846493044689,
0.991846493044689)))
REPRESENTATION_ITEM('')
SURFACE()
);
#2406=(
BOUNDED_SURFACE()
B_SPLINE_SURFACE(1,2,((#134776,#134777,#134778,#134779,#134780),(#134781,
#134782,#134783,#134784,#134785)),.UNSPECIFIED.,.F.,.F.,.F.)
B_SPLINE_SURFACE_WITH_KNOTS((2,2),(3,2,3),(0.710192959007034,1.),(0.504546746572823,
0.504719756175746,0.522020716468043),.UNSPECIFIED.)
GEOMETRIC_REPRESENTATION_ITEM()
RATIONAL_B_SPLINE_SURFACE(((0.996905579294439,0.996905579294439,0.996905579294439,
0.991635321911247,0.989306890555884),(0.996905579294439,0.996905579294439,
0.996905579294439,0.991635321911247,0.989306890555884)))
REPRESENTATION_ITEM('')
SURFACE()
);
#2407=(
BOUNDED_SURFACE()
B_SPLINE_SURFACE(1,2,((#134798,#134799,#134800,#134801,#134802,#134803,
#134804),(#134805,#134806,#134807,#134808,#134809,#134810,#134811)),
 .UNSPECIFIED.,.F.,.F.,.F.)
B_SPLINE_SURFACE_WITH_KNOTS((2,2),(3,2,2,3),(0.710318915639999,1.),(0.211398300093699,
0.214285714285714,0.228883374894809,0.22905822564282),.UNSPECIFIED.)
GEOMETRIC_REPRESENTATION_ITEM()
RATIONAL_B_SPLINE_SURFACE(((0.998054921708737,0.998986490969345,1.,0.994876086397764,
0.991846493044689,0.991846493044689,0.991846493044689),(0.998054921708737,
0.998986490969345,1.,0.994876086397764,0.991846493044689,0.991846493044689,
0.991846493044689)))
REPRESENTATION_ITEM('')
SURFACE()
);
#2408=(
BOUNDED_SURFACE()
B_SPLINE_SURFACE(1,2,((#134822,#134823,#134824,#134825,#134826),(#134827,
#134828,#134829,#134830,#134831)),.UNSPECIFIED.,.F.,.F.,.F.)
B_SPLINE_SURFACE_WITH_KNOTS((2,2),(3,2,3),(0.71019295900703,1.),(0.504546746572967,
0.504719756175888,0.522020716468043),.UNSPECIFIED.)
GEOMETRIC_REPRESENTATION_ITEM()
RATIONAL_B_SPLINE_SURFACE(((0.996905579294352,0.996905579294352,0.996905579294352,
0.991635321911228,0.989306890555884),(0.996905579294352,0.996905579294352,
0.996905579294352,0.991635321911228,0.989306890555884)))
REPRESENTATION_ITEM('')
SURFACE()
);
#2409=(
BOUNDED_SURFACE()
B_SPLINE_SURFACE(1,2,((#134844,#134845,#134846,#134847,#134848,#134849,
#134850),(#134851,#134852,#134853,#134854,#134855,#134856,#134857)),
 .UNSPECIFIED.,.F.,.F.,.F.)
B_SPLINE_SURFACE_WITH_KNOTS((2,2),(3,2,2,3),(0.710318915640028,1.),(0.2113983000937,
0.214285714285714,0.228883374894809,0.22905822564282),.UNSPECIFIED.)
GEOMETRIC_REPRESENTATION_ITEM()
RATIONAL_B_SPLINE_SURFACE(((0.998054921708738,0.998986490969345,1.,0.994876086397764,
0.991846493044689,0.991846493044689,0.991846493044689),(0.998054921708738,
0.998986490969345,1.,0.994876086397764,0.991846493044689,0.991846493044689,
0.991846493044689)))
REPRESENTATION_ITEM('')
SURFACE()
);
#2410=(
BOUNDED_SURFACE()
B_SPLINE_SURFACE(1,2,((#134872,#134873,#134874,#134875,#134876),(#134877,
#134878,#134879,#134880,#134881)),.UNSPECIFIED.,.F.,.F.,.F.)
B_SPLINE_SURFACE_WITH_KNOTS((2,2),(3,2,3),(0.710192959007035,1.),(0.504546746573141,
0.504719756176061,0.522020716468042),.UNSPECIFIED.)
GEOMETRIC_REPRESENTATION_ITEM()
RATIONAL_B_SPLINE_SURFACE(((0.996905579294247,0.996905579294247,0.996905579294247,
0.991635321911205,0.989306890555884),(0.996905579294247,0.996905579294247,
0.996905579294247,0.991635321911205,0.989306890555884)))
REPRESENTATION_ITEM('')
SURFACE()
);
#2411=(
BOUNDED_SURFACE()
B_SPLINE_SURFACE(1,2,((#134894,#134895,#134896,#134897,#134898,#134899,
#134900),(#134901,#134902,#134903,#134904,#134905,#134906,#134907)),
 .UNSPECIFIED.,.F.,.F.,.F.)
B_SPLINE_SURFACE_WITH_KNOTS((2,2),(3,2,2,3),(0.710318915639771,1.),(0.2113983000937,
0.214285714285714,0.228883374894809,0.22905822564282),.UNSPECIFIED.)
GEOMETRIC_REPRESENTATION_ITEM()
RATIONAL_B_SPLINE_SURFACE(((0.998054921708738,0.998986490969345,1.,0.994876086397764,
0.991846493044689,0.991846493044689,0.991846493044689),(0.998054921708738,
0.998986490969345,1.,0.994876086397764,0.991846493044689,0.991846493044689,
0.991846493044689)))
REPRESENTATION_ITEM('')
SURFACE()
);
#2412=(
BOUNDED_SURFACE()
B_SPLINE_SURFACE(1,2,((#134918,#134919,#134920,#134921,#134922),(#134923,
#134924,#134925,#134926,#134927)),.UNSPECIFIED.,.F.,.F.,.F.)
B_SPLINE_SURFACE_WITH_KNOTS((2,2),(3,2,3),(0.710192959007034,1.),(0.504546746573288,
0.504719756176206,0.522020716468041),.UNSPECIFIED.)
GEOMETRIC_REPRESENTATION_ITEM()
RATIONAL_B_SPLINE_SURFACE(((0.996905579294158,0.996905579294158,0.996905579294158,
0.991635321911186,0.989306890555884),(0.996905579294158,0.996905579294158,
0.996905579294158,0.991635321911186,0.989306890555884)))
REPRESENTATION_ITEM('')
SURFACE()
);
#2413=(
BOUNDED_SURFACE()
B_SPLINE_SURFACE(1,2,((#134940,#134941,#134942,#134943,#134944,#134945,
#134946),(#134947,#134948,#134949,#134950,#134951,#134952,#134953)),
 .UNSPECIFIED.,.F.,.F.,.F.)
B_SPLINE_SURFACE_WITH_KNOTS((2,2),(3,2,2,3),(0.710318915639696,1.),(0.2113983000937,
0.214285714285714,0.228883374894809,0.22905822564282),.UNSPECIFIED.)
GEOMETRIC_REPRESENTATION_ITEM()
RATIONAL_B_SPLINE_SURFACE(((0.998054921708738,0.998986490969345,1.,0.994876086397764,
0.991846493044689,0.991846493044689,0.991846493044689),(0.998054921708738,
0.998986490969345,1.,0.994876086397764,0.991846493044689,0.991846493044689,
0.991846493044689)))
REPRESENTATION_ITEM('')
SURFACE()
);
#2414=(
BOUNDED_SURFACE()
B_SPLINE_SURFACE(1,2,((#134964,#134965,#134966,#134967,#134968),(#134969,
#134970,#134971,#134972,#134973)),.UNSPECIFIED.,.F.,.F.,.F.)
B_SPLINE_SURFACE_WITH_KNOTS((2,2),(3,2,3),(0.710192959007031,1.),(0.504546746573288,
0.504719756176206,0.522020716468041),.UNSPECIFIED.)
GEOMETRIC_REPRESENTATION_ITEM()
RATIONAL_B_SPLINE_SURFACE(((0.996905579294158,0.996905579294158,0.996905579294158,
0.991635321911186,0.989306890555884),(0.996905579294158,0.996905579294158,
0.996905579294158,0.991635321911186,0.989306890555884)))
REPRESENTATION_ITEM('')
SURFACE()
);
#2415=(
BOUNDED_SURFACE()
B_SPLINE_SURFACE(1,2,((#134986,#134987,#134988,#134989,#134990,#134991,
#134992),(#134993,#134994,#134995,#134996,#134997,#134998,#134999)),
 .UNSPECIFIED.,.F.,.F.,.F.)
B_SPLINE_SURFACE_WITH_KNOTS((2,2),(3,2,2,3),(0.710318915640075,1.),(0.211398300093699,
0.214285714285714,0.228883374894809,0.22905822564282),.UNSPECIFIED.)
GEOMETRIC_REPRESENTATION_ITEM()
RATIONAL_B_SPLINE_SURFACE(((0.998054921708738,0.998986490969345,1.,0.994876086397764,
0.991846493044689,0.991846493044689,0.991846493044689),(0.998054921708738,
0.998986490969345,1.,0.994876086397764,0.991846493044689,0.991846493044689,
0.991846493044689)))
REPRESENTATION_ITEM('')
SURFACE()
);
#2416=(
BOUNDED_SURFACE()
B_SPLINE_SURFACE(1,2,((#135010,#135011,#135012,#135013,#135014),(#135015,
#135016,#135017,#135018,#135019)),.UNSPECIFIED.,.F.,.F.,.F.)
B_SPLINE_SURFACE_WITH_KNOTS((2,2),(3,2,3),(0.710192959007033,1.),(0.504546746573288,
0.504719756176206,0.522020716468041),.UNSPECIFIED.)
GEOMETRIC_REPRESENTATION_ITEM()
RATIONAL_B_SPLINE_SURFACE(((0.996905579294158,0.996905579294158,0.996905579294158,
0.991635321911186,0.989306890555884),(0.996905579294158,0.996905579294158,
0.996905579294158,0.991635321911186,0.989306890555884)))
REPRESENTATION_ITEM('')
SURFACE()
);
#2417=(
BOUNDED_SURFACE()
B_SPLINE_SURFACE(1,2,((#135032,#135033,#135034,#135035,#135036,#135037,
#135038),(#135039,#135040,#135041,#135042,#135043,#135044,#135045)),
 .UNSPECIFIED.,.F.,.F.,.F.)
B_SPLINE_SURFACE_WITH_KNOTS((2,2),(3,2,2,3),(0.710318915640075,1.),(0.211398300093695,
0.214285714285714,0.228883374894809,0.22905822564282),.UNSPECIFIED.)
GEOMETRIC_REPRESENTATION_ITEM()
RATIONAL_B_SPLINE_SURFACE(((0.998054921708735,0.998986490969344,1.,0.994876086397764,
0.991846493044689,0.991846493044689,0.991846493044689),(0.998054921708735,
0.998986490969344,1.,0.994876086397764,0.991846493044689,0.991846493044689,
0.991846493044689)))
REPRESENTATION_ITEM('')
SURFACE()
);
#2418=(
BOUNDED_SURFACE()
B_SPLINE_SURFACE(1,2,((#135056,#135057,#135058,#135059,#135060),(#135061,
#135062,#135063,#135064,#135065)),.UNSPECIFIED.,.F.,.F.,.F.)
B_SPLINE_SURFACE_WITH_KNOTS((2,2),(3,2,3),(0.71019295900703,1.),(0.504546746573288,
0.504719756176206,0.522020716468041),.UNSPECIFIED.)
GEOMETRIC_REPRESENTATION_ITEM()
RATIONAL_B_SPLINE_SURFACE(((0.996905579294158,0.996905579294158,0.996905579294158,
0.991635321911186,0.989306890555885),(0.996905579294158,0.996905579294158,
0.996905579294158,0.991635321911186,0.989306890555885)))
REPRESENTATION_ITEM('')
SURFACE()
);
#2419=(
BOUNDED_SURFACE()
B_SPLINE_SURFACE(1,2,((#135078,#135079,#135080,#135081,#135082,#135083,
#135084),(#135085,#135086,#135087,#135088,#135089,#135090,#135091)),
 .UNSPECIFIED.,.F.,.F.,.F.)
B_SPLINE_SURFACE_WITH_KNOTS((2,2),(3,2,2,3),(0.710318915640078,1.),(0.2113983000937,
0.214285714285714,0.228883374894809,0.22905822564282),.UNSPECIFIED.)
GEOMETRIC_REPRESENTATION_ITEM()
RATIONAL_B_SPLINE_SURFACE(((0.998054921708738,0.998986490969345,1.,0.994876086397764,
0.991846493044689,0.991846493044689,0.991846493044689),(0.998054921708738,
0.998986490969345,1.,0.994876086397764,0.991846493044689,0.991846493044689,
0.991846493044689)))
REPRESENTATION_ITEM('')
SURFACE()
);
#2420=(
BOUNDED_SURFACE()
B_SPLINE_SURFACE(1,2,((#135102,#135103,#135104,#135105,#135106),(#135107,
#135108,#135109,#135110,#135111)),.UNSPECIFIED.,.F.,.F.,.F.)
B_SPLINE_SURFACE_WITH_KNOTS((2,2),(3,2,3),(0.71019295900703,1.),(0.504546746573288,
0.504719756176206,0.522020716468041),.UNSPECIFIED.)
GEOMETRIC_REPRESENTATION_ITEM()
RATIONAL_B_SPLINE_SURFACE(((0.996905579294158,0.996905579294158,0.996905579294158,
0.991635321911186,0.989306890555884),(0.996905579294158,0.996905579294158,
0.996905579294158,0.991635321911186,0.989306890555884)))
REPRESENTATION_ITEM('')
SURFACE()
);
#2421=(
BOUNDED_SURFACE()
B_SPLINE_SURFACE(1,2,((#135124,#135125,#135126,#135127,#135128,#135129,
#135130),(#135131,#135132,#135133,#135134,#135135,#135136,#135137)),
 .UNSPECIFIED.,.F.,.F.,.F.)
B_SPLINE_SURFACE_WITH_KNOTS((2,2),(3,2,2,3),(0.710318915640077,1.),(0.2113983000937,
0.214285714285714,0.228883374894809,0.22905822564282),.UNSPECIFIED.)
GEOMETRIC_REPRESENTATION_ITEM()
RATIONAL_B_SPLINE_SURFACE(((0.998054921708738,0.998986490969345,1.,0.994876086397764,
0.991846493044689,0.991846493044689,0.991846493044689),(0.998054921708738,
0.998986490969345,1.,0.994876086397764,0.991846493044689,0.991846493044689,
0.991846493044689)))
REPRESENTATION_ITEM('')
SURFACE()
);
#2422=(
BOUNDED_SURFACE()
B_SPLINE_SURFACE(1,2,((#135148,#135149,#135150,#135151,#135152),(#135153,
#135154,#135155,#135156,#135157)),.UNSPECIFIED.,.F.,.F.,.F.)
B_SPLINE_SURFACE_WITH_KNOTS((2,2),(3,2,3),(0.710192959007036,1.),(0.504546746573288,
0.504719756176206,0.522020716468041),.UNSPECIFIED.)
GEOMETRIC_REPRESENTATION_ITEM()
RATIONAL_B_SPLINE_SURFACE(((0.996905579294158,0.996905579294158,0.996905579294158,
0.991635321911186,0.989306890555884),(0.996905579294158,0.996905579294158,
0.996905579294158,0.991635321911186,0.989306890555884)))
REPRESENTATION_ITEM('')
SURFACE()
);
#2423=(
BOUNDED_SURFACE()
B_SPLINE_SURFACE(1,2,((#135170,#135171,#135172,#135173,#135174,#135175,
#135176),(#135177,#135178,#135179,#135180,#135181,#135182,#135183)),
 .UNSPECIFIED.,.F.,.F.,.F.)
B_SPLINE_SURFACE_WITH_KNOTS((2,2),(3,2,2,3),(0.710318915640077,1.),(0.2113983000937,
0.214285714285714,0.228883374894809,0.22905822564282),.UNSPECIFIED.)
GEOMETRIC_REPRESENTATION_ITEM()
RATIONAL_B_SPLINE_SURFACE(((0.998054921708738,0.998986490969345,1.,0.994876086397764,
0.991846493044689,0.991846493044689,0.991846493044689),(0.998054921708738,
0.998986490969345,1.,0.994876086397764,0.991846493044689,0.991846493044689,
0.991846493044689)))
REPRESENTATION_ITEM('')
SURFACE()
);
#2424=(
BOUNDED_SURFACE()
B_SPLINE_SURFACE(1,2,((#135198,#135199,#135200,#135201,#135202),(#135203,
#135204,#135205,#135206,#135207)),.UNSPECIFIED.,.F.,.F.,.F.)
B_SPLINE_SURFACE_WITH_KNOTS((2,2),(3,2,3),(0.710192959007037,1.),(0.504546746573288,
0.504719756176206,0.522020716468041),.UNSPECIFIED.)
GEOMETRIC_REPRESENTATION_ITEM()
RATIONAL_B_SPLINE_SURFACE(((0.996905579294158,0.996905579294158,0.996905579294158,
0.991635321911186,0.989306890555884),(0.996905579294158,0.996905579294158,
0.996905579294158,0.991635321911186,0.989306890555884)))
REPRESENTATION_ITEM('')
SURFACE()
);
#2425=(
BOUNDED_SURFACE()
B_SPLINE_SURFACE(1,2,((#135220,#135221,#135222,#135223,#135224,#135225,
#135226),(#135227,#135228,#135229,#135230,#135231,#135232,#135233)),
 .UNSPECIFIED.,.F.,.F.,.F.)
B_SPLINE_SURFACE_WITH_KNOTS((2,2),(3,2,2,3),(0.710318915640079,1.),(0.2113983000937,
0.214285714285714,0.228883374894809,0.22905822564282),.UNSPECIFIED.)
GEOMETRIC_REPRESENTATION_ITEM()
RATIONAL_B_SPLINE_SURFACE(((0.998054921708738,0.998986490969345,1.,0.994876086397764,
0.991846493044689,0.991846493044689,0.991846493044689),(0.998054921708738,
0.998986490969345,1.,0.994876086397764,0.991846493044689,0.991846493044689,
0.991846493044689)))
REPRESENTATION_ITEM('')
SURFACE()
);
#2426=(
BOUNDED_SURFACE()
B_SPLINE_SURFACE(1,2,((#135248,#135249,#135250,#135251,#135252),(#135253,
#135254,#135255,#135256,#135257)),.UNSPECIFIED.,.F.,.F.,.F.)
B_SPLINE_SURFACE_WITH_KNOTS((2,2),(3,2,3),(0.71019295900703,1.),(0.504546746573288,
0.504719756176206,0.522020716468041),.UNSPECIFIED.)
GEOMETRIC_REPRESENTATION_ITEM()
RATIONAL_B_SPLINE_SURFACE(((0.996905579294158,0.996905579294158,0.996905579294158,
0.991635321911186,0.989306890555884),(0.996905579294158,0.996905579294158,
0.996905579294158,0.991635321911186,0.989306890555884)))
REPRESENTATION_ITEM('')
SURFACE()
);
#2427=(
BOUNDED_SURFACE()
B_SPLINE_SURFACE(1,2,((#135270,#135271,#135272,#135273,#135274,#135275,
#135276),(#135277,#135278,#135279,#135280,#135281,#135282,#135283)),
 .UNSPECIFIED.,.F.,.F.,.F.)
B_SPLINE_SURFACE_WITH_KNOTS((2,2),(3,2,2,3),(0.710318915640075,1.),(0.2113983000936,
0.214285714285714,0.228883374894809,0.229058225642821),.UNSPECIFIED.)
GEOMETRIC_REPRESENTATION_ITEM()
RATIONAL_B_SPLINE_SURFACE(((0.998054921708674,0.99898649096931,1.,0.994876086397764,
0.991846493044689,0.991846493044689,0.991846493044689),(0.998054921708674,
0.99898649096931,1.,0.994876086397764,0.991846493044689,0.991846493044689,
0.991846493044689)))
REPRESENTATION_ITEM('')
SURFACE()
);
#2428=(
BOUNDED_SURFACE()
B_SPLINE_SURFACE(1,2,((#135298,#135299,#135300,#135301,#135302),(#135303,
#135304,#135305,#135306,#135307)),.UNSPECIFIED.,.F.,.F.,.F.)
B_SPLINE_SURFACE_WITH_KNOTS((2,2),(3,2,3),(0.710192959007027,1.),(0.504546746573288,
0.504719756176206,0.522020716468041),.UNSPECIFIED.)
GEOMETRIC_REPRESENTATION_ITEM()
RATIONAL_B_SPLINE_SURFACE(((0.996905579294158,0.996905579294158,0.996905579294158,
0.991635321911186,0.989306890555884),(0.996905579294158,0.996905579294158,
0.996905579294158,0.991635321911186,0.989306890555884)))
REPRESENTATION_ITEM('')
SURFACE()
);
#2429=(
BOUNDED_SURFACE()
B_SPLINE_SURFACE(1,2,((#135320,#135321,#135322,#135323,#135324,#135325,
#135326),(#135327,#135328,#135329,#135330,#135331,#135332,#135333)),
 .UNSPECIFIED.,.F.,.F.,.F.)
B_SPLINE_SURFACE_WITH_KNOTS((2,2),(3,2,2,3),(0.710318915640073,1.),(0.2113983000937,
0.214285714285714,0.228883374894809,0.22905822564282),.UNSPECIFIED.)
GEOMETRIC_REPRESENTATION_ITEM()
RATIONAL_B_SPLINE_SURFACE(((0.998054921708738,0.998986490969345,1.,0.994876086397764,
0.991846493044689,0.991846493044689,0.991846493044689),(0.998054921708738,
0.998986490969345,1.,0.994876086397764,0.991846493044689,0.991846493044689,
0.991846493044689)))
REPRESENTATION_ITEM('')
SURFACE()
);
#2430=(
BOUNDED_SURFACE()
B_SPLINE_SURFACE(1,2,((#135344,#135345,#135346,#135347,#135348),(#135349,
#135350,#135351,#135352,#135353)),.UNSPECIFIED.,.F.,.F.,.F.)
B_SPLINE_SURFACE_WITH_KNOTS((2,2),(3,2,3),(0.710192959007035,1.),(0.504546746573288,
0.504719756176206,0.522020716468041),.UNSPECIFIED.)
GEOMETRIC_REPRESENTATION_ITEM()
RATIONAL_B_SPLINE_SURFACE(((0.996905579294158,0.996905579294158,0.996905579294158,
0.991635321911186,0.989306890555884),(0.996905579294158,0.996905579294158,
0.996905579294158,0.991635321911186,0.989306890555884)))
REPRESENTATION_ITEM('')
SURFACE()
);
#2431=(
BOUNDED_SURFACE()
B_SPLINE_SURFACE(1,2,((#135366,#135367,#135368,#135369,#135370,#135371,
#135372),(#135373,#135374,#135375,#135376,#135377,#135378,#135379)),
 .UNSPECIFIED.,.F.,.F.,.F.)
B_SPLINE_SURFACE_WITH_KNOTS((2,2),(3,2,2,3),(0.71031891564008,1.),(0.2113983000937,
0.214285714285714,0.228883374894809,0.22905822564282),.UNSPECIFIED.)
GEOMETRIC_REPRESENTATION_ITEM()
RATIONAL_B_SPLINE_SURFACE(((0.998054921708738,0.998986490969345,1.,0.994876086397764,
0.991846493044689,0.991846493044689,0.991846493044689),(0.998054921708738,
0.998986490969345,1.,0.994876086397764,0.991846493044689,0.991846493044689,
0.991846493044689)))
REPRESENTATION_ITEM('')
SURFACE()
);
#2432=(
BOUNDED_SURFACE()
B_SPLINE_SURFACE(1,2,((#135390,#135391,#135392,#135393,#135394),(#135395,
#135396,#135397,#135398,#135399)),.UNSPECIFIED.,.F.,.F.,.F.)
B_SPLINE_SURFACE_WITH_KNOTS((2,2),(3,2,3),(0.710192959007028,1.),(0.504546746573288,
0.504719756176206,0.522020716468041),.UNSPECIFIED.)
GEOMETRIC_REPRESENTATION_ITEM()
RATIONAL_B_SPLINE_SURFACE(((0.996905579294158,0.996905579294158,0.996905579294158,
0.991635321911186,0.989306890555884),(0.996905579294158,0.996905579294158,
0.996905579294158,0.991635321911186,0.989306890555884)))
REPRESENTATION_ITEM('')
SURFACE()
);
#2433=(
BOUNDED_SURFACE()
B_SPLINE_SURFACE(1,2,((#135412,#135413,#135414,#135415,#135416,#135417,
#135418),(#135419,#135420,#135421,#135422,#135423,#135424,#135425)),
 .UNSPECIFIED.,.F.,.F.,.F.)
B_SPLINE_SURFACE_WITH_KNOTS((2,2),(3,2,2,3),(0.710318915640078,1.),(0.2113983000937,
0.214285714285714,0.228883374894809,0.22905822564282),.UNSPECIFIED.)
GEOMETRIC_REPRESENTATION_ITEM()
RATIONAL_B_SPLINE_SURFACE(((0.998054921708738,0.998986490969345,1.,0.994876086397764,
0.991846493044689,0.991846493044689,0.991846493044689),(0.998054921708738,
0.998986490969345,1.,0.994876086397764,0.991846493044689,0.991846493044689,
0.991846493044689)))
REPRESENTATION_ITEM('')
SURFACE()
);
#2434=(
BOUNDED_SURFACE()
B_SPLINE_SURFACE(1,2,((#135436,#135437,#135438,#135439,#135440),(#135441,
#135442,#135443,#135444,#135445)),.UNSPECIFIED.,.F.,.F.,.F.)
B_SPLINE_SURFACE_WITH_KNOTS((2,2),(3,2,3),(0.710192959007034,1.),(0.504546746573288,
0.504719756176206,0.522020716468041),.UNSPECIFIED.)
GEOMETRIC_REPRESENTATION_ITEM()
RATIONAL_B_SPLINE_SURFACE(((0.996905579294158,0.996905579294158,0.996905579294158,
0.991635321911186,0.989306890555884),(0.996905579294158,0.996905579294158,
0.996905579294158,0.991635321911186,0.989306890555884)))
REPRESENTATION_ITEM('')
SURFACE()
);
#2435=(
BOUNDED_SURFACE()
B_SPLINE_SURFACE(1,2,((#135458,#135459,#135460,#135461,#135462,#135463,
#135464),(#135465,#135466,#135467,#135468,#135469,#135470,#135471)),
 .UNSPECIFIED.,.F.,.F.,.F.)
B_SPLINE_SURFACE_WITH_KNOTS((2,2),(3,2,2,3),(0.71031891564008,1.),(0.2113983000937,
0.214285714285714,0.228883374894809,0.22905822564282),.UNSPECIFIED.)
GEOMETRIC_REPRESENTATION_ITEM()
RATIONAL_B_SPLINE_SURFACE(((0.998054921708738,0.998986490969345,1.,0.994876086397764,
0.991846493044689,0.991846493044689,0.991846493044689),(0.998054921708738,
0.998986490969345,1.,0.994876086397764,0.991846493044689,0.991846493044689,
0.991846493044689)))
REPRESENTATION_ITEM('')
SURFACE()
);
#2436=(
BOUNDED_SURFACE()
B_SPLINE_SURFACE(1,2,((#135482,#135483,#135484,#135485,#135486),(#135487,
#135488,#135489,#135490,#135491)),.UNSPECIFIED.,.F.,.F.,.F.)
B_SPLINE_SURFACE_WITH_KNOTS((2,2),(3,2,3),(0.710192959007032,1.),(0.504546746573288,
0.504719756176206,0.522020716468041),.UNSPECIFIED.)
GEOMETRIC_REPRESENTATION_ITEM()
RATIONAL_B_SPLINE_SURFACE(((0.996905579294159,0.996905579294159,0.996905579294159,
0.991635321911186,0.989306890555885),(0.996905579294158,0.996905579294158,
0.996905579294158,0.991635321911186,0.989306890555885)))
REPRESENTATION_ITEM('')
SURFACE()
);
#2437=(
BOUNDED_SURFACE()
B_SPLINE_SURFACE(1,2,((#135504,#135505,#135506,#135507,#135508,#135509,
#135510),(#135511,#135512,#135513,#135514,#135515,#135516,#135517)),
 .UNSPECIFIED.,.F.,.F.,.F.)
B_SPLINE_SURFACE_WITH_KNOTS((2,2),(3,2,2,3),(0.710318915640082,1.),(0.2113983000937,
0.214285714285714,0.228883374894809,0.22905822564282),.UNSPECIFIED.)
GEOMETRIC_REPRESENTATION_ITEM()
RATIONAL_B_SPLINE_SURFACE(((0.998054921708738,0.998986490969345,1.,0.994876086397764,
0.991846493044689,0.991846493044689,0.991846493044689),(0.998054921708738,
0.998986490969345,1.,0.994876086397764,0.991846493044689,0.991846493044689,
0.991846493044689)))
REPRESENTATION_ITEM('')
SURFACE()
);
#2438=(
BOUNDED_SURFACE()
B_SPLINE_SURFACE(1,2,((#135528,#135529,#135530,#135531,#135532),(#135533,
#135534,#135535,#135536,#135537)),.UNSPECIFIED.,.F.,.F.,.F.)
B_SPLINE_SURFACE_WITH_KNOTS((2,2),(3,2,3),(0.710192959007032,1.),(0.504546746573288,
0.504719756176206,0.522020716468041),.UNSPECIFIED.)
GEOMETRIC_REPRESENTATION_ITEM()
RATIONAL_B_SPLINE_SURFACE(((0.996905579294159,0.996905579294159,0.996905579294159,
0.991635321911186,0.989306890555885),(0.996905579294158,0.996905579294158,
0.996905579294158,0.991635321911186,0.989306890555885)))
REPRESENTATION_ITEM('')
SURFACE()
);
#2439=(
BOUNDED_SURFACE()
B_SPLINE_SURFACE(1,2,((#135550,#135551,#135552,#135553,#135554,#135555,
#135556),(#135557,#135558,#135559,#135560,#135561,#135562,#135563)),
 .UNSPECIFIED.,.F.,.F.,.F.)
B_SPLINE_SURFACE_WITH_KNOTS((2,2),(3,2,2,3),(0.710318915639715,1.),(0.2113983000937,
0.214285714285714,0.228883374894809,0.22905822564282),.UNSPECIFIED.)
GEOMETRIC_REPRESENTATION_ITEM()
RATIONAL_B_SPLINE_SURFACE(((0.998054921708738,0.998986490969345,1.,0.994876086397764,
0.991846493044689,0.991846493044689,0.991846493044689),(0.998054921708738,
0.998986490969345,1.,0.994876086397764,0.991846493044689,0.991846493044689,
0.991846493044689)))
REPRESENTATION_ITEM('')
SURFACE()
);
#2440=(
BOUNDED_SURFACE()
B_SPLINE_SURFACE(1,2,((#135574,#135575,#135576,#135577,#135578),(#135579,
#135580,#135581,#135582,#135583)),.UNSPECIFIED.,.F.,.F.,.F.)
B_SPLINE_SURFACE_WITH_KNOTS((2,2),(3,2,3),(0.710192959006589,1.),(0.504546746573288,
0.504719756176206,0.522020716468041),.UNSPECIFIED.)
GEOMETRIC_REPRESENTATION_ITEM()
RATIONAL_B_SPLINE_SURFACE(((0.996905579294158,0.996905579294158,0.996905579294158,
0.991635321911186,0.989306890555884),(0.996905579294158,0.996905579294158,
0.996905579294158,0.991635321911186,0.989306890555884)))
REPRESENTATION_ITEM('')
SURFACE()
);
#2441=(
BOUNDED_SURFACE()
B_SPLINE_SURFACE(1,2,((#135596,#135597,#135598,#135599,#135600,#135601,
#135602),(#135603,#135604,#135605,#135606,#135607,#135608,#135609)),
 .UNSPECIFIED.,.F.,.F.,.F.)
B_SPLINE_SURFACE_WITH_KNOTS((2,2),(3,2,2,3),(0.710318915638234,1.),(0.211398300093588,
0.214285714285714,0.228883374913777,0.229058225661979),.UNSPECIFIED.)
GEOMETRIC_REPRESENTATION_ITEM()
RATIONAL_B_SPLINE_SURFACE(((0.998054921708666,0.998986490969306,1.,0.994876086391106,
0.991846493036816,0.991846493036816,0.991846493036816),(0.998054921708666,
0.998986490969306,1.,0.994876086391106,0.991846493036816,0.991846493036816,
0.991846493036816)))
REPRESENTATION_ITEM('')
SURFACE()
);
#2442=(
BOUNDED_SURFACE()
B_SPLINE_SURFACE(1,2,((#135620,#135621,#135622,#135623,#135624),(#135625,
#135626,#135627,#135628,#135629)),.UNSPECIFIED.,.F.,.F.,.F.)
B_SPLINE_SURFACE_WITH_KNOTS((2,2),(3,2,3),(0.710192959006379,1.),(0.504546746573287,
0.504719756176205,0.52202071646804),.UNSPECIFIED.)
GEOMETRIC_REPRESENTATION_ITEM()
RATIONAL_B_SPLINE_SURFACE(((0.996905579294159,0.996905579294159,0.996905579294159,
0.991635321911186,0.989306890555885),(0.996905579294159,0.996905579294159,
0.996905579294159,0.991635321911186,0.989306890555885)))
REPRESENTATION_ITEM('')
SURFACE()
);
#2443=(
BOUNDED_SURFACE()
B_SPLINE_SURFACE(1,2,((#135642,#135643,#135644,#135645,#135646,#135647,
#135648),(#135649,#135650,#135651,#135652,#135653,#135654,#135655)),
 .UNSPECIFIED.,.F.,.F.,.F.)
B_SPLINE_SURFACE_WITH_KNOTS((2,2),(3,2,2,3),(0.710318915639423,1.),(0.211398300093701,
0.214285714285714,0.228883374894811,0.229058225642822),.UNSPECIFIED.)
GEOMETRIC_REPRESENTATION_ITEM()
RATIONAL_B_SPLINE_SURFACE(((0.998054921708739,0.998986490969345,1.,0.994876086397763,
0.991846493044688,0.991846493044688,0.991846493044688),(0.998054921708739,
0.998986490969345,1.,0.994876086397763,0.991846493044688,0.991846493044688,
0.991846493044688)))
REPRESENTATION_ITEM('')
SURFACE()
);
#2444=(
BOUNDED_SURFACE()
B_SPLINE_SURFACE(1,2,((#135666,#135667,#135668,#135669,#135670),(#135671,
#135672,#135673,#135674,#135675)),.UNSPECIFIED.,.F.,.F.,.F.)
B_SPLINE_SURFACE_WITH_KNOTS((2,2),(3,2,3),(0.710192959006944,1.),(0.504546746573287,
0.504719756176205,0.52202071646804),.UNSPECIFIED.)
GEOMETRIC_REPRESENTATION_ITEM()
RATIONAL_B_SPLINE_SURFACE(((0.996905579294159,0.996905579294159,0.996905579294159,
0.991635321911186,0.989306890555885),(0.996905579294159,0.996905579294159,
0.996905579294159,0.991635321911186,0.989306890555885)))
REPRESENTATION_ITEM('')
SURFACE()
);
#2445=(
BOUNDED_SURFACE()
B_SPLINE_SURFACE(1,2,((#135688,#135689,#135690,#135691,#135692,#135693,
#135694),(#135695,#135696,#135697,#135698,#135699,#135700,#135701)),
 .UNSPECIFIED.,.F.,.F.,.F.)
B_SPLINE_SURFACE_WITH_KNOTS((2,2),(3,2,2,3),(0.710318915639994,1.),(0.211398300093701,
0.214285714285714,0.22888337489481,0.229058225642821),.UNSPECIFIED.)
GEOMETRIC_REPRESENTATION_ITEM()
RATIONAL_B_SPLINE_SURFACE(((0.998054921708739,0.998986490969345,1.,0.994876086397763,
0.991846493044689,0.991846493044689,0.991846493044689),(0.998054921708739,
0.998986490969345,1.,0.994876086397763,0.991846493044689,0.991846493044689,
0.991846493044689)))
REPRESENTATION_ITEM('')
SURFACE()
);
#2446=(
BOUNDED_SURFACE()
B_SPLINE_SURFACE(1,2,((#135712,#135713,#135714,#135715,#135716),(#135717,
#135718,#135719,#135720,#135721)),.UNSPECIFIED.,.F.,.F.,.F.)
B_SPLINE_SURFACE_WITH_KNOTS((2,2),(3,2,3),(0.710192959006949,1.),(0.504546746573287,
0.504719756176205,0.52202071646804),.UNSPECIFIED.)
GEOMETRIC_REPRESENTATION_ITEM()
RATIONAL_B_SPLINE_SURFACE(((0.996905579294159,0.996905579294159,0.996905579294159,
0.991635321911186,0.989306890555885),(0.996905579294159,0.996905579294159,
0.996905579294159,0.991635321911186,0.989306890555885)))
REPRESENTATION_ITEM('')
SURFACE()
);
#2447=(
BOUNDED_SURFACE()
B_SPLINE_SURFACE(1,2,((#135734,#135735,#135736,#135737,#135738,#135739,
#135740),(#135741,#135742,#135743,#135744,#135745,#135746,#135747)),
 .UNSPECIFIED.,.F.,.F.,.F.)
B_SPLINE_SURFACE_WITH_KNOTS((2,2),(3,2,2,3),(0.710318915640003,1.),(0.211398300093701,
0.214285714285714,0.228883374894811,0.229058225642822),.UNSPECIFIED.)
GEOMETRIC_REPRESENTATION_ITEM()
RATIONAL_B_SPLINE_SURFACE(((0.998054921708739,0.998986490969345,1.,0.994876086397763,
0.991846493044688,0.991846493044688,0.991846493044688),(0.998054921708739,
0.998986490969345,1.,0.994876086397763,0.991846493044688,0.991846493044688,
0.991846493044688)))
REPRESENTATION_ITEM('')
SURFACE()
);
#2448=(
BOUNDED_SURFACE()
B_SPLINE_SURFACE(1,2,((#135758,#135759,#135760,#135761,#135762),(#135763,
#135764,#135765,#135766,#135767)),.UNSPECIFIED.,.F.,.F.,.F.)
B_SPLINE_SURFACE_WITH_KNOTS((2,2),(3,2,3),(0.710192959006957,1.),(0.504546746573287,
0.504719756176205,0.52202071646804),.UNSPECIFIED.)
GEOMETRIC_REPRESENTATION_ITEM()
RATIONAL_B_SPLINE_SURFACE(((0.996905579294159,0.996905579294159,0.996905579294159,
0.991635321911186,0.989306890555885),(0.996905579294159,0.996905579294159,
0.996905579294159,0.991635321911186,0.989306890555885)))
REPRESENTATION_ITEM('')
SURFACE()
);
#2449=(
BOUNDED_SURFACE()
B_SPLINE_SURFACE(1,2,((#135780,#135781,#135782,#135783,#135784,#135785,
#135786),(#135787,#135788,#135789,#135790,#135791,#135792,#135793)),
 .UNSPECIFIED.,.F.,.F.,.F.)
B_SPLINE_SURFACE_WITH_KNOTS((2,2),(3,2,2,3),(0.710318915640001,1.),(0.211398300093701,
0.214285714285714,0.22888337489481,0.229058225642821),.UNSPECIFIED.)
GEOMETRIC_REPRESENTATION_ITEM()
RATIONAL_B_SPLINE_SURFACE(((0.998054921708739,0.998986490969345,1.,0.994876086397763,
0.991846493044689,0.991846493044689,0.991846493044689),(0.998054921708739,
0.998986490969345,1.,0.994876086397763,0.991846493044689,0.991846493044689,
0.991846493044689)))
REPRESENTATION_ITEM('')
SURFACE()
);
#2450=(
BOUNDED_SURFACE()
B_SPLINE_SURFACE(1,2,((#135804,#135805,#135806,#135807,#135808),(#135809,
#135810,#135811,#135812,#135813)),.UNSPECIFIED.,.F.,.F.,.F.)
B_SPLINE_SURFACE_WITH_KNOTS((2,2),(3,2,3),(0.710192959006349,1.),(0.504546746573239,
0.504719756176158,0.52202071646804),.UNSPECIFIED.)
GEOMETRIC_REPRESENTATION_ITEM()
RATIONAL_B_SPLINE_SURFACE(((0.996905579294188,0.996905579294188,0.996905579294188,
0.991635321911192,0.989306890555885),(0.996905579294188,0.996905579294188,
0.996905579294188,0.991635321911192,0.989306890555885)))
REPRESENTATION_ITEM('')
SURFACE()
);
#2451=(
BOUNDED_SURFACE()
B_SPLINE_SURFACE(1,2,((#135826,#135827,#135828,#135829,#135830,#135831,
#135832),(#135833,#135834,#135835,#135836,#135837,#135838,#135839)),
 .UNSPECIFIED.,.F.,.F.,.F.)
B_SPLINE_SURFACE_WITH_KNOTS((2,2),(3,2,2,3),(0.710318915639035,1.),(0.211398300093701,
0.214285714285714,0.22888337489481,0.229058225642821),.UNSPECIFIED.)
GEOMETRIC_REPRESENTATION_ITEM()
RATIONAL_B_SPLINE_SURFACE(((0.998054921708739,0.998986490969345,1.,0.994876086397763,
0.991846493044688,0.991846493044688,0.991846493044688),(0.998054921708739,
0.998986490969345,1.,0.994876086397763,0.991846493044688,0.991846493044688,
0.991846493044688)))
REPRESENTATION_ITEM('')
SURFACE()
);
#2452=(
BOUNDED_SURFACE()
B_SPLINE_SURFACE(1,2,((#135850,#135851,#135852,#135853,#135854),(#135855,
#135856,#135857,#135858,#135859)),.UNSPECIFIED.,.F.,.F.,.F.)
B_SPLINE_SURFACE_WITH_KNOTS((2,2),(3,2,3),(0.710192959006982,1.),(0.504546746573089,
0.504719756176009,0.522020716468041),.UNSPECIFIED.)
GEOMETRIC_REPRESENTATION_ITEM()
RATIONAL_B_SPLINE_SURFACE(((0.996905579294279,0.996905579294279,0.996905579294279,
0.991635321911212,0.989306890555884),(0.996905579294279,0.996905579294279,
0.996905579294279,0.991635321911212,0.989306890555884)))
REPRESENTATION_ITEM('')
SURFACE()
);
#2453=(
BOUNDED_SURFACE()
B_SPLINE_SURFACE(1,2,((#135872,#135873,#135874,#135875,#135876,#135877,
#135878),(#135879,#135880,#135881,#135882,#135883,#135884,#135885)),
 .UNSPECIFIED.,.F.,.F.,.F.)
B_SPLINE_SURFACE_WITH_KNOTS((2,2),(3,2,2,3),(0.710318915640038,1.),(0.211398300093701,
0.214285714285714,0.22888337489481,0.229058225642821),.UNSPECIFIED.)
GEOMETRIC_REPRESENTATION_ITEM()
RATIONAL_B_SPLINE_SURFACE(((0.998054921708739,0.998986490969345,1.,0.994876086397764,
0.991846493044689,0.991846493044689,0.991846493044689),(0.998054921708739,
0.998986490969345,1.,0.994876086397764,0.991846493044689,0.991846493044689,
0.991846493044689)))
REPRESENTATION_ITEM('')
SURFACE()
);
#2454=(
BOUNDED_SURFACE()
B_SPLINE_SURFACE(1,2,((#135896,#135897,#135898,#135899,#135900),(#135901,
#135902,#135903,#135904,#135905)),.UNSPECIFIED.,.F.,.F.,.F.)
B_SPLINE_SURFACE_WITH_KNOTS((2,2),(3,2,3),(0.710192959006966,1.),(0.504546746572885,
0.504719756175807,0.522020716468042),.UNSPECIFIED.)
GEOMETRIC_REPRESENTATION_ITEM()
RATIONAL_B_SPLINE_SURFACE(((0.996905579294401,0.996905579294401,0.996905579294401,
0.991635321911239,0.989306890555884),(0.996905579294401,0.996905579294401,
0.996905579294401,0.991635321911239,0.989306890555884)))
REPRESENTATION_ITEM('')
SURFACE()
);
#2455=(
BOUNDED_SURFACE()
B_SPLINE_SURFACE(1,2,((#135918,#135919,#135920,#135921,#135922,#135923,
#135924),(#135925,#135926,#135927,#135928,#135929,#135930,#135931)),
 .UNSPECIFIED.,.F.,.F.,.F.)
B_SPLINE_SURFACE_WITH_KNOTS((2,2),(3,2,2,3),(0.710318915640017,1.),(0.211398300093701,
0.214285714285714,0.22888337489481,0.229058225642821),.UNSPECIFIED.)
GEOMETRIC_REPRESENTATION_ITEM()
RATIONAL_B_SPLINE_SURFACE(((0.998054921708739,0.998986490969345,1.,0.994876086397764,
0.991846493044689,0.991846493044689,0.991846493044689),(0.998054921708739,
0.998986490969345,1.,0.994876086397764,0.991846493044689,0.991846493044689,
0.991846493044689)))
REPRESENTATION_ITEM('')
SURFACE()
);
#2456=(
BOUNDED_SURFACE()
B_SPLINE_SURFACE(1,2,((#135946,#135947,#135948,#135949,#135950),(#135951,
#135952,#135953,#135954,#135955)),.UNSPECIFIED.,.F.,.F.,.F.)
B_SPLINE_SURFACE_WITH_KNOTS((2,2),(3,2,3),(0.,0.290270016613605),(0.159799014184082,
0.176967058622922,0.177555991080089),.UNSPECIFIED.)
GEOMETRIC_REPRESENTATION_ITEM()
RATIONAL_B_SPLINE_SURFACE(((0.990927469170791,0.98775996257079,0.98748925405691,
0.98748925405691,0.98748925405691),(0.990927469170791,0.98775996257079,
0.98748925405691,0.98748925405691,0.98748925405691)))
REPRESENTATION_ITEM('')
SURFACE()
);
#2457=(
BOUNDED_SURFACE()
B_SPLINE_SURFACE(1,2,((#135968,#135969,#135970,#135971,#135972,#135973,
#135974),(#135975,#135976,#135977,#135978,#135979,#135980,#135981)),
 .UNSPECIFIED.,.F.,.F.,.F.)
B_SPLINE_SURFACE_WITH_KNOTS((2,2),(3,2,2,3),(0.,0.28980704099156),(0.556037361265318,
0.55621282302886,0.571428571428571,0.573758999383056),.UNSPECIFIED.)
GEOMETRIC_REPRESENTATION_ITEM()
RATIONAL_B_SPLINE_SURFACE(((0.991593692313265,0.991593692313265,0.991593692313265,
0.994659131878644,1.,0.999181998279397,0.998417372792936),(0.991593692313265,
0.991593692313265,0.991593692313265,0.994659131878644,1.,0.999181998279397,
0.998417372792936)))
REPRESENTATION_ITEM('')
SURFACE()
);
#2458=(
BOUNDED_SURFACE()
B_SPLINE_SURFACE(1,2,((#135996,#135997,#135998,#135999,#136000),(#136001,
#136002,#136003,#136004,#136005)),.UNSPECIFIED.,.F.,.F.,.F.)
B_SPLINE_SURFACE_WITH_KNOTS((2,2),(3,2,3),(0.,0.290270016636536),(0.159799014184195,
0.176967058622922,0.177555991102387),.UNSPECIFIED.)
GEOMETRIC_REPRESENTATION_ITEM()
RATIONAL_B_SPLINE_SURFACE(((0.990927469170749,0.987759962570789,0.987489254056911,
0.987489254056911,0.987489254056911),(0.990927469170749,0.987759962570789,
0.987489254056911,0.987489254056911,0.987489254056911)))
REPRESENTATION_ITEM('')
SURFACE()
);
#2459=(
BOUNDED_SURFACE()
B_SPLINE_SURFACE(1,2,((#136018,#136019,#136020,#136021,#136022,#136023,
#136024),(#136025,#136026,#136027,#136028,#136029,#136030,#136031)),
 .UNSPECIFIED.,.F.,.F.,.F.)
B_SPLINE_SURFACE_WITH_KNOTS((2,2),(3,2,2,3),(0.,0.289807040991559),(0.556037361265318,
0.55621282302886,0.571428571428571,0.573758999383056),.UNSPECIFIED.)
GEOMETRIC_REPRESENTATION_ITEM()
RATIONAL_B_SPLINE_SURFACE(((0.991593692313265,0.991593692313265,0.991593692313265,
0.994659131878644,1.,0.999181998279397,0.998417372792936),(0.991593692313265,
0.991593692313265,0.991593692313265,0.994659131878644,1.,0.999181998279397,
0.998417372792936)))
REPRESENTATION_ITEM('')
SURFACE()
);
#2460=(
BOUNDED_SURFACE()
B_SPLINE_SURFACE(1,2,((#136042,#136043,#136044,#136045,#136046),(#136047,
#136048,#136049,#136050,#136051)),.UNSPECIFIED.,.F.,.F.,.F.)
B_SPLINE_SURFACE_WITH_KNOTS((2,2),(3,2,3),(0.,0.290270016612959),(0.15979901418427,
0.176967058622922,0.177555991079012),.UNSPECIFIED.)
GEOMETRIC_REPRESENTATION_ITEM()
RATIONAL_B_SPLINE_SURFACE(((0.990927469170721,0.987759962570787,0.98748925405691,
0.98748925405691,0.98748925405691),(0.990927469170722,0.987759962570787,
0.98748925405691,0.98748925405691,0.98748925405691)))
REPRESENTATION_ITEM('')
SURFACE()
);
#2461=(
BOUNDED_SURFACE()
B_SPLINE_SURFACE(1,2,((#136064,#136065,#136066,#136067,#136068,#136069,
#136070),(#136071,#136072,#136073,#136074,#136075,#136076,#136077)),
 .UNSPECIFIED.,.F.,.F.,.F.)
B_SPLINE_SURFACE_WITH_KNOTS((2,2),(3,2,2,3),(0.,0.289807040992493),(0.556037361265318,
0.55621282302886,0.571428571428571,0.573758999383056),.UNSPECIFIED.)
GEOMETRIC_REPRESENTATION_ITEM()
RATIONAL_B_SPLINE_SURFACE(((0.991593692313265,0.991593692313265,0.991593692313265,
0.994659131878644,1.,0.999181998279397,0.998417372792936),(0.991593692313265,
0.991593692313265,0.991593692313265,0.994659131878644,1.,0.999181998279397,
0.998417372792936)))
REPRESENTATION_ITEM('')
SURFACE()
);
#2462=(
BOUNDED_SURFACE()
B_SPLINE_SURFACE(1,2,((#136092,#136093,#136094,#136095,#136096),(#136097,
#136098,#136099,#136100,#136101)),.UNSPECIFIED.,.F.,.F.,.F.)
B_SPLINE_SURFACE_WITH_KNOTS((2,2),(3,2,3),(0.,0.290270016625899),(0.159799014184081,
0.176967058622922,0.177555991091513),.UNSPECIFIED.)
GEOMETRIC_REPRESENTATION_ITEM()
RATIONAL_B_SPLINE_SURFACE(((0.990927469170791,0.98775996257079,0.98748925405691,
0.98748925405691,0.98748925405691),(0.990927469170791,0.98775996257079,
0.98748925405691,0.98748925405691,0.98748925405691)))
REPRESENTATION_ITEM('')
SURFACE()
);
#2463=(
BOUNDED_SURFACE()
B_SPLINE_SURFACE(1,2,((#136117,#136118,#136119,#136120,#136121,#136122,
#136123),(#136124,#136125,#136126,#136127,#136128,#136129,#136130)),
 .UNSPECIFIED.,.F.,.F.,.F.)
B_SPLINE_SURFACE_WITH_KNOTS((2,2),(3,2,2,3),(0.,0.289807040992489),(0.556037361265319,
0.55621282302886,0.571428571428571,0.573758999382975),.UNSPECIFIED.)
GEOMETRIC_REPRESENTATION_ITEM()
RATIONAL_B_SPLINE_SURFACE(((0.991593692313265,0.991593692313265,0.991593692313265,
0.994659131878644,1.,0.999181998279426,0.99841737279299),(0.991593692313265,
0.991593692313265,0.991593692313265,0.994659131878644,1.,0.999181998279426,
0.99841737279299)))
REPRESENTATION_ITEM('')
SURFACE()
);
#2464=(
BOUNDED_SURFACE()
B_SPLINE_SURFACE(1,2,((#136141,#136142,#136143,#136144,#136145),(#136146,
#136147,#136148,#136149,#136150)),.UNSPECIFIED.,.F.,.F.,.F.)
B_SPLINE_SURFACE_WITH_KNOTS((2,2),(3,2,3),(0.,0.290270016605119),(0.159799014184081,
0.176967058622922,0.177555991071273),.UNSPECIFIED.)
GEOMETRIC_REPRESENTATION_ITEM()
RATIONAL_B_SPLINE_SURFACE(((0.990927469170791,0.98775996257079,0.98748925405691,
0.98748925405691,0.98748925405691),(0.990927469170791,0.98775996257079,
0.98748925405691,0.98748925405691,0.98748925405691)))
REPRESENTATION_ITEM('')
SURFACE()
);
#2465=(
BOUNDED_SURFACE()
B_SPLINE_SURFACE(1,2,((#136163,#136164,#136165,#136166,#136167,#136168,
#136169),(#136170,#136171,#136172,#136173,#136174,#136175,#136176)),
 .UNSPECIFIED.,.F.,.F.,.F.)
B_SPLINE_SURFACE_WITH_KNOTS((2,2),(3,2,2,3),(0.,0.289807040992493),(0.556037361265319,
0.55621282302886,0.571428571428571,0.573758999382975),.UNSPECIFIED.)
GEOMETRIC_REPRESENTATION_ITEM()
RATIONAL_B_SPLINE_SURFACE(((0.991593692313265,0.991593692313265,0.991593692313265,
0.994659131878644,1.,0.999181998279426,0.99841737279299),(0.991593692313265,
0.991593692313265,0.991593692313265,0.994659131878644,1.,0.999181998279426,
0.99841737279299)))
REPRESENTATION_ITEM('')
SURFACE()
);
#2466=(
BOUNDED_SURFACE()
B_SPLINE_SURFACE(1,2,((#136191,#136192,#136193,#136194,#136195),(#136196,
#136197,#136198,#136199,#136200)),.UNSPECIFIED.,.F.,.F.,.F.)
B_SPLINE_SURFACE_WITH_KNOTS((2,2),(3,2,3),(0.,0.290270016611538),(0.15979901418427,
0.176967058622922,0.177555991077158),.UNSPECIFIED.)
GEOMETRIC_REPRESENTATION_ITEM()
RATIONAL_B_SPLINE_SURFACE(((0.990927469170722,0.987759962570787,0.98748925405691,
0.98748925405691,0.98748925405691),(0.990927469170722,0.987759962570787,
0.98748925405691,0.98748925405691,0.98748925405691)))
REPRESENTATION_ITEM('')
SURFACE()
);
#2467=(
BOUNDED_SURFACE()
B_SPLINE_SURFACE(1,2,((#136213,#136214,#136215,#136216,#136217,#136218,
#136219),(#136220,#136221,#136222,#136223,#136224,#136225,#136226)),
 .UNSPECIFIED.,.F.,.F.,.F.)
B_SPLINE_SURFACE_WITH_KNOTS((2,2),(3,2,2,3),(0.,0.289807040993075),(0.556037361265318,
0.55621282302886,0.571428571428571,0.573758999383056),.UNSPECIFIED.)
GEOMETRIC_REPRESENTATION_ITEM()
RATIONAL_B_SPLINE_SURFACE(((0.991593692313265,0.991593692313265,0.991593692313265,
0.994659131878644,1.,0.999181998279397,0.998417372792936),(0.991593692313265,
0.991593692313265,0.991593692313265,0.994659131878644,1.,0.999181998279397,
0.998417372792936)))
REPRESENTATION_ITEM('')
SURFACE()
);
#2468=(
BOUNDED_SURFACE()
B_SPLINE_SURFACE(1,2,((#136237,#136238,#136239,#136240,#136241),(#136242,
#136243,#136244,#136245,#136246)),.UNSPECIFIED.,.F.,.F.,.F.)
B_SPLINE_SURFACE_WITH_KNOTS((2,2),(3,2,3),(0.,0.29027001661619),(0.159799014184193,
0.176967058622922,0.177555991082371),.UNSPECIFIED.)
GEOMETRIC_REPRESENTATION_ITEM()
RATIONAL_B_SPLINE_SURFACE(((0.99092746917075,0.987759962570788,0.98748925405691,
0.98748925405691,0.98748925405691),(0.99092746917075,0.987759962570788,
0.98748925405691,0.98748925405691,0.98748925405691)))
REPRESENTATION_ITEM('')
SURFACE()
);
#2469=(
BOUNDED_SURFACE()
B_SPLINE_SURFACE(1,2,((#136259,#136260,#136261,#136262,#136263,#136264,
#136265),(#136266,#136267,#136268,#136269,#136270,#136271,#136272)),
 .UNSPECIFIED.,.F.,.F.,.F.)
B_SPLINE_SURFACE_WITH_KNOTS((2,2),(3,2,2,3),(0.,0.289807040992488),(0.556037361265318,
0.55621282302886,0.571428571428571,0.573758999383057),.UNSPECIFIED.)
GEOMETRIC_REPRESENTATION_ITEM()
RATIONAL_B_SPLINE_SURFACE(((0.991593692313265,0.991593692313265,0.991593692313265,
0.994659131878644,1.,0.999181998279397,0.998417372792936),(0.991593692313265,
0.991593692313265,0.991593692313265,0.994659131878644,1.,0.999181998279397,
0.998417372792936)))
REPRESENTATION_ITEM('')
SURFACE()
);
#2470=(
BOUNDED_SURFACE()
B_SPLINE_SURFACE(1,2,((#136287,#136288,#136289,#136290,#136291),(#136292,
#136293,#136294,#136295,#136296)),.UNSPECIFIED.,.F.,.F.,.F.)
B_SPLINE_SURFACE_WITH_KNOTS((2,2),(3,2,3),(0.,0.290270016643447),(0.159799014184081,
0.176967058622922,0.177555991109407),.UNSPECIFIED.)
GEOMETRIC_REPRESENTATION_ITEM()
RATIONAL_B_SPLINE_SURFACE(((0.990927469170791,0.98775996257079,0.98748925405691,
0.98748925405691,0.98748925405691),(0.990927469170791,0.98775996257079,
0.98748925405691,0.98748925405691,0.98748925405691)))
REPRESENTATION_ITEM('')
SURFACE()
);
#2471=(
BOUNDED_SURFACE()
B_SPLINE_SURFACE(1,2,((#136309,#136310,#136311,#136312,#136313,#136314,
#136315),(#136316,#136317,#136318,#136319,#136320,#136321,#136322)),
 .UNSPECIFIED.,.F.,.F.,.F.)
B_SPLINE_SURFACE_WITH_KNOTS((2,2),(3,2,2,3),(0.,0.289807040993064),(0.556037361265318,
0.55621282302886,0.571428571428571,0.573758999383056),.UNSPECIFIED.)
GEOMETRIC_REPRESENTATION_ITEM()
RATIONAL_B_SPLINE_SURFACE(((0.991593692313265,0.991593692313265,0.991593692313265,
0.994659131878644,1.,0.999181998279397,0.998417372792936),(0.991593692313265,
0.991593692313265,0.991593692313265,0.994659131878644,1.,0.999181998279397,
0.998417372792936)))
REPRESENTATION_ITEM('')
SURFACE()
);
#2472=(
BOUNDED_SURFACE()
B_SPLINE_SURFACE(1,2,((#136333,#136334,#136335,#136336,#136337),(#136338,
#136339,#136340,#136341,#136342)),.UNSPECIFIED.,.F.,.F.,.F.)
B_SPLINE_SURFACE_WITH_KNOTS((2,2),(3,2,3),(0.,0.290270016648069),(0.159799014184083,
0.176967058622922,0.177555991114313),.UNSPECIFIED.)
GEOMETRIC_REPRESENTATION_ITEM()
RATIONAL_B_SPLINE_SURFACE(((0.99092746917079,0.98775996257079,0.98748925405691,
0.98748925405691,0.98748925405691),(0.99092746917079,0.98775996257079,0.98748925405691,
0.98748925405691,0.98748925405691)))
REPRESENTATION_ITEM('')
SURFACE()
);
#2473=(
BOUNDED_SURFACE()
B_SPLINE_SURFACE(1,2,((#136355,#136356,#136357,#136358,#136359,#136360,
#136361),(#136362,#136363,#136364,#136365,#136366,#136367,#136368)),
 .UNSPECIFIED.,.F.,.F.,.F.)
B_SPLINE_SURFACE_WITH_KNOTS((2,2),(3,2,2,3),(0.,0.289807040992575),(0.556037361265319,
0.556212823028861,0.571428571428571,0.573758999383056),.UNSPECIFIED.)
GEOMETRIC_REPRESENTATION_ITEM()
RATIONAL_B_SPLINE_SURFACE(((0.991593692313265,0.991593692313265,0.991593692313265,
0.994659131878645,1.,0.999181998279397,0.998417372792936),(0.991593692313265,
0.991593692313265,0.991593692313265,0.994659131878645,1.,0.999181998279397,
0.998417372792936)))
REPRESENTATION_ITEM('')
SURFACE()
);
#2474=(
BOUNDED_SURFACE()
B_SPLINE_SURFACE(1,2,((#136379,#136380,#136381,#136382,#136383),(#136384,
#136385,#136386,#136387,#136388)),.UNSPECIFIED.,.F.,.F.,.F.)
B_SPLINE_SURFACE_WITH_KNOTS((2,2),(3,2,3),(0.,0.290270016630719),(0.159799014184082,
0.176967058622921,0.177555991097006),.UNSPECIFIED.)
GEOMETRIC_REPRESENTATION_ITEM()
RATIONAL_B_SPLINE_SURFACE(((0.990927469170791,0.98775996257079,0.98748925405691,
0.98748925405691,0.98748925405691),(0.990927469170791,0.98775996257079,
0.98748925405691,0.98748925405691,0.98748925405691)))
REPRESENTATION_ITEM('')
SURFACE()
);
#2475=(
BOUNDED_SURFACE()
B_SPLINE_SURFACE(1,2,((#136401,#136402,#136403,#136404,#136405,#136406,
#136407),(#136408,#136409,#136410,#136411,#136412,#136413,#136414)),
 .UNSPECIFIED.,.F.,.F.,.F.)
B_SPLINE_SURFACE_WITH_KNOTS((2,2),(3,2,2,3),(0.,0.28980704099257),(0.55603736126532,
0.556212823028861,0.571428571428571,0.573758999382978),.UNSPECIFIED.)
GEOMETRIC_REPRESENTATION_ITEM()
RATIONAL_B_SPLINE_SURFACE(((0.991593692313265,0.991593692313265,0.991593692313265,
0.994659131878645,1.,0.999181998279424,0.998417372792988),(0.991593692313266,
0.991593692313266,0.991593692313266,0.994659131878645,1.,0.999181998279424,
0.998417372792988)))
REPRESENTATION_ITEM('')
SURFACE()
);
#2476=(
BOUNDED_SURFACE()
B_SPLINE_SURFACE(1,2,((#136429,#136430,#136431,#136432,#136433),(#136434,
#136435,#136436,#136437,#136438)),.UNSPECIFIED.,.F.,.F.,.F.)
B_SPLINE_SURFACE_WITH_KNOTS((2,2),(3,2,3),(0.,0.290270016637826),(0.15979901418408,
0.176967058622921,0.17755599110352),.UNSPECIFIED.)
GEOMETRIC_REPRESENTATION_ITEM()
RATIONAL_B_SPLINE_SURFACE(((0.990927469170791,0.98775996257079,0.98748925405691,
0.98748925405691,0.98748925405691),(0.990927469170791,0.98775996257079,
0.98748925405691,0.98748925405691,0.98748925405691)))
REPRESENTATION_ITEM('')
SURFACE()
);
#2477=(
BOUNDED_SURFACE()
B_SPLINE_SURFACE(1,2,((#136451,#136452,#136453,#136454,#136455,#136456,
#136457),(#136458,#136459,#136460,#136461,#136462,#136463,#136464)),
 .UNSPECIFIED.,.F.,.F.,.F.)
B_SPLINE_SURFACE_WITH_KNOTS((2,2),(3,2,2,3),(0.,0.28980704099316),(0.556037361265319,
0.556212823028861,0.571428571428571,0.573758999383057),.UNSPECIFIED.)
GEOMETRIC_REPRESENTATION_ITEM()
RATIONAL_B_SPLINE_SURFACE(((0.991593692313265,0.991593692313265,0.991593692313265,
0.994659131878645,1.,0.999181998279397,0.998417372792936),(0.991593692313265,
0.991593692313265,0.991593692313265,0.994659131878645,1.,0.999181998279397,
0.998417372792936)))
REPRESENTATION_ITEM('')
SURFACE()
);
#2478=(
BOUNDED_SURFACE()
B_SPLINE_SURFACE(1,2,((#136470,#136471,#136472,#136473,#136474),(#136475,
#136476,#136477,#136478,#136479)),.UNSPECIFIED.,.F.,.F.,.F.)
B_SPLINE_SURFACE_WITH_KNOTS((2,2),(3,2,3),(0.,0.290270016637931),(0.15979901418408,
0.176967058622921,0.177555991104342),.UNSPECIFIED.)
GEOMETRIC_REPRESENTATION_ITEM()
RATIONAL_B_SPLINE_SURFACE(((0.990927469170792,0.98775996257079,0.98748925405691,
0.98748925405691,0.98748925405691),(0.990927469170792,0.98775996257079,
0.98748925405691,0.98748925405691,0.98748925405691)))
REPRESENTATION_ITEM('')
SURFACE()
);
#2479=(
BOUNDED_SURFACE()
B_SPLINE_SURFACE(1,2,((#136492,#136493,#136494,#136495,#136496,#136497,
#136498),(#136499,#136500,#136501,#136502,#136503,#136504,#136505)),
 .UNSPECIFIED.,.F.,.F.,.F.)
B_SPLINE_SURFACE_WITH_KNOTS((2,2),(3,2,2,3),(0.,0.289807040992571),(0.556037361265319,
0.556212823028861,0.571428571428571,0.573758999383057),.UNSPECIFIED.)
GEOMETRIC_REPRESENTATION_ITEM()
RATIONAL_B_SPLINE_SURFACE(((0.991593692313266,0.991593692313266,0.991593692313266,
0.994659131878645,1.,0.999181998279397,0.998417372792936),(0.991593692313266,
0.991593692313266,0.991593692313266,0.994659131878645,1.,0.999181998279397,
0.998417372792936)))
REPRESENTATION_ITEM('')
SURFACE()
);
#2480=(
BOUNDED_SURFACE()
B_SPLINE_SURFACE(1,2,((#136511,#136512,#136513,#136514,#136515),(#136516,
#136517,#136518,#136519,#136520)),.UNSPECIFIED.,.F.,.F.,.F.)
B_SPLINE_SURFACE_WITH_KNOTS((2,2),(3,2,3),(0.,0.290270016625139),(0.159799014184192,
0.176967058622921,0.177555991091401),.UNSPECIFIED.)
GEOMETRIC_REPRESENTATION_ITEM()
RATIONAL_B_SPLINE_SURFACE(((0.99092746917075,0.987759962570789,0.98748925405691,
0.98748925405691,0.98748925405691),(0.99092746917075,0.987759962570789,
0.98748925405691,0.98748925405691,0.98748925405691)))
REPRESENTATION_ITEM('')
SURFACE()
);
#2481=(
BOUNDED_SURFACE()
B_SPLINE_SURFACE(1,2,((#136533,#136534,#136535,#136536,#136537,#136538,
#136539),(#136540,#136541,#136542,#136543,#136544,#136545,#136546)),
 .UNSPECIFIED.,.F.,.F.,.F.)
B_SPLINE_SURFACE_WITH_KNOTS((2,2),(3,2,2,3),(0.,0.289807040993071),(0.556037361265319,
0.556212823028861,0.571428571428571,0.573758999383058),.UNSPECIFIED.)
GEOMETRIC_REPRESENTATION_ITEM()
RATIONAL_B_SPLINE_SURFACE(((0.991593692313265,0.991593692313265,0.991593692313265,
0.994659131878645,1.,0.999181998279397,0.998417372792936),(0.991593692313265,
0.991593692313265,0.991593692313265,0.994659131878645,1.,0.999181998279397,
0.998417372792936)))
REPRESENTATION_ITEM('')
SURFACE()
);
#2482=(
BOUNDED_SURFACE()
B_SPLINE_SURFACE(1,2,((#136557,#136558,#136559,#136560,#136561),(#136562,
#136563,#136564,#136565,#136566)),.UNSPECIFIED.,.F.,.F.,.F.)
B_SPLINE_SURFACE_WITH_KNOTS((2,2),(3,2,3),(0.,0.29027001664356),(0.15979901418408,
0.176967058622921,0.177555991109305),.UNSPECIFIED.)
GEOMETRIC_REPRESENTATION_ITEM()
RATIONAL_B_SPLINE_SURFACE(((0.990927469170792,0.98775996257079,0.98748925405691,
0.98748925405691,0.98748925405691),(0.990927469170792,0.98775996257079,
0.98748925405691,0.98748925405691,0.98748925405691)))
REPRESENTATION_ITEM('')
SURFACE()
);
#2483=(
BOUNDED_SURFACE()
B_SPLINE_SURFACE(1,2,((#136579,#136580,#136581,#136582,#136583,#136584,
#136585),(#136586,#136587,#136588,#136589,#136590,#136591,#136592)),
 .UNSPECIFIED.,.F.,.F.,.F.)
B_SPLINE_SURFACE_WITH_KNOTS((2,2),(3,2,2,3),(0.,0.289807040992579),(0.556037361265319,
0.556212823028861,0.571428571428571,0.573758999383058),.UNSPECIFIED.)
GEOMETRIC_REPRESENTATION_ITEM()
RATIONAL_B_SPLINE_SURFACE(((0.991593692313266,0.991593692313266,0.991593692313266,
0.994659131878645,1.,0.999181998279397,0.998417372792936),(0.991593692313266,
0.991593692313266,0.991593692313266,0.994659131878645,1.,0.999181998279397,
0.998417372792936)))
REPRESENTATION_ITEM('')
SURFACE()
);
#2484=(
BOUNDED_SURFACE()
B_SPLINE_SURFACE(1,2,((#136607,#136608,#136609,#136610,#136611),(#136612,
#136613,#136614,#136615,#136616)),.UNSPECIFIED.,.F.,.F.,.F.)
B_SPLINE_SURFACE_WITH_KNOTS((2,2),(3,2,3),(0.,0.290270016658068),(0.15979901418408,
0.176967058622921,0.177555991124176),.UNSPECIFIED.)
GEOMETRIC_REPRESENTATION_ITEM()
RATIONAL_B_SPLINE_SURFACE(((0.990927469170792,0.98775996257079,0.98748925405691,
0.98748925405691,0.98748925405691),(0.990927469170792,0.98775996257079,
0.98748925405691,0.98748925405691,0.98748925405691)))
REPRESENTATION_ITEM('')
SURFACE()
);
#2485=(
BOUNDED_SURFACE()
B_SPLINE_SURFACE(1,2,((#136629,#136630,#136631,#136632,#136633,#136634,
#136635),(#136636,#136637,#136638,#136639,#136640,#136641,#136642)),
 .UNSPECIFIED.,.F.,.F.,.F.)
B_SPLINE_SURFACE_WITH_KNOTS((2,2),(3,2,2,3),(0.,0.289807040993077),(0.55603736126532,
0.556212823028861,0.571428571428571,0.573758999382976),.UNSPECIFIED.)
GEOMETRIC_REPRESENTATION_ITEM()
RATIONAL_B_SPLINE_SURFACE(((0.991593692313265,0.991593692313265,0.991593692313265,
0.994659131878645,1.,0.999181998279425,0.998417372792989),(0.991593692313265,
0.991593692313265,0.991593692313265,0.994659131878645,1.,0.999181998279425,
0.998417372792989)))
REPRESENTATION_ITEM('')
SURFACE()
);
#2486=(
BOUNDED_SURFACE()
B_SPLINE_SURFACE(1,2,((#136653,#136654,#136655,#136656,#136657),(#136658,
#136659,#136660,#136661,#136662)),.UNSPECIFIED.,.F.,.F.,.F.)
B_SPLINE_SURFACE_WITH_KNOTS((2,2),(3,2,3),(0.,0.29027001664428),(0.159799014184081,
0.176967058622921,0.177555991110565),.UNSPECIFIED.)
GEOMETRIC_REPRESENTATION_ITEM()
RATIONAL_B_SPLINE_SURFACE(((0.990927469170791,0.98775996257079,0.98748925405691,
0.98748925405691,0.98748925405691),(0.990927469170791,0.98775996257079,
0.98748925405691,0.98748925405691,0.98748925405691)))
REPRESENTATION_ITEM('')
SURFACE()
);
#2487=(
BOUNDED_SURFACE()
B_SPLINE_SURFACE(1,2,((#136678,#136679,#136680,#136681,#136682,#136683,
#136684),(#136685,#136686,#136687,#136688,#136689,#136690,#136691)),
 .UNSPECIFIED.,.F.,.F.,.F.)
B_SPLINE_SURFACE_WITH_KNOTS((2,2),(3,2,2,3),(0.,0.289807040992854),(0.556037361265321,
0.556212823028862,0.571428571428571,0.573758999382978),.UNSPECIFIED.)
GEOMETRIC_REPRESENTATION_ITEM()
RATIONAL_B_SPLINE_SURFACE(((0.991593692313266,0.991593692313266,0.991593692313266,
0.994659131878645,1.,0.999181998279425,0.998417372792988),(0.991593692313266,
0.991593692313266,0.991593692313266,0.994659131878645,1.,0.999181998279425,
0.998417372792988)))
REPRESENTATION_ITEM('')
SURFACE()
);
#2488=(
BOUNDED_SURFACE()
B_SPLINE_SURFACE(1,2,((#136697,#136698,#136699,#136700,#136701),(#136702,
#136703,#136704,#136705,#136706)),.UNSPECIFIED.,.F.,.F.,.F.)
B_SPLINE_SURFACE_WITH_KNOTS((2,2),(3,2,3),(0.,0.290270016616668),(0.159799014184082,
0.176967058622921,0.177555991082798),.UNSPECIFIED.)
GEOMETRIC_REPRESENTATION_ITEM()
RATIONAL_B_SPLINE_SURFACE(((0.990927469170791,0.98775996257079,0.98748925405691,
0.98748925405691,0.98748925405691),(0.990927469170791,0.98775996257079,
0.98748925405691,0.98748925405691,0.98748925405691)))
REPRESENTATION_ITEM('')
SURFACE()
);
#2489=(
BOUNDED_SURFACE()
B_SPLINE_SURFACE(1,2,((#136719,#136720,#136721,#136722,#136723,#136724,
#136725),(#136726,#136727,#136728,#136729,#136730,#136731,#136732)),
 .UNSPECIFIED.,.F.,.F.,.F.)
B_SPLINE_SURFACE_WITH_KNOTS((2,2),(3,2,2,3),(0.,0.289807040993902),(0.55603736126532,
0.556212823028861,0.571428571428571,0.573758999382978),.UNSPECIFIED.)
GEOMETRIC_REPRESENTATION_ITEM()
RATIONAL_B_SPLINE_SURFACE(((0.991593692313265,0.991593692313265,0.991593692313265,
0.994659131878645,1.,0.999181998279424,0.998417372792988),(0.991593692313266,
0.991593692313266,0.991593692313266,0.994659131878645,1.,0.999181998279424,
0.998417372792988)))
REPRESENTATION_ITEM('')
SURFACE()
);
#2490=(
BOUNDED_SURFACE()
B_SPLINE_SURFACE(1,2,((#136747,#136748,#136749,#136750,#136751),(#136752,
#136753,#136754,#136755,#136756)),.UNSPECIFIED.,.F.,.F.,.F.)
B_SPLINE_SURFACE_WITH_KNOTS((2,2),(3,2,3),(0.,0.290270016636515),(0.15979901418409,
0.176967058622921,0.177555991102485),.UNSPECIFIED.)
GEOMETRIC_REPRESENTATION_ITEM()
RATIONAL_B_SPLINE_SURFACE(((0.990927469170788,0.98775996257079,0.98748925405691,
0.98748925405691,0.98748925405691),(0.990927469170788,0.98775996257079,
0.98748925405691,0.98748925405691,0.98748925405691)))
REPRESENTATION_ITEM('')
SURFACE()
);
#2491=(
BOUNDED_SURFACE()
B_SPLINE_SURFACE(1,2,((#136769,#136770,#136771,#136772,#136773,#136774,
#136775),(#136776,#136777,#136778,#136779,#136780,#136781,#136782)),
 .UNSPECIFIED.,.F.,.F.,.F.)
B_SPLINE_SURFACE_WITH_KNOTS((2,2),(3,2,2,3),(0.,0.289807040992609),(0.556037361265319,
0.556212823028861,0.571428571428571,0.573758999383058),.UNSPECIFIED.)
GEOMETRIC_REPRESENTATION_ITEM()
RATIONAL_B_SPLINE_SURFACE(((0.991593692313265,0.991593692313265,0.991593692313265,
0.994659131878645,1.,0.999181998279397,0.998417372792936),(0.991593692313265,
0.991593692313265,0.991593692313265,0.994659131878645,1.,0.999181998279397,
0.998417372792936)))
REPRESENTATION_ITEM('')
SURFACE()
);
#2492=(
BOUNDED_SURFACE()
B_SPLINE_SURFACE(1,2,((#136788,#136789,#136790,#136791,#136792),(#136793,
#136794,#136795,#136796,#136797)),.UNSPECIFIED.,.F.,.F.,.F.)
B_SPLINE_SURFACE_WITH_KNOTS((2,2),(3,2,3),(0.,0.290270016618184),(0.15979901418402,
0.176967058622921,0.17755599108467),.UNSPECIFIED.)
GEOMETRIC_REPRESENTATION_ITEM()
RATIONAL_B_SPLINE_SURFACE(((0.990927469170814,0.987759962570791,0.98748925405691,
0.98748925405691,0.98748925405691),(0.990927469170814,0.987759962570791,
0.98748925405691,0.98748925405691,0.98748925405691)))
REPRESENTATION_ITEM('')
SURFACE()
);
#2493=(
BOUNDED_SURFACE()
B_SPLINE_SURFACE(1,2,((#136810,#136811,#136812,#136813,#136814,#136815,
#136816),(#136817,#136818,#136819,#136820,#136821,#136822,#136823)),
 .UNSPECIFIED.,.F.,.F.,.F.)
B_SPLINE_SURFACE_WITH_KNOTS((2,2),(3,2,2,3),(0.,0.289807040992497),(0.55603736126532,
0.556212823028861,0.571428571428571,0.573758999382969),.UNSPECIFIED.)
GEOMETRIC_REPRESENTATION_ITEM()
RATIONAL_B_SPLINE_SURFACE(((0.991593692313265,0.991593692313265,0.991593692313265,
0.994659131878645,1.,0.999181998279428,0.998417372792994),(0.991593692313265,
0.991593692313265,0.991593692313265,0.994659131878645,1.,0.999181998279428,
0.998417372792994)))
REPRESENTATION_ITEM('')
SURFACE()
);
#2494=(
BOUNDED_SURFACE()
B_SPLINE_SURFACE(1,2,((#136838,#136839,#136840,#136841,#136842),(#136843,
#136844,#136845,#136846,#136847)),.UNSPECIFIED.,.F.,.F.,.F.)
B_SPLINE_SURFACE_WITH_KNOTS((2,2),(3,2,3),(0.,0.2902700166395),(0.159799014184269,
0.176967058622921,0.177555991105355),.UNSPECIFIED.)
GEOMETRIC_REPRESENTATION_ITEM()
RATIONAL_B_SPLINE_SURFACE(((0.990927469170722,0.987759962570788,0.98748925405691,
0.98748925405691,0.98748925405691),(0.990927469170722,0.987759962570787,
0.98748925405691,0.98748925405691,0.98748925405691)))
REPRESENTATION_ITEM('')
SURFACE()
);
#2495=(
BOUNDED_SURFACE()
B_SPLINE_SURFACE(1,2,((#136863,#136864,#136865,#136866,#136867,#136868,
#136869),(#136870,#136871,#136872,#136873,#136874,#136875,#136876)),
 .UNSPECIFIED.,.F.,.F.,.F.)
B_SPLINE_SURFACE_WITH_KNOTS((2,2),(3,2,2,3),(0.,0.289807040993133),(0.55603736126532,
0.556212823028862,0.571428571428571,0.573758999383058),.UNSPECIFIED.)
GEOMETRIC_REPRESENTATION_ITEM()
RATIONAL_B_SPLINE_SURFACE(((0.991593692313266,0.991593692313266,0.991593692313266,
0.994659131878645,1.,0.999181998279396,0.998417372792935),(0.991593692313266,
0.991593692313266,0.991593692313266,0.994659131878645,1.,0.999181998279396,
0.998417372792935)))
REPRESENTATION_ITEM('')
SURFACE()
);
#2496=(
BOUNDED_SURFACE()
B_SPLINE_SURFACE(1,2,((#136887,#136888,#136889,#136890,#136891),(#136892,
#136893,#136894,#136895,#136896)),.UNSPECIFIED.,.F.,.F.,.F.)
B_SPLINE_SURFACE_WITH_KNOTS((2,2),(3,2,3),(0.,0.290270016635147),(0.159799014184073,
0.176967058622922,0.177555991100849),.UNSPECIFIED.)
GEOMETRIC_REPRESENTATION_ITEM()
RATIONAL_B_SPLINE_SURFACE(((0.990927469170794,0.98775996257079,0.98748925405691,
0.98748925405691,0.98748925405691),(0.990927469170794,0.98775996257079,
0.98748925405691,0.98748925405691,0.98748925405691)))
REPRESENTATION_ITEM('')
SURFACE()
);
#2497=(
BOUNDED_SURFACE()
B_SPLINE_SURFACE(1,2,((#136912,#136913,#136914,#136915,#136916,#136917,
#136918),(#136919,#136920,#136921,#136922,#136923,#136924,#136925)),
 .UNSPECIFIED.,.F.,.F.,.F.)
B_SPLINE_SURFACE_WITH_KNOTS((2,2),(3,2,2,3),(0.,0.289807040991732),(0.55603736126532,
0.556212823028861,0.571428571428571,0.573758999382983),.UNSPECIFIED.)
GEOMETRIC_REPRESENTATION_ITEM()
RATIONAL_B_SPLINE_SURFACE(((0.991593692313265,0.991593692313265,0.991593692313265,
0.994659131878645,1.,0.999181998279423,0.998417372792985),(0.991593692313265,
0.991593692313265,0.991593692313265,0.994659131878645,1.,0.999181998279423,
0.998417372792985)))
REPRESENTATION_ITEM('')
SURFACE()
);
#2498=(
BOUNDED_SURFACE()
B_SPLINE_SURFACE(1,2,((#136936,#136937,#136938,#136939,#136940),(#136941,
#136942,#136943,#136944,#136945)),.UNSPECIFIED.,.F.,.F.,.F.)
B_SPLINE_SURFACE_WITH_KNOTS((2,2),(3,2,3),(0.,0.290270016625215),(0.159799014184268,
0.176967058622921,0.177555991091437),.UNSPECIFIED.)
GEOMETRIC_REPRESENTATION_ITEM()
RATIONAL_B_SPLINE_SURFACE(((0.990927469170722,0.987759962570787,0.98748925405691,
0.98748925405691,0.98748925405691),(0.990927469170722,0.987759962570787,
0.98748925405691,0.98748925405691,0.98748925405691)))
REPRESENTATION_ITEM('')
SURFACE()
);
#2499=(
BOUNDED_SURFACE()
B_SPLINE_SURFACE(1,2,((#136958,#136959,#136960,#136961,#136962,#136963,
#136964),(#136965,#136966,#136967,#136968,#136969,#136970,#136971)),
 .UNSPECIFIED.,.F.,.F.,.F.)
B_SPLINE_SURFACE_WITH_KNOTS((2,2),(3,2,2,3),(0.,0.289807040992884),(0.556037361265319,
0.556212823028861,0.571428571428571,0.573758999383057),.UNSPECIFIED.)
GEOMETRIC_REPRESENTATION_ITEM()
RATIONAL_B_SPLINE_SURFACE(((0.991593692313265,0.991593692313265,0.991593692313265,
0.994659131878645,1.,0.999181998279397,0.998417372792936),(0.991593692313266,
0.991593692313266,0.991593692313266,0.994659131878645,1.,0.999181998279397,
0.998417372792936)))
REPRESENTATION_ITEM('')
SURFACE()
);
#2500=(
BOUNDED_SURFACE()
B_SPLINE_SURFACE(1,2,((#136986,#136987,#136988,#136989,#136990),(#136991,
#136992,#136993,#136994,#136995)),.UNSPECIFIED.,.F.,.F.,.F.)
B_SPLINE_SURFACE_WITH_KNOTS((2,2),(3,2,3),(0.,0.290270016640829),(0.159799014184241,
0.176967058622921,0.17755599110692),.UNSPECIFIED.)
GEOMETRIC_REPRESENTATION_ITEM()
RATIONAL_B_SPLINE_SURFACE(((0.990927469170732,0.987759962570788,0.98748925405691,
0.98748925405691,0.98748925405691),(0.990927469170732,0.987759962570788,
0.98748925405691,0.98748925405691,0.98748925405691)))
REPRESENTATION_ITEM('')
SURFACE()
);
#2501=(
BOUNDED_SURFACE()
B_SPLINE_SURFACE(1,2,((#137008,#137009,#137010,#137011,#137012,#137013,
#137014),(#137015,#137016,#137017,#137018,#137019,#137020,#137021)),
 .UNSPECIFIED.,.F.,.F.,.F.)
B_SPLINE_SURFACE_WITH_KNOTS((2,2),(3,2,2,3),(0.,0.289807040992694),(0.556037361265319,
0.556212823028861,0.571428571428571,0.573758999383043),.UNSPECIFIED.)
GEOMETRIC_REPRESENTATION_ITEM()
RATIONAL_B_SPLINE_SURFACE(((0.991593692313266,0.991593692313266,0.991593692313266,
0.994659131878645,1.,0.999181998279402,0.998417372792945),(0.991593692313266,
0.991593692313266,0.991593692313266,0.994659131878645,1.,0.999181998279402,
0.998417372792945)))
REPRESENTATION_ITEM('')
SURFACE()
);
#2502=(
BOUNDED_SURFACE()
B_SPLINE_SURFACE(1,2,((#137036,#137037,#137038,#137039,#137040),(#137041,
#137042,#137043,#137044,#137045)),.UNSPECIFIED.,.F.,.F.,.F.)
B_SPLINE_SURFACE_WITH_KNOTS((2,2),(3,2,3),(0.,0.29027001662598),(0.159799014184254,
0.176967058622921,0.177555991092038),.UNSPECIFIED.)
GEOMETRIC_REPRESENTATION_ITEM()
RATIONAL_B_SPLINE_SURFACE(((0.990927469170727,0.987759962570788,0.98748925405691,
0.98748925405691,0.98748925405691),(0.990927469170727,0.987759962570788,
0.98748925405691,0.98748925405691,0.98748925405691)))
REPRESENTATION_ITEM('')
SURFACE()
);
#2503=(
BOUNDED_SURFACE()
B_SPLINE_SURFACE(1,2,((#137058,#137059,#137060,#137061,#137062,#137063,
#137064),(#137065,#137066,#137067,#137068,#137069,#137070,#137071)),
 .UNSPECIFIED.,.F.,.F.,.F.)
B_SPLINE_SURFACE_WITH_KNOTS((2,2),(3,2,2,3),(0.,0.289807040993741),(0.55603736126532,
0.556212823028862,0.571428571428571,0.573758999383057),.UNSPECIFIED.)
GEOMETRIC_REPRESENTATION_ITEM()
RATIONAL_B_SPLINE_SURFACE(((0.991593692313266,0.991593692313266,0.991593692313266,
0.994659131878645,1.,0.999181998279397,0.998417372792936),(0.991593692313266,
0.991593692313266,0.991593692313266,0.994659131878645,1.,0.999181998279397,
0.998417372792936)))
REPRESENTATION_ITEM('')
SURFACE()
);
#2504=(
BOUNDED_SURFACE()
B_SPLINE_SURFACE(1,2,((#137077,#137078,#137079,#137080,#137081),(#137082,
#137083,#137084,#137085,#137086)),.UNSPECIFIED.,.F.,.F.,.F.)
B_SPLINE_SURFACE_WITH_KNOTS((2,2),(3,2,3),(0.,0.290270016597558),(0.159799014184244,
0.176967058622922,0.177555991064019),.UNSPECIFIED.)
GEOMETRIC_REPRESENTATION_ITEM()
RATIONAL_B_SPLINE_SURFACE(((0.990927469170731,0.987759962570788,0.98748925405691,
0.98748925405691,0.98748925405691),(0.990927469170731,0.987759962570788,
0.98748925405691,0.98748925405691,0.98748925405691)))
REPRESENTATION_ITEM('')
SURFACE()
);
#2505=(
BOUNDED_SURFACE()
B_SPLINE_SURFACE(1,2,((#137099,#137100,#137101,#137102,#137103,#137104,
#137105),(#137106,#137107,#137108,#137109,#137110,#137111,#137112)),
 .UNSPECIFIED.,.F.,.F.,.F.)
B_SPLINE_SURFACE_WITH_KNOTS((2,2),(3,2,2,3),(0.,0.289807040991906),(0.556037361265319,
0.556212823028861,0.571428571428571,0.573758999383057),.UNSPECIFIED.)
GEOMETRIC_REPRESENTATION_ITEM()
RATIONAL_B_SPLINE_SURFACE(((0.991593692313266,0.991593692313266,0.991593692313266,
0.994659131878645,1.,0.999181998279397,0.998417372792936),(0.991593692313266,
0.991593692313266,0.991593692313266,0.994659131878645,1.,0.999181998279397,
0.998417372792936)))
REPRESENTATION_ITEM('')
SURFACE()
);
#2506=(
BOUNDED_SURFACE()
B_SPLINE_SURFACE(1,2,((#137118,#137119,#137120,#137121,#137122),(#137123,
#137124,#137125,#137126,#137127)),.UNSPECIFIED.,.F.,.F.,.F.)
B_SPLINE_SURFACE_WITH_KNOTS((2,2),(3,2,3),(0.,0.290270016589869),(0.159799014184269,
0.176967058622921,0.177555991056242),.UNSPECIFIED.)
GEOMETRIC_REPRESENTATION_ITEM()
RATIONAL_B_SPLINE_SURFACE(((0.990927469170722,0.987759962570787,0.98748925405691,
0.98748925405691,0.98748925405691),(0.990927469170722,0.987759962570787,
0.98748925405691,0.98748925405691,0.98748925405691)))
REPRESENTATION_ITEM('')
SURFACE()
);
#2507=(
BOUNDED_SURFACE()
B_SPLINE_SURFACE(1,2,((#137140,#137141,#137142,#137143,#137144,#137145,
#137146),(#137147,#137148,#137149,#137150,#137151,#137152,#137153)),
 .UNSPECIFIED.,.F.,.F.,.F.)
B_SPLINE_SURFACE_WITH_KNOTS((2,2),(3,2,2,3),(0.,0.289807040993049),(0.556037361265319,
0.556212823028861,0.571428571428571,0.573758999383058),.UNSPECIFIED.)
GEOMETRIC_REPRESENTATION_ITEM()
RATIONAL_B_SPLINE_SURFACE(((0.991593692313265,0.991593692313265,0.991593692313265,
0.994659131878645,1.,0.999181998279397,0.998417372792936),(0.991593692313265,
0.991593692313265,0.991593692313265,0.994659131878645,1.,0.999181998279397,
0.998417372792936)))
REPRESENTATION_ITEM('')
SURFACE()
);
#2508=(
BOUNDED_SURFACE()
B_SPLINE_SURFACE(1,2,((#137168,#137169,#137170,#137171,#137172),(#137173,
#137174,#137175,#137176,#137177)),.UNSPECIFIED.,.F.,.F.,.F.)
B_SPLINE_SURFACE_WITH_KNOTS((2,2),(3,2,3),(0.,0.290270016612988),(0.15979901418427,
0.176967058622921,0.17755599107958),.UNSPECIFIED.)
GEOMETRIC_REPRESENTATION_ITEM()
RATIONAL_B_SPLINE_SURFACE(((0.990927469170722,0.987759962570788,0.98748925405691,
0.98748925405691,0.98748925405691),(0.990927469170721,0.987759962570787,
0.98748925405691,0.98748925405691,0.98748925405691)))
REPRESENTATION_ITEM('')
SURFACE()
);
#2509=(
BOUNDED_SURFACE()
B_SPLINE_SURFACE(1,2,((#137190,#137191,#137192,#137193,#137194,#137195,
#137196),(#137197,#137198,#137199,#137200,#137201,#137202,#137203)),
 .UNSPECIFIED.,.F.,.F.,.F.)
B_SPLINE_SURFACE_WITH_KNOTS((2,2),(3,2,2,3),(0.,0.28980704099156),(0.556037361265318,
0.55621282302886,0.571428571428571,0.573758999383056),.UNSPECIFIED.)
GEOMETRIC_REPRESENTATION_ITEM()
RATIONAL_B_SPLINE_SURFACE(((0.991593692313265,0.991593692313265,0.991593692313265,
0.994659131878644,1.,0.999181998279397,0.998417372792936),(0.991593692313265,
0.991593692313265,0.991593692313265,0.994659131878644,1.,0.999181998279397,
0.998417372792936)))
REPRESENTATION_ITEM('')
SURFACE()
);
#2510=(
BOUNDED_SURFACE()
B_SPLINE_SURFACE(1,2,((#137209,#137210,#137211,#137212,#137213),(#137214,
#137215,#137216,#137217,#137218)),.UNSPECIFIED.,.F.,.F.,.F.)
B_SPLINE_SURFACE_WITH_KNOTS((2,2),(3,2,3),(0.,0.290270016622051),(0.15979901418408,
0.176967058622922,0.177555991088182),.UNSPECIFIED.)
GEOMETRIC_REPRESENTATION_ITEM()
RATIONAL_B_SPLINE_SURFACE(((0.990927469170791,0.98775996257079,0.98748925405691,
0.98748925405691,0.98748925405691),(0.990927469170791,0.98775996257079,
0.98748925405691,0.98748925405691,0.98748925405691)))
REPRESENTATION_ITEM('')
SURFACE()
);
#2511=(
BOUNDED_SURFACE()
B_SPLINE_SURFACE(1,2,((#137231,#137232,#137233,#137234,#137235,#137236,
#137237),(#137238,#137239,#137240,#137241,#137242,#137243,#137244)),
 .UNSPECIFIED.,.F.,.F.,.F.)
B_SPLINE_SURFACE_WITH_KNOTS((2,2),(3,2,2,3),(0.,0.289807040991555),(0.556037361265319,
0.55621282302886,0.571428571428571,0.573758999382975),.UNSPECIFIED.)
GEOMETRIC_REPRESENTATION_ITEM()
RATIONAL_B_SPLINE_SURFACE(((0.991593692313265,0.991593692313265,0.991593692313265,
0.994659131878644,1.,0.999181998279426,0.99841737279299),(0.991593692313265,
0.991593692313265,0.991593692313265,0.994659131878644,1.,0.999181998279426,
0.99841737279299)))
REPRESENTATION_ITEM('')
SURFACE()
);
#2512=(
BOUNDED_SURFACE()
B_SPLINE_SURFACE(1,2,((#137255,#137256,#137257,#137258,#137259),(#137260,
#137261,#137262,#137263,#137264)),.UNSPECIFIED.,.F.,.F.,.F.)
B_SPLINE_SURFACE_WITH_KNOTS((2,2),(3,2,3),(0.,0.29027001662738),(0.159799014184193,
0.176967058622922,0.1775559910934),.UNSPECIFIED.)
GEOMETRIC_REPRESENTATION_ITEM()
RATIONAL_B_SPLINE_SURFACE(((0.99092746917075,0.987759962570788,0.98748925405691,
0.98748925405691,0.98748925405691),(0.99092746917075,0.987759962570788,
0.98748925405691,0.98748925405691,0.98748925405691)))
REPRESENTATION_ITEM('')
SURFACE()
);
#2513=(
BOUNDED_SURFACE()
B_SPLINE_SURFACE(1,2,((#137280,#137281,#137282,#137283,#137284,#137285,
#137286),(#137287,#137288,#137289,#137290,#137291,#137292,#137293)),
 .UNSPECIFIED.,.F.,.F.,.F.)
B_SPLINE_SURFACE_WITH_KNOTS((2,2),(3,2,2,3),(0.,0.289807040991561),(0.556037361265318,
0.55621282302886,0.571428571428571,0.573758999383057),.UNSPECIFIED.)
GEOMETRIC_REPRESENTATION_ITEM()
RATIONAL_B_SPLINE_SURFACE(((0.991593692313265,0.991593692313265,0.991593692313265,
0.994659131878644,1.,0.999181998279397,0.998417372792936),(0.991593692313265,
0.991593692313265,0.991593692313265,0.994659131878644,1.,0.999181998279397,
0.998417372792936)))
REPRESENTATION_ITEM('')
SURFACE()
);
#2514=(
BOUNDED_SURFACE()
B_SPLINE_SURFACE(1,2,((#137308,#137309,#137310,#137311,#137312),(#137313,
#137314,#137315,#137316,#137317)),.UNSPECIFIED.,.F.,.F.,.F.)
B_SPLINE_SURFACE_WITH_KNOTS((2,2),(3,2,3),(0.,0.290268982604117),(0.504616569533924,
0.52191752982614,0.522505428232031),.UNSPECIFIED.)
GEOMETRIC_REPRESENTATION_ITEM()
RATIONAL_B_SPLINE_SURFACE(((0.996968549833844,0.991680746768616,0.989334769731189,
0.989334769731189,0.989334769731189),(0.996968549833844,0.991680746768616,
0.989334769731189,0.989334769731189,0.989334769731189)))
REPRESENTATION_ITEM('')
SURFACE()
);
#2515=(
BOUNDED_SURFACE()
B_SPLINE_SURFACE(1,2,((#137328,#137329,#137330,#137331,#137332),(#137333,
#137334,#137335,#137336,#137337)),.UNSPECIFIED.,.F.,.F.,.F.)
B_SPLINE_SURFACE_WITH_KNOTS((2,2),(3,2,3),(0.,0.289807040991617),(0.211502584834065,
0.214285714285714,0.228987659635173),.UNSPECIFIED.)
GEOMETRIC_REPRESENTATION_ITEM()
RATIONAL_B_SPLINE_SURFACE(((0.998122319569323,0.999023095875705,1.,0.994839481491405,
0.99180331349328),(0.998122319569323,0.999023095875705,1.,0.994839481491405,
0.99180331349328)))
REPRESENTATION_ITEM('')
SURFACE()
);
#2516=(
BOUNDED_SURFACE()
B_SPLINE_SURFACE(1,2,((#137360,#137361,#137362,#137363,#137364),(#137365,
#137366,#137367,#137368,#137369)),.UNSPECIFIED.,.F.,.F.,.F.)
B_SPLINE_SURFACE_WITH_KNOTS((2,2),(3,2,3),(0.,0.290268982619199),(0.504616569534225,
0.521917529826141,0.522505428247126),.UNSPECIFIED.)
GEOMETRIC_REPRESENTATION_ITEM()
RATIONAL_B_SPLINE_SURFACE(((0.99696854983366,0.991680746768575,0.989334769731189,
0.989334769731189,0.989334769731189),(0.99696854983366,0.991680746768575,
0.989334769731189,0.989334769731189,0.989334769731189)))
REPRESENTATION_ITEM('')
SURFACE()
);
#2517=(
BOUNDED_SURFACE()
B_SPLINE_SURFACE(1,2,((#137371,#137372,#137373,#137374,#137375),(#137376,
#137377,#137378,#137379,#137380)),.UNSPECIFIED.,.F.,.F.,.F.)
B_SPLINE_SURFACE_WITH_KNOTS((2,2),(3,2,3),(0.,0.289807040991574),(0.211502584834048,
0.214285714285714,0.228987659635174),.UNSPECIFIED.)
GEOMETRIC_REPRESENTATION_ITEM()
RATIONAL_B_SPLINE_SURFACE(((0.998122319569312,0.999023095875699,1.,0.994839481491404,
0.99180331349328),(0.998122319569312,0.999023095875699,1.,0.994839481491404,
0.99180331349328)))
REPRESENTATION_ITEM('')
SURFACE()
);
#2518=(
BOUNDED_SURFACE()
B_SPLINE_SURFACE(1,2,((#137403,#137404,#137405,#137406,#137407),(#137408,
#137409,#137410,#137411,#137412)),.UNSPECIFIED.,.F.,.F.,.F.)
B_SPLINE_SURFACE_WITH_KNOTS((2,2),(3,2,3),(0.,0.290268982597261),(0.504616569534328,
0.521917529826141,0.522505428225168),.UNSPECIFIED.)
GEOMETRIC_REPRESENTATION_ITEM()
RATIONAL_B_SPLINE_SURFACE(((0.996968549833597,0.99168074676856,0.989334769731189,
0.989334769731189,0.989334769731189),(0.996968549833597,0.99168074676856,
0.989334769731189,0.989334769731189,0.989334769731189)))
REPRESENTATION_ITEM('')
SURFACE()
);
#2519=(
BOUNDED_SURFACE()
B_SPLINE_SURFACE(1,2,((#137414,#137415,#137416,#137417,#137418),(#137419,
#137420,#137421,#137422,#137423)),.UNSPECIFIED.,.F.,.F.,.F.)
B_SPLINE_SURFACE_WITH_KNOTS((2,2),(3,2,3),(0.,0.289807040991561),(0.21150258483404,
0.214285714285714,0.228987659635174),.UNSPECIFIED.)
GEOMETRIC_REPRESENTATION_ITEM()
RATIONAL_B_SPLINE_SURFACE(((0.998122319569306,0.999023095875696,1.,0.994839481491404,
0.99180331349328),(0.998122319569306,0.999023095875696,1.,0.994839481491404,
0.99180331349328)))
REPRESENTATION_ITEM('')
SURFACE()
);
#2520=(
BOUNDED_SURFACE()
B_SPLINE_SURFACE(1,2,((#137446,#137447,#137448,#137449,#137450),(#137451,
#137452,#137453,#137454,#137455)),.UNSPECIFIED.,.F.,.F.,.F.)
B_SPLINE_SURFACE_WITH_KNOTS((2,2),(3,2,3),(0.,0.290268982610398),(0.504616569534327,
0.521917529826141,0.52250542823832),.UNSPECIFIED.)
GEOMETRIC_REPRESENTATION_ITEM()
RATIONAL_B_SPLINE_SURFACE(((0.996968549833597,0.991680746768561,0.989334769731189,
0.989334769731189,0.989334769731189),(0.996968549833597,0.991680746768561,
0.989334769731189,0.989334769731189,0.989334769731189)))
REPRESENTATION_ITEM('')
SURFACE()
);
#2521=(
BOUNDED_SURFACE()
B_SPLINE_SURFACE(1,2,((#137457,#137458,#137459,#137460,#137461),(#137462,
#137463,#137464,#137465,#137466)),.UNSPECIFIED.,.F.,.F.,.F.)
B_SPLINE_SURFACE_WITH_KNOTS((2,2),(3,2,3),(0.,0.289807040991562),(0.211502584834064,
0.214285714285714,0.228987659635173),.UNSPECIFIED.)
GEOMETRIC_REPRESENTATION_ITEM()
RATIONAL_B_SPLINE_SURFACE(((0.998122319569322,0.999023095875704,1.,0.994839481491405,
0.99180331349328),(0.998122319569322,0.999023095875704,1.,0.994839481491405,
0.99180331349328)))
REPRESENTATION_ITEM('')
SURFACE()
);
#2522=(
BOUNDED_SURFACE()
B_SPLINE_SURFACE(1,2,((#137489,#137490,#137491,#137492,#137493),(#137494,
#137495,#137496,#137497,#137498)),.UNSPECIFIED.,.F.,.F.,.F.)
B_SPLINE_SURFACE_WITH_KNOTS((2,2),(3,2,3),(0.,0.29026898260331),(0.504616569533844,
0.521917529826141,0.522505428231226),.UNSPECIFIED.)
GEOMETRIC_REPRESENTATION_ITEM()
RATIONAL_B_SPLINE_SURFACE(((0.996968549833893,0.991680746768626,0.989334769731189,
0.989334769731189,0.989334769731189),(0.996968549833893,0.991680746768626,
0.989334769731189,0.989334769731189,0.989334769731189)))
REPRESENTATION_ITEM('')
SURFACE()
);
#2523=(
BOUNDED_SURFACE()
B_SPLINE_SURFACE(1,2,((#137500,#137501,#137502,#137503,#137504),(#137505,
#137506,#137507,#137508,#137509)),.UNSPECIFIED.,.F.,.F.,.F.)
B_SPLINE_SURFACE_WITH_KNOTS((2,2),(3,2,3),(0.,0.289807040991557),(0.211502584834063,
0.214285714285714,0.228987659635058),.UNSPECIFIED.)
GEOMETRIC_REPRESENTATION_ITEM()
RATIONAL_B_SPLINE_SURFACE(((0.998122319569322,0.999023095875704,1.,0.994839481491445,
0.991803313493328),(0.998122319569322,0.999023095875704,1.,0.994839481491445,
0.991803313493328)))
REPRESENTATION_ITEM('')
SURFACE()
);
#2524=(
BOUNDED_SURFACE()
B_SPLINE_SURFACE(1,2,((#137532,#137533,#137534,#137535,#137536),(#137537,
#137538,#137539,#137540,#137541)),.UNSPECIFIED.,.F.,.F.,.F.)
B_SPLINE_SURFACE_WITH_KNOTS((2,2),(3,2,3),(0.,0.290268982592995),(0.504616569533987,
0.521917529826141,0.522505428220914),.UNSPECIFIED.)
GEOMETRIC_REPRESENTATION_ITEM()
RATIONAL_B_SPLINE_SURFACE(((0.996968549833805,0.991680746768607,0.989334769731189,
0.989334769731189,0.989334769731189),(0.996968549833805,0.991680746768607,
0.989334769731189,0.989334769731189,0.989334769731189)))
REPRESENTATION_ITEM('')
SURFACE()
);
#2525=(
BOUNDED_SURFACE()
B_SPLINE_SURFACE(1,2,((#137543,#137544,#137545,#137546,#137547),(#137548,
#137549,#137550,#137551,#137552)),.UNSPECIFIED.,.F.,.F.,.F.)
B_SPLINE_SURFACE_WITH_KNOTS((2,2),(3,2,3),(0.,0.289807040991557),(0.211502584834064,
0.214285714285714,0.228987659635173),.UNSPECIFIED.)
GEOMETRIC_REPRESENTATION_ITEM()
RATIONAL_B_SPLINE_SURFACE(((0.998122319569322,0.999023095875704,1.,0.994839481491405,
0.99180331349328),(0.998122319569322,0.999023095875704,1.,0.994839481491405,
0.99180331349328)))
REPRESENTATION_ITEM('')
SURFACE()
);
#2526=(
BOUNDED_SURFACE()
B_SPLINE_SURFACE(1,2,((#137575,#137576,#137577,#137578,#137579),(#137580,
#137581,#137582,#137583,#137584)),.UNSPECIFIED.,.F.,.F.,.F.)
B_SPLINE_SURFACE_WITH_KNOTS((2,2),(3,2,3),(0.,0.290268982594292),(0.50461656953416,
0.521917529826141,0.522505428222218),.UNSPECIFIED.)
GEOMETRIC_REPRESENTATION_ITEM()
RATIONAL_B_SPLINE_SURFACE(((0.996968549833699,0.991680746768583,0.989334769731189,
0.989334769731189,0.989334769731189),(0.996968549833699,0.991680746768583,
0.989334769731189,0.989334769731189,0.989334769731189)))
REPRESENTATION_ITEM('')
SURFACE()
);
#2527=(
BOUNDED_SURFACE()
B_SPLINE_SURFACE(1,2,((#137586,#137587,#137588,#137589,#137590),(#137591,
#137592,#137593,#137594,#137595)),.UNSPECIFIED.,.F.,.F.,.F.)
B_SPLINE_SURFACE_WITH_KNOTS((2,2),(3,2,3),(0.,0.28980704099156),(0.211502584834035,
0.214285714285714,0.228987659635174),.UNSPECIFIED.)
GEOMETRIC_REPRESENTATION_ITEM()
RATIONAL_B_SPLINE_SURFACE(((0.998122319569303,0.999023095875694,1.,0.994839481491404,
0.99180331349328),(0.998122319569303,0.999023095875694,1.,0.994839481491404,
0.99180331349328)))
REPRESENTATION_ITEM('')
SURFACE()
);
#2528=(
BOUNDED_SURFACE()
B_SPLINE_SURFACE(1,2,((#137603,#137604,#137605,#137606,#137607),(#137608,
#137609,#137610,#137611,#137612)),.UNSPECIFIED.,.F.,.F.,.F.)
B_SPLINE_SURFACE_WITH_KNOTS((2,2),(3,2,3),(0.,0.289946589047145),(0.504616569534328,
0.521917529826141,0.522183034675071),.UNSPECIFIED.)
GEOMETRIC_REPRESENTATION_ITEM()
RATIONAL_B_SPLINE_SURFACE(((0.996968549833597,0.991680746768561,0.989334769731189,
0.989334769731189,0.989334769731189),(0.996968549833597,0.991680746768561,
0.989334769731189,0.989334769731189,0.989334769731189)))
REPRESENTATION_ITEM('')
SURFACE()
);
#2529=(
BOUNDED_SURFACE()
B_SPLINE_SURFACE(1,2,((#137614,#137615,#137616,#137617,#137618),(#137619,
#137620,#137621,#137622,#137623)),.UNSPECIFIED.,.F.,.F.,.F.)
B_SPLINE_SURFACE_WITH_KNOTS((2,2),(3,2,3),(0.,0.289807040991555),(0.211502584834064,
0.214285714285714,0.228987659635174),.UNSPECIFIED.)
GEOMETRIC_REPRESENTATION_ITEM()
RATIONAL_B_SPLINE_SURFACE(((0.998122319569322,0.999023095875704,1.,0.994839481491404,
0.99180331349328),(0.998122319569322,0.999023095875704,1.,0.994839481491404,
0.99180331349328)))
REPRESENTATION_ITEM('')
SURFACE()
);
#2530=(
BOUNDED_SURFACE()
B_SPLINE_SURFACE(1,2,((#137646,#137647,#137648,#137649,#137650),(#137651,
#137652,#137653,#137654,#137655)),.UNSPECIFIED.,.F.,.F.,.F.)
B_SPLINE_SURFACE_WITH_KNOTS((2,2),(3,2,3),(0.,0.290268982610033),(0.504616569534328,
0.521917529826141,0.522505428237962),.UNSPECIFIED.)
GEOMETRIC_REPRESENTATION_ITEM()
RATIONAL_B_SPLINE_SURFACE(((0.996968549833597,0.991680746768561,0.989334769731189,
0.989334769731189,0.989334769731189),(0.996968549833597,0.991680746768561,
0.989334769731189,0.989334769731189,0.989334769731189)))
REPRESENTATION_ITEM('')
SURFACE()
);
#2531=(
BOUNDED_SURFACE()
B_SPLINE_SURFACE(1,2,((#137657,#137658,#137659,#137660,#137661),(#137662,
#137663,#137664,#137665,#137666)),.UNSPECIFIED.,.F.,.F.,.F.)
B_SPLINE_SURFACE_WITH_KNOTS((2,2),(3,2,3),(0.,0.289807040991566),(0.211502584834064,
0.214285714285714,0.228987659635174),.UNSPECIFIED.)
GEOMETRIC_REPRESENTATION_ITEM()
RATIONAL_B_SPLINE_SURFACE(((0.998122319569322,0.999023095875704,1.,0.994839481491404,
0.99180331349328),(0.998122319569322,0.999023095875704,1.,0.994839481491404,
0.99180331349328)))
REPRESENTATION_ITEM('')
SURFACE()
);
#2532=(
BOUNDED_SURFACE()
B_SPLINE_SURFACE(1,2,((#137689,#137690,#137691,#137692,#137693),(#137694,
#137695,#137696,#137697,#137698)),.UNSPECIFIED.,.F.,.F.,.F.)
B_SPLINE_SURFACE_WITH_KNOTS((2,2),(3,2,3),(0.,0.290268982603647),(0.504616569534328,
0.521917529826141,0.522505428231568),.UNSPECIFIED.)
GEOMETRIC_REPRESENTATION_ITEM()
RATIONAL_B_SPLINE_SURFACE(((0.996968549833597,0.99168074676856,0.989334769731189,
0.989334769731189,0.989334769731189),(0.996968549833597,0.99168074676856,
0.989334769731189,0.989334769731189,0.989334769731189)))
REPRESENTATION_ITEM('')
SURFACE()
);
#2533=(
BOUNDED_SURFACE()
B_SPLINE_SURFACE(1,2,((#137700,#137701,#137702,#137703,#137704),(#137705,
#137706,#137707,#137708,#137709)),.UNSPECIFIED.,.F.,.F.,.F.)
B_SPLINE_SURFACE_WITH_KNOTS((2,2),(3,2,3),(0.,0.289807040991558),(0.21150258483406,
0.214285714285714,0.228987659635174),.UNSPECIFIED.)
GEOMETRIC_REPRESENTATION_ITEM()
RATIONAL_B_SPLINE_SURFACE(((0.998122319569319,0.999023095875703,1.,0.994839481491405,
0.99180331349328),(0.998122319569319,0.999023095875703,1.,0.994839481491405,
0.99180331349328)))
REPRESENTATION_ITEM('')
SURFACE()
);
#2534=(
BOUNDED_SURFACE()
B_SPLINE_SURFACE(1,2,((#137732,#137733,#137734,#137735,#137736),(#137737,
#137738,#137739,#137740,#137741)),.UNSPECIFIED.,.F.,.F.,.F.)
B_SPLINE_SURFACE_WITH_KNOTS((2,2),(3,2,3),(0.,0.290268982606492),(0.504616569534328,
0.521917529826141,0.522505428234414),.UNSPECIFIED.)
GEOMETRIC_REPRESENTATION_ITEM()
RATIONAL_B_SPLINE_SURFACE(((0.996968549833597,0.99168074676856,0.989334769731189,
0.989334769731189,0.989334769731189),(0.996968549833597,0.99168074676856,
0.989334769731189,0.989334769731189,0.989334769731189)))
REPRESENTATION_ITEM('')
SURFACE()
);
#2535=(
BOUNDED_SURFACE()
B_SPLINE_SURFACE(1,2,((#137743,#137744,#137745,#137746,#137747),(#137748,
#137749,#137750,#137751,#137752)),.UNSPECIFIED.,.F.,.F.,.F.)
B_SPLINE_SURFACE_WITH_KNOTS((2,2),(3,2,3),(0.,0.289807040991564),(0.211502584834064,
0.214285714285714,0.228987659635174),.UNSPECIFIED.)
GEOMETRIC_REPRESENTATION_ITEM()
RATIONAL_B_SPLINE_SURFACE(((0.998122319569322,0.999023095875704,1.,0.994839481491405,
0.99180331349328),(0.998122319569322,0.999023095875704,1.,0.994839481491405,
0.99180331349328)))
REPRESENTATION_ITEM('')
SURFACE()
);
#2536=(
BOUNDED_SURFACE()
B_SPLINE_SURFACE(1,2,((#137775,#137776,#137777,#137778,#137779),(#137780,
#137781,#137782,#137783,#137784)),.UNSPECIFIED.,.F.,.F.,.F.)
B_SPLINE_SURFACE_WITH_KNOTS((2,2),(3,2,3),(0.,0.290268982616428),(0.504616569534328,
0.521917529826141,0.522505428244344),.UNSPECIFIED.)
GEOMETRIC_REPRESENTATION_ITEM()
RATIONAL_B_SPLINE_SURFACE(((0.996968549833597,0.99168074676856,0.989334769731189,
0.989334769731189,0.989334769731189),(0.996968549833597,0.99168074676856,
0.989334769731189,0.989334769731189,0.989334769731189)))
REPRESENTATION_ITEM('')
SURFACE()
);
#2537=(
BOUNDED_SURFACE()
B_SPLINE_SURFACE(1,2,((#137786,#137787,#137788,#137789,#137790),(#137791,
#137792,#137793,#137794,#137795)),.UNSPECIFIED.,.F.,.F.,.F.)
B_SPLINE_SURFACE_WITH_KNOTS((2,2),(3,2,3),(0.,0.289807040991564),(0.211502584834024,
0.214285714285714,0.228987659635174),.UNSPECIFIED.)
GEOMETRIC_REPRESENTATION_ITEM()
RATIONAL_B_SPLINE_SURFACE(((0.998122319569296,0.99902309587569,1.,0.994839481491404,
0.99180331349328),(0.998122319569296,0.99902309587569,1.,0.994839481491404,
0.99180331349328)))
REPRESENTATION_ITEM('')
SURFACE()
);
#2538=(
BOUNDED_SURFACE()
B_SPLINE_SURFACE(1,2,((#137818,#137819,#137820,#137821,#137822),(#137823,
#137824,#137825,#137826,#137827)),.UNSPECIFIED.,.F.,.F.,.F.)
B_SPLINE_SURFACE_WITH_KNOTS((2,2),(3,2,3),(0.,0.29026898259843),(0.504616569534328,
0.521917529826141,0.522505428226351),.UNSPECIFIED.)
GEOMETRIC_REPRESENTATION_ITEM()
RATIONAL_B_SPLINE_SURFACE(((0.996968549833597,0.991680746768561,0.989334769731189,
0.989334769731189,0.989334769731189),(0.996968549833597,0.991680746768561,
0.989334769731189,0.989334769731189,0.989334769731189)))
REPRESENTATION_ITEM('')
SURFACE()
);
#2539=(
BOUNDED_SURFACE()
B_SPLINE_SURFACE(1,2,((#137829,#137830,#137831,#137832,#137833),(#137834,
#137835,#137836,#137837,#137838)),.UNSPECIFIED.,.F.,.F.,.F.)
B_SPLINE_SURFACE_WITH_KNOTS((2,2),(3,2,3),(0.,0.28980704099156),(0.211502584834064,
0.214285714285714,0.228987659635174),.UNSPECIFIED.)
GEOMETRIC_REPRESENTATION_ITEM()
RATIONAL_B_SPLINE_SURFACE(((0.998122319569322,0.999023095875704,1.,0.994839481491404,
0.99180331349328),(0.998122319569322,0.999023095875704,1.,0.994839481491404,
0.99180331349328)))
REPRESENTATION_ITEM('')
SURFACE()
);
#2540=(
BOUNDED_SURFACE()
B_SPLINE_SURFACE(1,2,((#137861,#137862,#137863,#137864,#137865),(#137866,
#137867,#137868,#137869,#137870)),.UNSPECIFIED.,.F.,.F.,.F.)
B_SPLINE_SURFACE_WITH_KNOTS((2,2),(3,2,3),(0.,0.290268982603716),(0.504616569534328,
0.521917529826141,0.52250542823164),.UNSPECIFIED.)
GEOMETRIC_REPRESENTATION_ITEM()
RATIONAL_B_SPLINE_SURFACE(((0.996968549833597,0.99168074676856,0.989334769731189,
0.989334769731189,0.989334769731189),(0.996968549833597,0.99168074676856,
0.989334769731189,0.989334769731189,0.989334769731189)))
REPRESENTATION_ITEM('')
SURFACE()
);
#2541=(
BOUNDED_SURFACE()
B_SPLINE_SURFACE(1,2,((#137872,#137873,#137874,#137875,#137876),(#137877,
#137878,#137879,#137880,#137881)),.UNSPECIFIED.,.F.,.F.,.F.)
B_SPLINE_SURFACE_WITH_KNOTS((2,2),(3,2,3),(0.,0.28980704099156),(0.211502584834064,
0.214285714285714,0.228987659635174),.UNSPECIFIED.)
GEOMETRIC_REPRESENTATION_ITEM()
RATIONAL_B_SPLINE_SURFACE(((0.998122319569322,0.999023095875704,1.,0.994839481491404,
0.99180331349328),(0.998122319569322,0.999023095875704,1.,0.994839481491404,
0.99180331349328)))
REPRESENTATION_ITEM('')
SURFACE()
);
#2542=(
BOUNDED_SURFACE()
B_SPLINE_SURFACE(1,2,((#137904,#137905,#137906,#137907,#137908),(#137909,
#137910,#137911,#137912,#137913)),.UNSPECIFIED.,.F.,.F.,.F.)
B_SPLINE_SURFACE_WITH_KNOTS((2,2),(3,2,3),(0.,0.290268982599203),(0.504616569534328,
0.521917529826141,0.52250542822713),.UNSPECIFIED.)
GEOMETRIC_REPRESENTATION_ITEM()
RATIONAL_B_SPLINE_SURFACE(((0.996968549833597,0.991680746768561,0.989334769731189,
0.989334769731189,0.989334769731189),(0.996968549833597,0.991680746768561,
0.989334769731189,0.989334769731189,0.989334769731189)))
REPRESENTATION_ITEM('')
SURFACE()
);
#2543=(
BOUNDED_SURFACE()
B_SPLINE_SURFACE(1,2,((#137915,#137916,#137917,#137918,#137919),(#137920,
#137921,#137922,#137923,#137924)),.UNSPECIFIED.,.F.,.F.,.F.)
B_SPLINE_SURFACE_WITH_KNOTS((2,2),(3,2,3),(0.,0.289807040991561),(0.211502584833965,
0.214285714285714,0.228987659635174),.UNSPECIFIED.)
GEOMETRIC_REPRESENTATION_ITEM()
RATIONAL_B_SPLINE_SURFACE(((0.998122319569258,0.99902309587567,1.,0.994839481491404,
0.99180331349328),(0.998122319569258,0.99902309587567,1.,0.994839481491404,
0.99180331349328)))
REPRESENTATION_ITEM('')
SURFACE()
);
#2544=(
BOUNDED_SURFACE()
B_SPLINE_SURFACE(1,2,((#137947,#137948,#137949,#137950,#137951),(#137952,
#137953,#137954,#137955,#137956)),.UNSPECIFIED.,.F.,.F.,.F.)
B_SPLINE_SURFACE_WITH_KNOTS((2,2),(3,2,3),(0.,0.290268982598464),(0.504616569534328,
0.521917529826141,0.522505428226386),.UNSPECIFIED.)
GEOMETRIC_REPRESENTATION_ITEM()
RATIONAL_B_SPLINE_SURFACE(((0.996968549833597,0.99168074676856,0.989334769731189,
0.989334769731189,0.989334769731189),(0.996968549833597,0.99168074676856,
0.989334769731189,0.989334769731189,0.989334769731189)))
REPRESENTATION_ITEM('')
SURFACE()
);
#2545=(
BOUNDED_SURFACE()
B_SPLINE_SURFACE(1,2,((#137958,#137959,#137960,#137961,#137962),(#137963,
#137964,#137965,#137966,#137967)),.UNSPECIFIED.,.F.,.F.,.F.)
B_SPLINE_SURFACE_WITH_KNOTS((2,2),(3,2,3),(0.,0.289807040991561),(0.211502584833903,
0.214285714285714,0.228987659635175),.UNSPECIFIED.)
GEOMETRIC_REPRESENTATION_ITEM()
RATIONAL_B_SPLINE_SURFACE(((0.998122319569217,0.999023095875648,1.,0.994839481491404,
0.991803313493279),(0.998122319569217,0.999023095875648,1.,0.994839481491404,
0.991803313493279)))
REPRESENTATION_ITEM('')
SURFACE()
);
#2546=(
BOUNDED_SURFACE()
B_SPLINE_SURFACE(1,2,((#137990,#137991,#137992,#137993,#137994),(#137995,
#137996,#137997,#137998,#137999)),.UNSPECIFIED.,.F.,.F.,.F.)
B_SPLINE_SURFACE_WITH_KNOTS((2,2),(3,2,3),(0.,0.290268982577918),(0.504616569534328,
0.521917529826141,0.522505428205845),.UNSPECIFIED.)
GEOMETRIC_REPRESENTATION_ITEM()
RATIONAL_B_SPLINE_SURFACE(((0.996968549833597,0.99168074676856,0.989334769731189,
0.989334769731189,0.989334769731189),(0.996968549833597,0.99168074676856,
0.989334769731189,0.989334769731189,0.989334769731189)))
REPRESENTATION_ITEM('')
SURFACE()
);
#2547=(
BOUNDED_SURFACE()
B_SPLINE_SURFACE(1,2,((#138001,#138002,#138003,#138004,#138005),(#138006,
#138007,#138008,#138009,#138010)),.UNSPECIFIED.,.F.,.F.,.F.)
B_SPLINE_SURFACE_WITH_KNOTS((2,2),(3,2,3),(0.,0.289807040991564),(0.211502584833963,
0.214285714285714,0.228987659635174),.UNSPECIFIED.)
GEOMETRIC_REPRESENTATION_ITEM()
RATIONAL_B_SPLINE_SURFACE(((0.998122319569257,0.999023095875669,1.,0.994839481491404,
0.99180331349328),(0.998122319569257,0.999023095875669,1.,0.994839481491404,
0.99180331349328)))
REPRESENTATION_ITEM('')
SURFACE()
);
#2548=(
BOUNDED_SURFACE()
B_SPLINE_SURFACE(1,2,((#138033,#138034,#138035,#138036,#138037),(#138038,
#138039,#138040,#138041,#138042)),.UNSPECIFIED.,.F.,.F.,.F.)
B_SPLINE_SURFACE_WITH_KNOTS((2,2),(3,2,3),(0.,0.290268982592395),(0.504616569534328,
0.521917529826141,0.522505428220313),.UNSPECIFIED.)
GEOMETRIC_REPRESENTATION_ITEM()
RATIONAL_B_SPLINE_SURFACE(((0.996968549833597,0.99168074676856,0.989334769731189,
0.989334769731189,0.989334769731189),(0.996968549833597,0.99168074676856,
0.989334769731189,0.989334769731189,0.989334769731189)))
REPRESENTATION_ITEM('')
SURFACE()
);
#2549=(
BOUNDED_SURFACE()
B_SPLINE_SURFACE(1,2,((#138044,#138045,#138046,#138047,#138048),(#138049,
#138050,#138051,#138052,#138053)),.UNSPECIFIED.,.F.,.F.,.F.)
B_SPLINE_SURFACE_WITH_KNOTS((2,2),(3,2,3),(0.,0.28980704099156),(0.211502584833935,
0.214285714285714,0.228987659635175),.UNSPECIFIED.)
GEOMETRIC_REPRESENTATION_ITEM()
RATIONAL_B_SPLINE_SURFACE(((0.998122319569238,0.999023095875659,1.,0.994839481491404,
0.991803313493279),(0.998122319569238,0.999023095875659,1.,0.994839481491404,
0.991803313493279)))
REPRESENTATION_ITEM('')
SURFACE()
);
#2550=(
BOUNDED_SURFACE()
B_SPLINE_SURFACE(1,2,((#138076,#138077,#138078,#138079,#138080),(#138081,
#138082,#138083,#138084,#138085)),.UNSPECIFIED.,.F.,.F.,.F.)
B_SPLINE_SURFACE_WITH_KNOTS((2,2),(3,2,3),(0.,0.290268982611678),(0.504616569534328,
0.521917529826141,0.522505428239596),.UNSPECIFIED.)
GEOMETRIC_REPRESENTATION_ITEM()
RATIONAL_B_SPLINE_SURFACE(((0.996968549833597,0.99168074676856,0.989334769731189,
0.989334769731189,0.989334769731189),(0.996968549833597,0.99168074676856,
0.989334769731189,0.989334769731189,0.989334769731189)))
REPRESENTATION_ITEM('')
SURFACE()
);
#2551=(
BOUNDED_SURFACE()
B_SPLINE_SURFACE(1,2,((#138087,#138088,#138089,#138090,#138091),(#138092,
#138093,#138094,#138095,#138096)),.UNSPECIFIED.,.F.,.F.,.F.)
B_SPLINE_SURFACE_WITH_KNOTS((2,2),(3,2,3),(0.,0.289807040991559),(0.211502584833671,
0.214285714285714,0.228987659635176),.UNSPECIFIED.)
GEOMETRIC_REPRESENTATION_ITEM()
RATIONAL_B_SPLINE_SURFACE(((0.998122319569068,0.999023095875566,1.,0.994839481491404,
0.991803313493279),(0.998122319569068,0.999023095875566,1.,0.994839481491404,
0.991803313493279)))
REPRESENTATION_ITEM('')
SURFACE()
);
#2552=(
BOUNDED_SURFACE()
B_SPLINE_SURFACE(1,2,((#138119,#138120,#138121,#138122,#138123),(#138124,
#138125,#138126,#138127,#138128)),.UNSPECIFIED.,.F.,.F.,.F.)
B_SPLINE_SURFACE_WITH_KNOTS((2,2),(3,2,3),(0.,0.290268982583992),(0.504616569534328,
0.521917529826141,0.522505428211919),.UNSPECIFIED.)
GEOMETRIC_REPRESENTATION_ITEM()
RATIONAL_B_SPLINE_SURFACE(((0.996968549833597,0.99168074676856,0.989334769731189,
0.989334769731189,0.989334769731189),(0.996968549833597,0.99168074676856,
0.989334769731189,0.989334769731189,0.989334769731189)))
REPRESENTATION_ITEM('')
SURFACE()
);
#2553=(
BOUNDED_SURFACE()
B_SPLINE_SURFACE(1,2,((#138130,#138131,#138132,#138133,#138134),(#138135,
#138136,#138137,#138138,#138139)),.UNSPECIFIED.,.F.,.F.,.F.)
B_SPLINE_SURFACE_WITH_KNOTS((2,2),(3,2,3),(0.,0.289807040991556),(0.211502584833923,
0.214285714285714,0.228987659635175),.UNSPECIFIED.)
GEOMETRIC_REPRESENTATION_ITEM()
RATIONAL_B_SPLINE_SURFACE(((0.99812231956923,0.999023095875655,1.,0.994839481491404,
0.99180331349328),(0.99812231956923,0.999023095875655,1.,0.994839481491404,
0.99180331349328)))
REPRESENTATION_ITEM('')
SURFACE()
);
#2554=(
BOUNDED_SURFACE()
B_SPLINE_SURFACE(1,2,((#138156,#138157,#138158,#138159,#138160),(#138161,
#138162,#138163,#138164,#138165)),.UNSPECIFIED.,.F.,.F.,.F.)
B_SPLINE_SURFACE_WITH_KNOTS((2,2),(3,2,3),(0.,0.290268982617608),(0.504616569534328,
0.521917529826141,0.522505428236512),.UNSPECIFIED.)
GEOMETRIC_REPRESENTATION_ITEM()
RATIONAL_B_SPLINE_SURFACE(((0.996968549833597,0.991680746768561,0.989334769731189,
0.989334769731189,0.989334769731189),(0.996968549833597,0.991680746768561,
0.989334769731189,0.989334769731189,0.989334769731189)))
REPRESENTATION_ITEM('')
SURFACE()
);
#2555=(
BOUNDED_SURFACE()
B_SPLINE_SURFACE(1,2,((#138173,#138174,#138175,#138176,#138177),(#138178,
#138179,#138180,#138181,#138182)),.UNSPECIFIED.,.F.,.F.,.F.)
B_SPLINE_SURFACE_WITH_KNOTS((2,2),(3,2,3),(0.,0.289807040991561),(0.21150258483406,
0.214285714285714,0.228987659635174),.UNSPECIFIED.)
GEOMETRIC_REPRESENTATION_ITEM()
RATIONAL_B_SPLINE_SURFACE(((0.998122319569319,0.999023095875703,1.,0.994839481491404,
0.99180331349328),(0.998122319569319,0.999023095875703,1.,0.994839481491404,
0.99180331349328)))
REPRESENTATION_ITEM('')
SURFACE()
);
#2556=(
BOUNDED_SURFACE()
B_SPLINE_SURFACE(1,2,((#138205,#138206,#138207,#138208,#138209),(#138210,
#138211,#138212,#138213,#138214)),.UNSPECIFIED.,.F.,.F.,.F.)
B_SPLINE_SURFACE_WITH_KNOTS((2,2),(3,2,3),(0.,0.290268982598661),(0.504616569534328,
0.521917529826141,0.522505428226585),.UNSPECIFIED.)
GEOMETRIC_REPRESENTATION_ITEM()
RATIONAL_B_SPLINE_SURFACE(((0.996968549833597,0.99168074676856,0.989334769731189,
0.989334769731189,0.989334769731189),(0.996968549833597,0.99168074676856,
0.989334769731189,0.989334769731189,0.989334769731189)))
REPRESENTATION_ITEM('')
SURFACE()
);
#2557=(
BOUNDED_SURFACE()
B_SPLINE_SURFACE(1,2,((#138216,#138217,#138218,#138219,#138220),(#138221,
#138222,#138223,#138224,#138225)),.UNSPECIFIED.,.F.,.F.,.F.)
B_SPLINE_SURFACE_WITH_KNOTS((2,2),(3,2,3),(0.,0.289807040993648),(0.211502584834061,
0.214285714285714,0.228987659635175),.UNSPECIFIED.)
GEOMETRIC_REPRESENTATION_ITEM()
RATIONAL_B_SPLINE_SURFACE(((0.99812231956932,0.999023095875703,1.,0.994839481491404,
0.99180331349328),(0.99812231956932,0.999023095875703,1.,0.994839481491404,
0.991803313493279)))
REPRESENTATION_ITEM('')
SURFACE()
);
#2558=(
BOUNDED_SURFACE()
B_SPLINE_SURFACE(1,2,((#138248,#138249,#138250,#138251,#138252),(#138253,
#138254,#138255,#138256,#138257)),.UNSPECIFIED.,.F.,.F.,.F.)
B_SPLINE_SURFACE_WITH_KNOTS((2,2),(3,2,3),(0.,0.290268982618429),(0.504616569534327,
0.521917529826142,0.522505428246144),.UNSPECIFIED.)
GEOMETRIC_REPRESENTATION_ITEM()
RATIONAL_B_SPLINE_SURFACE(((0.996968549833597,0.99168074676856,0.989334769731189,
0.989334769731189,0.989334769731189),(0.996968549833597,0.99168074676856,
0.989334769731189,0.989334769731189,0.989334769731189)))
REPRESENTATION_ITEM('')
SURFACE()
);
#2559=(
BOUNDED_SURFACE()
B_SPLINE_SURFACE(1,2,((#138259,#138260,#138261,#138262,#138263),(#138264,
#138265,#138266,#138267,#138268)),.UNSPECIFIED.,.F.,.F.,.F.)
B_SPLINE_SURFACE_WITH_KNOTS((2,2),(3,2,3),(0.,0.289807040992029),(0.211502584834065,
0.214285714285714,0.228987659635175),.UNSPECIFIED.)
GEOMETRIC_REPRESENTATION_ITEM()
RATIONAL_B_SPLINE_SURFACE(((0.998122319569323,0.999023095875705,1.,0.994839481491404,
0.991803313493279),(0.998122319569323,0.999023095875705,1.,0.994839481491404,
0.991803313493279)))
REPRESENTATION_ITEM('')
SURFACE()
);
#2560=(
BOUNDED_SURFACE()
B_SPLINE_SURFACE(1,2,((#138291,#138292,#138293,#138294,#138295),(#138296,
#138297,#138298,#138299,#138300)),.UNSPECIFIED.,.F.,.F.,.F.)
B_SPLINE_SURFACE_WITH_KNOTS((2,2),(3,2,3),(0.,0.290268982582821),(0.504616569534327,
0.52191752982614,0.522505428210736),.UNSPECIFIED.)
GEOMETRIC_REPRESENTATION_ITEM()
RATIONAL_B_SPLINE_SURFACE(((0.996968549833597,0.991680746768561,0.989334769731189,
0.989334769731189,0.989334769731189),(0.996968549833597,0.991680746768561,
0.989334769731189,0.989334769731189,0.989334769731189)))
REPRESENTATION_ITEM('')
SURFACE()
);
#2561=(
BOUNDED_SURFACE()
B_SPLINE_SURFACE(1,2,((#138302,#138303,#138304,#138305,#138306),(#138307,
#138308,#138309,#138310,#138311)),.UNSPECIFIED.,.F.,.F.,.F.)
B_SPLINE_SURFACE_WITH_KNOTS((2,2),(3,2,3),(0.,0.289807040991643),(0.211502584834065,
0.214285714285714,0.228987659635175),.UNSPECIFIED.)
GEOMETRIC_REPRESENTATION_ITEM()
RATIONAL_B_SPLINE_SURFACE(((0.998122319569323,0.999023095875705,1.,0.994839481491404,
0.991803313493279),(0.998122319569323,0.999023095875705,1.,0.994839481491404,
0.991803313493279)))
REPRESENTATION_ITEM('')
SURFACE()
);
#2562=(
BOUNDED_SURFACE()
B_SPLINE_SURFACE(1,2,((#138334,#138335,#138336,#138337,#138338),(#138339,
#138340,#138341,#138342,#138343)),.UNSPECIFIED.,.F.,.F.,.F.)
B_SPLINE_SURFACE_WITH_KNOTS((2,2),(3,2,3),(0.,0.290268982593328),(0.504616569534327,
0.521917529826142,0.522505428221249),.UNSPECIFIED.)
GEOMETRIC_REPRESENTATION_ITEM()
RATIONAL_B_SPLINE_SURFACE(((0.996968549833597,0.99168074676856,0.989334769731189,
0.989334769731189,0.989334769731189),(0.996968549833597,0.99168074676856,
0.989334769731189,0.989334769731189,0.989334769731189)))
REPRESENTATION_ITEM('')
SURFACE()
);
#2563=(
BOUNDED_SURFACE()
B_SPLINE_SURFACE(1,2,((#138345,#138346,#138347,#138348,#138349),(#138350,
#138351,#138352,#138353,#138354)),.UNSPECIFIED.,.F.,.F.,.F.)
B_SPLINE_SURFACE_WITH_KNOTS((2,2),(3,2,3),(0.,0.289807040991633),(0.211502584834064,
0.214285714285714,0.228987659635175),.UNSPECIFIED.)
GEOMETRIC_REPRESENTATION_ITEM()
RATIONAL_B_SPLINE_SURFACE(((0.998122319569322,0.999023095875704,1.,0.994839481491404,
0.991803313493279),(0.998122319569322,0.999023095875704,1.,0.994839481491404,
0.991803313493279)))
REPRESENTATION_ITEM('')
SURFACE()
);
#2564=(
BOUNDED_SURFACE()
B_SPLINE_SURFACE(1,2,((#138377,#138378,#138379,#138380,#138381),(#138382,
#138383,#138384,#138385,#138386)),.UNSPECIFIED.,.F.,.F.,.F.)
B_SPLINE_SURFACE_WITH_KNOTS((2,2),(3,2,3),(0.,0.290268982634772),(0.504616569534327,
0.521917529826142,0.522505428262693),.UNSPECIFIED.)
GEOMETRIC_REPRESENTATION_ITEM()
RATIONAL_B_SPLINE_SURFACE(((0.996968549833597,0.99168074676856,0.989334769731189,
0.989334769731189,0.989334769731189),(0.996968549833597,0.991680746768561,
0.989334769731189,0.989334769731189,0.989334769731189)))
REPRESENTATION_ITEM('')
SURFACE()
);
#2565=(
BOUNDED_SURFACE()
B_SPLINE_SURFACE(1,2,((#138388,#138389,#138390,#138391,#138392),(#138393,
#138394,#138395,#138396,#138397)),.UNSPECIFIED.,.F.,.F.,.F.)
B_SPLINE_SURFACE_WITH_KNOTS((2,2),(3,2,3),(0.,0.289807040991638),(0.211502584834065,
0.214285714285714,0.228987659635174),.UNSPECIFIED.)
GEOMETRIC_REPRESENTATION_ITEM()
RATIONAL_B_SPLINE_SURFACE(((0.998122319569323,0.999023095875705,1.,0.994839481491404,
0.99180331349328),(0.998122319569323,0.999023095875705,1.,0.994839481491404,
0.99180331349328)))
REPRESENTATION_ITEM('')
SURFACE()
);
#2566=(
BOUNDED_SURFACE()
B_SPLINE_SURFACE(1,2,((#138420,#138421,#138422,#138423,#138424),(#138425,
#138426,#138427,#138428,#138429)),.UNSPECIFIED.,.F.,.F.,.F.)
B_SPLINE_SURFACE_WITH_KNOTS((2,2),(3,2,3),(0.,0.290268982580509),(0.504616569534258,
0.521917529826143,0.522505428208433),.UNSPECIFIED.)
GEOMETRIC_REPRESENTATION_ITEM()
RATIONAL_B_SPLINE_SURFACE(((0.99696854983364,0.991680746768569,0.989334769731188,
0.989334769731188,0.989334769731188),(0.99696854983364,0.991680746768569,
0.989334769731188,0.989334769731188,0.989334769731188)))
REPRESENTATION_ITEM('')
SURFACE()
);
#2567=(
BOUNDED_SURFACE()
B_SPLINE_SURFACE(1,2,((#138431,#138432,#138433,#138434,#138435),(#138436,
#138437,#138438,#138439,#138440)),.UNSPECIFIED.,.F.,.F.,.F.)
B_SPLINE_SURFACE_WITH_KNOTS((2,2),(3,2,3),(0.,0.289807040991953),(0.211502584834065,
0.214285714285714,0.228987659634945),.UNSPECIFIED.)
GEOMETRIC_REPRESENTATION_ITEM()
RATIONAL_B_SPLINE_SURFACE(((0.998122319569323,0.999023095875705,1.,0.994839481491485,
0.991803313493374),(0.998122319569323,0.999023095875705,1.,0.994839481491485,
0.991803313493374)))
REPRESENTATION_ITEM('')
SURFACE()
);
#2568=(
BOUNDED_SURFACE()
B_SPLINE_SURFACE(1,2,((#138463,#138464,#138465,#138466,#138467),(#138468,
#138469,#138470,#138471,#138472)),.UNSPECIFIED.,.F.,.F.,.F.)
B_SPLINE_SURFACE_WITH_KNOTS((2,2),(3,2,3),(0.,0.290268982596918),(0.504616569534069,
0.52191752982614,0.522505428224833),.UNSPECIFIED.)
GEOMETRIC_REPRESENTATION_ITEM()
RATIONAL_B_SPLINE_SURFACE(((0.996968549833755,0.991680746768596,0.989334769731189,
0.989334769731189,0.989334769731189),(0.996968549833755,0.991680746768596,
0.989334769731189,0.989334769731189,0.989334769731189)))
REPRESENTATION_ITEM('')
SURFACE()
);
#2569=(
BOUNDED_SURFACE()
B_SPLINE_SURFACE(1,2,((#138474,#138475,#138476,#138477,#138478),(#138479,
#138480,#138481,#138482,#138483)),.UNSPECIFIED.,.F.,.F.,.F.)
B_SPLINE_SURFACE_WITH_KNOTS((2,2),(3,2,3),(0.,0.289807040991604),(0.211502584834065,
0.214285714285714,0.228987659635174),.UNSPECIFIED.)
GEOMETRIC_REPRESENTATION_ITEM()
RATIONAL_B_SPLINE_SURFACE(((0.998122319569323,0.999023095875705,1.,0.994839481491404,
0.99180331349328),(0.998122319569323,0.999023095875705,1.,0.994839481491404,
0.99180331349328)))
REPRESENTATION_ITEM('')
SURFACE()
);
#2570=(
BOUNDED_SURFACE()
B_SPLINE_SURFACE(1,2,((#138506,#138507,#138508,#138509,#138510),(#138511,
#138512,#138513,#138514,#138515)),.UNSPECIFIED.,.F.,.F.,.F.)
B_SPLINE_SURFACE_WITH_KNOTS((2,2),(3,2,3),(0.,0.290268982595245),(0.504616569533905,
0.52191752982614,0.52250542822317),.UNSPECIFIED.)
GEOMETRIC_REPRESENTATION_ITEM()
RATIONAL_B_SPLINE_SURFACE(((0.996968549833855,0.991680746768618,0.989334769731189,
0.989334769731189,0.989334769731189),(0.996968549833855,0.991680746768618,
0.989334769731189,0.989334769731189,0.989334769731189)))
REPRESENTATION_ITEM('')
SURFACE()
);
#2571=(
BOUNDED_SURFACE()
B_SPLINE_SURFACE(1,2,((#138529,#138530,#138531,#138532,#138533),(#138534,
#138535,#138536,#138537,#138538)),.UNSPECIFIED.,.F.,.F.,.F.)
B_SPLINE_SURFACE_WITH_KNOTS((2,2),(3,2,3),(0.,0.289807040991612),(0.211502584834063,
0.214285714285714,0.228987659635174),.UNSPECIFIED.)
GEOMETRIC_REPRESENTATION_ITEM()
RATIONAL_B_SPLINE_SURFACE(((0.998122319569321,0.999023095875704,1.,0.994839481491404,
0.99180331349328),(0.998122319569321,0.999023095875704,1.,0.994839481491404,
0.99180331349328)))
REPRESENTATION_ITEM('')
SURFACE()
);
#2572=(
BOUNDED_SURFACE()
B_SPLINE_SURFACE(1,2,((#138540,#138541,#138542,#138543,#138544),(#138545,
#138546,#138547,#138548,#138549)),.UNSPECIFIED.,.F.,.F.,.F.)
B_SPLINE_SURFACE_WITH_KNOTS((2,2),(3,2,3),(0.710192959008319,1.),(0.159729727643096,
0.159901408087482,0.177069452526135),.UNSPECIFIED.)
GEOMETRIC_REPRESENTATION_ITEM()
RATIONAL_B_SPLINE_SURFACE(((0.990889788836284,0.990889788836284,0.990889788836284,
0.987739559362111,0.987486127973996),(0.990889788836284,0.990889788836284,
0.990889788836284,0.987739559362111,0.987486127973996)))
REPRESENTATION_ITEM('')
SURFACE()
);
#2573=(
BOUNDED_SURFACE()
B_SPLINE_SURFACE(1,2,((#138560,#138561,#138562,#138563,#138564),(#138565,
#138566,#138567,#138568,#138569)),.UNSPECIFIED.,.F.,.F.,.F.)
B_SPLINE_SURFACE_WITH_KNOTS((2,2),(3,2,3),(0.710318915639718,1.),(0.556108173865714,
0.571428571428571,0.57365435021991),.UNSPECIFIED.)
GEOMETRIC_REPRESENTATION_ITEM()
RATIONAL_B_SPLINE_SURFACE(((0.991551633675927,0.994622399056525,1.,0.999218731101516,
0.99848615229188),(0.991551633675927,0.994622399056525,1.,0.999218731101516,
0.99848615229188)))
REPRESENTATION_ITEM('')
SURFACE()
);
#2574=(
BOUNDED_SURFACE()
B_SPLINE_SURFACE(1,2,((#138586,#138587,#138588,#138589,#138590),(#138591,
#138592,#138593,#138594,#138595)),.UNSPECIFIED.,.F.,.F.,.F.)
B_SPLINE_SURFACE_WITH_KNOTS((2,2),(3,2,3),(0.710192959008343,1.),(0.159729727643021,
0.159901408087408,0.177069452526135),.UNSPECIFIED.)
GEOMETRIC_REPRESENTATION_ITEM()
RATIONAL_B_SPLINE_SURFACE(((0.990889788836311,0.990889788836311,0.990889788836311,
0.987739559362112,0.987486127973996),(0.990889788836311,0.990889788836311,
0.990889788836311,0.987739559362112,0.987486127973996)))
REPRESENTATION_ITEM('')
SURFACE()
);
#2575=(
BOUNDED_SURFACE()
B_SPLINE_SURFACE(1,2,((#138603,#138604,#138605,#138606,#138607),(#138608,
#138609,#138610,#138611,#138612)),.UNSPECIFIED.,.F.,.F.,.F.)
B_SPLINE_SURFACE_WITH_KNOTS((2,2),(3,2,3),(0.710318915639972,1.),(0.556108173865714,
0.571428571428571,0.57365435021991),.UNSPECIFIED.)
GEOMETRIC_REPRESENTATION_ITEM()
RATIONAL_B_SPLINE_SURFACE(((0.991551633675927,0.994622399056525,1.,0.999218731101516,
0.99848615229188),(0.991551633675927,0.994622399056525,1.,0.999218731101516,
0.99848615229188)))
REPRESENTATION_ITEM('')
SURFACE()
);
#2576=(
BOUNDED_SURFACE()
B_SPLINE_SURFACE(1,2,((#138629,#138630,#138631,#138632,#138633),(#138634,
#138635,#138636,#138637,#138638)),.UNSPECIFIED.,.F.,.F.,.F.)
B_SPLINE_SURFACE_WITH_KNOTS((2,2),(3,2,3),(0.710192959008338,1.),(0.159729727643096,
0.159901408087482,0.177069452526135),.UNSPECIFIED.)
GEOMETRIC_REPRESENTATION_ITEM()
RATIONAL_B_SPLINE_SURFACE(((0.990889788836284,0.990889788836284,0.990889788836284,
0.987739559362111,0.987486127973996),(0.990889788836284,0.990889788836284,
0.990889788836284,0.987739559362111,0.987486127973996)))
REPRESENTATION_ITEM('')
SURFACE()
);
#2577=(
BOUNDED_SURFACE()
B_SPLINE_SURFACE(1,2,((#138646,#138647,#138648,#138649,#138650),(#138651,
#138652,#138653,#138654,#138655)),.UNSPECIFIED.,.F.,.F.,.F.)
B_SPLINE_SURFACE_WITH_KNOTS((2,2),(3,2,3),(0.710318915639015,1.),(0.556108173865714,
0.571428571428571,0.57365435021991),.UNSPECIFIED.)
GEOMETRIC_REPRESENTATION_ITEM()
RATIONAL_B_SPLINE_SURFACE(((0.991551633675927,0.994622399056525,1.,0.999218731101516,
0.99848615229188),(0.991551633675927,0.994622399056525,1.,0.999218731101516,
0.99848615229188)))
REPRESENTATION_ITEM('')
SURFACE()
);
#2578=(
BOUNDED_SURFACE()
B_SPLINE_SURFACE(1,2,((#138672,#138673,#138674,#138675,#138676),(#138677,
#138678,#138679,#138680,#138681)),.UNSPECIFIED.,.F.,.F.,.F.)
B_SPLINE_SURFACE_WITH_KNOTS((2,2),(3,2,3),(0.710192959007381,1.),(0.159729727643019,
0.159901408087406,0.177069452526135),.UNSPECIFIED.)
GEOMETRIC_REPRESENTATION_ITEM()
RATIONAL_B_SPLINE_SURFACE(((0.990889788836312,0.990889788836312,0.990889788836312,
0.987739559362112,0.987486127973996),(0.990889788836312,0.990889788836312,
0.990889788836312,0.987739559362112,0.987486127973996)))
REPRESENTATION_ITEM('')
SURFACE()
);
#2579=(
BOUNDED_SURFACE()
B_SPLINE_SURFACE(1,2,((#138689,#138690,#138691,#138692,#138693),(#138694,
#138695,#138696,#138697,#138698)),.UNSPECIFIED.,.F.,.F.,.F.)
B_SPLINE_SURFACE_WITH_KNOTS((2,2),(3,2,3),(0.710318915639014,1.),(0.556108173865714,
0.571428571428571,0.57365435021991),.UNSPECIFIED.)
GEOMETRIC_REPRESENTATION_ITEM()
RATIONAL_B_SPLINE_SURFACE(((0.991551633675927,0.994622399056525,1.,0.999218731101516,
0.99848615229188),(0.991551633675927,0.994622399056525,1.,0.999218731101516,
0.99848615229188)))
REPRESENTATION_ITEM('')
SURFACE()
);
#2580=(
BOUNDED_SURFACE()
B_SPLINE_SURFACE(1,2,((#138715,#138716,#138717,#138718,#138719),(#138720,
#138721,#138722,#138723,#138724)),.UNSPECIFIED.,.F.,.F.,.F.)
B_SPLINE_SURFACE_WITH_KNOTS((2,2),(3,2,3),(0.710192959007375,1.),(0.159729727643019,
0.159901408087406,0.177069452526135),.UNSPECIFIED.)
GEOMETRIC_REPRESENTATION_ITEM()
RATIONAL_B_SPLINE_SURFACE(((0.990889788836312,0.990889788836312,0.990889788836312,
0.987739559362112,0.987486127973996),(0.990889788836312,0.990889788836312,
0.990889788836312,0.987739559362112,0.987486127973996)))
REPRESENTATION_ITEM('')
SURFACE()
);
#2581=(
BOUNDED_SURFACE()
B_SPLINE_SURFACE(1,2,((#138732,#138733,#138734,#138735,#138736),(#138737,
#138738,#138739,#138740,#138741)),.UNSPECIFIED.,.F.,.F.,.F.)
B_SPLINE_SURFACE_WITH_KNOTS((2,2),(3,2,3),(0.710318915639014,1.),(0.556108173865714,
0.571428571428571,0.57365435021991),.UNSPECIFIED.)
GEOMETRIC_REPRESENTATION_ITEM()
RATIONAL_B_SPLINE_SURFACE(((0.991551633675927,0.994622399056525,1.,0.999218731101516,
0.99848615229188),(0.991551633675927,0.994622399056525,1.,0.999218731101516,
0.99848615229188)))
REPRESENTATION_ITEM('')
SURFACE()
);
#2582=(
BOUNDED_SURFACE()
B_SPLINE_SURFACE(1,2,((#138758,#138759,#138760,#138761,#138762),(#138763,
#138764,#138765,#138766,#138767)),.UNSPECIFIED.,.F.,.F.,.F.)
B_SPLINE_SURFACE_WITH_KNOTS((2,2),(3,2,3),(0.710192959007376,1.),(0.159729727643096,
0.159901408087482,0.177069452526135),.UNSPECIFIED.)
GEOMETRIC_REPRESENTATION_ITEM()
RATIONAL_B_SPLINE_SURFACE(((0.990889788836284,0.990889788836284,0.990889788836284,
0.987739559362111,0.987486127973996),(0.990889788836284,0.990889788836284,
0.990889788836284,0.987739559362111,0.987486127973996)))
REPRESENTATION_ITEM('')
SURFACE()
);
#2583=(
BOUNDED_SURFACE()
B_SPLINE_SURFACE(1,2,((#138775,#138776,#138777,#138778,#138779),(#138780,
#138781,#138782,#138783,#138784)),.UNSPECIFIED.,.F.,.F.,.F.)
B_SPLINE_SURFACE_WITH_KNOTS((2,2),(3,2,3),(0.710318915638436,1.),(0.556108173865714,
0.571428571428571,0.57365435021991),.UNSPECIFIED.)
GEOMETRIC_REPRESENTATION_ITEM()
RATIONAL_B_SPLINE_SURFACE(((0.991551633675927,0.994622399056525,1.,0.999218731101516,
0.99848615229188),(0.991551633675927,0.994622399056525,1.,0.999218731101516,
0.99848615229188)))
REPRESENTATION_ITEM('')
SURFACE()
);
#2584=(
BOUNDED_SURFACE()
B_SPLINE_SURFACE(1,2,((#138801,#138802,#138803,#138804,#138805),(#138806,
#138807,#138808,#138809,#138810)),.UNSPECIFIED.,.F.,.F.,.F.)
B_SPLINE_SURFACE_WITH_KNOTS((2,2),(3,2,3),(0.710192959006793,1.),(0.159729727643019,
0.159901408087406,0.177069452526135),.UNSPECIFIED.)
GEOMETRIC_REPRESENTATION_ITEM()
RATIONAL_B_SPLINE_SURFACE(((0.990889788836311,0.990889788836311,0.990889788836311,
0.987739559362112,0.987486127973996),(0.990889788836311,0.990889788836311,
0.990889788836311,0.987739559362112,0.987486127973996)))
REPRESENTATION_ITEM('')
SURFACE()
);
#2585=(
BOUNDED_SURFACE()
B_SPLINE_SURFACE(1,2,((#138818,#138819,#138820,#138821,#138822),(#138823,
#138824,#138825,#138826,#138827)),.UNSPECIFIED.,.F.,.F.,.F.)
B_SPLINE_SURFACE_WITH_KNOTS((2,2),(3,2,3),(0.710318915639023,1.),(0.556108173865714,
0.571428571428571,0.57365435021991),.UNSPECIFIED.)
GEOMETRIC_REPRESENTATION_ITEM()
RATIONAL_B_SPLINE_SURFACE(((0.991551633675927,0.994622399056525,1.,0.999218731101516,
0.99848615229188),(0.991551633675927,0.994622399056525,1.,0.999218731101516,
0.99848615229188)))
REPRESENTATION_ITEM('')
SURFACE()
);
#2586=(
BOUNDED_SURFACE()
B_SPLINE_SURFACE(1,2,((#138844,#138845,#138846,#138847,#138848),(#138849,
#138850,#138851,#138852,#138853)),.UNSPECIFIED.,.F.,.F.,.F.)
B_SPLINE_SURFACE_WITH_KNOTS((2,2),(3,2,3),(0.710192959007382,1.),(0.159729727643096,
0.159901408087482,0.177069452526135),.UNSPECIFIED.)
GEOMETRIC_REPRESENTATION_ITEM()
RATIONAL_B_SPLINE_SURFACE(((0.990889788836284,0.990889788836284,0.990889788836284,
0.987739559362111,0.987486127973996),(0.990889788836284,0.990889788836284,
0.990889788836284,0.987739559362111,0.987486127973996)))
REPRESENTATION_ITEM('')
SURFACE()
);
#2587=(
BOUNDED_SURFACE()
B_SPLINE_SURFACE(1,2,((#138861,#138862,#138863,#138864,#138865),(#138866,
#138867,#138868,#138869,#138870)),.UNSPECIFIED.,.F.,.F.,.F.)
B_SPLINE_SURFACE_WITH_KNOTS((2,2),(3,2,3),(0.710318915638469,1.),(0.556108173865714,
0.571428571428571,0.57365435021991),.UNSPECIFIED.)
GEOMETRIC_REPRESENTATION_ITEM()
RATIONAL_B_SPLINE_SURFACE(((0.991551633675927,0.994622399056525,1.,0.999218731101516,
0.99848615229188),(0.991551633675927,0.994622399056525,1.,0.999218731101516,
0.99848615229188)))
REPRESENTATION_ITEM('')
SURFACE()
);
#2588=(
BOUNDED_SURFACE()
B_SPLINE_SURFACE(1,2,((#138887,#138888,#138889,#138890,#138891),(#138892,
#138893,#138894,#138895,#138896)),.UNSPECIFIED.,.F.,.F.,.F.)
B_SPLINE_SURFACE_WITH_KNOTS((2,2),(3,2,3),(0.710192959006827,1.),(0.159729727643096,
0.159901408087482,0.177069452526135),.UNSPECIFIED.)
GEOMETRIC_REPRESENTATION_ITEM()
RATIONAL_B_SPLINE_SURFACE(((0.990889788836284,0.990889788836284,0.990889788836284,
0.987739559362111,0.987486127973996),(0.990889788836284,0.990889788836284,
0.990889788836284,0.987739559362111,0.987486127973996)))
REPRESENTATION_ITEM('')
SURFACE()
);
#2589=(
BOUNDED_SURFACE()
B_SPLINE_SURFACE(1,2,((#138904,#138905,#138906,#138907,#138908),(#138909,
#138910,#138911,#138912,#138913)),.UNSPECIFIED.,.F.,.F.,.F.)
B_SPLINE_SURFACE_WITH_KNOTS((2,2),(3,2,3),(0.710318915638963,1.),(0.556108173865715,
0.571428571428571,0.57365435021991),.UNSPECIFIED.)
GEOMETRIC_REPRESENTATION_ITEM()
RATIONAL_B_SPLINE_SURFACE(((0.991551633675927,0.994622399056526,1.,0.999218731101516,
0.99848615229188),(0.991551633675927,0.994622399056526,1.,0.999218731101516,
0.99848615229188)))
REPRESENTATION_ITEM('')
SURFACE()
);
#2590=(
BOUNDED_SURFACE()
B_SPLINE_SURFACE(1,2,((#138930,#138931,#138932,#138933,#138934),(#138935,
#138936,#138937,#138938,#138939)),.UNSPECIFIED.,.F.,.F.,.F.)
B_SPLINE_SURFACE_WITH_KNOTS((2,2),(3,2,3),(0.710192959007322,1.),(0.15972972764302,
0.159901408087407,0.177069452526134),.UNSPECIFIED.)
GEOMETRIC_REPRESENTATION_ITEM()
RATIONAL_B_SPLINE_SURFACE(((0.990889788836311,0.990889788836311,0.990889788836311,
0.987739559362112,0.987486127973996),(0.990889788836311,0.990889788836311,
0.990889788836311,0.987739559362112,0.987486127973996)))
REPRESENTATION_ITEM('')
SURFACE()
);
#2591=(
BOUNDED_SURFACE()
B_SPLINE_SURFACE(1,2,((#138947,#138948,#138949,#138950,#138951),(#138952,
#138953,#138954,#138955,#138956)),.UNSPECIFIED.,.F.,.F.,.F.)
B_SPLINE_SURFACE_WITH_KNOTS((2,2),(3,2,3),(0.710318915638946,1.),(0.556108173865715,
0.571428571428571,0.573654350219911),.UNSPECIFIED.)
GEOMETRIC_REPRESENTATION_ITEM()
RATIONAL_B_SPLINE_SURFACE(((0.991551633675927,0.994622399056526,1.,0.999218731101516,
0.99848615229188),(0.991551633675927,0.994622399056526,1.,0.999218731101516,
0.99848615229188)))
REPRESENTATION_ITEM('')
SURFACE()
);
#2592=(
BOUNDED_SURFACE()
B_SPLINE_SURFACE(1,2,((#138973,#138974,#138975,#138976,#138977),(#138978,
#138979,#138980,#138981,#138982)),.UNSPECIFIED.,.F.,.F.,.F.)
B_SPLINE_SURFACE_WITH_KNOTS((2,2),(3,2,3),(0.710192959007309,1.),(0.159729727643095,
0.159901408087481,0.177069452526134),.UNSPECIFIED.)
GEOMETRIC_REPRESENTATION_ITEM()
RATIONAL_B_SPLINE_SURFACE(((0.990889788836284,0.990889788836284,0.990889788836284,
0.987739559362111,0.987486127973996),(0.990889788836284,0.990889788836284,
0.990889788836284,0.987739559362111,0.987486127973996)))
REPRESENTATION_ITEM('')
SURFACE()
);
#2593=(
BOUNDED_SURFACE()
B_SPLINE_SURFACE(1,2,((#138990,#138991,#138992,#138993,#138994),(#138995,
#138996,#138997,#138998,#138999)),.UNSPECIFIED.,.F.,.F.,.F.)
B_SPLINE_SURFACE_WITH_KNOTS((2,2),(3,2,3),(0.710318915638348,1.),(0.556108173865715,
0.571428571428571,0.573654350219911),.UNSPECIFIED.)
GEOMETRIC_REPRESENTATION_ITEM()
RATIONAL_B_SPLINE_SURFACE(((0.991551633675927,0.994622399056526,1.,0.999218731101516,
0.99848615229188),(0.991551633675927,0.994622399056526,1.,0.999218731101516,
0.99848615229188)))
REPRESENTATION_ITEM('')
SURFACE()
);
#2594=(
BOUNDED_SURFACE()
B_SPLINE_SURFACE(1,2,((#139016,#139017,#139018,#139019,#139020),(#139021,
#139022,#139023,#139024,#139025)),.UNSPECIFIED.,.F.,.F.,.F.)
B_SPLINE_SURFACE_WITH_KNOTS((2,2),(3,2,3),(0.710192959006703,1.),(0.159729727643095,
0.159901408087481,0.177069452526134),.UNSPECIFIED.)
GEOMETRIC_REPRESENTATION_ITEM()
RATIONAL_B_SPLINE_SURFACE(((0.990889788836284,0.990889788836284,0.990889788836284,
0.987739559362111,0.987486127973996),(0.990889788836284,0.990889788836284,
0.990889788836284,0.987739559362111,0.987486127973996)))
REPRESENTATION_ITEM('')
SURFACE()
);
#2595=(
BOUNDED_SURFACE()
B_SPLINE_SURFACE(1,2,((#139033,#139034,#139035,#139036,#139037),(#139038,
#139039,#139040,#139041,#139042)),.UNSPECIFIED.,.F.,.F.,.F.)
B_SPLINE_SURFACE_WITH_KNOTS((2,2),(3,2,3),(0.710318915638935,1.),(0.556108173865715,
0.571428571428571,0.573654350219911),.UNSPECIFIED.)
GEOMETRIC_REPRESENTATION_ITEM()
RATIONAL_B_SPLINE_SURFACE(((0.991551633675927,0.994622399056526,1.,0.999218731101516,
0.99848615229188),(0.991551633675927,0.994622399056526,1.,0.999218731101516,
0.99848615229188)))
REPRESENTATION_ITEM('')
SURFACE()
);
#2596=(
BOUNDED_SURFACE()
B_SPLINE_SURFACE(1,2,((#139059,#139060,#139061,#139062,#139063),(#139064,
#139065,#139066,#139067,#139068)),.UNSPECIFIED.,.F.,.F.,.F.)
B_SPLINE_SURFACE_WITH_KNOTS((2,2),(3,2,3),(0.710192959007288,1.),(0.159729727643018,
0.159901408087405,0.177069452526134),.UNSPECIFIED.)
GEOMETRIC_REPRESENTATION_ITEM()
RATIONAL_B_SPLINE_SURFACE(((0.990889788836312,0.990889788836312,0.990889788836312,
0.987739559362112,0.987486127973996),(0.990889788836312,0.990889788836312,
0.990889788836312,0.987739559362112,0.987486127973996)))
REPRESENTATION_ITEM('')
SURFACE()
);
#2597=(
BOUNDED_SURFACE()
B_SPLINE_SURFACE(1,2,((#139076,#139077,#139078,#139079,#139080),(#139081,
#139082,#139083,#139084,#139085)),.UNSPECIFIED.,.F.,.F.,.F.)
B_SPLINE_SURFACE_WITH_KNOTS((2,2),(3,2,3),(0.710318915638428,1.),(0.556108173865715,
0.571428571428571,0.573654350219911),.UNSPECIFIED.)
GEOMETRIC_REPRESENTATION_ITEM()
RATIONAL_B_SPLINE_SURFACE(((0.991551633675927,0.994622399056526,1.,0.999218731101516,
0.99848615229188),(0.991551633675927,0.994622399056526,1.,0.999218731101516,
0.99848615229188)))
REPRESENTATION_ITEM('')
SURFACE()
);
#2598=(
BOUNDED_SURFACE()
B_SPLINE_SURFACE(1,2,((#139102,#139103,#139104,#139105,#139106),(#139107,
#139108,#139109,#139110,#139111)),.UNSPECIFIED.,.F.,.F.,.F.)
B_SPLINE_SURFACE_WITH_KNOTS((2,2),(3,2,3),(0.710192959006786,1.),(0.159729727643095,
0.159901408087481,0.177069452526134),.UNSPECIFIED.)
GEOMETRIC_REPRESENTATION_ITEM()
RATIONAL_B_SPLINE_SURFACE(((0.990889788836284,0.990889788836284,0.990889788836284,
0.987739559362111,0.987486127973996),(0.990889788836284,0.990889788836284,
0.990889788836284,0.987739559362111,0.987486127973996)))
REPRESENTATION_ITEM('')
SURFACE()
);
#2599=(
BOUNDED_SURFACE()
B_SPLINE_SURFACE(1,2,((#139119,#139120,#139121,#139122,#139123),(#139124,
#139125,#139126,#139127,#139128)),.UNSPECIFIED.,.F.,.F.,.F.)
B_SPLINE_SURFACE_WITH_KNOTS((2,2),(3,2,3),(0.710318915638931,1.),(0.556108173865715,
0.571428571428571,0.573654350219911),.UNSPECIFIED.)
GEOMETRIC_REPRESENTATION_ITEM()
RATIONAL_B_SPLINE_SURFACE(((0.991551633675927,0.994622399056526,1.,0.999218731101516,
0.99848615229188),(0.991551633675927,0.994622399056526,1.,0.999218731101516,
0.99848615229188)))
REPRESENTATION_ITEM('')
SURFACE()
);
#2600=(
BOUNDED_SURFACE()
B_SPLINE_SURFACE(1,2,((#139136,#139137,#139138,#139139,#139140),(#139141,
#139142,#139143,#139144,#139145)),.UNSPECIFIED.,.F.,.F.,.F.)
B_SPLINE_SURFACE_WITH_KNOTS((2,2),(3,2,3),(0.710192959007286,1.),(0.159729727643018,
0.159901408087405,0.177069452526134),.UNSPECIFIED.)
GEOMETRIC_REPRESENTATION_ITEM()
RATIONAL_B_SPLINE_SURFACE(((0.990889788836312,0.990889788836312,0.990889788836312,
0.987739559362112,0.987486127973996),(0.990889788836312,0.990889788836312,
0.990889788836312,0.987739559362112,0.987486127973996)))
REPRESENTATION_ITEM('')
SURFACE()
);
#2601=(
BOUNDED_SURFACE()
B_SPLINE_SURFACE(1,2,((#139147,#139148,#139149,#139150,#139151),(#139152,
#139153,#139154,#139155,#139156)),.UNSPECIFIED.,.F.,.F.,.F.)
B_SPLINE_SURFACE_WITH_KNOTS((2,2),(3,2,3),(0.710318915638446,1.),(0.556108173865715,
0.571428571428571,0.573654350219911),.UNSPECIFIED.)
GEOMETRIC_REPRESENTATION_ITEM()
RATIONAL_B_SPLINE_SURFACE(((0.991551633675927,0.994622399056526,1.,0.999218731101516,
0.99848615229188),(0.991551633675927,0.994622399056526,1.,0.999218731101516,
0.99848615229188)))
REPRESENTATION_ITEM('')
SURFACE()
);
#2602=(
BOUNDED_SURFACE()
B_SPLINE_SURFACE(1,2,((#139173,#139174,#139175,#139176,#139177),(#139178,
#139179,#139180,#139181,#139182)),.UNSPECIFIED.,.F.,.F.,.F.)
B_SPLINE_SURFACE_WITH_KNOTS((2,2),(3,2,3),(0.710192959006802,1.),(0.15972972764302,
0.159901408087407,0.177069452526134),.UNSPECIFIED.)
GEOMETRIC_REPRESENTATION_ITEM()
RATIONAL_B_SPLINE_SURFACE(((0.990889788836311,0.990889788836311,0.990889788836311,
0.987739559362112,0.987486127973996),(0.990889788836311,0.990889788836311,
0.990889788836311,0.987739559362112,0.987486127973996)))
REPRESENTATION_ITEM('')
SURFACE()
);
#2603=(
BOUNDED_SURFACE()
B_SPLINE_SURFACE(1,2,((#139190,#139191,#139192,#139193,#139194),(#139195,
#139196,#139197,#139198,#139199)),.UNSPECIFIED.,.F.,.F.,.F.)
B_SPLINE_SURFACE_WITH_KNOTS((2,2),(3,2,3),(0.710318915638684,1.),(0.556108173865715,
0.571428571428571,0.573654350219911),.UNSPECIFIED.)
GEOMETRIC_REPRESENTATION_ITEM()
RATIONAL_B_SPLINE_SURFACE(((0.991551633675927,0.994622399056526,1.,0.999218731101516,
0.99848615229188),(0.991551633675927,0.994622399056526,1.,0.999218731101516,
0.99848615229188)))
REPRESENTATION_ITEM('')
SURFACE()
);
#2604=(
BOUNDED_SURFACE()
B_SPLINE_SURFACE(1,2,((#139216,#139217,#139218,#139219,#139220),(#139221,
#139222,#139223,#139224,#139225)),.UNSPECIFIED.,.F.,.F.,.F.)
B_SPLINE_SURFACE_WITH_KNOTS((2,2),(3,2,3),(0.710192959007044,1.),(0.15972972764302,
0.159901408087407,0.177069452526134),.UNSPECIFIED.)
GEOMETRIC_REPRESENTATION_ITEM()
RATIONAL_B_SPLINE_SURFACE(((0.990889788836311,0.990889788836311,0.990889788836311,
0.987739559362112,0.987486127973996),(0.990889788836311,0.990889788836311,
0.990889788836311,0.987739559362112,0.987486127973996)))
REPRESENTATION_ITEM('')
SURFACE()
);
#2605=(
BOUNDED_SURFACE()
B_SPLINE_SURFACE(1,2,((#139233,#139234,#139235,#139236,#139237),(#139238,
#139239,#139240,#139241,#139242)),.UNSPECIFIED.,.F.,.F.,.F.)
B_SPLINE_SURFACE_WITH_KNOTS((2,2),(3,2,3),(0.710318915637618,1.),(0.556108173865715,
0.571428571428571,0.573654350219911),.UNSPECIFIED.)
GEOMETRIC_REPRESENTATION_ITEM()
RATIONAL_B_SPLINE_SURFACE(((0.991551633675927,0.994622399056526,1.,0.999218731101516,
0.99848615229188),(0.991551633675927,0.994622399056526,1.,0.999218731101516,
0.99848615229188)))
REPRESENTATION_ITEM('')
SURFACE()
);
#2606=(
BOUNDED_SURFACE()
B_SPLINE_SURFACE(1,2,((#139259,#139260,#139261,#139262,#139263),(#139264,
#139265,#139266,#139267,#139268)),.UNSPECIFIED.,.F.,.F.,.F.)
B_SPLINE_SURFACE_WITH_KNOTS((2,2),(3,2,3),(0.710192959005978,1.),(0.159729727643095,
0.159901408087481,0.177069452526134),.UNSPECIFIED.)
GEOMETRIC_REPRESENTATION_ITEM()
RATIONAL_B_SPLINE_SURFACE(((0.990889788836284,0.990889788836284,0.990889788836284,
0.987739559362111,0.987486127973996),(0.990889788836284,0.990889788836284,
0.990889788836284,0.987739559362111,0.987486127973996)))
REPRESENTATION_ITEM('')
SURFACE()
);
#2607=(
BOUNDED_SURFACE()
B_SPLINE_SURFACE(1,2,((#139276,#139277,#139278,#139279,#139280),(#139281,
#139282,#139283,#139284,#139285)),.UNSPECIFIED.,.F.,.F.,.F.)
B_SPLINE_SURFACE_WITH_KNOTS((2,2),(3,2,3),(0.710318915638879,1.),(0.556108173865715,
0.571428571428571,0.573654350219911),.UNSPECIFIED.)
GEOMETRIC_REPRESENTATION_ITEM()
RATIONAL_B_SPLINE_SURFACE(((0.991551633675927,0.994622399056526,1.,0.999218731101516,
0.99848615229188),(0.991551633675927,0.994622399056526,1.,0.999218731101516,
0.99848615229188)))
REPRESENTATION_ITEM('')
SURFACE()
);
#2608=(
BOUNDED_SURFACE()
B_SPLINE_SURFACE(1,2,((#139302,#139303,#139304,#139305,#139306),(#139307,
#139308,#139309,#139310,#139311)),.UNSPECIFIED.,.F.,.F.,.F.)
B_SPLINE_SURFACE_WITH_KNOTS((2,2),(3,2,3),(0.710192959007236,1.),(0.159729727642845,
0.159901408087234,0.177069452526135),.UNSPECIFIED.)
GEOMETRIC_REPRESENTATION_ITEM()
RATIONAL_B_SPLINE_SURFACE(((0.990889788836375,0.990889788836375,0.990889788836375,
0.987739559362115,0.987486127973996),(0.990889788836375,0.990889788836375,
0.990889788836375,0.987739559362115,0.987486127973996)))
REPRESENTATION_ITEM('')
SURFACE()
);
#2609=(
BOUNDED_SURFACE()
B_SPLINE_SURFACE(1,2,((#139319,#139320,#139321,#139322,#139323),(#139324,
#139325,#139326,#139327,#139328)),.UNSPECIFIED.,.F.,.F.,.F.)
B_SPLINE_SURFACE_WITH_KNOTS((2,2),(3,2,3),(0.710318915639,1.),(0.556108173865715,
0.571428571428571,0.573654350219911),.UNSPECIFIED.)
GEOMETRIC_REPRESENTATION_ITEM()
RATIONAL_B_SPLINE_SURFACE(((0.991551633675927,0.994622399056526,1.,0.999218731101516,
0.99848615229188),(0.991551633675927,0.994622399056526,1.,0.999218731101516,
0.99848615229188)))
REPRESENTATION_ITEM('')
SURFACE()
);
#2610=(
BOUNDED_SURFACE()
B_SPLINE_SURFACE(1,2,((#139345,#139346,#139347,#139348,#139349),(#139350,
#139351,#139352,#139353,#139354)),.UNSPECIFIED.,.F.,.F.,.F.)
B_SPLINE_SURFACE_WITH_KNOTS((2,2),(3,2,3),(0.710192959007357,1.),(0.159729727643095,
0.159901408087481,0.177069452526134),.UNSPECIFIED.)
GEOMETRIC_REPRESENTATION_ITEM()
RATIONAL_B_SPLINE_SURFACE(((0.990889788836284,0.990889788836284,0.990889788836284,
0.987739559362111,0.987486127973996),(0.990889788836284,0.990889788836284,
0.990889788836284,0.987739559362111,0.987486127973996)))
REPRESENTATION_ITEM('')
SURFACE()
);
#2611=(
BOUNDED_SURFACE()
B_SPLINE_SURFACE(1,2,((#139362,#139363,#139364,#139365,#139366),(#139367,
#139368,#139369,#139370,#139371)),.UNSPECIFIED.,.F.,.F.,.F.)
B_SPLINE_SURFACE_WITH_KNOTS((2,2),(3,2,3),(0.710318915638369,1.),(0.556108173865716,
0.571428571428571,0.573654350219912),.UNSPECIFIED.)
GEOMETRIC_REPRESENTATION_ITEM()
RATIONAL_B_SPLINE_SURFACE(((0.991551633675927,0.994622399056526,1.,0.999218731101515,
0.998486152291879),(0.991551633675927,0.994622399056526,1.,0.999218731101515,
0.998486152291879)))
REPRESENTATION_ITEM('')
SURFACE()
);
#2612=(
BOUNDED_SURFACE()
B_SPLINE_SURFACE(1,2,((#139388,#139389,#139390,#139391,#139392),(#139393,
#139394,#139395,#139396,#139397)),.UNSPECIFIED.,.F.,.F.,.F.)
B_SPLINE_SURFACE_WITH_KNOTS((2,2),(3,2,3),(0.710192959006723,1.),(0.159729727643025,
0.159901408087412,0.177069452526135),.UNSPECIFIED.)
GEOMETRIC_REPRESENTATION_ITEM()
RATIONAL_B_SPLINE_SURFACE(((0.99088978883631,0.99088978883631,0.99088978883631,
0.987739559362112,0.987486127973996),(0.99088978883631,0.99088978883631,
0.99088978883631,0.987739559362112,0.987486127973996)))
REPRESENTATION_ITEM('')
SURFACE()
);
#2613=(
BOUNDED_SURFACE()
B_SPLINE_SURFACE(1,2,((#139405,#139406,#139407,#139408,#139409),(#139410,
#139411,#139412,#139413,#139414)),.UNSPECIFIED.,.F.,.F.,.F.)
B_SPLINE_SURFACE_WITH_KNOTS((2,2),(3,2,3),(0.710318915639743,1.),(0.556108173865715,
0.571428571428571,0.573654350219911),.UNSPECIFIED.)
GEOMETRIC_REPRESENTATION_ITEM()
RATIONAL_B_SPLINE_SURFACE(((0.991551633675927,0.994622399056526,1.,0.999218731101516,
0.99848615229188),(0.991551633675927,0.994622399056526,1.,0.999218731101516,
0.99848615229188)))
REPRESENTATION_ITEM('')
SURFACE()
);
#2614=(
BOUNDED_SURFACE()
B_SPLINE_SURFACE(1,2,((#139431,#139432,#139433,#139434,#139435),(#139436,
#139437,#139438,#139439,#139440)),.UNSPECIFIED.,.F.,.F.,.F.)
B_SPLINE_SURFACE_WITH_KNOTS((2,2),(3,2,3),(0.710192959008268,1.),(0.159729727643095,
0.159901408087481,0.177069452526134),.UNSPECIFIED.)
GEOMETRIC_REPRESENTATION_ITEM()
RATIONAL_B_SPLINE_SURFACE(((0.990889788836284,0.990889788836284,0.990889788836284,
0.987739559362111,0.987486127973996),(0.990889788836284,0.990889788836284,
0.990889788836284,0.987739559362111,0.987486127973996)))
REPRESENTATION_ITEM('')
SURFACE()
);
#2615=(
BOUNDED_SURFACE()
B_SPLINE_SURFACE(1,2,((#139448,#139449,#139450,#139451,#139452),(#139453,
#139454,#139455,#139456,#139457)),.UNSPECIFIED.,.F.,.F.,.F.)
B_SPLINE_SURFACE_WITH_KNOTS((2,2),(3,2,3),(0.710318915638758,1.),(0.556108173865715,
0.571428571428571,0.573654350219911),.UNSPECIFIED.)
GEOMETRIC_REPRESENTATION_ITEM()
RATIONAL_B_SPLINE_SURFACE(((0.991551633675927,0.994622399056526,1.,0.999218731101516,
0.99848615229188),(0.991551633675927,0.994622399056526,1.,0.999218731101516,
0.99848615229188)))
REPRESENTATION_ITEM('')
SURFACE()
);
#2616=(
BOUNDED_SURFACE()
B_SPLINE_SURFACE(1,2,((#139474,#139475,#139476,#139477,#139478),(#139479,
#139480,#139481,#139482,#139483)),.UNSPECIFIED.,.F.,.F.,.F.)
B_SPLINE_SURFACE_WITH_KNOTS((2,2),(3,2,3),(0.710192959007121,1.),(0.159729727643082,
0.159901408087468,0.177069452526134),.UNSPECIFIED.)
GEOMETRIC_REPRESENTATION_ITEM()
RATIONAL_B_SPLINE_SURFACE(((0.990889788836289,0.990889788836289,0.990889788836289,
0.987739559362111,0.987486127973996),(0.990889788836289,0.990889788836289,
0.990889788836289,0.987739559362111,0.987486127973996)))
REPRESENTATION_ITEM('')
SURFACE()
);
#2617=(
BOUNDED_SURFACE()
B_SPLINE_SURFACE(1,2,((#139491,#139492,#139493,#139494,#139495),(#139496,
#139497,#139498,#139499,#139500)),.UNSPECIFIED.,.F.,.F.,.F.)
B_SPLINE_SURFACE_WITH_KNOTS((2,2),(3,2,3),(0.710318915638947,1.),(0.556108173865715,
0.571428571428571,0.573654350219911),.UNSPECIFIED.)
GEOMETRIC_REPRESENTATION_ITEM()
RATIONAL_B_SPLINE_SURFACE(((0.991551633675927,0.994622399056526,1.,0.999218731101516,
0.99848615229188),(0.991551633675927,0.994622399056526,1.,0.999218731101516,
0.99848615229188)))
REPRESENTATION_ITEM('')
SURFACE()
);
#2618=(
BOUNDED_SURFACE()
B_SPLINE_SURFACE(1,2,((#139517,#139518,#139519,#139520,#139521),(#139522,
#139523,#139524,#139525,#139526)),.UNSPECIFIED.,.F.,.F.,.F.)
B_SPLINE_SURFACE_WITH_KNOTS((2,2),(3,2,3),(0.710192959007308,1.),(0.159729727643095,
0.159901408087481,0.177069452526134),.UNSPECIFIED.)
GEOMETRIC_REPRESENTATION_ITEM()
RATIONAL_B_SPLINE_SURFACE(((0.990889788836284,0.990889788836284,0.990889788836284,
0.987739559362111,0.987486127973996),(0.990889788836284,0.990889788836284,
0.990889788836284,0.987739559362111,0.987486127973996)))
REPRESENTATION_ITEM('')
SURFACE()
);
#2619=(
BOUNDED_SURFACE()
B_SPLINE_SURFACE(1,2,((#139534,#139535,#139536,#139537,#139538),(#139539,
#139540,#139541,#139542,#139543)),.UNSPECIFIED.,.F.,.F.,.F.)
B_SPLINE_SURFACE_WITH_KNOTS((2,2),(3,2,3),(0.710318915637903,1.),(0.556108173865716,
0.571428571428571,0.573654350219911),.UNSPECIFIED.)
GEOMETRIC_REPRESENTATION_ITEM()
RATIONAL_B_SPLINE_SURFACE(((0.991551633675927,0.994622399056526,1.,0.999218731101516,
0.99848615229188),(0.991551633675927,0.994622399056526,1.,0.999218731101516,
0.99848615229188)))
REPRESENTATION_ITEM('')
SURFACE()
);
#2620=(
BOUNDED_SURFACE()
B_SPLINE_SURFACE(1,2,((#139560,#139561,#139562,#139563,#139564),(#139565,
#139566,#139567,#139568,#139569)),.UNSPECIFIED.,.F.,.F.,.F.)
B_SPLINE_SURFACE_WITH_KNOTS((2,2),(3,2,3),(0.710192959006264,1.),(0.15972972764307,
0.159901408087457,0.177069452526135),.UNSPECIFIED.)
GEOMETRIC_REPRESENTATION_ITEM()
RATIONAL_B_SPLINE_SURFACE(((0.990889788836293,0.990889788836293,0.990889788836293,
0.987739559362111,0.987486127973996),(0.990889788836293,0.990889788836293,
0.990889788836293,0.987739559362111,0.987486127973996)))
REPRESENTATION_ITEM('')
SURFACE()
);
#2621=(
BOUNDED_SURFACE()
B_SPLINE_SURFACE(1,2,((#139577,#139578,#139579,#139580,#139581),(#139582,
#139583,#139584,#139585,#139586)),.UNSPECIFIED.,.F.,.F.,.F.)
B_SPLINE_SURFACE_WITH_KNOTS((2,2),(3,2,3),(0.710318915639728,1.),(0.556108173865715,
0.571428571428571,0.573654350219911),.UNSPECIFIED.)
GEOMETRIC_REPRESENTATION_ITEM()
RATIONAL_B_SPLINE_SURFACE(((0.991551633675927,0.994622399056526,1.,0.999218731101516,
0.99848615229188),(0.991551633675927,0.994622399056526,1.,0.999218731101516,
0.99848615229188)))
REPRESENTATION_ITEM('')
SURFACE()
);
#2622=(
BOUNDED_SURFACE()
B_SPLINE_SURFACE(1,2,((#139603,#139604,#139605,#139606,#139607),(#139608,
#139609,#139610,#139611,#139612)),.UNSPECIFIED.,.F.,.F.,.F.)
B_SPLINE_SURFACE_WITH_KNOTS((2,2),(3,2,3),(0.710192959008098,1.),(0.159729727643095,
0.159901408087481,0.177069452526134),.UNSPECIFIED.)
GEOMETRIC_REPRESENTATION_ITEM()
RATIONAL_B_SPLINE_SURFACE(((0.990889788836284,0.990889788836284,0.990889788836284,
0.987739559362111,0.987486127973996),(0.990889788836284,0.990889788836284,
0.990889788836284,0.987739559362111,0.987486127973996)))
REPRESENTATION_ITEM('')
SURFACE()
);
#2623=(
BOUNDED_SURFACE()
B_SPLINE_SURFACE(1,2,((#139620,#139621,#139622,#139623,#139624),(#139625,
#139626,#139627,#139628,#139629)),.UNSPECIFIED.,.F.,.F.,.F.)
B_SPLINE_SURFACE_WITH_KNOTS((2,2),(3,2,3),(0.71031891563859,1.),(0.556108173865715,
0.571428571428571,0.573654350219927),.UNSPECIFIED.)
GEOMETRIC_REPRESENTATION_ITEM()
RATIONAL_B_SPLINE_SURFACE(((0.991551633675927,0.994622399056526,1.,0.99921873110151,
0.998486152291869),(0.991551633675927,0.994622399056526,1.,0.99921873110151,
0.998486152291869)))
REPRESENTATION_ITEM('')
SURFACE()
);
#2624=(
BOUNDED_SURFACE()
B_SPLINE_SURFACE(1,2,((#139646,#139647,#139648,#139649,#139650),(#139651,
#139652,#139653,#139654,#139655)),.UNSPECIFIED.,.F.,.F.,.F.)
B_SPLINE_SURFACE_WITH_KNOTS((2,2),(3,2,3),(0.710192959006948,1.),(0.159729727643096,
0.159901408087482,0.177069452526134),.UNSPECIFIED.)
GEOMETRIC_REPRESENTATION_ITEM()
RATIONAL_B_SPLINE_SURFACE(((0.990889788836284,0.990889788836284,0.990889788836284,
0.987739559362111,0.987486127973996),(0.990889788836284,0.990889788836284,
0.990889788836284,0.987739559362111,0.987486127973996)))
REPRESENTATION_ITEM('')
SURFACE()
);
#2625=(
BOUNDED_SURFACE()
B_SPLINE_SURFACE(1,2,((#139663,#139664,#139665,#139666,#139667),(#139668,
#139669,#139670,#139671,#139672)),.UNSPECIFIED.,.F.,.F.,.F.)
B_SPLINE_SURFACE_WITH_KNOTS((2,2),(3,2,3),(0.710318915639458,1.),(0.556108173865714,
0.571428571428571,0.57365435021991),.UNSPECIFIED.)
GEOMETRIC_REPRESENTATION_ITEM()
RATIONAL_B_SPLINE_SURFACE(((0.991551633675927,0.994622399056525,1.,0.999218731101516,
0.99848615229188),(0.991551633675927,0.994622399056525,1.,0.999218731101516,
0.99848615229188)))
REPRESENTATION_ITEM('')
SURFACE()
);
#2626=(
BOUNDED_SURFACE()
B_SPLINE_SURFACE(1,2,((#139689,#139690,#139691,#139692,#139693),(#139694,
#139695,#139696,#139697,#139698)),.UNSPECIFIED.,.F.,.F.,.F.)
B_SPLINE_SURFACE_WITH_KNOTS((2,2),(3,2,3),(0.710192959008439,1.),(0.159729727643019,
0.159901408087406,0.177069452526135),.UNSPECIFIED.)
GEOMETRIC_REPRESENTATION_ITEM()
RATIONAL_B_SPLINE_SURFACE(((0.990889788836312,0.990889788836312,0.990889788836312,
0.987739559362112,0.987486127973996),(0.990889788836312,0.990889788836312,
0.990889788836312,0.987739559362112,0.987486127973996)))
REPRESENTATION_ITEM('')
SURFACE()
);
#2627=(
BOUNDED_SURFACE()
B_SPLINE_SURFACE(1,2,((#139706,#139707,#139708,#139709,#139710),(#139711,
#139712,#139713,#139714,#139715)),.UNSPECIFIED.,.F.,.F.,.F.)
B_SPLINE_SURFACE_WITH_KNOTS((2,2),(3,2,3),(0.710318915639948,1.),(0.556108173865714,
0.571428571428571,0.57365435021991),.UNSPECIFIED.)
GEOMETRIC_REPRESENTATION_ITEM()
RATIONAL_B_SPLINE_SURFACE(((0.991551633675927,0.994622399056525,1.,0.999218731101516,
0.99848615229188),(0.991551633675927,0.994622399056525,1.,0.999218731101516,
0.99848615229188)))
REPRESENTATION_ITEM('')
SURFACE()
);
#2628=(
BOUNDED_SURFACE()
B_SPLINE_SURFACE(1,2,((#139732,#139733,#139734,#139735,#139736),(#139737,
#139738,#139739,#139740,#139741)),.UNSPECIFIED.,.F.,.F.,.F.)
B_SPLINE_SURFACE_WITH_KNOTS((2,2),(3,2,3),(0.710192959008305,1.),(0.159729727643019,
0.159901408087406,0.177069452526135),.UNSPECIFIED.)
GEOMETRIC_REPRESENTATION_ITEM()
RATIONAL_B_SPLINE_SURFACE(((0.990889788836311,0.990889788836311,0.990889788836311,
0.987739559362112,0.987486127973996),(0.990889788836311,0.990889788836311,
0.990889788836311,0.987739559362112,0.987486127973996)))
REPRESENTATION_ITEM('')
SURFACE()
);
#2629=(
BOUNDED_SURFACE()
B_SPLINE_SURFACE(1,2,((#139761,#139762,#139763,#139764,#139765),(#139766,
#139767,#139768,#139769,#139770)),.UNSPECIFIED.,.F.,.F.,.F.)
B_SPLINE_SURFACE_WITH_KNOTS((2,2),(3,2,3),(0.710318915639714,1.),(0.556108173865714,
0.571428571428571,0.57365435021991),.UNSPECIFIED.)
GEOMETRIC_REPRESENTATION_ITEM()
RATIONAL_B_SPLINE_SURFACE(((0.991551633675927,0.994622399056525,1.,0.999218731101516,
0.99848615229188),(0.991551633675927,0.994622399056525,1.,0.999218731101516,
0.99848615229188)))
REPRESENTATION_ITEM('')
SURFACE()
);
#2630=(
BOUNDED_SURFACE()
B_SPLINE_SURFACE(1,2,((#139772,#139773,#139774,#139775,#139776),(#139777,
#139778,#139779,#139780,#139781)),.UNSPECIFIED.,.F.,.F.,.F.)
B_SPLINE_SURFACE_WITH_KNOTS((2,2),(3,2,3),(0.70971070997379,1.),(0.194028469417326,
0.211502584834065,0.21211079066313),.UNSPECIFIED.)
GEOMETRIC_REPRESENTATION_ITEM()
RATIONAL_B_SPLINE_SURFACE(((0.989812124691679,0.992466718773227,0.998122319569323,
0.998122319569323,0.998122319569323),(0.989812124691679,0.992466718773227,
0.998122319569323,0.998122319569323,0.998122319569323)))
REPRESENTATION_ITEM('')
SURFACE()
);
#2631=(
BOUNDED_SURFACE()
B_SPLINE_SURFACE(1,2,((#139790,#139791,#139792),(#139793,#139794,#139795)),
 .UNSPECIFIED.,.F.,.F.,.F.)
B_SPLINE_SURFACE_WITH_KNOTS((2,2),(3,3),(0.710192959008376,1.),(0.52191752982614,
0.539102123117534),.UNSPECIFIED.)
GEOMETRIC_REPRESENTATION_ITEM()
RATIONAL_B_SPLINE_SURFACE(((0.989334769731189,0.987004571835916,0.987576759359605),
(0.989334769731189,0.987004571835916,0.987576759359605)))
REPRESENTATION_ITEM('')
SURFACE()
);
#2632=(
BOUNDED_SURFACE()
B_SPLINE_SURFACE(1,2,((#139804,#139805,#139806,#139807,#139808),(#139809,
#139810,#139811,#139812,#139813)),.UNSPECIFIED.,.F.,.F.,.F.)
B_SPLINE_SURFACE_WITH_KNOTS((2,2),(3,2,3),(0.709710709962227,1.),(0.194028469417326,
0.211502584834064,0.212110790674692),.UNSPECIFIED.)
GEOMETRIC_REPRESENTATION_ITEM()
RATIONAL_B_SPLINE_SURFACE(((0.989812124691679,0.992466718773227,0.998122319569322,
0.998122319569323,0.998122319569323),(0.989812124691679,0.992466718773227,
0.998122319569322,0.998122319569322,0.998122319569322)))
REPRESENTATION_ITEM('')
SURFACE()
);
#2633=(
BOUNDED_SURFACE()
B_SPLINE_SURFACE(1,2,((#139815,#139816,#139817),(#139818,#139819,#139820)),
 .UNSPECIFIED.,.F.,.F.,.F.)
B_SPLINE_SURFACE_WITH_KNOTS((2,2),(3,3),(0.710192959008442,1.),(0.521917529826125,
0.539102123117535),.UNSPECIFIED.)
GEOMETRIC_REPRESENTATION_ITEM()
RATIONAL_B_SPLINE_SURFACE(((0.989334769731193,0.987004571835915,0.987576759359605),
(0.989334769731193,0.987004571835915,0.987576759359605)))
REPRESENTATION_ITEM('')
SURFACE()
);
#2634=(
BOUNDED_SURFACE()
B_SPLINE_SURFACE(1,2,((#139829,#139830,#139831,#139832,#139833),(#139834,
#139835,#139836,#139837,#139838)),.UNSPECIFIED.,.F.,.F.,.F.)
B_SPLINE_SURFACE_WITH_KNOTS((2,2),(3,2,3),(0.709710709965086,1.),(0.194028469417325,
0.211502584834064,0.21211079067188),.UNSPECIFIED.)
GEOMETRIC_REPRESENTATION_ITEM()
RATIONAL_B_SPLINE_SURFACE(((0.989812124691679,0.992466718773227,0.998122319569322,
0.998122319569322,0.998122319569322),(0.989812124691679,0.992466718773227,
0.998122319569322,0.998122319569322,0.998122319569322)))
REPRESENTATION_ITEM('')
SURFACE()
);
#2635=(
BOUNDED_SURFACE()
B_SPLINE_SURFACE(1,2,((#139840,#139841,#139842),(#139843,#139844,#139845)),
 .UNSPECIFIED.,.F.,.F.,.F.)
B_SPLINE_SURFACE_WITH_KNOTS((2,2),(3,3),(0.71019295900844,1.),(0.521917529826117,
0.539102123117535),.UNSPECIFIED.)
GEOMETRIC_REPRESENTATION_ITEM()
RATIONAL_B_SPLINE_SURFACE(((0.989334769731195,0.987004571835915,0.987576759359605),
(0.989334769731195,0.987004571835915,0.987576759359605)))
REPRESENTATION_ITEM('')
SURFACE()
);
#2636=(
BOUNDED_SURFACE()
B_SPLINE_SURFACE(1,2,((#139854,#139855,#139856,#139857,#139858),(#139859,
#139860,#139861,#139862,#139863)),.UNSPECIFIED.,.F.,.F.,.F.)
B_SPLINE_SURFACE_WITH_KNOTS((2,2),(3,2,3),(0.70971070997195,1.),(0.194028469417325,
0.211502584834064,0.212110790665034),.UNSPECIFIED.)
GEOMETRIC_REPRESENTATION_ITEM()
RATIONAL_B_SPLINE_SURFACE(((0.989812124691679,0.992466718773227,0.998122319569322,
0.998122319569322,0.998122319569322),(0.989812124691679,0.992466718773227,
0.998122319569322,0.998122319569322,0.998122319569322)))
REPRESENTATION_ITEM('')
SURFACE()
);
#2637=(
BOUNDED_SURFACE()
B_SPLINE_SURFACE(1,2,((#139865,#139866,#139867),(#139868,#139869,#139870)),
 .UNSPECIFIED.,.F.,.F.,.F.)
B_SPLINE_SURFACE_WITH_KNOTS((2,2),(3,3),(0.710192959008441,1.),(0.521917529826141,
0.539102123117535),.UNSPECIFIED.)
GEOMETRIC_REPRESENTATION_ITEM()
RATIONAL_B_SPLINE_SURFACE(((0.989334769731189,0.987004571835916,0.987576759359605),
(0.989334769731189,0.987004571835916,0.987576759359605)))
REPRESENTATION_ITEM('')
SURFACE()
);
#2638=(
BOUNDED_SURFACE()
B_SPLINE_SURFACE(1,2,((#139879,#139880,#139881,#139882,#139883),(#139884,
#139885,#139886,#139887,#139888)),.UNSPECIFIED.,.F.,.F.,.F.)
B_SPLINE_SURFACE_WITH_KNOTS((2,2),(3,2,3),(0.709710709990175,1.),(0.194028469417325,
0.211502584834064,0.212110790646804),.UNSPECIFIED.)
GEOMETRIC_REPRESENTATION_ITEM()
RATIONAL_B_SPLINE_SURFACE(((0.989812124691679,0.992466718773227,0.998122319569322,
0.998122319569322,0.998122319569322),(0.989812124691679,0.992466718773227,
0.998122319569322,0.998122319569322,0.998122319569322)))
REPRESENTATION_ITEM('')
SURFACE()
);
#2639=(
BOUNDED_SURFACE()
B_SPLINE_SURFACE(1,2,((#139890,#139891,#139892),(#139893,#139894,#139895)),
 .UNSPECIFIED.,.F.,.F.,.F.)
B_SPLINE_SURFACE_WITH_KNOTS((2,2),(3,3),(0.710192959008441,1.),(0.52191752982614,
0.539102123117535),.UNSPECIFIED.)
GEOMETRIC_REPRESENTATION_ITEM()
RATIONAL_B_SPLINE_SURFACE(((0.989334769731189,0.987004571835916,0.987576759359605),
(0.989334769731189,0.987004571835916,0.987576759359605)))
REPRESENTATION_ITEM('')
SURFACE()
);
#2640=(
BOUNDED_SURFACE()
B_SPLINE_SURFACE(1,2,((#139904,#139905,#139906,#139907,#139908),(#139909,
#139910,#139911,#139912,#139913)),.UNSPECIFIED.,.F.,.F.,.F.)
B_SPLINE_SURFACE_WITH_KNOTS((2,2),(3,2,3),(0.709710709979902,1.),(0.194028469417325,
0.211502584834064,0.21211079065708),.UNSPECIFIED.)
GEOMETRIC_REPRESENTATION_ITEM()
RATIONAL_B_SPLINE_SURFACE(((0.989812124691679,0.992466718773227,0.998122319569322,
0.998122319569322,0.998122319569322),(0.989812124691679,0.992466718773227,
0.998122319569322,0.998122319569322,0.998122319569322)))
REPRESENTATION_ITEM('')
SURFACE()
);
#2641=(
BOUNDED_SURFACE()
B_SPLINE_SURFACE(1,2,((#139915,#139916,#139917),(#139918,#139919,#139920)),
 .UNSPECIFIED.,.F.,.F.,.F.)
B_SPLINE_SURFACE_WITH_KNOTS((2,2),(3,3),(0.710192959008441,1.),(0.521917529826141,
0.539102123117535),.UNSPECIFIED.)
GEOMETRIC_REPRESENTATION_ITEM()
RATIONAL_B_SPLINE_SURFACE(((0.989334769731189,0.987004571835916,0.987576759359605),
(0.989334769731189,0.987004571835916,0.987576759359605)))
REPRESENTATION_ITEM('')
SURFACE()
);
#2642=(
BOUNDED_SURFACE()
B_SPLINE_SURFACE(1,2,((#139929,#139930,#139931,#139932,#139933),(#139934,
#139935,#139936,#139937,#139938)),.UNSPECIFIED.,.F.,.F.,.F.)
B_SPLINE_SURFACE_WITH_KNOTS((2,2),(3,2,3),(0.709710709965924,1.),(0.194028469417325,
0.211502584834064,0.21211079067106),.UNSPECIFIED.)
GEOMETRIC_REPRESENTATION_ITEM()
RATIONAL_B_SPLINE_SURFACE(((0.989812124691679,0.992466718773227,0.998122319569322,
0.998122319569322,0.998122319569322),(0.989812124691679,0.992466718773227,
0.998122319569322,0.998122319569322,0.998122319569322)))
REPRESENTATION_ITEM('')
SURFACE()
);
#2643=(
BOUNDED_SURFACE()
B_SPLINE_SURFACE(1,2,((#139940,#139941,#139942),(#139943,#139944,#139945)),
 .UNSPECIFIED.,.F.,.F.,.F.)
B_SPLINE_SURFACE_WITH_KNOTS((2,2),(3,3),(0.710192959008442,1.),(0.521917529826113,
0.539102123117535),.UNSPECIFIED.)
GEOMETRIC_REPRESENTATION_ITEM()
RATIONAL_B_SPLINE_SURFACE(((0.989334769731196,0.987004571835915,0.987576759359605),
(0.989334769731196,0.987004571835915,0.987576759359605)))
REPRESENTATION_ITEM('')
SURFACE()
);
#2644=(
BOUNDED_SURFACE()
B_SPLINE_SURFACE(1,2,((#139954,#139955,#139956,#139957,#139958),(#139959,
#139960,#139961,#139962,#139963)),.UNSPECIFIED.,.F.,.F.,.F.)
B_SPLINE_SURFACE_WITH_KNOTS((2,2),(3,2,3),(0.710051238894138,1.),(0.194028469417325,
0.211502584834064,0.211770261742845),.UNSPECIFIED.)
GEOMETRIC_REPRESENTATION_ITEM()
RATIONAL_B_SPLINE_SURFACE(((0.989812124691679,0.992466718773227,0.998122319569322,
0.998122319569322,0.998122319569322),(0.989812124691679,0.992466718773227,
0.998122319569322,0.998122319569322,0.998122319569322)))
REPRESENTATION_ITEM('')
SURFACE()
);
#2645=(
BOUNDED_SURFACE()
B_SPLINE_SURFACE(1,2,((#139965,#139966,#139967),(#139968,#139969,#139970)),
 .UNSPECIFIED.,.F.,.F.,.F.)
B_SPLINE_SURFACE_WITH_KNOTS((2,2),(3,3),(0.710192959008442,1.),(0.521917529826141,
0.539102123117535),.UNSPECIFIED.)
GEOMETRIC_REPRESENTATION_ITEM()
RATIONAL_B_SPLINE_SURFACE(((0.989334769731189,0.987004571835916,0.987576759359605),
(0.989334769731189,0.987004571835916,0.987576759359605)))
REPRESENTATION_ITEM('')
SURFACE()
);
#2646=(
BOUNDED_SURFACE()
B_SPLINE_SURFACE(1,2,((#139979,#139980,#139981,#139982,#139983),(#139984,
#139985,#139986,#139987,#139988)),.UNSPECIFIED.,.F.,.F.,.F.)
B_SPLINE_SURFACE_WITH_KNOTS((2,2),(3,2,3),(0.709710709982408,1.),(0.194028469417325,
0.211502584834064,0.212110790654572),.UNSPECIFIED.)
GEOMETRIC_REPRESENTATION_ITEM()
RATIONAL_B_SPLINE_SURFACE(((0.989812124691679,0.992466718773227,0.998122319569322,
0.998122319569322,0.998122319569322),(0.989812124691679,0.992466718773227,
0.998122319569322,0.998122319569322,0.998122319569322)))
REPRESENTATION_ITEM('')
SURFACE()
);
#2647=(
BOUNDED_SURFACE()
B_SPLINE_SURFACE(1,2,((#139990,#139991,#139992),(#139993,#139994,#139995)),
 .UNSPECIFIED.,.F.,.F.,.F.)
B_SPLINE_SURFACE_WITH_KNOTS((2,2),(3,3),(0.710192959008443,1.),(0.521917529826141,
0.539102123117535),.UNSPECIFIED.)
GEOMETRIC_REPRESENTATION_ITEM()
RATIONAL_B_SPLINE_SURFACE(((0.989334769731189,0.987004571835916,0.987576759359605),
(0.989334769731189,0.987004571835916,0.987576759359605)))
REPRESENTATION_ITEM('')
SURFACE()
);
#2648=(
BOUNDED_SURFACE()
B_SPLINE_SURFACE(1,2,((#140004,#140005,#140006,#140007,#140008),(#140009,
#140010,#140011,#140012,#140013)),.UNSPECIFIED.,.F.,.F.,.F.)
B_SPLINE_SURFACE_WITH_KNOTS((2,2),(3,2,3),(0.709710709998254,1.),(0.194028469417325,
0.211502584834064,0.212110790638721),.UNSPECIFIED.)
GEOMETRIC_REPRESENTATION_ITEM()
RATIONAL_B_SPLINE_SURFACE(((0.989812124691679,0.992466718773227,0.998122319569322,
0.998122319569322,0.998122319569322),(0.989812124691679,0.992466718773227,
0.998122319569322,0.998122319569322,0.998122319569322)))
REPRESENTATION_ITEM('')
SURFACE()
);
#2649=(
BOUNDED_SURFACE()
B_SPLINE_SURFACE(1,2,((#140015,#140016,#140017),(#140018,#140019,#140020)),
 .UNSPECIFIED.,.F.,.F.,.F.)
B_SPLINE_SURFACE_WITH_KNOTS((2,2),(3,3),(0.710192959008444,1.),(0.521917529826137,
0.539102123117535),.UNSPECIFIED.)
GEOMETRIC_REPRESENTATION_ITEM()
RATIONAL_B_SPLINE_SURFACE(((0.98933476973119,0.987004571835916,0.987576759359605),
(0.98933476973119,0.987004571835916,0.987576759359605)))
REPRESENTATION_ITEM('')
SURFACE()
);
#2650=(
BOUNDED_SURFACE()
B_SPLINE_SURFACE(1,2,((#140029,#140030,#140031,#140032,#140033),(#140034,
#140035,#140036,#140037,#140038)),.UNSPECIFIED.,.F.,.F.,.F.)
B_SPLINE_SURFACE_WITH_KNOTS((2,2),(3,2,3),(0.709710709967905,1.),(0.194028469417325,
0.211502584834064,0.212110790669077),.UNSPECIFIED.)
GEOMETRIC_REPRESENTATION_ITEM()
RATIONAL_B_SPLINE_SURFACE(((0.989812124691679,0.992466718773227,0.998122319569322,
0.998122319569322,0.998122319569322),(0.989812124691679,0.992466718773227,
0.998122319569322,0.998122319569322,0.998122319569322)))
REPRESENTATION_ITEM('')
SURFACE()
);
#2651=(
BOUNDED_SURFACE()
B_SPLINE_SURFACE(1,2,((#140040,#140041,#140042),(#140043,#140044,#140045)),
 .UNSPECIFIED.,.F.,.F.,.F.)
B_SPLINE_SURFACE_WITH_KNOTS((2,2),(3,3),(0.71019295900844,1.),(0.521917529826141,
0.539102123117535),.UNSPECIFIED.)
GEOMETRIC_REPRESENTATION_ITEM()
RATIONAL_B_SPLINE_SURFACE(((0.989334769731189,0.987004571835916,0.987576759359605),
(0.989334769731189,0.987004571835916,0.987576759359605)))
REPRESENTATION_ITEM('')
SURFACE()
);
#2652=(
BOUNDED_SURFACE()
B_SPLINE_SURFACE(1,2,((#140054,#140055,#140056,#140057,#140058),(#140059,
#140060,#140061,#140062,#140063)),.UNSPECIFIED.,.F.,.F.,.F.)
B_SPLINE_SURFACE_WITH_KNOTS((2,2),(3,2,3),(0.709710709971499,1.),(0.194028469417325,
0.211502584834064,0.212110790665475),.UNSPECIFIED.)
GEOMETRIC_REPRESENTATION_ITEM()
RATIONAL_B_SPLINE_SURFACE(((0.989812124691679,0.992466718773227,0.998122319569322,
0.998122319569322,0.998122319569322),(0.989812124691679,0.992466718773227,
0.998122319569322,0.998122319569322,0.998122319569322)))
REPRESENTATION_ITEM('')
SURFACE()
);
#2653=(
BOUNDED_SURFACE()
B_SPLINE_SURFACE(1,2,((#140065,#140066,#140067),(#140068,#140069,#140070)),
 .UNSPECIFIED.,.F.,.F.,.F.)
B_SPLINE_SURFACE_WITH_KNOTS((2,2),(3,3),(0.710192959008441,1.),(0.521917529826102,
0.539102123117535),.UNSPECIFIED.)
GEOMETRIC_REPRESENTATION_ITEM()
RATIONAL_B_SPLINE_SURFACE(((0.989334769731199,0.987004571835914,0.987576759359605),
(0.989334769731199,0.987004571835914,0.987576759359605)))
REPRESENTATION_ITEM('')
SURFACE()
);
#2654=(
BOUNDED_SURFACE()
B_SPLINE_SURFACE(1,2,((#140079,#140080,#140081,#140082,#140083),(#140084,
#140085,#140086,#140087,#140088)),.UNSPECIFIED.,.F.,.F.,.F.)
B_SPLINE_SURFACE_WITH_KNOTS((2,2),(3,2,3),(0.709710709957041,1.),(0.194028469417325,
0.211502584834064,0.212110790679937),.UNSPECIFIED.)
GEOMETRIC_REPRESENTATION_ITEM()
RATIONAL_B_SPLINE_SURFACE(((0.989812124691679,0.992466718773227,0.998122319569322,
0.998122319569322,0.998122319569322),(0.989812124691679,0.992466718773227,
0.998122319569322,0.998122319569322,0.998122319569322)))
REPRESENTATION_ITEM('')
SURFACE()
);
#2655=(
BOUNDED_SURFACE()
B_SPLINE_SURFACE(1,2,((#140090,#140091,#140092),(#140093,#140094,#140095)),
 .UNSPECIFIED.,.F.,.F.,.F.)
B_SPLINE_SURFACE_WITH_KNOTS((2,2),(3,3),(0.710192959008445,1.),(0.521917529826141,
0.539102123117535),.UNSPECIFIED.)
GEOMETRIC_REPRESENTATION_ITEM()
RATIONAL_B_SPLINE_SURFACE(((0.989334769731189,0.987004571835916,0.987576759359605),
(0.989334769731189,0.987004571835916,0.987576759359605)))
REPRESENTATION_ITEM('')
SURFACE()
);
#2656=(
BOUNDED_SURFACE()
B_SPLINE_SURFACE(1,2,((#140104,#140105,#140106,#140107,#140108),(#140109,
#140110,#140111,#140112,#140113)),.UNSPECIFIED.,.F.,.F.,.F.)
B_SPLINE_SURFACE_WITH_KNOTS((2,2),(3,2,3),(0.70971070996417,1.),(0.194028469417325,
0.211502584834064,0.212110790672805),.UNSPECIFIED.)
GEOMETRIC_REPRESENTATION_ITEM()
RATIONAL_B_SPLINE_SURFACE(((0.989812124691679,0.992466718773227,0.998122319569322,
0.998122319569322,0.998122319569322),(0.989812124691679,0.992466718773227,
0.998122319569322,0.998122319569322,0.998122319569322)))
REPRESENTATION_ITEM('')
SURFACE()
);
#2657=(
BOUNDED_SURFACE()
B_SPLINE_SURFACE(1,2,((#140115,#140116,#140117),(#140118,#140119,#140120)),
 .UNSPECIFIED.,.F.,.F.,.F.)
B_SPLINE_SURFACE_WITH_KNOTS((2,2),(3,3),(0.710192959008445,1.),(0.521917529826141,
0.539102123117535),.UNSPECIFIED.)
GEOMETRIC_REPRESENTATION_ITEM()
RATIONAL_B_SPLINE_SURFACE(((0.989334769731189,0.987004571835916,0.987576759359605),
(0.989334769731189,0.987004571835916,0.987576759359605)))
REPRESENTATION_ITEM('')
SURFACE()
);
#2658=(
BOUNDED_SURFACE()
B_SPLINE_SURFACE(1,2,((#140129,#140130,#140131,#140132,#140133),(#140134,
#140135,#140136,#140137,#140138)),.UNSPECIFIED.,.F.,.F.,.F.)
B_SPLINE_SURFACE_WITH_KNOTS((2,2),(3,2,3),(0.709710709982169,1.),(0.194028469417325,
0.211502584834064,0.212110790654813),.UNSPECIFIED.)
GEOMETRIC_REPRESENTATION_ITEM()
RATIONAL_B_SPLINE_SURFACE(((0.989812124691679,0.992466718773227,0.998122319569322,
0.998122319569322,0.998122319569322),(0.989812124691679,0.992466718773227,
0.998122319569322,0.998122319569322,0.998122319569322)))
REPRESENTATION_ITEM('')
SURFACE()
);
#2659=(
BOUNDED_SURFACE()
B_SPLINE_SURFACE(1,2,((#140140,#140141,#140142),(#140143,#140144,#140145)),
 .UNSPECIFIED.,.F.,.F.,.F.)
B_SPLINE_SURFACE_WITH_KNOTS((2,2),(3,3),(0.710192959008441,1.),(0.521917529826049,
0.539102123117536),.UNSPECIFIED.)
GEOMETRIC_REPRESENTATION_ITEM()
RATIONAL_B_SPLINE_SURFACE(((0.989334769731214,0.987004571835913,0.987576759359605),
(0.989334769731214,0.987004571835913,0.987576759359605)))
REPRESENTATION_ITEM('')
SURFACE()
);
#2660=(
BOUNDED_SURFACE()
B_SPLINE_SURFACE(1,2,((#140154,#140155,#140156,#140157,#140158),(#140159,
#140160,#140161,#140162,#140163)),.UNSPECIFIED.,.F.,.F.,.F.)
B_SPLINE_SURFACE_WITH_KNOTS((2,2),(3,2,3),(0.709710709986515,1.),(0.194028469417325,
0.211502584834064,0.212110790650462),.UNSPECIFIED.)
GEOMETRIC_REPRESENTATION_ITEM()
RATIONAL_B_SPLINE_SURFACE(((0.989812124691679,0.992466718773227,0.998122319569322,
0.998122319569322,0.998122319569322),(0.989812124691679,0.992466718773227,
0.998122319569322,0.998122319569322,0.998122319569322)))
REPRESENTATION_ITEM('')
SURFACE()
);
#2661=(
BOUNDED_SURFACE()
B_SPLINE_SURFACE(1,2,((#140165,#140166,#140167),(#140168,#140169,#140170)),
 .UNSPECIFIED.,.F.,.F.,.F.)
B_SPLINE_SURFACE_WITH_KNOTS((2,2),(3,3),(0.71019295900844,1.),(0.521917529825981,
0.539102123117536),.UNSPECIFIED.)
GEOMETRIC_REPRESENTATION_ITEM()
RATIONAL_B_SPLINE_SURFACE(((0.989334769731232,0.98700457183591,0.987576759359605),
(0.989334769731232,0.98700457183591,0.987576759359605)))
REPRESENTATION_ITEM('')
SURFACE()
);
#2662=(
BOUNDED_SURFACE()
B_SPLINE_SURFACE(1,2,((#140179,#140180,#140181,#140182,#140183),(#140184,
#140185,#140186,#140187,#140188)),.UNSPECIFIED.,.F.,.F.,.F.)
B_SPLINE_SURFACE_WITH_KNOTS((2,2),(3,2,3),(0.709710709987791,1.),(0.194028469417325,
0.211502584834064,0.212110790649188),.UNSPECIFIED.)
GEOMETRIC_REPRESENTATION_ITEM()
RATIONAL_B_SPLINE_SURFACE(((0.989812124691679,0.992466718773227,0.998122319569322,
0.998122319569322,0.998122319569322),(0.989812124691679,0.992466718773227,
0.998122319569322,0.998122319569322,0.998122319569322)))
REPRESENTATION_ITEM('')
SURFACE()
);
#2663=(
BOUNDED_SURFACE()
B_SPLINE_SURFACE(1,2,((#140190,#140191,#140192),(#140193,#140194,#140195)),
 .UNSPECIFIED.,.F.,.F.,.F.)
B_SPLINE_SURFACE_WITH_KNOTS((2,2),(3,3),(0.710192959008445,1.),(0.521917529826041,
0.539102123117536),.UNSPECIFIED.)
GEOMETRIC_REPRESENTATION_ITEM()
RATIONAL_B_SPLINE_SURFACE(((0.989334769731216,0.987004571835912,0.987576759359605),
(0.989334769731216,0.987004571835912,0.987576759359605)))
REPRESENTATION_ITEM('')
SURFACE()
);
#2664=(
BOUNDED_SURFACE()
B_SPLINE_SURFACE(1,2,((#140204,#140205,#140206,#140207,#140208),(#140209,
#140210,#140211,#140212,#140213)),.UNSPECIFIED.,.F.,.F.,.F.)
B_SPLINE_SURFACE_WITH_KNOTS((2,2),(3,2,3),(0.709710709992596,1.),(0.194028469417325,
0.211502584834064,0.212110790644383),.UNSPECIFIED.)
GEOMETRIC_REPRESENTATION_ITEM()
RATIONAL_B_SPLINE_SURFACE(((0.989812124691679,0.992466718773227,0.998122319569322,
0.998122319569323,0.998122319569323),(0.989812124691679,0.992466718773227,
0.998122319569322,0.998122319569322,0.998122319569322)))
REPRESENTATION_ITEM('')
SURFACE()
);
#2665=(
BOUNDED_SURFACE()
B_SPLINE_SURFACE(1,2,((#140215,#140216,#140217),(#140218,#140219,#140220)),
 .UNSPECIFIED.,.F.,.F.,.F.)
B_SPLINE_SURFACE_WITH_KNOTS((2,2),(3,3),(0.710192959008442,1.),(0.521917529826013,
0.539102123117536),.UNSPECIFIED.)
GEOMETRIC_REPRESENTATION_ITEM()
RATIONAL_B_SPLINE_SURFACE(((0.989334769731223,0.987004571835911,0.987576759359605),
(0.989334769731223,0.987004571835911,0.987576759359605)))
REPRESENTATION_ITEM('')
SURFACE()
);
#2666=(
BOUNDED_SURFACE()
B_SPLINE_SURFACE(1,2,((#140229,#140230,#140231,#140232,#140233),(#140234,
#140235,#140236,#140237,#140238)),.UNSPECIFIED.,.F.,.F.,.F.)
B_SPLINE_SURFACE_WITH_KNOTS((2,2),(3,2,3),(0.709710709982975,1.),(0.194028469417325,
0.211502584834064,0.212110790654003),.UNSPECIFIED.)
GEOMETRIC_REPRESENTATION_ITEM()
RATIONAL_B_SPLINE_SURFACE(((0.989812124691679,0.992466718773227,0.998122319569322,
0.998122319569323,0.998122319569323),(0.989812124691679,0.992466718773227,
0.998122319569322,0.998122319569322,0.998122319569322)))
REPRESENTATION_ITEM('')
SURFACE()
);
#2667=(
BOUNDED_SURFACE()
B_SPLINE_SURFACE(1,2,((#140240,#140241,#140242),(#140243,#140244,#140245)),
 .UNSPECIFIED.,.F.,.F.,.F.)
B_SPLINE_SURFACE_WITH_KNOTS((2,2),(3,3),(0.710192959008441,1.),(0.521917529825751,
0.539102123117537),.UNSPECIFIED.)
GEOMETRIC_REPRESENTATION_ITEM()
RATIONAL_B_SPLINE_SURFACE(((0.989334769731294,0.987004571835902,0.987576759359605),
(0.989334769731294,0.987004571835902,0.987576759359605)))
REPRESENTATION_ITEM('')
SURFACE()
);
#2668=(
BOUNDED_SURFACE()
B_SPLINE_SURFACE(1,2,((#140254,#140255,#140256,#140257,#140258),(#140259,
#140260,#140261,#140262,#140263)),.UNSPECIFIED.,.F.,.F.,.F.)
B_SPLINE_SURFACE_WITH_KNOTS((2,2),(3,2,3),(0.709710709986856,1.),(0.194028469417325,
0.211502584834064,0.212110790650128),.UNSPECIFIED.)
GEOMETRIC_REPRESENTATION_ITEM()
RATIONAL_B_SPLINE_SURFACE(((0.989812124691679,0.992466718773227,0.998122319569322,
0.998122319569322,0.998122319569322),(0.989812124691679,0.992466718773227,
0.998122319569322,0.998122319569322,0.998122319569322)))
REPRESENTATION_ITEM('')
SURFACE()
);
#2669=(
BOUNDED_SURFACE()
B_SPLINE_SURFACE(1,2,((#140265,#140266,#140267),(#140268,#140269,#140270)),
 .UNSPECIFIED.,.F.,.F.,.F.)
B_SPLINE_SURFACE_WITH_KNOTS((2,2),(3,3),(0.710192959008443,1.),(0.521917529826001,
0.539102123117536),.UNSPECIFIED.)
GEOMETRIC_REPRESENTATION_ITEM()
RATIONAL_B_SPLINE_SURFACE(((0.989334769731227,0.987004571835911,0.987576759359605),
(0.989334769731227,0.987004571835911,0.987576759359605)))
REPRESENTATION_ITEM('')
SURFACE()
);
#2670=(
BOUNDED_SURFACE()
B_SPLINE_SURFACE(1,2,((#140279,#140280,#140281,#140282,#140283),(#140284,
#140285,#140286,#140287,#140288)),.UNSPECIFIED.,.F.,.F.,.F.)
B_SPLINE_SURFACE_WITH_KNOTS((2,2),(3,2,3),(0.709710709984816,1.),(0.194028469417325,
0.211502584834064,0.212110790643416),.UNSPECIFIED.)
GEOMETRIC_REPRESENTATION_ITEM()
RATIONAL_B_SPLINE_SURFACE(((0.989812124691679,0.992466718773227,0.998122319569322,
0.998122319569322,0.998122319569322),(0.989812124691679,0.992466718773227,
0.998122319569322,0.998122319569322,0.998122319569322)))
REPRESENTATION_ITEM('')
SURFACE()
);
#2671=(
BOUNDED_SURFACE()
B_SPLINE_SURFACE(1,2,((#140290,#140291,#140292),(#140293,#140294,#140295)),
 .UNSPECIFIED.,.F.,.F.,.F.)
B_SPLINE_SURFACE_WITH_KNOTS((2,2),(3,3),(0.710192959008051,1.),(0.521917529826138,
0.539102123117534),.UNSPECIFIED.)
GEOMETRIC_REPRESENTATION_ITEM()
RATIONAL_B_SPLINE_SURFACE(((0.98933476973119,0.987004571835916,0.987576759359605),
(0.98933476973119,0.987004571835916,0.987576759359605)))
REPRESENTATION_ITEM('')
SURFACE()
);
#2672=(
BOUNDED_SURFACE()
B_SPLINE_SURFACE(1,2,((#140304,#140305,#140306,#140307,#140308),(#140309,
#140310,#140311,#140312,#140313)),.UNSPECIFIED.,.F.,.F.,.F.)
B_SPLINE_SURFACE_WITH_KNOTS((2,2),(3,2,3),(0.709710709980223,1.),(0.194028469417326,
0.211502584834066,0.212110790656374),.UNSPECIFIED.)
GEOMETRIC_REPRESENTATION_ITEM()
RATIONAL_B_SPLINE_SURFACE(((0.989812124691679,0.992466718773228,0.998122319569323,
0.998122319569323,0.998122319569323),(0.989812124691679,0.992466718773228,
0.998122319569323,0.998122319569323,0.998122319569323)))
REPRESENTATION_ITEM('')
SURFACE()
);
#2673=(
BOUNDED_SURFACE()
B_SPLINE_SURFACE(1,2,((#140315,#140316,#140317),(#140318,#140319,#140320)),
 .UNSPECIFIED.,.F.,.F.,.F.)
B_SPLINE_SURFACE_WITH_KNOTS((2,2),(3,3),(0.710192959006369,1.),(0.521917529826136,
0.539102123117534),.UNSPECIFIED.)
GEOMETRIC_REPRESENTATION_ITEM()
RATIONAL_B_SPLINE_SURFACE(((0.98933476973119,0.987004571835916,0.987576759359605),
(0.98933476973119,0.987004571835916,0.987576759359605)))
REPRESENTATION_ITEM('')
SURFACE()
);
#2674=(
BOUNDED_SURFACE()
B_SPLINE_SURFACE(1,2,((#140329,#140330,#140331,#140332,#140333),(#140334,
#140335,#140336,#140337,#140338)),.UNSPECIFIED.,.F.,.F.,.F.)
B_SPLINE_SURFACE_WITH_KNOTS((2,2),(3,2,3),(0.709710709983031,1.),(0.194028469417326,
0.211502584834067,0.212110790652154),.UNSPECIFIED.)
GEOMETRIC_REPRESENTATION_ITEM()
RATIONAL_B_SPLINE_SURFACE(((0.989812124691679,0.992466718773228,0.998122319569324,
0.998122319569324,0.998122319569324),(0.989812124691679,0.992466718773228,
0.998122319569324,0.998122319569324,0.998122319569324)))
REPRESENTATION_ITEM('')
SURFACE()
);
#2675=(
BOUNDED_SURFACE()
B_SPLINE_SURFACE(1,2,((#140340,#140341,#140342),(#140343,#140344,#140345)),
 .UNSPECIFIED.,.F.,.F.,.F.)
B_SPLINE_SURFACE_WITH_KNOTS((2,2),(3,3),(0.710192959007972,1.),(0.52191752982614,
0.539102123117534),.UNSPECIFIED.)
GEOMETRIC_REPRESENTATION_ITEM()
RATIONAL_B_SPLINE_SURFACE(((0.989334769731189,0.987004571835916,0.987576759359604),
(0.989334769731189,0.987004571835916,0.987576759359605)))
REPRESENTATION_ITEM('')
SURFACE()
);
#2676=(
BOUNDED_SURFACE()
B_SPLINE_SURFACE(1,2,((#140354,#140355,#140356,#140357,#140358),(#140359,
#140360,#140361,#140362,#140363)),.UNSPECIFIED.,.F.,.F.,.F.)
B_SPLINE_SURFACE_WITH_KNOTS((2,2),(3,2,3),(0.709710709977382,1.),(0.194028469417326,
0.211502584834065,0.212110790659135),.UNSPECIFIED.)
GEOMETRIC_REPRESENTATION_ITEM()
RATIONAL_B_SPLINE_SURFACE(((0.989812124691679,0.992466718773227,0.998122319569323,
0.998122319569323,0.998122319569323),(0.989812124691679,0.992466718773227,
0.998122319569323,0.998122319569323,0.998122319569323)))
REPRESENTATION_ITEM('')
SURFACE()
);
#2677=(
BOUNDED_SURFACE()
B_SPLINE_SURFACE(1,2,((#140365,#140366,#140367),(#140368,#140369,#140370)),
 .UNSPECIFIED.,.F.,.F.,.F.)
B_SPLINE_SURFACE_WITH_KNOTS((2,2),(3,3),(0.710192959008356,1.),(0.52191752982614,
0.539102123117534),.UNSPECIFIED.)
GEOMETRIC_REPRESENTATION_ITEM()
RATIONAL_B_SPLINE_SURFACE(((0.989334769731189,0.987004571835916,0.987576759359605),
(0.989334769731189,0.987004571835916,0.987576759359605)))
REPRESENTATION_ITEM('')
SURFACE()
);
#2678=(
BOUNDED_SURFACE()
B_SPLINE_SURFACE(1,2,((#140379,#140380,#140381,#140382,#140383),(#140384,
#140385,#140386,#140387,#140388)),.UNSPECIFIED.,.F.,.F.,.F.)
B_SPLINE_SURFACE_WITH_KNOTS((2,2),(3,2,3),(0.709710709982804,1.),(0.194028469417326,
0.211502584834067,0.212110790654097),.UNSPECIFIED.)
GEOMETRIC_REPRESENTATION_ITEM()
RATIONAL_B_SPLINE_SURFACE(((0.989812124691679,0.992466718773228,0.998122319569324,
0.998122319569324,0.998122319569324),(0.989812124691679,0.992466718773228,
0.998122319569324,0.998122319569324,0.998122319569324)))
REPRESENTATION_ITEM('')
SURFACE()
);
#2679=(
BOUNDED_SURFACE()
B_SPLINE_SURFACE(1,2,((#140390,#140391,#140392),(#140393,#140394,#140395)),
 .UNSPECIFIED.,.F.,.F.,.F.)
B_SPLINE_SURFACE_WITH_KNOTS((2,2),(3,3),(0.71019295900836,1.),(0.521917529826139,
0.539102123117534),.UNSPECIFIED.)
GEOMETRIC_REPRESENTATION_ITEM()
RATIONAL_B_SPLINE_SURFACE(((0.989334769731189,0.987004571835916,0.987576759359605),
(0.989334769731189,0.987004571835916,0.987576759359605)))
REPRESENTATION_ITEM('')
SURFACE()
);
#2680=(
BOUNDED_SURFACE()
B_SPLINE_SURFACE(1,2,((#140404,#140405,#140406,#140407,#140408),(#140409,
#140410,#140411,#140412,#140413)),.UNSPECIFIED.,.F.,.F.,.F.)
B_SPLINE_SURFACE_WITH_KNOTS((2,2),(3,2,3),(0.709710709971706,1.),(0.194028469417326,
0.211502584834067,0.212110790665193),.UNSPECIFIED.)
GEOMETRIC_REPRESENTATION_ITEM()
RATIONAL_B_SPLINE_SURFACE(((0.989812124691679,0.992466718773228,0.998122319569324,
0.998122319569324,0.998122319569324),(0.989812124691679,0.992466718773228,
0.998122319569324,0.998122319569324,0.998122319569324)))
REPRESENTATION_ITEM('')
SURFACE()
);
#2681=(
BOUNDED_SURFACE()
B_SPLINE_SURFACE(1,2,((#140415,#140416,#140417),(#140418,#140419,#140420)),
 .UNSPECIFIED.,.F.,.F.,.F.)
B_SPLINE_SURFACE_WITH_KNOTS((2,2),(3,3),(0.710192959008365,1.),(0.52191752982614,
0.539102123117534),.UNSPECIFIED.)
GEOMETRIC_REPRESENTATION_ITEM()
RATIONAL_B_SPLINE_SURFACE(((0.989334769731189,0.987004571835916,0.987576759359605),
(0.989334769731189,0.987004571835916,0.987576759359605)))
REPRESENTATION_ITEM('')
SURFACE()
);
#2682=(
BOUNDED_SURFACE()
B_SPLINE_SURFACE(1,2,((#140429,#140430,#140431,#140432,#140433),(#140434,
#140435,#140436,#140437,#140438)),.UNSPECIFIED.,.F.,.F.,.F.)
B_SPLINE_SURFACE_WITH_KNOTS((2,2),(3,2,3),(0.709710709972218,1.),(0.194028469417326,
0.211502584834069,0.212110790664693),.UNSPECIFIED.)
GEOMETRIC_REPRESENTATION_ITEM()
RATIONAL_B_SPLINE_SURFACE(((0.989812124691679,0.992466718773228,0.998122319569325,
0.998122319569325,0.998122319569325),(0.989812124691679,0.992466718773228,
0.998122319569325,0.998122319569325,0.998122319569325)))
REPRESENTATION_ITEM('')
SURFACE()
);
#2683=(
BOUNDED_SURFACE()
B_SPLINE_SURFACE(1,2,((#140440,#140441,#140442),(#140443,#140444,#140445)),
 .UNSPECIFIED.,.F.,.F.,.F.)
B_SPLINE_SURFACE_WITH_KNOTS((2,2),(3,3),(0.710192959008044,1.),(0.52191752982614,
0.539102123117534),.UNSPECIFIED.)
GEOMETRIC_REPRESENTATION_ITEM()
RATIONAL_B_SPLINE_SURFACE(((0.989334769731189,0.987004571835916,0.987576759359605),
(0.989334769731189,0.987004571835916,0.987576759359605)))
REPRESENTATION_ITEM('')
SURFACE()
);
#2684=(
BOUNDED_SURFACE()
B_SPLINE_SURFACE(1,2,((#140454,#140455,#140456,#140457,#140458),(#140459,
#140460,#140461,#140462,#140463)),.UNSPECIFIED.,.F.,.F.,.F.)
B_SPLINE_SURFACE_WITH_KNOTS((2,2),(3,2,3),(0.709710709979372,1.),(0.194028469417326,
0.211502584834065,0.212110790657219),.UNSPECIFIED.)
GEOMETRIC_REPRESENTATION_ITEM()
RATIONAL_B_SPLINE_SURFACE(((0.989812124691679,0.992466718773227,0.998122319569323,
0.998122319569323,0.998122319569323),(0.989812124691679,0.992466718773227,
0.998122319569323,0.998122319569323,0.998122319569323)))
REPRESENTATION_ITEM('')
SURFACE()
);
#2685=(
BOUNDED_SURFACE()
B_SPLINE_SURFACE(1,2,((#140465,#140466,#140467),(#140468,#140469,#140470)),
 .UNSPECIFIED.,.F.,.F.,.F.)
B_SPLINE_SURFACE_WITH_KNOTS((2,2),(3,3),(0.710192959008388,1.),(0.52191752982614,
0.539102123117534),.UNSPECIFIED.)
GEOMETRIC_REPRESENTATION_ITEM()
RATIONAL_B_SPLINE_SURFACE(((0.989334769731189,0.987004571835916,0.987576759359605),
(0.989334769731189,0.987004571835916,0.987576759359605)))
REPRESENTATION_ITEM('')
SURFACE()
);
#2686=(
BOUNDED_SURFACE()
B_SPLINE_SURFACE(1,2,((#140479,#140480,#140481,#140482,#140483),(#140484,
#140485,#140486,#140487,#140488)),.UNSPECIFIED.,.F.,.F.,.F.)
B_SPLINE_SURFACE_WITH_KNOTS((2,2),(3,2,3),(0.709710709969892,1.),(0.194028469417326,
0.211502584834065,0.212110790667046),.UNSPECIFIED.)
GEOMETRIC_REPRESENTATION_ITEM()
RATIONAL_B_SPLINE_SURFACE(((0.989812124691679,0.992466718773227,0.998122319569323,
0.998122319569323,0.998122319569323),(0.989812124691679,0.992466718773227,
0.998122319569323,0.998122319569323,0.998122319569323)))
REPRESENTATION_ITEM('')
SURFACE()
);
#2687=(
BOUNDED_SURFACE()
B_SPLINE_SURFACE(1,2,((#140490,#140491,#140492),(#140493,#140494,#140495)),
 .UNSPECIFIED.,.F.,.F.,.F.)
B_SPLINE_SURFACE_WITH_KNOTS((2,2),(3,3),(0.710192959008377,1.),(0.521917529826137,
0.539102123117534),.UNSPECIFIED.)
GEOMETRIC_REPRESENTATION_ITEM()
RATIONAL_B_SPLINE_SURFACE(((0.98933476973119,0.987004571835916,0.987576759359605),
(0.98933476973119,0.987004571835916,0.987576759359605)))
REPRESENTATION_ITEM('')
SURFACE()
);
#2688=(
BOUNDED_SURFACE()
B_SPLINE_SURFACE(1,2,((#140497,#140498,#140499,#140500,#140501),(#140502,
#140503,#140504,#140505,#140506)),.UNSPECIFIED.,.F.,.F.,.F.)
B_SPLINE_SURFACE_WITH_KNOTS((2,2),(3,2,3),(0.,0.289807040991683),(0.573480748819789,
0.57365435021991,0.591014490232052),.UNSPECIFIED.)
GEOMETRIC_REPRESENTATION_ITEM()
RATIONAL_B_SPLINE_SURFACE(((0.99848615229188,0.99848615229188,0.99848615229188,
0.992772345172012,0.990020524139833),(0.99848615229188,0.99848615229188,
0.99848615229188,0.992772345172012,0.990020524139833)))
REPRESENTATION_ITEM('')
SURFACE()
);
#2689=(
BOUNDED_SURFACE()
B_SPLINE_SURFACE(1,2,((#140515,#140516,#140517,#140518,#140519),(#140520,
#140521,#140522,#140523,#140524)),.UNSPECIFIED.,.F.,.F.,.F.)
B_SPLINE_SURFACE_WITH_KNOTS((2,2),(3,2,3),(0.,0.289681084360264),(0.142474614281368,
0.142857142857143,0.159901408087482),.UNSPECIFIED.)
GEOMETRIC_REPRESENTATION_ITEM()
RATIONAL_B_SPLINE_SURFACE(((0.999732896029238,0.999865728939373,1.,0.994017305594881,
0.990889788836284),(0.999732896029238,0.999865728939373,1.,0.994017305594881,
0.990889788836284)))
REPRESENTATION_ITEM('')
SURFACE()
);
#2690=(
BOUNDED_SURFACE()
B_SPLINE_SURFACE(1,2,((#140533,#140534,#140535,#140536,#140537),(#140538,
#140539,#140540,#140541,#140542)),.UNSPECIFIED.,.F.,.F.,.F.)
B_SPLINE_SURFACE_WITH_KNOTS((2,2),(3,2,3),(0.,0.289807040991656),(0.573480748819709,
0.573654350219831,0.591014490232052),.UNSPECIFIED.)
GEOMETRIC_REPRESENTATION_ITEM()
RATIONAL_B_SPLINE_SURFACE(((0.998486152291932,0.998486152291932,0.998486152291932,
0.992772345172024,0.990020524139833),(0.998486152291932,0.998486152291932,
0.998486152291932,0.992772345172024,0.990020524139833)))
REPRESENTATION_ITEM('')
SURFACE()
);
#2691=(
BOUNDED_SURFACE()
B_SPLINE_SURFACE(1,2,((#140544,#140545,#140546,#140547,#140548),(#140549,
#140550,#140551,#140552,#140553)),.UNSPECIFIED.,.F.,.F.,.F.)
B_SPLINE_SURFACE_WITH_KNOTS((2,2),(3,2,3),(0.,0.289681084359915),(0.142474614281368,
0.142857142857143,0.159901408087482),.UNSPECIFIED.)
GEOMETRIC_REPRESENTATION_ITEM()
RATIONAL_B_SPLINE_SURFACE(((0.999732896029238,0.999865728939373,1.,0.994017305594881,
0.990889788836284),(0.999732896029238,0.999865728939373,1.,0.994017305594881,
0.990889788836284)))
REPRESENTATION_ITEM('')
SURFACE()
);
#2692=(
BOUNDED_SURFACE()
B_SPLINE_SURFACE(1,2,((#140562,#140563,#140564,#140565,#140566),(#140567,
#140568,#140569,#140570,#140571)),.UNSPECIFIED.,.F.,.F.,.F.)
B_SPLINE_SURFACE_WITH_KNOTS((2,2),(3,2,3),(0.,0.289807040991664),(0.573480748819789,
0.57365435021991,0.591014490232052),.UNSPECIFIED.)
GEOMETRIC_REPRESENTATION_ITEM()
RATIONAL_B_SPLINE_SURFACE(((0.99848615229188,0.99848615229188,0.99848615229188,
0.992772345172011,0.990020524139833),(0.99848615229188,0.99848615229188,
0.99848615229188,0.992772345172011,0.990020524139833)))
REPRESENTATION_ITEM('')
SURFACE()
);
#2693=(
BOUNDED_SURFACE()
B_SPLINE_SURFACE(1,2,((#140573,#140574,#140575,#140576,#140577),(#140578,
#140579,#140580,#140581,#140582)),.UNSPECIFIED.,.F.,.F.,.F.)
B_SPLINE_SURFACE_WITH_KNOTS((2,2),(3,2,3),(0.,0.289681084359918),(0.142474614281368,
0.142857142857143,0.159901408087482),.UNSPECIFIED.)
GEOMETRIC_REPRESENTATION_ITEM()
RATIONAL_B_SPLINE_SURFACE(((0.999732896029238,0.999865728939373,1.,0.994017305594881,
0.990889788836284),(0.999732896029238,0.999865728939373,1.,0.994017305594881,
0.990889788836284)))
REPRESENTATION_ITEM('')
SURFACE()
);
#2694=(
BOUNDED_SURFACE()
B_SPLINE_SURFACE(1,2,((#140591,#140592,#140593,#140594,#140595),(#140596,
#140597,#140598,#140599,#140600)),.UNSPECIFIED.,.F.,.F.,.F.)
B_SPLINE_SURFACE_WITH_KNOTS((2,2),(3,2,3),(0.,0.289807040992624),(0.573480748819707,
0.573654350219829,0.591014490232052),.UNSPECIFIED.)
GEOMETRIC_REPRESENTATION_ITEM()
RATIONAL_B_SPLINE_SURFACE(((0.998486152291933,0.998486152291933,0.998486152291933,
0.992772345172024,0.990020524139833),(0.998486152291933,0.998486152291933,
0.998486152291933,0.992772345172024,0.990020524139833)))
REPRESENTATION_ITEM('')
SURFACE()
);
#2695=(
BOUNDED_SURFACE()
B_SPLINE_SURFACE(1,2,((#140602,#140603,#140604,#140605,#140606),(#140607,
#140608,#140609,#140610,#140611)),.UNSPECIFIED.,.F.,.F.,.F.)
B_SPLINE_SURFACE_WITH_KNOTS((2,2),(3,2,3),(0.,0.289681084360269),(0.142474614281368,
0.142857142857143,0.159901408087482),.UNSPECIFIED.)
GEOMETRIC_REPRESENTATION_ITEM()
RATIONAL_B_SPLINE_SURFACE(((0.999732896029238,0.999865728939373,1.,0.994017305594881,
0.990889788836284),(0.999732896029238,0.999865728939373,1.,0.994017305594881,
0.990889788836284)))
REPRESENTATION_ITEM('')
SURFACE()
);
#2696=(
BOUNDED_SURFACE()
B_SPLINE_SURFACE(1,2,((#140620,#140621,#140622,#140623,#140624),(#140625,
#140626,#140627,#140628,#140629)),.UNSPECIFIED.,.F.,.F.,.F.)
B_SPLINE_SURFACE_WITH_KNOTS((2,2),(3,2,3),(0.,0.289807040992624),(0.573480748819707,
0.573654350219829,0.591014490232052),.UNSPECIFIED.)
GEOMETRIC_REPRESENTATION_ITEM()
RATIONAL_B_SPLINE_SURFACE(((0.998486152291934,0.998486152291934,0.998486152291934,
0.992772345172024,0.990020524139833),(0.998486152291934,0.998486152291934,
0.998486152291934,0.992772345172024,0.990020524139833)))
REPRESENTATION_ITEM('')
SURFACE()
);
#2697=(
BOUNDED_SURFACE()
B_SPLINE_SURFACE(1,2,((#140631,#140632,#140633,#140634,#140635),(#140636,
#140637,#140638,#140639,#140640),(#140641,#140642,#140643,#140644,#140645)),
 .UNSPECIFIED.,.F.,.F.,.F.)
B_SPLINE_SURFACE_WITH_KNOTS((2,1,2),(3,2,3),(-0.00289681084359923,0.,0.289681084359923),
(0.142474614281368,0.142857142857143,0.159901408087482),.UNSPECIFIED.)
GEOMETRIC_REPRESENTATION_ITEM()
RATIONAL_B_SPLINE_SURFACE(((0.999732896029238,0.999865728939373,1.,0.994017305594881,
0.990889788836284),(0.999732896029238,0.999865728939373,1.,0.994017305594881,
0.990889788836284),(0.999732896029238,0.999865728939373,1.,0.994017305594881,
0.990889788836284)))
REPRESENTATION_ITEM('')
SURFACE()
);
#2698=(
BOUNDED_SURFACE()
B_SPLINE_SURFACE(1,2,((#140654,#140655,#140656,#140657,#140658),(#140659,
#140660,#140661,#140662,#140663)),.UNSPECIFIED.,.F.,.F.,.F.)
B_SPLINE_SURFACE_WITH_KNOTS((2,2),(3,2,3),(0.,0.289807040992624),(0.573480748819789,
0.57365435021991,0.591014490232052),.UNSPECIFIED.)
GEOMETRIC_REPRESENTATION_ITEM()
RATIONAL_B_SPLINE_SURFACE(((0.99848615229188,0.99848615229188,0.99848615229188,
0.992772345172012,0.990020524139833),(0.99848615229188,0.99848615229188,
0.99848615229188,0.992772345172012,0.990020524139833)))
REPRESENTATION_ITEM('')
SURFACE()
);
#2699=(
BOUNDED_SURFACE()
B_SPLINE_SURFACE(1,2,((#140665,#140666,#140667,#140668,#140669),(#140670,
#140671,#140672,#140673,#140674)),.UNSPECIFIED.,.F.,.F.,.F.)
B_SPLINE_SURFACE_WITH_KNOTS((2,2),(3,2,3),(0.,0.28968108435992),(0.142474614281368,
0.142857142857143,0.159901408087482),.UNSPECIFIED.)
GEOMETRIC_REPRESENTATION_ITEM()
RATIONAL_B_SPLINE_SURFACE(((0.999732896029238,0.999865728939373,1.,0.994017305594881,
0.990889788836284),(0.999732896029238,0.999865728939373,1.,0.994017305594881,
0.990889788836284)))
REPRESENTATION_ITEM('')
SURFACE()
);
#2700=(
BOUNDED_SURFACE()
B_SPLINE_SURFACE(1,2,((#140683,#140684,#140685,#140686,#140687),(#140688,
#140689,#140690,#140691,#140692)),.UNSPECIFIED.,.F.,.F.,.F.)
B_SPLINE_SURFACE_WITH_KNOTS((2,2),(3,2,3),(0.,0.289807040993208),(0.573480748819707,
0.573654350219829,0.591014490232052),.UNSPECIFIED.)
GEOMETRIC_REPRESENTATION_ITEM()
RATIONAL_B_SPLINE_SURFACE(((0.998486152291933,0.998486152291933,0.998486152291933,
0.992772345172024,0.990020524139833),(0.998486152291933,0.998486152291933,
0.998486152291933,0.992772345172024,0.990020524139833)))
REPRESENTATION_ITEM('')
SURFACE()
);
#2701=(
BOUNDED_SURFACE()
B_SPLINE_SURFACE(1,2,((#140694,#140695,#140696,#140697,#140698),(#140699,
#140700,#140701,#140702,#140703)),.UNSPECIFIED.,.F.,.F.,.F.)
B_SPLINE_SURFACE_WITH_KNOTS((2,2),(3,2,3),(0.,0.289681084359919),(0.142474614281368,
0.142857142857143,0.159901408087482),.UNSPECIFIED.)
GEOMETRIC_REPRESENTATION_ITEM()
RATIONAL_B_SPLINE_SURFACE(((0.999732896029238,0.999865728939373,1.,0.994017305594881,
0.990889788836284),(0.999732896029238,0.999865728939373,1.,0.994017305594881,
0.990889788836284)))
REPRESENTATION_ITEM('')
SURFACE()
);
#2702=(
BOUNDED_SURFACE()
B_SPLINE_SURFACE(1,2,((#140712,#140713,#140714,#140715,#140716),(#140717,
#140718,#140719,#140720,#140721)),.UNSPECIFIED.,.F.,.F.,.F.)
B_SPLINE_SURFACE_WITH_KNOTS((2,2),(3,2,3),(0.,0.289807040992617),(0.573480748819789,
0.57365435021991,0.591014490232052),.UNSPECIFIED.)
GEOMETRIC_REPRESENTATION_ITEM()
RATIONAL_B_SPLINE_SURFACE(((0.99848615229188,0.99848615229188,0.99848615229188,
0.992772345172011,0.990020524139833),(0.99848615229188,0.99848615229188,
0.99848615229188,0.992772345172011,0.990020524139833)))
REPRESENTATION_ITEM('')
SURFACE()
);
#2703=(
BOUNDED_SURFACE()
B_SPLINE_SURFACE(1,2,((#140723,#140724,#140725,#140726,#140727),(#140728,
#140729,#140730,#140731,#140732)),.UNSPECIFIED.,.F.,.F.,.F.)
B_SPLINE_SURFACE_WITH_KNOTS((2,2),(3,2,3),(0.,0.289681084359923),(0.142474614281368,
0.142857142857143,0.159901408087482),.UNSPECIFIED.)
GEOMETRIC_REPRESENTATION_ITEM()
RATIONAL_B_SPLINE_SURFACE(((0.999732896029238,0.999865728939373,1.,0.994017305594881,
0.990889788836283),(0.999732896029238,0.999865728939373,1.,0.994017305594881,
0.990889788836283)))
REPRESENTATION_ITEM('')
SURFACE()
);
#2704=(
BOUNDED_SURFACE()
B_SPLINE_SURFACE(1,2,((#140741,#140742,#140743,#140744,#140745),(#140746,
#140747,#140748,#140749,#140750)),.UNSPECIFIED.,.F.,.F.,.F.)
B_SPLINE_SURFACE_WITH_KNOTS((2,2),(3,2,3),(0.,0.289807040993175),(0.573480748819789,
0.57365435021991,0.591014490232052),.UNSPECIFIED.)
GEOMETRIC_REPRESENTATION_ITEM()
RATIONAL_B_SPLINE_SURFACE(((0.99848615229188,0.99848615229188,0.99848615229188,
0.992772345172012,0.990020524139833),(0.99848615229188,0.99848615229188,
0.99848615229188,0.992772345172012,0.990020524139833)))
REPRESENTATION_ITEM('')
SURFACE()
);
#2705=(
BOUNDED_SURFACE()
B_SPLINE_SURFACE(1,2,((#140752,#140753,#140754,#140755,#140756),(#140757,
#140758,#140759,#140760,#140761)),.UNSPECIFIED.,.F.,.F.,.F.)
B_SPLINE_SURFACE_WITH_KNOTS((2,2),(3,2,3),(0.,0.289681084360261),(0.142474614281368,
0.142857142857143,0.159901408087482),.UNSPECIFIED.)
GEOMETRIC_REPRESENTATION_ITEM()
RATIONAL_B_SPLINE_SURFACE(((0.999732896029238,0.999865728939373,1.,0.994017305594881,
0.990889788836283),(0.999732896029238,0.999865728939373,1.,0.994017305594881,
0.990889788836284)))
REPRESENTATION_ITEM('')
SURFACE()
);
#2706=(
BOUNDED_SURFACE()
B_SPLINE_SURFACE(1,2,((#140770,#140771,#140772,#140773,#140774),(#140775,
#140776,#140777,#140778,#140779)),.UNSPECIFIED.,.F.,.F.,.F.)
B_SPLINE_SURFACE_WITH_KNOTS((2,2),(3,2,3),(0.,0.289807040992678),(0.57348074881971,
0.573654350219832,0.591014490232052),.UNSPECIFIED.)
GEOMETRIC_REPRESENTATION_ITEM()
RATIONAL_B_SPLINE_SURFACE(((0.998486152291931,0.998486152291931,0.998486152291931,
0.992772345172024,0.990020524139833),(0.998486152291931,0.998486152291931,
0.998486152291931,0.992772345172024,0.990020524139833)))
REPRESENTATION_ITEM('')
SURFACE()
);
#2707=(
BOUNDED_SURFACE()
B_SPLINE_SURFACE(1,2,((#140781,#140782,#140783,#140784,#140785),(#140786,
#140787,#140788,#140789,#140790)),.UNSPECIFIED.,.F.,.F.,.F.)
B_SPLINE_SURFACE_WITH_KNOTS((2,2),(3,2,3),(0.,0.289681084359922),(0.142474614281367,
0.142857142857143,0.159901408087481),.UNSPECIFIED.)
GEOMETRIC_REPRESENTATION_ITEM()
RATIONAL_B_SPLINE_SURFACE(((0.999732896029237,0.999865728939372,1.,0.994017305594881,
0.990889788836284),(0.999732896029237,0.999865728939372,1.,0.994017305594881,
0.990889788836284)))
REPRESENTATION_ITEM('')
SURFACE()
);
#2708=(
BOUNDED_SURFACE()
B_SPLINE_SURFACE(1,2,((#140799,#140800,#140801,#140802,#140803),(#140804,
#140805,#140806,#140807,#140808)),.UNSPECIFIED.,.F.,.F.,.F.)
B_SPLINE_SURFACE_WITH_KNOTS((2,2),(3,2,3),(0.,0.289807040992689),(0.57348074881979,
0.573654350219911,0.591014490232053),.UNSPECIFIED.)
GEOMETRIC_REPRESENTATION_ITEM()
RATIONAL_B_SPLINE_SURFACE(((0.99848615229188,0.99848615229188,0.99848615229188,
0.992772345172011,0.990020524139833),(0.99848615229188,0.99848615229188,
0.99848615229188,0.992772345172011,0.990020524139833)))
REPRESENTATION_ITEM('')
SURFACE()
);
#2709=(
BOUNDED_SURFACE()
B_SPLINE_SURFACE(1,2,((#140810,#140811,#140812,#140813,#140814),(#140815,
#140816,#140817,#140818,#140819)),.UNSPECIFIED.,.F.,.F.,.F.)
B_SPLINE_SURFACE_WITH_KNOTS((2,2),(3,2,3),(0.,0.28968108436027),(0.142474614281367,
0.142857142857143,0.159901408087481),.UNSPECIFIED.)
GEOMETRIC_REPRESENTATION_ITEM()
RATIONAL_B_SPLINE_SURFACE(((0.999732896029238,0.999865728939373,1.,0.994017305594881,
0.990889788836284),(0.999732896029238,0.999865728939373,1.,0.994017305594881,
0.990889788836284)))
REPRESENTATION_ITEM('')
SURFACE()
);
#2710=(
BOUNDED_SURFACE()
B_SPLINE_SURFACE(1,2,((#140828,#140829,#140830,#140831,#140832),(#140833,
#140834,#140835,#140836,#140837)),.UNSPECIFIED.,.F.,.F.,.F.)
B_SPLINE_SURFACE_WITH_KNOTS((2,2),(3,2,3),(0.,0.289807040993298),(0.57348074881979,
0.573654350219911,0.591014490232053),.UNSPECIFIED.)
GEOMETRIC_REPRESENTATION_ITEM()
RATIONAL_B_SPLINE_SURFACE(((0.99848615229188,0.99848615229188,0.99848615229188,
0.992772345172011,0.990020524139833),(0.99848615229188,0.99848615229188,
0.99848615229188,0.992772345172011,0.990020524139833)))
REPRESENTATION_ITEM('')
SURFACE()
);
#2711=(
BOUNDED_SURFACE()
B_SPLINE_SURFACE(1,2,((#140839,#140840,#140841,#140842,#140843),(#140844,
#140845,#140846,#140847,#140848)),.UNSPECIFIED.,.F.,.F.,.F.)
B_SPLINE_SURFACE_WITH_KNOTS((2,2),(3,2,3),(0.,0.289681084360275),(0.142474614281367,
0.142857142857143,0.159901408087481),.UNSPECIFIED.)
GEOMETRIC_REPRESENTATION_ITEM()
RATIONAL_B_SPLINE_SURFACE(((0.999732896029237,0.999865728939372,1.,0.994017305594881,
0.990889788836284),(0.999732896029237,0.999865728939372,1.,0.994017305594881,
0.990889788836284)))
REPRESENTATION_ITEM('')
SURFACE()
);
#2712=(
BOUNDED_SURFACE()
B_SPLINE_SURFACE(1,2,((#140857,#140858,#140859,#140860,#140861),(#140862,
#140863,#140864,#140865,#140866)),.UNSPECIFIED.,.F.,.F.,.F.)
B_SPLINE_SURFACE_WITH_KNOTS((2,2),(3,2,3),(0.,0.28980704099271),(0.573480748819708,
0.57365435021983,0.591014490232053),.UNSPECIFIED.)
GEOMETRIC_REPRESENTATION_ITEM()
RATIONAL_B_SPLINE_SURFACE(((0.998486152291933,0.998486152291933,0.998486152291933,
0.992772345172024,0.990020524139833),(0.998486152291933,0.998486152291933,
0.998486152291933,0.992772345172024,0.990020524139833)))
REPRESENTATION_ITEM('')
SURFACE()
);
#2713=(
BOUNDED_SURFACE()
B_SPLINE_SURFACE(1,2,((#140868,#140869,#140870,#140871,#140872),(#140873,
#140874,#140875,#140876,#140877)),.UNSPECIFIED.,.F.,.F.,.F.)
B_SPLINE_SURFACE_WITH_KNOTS((2,2),(3,2,3),(0.,0.28968108435992),(0.142474614281367,
0.142857142857143,0.159901408087481),.UNSPECIFIED.)
GEOMETRIC_REPRESENTATION_ITEM()
RATIONAL_B_SPLINE_SURFACE(((0.999732896029237,0.999865728939372,1.,0.994017305594881,
0.990889788836284),(0.999732896029237,0.999865728939372,1.,0.994017305594881,
0.990889788836284)))
REPRESENTATION_ITEM('')
SURFACE()
);
#2714=(
BOUNDED_SURFACE()
B_SPLINE_SURFACE(1,2,((#140886,#140887,#140888,#140889,#140890),(#140891,
#140892,#140893,#140894,#140895)),.UNSPECIFIED.,.F.,.F.,.F.)
B_SPLINE_SURFACE_WITH_KNOTS((2,2),(3,2,3),(0.,0.289807040993208),(0.57348074881979,
0.573654350219911,0.591014490232053),.UNSPECIFIED.)
GEOMETRIC_REPRESENTATION_ITEM()
RATIONAL_B_SPLINE_SURFACE(((0.99848615229188,0.99848615229188,0.99848615229188,
0.992772345172011,0.990020524139833),(0.99848615229188,0.99848615229188,
0.99848615229188,0.992772345172011,0.990020524139833)))
REPRESENTATION_ITEM('')
SURFACE()
);
#2715=(
BOUNDED_SURFACE()
B_SPLINE_SURFACE(1,2,((#140897,#140898,#140899,#140900,#140901),(#140902,
#140903,#140904,#140905,#140906),(#140907,#140908,#140909,#140910,#140911)),
 .UNSPECIFIED.,.F.,.F.,.F.)
B_SPLINE_SURFACE_WITH_KNOTS((2,1,2),(3,2,3),(-0.00289681084359918,0.,0.289681084359918),
(0.142474614281366,0.142857142857143,0.159901408087481),.UNSPECIFIED.)
GEOMETRIC_REPRESENTATION_ITEM()
RATIONAL_B_SPLINE_SURFACE(((0.999732896029237,0.999865728939372,1.,0.994017305594881,
0.990889788836284),(0.999732896029237,0.999865728939372,1.,0.994017305594881,
0.990889788836284),(0.999732896029237,0.999865728939372,1.,0.994017305594881,
0.990889788836284)))
REPRESENTATION_ITEM('')
SURFACE()
);
#2716=(
BOUNDED_SURFACE()
B_SPLINE_SURFACE(1,2,((#140920,#140921,#140922,#140923,#140924),(#140925,
#140926,#140927,#140928,#140929)),.UNSPECIFIED.,.F.,.F.,.F.)
B_SPLINE_SURFACE_WITH_KNOTS((2,2),(3,2,3),(0.,0.289807040992711),(0.573480748819708,
0.57365435021983,0.591014490232053),.UNSPECIFIED.)
GEOMETRIC_REPRESENTATION_ITEM()
RATIONAL_B_SPLINE_SURFACE(((0.998486152291933,0.998486152291933,0.998486152291933,
0.992772345172024,0.990020524139833),(0.998486152291933,0.998486152291933,
0.998486152291933,0.992772345172024,0.990020524139833)))
REPRESENTATION_ITEM('')
SURFACE()
);
#2717=(
BOUNDED_SURFACE()
B_SPLINE_SURFACE(1,2,((#140931,#140932,#140933,#140934,#140935),(#140936,
#140937,#140938,#140939,#140940)),.UNSPECIFIED.,.F.,.F.,.F.)
B_SPLINE_SURFACE_WITH_KNOTS((2,2),(3,2,3),(0.,0.289681084360276),(0.142474614281367,
0.142857142857143,0.159901408087481),.UNSPECIFIED.)
GEOMETRIC_REPRESENTATION_ITEM()
RATIONAL_B_SPLINE_SURFACE(((0.999732896029237,0.999865728939372,1.,0.994017305594881,
0.990889788836284),(0.999732896029237,0.999865728939372,1.,0.994017305594881,
0.990889788836284)))
REPRESENTATION_ITEM('')
SURFACE()
);
#2718=(
BOUNDED_SURFACE()
B_SPLINE_SURFACE(1,2,((#140949,#140950,#140951,#140952,#140953),(#140954,
#140955,#140956,#140957,#140958)),.UNSPECIFIED.,.F.,.F.,.F.)
B_SPLINE_SURFACE_WITH_KNOTS((2,2),(3,2,3),(0.,0.289807040993198),(0.57348074881971,
0.573654350219832,0.591014490232053),.UNSPECIFIED.)
GEOMETRIC_REPRESENTATION_ITEM()
RATIONAL_B_SPLINE_SURFACE(((0.998486152291932,0.998486152291932,0.998486152291932,
0.992772345172024,0.990020524139833),(0.998486152291932,0.998486152291932,
0.998486152291932,0.992772345172024,0.990020524139833)))
REPRESENTATION_ITEM('')
SURFACE()
);
#2719=(
BOUNDED_SURFACE()
B_SPLINE_SURFACE(1,2,((#140960,#140961,#140962,#140963,#140964),(#140965,
#140966,#140967,#140968,#140969)),.UNSPECIFIED.,.F.,.F.,.F.)
B_SPLINE_SURFACE_WITH_KNOTS((2,2),(3,2,3),(0.,0.289681084359923),(0.142474614281367,
0.142857142857143,0.159901408087481),.UNSPECIFIED.)
GEOMETRIC_REPRESENTATION_ITEM()
RATIONAL_B_SPLINE_SURFACE(((0.999732896029238,0.999865728939373,1.,0.994017305594881,
0.990889788836284),(0.999732896029238,0.999865728939373,1.,0.994017305594881,
0.990889788836284)))
REPRESENTATION_ITEM('')
SURFACE()
);
#2720=(
BOUNDED_SURFACE()
B_SPLINE_SURFACE(1,2,((#140978,#140979,#140980,#140981,#140982),(#140983,
#140984,#140985,#140986,#140987)),.UNSPECIFIED.,.F.,.F.,.F.)
B_SPLINE_SURFACE_WITH_KNOTS((2,2),(3,2,3),(0.,0.289807040992956),(0.57348074881971,
0.573654350219832,0.591014490232053),.UNSPECIFIED.)
GEOMETRIC_REPRESENTATION_ITEM()
RATIONAL_B_SPLINE_SURFACE(((0.998486152291931,0.998486152291931,0.998486152291931,
0.992772345172023,0.990020524139833),(0.998486152291931,0.998486152291931,
0.998486152291931,0.992772345172023,0.990020524139833)))
REPRESENTATION_ITEM('')
SURFACE()
);
#2721=(
BOUNDED_SURFACE()
B_SPLINE_SURFACE(1,2,((#140989,#140990,#140991,#140992,#140993),(#140994,
#140995,#140996,#140997,#140998)),.UNSPECIFIED.,.F.,.F.,.F.)
B_SPLINE_SURFACE_WITH_KNOTS((2,2),(3,2,3),(0.,0.289681084359924),(0.142474614281367,
0.142857142857143,0.159901408087481),.UNSPECIFIED.)
GEOMETRIC_REPRESENTATION_ITEM()
RATIONAL_B_SPLINE_SURFACE(((0.999732896029237,0.999865728939372,1.,0.994017305594881,
0.990889788836284),(0.999732896029237,0.999865728939372,1.,0.994017305594881,
0.990889788836284)))
REPRESENTATION_ITEM('')
SURFACE()
);
#2722=(
BOUNDED_SURFACE()
B_SPLINE_SURFACE(1,2,((#141007,#141008,#141009,#141010,#141011),(#141012,
#141013,#141014,#141015,#141016)),.UNSPECIFIED.,.F.,.F.,.F.)
B_SPLINE_SURFACE_WITH_KNOTS((2,2),(3,2,3),(0.,0.289807040994019),(0.57348074881979,
0.573654350219911,0.591014490232053),.UNSPECIFIED.)
GEOMETRIC_REPRESENTATION_ITEM()
RATIONAL_B_SPLINE_SURFACE(((0.99848615229188,0.99848615229188,0.99848615229188,
0.992772345172011,0.990020524139833),(0.99848615229188,0.99848615229188,
0.99848615229188,0.992772345172011,0.990020524139833)))
REPRESENTATION_ITEM('')
SURFACE()
);
#2723=(
BOUNDED_SURFACE()
B_SPLINE_SURFACE(1,2,((#141018,#141019,#141020,#141021,#141022),(#141023,
#141024,#141025,#141026,#141027),(#141028,#141029,#141030,#141031,#141032)),
 .UNSPECIFIED.,.F.,.F.,.F.)
B_SPLINE_SURFACE_WITH_KNOTS((2,1,2),(3,2,3),(-0.00289681084360293,0.,0.289681084360293),
(0.142474614281367,0.142857142857143,0.159901408087481),.UNSPECIFIED.)
GEOMETRIC_REPRESENTATION_ITEM()
RATIONAL_B_SPLINE_SURFACE(((0.999732896029237,0.999865728939372,1.,0.994017305594881,
0.990889788836284),(0.999732896029237,0.999865728939372,1.,0.994017305594881,
0.990889788836284),(0.999732896029237,0.999865728939372,1.,0.994017305594881,
0.990889788836284)))
REPRESENTATION_ITEM('')
SURFACE()
);
#2724=(
BOUNDED_SURFACE()
B_SPLINE_SURFACE(1,2,((#141041,#141042,#141043,#141044,#141045),(#141046,
#141047,#141048,#141049,#141050)),.UNSPECIFIED.,.F.,.F.,.F.)
B_SPLINE_SURFACE_WITH_KNOTS((2,2),(3,2,3),(0.,0.28980704099276),(0.573480748819524,
0.573654350219648,0.591014490232054),.UNSPECIFIED.)
GEOMETRIC_REPRESENTATION_ITEM()
RATIONAL_B_SPLINE_SURFACE(((0.998486152292053,0.998486152292053,0.998486152292053,
0.992772345172052,0.990020524139832),(0.998486152292053,0.998486152292053,
0.998486152292053,0.992772345172052,0.990020524139832)))
REPRESENTATION_ITEM('')
SURFACE()
);
#2725=(
BOUNDED_SURFACE()
B_SPLINE_SURFACE(1,2,((#141052,#141053,#141054,#141055,#141056),(#141057,
#141058,#141059,#141060,#141061)),.UNSPECIFIED.,.F.,.F.,.F.)
B_SPLINE_SURFACE_WITH_KNOTS((2,2),(3,2,3),(0.,0.289681084359925),(0.142474614281366,
0.142857142857143,0.159901408087481),.UNSPECIFIED.)
GEOMETRIC_REPRESENTATION_ITEM()
RATIONAL_B_SPLINE_SURFACE(((0.999732896029237,0.999865728939372,1.,0.994017305594881,
0.990889788836284),(0.999732896029237,0.999865728939372,1.,0.994017305594881,
0.990889788836284)))
REPRESENTATION_ITEM('')
SURFACE()
);
#2726=(
BOUNDED_SURFACE()
B_SPLINE_SURFACE(1,2,((#141070,#141071,#141072,#141073,#141074),(#141075,
#141076,#141077,#141078,#141079)),.UNSPECIFIED.,.F.,.F.,.F.)
B_SPLINE_SURFACE_WITH_KNOTS((2,2),(3,2,3),(0.,0.289807040992642),(0.57348074881979,
0.573654350219911,0.591014490232053),.UNSPECIFIED.)
GEOMETRIC_REPRESENTATION_ITEM()
RATIONAL_B_SPLINE_SURFACE(((0.99848615229188,0.99848615229188,0.99848615229188,
0.992772345172011,0.990020524139833),(0.99848615229188,0.99848615229188,
0.99848615229188,0.992772345172011,0.990020524139833)))
REPRESENTATION_ITEM('')
SURFACE()
);
#2727=(
BOUNDED_SURFACE()
B_SPLINE_SURFACE(1,2,((#141081,#141082,#141083,#141084,#141085),(#141086,
#141087,#141088,#141089,#141090)),.UNSPECIFIED.,.F.,.F.,.F.)
B_SPLINE_SURFACE_WITH_KNOTS((2,2),(3,2,3),(0.,0.289681084360439),(0.142474614281367,
0.142857142857143,0.159901408087482),.UNSPECIFIED.)
GEOMETRIC_REPRESENTATION_ITEM()
RATIONAL_B_SPLINE_SURFACE(((0.999732896029237,0.999865728939372,1.,0.994017305594881,
0.990889788836284),(0.999732896029237,0.999865728939372,1.,0.994017305594881,
0.990889788836284)))
REPRESENTATION_ITEM('')
SURFACE()
);
#2728=(
BOUNDED_SURFACE()
B_SPLINE_SURFACE(1,2,((#141099,#141100,#141101,#141102,#141103),(#141104,
#141105,#141106,#141107,#141108)),.UNSPECIFIED.,.F.,.F.,.F.)
B_SPLINE_SURFACE_WITH_KNOTS((2,2),(3,2,3),(0.,0.289807040993272),(0.573480748819715,
0.573654350219837,0.591014490232053),.UNSPECIFIED.)
GEOMETRIC_REPRESENTATION_ITEM()
RATIONAL_B_SPLINE_SURFACE(((0.998486152291929,0.998486152291929,0.998486152291929,
0.992772345172023,0.990020524139833),(0.998486152291929,0.998486152291929,
0.998486152291929,0.992772345172023,0.990020524139833)))
REPRESENTATION_ITEM('')
SURFACE()
);
#2729=(
BOUNDED_SURFACE()
B_SPLINE_SURFACE(1,2,((#141110,#141111,#141112,#141113,#141114),(#141115,
#141116,#141117,#141118,#141119)),.UNSPECIFIED.,.F.,.F.,.F.)
B_SPLINE_SURFACE_WITH_KNOTS((2,2),(3,2,3),(0.,0.289681084360251),(0.142474614281367,
0.142857142857143,0.159901408087481),.UNSPECIFIED.)
GEOMETRIC_REPRESENTATION_ITEM()
RATIONAL_B_SPLINE_SURFACE(((0.999732896029238,0.999865728939373,1.,0.994017305594881,
0.990889788836284),(0.999732896029238,0.999865728939373,1.,0.994017305594881,
0.990889788836284)))
REPRESENTATION_ITEM('')
SURFACE()
);
#2730=(
BOUNDED_SURFACE()
B_SPLINE_SURFACE(1,2,((#141128,#141129,#141130,#141131,#141132),(#141133,
#141134,#141135,#141136,#141137)),.UNSPECIFIED.,.F.,.F.,.F.)
B_SPLINE_SURFACE_WITH_KNOTS((2,2),(3,2,3),(0.,0.289807040991733),(0.57348074881979,
0.573654350219911,0.591014490232053),.UNSPECIFIED.)
GEOMETRIC_REPRESENTATION_ITEM()
RATIONAL_B_SPLINE_SURFACE(((0.99848615229188,0.99848615229188,0.99848615229188,
0.992772345172011,0.990020524139833),(0.99848615229188,0.99848615229188,
0.99848615229188,0.992772345172011,0.990020524139833)))
REPRESENTATION_ITEM('')
SURFACE()
);
#2731=(
BOUNDED_SURFACE()
B_SPLINE_SURFACE(1,2,((#141139,#141140,#141141,#141142,#141143),(#141144,
#141145,#141146,#141147,#141148)),.UNSPECIFIED.,.F.,.F.,.F.)
B_SPLINE_SURFACE_WITH_KNOTS((2,2),(3,2,3),(0.,0.289681084360222),(0.142474614281367,
0.142857142857143,0.159901408087481),.UNSPECIFIED.)
GEOMETRIC_REPRESENTATION_ITEM()
RATIONAL_B_SPLINE_SURFACE(((0.999732896029237,0.999865728939372,1.,0.994017305594881,
0.990889788836284),(0.999732896029237,0.999865728939372,1.,0.994017305594881,
0.990889788836284)))
REPRESENTATION_ITEM('')
SURFACE()
);
#2732=(
BOUNDED_SURFACE()
B_SPLINE_SURFACE(1,2,((#141157,#141158,#141159,#141160,#141161),(#141162,
#141163,#141164,#141165,#141166)),.UNSPECIFIED.,.F.,.F.,.F.)
B_SPLINE_SURFACE_WITH_KNOTS((2,2),(3,2,3),(0.,0.289807040992883),(0.573480748819775,
0.573654350219897,0.591014490232053),.UNSPECIFIED.)
GEOMETRIC_REPRESENTATION_ITEM()
RATIONAL_B_SPLINE_SURFACE(((0.998486152291889,0.998486152291889,0.998486152291889,
0.992772345172013,0.990020524139833),(0.998486152291889,0.998486152291889,
0.998486152291889,0.992772345172013,0.990020524139833)))
REPRESENTATION_ITEM('')
SURFACE()
);
#2733=(
BOUNDED_SURFACE()
B_SPLINE_SURFACE(1,2,((#141168,#141169,#141170,#141171,#141172),(#141173,
#141174,#141175,#141176,#141177)),.UNSPECIFIED.,.F.,.F.,.F.)
B_SPLINE_SURFACE_WITH_KNOTS((2,2),(3,2,3),(0.,0.289681084359925),(0.142474614281367,
0.142857142857143,0.159901408087481),.UNSPECIFIED.)
GEOMETRIC_REPRESENTATION_ITEM()
RATIONAL_B_SPLINE_SURFACE(((0.999732896029237,0.999865728939372,1.,0.994017305594881,
0.990889788836284),(0.999732896029237,0.999865728939372,1.,0.994017305594881,
0.990889788836284)))
REPRESENTATION_ITEM('')
SURFACE()
);
#2734=(
BOUNDED_SURFACE()
B_SPLINE_SURFACE(1,2,((#141186,#141187,#141188,#141189,#141190),(#141191,
#141192,#141193,#141194,#141195)),.UNSPECIFIED.,.F.,.F.,.F.)
B_SPLINE_SURFACE_WITH_KNOTS((2,2),(3,2,3),(0.,0.289807040992693),(0.57348074881979,
0.573654350219911,0.591014490232053),.UNSPECIFIED.)
GEOMETRIC_REPRESENTATION_ITEM()
RATIONAL_B_SPLINE_SURFACE(((0.99848615229188,0.99848615229188,0.99848615229188,
0.992772345172011,0.990020524139833),(0.99848615229188,0.99848615229188,
0.99848615229188,0.992772345172011,0.990020524139833)))
REPRESENTATION_ITEM('')
SURFACE()
);
#2735=(
BOUNDED_SURFACE()
B_SPLINE_SURFACE(1,2,((#141197,#141198,#141199,#141200,#141201),(#141202,
#141203,#141204,#141205,#141206),(#141207,#141208,#141209,#141210,#141211)),
 .UNSPECIFIED.,.F.,.F.,.F.)
B_SPLINE_SURFACE_WITH_KNOTS((2,1,2),(3,2,3),(-0.00289681084359929,0.,0.289681084359929),
(0.142474614281367,0.142857142857143,0.159901408087481),.UNSPECIFIED.)
GEOMETRIC_REPRESENTATION_ITEM()
RATIONAL_B_SPLINE_SURFACE(((0.999732896029238,0.999865728939373,1.,0.994017305594881,
0.990889788836284),(0.999732896029238,0.999865728939373,1.,0.994017305594881,
0.990889788836284),(0.999732896029238,0.999865728939373,1.,0.994017305594881,
0.990889788836284)))
REPRESENTATION_ITEM('')
SURFACE()
);
#2736=(
BOUNDED_SURFACE()
B_SPLINE_SURFACE(1,2,((#141220,#141221,#141222,#141223,#141224),(#141225,
#141226,#141227,#141228,#141229)),.UNSPECIFIED.,.F.,.F.,.F.)
B_SPLINE_SURFACE_WITH_KNOTS((2,2),(3,2,3),(0.,0.289807040993738),(0.573480748819763,
0.573654350219885,0.591014490232053),.UNSPECIFIED.)
GEOMETRIC_REPRESENTATION_ITEM()
RATIONAL_B_SPLINE_SURFACE(((0.998486152291897,0.998486152291897,0.998486152291897,
0.992772345172015,0.990020524139833),(0.998486152291897,0.998486152291897,
0.998486152291897,0.992772345172015,0.990020524139833)))
REPRESENTATION_ITEM('')
SURFACE()
);
#2737=(
BOUNDED_SURFACE()
B_SPLINE_SURFACE(1,2,((#141231,#141232,#141233,#141234,#141235),(#141236,
#141237,#141238,#141239,#141240),(#141241,#141242,#141243,#141244,#141245)),
 .UNSPECIFIED.,.F.,.F.,.F.)
B_SPLINE_SURFACE_WITH_KNOTS((2,1,2),(3,2,3),(-0.00289681084360253,0.,0.289681084360253),
(0.142474614281367,0.142857142857143,0.159901408087481),.UNSPECIFIED.)
GEOMETRIC_REPRESENTATION_ITEM()
RATIONAL_B_SPLINE_SURFACE(((0.999732896029237,0.999865728939372,1.,0.994017305594881,
0.990889788836284),(0.999732896029237,0.999865728939372,1.,0.994017305594881,
0.990889788836284),(0.999732896029237,0.999865728939372,1.,0.994017305594881,
0.990889788836284)))
REPRESENTATION_ITEM('')
SURFACE()
);
#2738=(
BOUNDED_SURFACE()
B_SPLINE_SURFACE(1,2,((#141254,#141255,#141256,#141257,#141258),(#141259,
#141260,#141261,#141262,#141263)),.UNSPECIFIED.,.F.,.F.,.F.)
B_SPLINE_SURFACE_WITH_KNOTS((2,2),(3,2,3),(0.,0.289807040991898),(0.57348074881979,
0.573654350219911,0.591014490232053),.UNSPECIFIED.)
GEOMETRIC_REPRESENTATION_ITEM()
RATIONAL_B_SPLINE_SURFACE(((0.99848615229188,0.99848615229188,0.99848615229188,
0.992772345172011,0.990020524139833),(0.99848615229188,0.99848615229188,
0.99848615229188,0.992772345172011,0.990020524139833)))
REPRESENTATION_ITEM('')
SURFACE()
);
#2739=(
BOUNDED_SURFACE()
B_SPLINE_SURFACE(1,2,((#141265,#141266,#141267,#141268,#141269),(#141270,
#141271,#141272,#141273,#141274)),.UNSPECIFIED.,.F.,.F.,.F.)
B_SPLINE_SURFACE_WITH_KNOTS((2,2),(3,2,3),(0.,0.289681084361046),(0.142474614281368,
0.142857142857143,0.159901408087495),.UNSPECIFIED.)
GEOMETRIC_REPRESENTATION_ITEM()
RATIONAL_B_SPLINE_SURFACE(((0.999732896029238,0.999865728939373,1.,0.994017305594876,
0.990889788836279),(0.999732896029238,0.999865728939373,1.,0.994017305594876,
0.990889788836279)))
REPRESENTATION_ITEM('')
SURFACE()
);
#2740=(
BOUNDED_SURFACE()
B_SPLINE_SURFACE(1,2,((#141283,#141284,#141285,#141286,#141287),(#141288,
#141289,#141290,#141291,#141292)),.UNSPECIFIED.,.F.,.F.,.F.)
B_SPLINE_SURFACE_WITH_KNOTS((2,2),(3,2,3),(0.,0.28980704099156),(0.573480748819789,
0.57365435021991,0.591014490232052),.UNSPECIFIED.)
GEOMETRIC_REPRESENTATION_ITEM()
RATIONAL_B_SPLINE_SURFACE(((0.99848615229188,0.99848615229188,0.99848615229188,
0.992772345172012,0.990020524139833),(0.99848615229188,0.99848615229188,
0.99848615229188,0.992772345172012,0.990020524139833)))
REPRESENTATION_ITEM('')
SURFACE()
);
#2741=(
BOUNDED_SURFACE()
B_SPLINE_SURFACE(1,2,((#141294,#141295,#141296,#141297,#141298),(#141299,
#141300,#141301,#141302,#141303)),.UNSPECIFIED.,.F.,.F.,.F.)
B_SPLINE_SURFACE_WITH_KNOTS((2,2),(3,2,3),(0.,0.289681084360513),(0.142474614281368,
0.142857142857143,0.159901408087482),.UNSPECIFIED.)
GEOMETRIC_REPRESENTATION_ITEM()
RATIONAL_B_SPLINE_SURFACE(((0.999732896029238,0.999865728939373,1.,0.994017305594881,
0.990889788836284),(0.999732896029238,0.999865728939373,1.,0.994017305594881,
0.990889788836284)))
REPRESENTATION_ITEM('')
SURFACE()
);
#2742=(
BOUNDED_SURFACE()
B_SPLINE_SURFACE(1,2,((#141312,#141313,#141314,#141315,#141316),(#141317,
#141318,#141319,#141320,#141321)),.UNSPECIFIED.,.F.,.F.,.F.)
B_SPLINE_SURFACE_WITH_KNOTS((2,2),(3,2,3),(0.,0.289807040991555),(0.573480748819707,
0.573654350219829,0.591014490232052),.UNSPECIFIED.)
GEOMETRIC_REPRESENTATION_ITEM()
RATIONAL_B_SPLINE_SURFACE(((0.998486152291934,0.998486152291934,0.998486152291934,
0.992772345172024,0.990020524139833),(0.998486152291934,0.998486152291934,
0.998486152291934,0.992772345172024,0.990020524139833)))
REPRESENTATION_ITEM('')
SURFACE()
);
#2743=(
BOUNDED_SURFACE()
B_SPLINE_SURFACE(1,2,((#141323,#141324,#141325,#141326,#141327),(#141328,
#141329,#141330,#141331,#141332)),.UNSPECIFIED.,.F.,.F.,.F.)
B_SPLINE_SURFACE_WITH_KNOTS((2,2),(3,2,3),(0.,0.289681084359919),(0.142474614281368,
0.142857142857143,0.159901408087482),.UNSPECIFIED.)
GEOMETRIC_REPRESENTATION_ITEM()
RATIONAL_B_SPLINE_SURFACE(((0.999732896029238,0.999865728939373,1.,0.994017305594881,
0.990889788836283),(0.999732896029238,0.999865728939373,1.,0.994017305594881,
0.990889788836283)))
REPRESENTATION_ITEM('')
SURFACE()
);
#2744=(
BOUNDED_SURFACE()
B_SPLINE_SURFACE(1,2,((#141341,#141342,#141343,#141344,#141345),(#141346,
#141347,#141348,#141349,#141350)),.UNSPECIFIED.,.F.,.F.,.F.)
B_SPLINE_SURFACE_WITH_KNOTS((2,2),(3,2,3),(0.,0.289807040991694),(0.573480748819707,
0.573654350219829,0.591014490232052),.UNSPECIFIED.)
GEOMETRIC_REPRESENTATION_ITEM()
RATIONAL_B_SPLINE_SURFACE(((0.998486152291934,0.998486152291934,0.998486152291934,
0.992772345172024,0.990020524139833),(0.998486152291934,0.998486152291934,
0.998486152291934,0.992772345172024,0.990020524139833)))
REPRESENTATION_ITEM('')
SURFACE()
);
#2745=(
BOUNDED_SURFACE()
B_SPLINE_SURFACE(1,2,((#141352,#141353,#141354,#141355,#141356),(#141357,
#141358,#141359,#141360,#141361),(#141362,#141363,#141364,#141365,#141366)),
 .UNSPECIFIED.,.F.,.F.,.F.)
B_SPLINE_SURFACE_WITH_KNOTS((2,1,2),(3,2,3),(-0.00289681084360272,0.,0.289681084360272),
(0.142474614281368,0.142857142857143,0.159901408087482),.UNSPECIFIED.)
GEOMETRIC_REPRESENTATION_ITEM()
RATIONAL_B_SPLINE_SURFACE(((0.999732896029238,0.999865728939373,1.,0.994017305594881,
0.990889788836284),(0.999732896029238,0.999865728939373,1.,0.994017305594881,
0.990889788836284),(0.999732896029238,0.999865728939373,1.,0.994017305594881,
0.990889788836284)))
REPRESENTATION_ITEM('')
SURFACE()
);
#2746=(
BOUNDED_SURFACE()
B_SPLINE_SURFACE(1,2,((#141368,#141369,#141370),(#141371,#141372,#141373)),
 .UNSPECIFIED.,.F.,.F.,.F.)
B_SPLINE_SURFACE_WITH_KNOTS((2,2),(3,3),(0.,0.289807040991566),(0.194132688793569,
0.211606804210308),.UNSPECIFIED.)
GEOMETRIC_REPRESENTATION_ITEM()
RATIONAL_B_SPLINE_SURFACE(((0.989843896581211,0.992516389311156,0.998189888755648),
(0.989843896581211,0.992516389311156,0.998189888755648)))
REPRESENTATION_ITEM('')
SURFACE()
);
#2747=(
BOUNDED_SURFACE()
B_SPLINE_SURFACE(1,2,((#141390,#141391,#141392,#141393,#141394),(#141395,
#141396,#141397,#141398,#141399)),.UNSPECIFIED.,.F.,.F.,.F.)
B_SPLINE_SURFACE_WITH_KNOTS((2,2),(3,2,3),(0.,0.290272734870772),(0.521815037222016,
0.53899963051341,0.539591284257231),.UNSPECIFIED.)
GEOMETRIC_REPRESENTATION_ITEM()
RATIONAL_B_SPLINE_SURFACE(((0.989362668575565,0.987015160230477,0.987570037304351,
0.987570037304351,0.987570037304351),(0.989362668575565,0.987015160230477,
0.987570037304351,0.987570037304351,0.987570037304351)))
REPRESENTATION_ITEM('')
SURFACE()
);
#2748=(
BOUNDED_SURFACE()
B_SPLINE_SURFACE(1,2,((#141401,#141402,#141403),(#141404,#141405,#141406)),
 .UNSPECIFIED.,.F.,.F.,.F.)
B_SPLINE_SURFACE_WITH_KNOTS((2,2),(3,3),(0.,0.289807040991565),(0.194132688793569,
0.211606804210307),.UNSPECIFIED.)
GEOMETRIC_REPRESENTATION_ITEM()
RATIONAL_B_SPLINE_SURFACE(((0.989843896581211,0.992516389311156,0.998189888755648),
(0.989843896581211,0.992516389311156,0.998189888755648)))
REPRESENTATION_ITEM('')
SURFACE()
);
#2749=(
BOUNDED_SURFACE()
B_SPLINE_SURFACE(1,2,((#141423,#141424,#141425,#141426,#141427),(#141428,
#141429,#141430,#141431,#141432)),.UNSPECIFIED.,.F.,.F.,.F.)
B_SPLINE_SURFACE_WITH_KNOTS((2,2),(3,2,3),(0.,0.290272734853992),(0.521815037222017,
0.538999630513411,0.539591284240711),.UNSPECIFIED.)
GEOMETRIC_REPRESENTATION_ITEM()
RATIONAL_B_SPLINE_SURFACE(((0.989362668575565,0.987015160230477,0.987570037304351,
0.987570037304351,0.987570037304351),(0.989362668575565,0.987015160230477,
0.987570037304351,0.987570037304351,0.987570037304351)))
REPRESENTATION_ITEM('')
SURFACE()
);
#2750=(
BOUNDED_SURFACE()
B_SPLINE_SURFACE(1,2,((#141434,#141435,#141436),(#141437,#141438,#141439)),
 .UNSPECIFIED.,.F.,.F.,.F.)
B_SPLINE_SURFACE_WITH_KNOTS((2,2),(3,3),(0.,0.289807040991569),(0.194132688793568,
0.211606804210307),.UNSPECIFIED.)
GEOMETRIC_REPRESENTATION_ITEM()
RATIONAL_B_SPLINE_SURFACE(((0.989843896581211,0.992516389311156,0.998189888755648),
(0.989843896581211,0.992516389311156,0.998189888755648)))
REPRESENTATION_ITEM('')
SURFACE()
);
#2751=(
BOUNDED_SURFACE()
B_SPLINE_SURFACE(1,2,((#141456,#141457,#141458,#141459,#141460),(#141461,
#141462,#141463,#141464,#141465)),.UNSPECIFIED.,.F.,.F.,.F.)
B_SPLINE_SURFACE_WITH_KNOTS((2,2),(3,2,3),(0.,0.290272734861209),(0.521815037222017,
0.538999630513411,0.539591284247956),.UNSPECIFIED.)
GEOMETRIC_REPRESENTATION_ITEM()
RATIONAL_B_SPLINE_SURFACE(((0.989362668575565,0.987015160230477,0.987570037304351,
0.987570037304351,0.987570037304351),(0.989362668575565,0.987015160230477,
0.987570037304351,0.987570037304351,0.987570037304351)))
REPRESENTATION_ITEM('')
SURFACE()
);
#2752=(
BOUNDED_SURFACE()
B_SPLINE_SURFACE(1,2,((#141467,#141468,#141469),(#141470,#141471,#141472)),
 .UNSPECIFIED.,.F.,.F.,.F.)
B_SPLINE_SURFACE_WITH_KNOTS((2,2),(3,3),(0.,0.289807040991558),(0.194132688793568,
0.211606804210307),.UNSPECIFIED.)
GEOMETRIC_REPRESENTATION_ITEM()
RATIONAL_B_SPLINE_SURFACE(((0.989843896581211,0.992516389311156,0.998189888755648),
(0.989843896581211,0.992516389311156,0.998189888755648)))
REPRESENTATION_ITEM('')
SURFACE()
);
#2753=(
BOUNDED_SURFACE()
B_SPLINE_SURFACE(1,2,((#141489,#141490,#141491,#141492,#141493),(#141494,
#141495,#141496,#141497,#141498)),.UNSPECIFIED.,.F.,.F.,.F.)
B_SPLINE_SURFACE_WITH_KNOTS((2,2),(3,2,3),(0.,0.290272734854879),(0.521815037222017,
0.538999630513411,0.539591284241346),.UNSPECIFIED.)
GEOMETRIC_REPRESENTATION_ITEM()
RATIONAL_B_SPLINE_SURFACE(((0.989362668575565,0.987015160230477,0.987570037304351,
0.987570037304351,0.987570037304351),(0.989362668575565,0.987015160230477,
0.987570037304351,0.987570037304351,0.987570037304351)))
REPRESENTATION_ITEM('')
SURFACE()
);
#2754=(
BOUNDED_SURFACE()
B_SPLINE_SURFACE(1,2,((#141500,#141501,#141502),(#141503,#141504,#141505)),
 .UNSPECIFIED.,.F.,.F.,.F.)
B_SPLINE_SURFACE_WITH_KNOTS((2,2),(3,3),(0.,0.28980704099156),(0.194132688793568,
0.211606804210307),.UNSPECIFIED.)
GEOMETRIC_REPRESENTATION_ITEM()
RATIONAL_B_SPLINE_SURFACE(((0.989843896581211,0.992516389311156,0.998189888755648),
(0.989843896581211,0.992516389311156,0.998189888755648)))
REPRESENTATION_ITEM('')
SURFACE()
);
#2755=(
BOUNDED_SURFACE()
B_SPLINE_SURFACE(1,2,((#141522,#141523,#141524,#141525,#141526),(#141527,
#141528,#141529,#141530,#141531)),.UNSPECIFIED.,.F.,.F.,.F.)
B_SPLINE_SURFACE_WITH_KNOTS((2,2),(3,2,3),(0.,0.290272734843646),(0.521815037222017,
0.538999630513411,0.539591284230401),.UNSPECIFIED.)
GEOMETRIC_REPRESENTATION_ITEM()
RATIONAL_B_SPLINE_SURFACE(((0.989362668575565,0.987015160230477,0.987570037304351,
0.987570037304351,0.987570037304351),(0.989362668575565,0.987015160230477,
0.987570037304351,0.987570037304351,0.987570037304351)))
REPRESENTATION_ITEM('')
SURFACE()
);
#2756=(
BOUNDED_SURFACE()
B_SPLINE_SURFACE(1,2,((#141533,#141534,#141535),(#141536,#141537,#141538)),
 .UNSPECIFIED.,.F.,.F.,.F.)
B_SPLINE_SURFACE_WITH_KNOTS((2,2),(3,3),(0.,0.289807040991562),(0.194132688793568,
0.211606804210307),.UNSPECIFIED.)
GEOMETRIC_REPRESENTATION_ITEM()
RATIONAL_B_SPLINE_SURFACE(((0.989843896581211,0.992516389311156,0.998189888755648),
(0.989843896581211,0.992516389311156,0.998189888755648)))
REPRESENTATION_ITEM('')
SURFACE()
);
#2757=(
BOUNDED_SURFACE()
B_SPLINE_SURFACE(1,2,((#141555,#141556,#141557,#141558,#141559),(#141560,
#141561,#141562,#141563,#141564)),.UNSPECIFIED.,.F.,.F.,.F.)
B_SPLINE_SURFACE_WITH_KNOTS((2,2),(3,2,3),(0.,0.290272734900014),(0.521815037222017,
0.538999630513411,0.53959128428651),.UNSPECIFIED.)
GEOMETRIC_REPRESENTATION_ITEM()
RATIONAL_B_SPLINE_SURFACE(((0.989362668575565,0.987015160230477,0.987570037304351,
0.987570037304351,0.987570037304351),(0.989362668575565,0.987015160230477,
0.987570037304351,0.987570037304351,0.987570037304351)))
REPRESENTATION_ITEM('')
SURFACE()
);
#2758=(
BOUNDED_SURFACE()
B_SPLINE_SURFACE(1,2,((#141566,#141567,#141568),(#141569,#141570,#141571)),
 .UNSPECIFIED.,.F.,.F.,.F.)
B_SPLINE_SURFACE_WITH_KNOTS((2,2),(3,3),(0.,0.289807040991558),(0.194132688793568,
0.211606804210307),.UNSPECIFIED.)
GEOMETRIC_REPRESENTATION_ITEM()
RATIONAL_B_SPLINE_SURFACE(((0.989843896581211,0.992516389311156,0.998189888755648),
(0.98984389658121,0.992516389311155,0.998189888755648)))
REPRESENTATION_ITEM('')
SURFACE()
);
#2759=(
BOUNDED_SURFACE()
B_SPLINE_SURFACE(1,2,((#141588,#141589,#141590,#141591,#141592),(#141593,
#141594,#141595,#141596,#141597)),.UNSPECIFIED.,.F.,.F.,.F.)
B_SPLINE_SURFACE_WITH_KNOTS((2,2),(3,2,3),(0.,0.29027273486563),(0.521815037222018,
0.538999630513412,0.53959128425217),.UNSPECIFIED.)
GEOMETRIC_REPRESENTATION_ITEM()
RATIONAL_B_SPLINE_SURFACE(((0.989362668575565,0.987015160230477,0.987570037304351,
0.987570037304351,0.987570037304351),(0.989362668575565,0.987015160230477,
0.987570037304351,0.987570037304351,0.987570037304351)))
REPRESENTATION_ITEM('')
SURFACE()
);
#2760=(
BOUNDED_SURFACE()
B_SPLINE_SURFACE(1,2,((#141599,#141600,#141601),(#141602,#141603,#141604)),
 .UNSPECIFIED.,.F.,.F.,.F.)
B_SPLINE_SURFACE_WITH_KNOTS((2,2),(3,3),(0.,0.289807040991555),(0.194132688793568,
0.211606804210307),.UNSPECIFIED.)
GEOMETRIC_REPRESENTATION_ITEM()
RATIONAL_B_SPLINE_SURFACE(((0.989843896581211,0.992516389311156,0.998189888755647),
(0.989843896581211,0.992516389311156,0.998189888755647)))
REPRESENTATION_ITEM('')
SURFACE()
);
#2761=(
BOUNDED_SURFACE()
B_SPLINE_SURFACE(1,2,((#141621,#141622,#141623,#141624,#141625),(#141626,
#141627,#141628,#141629,#141630)),.UNSPECIFIED.,.F.,.F.,.F.)
B_SPLINE_SURFACE_WITH_KNOTS((2,2),(3,2,3),(0.,0.290272734845788),(0.521815037222017,
0.538999630513411,0.53959128423262),.UNSPECIFIED.)
GEOMETRIC_REPRESENTATION_ITEM()
RATIONAL_B_SPLINE_SURFACE(((0.989362668575565,0.987015160230477,0.987570037304351,
0.987570037304351,0.987570037304351),(0.989362668575565,0.987015160230477,
0.987570037304351,0.987570037304351,0.987570037304351)))
REPRESENTATION_ITEM('')
SURFACE()
);
#2762=(
BOUNDED_SURFACE()
B_SPLINE_SURFACE(1,2,((#141632,#141633,#141634),(#141635,#141636,#141637)),
 .UNSPECIFIED.,.F.,.F.,.F.)
B_SPLINE_SURFACE_WITH_KNOTS((2,2),(3,3),(0.,0.289807040991559),(0.194132688793568,
0.211606804210307),.UNSPECIFIED.)
GEOMETRIC_REPRESENTATION_ITEM()
RATIONAL_B_SPLINE_SURFACE(((0.989843896581211,0.992516389311155,0.998189888755647),
(0.98984389658121,0.992516389311155,0.998189888755647)))
REPRESENTATION_ITEM('')
SURFACE()
);
#2763=(
BOUNDED_SURFACE()
B_SPLINE_SURFACE(1,2,((#141654,#141655,#141656,#141657,#141658),(#141659,
#141660,#141661,#141662,#141663)),.UNSPECIFIED.,.F.,.F.,.F.)
B_SPLINE_SURFACE_WITH_KNOTS((2,2),(3,2,3),(0.,0.290272734861932),(0.521815037222016,
0.538999630513411,0.539591284248474),.UNSPECIFIED.)
GEOMETRIC_REPRESENTATION_ITEM()
RATIONAL_B_SPLINE_SURFACE(((0.989362668575565,0.987015160230477,0.987570037304351,
0.987570037304351,0.987570037304351),(0.989362668575565,0.987015160230477,
0.987570037304351,0.987570037304351,0.987570037304351)))
REPRESENTATION_ITEM('')
SURFACE()
);
#2764=(
BOUNDED_SURFACE()
B_SPLINE_SURFACE(1,2,((#141665,#141666,#141667),(#141668,#141669,#141670)),
 .UNSPECIFIED.,.F.,.F.,.F.)
B_SPLINE_SURFACE_WITH_KNOTS((2,2),(3,3),(0.,0.289807040991563),(0.194132688793568,
0.211606804210303),.UNSPECIFIED.)
GEOMETRIC_REPRESENTATION_ITEM()
RATIONAL_B_SPLINE_SURFACE(((0.989843896581211,0.992516389311155,0.998189888755645),
(0.989843896581211,0.992516389311155,0.998189888755645)))
REPRESENTATION_ITEM('')
SURFACE()
);
#2765=(
BOUNDED_SURFACE()
B_SPLINE_SURFACE(1,2,((#141687,#141688,#141689,#141690,#141691),(#141692,
#141693,#141694,#141695,#141696)),.UNSPECIFIED.,.F.,.F.,.F.)
B_SPLINE_SURFACE_WITH_KNOTS((2,2),(3,2,3),(0.,0.290272734862812),(0.521815037221715,
0.538999630513411,0.539591284249576),.UNSPECIFIED.)
GEOMETRIC_REPRESENTATION_ITEM()
RATIONAL_B_SPLINE_SURFACE(((0.989362668575647,0.987015160230467,0.987570037304351,
0.987570037304351,0.987570037304351),(0.989362668575647,0.987015160230467,
0.987570037304351,0.987570037304351,0.987570037304351)))
REPRESENTATION_ITEM('')
SURFACE()
);
#2766=(
BOUNDED_SURFACE()
B_SPLINE_SURFACE(1,2,((#141698,#141699,#141700),(#141701,#141702,#141703)),
 .UNSPECIFIED.,.F.,.F.,.F.)
B_SPLINE_SURFACE_WITH_KNOTS((2,2),(3,3),(0.,0.289807040991562),(0.194132688793568,
0.211606804210307),.UNSPECIFIED.)
GEOMETRIC_REPRESENTATION_ITEM()
RATIONAL_B_SPLINE_SURFACE(((0.989843896581211,0.992516389311156,0.998189888755648),
(0.989843896581211,0.992516389311156,0.998189888755648)))
REPRESENTATION_ITEM('')
SURFACE()
);
#2767=(
BOUNDED_SURFACE()
B_SPLINE_SURFACE(1,2,((#141720,#141721,#141722,#141723,#141724),(#141725,
#141726,#141727,#141728,#141729)),.UNSPECIFIED.,.F.,.F.,.F.)
B_SPLINE_SURFACE_WITH_KNOTS((2,2),(3,2,3),(0.,0.290272734843879),(0.521815037222017,
0.538999630513411,0.539591284230428),.UNSPECIFIED.)
GEOMETRIC_REPRESENTATION_ITEM()
RATIONAL_B_SPLINE_SURFACE(((0.989362668575565,0.987015160230477,0.987570037304351,
0.987570037304351,0.987570037304351),(0.989362668575565,0.987015160230477,
0.987570037304351,0.987570037304351,0.987570037304351)))
REPRESENTATION_ITEM('')
SURFACE()
);
#2768=(
BOUNDED_SURFACE()
B_SPLINE_SURFACE(1,2,((#141731,#141732,#141733),(#141734,#141735,#141736)),
 .UNSPECIFIED.,.F.,.F.,.F.)
B_SPLINE_SURFACE_WITH_KNOTS((2,2),(3,3),(0.,0.289807040991565),(0.194132688793568,
0.211606804210307),.UNSPECIFIED.)
GEOMETRIC_REPRESENTATION_ITEM()
RATIONAL_B_SPLINE_SURFACE(((0.989843896581211,0.992516389311156,0.998189888755648),
(0.989843896581211,0.992516389311156,0.998189888755648)))
REPRESENTATION_ITEM('')
SURFACE()
);
#2769=(
BOUNDED_SURFACE()
B_SPLINE_SURFACE(1,2,((#141753,#141754,#141755,#141756,#141757),(#141758,
#141759,#141760,#141761,#141762)),.UNSPECIFIED.,.F.,.F.,.F.)
B_SPLINE_SURFACE_WITH_KNOTS((2,2),(3,2,3),(0.,0.290272734865575),(0.52181503722185,
0.538999630513411,0.539591284252381),.UNSPECIFIED.)
GEOMETRIC_REPRESENTATION_ITEM()
RATIONAL_B_SPLINE_SURFACE(((0.989362668575611,0.987015160230471,0.987570037304351,
0.987570037304351,0.987570037304351),(0.989362668575611,0.987015160230471,
0.987570037304351,0.987570037304351,0.987570037304351)))
REPRESENTATION_ITEM('')
SURFACE()
);
#2770=(
BOUNDED_SURFACE()
B_SPLINE_SURFACE(1,2,((#141764,#141765,#141766),(#141767,#141768,#141769)),
 .UNSPECIFIED.,.F.,.F.,.F.)
B_SPLINE_SURFACE_WITH_KNOTS((2,2),(3,3),(0.,0.289807040991564),(0.194132688793568,
0.211606804210307),.UNSPECIFIED.)
GEOMETRIC_REPRESENTATION_ITEM()
RATIONAL_B_SPLINE_SURFACE(((0.989843896581211,0.992516389311155,0.998189888755648),
(0.989843896581211,0.992516389311155,0.998189888755648)))
REPRESENTATION_ITEM('')
SURFACE()
);
#2771=(
BOUNDED_SURFACE()
B_SPLINE_SURFACE(1,2,((#141786,#141787,#141788,#141789,#141790),(#141791,
#141792,#141793,#141794,#141795)),.UNSPECIFIED.,.F.,.F.,.F.)
B_SPLINE_SURFACE_WITH_KNOTS((2,2),(3,2,3),(0.,0.290272734871367),(0.52181503722181,
0.538999630513411,0.539591284258078),.UNSPECIFIED.)
GEOMETRIC_REPRESENTATION_ITEM()
RATIONAL_B_SPLINE_SURFACE(((0.989362668575621,0.98701516023047,0.987570037304351,
0.987570037304351,0.987570037304351),(0.989362668575621,0.98701516023047,
0.987570037304351,0.987570037304351,0.987570037304351)))
REPRESENTATION_ITEM('')
SURFACE()
);
#2772=(
BOUNDED_SURFACE()
B_SPLINE_SURFACE(1,2,((#141797,#141798,#141799),(#141800,#141801,#141802)),
 .UNSPECIFIED.,.F.,.F.,.F.)
B_SPLINE_SURFACE_WITH_KNOTS((2,2),(3,3),(0.,0.289807040991565),(0.194132688793568,
0.211606804210307),.UNSPECIFIED.)
GEOMETRIC_REPRESENTATION_ITEM()
RATIONAL_B_SPLINE_SURFACE(((0.989843896581211,0.992516389311155,0.998189888755648),
(0.989843896581211,0.992516389311155,0.998189888755648)))
REPRESENTATION_ITEM('')
SURFACE()
);
#2773=(
BOUNDED_SURFACE()
B_SPLINE_SURFACE(1,2,((#141819,#141820,#141821,#141822,#141823),(#141824,
#141825,#141826,#141827,#141828)),.UNSPECIFIED.,.F.,.F.,.F.)
B_SPLINE_SURFACE_WITH_KNOTS((2,2),(3,2,3),(0.,0.290272734855448),(0.521815037221533,
0.538999630513411,0.539591284242046),.UNSPECIFIED.)
GEOMETRIC_REPRESENTATION_ITEM()
RATIONAL_B_SPLINE_SURFACE(((0.989362668575697,0.987015160230461,0.987570037304351,
0.987570037304351,0.987570037304351),(0.989362668575697,0.987015160230461,
0.987570037304351,0.987570037304351,0.987570037304351)))
REPRESENTATION_ITEM('')
SURFACE()
);
#2774=(
BOUNDED_SURFACE()
B_SPLINE_SURFACE(1,2,((#141830,#141831,#141832),(#141833,#141834,#141835)),
 .UNSPECIFIED.,.F.,.F.,.F.)
B_SPLINE_SURFACE_WITH_KNOTS((2,2),(3,3),(0.,0.28980704099156),(0.194132688793568,
0.211606804210307),.UNSPECIFIED.)
GEOMETRIC_REPRESENTATION_ITEM()
RATIONAL_B_SPLINE_SURFACE(((0.989843896581211,0.992516389311155,0.998189888755648),
(0.989843896581211,0.992516389311155,0.998189888755648)))
REPRESENTATION_ITEM('')
SURFACE()
);
#2775=(
BOUNDED_SURFACE()
B_SPLINE_SURFACE(1,2,((#141843,#141844,#141845,#141846,#141847),(#141848,
#141849,#141850,#141851,#141852)),.UNSPECIFIED.,.F.,.F.,.F.)
B_SPLINE_SURFACE_WITH_KNOTS((2,2),(3,2,3),(0.,0.290272734861199),(0.521815037221924,
0.538999630513411,0.539591284247793),.UNSPECIFIED.)
GEOMETRIC_REPRESENTATION_ITEM()
RATIONAL_B_SPLINE_SURFACE(((0.98936266857559,0.987015160230474,0.987570037304351,
0.987570037304351,0.987570037304351),(0.98936266857559,0.987015160230474,
0.987570037304351,0.987570037304351,0.987570037304351)))
REPRESENTATION_ITEM('')
SURFACE()
);
#2776=(
BOUNDED_SURFACE()
B_SPLINE_SURFACE(1,2,((#141854,#141855,#141856),(#141857,#141858,#141859)),
 .UNSPECIFIED.,.F.,.F.,.F.)
B_SPLINE_SURFACE_WITH_KNOTS((2,2),(3,3),(0.,0.289807040991564),(0.194132688793568,
0.211606804210307),.UNSPECIFIED.)
GEOMETRIC_REPRESENTATION_ITEM()
RATIONAL_B_SPLINE_SURFACE(((0.989843896581211,0.992516389311156,0.998189888755648),
(0.989843896581211,0.992516389311156,0.998189888755648)))
REPRESENTATION_ITEM('')
SURFACE()
);
#2777=(
BOUNDED_SURFACE()
B_SPLINE_SURFACE(1,2,((#141876,#141877,#141878,#141879,#141880),(#141881,
#141882,#141883,#141884,#141885)),.UNSPECIFIED.,.F.,.F.,.F.)
B_SPLINE_SURFACE_WITH_KNOTS((2,2),(3,2,3),(0.,0.290272734855005),(0.521815037222017,
0.538999630513411,0.539591284241809),.UNSPECIFIED.)
GEOMETRIC_REPRESENTATION_ITEM()
RATIONAL_B_SPLINE_SURFACE(((0.989362668575565,0.987015160230477,0.987570037304351,
0.987570037304351,0.987570037304351),(0.989362668575565,0.987015160230477,
0.987570037304351,0.987570037304351,0.987570037304351)))
REPRESENTATION_ITEM('')
SURFACE()
);
#2778=(
BOUNDED_SURFACE()
B_SPLINE_SURFACE(1,2,((#141887,#141888,#141889),(#141890,#141891,#141892)),
 .UNSPECIFIED.,.F.,.F.,.F.)
B_SPLINE_SURFACE_WITH_KNOTS((2,2),(3,3),(0.,0.28980704099156),(0.194132688793568,
0.211606804210307),.UNSPECIFIED.)
GEOMETRIC_REPRESENTATION_ITEM()
RATIONAL_B_SPLINE_SURFACE(((0.98984389658121,0.992516389311155,0.998189888755648),
(0.98984389658121,0.992516389311155,0.998189888755648)))
REPRESENTATION_ITEM('')
SURFACE()
);
#2779=(
BOUNDED_SURFACE()
B_SPLINE_SURFACE(1,2,((#141909,#141910,#141911,#141912,#141913),(#141914,
#141915,#141916,#141917,#141918)),.UNSPECIFIED.,.F.,.F.,.F.)
B_SPLINE_SURFACE_WITH_KNOTS((2,2),(3,2,3),(0.,0.290272734863187),(0.521815037222017,
0.538999630513411,0.539591284249797),.UNSPECIFIED.)
GEOMETRIC_REPRESENTATION_ITEM()
RATIONAL_B_SPLINE_SURFACE(((0.989362668575565,0.987015160230477,0.987570037304351,
0.987570037304351,0.987570037304351),(0.989362668575565,0.987015160230477,
0.987570037304351,0.987570037304351,0.987570037304351)))
REPRESENTATION_ITEM('')
SURFACE()
);
#2780=(
BOUNDED_SURFACE()
B_SPLINE_SURFACE(1,2,((#141920,#141921,#141922),(#141923,#141924,#141925)),
 .UNSPECIFIED.,.F.,.F.,.F.)
B_SPLINE_SURFACE_WITH_KNOTS((2,2),(3,3),(0.,0.289807040991561),(0.194132688793568,
0.211606804210307),.UNSPECIFIED.)
GEOMETRIC_REPRESENTATION_ITEM()
RATIONAL_B_SPLINE_SURFACE(((0.989843896581211,0.992516389311156,0.998189888755648),
(0.989843896581211,0.992516389311156,0.998189888755648)))
REPRESENTATION_ITEM('')
SURFACE()
);
#2781=(
BOUNDED_SURFACE()
B_SPLINE_SURFACE(1,2,((#141942,#141943,#141944,#141945,#141946),(#141947,
#141948,#141949,#141950,#141951)),.UNSPECIFIED.,.F.,.F.,.F.)
B_SPLINE_SURFACE_WITH_KNOTS((2,2),(3,2,3),(0.,0.2902727348764),(0.521815037222017,
0.538999630513411,0.539591284262947),.UNSPECIFIED.)
GEOMETRIC_REPRESENTATION_ITEM()
RATIONAL_B_SPLINE_SURFACE(((0.989362668575565,0.987015160230477,0.987570037304351,
0.987570037304351,0.987570037304351),(0.989362668575565,0.987015160230477,
0.987570037304351,0.987570037304351,0.987570037304351)))
REPRESENTATION_ITEM('')
SURFACE()
);
#2782=(
BOUNDED_SURFACE()
B_SPLINE_SURFACE(1,2,((#141953,#141954,#141955),(#141956,#141957,#141958)),
 .UNSPECIFIED.,.F.,.F.,.F.)
B_SPLINE_SURFACE_WITH_KNOTS((2,2),(3,3),(0.,0.289807040991562),(0.194132688793568,
0.211606804210307),.UNSPECIFIED.)
GEOMETRIC_REPRESENTATION_ITEM()
RATIONAL_B_SPLINE_SURFACE(((0.989843896581211,0.992516389311156,0.998189888755648),
(0.989843896581211,0.992516389311156,0.998189888755648)))
REPRESENTATION_ITEM('')
SURFACE()
);
#2783=(
BOUNDED_SURFACE()
B_SPLINE_SURFACE(1,2,((#141975,#141976,#141977,#141978,#141979),(#141980,
#141981,#141982,#141983,#141984)),.UNSPECIFIED.,.F.,.F.,.F.)
B_SPLINE_SURFACE_WITH_KNOTS((2,2),(3,2,3),(0.,0.290272734866835),(0.521815037222017,
0.538999630513411,0.539591284253334),.UNSPECIFIED.)
GEOMETRIC_REPRESENTATION_ITEM()
RATIONAL_B_SPLINE_SURFACE(((0.989362668575565,0.987015160230477,0.987570037304351,
0.987570037304351,0.987570037304351),(0.989362668575565,0.987015160230477,
0.987570037304351,0.987570037304351,0.987570037304351)))
REPRESENTATION_ITEM('')
SURFACE()
);
#2784=(
BOUNDED_SURFACE()
B_SPLINE_SURFACE(1,2,((#141986,#141987,#141988),(#141989,#141990,#141991)),
 .UNSPECIFIED.,.F.,.F.,.F.)
B_SPLINE_SURFACE_WITH_KNOTS((2,2),(3,3),(0.,0.289807040991556),(0.194132688793568,
0.211606804210307),.UNSPECIFIED.)
GEOMETRIC_REPRESENTATION_ITEM()
RATIONAL_B_SPLINE_SURFACE(((0.98984389658121,0.992516389311155,0.998189888755648),
(0.98984389658121,0.992516389311155,0.998189888755648)))
REPRESENTATION_ITEM('')
SURFACE()
);
#2785=(
BOUNDED_SURFACE()
B_SPLINE_SURFACE(1,2,((#142002,#142003,#142004,#142005,#142006),(#142007,
#142008,#142009,#142010,#142011)),.UNSPECIFIED.,.F.,.F.,.F.)
B_SPLINE_SURFACE_WITH_KNOTS((2,2),(3,2,3),(0.,0.290272727434781),(0.521815037222017,
0.538999630513411,0.539591276818006),.UNSPECIFIED.)
GEOMETRIC_REPRESENTATION_ITEM()
RATIONAL_B_SPLINE_SURFACE(((0.989362668575565,0.987015160230477,0.987570037304351,
0.987570037304351,0.987570037304351),(0.989362668575565,0.987015160230477,
0.987570037304351,0.987570037304351,0.987570037304351)))
REPRESENTATION_ITEM('')
SURFACE()
);
#2786=(
BOUNDED_SURFACE()
B_SPLINE_SURFACE(1,2,((#142019,#142020,#142021),(#142022,#142023,#142024)),
 .UNSPECIFIED.,.F.,.F.,.F.)
B_SPLINE_SURFACE_WITH_KNOTS((2,2),(3,3),(0.,0.28980704099156),(0.194132688793264,
0.211606804210309),.UNSPECIFIED.)
GEOMETRIC_REPRESENTATION_ITEM()
RATIONAL_B_SPLINE_SURFACE(((0.989843896581117,0.992516389311057,0.998189888755649),
(0.989843896581118,0.992516389311057,0.998189888755649)))
REPRESENTATION_ITEM('')
SURFACE()
);
#2787=(
BOUNDED_SURFACE()
B_SPLINE_SURFACE(1,2,((#142041,#142042,#142043,#142044,#142045),(#142046,
#142047,#142048,#142049,#142050)),.UNSPECIFIED.,.F.,.F.,.F.)
B_SPLINE_SURFACE_WITH_KNOTS((2,2),(3,2,3),(0.,0.290272734887809),(0.521815037221999,
0.538999630513411,0.539591284274294),.UNSPECIFIED.)
GEOMETRIC_REPRESENTATION_ITEM()
RATIONAL_B_SPLINE_SURFACE(((0.98936266857557,0.987015160230476,0.987570037304351,
0.987570037304351,0.987570037304351),(0.98936266857557,0.987015160230476,
0.987570037304351,0.987570037304351,0.987570037304351)))
REPRESENTATION_ITEM('')
SURFACE()
);
#2788=(
BOUNDED_SURFACE()
B_SPLINE_SURFACE(1,2,((#142052,#142053,#142054),(#142055,#142056,#142057)),
 .UNSPECIFIED.,.F.,.F.,.F.)
B_SPLINE_SURFACE_WITH_KNOTS((2,2),(3,3),(0.,0.289807040991945),(0.194132688793569,
0.211606804210309),.UNSPECIFIED.)
GEOMETRIC_REPRESENTATION_ITEM()
RATIONAL_B_SPLINE_SURFACE(((0.989843896581211,0.992516389311156,0.998189888755649),
(0.989843896581211,0.992516389311156,0.998189888755649)))
REPRESENTATION_ITEM('')
SURFACE()
);
#2789=(
BOUNDED_SURFACE()
B_SPLINE_SURFACE(1,2,((#142074,#142075,#142076,#142077,#142078),(#142079,
#142080,#142081,#142082,#142083)),.UNSPECIFIED.,.F.,.F.,.F.)
B_SPLINE_SURFACE_WITH_KNOTS((2,2),(3,2,3),(0.,0.290272734855651),(0.521815037222016,
0.53899963051341,0.539591284242329),.UNSPECIFIED.)
GEOMETRIC_REPRESENTATION_ITEM()
RATIONAL_B_SPLINE_SURFACE(((0.989362668575565,0.987015160230477,0.987570037304351,
0.987570037304351,0.987570037304351),(0.989362668575565,0.987015160230477,
0.987570037304351,0.987570037304351,0.987570037304351)))
REPRESENTATION_ITEM('')
SURFACE()
);
#2790=(
BOUNDED_SURFACE()
B_SPLINE_SURFACE(1,2,((#142085,#142086,#142087),(#142088,#142089,#142090)),
 .UNSPECIFIED.,.F.,.F.,.F.)
B_SPLINE_SURFACE_WITH_KNOTS((2,2),(3,3),(0.,0.289807040993353),(0.194132688793569,
0.211606804210308),.UNSPECIFIED.)
GEOMETRIC_REPRESENTATION_ITEM()
RATIONAL_B_SPLINE_SURFACE(((0.989843896581211,0.992516389311156,0.998189888755648),
(0.989843896581211,0.992516389311156,0.998189888755648)))
REPRESENTATION_ITEM('')
SURFACE()
);
#2791=(
BOUNDED_SURFACE()
B_SPLINE_SURFACE(1,2,((#142107,#142108,#142109,#142110,#142111),(#142112,
#142113,#142114,#142115,#142116)),.UNSPECIFIED.,.F.,.F.,.F.)
B_SPLINE_SURFACE_WITH_KNOTS((2,2),(3,2,3),(0.,0.290272734899145),(0.521815037222016,
0.53899963051341,0.539591284285509),.UNSPECIFIED.)
GEOMETRIC_REPRESENTATION_ITEM()
RATIONAL_B_SPLINE_SURFACE(((0.989362668575565,0.987015160230477,0.987570037304351,
0.987570037304351,0.987570037304351),(0.989362668575565,0.987015160230477,
0.987570037304351,0.987570037304351,0.987570037304351)))
REPRESENTATION_ITEM('')
SURFACE()
);
#2792=(
BOUNDED_SURFACE()
B_SPLINE_SURFACE(1,2,((#142118,#142119,#142120),(#142121,#142122,#142123)),
 .UNSPECIFIED.,.F.,.F.,.F.)
B_SPLINE_SURFACE_WITH_KNOTS((2,2),(3,3),(0.,0.289807040992025),(0.194132688793569,
0.211606804210308),.UNSPECIFIED.)
GEOMETRIC_REPRESENTATION_ITEM()
RATIONAL_B_SPLINE_SURFACE(((0.989843896581211,0.992516389311156,0.998189888755648),
(0.989843896581211,0.992516389311156,0.998189888755648)))
REPRESENTATION_ITEM('')
SURFACE()
);
#2793=(
BOUNDED_SURFACE()
B_SPLINE_SURFACE(1,2,((#142140,#142141,#142142,#142143,#142144),(#142145,
#142146,#142147,#142148,#142149)),.UNSPECIFIED.,.F.,.F.,.F.)
B_SPLINE_SURFACE_WITH_KNOTS((2,2),(3,2,3),(0.,0.290272734836377),(0.521815037222016,
0.53899963051341,0.539591284223044),.UNSPECIFIED.)
GEOMETRIC_REPRESENTATION_ITEM()
RATIONAL_B_SPLINE_SURFACE(((0.989362668575565,0.987015160230477,0.987570037304351,
0.987570037304351,0.987570037304351),(0.989362668575565,0.987015160230477,
0.987570037304351,0.987570037304351,0.987570037304351)))
REPRESENTATION_ITEM('')
SURFACE()
);
#2794=(
BOUNDED_SURFACE()
B_SPLINE_SURFACE(1,2,((#142151,#142152,#142153),(#142154,#142155,#142156)),
 .UNSPECIFIED.,.F.,.F.,.F.)
B_SPLINE_SURFACE_WITH_KNOTS((2,2),(3,3),(0.,0.289807040991644),(0.194132688793569,
0.211606804210308),.UNSPECIFIED.)
GEOMETRIC_REPRESENTATION_ITEM()
RATIONAL_B_SPLINE_SURFACE(((0.989843896581211,0.992516389311156,0.998189888755648),
(0.989843896581211,0.992516389311156,0.998189888755648)))
REPRESENTATION_ITEM('')
SURFACE()
);
#2795=(
BOUNDED_SURFACE()
B_SPLINE_SURFACE(1,2,((#142173,#142174,#142175,#142176,#142177),(#142178,
#142179,#142180,#142181,#142182)),.UNSPECIFIED.,.F.,.F.,.F.)
B_SPLINE_SURFACE_WITH_KNOTS((2,2),(3,2,3),(0.,0.290272734853426),(0.521815037222016,
0.53899963051341,0.539591284240079),.UNSPECIFIED.)
GEOMETRIC_REPRESENTATION_ITEM()
RATIONAL_B_SPLINE_SURFACE(((0.989362668575565,0.987015160230477,0.987570037304351,
0.987570037304351,0.987570037304351),(0.989362668575565,0.987015160230477,
0.987570037304351,0.987570037304351,0.987570037304351)))
REPRESENTATION_ITEM('')
SURFACE()
);
#2796=(
BOUNDED_SURFACE()
B_SPLINE_SURFACE(1,2,((#142184,#142185,#142186),(#142187,#142188,#142189)),
 .UNSPECIFIED.,.F.,.F.,.F.)
B_SPLINE_SURFACE_WITH_KNOTS((2,2),(3,3),(0.,0.28980704099164),(0.194132688793569,
0.211606804210308),.UNSPECIFIED.)
GEOMETRIC_REPRESENTATION_ITEM()
RATIONAL_B_SPLINE_SURFACE(((0.989843896581211,0.992516389311156,0.998189888755648),
(0.989843896581211,0.992516389311156,0.998189888755648)))
REPRESENTATION_ITEM('')
SURFACE()
);
#2797=(
BOUNDED_SURFACE()
B_SPLINE_SURFACE(1,2,((#142206,#142207,#142208,#142209,#142210),(#142211,
#142212,#142213,#142214,#142215)),.UNSPECIFIED.,.F.,.F.,.F.)
B_SPLINE_SURFACE_WITH_KNOTS((2,2),(3,2,3),(0.,0.290272734846835),(0.521815037222016,
0.53899963051341,0.539591284233596),.UNSPECIFIED.)
GEOMETRIC_REPRESENTATION_ITEM()
RATIONAL_B_SPLINE_SURFACE(((0.989362668575565,0.987015160230477,0.987570037304351,
0.987570037304351,0.987570037304351),(0.989362668575565,0.987015160230477,
0.987570037304351,0.987570037304351,0.987570037304351)))
REPRESENTATION_ITEM('')
SURFACE()
);
#2798=(
BOUNDED_SURFACE()
B_SPLINE_SURFACE(1,2,((#142217,#142218,#142219),(#142220,#142221,#142222)),
 .UNSPECIFIED.,.F.,.F.,.F.)
B_SPLINE_SURFACE_WITH_KNOTS((2,2),(3,3),(0.,0.289807040991632),(0.194132688793569,
0.211606804210308),.UNSPECIFIED.)
GEOMETRIC_REPRESENTATION_ITEM()
RATIONAL_B_SPLINE_SURFACE(((0.989843896581211,0.992516389311156,0.998189888755648),
(0.989843896581211,0.992516389311156,0.998189888755648)))
REPRESENTATION_ITEM('')
SURFACE()
);
#2799=(
BOUNDED_SURFACE()
B_SPLINE_SURFACE(1,2,((#142239,#142240,#142241,#142242,#142243),(#142244,
#142245,#142246,#142247,#142248)),.UNSPECIFIED.,.F.,.F.,.F.)
B_SPLINE_SURFACE_WITH_KNOTS((2,2),(3,2,3),(0.,0.290272734853011),(0.521815037222016,
0.53899963051341,0.539591284239539),.UNSPECIFIED.)
GEOMETRIC_REPRESENTATION_ITEM()
RATIONAL_B_SPLINE_SURFACE(((0.989362668575565,0.987015160230477,0.987570037304351,
0.987570037304351,0.987570037304351),(0.989362668575565,0.987015160230477,
0.987570037304351,0.987570037304351,0.987570037304351)))
REPRESENTATION_ITEM('')
SURFACE()
);
#2800=(
BOUNDED_SURFACE()
B_SPLINE_SURFACE(1,2,((#142250,#142251,#142252),(#142253,#142254,#142255)),
 .UNSPECIFIED.,.F.,.F.,.F.)
B_SPLINE_SURFACE_WITH_KNOTS((2,2),(3,3),(0.,0.289807040991908),(0.194132688793569,
0.211606804210308),.UNSPECIFIED.)
GEOMETRIC_REPRESENTATION_ITEM()
RATIONAL_B_SPLINE_SURFACE(((0.989843896581211,0.992516389311156,0.998189888755648),
(0.989843896581211,0.992516389311156,0.998189888755648)))
REPRESENTATION_ITEM('')
SURFACE()
);
#2801=(
BOUNDED_SURFACE()
B_SPLINE_SURFACE(1,2,((#142272,#142273,#142274,#142275,#142276),(#142277,
#142278,#142279,#142280,#142281)),.UNSPECIFIED.,.F.,.F.,.F.)
B_SPLINE_SURFACE_WITH_KNOTS((2,2),(3,2,3),(0.,0.290272734854809),(0.521815037222016,
0.53899963051341,0.539591284241502),.UNSPECIFIED.)
GEOMETRIC_REPRESENTATION_ITEM()
RATIONAL_B_SPLINE_SURFACE(((0.989362668575565,0.987015160230477,0.987570037304351,
0.987570037304351,0.987570037304351),(0.989362668575565,0.987015160230477,
0.987570037304351,0.987570037304351,0.987570037304351)))
REPRESENTATION_ITEM('')
SURFACE()
);
#2802=(
BOUNDED_SURFACE()
B_SPLINE_SURFACE(1,2,((#142283,#142284,#142285),(#142286,#142287,#142288)),
 .UNSPECIFIED.,.F.,.F.,.F.)
B_SPLINE_SURFACE_WITH_KNOTS((2,2),(3,3),(0.,0.289807040991557),(0.194132688793569,
0.211606804210308),.UNSPECIFIED.)
GEOMETRIC_REPRESENTATION_ITEM()
RATIONAL_B_SPLINE_SURFACE(((0.989843896581211,0.992516389311156,0.998189888755648),
(0.989843896581211,0.992516389311156,0.998189888755648)))
REPRESENTATION_ITEM('')
SURFACE()
);
#2803=(
BOUNDED_SURFACE()
B_SPLINE_SURFACE(1,2,((#142305,#142306,#142307,#142308,#142309),(#142310,
#142311,#142312,#142313,#142314)),.UNSPECIFIED.,.F.,.F.,.F.)
B_SPLINE_SURFACE_WITH_KNOTS((2,2),(3,2,3),(0.,0.290272734849359),(0.521815037222016,
0.53899963051341,0.53959128423595),.UNSPECIFIED.)
GEOMETRIC_REPRESENTATION_ITEM()
RATIONAL_B_SPLINE_SURFACE(((0.989362668575565,0.987015160230477,0.987570037304351,
0.987570037304351,0.987570037304351),(0.989362668575565,0.987015160230477,
0.987570037304351,0.987570037304351,0.987570037304351)))
REPRESENTATION_ITEM('')
SURFACE()
);
#2804=(
BOUNDED_SURFACE()
B_SPLINE_SURFACE(1,2,((#142316,#142317,#142318,#142319,#142320),(#142321,
#142322,#142323,#142324,#142325)),.UNSPECIFIED.,.F.,.F.,.F.)
B_SPLINE_SURFACE_WITH_KNOTS((2,2),(3,2,3),(0.710318915639631,1.),(0.573550810617452,
0.590910950629594,0.591084552029715),.UNSPECIFIED.)
GEOMETRIC_REPRESENTATION_ITEM()
RATIONAL_B_SPLINE_SURFACE(((0.998554414400195,0.992822941359326,0.990053454406147,
0.990053454406147,0.990053454406147),(0.998554414400195,0.992822941359326,
0.990053454406147,0.990053454406147,0.990053454406147)))
REPRESENTATION_ITEM('')
SURFACE()
);
#2805=(
BOUNDED_SURFACE()
B_SPLINE_SURFACE(1,2,((#142336,#142337,#142338,#142339,#142340,#142341,
#142342),(#142343,#142344,#142345,#142346,#142347,#142348,#142349)),
 .UNSPECIFIED.,.F.,.F.,.F.)
B_SPLINE_SURFACE_WITH_KNOTS((2,2),(3,2,2,3),(0.710192959007995,1.),(0.142404283483303,
0.142578551421364,0.142857142857143,0.160005345227479),.UNSPECIFIED.)
GEOMETRIC_REPRESENTATION_ITEM()
RATIONAL_B_SPLINE_SURFACE(((0.999805186472059,0.999805186472059,0.999805186472059,
0.999902211834795,1.,0.993980822699459,0.990851751371591),(0.999805186472059,
0.999805186472059,0.999805186472059,0.999902211834795,1.,0.993980822699459,
0.990851751371591)))
REPRESENTATION_ITEM('')
SURFACE()
);
#2806=(
BOUNDED_SURFACE()
B_SPLINE_SURFACE(1,2,((#142357,#142358,#142359,#142360,#142361),(#142362,
#142363,#142364,#142365,#142366)),.UNSPECIFIED.,.F.,.F.,.F.)
B_SPLINE_SURFACE_WITH_KNOTS((2,2),(3,2,3),(0.71031891563998,1.),(0.573550810617373,
0.590910950629594,0.591084552029716),.UNSPECIFIED.)
GEOMETRIC_REPRESENTATION_ITEM()
RATIONAL_B_SPLINE_SURFACE(((0.998554414400247,0.992822941359339,0.990053454406147,
0.990053454406147,0.990053454406147),(0.998554414400247,0.992822941359339,
0.990053454406147,0.990053454406147,0.990053454406147)))
REPRESENTATION_ITEM('')
SURFACE()
);
#2807=(
BOUNDED_SURFACE()
B_SPLINE_SURFACE(1,2,((#142377,#142378,#142379,#142380,#142381,#142382,
#142383),(#142384,#142385,#142386,#142387,#142388,#142389,#142390)),
 .UNSPECIFIED.,.F.,.F.,.F.)
B_SPLINE_SURFACE_WITH_KNOTS((2,2),(3,2,2,3),(0.710192959008341,1.),(0.142404283483303,
0.142578551421364,0.142857142857143,0.160005345227478),.UNSPECIFIED.)
GEOMETRIC_REPRESENTATION_ITEM()
RATIONAL_B_SPLINE_SURFACE(((0.999805186472059,0.999805186472059,0.999805186472059,
0.999902211834795,1.,0.993980822699459,0.990851751371591),(0.999805186472059,
0.999805186472059,0.999805186472059,0.999902211834795,1.,0.993980822699459,
0.990851751371591)))
REPRESENTATION_ITEM('')
SURFACE()
);
#2808=(
BOUNDED_SURFACE()
B_SPLINE_SURFACE(1,2,((#142398,#142399,#142400,#142401,#142402),(#142403,
#142404,#142405,#142406,#142407)),.UNSPECIFIED.,.F.,.F.,.F.)
B_SPLINE_SURFACE_WITH_KNOTS((2,2),(3,2,3),(0.710318915639972,1.),(0.573550810617452,
0.590910950629594,0.591084552029715),.UNSPECIFIED.)
GEOMETRIC_REPRESENTATION_ITEM()
RATIONAL_B_SPLINE_SURFACE(((0.998554414400195,0.992822941359326,0.990053454406148,
0.990053454406148,0.990053454406148),(0.998554414400195,0.992822941359326,
0.990053454406148,0.990053454406148,0.990053454406148)))
REPRESENTATION_ITEM('')
SURFACE()
);
#2809=(
BOUNDED_SURFACE()
B_SPLINE_SURFACE(1,2,((#142418,#142419,#142420,#142421,#142422,#142423,
#142424),(#142425,#142426,#142427,#142428,#142429,#142430,#142431)),
 .UNSPECIFIED.,.F.,.F.,.F.)
B_SPLINE_SURFACE_WITH_KNOTS((2,2),(3,2,2,3),(0.710192959008339,1.),(0.142404283483303,
0.142578551421364,0.142857142857143,0.160005345227479),.UNSPECIFIED.)
GEOMETRIC_REPRESENTATION_ITEM()
RATIONAL_B_SPLINE_SURFACE(((0.999805186472059,0.999805186472059,0.999805186472059,
0.999902211834795,1.,0.993980822699459,0.990851751371591),(0.999805186472059,
0.999805186472059,0.999805186472059,0.999902211834795,1.,0.993980822699459,
0.990851751371591)))
REPRESENTATION_ITEM('')
SURFACE()
);
#2810=(
BOUNDED_SURFACE()
B_SPLINE_SURFACE(1,2,((#142439,#142440,#142441,#142442,#142443),(#142444,
#142445,#142446,#142447,#142448)),.UNSPECIFIED.,.F.,.F.,.F.)
B_SPLINE_SURFACE_WITH_KNOTS((2,2),(3,2,3),(0.710318915639019,1.),(0.573550810617371,
0.590910950629594,0.591084552029716),.UNSPECIFIED.)
GEOMETRIC_REPRESENTATION_ITEM()
RATIONAL_B_SPLINE_SURFACE(((0.998554414400249,0.992822941359339,0.990053454406148,
0.990053454406148,0.990053454406148),(0.998554414400249,0.992822941359339,
0.990053454406148,0.990053454406148,0.990053454406148)))
REPRESENTATION_ITEM('')
SURFACE()
);
#2811=(
BOUNDED_SURFACE()
B_SPLINE_SURFACE(1,2,((#142459,#142460,#142461,#142462,#142463,#142464,
#142465),(#142466,#142467,#142468,#142469,#142470,#142471,#142472)),
 .UNSPECIFIED.,.F.,.F.,.F.)
B_SPLINE_SURFACE_WITH_KNOTS((2,2),(3,2,2,3),(0.710192959007381,1.),(0.142404283483303,
0.142578551421364,0.142857142857143,0.160005345227478),.UNSPECIFIED.)
GEOMETRIC_REPRESENTATION_ITEM()
RATIONAL_B_SPLINE_SURFACE(((0.999805186472059,0.999805186472059,0.999805186472059,
0.999902211834795,1.,0.993980822699459,0.990851751371591),(0.999805186472059,
0.999805186472059,0.999805186472059,0.999902211834795,1.,0.993980822699459,
0.990851751371591)))
REPRESENTATION_ITEM('')
SURFACE()
);
#2812=(
BOUNDED_SURFACE()
B_SPLINE_SURFACE(1,2,((#142480,#142481,#142482,#142483,#142484),(#142485,
#142486,#142487,#142488,#142489)),.UNSPECIFIED.,.F.,.F.,.F.)
B_SPLINE_SURFACE_WITH_KNOTS((2,2),(3,2,3),(0.710318915639016,1.),(0.57355081061737,
0.590910950629594,0.591084552029716),.UNSPECIFIED.)
GEOMETRIC_REPRESENTATION_ITEM()
RATIONAL_B_SPLINE_SURFACE(((0.998554414400249,0.992822941359339,0.990053454406148,
0.990053454406148,0.990053454406148),(0.998554414400249,0.992822941359339,
0.990053454406148,0.990053454406148,0.990053454406148)))
REPRESENTATION_ITEM('')
SURFACE()
);
#2813=(
BOUNDED_SURFACE()
B_SPLINE_SURFACE(1,2,((#142500,#142501,#142502,#142503,#142504,#142505,
#142506),(#142507,#142508,#142509,#142510,#142511,#142512,#142513)),
 .UNSPECIFIED.,.F.,.F.,.F.)
B_SPLINE_SURFACE_WITH_KNOTS((2,2),(3,2,2,3),(0.710192959007377,1.),(0.142404283483303,
0.142578551421364,0.142857142857143,0.160005345227478),.UNSPECIFIED.)
GEOMETRIC_REPRESENTATION_ITEM()
RATIONAL_B_SPLINE_SURFACE(((0.999805186472059,0.999805186472059,0.999805186472059,
0.999902211834795,1.,0.993980822699459,0.990851751371591),(0.999805186472059,
0.999805186472059,0.999805186472059,0.999902211834795,1.,0.993980822699459,
0.990851751371591)))
REPRESENTATION_ITEM('')
SURFACE()
);
#2814=(
BOUNDED_SURFACE()
B_SPLINE_SURFACE(1,2,((#142521,#142522,#142523,#142524,#142525),(#142526,
#142527,#142528,#142529,#142530)),.UNSPECIFIED.,.F.,.F.,.F.)
B_SPLINE_SURFACE_WITH_KNOTS((2,2),(3,2,3),(0.71031891563902,1.),(0.573550810617172,
0.590910950629594,0.591084552029718),.UNSPECIFIED.)
GEOMETRIC_REPRESENTATION_ITEM()
RATIONAL_B_SPLINE_SURFACE(((0.99855441440038,0.992822941359371,0.990053454406147,
0.990053454406147,0.990053454406147),(0.99855441440038,0.992822941359371,
0.990053454406147,0.990053454406147,0.990053454406147)))
REPRESENTATION_ITEM('')
SURFACE()
);
#2815=(
BOUNDED_SURFACE()
B_SPLINE_SURFACE(1,2,((#142541,#142542,#142543,#142544,#142545,#142546,
#142547),(#142548,#142549,#142550,#142551,#142552,#142553,#142554)),
 .UNSPECIFIED.,.F.,.F.,.F.)
B_SPLINE_SURFACE_WITH_KNOTS((2,2),(3,2,2,3),(0.71019295900738,1.),(0.142404283483303,
0.142578551421364,0.142857142857143,0.160005345227479),.UNSPECIFIED.)
GEOMETRIC_REPRESENTATION_ITEM()
RATIONAL_B_SPLINE_SURFACE(((0.999805186472059,0.999805186472059,0.999805186472059,
0.999902211834795,1.,0.993980822699459,0.990851751371591),(0.999805186472059,
0.999805186472059,0.999805186472059,0.999902211834795,1.,0.993980822699459,
0.990851751371591)))
REPRESENTATION_ITEM('')
SURFACE()
);
#2816=(
BOUNDED_SURFACE()
B_SPLINE_SURFACE(1,2,((#142562,#142563,#142564,#142565,#142566),(#142567,
#142568,#142569,#142570,#142571)),.UNSPECIFIED.,.F.,.F.,.F.)
B_SPLINE_SURFACE_WITH_KNOTS((2,2),(3,2,3),(0.710318915638433,1.),(0.573550810617371,
0.590910950629594,0.591084552029716),.UNSPECIFIED.)
GEOMETRIC_REPRESENTATION_ITEM()
RATIONAL_B_SPLINE_SURFACE(((0.998554414400249,0.992822941359339,0.990053454406148,
0.990053454406148,0.990053454406148),(0.998554414400249,0.992822941359339,
0.990053454406148,0.990053454406148,0.990053454406148)))
REPRESENTATION_ITEM('')
SURFACE()
);
#2817=(
BOUNDED_SURFACE()
B_SPLINE_SURFACE(1,2,((#142582,#142583,#142584,#142585,#142586,#142587,
#142588),(#142589,#142590,#142591,#142592,#142593,#142594,#142595)),
 .UNSPECIFIED.,.F.,.F.,.F.)
B_SPLINE_SURFACE_WITH_KNOTS((2,2),(3,2,2,3),(0.710192959006795,1.),(0.142404283483303,
0.142578551421364,0.142857142857143,0.160005345227478),.UNSPECIFIED.)
GEOMETRIC_REPRESENTATION_ITEM()
RATIONAL_B_SPLINE_SURFACE(((0.999805186472059,0.999805186472059,0.999805186472059,
0.999902211834795,1.,0.993980822699459,0.990851751371591),(0.999805186472059,
0.999805186472059,0.999805186472059,0.999902211834795,1.,0.993980822699459,
0.990851751371591)))
REPRESENTATION_ITEM('')
SURFACE()
);
#2818=(
BOUNDED_SURFACE()
B_SPLINE_SURFACE(1,2,((#142603,#142604,#142605,#142606,#142607),(#142608,
#142609,#142610,#142611,#142612)),.UNSPECIFIED.,.F.,.F.,.F.)
B_SPLINE_SURFACE_WITH_KNOTS((2,2),(3,2,3),(0.710318915639023,1.),(0.573550810617172,
0.590910950629594,0.591084552029718),.UNSPECIFIED.)
GEOMETRIC_REPRESENTATION_ITEM()
RATIONAL_B_SPLINE_SURFACE(((0.99855441440038,0.992822941359371,0.990053454406148,
0.990053454406148,0.990053454406148),(0.99855441440038,0.992822941359371,
0.990053454406148,0.990053454406148,0.990053454406148)))
REPRESENTATION_ITEM('')
SURFACE()
);
#2819=(
BOUNDED_SURFACE()
B_SPLINE_SURFACE(1,2,((#142623,#142624,#142625,#142626,#142627,#142628,
#142629),(#142630,#142631,#142632,#142633,#142634,#142635,#142636)),
 .UNSPECIFIED.,.F.,.F.,.F.)
B_SPLINE_SURFACE_WITH_KNOTS((2,2),(3,2,2,3),(0.710192959007378,1.),(0.142404283483303,
0.142578551421364,0.142857142857143,0.160005345227479),.UNSPECIFIED.)
GEOMETRIC_REPRESENTATION_ITEM()
RATIONAL_B_SPLINE_SURFACE(((0.999805186472059,0.999805186472059,0.999805186472059,
0.999902211834795,1.,0.993980822699459,0.990851751371591),(0.999805186472059,
0.999805186472059,0.999805186472059,0.999902211834795,1.,0.993980822699459,
0.990851751371591)))
REPRESENTATION_ITEM('')
SURFACE()
);
#2820=(
BOUNDED_SURFACE()
B_SPLINE_SURFACE(1,2,((#142644,#142645,#142646,#142647,#142648),(#142649,
#142650,#142651,#142652,#142653)),.UNSPECIFIED.,.F.,.F.,.F.)
B_SPLINE_SURFACE_WITH_KNOTS((2,2),(3,2,3),(0.710318915638463,1.),(0.573550810617452,
0.590910950629594,0.591084552029715),.UNSPECIFIED.)
GEOMETRIC_REPRESENTATION_ITEM()
RATIONAL_B_SPLINE_SURFACE(((0.998554414400195,0.992822941359326,0.990053454406147,
0.990053454406147,0.990053454406147),(0.998554414400195,0.992822941359326,
0.990053454406147,0.990053454406147,0.990053454406147)))
REPRESENTATION_ITEM('')
SURFACE()
);
#2821=(
BOUNDED_SURFACE()
B_SPLINE_SURFACE(1,2,((#142664,#142665,#142666,#142667,#142668,#142669,
#142670),(#142671,#142672,#142673,#142674,#142675,#142676,#142677)),
 .UNSPECIFIED.,.F.,.F.,.F.)
B_SPLINE_SURFACE_WITH_KNOTS((2,2),(3,2,2,3),(0.71019295900683,1.),(0.142404283483303,
0.142578551421364,0.142857142857143,0.160005345227479),.UNSPECIFIED.)
GEOMETRIC_REPRESENTATION_ITEM()
RATIONAL_B_SPLINE_SURFACE(((0.999805186472059,0.999805186472059,0.999805186472059,
0.999902211834795,1.,0.993980822699459,0.990851751371591),(0.999805186472059,
0.999805186472059,0.999805186472059,0.999902211834795,1.,0.993980822699459,
0.990851751371591)))
REPRESENTATION_ITEM('')
SURFACE()
);
#2822=(
BOUNDED_SURFACE()
B_SPLINE_SURFACE(1,2,((#142685,#142686,#142687,#142688,#142689),(#142690,
#142691,#142692,#142693,#142694)),.UNSPECIFIED.,.F.,.F.,.F.)
B_SPLINE_SURFACE_WITH_KNOTS((2,2),(3,2,3),(0.710318915638654,1.),(0.573550810617177,
0.590910950629594,0.591084552029718),.UNSPECIFIED.)
GEOMETRIC_REPRESENTATION_ITEM()
RATIONAL_B_SPLINE_SURFACE(((0.998554414400376,0.99282294135937,0.990053454406147,
0.990053454406147,0.990053454406147),(0.998554414400376,0.99282294135937,
0.990053454406147,0.990053454406147,0.990053454406147)))
REPRESENTATION_ITEM('')
SURFACE()
);
#2823=(
BOUNDED_SURFACE()
B_SPLINE_SURFACE(1,2,((#142705,#142706,#142707,#142708,#142709,#142710,
#142711),(#142712,#142713,#142714,#142715,#142716,#142717,#142718)),
 .UNSPECIFIED.,.F.,.F.,.F.)
B_SPLINE_SURFACE_WITH_KNOTS((2,2),(3,2,2,3),(0.710192959007013,1.),(0.142404283483303,
0.142578551421363,0.142857142857143,0.160005345227404),.UNSPECIFIED.)
GEOMETRIC_REPRESENTATION_ITEM()
RATIONAL_B_SPLINE_SURFACE(((0.999805186472058,0.999805186472058,0.999805186472058,
0.999902211834794,1.,0.993980822699486,0.990851751371619),(0.999805186472058,
0.999805186472058,0.999805186472058,0.999902211834794,1.,0.993980822699486,
0.990851751371619)))
REPRESENTATION_ITEM('')
SURFACE()
);
#2824=(
BOUNDED_SURFACE()
B_SPLINE_SURFACE(1,2,((#142726,#142727,#142728,#142729,#142730),(#142731,
#142732,#142733,#142734,#142735)),.UNSPECIFIED.,.F.,.F.,.F.)
B_SPLINE_SURFACE_WITH_KNOTS((2,2),(3,2,3),(0.710318915638625,1.),(0.573550810617173,
0.590910950629595,0.591084552029719),.UNSPECIFIED.)
GEOMETRIC_REPRESENTATION_ITEM()
RATIONAL_B_SPLINE_SURFACE(((0.998554414400379,0.99282294135937,0.990053454406147,
0.990053454406147,0.990053454406147),(0.998554414400379,0.99282294135937,
0.990053454406147,0.990053454406147,0.990053454406147)))
REPRESENTATION_ITEM('')
SURFACE()
);
#2825=(
BOUNDED_SURFACE()
B_SPLINE_SURFACE(1,2,((#142746,#142747,#142748,#142749,#142750,#142751,
#142752),(#142753,#142754,#142755,#142756,#142757,#142758,#142759)),
 .UNSPECIFIED.,.F.,.F.,.F.)
B_SPLINE_SURFACE_WITH_KNOTS((2,2),(3,2,2,3),(0.710192959006981,1.),(0.142404283483302,
0.142578551421363,0.142857142857143,0.160005345227478),.UNSPECIFIED.)
GEOMETRIC_REPRESENTATION_ITEM()
RATIONAL_B_SPLINE_SURFACE(((0.999805186472059,0.999805186472059,0.999805186472059,
0.999902211834794,1.,0.993980822699459,0.990851751371592),(0.999805186472059,
0.999805186472059,0.999805186472059,0.999902211834794,1.,0.993980822699459,
0.990851751371592)))
REPRESENTATION_ITEM('')
SURFACE()
);
#2826=(
BOUNDED_SURFACE()
B_SPLINE_SURFACE(1,2,((#142767,#142768,#142769,#142770,#142771),(#142772,
#142773,#142774,#142775,#142776)),.UNSPECIFIED.,.F.,.F.,.F.)
B_SPLINE_SURFACE_WITH_KNOTS((2,2),(3,2,3),(0.710318915638347,1.),(0.573550810617173,
0.590910950629595,0.591084552029719),.UNSPECIFIED.)
GEOMETRIC_REPRESENTATION_ITEM()
RATIONAL_B_SPLINE_SURFACE(((0.998554414400379,0.99282294135937,0.990053454406147,
0.990053454406147,0.990053454406147),(0.998554414400379,0.99282294135937,
0.990053454406147,0.990053454406147,0.990053454406147)))
REPRESENTATION_ITEM('')
SURFACE()
);
#2827=(
BOUNDED_SURFACE()
B_SPLINE_SURFACE(1,2,((#142787,#142788,#142789,#142790,#142791,#142792,
#142793),(#142794,#142795,#142796,#142797,#142798,#142799,#142800)),
 .UNSPECIFIED.,.F.,.F.,.F.)
B_SPLINE_SURFACE_WITH_KNOTS((2,2),(3,2,2,3),(0.7101929590067,1.),(0.142404283483302,
0.142578551421363,0.142857142857143,0.160005345227478),.UNSPECIFIED.)
GEOMETRIC_REPRESENTATION_ITEM()
RATIONAL_B_SPLINE_SURFACE(((0.999805186472058,0.999805186472058,0.999805186472058,
0.999902211834794,1.,0.993980822699459,0.990851751371591),(0.999805186472058,
0.999805186472058,0.999805186472058,0.999902211834794,1.,0.993980822699459,
0.990851751371591)))
REPRESENTATION_ITEM('')
SURFACE()
);
#2828=(
BOUNDED_SURFACE()
B_SPLINE_SURFACE(1,2,((#142808,#142809,#142810,#142811,#142812),(#142813,
#142814,#142815,#142816,#142817)),.UNSPECIFIED.,.F.,.F.,.F.)
B_SPLINE_SURFACE_WITH_KNOTS((2,2),(3,2,3),(0.710318915638931,1.),(0.573550810617173,
0.590910950629595,0.591084552029719),.UNSPECIFIED.)
GEOMETRIC_REPRESENTATION_ITEM()
RATIONAL_B_SPLINE_SURFACE(((0.998554414400379,0.99282294135937,0.990053454406147,
0.990053454406147,0.990053454406147),(0.998554414400379,0.99282294135937,
0.990053454406147,0.990053454406147,0.990053454406147)))
REPRESENTATION_ITEM('')
SURFACE()
);
#2829=(
BOUNDED_SURFACE()
B_SPLINE_SURFACE(1,2,((#142828,#142829,#142830,#142831,#142832,#142833,
#142834),(#142835,#142836,#142837,#142838,#142839,#142840,#142841)),
 .UNSPECIFIED.,.F.,.F.,.F.)
B_SPLINE_SURFACE_WITH_KNOTS((2,2),(3,2,2,3),(0.710192959007288,1.),(0.142404283483303,
0.142578551421363,0.142857142857143,0.160005345227401),.UNSPECIFIED.)
GEOMETRIC_REPRESENTATION_ITEM()
RATIONAL_B_SPLINE_SURFACE(((0.999805186472058,0.999805186472058,0.999805186472058,
0.999902211834794,1.,0.993980822699486,0.990851751371619),(0.999805186472058,
0.999805186472058,0.999805186472058,0.999902211834794,1.,0.993980822699486,
0.990851751371619)))
REPRESENTATION_ITEM('')
SURFACE()
);
#2830=(
BOUNDED_SURFACE()
B_SPLINE_SURFACE(1,2,((#142849,#142850,#142851,#142852,#142853),(#142854,
#142855,#142856,#142857,#142858)),.UNSPECIFIED.,.F.,.F.,.F.)
B_SPLINE_SURFACE_WITH_KNOTS((2,2),(3,2,3),(0.710318915638101,1.),(0.573550810617453,
0.590910950629595,0.591084552029716),.UNSPECIFIED.)
GEOMETRIC_REPRESENTATION_ITEM()
RATIONAL_B_SPLINE_SURFACE(((0.998554414400194,0.992822941359325,0.990053454406147,
0.990053454406147,0.990053454406147),(0.998554414400194,0.992822941359325,
0.990053454406147,0.990053454406147,0.990053454406147)))
REPRESENTATION_ITEM('')
SURFACE()
);
#2831=(
BOUNDED_SURFACE()
B_SPLINE_SURFACE(1,2,((#142869,#142870,#142871,#142872,#142873,#142874,
#142875),(#142876,#142877,#142878,#142879,#142880,#142881,#142882)),
 .UNSPECIFIED.,.F.,.F.,.F.)
B_SPLINE_SURFACE_WITH_KNOTS((2,2),(3,2,2,3),(0.710192959006456,1.),(0.142404283483302,
0.142578551421363,0.142857142857143,0.160005345227478),.UNSPECIFIED.)
GEOMETRIC_REPRESENTATION_ITEM()
RATIONAL_B_SPLINE_SURFACE(((0.999805186472058,0.999805186472058,0.999805186472058,
0.999902211834794,1.,0.993980822699459,0.990851751371591),(0.999805186472058,
0.999805186472058,0.999805186472058,0.999902211834794,1.,0.993980822699459,
0.990851751371591)))
REPRESENTATION_ITEM('')
SURFACE()
);
#2832=(
BOUNDED_SURFACE()
B_SPLINE_SURFACE(1,2,((#142890,#142891,#142892,#142893,#142894),(#142895,
#142896,#142897,#142898,#142899)),.UNSPECIFIED.,.F.,.F.,.F.)
B_SPLINE_SURFACE_WITH_KNOTS((2,2),(3,2,3),(0.710318915638601,1.),(0.573550810617173,
0.590910950629595,0.591084552029719),.UNSPECIFIED.)
GEOMETRIC_REPRESENTATION_ITEM()
RATIONAL_B_SPLINE_SURFACE(((0.998554414400379,0.99282294135937,0.990053454406147,
0.990053454406147,0.990053454406147),(0.998554414400379,0.99282294135937,
0.990053454406147,0.990053454406147,0.990053454406147)))
REPRESENTATION_ITEM('')
SURFACE()
);
#2833=(
BOUNDED_SURFACE()
B_SPLINE_SURFACE(1,2,((#142910,#142911,#142912,#142913,#142914,#142915,
#142916),(#142917,#142918,#142919,#142920,#142921,#142922,#142923)),
 .UNSPECIFIED.,.F.,.F.,.F.)
B_SPLINE_SURFACE_WITH_KNOTS((2,2),(3,2,2,3),(0.710192959006956,1.),(0.142404283483303,
0.142578551421363,0.142857142857143,0.160005345227402),.UNSPECIFIED.)
GEOMETRIC_REPRESENTATION_ITEM()
RATIONAL_B_SPLINE_SURFACE(((0.999805186472059,0.999805186472059,0.999805186472059,
0.999902211834794,1.,0.993980822699486,0.990851751371619),(0.999805186472059,
0.999805186472059,0.999805186472059,0.999902211834794,1.,0.993980822699486,
0.990851751371619)))
REPRESENTATION_ITEM('')
SURFACE()
);
#2834=(
BOUNDED_SURFACE()
B_SPLINE_SURFACE(1,2,((#142931,#142932,#142933,#142934,#142935),(#142936,
#142937,#142938,#142939,#142940)),.UNSPECIFIED.,.F.,.F.,.F.)
B_SPLINE_SURFACE_WITH_KNOTS((2,2),(3,2,3),(0.710318915638125,1.),(0.573550810617373,
0.590910950629595,0.591084552029717),.UNSPECIFIED.)
GEOMETRIC_REPRESENTATION_ITEM()
RATIONAL_B_SPLINE_SURFACE(((0.998554414400247,0.992822941359338,0.990053454406147,
0.990053454406147,0.990053454406147),(0.998554414400247,0.992822941359338,
0.990053454406147,0.990053454406147,0.990053454406147)))
REPRESENTATION_ITEM('')
SURFACE()
);
#2835=(
BOUNDED_SURFACE()
B_SPLINE_SURFACE(1,2,((#142951,#142952,#142953,#142954,#142955,#142956,
#142957),(#142958,#142959,#142960,#142961,#142962,#142963,#142964)),
 .UNSPECIFIED.,.F.,.F.,.F.)
B_SPLINE_SURFACE_WITH_KNOTS((2,2),(3,2,2,3),(0.710192959006485,1.),(0.142404283483302,
0.142578551421363,0.142857142857143,0.160005345227477),.UNSPECIFIED.)
GEOMETRIC_REPRESENTATION_ITEM()
RATIONAL_B_SPLINE_SURFACE(((0.999805186472059,0.999805186472059,0.999805186472059,
0.999902211834794,1.,0.99398082269946,0.990851751371592),(0.999805186472059,
0.999805186472059,0.999805186472059,0.999902211834794,1.,0.99398082269946,
0.990851751371592)))
REPRESENTATION_ITEM('')
SURFACE()
);
#2836=(
BOUNDED_SURFACE()
B_SPLINE_SURFACE(1,2,((#142972,#142973,#142974,#142975,#142976),(#142977,
#142978,#142979,#142980,#142981)),.UNSPECIFIED.,.F.,.F.,.F.)
B_SPLINE_SURFACE_WITH_KNOTS((2,2),(3,2,3),(0.710318915638373,1.),(0.573550810617177,
0.590910950629595,0.591084552029719),.UNSPECIFIED.)
GEOMETRIC_REPRESENTATION_ITEM()
RATIONAL_B_SPLINE_SURFACE(((0.998554414400376,0.992822941359369,0.990053454406147,
0.990053454406147,0.990053454406147),(0.998554414400376,0.992822941359369,
0.990053454406147,0.990053454406147,0.990053454406147)))
REPRESENTATION_ITEM('')
SURFACE()
);
#2837=(
BOUNDED_SURFACE()
B_SPLINE_SURFACE(1,2,((#142992,#142993,#142994,#142995,#142996,#142997,
#142998),(#142999,#143000,#143001,#143002,#143003,#143004,#143005)),
 .UNSPECIFIED.,.F.,.F.,.F.)
B_SPLINE_SURFACE_WITH_KNOTS((2,2),(3,2,2,3),(0.710192959006736,1.),(0.142404283483303,
0.142578551421363,0.142857142857143,0.160005345227404),.UNSPECIFIED.)
GEOMETRIC_REPRESENTATION_ITEM()
RATIONAL_B_SPLINE_SURFACE(((0.999805186472058,0.999805186472058,0.999805186472058,
0.999902211834794,1.,0.993980822699486,0.990851751371619),(0.999805186472058,
0.999805186472058,0.999805186472058,0.999902211834794,1.,0.993980822699486,
0.990851751371619)))
REPRESENTATION_ITEM('')
SURFACE()
);
#2838=(
BOUNDED_SURFACE()
B_SPLINE_SURFACE(1,2,((#143013,#143014,#143015,#143016,#143017),(#143018,
#143019,#143020,#143021,#143022)),.UNSPECIFIED.,.F.,.F.,.F.)
B_SPLINE_SURFACE_WITH_KNOTS((2,2),(3,2,3),(0.710318915637221,1.),(0.573550810617203,
0.590910950629595,0.591084552029719),.UNSPECIFIED.)
GEOMETRIC_REPRESENTATION_ITEM()
RATIONAL_B_SPLINE_SURFACE(((0.998554414400359,0.992822941359365,0.990053454406147,
0.990053454406147,0.990053454406147),(0.998554414400359,0.992822941359365,
0.990053454406147,0.990053454406147,0.990053454406147)))
REPRESENTATION_ITEM('')
SURFACE()
);
#2839=(
BOUNDED_SURFACE()
B_SPLINE_SURFACE(1,2,((#143033,#143034,#143035,#143036,#143037,#143038,
#143039),(#143040,#143041,#143042,#143043,#143044,#143045,#143046)),
 .UNSPECIFIED.,.F.,.F.,.F.)
B_SPLINE_SURFACE_WITH_KNOTS((2,2),(3,2,2,3),(0.710192959005574,1.),(0.142404283483302,
0.142578551421363,0.142857142857143,0.160005345227478),.UNSPECIFIED.)
GEOMETRIC_REPRESENTATION_ITEM()
RATIONAL_B_SPLINE_SURFACE(((0.999805186472059,0.999805186472059,0.999805186472059,
0.999902211834794,1.,0.993980822699459,0.990851751371591),(0.999805186472059,
0.999805186472059,0.999805186472059,0.999902211834794,1.,0.993980822699459,
0.990851751371591)))
REPRESENTATION_ITEM('')
SURFACE()
);
#2840=(
BOUNDED_SURFACE()
B_SPLINE_SURFACE(1,2,((#143054,#143055,#143056,#143057,#143058),(#143059,
#143060,#143061,#143062,#143063)),.UNSPECIFIED.,.F.,.F.,.F.)
B_SPLINE_SURFACE_WITH_KNOTS((2,2),(3,2,3),(0.710318915638881,1.),(0.573550810617188,
0.590910950629595,0.591084552029719),.UNSPECIFIED.)
GEOMETRIC_REPRESENTATION_ITEM()
RATIONAL_B_SPLINE_SURFACE(((0.998554414400369,0.992822941359368,0.990053454406147,
0.990053454406147,0.990053454406147),(0.998554414400369,0.992822941359368,
0.990053454406147,0.990053454406147,0.990053454406147)))
REPRESENTATION_ITEM('')
SURFACE()
);
#2841=(
BOUNDED_SURFACE()
B_SPLINE_SURFACE(1,2,((#143074,#143075,#143076,#143077,#143078,#143079,
#143080),(#143081,#143082,#143083,#143084,#143085,#143086,#143087)),
 .UNSPECIFIED.,.F.,.F.,.F.)
B_SPLINE_SURFACE_WITH_KNOTS((2,2),(3,2,2,3),(0.710192959007234,1.),(0.142404283483302,
0.142578551421363,0.142857142857143,0.160005345227477),.UNSPECIFIED.)
GEOMETRIC_REPRESENTATION_ITEM()
RATIONAL_B_SPLINE_SURFACE(((0.999805186472058,0.999805186472058,0.999805186472058,
0.999902211834794,1.,0.99398082269946,0.990851751371592),(0.999805186472058,
0.999805186472058,0.999805186472058,0.999902211834794,1.,0.99398082269946,
0.990851751371592)))
REPRESENTATION_ITEM('')
SURFACE()
);
#2842=(
BOUNDED_SURFACE()
B_SPLINE_SURFACE(1,2,((#143095,#143096,#143097,#143098,#143099),(#143100,
#143101,#143102,#143103,#143104)),.UNSPECIFIED.,.F.,.F.,.F.)
B_SPLINE_SURFACE_WITH_KNOTS((2,2),(3,2,3),(0.710318915638999,1.),(0.573550810617075,
0.590910950629595,0.59108455202972),.UNSPECIFIED.)
GEOMETRIC_REPRESENTATION_ITEM()
RATIONAL_B_SPLINE_SURFACE(((0.998554414400444,0.992822941359386,0.990053454406147,
0.990053454406147,0.990053454406147),(0.998554414400444,0.992822941359386,
0.990053454406147,0.990053454406147,0.990053454406147)))
REPRESENTATION_ITEM('')
SURFACE()
);
#2843=(
BOUNDED_SURFACE()
B_SPLINE_SURFACE(1,2,((#143115,#143116,#143117,#143118,#143119,#143120,
#143121),(#143122,#143123,#143124,#143125,#143126,#143127,#143128)),
 .UNSPECIFIED.,.F.,.F.,.F.)
B_SPLINE_SURFACE_WITH_KNOTS((2,2),(3,2,2,3),(0.710192959007354,1.),(0.142404283483302,
0.142578551421363,0.142857142857143,0.160005345227479),.UNSPECIFIED.)
GEOMETRIC_REPRESENTATION_ITEM()
RATIONAL_B_SPLINE_SURFACE(((0.999805186472058,0.999805186472058,0.999805186472058,
0.999902211834794,1.,0.993980822699459,0.990851751371591),(0.999805186472058,
0.999805186472058,0.999805186472058,0.999902211834794,1.,0.993980822699459,
0.990851751371591)))
REPRESENTATION_ITEM('')
SURFACE()
);
#2844=(
BOUNDED_SURFACE()
B_SPLINE_SURFACE(1,2,((#143136,#143137,#143138,#143139,#143140),(#143141,
#143142,#143143,#143144,#143145)),.UNSPECIFIED.,.F.,.F.,.F.)
B_SPLINE_SURFACE_WITH_KNOTS((2,2),(3,2,3),(0.710318915638156,1.),(0.573550810617127,
0.590910950629595,0.59108455202972),.UNSPECIFIED.)
GEOMETRIC_REPRESENTATION_ITEM()
RATIONAL_B_SPLINE_SURFACE(((0.99855441440041,0.992822941359378,0.990053454406147,
0.990053454406147,0.990053454406147),(0.99855441440041,0.992822941359377,
0.990053454406147,0.990053454406147,0.990053454406147)))
REPRESENTATION_ITEM('')
SURFACE()
);
#2845=(
BOUNDED_SURFACE()
B_SPLINE_SURFACE(1,2,((#143156,#143157,#143158,#143159,#143160,#143161,
#143162),(#143163,#143164,#143165,#143166,#143167,#143168,#143169)),
 .UNSPECIFIED.,.F.,.F.,.F.)
B_SPLINE_SURFACE_WITH_KNOTS((2,2),(3,2,2,3),(0.710192959006509,1.),(0.142404283483303,
0.142578551421363,0.142857142857143,0.160005345227408),.UNSPECIFIED.)
GEOMETRIC_REPRESENTATION_ITEM()
RATIONAL_B_SPLINE_SURFACE(((0.999805186472059,0.999805186472059,0.999805186472059,
0.999902211834794,1.,0.993980822699484,0.990851751371617),(0.999805186472059,
0.999805186472059,0.999805186472059,0.999902211834794,1.,0.993980822699484,
0.990851751371617)))
REPRESENTATION_ITEM('')
SURFACE()
);
#2846=(
BOUNDED_SURFACE()
B_SPLINE_SURFACE(1,2,((#143177,#143178,#143179,#143180,#143181),(#143182,
#143183,#143184,#143185,#143186)),.UNSPECIFIED.,.F.,.F.,.F.)
B_SPLINE_SURFACE_WITH_KNOTS((2,2),(3,2,3),(0.710318915639619,1.),(0.573550810617337,
0.590910950629595,0.591084552029718),.UNSPECIFIED.)
GEOMETRIC_REPRESENTATION_ITEM()
RATIONAL_B_SPLINE_SURFACE(((0.998554414400271,0.992822941359344,0.990053454406147,
0.990053454406147,0.990053454406147),(0.998554414400271,0.992822941359344,
0.990053454406147,0.990053454406147,0.990053454406147)))
REPRESENTATION_ITEM('')
SURFACE()
);
#2847=(
BOUNDED_SURFACE()
B_SPLINE_SURFACE(1,2,((#143194,#143195,#143196,#143197,#143198,#143199,
#143200),(#143201,#143202,#143203,#143204,#143205,#143206,#143207)),
 .UNSPECIFIED.,.F.,.F.,.F.)
B_SPLINE_SURFACE_WITH_KNOTS((2,2),(3,2,2,3),(0.710192959007984,1.),(0.142404283483302,
0.142578551421363,0.142857142857143,0.160005345227478),.UNSPECIFIED.)
GEOMETRIC_REPRESENTATION_ITEM()
RATIONAL_B_SPLINE_SURFACE(((0.999805186472059,0.999805186472059,0.999805186472059,
0.999902211834794,1.,0.993980822699459,0.990851751371592),(0.999805186472059,
0.999805186472059,0.999805186472059,0.999902211834794,1.,0.993980822699459,
0.990851751371591)))
REPRESENTATION_ITEM('')
SURFACE()
);
#2848=(
BOUNDED_SURFACE()
B_SPLINE_SURFACE(1,2,((#143209,#143210,#143211,#143212,#143213),(#143214,
#143215,#143216,#143217,#143218)),.UNSPECIFIED.,.F.,.F.,.F.)
B_SPLINE_SURFACE_WITH_KNOTS((2,2),(3,2,3),(0.710318915638755,1.),(0.573550810617439,
0.590910950629595,0.591084552029717),.UNSPECIFIED.)
GEOMETRIC_REPRESENTATION_ITEM()
RATIONAL_B_SPLINE_SURFACE(((0.998554414400204,0.992822941359328,0.990053454406147,
0.990053454406147,0.990053454406147),(0.998554414400204,0.992822941359328,
0.990053454406147,0.990053454406147,0.990053454406147)))
REPRESENTATION_ITEM('')
SURFACE()
);
#2849=(
BOUNDED_SURFACE()
B_SPLINE_SURFACE(1,2,((#143229,#143230,#143231,#143232,#143233,#143234,
#143235),(#143236,#143237,#143238,#143239,#143240,#143241,#143242)),
 .UNSPECIFIED.,.F.,.F.,.F.)
B_SPLINE_SURFACE_WITH_KNOTS((2,2),(3,2,2,3),(0.710192959007117,1.),(0.142404283483302,
0.142578551421363,0.142857142857143,0.160005345227477),.UNSPECIFIED.)
GEOMETRIC_REPRESENTATION_ITEM()
RATIONAL_B_SPLINE_SURFACE(((0.999805186472059,0.999805186472059,0.999805186472059,
0.999902211834794,1.,0.99398082269946,0.990851751371592),(0.999805186472059,
0.999805186472059,0.999805186472059,0.999902211834794,1.,0.99398082269946,
0.990851751371592)))
REPRESENTATION_ITEM('')
SURFACE()
);
#2850=(
BOUNDED_SURFACE()
B_SPLINE_SURFACE(1,2,((#143250,#143251,#143252,#143253,#143254),(#143255,
#143256,#143257,#143258,#143259)),.UNSPECIFIED.,.F.,.F.,.F.)
B_SPLINE_SURFACE_WITH_KNOTS((2,2),(3,2,3),(0.710318915638949,1.),(0.573550810617453,
0.590910950629595,0.591084552029716),.UNSPECIFIED.)
GEOMETRIC_REPRESENTATION_ITEM()
RATIONAL_B_SPLINE_SURFACE(((0.998554414400194,0.992822941359325,0.990053454406147,
0.990053454406147,0.990053454406147),(0.998554414400194,0.992822941359325,
0.990053454406147,0.990053454406147,0.990053454406147)))
REPRESENTATION_ITEM('')
SURFACE()
);
#2851=(
BOUNDED_SURFACE()
B_SPLINE_SURFACE(1,2,((#143270,#143271,#143272,#143273,#143274,#143275,
#143276),(#143277,#143278,#143279,#143280,#143281,#143282,#143283)),
 .UNSPECIFIED.,.F.,.F.,.F.)
B_SPLINE_SURFACE_WITH_KNOTS((2,2),(3,2,2,3),(0.710192959007312,1.),(0.142404283483302,
0.142578551421363,0.142857142857143,0.160005345227478),.UNSPECIFIED.)
GEOMETRIC_REPRESENTATION_ITEM()
RATIONAL_B_SPLINE_SURFACE(((0.999805186472059,0.999805186472059,0.999805186472059,
0.999902211834794,1.,0.993980822699459,0.990851751371591),(0.999805186472059,
0.999805186472059,0.999805186472059,0.999902211834794,1.,0.993980822699459,
0.990851751371591)))
REPRESENTATION_ITEM('')
SURFACE()
);
#2852=(
BOUNDED_SURFACE()
B_SPLINE_SURFACE(1,2,((#143291,#143292,#143293,#143294,#143295),(#143296,
#143297,#143298,#143299,#143300)),.UNSPECIFIED.,.F.,.F.,.F.)
B_SPLINE_SURFACE_WITH_KNOTS((2,2),(3,2,3),(0.710318915637703,1.),(0.573550810617427,
0.590910950629595,0.591084552029717),.UNSPECIFIED.)
GEOMETRIC_REPRESENTATION_ITEM()
RATIONAL_B_SPLINE_SURFACE(((0.998554414400211,0.992822941359329,0.990053454406147,
0.990053454406147,0.990053454406147),(0.998554414400211,0.992822941359329,
0.990053454406147,0.990053454406147,0.990053454406147)))
REPRESENTATION_ITEM('')
SURFACE()
);
#2853=(
BOUNDED_SURFACE()
B_SPLINE_SURFACE(1,2,((#143311,#143312,#143313,#143314,#143315,#143316,
#143317),(#143318,#143319,#143320,#143321,#143322,#143323,#143324)),
 .UNSPECIFIED.,.F.,.F.,.F.)
B_SPLINE_SURFACE_WITH_KNOTS((2,2),(3,2,2,3),(0.710192959006066,1.),(0.142404283483302,
0.142578551421363,0.142857142857143,0.160005345227477),.UNSPECIFIED.)
GEOMETRIC_REPRESENTATION_ITEM()
RATIONAL_B_SPLINE_SURFACE(((0.999805186472059,0.999805186472059,0.999805186472059,
0.999902211834794,1.,0.99398082269946,0.990851751371592),(0.999805186472059,
0.999805186472059,0.999805186472059,0.999902211834794,1.,0.99398082269946,
0.990851751371592)))
REPRESENTATION_ITEM('')
SURFACE()
);
#2854=(
BOUNDED_SURFACE()
B_SPLINE_SURFACE(1,2,((#143332,#143333,#143334,#143335,#143336),(#143337,
#143338,#143339,#143340,#143341)),.UNSPECIFIED.,.F.,.F.,.F.)
B_SPLINE_SURFACE_WITH_KNOTS((2,2),(3,2,3),(0.710318915639711,1.),(0.573550810617425,
0.590910950629665,0.591084552029787),.UNSPECIFIED.)
GEOMETRIC_REPRESENTATION_ITEM()
RATIONAL_B_SPLINE_SURFACE(((0.998554414400213,0.992822941359307,0.990053454406125,
0.990053454406125,0.990053454406125),(0.998554414400213,0.992822941359307,
0.990053454406125,0.990053454406125,0.990053454406125)))
REPRESENTATION_ITEM('')
SURFACE()
);
#2855=(
BOUNDED_SURFACE()
B_SPLINE_SURFACE(1,2,((#143352,#143353,#143354,#143355,#143356,#143357,
#143358),(#143359,#143360,#143361,#143362,#143363,#143364,#143365)),
 .UNSPECIFIED.,.F.,.F.,.F.)
B_SPLINE_SURFACE_WITH_KNOTS((2,2),(3,2,2,3),(0.71019295900807,1.),(0.142404283483303,
0.142578551421364,0.142857142857143,0.160005345227478),.UNSPECIFIED.)
GEOMETRIC_REPRESENTATION_ITEM()
RATIONAL_B_SPLINE_SURFACE(((0.999805186472059,0.999805186472059,0.999805186472059,
0.999902211834795,1.,0.993980822699459,0.990851751371591),(0.999805186472059,
0.999805186472059,0.999805186472059,0.999902211834795,1.,0.993980822699459,
0.990851751371591)))
REPRESENTATION_ITEM('')
SURFACE()
);
#2856=(
BOUNDED_SURFACE()
B_SPLINE_SURFACE(1,2,((#143373,#143374,#143375,#143376,#143377),(#143378,
#143379,#143380,#143381,#143382)),.UNSPECIFIED.,.F.,.F.,.F.)
B_SPLINE_SURFACE_WITH_KNOTS((2,2),(3,2,3),(0.710318915640079,1.),(0.573550810617452,
0.590910950629594,0.591084552029715),.UNSPECIFIED.)
GEOMETRIC_REPRESENTATION_ITEM()
RATIONAL_B_SPLINE_SURFACE(((0.998554414400195,0.992822941359326,0.990053454406147,
0.990053454406147,0.990053454406147),(0.998554414400195,0.992822941359326,
0.990053454406147,0.990053454406147,0.990053454406147)))
REPRESENTATION_ITEM('')
SURFACE()
);
#2857=(
BOUNDED_SURFACE()
B_SPLINE_SURFACE(1,2,((#143393,#143394,#143395,#143396,#143397,#143398,
#143399),(#143400,#143401,#143402,#143403,#143404,#143405,#143406)),
 .UNSPECIFIED.,.F.,.F.,.F.)
B_SPLINE_SURFACE_WITH_KNOTS((2,2),(3,2,2,3),(0.710192959008443,1.),(0.142404283483303,
0.142578551421364,0.142857142857143,0.160005345227479),.UNSPECIFIED.)
GEOMETRIC_REPRESENTATION_ITEM()
RATIONAL_B_SPLINE_SURFACE(((0.999805186472059,0.999805186472059,0.999805186472059,
0.999902211834795,1.,0.993980822699459,0.990851751371591),(0.999805186472059,
0.999805186472059,0.999805186472059,0.999902211834795,1.,0.993980822699459,
0.990851751371591)))
REPRESENTATION_ITEM('')
SURFACE()
);
#2858=(
BOUNDED_SURFACE()
B_SPLINE_SURFACE(1,2,((#143414,#143415,#143416,#143417,#143418),(#143419,
#143420,#143421,#143422,#143423)),.UNSPECIFIED.,.F.,.F.,.F.)
B_SPLINE_SURFACE_WITH_KNOTS((2,2),(3,2,3),(0.710318915639753,1.),(0.57355081061737,
0.590910950629594,0.591084552029716),.UNSPECIFIED.)
GEOMETRIC_REPRESENTATION_ITEM()
RATIONAL_B_SPLINE_SURFACE(((0.998554414400249,0.992822941359339,0.990053454406148,
0.990053454406148,0.990053454406148),(0.998554414400249,0.992822941359339,
0.990053454406148,0.990053454406148,0.990053454406148)))
REPRESENTATION_ITEM('')
SURFACE()
);
#2859=(
BOUNDED_SURFACE()
B_SPLINE_SURFACE(1,2,((#143434,#143435,#143436,#143437,#143438,#143439,
#143440),(#143441,#143442,#143443,#143444,#143445,#143446,#143447)),
 .UNSPECIFIED.,.F.,.F.,.F.)
B_SPLINE_SURFACE_WITH_KNOTS((2,2),(3,2,2,3),(0.710192959008108,1.),(0.142404283483303,
0.142578551421364,0.142857142857143,0.160005345227478),.UNSPECIFIED.)
GEOMETRIC_REPRESENTATION_ITEM()
RATIONAL_B_SPLINE_SURFACE(((0.999805186472059,0.999805186472059,0.999805186472059,
0.999902211834795,1.,0.993980822699459,0.990851751371591),(0.999805186472059,
0.999805186472059,0.999805186472059,0.999902211834795,1.,0.993980822699459,
0.990851751371591)))
REPRESENTATION_ITEM('')
SURFACE()
);
#2860=(
BOUNDED_SURFACE()
B_SPLINE_SURFACE(1,2,((#143455,#143456,#143457,#143458,#143459),(#143460,
#143461,#143462,#143463,#143464)),.UNSPECIFIED.,.F.,.F.,.F.)
B_SPLINE_SURFACE_WITH_KNOTS((2,2),(3,2,3),(0.710318915639617,1.),(0.573550810617172,
0.590910950629594,0.591084552029718),.UNSPECIFIED.)
GEOMETRIC_REPRESENTATION_ITEM()
RATIONAL_B_SPLINE_SURFACE(((0.99855441440038,0.992822941359371,0.990053454406148,
0.990053454406148,0.990053454406148),(0.99855441440038,0.992822941359371,
0.990053454406147,0.990053454406147,0.990053454406147)))
REPRESENTATION_ITEM('')
SURFACE()
);
#2861=(
BOUNDED_SURFACE()
B_SPLINE_SURFACE(1,2,((#143475,#143476,#143477,#143478,#143479,#143480,
#143481),(#143482,#143483,#143484,#143485,#143486,#143487,#143488)),
 .UNSPECIFIED.,.F.,.F.,.F.)
B_SPLINE_SURFACE_WITH_KNOTS((2,2),(3,2,2,3),(0.710192959007976,1.),(0.142404283483304,
0.142578551421364,0.142857142857143,0.160005345227403),.UNSPECIFIED.)
GEOMETRIC_REPRESENTATION_ITEM()
RATIONAL_B_SPLINE_SURFACE(((0.999805186472059,0.999805186472059,0.999805186472059,
0.999902211834795,1.,0.993980822699486,0.990851751371619),(0.999805186472059,
0.999805186472059,0.999805186472059,0.999902211834795,1.,0.993980822699486,
0.990851751371619)))
REPRESENTATION_ITEM('')
SURFACE()
);
#2862=(
BOUNDED_SURFACE()
B_SPLINE_SURFACE(1,2,((#143496,#143497,#143498),(#143499,#143500,#143501)),
 .UNSPECIFIED.,.F.,.F.,.F.)
B_SPLINE_SURFACE_WITH_KNOTS((2,2),(3,3),(0.710192959008443,1.),(0.53899963051341,
0.556316102183953),.UNSPECIFIED.)
GEOMETRIC_REPRESENTATION_ITEM()
RATIONAL_B_SPLINE_SURFACE(((0.987570037304351,0.988129172627919,0.99163541140107),
(0.987570037304351,0.988129172627919,0.99163541140107)))
REPRESENTATION_ITEM('')
SURFACE()
);
#2863=(
BOUNDED_SURFACE()
B_SPLINE_SURFACE(1,2,((#143510,#143511,#143512,#143513,#143514),(#143515,
#143516,#143517,#143518,#143519)),.UNSPECIFIED.,.F.,.F.,.F.)
B_SPLINE_SURFACE_WITH_KNOTS((2,2),(3,2,3),(0.709720368233181,1.),(0.176864064841898,
0.194132688793569,0.194731236525192),.UNSPECIFIED.)
GEOMETRIC_REPRESENTATION_ITEM()
RATIONAL_B_SPLINE_SURFACE(((0.987492606357657,0.987202831733786,0.989843896581211,
0.989843896581211,0.989843896581211),(0.987492606357657,0.987202831733786,
0.989843896581211,0.989843896581211,0.989843896581211)))
REPRESENTATION_ITEM('')
SURFACE()
);
#2864=(
BOUNDED_SURFACE()
B_SPLINE_SURFACE(1,2,((#143521,#143522,#143523),(#143524,#143525,#143526)),
 .UNSPECIFIED.,.F.,.F.,.F.)
B_SPLINE_SURFACE_WITH_KNOTS((2,2),(3,3),(0.710192959008437,1.),(0.53899963051341,
0.556316102183956),.UNSPECIFIED.)
GEOMETRIC_REPRESENTATION_ITEM()
RATIONAL_B_SPLINE_SURFACE(((0.987570037304351,0.988129172627919,0.991635411401071),
(0.987570037304351,0.988129172627919,0.991635411401071)))
REPRESENTATION_ITEM('')
SURFACE()
);
#2865=(
BOUNDED_SURFACE()
B_SPLINE_SURFACE(1,2,((#143535,#143536,#143537,#143538,#143539),(#143540,
#143541,#143542,#143543,#143544)),.UNSPECIFIED.,.F.,.F.,.F.)
B_SPLINE_SURFACE_WITH_KNOTS((2,2),(3,2,3),(0.70972036823745,1.),(0.176864064841898,
0.194132688793568,0.194731236520925),.UNSPECIFIED.)
GEOMETRIC_REPRESENTATION_ITEM()
RATIONAL_B_SPLINE_SURFACE(((0.987492606357657,0.987202831733786,0.989843896581211,
0.989843896581211,0.989843896581211),(0.987492606357657,0.987202831733786,
0.989843896581211,0.989843896581211,0.989843896581211)))
REPRESENTATION_ITEM('')
SURFACE()
);
#2866=(
BOUNDED_SURFACE()
B_SPLINE_SURFACE(1,2,((#143546,#143547,#143548),(#143549,#143550,#143551)),
 .UNSPECIFIED.,.F.,.F.,.F.)
B_SPLINE_SURFACE_WITH_KNOTS((2,2),(3,3),(0.710192959008441,1.),(0.538999630513411,
0.556316102183955),.UNSPECIFIED.)
GEOMETRIC_REPRESENTATION_ITEM()
RATIONAL_B_SPLINE_SURFACE(((0.987570037304351,0.988129172627919,0.99163541140107),
(0.987570037304351,0.988129172627919,0.99163541140107)))
REPRESENTATION_ITEM('')
SURFACE()
);
#2867=(
BOUNDED_SURFACE()
B_SPLINE_SURFACE(1,2,((#143560,#143561,#143562,#143563,#143564),(#143565,
#143566,#143567,#143568,#143569)),.UNSPECIFIED.,.F.,.F.,.F.)
B_SPLINE_SURFACE_WITH_KNOTS((2,2),(3,2,3),(0.709720368250085,1.),(0.176864064841897,
0.194132688793568,0.194731236508284),.UNSPECIFIED.)
GEOMETRIC_REPRESENTATION_ITEM()
RATIONAL_B_SPLINE_SURFACE(((0.987492606357657,0.987202831733786,0.989843896581211,
0.989843896581211,0.989843896581211),(0.987492606357657,0.987202831733786,
0.989843896581211,0.989843896581211,0.989843896581211)))
REPRESENTATION_ITEM('')
SURFACE()
);
#2868=(
BOUNDED_SURFACE()
B_SPLINE_SURFACE(1,2,((#143571,#143572,#143573),(#143574,#143575,#143576)),
 .UNSPECIFIED.,.F.,.F.,.F.)
B_SPLINE_SURFACE_WITH_KNOTS((2,2),(3,3),(0.71019295900844,1.),(0.538999630513411,
0.556316102183955),.UNSPECIFIED.)
GEOMETRIC_REPRESENTATION_ITEM()
RATIONAL_B_SPLINE_SURFACE(((0.987570037304351,0.988129172627919,0.99163541140107),
(0.987570037304351,0.988129172627919,0.99163541140107)))
REPRESENTATION_ITEM('')
SURFACE()
);
#2869=(
BOUNDED_SURFACE()
B_SPLINE_SURFACE(1,2,((#143585,#143586,#143587,#143588,#143589),(#143590,
#143591,#143592,#143593,#143594)),.UNSPECIFIED.,.F.,.F.,.F.)
B_SPLINE_SURFACE_WITH_KNOTS((2,2),(3,2,3),(0.709720368246354,1.),(0.176864064841897,
0.194132688793568,0.194731236512029),.UNSPECIFIED.)
GEOMETRIC_REPRESENTATION_ITEM()
RATIONAL_B_SPLINE_SURFACE(((0.987492606357657,0.987202831733786,0.989843896581211,
0.989843896581211,0.989843896581211),(0.987492606357657,0.987202831733786,
0.989843896581211,0.989843896581211,0.989843896581211)))
REPRESENTATION_ITEM('')
SURFACE()
);
#2870=(
BOUNDED_SURFACE()
B_SPLINE_SURFACE(1,2,((#143596,#143597,#143598),(#143599,#143600,#143601)),
 .UNSPECIFIED.,.F.,.F.,.F.)
B_SPLINE_SURFACE_WITH_KNOTS((2,2),(3,3),(0.710192959008441,1.),(0.538999630513411,
0.556316102183958),.UNSPECIFIED.)
GEOMETRIC_REPRESENTATION_ITEM()
RATIONAL_B_SPLINE_SURFACE(((0.987570037304351,0.988129172627919,0.991635411401071),
(0.987570037304351,0.988129172627919,0.991635411401071)))
REPRESENTATION_ITEM('')
SURFACE()
);
#2871=(
BOUNDED_SURFACE()
B_SPLINE_SURFACE(1,2,((#143610,#143611,#143612,#143613,#143614),(#143615,
#143616,#143617,#143618,#143619)),.UNSPECIFIED.,.F.,.F.,.F.)
B_SPLINE_SURFACE_WITH_KNOTS((2,2),(3,2,3),(0.709720368243867,1.),(0.176864064841897,
0.194132688793568,0.19473123651451),.UNSPECIFIED.)
GEOMETRIC_REPRESENTATION_ITEM()
RATIONAL_B_SPLINE_SURFACE(((0.987492606357657,0.987202831733786,0.989843896581211,
0.989843896581211,0.989843896581211),(0.987492606357657,0.987202831733786,
0.989843896581211,0.989843896581211,0.989843896581211)))
REPRESENTATION_ITEM('')
SURFACE()
);
#2872=(
BOUNDED_SURFACE()
B_SPLINE_SURFACE(1,2,((#143621,#143622,#143623),(#143624,#143625,#143626)),
 .UNSPECIFIED.,.F.,.F.,.F.)
B_SPLINE_SURFACE_WITH_KNOTS((2,2),(3,3),(0.710192959008442,1.),(0.538999630513411,
0.556316102183957),.UNSPECIFIED.)
GEOMETRIC_REPRESENTATION_ITEM()
RATIONAL_B_SPLINE_SURFACE(((0.987570037304351,0.988129172627919,0.991635411401071),
(0.987570037304351,0.988129172627919,0.991635411401071)))
REPRESENTATION_ITEM('')
SURFACE()
);
#2873=(
BOUNDED_SURFACE()
B_SPLINE_SURFACE(1,2,((#143635,#143636,#143637,#143638,#143639),(#143640,
#143641,#143642,#143643,#143644)),.UNSPECIFIED.,.F.,.F.,.F.)
B_SPLINE_SURFACE_WITH_KNOTS((2,2),(3,2,3),(0.709720368232269,1.),(0.176864064841897,
0.194132688793568,0.194731236526112),.UNSPECIFIED.)
GEOMETRIC_REPRESENTATION_ITEM()
RATIONAL_B_SPLINE_SURFACE(((0.987492606357657,0.987202831733786,0.98984389658121,
0.98984389658121,0.98984389658121),(0.987492606357657,0.987202831733786,
0.98984389658121,0.98984389658121,0.98984389658121)))
REPRESENTATION_ITEM('')
SURFACE()
);
#2874=(
BOUNDED_SURFACE()
B_SPLINE_SURFACE(1,2,((#143646,#143647,#143648),(#143649,#143650,#143651)),
 .UNSPECIFIED.,.F.,.F.,.F.)
B_SPLINE_SURFACE_WITH_KNOTS((2,2),(3,3),(0.710192959008441,1.),(0.538999630513411,
0.556316102183954),.UNSPECIFIED.)
GEOMETRIC_REPRESENTATION_ITEM()
RATIONAL_B_SPLINE_SURFACE(((0.987570037304351,0.988129172627919,0.99163541140107),
(0.987570037304351,0.988129172627919,0.99163541140107)))
REPRESENTATION_ITEM('')
SURFACE()
);
#2875=(
BOUNDED_SURFACE()
B_SPLINE_SURFACE(1,2,((#143660,#143661,#143662,#143663,#143664),(#143665,
#143666,#143667,#143668,#143669)),.UNSPECIFIED.,.F.,.F.,.F.)
B_SPLINE_SURFACE_WITH_KNOTS((2,2),(3,2,3),(0.709720368241591,1.),(0.176864064841897,
0.194132688793568,0.194731236516793),.UNSPECIFIED.)
GEOMETRIC_REPRESENTATION_ITEM()
RATIONAL_B_SPLINE_SURFACE(((0.987492606357657,0.987202831733786,0.989843896581211,
0.989843896581211,0.989843896581211),(0.987492606357657,0.987202831733786,
0.989843896581211,0.989843896581211,0.989843896581211)))
REPRESENTATION_ITEM('')
SURFACE()
);
#2876=(
BOUNDED_SURFACE()
B_SPLINE_SURFACE(1,2,((#143671,#143672,#143673),(#143674,#143675,#143676)),
 .UNSPECIFIED.,.F.,.F.,.F.)
B_SPLINE_SURFACE_WITH_KNOTS((2,2),(3,3),(0.710192959008444,1.),(0.538999630513411,
0.556316102183958),.UNSPECIFIED.)
GEOMETRIC_REPRESENTATION_ITEM()
RATIONAL_B_SPLINE_SURFACE(((0.987570037304351,0.988129172627919,0.991635411401071),
(0.987570037304351,0.988129172627919,0.991635411401071)))
REPRESENTATION_ITEM('')
SURFACE()
);
#2877=(
BOUNDED_SURFACE()
B_SPLINE_SURFACE(1,2,((#143685,#143686,#143687,#143688,#143689),(#143690,
#143691,#143692,#143693,#143694)),.UNSPECIFIED.,.F.,.F.,.F.)
B_SPLINE_SURFACE_WITH_KNOTS((2,2),(3,2,3),(0.709720368224627,1.),(0.176864064841897,
0.194132688793568,0.194731236533751),.UNSPECIFIED.)
GEOMETRIC_REPRESENTATION_ITEM()
RATIONAL_B_SPLINE_SURFACE(((0.987492606357657,0.987202831733786,0.989843896581211,
0.989843896581211,0.989843896581211),(0.987492606357657,0.987202831733786,
0.98984389658121,0.98984389658121,0.98984389658121)))
REPRESENTATION_ITEM('')
SURFACE()
);
#2878=(
BOUNDED_SURFACE()
B_SPLINE_SURFACE(1,2,((#143696,#143697,#143698),(#143699,#143700,#143701)),
 .UNSPECIFIED.,.F.,.F.,.F.)
B_SPLINE_SURFACE_WITH_KNOTS((2,2),(3,3),(0.710192959008446,1.),(0.538999630513411,
0.556316102183958),.UNSPECIFIED.)
GEOMETRIC_REPRESENTATION_ITEM()
RATIONAL_B_SPLINE_SURFACE(((0.987570037304351,0.988129172627919,0.991635411401071),
(0.987570037304351,0.988129172627919,0.991635411401071)))
REPRESENTATION_ITEM('')
SURFACE()
);
#2879=(
BOUNDED_SURFACE()
B_SPLINE_SURFACE(1,2,((#143710,#143711,#143712,#143713,#143714),(#143715,
#143716,#143717,#143718,#143719)),.UNSPECIFIED.,.F.,.F.,.F.)
B_SPLINE_SURFACE_WITH_KNOTS((2,2),(3,2,3),(0.709720368239206,1.),(0.176864064841897,
0.194132688793568,0.194731236519174),.UNSPECIFIED.)
GEOMETRIC_REPRESENTATION_ITEM()
RATIONAL_B_SPLINE_SURFACE(((0.987492606357657,0.987202831733786,0.989843896581211,
0.989843896581211,0.989843896581211),(0.987492606357657,0.987202831733786,
0.989843896581211,0.989843896581211,0.989843896581211)))
REPRESENTATION_ITEM('')
SURFACE()
);
#2880=(
BOUNDED_SURFACE()
B_SPLINE_SURFACE(1,2,((#143721,#143722,#143723),(#143724,#143725,#143726)),
 .UNSPECIFIED.,.F.,.F.,.F.)
B_SPLINE_SURFACE_WITH_KNOTS((2,2),(3,3),(0.710192959008439,1.),(0.538999630513411,
0.556316102183958),.UNSPECIFIED.)
GEOMETRIC_REPRESENTATION_ITEM()
RATIONAL_B_SPLINE_SURFACE(((0.987570037304351,0.988129172627919,0.991635411401071),
(0.987570037304351,0.988129172627919,0.991635411401071)))
REPRESENTATION_ITEM('')
SURFACE()
);
#2881=(
BOUNDED_SURFACE()
B_SPLINE_SURFACE(1,2,((#143735,#143736,#143737,#143738,#143739),(#143740,
#143741,#143742,#143743,#143744)),.UNSPECIFIED.,.F.,.F.,.F.)
B_SPLINE_SURFACE_WITH_KNOTS((2,2),(3,2,3),(0.709720368220064,1.),(0.176864064841897,
0.194132688793568,0.194731236538315),.UNSPECIFIED.)
GEOMETRIC_REPRESENTATION_ITEM()
RATIONAL_B_SPLINE_SURFACE(((0.987492606357657,0.987202831733786,0.98984389658121,
0.98984389658121,0.98984389658121),(0.987492606357657,0.987202831733786,
0.989843896581211,0.989843896581211,0.989843896581211)))
REPRESENTATION_ITEM('')
SURFACE()
);
#2882=(
BOUNDED_SURFACE()
B_SPLINE_SURFACE(1,2,((#143746,#143747,#143748),(#143749,#143750,#143751)),
 .UNSPECIFIED.,.F.,.F.,.F.)
B_SPLINE_SURFACE_WITH_KNOTS((2,2),(3,3),(0.710192959008444,1.),(0.538999630513411,
0.556316102183958),.UNSPECIFIED.)
GEOMETRIC_REPRESENTATION_ITEM()
RATIONAL_B_SPLINE_SURFACE(((0.987570037304351,0.988129172627919,0.991635411401071),
(0.987570037304351,0.988129172627919,0.991635411401071)))
REPRESENTATION_ITEM('')
SURFACE()
);
#2883=(
BOUNDED_SURFACE()
B_SPLINE_SURFACE(1,2,((#143760,#143761,#143762,#143763,#143764),(#143765,
#143766,#143767,#143768,#143769)),.UNSPECIFIED.,.F.,.F.,.F.)
B_SPLINE_SURFACE_WITH_KNOTS((2,2),(3,2,3),(0.709720368252039,1.),(0.176864064841897,
0.194132688793568,0.194731236506339),.UNSPECIFIED.)
GEOMETRIC_REPRESENTATION_ITEM()
RATIONAL_B_SPLINE_SURFACE(((0.987492606357657,0.987202831733786,0.989843896581211,
0.989843896581211,0.989843896581211),(0.987492606357657,0.987202831733786,
0.989843896581211,0.989843896581211,0.989843896581211)))
REPRESENTATION_ITEM('')
SURFACE()
);
#2884=(
BOUNDED_SURFACE()
B_SPLINE_SURFACE(1,2,((#143771,#143772,#143773),(#143774,#143775,#143776)),
 .UNSPECIFIED.,.F.,.F.,.F.)
B_SPLINE_SURFACE_WITH_KNOTS((2,2),(3,3),(0.710192959008441,1.),(0.538999630513411,
0.556316102183958),.UNSPECIFIED.)
GEOMETRIC_REPRESENTATION_ITEM()
RATIONAL_B_SPLINE_SURFACE(((0.987570037304351,0.988129172627919,0.991635411401071),
(0.987570037304351,0.988129172627919,0.991635411401071)))
REPRESENTATION_ITEM('')
SURFACE()
);
#2885=(
BOUNDED_SURFACE()
B_SPLINE_SURFACE(1,2,((#143785,#143786,#143787,#143788,#143789),(#143790,
#143791,#143792,#143793,#143794)),.UNSPECIFIED.,.F.,.F.,.F.)
B_SPLINE_SURFACE_WITH_KNOTS((2,2),(3,2,3),(0.709720368247964,1.),(0.176864064841897,
0.194132688793568,0.194731236510412),.UNSPECIFIED.)
GEOMETRIC_REPRESENTATION_ITEM()
RATIONAL_B_SPLINE_SURFACE(((0.987492606357657,0.987202831733786,0.989843896581211,
0.989843896581211,0.989843896581211),(0.987492606357657,0.987202831733786,
0.989843896581211,0.989843896581211,0.989843896581211)))
REPRESENTATION_ITEM('')
SURFACE()
);
#2886=(
BOUNDED_SURFACE()
B_SPLINE_SURFACE(1,2,((#143796,#143797,#143798),(#143799,#143800,#143801)),
 .UNSPECIFIED.,.F.,.F.,.F.)
B_SPLINE_SURFACE_WITH_KNOTS((2,2),(3,3),(0.71019295900844,1.),(0.538999630513411,
0.556316102183955),.UNSPECIFIED.)
GEOMETRIC_REPRESENTATION_ITEM()
RATIONAL_B_SPLINE_SURFACE(((0.987570037304351,0.988129172627919,0.99163541140107),
(0.987570037304351,0.988129172627919,0.99163541140107)))
REPRESENTATION_ITEM('')
SURFACE()
);
#2887=(
BOUNDED_SURFACE()
B_SPLINE_SURFACE(1,2,((#143810,#143811,#143812,#143813,#143814),(#143815,
#143816,#143817,#143818,#143819)),.UNSPECIFIED.,.F.,.F.,.F.)
B_SPLINE_SURFACE_WITH_KNOTS((2,2),(3,2,3),(0.7097203682361,1.),(0.176864064841897,
0.194132688793568,0.194731236522273),.UNSPECIFIED.)
GEOMETRIC_REPRESENTATION_ITEM()
RATIONAL_B_SPLINE_SURFACE(((0.987492606357657,0.987202831733786,0.989843896581211,
0.989843896581211,0.989843896581211),(0.987492606357657,0.987202831733786,
0.98984389658121,0.98984389658121,0.98984389658121)))
REPRESENTATION_ITEM('')
SURFACE()
);
#2888=(
BOUNDED_SURFACE()
B_SPLINE_SURFACE(1,2,((#143821,#143822,#143823),(#143824,#143825,#143826)),
 .UNSPECIFIED.,.F.,.F.,.F.)
B_SPLINE_SURFACE_WITH_KNOTS((2,2),(3,3),(0.710192959008442,1.),(0.538999630513411,
0.556316102183955),.UNSPECIFIED.)
GEOMETRIC_REPRESENTATION_ITEM()
RATIONAL_B_SPLINE_SURFACE(((0.987570037304351,0.988129172627919,0.99163541140107),
(0.987570037304351,0.988129172627919,0.99163541140107)))
REPRESENTATION_ITEM('')
SURFACE()
);
#2889=(
BOUNDED_SURFACE()
B_SPLINE_SURFACE(1,2,((#143835,#143836,#143837,#143838,#143839),(#143840,
#143841,#143842,#143843,#143844)),.UNSPECIFIED.,.F.,.F.,.F.)
B_SPLINE_SURFACE_WITH_KNOTS((2,2),(3,2,3),(0.709720368226764,1.),(0.176864064841897,
0.194132688793568,0.194731236531613),.UNSPECIFIED.)
GEOMETRIC_REPRESENTATION_ITEM()
RATIONAL_B_SPLINE_SURFACE(((0.987492606357657,0.987202831733786,0.989843896581211,
0.989843896581211,0.989843896581211),(0.987492606357657,0.987202831733786,
0.989843896581211,0.989843896581211,0.989843896581211)))
REPRESENTATION_ITEM('')
SURFACE()
);
#2890=(
BOUNDED_SURFACE()
B_SPLINE_SURFACE(1,2,((#143846,#143847,#143848),(#143849,#143850,#143851)),
 .UNSPECIFIED.,.F.,.F.,.F.)
B_SPLINE_SURFACE_WITH_KNOTS((2,2),(3,3),(0.710192959008444,1.),(0.538999630513411,
0.556316102183958),.UNSPECIFIED.)
GEOMETRIC_REPRESENTATION_ITEM()
RATIONAL_B_SPLINE_SURFACE(((0.987570037304351,0.988129172627919,0.991635411401071),
(0.987570037304351,0.988129172627919,0.991635411401071)))
REPRESENTATION_ITEM('')
SURFACE()
);
#2891=(
BOUNDED_SURFACE()
B_SPLINE_SURFACE(1,2,((#143860,#143861,#143862,#143863,#143864),(#143865,
#143866,#143867,#143868,#143869)),.UNSPECIFIED.,.F.,.F.,.F.)
B_SPLINE_SURFACE_WITH_KNOTS((2,2),(3,2,3),(0.709720368237924,1.),(0.176864064841897,
0.194132688793568,0.194731236520456),.UNSPECIFIED.)
GEOMETRIC_REPRESENTATION_ITEM()
RATIONAL_B_SPLINE_SURFACE(((0.987492606357657,0.987202831733786,0.989843896581211,
0.989843896581211,0.989843896581211),(0.987492606357657,0.987202831733786,
0.989843896581211,0.989843896581211,0.989843896581211)))
REPRESENTATION_ITEM('')
SURFACE()
);
#2892=(
BOUNDED_SURFACE()
B_SPLINE_SURFACE(1,2,((#143871,#143872,#143873),(#143874,#143875,#143876)),
 .UNSPECIFIED.,.F.,.F.,.F.)
B_SPLINE_SURFACE_WITH_KNOTS((2,2),(3,3),(0.710192959008442,1.),(0.538999630513411,
0.556316102183955),.UNSPECIFIED.)
GEOMETRIC_REPRESENTATION_ITEM()
RATIONAL_B_SPLINE_SURFACE(((0.987570037304351,0.988129172627919,0.99163541140107),
(0.987570037304351,0.988129172627919,0.99163541140107)))
REPRESENTATION_ITEM('')
SURFACE()
);
#2893=(
BOUNDED_SURFACE()
B_SPLINE_SURFACE(1,2,((#143885,#143886,#143887,#143888,#143889),(#143890,
#143891,#143892,#143893,#143894)),.UNSPECIFIED.,.F.,.F.,.F.)
B_SPLINE_SURFACE_WITH_KNOTS((2,2),(3,2,3),(0.709720368221021,1.),(0.176864064841897,
0.194132688793568,0.194731236537358),.UNSPECIFIED.)
GEOMETRIC_REPRESENTATION_ITEM()
RATIONAL_B_SPLINE_SURFACE(((0.987492606357657,0.987202831733786,0.98984389658121,
0.98984389658121,0.98984389658121),(0.987492606357657,0.987202831733786,
0.98984389658121,0.98984389658121,0.98984389658121)))
REPRESENTATION_ITEM('')
SURFACE()
);
#2894=(
BOUNDED_SURFACE()
B_SPLINE_SURFACE(1,2,((#143896,#143897,#143898),(#143899,#143900,#143901)),
 .UNSPECIFIED.,.F.,.F.,.F.)
B_SPLINE_SURFACE_WITH_KNOTS((2,2),(3,3),(0.71019295900844,1.),(0.538999630513411,
0.556316102183957),.UNSPECIFIED.)
GEOMETRIC_REPRESENTATION_ITEM()
RATIONAL_B_SPLINE_SURFACE(((0.987570037304351,0.988129172627919,0.991635411401071),
(0.987570037304351,0.988129172627919,0.991635411401071)))
REPRESENTATION_ITEM('')
SURFACE()
);
#2895=(
BOUNDED_SURFACE()
B_SPLINE_SURFACE(1,2,((#143910,#143911,#143912,#143913,#143914),(#143915,
#143916,#143917,#143918,#143919)),.UNSPECIFIED.,.F.,.F.,.F.)
B_SPLINE_SURFACE_WITH_KNOTS((2,2),(3,2,3),(0.709720368226753,1.),(0.176864064841897,
0.194132688793568,0.194731236531624),.UNSPECIFIED.)
GEOMETRIC_REPRESENTATION_ITEM()
RATIONAL_B_SPLINE_SURFACE(((0.987492606357657,0.987202831733786,0.989843896581211,
0.989843896581211,0.989843896581211),(0.987492606357657,0.987202831733786,
0.98984389658121,0.98984389658121,0.98984389658121)))
REPRESENTATION_ITEM('')
SURFACE()
);
#2896=(
BOUNDED_SURFACE()
B_SPLINE_SURFACE(1,2,((#143921,#143922,#143923),(#143924,#143925,#143926)),
 .UNSPECIFIED.,.F.,.F.,.F.)
B_SPLINE_SURFACE_WITH_KNOTS((2,2),(3,3),(0.710192959008443,1.),(0.538999630513411,
0.556316102183958),.UNSPECIFIED.)
GEOMETRIC_REPRESENTATION_ITEM()
RATIONAL_B_SPLINE_SURFACE(((0.987570037304351,0.988129172627919,0.991635411401071),
(0.987570037304351,0.988129172627919,0.991635411401071)))
REPRESENTATION_ITEM('')
SURFACE()
);
#2897=(
BOUNDED_SURFACE()
B_SPLINE_SURFACE(1,2,((#143935,#143936,#143937,#143938,#143939),(#143940,
#143941,#143942,#143943,#143944)),.UNSPECIFIED.,.F.,.F.,.F.)
B_SPLINE_SURFACE_WITH_KNOTS((2,2),(3,2,3),(0.709720368249467,1.),(0.176864064841897,
0.194132688793568,0.19473123650891),.UNSPECIFIED.)
GEOMETRIC_REPRESENTATION_ITEM()
RATIONAL_B_SPLINE_SURFACE(((0.987492606357657,0.987202831733786,0.989843896581211,
0.989843896581211,0.989843896581211),(0.987492606357657,0.987202831733786,
0.989843896581211,0.989843896581211,0.989843896581211)))
REPRESENTATION_ITEM('')
SURFACE()
);
#2898=(
BOUNDED_SURFACE()
B_SPLINE_SURFACE(1,2,((#143946,#143947,#143948),(#143949,#143950,#143951)),
 .UNSPECIFIED.,.F.,.F.,.F.)
B_SPLINE_SURFACE_WITH_KNOTS((2,2),(3,3),(0.710192959008441,1.),(0.538999630513411,
0.556316102183958),.UNSPECIFIED.)
GEOMETRIC_REPRESENTATION_ITEM()
RATIONAL_B_SPLINE_SURFACE(((0.987570037304351,0.988129172627919,0.991635411401071),
(0.987570037304351,0.988129172627919,0.991635411401071)))
REPRESENTATION_ITEM('')
SURFACE()
);
#2899=(
BOUNDED_SURFACE()
B_SPLINE_SURFACE(1,2,((#143960,#143961,#143962,#143963,#143964),(#143965,
#143966,#143967,#143968,#143969)),.UNSPECIFIED.,.F.,.F.,.F.)
B_SPLINE_SURFACE_WITH_KNOTS((2,2),(3,2,3),(0.709720368252126,1.),(0.176864064841897,
0.194132688793568,0.194731236506258),.UNSPECIFIED.)
GEOMETRIC_REPRESENTATION_ITEM()
RATIONAL_B_SPLINE_SURFACE(((0.987492606357657,0.987202831733786,0.989843896581211,
0.989843896581211,0.989843896581211),(0.987492606357657,0.987202831733786,
0.989843896581211,0.989843896581211,0.989843896581211)))
REPRESENTATION_ITEM('')
SURFACE()
);
#2900=(
BOUNDED_SURFACE()
B_SPLINE_SURFACE(1,2,((#143971,#143972,#143973),(#143974,#143975,#143976)),
 .UNSPECIFIED.,.F.,.F.,.F.)
B_SPLINE_SURFACE_WITH_KNOTS((2,2),(3,3),(0.71019295900844,1.),(0.538999630513411,
0.556316102183955),.UNSPECIFIED.)
GEOMETRIC_REPRESENTATION_ITEM()
RATIONAL_B_SPLINE_SURFACE(((0.987570037304351,0.988129172627919,0.99163541140107),
(0.987570037304351,0.988129172627919,0.99163541140107)))
REPRESENTATION_ITEM('')
SURFACE()
);
#2901=(
BOUNDED_SURFACE()
B_SPLINE_SURFACE(1,2,((#143985,#143986,#143987,#143988,#143989),(#143990,
#143991,#143992,#143993,#143994)),.UNSPECIFIED.,.F.,.F.,.F.)
B_SPLINE_SURFACE_WITH_KNOTS((2,2),(3,2,3),(0.709720368257119,1.),(0.176864064841897,
0.194132688793568,0.194731236312158),.UNSPECIFIED.)
GEOMETRIC_REPRESENTATION_ITEM()
RATIONAL_B_SPLINE_SURFACE(((0.987492606357657,0.987202831733786,0.98984389658121,
0.98984389658121,0.98984389658121),(0.987492606357657,0.987202831733786,
0.98984389658121,0.98984389658121,0.98984389658121)))
REPRESENTATION_ITEM('')
SURFACE()
);
#2902=(
BOUNDED_SURFACE()
B_SPLINE_SURFACE(1,2,((#143996,#143997,#143998),(#143999,#144000,#144001)),
 .UNSPECIFIED.,.F.,.F.,.F.)
B_SPLINE_SURFACE_WITH_KNOTS((2,2),(3,3),(0.710192959008293,1.),(0.538999630513123,
0.556316102183955),.UNSPECIFIED.)
GEOMETRIC_REPRESENTATION_ITEM()
RATIONAL_B_SPLINE_SURFACE(((0.987570037304332,0.988129172627861,0.99163541140107),
(0.987570037304332,0.988129172627861,0.99163541140107)))
REPRESENTATION_ITEM('')
SURFACE()
);
#2903=(
BOUNDED_SURFACE()
B_SPLINE_SURFACE(1,2,((#144010,#144011,#144012,#144013,#144014),(#144015,
#144016,#144017,#144018,#144019)),.UNSPECIFIED.,.F.,.F.,.F.)
B_SPLINE_SURFACE_WITH_KNOTS((2,2),(3,2,3),(0.709720368254059,1.),(0.176864064841898,
0.194132688793569,0.194731236504179),.UNSPECIFIED.)
GEOMETRIC_REPRESENTATION_ITEM()
RATIONAL_B_SPLINE_SURFACE(((0.987492606357657,0.987202831733786,0.989843896581211,
0.989843896581211,0.989843896581211),(0.987492606357657,0.987202831733786,
0.989843896581211,0.989843896581211,0.989843896581211)))
REPRESENTATION_ITEM('')
SURFACE()
);
#2904=(
BOUNDED_SURFACE()
B_SPLINE_SURFACE(1,2,((#144021,#144022,#144023),(#144024,#144025,#144026)),
 .UNSPECIFIED.,.F.,.F.,.F.)
B_SPLINE_SURFACE_WITH_KNOTS((2,2),(3,3),(0.71019295900805,1.),(0.53899963051341,
0.556316102183953),.UNSPECIFIED.)
GEOMETRIC_REPRESENTATION_ITEM()
RATIONAL_B_SPLINE_SURFACE(((0.987570037304351,0.988129172627919,0.99163541140107),
(0.987570037304351,0.988129172627919,0.99163541140107)))
REPRESENTATION_ITEM('')
SURFACE()
);
#2905=(
BOUNDED_SURFACE()
B_SPLINE_SURFACE(1,2,((#144035,#144036,#144037,#144038,#144039),(#144040,
#144041,#144042,#144043,#144044)),.UNSPECIFIED.,.F.,.F.,.F.)
B_SPLINE_SURFACE_WITH_KNOTS((2,2),(3,2,3),(0.709720368249968,1.),(0.176864064841898,
0.194132688793569,0.194731236508023),.UNSPECIFIED.)
GEOMETRIC_REPRESENTATION_ITEM()
RATIONAL_B_SPLINE_SURFACE(((0.987492606357657,0.987202831733786,0.989843896581211,
0.989843896581211,0.989843896581211),(0.987492606357657,0.987202831733786,
0.989843896581211,0.989843896581211,0.989843896581211)))
REPRESENTATION_ITEM('')
SURFACE()
);
#2906=(
BOUNDED_SURFACE()
B_SPLINE_SURFACE(1,2,((#144046,#144047,#144048),(#144049,#144050,#144051)),
 .UNSPECIFIED.,.F.,.F.,.F.)
B_SPLINE_SURFACE_WITH_KNOTS((2,2),(3,3),(0.710192959006647,1.),(0.53899963051341,
0.556316102183956),.UNSPECIFIED.)
GEOMETRIC_REPRESENTATION_ITEM()
RATIONAL_B_SPLINE_SURFACE(((0.987570037304351,0.988129172627919,0.991635411401071),
(0.987570037304351,0.988129172627919,0.991635411401071)))
REPRESENTATION_ITEM('')
SURFACE()
);
#2907=(
BOUNDED_SURFACE()
B_SPLINE_SURFACE(1,2,((#144060,#144061,#144062,#144063,#144064),(#144065,
#144066,#144067,#144068,#144069)),.UNSPECIFIED.,.F.,.F.,.F.)
B_SPLINE_SURFACE_WITH_KNOTS((2,2),(3,2,3),(0.709720368240864,1.),(0.176864064841898,
0.194132688793569,0.194731236515723),.UNSPECIFIED.)
GEOMETRIC_REPRESENTATION_ITEM()
RATIONAL_B_SPLINE_SURFACE(((0.987492606357657,0.987202831733786,0.989843896581211,
0.989843896581211,0.989843896581211),(0.987492606357657,0.987202831733786,
0.989843896581211,0.989843896581211,0.989843896581211)))
REPRESENTATION_ITEM('')
SURFACE()
);
#2908=(
BOUNDED_SURFACE()
B_SPLINE_SURFACE(1,2,((#144071,#144072,#144073),(#144074,#144075,#144076)),
 .UNSPECIFIED.,.F.,.F.,.F.)
B_SPLINE_SURFACE_WITH_KNOTS((2,2),(3,3),(0.710192959007974,1.),(0.53899963051341,
0.556316102183953),.UNSPECIFIED.)
GEOMETRIC_REPRESENTATION_ITEM()
RATIONAL_B_SPLINE_SURFACE(((0.987570037304351,0.988129172627919,0.99163541140107),
(0.987570037304351,0.988129172627919,0.99163541140107)))
REPRESENTATION_ITEM('')
SURFACE()
);
#2909=(
BOUNDED_SURFACE()
B_SPLINE_SURFACE(1,2,((#144085,#144086,#144087,#144088,#144089),(#144090,
#144091,#144092,#144093,#144094)),.UNSPECIFIED.,.F.,.F.,.F.)
B_SPLINE_SURFACE_WITH_KNOTS((2,2),(3,2,3),(0.709720368223987,1.),(0.176864064841898,
0.194132688793569,0.194731236533929),.UNSPECIFIED.)
GEOMETRIC_REPRESENTATION_ITEM()
RATIONAL_B_SPLINE_SURFACE(((0.987492606357657,0.987202831733786,0.989843896581211,
0.989843896581211,0.989843896581211),(0.987492606357657,0.987202831733786,
0.989843896581211,0.989843896581211,0.989843896581211)))
REPRESENTATION_ITEM('')
SURFACE()
);
#2910=(
BOUNDED_SURFACE()
B_SPLINE_SURFACE(1,2,((#144096,#144097,#144098),(#144099,#144100,#144101)),
 .UNSPECIFIED.,.F.,.F.,.F.)
B_SPLINE_SURFACE_WITH_KNOTS((2,2),(3,3),(0.710192959008353,1.),(0.53899963051341,
0.556316102183954),.UNSPECIFIED.)
GEOMETRIC_REPRESENTATION_ITEM()
RATIONAL_B_SPLINE_SURFACE(((0.987570037304351,0.988129172627919,0.99163541140107),
(0.987570037304351,0.988129172627919,0.99163541140107)))
REPRESENTATION_ITEM('')
SURFACE()
);
#2911=(
BOUNDED_SURFACE()
B_SPLINE_SURFACE(1,2,((#144110,#144111,#144112,#144113,#144114),(#144115,
#144116,#144117,#144118,#144119)),.UNSPECIFIED.,.F.,.F.,.F.)
B_SPLINE_SURFACE_WITH_KNOTS((2,2),(3,2,3),(0.70972036823388,1.),(0.176864064841898,
0.194132688793569,0.194731236524411),.UNSPECIFIED.)
GEOMETRIC_REPRESENTATION_ITEM()
RATIONAL_B_SPLINE_SURFACE(((0.987492606357657,0.987202831733786,0.989843896581211,
0.989843896581211,0.989843896581211),(0.987492606357657,0.987202831733786,
0.989843896581211,0.989843896581211,0.989843896581211)))
REPRESENTATION_ITEM('')
SURFACE()
);
#2912=(
BOUNDED_SURFACE()
B_SPLINE_SURFACE(1,2,((#144121,#144122,#144123),(#144124,#144125,#144126)),
 .UNSPECIFIED.,.F.,.F.,.F.)
B_SPLINE_SURFACE_WITH_KNOTS((2,2),(3,3),(0.710192959008359,1.),(0.53899963051341,
0.556316102183956),.UNSPECIFIED.)
GEOMETRIC_REPRESENTATION_ITEM()
RATIONAL_B_SPLINE_SURFACE(((0.987570037304351,0.988129172627919,0.991635411401071),
(0.987570037304351,0.988129172627919,0.991635411401071)))
REPRESENTATION_ITEM('')
SURFACE()
);
#2913=(
BOUNDED_SURFACE()
B_SPLINE_SURFACE(1,2,((#144135,#144136,#144137,#144138,#144139),(#144140,
#144141,#144142,#144143,#144144)),.UNSPECIFIED.,.F.,.F.,.F.)
B_SPLINE_SURFACE_WITH_KNOTS((2,2),(3,2,3),(0.709720368257934,1.),(0.176864064841898,
0.194132688793569,0.194731236500374),.UNSPECIFIED.)
GEOMETRIC_REPRESENTATION_ITEM()
RATIONAL_B_SPLINE_SURFACE(((0.987492606357657,0.987202831733786,0.989843896581211,
0.989843896581211,0.989843896581211),(0.987492606357657,0.987202831733786,
0.989843896581211,0.989843896581211,0.989843896581211)))
REPRESENTATION_ITEM('')
SURFACE()
);
#2914=(
BOUNDED_SURFACE()
B_SPLINE_SURFACE(1,2,((#144146,#144147,#144148),(#144149,#144150,#144151)),
 .UNSPECIFIED.,.F.,.F.,.F.)
B_SPLINE_SURFACE_WITH_KNOTS((2,2),(3,3),(0.710192959008367,1.),(0.53899963051341,
0.556316102183953),.UNSPECIFIED.)
GEOMETRIC_REPRESENTATION_ITEM()
RATIONAL_B_SPLINE_SURFACE(((0.987570037304351,0.988129172627919,0.99163541140107),
(0.987570037304351,0.988129172627919,0.99163541140107)))
REPRESENTATION_ITEM('')
SURFACE()
);
#2915=(
BOUNDED_SURFACE()
B_SPLINE_SURFACE(1,2,((#144160,#144161,#144162,#144163,#144164),(#144165,
#144166,#144167,#144168,#144169)),.UNSPECIFIED.,.F.,.F.,.F.)
B_SPLINE_SURFACE_WITH_KNOTS((2,2),(3,2,3),(0.70972036823852,1.),(0.176864064841898,
0.194132688793569,0.194731236519792),.UNSPECIFIED.)
GEOMETRIC_REPRESENTATION_ITEM()
RATIONAL_B_SPLINE_SURFACE(((0.987492606357657,0.987202831733786,0.989843896581211,
0.989843896581211,0.989843896581211),(0.987492606357657,0.987202831733786,
0.989843896581211,0.989843896581211,0.989843896581211)))
REPRESENTATION_ITEM('')
SURFACE()
);
#2916=(
BOUNDED_SURFACE()
B_SPLINE_SURFACE(1,2,((#144171,#144172,#144173),(#144174,#144175,#144176)),
 .UNSPECIFIED.,.F.,.F.,.F.)
B_SPLINE_SURFACE_WITH_KNOTS((2,2),(3,3),(0.710192959008085,1.),(0.53899963051341,
0.556316102183954),.UNSPECIFIED.)
GEOMETRIC_REPRESENTATION_ITEM()
RATIONAL_B_SPLINE_SURFACE(((0.987570037304351,0.988129172627919,0.99163541140107),
(0.987570037304351,0.988129172627919,0.99163541140107)))
REPRESENTATION_ITEM('')
SURFACE()
);
#2917=(
BOUNDED_SURFACE()
B_SPLINE_SURFACE(1,2,((#144185,#144186,#144187,#144188,#144189),(#144190,
#144191,#144192,#144193,#144194)),.UNSPECIFIED.,.F.,.F.,.F.)
B_SPLINE_SURFACE_WITH_KNOTS((2,2),(3,2,3),(0.709720368237269,1.),(0.176864064841898,
0.194132688793569,0.194731236520761),.UNSPECIFIED.)
GEOMETRIC_REPRESENTATION_ITEM()
RATIONAL_B_SPLINE_SURFACE(((0.987492606357657,0.987202831733786,0.989843896581211,
0.989843896581211,0.989843896581211),(0.987492606357657,0.987202831733786,
0.989843896581211,0.989843896581211,0.989843896581211)))
REPRESENTATION_ITEM('')
SURFACE()
);
#2918=(
BOUNDED_SURFACE()
B_SPLINE_SURFACE(1,2,((#144196,#144197,#144198),(#144199,#144200,#144201)),
 .UNSPECIFIED.,.F.,.F.,.F.)
B_SPLINE_SURFACE_WITH_KNOTS((2,2),(3,3),(0.710192959008438,1.),(0.53899963051341,
0.556316102183956),.UNSPECIFIED.)
GEOMETRIC_REPRESENTATION_ITEM()
RATIONAL_B_SPLINE_SURFACE(((0.987570037304351,0.988129172627919,0.991635411401071),
(0.987570037304351,0.988129172627919,0.991635411401071)))
REPRESENTATION_ITEM('')
SURFACE()
);
#2919=(
BOUNDED_SURFACE()
B_SPLINE_SURFACE(1,2,((#144210,#144211,#144212,#144213,#144214),(#144215,
#144216,#144217,#144218,#144219)),.UNSPECIFIED.,.F.,.F.,.F.)
B_SPLINE_SURFACE_WITH_KNOTS((2,2),(3,2,3),(0.70972036823978,1.),(0.176864064841898,
0.194132688793569,0.194731236518602),.UNSPECIFIED.)
GEOMETRIC_REPRESENTATION_ITEM()
RATIONAL_B_SPLINE_SURFACE(((0.987492606357657,0.987202831733786,0.989843896581211,
0.989843896581211,0.989843896581211),(0.987492606357657,0.987202831733786,
0.989843896581211,0.989843896581211,0.989843896581211)))
REPRESENTATION_ITEM('')
SURFACE()
);
#2920=(
BOUNDED_SURFACE()
B_SPLINE_SURFACE(1,2,((#144221,#144222,#144223),(#144224,#144225,#144226)),
 .UNSPECIFIED.,.F.,.F.,.F.)
B_SPLINE_SURFACE_WITH_KNOTS((2,2),(3,3),(0.,0.28968108435992),(0.125066077454537,
0.142578551421365),.UNSPECIFIED.)
GEOMETRIC_REPRESENTATION_ITEM()
RATIONAL_B_SPLINE_SURFACE(((0.990621203777022,0.993706096834649,0.999805186472059),
(0.990621203777022,0.993706096834649,0.999805186472059)))
REPRESENTATION_ITEM('')
SURFACE()
);
#2921=(
BOUNDED_SURFACE()
B_SPLINE_SURFACE(1,2,((#144235,#144236,#144237),(#144238,#144239,#144240)),
 .UNSPECIFIED.,.F.,.F.,.F.)
B_SPLINE_SURFACE_WITH_KNOTS((2,2),(3,3),(0.,0.289807040992006),(0.590910950629593,
0.60808458519997),.UNSPECIFIED.)
GEOMETRIC_REPRESENTATION_ITEM()
RATIONAL_B_SPLINE_SURFACE(((0.990053454406147,0.987313720921968,0.987472672298934),
(0.990053454406147,0.987313720921968,0.987472672298934)))
REPRESENTATION_ITEM('')
SURFACE()
);
#2922=(
BOUNDED_SURFACE()
B_SPLINE_SURFACE(1,2,((#144242,#144243,#144244),(#144245,#144246,#144247)),
 .UNSPECIFIED.,.F.,.F.,.F.)
B_SPLINE_SURFACE_WITH_KNOTS((2,2),(3,3),(0.,0.289681084359914),(0.125066077454537,
0.142578551421365),.UNSPECIFIED.)
GEOMETRIC_REPRESENTATION_ITEM()
RATIONAL_B_SPLINE_SURFACE(((0.990621203777022,0.993706096834649,0.999805186472059),
(0.990621203777022,0.993706096834649,0.999805186472059)))
REPRESENTATION_ITEM('')
SURFACE()
);
#2923=(
BOUNDED_SURFACE()
B_SPLINE_SURFACE(1,2,((#144256,#144257,#144258),(#144259,#144260,#144261)),
 .UNSPECIFIED.,.F.,.F.,.F.)
B_SPLINE_SURFACE_WITH_KNOTS((2,2),(3,3),(0.,0.289807040991665),(0.590910950629593,
0.608084585199969),.UNSPECIFIED.)
GEOMETRIC_REPRESENTATION_ITEM()
RATIONAL_B_SPLINE_SURFACE(((0.990053454406147,0.987313720921968,0.987472672298934),
(0.990053454406147,0.987313720921968,0.987472672298934)))
REPRESENTATION_ITEM('')
SURFACE()
);
#2924=(
BOUNDED_SURFACE()
B_SPLINE_SURFACE(1,2,((#144263,#144264,#144265),(#144266,#144267,#144268)),
 .UNSPECIFIED.,.F.,.F.,.F.)
B_SPLINE_SURFACE_WITH_KNOTS((2,2),(3,3),(0.,0.289681084359915),(0.125066077454537,
0.142578551421364),.UNSPECIFIED.)
GEOMETRIC_REPRESENTATION_ITEM()
RATIONAL_B_SPLINE_SURFACE(((0.990621203777022,0.993706096834649,0.999805186472059),
(0.990621203777022,0.993706096834649,0.999805186472059)))
REPRESENTATION_ITEM('')
SURFACE()
);
#2925=(
BOUNDED_SURFACE()
B_SPLINE_SURFACE(1,2,((#144277,#144278,#144279),(#144280,#144281,#144282)),
 .UNSPECIFIED.,.F.,.F.,.F.)
B_SPLINE_SURFACE_WITH_KNOTS((2,2),(3,3),(0.,0.289807040991665),(0.590910950629593,
0.60808458519997),.UNSPECIFIED.)
GEOMETRIC_REPRESENTATION_ITEM()
RATIONAL_B_SPLINE_SURFACE(((0.990053454406147,0.987313720921968,0.987472672298934),
(0.990053454406147,0.987313720921968,0.987472672298934)))
REPRESENTATION_ITEM('')
SURFACE()
);
#2926=(
BOUNDED_SURFACE()
B_SPLINE_SURFACE(1,2,((#144284,#144285,#144286),(#144287,#144288,#144289)),
 .UNSPECIFIED.,.F.,.F.,.F.)
B_SPLINE_SURFACE_WITH_KNOTS((2,2),(3,3),(0.,0.289681084359919),(0.125066077454537,
0.142578551421365),.UNSPECIFIED.)
GEOMETRIC_REPRESENTATION_ITEM()
RATIONAL_B_SPLINE_SURFACE(((0.990621203777022,0.993706096834649,0.999805186472059),
(0.990621203777022,0.993706096834649,0.999805186472059)))
REPRESENTATION_ITEM('')
SURFACE()
);
#2927=(
BOUNDED_SURFACE()
B_SPLINE_SURFACE(1,2,((#144298,#144299,#144300),(#144301,#144302,#144303)),
 .UNSPECIFIED.,.F.,.F.,.F.)
B_SPLINE_SURFACE_WITH_KNOTS((2,2),(3,3),(0.,0.289807040992624),(0.590910950629593,
0.60808458519997),.UNSPECIFIED.)
GEOMETRIC_REPRESENTATION_ITEM()
RATIONAL_B_SPLINE_SURFACE(((0.990053454406147,0.987313720921968,0.987472672298934),
(0.990053454406147,0.987313720921968,0.987472672298934)))
REPRESENTATION_ITEM('')
SURFACE()
);
#2928=(
BOUNDED_SURFACE()
B_SPLINE_SURFACE(1,2,((#144305,#144306,#144307),(#144308,#144309,#144310)),
 .UNSPECIFIED.,.F.,.F.,.F.)
B_SPLINE_SURFACE_WITH_KNOTS((2,2),(3,3),(0.,0.289681084359914),(0.125066077454537,
0.142578551421365),.UNSPECIFIED.)
GEOMETRIC_REPRESENTATION_ITEM()
RATIONAL_B_SPLINE_SURFACE(((0.990621203777022,0.993706096834649,0.999805186472059),
(0.990621203777022,0.993706096834649,0.999805186472059)))
REPRESENTATION_ITEM('')
SURFACE()
);
#2929=(
BOUNDED_SURFACE()
B_SPLINE_SURFACE(1,2,((#144319,#144320,#144321),(#144322,#144323,#144324)),
 .UNSPECIFIED.,.F.,.F.,.F.)
B_SPLINE_SURFACE_WITH_KNOTS((2,2),(3,3),(0.,0.289807040992624),(0.590910950629593,
0.60808458519997),.UNSPECIFIED.)
GEOMETRIC_REPRESENTATION_ITEM()
RATIONAL_B_SPLINE_SURFACE(((0.990053454406147,0.987313720921968,0.987472672298934),
(0.990053454406147,0.987313720921968,0.987472672298934)))
REPRESENTATION_ITEM('')
SURFACE()
);
#2930=(
BOUNDED_SURFACE()
B_SPLINE_SURFACE(1,2,((#144326,#144327,#144328),(#144329,#144330,#144331)),
 .UNSPECIFIED.,.F.,.F.,.F.)
B_SPLINE_SURFACE_WITH_KNOTS((2,2),(3,3),(0.,0.289681084359924),(0.125066077454536,
0.142578551421364),.UNSPECIFIED.)
GEOMETRIC_REPRESENTATION_ITEM()
RATIONAL_B_SPLINE_SURFACE(((0.990621203777022,0.993706096834649,0.999805186472059),
(0.990621203777022,0.993706096834649,0.999805186472059)))
REPRESENTATION_ITEM('')
SURFACE()
);
#2931=(
BOUNDED_SURFACE()
B_SPLINE_SURFACE(1,2,((#144340,#144341,#144342),(#144343,#144344,#144345)),
 .UNSPECIFIED.,.F.,.F.,.F.)
B_SPLINE_SURFACE_WITH_KNOTS((2,2),(3,3),(0.,0.289807040992623),(0.590910950629593,
0.60808458519997),.UNSPECIFIED.)
GEOMETRIC_REPRESENTATION_ITEM()
RATIONAL_B_SPLINE_SURFACE(((0.990053454406147,0.987313720921968,0.987472672298934),
(0.990053454406147,0.987313720921968,0.987472672298934)))
REPRESENTATION_ITEM('')
SURFACE()
);
#2932=(
BOUNDED_SURFACE()
B_SPLINE_SURFACE(1,2,((#144347,#144348,#144349),(#144350,#144351,#144352)),
 .UNSPECIFIED.,.F.,.F.,.F.)
B_SPLINE_SURFACE_WITH_KNOTS((2,2),(3,3),(0.,0.289681084359918),(0.125066077454537,
0.142578551421364),.UNSPECIFIED.)
GEOMETRIC_REPRESENTATION_ITEM()
RATIONAL_B_SPLINE_SURFACE(((0.990621203777022,0.993706096834649,0.999805186472059),
(0.990621203777022,0.993706096834649,0.999805186472059)))
REPRESENTATION_ITEM('')
SURFACE()
);
#2933=(
BOUNDED_SURFACE()
B_SPLINE_SURFACE(1,2,((#144361,#144362,#144363),(#144364,#144365,#144366)),
 .UNSPECIFIED.,.F.,.F.,.F.)
B_SPLINE_SURFACE_WITH_KNOTS((2,2),(3,3),(0.,0.289807040993204),(0.590910950629594,
0.60808458519997),.UNSPECIFIED.)
GEOMETRIC_REPRESENTATION_ITEM()
RATIONAL_B_SPLINE_SURFACE(((0.990053454406147,0.987313720921968,0.987472672298934),
(0.990053454406147,0.987313720921968,0.987472672298934)))
REPRESENTATION_ITEM('')
SURFACE()
);
#2934=(
BOUNDED_SURFACE()
B_SPLINE_SURFACE(1,2,((#144368,#144369,#144370),(#144371,#144372,#144373)),
 .UNSPECIFIED.,.F.,.F.,.F.)
B_SPLINE_SURFACE_WITH_KNOTS((2,2),(3,3),(0.,0.28968108435992),(0.125066077454537,
0.142578551421364),.UNSPECIFIED.)
GEOMETRIC_REPRESENTATION_ITEM()
RATIONAL_B_SPLINE_SURFACE(((0.990621203777022,0.993706096834649,0.999805186472059),
(0.990621203777022,0.993706096834649,0.999805186472059)))
REPRESENTATION_ITEM('')
SURFACE()
);
#2935=(
BOUNDED_SURFACE()
B_SPLINE_SURFACE(1,2,((#144382,#144383,#144384),(#144385,#144386,#144387)),
 .UNSPECIFIED.,.F.,.F.,.F.)
B_SPLINE_SURFACE_WITH_KNOTS((2,2),(3,3),(0.,0.289807040992621),(0.590910950629593,
0.60808458519997),.UNSPECIFIED.)
GEOMETRIC_REPRESENTATION_ITEM()
RATIONAL_B_SPLINE_SURFACE(((0.990053454406147,0.987313720921968,0.987472672298933),
(0.990053454406147,0.987313720921968,0.987472672298933)))
REPRESENTATION_ITEM('')
SURFACE()
);
#2936=(
BOUNDED_SURFACE()
B_SPLINE_SURFACE(1,2,((#144389,#144390,#144391),(#144392,#144393,#144394)),
 .UNSPECIFIED.,.F.,.F.,.F.)
B_SPLINE_SURFACE_WITH_KNOTS((2,2),(3,3),(0.,0.289681084359924),(0.125066077454537,
0.142578551421365),.UNSPECIFIED.)
GEOMETRIC_REPRESENTATION_ITEM()
RATIONAL_B_SPLINE_SURFACE(((0.990621203777022,0.993706096834649,0.999805186472059),
(0.990621203777022,0.993706096834649,0.999805186472059)))
REPRESENTATION_ITEM('')
SURFACE()
);
#2937=(
BOUNDED_SURFACE()
B_SPLINE_SURFACE(1,2,((#144403,#144404,#144405),(#144406,#144407,#144408)),
 .UNSPECIFIED.,.F.,.F.,.F.)
B_SPLINE_SURFACE_WITH_KNOTS((2,2),(3,3),(0.,0.289807040993174),(0.590910950629593,
0.60808458519997),.UNSPECIFIED.)
GEOMETRIC_REPRESENTATION_ITEM()
RATIONAL_B_SPLINE_SURFACE(((0.990053454406147,0.987313720921968,0.987472672298934),
(0.990053454406147,0.987313720921968,0.987472672298934)))
REPRESENTATION_ITEM('')
SURFACE()
);
#2938=(
BOUNDED_SURFACE()
B_SPLINE_SURFACE(1,2,((#144410,#144411,#144412),(#144413,#144414,#144415)),
 .UNSPECIFIED.,.F.,.F.,.F.)
B_SPLINE_SURFACE_WITH_KNOTS((2,2),(3,3),(0.,0.289681084359917),(0.125066077454537,
0.142578551421364),.UNSPECIFIED.)
GEOMETRIC_REPRESENTATION_ITEM()
RATIONAL_B_SPLINE_SURFACE(((0.990621203777022,0.993706096834649,0.999805186472059),
(0.990621203777022,0.993706096834649,0.999805186472059)))
REPRESENTATION_ITEM('')
SURFACE()
);
#2939=(
BOUNDED_SURFACE()
B_SPLINE_SURFACE(1,2,((#144424,#144425,#144426),(#144427,#144428,#144429)),
 .UNSPECIFIED.,.F.,.F.,.F.)
B_SPLINE_SURFACE_WITH_KNOTS((2,2),(3,3),(0.,0.289807040992982),(0.590910950629594,
0.60808458519997),.UNSPECIFIED.)
GEOMETRIC_REPRESENTATION_ITEM()
RATIONAL_B_SPLINE_SURFACE(((0.990053454406147,0.987313720921968,0.987472672298933),
(0.990053454406147,0.987313720921968,0.987472672298933)))
REPRESENTATION_ITEM('')
SURFACE()
);
#2940=(
BOUNDED_SURFACE()
B_SPLINE_SURFACE(1,2,((#144431,#144432,#144433),(#144434,#144435,#144436)),
 .UNSPECIFIED.,.F.,.F.,.F.)
B_SPLINE_SURFACE_WITH_KNOTS((2,2),(3,3),(0.,0.289681084359923),(0.125066077454536,
0.142578551421363),.UNSPECIFIED.)
GEOMETRIC_REPRESENTATION_ITEM()
RATIONAL_B_SPLINE_SURFACE(((0.990621203777021,0.993706096834649,0.999805186472059),
(0.990621203777021,0.993706096834649,0.999805186472059)))
REPRESENTATION_ITEM('')
SURFACE()
);
#2941=(
BOUNDED_SURFACE()
B_SPLINE_SURFACE(1,2,((#144445,#144446,#144447),(#144448,#144449,#144450)),
 .UNSPECIFIED.,.F.,.F.,.F.)
B_SPLINE_SURFACE_WITH_KNOTS((2,2),(3,3),(0.,0.289807040993021),(0.590910950629594,
0.608084585199971),.UNSPECIFIED.)
GEOMETRIC_REPRESENTATION_ITEM()
RATIONAL_B_SPLINE_SURFACE(((0.990053454406147,0.987313720921968,0.987472672298934),
(0.990053454406147,0.987313720921968,0.987472672298934)))
REPRESENTATION_ITEM('')
SURFACE()
);
#2942=(
BOUNDED_SURFACE()
B_SPLINE_SURFACE(1,2,((#144452,#144453,#144454),(#144455,#144456,#144457)),
 .UNSPECIFIED.,.F.,.F.,.F.)
B_SPLINE_SURFACE_WITH_KNOTS((2,2),(3,3),(0.,0.289681084359917),(0.125066077454535,
0.142578551421363),.UNSPECIFIED.)
GEOMETRIC_REPRESENTATION_ITEM()
RATIONAL_B_SPLINE_SURFACE(((0.990621203777021,0.993706096834649,0.999805186472059),
(0.990621203777021,0.993706096834649,0.999805186472059)))
REPRESENTATION_ITEM('')
SURFACE()
);
#2943=(
BOUNDED_SURFACE()
B_SPLINE_SURFACE(1,2,((#144466,#144467,#144468),(#144469,#144470,#144471)),
 .UNSPECIFIED.,.F.,.F.,.F.)
B_SPLINE_SURFACE_WITH_KNOTS((2,2),(3,3),(0.,0.289807040993297),(0.590910950629594,
0.608084585199971),.UNSPECIFIED.)
GEOMETRIC_REPRESENTATION_ITEM()
RATIONAL_B_SPLINE_SURFACE(((0.990053454406147,0.987313720921968,0.987472672298934),
(0.990053454406147,0.987313720921968,0.987472672298934)))
REPRESENTATION_ITEM('')
SURFACE()
);
#2944=(
BOUNDED_SURFACE()
B_SPLINE_SURFACE(1,2,((#144473,#144474,#144475),(#144476,#144477,#144478)),
 .UNSPECIFIED.,.F.,.F.,.F.)
B_SPLINE_SURFACE_WITH_KNOTS((2,2),(3,3),(0.,0.289681084359922),(0.125066077454535,
0.142578551421363),.UNSPECIFIED.)
GEOMETRIC_REPRESENTATION_ITEM()
RATIONAL_B_SPLINE_SURFACE(((0.990621203777021,0.993706096834649,0.999805186472059),
(0.990621203777021,0.993706096834649,0.999805186472059)))
REPRESENTATION_ITEM('')
SURFACE()
);
#2945=(
BOUNDED_SURFACE()
B_SPLINE_SURFACE(1,2,((#144487,#144488,#144489),(#144490,#144491,#144492)),
 .UNSPECIFIED.,.F.,.F.,.F.)
B_SPLINE_SURFACE_WITH_KNOTS((2,2),(3,3),(0.,0.289807040992709),(0.590910950629594,
0.608084585199971),.UNSPECIFIED.)
GEOMETRIC_REPRESENTATION_ITEM()
RATIONAL_B_SPLINE_SURFACE(((0.990053454406147,0.987313720921968,0.987472672298934),
(0.990053454406147,0.987313720921968,0.987472672298934)))
REPRESENTATION_ITEM('')
SURFACE()
);
#2946=(
BOUNDED_SURFACE()
B_SPLINE_SURFACE(1,2,((#144494,#144495,#144496),(#144497,#144498,#144499)),
 .UNSPECIFIED.,.F.,.F.,.F.)
B_SPLINE_SURFACE_WITH_KNOTS((2,2),(3,3),(0.,0.289681084359921),(0.125066077454536,
0.142578551421363),.UNSPECIFIED.)
GEOMETRIC_REPRESENTATION_ITEM()
RATIONAL_B_SPLINE_SURFACE(((0.990621203777021,0.993706096834649,0.999805186472059),
(0.990621203777021,0.993706096834649,0.999805186472059)))
REPRESENTATION_ITEM('')
SURFACE()
);
#2947=(
BOUNDED_SURFACE()
B_SPLINE_SURFACE(1,2,((#144508,#144509,#144510),(#144511,#144512,#144513)),
 .UNSPECIFIED.,.F.,.F.,.F.)
B_SPLINE_SURFACE_WITH_KNOTS((2,2),(3,3),(0.,0.289807040993544),(0.590910950629594,
0.608084585199971),.UNSPECIFIED.)
GEOMETRIC_REPRESENTATION_ITEM()
RATIONAL_B_SPLINE_SURFACE(((0.990053454406147,0.987313720921967,0.987472672298934),
(0.990053454406147,0.987313720921967,0.987472672298934)))
REPRESENTATION_ITEM('')
SURFACE()
);
#2948=(
BOUNDED_SURFACE()
B_SPLINE_SURFACE(1,2,((#144515,#144516,#144517),(#144518,#144519,#144520)),
 .UNSPECIFIED.,.F.,.F.,.F.)
B_SPLINE_SURFACE_WITH_KNOTS((2,2),(3,3),(0.,0.289681084359919),(0.125066077454536,
0.142578551421363),.UNSPECIFIED.)
GEOMETRIC_REPRESENTATION_ITEM()
RATIONAL_B_SPLINE_SURFACE(((0.990621203777021,0.993706096834649,0.999805186472059),
(0.990621203777021,0.993706096834649,0.999805186472059)))
REPRESENTATION_ITEM('')
SURFACE()
);
#2949=(
BOUNDED_SURFACE()
B_SPLINE_SURFACE(1,2,((#144529,#144530,#144531),(#144532,#144533,#144534)),
 .UNSPECIFIED.,.F.,.F.,.F.)
B_SPLINE_SURFACE_WITH_KNOTS((2,2),(3,3),(0.,0.289807040993043),(0.590910950629594,
0.608084585199971),.UNSPECIFIED.)
GEOMETRIC_REPRESENTATION_ITEM()
RATIONAL_B_SPLINE_SURFACE(((0.990053454406147,0.987313720921967,0.987472672298933),
(0.990053454406147,0.987313720921967,0.987472672298933)))
REPRESENTATION_ITEM('')
SURFACE()
);
#2950=(
BOUNDED_SURFACE()
B_SPLINE_SURFACE(1,2,((#144536,#144537,#144538),(#144539,#144540,#144541)),
 .UNSPECIFIED.,.F.,.F.,.F.)
B_SPLINE_SURFACE_WITH_KNOTS((2,2),(3,3),(0.,0.289681084359923),(0.125066077454536,
0.142578551421363),.UNSPECIFIED.)
GEOMETRIC_REPRESENTATION_ITEM()
RATIONAL_B_SPLINE_SURFACE(((0.990621203777021,0.993706096834649,0.999805186472059),
(0.990621203777021,0.993706096834649,0.999805186472059)))
REPRESENTATION_ITEM('')
SURFACE()
);
#2951=(
BOUNDED_SURFACE()
B_SPLINE_SURFACE(1,2,((#144550,#144551,#144552),(#144553,#144554,#144555)),
 .UNSPECIFIED.,.F.,.F.,.F.)
B_SPLINE_SURFACE_WITH_KNOTS((2,2),(3,3),(0.,0.289807040993516),(0.590910950629594,
0.608084585199971),.UNSPECIFIED.)
GEOMETRIC_REPRESENTATION_ITEM()
RATIONAL_B_SPLINE_SURFACE(((0.990053454406147,0.987313720921967,0.987472672298933),
(0.990053454406147,0.987313720921967,0.987472672298933)))
REPRESENTATION_ITEM('')
SURFACE()
);
#2952=(
BOUNDED_SURFACE()
B_SPLINE_SURFACE(1,2,((#144557,#144558,#144559),(#144560,#144561,#144562)),
 .UNSPECIFIED.,.F.,.F.,.F.)
B_SPLINE_SURFACE_WITH_KNOTS((2,2),(3,3),(0.,0.289681084359921),(0.125066077454535,
0.142578551421364),.UNSPECIFIED.)
GEOMETRIC_REPRESENTATION_ITEM()
RATIONAL_B_SPLINE_SURFACE(((0.990621203777021,0.993706096834649,0.999805186472059),
(0.990621203777021,0.993706096834649,0.999805186472059)))
REPRESENTATION_ITEM('')
SURFACE()
);
#2953=(
BOUNDED_SURFACE()
B_SPLINE_SURFACE(1,2,((#144571,#144572,#144573),(#144574,#144575,#144576)),
 .UNSPECIFIED.,.F.,.F.,.F.)
B_SPLINE_SURFACE_WITH_KNOTS((2,2),(3,3),(0.,0.28980704099326),(0.590910950629594,
0.608084585199971),.UNSPECIFIED.)
GEOMETRIC_REPRESENTATION_ITEM()
RATIONAL_B_SPLINE_SURFACE(((0.990053454406147,0.987313720921968,0.987472672298934),
(0.990053454406147,0.987313720921968,0.987472672298934)))
REPRESENTATION_ITEM('')
SURFACE()
);
#2954=(
BOUNDED_SURFACE()
B_SPLINE_SURFACE(1,2,((#144578,#144579,#144580),(#144581,#144582,#144583)),
 .UNSPECIFIED.,.F.,.F.,.F.)
B_SPLINE_SURFACE_WITH_KNOTS((2,2),(3,3),(0.,0.28968108435992),(0.125066077454535,
0.142578551421363),.UNSPECIFIED.)
GEOMETRIC_REPRESENTATION_ITEM()
RATIONAL_B_SPLINE_SURFACE(((0.990621203777021,0.993706096834649,0.999805186472059),
(0.990621203777021,0.993706096834649,0.999805186472059)))
REPRESENTATION_ITEM('')
SURFACE()
);
#2955=(
BOUNDED_SURFACE()
B_SPLINE_SURFACE(1,2,((#144592,#144593,#144594),(#144595,#144596,#144597)),
 .UNSPECIFIED.,.F.,.F.,.F.)
B_SPLINE_SURFACE_WITH_KNOTS((2,2),(3,3),(0.,0.289807040994422),(0.590910950629595,
0.608084585199971),.UNSPECIFIED.)
GEOMETRIC_REPRESENTATION_ITEM()
RATIONAL_B_SPLINE_SURFACE(((0.990053454406147,0.987313720921968,0.987472672298934),
(0.990053454406147,0.987313720921968,0.987472672298934)))
REPRESENTATION_ITEM('')
SURFACE()
);
#2956=(
BOUNDED_SURFACE()
B_SPLINE_SURFACE(1,2,((#144599,#144600,#144601),(#144602,#144603,#144604)),
 .UNSPECIFIED.,.F.,.F.,.F.)
B_SPLINE_SURFACE_WITH_KNOTS((2,2),(3,3),(0.,0.289681084359924),(0.125066077454535,
0.142578551421363),.UNSPECIFIED.)
GEOMETRIC_REPRESENTATION_ITEM()
RATIONAL_B_SPLINE_SURFACE(((0.990621203777021,0.993706096834649,0.999805186472059),
(0.990621203777021,0.993706096834649,0.999805186472059)))
REPRESENTATION_ITEM('')
SURFACE()
);
#2957=(
BOUNDED_SURFACE()
B_SPLINE_SURFACE(1,2,((#144613,#144614,#144615),(#144616,#144617,#144618)),
 .UNSPECIFIED.,.F.,.F.,.F.)
B_SPLINE_SURFACE_WITH_KNOTS((2,2),(3,3),(0.,0.289807040992761),(0.590910950629594,
0.608084585199971),.UNSPECIFIED.)
GEOMETRIC_REPRESENTATION_ITEM()
RATIONAL_B_SPLINE_SURFACE(((0.990053454406147,0.987313720921967,0.987472672298933),
(0.990053454406147,0.987313720921967,0.987472672298933)))
REPRESENTATION_ITEM('')
SURFACE()
);
#2958=(
BOUNDED_SURFACE()
B_SPLINE_SURFACE(1,2,((#144620,#144621,#144622),(#144623,#144624,#144625)),
 .UNSPECIFIED.,.F.,.F.,.F.)
B_SPLINE_SURFACE_WITH_KNOTS((2,2),(3,3),(0.,0.289681084359926),(0.125066077454535,
0.142578551421363),.UNSPECIFIED.)
GEOMETRIC_REPRESENTATION_ITEM()
RATIONAL_B_SPLINE_SURFACE(((0.990621203777021,0.993706096834649,0.999805186472059),
(0.990621203777021,0.993706096834649,0.999805186472059)))
REPRESENTATION_ITEM('')
SURFACE()
);
#2959=(
BOUNDED_SURFACE()
B_SPLINE_SURFACE(1,2,((#144634,#144635,#144636),(#144637,#144638,#144639)),
 .UNSPECIFIED.,.F.,.F.,.F.)
B_SPLINE_SURFACE_WITH_KNOTS((2,2),(3,3),(0.,0.289807040992643),(0.590910950629594,
0.608084585199971),.UNSPECIFIED.)
GEOMETRIC_REPRESENTATION_ITEM()
RATIONAL_B_SPLINE_SURFACE(((0.990053454406147,0.987313720921968,0.987472672298934),
(0.990053454406147,0.987313720921967,0.987472672298933)))
REPRESENTATION_ITEM('')
SURFACE()
);
#2960=(
BOUNDED_SURFACE()
B_SPLINE_SURFACE(1,2,((#144641,#144642,#144643),(#144644,#144645,#144646)),
 .UNSPECIFIED.,.F.,.F.,.F.)
B_SPLINE_SURFACE_WITH_KNOTS((2,2),(3,3),(0.,0.28968108435992),(0.125066077454535,
0.142578551421364),.UNSPECIFIED.)
GEOMETRIC_REPRESENTATION_ITEM()
RATIONAL_B_SPLINE_SURFACE(((0.990621203777021,0.993706096834649,0.999805186472059),
(0.990621203777021,0.993706096834649,0.999805186472059)))
REPRESENTATION_ITEM('')
SURFACE()
);
#2961=(
BOUNDED_SURFACE()
B_SPLINE_SURFACE(1,2,((#144655,#144656,#144657),(#144658,#144659,#144660)),
 .UNSPECIFIED.,.F.,.F.,.F.)
B_SPLINE_SURFACE_WITH_KNOTS((2,2),(3,3),(0.,0.289807040993492),(0.590910950629594,
0.608084585199971),.UNSPECIFIED.)
GEOMETRIC_REPRESENTATION_ITEM()
RATIONAL_B_SPLINE_SURFACE(((0.990053454406147,0.987313720921968,0.987472672298934),
(0.990053454406147,0.987313720921968,0.987472672298934)))
REPRESENTATION_ITEM('')
SURFACE()
);
#2962=(
BOUNDED_SURFACE()
B_SPLINE_SURFACE(1,2,((#144662,#144663,#144664),(#144665,#144666,#144667)),
 .UNSPECIFIED.,.F.,.F.,.F.)
B_SPLINE_SURFACE_WITH_KNOTS((2,2),(3,3),(0.,0.28968108435993),(0.125066077454536,
0.142578551421364),.UNSPECIFIED.)
GEOMETRIC_REPRESENTATION_ITEM()
RATIONAL_B_SPLINE_SURFACE(((0.990621203777021,0.993706096834649,0.999805186472059),
(0.990621203777021,0.993706096834649,0.999805186472059)))
REPRESENTATION_ITEM('')
SURFACE()
);
#2963=(
BOUNDED_SURFACE()
B_SPLINE_SURFACE(1,2,((#144676,#144677,#144678),(#144679,#144680,#144681)),
 .UNSPECIFIED.,.F.,.F.,.F.)
B_SPLINE_SURFACE_WITH_KNOTS((2,2),(3,3),(0.,0.289807040992016),(0.590910950629594,
0.608084585199971),.UNSPECIFIED.)
GEOMETRIC_REPRESENTATION_ITEM()
RATIONAL_B_SPLINE_SURFACE(((0.990053454406147,0.987313720921968,0.987472672298934),
(0.990053454406147,0.987313720921968,0.987472672298934)))
REPRESENTATION_ITEM('')
SURFACE()
);
#2964=(
BOUNDED_SURFACE()
B_SPLINE_SURFACE(1,2,((#144683,#144684,#144685),(#144686,#144687,#144688)),
 .UNSPECIFIED.,.F.,.F.,.F.)
B_SPLINE_SURFACE_WITH_KNOTS((2,2),(3,3),(0.,0.289681084359924),(0.125066077454536,
0.142578551421363),.UNSPECIFIED.)
GEOMETRIC_REPRESENTATION_ITEM()
RATIONAL_B_SPLINE_SURFACE(((0.990621203777021,0.993706096834649,0.999805186472059),
(0.990621203777021,0.993706096834649,0.999805186472059)))
REPRESENTATION_ITEM('')
SURFACE()
);
#2965=(
BOUNDED_SURFACE()
B_SPLINE_SURFACE(1,2,((#144697,#144698,#144699),(#144700,#144701,#144702)),
 .UNSPECIFIED.,.F.,.F.,.F.)
B_SPLINE_SURFACE_WITH_KNOTS((2,2),(3,3),(0.,0.289807040992888),(0.590910950629594,
0.608084585199975),.UNSPECIFIED.)
GEOMETRIC_REPRESENTATION_ITEM()
RATIONAL_B_SPLINE_SURFACE(((0.990053454406147,0.987313720921967,0.987472672298934),
(0.990053454406147,0.987313720921967,0.987472672298934)))
REPRESENTATION_ITEM('')
SURFACE()
);
#2966=(
BOUNDED_SURFACE()
B_SPLINE_SURFACE(1,2,((#144704,#144705,#144706),(#144707,#144708,#144709)),
 .UNSPECIFIED.,.F.,.F.,.F.)
B_SPLINE_SURFACE_WITH_KNOTS((2,2),(3,3),(0.,0.289681084359926),(0.125066077454535,
0.142578551421364),.UNSPECIFIED.)
GEOMETRIC_REPRESENTATION_ITEM()
RATIONAL_B_SPLINE_SURFACE(((0.990621203777021,0.993706096834649,0.999805186472059),
(0.990621203777021,0.993706096834649,0.999805186472059)))
REPRESENTATION_ITEM('')
SURFACE()
);
#2967=(
BOUNDED_SURFACE()
B_SPLINE_SURFACE(1,2,((#144718,#144719,#144720),(#144721,#144722,#144723)),
 .UNSPECIFIED.,.F.,.F.,.F.)
B_SPLINE_SURFACE_WITH_KNOTS((2,2),(3,3),(0.,0.289807040992692),(0.590910950629594,
0.608084585199971),.UNSPECIFIED.)
GEOMETRIC_REPRESENTATION_ITEM()
RATIONAL_B_SPLINE_SURFACE(((0.990053454406147,0.987313720921968,0.987472672298934),
(0.990053454406147,0.987313720921967,0.987472672298933)))
REPRESENTATION_ITEM('')
SURFACE()
);
#2968=(
BOUNDED_SURFACE()
B_SPLINE_SURFACE(1,2,((#144725,#144726,#144727),(#144728,#144729,#144730)),
 .UNSPECIFIED.,.F.,.F.,.F.)
B_SPLINE_SURFACE_WITH_KNOTS((2,2),(3,3),(0.,0.289681084359928),(0.125066077454535,
0.142578551421363),.UNSPECIFIED.)
GEOMETRIC_REPRESENTATION_ITEM()
RATIONAL_B_SPLINE_SURFACE(((0.990621203777021,0.993706096834649,0.999805186472059),
(0.990621203777021,0.993706096834649,0.999805186472059)))
REPRESENTATION_ITEM('')
SURFACE()
);
#2969=(
BOUNDED_SURFACE()
B_SPLINE_SURFACE(1,2,((#144739,#144740,#144741),(#144742,#144743,#144744)),
 .UNSPECIFIED.,.F.,.F.,.F.)
B_SPLINE_SURFACE_WITH_KNOTS((2,2),(3,3),(0.,0.289807040993932),(0.590910950629594,
0.608084585199971),.UNSPECIFIED.)
GEOMETRIC_REPRESENTATION_ITEM()
RATIONAL_B_SPLINE_SURFACE(((0.990053454406147,0.987313720921968,0.987472672298934),
(0.990053454406147,0.987313720921968,0.987472672298934)))
REPRESENTATION_ITEM('')
SURFACE()
);
#2970=(
BOUNDED_SURFACE()
B_SPLINE_SURFACE(1,2,((#144746,#144747,#144748),(#144749,#144750,#144751)),
 .UNSPECIFIED.,.F.,.F.,.F.)
B_SPLINE_SURFACE_WITH_KNOTS((2,2),(3,3),(0.,0.289681084359915),(0.125066077454536,
0.142578551421431),.UNSPECIFIED.)
GEOMETRIC_REPRESENTATION_ITEM()
RATIONAL_B_SPLINE_SURFACE(((0.990621203777022,0.993706096834661,0.999805186472106),
(0.990621203777022,0.993706096834661,0.999805186472106)))
REPRESENTATION_ITEM('')
SURFACE()
);
#2971=(
BOUNDED_SURFACE()
B_SPLINE_SURFACE(1,2,((#144760,#144761,#144762),(#144763,#144764,#144765)),
 .UNSPECIFIED.,.F.,.F.,.F.)
B_SPLINE_SURFACE_WITH_KNOTS((2,2),(3,3),(0.,0.28980704099156),(0.590910950629593,
0.60808458519997),.UNSPECIFIED.)
GEOMETRIC_REPRESENTATION_ITEM()
RATIONAL_B_SPLINE_SURFACE(((0.990053454406147,0.987313720921968,0.987472672298934),
(0.990053454406147,0.987313720921968,0.987472672298934)))
REPRESENTATION_ITEM('')
SURFACE()
);
#2972=(
BOUNDED_SURFACE()
B_SPLINE_SURFACE(1,2,((#144767,#144768,#144769),(#144770,#144771,#144772)),
 .UNSPECIFIED.,.F.,.F.,.F.)
B_SPLINE_SURFACE_WITH_KNOTS((2,2),(3,3),(0.,0.289681084359916),(0.125066077454537,
0.142578551421365),.UNSPECIFIED.)
GEOMETRIC_REPRESENTATION_ITEM()
RATIONAL_B_SPLINE_SURFACE(((0.990621203777022,0.993706096834649,0.999805186472059),
(0.990621203777022,0.993706096834649,0.999805186472059)))
REPRESENTATION_ITEM('')
SURFACE()
);
#2973=(
BOUNDED_SURFACE()
B_SPLINE_SURFACE(1,2,((#144781,#144782,#144783),(#144784,#144785,#144786)),
 .UNSPECIFIED.,.F.,.F.,.F.)
B_SPLINE_SURFACE_WITH_KNOTS((2,2),(3,3),(0.,0.289807040991557),(0.590910950629593,
0.60808458519997),.UNSPECIFIED.)
GEOMETRIC_REPRESENTATION_ITEM()
RATIONAL_B_SPLINE_SURFACE(((0.990053454406147,0.987313720921968,0.987472672298933),
(0.990053454406147,0.987313720921968,0.987472672298933)))
REPRESENTATION_ITEM('')
SURFACE()
);
#2974=(
BOUNDED_SURFACE()
B_SPLINE_SURFACE(1,2,((#144788,#144789,#144790),(#144791,#144792,#144793)),
 .UNSPECIFIED.,.F.,.F.,.F.)
B_SPLINE_SURFACE_WITH_KNOTS((2,2),(3,3),(0.,0.289681084359917),(0.125066077454537,
0.142578551421365),.UNSPECIFIED.)
GEOMETRIC_REPRESENTATION_ITEM()
RATIONAL_B_SPLINE_SURFACE(((0.990621203777022,0.993706096834649,0.999805186472059),
(0.990621203777022,0.993706096834649,0.999805186472059)))
REPRESENTATION_ITEM('')
SURFACE()
);
#2975=(
BOUNDED_SURFACE()
B_SPLINE_SURFACE(1,2,((#144802,#144803,#144804),(#144805,#144806,#144807)),
 .UNSPECIFIED.,.F.,.F.,.F.)
B_SPLINE_SURFACE_WITH_KNOTS((2,2),(3,3),(0.,0.289807040991893),(0.590910950629593,
0.60808458519997),.UNSPECIFIED.)
GEOMETRIC_REPRESENTATION_ITEM()
RATIONAL_B_SPLINE_SURFACE(((0.990053454406147,0.987313720921968,0.987472672298934),
(0.990053454406147,0.987313720921968,0.987472672298934)))
REPRESENTATION_ITEM('')
SURFACE()
);
#2976=(
BOUNDED_SURFACE()
B_SPLINE_SURFACE(1,2,((#144809,#144810,#144811),(#144812,#144813,#144814)),
 .UNSPECIFIED.,.F.,.F.,.F.)
B_SPLINE_SURFACE_WITH_KNOTS((2,2),(3,3),(0.,0.289681084359919),(0.125066077454537,
0.142578551421364),.UNSPECIFIED.)
GEOMETRIC_REPRESENTATION_ITEM()
RATIONAL_B_SPLINE_SURFACE(((0.990621203777022,0.993706096834649,0.999805186472059),
(0.990621203777022,0.993706096834649,0.999805186472059)))
REPRESENTATION_ITEM('')
SURFACE()
);
#2977=(
BOUNDED_SURFACE()
B_SPLINE_SURFACE(1,2,((#144823,#144824,#144825),(#144826,#144827,#144828)),
 .UNSPECIFIED.,.F.,.F.,.F.)
B_SPLINE_SURFACE_WITH_KNOTS((2,2),(3,3),(0.,0.289807040992024),(0.590910950629593,
0.60808458519997),.UNSPECIFIED.)
GEOMETRIC_REPRESENTATION_ITEM()
RATIONAL_B_SPLINE_SURFACE(((0.990053454406147,0.987313720921968,0.987472672298933),
(0.990053454406147,0.987313720921968,0.987472672298933)))
REPRESENTATION_ITEM('')
SURFACE()
);
#2978=(
BOUNDED_SURFACE()
B_SPLINE_SURFACE(1,2,((#144830,#144831,#144832),(#144833,#144834,#144835)),
 .UNSPECIFIED.,.F.,.F.,.F.)
B_SPLINE_SURFACE_WITH_KNOTS((2,2),(3,3),(0.,0.28968108435992),(0.538896351358318,
0.556212823028861),.UNSPECIFIED.)
GEOMETRIC_REPRESENTATION_ITEM()
RATIONAL_B_SPLINE_SURFACE(((0.987563472532048,0.988105030697865,0.991593692313265),
(0.987563472532048,0.988105030697865,0.991593692313265)))
REPRESENTATION_ITEM('')
SURFACE()
);
#2979=(
BOUNDED_SURFACE()
B_SPLINE_SURFACE(1,2,((#144846,#144847,#144848),(#144849,#144850,#144851)),
 .UNSPECIFIED.,.F.,.F.,.F.)
B_SPLINE_SURFACE_WITH_KNOTS((2,2),(3,3),(0.,0.289807040991565),(0.176967058622922,
0.194235682574593),.UNSPECIFIED.)
GEOMETRIC_REPRESENTATION_ITEM()
RATIONAL_B_SPLINE_SURFACE(((0.98748925405691,0.987216959588932,0.989875504592249),
(0.98748925405691,0.987216959588932,0.989875504592249)))
REPRESENTATION_ITEM('')
SURFACE()
);
#2980=(
BOUNDED_SURFACE()
B_SPLINE_SURFACE(1,2,((#144868,#144869,#144870),(#144871,#144872,#144873)),
 .UNSPECIFIED.,.F.,.F.,.F.)
B_SPLINE_SURFACE_WITH_KNOTS((2,2),(3,3),(0.,0.289681084359927),(0.538896351358318,
0.556212823028864),.UNSPECIFIED.)
GEOMETRIC_REPRESENTATION_ITEM()
RATIONAL_B_SPLINE_SURFACE(((0.987563472532048,0.988105030697865,0.991593692313266),
(0.987563472532048,0.988105030697865,0.991593692313266)))
REPRESENTATION_ITEM('')
SURFACE()
);
#2981=(
BOUNDED_SURFACE()
B_SPLINE_SURFACE(1,2,((#144875,#144876,#144877),(#144878,#144879,#144880)),
 .UNSPECIFIED.,.F.,.F.,.F.)
B_SPLINE_SURFACE_WITH_KNOTS((2,2),(3,3),(0.,0.289807040991563),(0.176967058622922,
0.194235682574592),.UNSPECIFIED.)
GEOMETRIC_REPRESENTATION_ITEM()
RATIONAL_B_SPLINE_SURFACE(((0.98748925405691,0.987216959588932,0.989875504592249),
(0.98748925405691,0.987216959588932,0.989875504592249)))
REPRESENTATION_ITEM('')
SURFACE()
);
#2982=(
BOUNDED_SURFACE()
B_SPLINE_SURFACE(1,2,((#144897,#144898,#144899),(#144900,#144901,#144902)),
 .UNSPECIFIED.,.F.,.F.,.F.)
B_SPLINE_SURFACE_WITH_KNOTS((2,2),(3,3),(0.,0.289681084359915),(0.538896351358319,
0.556212823028862),.UNSPECIFIED.)
GEOMETRIC_REPRESENTATION_ITEM()
RATIONAL_B_SPLINE_SURFACE(((0.987563472532048,0.988105030697866,0.991593692313266),
(0.987563472532048,0.988105030697866,0.991593692313266)))
REPRESENTATION_ITEM('')
SURFACE()
);
#2983=(
BOUNDED_SURFACE()
B_SPLINE_SURFACE(1,2,((#144904,#144905,#144906),(#144907,#144908,#144909)),
 .UNSPECIFIED.,.F.,.F.,.F.)
B_SPLINE_SURFACE_WITH_KNOTS((2,2),(3,3),(0.,0.289807040991566),(0.176967058622921,
0.194235682574592),.UNSPECIFIED.)
GEOMETRIC_REPRESENTATION_ITEM()
RATIONAL_B_SPLINE_SURFACE(((0.98748925405691,0.987216959588932,0.989875504592249),
(0.98748925405691,0.987216959588932,0.989875504592249)))
REPRESENTATION_ITEM('')
SURFACE()
);
#2984=(
BOUNDED_SURFACE()
B_SPLINE_SURFACE(1,2,((#144926,#144927,#144928),(#144929,#144930,#144931)),
 .UNSPECIFIED.,.F.,.F.,.F.)
B_SPLINE_SURFACE_WITH_KNOTS((2,2),(3,3),(0.,0.289681084359933),(0.538896351358319,
0.556212823028862),.UNSPECIFIED.)
GEOMETRIC_REPRESENTATION_ITEM()
RATIONAL_B_SPLINE_SURFACE(((0.987563472532048,0.988105030697866,0.991593692313266),
(0.987563472532048,0.988105030697866,0.991593692313266)))
REPRESENTATION_ITEM('')
SURFACE()
);
#2985=(
BOUNDED_SURFACE()
B_SPLINE_SURFACE(1,2,((#144933,#144934,#144935),(#144936,#144937,#144938)),
 .UNSPECIFIED.,.F.,.F.,.F.)
B_SPLINE_SURFACE_WITH_KNOTS((2,2),(3,3),(0.,0.289807040991557),(0.176967058622921,
0.194235682574592),.UNSPECIFIED.)
GEOMETRIC_REPRESENTATION_ITEM()
RATIONAL_B_SPLINE_SURFACE(((0.98748925405691,0.987216959588932,0.989875504592249),
(0.98748925405691,0.987216959588932,0.989875504592249)))
REPRESENTATION_ITEM('')
SURFACE()
);
#2986=(
BOUNDED_SURFACE()
B_SPLINE_SURFACE(1,2,((#144955,#144956,#144957),(#144958,#144959,#144960)),
 .UNSPECIFIED.,.F.,.F.,.F.)
B_SPLINE_SURFACE_WITH_KNOTS((2,2),(3,3),(0.,0.289681084359922),(0.538896351358319,
0.556212823028865),.UNSPECIFIED.)
GEOMETRIC_REPRESENTATION_ITEM()
RATIONAL_B_SPLINE_SURFACE(((0.987563472532048,0.988105030697866,0.991593692313267),
(0.987563472532048,0.988105030697866,0.991593692313267)))
REPRESENTATION_ITEM('')
SURFACE()
);
#2987=(
BOUNDED_SURFACE()
B_SPLINE_SURFACE(1,2,((#144962,#144963,#144964),(#144965,#144966,#144967)),
 .UNSPECIFIED.,.F.,.F.,.F.)
B_SPLINE_SURFACE_WITH_KNOTS((2,2),(3,3),(0.,0.289807040991562),(0.176967058622921,
0.194235682574592),.UNSPECIFIED.)
GEOMETRIC_REPRESENTATION_ITEM()
RATIONAL_B_SPLINE_SURFACE(((0.98748925405691,0.987216959588932,0.989875504592249),
(0.98748925405691,0.987216959588932,0.989875504592249)))
REPRESENTATION_ITEM('')
SURFACE()
);
#2988=(
BOUNDED_SURFACE()
B_SPLINE_SURFACE(1,2,((#144984,#144985,#144986),(#144987,#144988,#144989)),
 .UNSPECIFIED.,.F.,.F.,.F.)
B_SPLINE_SURFACE_WITH_KNOTS((2,2),(3,3),(0.,0.289681084359927),(0.538896351358319,
0.556212823028865),.UNSPECIFIED.)
GEOMETRIC_REPRESENTATION_ITEM()
RATIONAL_B_SPLINE_SURFACE(((0.987563472532048,0.988105030697866,0.991593692313267),
(0.987563472532048,0.988105030697866,0.991593692313267)))
REPRESENTATION_ITEM('')
SURFACE()
);
#2989=(
BOUNDED_SURFACE()
B_SPLINE_SURFACE(1,2,((#144991,#144992,#144993),(#144994,#144995,#144996)),
 .UNSPECIFIED.,.F.,.F.,.F.)
B_SPLINE_SURFACE_WITH_KNOTS((2,2),(3,3),(0.,0.289807040991562),(0.176967058622921,
0.194235682574592),.UNSPECIFIED.)
GEOMETRIC_REPRESENTATION_ITEM()
RATIONAL_B_SPLINE_SURFACE(((0.98748925405691,0.987216959588931,0.989875504592249),
(0.98748925405691,0.987216959588932,0.989875504592249)))
REPRESENTATION_ITEM('')
SURFACE()
);
#2990=(
BOUNDED_SURFACE()
B_SPLINE_SURFACE(1,2,((#145013,#145014,#145015),(#145016,#145017,#145018)),
 .UNSPECIFIED.,.F.,.F.,.F.)
B_SPLINE_SURFACE_WITH_KNOTS((2,2),(3,3),(0.,0.289681084359927),(0.538896351358319,
0.556212823028862),.UNSPECIFIED.)
GEOMETRIC_REPRESENTATION_ITEM()
RATIONAL_B_SPLINE_SURFACE(((0.987563472532048,0.988105030697866,0.991593692313266),
(0.987563472532048,0.988105030697866,0.991593692313266)))
REPRESENTATION_ITEM('')
SURFACE()
);
#2991=(
BOUNDED_SURFACE()
B_SPLINE_SURFACE(1,2,((#145020,#145021,#145022),(#145023,#145024,#145025)),
 .UNSPECIFIED.,.F.,.F.,.F.)
B_SPLINE_SURFACE_WITH_KNOTS((2,2),(3,3),(0.,0.289807040991558),(0.176967058622921,
0.194235682574592),.UNSPECIFIED.)
GEOMETRIC_REPRESENTATION_ITEM()
RATIONAL_B_SPLINE_SURFACE(((0.98748925405691,0.987216959588932,0.989875504592249),
(0.98748925405691,0.987216959588931,0.989875504592248)))
REPRESENTATION_ITEM('')
SURFACE()
);
#2992=(
BOUNDED_SURFACE()
B_SPLINE_SURFACE(1,2,((#145033,#145034,#145035),(#145036,#145037,#145038)),
 .UNSPECIFIED.,.F.,.F.,.F.)
B_SPLINE_SURFACE_WITH_KNOTS((2,2),(3,3),(0.,0.289681084359916),(0.538896351358319,
0.556212823028865),.UNSPECIFIED.)
GEOMETRIC_REPRESENTATION_ITEM()
RATIONAL_B_SPLINE_SURFACE(((0.987563472532048,0.988105030697866,0.991593692313267),
(0.987563472532048,0.988105030697866,0.991593692313267)))
REPRESENTATION_ITEM('')
SURFACE()
);
#2993=(
BOUNDED_SURFACE()
B_SPLINE_SURFACE(1,2,((#145040,#145041,#145042),(#145043,#145044,#145045)),
 .UNSPECIFIED.,.F.,.F.,.F.)
B_SPLINE_SURFACE_WITH_KNOTS((2,2),(3,3),(0.,0.289807040991561),(0.176967058622921,
0.194235682574592),.UNSPECIFIED.)
GEOMETRIC_REPRESENTATION_ITEM()
RATIONAL_B_SPLINE_SURFACE(((0.98748925405691,0.987216959588931,0.989875504592248),
(0.98748925405691,0.987216959588931,0.989875504592248)))
REPRESENTATION_ITEM('')
SURFACE()
);
#2994=(
BOUNDED_SURFACE()
B_SPLINE_SURFACE(1,2,((#145062,#145063,#145064),(#145065,#145066,#145067)),
 .UNSPECIFIED.,.F.,.F.,.F.)
B_SPLINE_SURFACE_WITH_KNOTS((2,2),(3,3),(0.,0.289681084359916),(0.538896351358319,
0.556212823028865),.UNSPECIFIED.)
GEOMETRIC_REPRESENTATION_ITEM()
RATIONAL_B_SPLINE_SURFACE(((0.987563472532048,0.988105030697866,0.991593692313267),
(0.987563472532048,0.988105030697866,0.991593692313267)))
REPRESENTATION_ITEM('')
SURFACE()
);
#2995=(
BOUNDED_SURFACE()
B_SPLINE_SURFACE(1,2,((#145069,#145070,#145071),(#145072,#145073,#145074)),
 .UNSPECIFIED.,.F.,.F.,.F.)
B_SPLINE_SURFACE_WITH_KNOTS((2,2),(3,3),(0.,0.289807040991563),(0.176967058622921,
0.194235682574592),.UNSPECIFIED.)
GEOMETRIC_REPRESENTATION_ITEM()
RATIONAL_B_SPLINE_SURFACE(((0.98748925405691,0.987216959588931,0.989875504592249),
(0.98748925405691,0.987216959588931,0.989875504592249)))
REPRESENTATION_ITEM('')
SURFACE()
);
#2996=(
BOUNDED_SURFACE()
B_SPLINE_SURFACE(1,2,((#145091,#145092,#145093),(#145094,#145095,#145096)),
 .UNSPECIFIED.,.F.,.F.,.F.)
B_SPLINE_SURFACE_WITH_KNOTS((2,2),(3,3),(0.,0.289681084359914),(0.538896351358319,
0.556212823028865),.UNSPECIFIED.)
GEOMETRIC_REPRESENTATION_ITEM()
RATIONAL_B_SPLINE_SURFACE(((0.987563472532048,0.988105030697866,0.991593692313267),
(0.987563472532048,0.988105030697866,0.991593692313267)))
REPRESENTATION_ITEM('')
SURFACE()
);
#2997=(
BOUNDED_SURFACE()
B_SPLINE_SURFACE(1,2,((#145098,#145099,#145100),(#145101,#145102,#145103)),
 .UNSPECIFIED.,.F.,.F.,.F.)
B_SPLINE_SURFACE_WITH_KNOTS((2,2),(3,3),(0.,0.289807040991564),(0.176967058622921,
0.194235682574592),.UNSPECIFIED.)
GEOMETRIC_REPRESENTATION_ITEM()
RATIONAL_B_SPLINE_SURFACE(((0.98748925405691,0.987216959588931,0.989875504592249),
(0.98748925405691,0.987216959588931,0.989875504592249)))
REPRESENTATION_ITEM('')
SURFACE()
);
#2998=(
BOUNDED_SURFACE()
B_SPLINE_SURFACE(1,2,((#145120,#145121,#145122),(#145123,#145124,#145125)),
 .UNSPECIFIED.,.F.,.F.,.F.)
B_SPLINE_SURFACE_WITH_KNOTS((2,2),(3,3),(0.,0.289681084359916),(0.538896351358319,
0.556212823028865),.UNSPECIFIED.)
GEOMETRIC_REPRESENTATION_ITEM()
RATIONAL_B_SPLINE_SURFACE(((0.987563472532048,0.988105030697866,0.991593692313267),
(0.987563472532048,0.988105030697866,0.991593692313267)))
REPRESENTATION_ITEM('')
SURFACE()
);
#2999=(
BOUNDED_SURFACE()
B_SPLINE_SURFACE(1,2,((#145127,#145128,#145129),(#145130,#145131,#145132)),
 .UNSPECIFIED.,.F.,.F.,.F.)
B_SPLINE_SURFACE_WITH_KNOTS((2,2),(3,3),(0.,0.289807040991562),(0.176967058622921,
0.194235682574592),.UNSPECIFIED.)
GEOMETRIC_REPRESENTATION_ITEM()
RATIONAL_B_SPLINE_SURFACE(((0.98748925405691,0.987216959588931,0.989875504592249),
(0.98748925405691,0.987216959588931,0.989875504592249)))
REPRESENTATION_ITEM('')
SURFACE()
);
#3000=(
BOUNDED_SURFACE()
B_SPLINE_SURFACE(1,2,((#145149,#145150,#145151),(#145152,#145153,#145154)),
 .UNSPECIFIED.,.F.,.F.,.F.)
B_SPLINE_SURFACE_WITH_KNOTS((2,2),(3,3),(0.,0.289681084359921),(0.538896351358319,
0.556212823028865),.UNSPECIFIED.)
GEOMETRIC_REPRESENTATION_ITEM()
RATIONAL_B_SPLINE_SURFACE(((0.987563472532048,0.988105030697866,0.991593692313267),
(0.987563472532048,0.988105030697866,0.991593692313267)))
REPRESENTATION_ITEM('')
SURFACE()
);
#3001=(
BOUNDED_SURFACE()
B_SPLINE_SURFACE(1,2,((#145156,#145157,#145158),(#145159,#145160,#145161)),
 .UNSPECIFIED.,.F.,.F.,.F.)
B_SPLINE_SURFACE_WITH_KNOTS((2,2),(3,3),(0.,0.289807040991563),(0.176967058622921,
0.194235682574592),.UNSPECIFIED.)
GEOMETRIC_REPRESENTATION_ITEM()
RATIONAL_B_SPLINE_SURFACE(((0.98748925405691,0.987216959588931,0.989875504592249),
(0.98748925405691,0.987216959588931,0.989875504592249)))
REPRESENTATION_ITEM('')
SURFACE()
);
#3002=(
BOUNDED_SURFACE()
B_SPLINE_SURFACE(1,2,((#145178,#145179,#145180),(#145181,#145182,#145183)),
 .UNSPECIFIED.,.F.,.F.,.F.)
B_SPLINE_SURFACE_WITH_KNOTS((2,2),(3,3),(0.,0.289681084359926),(0.538896351358319,
0.556212823028862),.UNSPECIFIED.)
GEOMETRIC_REPRESENTATION_ITEM()
RATIONAL_B_SPLINE_SURFACE(((0.987563472532048,0.988105030697866,0.991593692313266),
(0.987563472532048,0.988105030697866,0.991593692313266)))
REPRESENTATION_ITEM('')
SURFACE()
);
#3003=(
BOUNDED_SURFACE()
B_SPLINE_SURFACE(1,2,((#145185,#145186,#145187),(#145188,#145189,#145190)),
 .UNSPECIFIED.,.F.,.F.,.F.)
B_SPLINE_SURFACE_WITH_KNOTS((2,2),(3,3),(0.,0.289807040991567),(0.176967058622921,
0.194235682574592),.UNSPECIFIED.)
GEOMETRIC_REPRESENTATION_ITEM()
RATIONAL_B_SPLINE_SURFACE(((0.98748925405691,0.987216959588931,0.989875504592249),
(0.98748925405691,0.987216959588931,0.989875504592249)))
REPRESENTATION_ITEM('')
SURFACE()
);
#3004=(
BOUNDED_SURFACE()
B_SPLINE_SURFACE(1,2,((#145207,#145208,#145209),(#145210,#145211,#145212)),
 .UNSPECIFIED.,.F.,.F.,.F.)
B_SPLINE_SURFACE_WITH_KNOTS((2,2),(3,3),(0.,0.289681084359921),(0.538896351358319,
0.556212823028862),.UNSPECIFIED.)
GEOMETRIC_REPRESENTATION_ITEM()
RATIONAL_B_SPLINE_SURFACE(((0.987563472532048,0.988105030697866,0.991593692313266),
(0.987563472532048,0.988105030697866,0.991593692313266)))
REPRESENTATION_ITEM('')
SURFACE()
);
#3005=(
BOUNDED_SURFACE()
B_SPLINE_SURFACE(1,2,((#145214,#145215,#145216),(#145217,#145218,#145219)),
 .UNSPECIFIED.,.F.,.F.,.F.)
B_SPLINE_SURFACE_WITH_KNOTS((2,2),(3,3),(0.,0.289807040991564),(0.176967058622921,
0.194235682574592),.UNSPECIFIED.)
GEOMETRIC_REPRESENTATION_ITEM()
RATIONAL_B_SPLINE_SURFACE(((0.98748925405691,0.987216959588932,0.989875504592249),
(0.98748925405691,0.987216959588932,0.989875504592249)))
REPRESENTATION_ITEM('')
SURFACE()
);
#3006=(
BOUNDED_SURFACE()
B_SPLINE_SURFACE(1,2,((#145236,#145237,#145238),(#145239,#145240,#145241)),
 .UNSPECIFIED.,.F.,.F.,.F.)
B_SPLINE_SURFACE_WITH_KNOTS((2,2),(3,3),(0.,0.28968108435992),(0.538896351358319,
0.556212823028865),.UNSPECIFIED.)
GEOMETRIC_REPRESENTATION_ITEM()
RATIONAL_B_SPLINE_SURFACE(((0.987563472532048,0.988105030697866,0.991593692313267),
(0.987563472532048,0.988105030697866,0.991593692313267)))
REPRESENTATION_ITEM('')
SURFACE()
);
#3007=(
BOUNDED_SURFACE()
B_SPLINE_SURFACE(1,2,((#145243,#145244,#145245),(#145246,#145247,#145248)),
 .UNSPECIFIED.,.F.,.F.,.F.)
B_SPLINE_SURFACE_WITH_KNOTS((2,2),(3,3),(0.,0.289807040991561),(0.176967058622921,
0.194235682574592),.UNSPECIFIED.)
GEOMETRIC_REPRESENTATION_ITEM()
RATIONAL_B_SPLINE_SURFACE(((0.98748925405691,0.987216959588932,0.989875504592249),
(0.98748925405691,0.987216959588932,0.989875504592249)))
REPRESENTATION_ITEM('')
SURFACE()
);
#3008=(
BOUNDED_SURFACE()
B_SPLINE_SURFACE(1,2,((#145265,#145266,#145267),(#145268,#145269,#145270)),
 .UNSPECIFIED.,.F.,.F.,.F.)
B_SPLINE_SURFACE_WITH_KNOTS((2,2),(3,3),(0.,0.289681084359919),(0.538896351358319,
0.556212823028862),.UNSPECIFIED.)
GEOMETRIC_REPRESENTATION_ITEM()
RATIONAL_B_SPLINE_SURFACE(((0.987563472532048,0.988105030697866,0.991593692313266),
(0.987563472532048,0.988105030697866,0.991593692313266)))
REPRESENTATION_ITEM('')
SURFACE()
);
#3009=(
BOUNDED_SURFACE()
B_SPLINE_SURFACE(1,2,((#145272,#145273,#145274),(#145275,#145276,#145277)),
 .UNSPECIFIED.,.F.,.F.,.F.)
B_SPLINE_SURFACE_WITH_KNOTS((2,2),(3,3),(0.,0.289807040991558),(0.176967058622921,
0.194235682574592),.UNSPECIFIED.)
GEOMETRIC_REPRESENTATION_ITEM()
RATIONAL_B_SPLINE_SURFACE(((0.98748925405691,0.987216959588931,0.989875504592249),
(0.98748925405691,0.987216959588931,0.989875504592249)))
REPRESENTATION_ITEM('')
SURFACE()
);
#3010=(
BOUNDED_SURFACE()
B_SPLINE_SURFACE(1,2,((#145294,#145295,#145296),(#145297,#145298,#145299)),
 .UNSPECIFIED.,.F.,.F.,.F.)
B_SPLINE_SURFACE_WITH_KNOTS((2,2),(3,3),(0.,0.289681084359921),(0.538896351358319,
0.556212823028865),.UNSPECIFIED.)
GEOMETRIC_REPRESENTATION_ITEM()
RATIONAL_B_SPLINE_SURFACE(((0.987563472532048,0.988105030697866,0.991593692313267),
(0.987563472532048,0.988105030697866,0.991593692313267)))
REPRESENTATION_ITEM('')
SURFACE()
);
#3011=(
BOUNDED_SURFACE()
B_SPLINE_SURFACE(1,2,((#145301,#145302,#145303),(#145304,#145305,#145306)),
 .UNSPECIFIED.,.F.,.F.,.F.)
B_SPLINE_SURFACE_WITH_KNOTS((2,2),(3,3),(0.,0.289807040991562),(0.176967058622921,
0.194235682574592),.UNSPECIFIED.)
GEOMETRIC_REPRESENTATION_ITEM()
RATIONAL_B_SPLINE_SURFACE(((0.98748925405691,0.987216959588931,0.989875504592249),
(0.98748925405691,0.987216959588931,0.989875504592249)))
REPRESENTATION_ITEM('')
SURFACE()
);
#3012=(
BOUNDED_SURFACE()
B_SPLINE_SURFACE(1,2,((#145323,#145324,#145325),(#145326,#145327,#145328)),
 .UNSPECIFIED.,.F.,.F.,.F.)
B_SPLINE_SURFACE_WITH_KNOTS((2,2),(3,3),(0.,0.28968108435992),(0.538896351358319,
0.556212823028865),.UNSPECIFIED.)
GEOMETRIC_REPRESENTATION_ITEM()
RATIONAL_B_SPLINE_SURFACE(((0.987563472532048,0.988105030697866,0.991593692313267),
(0.987563472532048,0.988105030697866,0.991593692313267)))
REPRESENTATION_ITEM('')
SURFACE()
);
#3013=(
BOUNDED_SURFACE()
B_SPLINE_SURFACE(1,2,((#145330,#145331,#145332),(#145333,#145334,#145335)),
 .UNSPECIFIED.,.F.,.F.,.F.)
B_SPLINE_SURFACE_WITH_KNOTS((2,2),(3,3),(0.,0.289807040991561),(0.176967058622921,
0.194235682574592),.UNSPECIFIED.)
GEOMETRIC_REPRESENTATION_ITEM()
RATIONAL_B_SPLINE_SURFACE(((0.98748925405691,0.987216959588931,0.989875504592249),
(0.98748925405691,0.987216959588931,0.989875504592249)))
REPRESENTATION_ITEM('')
SURFACE()
);
#3014=(
BOUNDED_SURFACE()
B_SPLINE_SURFACE(1,2,((#145352,#145353,#145354),(#145355,#145356,#145357)),
 .UNSPECIFIED.,.F.,.F.,.F.)
B_SPLINE_SURFACE_WITH_KNOTS((2,2),(3,3),(0.,0.289681084359922),(0.538896351358319,
0.556212823028865),.UNSPECIFIED.)
GEOMETRIC_REPRESENTATION_ITEM()
RATIONAL_B_SPLINE_SURFACE(((0.987563472532048,0.988105030697866,0.991593692313267),
(0.987563472532048,0.988105030697866,0.991593692313267)))
REPRESENTATION_ITEM('')
SURFACE()
);
#3015=(
BOUNDED_SURFACE()
B_SPLINE_SURFACE(1,2,((#145359,#145360,#145361),(#145362,#145363,#145364)),
 .UNSPECIFIED.,.F.,.F.,.F.)
B_SPLINE_SURFACE_WITH_KNOTS((2,2),(3,3),(0.,0.289807040991556),(0.176967058622921,
0.194235682574592),.UNSPECIFIED.)
GEOMETRIC_REPRESENTATION_ITEM()
RATIONAL_B_SPLINE_SURFACE(((0.98748925405691,0.987216959588931,0.989875504592249),
(0.98748925405691,0.987216959588931,0.989875504592249)))
REPRESENTATION_ITEM('')
SURFACE()
);
#3016=(
BOUNDED_SURFACE()
B_SPLINE_SURFACE(1,2,((#145375,#145376,#145377),(#145378,#145379,#145380)),
 .UNSPECIFIED.,.F.,.F.,.F.)
B_SPLINE_SURFACE_WITH_KNOTS((2,2),(3,3),(0.,0.289681084359922),(0.538896351358319,
0.556212823028862),.UNSPECIFIED.)
GEOMETRIC_REPRESENTATION_ITEM()
RATIONAL_B_SPLINE_SURFACE(((0.987563472532048,0.988105030697866,0.991593692313266),
(0.987563472532048,0.988105030697866,0.991593692313266)))
REPRESENTATION_ITEM('')
SURFACE()
);
#3017=(
BOUNDED_SURFACE()
B_SPLINE_SURFACE(1,2,((#145388,#145389,#145390),(#145391,#145392,#145393)),
 .UNSPECIFIED.,.F.,.F.,.F.)
B_SPLINE_SURFACE_WITH_KNOTS((2,2),(3,3),(0.,0.289807040991561),(0.176967058622921,
0.194235682574592),.UNSPECIFIED.)
GEOMETRIC_REPRESENTATION_ITEM()
RATIONAL_B_SPLINE_SURFACE(((0.98748925405691,0.987216959588932,0.989875504592249),
(0.98748925405691,0.987216959588932,0.989875504592249)))
REPRESENTATION_ITEM('')
SURFACE()
);
#3018=(
BOUNDED_SURFACE()
B_SPLINE_SURFACE(1,2,((#145410,#145411,#145412),(#145413,#145414,#145415)),
 .UNSPECIFIED.,.F.,.F.,.F.)
B_SPLINE_SURFACE_WITH_KNOTS((2,2),(3,3),(0.,0.289681084359924),(0.538896351358319,
0.556212823028861),.UNSPECIFIED.)
GEOMETRIC_REPRESENTATION_ITEM()
RATIONAL_B_SPLINE_SURFACE(((0.987563472532048,0.988105030697866,0.991593692313265),
(0.987563472532048,0.988105030697866,0.991593692313265)))
REPRESENTATION_ITEM('')
SURFACE()
);
#3019=(
BOUNDED_SURFACE()
B_SPLINE_SURFACE(1,2,((#145417,#145418,#145419),(#145420,#145421,#145422)),
 .UNSPECIFIED.,.F.,.F.,.F.)
B_SPLINE_SURFACE_WITH_KNOTS((2,2),(3,3),(0.,0.2898070409917),(0.176967058622922,
0.194235682574593),.UNSPECIFIED.)
GEOMETRIC_REPRESENTATION_ITEM()
RATIONAL_B_SPLINE_SURFACE(((0.98748925405691,0.987216959588932,0.989875504592249),
(0.98748925405691,0.987216959588932,0.989875504592249)))
REPRESENTATION_ITEM('')
SURFACE()
);
#3020=(
BOUNDED_SURFACE()
B_SPLINE_SURFACE(1,2,((#145439,#145440,#145441),(#145442,#145443,#145444)),
 .UNSPECIFIED.,.F.,.F.,.F.)
B_SPLINE_SURFACE_WITH_KNOTS((2,2),(3,3),(0.,0.289681084359922),(0.538896351358318,
0.556212823028861),.UNSPECIFIED.)
GEOMETRIC_REPRESENTATION_ITEM()
RATIONAL_B_SPLINE_SURFACE(((0.987563472532048,0.988105030697865,0.991593692313265),
(0.987563472532048,0.988105030697865,0.991593692313265)))
REPRESENTATION_ITEM('')
SURFACE()
);
#3021=(
BOUNDED_SURFACE()
B_SPLINE_SURFACE(1,2,((#145446,#145447,#145448),(#145449,#145450,#145451)),
 .UNSPECIFIED.,.F.,.F.,.F.)
B_SPLINE_SURFACE_WITH_KNOTS((2,2),(3,3),(0.,0.289807040991948),(0.176967058622922,
0.194235682574593),.UNSPECIFIED.)
GEOMETRIC_REPRESENTATION_ITEM()
RATIONAL_B_SPLINE_SURFACE(((0.98748925405691,0.987216959588932,0.989875504592249),
(0.98748925405691,0.987216959588932,0.989875504592249)))
REPRESENTATION_ITEM('')
SURFACE()
);
#3022=(
BOUNDED_SURFACE()
B_SPLINE_SURFACE(1,2,((#145468,#145469,#145470),(#145471,#145472,#145473)),
 .UNSPECIFIED.,.F.,.F.,.F.)
B_SPLINE_SURFACE_WITH_KNOTS((2,2),(3,3),(0.,0.289681084359918),(0.538896351358318,
0.556212823028864),.UNSPECIFIED.)
GEOMETRIC_REPRESENTATION_ITEM()
RATIONAL_B_SPLINE_SURFACE(((0.987563472532048,0.988105030697865,0.991593692313266),
(0.987563472532048,0.988105030697865,0.991593692313266)))
REPRESENTATION_ITEM('')
SURFACE()
);
#3023=(
BOUNDED_SURFACE()
B_SPLINE_SURFACE(1,2,((#145475,#145476,#145477),(#145478,#145479,#145480)),
 .UNSPECIFIED.,.F.,.F.,.F.)
B_SPLINE_SURFACE_WITH_KNOTS((2,2),(3,3),(0.,0.289807040993356),(0.176967058622922,
0.194235682574593),.UNSPECIFIED.)
GEOMETRIC_REPRESENTATION_ITEM()
RATIONAL_B_SPLINE_SURFACE(((0.98748925405691,0.987216959588932,0.989875504592249),
(0.98748925405691,0.987216959588932,0.989875504592249)))
REPRESENTATION_ITEM('')
SURFACE()
);
#3024=(
BOUNDED_SURFACE()
B_SPLINE_SURFACE(1,2,((#145497,#145498,#145499),(#145500,#145501,#145502)),
 .UNSPECIFIED.,.F.,.F.,.F.)
B_SPLINE_SURFACE_WITH_KNOTS((2,2),(3,3),(0.,0.289681084360124),(0.538896351358318,
0.556212823028861),.UNSPECIFIED.)
GEOMETRIC_REPRESENTATION_ITEM()
RATIONAL_B_SPLINE_SURFACE(((0.987563472532048,0.988105030697865,0.991593692313265),
(0.987563472532048,0.988105030697865,0.991593692313265)))
REPRESENTATION_ITEM('')
SURFACE()
);
#3025=(
BOUNDED_SURFACE()
B_SPLINE_SURFACE(1,2,((#145504,#145505,#145506),(#145507,#145508,#145509)),
 .UNSPECIFIED.,.F.,.F.,.F.)
B_SPLINE_SURFACE_WITH_KNOTS((2,2),(3,3),(0.,0.289807040992024),(0.176967058622922,
0.194235682574593),.UNSPECIFIED.)
GEOMETRIC_REPRESENTATION_ITEM()
RATIONAL_B_SPLINE_SURFACE(((0.98748925405691,0.987216959588932,0.989875504592249),
(0.98748925405691,0.987216959588932,0.989875504592249)))
REPRESENTATION_ITEM('')
SURFACE()
);
#3026=(
BOUNDED_SURFACE()
B_SPLINE_SURFACE(1,2,((#145526,#145527,#145528),(#145529,#145530,#145531)),
 .UNSPECIFIED.,.F.,.F.,.F.)
B_SPLINE_SURFACE_WITH_KNOTS((2,2),(3,3),(0.,0.289681084359929),(0.538896351358318,
0.556212823028861),.UNSPECIFIED.)
GEOMETRIC_REPRESENTATION_ITEM()
RATIONAL_B_SPLINE_SURFACE(((0.987563472532048,0.988105030697865,0.991593692313265),
(0.987563472532048,0.988105030697865,0.991593692313265)))
REPRESENTATION_ITEM('')
SURFACE()
);
#3027=(
BOUNDED_SURFACE()
B_SPLINE_SURFACE(1,2,((#145533,#145534,#145535),(#145536,#145537,#145538)),
 .UNSPECIFIED.,.F.,.F.,.F.)
B_SPLINE_SURFACE_WITH_KNOTS((2,2),(3,3),(0.,0.289807040991646),(0.176967058622922,
0.194235682574593),.UNSPECIFIED.)
GEOMETRIC_REPRESENTATION_ITEM()
RATIONAL_B_SPLINE_SURFACE(((0.98748925405691,0.987216959588932,0.989875504592249),
(0.98748925405691,0.987216959588932,0.989875504592249)))
REPRESENTATION_ITEM('')
SURFACE()
);
#3028=(
BOUNDED_SURFACE()
B_SPLINE_SURFACE(1,2,((#145555,#145556,#145557),(#145558,#145559,#145560)),
 .UNSPECIFIED.,.F.,.F.,.F.)
B_SPLINE_SURFACE_WITH_KNOTS((2,2),(3,3),(0.,0.289681084359921),(0.538896351358318,
0.556212823028864),.UNSPECIFIED.)
GEOMETRIC_REPRESENTATION_ITEM()
RATIONAL_B_SPLINE_SURFACE(((0.987563472532048,0.988105030697865,0.991593692313266),
(0.987563472532048,0.988105030697865,0.991593692313266)))
REPRESENTATION_ITEM('')
SURFACE()
);
#3029=(
BOUNDED_SURFACE()
B_SPLINE_SURFACE(1,2,((#145562,#145563,#145564),(#145565,#145566,#145567)),
 .UNSPECIFIED.,.F.,.F.,.F.)
B_SPLINE_SURFACE_WITH_KNOTS((2,2),(3,3),(0.,0.289807040991639),(0.176967058622922,
0.194235682574593),.UNSPECIFIED.)
GEOMETRIC_REPRESENTATION_ITEM()
RATIONAL_B_SPLINE_SURFACE(((0.98748925405691,0.987216959588932,0.989875504592249),
(0.98748925405691,0.987216959588932,0.989875504592249)))
REPRESENTATION_ITEM('')
SURFACE()
);
#3030=(
BOUNDED_SURFACE()
B_SPLINE_SURFACE(1,2,((#145584,#145585,#145586),(#145587,#145588,#145589)),
 .UNSPECIFIED.,.F.,.F.,.F.)
B_SPLINE_SURFACE_WITH_KNOTS((2,2),(3,3),(0.,0.289681084359917),(0.538896351358318,
0.556212823028861),.UNSPECIFIED.)
GEOMETRIC_REPRESENTATION_ITEM()
RATIONAL_B_SPLINE_SURFACE(((0.987563472532048,0.988105030697865,0.991593692313265),
(0.987563472532048,0.988105030697865,0.991593692313265)))
REPRESENTATION_ITEM('')
SURFACE()
);
#3031=(
BOUNDED_SURFACE()
B_SPLINE_SURFACE(1,2,((#145591,#145592,#145593),(#145594,#145595,#145596)),
 .UNSPECIFIED.,.F.,.F.,.F.)
B_SPLINE_SURFACE_WITH_KNOTS((2,2),(3,3),(0.,0.28980704099163),(0.176967058622922,
0.194235682574593),.UNSPECIFIED.)
GEOMETRIC_REPRESENTATION_ITEM()
RATIONAL_B_SPLINE_SURFACE(((0.98748925405691,0.987216959588932,0.989875504592249),
(0.98748925405691,0.987216959588932,0.989875504592249)))
REPRESENTATION_ITEM('')
SURFACE()
);
#3032=(
BOUNDED_SURFACE()
B_SPLINE_SURFACE(1,2,((#145613,#145614,#145615),(#145616,#145617,#145618)),
 .UNSPECIFIED.,.F.,.F.,.F.)
B_SPLINE_SURFACE_WITH_KNOTS((2,2),(3,3),(0.,0.28968108435992),(0.538896351358318,
0.556212823028861),.UNSPECIFIED.)
GEOMETRIC_REPRESENTATION_ITEM()
RATIONAL_B_SPLINE_SURFACE(((0.987563472532048,0.988105030697865,0.991593692313265),
(0.987563472532048,0.988105030697865,0.991593692313265)))
REPRESENTATION_ITEM('')
SURFACE()
);
#3033=(
BOUNDED_SURFACE()
B_SPLINE_SURFACE(1,2,((#145620,#145621,#145622),(#145623,#145624,#145625)),
 .UNSPECIFIED.,.F.,.F.,.F.)
B_SPLINE_SURFACE_WITH_KNOTS((2,2),(3,3),(0.,0.28980704099191),(0.176967058622922,
0.194235682574593),.UNSPECIFIED.)
GEOMETRIC_REPRESENTATION_ITEM()
RATIONAL_B_SPLINE_SURFACE(((0.98748925405691,0.987216959588932,0.989875504592249),
(0.98748925405691,0.987216959588932,0.989875504592249)))
REPRESENTATION_ITEM('')
SURFACE()
);
#3034=(
BOUNDED_SURFACE()
B_SPLINE_SURFACE(1,2,((#145642,#145643,#145644),(#145645,#145646,#145647)),
 .UNSPECIFIED.,.F.,.F.,.F.)
B_SPLINE_SURFACE_WITH_KNOTS((2,2),(3,3),(0.,0.289681084359926),(0.538896351358318,
0.556212823028864),.UNSPECIFIED.)
GEOMETRIC_REPRESENTATION_ITEM()
RATIONAL_B_SPLINE_SURFACE(((0.987563472532048,0.988105030697865,0.991593692313266),
(0.987563472532048,0.988105030697865,0.991593692313266)))
REPRESENTATION_ITEM('')
SURFACE()
);
#3035=(
BOUNDED_SURFACE()
B_SPLINE_SURFACE(1,2,((#145655,#145656,#145657),(#145658,#145659,#145660)),
 .UNSPECIFIED.,.F.,.F.,.F.)
B_SPLINE_SURFACE_WITH_KNOTS((2,2),(3,3),(0.,0.289807040991561),(0.176967058622922,
0.194235682574593),.UNSPECIFIED.)
GEOMETRIC_REPRESENTATION_ITEM()
RATIONAL_B_SPLINE_SURFACE(((0.98748925405691,0.987216959588932,0.989875504592249),
(0.98748925405691,0.987216959588932,0.989875504592249)))
REPRESENTATION_ITEM('')
SURFACE()
);
#3036=(
BOUNDED_SURFACE()
B_SPLINE_SURFACE(1,2,((#145662,#145663,#145664),(#145665,#145666,#145667)),
 .UNSPECIFIED.,.F.,.F.,.F.)
B_SPLINE_SURFACE_WITH_KNOTS((2,2),(3,3),(0.710192959007979,1.),(0.125170525609408,
0.142682999576236),.UNSPECIFIED.)
GEOMETRIC_REPRESENTATION_ITEM()
RATIONAL_B_SPLINE_SURFACE(((0.990658108926709,0.993760979299921,0.999878046252917),
(0.990658108926709,0.993760979299921,0.999878046252917)))
REPRESENTATION_ITEM('')
SURFACE()
);
#3037=(
BOUNDED_SURFACE()
B_SPLINE_SURFACE(1,2,((#145678,#145679,#145680,#145681,#145682),(#145683,
#145684,#145685,#145686,#145687)),.UNSPECIFIED.,.F.,.F.,.F.)
B_SPLINE_SURFACE_WITH_KNOTS((2,2),(3,2,3),(0.709728555967135,1.),(0.590808523385635,
0.607982157956011,0.608572517827272),.UNSPECIFIED.)
GEOMETRIC_REPRESENTATION_ITEM()
RATIONAL_B_SPLINE_SURFACE(((0.990086238235256,0.987329216372183,0.987470879370256,
0.987470879370256,0.987470879370256),(0.990086238235256,0.987329216372183,
0.987470879370256,0.987470879370256,0.987470879370256)))
REPRESENTATION_ITEM('')
SURFACE()
);
#3038=(
BOUNDED_SURFACE()
B_SPLINE_SURFACE(1,2,((#145698,#145699,#145700),(#145701,#145702,#145703)),
 .UNSPECIFIED.,.F.,.F.,.F.)
B_SPLINE_SURFACE_WITH_KNOTS((2,2),(3,3),(0.710192959007996,1.),(0.125170525609408,
0.142682999576236),.UNSPECIFIED.)
GEOMETRIC_REPRESENTATION_ITEM()
RATIONAL_B_SPLINE_SURFACE(((0.990658108926709,0.993760979299921,0.999878046252917),
(0.990658108926709,0.993760979299921,0.999878046252917)))
REPRESENTATION_ITEM('')
SURFACE()
);
#3039=(
BOUNDED_SURFACE()
B_SPLINE_SURFACE(1,2,((#145711,#145712,#145713,#145714,#145715),(#145716,
#145717,#145718,#145719,#145720)),.UNSPECIFIED.,.F.,.F.,.F.)
B_SPLINE_SURFACE_WITH_KNOTS((2,2),(3,2,3),(0.709728555997542,1.),(0.590808523385635,
0.607982157956011,0.608572517839914),.UNSPECIFIED.)
GEOMETRIC_REPRESENTATION_ITEM()
RATIONAL_B_SPLINE_SURFACE(((0.990086238235256,0.987329216372183,0.987470879370256,
0.987470879370256,0.987470879370256),(0.990086238235256,0.987329216372183,
0.987470879370256,0.987470879370256,0.987470879370256)))
REPRESENTATION_ITEM('')
SURFACE()
);
#3040=(
BOUNDED_SURFACE()
B_SPLINE_SURFACE(1,2,((#145731,#145732,#145733),(#145734,#145735,#145736)),
 .UNSPECIFIED.,.F.,.F.,.F.)
B_SPLINE_SURFACE_WITH_KNOTS((2,2),(3,3),(0.710192959008342,1.),(0.125170525609408,
0.142682999576236),.UNSPECIFIED.)
GEOMETRIC_REPRESENTATION_ITEM()
RATIONAL_B_SPLINE_SURFACE(((0.990658108926709,0.993760979299921,0.999878046252917),
(0.990658108926709,0.993760979299921,0.999878046252917)))
REPRESENTATION_ITEM('')
SURFACE()
);
#3041=(
BOUNDED_SURFACE()
B_SPLINE_SURFACE(1,2,((#145744,#145745,#145746,#145747,#145748),(#145749,
#145750,#145751,#145752,#145753)),.UNSPECIFIED.,.F.,.F.,.F.)
B_SPLINE_SURFACE_WITH_KNOTS((2,2),(3,2,3),(0.709728555976075,1.),(0.590808523385635,
0.607982157956012,0.608572517860657),.UNSPECIFIED.)
GEOMETRIC_REPRESENTATION_ITEM()
RATIONAL_B_SPLINE_SURFACE(((0.990086238235256,0.987329216372183,0.987470879370256,
0.987470879370256,0.987470879370256),(0.990086238235256,0.987329216372183,
0.987470879370256,0.987470879370256,0.987470879370256)))
REPRESENTATION_ITEM('')
SURFACE()
);
#3042=(
BOUNDED_SURFACE()
B_SPLINE_SURFACE(1,2,((#145764,#145765,#145766),(#145767,#145768,#145769)),
 .UNSPECIFIED.,.F.,.F.,.F.)
B_SPLINE_SURFACE_WITH_KNOTS((2,2),(3,3),(0.710192959008336,1.),(0.125170525609409,
0.142682999576236),.UNSPECIFIED.)
GEOMETRIC_REPRESENTATION_ITEM()
RATIONAL_B_SPLINE_SURFACE(((0.990658108926709,0.993760979299921,0.999878046252917),
(0.990658108926709,0.993760979299921,0.999878046252917)))
REPRESENTATION_ITEM('')
SURFACE()
);
#3043=(
BOUNDED_SURFACE()
B_SPLINE_SURFACE(1,2,((#145777,#145778,#145779,#145780,#145781),(#145782,
#145783,#145784,#145785,#145786)),.UNSPECIFIED.,.F.,.F.,.F.)
B_SPLINE_SURFACE_WITH_KNOTS((2,2),(3,2,3),(0.709728555936133,1.),(0.590808523385635,
0.607982157956012,0.608572517857657),.UNSPECIFIED.)
GEOMETRIC_REPRESENTATION_ITEM()
RATIONAL_B_SPLINE_SURFACE(((0.990086238235256,0.987329216372183,0.987470879370255,
0.987470879370255,0.987470879370255),(0.990086238235256,0.987329216372183,
0.987470879370255,0.987470879370255,0.987470879370255)))
REPRESENTATION_ITEM('')
SURFACE()
);
#3044=(
BOUNDED_SURFACE()
B_SPLINE_SURFACE(1,2,((#145797,#145798,#145799),(#145800,#145801,#145802)),
 .UNSPECIFIED.,.F.,.F.,.F.)
B_SPLINE_SURFACE_WITH_KNOTS((2,2),(3,3),(0.71019295900738,1.),(0.125170525609408,
0.142682999576236),.UNSPECIFIED.)
GEOMETRIC_REPRESENTATION_ITEM()
RATIONAL_B_SPLINE_SURFACE(((0.990658108926709,0.993760979299921,0.999878046252917),
(0.990658108926709,0.993760979299921,0.999878046252917)))
REPRESENTATION_ITEM('')
SURFACE()
);
#3045=(
BOUNDED_SURFACE()
B_SPLINE_SURFACE(1,2,((#145810,#145811,#145812,#145813,#145814),(#145815,
#145816,#145817,#145818,#145819)),.UNSPECIFIED.,.F.,.F.,.F.)
B_SPLINE_SURFACE_WITH_KNOTS((2,2),(3,2,3),(0.709728555933635,1.),(0.590808523385635,
0.607982157956011,0.608572517860158),.UNSPECIFIED.)
GEOMETRIC_REPRESENTATION_ITEM()
RATIONAL_B_SPLINE_SURFACE(((0.990086238235256,0.987329216372183,0.987470879370256,
0.987470879370256,0.987470879370256),(0.990086238235256,0.987329216372183,
0.987470879370256,0.987470879370256,0.987470879370256)))
REPRESENTATION_ITEM('')
SURFACE()
);
#3046=(
BOUNDED_SURFACE()
B_SPLINE_SURFACE(1,2,((#145830,#145831,#145832),(#145833,#145834,#145835)),
 .UNSPECIFIED.,.F.,.F.,.F.)
B_SPLINE_SURFACE_WITH_KNOTS((2,2),(3,3),(0.710192959007375,1.),(0.125170525609408,
0.142682999576236),.UNSPECIFIED.)
GEOMETRIC_REPRESENTATION_ITEM()
RATIONAL_B_SPLINE_SURFACE(((0.990658108926709,0.993760979299921,0.999878046252917),
(0.990658108926709,0.993760979299921,0.999878046252917)))
REPRESENTATION_ITEM('')
SURFACE()
);
#3047=(
BOUNDED_SURFACE()
B_SPLINE_SURFACE(1,2,((#145843,#145844,#145845,#145846,#145847),(#145848,
#145849,#145850,#145851,#145852)),.UNSPECIFIED.,.F.,.F.,.F.)
B_SPLINE_SURFACE_WITH_KNOTS((2,2),(3,2,3),(0.709728555952784,1.),(0.590808523385635,
0.607982157956011,0.60857251784101),.UNSPECIFIED.)
GEOMETRIC_REPRESENTATION_ITEM()
RATIONAL_B_SPLINE_SURFACE(((0.990086238235256,0.987329216372183,0.987470879370255,
0.987470879370255,0.987470879370255),(0.990086238235256,0.987329216372183,
0.987470879370255,0.987470879370255,0.987470879370255)))
REPRESENTATION_ITEM('')
SURFACE()
);
#3048=(
BOUNDED_SURFACE()
B_SPLINE_SURFACE(1,2,((#145863,#145864,#145865),(#145866,#145867,#145868)),
 .UNSPECIFIED.,.F.,.F.,.F.)
B_SPLINE_SURFACE_WITH_KNOTS((2,2),(3,3),(0.71019295900738,1.),(0.125170525609408,
0.142682999576236),.UNSPECIFIED.)
GEOMETRIC_REPRESENTATION_ITEM()
RATIONAL_B_SPLINE_SURFACE(((0.990658108926709,0.993760979299922,0.999878046252917),
(0.990658108926709,0.993760979299922,0.999878046252917)))
REPRESENTATION_ITEM('')
SURFACE()
);
#3049=(
BOUNDED_SURFACE()
B_SPLINE_SURFACE(1,2,((#145876,#145877,#145878,#145879,#145880),(#145881,
#145882,#145883,#145884,#145885)),.UNSPECIFIED.,.F.,.F.,.F.)
B_SPLINE_SURFACE_WITH_KNOTS((2,2),(3,2,3),(0.709728555955733,1.),(0.590808523385635,
0.607982157956011,0.608572517837478),.UNSPECIFIED.)
GEOMETRIC_REPRESENTATION_ITEM()
RATIONAL_B_SPLINE_SURFACE(((0.990086238235256,0.987329216372183,0.987470879370255,
0.987470879370255,0.987470879370255),(0.990086238235256,0.987329216372183,
0.987470879370255,0.987470879370255,0.987470879370255)))
REPRESENTATION_ITEM('')
SURFACE()
);
#3050=(
BOUNDED_SURFACE()
B_SPLINE_SURFACE(1,2,((#145896,#145897,#145898),(#145899,#145900,#145901)),
 .UNSPECIFIED.,.F.,.F.,.F.)
B_SPLINE_SURFACE_WITH_KNOTS((2,2),(3,3),(0.710192959006796,1.),(0.125170525609408,
0.142682999576236),.UNSPECIFIED.)
GEOMETRIC_REPRESENTATION_ITEM()
RATIONAL_B_SPLINE_SURFACE(((0.990658108926709,0.993760979299921,0.999878046252917),
(0.990658108926709,0.993760979299921,0.999878046252917)))
REPRESENTATION_ITEM('')
SURFACE()
);
#3051=(
BOUNDED_SURFACE()
B_SPLINE_SURFACE(1,2,((#145909,#145910,#145911,#145912,#145913),(#145914,
#145915,#145916,#145917,#145918)),.UNSPECIFIED.,.F.,.F.,.F.)
B_SPLINE_SURFACE_WITH_KNOTS((2,2),(3,2,3),(0.709728555987901,1.),(0.590808523385635,
0.607982157956011,0.608572517848439),.UNSPECIFIED.)
GEOMETRIC_REPRESENTATION_ITEM()
RATIONAL_B_SPLINE_SURFACE(((0.990086238235256,0.987329216372183,0.987470879370255,
0.987470879370255,0.987470879370255),(0.990086238235256,0.987329216372183,
0.987470879370255,0.987470879370255,0.987470879370255)))
REPRESENTATION_ITEM('')
SURFACE()
);
#3052=(
BOUNDED_SURFACE()
B_SPLINE_SURFACE(1,2,((#145929,#145930,#145931),(#145932,#145933,#145934)),
 .UNSPECIFIED.,.F.,.F.,.F.)
B_SPLINE_SURFACE_WITH_KNOTS((2,2),(3,3),(0.710192959007385,1.),(0.125170525609408,
0.142682999576236),.UNSPECIFIED.)
GEOMETRIC_REPRESENTATION_ITEM()
RATIONAL_B_SPLINE_SURFACE(((0.990658108926709,0.993760979299921,0.999878046252917),
(0.990658108926709,0.993760979299921,0.999878046252917)))
REPRESENTATION_ITEM('')
SURFACE()
);
#3053=(
BOUNDED_SURFACE()
B_SPLINE_SURFACE(1,2,((#145942,#145943,#145944,#145945,#145946),(#145947,
#145948,#145949,#145950,#145951)),.UNSPECIFIED.,.F.,.F.,.F.)
B_SPLINE_SURFACE_WITH_KNOTS((2,2),(3,2,3),(0.709728556004289,1.),(0.590808523385635,
0.607982157956011,0.608572517831713),.UNSPECIFIED.)
GEOMETRIC_REPRESENTATION_ITEM()
RATIONAL_B_SPLINE_SURFACE(((0.990086238235256,0.987329216372183,0.987470879370255,
0.987470879370255,0.987470879370255),(0.990086238235256,0.987329216372183,
0.987470879370255,0.987470879370255,0.987470879370255)))
REPRESENTATION_ITEM('')
SURFACE()
);
#3054=(
BOUNDED_SURFACE()
B_SPLINE_SURFACE(1,2,((#145962,#145963,#145964),(#145965,#145966,#145967)),
 .UNSPECIFIED.,.F.,.F.,.F.)
B_SPLINE_SURFACE_WITH_KNOTS((2,2),(3,3),(0.71019295900683,1.),(0.125170525609408,
0.142682999576236),.UNSPECIFIED.)
GEOMETRIC_REPRESENTATION_ITEM()
RATIONAL_B_SPLINE_SURFACE(((0.990658108926709,0.993760979299921,0.999878046252917),
(0.990658108926709,0.993760979299921,0.999878046252917)))
REPRESENTATION_ITEM('')
SURFACE()
);
#3055=(
BOUNDED_SURFACE()
B_SPLINE_SURFACE(1,2,((#145975,#145976,#145977,#145978,#145979),(#145980,
#145981,#145982,#145983,#145984)),.UNSPECIFIED.,.F.,.F.,.F.)
B_SPLINE_SURFACE_WITH_KNOTS((2,2),(3,2,3),(0.709728556000902,1.),(0.590808523385636,
0.607982157956011,0.6085725178347),.UNSPECIFIED.)
GEOMETRIC_REPRESENTATION_ITEM()
RATIONAL_B_SPLINE_SURFACE(((0.990086238235256,0.987329216372183,0.987470879370255,
0.987470879370255,0.987470879370255),(0.990086238235256,0.987329216372183,
0.987470879370255,0.987470879370255,0.987470879370255)))
REPRESENTATION_ITEM('')
SURFACE()
);
#3056=(
BOUNDED_SURFACE()
B_SPLINE_SURFACE(1,2,((#145995,#145996,#145997),(#145998,#145999,#146000)),
 .UNSPECIFIED.,.F.,.F.,.F.)
B_SPLINE_SURFACE_WITH_KNOTS((2,2),(3,3),(0.710192959007012,1.),(0.125170525609407,
0.142682999576235),.UNSPECIFIED.)
GEOMETRIC_REPRESENTATION_ITEM()
RATIONAL_B_SPLINE_SURFACE(((0.990658108926708,0.993760979299921,0.999878046252916),
(0.990658108926708,0.993760979299921,0.999878046252916)))
REPRESENTATION_ITEM('')
SURFACE()
);
#3057=(
BOUNDED_SURFACE()
B_SPLINE_SURFACE(1,2,((#146008,#146009,#146010,#146011,#146012),(#146013,
#146014,#146015,#146016,#146017)),.UNSPECIFIED.,.F.,.F.,.F.)
B_SPLINE_SURFACE_WITH_KNOTS((2,2),(3,2,3),(0.709728555986702,1.),(0.590808523385636,
0.607982157956012,0.608572517849571),.UNSPECIFIED.)
GEOMETRIC_REPRESENTATION_ITEM()
RATIONAL_B_SPLINE_SURFACE(((0.990086238235256,0.987329216372183,0.987470879370255,
0.987470879370255,0.987470879370255),(0.990086238235256,0.987329216372183,
0.987470879370255,0.987470879370255,0.987470879370255)))
REPRESENTATION_ITEM('')
SURFACE()
);
#3058=(
BOUNDED_SURFACE()
B_SPLINE_SURFACE(1,2,((#146028,#146029,#146030),(#146031,#146032,#146033)),
 .UNSPECIFIED.,.F.,.F.,.F.)
B_SPLINE_SURFACE_WITH_KNOTS((2,2),(3,3),(0.710192959006983,1.),(0.125170525609407,
0.142682999576235),.UNSPECIFIED.)
GEOMETRIC_REPRESENTATION_ITEM()
RATIONAL_B_SPLINE_SURFACE(((0.990658108926708,0.993760979299921,0.999878046252916),
(0.990658108926708,0.993760979299921,0.999878046252916)))
REPRESENTATION_ITEM('')
SURFACE()
);
#3059=(
BOUNDED_SURFACE()
B_SPLINE_SURFACE(1,2,((#146041,#146042,#146043,#146044,#146045),(#146046,
#146047,#146048,#146049,#146050)),.UNSPECIFIED.,.F.,.F.,.F.)
B_SPLINE_SURFACE_WITH_KNOTS((2,2),(3,2,3),(0.709728555941526,1.),(0.590808523385636,
0.607982157956012,0.6085725178516),.UNSPECIFIED.)
GEOMETRIC_REPRESENTATION_ITEM()
RATIONAL_B_SPLINE_SURFACE(((0.990086238235256,0.987329216372183,0.987470879370255,
0.987470879370255,0.987470879370255),(0.990086238235256,0.987329216372183,
0.987470879370255,0.987470879370255,0.987470879370255)))
REPRESENTATION_ITEM('')
SURFACE()
);
#3060=(
BOUNDED_SURFACE()
B_SPLINE_SURFACE(1,2,((#146061,#146062,#146063),(#146064,#146065,#146066)),
 .UNSPECIFIED.,.F.,.F.,.F.)
B_SPLINE_SURFACE_WITH_KNOTS((2,2),(3,3),(0.710192959006704,1.),(0.125170525609407,
0.142682999576235),.UNSPECIFIED.)
GEOMETRIC_REPRESENTATION_ITEM()
RATIONAL_B_SPLINE_SURFACE(((0.990658108926708,0.993760979299921,0.999878046252916),
(0.990658108926708,0.993760979299921,0.999878046252916)))
REPRESENTATION_ITEM('')
SURFACE()
);
#3061=(
BOUNDED_SURFACE()
B_SPLINE_SURFACE(1,2,((#146074,#146075,#146076,#146077,#146078),(#146079,
#146080,#146081,#146082,#146083)),.UNSPECIFIED.,.F.,.F.,.F.)
B_SPLINE_SURFACE_WITH_KNOTS((2,2),(3,2,3),(0.709728555981745,1.),(0.590808523385636,
0.607982157956012,0.608572517854524),.UNSPECIFIED.)
GEOMETRIC_REPRESENTATION_ITEM()
RATIONAL_B_SPLINE_SURFACE(((0.990086238235256,0.987329216372183,0.987470879370255,
0.987470879370255,0.987470879370255),(0.990086238235256,0.987329216372183,
0.987470879370255,0.987470879370255,0.987470879370255)))
REPRESENTATION_ITEM('')
SURFACE()
);
#3062=(
BOUNDED_SURFACE()
B_SPLINE_SURFACE(1,2,((#146094,#146095,#146096),(#146097,#146098,#146099)),
 .UNSPECIFIED.,.F.,.F.,.F.)
B_SPLINE_SURFACE_WITH_KNOTS((2,2),(3,3),(0.710192959007287,1.),(0.125170525609407,
0.142682999576235),.UNSPECIFIED.)
GEOMETRIC_REPRESENTATION_ITEM()
RATIONAL_B_SPLINE_SURFACE(((0.990658108926708,0.993760979299921,0.999878046252916),
(0.990658108926708,0.993760979299921,0.999878046252916)))
REPRESENTATION_ITEM('')
SURFACE()
);
#3063=(
BOUNDED_SURFACE()
B_SPLINE_SURFACE(1,2,((#146107,#146108,#146109,#146110,#146111),(#146112,
#146113,#146114,#146115,#146116)),.UNSPECIFIED.,.F.,.F.,.F.)
B_SPLINE_SURFACE_WITH_KNOTS((2,2),(3,2,3),(0.709728555951994,1.),(0.590808523385636,
0.607982157956013,0.608572517840887),.UNSPECIFIED.)
GEOMETRIC_REPRESENTATION_ITEM()
RATIONAL_B_SPLINE_SURFACE(((0.990086238235256,0.987329216372183,0.987470879370255,
0.987470879370255,0.987470879370255),(0.990086238235256,0.987329216372183,
0.987470879370255,0.987470879370255,0.987470879370255)))
REPRESENTATION_ITEM('')
SURFACE()
);
#3064=(
BOUNDED_SURFACE()
B_SPLINE_SURFACE(1,2,((#146124,#146125,#146126),(#146127,#146128,#146129)),
 .UNSPECIFIED.,.F.,.F.,.F.)
B_SPLINE_SURFACE_WITH_KNOTS((2,2),(3,3),(0.710192959006456,1.),(0.125170525609407,
0.142682999576235),.UNSPECIFIED.)
GEOMETRIC_REPRESENTATION_ITEM()
RATIONAL_B_SPLINE_SURFACE(((0.990658108926708,0.993760979299921,0.999878046252916),
(0.990658108926708,0.993760979299921,0.999878046252916)))
REPRESENTATION_ITEM('')
SURFACE()
);
#3065=(
BOUNDED_SURFACE()
B_SPLINE_SURFACE(1,2,((#146131,#146132,#146133,#146134,#146135),(#146136,
#146137,#146138,#146139,#146140)),.UNSPECIFIED.,.F.,.F.,.F.)
B_SPLINE_SURFACE_WITH_KNOTS((2,2),(3,2,3),(0.709728555938271,1.),(0.590808523385636,
0.607982157956013,0.608572517855104),.UNSPECIFIED.)
GEOMETRIC_REPRESENTATION_ITEM()
RATIONAL_B_SPLINE_SURFACE(((0.990086238235256,0.987329216372183,0.987470879370255,
0.987470879370255,0.987470879370255),(0.990086238235256,0.987329216372183,
0.987470879370255,0.987470879370255,0.987470879370255)))
REPRESENTATION_ITEM('')
SURFACE()
);
#3066=(
BOUNDED_SURFACE()
B_SPLINE_SURFACE(1,2,((#146151,#146152,#146153),(#146154,#146155,#146156)),
 .UNSPECIFIED.,.F.,.F.,.F.)
B_SPLINE_SURFACE_WITH_KNOTS((2,2),(3,3),(0.710192959006957,1.),(0.125170525609407,
0.142682999576235),.UNSPECIFIED.)
GEOMETRIC_REPRESENTATION_ITEM()
RATIONAL_B_SPLINE_SURFACE(((0.990658108926708,0.993760979299921,0.999878046252916),
(0.990658108926708,0.993760979299921,0.999878046252916)))
REPRESENTATION_ITEM('')
SURFACE()
);
#3067=(
BOUNDED_SURFACE()
B_SPLINE_SURFACE(1,2,((#146164,#146165,#146166,#146167,#146168),(#146169,
#146170,#146171,#146172,#146173)),.UNSPECIFIED.,.F.,.F.,.F.)
B_SPLINE_SURFACE_WITH_KNOTS((2,2),(3,2,3),(0.709728555977483,1.),(0.590808523385636,
0.607982157956013,0.608572517858113),.UNSPECIFIED.)
GEOMETRIC_REPRESENTATION_ITEM()
RATIONAL_B_SPLINE_SURFACE(((0.990086238235256,0.987329216372183,0.987470879370256,
0.987470879370256,0.987470879370256),(0.990086238235256,0.987329216372183,
0.987470879370256,0.987470879370256,0.987470879370256)))
REPRESENTATION_ITEM('')
SURFACE()
);
#3068=(
BOUNDED_SURFACE()
B_SPLINE_SURFACE(1,2,((#146184,#146185,#146186),(#146187,#146188,#146189)),
 .UNSPECIFIED.,.F.,.F.,.F.)
B_SPLINE_SURFACE_WITH_KNOTS((2,2),(3,3),(0.710192959006483,1.),(0.125170525609407,
0.142682999576235),.UNSPECIFIED.)
GEOMETRIC_REPRESENTATION_ITEM()
RATIONAL_B_SPLINE_SURFACE(((0.990658108926708,0.993760979299921,0.999878046252916),
(0.990658108926708,0.993760979299921,0.999878046252916)))
REPRESENTATION_ITEM('')
SURFACE()
);
#3069=(
BOUNDED_SURFACE()
B_SPLINE_SURFACE(1,2,((#146197,#146198,#146199,#146200,#146201),(#146202,
#146203,#146204,#146205,#146206)),.UNSPECIFIED.,.F.,.F.,.F.)
B_SPLINE_SURFACE_WITH_KNOTS((2,2),(3,2,3),(0.709728556027411,1.),(0.590808523385636,
0.607982157956012,0.608572517808381),.UNSPECIFIED.)
GEOMETRIC_REPRESENTATION_ITEM()
RATIONAL_B_SPLINE_SURFACE(((0.990086238235256,0.987329216372183,0.987470879370255,
0.987470879370255,0.987470879370255),(0.990086238235256,0.987329216372183,
0.987470879370255,0.987470879370255,0.987470879370255)))
REPRESENTATION_ITEM('')
SURFACE()
);
#3070=(
BOUNDED_SURFACE()
B_SPLINE_SURFACE(1,2,((#146217,#146218,#146219),(#146220,#146221,#146222)),
 .UNSPECIFIED.,.F.,.F.,.F.)
B_SPLINE_SURFACE_WITH_KNOTS((2,2),(3,3),(0.710192959006738,1.),(0.125170525609407,
0.142682999576235),.UNSPECIFIED.)
GEOMETRIC_REPRESENTATION_ITEM()
RATIONAL_B_SPLINE_SURFACE(((0.990658108926708,0.993760979299921,0.999878046252916),
(0.990658108926708,0.993760979299921,0.999878046252916)))
REPRESENTATION_ITEM('')
SURFACE()
);
#3071=(
BOUNDED_SURFACE()
B_SPLINE_SURFACE(1,2,((#146230,#146231,#146232,#146233,#146234),(#146235,
#146236,#146237,#146238,#146239)),.UNSPECIFIED.,.F.,.F.,.F.)
B_SPLINE_SURFACE_WITH_KNOTS((2,2),(3,2,3),(0.709728555976806,1.),(0.590808523385636,
0.607982157956012,0.608572517857857),.UNSPECIFIED.)
GEOMETRIC_REPRESENTATION_ITEM()
RATIONAL_B_SPLINE_SURFACE(((0.990086238235256,0.987329216372183,0.987470879370255,
0.987470879370255,0.987470879370255),(0.990086238235256,0.987329216372183,
0.987470879370255,0.987470879370255,0.987470879370255)))
REPRESENTATION_ITEM('')
SURFACE()
);
#3072=(
BOUNDED_SURFACE()
B_SPLINE_SURFACE(1,2,((#146250,#146251,#146252),(#146253,#146254,#146255)),
 .UNSPECIFIED.,.F.,.F.,.F.)
B_SPLINE_SURFACE_WITH_KNOTS((2,2),(3,3),(0.710192959005573,1.),(0.125170525609407,
0.142682999576235),.UNSPECIFIED.)
GEOMETRIC_REPRESENTATION_ITEM()
RATIONAL_B_SPLINE_SURFACE(((0.990658108926708,0.993760979299921,0.999878046252916),
(0.990658108926708,0.993760979299921,0.999878046252916)))
REPRESENTATION_ITEM('')
SURFACE()
);
#3073=(
BOUNDED_SURFACE()
B_SPLINE_SURFACE(1,2,((#146263,#146264,#146265,#146266,#146267),(#146268,
#146269,#146270,#146271,#146272)),.UNSPECIFIED.,.F.,.F.,.F.)
B_SPLINE_SURFACE_WITH_KNOTS((2,2),(3,2,3),(0.709728555966191,1.),(0.590808523385636,
0.607982157956012,0.608572517827467),.UNSPECIFIED.)
GEOMETRIC_REPRESENTATION_ITEM()
RATIONAL_B_SPLINE_SURFACE(((0.990086238235256,0.987329216372183,0.987470879370255,
0.987470879370255,0.987470879370255),(0.990086238235256,0.987329216372183,
0.987470879370255,0.987470879370255,0.987470879370255)))
REPRESENTATION_ITEM('')
SURFACE()
);
#3074=(
BOUNDED_SURFACE()
B_SPLINE_SURFACE(1,2,((#146283,#146284,#146285),(#146286,#146287,#146288)),
 .UNSPECIFIED.,.F.,.F.,.F.)
B_SPLINE_SURFACE_WITH_KNOTS((2,2),(3,3),(0.710192959007236,1.),(0.125170525609407,
0.142682999576235),.UNSPECIFIED.)
GEOMETRIC_REPRESENTATION_ITEM()
RATIONAL_B_SPLINE_SURFACE(((0.990658108926708,0.993760979299921,0.999878046252916),
(0.990658108926708,0.993760979299921,0.999878046252916)))
REPRESENTATION_ITEM('')
SURFACE()
);
#3075=(
BOUNDED_SURFACE()
B_SPLINE_SURFACE(1,2,((#146296,#146297,#146298,#146299,#146300),(#146301,
#146302,#146303,#146304,#146305)),.UNSPECIFIED.,.F.,.F.,.F.)
B_SPLINE_SURFACE_WITH_KNOTS((2,2),(3,2,3),(0.709728555981059,1.),(0.590808523385636,
0.607982157956012,0.608572517855585),.UNSPECIFIED.)
GEOMETRIC_REPRESENTATION_ITEM()
RATIONAL_B_SPLINE_SURFACE(((0.990086238235256,0.987329216372183,0.987470879370255,
0.987470879370255,0.987470879370255),(0.990086238235256,0.987329216372183,
0.987470879370255,0.987470879370255,0.987470879370255)))
REPRESENTATION_ITEM('')
SURFACE()
);
#3076=(
BOUNDED_SURFACE()
B_SPLINE_SURFACE(1,2,((#146316,#146317,#146318),(#146319,#146320,#146321)),
 .UNSPECIFIED.,.F.,.F.,.F.)
B_SPLINE_SURFACE_WITH_KNOTS((2,2),(3,3),(0.710192959007354,1.),(0.125170525609407,
0.142682999576235),.UNSPECIFIED.)
GEOMETRIC_REPRESENTATION_ITEM()
RATIONAL_B_SPLINE_SURFACE(((0.990658108926708,0.993760979299921,0.999878046252916),
(0.990658108926708,0.993760979299921,0.999878046252916)))
REPRESENTATION_ITEM('')
SURFACE()
);
#3077=(
BOUNDED_SURFACE()
B_SPLINE_SURFACE(1,2,((#146329,#146330,#146331,#146332,#146333),(#146334,
#146335,#146336,#146337,#146338)),.UNSPECIFIED.,.F.,.F.,.F.)
B_SPLINE_SURFACE_WITH_KNOTS((2,2),(3,2,3),(0.709728555961017,1.),(0.590808523385636,
0.607982157956012,0.608572517831906),.UNSPECIFIED.)
GEOMETRIC_REPRESENTATION_ITEM()
RATIONAL_B_SPLINE_SURFACE(((0.990086238235256,0.987329216372183,0.987470879370255,
0.987470879370255,0.987470879370255),(0.990086238235256,0.987329216372183,
0.987470879370255,0.987470879370255,0.987470879370255)))
REPRESENTATION_ITEM('')
SURFACE()
);
#3078=(
BOUNDED_SURFACE()
B_SPLINE_SURFACE(1,2,((#146349,#146350,#146351),(#146352,#146353,#146354)),
 .UNSPECIFIED.,.F.,.F.,.F.)
B_SPLINE_SURFACE_WITH_KNOTS((2,2),(3,3),(0.710192959006508,1.),(0.125170525609407,
0.142682999576236),.UNSPECIFIED.)
GEOMETRIC_REPRESENTATION_ITEM()
RATIONAL_B_SPLINE_SURFACE(((0.990658108926708,0.993760979299921,0.999878046252916),
(0.990658108926708,0.993760979299921,0.999878046252916)))
REPRESENTATION_ITEM('')
SURFACE()
);
#3079=(
BOUNDED_SURFACE()
B_SPLINE_SURFACE(1,2,((#146362,#146363,#146364,#146365,#146366),(#146367,
#146368,#146369,#146370,#146371)),.UNSPECIFIED.,.F.,.F.,.F.)
B_SPLINE_SURFACE_WITH_KNOTS((2,2),(3,2,3),(0.709728555958552,1.),(0.590808523385636,
0.607982157956012,0.608572517835848),.UNSPECIFIED.)
GEOMETRIC_REPRESENTATION_ITEM()
RATIONAL_B_SPLINE_SURFACE(((0.990086238235256,0.987329216372183,0.987470879370255,
0.987470879370255,0.987470879370255),(0.990086238235256,0.987329216372183,
0.987470879370255,0.987470879370255,0.987470879370255)))
REPRESENTATION_ITEM('')
SURFACE()
);
#3080=(
BOUNDED_SURFACE()
B_SPLINE_SURFACE(1,2,((#146382,#146383,#146384),(#146385,#146386,#146387)),
 .UNSPECIFIED.,.F.,.F.,.F.)
B_SPLINE_SURFACE_WITH_KNOTS((2,2),(3,3),(0.710192959007983,1.),(0.125170525609407,
0.142682999576235),.UNSPECIFIED.)
GEOMETRIC_REPRESENTATION_ITEM()
RATIONAL_B_SPLINE_SURFACE(((0.990658108926708,0.993760979299921,0.999878046252916),
(0.990658108926708,0.993760979299921,0.999878046252916)))
REPRESENTATION_ITEM('')
SURFACE()
);
#3081=(
BOUNDED_SURFACE()
B_SPLINE_SURFACE(1,2,((#146395,#146396,#146397,#146398,#146399),(#146400,
#146401,#146402,#146403,#146404)),.UNSPECIFIED.,.F.,.F.,.F.)
B_SPLINE_SURFACE_WITH_KNOTS((2,2),(3,2,3),(0.709728555999848,1.),(0.590808523385636,
0.607982157956017,0.608572517836349),.UNSPECIFIED.)
GEOMETRIC_REPRESENTATION_ITEM()
RATIONAL_B_SPLINE_SURFACE(((0.990086238235256,0.987329216372182,0.987470879370255,
0.987470879370255,0.987470879370255),(0.990086238235256,0.987329216372182,
0.987470879370255,0.987470879370255,0.987470879370255)))
REPRESENTATION_ITEM('')
SURFACE()
);
#3082=(
BOUNDED_SURFACE()
B_SPLINE_SURFACE(1,2,((#146415,#146416,#146417),(#146418,#146419,#146420)),
 .UNSPECIFIED.,.F.,.F.,.F.)
B_SPLINE_SURFACE_WITH_KNOTS((2,2),(3,3),(0.710192959007115,1.),(0.125170525609407,
0.142682999576235),.UNSPECIFIED.)
GEOMETRIC_REPRESENTATION_ITEM()
RATIONAL_B_SPLINE_SURFACE(((0.990658108926708,0.993760979299921,0.999878046252916),
(0.990658108926708,0.993760979299921,0.999878046252916)))
REPRESENTATION_ITEM('')
SURFACE()
);
#3083=(
BOUNDED_SURFACE()
B_SPLINE_SURFACE(1,2,((#146428,#146429,#146430,#146431,#146432),(#146433,
#146434,#146435,#146436,#146437)),.UNSPECIFIED.,.F.,.F.,.F.)
B_SPLINE_SURFACE_WITH_KNOTS((2,2),(3,2,3),(0.709728555987099,1.),(0.590808523385636,
0.607982157956012,0.608572517849034),.UNSPECIFIED.)
GEOMETRIC_REPRESENTATION_ITEM()
RATIONAL_B_SPLINE_SURFACE(((0.990086238235256,0.987329216372183,0.987470879370255,
0.987470879370255,0.987470879370255),(0.990086238235256,0.987329216372183,
0.987470879370255,0.987470879370255,0.987470879370255)))
REPRESENTATION_ITEM('')
SURFACE()
);
#3084=(
BOUNDED_SURFACE()
B_SPLINE_SURFACE(1,2,((#146448,#146449,#146450),(#146451,#146452,#146453)),
 .UNSPECIFIED.,.F.,.F.,.F.)
B_SPLINE_SURFACE_WITH_KNOTS((2,2),(3,3),(0.710192959007309,1.),(0.125170525609407,
0.142682999576235),.UNSPECIFIED.)
GEOMETRIC_REPRESENTATION_ITEM()
RATIONAL_B_SPLINE_SURFACE(((0.990658108926708,0.993760979299921,0.999878046252916),
(0.990658108926708,0.993760979299921,0.999878046252916)))
REPRESENTATION_ITEM('')
SURFACE()
);
#3085=(
BOUNDED_SURFACE()
B_SPLINE_SURFACE(1,2,((#146461,#146462,#146463,#146464,#146465),(#146466,
#146467,#146468,#146469,#146470)),.UNSPECIFIED.,.F.,.F.,.F.)
B_SPLINE_SURFACE_WITH_KNOTS((2,2),(3,2,3),(0.709728555962953,1.),(0.590808523385636,
0.607982157956012,0.608572517871884),.UNSPECIFIED.)
GEOMETRIC_REPRESENTATION_ITEM()
RATIONAL_B_SPLINE_SURFACE(((0.990086238235256,0.987329216372183,0.987470879370255,
0.987470879370255,0.987470879370255),(0.990086238235256,0.987329216372183,
0.987470879370255,0.987470879370255,0.987470879370255)))
REPRESENTATION_ITEM('')
SURFACE()
);
#3086=(
BOUNDED_SURFACE()
B_SPLINE_SURFACE(1,2,((#146481,#146482,#146483),(#146484,#146485,#146486)),
 .UNSPECIFIED.,.F.,.F.,.F.)
B_SPLINE_SURFACE_WITH_KNOTS((2,2),(3,3),(0.710192959006066,1.),(0.125170525609408,
0.142682999576235),.UNSPECIFIED.)
GEOMETRIC_REPRESENTATION_ITEM()
RATIONAL_B_SPLINE_SURFACE(((0.990658108926709,0.993760979299921,0.999878046252916),
(0.990658108926709,0.993760979299921,0.999878046252916)))
REPRESENTATION_ITEM('')
SURFACE()
);
#3087=(
BOUNDED_SURFACE()
B_SPLINE_SURFACE(1,2,((#146494,#146495,#146496,#146497,#146498),(#146499,
#146500,#146501,#146502,#146503)),.UNSPECIFIED.,.F.,.F.,.F.)
B_SPLINE_SURFACE_WITH_KNOTS((2,2),(3,2,3),(0.709728555944512,1.),(0.590808523385635,
0.607982157956011,0.608572517850343),.UNSPECIFIED.)
GEOMETRIC_REPRESENTATION_ITEM()
RATIONAL_B_SPLINE_SURFACE(((0.990086238235256,0.987329216372183,0.987470879370255,
0.987470879370255,0.987470879370255),(0.990086238235256,0.987329216372183,
0.987470879370255,0.987470879370255,0.987470879370255)))
REPRESENTATION_ITEM('')
SURFACE()
);
#3088=(
BOUNDED_SURFACE()
B_SPLINE_SURFACE(1,2,((#146514,#146515,#146516),(#146517,#146518,#146519)),
 .UNSPECIFIED.,.F.,.F.,.F.)
B_SPLINE_SURFACE_WITH_KNOTS((2,2),(3,3),(0.710192959008445,1.),(0.125170525609408,
0.142682999576236),.UNSPECIFIED.)
GEOMETRIC_REPRESENTATION_ITEM()
RATIONAL_B_SPLINE_SURFACE(((0.990658108926709,0.993760979299921,0.999878046252917),
(0.990658108926709,0.993760979299921,0.999878046252917)))
REPRESENTATION_ITEM('')
SURFACE()
);
#3089=(
BOUNDED_SURFACE()
B_SPLINE_SURFACE(1,2,((#146527,#146528,#146529,#146530,#146531),(#146532,
#146533,#146534,#146535,#146536)),.UNSPECIFIED.,.F.,.F.,.F.)
B_SPLINE_SURFACE_WITH_KNOTS((2,2),(3,2,3),(0.709728555951602,1.),(0.590808523385635,
0.607982157956011,0.608572517843256),.UNSPECIFIED.)
GEOMETRIC_REPRESENTATION_ITEM()
RATIONAL_B_SPLINE_SURFACE(((0.990086238235256,0.987329216372183,0.987470879370255,
0.987470879370255,0.987470879370255),(0.990086238235256,0.987329216372183,
0.987470879370255,0.987470879370255,0.987470879370255)))
REPRESENTATION_ITEM('')
SURFACE()
);
#3090=(
BOUNDED_SURFACE()
B_SPLINE_SURFACE(1,2,((#146547,#146548,#146549),(#146550,#146551,#146552)),
 .UNSPECIFIED.,.F.,.F.,.F.)
B_SPLINE_SURFACE_WITH_KNOTS((2,2),(3,3),(0.710192959008442,1.),(0.125170525609408,
0.142682999576236),.UNSPECIFIED.)
GEOMETRIC_REPRESENTATION_ITEM()
RATIONAL_B_SPLINE_SURFACE(((0.990658108926709,0.993760979299921,0.999878046252917),
(0.990658108926709,0.993760979299921,0.999878046252917)))
REPRESENTATION_ITEM('')
SURFACE()
);
#3091=(
BOUNDED_SURFACE()
B_SPLINE_SURFACE(1,2,((#146560,#146561,#146562,#146563,#146564),(#146565,
#146566,#146567,#146568,#146569)),.UNSPECIFIED.,.F.,.F.,.F.)
B_SPLINE_SURFACE_WITH_KNOTS((2,2),(3,2,3),(0.70972855596089,1.),(0.590808523385635,
0.607982157956011,0.608572517833635),.UNSPECIFIED.)
GEOMETRIC_REPRESENTATION_ITEM()
RATIONAL_B_SPLINE_SURFACE(((0.990086238235256,0.987329216372183,0.987470879370256,
0.987470879370256,0.987470879370256),(0.990086238235256,0.987329216372183,
0.987470879370256,0.987470879370256,0.987470879370256)))
REPRESENTATION_ITEM('')
SURFACE()
);
#3092=(
BOUNDED_SURFACE()
B_SPLINE_SURFACE(1,2,((#146580,#146581,#146582),(#146583,#146584,#146585)),
 .UNSPECIFIED.,.F.,.F.,.F.)
B_SPLINE_SURFACE_WITH_KNOTS((2,2),(3,3),(0.71019295900811,1.),(0.125170525609408,
0.142682999576236),.UNSPECIFIED.)
GEOMETRIC_REPRESENTATION_ITEM()
RATIONAL_B_SPLINE_SURFACE(((0.990658108926709,0.993760979299922,0.999878046252917),
(0.990658108926709,0.993760979299922,0.999878046252917)))
REPRESENTATION_ITEM('')
SURFACE()
);
#3093=(
BOUNDED_SURFACE()
B_SPLINE_SURFACE(1,2,((#146599,#146600,#146601,#146602,#146603),(#146604,
#146605,#146606,#146607,#146608)),.UNSPECIFIED.,.F.,.F.,.F.)
B_SPLINE_SURFACE_WITH_KNOTS((2,2),(3,2,3),(0.709728555969186,1.),(0.590808523385635,
0.607982157956011,0.608572517825209),.UNSPECIFIED.)
GEOMETRIC_REPRESENTATION_ITEM()
RATIONAL_B_SPLINE_SURFACE(((0.990086238235256,0.987329216372183,0.987470879370256,
0.987470879370256,0.987470879370256),(0.990086238235256,0.987329216372183,
0.987470879370256,0.987470879370256,0.987470879370256)))
REPRESENTATION_ITEM('')
SURFACE()
);
#3094=(
BOUNDED_SURFACE()
B_SPLINE_SURFACE(1,2,((#146610,#146611,#146612,#146613,#146614),(#146615,
#146616,#146617,#146618,#146619)),.UNSPECIFIED.,.F.,.F.,.F.)
B_SPLINE_SURFACE_WITH_KNOTS((2,2),(3,2,3),(0.709729983312017,1.),(0.159799014184144,
0.176967058622922,0.177555991154001),.UNSPECIFIED.)
GEOMETRIC_REPRESENTATION_ITEM()
RATIONAL_B_SPLINE_SURFACE(((0.990927469170768,0.987759962570789,0.98748925405691,
0.98748925405691,0.98748925405691),(0.990927469170768,0.987759962570789,
0.98748925405691,0.98748925405691,0.98748925405691)))
REPRESENTATION_ITEM('')
SURFACE()
);
#3095=(
BOUNDED_SURFACE()
B_SPLINE_SURFACE(1,2,((#146635,#146636,#146637,#146638,#146639,#146640,
#146641),(#146642,#146643,#146644,#146645,#146646,#146647,#146648)),
 .UNSPECIFIED.,.F.,.F.,.F.)
B_SPLINE_SURFACE_WITH_KNOTS((2,2),(3,2,2,3),(0.710192959008444,1.),(0.556037361265319,
0.556212823028861,0.571428571428571,0.573758999383056),.UNSPECIFIED.)
GEOMETRIC_REPRESENTATION_ITEM()
RATIONAL_B_SPLINE_SURFACE(((0.991593692313265,0.991593692313265,0.991593692313265,
0.994659131878645,1.,0.999181998279397,0.998417372792936),(0.991593692313265,
0.991593692313265,0.991593692313265,0.994659131878644,1.,0.999181998279397,
0.998417372792936)))
REPRESENTATION_ITEM('')
SURFACE()
);
#3096=(
BOUNDED_SURFACE()
B_SPLINE_SURFACE(1,2,((#146670,#146671,#146672,#146673,#146674),(#146675,
#146676,#146677,#146678,#146679)),.UNSPECIFIED.,.F.,.F.,.F.)
B_SPLINE_SURFACE_WITH_KNOTS((2,2),(3,2,3),(0.709729983378474,1.),(0.159799014184072,
0.176967058622925,0.177555991087653),.UNSPECIFIED.)
GEOMETRIC_REPRESENTATION_ITEM()
RATIONAL_B_SPLINE_SURFACE(((0.990927469170795,0.98775996257079,0.98748925405691,
0.98748925405691,0.98748925405691),(0.990927469170795,0.98775996257079,
0.98748925405691,0.98748925405691,0.98748925405691)))
REPRESENTATION_ITEM('')
SURFACE()
);
#3097=(
BOUNDED_SURFACE()
B_SPLINE_SURFACE(1,2,((#146681,#146682,#146683,#146684,#146685,#146686,
#146687),(#146688,#146689,#146690,#146691,#146692,#146693,#146694)),
 .UNSPECIFIED.,.F.,.F.,.F.)
B_SPLINE_SURFACE_WITH_KNOTS((2,2),(3,2,2,3),(0.710192959008435,1.),(0.556037361265319,
0.556212823028861,0.571428571428571,0.573758999383057),.UNSPECIFIED.)
GEOMETRIC_REPRESENTATION_ITEM()
RATIONAL_B_SPLINE_SURFACE(((0.991593692313265,0.991593692313265,0.991593692313265,
0.994659131878645,1.,0.999181998279397,0.998417372792936),(0.991593692313265,
0.991593692313265,0.991593692313265,0.994659131878645,1.,0.999181998279397,
0.998417372792936)))
REPRESENTATION_ITEM('')
SURFACE()
);
#3098=(
BOUNDED_SURFACE()
B_SPLINE_SURFACE(1,2,((#146711,#146712,#146713,#146714,#146715),(#146716,
#146717,#146718,#146719,#146720)),.UNSPECIFIED.,.F.,.F.,.F.)
B_SPLINE_SURFACE_WITH_KNOTS((2,2),(3,2,3),(0.709729983387492,1.),(0.15979901418427,
0.176967058622921,0.177555991079107),.UNSPECIFIED.)
GEOMETRIC_REPRESENTATION_ITEM()
RATIONAL_B_SPLINE_SURFACE(((0.990927469170722,0.987759962570788,0.98748925405691,
0.98748925405691,0.98748925405691),(0.990927469170722,0.987759962570788,
0.98748925405691,0.98748925405691,0.98748925405691)))
REPRESENTATION_ITEM('')
SURFACE()
);
#3099=(
BOUNDED_SURFACE()
B_SPLINE_SURFACE(1,2,((#146722,#146723,#146724,#146725,#146726,#146727,
#146728),(#146729,#146730,#146731,#146732,#146733,#146734,#146735)),
 .UNSPECIFIED.,.F.,.F.,.F.)
B_SPLINE_SURFACE_WITH_KNOTS((2,2),(3,2,2,3),(0.710192959008441,1.),(0.55603736126532,
0.556212823028862,0.571428571428571,0.573758999383058),.UNSPECIFIED.)
GEOMETRIC_REPRESENTATION_ITEM()
RATIONAL_B_SPLINE_SURFACE(((0.991593692313266,0.991593692313266,0.991593692313266,
0.994659131878645,1.,0.999181998279397,0.998417372792936),(0.991593692313266,
0.991593692313266,0.991593692313266,0.994659131878645,1.,0.999181998279397,
0.998417372792936)))
REPRESENTATION_ITEM('')
SURFACE()
);
#3100=(
BOUNDED_SURFACE()
B_SPLINE_SURFACE(1,2,((#146761,#146762,#146763,#146764,#146765),(#146766,
#146767,#146768,#146769,#146770)),.UNSPECIFIED.,.F.,.F.,.F.)
B_SPLINE_SURFACE_WITH_KNOTS((2,2),(3,2,3),(0.709729983410559,1.),(0.159799014184008,
0.176967058622921,0.177555991055812),.UNSPECIFIED.)
GEOMETRIC_REPRESENTATION_ITEM()
RATIONAL_B_SPLINE_SURFACE(((0.990927469170818,0.987759962570791,0.98748925405691,
0.98748925405691,0.98748925405691),(0.990927469170818,0.987759962570792,
0.98748925405691,0.98748925405691,0.98748925405691)))
REPRESENTATION_ITEM('')
SURFACE()
);
#3101=(
BOUNDED_SURFACE()
B_SPLINE_SURFACE(1,2,((#146772,#146773,#146774,#146775,#146776,#146777,
#146778),(#146779,#146780,#146781,#146782,#146783,#146784,#146785)),
 .UNSPECIFIED.,.F.,.F.,.F.)
B_SPLINE_SURFACE_WITH_KNOTS((2,2),(3,2,2,3),(0.710192959008438,1.),(0.55603736126532,
0.556212823028862,0.571428571428571,0.573758999383057),.UNSPECIFIED.)
GEOMETRIC_REPRESENTATION_ITEM()
RATIONAL_B_SPLINE_SURFACE(((0.991593692313266,0.991593692313266,0.991593692313266,
0.994659131878645,1.,0.999181998279397,0.998417372792936),(0.991593692313266,
0.991593692313266,0.991593692313266,0.994659131878645,1.,0.999181998279397,
0.998417372792936)))
REPRESENTATION_ITEM('')
SURFACE()
);
#3102=(
BOUNDED_SURFACE()
B_SPLINE_SURFACE(1,2,((#146802,#146803,#146804,#146805,#146806),(#146807,
#146808,#146809,#146810,#146811)),.UNSPECIFIED.,.F.,.F.,.F.)
B_SPLINE_SURFACE_WITH_KNOTS((2,2),(3,2,3),(0.709729983402952,1.),(0.159799014184145,
0.176967058622924,0.177555991063508),.UNSPECIFIED.)
GEOMETRIC_REPRESENTATION_ITEM()
RATIONAL_B_SPLINE_SURFACE(((0.990927469170767,0.987759962570789,0.98748925405691,
0.98748925405691,0.98748925405691),(0.990927469170767,0.987759962570789,
0.98748925405691,0.98748925405691,0.98748925405691)))
REPRESENTATION_ITEM('')
SURFACE()
);
#3103=(
BOUNDED_SURFACE()
B_SPLINE_SURFACE(1,2,((#146813,#146814,#146815,#146816,#146817,#146818,
#146819),(#146820,#146821,#146822,#146823,#146824,#146825,#146826)),
 .UNSPECIFIED.,.F.,.F.,.F.)
B_SPLINE_SURFACE_WITH_KNOTS((2,2),(3,2,2,3),(0.710192959008438,1.),(0.55603736126532,
0.556212823028862,0.571428571428571,0.573758999383058),.UNSPECIFIED.)
GEOMETRIC_REPRESENTATION_ITEM()
RATIONAL_B_SPLINE_SURFACE(((0.991593692313266,0.991593692313266,0.991593692313266,
0.994659131878645,1.,0.999181998279397,0.998417372792936),(0.991593692313266,
0.991593692313266,0.991593692313266,0.994659131878645,1.,0.999181998279397,
0.998417372792936)))
REPRESENTATION_ITEM('')
SURFACE()
);
#3104=(
BOUNDED_SURFACE()
B_SPLINE_SURFACE(1,2,((#146843,#146844,#146845,#146846,#146847),(#146848,
#146849,#146850,#146851,#146852)),.UNSPECIFIED.,.F.,.F.,.F.)
B_SPLINE_SURFACE_WITH_KNOTS((2,2),(3,2,3),(0.709729983374391,1.),(0.159799014184268,
0.176967058622924,0.177555991091671),.UNSPECIFIED.)
GEOMETRIC_REPRESENTATION_ITEM()
RATIONAL_B_SPLINE_SURFACE(((0.990927469170722,0.987759962570787,0.98748925405691,
0.98748925405691,0.98748925405691),(0.990927469170722,0.987759962570787,
0.98748925405691,0.98748925405691,0.98748925405691)))
REPRESENTATION_ITEM('')
SURFACE()
);
#3105=(
BOUNDED_SURFACE()
B_SPLINE_SURFACE(1,2,((#146854,#146855,#146856,#146857,#146858,#146859,
#146860),(#146861,#146862,#146863,#146864,#146865,#146866,#146867)),
 .UNSPECIFIED.,.F.,.F.,.F.)
B_SPLINE_SURFACE_WITH_KNOTS((2,2),(3,2,2,3),(0.710192959008442,1.),(0.55603736126532,
0.556212823028862,0.571428571428571,0.573758999383058),.UNSPECIFIED.)
GEOMETRIC_REPRESENTATION_ITEM()
RATIONAL_B_SPLINE_SURFACE(((0.991593692313266,0.991593692313266,0.991593692313266,
0.994659131878645,1.,0.999181998279397,0.998417372792936),(0.991593692313266,
0.991593692313266,0.991593692313266,0.994659131878645,1.,0.999181998279397,
0.998417372792936)))
REPRESENTATION_ITEM('')
SURFACE()
);
#3106=(
BOUNDED_SURFACE()
B_SPLINE_SURFACE(1,2,((#146893,#146894,#146895,#146896,#146897),(#146898,
#146899,#146900,#146901,#146902)),.UNSPECIFIED.,.F.,.F.,.F.)
B_SPLINE_SURFACE_WITH_KNOTS((2,2),(3,2,3),(0.709729983359613,1.),(0.159799014184268,
0.176967058622921,0.177555991106485),.UNSPECIFIED.)
GEOMETRIC_REPRESENTATION_ITEM()
RATIONAL_B_SPLINE_SURFACE(((0.990927469170722,0.987759962570787,0.98748925405691,
0.98748925405691,0.98748925405691),(0.990927469170722,0.987759962570787,
0.98748925405691,0.98748925405691,0.98748925405691)))
REPRESENTATION_ITEM('')
SURFACE()
);
#3107=(
BOUNDED_SURFACE()
B_SPLINE_SURFACE(1,2,((#146904,#146905,#146906,#146907,#146908,#146909,
#146910),(#146911,#146912,#146913,#146914,#146915,#146916,#146917)),
 .UNSPECIFIED.,.F.,.F.,.F.)
B_SPLINE_SURFACE_WITH_KNOTS((2,2),(3,2,2,3),(0.71019295900844,1.),(0.55603736126532,
0.556212823028862,0.571428571428571,0.573758999383058),.UNSPECIFIED.)
GEOMETRIC_REPRESENTATION_ITEM()
RATIONAL_B_SPLINE_SURFACE(((0.991593692313266,0.991593692313266,0.991593692313266,
0.994659131878645,1.,0.999181998279397,0.998417372792936),(0.991593692313266,
0.991593692313266,0.991593692313266,0.994659131878645,1.,0.999181998279397,
0.998417372792936)))
REPRESENTATION_ITEM('')
SURFACE()
);
#3108=(
BOUNDED_SURFACE()
B_SPLINE_SURFACE(1,2,((#146943,#146944,#146945,#146946,#146947),(#146948,
#146949,#146950,#146951,#146952)),.UNSPECIFIED.,.F.,.F.,.F.)
B_SPLINE_SURFACE_WITH_KNOTS((2,2),(3,2,3),(0.710058121447169,1.),(0.159799014184268,
0.176967058622924,0.177227853019055),.UNSPECIFIED.)
GEOMETRIC_REPRESENTATION_ITEM()
RATIONAL_B_SPLINE_SURFACE(((0.990927469170722,0.987759962570787,0.98748925405691,
0.98748925405691,0.98748925405691),(0.990927469170722,0.987759962570787,
0.98748925405691,0.98748925405691,0.98748925405691)))
REPRESENTATION_ITEM('')
SURFACE()
);
#3109=(
BOUNDED_SURFACE()
B_SPLINE_SURFACE(1,2,((#146954,#146955,#146956,#146957,#146958,#146959,
#146960),(#146961,#146962,#146963,#146964,#146965,#146966,#146967)),
 .UNSPECIFIED.,.F.,.F.,.F.)
B_SPLINE_SURFACE_WITH_KNOTS((2,2),(3,2,2,3),(0.710192959008443,1.),(0.55603736126532,
0.556212823028862,0.571428571428571,0.573758999383058),.UNSPECIFIED.)
GEOMETRIC_REPRESENTATION_ITEM()
RATIONAL_B_SPLINE_SURFACE(((0.991593692313266,0.991593692313266,0.991593692313266,
0.994659131878645,1.,0.999181998279397,0.998417372792936),(0.991593692313266,
0.991593692313266,0.991593692313266,0.994659131878645,1.,0.999181998279397,
0.998417372792936)))
REPRESENTATION_ITEM('')
SURFACE()
);
#3110=(
BOUNDED_SURFACE()
B_SPLINE_SURFACE(1,2,((#146992,#146993,#146994,#146995,#146996),(#146997,
#146998,#146999,#147000,#147001)),.UNSPECIFIED.,.F.,.F.,.F.)
B_SPLINE_SURFACE_WITH_KNOTS((2,2),(3,2,3),(0.709729983365709,1.),(0.159799014184269,
0.176967058622924,0.177555991099995),.UNSPECIFIED.)
GEOMETRIC_REPRESENTATION_ITEM()
RATIONAL_B_SPLINE_SURFACE(((0.990927469170722,0.987759962570787,0.98748925405691,
0.98748925405691,0.98748925405691),(0.990927469170722,0.987759962570787,
0.98748925405691,0.98748925405691,0.98748925405691)))
REPRESENTATION_ITEM('')
SURFACE()
);
#3111=(
BOUNDED_SURFACE()
B_SPLINE_SURFACE(1,2,((#147003,#147004,#147005,#147006,#147007,#147008,
#147009),(#147010,#147011,#147012,#147013,#147014,#147015,#147016)),
 .UNSPECIFIED.,.F.,.F.,.F.)
B_SPLINE_SURFACE_WITH_KNOTS((2,2),(3,2,2,3),(0.710192959008441,1.),(0.55603736126532,
0.556212823028862,0.571428571428571,0.573758999383058),.UNSPECIFIED.)
GEOMETRIC_REPRESENTATION_ITEM()
RATIONAL_B_SPLINE_SURFACE(((0.991593692313266,0.991593692313266,0.991593692313266,
0.994659131878645,1.,0.999181998279397,0.998417372792936),(0.991593692313266,
0.991593692313266,0.991593692313266,0.994659131878645,1.,0.999181998279397,
0.998417372792936)))
REPRESENTATION_ITEM('')
SURFACE()
);
#3112=(
BOUNDED_SURFACE()
B_SPLINE_SURFACE(1,2,((#147041,#147042,#147043,#147044,#147045),(#147046,
#147047,#147048,#147049,#147050)),.UNSPECIFIED.,.F.,.F.,.F.)
B_SPLINE_SURFACE_WITH_KNOTS((2,2),(3,2,3),(0.709729983361247,1.),(0.159799014184269,
0.176967058622924,0.177555991104612),.UNSPECIFIED.)
GEOMETRIC_REPRESENTATION_ITEM()
RATIONAL_B_SPLINE_SURFACE(((0.990927469170722,0.987759962570787,0.98748925405691,
0.98748925405691,0.98748925405691),(0.990927469170722,0.987759962570787,
0.98748925405691,0.98748925405691,0.98748925405691)))
REPRESENTATION_ITEM('')
SURFACE()
);
#3113=(
BOUNDED_SURFACE()
B_SPLINE_SURFACE(1,2,((#147052,#147053,#147054,#147055,#147056,#147057,
#147058),(#147059,#147060,#147061,#147062,#147063,#147064,#147065)),
 .UNSPECIFIED.,.F.,.F.,.F.)
B_SPLINE_SURFACE_WITH_KNOTS((2,2),(3,2,2,3),(0.71019295900844,1.),(0.556037361265321,
0.556212823028862,0.571428571428571,0.573758999382983),.UNSPECIFIED.)
GEOMETRIC_REPRESENTATION_ITEM()
RATIONAL_B_SPLINE_SURFACE(((0.991593692313266,0.991593692313266,0.991593692313266,
0.994659131878645,1.,0.999181998279423,0.998417372792985),(0.991593692313266,
0.991593692313266,0.991593692313266,0.994659131878645,1.,0.999181998279423,
0.998417372792985)))
REPRESENTATION_ITEM('')
SURFACE()
);
#3114=(
BOUNDED_SURFACE()
B_SPLINE_SURFACE(1,2,((#147091,#147092,#147093,#147094,#147095),(#147096,
#147097,#147098,#147099,#147100)),.UNSPECIFIED.,.F.,.F.,.F.)
B_SPLINE_SURFACE_WITH_KNOTS((2,2),(3,2,3),(0.709729983382268,1.),(0.159799014184052,
0.176967058622924,0.177555991084222),.UNSPECIFIED.)
GEOMETRIC_REPRESENTATION_ITEM()
RATIONAL_B_SPLINE_SURFACE(((0.990927469170802,0.98775996257079,0.98748925405691,
0.98748925405691,0.98748925405691),(0.990927469170802,0.98775996257079,
0.98748925405691,0.98748925405691,0.98748925405691)))
REPRESENTATION_ITEM('')
SURFACE()
);
#3115=(
BOUNDED_SURFACE()
B_SPLINE_SURFACE(1,2,((#147102,#147103,#147104,#147105,#147106,#147107,
#147108),(#147109,#147110,#147111,#147112,#147113,#147114,#147115)),
 .UNSPECIFIED.,.F.,.F.,.F.)
B_SPLINE_SURFACE_WITH_KNOTS((2,2),(3,2,2,3),(0.71019295900844,1.),(0.55603736126532,
0.556212823028862,0.571428571428571,0.573758999383058),.UNSPECIFIED.)
GEOMETRIC_REPRESENTATION_ITEM()
RATIONAL_B_SPLINE_SURFACE(((0.991593692313266,0.991593692313266,0.991593692313266,
0.994659131878645,1.,0.999181998279397,0.998417372792936),(0.991593692313266,
0.991593692313266,0.991593692313266,0.994659131878645,1.,0.999181998279397,
0.998417372792936)))
REPRESENTATION_ITEM('')
SURFACE()
);
#3116=(
BOUNDED_SURFACE()
B_SPLINE_SURFACE(1,2,((#147132,#147133,#147134,#147135,#147136),(#147137,
#147138,#147139,#147140,#147141)),.UNSPECIFIED.,.F.,.F.,.F.)
B_SPLINE_SURFACE_WITH_KNOTS((2,2),(3,2,3),(0.709729983363911,1.),(0.159799014184268,
0.176967058622924,0.177555991102057),.UNSPECIFIED.)
GEOMETRIC_REPRESENTATION_ITEM()
RATIONAL_B_SPLINE_SURFACE(((0.990927469170722,0.987759962570787,0.98748925405691,
0.98748925405691,0.98748925405691),(0.990927469170722,0.987759962570787,
0.98748925405691,0.98748925405691,0.98748925405691)))
REPRESENTATION_ITEM('')
SURFACE()
);
#3117=(
BOUNDED_SURFACE()
B_SPLINE_SURFACE(1,2,((#147143,#147144,#147145,#147146,#147147,#147148,
#147149),(#147150,#147151,#147152,#147153,#147154,#147155,#147156)),
 .UNSPECIFIED.,.F.,.F.,.F.)
B_SPLINE_SURFACE_WITH_KNOTS((2,2),(3,2,2,3),(0.710192959008439,1.),(0.55603736126532,
0.556212823028862,0.571428571428571,0.573758999383058),.UNSPECIFIED.)
GEOMETRIC_REPRESENTATION_ITEM()
RATIONAL_B_SPLINE_SURFACE(((0.991593692313266,0.991593692313266,0.991593692313266,
0.994659131878645,1.,0.999181998279397,0.998417372792936),(0.991593692313266,
0.991593692313266,0.991593692313266,0.994659131878645,1.,0.999181998279397,
0.998417372792936)))
REPRESENTATION_ITEM('')
SURFACE()
);
#3118=(
BOUNDED_SURFACE()
B_SPLINE_SURFACE(1,2,((#147182,#147183,#147184,#147185,#147186),(#147187,
#147188,#147189,#147190,#147191)),.UNSPECIFIED.,.F.,.F.,.F.)
B_SPLINE_SURFACE_WITH_KNOTS((2,2),(3,2,3),(0.709729983383673,1.),(0.159799014184268,
0.176967058622921,0.177555991082457),.UNSPECIFIED.)
GEOMETRIC_REPRESENTATION_ITEM()
RATIONAL_B_SPLINE_SURFACE(((0.990927469170722,0.987759962570787,0.98748925405691,
0.98748925405691,0.98748925405691),(0.990927469170722,0.987759962570787,
0.98748925405691,0.98748925405691,0.98748925405691)))
REPRESENTATION_ITEM('')
SURFACE()
);
#3119=(
BOUNDED_SURFACE()
B_SPLINE_SURFACE(1,2,((#147193,#147194,#147195,#147196,#147197,#147198,
#147199),(#147200,#147201,#147202,#147203,#147204,#147205,#147206)),
 .UNSPECIFIED.,.F.,.F.,.F.)
B_SPLINE_SURFACE_WITH_KNOTS((2,2),(3,2,2,3),(0.710192959008439,1.),(0.55603736126532,
0.556212823028862,0.571428571428571,0.573758999383058),.UNSPECIFIED.)
GEOMETRIC_REPRESENTATION_ITEM()
RATIONAL_B_SPLINE_SURFACE(((0.991593692313266,0.991593692313266,0.991593692313266,
0.994659131878645,1.,0.999181998279397,0.998417372792936),(0.991593692313266,
0.991593692313266,0.991593692313266,0.994659131878645,1.,0.999181998279397,
0.998417372792936)))
REPRESENTATION_ITEM('')
SURFACE()
);
#3120=(
BOUNDED_SURFACE()
B_SPLINE_SURFACE(1,2,((#147226,#147227,#147228,#147229,#147230),(#147231,
#147232,#147233,#147234,#147235)),.UNSPECIFIED.,.F.,.F.,.F.)
B_SPLINE_SURFACE_WITH_KNOTS((2,2),(3,2,3),(0.709729983356482,1.),(0.159799014184268,
0.176967058622921,0.177555991109801),.UNSPECIFIED.)
GEOMETRIC_REPRESENTATION_ITEM()
RATIONAL_B_SPLINE_SURFACE(((0.990927469170722,0.987759962570787,0.98748925405691,
0.98748925405691,0.98748925405691),(0.990927469170722,0.987759962570787,
0.98748925405691,0.98748925405691,0.98748925405691)))
REPRESENTATION_ITEM('')
SURFACE()
);
#3121=(
BOUNDED_SURFACE()
B_SPLINE_SURFACE(1,2,((#147237,#147238,#147239,#147240,#147241,#147242,
#147243),(#147244,#147245,#147246,#147247,#147248,#147249,#147250)),
 .UNSPECIFIED.,.F.,.F.,.F.)
B_SPLINE_SURFACE_WITH_KNOTS((2,2),(3,2,2,3),(0.710192959008445,1.),(0.55603736126532,
0.556212823028862,0.571428571428571,0.573758999383058),.UNSPECIFIED.)
GEOMETRIC_REPRESENTATION_ITEM()
RATIONAL_B_SPLINE_SURFACE(((0.991593692313266,0.991593692313266,0.991593692313266,
0.994659131878645,1.,0.999181998279397,0.998417372792936),(0.991593692313266,
0.991593692313266,0.991593692313266,0.994659131878645,1.,0.999181998279397,
0.998417372792936)))
REPRESENTATION_ITEM('')
SURFACE()
);
#3122=(
BOUNDED_SURFACE()
B_SPLINE_SURFACE(1,2,((#147272,#147273,#147274,#147275,#147276),(#147277,
#147278,#147279,#147280,#147281)),.UNSPECIFIED.,.F.,.F.,.F.)
B_SPLINE_SURFACE_WITH_KNOTS((2,2),(3,2,3),(0.709729983342325,1.),(0.159799014184269,
0.176967058622924,0.177555991123784),.UNSPECIFIED.)
GEOMETRIC_REPRESENTATION_ITEM()
RATIONAL_B_SPLINE_SURFACE(((0.990927469170722,0.987759962570787,0.98748925405691,
0.98748925405691,0.98748925405691),(0.990927469170722,0.987759962570787,
0.98748925405691,0.98748925405691,0.98748925405691)))
REPRESENTATION_ITEM('')
SURFACE()
);
#3123=(
BOUNDED_SURFACE()
B_SPLINE_SURFACE(1,2,((#147283,#147284,#147285,#147286,#147287,#147288,
#147289),(#147290,#147291,#147292,#147293,#147294,#147295,#147296)),
 .UNSPECIFIED.,.F.,.F.,.F.)
B_SPLINE_SURFACE_WITH_KNOTS((2,2),(3,2,2,3),(0.710192959008445,1.),(0.55603736126532,
0.556212823028862,0.571428571428571,0.573758999383058),.UNSPECIFIED.)
GEOMETRIC_REPRESENTATION_ITEM()
RATIONAL_B_SPLINE_SURFACE(((0.991593692313266,0.991593692313266,0.991593692313266,
0.994659131878645,1.,0.999181998279397,0.998417372792936),(0.991593692313266,
0.991593692313266,0.991593692313266,0.994659131878645,1.,0.999181998279397,
0.998417372792936)))
REPRESENTATION_ITEM('')
SURFACE()
);
#3124=(
BOUNDED_SURFACE()
B_SPLINE_SURFACE(1,2,((#147322,#147323,#147324,#147325,#147326),(#147327,
#147328,#147329,#147330,#147331)),.UNSPECIFIED.,.F.,.F.,.F.)
B_SPLINE_SURFACE_WITH_KNOTS((2,2),(3,2,3),(0.709729983366589,1.),(0.159799014184268,
0.176967058622921,0.177555991099152),.UNSPECIFIED.)
GEOMETRIC_REPRESENTATION_ITEM()
RATIONAL_B_SPLINE_SURFACE(((0.990927469170722,0.987759962570787,0.98748925405691,
0.98748925405691,0.98748925405691),(0.990927469170722,0.987759962570787,
0.98748925405691,0.98748925405691,0.98748925405691)))
REPRESENTATION_ITEM('')
SURFACE()
);
#3125=(
BOUNDED_SURFACE()
B_SPLINE_SURFACE(1,2,((#147333,#147334,#147335,#147336,#147337,#147338,
#147339),(#147340,#147341,#147342,#147343,#147344,#147345,#147346)),
 .UNSPECIFIED.,.F.,.F.,.F.)
B_SPLINE_SURFACE_WITH_KNOTS((2,2),(3,2,2,3),(0.710192959008445,1.),(0.55603736126532,
0.556212823028862,0.571428571428571,0.573758999383058),.UNSPECIFIED.)
GEOMETRIC_REPRESENTATION_ITEM()
RATIONAL_B_SPLINE_SURFACE(((0.991593692313266,0.991593692313266,0.991593692313266,
0.994659131878645,1.,0.999181998279397,0.998417372792936),(0.991593692313266,
0.991593692313266,0.991593692313266,0.994659131878645,1.,0.999181998279397,
0.998417372792936)))
REPRESENTATION_ITEM('')
SURFACE()
);
#3126=(
BOUNDED_SURFACE()
B_SPLINE_SURFACE(1,2,((#147368,#147369,#147370,#147371,#147372),(#147373,
#147374,#147375,#147376,#147377)),.UNSPECIFIED.,.F.,.F.,.F.)
B_SPLINE_SURFACE_WITH_KNOTS((2,2),(3,2,3),(0.70972998337526,1.),(0.159799014184269,
0.176967058622924,0.177555991090998),.UNSPECIFIED.)
GEOMETRIC_REPRESENTATION_ITEM()
RATIONAL_B_SPLINE_SURFACE(((0.990927469170722,0.987759962570787,0.98748925405691,
0.98748925405691,0.98748925405691),(0.990927469170722,0.987759962570787,
0.98748925405691,0.98748925405691,0.98748925405691)))
REPRESENTATION_ITEM('')
SURFACE()
);
#3127=(
BOUNDED_SURFACE()
B_SPLINE_SURFACE(1,2,((#147379,#147380,#147381,#147382,#147383,#147384,
#147385),(#147386,#147387,#147388,#147389,#147390,#147391,#147392)),
 .UNSPECIFIED.,.F.,.F.,.F.)
B_SPLINE_SURFACE_WITH_KNOTS((2,2),(3,2,2,3),(0.71019295900844,1.),(0.55603736126532,
0.556212823028862,0.571428571428571,0.573758999383058),.UNSPECIFIED.)
GEOMETRIC_REPRESENTATION_ITEM()
RATIONAL_B_SPLINE_SURFACE(((0.991593692313266,0.991593692313266,0.991593692313266,
0.994659131878645,1.,0.999181998279397,0.998417372792936),(0.991593692313266,
0.991593692313266,0.991593692313266,0.994659131878645,1.,0.999181998279397,
0.998417372792936)))
REPRESENTATION_ITEM('')
SURFACE()
);
#3128=(
BOUNDED_SURFACE()
B_SPLINE_SURFACE(1,2,((#147409,#147410,#147411,#147412,#147413),(#147414,
#147415,#147416,#147417,#147418)),.UNSPECIFIED.,.F.,.F.,.F.)
B_SPLINE_SURFACE_WITH_KNOTS((2,2),(3,2,3),(0.70972998336251,1.),(0.159799014184269,
0.176967058622924,0.177555991103904),.UNSPECIFIED.)
GEOMETRIC_REPRESENTATION_ITEM()
RATIONAL_B_SPLINE_SURFACE(((0.990927469170722,0.987759962570787,0.98748925405691,
0.98748925405691,0.98748925405691),(0.990927469170722,0.987759962570787,
0.98748925405691,0.98748925405691,0.98748925405691)))
REPRESENTATION_ITEM('')
SURFACE()
);
#3129=(
BOUNDED_SURFACE()
B_SPLINE_SURFACE(1,2,((#147420,#147421,#147422,#147423,#147424,#147425,
#147426),(#147427,#147428,#147429,#147430,#147431,#147432,#147433)),
 .UNSPECIFIED.,.F.,.F.,.F.)
B_SPLINE_SURFACE_WITH_KNOTS((2,2),(3,2,2,3),(0.710192959008445,1.),(0.55603736126532,
0.556212823028862,0.571428571428571,0.573758999383058),.UNSPECIFIED.)
GEOMETRIC_REPRESENTATION_ITEM()
RATIONAL_B_SPLINE_SURFACE(((0.991593692313266,0.991593692313266,0.991593692313266,
0.994659131878645,1.,0.999181998279397,0.998417372792936),(0.991593692313266,
0.991593692313266,0.991593692313266,0.994659131878645,1.,0.999181998279397,
0.998417372792936)))
REPRESENTATION_ITEM('')
SURFACE()
);
#3130=(
BOUNDED_SURFACE()
B_SPLINE_SURFACE(1,2,((#147455,#147456,#147457,#147458,#147459),(#147460,
#147461,#147462,#147463,#147464)),.UNSPECIFIED.,.F.,.F.,.F.)
B_SPLINE_SURFACE_WITH_KNOTS((2,2),(3,2,3),(0.709729983362568,1.),(0.159799014184268,
0.176967058622924,0.177555991103127),.UNSPECIFIED.)
GEOMETRIC_REPRESENTATION_ITEM()
RATIONAL_B_SPLINE_SURFACE(((0.990927469170722,0.987759962570787,0.98748925405691,
0.98748925405691,0.98748925405691),(0.990927469170722,0.987759962570787,
0.98748925405691,0.98748925405691,0.98748925405691)))
REPRESENTATION_ITEM('')
SURFACE()
);
#3131=(
BOUNDED_SURFACE()
B_SPLINE_SURFACE(1,2,((#147466,#147467,#147468,#147469,#147470,#147471,
#147472),(#147473,#147474,#147475,#147476,#147477,#147478,#147479)),
 .UNSPECIFIED.,.F.,.F.,.F.)
B_SPLINE_SURFACE_WITH_KNOTS((2,2),(3,2,2,3),(0.71019295900844,1.),(0.55603736126532,
0.556212823028862,0.571428571428571,0.573758999383058),.UNSPECIFIED.)
GEOMETRIC_REPRESENTATION_ITEM()
RATIONAL_B_SPLINE_SURFACE(((0.991593692313266,0.991593692313266,0.991593692313266,
0.994659131878645,1.,0.999181998279397,0.998417372792936),(0.991593692313266,
0.991593692313266,0.991593692313266,0.994659131878645,1.,0.999181998279397,
0.998417372792936)))
REPRESENTATION_ITEM('')
SURFACE()
);
#3132=(
BOUNDED_SURFACE()
B_SPLINE_SURFACE(1,2,((#147505,#147506,#147507,#147508,#147509),(#147510,
#147511,#147512,#147513,#147514)),.UNSPECIFIED.,.F.,.F.,.F.)
B_SPLINE_SURFACE_WITH_KNOTS((2,2),(3,2,3),(0.709729983342911,1.),(0.159799014184268,
0.176967058622921,0.177555991081652),.UNSPECIFIED.)
GEOMETRIC_REPRESENTATION_ITEM()
RATIONAL_B_SPLINE_SURFACE(((0.990927469170722,0.987759962570787,0.98748925405691,
0.98748925405691,0.98748925405691),(0.990927469170722,0.987759962570787,
0.98748925405691,0.98748925405691,0.98748925405691)))
REPRESENTATION_ITEM('')
SURFACE()
);
#3133=(
BOUNDED_SURFACE()
B_SPLINE_SURFACE(1,2,((#147516,#147517,#147518,#147519,#147520,#147521,
#147522),(#147523,#147524,#147525,#147526,#147527,#147528,#147529)),
 .UNSPECIFIED.,.F.,.F.,.F.)
B_SPLINE_SURFACE_WITH_KNOTS((2,2),(3,2,2,3),(0.710192959008303,1.),(0.55603736126532,
0.556212823028862,0.571428571428571,0.573758999383056),.UNSPECIFIED.)
GEOMETRIC_REPRESENTATION_ITEM()
RATIONAL_B_SPLINE_SURFACE(((0.991593692313266,0.991593692313266,0.991593692313266,
0.994659131878645,1.,0.999181998279397,0.998417372792937),(0.991593692313266,
0.991593692313266,0.991593692313266,0.994659131878645,1.,0.999181998279397,
0.998417372792937)))
REPRESENTATION_ITEM('')
SURFACE()
);
#3134=(
BOUNDED_SURFACE()
B_SPLINE_SURFACE(1,2,((#147551,#147552,#147553,#147554,#147555),(#147556,
#147557,#147558,#147559,#147560)),.UNSPECIFIED.,.F.,.F.,.F.)
B_SPLINE_SURFACE_WITH_KNOTS((2,2),(3,2,3),(0.709729983351992,1.),(0.159799014184233,
0.176967058622922,0.177555991114115),.UNSPECIFIED.)
GEOMETRIC_REPRESENTATION_ITEM()
RATIONAL_B_SPLINE_SURFACE(((0.990927469170735,0.987759962570788,0.98748925405691,
0.98748925405691,0.98748925405691),(0.990927469170735,0.987759962570788,
0.98748925405691,0.98748925405691,0.98748925405691)))
REPRESENTATION_ITEM('')
SURFACE()
);
#3135=(
BOUNDED_SURFACE()
B_SPLINE_SURFACE(1,2,((#147562,#147563,#147564,#147565,#147566,#147567,
#147568),(#147569,#147570,#147571,#147572,#147573,#147574,#147575)),
 .UNSPECIFIED.,.F.,.F.,.F.)
B_SPLINE_SURFACE_WITH_KNOTS((2,2),(3,2,2,3),(0.710192959008295,1.),(0.556037361265319,
0.556212823028861,0.571428571428571,0.573758999383057),.UNSPECIFIED.)
GEOMETRIC_REPRESENTATION_ITEM()
RATIONAL_B_SPLINE_SURFACE(((0.991593692313265,0.991593692313265,0.991593692313265,
0.994659131878645,1.,0.999181998279397,0.998417372792936),(0.991593692313265,
0.991593692313265,0.991593692313265,0.994659131878644,1.,0.999181998279397,
0.998417372792936)))
REPRESENTATION_ITEM('')
SURFACE()
);
#3136=(
BOUNDED_SURFACE()
B_SPLINE_SURFACE(1,2,((#147597,#147598,#147599,#147600,#147601),(#147602,
#147603,#147604,#147605,#147606)),.UNSPECIFIED.,.F.,.F.,.F.)
B_SPLINE_SURFACE_WITH_KNOTS((2,2),(3,2,3),(0.709729983356803,1.),(0.159799014184073,
0.176967058622922,0.177555991109014),.UNSPECIFIED.)
GEOMETRIC_REPRESENTATION_ITEM()
RATIONAL_B_SPLINE_SURFACE(((0.990927469170794,0.98775996257079,0.98748925405691,
0.98748925405691,0.98748925405691),(0.990927469170794,0.98775996257079,
0.98748925405691,0.98748925405691,0.98748925405691)))
REPRESENTATION_ITEM('')
SURFACE()
);
#3137=(
BOUNDED_SURFACE()
B_SPLINE_SURFACE(1,2,((#147608,#147609,#147610,#147611,#147612,#147613,
#147614),(#147615,#147616,#147617,#147618,#147619,#147620,#147621)),
 .UNSPECIFIED.,.F.,.F.,.F.)
B_SPLINE_SURFACE_WITH_KNOTS((2,2),(3,2,2,3),(0.710192959008051,1.),(0.556037361265319,
0.556212823028861,0.571428571428571,0.573758999383057),.UNSPECIFIED.)
GEOMETRIC_REPRESENTATION_ITEM()
RATIONAL_B_SPLINE_SURFACE(((0.991593692313265,0.991593692313265,0.991593692313265,
0.994659131878644,1.,0.999181998279397,0.998417372792936),(0.991593692313265,
0.991593692313265,0.991593692313265,0.994659131878644,1.,0.999181998279397,
0.998417372792936)))
REPRESENTATION_ITEM('')
SURFACE()
);
#3138=(
BOUNDED_SURFACE()
B_SPLINE_SURFACE(1,2,((#147647,#147648,#147649,#147650,#147651),(#147652,
#147653,#147654,#147655,#147656)),.UNSPECIFIED.,.F.,.F.,.F.)
B_SPLINE_SURFACE_WITH_KNOTS((2,2),(3,2,3),(0.709729983383856,1.),(0.159799014184014,
0.176967058622925,0.177555991081937),.UNSPECIFIED.)
GEOMETRIC_REPRESENTATION_ITEM()
RATIONAL_B_SPLINE_SURFACE(((0.990927469170816,0.98775996257079,0.98748925405691,
0.98748925405691,0.98748925405691),(0.990927469170816,0.987759962570791,
0.98748925405691,0.98748925405691,0.98748925405691)))
REPRESENTATION_ITEM('')
SURFACE()
);
#3139=(
BOUNDED_SURFACE()
B_SPLINE_SURFACE(1,2,((#147658,#147659,#147660,#147661,#147662,#147663,
#147664),(#147665,#147666,#147667,#147668,#147669,#147670,#147671)),
 .UNSPECIFIED.,.F.,.F.,.F.)
B_SPLINE_SURFACE_WITH_KNOTS((2,2),(3,2,2,3),(0.710192959006645,1.),(0.556037361265319,
0.556212823028861,0.571428571428571,0.573758999383057),.UNSPECIFIED.)
GEOMETRIC_REPRESENTATION_ITEM()
RATIONAL_B_SPLINE_SURFACE(((0.991593692313265,0.991593692313265,0.991593692313265,
0.994659131878645,1.,0.999181998279397,0.998417372792936),(0.991593692313265,
0.991593692313265,0.991593692313265,0.994659131878645,1.,0.999181998279397,
0.998417372792936)))
REPRESENTATION_ITEM('')
SURFACE()
);
#3140=(
BOUNDED_SURFACE()
B_SPLINE_SURFACE(1,2,((#147693,#147694,#147695,#147696,#147697),(#147698,
#147699,#147700,#147701,#147702)),.UNSPECIFIED.,.F.,.F.,.F.)
B_SPLINE_SURFACE_WITH_KNOTS((2,2),(3,2,3),(0.709729983386952,1.),(0.15979901418427,
0.176967058622922,0.177555991076872),.UNSPECIFIED.)
GEOMETRIC_REPRESENTATION_ITEM()
RATIONAL_B_SPLINE_SURFACE(((0.990927469170722,0.987759962570787,0.98748925405691,
0.98748925405691,0.98748925405691),(0.990927469170722,0.987759962570787,
0.98748925405691,0.98748925405691,0.98748925405691)))
REPRESENTATION_ITEM('')
SURFACE()
);
#3141=(
BOUNDED_SURFACE()
B_SPLINE_SURFACE(1,2,((#147704,#147705,#147706,#147707,#147708,#147709,
#147710),(#147711,#147712,#147713,#147714,#147715,#147716,#147717)),
 .UNSPECIFIED.,.F.,.F.,.F.)
B_SPLINE_SURFACE_WITH_KNOTS((2,2),(3,2,2,3),(0.710192959007974,1.),(0.556037361265319,
0.556212823028861,0.571428571428571,0.573758999383056),.UNSPECIFIED.)
GEOMETRIC_REPRESENTATION_ITEM()
RATIONAL_B_SPLINE_SURFACE(((0.991593692313265,0.991593692313265,0.991593692313265,
0.994659131878644,1.,0.999181998279397,0.998417372792936),(0.991593692313265,
0.991593692313265,0.991593692313265,0.994659131878644,1.,0.999181998279397,
0.998417372792936)))
REPRESENTATION_ITEM('')
SURFACE()
);
#3142=(
BOUNDED_SURFACE()
B_SPLINE_SURFACE(1,2,((#147743,#147744,#147745,#147746,#147747),(#147748,
#147749,#147750,#147751,#147752)),.UNSPECIFIED.,.F.,.F.,.F.)
B_SPLINE_SURFACE_WITH_KNOTS((2,2),(3,2,3),(0.709729983394837,1.),(0.159799014184242,
0.176967058622922,0.177555991070855),.UNSPECIFIED.)
GEOMETRIC_REPRESENTATION_ITEM()
RATIONAL_B_SPLINE_SURFACE(((0.990927469170732,0.987759962570788,0.98748925405691,
0.98748925405691,0.98748925405691),(0.990927469170732,0.987759962570788,
0.98748925405691,0.98748925405691,0.98748925405691)))
REPRESENTATION_ITEM('')
SURFACE()
);
#3143=(
BOUNDED_SURFACE()
B_SPLINE_SURFACE(1,2,((#147754,#147755,#147756,#147757,#147758,#147759,
#147760),(#147761,#147762,#147763,#147764,#147765,#147766,#147767)),
 .UNSPECIFIED.,.F.,.F.,.F.)
B_SPLINE_SURFACE_WITH_KNOTS((2,2),(3,2,2,3),(0.710192959008354,1.),(0.556037361265319,
0.556212823028861,0.571428571428571,0.573758999383057),.UNSPECIFIED.)
GEOMETRIC_REPRESENTATION_ITEM()
RATIONAL_B_SPLINE_SURFACE(((0.991593692313265,0.991593692313265,0.991593692313265,
0.994659131878645,1.,0.999181998279397,0.998417372792936),(0.991593692313265,
0.991593692313265,0.991593692313265,0.994659131878645,1.,0.999181998279397,
0.998417372792936)))
REPRESENTATION_ITEM('')
SURFACE()
);
#3144=(
BOUNDED_SURFACE()
B_SPLINE_SURFACE(1,2,((#147792,#147793,#147794,#147795,#147796),(#147797,
#147798,#147799,#147800,#147801)),.UNSPECIFIED.,.F.,.F.,.F.)
B_SPLINE_SURFACE_WITH_KNOTS((2,2),(3,2,3),(0.70972998337482,1.),(0.15979901418427,
0.176967058622925,0.177555991090709),.UNSPECIFIED.)
GEOMETRIC_REPRESENTATION_ITEM()
RATIONAL_B_SPLINE_SURFACE(((0.990927469170721,0.987759962570786,0.98748925405691,
0.98748925405691,0.98748925405691),(0.990927469170722,0.987759962570787,
0.98748925405691,0.98748925405691,0.98748925405691)))
REPRESENTATION_ITEM('')
SURFACE()
);
#3145=(
BOUNDED_SURFACE()
B_SPLINE_SURFACE(1,2,((#147803,#147804,#147805,#147806,#147807,#147808,
#147809),(#147810,#147811,#147812,#147813,#147814,#147815,#147816)),
 .UNSPECIFIED.,.F.,.F.,.F.)
B_SPLINE_SURFACE_WITH_KNOTS((2,2),(3,2,2,3),(0.710192959008358,1.),(0.556037361265319,
0.556212823028861,0.571428571428571,0.573758999383057),.UNSPECIFIED.)
GEOMETRIC_REPRESENTATION_ITEM()
RATIONAL_B_SPLINE_SURFACE(((0.991593692313265,0.991593692313265,0.991593692313265,
0.994659131878645,1.,0.999181998279397,0.998417372792936),(0.991593692313265,
0.991593692313265,0.991593692313265,0.994659131878645,1.,0.999181998279397,
0.998417372792936)))
REPRESENTATION_ITEM('')
SURFACE()
);
#3146=(
BOUNDED_SURFACE()
B_SPLINE_SURFACE(1,2,((#147842,#147843,#147844,#147845,#147846),(#147847,
#147848,#147849,#147850,#147851)),.UNSPECIFIED.,.F.,.F.,.F.)
B_SPLINE_SURFACE_WITH_KNOTS((2,2),(3,2,3),(0.709729983387421,1.),(0.15979901418427,
0.176967058622922,0.177555991078557),.UNSPECIFIED.)
GEOMETRIC_REPRESENTATION_ITEM()
RATIONAL_B_SPLINE_SURFACE(((0.990927469170721,0.987759962570787,0.98748925405691,
0.98748925405691,0.98748925405691),(0.990927469170721,0.987759962570787,
0.98748925405691,0.98748925405691,0.98748925405691)))
REPRESENTATION_ITEM('')
SURFACE()
);
#3147=(
BOUNDED_SURFACE()
B_SPLINE_SURFACE(1,2,((#147853,#147854,#147855,#147856,#147857,#147858,
#147859),(#147860,#147861,#147862,#147863,#147864,#147865,#147866)),
 .UNSPECIFIED.,.F.,.F.,.F.)
B_SPLINE_SURFACE_WITH_KNOTS((2,2),(3,2,2,3),(0.710192959008366,1.),(0.556037361265319,
0.556212823028861,0.571428571428571,0.573758999383057),.UNSPECIFIED.)
GEOMETRIC_REPRESENTATION_ITEM()
RATIONAL_B_SPLINE_SURFACE(((0.991593692313265,0.991593692313265,0.991593692313265,
0.994659131878644,1.,0.999181998279397,0.998417372792936),(0.991593692313265,
0.991593692313265,0.991593692313265,0.994659131878644,1.,0.999181998279397,
0.998417372792936)))
REPRESENTATION_ITEM('')
SURFACE()
);
#3148=(
BOUNDED_SURFACE()
B_SPLINE_SURFACE(1,2,((#147888,#147889,#147890,#147891,#147892),(#147893,
#147894,#147895,#147896,#147897)),.UNSPECIFIED.,.F.,.F.,.F.)
B_SPLINE_SURFACE_WITH_KNOTS((2,2),(3,2,3),(0.709729983360727,1.),(0.159799014183978,
0.176967058622922,0.177555991105049),.UNSPECIFIED.)
GEOMETRIC_REPRESENTATION_ITEM()
RATIONAL_B_SPLINE_SURFACE(((0.990927469170829,0.987759962570792,0.98748925405691,
0.98748925405691,0.98748925405691),(0.990927469170829,0.987759962570792,
0.98748925405691,0.98748925405691,0.98748925405691)))
REPRESENTATION_ITEM('')
SURFACE()
);
#3149=(
BOUNDED_SURFACE()
B_SPLINE_SURFACE(1,2,((#147899,#147900,#147901,#147902,#147903,#147904,
#147905),(#147906,#147907,#147908,#147909,#147910,#147911,#147912)),
 .UNSPECIFIED.,.F.,.F.,.F.)
B_SPLINE_SURFACE_WITH_KNOTS((2,2),(3,2,2,3),(0.710192959008086,1.),(0.556037361265319,
0.556212823028861,0.571428571428571,0.573758999383056),.UNSPECIFIED.)
GEOMETRIC_REPRESENTATION_ITEM()
RATIONAL_B_SPLINE_SURFACE(((0.991593692313265,0.991593692313265,0.991593692313265,
0.994659131878644,1.,0.999181998279397,0.998417372792937),(0.991593692313265,
0.991593692313265,0.991593692313265,0.994659131878644,1.,0.999181998279397,
0.998417372792937)))
REPRESENTATION_ITEM('')
SURFACE()
);
#3150=(
BOUNDED_SURFACE()
B_SPLINE_SURFACE(1,2,((#147938,#147939,#147940,#147941,#147942),(#147943,
#147944,#147945,#147946,#147947)),.UNSPECIFIED.,.F.,.F.,.F.)
B_SPLINE_SURFACE_WITH_KNOTS((2,2),(3,2,3),(0.709729983386537,1.),(0.159799014184215,
0.176967058622925,0.177555991079593),.UNSPECIFIED.)
GEOMETRIC_REPRESENTATION_ITEM()
RATIONAL_B_SPLINE_SURFACE(((0.990927469170742,0.987759962570788,0.98748925405691,
0.98748925405691,0.98748925405691),(0.990927469170742,0.987759962570788,
0.98748925405691,0.98748925405691,0.98748925405691)))
REPRESENTATION_ITEM('')
SURFACE()
);
#3151=(
BOUNDED_SURFACE()
B_SPLINE_SURFACE(1,2,((#147949,#147950,#147951,#147952,#147953,#147954,
#147955),(#147956,#147957,#147958,#147959,#147960,#147961,#147962)),
 .UNSPECIFIED.,.F.,.F.,.F.)
B_SPLINE_SURFACE_WITH_KNOTS((2,2),(3,2,2,3),(0.710192959008437,1.),(0.556037361265319,
0.556212823028861,0.571428571428571,0.573758999383056),.UNSPECIFIED.)
GEOMETRIC_REPRESENTATION_ITEM()
RATIONAL_B_SPLINE_SURFACE(((0.991593692313265,0.991593692313265,0.991593692313265,
0.994659131878644,1.,0.999181998279397,0.998417372792936),(0.991593692313265,
0.991593692313265,0.991593692313265,0.994659131878644,1.,0.999181998279397,
0.998417372792936)))
REPRESENTATION_ITEM('')
SURFACE()
);
#3152=(
BOUNDED_SURFACE()
B_SPLINE_SURFACE(1,2,((#147977,#147978,#147979),(#147980,#147981,#147982)),
 .UNSPECIFIED.,.F.,.F.,.F.)
B_SPLINE_SURFACE_WITH_KNOTS((2,2),(3,3),(0.,0.289807040992016),(0.607982157956011,
0.625273655815328),.UNSPECIFIED.)
GEOMETRIC_REPRESENTATION_ITEM()
RATIONAL_B_SPLINE_SURFACE(((0.987470879370255,0.987613514606721,0.990694758798812),
(0.987470879370255,0.987613514606721,0.990694758798812)))
REPRESENTATION_ITEM('')
SURFACE()
);
#3153=(
BOUNDED_SURFACE()
B_SPLINE_SURFACE(1,2,((#147991,#147992,#147993,#147994,#147995),(#147996,
#147997,#147998,#147999,#148000)),.UNSPECIFIED.,.F.,.F.,.F.)
B_SPLINE_SURFACE_WITH_KNOTS((2,2),(3,2,3),(0.,0.290280981347481),(0.107879027750091,
0.125170525609409,0.125770422812313),.UNSPECIFIED.)
GEOMETRIC_REPRESENTATION_ITEM()
RATIONAL_B_SPLINE_SURFACE(((0.987469282487682,0.987594391229382,0.990658108926709,
0.990658108926709,0.990658108926709),(0.987469282487682,0.987594391229382,
0.990658108926709,0.990658108926709,0.990658108926709)))
REPRESENTATION_ITEM('')
SURFACE()
);
#3154=(
BOUNDED_SURFACE()
B_SPLINE_SURFACE(1,2,((#148009,#148010,#148011),(#148012,#148013,#148014)),
 .UNSPECIFIED.,.F.,.F.,.F.)
B_SPLINE_SURFACE_WITH_KNOTS((2,2),(3,3),(0.,0.289807040992005),(0.607982157956011,
0.625273655815328),.UNSPECIFIED.)
GEOMETRIC_REPRESENTATION_ITEM()
RATIONAL_B_SPLINE_SURFACE(((0.987470879370255,0.98761351460672,0.990694758798812),
(0.987470879370256,0.987613514606721,0.990694758798812)))
REPRESENTATION_ITEM('')
SURFACE()
);
#3155=(
BOUNDED_SURFACE()
B_SPLINE_SURFACE(1,2,((#148016,#148017,#148018,#148019,#148020),(#148021,
#148022,#148023,#148024,#148025)),.UNSPECIFIED.,.F.,.F.,.F.)
B_SPLINE_SURFACE_WITH_KNOTS((2,2),(3,2,3),(0.,0.290280981348683),(0.107879027750092,
0.125170525609408,0.125770422854449),.UNSPECIFIED.)
GEOMETRIC_REPRESENTATION_ITEM()
RATIONAL_B_SPLINE_SURFACE(((0.987469282487682,0.987594391229382,0.990658108926709,
0.990658108926709,0.990658108926709),(0.987469282487682,0.987594391229382,
0.990658108926709,0.990658108926709,0.990658108926709)))
REPRESENTATION_ITEM('')
SURFACE()
);
#3156=(
BOUNDED_SURFACE()
B_SPLINE_SURFACE(1,2,((#148034,#148035,#148036),(#148037,#148038,#148039)),
 .UNSPECIFIED.,.F.,.F.,.F.)
B_SPLINE_SURFACE_WITH_KNOTS((2,2),(3,3),(0.,0.289807040991657),(0.607982157956011,
0.625273655815328),.UNSPECIFIED.)
GEOMETRIC_REPRESENTATION_ITEM()
RATIONAL_B_SPLINE_SURFACE(((0.987470879370255,0.98761351460672,0.990694758798812),
(0.987470879370256,0.987613514606721,0.990694758798812)))
REPRESENTATION_ITEM('')
SURFACE()
);
#3157=(
BOUNDED_SURFACE()
B_SPLINE_SURFACE(1,2,((#148041,#148042,#148043,#148044,#148045),(#148046,
#148047,#148048,#148049,#148050)),.UNSPECIFIED.,.F.,.F.,.F.)
B_SPLINE_SURFACE_WITH_KNOTS((2,2),(3,2,3),(0.,0.290280981345748),(0.107879027750092,
0.125170525609409,0.125770422850796),.UNSPECIFIED.)
GEOMETRIC_REPRESENTATION_ITEM()
RATIONAL_B_SPLINE_SURFACE(((0.987469282487682,0.987594391229382,0.990658108926709,
0.990658108926709,0.990658108926709),(0.987469282487682,0.987594391229382,
0.990658108926709,0.990658108926709,0.990658108926709)))
REPRESENTATION_ITEM('')
SURFACE()
);
#3158=(
BOUNDED_SURFACE()
B_SPLINE_SURFACE(1,2,((#148059,#148060,#148061),(#148062,#148063,#148064)),
 .UNSPECIFIED.,.F.,.F.,.F.)
B_SPLINE_SURFACE_WITH_KNOTS((2,2),(3,3),(0.,0.289807040991666),(0.607982157956011,
0.625273655815328),.UNSPECIFIED.)
GEOMETRIC_REPRESENTATION_ITEM()
RATIONAL_B_SPLINE_SURFACE(((0.987470879370255,0.98761351460672,0.990694758798812),
(0.987470879370256,0.987613514606721,0.990694758798812)))
REPRESENTATION_ITEM('')
SURFACE()
);
#3159=(
BOUNDED_SURFACE()
B_SPLINE_SURFACE(1,2,((#148066,#148067,#148068,#148069,#148070),(#148071,
#148072,#148073,#148074,#148075)),.UNSPECIFIED.,.F.,.F.,.F.)
B_SPLINE_SURFACE_WITH_KNOTS((2,2),(3,2,3),(0.,0.290280981338847),(0.107879027750092,
0.125170525609409,0.125770422803681),.UNSPECIFIED.)
GEOMETRIC_REPRESENTATION_ITEM()
RATIONAL_B_SPLINE_SURFACE(((0.987469282487682,0.987594391229382,0.990658108926709,
0.990658108926709,0.990658108926709),(0.987469282487682,0.987594391229382,
0.990658108926709,0.990658108926709,0.990658108926709)))
REPRESENTATION_ITEM('')
SURFACE()
);
#3160=(
BOUNDED_SURFACE()
B_SPLINE_SURFACE(1,2,((#148084,#148085,#148086),(#148087,#148088,#148089)),
 .UNSPECIFIED.,.F.,.F.,.F.)
B_SPLINE_SURFACE_WITH_KNOTS((2,2),(3,3),(0.,0.289807040992623),(0.607982157956011,
0.625273655815328),.UNSPECIFIED.)
GEOMETRIC_REPRESENTATION_ITEM()
RATIONAL_B_SPLINE_SURFACE(((0.987470879370255,0.98761351460672,0.990694758798812),
(0.987470879370256,0.987613514606721,0.990694758798812)))
REPRESENTATION_ITEM('')
SURFACE()
);
#3161=(
BOUNDED_SURFACE()
B_SPLINE_SURFACE(1,2,((#148091,#148092,#148093,#148094,#148095),(#148096,
#148097,#148098,#148099,#148100)),.UNSPECIFIED.,.F.,.F.,.F.)
B_SPLINE_SURFACE_WITH_KNOTS((2,2),(3,2,3),(0.,0.29028098133501),(0.107879027750092,
0.125170525609408,0.125770422799848),.UNSPECIFIED.)
GEOMETRIC_REPRESENTATION_ITEM()
RATIONAL_B_SPLINE_SURFACE(((0.987469282487682,0.987594391229382,0.990658108926709,
0.990658108926709,0.990658108926709),(0.987469282487682,0.987594391229382,
0.990658108926709,0.990658108926709,0.990658108926709)))
REPRESENTATION_ITEM('')
SURFACE()
);
#3162=(
BOUNDED_SURFACE()
B_SPLINE_SURFACE(1,2,((#148109,#148110,#148111),(#148112,#148113,#148114)),
 .UNSPECIFIED.,.F.,.F.,.F.)
B_SPLINE_SURFACE_WITH_KNOTS((2,2),(3,3),(0.,0.289807040992625),(0.607982157956011,
0.625273655815328),.UNSPECIFIED.)
GEOMETRIC_REPRESENTATION_ITEM()
RATIONAL_B_SPLINE_SURFACE(((0.987470879370255,0.98761351460672,0.990694758798812),
(0.987470879370255,0.987613514606721,0.990694758798812)))
REPRESENTATION_ITEM('')
SURFACE()
);
#3163=(
BOUNDED_SURFACE()
B_SPLINE_SURFACE(1,2,((#148116,#148117,#148118,#148119,#148120),(#148121,
#148122,#148123,#148124,#148125)),.UNSPECIFIED.,.F.,.F.,.F.)
B_SPLINE_SURFACE_WITH_KNOTS((2,2),(3,2,3),(0.,0.290280981347237),(0.107879027750092,
0.125170525609408,0.125770422812067),.UNSPECIFIED.)
GEOMETRIC_REPRESENTATION_ITEM()
RATIONAL_B_SPLINE_SURFACE(((0.987469282487682,0.987594391229382,0.990658108926709,
0.990658108926709,0.990658108926709),(0.987469282487682,0.987594391229382,
0.990658108926709,0.990658108926709,0.990658108926709)))
REPRESENTATION_ITEM('')
SURFACE()
);
#3164=(
BOUNDED_SURFACE()
B_SPLINE_SURFACE(1,2,((#148134,#148135,#148136),(#148137,#148138,#148139)),
 .UNSPECIFIED.,.F.,.F.,.F.)
B_SPLINE_SURFACE_WITH_KNOTS((2,2),(3,3),(0.,0.28980704099262),(0.607982157956011,
0.625273655815328),.UNSPECIFIED.)
GEOMETRIC_REPRESENTATION_ITEM()
RATIONAL_B_SPLINE_SURFACE(((0.987470879370255,0.98761351460672,0.990694758798812),
(0.987470879370255,0.98761351460672,0.990694758798812)))
REPRESENTATION_ITEM('')
SURFACE()
);
#3165=(
BOUNDED_SURFACE()
B_SPLINE_SURFACE(1,2,((#148141,#148142,#148143,#148144,#148145),(#148146,
#148147,#148148,#148149,#148150)),.UNSPECIFIED.,.F.,.F.,.F.)
B_SPLINE_SURFACE_WITH_KNOTS((2,2),(3,2,3),(0.,0.290280981331832),(0.107879027750092,
0.125170525609408,0.125770422796665),.UNSPECIFIED.)
GEOMETRIC_REPRESENTATION_ITEM()
RATIONAL_B_SPLINE_SURFACE(((0.987469282487682,0.987594391229382,0.990658108926709,
0.990658108926709,0.990658108926709),(0.987469282487682,0.987594391229382,
0.990658108926709,0.990658108926709,0.990658108926709)))
REPRESENTATION_ITEM('')
SURFACE()
);
#3166=(
BOUNDED_SURFACE()
B_SPLINE_SURFACE(1,2,((#148159,#148160,#148161),(#148162,#148163,#148164)),
 .UNSPECIFIED.,.F.,.F.,.F.)
B_SPLINE_SURFACE_WITH_KNOTS((2,2),(3,3),(0.,0.289807040993203),(0.607982157956011,
0.625273655815328),.UNSPECIFIED.)
GEOMETRIC_REPRESENTATION_ITEM()
RATIONAL_B_SPLINE_SURFACE(((0.987470879370255,0.98761351460672,0.990694758798812),
(0.987470879370255,0.98761351460672,0.990694758798812)))
REPRESENTATION_ITEM('')
SURFACE()
);
#3167=(
BOUNDED_SURFACE()
B_SPLINE_SURFACE(1,2,((#148166,#148167,#148168,#148169,#148170),(#148171,
#148172,#148173,#148174,#148175)),.UNSPECIFIED.,.F.,.F.,.F.)
B_SPLINE_SURFACE_WITH_KNOTS((2,2),(3,2,3),(0.,0.290280981329886),(0.107879027750092,
0.125170525609408,0.125770422835485),.UNSPECIFIED.)
GEOMETRIC_REPRESENTATION_ITEM()
RATIONAL_B_SPLINE_SURFACE(((0.987469282487682,0.987594391229382,0.990658108926709,
0.990658108926709,0.990658108926709),(0.987469282487682,0.987594391229382,
0.990658108926709,0.990658108926709,0.990658108926709)))
REPRESENTATION_ITEM('')
SURFACE()
);
#3168=(
BOUNDED_SURFACE()
B_SPLINE_SURFACE(1,2,((#148184,#148185,#148186),(#148187,#148188,#148189)),
 .UNSPECIFIED.,.F.,.F.,.F.)
B_SPLINE_SURFACE_WITH_KNOTS((2,2),(3,3),(0.,0.289807040992614),(0.607982157956011,
0.625273655815328),.UNSPECIFIED.)
GEOMETRIC_REPRESENTATION_ITEM()
RATIONAL_B_SPLINE_SURFACE(((0.987470879370255,0.98761351460672,0.990694758798812),
(0.987470879370255,0.98761351460672,0.990694758798812)))
REPRESENTATION_ITEM('')
SURFACE()
);
#3169=(
BOUNDED_SURFACE()
B_SPLINE_SURFACE(1,2,((#148191,#148192,#148193,#148194,#148195),(#148196,
#148197,#148198,#148199,#148200)),.UNSPECIFIED.,.F.,.F.,.F.)
B_SPLINE_SURFACE_WITH_KNOTS((2,2),(3,2,3),(0.,0.290280981327799),(0.107879027750091,
0.125170525609408,0.125770422833613),.UNSPECIFIED.)
GEOMETRIC_REPRESENTATION_ITEM()
RATIONAL_B_SPLINE_SURFACE(((0.987469282487682,0.987594391229382,0.990658108926709,
0.990658108926709,0.990658108926709),(0.987469282487682,0.987594391229382,
0.990658108926709,0.990658108926709,0.990658108926709)))
REPRESENTATION_ITEM('')
SURFACE()
);
#3170=(
BOUNDED_SURFACE()
B_SPLINE_SURFACE(1,2,((#148209,#148210,#148211),(#148212,#148213,#148214)),
 .UNSPECIFIED.,.F.,.F.,.F.)
B_SPLINE_SURFACE_WITH_KNOTS((2,2),(3,3),(0.,0.289807040993169),(0.607982157956011,
0.625273655815328),.UNSPECIFIED.)
GEOMETRIC_REPRESENTATION_ITEM()
RATIONAL_B_SPLINE_SURFACE(((0.987470879370255,0.98761351460672,0.990694758798812),
(0.987470879370255,0.98761351460672,0.990694758798812)))
REPRESENTATION_ITEM('')
SURFACE()
);
#3171=(
BOUNDED_SURFACE()
B_SPLINE_SURFACE(1,2,((#148216,#148217,#148218,#148219,#148220),(#148221,
#148222,#148223,#148224,#148225)),.UNSPECIFIED.,.F.,.F.,.F.)
B_SPLINE_SURFACE_WITH_KNOTS((2,2),(3,2,3),(0.,0.290280981354195),(0.107879027750092,
0.125170525609409,0.125770422859419),.UNSPECIFIED.)
GEOMETRIC_REPRESENTATION_ITEM()
RATIONAL_B_SPLINE_SURFACE(((0.987469282487682,0.987594391229382,0.990658108926709,
0.990658108926709,0.990658108926709),(0.987469282487682,0.987594391229382,
0.990658108926709,0.990658108926709,0.990658108926709)))
REPRESENTATION_ITEM('')
SURFACE()
);
#3172=(
BOUNDED_SURFACE()
B_SPLINE_SURFACE(1,2,((#148234,#148235,#148236),(#148237,#148238,#148239)),
 .UNSPECIFIED.,.F.,.F.,.F.)
B_SPLINE_SURFACE_WITH_KNOTS((2,2),(3,3),(0.,0.289807040992984),(0.607982157956012,
0.625273655815328),.UNSPECIFIED.)
GEOMETRIC_REPRESENTATION_ITEM()
RATIONAL_B_SPLINE_SURFACE(((0.987470879370255,0.987613514606721,0.990694758798812),
(0.987470879370255,0.987613514606721,0.990694758798812)))
REPRESENTATION_ITEM('')
SURFACE()
);
#3173=(
BOUNDED_SURFACE()
B_SPLINE_SURFACE(1,2,((#148241,#148242,#148243,#148244,#148245),(#148246,
#148247,#148248,#148249,#148250)),.UNSPECIFIED.,.F.,.F.,.F.)
B_SPLINE_SURFACE_WITH_KNOTS((2,2),(3,2,3),(0.,0.290280981333798),(0.10787902775009,
0.125170525609407,0.125770422839726),.UNSPECIFIED.)
GEOMETRIC_REPRESENTATION_ITEM()
RATIONAL_B_SPLINE_SURFACE(((0.987469282487682,0.987594391229382,0.990658108926708,
0.990658108926708,0.990658108926708),(0.987469282487682,0.987594391229382,
0.990658108926708,0.990658108926708,0.990658108926708)))
REPRESENTATION_ITEM('')
SURFACE()
);
#3174=(
BOUNDED_SURFACE()
B_SPLINE_SURFACE(1,2,((#148259,#148260,#148261),(#148262,#148263,#148264)),
 .UNSPECIFIED.,.F.,.F.,.F.)
B_SPLINE_SURFACE_WITH_KNOTS((2,2),(3,3),(0.,0.289807040993017),(0.607982157956012,
0.625273655815329),.UNSPECIFIED.)
GEOMETRIC_REPRESENTATION_ITEM()
RATIONAL_B_SPLINE_SURFACE(((0.987470879370255,0.987613514606721,0.990694758798813),
(0.987470879370255,0.987613514606721,0.990694758798813)))
REPRESENTATION_ITEM('')
SURFACE()
);
#3175=(
BOUNDED_SURFACE()
B_SPLINE_SURFACE(1,2,((#148266,#148267,#148268,#148269,#148270),(#148271,
#148272,#148273,#148274,#148275)),.UNSPECIFIED.,.F.,.F.,.F.)
B_SPLINE_SURFACE_WITH_KNOTS((2,2),(3,2,3),(0.,0.290280981342294),(0.10787902775009,
0.125170525609407,0.125770422807127),.UNSPECIFIED.)
GEOMETRIC_REPRESENTATION_ITEM()
RATIONAL_B_SPLINE_SURFACE(((0.987469282487682,0.987594391229382,0.990658108926708,
0.990658108926708,0.990658108926708),(0.987469282487682,0.987594391229382,
0.990658108926708,0.990658108926708,0.990658108926708)))
REPRESENTATION_ITEM('')
SURFACE()
);
#3176=(
BOUNDED_SURFACE()
B_SPLINE_SURFACE(1,2,((#148284,#148285,#148286),(#148287,#148288,#148289)),
 .UNSPECIFIED.,.F.,.F.,.F.)
B_SPLINE_SURFACE_WITH_KNOTS((2,2),(3,3),(0.,0.289807040993289),(0.607982157956012,
0.625273655815329),.UNSPECIFIED.)
GEOMETRIC_REPRESENTATION_ITEM()
RATIONAL_B_SPLINE_SURFACE(((0.987470879370255,0.987613514606721,0.990694758798813),
(0.987470879370255,0.987613514606721,0.990694758798813)))
REPRESENTATION_ITEM('')
SURFACE()
);
#3177=(
BOUNDED_SURFACE()
B_SPLINE_SURFACE(1,2,((#148291,#148292,#148293,#148294,#148295),(#148296,
#148297,#148298,#148299,#148300)),.UNSPECIFIED.,.F.,.F.,.F.)
B_SPLINE_SURFACE_WITH_KNOTS((2,2),(3,2,3),(0.,0.290280981336171),(0.10787902775009,
0.125170525609407,0.125770422841787),.UNSPECIFIED.)
GEOMETRIC_REPRESENTATION_ITEM()
RATIONAL_B_SPLINE_SURFACE(((0.987469282487682,0.987594391229382,0.990658108926709,
0.990658108926709,0.990658108926709),(0.987469282487682,0.987594391229382,
0.990658108926709,0.990658108926709,0.990658108926709)))
REPRESENTATION_ITEM('')
SURFACE()
);
#3178=(
BOUNDED_SURFACE()
B_SPLINE_SURFACE(1,2,((#148309,#148310,#148311),(#148312,#148313,#148314)),
 .UNSPECIFIED.,.F.,.F.,.F.)
B_SPLINE_SURFACE_WITH_KNOTS((2,2),(3,3),(0.,0.28980704099271),(0.607982157956012,
0.625273655815329),.UNSPECIFIED.)
GEOMETRIC_REPRESENTATION_ITEM()
RATIONAL_B_SPLINE_SURFACE(((0.987470879370255,0.987613514606721,0.990694758798813),
(0.987470879370255,0.987613514606721,0.990694758798813)))
REPRESENTATION_ITEM('')
SURFACE()
);
#3179=(
BOUNDED_SURFACE()
B_SPLINE_SURFACE(1,2,((#148316,#148317,#148318,#148319,#148320),(#148321,
#148322,#148323,#148324,#148325)),.UNSPECIFIED.,.F.,.F.,.F.)
B_SPLINE_SURFACE_WITH_KNOTS((2,2),(3,2,3),(0.,0.290280981341405),(0.10787902775009,
0.125170525609408,0.125770422806235),.UNSPECIFIED.)
GEOMETRIC_REPRESENTATION_ITEM()
RATIONAL_B_SPLINE_SURFACE(((0.987469282487682,0.987594391229382,0.990658108926709,
0.990658108926709,0.990658108926709),(0.987469282487682,0.987594391229382,
0.990658108926709,0.990658108926709,0.990658108926709)))
REPRESENTATION_ITEM('')
SURFACE()
);
#3180=(
BOUNDED_SURFACE()
B_SPLINE_SURFACE(1,2,((#148334,#148335,#148336),(#148337,#148338,#148339)),
 .UNSPECIFIED.,.F.,.F.,.F.)
B_SPLINE_SURFACE_WITH_KNOTS((2,2),(3,3),(0.,0.289807040993545),(0.607982157956012,
0.625273655815329),.UNSPECIFIED.)
GEOMETRIC_REPRESENTATION_ITEM()
RATIONAL_B_SPLINE_SURFACE(((0.987470879370255,0.987613514606721,0.990694758798813),
(0.987470879370255,0.987613514606721,0.990694758798813)))
REPRESENTATION_ITEM('')
SURFACE()
);
#3181=(
BOUNDED_SURFACE()
B_SPLINE_SURFACE(1,2,((#148341,#148342,#148343,#148344,#148345),(#148346,
#148347,#148348,#148349,#148350)),.UNSPECIFIED.,.F.,.F.,.F.)
B_SPLINE_SURFACE_WITH_KNOTS((2,2),(3,2,3),(0.,0.29028098133396),(0.107879027750091,
0.125170525609408,0.125770422798795),.UNSPECIFIED.)
GEOMETRIC_REPRESENTATION_ITEM()
RATIONAL_B_SPLINE_SURFACE(((0.987469282487682,0.987594391229382,0.990658108926709,
0.990658108926709,0.990658108926709),(0.987469282487682,0.987594391229382,
0.990658108926709,0.990658108926709,0.990658108926709)))
REPRESENTATION_ITEM('')
SURFACE()
);
#3182=(
BOUNDED_SURFACE()
B_SPLINE_SURFACE(1,2,((#148359,#148360,#148361),(#148362,#148363,#148364)),
 .UNSPECIFIED.,.F.,.F.,.F.)
B_SPLINE_SURFACE_WITH_KNOTS((2,2),(3,3),(0.,0.289807040993042),(0.607982157956012,
0.625273655815329),.UNSPECIFIED.)
GEOMETRIC_REPRESENTATION_ITEM()
RATIONAL_B_SPLINE_SURFACE(((0.987470879370255,0.987613514606721,0.990694758798813),
(0.987470879370255,0.987613514606721,0.990694758798813)))
REPRESENTATION_ITEM('')
SURFACE()
);
#3183=(
BOUNDED_SURFACE()
B_SPLINE_SURFACE(1,2,((#148366,#148367,#148368,#148369,#148370),(#148371,
#148372,#148373,#148374,#148375)),.UNSPECIFIED.,.F.,.F.,.F.)
B_SPLINE_SURFACE_WITH_KNOTS((2,2),(3,2,3),(0.,0.290280981332549),(0.10787902775009,
0.125170525609408,0.125770422838297),.UNSPECIFIED.)
GEOMETRIC_REPRESENTATION_ITEM()
RATIONAL_B_SPLINE_SURFACE(((0.987469282487682,0.987594391229382,0.990658108926708,
0.990658108926708,0.990658108926708),(0.987469282487682,0.987594391229382,
0.990658108926708,0.990658108926708,0.990658108926708)))
REPRESENTATION_ITEM('')
SURFACE()
);
#3184=(
BOUNDED_SURFACE()
B_SPLINE_SURFACE(1,2,((#148384,#148385,#148386),(#148387,#148388,#148389)),
 .UNSPECIFIED.,.F.,.F.,.F.)
B_SPLINE_SURFACE_WITH_KNOTS((2,2),(3,3),(0.,0.289807040993511),(0.607982157956012,
0.625273655815329),.UNSPECIFIED.)
GEOMETRIC_REPRESENTATION_ITEM()
RATIONAL_B_SPLINE_SURFACE(((0.987470879370255,0.987613514606721,0.990694758798813),
(0.987470879370255,0.987613514606721,0.990694758798813)))
REPRESENTATION_ITEM('')
SURFACE()
);
#3185=(
BOUNDED_SURFACE()
B_SPLINE_SURFACE(1,2,((#148391,#148392,#148393,#148394,#148395),(#148396,
#148397,#148398,#148399,#148400)),.UNSPECIFIED.,.F.,.F.,.F.)
B_SPLINE_SURFACE_WITH_KNOTS((2,2),(3,2,3),(0.,0.290280981335985),(0.10787902775009,
0.125170525609407,0.125770422841674),.UNSPECIFIED.)
GEOMETRIC_REPRESENTATION_ITEM()
RATIONAL_B_SPLINE_SURFACE(((0.987469282487682,0.987594391229382,0.990658108926709,
0.990658108926709,0.990658108926709),(0.987469282487682,0.987594391229382,
0.990658108926709,0.990658108926709,0.990658108926709)))
REPRESENTATION_ITEM('')
SURFACE()
);
#3186=(
BOUNDED_SURFACE()
B_SPLINE_SURFACE(1,2,((#148409,#148410,#148411),(#148412,#148413,#148414)),
 .UNSPECIFIED.,.F.,.F.,.F.)
B_SPLINE_SURFACE_WITH_KNOTS((2,2),(3,3),(0.,0.289807040993257),(0.607982157956012,
0.625273655815329),.UNSPECIFIED.)
GEOMETRIC_REPRESENTATION_ITEM()
RATIONAL_B_SPLINE_SURFACE(((0.987470879370255,0.987613514606721,0.990694758798813),
(0.987470879370255,0.987613514606721,0.990694758798813)))
REPRESENTATION_ITEM('')
SURFACE()
);
#3187=(
BOUNDED_SURFACE()
B_SPLINE_SURFACE(1,2,((#148416,#148417,#148418,#148419,#148420),(#148421,
#148422,#148423,#148424,#148425)),.UNSPECIFIED.,.F.,.F.,.F.)
B_SPLINE_SURFACE_WITH_KNOTS((2,2),(3,2,3),(0.,0.290280981317335),(0.10787902775009,
0.125170525609407,0.125770422823056),.UNSPECIFIED.)
GEOMETRIC_REPRESENTATION_ITEM()
RATIONAL_B_SPLINE_SURFACE(((0.987469282487682,0.987594391229382,0.990658108926708,
0.990658108926708,0.990658108926708),(0.987469282487682,0.987594391229382,
0.990658108926708,0.990658108926708,0.990658108926708)))
REPRESENTATION_ITEM('')
SURFACE()
);
#3188=(
BOUNDED_SURFACE()
B_SPLINE_SURFACE(1,2,((#148434,#148435,#148436),(#148437,#148438,#148439)),
 .UNSPECIFIED.,.F.,.F.,.F.)
B_SPLINE_SURFACE_WITH_KNOTS((2,2),(3,3),(0.,0.289807040994421),(0.607982157956012,
0.625273655815329),.UNSPECIFIED.)
GEOMETRIC_REPRESENTATION_ITEM()
RATIONAL_B_SPLINE_SURFACE(((0.987470879370255,0.987613514606721,0.990694758798813),
(0.987470879370255,0.987613514606721,0.990694758798813)))
REPRESENTATION_ITEM('')
SURFACE()
);
#3189=(
BOUNDED_SURFACE()
B_SPLINE_SURFACE(1,2,((#148441,#148442,#148443,#148444,#148445),(#148446,
#148447,#148448,#148449,#148450)),.UNSPECIFIED.,.F.,.F.,.F.)
B_SPLINE_SURFACE_WITH_KNOTS((2,2),(3,2,3),(0.,0.290280981346559),(0.10787902775009,
0.125170525609407,0.125770422811388),.UNSPECIFIED.)
GEOMETRIC_REPRESENTATION_ITEM()
RATIONAL_B_SPLINE_SURFACE(((0.987469282487682,0.987594391229382,0.990658108926708,
0.990658108926708,0.990658108926708),(0.987469282487682,0.987594391229382,
0.990658108926708,0.990658108926708,0.990658108926708)))
REPRESENTATION_ITEM('')
SURFACE()
);
#3190=(
BOUNDED_SURFACE()
B_SPLINE_SURFACE(1,2,((#148459,#148460,#148461),(#148462,#148463,#148464)),
 .UNSPECIFIED.,.F.,.F.,.F.)
B_SPLINE_SURFACE_WITH_KNOTS((2,2),(3,3),(0.,0.28980704099276),(0.607982157956012,
0.625273655815329),.UNSPECIFIED.)
GEOMETRIC_REPRESENTATION_ITEM()
RATIONAL_B_SPLINE_SURFACE(((0.987470879370255,0.987613514606721,0.990694758798813),
(0.987470879370255,0.987613514606721,0.990694758798813)))
REPRESENTATION_ITEM('')
SURFACE()
);
#3191=(
BOUNDED_SURFACE()
B_SPLINE_SURFACE(1,2,((#148466,#148467,#148468,#148469,#148470),(#148471,
#148472,#148473,#148474,#148475)),.UNSPECIFIED.,.F.,.F.,.F.)
B_SPLINE_SURFACE_WITH_KNOTS((2,2),(3,2,3),(0.,0.29028098134186),(0.10787902775009,
0.125170525609407,0.125770422847784),.UNSPECIFIED.)
GEOMETRIC_REPRESENTATION_ITEM()
RATIONAL_B_SPLINE_SURFACE(((0.987469282487682,0.987594391229382,0.990658108926708,
0.990658108926708,0.990658108926708),(0.987469282487682,0.987594391229382,
0.990658108926708,0.990658108926708,0.990658108926708)))
REPRESENTATION_ITEM('')
SURFACE()
);
#3192=(
BOUNDED_SURFACE()
B_SPLINE_SURFACE(1,2,((#148484,#148485,#148486),(#148487,#148488,#148489)),
 .UNSPECIFIED.,.F.,.F.,.F.)
B_SPLINE_SURFACE_WITH_KNOTS((2,2),(3,3),(0.,0.289807040992648),(0.607982157956012,
0.625273655815329),.UNSPECIFIED.)
GEOMETRIC_REPRESENTATION_ITEM()
RATIONAL_B_SPLINE_SURFACE(((0.987470879370255,0.987613514606721,0.990694758798813),
(0.987470879370255,0.987613514606721,0.990694758798813)))
REPRESENTATION_ITEM('')
SURFACE()
);
#3193=(
BOUNDED_SURFACE()
B_SPLINE_SURFACE(1,2,((#148491,#148492,#148493,#148494,#148495),(#148496,
#148497,#148498,#148499,#148500)),.UNSPECIFIED.,.F.,.F.,.F.)
B_SPLINE_SURFACE_WITH_KNOTS((2,2),(3,2,3),(0.,0.290280981333718),(0.107879027750091,
0.125170525609407,0.12577042279855),.UNSPECIFIED.)
GEOMETRIC_REPRESENTATION_ITEM()
RATIONAL_B_SPLINE_SURFACE(((0.987469282487682,0.987594391229382,0.990658108926708,
0.990658108926708,0.990658108926708),(0.987469282487682,0.987594391229382,
0.990658108926708,0.990658108926708,0.990658108926708)))
REPRESENTATION_ITEM('')
SURFACE()
);
#3194=(
BOUNDED_SURFACE()
B_SPLINE_SURFACE(1,2,((#148509,#148510,#148511),(#148512,#148513,#148514)),
 .UNSPECIFIED.,.F.,.F.,.F.)
B_SPLINE_SURFACE_WITH_KNOTS((2,2),(3,3),(0.,0.289807040993488),(0.607982157956012,
0.625273655815329),.UNSPECIFIED.)
GEOMETRIC_REPRESENTATION_ITEM()
RATIONAL_B_SPLINE_SURFACE(((0.987470879370255,0.987613514606721,0.990694758798813),
(0.987470879370255,0.987613514606721,0.990694758798813)))
REPRESENTATION_ITEM('')
SURFACE()
);
#3195=(
BOUNDED_SURFACE()
B_SPLINE_SURFACE(1,2,((#148516,#148517,#148518,#148519,#148520),(#148521,
#148522,#148523,#148524,#148525)),.UNSPECIFIED.,.F.,.F.,.F.)
B_SPLINE_SURFACE_WITH_KNOTS((2,2),(3,2,3),(0.,0.290280981329807),(0.107879027750091,
0.125170525609407,0.125770422794629),.UNSPECIFIED.)
GEOMETRIC_REPRESENTATION_ITEM()
RATIONAL_B_SPLINE_SURFACE(((0.987469282487682,0.987594391229382,0.990658108926708,
0.990658108926708,0.990658108926708),(0.987469282487682,0.987594391229382,
0.990658108926708,0.990658108926708,0.990658108926708)))
REPRESENTATION_ITEM('')
SURFACE()
);
#3196=(
BOUNDED_SURFACE()
B_SPLINE_SURFACE(1,2,((#148534,#148535,#148536),(#148537,#148538,#148539)),
 .UNSPECIFIED.,.F.,.F.,.F.)
B_SPLINE_SURFACE_WITH_KNOTS((2,2),(3,3),(0.,0.289807040992018),(0.607982157956012,
0.62527365581533),.UNSPECIFIED.)
GEOMETRIC_REPRESENTATION_ITEM()
RATIONAL_B_SPLINE_SURFACE(((0.987470879370255,0.987613514606721,0.990694758798813),
(0.987470879370255,0.987613514606721,0.990694758798813)))
REPRESENTATION_ITEM('')
SURFACE()
);
#3197=(
BOUNDED_SURFACE()
B_SPLINE_SURFACE(1,2,((#148541,#148542,#148543,#148544,#148545),(#148546,
#148547,#148548,#148549,#148550)),.UNSPECIFIED.,.F.,.F.,.F.)
B_SPLINE_SURFACE_WITH_KNOTS((2,2),(3,2,3),(0.,0.290280981334961),(0.10787902775009,
0.125170525609412,0.125770422840683),.UNSPECIFIED.)
GEOMETRIC_REPRESENTATION_ITEM()
RATIONAL_B_SPLINE_SURFACE(((0.987469282487682,0.987594391229382,0.99065810892671,
0.99065810892671,0.99065810892671),(0.987469282487682,0.987594391229382,
0.99065810892671,0.99065810892671,0.99065810892671)))
REPRESENTATION_ITEM('')
SURFACE()
);
#3198=(
BOUNDED_SURFACE()
B_SPLINE_SURFACE(1,2,((#148559,#148560,#148561),(#148562,#148563,#148564)),
 .UNSPECIFIED.,.F.,.F.,.F.)
B_SPLINE_SURFACE_WITH_KNOTS((2,2),(3,3),(0.,0.289807040992891),(0.607982157956012,
0.625273655815329),.UNSPECIFIED.)
GEOMETRIC_REPRESENTATION_ITEM()
RATIONAL_B_SPLINE_SURFACE(((0.987470879370255,0.987613514606721,0.990694758798813),
(0.987470879370255,0.987613514606721,0.990694758798813)))
REPRESENTATION_ITEM('')
SURFACE()
);
#3199=(
BOUNDED_SURFACE()
B_SPLINE_SURFACE(1,2,((#148566,#148567,#148568,#148569,#148570),(#148571,
#148572,#148573,#148574,#148575)),.UNSPECIFIED.,.F.,.F.,.F.)
B_SPLINE_SURFACE_WITH_KNOTS((2,2),(3,2,3),(0.,0.290280981350767),(0.10787902775009,
0.125170525609407,0.125770422856224),.UNSPECIFIED.)
GEOMETRIC_REPRESENTATION_ITEM()
RATIONAL_B_SPLINE_SURFACE(((0.987469282487682,0.987594391229382,0.990658108926708,
0.990658108926708,0.990658108926708),(0.987469282487682,0.987594391229382,
0.990658108926708,0.990658108926708,0.990658108926708)))
REPRESENTATION_ITEM('')
SURFACE()
);
#3200=(
BOUNDED_SURFACE()
B_SPLINE_SURFACE(1,2,((#148584,#148585,#148586),(#148587,#148588,#148589)),
 .UNSPECIFIED.,.F.,.F.,.F.)
B_SPLINE_SURFACE_WITH_KNOTS((2,2),(3,3),(0.,0.289807040992687),(0.607982157956012,
0.625273655815329),.UNSPECIFIED.)
GEOMETRIC_REPRESENTATION_ITEM()
RATIONAL_B_SPLINE_SURFACE(((0.987470879370255,0.987613514606721,0.990694758798813),
(0.987470879370255,0.987613514606721,0.990694758798813)))
REPRESENTATION_ITEM('')
SURFACE()
);
#3201=(
BOUNDED_SURFACE()
B_SPLINE_SURFACE(1,2,((#148591,#148592,#148593,#148594,#148595),(#148596,
#148597,#148598,#148599,#148600)),.UNSPECIFIED.,.F.,.F.,.F.)
B_SPLINE_SURFACE_WITH_KNOTS((2,2),(3,2,3),(0.,0.290280981338245),(0.107879027750092,
0.125170525609407,0.125770422843646),.UNSPECIFIED.)
GEOMETRIC_REPRESENTATION_ITEM()
RATIONAL_B_SPLINE_SURFACE(((0.987469282487682,0.987594391229382,0.990658108926709,
0.990658108926709,0.990658108926709),(0.987469282487682,0.987594391229382,
0.990658108926709,0.990658108926709,0.990658108926709)))
REPRESENTATION_ITEM('')
SURFACE()
);
#3202=(
BOUNDED_SURFACE()
B_SPLINE_SURFACE(1,2,((#148609,#148610,#148611),(#148612,#148613,#148614)),
 .UNSPECIFIED.,.F.,.F.,.F.)
B_SPLINE_SURFACE_WITH_KNOTS((2,2),(3,3),(0.,0.28980704099156),(0.607982157956011,
0.625273655815328),.UNSPECIFIED.)
GEOMETRIC_REPRESENTATION_ITEM()
RATIONAL_B_SPLINE_SURFACE(((0.987470879370255,0.98761351460672,0.990694758798812),
(0.987470879370256,0.987613514606721,0.990694758798812)))
REPRESENTATION_ITEM('')
SURFACE()
);
#3203=(
BOUNDED_SURFACE()
B_SPLINE_SURFACE(1,2,((#148616,#148617,#148618,#148619,#148620),(#148621,
#148622,#148623,#148624,#148625)),.UNSPECIFIED.,.F.,.F.,.F.)
B_SPLINE_SURFACE_WITH_KNOTS((2,2),(3,2,3),(0.,0.290280981347015),(0.107879027750092,
0.125170525609408,0.125770422811853),.UNSPECIFIED.)
GEOMETRIC_REPRESENTATION_ITEM()
RATIONAL_B_SPLINE_SURFACE(((0.987469282487682,0.987594391229382,0.990658108926709,
0.990658108926709,0.990658108926709),(0.987469282487682,0.987594391229382,
0.990658108926709,0.990658108926709,0.990658108926709)))
REPRESENTATION_ITEM('')
SURFACE()
);
#3204=(
BOUNDED_SURFACE()
B_SPLINE_SURFACE(1,2,((#148634,#148635,#148636),(#148637,#148638,#148639)),
 .UNSPECIFIED.,.F.,.F.,.F.)
B_SPLINE_SURFACE_WITH_KNOTS((2,2),(3,3),(0.,0.289807040991555),(0.607982157956011,
0.625273655815328),.UNSPECIFIED.)
GEOMETRIC_REPRESENTATION_ITEM()
RATIONAL_B_SPLINE_SURFACE(((0.987470879370255,0.98761351460672,0.990694758798812),
(0.987470879370255,0.98761351460672,0.990694758798812)))
REPRESENTATION_ITEM('')
SURFACE()
);
#3205=(
BOUNDED_SURFACE()
B_SPLINE_SURFACE(1,2,((#148641,#148642,#148643,#148644,#148645),(#148646,
#148647,#148648,#148649,#148650)),.UNSPECIFIED.,.F.,.F.,.F.)
B_SPLINE_SURFACE_WITH_KNOTS((2,2),(3,2,3),(0.,0.29028098134296),(0.107879027750092,
0.125170525609409,0.125770422807798),.UNSPECIFIED.)
GEOMETRIC_REPRESENTATION_ITEM()
RATIONAL_B_SPLINE_SURFACE(((0.987469282487682,0.987594391229382,0.990658108926709,
0.990658108926709,0.990658108926709),(0.987469282487682,0.987594391229382,
0.990658108926709,0.990658108926709,0.990658108926709)))
REPRESENTATION_ITEM('')
SURFACE()
);
#3206=(
BOUNDED_SURFACE()
B_SPLINE_SURFACE(1,2,((#148659,#148660,#148661),(#148662,#148663,#148664)),
 .UNSPECIFIED.,.F.,.F.,.F.)
B_SPLINE_SURFACE_WITH_KNOTS((2,2),(3,3),(0.,0.28980704099156),(0.607982157956011,
0.625273655815328),.UNSPECIFIED.)
GEOMETRIC_REPRESENTATION_ITEM()
RATIONAL_B_SPLINE_SURFACE(((0.987470879370255,0.98761351460672,0.990694758798812),
(0.987470879370256,0.987613514606721,0.990694758798812)))
REPRESENTATION_ITEM('')
SURFACE()
);
#3207=(
BOUNDED_SURFACE()
B_SPLINE_SURFACE(1,2,((#148666,#148667,#148668,#148669,#148670),(#148671,
#148672,#148673,#148674,#148675)),.UNSPECIFIED.,.F.,.F.,.F.)
B_SPLINE_SURFACE_WITH_KNOTS((2,2),(3,2,3),(0.,0.290280981340027),(0.107879027750092,
0.125170525609409,0.125770422804864),.UNSPECIFIED.)
GEOMETRIC_REPRESENTATION_ITEM()
RATIONAL_B_SPLINE_SURFACE(((0.987469282487682,0.987594391229382,0.990658108926709,
0.990658108926709,0.990658108926709),(0.987469282487682,0.987594391229382,
0.990658108926709,0.990658108926709,0.990658108926709)))
REPRESENTATION_ITEM('')
SURFACE()
);
#3208=(
BOUNDED_SURFACE()
B_SPLINE_SURFACE(1,2,((#148684,#148685,#148686),(#148687,#148688,#148689)),
 .UNSPECIFIED.,.F.,.F.,.F.)
B_SPLINE_SURFACE_WITH_KNOTS((2,2),(3,3),(0.,0.289807040991888),(0.607982157956011,
0.625273655815328),.UNSPECIFIED.)
GEOMETRIC_REPRESENTATION_ITEM()
RATIONAL_B_SPLINE_SURFACE(((0.987470879370255,0.98761351460672,0.990694758798812),
(0.987470879370255,0.98761351460672,0.990694758798812)))
REPRESENTATION_ITEM('')
SURFACE()
);
#3209=(
BOUNDED_SURFACE()
B_SPLINE_SURFACE(1,2,((#148691,#148692,#148693,#148694,#148695),(#148696,
#148697,#148698,#148699,#148700)),.UNSPECIFIED.,.F.,.F.,.F.)
B_SPLINE_SURFACE_WITH_KNOTS((2,2),(3,2,3),(0.,0.290280981336771),(0.107879027750092,
0.125170525609409,0.125770422801606),.UNSPECIFIED.)
GEOMETRIC_REPRESENTATION_ITEM()
RATIONAL_B_SPLINE_SURFACE(((0.987469282487682,0.987594391229382,0.990658108926709,
0.990658108926709,0.990658108926709),(0.987469282487682,0.987594391229382,
0.990658108926709,0.990658108926709,0.990658108926709)))
REPRESENTATION_ITEM('')
SURFACE()
);
#3210=(
BOUNDED_SURFACE()
B_SPLINE_SURFACE(1,2,((#148702,#148703,#148704,#148705,#148706),(#148707,
#148708,#148709,#148710,#148711)),.UNSPECIFIED.,.F.,.F.,.F.)
B_SPLINE_SURFACE_WITH_KNOTS((2,2),(3,2,3),(0.,0.29039631629416),(0.159312132641873,
0.159901408087358,0.177069452526136),.UNSPECIFIED.)
GEOMETRIC_REPRESENTATION_ITEM()
RATIONAL_B_SPLINE_SURFACE(((0.990889788836329,0.990889788836329,0.990889788836329,
0.987739559362113,0.987486127973996),(0.990889788836329,0.990889788836329,
0.990889788836329,0.987739559362113,0.987486127973996)))
REPRESENTATION_ITEM('')
SURFACE()
);
#3211=(
BOUNDED_SURFACE()
B_SPLINE_SURFACE(1,2,((#148734,#148735,#148736,#148737,#148738),(#148739,
#148740,#148741,#148742,#148743)),.UNSPECIFIED.,.F.,.F.,.F.)
B_SPLINE_SURFACE_WITH_KNOTS((2,2),(3,2,3),(0.,0.28968108435992),(0.556108173865714,
0.571428571428571,0.57365435021991),.UNSPECIFIED.)
GEOMETRIC_REPRESENTATION_ITEM()
RATIONAL_B_SPLINE_SURFACE(((0.991551633675927,0.994622399056525,1.,0.999218731101516,
0.99848615229188),(0.991551633675927,0.994622399056525,1.,0.999218731101516,
0.99848615229188)))
REPRESENTATION_ITEM('')
SURFACE()
);
#3212=(
BOUNDED_SURFACE()
B_SPLINE_SURFACE(1,2,((#148745,#148746,#148747,#148748,#148749),(#148750,
#148751,#148752,#148753,#148754)),.UNSPECIFIED.,.F.,.F.,.F.)
B_SPLINE_SURFACE_WITH_KNOTS((2,2),(3,2,3),(0.,0.290396316319309),(0.159312132616718,
0.159901408087285,0.177069452526139),.UNSPECIFIED.)
GEOMETRIC_REPRESENTATION_ITEM()
RATIONAL_B_SPLINE_SURFACE(((0.990889788836356,0.990889788836356,0.990889788836356,
0.987739559362113,0.987486127973996),(0.990889788836356,0.990889788836356,
0.990889788836356,0.987739559362113,0.987486127973996)))
REPRESENTATION_ITEM('')
SURFACE()
);
#3213=(
BOUNDED_SURFACE()
B_SPLINE_SURFACE(1,2,((#148777,#148778,#148779,#148780,#148781),(#148782,
#148783,#148784,#148785,#148786)),.UNSPECIFIED.,.F.,.F.,.F.)
B_SPLINE_SURFACE_WITH_KNOTS((2,2),(3,2,3),(0.,0.289681084359924),(0.556108173865715,
0.571428571428571,0.57365435021991),.UNSPECIFIED.)
GEOMETRIC_REPRESENTATION_ITEM()
RATIONAL_B_SPLINE_SURFACE(((0.991551633675927,0.994622399056525,1.,0.999218731101516,
0.99848615229188),(0.991551633675927,0.994622399056525,1.,0.999218731101516,
0.99848615229188)))
REPRESENTATION_ITEM('')
SURFACE()
);
#3214=(
BOUNDED_SURFACE()
B_SPLINE_SURFACE(1,2,((#148788,#148789,#148790,#148791,#148792),(#148793,
#148794,#148795,#148796,#148797)),.UNSPECIFIED.,.F.,.F.,.F.)
B_SPLINE_SURFACE_WITH_KNOTS((2,2),(3,2,3),(0.,0.290396316297934),(0.159312132638105,
0.159901408087482,0.177069452526134),.UNSPECIFIED.)
GEOMETRIC_REPRESENTATION_ITEM()
RATIONAL_B_SPLINE_SURFACE(((0.990889788836284,0.990889788836284,0.990889788836284,
0.987739559362111,0.987486127973996),(0.990889788836283,0.990889788836283,
0.990889788836283,0.987739559362111,0.987486127973996)))
REPRESENTATION_ITEM('')
SURFACE()
);
#3215=(
BOUNDED_SURFACE()
B_SPLINE_SURFACE(1,2,((#148820,#148821,#148822,#148823,#148824),(#148825,
#148826,#148827,#148828,#148829)),.UNSPECIFIED.,.F.,.F.,.F.)
B_SPLINE_SURFACE_WITH_KNOTS((2,2),(3,2,3),(0.,0.289681084359914),(0.556108173865715,
0.571428571428571,0.573654350219911),.UNSPECIFIED.)
GEOMETRIC_REPRESENTATION_ITEM()
RATIONAL_B_SPLINE_SURFACE(((0.991551633675927,0.994622399056526,1.,0.999218731101516,
0.99848615229188),(0.991551633675927,0.994622399056526,1.,0.999218731101516,
0.99848615229188)))
REPRESENTATION_ITEM('')
SURFACE()
);
#3216=(
BOUNDED_SURFACE()
B_SPLINE_SURFACE(1,2,((#148831,#148832,#148833,#148834,#148835),(#148836,
#148837,#148838,#148839,#148840)),.UNSPECIFIED.,.F.,.F.,.F.)
B_SPLINE_SURFACE_WITH_KNOTS((2,2),(3,2,3),(0.,0.290396316309596),(0.159312132626429,
0.159901408087222,0.177069452526135),.UNSPECIFIED.)
GEOMETRIC_REPRESENTATION_ITEM()
RATIONAL_B_SPLINE_SURFACE(((0.990889788836379,0.990889788836379,0.990889788836379,
0.987739559362115,0.987486127973996),(0.990889788836379,0.990889788836379,
0.990889788836379,0.987739559362115,0.987486127973996)))
REPRESENTATION_ITEM('')
SURFACE()
);
#3217=(
BOUNDED_SURFACE()
B_SPLINE_SURFACE(1,2,((#148863,#148864,#148865,#148866,#148867),(#148868,
#148869,#148870,#148871,#148872)),.UNSPECIFIED.,.F.,.F.,.F.)
B_SPLINE_SURFACE_WITH_KNOTS((2,2),(3,2,3),(0.,0.289681084359931),(0.556108173865715,
0.571428571428571,0.573654350219911),.UNSPECIFIED.)
GEOMETRIC_REPRESENTATION_ITEM()
RATIONAL_B_SPLINE_SURFACE(((0.991551633675927,0.994622399056526,1.,0.999218731101516,
0.99848615229188),(0.991551633675927,0.994622399056526,1.,0.999218731101516,
0.99848615229188)))
REPRESENTATION_ITEM('')
SURFACE()
);
#3218=(
BOUNDED_SURFACE()
B_SPLINE_SURFACE(1,2,((#148874,#148875,#148876,#148877,#148878),(#148879,
#148880,#148881,#148882,#148883)),.UNSPECIFIED.,.F.,.F.,.F.)
B_SPLINE_SURFACE_WITH_KNOTS((2,2),(3,2,3),(0.,0.29039631632092),(0.159312132615108,
0.159901408087359,0.177069452526138),.UNSPECIFIED.)
GEOMETRIC_REPRESENTATION_ITEM()
RATIONAL_B_SPLINE_SURFACE(((0.990889788836329,0.990889788836329,0.990889788836329,
0.987739559362112,0.987486127973996),(0.990889788836329,0.990889788836329,
0.990889788836329,0.987739559362112,0.987486127973996)))
REPRESENTATION_ITEM('')
SURFACE()
);
#3219=(
BOUNDED_SURFACE()
B_SPLINE_SURFACE(1,2,((#148906,#148907,#148908,#148909,#148910),(#148911,
#148912,#148913,#148914,#148915)),.UNSPECIFIED.,.F.,.F.,.F.)
B_SPLINE_SURFACE_WITH_KNOTS((2,2),(3,2,3),(0.,0.289681084359921),(0.556108173865716,
0.571428571428571,0.573654350219911),.UNSPECIFIED.)
GEOMETRIC_REPRESENTATION_ITEM()
RATIONAL_B_SPLINE_SURFACE(((0.991551633675927,0.994622399056526,1.,0.999218731101516,
0.99848615229188),(0.991551633675927,0.994622399056526,1.,0.999218731101516,
0.99848615229188)))
REPRESENTATION_ITEM('')
SURFACE()
);
#3220=(
BOUNDED_SURFACE()
B_SPLINE_SURFACE(1,2,((#148917,#148918,#148919,#148920,#148921),(#148922,
#148923,#148924,#148925,#148926)),.UNSPECIFIED.,.F.,.F.,.F.)
B_SPLINE_SURFACE_WITH_KNOTS((2,2),(3,2,3),(0.,0.290396316312529),(0.159312132623513,
0.159901408087481,0.177069452526137),.UNSPECIFIED.)
GEOMETRIC_REPRESENTATION_ITEM()
RATIONAL_B_SPLINE_SURFACE(((0.990889788836284,0.990889788836284,0.990889788836284,
0.987739559362111,0.987486127973996),(0.990889788836284,0.990889788836284,
0.990889788836284,0.987739559362111,0.987486127973996)))
REPRESENTATION_ITEM('')
SURFACE()
);
#3221=(
BOUNDED_SURFACE()
B_SPLINE_SURFACE(1,2,((#148949,#148950,#148951,#148952,#148953),(#148954,
#148955,#148956,#148957,#148958)),.UNSPECIFIED.,.F.,.F.,.F.)
B_SPLINE_SURFACE_WITH_KNOTS((2,2),(3,2,3),(0.,0.289681084359925),(0.556108173865716,
0.571428571428571,0.573654350219911),.UNSPECIFIED.)
GEOMETRIC_REPRESENTATION_ITEM()
RATIONAL_B_SPLINE_SURFACE(((0.991551633675927,0.994622399056526,1.,0.999218731101516,
0.99848615229188),(0.991551633675927,0.994622399056526,1.,0.999218731101516,
0.99848615229188)))
REPRESENTATION_ITEM('')
SURFACE()
);
#3222=(
BOUNDED_SURFACE()
B_SPLINE_SURFACE(1,2,((#148960,#148961,#148962,#148963,#148964),(#148965,
#148966,#148967,#148968,#148969)),.UNSPECIFIED.,.F.,.F.,.F.)
B_SPLINE_SURFACE_WITH_KNOTS((2,2),(3,2,3),(0.,0.290396316323544),(0.159312132612491,
0.159901408087481,0.177069452526134),.UNSPECIFIED.)
GEOMETRIC_REPRESENTATION_ITEM()
RATIONAL_B_SPLINE_SURFACE(((0.990889788836284,0.990889788836284,0.990889788836284,
0.987739559362111,0.987486127973996),(0.990889788836284,0.990889788836284,
0.990889788836284,0.987739559362111,0.987486127973996)))
REPRESENTATION_ITEM('')
SURFACE()
);
#3223=(
BOUNDED_SURFACE()
B_SPLINE_SURFACE(1,2,((#148992,#148993,#148994,#148995,#148996),(#148997,
#148998,#148999,#149000,#149001)),.UNSPECIFIED.,.F.,.F.,.F.)
B_SPLINE_SURFACE_WITH_KNOTS((2,2),(3,2,3),(0.,0.289681084359926),(0.556108173865715,
0.571428571428571,0.573654350219911),.UNSPECIFIED.)
GEOMETRIC_REPRESENTATION_ITEM()
RATIONAL_B_SPLINE_SURFACE(((0.991551633675927,0.994622399056526,1.,0.999218731101516,
0.99848615229188),(0.991551633675927,0.994622399056526,1.,0.999218731101516,
0.99848615229188)))
REPRESENTATION_ITEM('')
SURFACE()
);
#3224=(
BOUNDED_SURFACE()
B_SPLINE_SURFACE(1,2,((#149003,#149004,#149005,#149006,#149007),(#149008,
#149009,#149010,#149011,#149012)),.UNSPECIFIED.,.F.,.F.,.F.)
B_SPLINE_SURFACE_WITH_KNOTS((2,2),(3,2,3),(0.,0.290396316297854),(0.159312132638184,
0.159901408087481,0.177069452526137),.UNSPECIFIED.)
GEOMETRIC_REPRESENTATION_ITEM()
RATIONAL_B_SPLINE_SURFACE(((0.990889788836284,0.990889788836284,0.990889788836284,
0.987739559362111,0.987486127973996),(0.990889788836284,0.990889788836284,
0.990889788836284,0.987739559362111,0.987486127973996)))
REPRESENTATION_ITEM('')
SURFACE()
);
#3225=(
BOUNDED_SURFACE()
B_SPLINE_SURFACE(1,2,((#149035,#149036,#149037,#149038,#149039),(#149040,
#149041,#149042,#149043,#149044)),.UNSPECIFIED.,.F.,.F.,.F.)
B_SPLINE_SURFACE_WITH_KNOTS((2,2),(3,2,3),(0.,0.289681084359916),(0.556108173865716,
0.571428571428571,0.573654350219911),.UNSPECIFIED.)
GEOMETRIC_REPRESENTATION_ITEM()
RATIONAL_B_SPLINE_SURFACE(((0.991551633675927,0.994622399056526,1.,0.999218731101516,
0.99848615229188),(0.991551633675927,0.994622399056526,1.,0.999218731101516,
0.99848615229188)))
REPRESENTATION_ITEM('')
SURFACE()
);
#3226=(
BOUNDED_SURFACE()
B_SPLINE_SURFACE(1,2,((#149046,#149047,#149048,#149049,#149050),(#149051,
#149052,#149053,#149054,#149055)),.UNSPECIFIED.,.F.,.F.,.F.)
B_SPLINE_SURFACE_WITH_KNOTS((2,2),(3,2,3),(0.,0.290396316321037),(0.159312132615002,
0.159901408087481,0.177069452526137),.UNSPECIFIED.)
GEOMETRIC_REPRESENTATION_ITEM()
RATIONAL_B_SPLINE_SURFACE(((0.990889788836284,0.990889788836284,0.990889788836284,
0.987739559362111,0.987486127973996),(0.990889788836284,0.990889788836284,
0.990889788836284,0.987739559362111,0.987486127973996)))
REPRESENTATION_ITEM('')
SURFACE()
);
#3227=(
BOUNDED_SURFACE()
B_SPLINE_SURFACE(1,2,((#149078,#149079,#149080,#149081,#149082),(#149083,
#149084,#149085,#149086,#149087)),.UNSPECIFIED.,.F.,.F.,.F.)
B_SPLINE_SURFACE_WITH_KNOTS((2,2),(3,2,3),(0.,0.289681084359916),(0.556108173865716,
0.571428571428571,0.573654350219911),.UNSPECIFIED.)
GEOMETRIC_REPRESENTATION_ITEM()
RATIONAL_B_SPLINE_SURFACE(((0.991551633675927,0.994622399056526,1.,0.999218731101516,
0.99848615229188),(0.991551633675927,0.994622399056526,1.,0.999218731101516,
0.99848615229188)))
REPRESENTATION_ITEM('')
SURFACE()
);
#3228=(
BOUNDED_SURFACE()
B_SPLINE_SURFACE(1,2,((#149089,#149090,#149091,#149092,#149093),(#149094,
#149095,#149096,#149097,#149098)),.UNSPECIFIED.,.F.,.F.,.F.)
B_SPLINE_SURFACE_WITH_KNOTS((2,2),(3,2,3),(0.,0.290396316329746),(0.159312132606293,
0.159901408087481,0.177069452526137),.UNSPECIFIED.)
GEOMETRIC_REPRESENTATION_ITEM()
RATIONAL_B_SPLINE_SURFACE(((0.990889788836284,0.990889788836284,0.990889788836284,
0.987739559362111,0.987486127973996),(0.990889788836284,0.990889788836284,
0.990889788836284,0.987739559362111,0.987486127973996)))
REPRESENTATION_ITEM('')
SURFACE()
);
#3229=(
BOUNDED_SURFACE()
B_SPLINE_SURFACE(1,2,((#149121,#149122,#149123,#149124,#149125),(#149126,
#149127,#149128,#149129,#149130)),.UNSPECIFIED.,.F.,.F.,.F.)
B_SPLINE_SURFACE_WITH_KNOTS((2,2),(3,2,3),(0.,0.289681084359916),(0.556108173865716,
0.571428571428571,0.573654350219912),.UNSPECIFIED.)
GEOMETRIC_REPRESENTATION_ITEM()
RATIONAL_B_SPLINE_SURFACE(((0.991551633675927,0.994622399056526,1.,0.999218731101516,
0.998486152291879),(0.991551633675927,0.994622399056526,1.,0.999218731101516,
0.998486152291879)))
REPRESENTATION_ITEM('')
SURFACE()
);
#3230=(
BOUNDED_SURFACE()
B_SPLINE_SURFACE(1,2,((#149132,#149133,#149134,#149135,#149136),(#149137,
#149138,#149139,#149140,#149141)),.UNSPECIFIED.,.F.,.F.,.F.)
B_SPLINE_SURFACE_WITH_KNOTS((2,2),(3,2,3),(0.,0.290396316316584),(0.15931213261945,
0.159901408087403,0.177069452526137),.UNSPECIFIED.)
GEOMETRIC_REPRESENTATION_ITEM()
RATIONAL_B_SPLINE_SURFACE(((0.990889788836313,0.990889788836313,0.990889788836313,
0.987739559362112,0.987486127973996),(0.990889788836313,0.990889788836313,
0.990889788836313,0.987739559362112,0.987486127973996)))
REPRESENTATION_ITEM('')
SURFACE()
);
#3231=(
BOUNDED_SURFACE()
B_SPLINE_SURFACE(1,2,((#149164,#149165,#149166,#149167,#149168),(#149169,
#149170,#149171,#149172,#149173)),.UNSPECIFIED.,.F.,.F.,.F.)
B_SPLINE_SURFACE_WITH_KNOTS((2,2),(3,2,3),(0.,0.289681084359918),(0.556108173865716,
0.571428571428571,0.573654350219911),.UNSPECIFIED.)
GEOMETRIC_REPRESENTATION_ITEM()
RATIONAL_B_SPLINE_SURFACE(((0.991551633675927,0.994622399056526,1.,0.999218731101516,
0.99848615229188),(0.991551633675927,0.994622399056526,1.,0.999218731101516,
0.99848615229188)))
REPRESENTATION_ITEM('')
SURFACE()
);
#3232=(
BOUNDED_SURFACE()
B_SPLINE_SURFACE(1,2,((#149175,#149176,#149177,#149178,#149179),(#149180,
#149181,#149182,#149183,#149184)),.UNSPECIFIED.,.F.,.F.,.F.)
B_SPLINE_SURFACE_WITH_KNOTS((2,2),(3,2,3),(0.,0.290396316309421),(0.159312132626621,
0.159901408087481,0.177069452526137),.UNSPECIFIED.)
GEOMETRIC_REPRESENTATION_ITEM()
RATIONAL_B_SPLINE_SURFACE(((0.990889788836284,0.990889788836284,0.990889788836284,
0.987739559362111,0.987486127973996),(0.990889788836284,0.990889788836284,
0.990889788836284,0.987739559362111,0.987486127973996)))
REPRESENTATION_ITEM('')
SURFACE()
);
#3233=(
BOUNDED_SURFACE()
B_SPLINE_SURFACE(1,2,((#149207,#149208,#149209,#149210,#149211),(#149212,
#149213,#149214,#149215,#149216)),.UNSPECIFIED.,.F.,.F.,.F.)
B_SPLINE_SURFACE_WITH_KNOTS((2,2),(3,2,3),(0.,0.28968108435992),(0.556108173865716,
0.571428571428571,0.573654350219911),.UNSPECIFIED.)
GEOMETRIC_REPRESENTATION_ITEM()
RATIONAL_B_SPLINE_SURFACE(((0.991551633675927,0.994622399056526,1.,0.999218731101516,
0.99848615229188),(0.991551633675927,0.994622399056526,1.,0.999218731101516,
0.99848615229188)))
REPRESENTATION_ITEM('')
SURFACE()
);
#3234=(
BOUNDED_SURFACE()
B_SPLINE_SURFACE(1,2,((#149218,#149219,#149220,#149221,#149222),(#149223,
#149224,#149225,#149226,#149227)),.UNSPECIFIED.,.F.,.F.,.F.)
B_SPLINE_SURFACE_WITH_KNOTS((2,2),(3,2,3),(0.,0.290396316330743),(0.159312132605295,
0.159901408087481,0.177069452526134),.UNSPECIFIED.)
GEOMETRIC_REPRESENTATION_ITEM()
RATIONAL_B_SPLINE_SURFACE(((0.990889788836284,0.990889788836284,0.990889788836284,
0.987739559362111,0.987486127973996),(0.990889788836284,0.990889788836284,
0.990889788836284,0.987739559362111,0.987486127973996)))
REPRESENTATION_ITEM('')
SURFACE()
);
#3235=(
BOUNDED_SURFACE()
B_SPLINE_SURFACE(1,2,((#149250,#149251,#149252,#149253,#149254),(#149255,
#149256,#149257,#149258,#149259)),.UNSPECIFIED.,.F.,.F.,.F.)
B_SPLINE_SURFACE_WITH_KNOTS((2,2),(3,2,3),(0.,0.28968108435992),(0.556108173865715,
0.571428571428571,0.573654350219911),.UNSPECIFIED.)
GEOMETRIC_REPRESENTATION_ITEM()
RATIONAL_B_SPLINE_SURFACE(((0.991551633675927,0.994622399056526,1.,0.999218731101516,
0.99848615229188),(0.991551633675927,0.994622399056526,1.,0.999218731101516,
0.99848615229188)))
REPRESENTATION_ITEM('')
SURFACE()
);
#3236=(
BOUNDED_SURFACE()
B_SPLINE_SURFACE(1,2,((#149261,#149262,#149263,#149264,#149265),(#149266,
#149267,#149268,#149269,#149270)),.UNSPECIFIED.,.F.,.F.,.F.)
B_SPLINE_SURFACE_WITH_KNOTS((2,2),(3,2,3),(0.,0.290396316298905),(0.159312132637135,
0.159901408087481,0.177069452526134),.UNSPECIFIED.)
GEOMETRIC_REPRESENTATION_ITEM()
RATIONAL_B_SPLINE_SURFACE(((0.990889788836284,0.990889788836284,0.990889788836284,
0.987739559362111,0.987486127973996),(0.990889788836284,0.990889788836284,
0.990889788836284,0.987739559362111,0.987486127973996)))
REPRESENTATION_ITEM('')
SURFACE()
);
#3237=(
BOUNDED_SURFACE()
B_SPLINE_SURFACE(1,2,((#149293,#149294,#149295,#149296,#149297),(#149298,
#149299,#149300,#149301,#149302)),.UNSPECIFIED.,.F.,.F.,.F.)
B_SPLINE_SURFACE_WITH_KNOTS((2,2),(3,2,3),(0.,0.289681084359918),(0.556108173865715,
0.571428571428571,0.573654350219912),.UNSPECIFIED.)
GEOMETRIC_REPRESENTATION_ITEM()
RATIONAL_B_SPLINE_SURFACE(((0.991551633675927,0.994622399056526,1.,0.999218731101516,
0.998486152291879),(0.991551633675927,0.994622399056526,1.,0.999218731101516,
0.998486152291879)))
REPRESENTATION_ITEM('')
SURFACE()
);
#3238=(
BOUNDED_SURFACE()
B_SPLINE_SURFACE(1,2,((#149304,#149305,#149306,#149307,#149308),(#149309,
#149310,#149311,#149312,#149313)),.UNSPECIFIED.,.F.,.F.,.F.)
B_SPLINE_SURFACE_WITH_KNOTS((2,2),(3,2,3),(0.,0.290030945106622),(0.159677503829416,
0.159901408087481,0.177069452526137),.UNSPECIFIED.)
GEOMETRIC_REPRESENTATION_ITEM()
RATIONAL_B_SPLINE_SURFACE(((0.990889788836284,0.990889788836284,0.990889788836284,
0.987739559362111,0.987486127973996),(0.990889788836284,0.990889788836284,
0.990889788836284,0.987739559362111,0.987486127973996)))
REPRESENTATION_ITEM('')
SURFACE()
);
#3239=(
BOUNDED_SURFACE()
B_SPLINE_SURFACE(1,2,((#149321,#149322,#149323,#149324,#149325),(#149326,
#149327,#149328,#149329,#149330)),.UNSPECIFIED.,.F.,.F.,.F.)
B_SPLINE_SURFACE_WITH_KNOTS((2,2),(3,2,3),(0.,0.289681084359918),(0.556108173865716,
0.571428571428571,0.573654350219912),.UNSPECIFIED.)
GEOMETRIC_REPRESENTATION_ITEM()
RATIONAL_B_SPLINE_SURFACE(((0.991551633675927,0.994622399056526,1.,0.999218731101515,
0.998486152291879),(0.991551633675927,0.994622399056526,1.,0.999218731101515,
0.998486152291879)))
REPRESENTATION_ITEM('')
SURFACE()
);
#3240=(
BOUNDED_SURFACE()
B_SPLINE_SURFACE(1,2,((#149332,#149333,#149334,#149335,#149336),(#149337,
#149338,#149339,#149340,#149341)),.UNSPECIFIED.,.F.,.F.,.F.)
B_SPLINE_SURFACE_WITH_KNOTS((2,2),(3,2,3),(0.,0.290396316295841),(0.159312132640196,
0.159901408087481,0.177069452526134),.UNSPECIFIED.)
GEOMETRIC_REPRESENTATION_ITEM()
RATIONAL_B_SPLINE_SURFACE(((0.990889788836284,0.990889788836284,0.990889788836284,
0.987739559362111,0.987486127973996),(0.990889788836284,0.990889788836284,
0.990889788836284,0.987739559362111,0.987486127973996)))
REPRESENTATION_ITEM('')
SURFACE()
);
#3241=(
BOUNDED_SURFACE()
B_SPLINE_SURFACE(1,2,((#149364,#149365,#149366,#149367,#149368),(#149369,
#149370,#149371,#149372,#149373)),.UNSPECIFIED.,.F.,.F.,.F.)
B_SPLINE_SURFACE_WITH_KNOTS((2,2),(3,2,3),(0.,0.289681084359917),(0.556108173865715,
0.571428571428571,0.573654350219912),.UNSPECIFIED.)
GEOMETRIC_REPRESENTATION_ITEM()
RATIONAL_B_SPLINE_SURFACE(((0.991551633675927,0.994622399056526,1.,0.999218731101515,
0.998486152291879),(0.991551633675927,0.994622399056526,1.,0.999218731101515,
0.998486152291879)))
REPRESENTATION_ITEM('')
SURFACE()
);
#3242=(
BOUNDED_SURFACE()
B_SPLINE_SURFACE(1,2,((#149375,#149376,#149377,#149378,#149379),(#149380,
#149381,#149382,#149383,#149384)),.UNSPECIFIED.,.F.,.F.,.F.)
B_SPLINE_SURFACE_WITH_KNOTS((2,2),(3,2,3),(0.,0.290396316316367),(0.159312132619674,
0.159901408087481,0.177069452526137),.UNSPECIFIED.)
GEOMETRIC_REPRESENTATION_ITEM()
RATIONAL_B_SPLINE_SURFACE(((0.990889788836284,0.990889788836284,0.990889788836284,
0.987739559362111,0.987486127973996),(0.990889788836284,0.990889788836284,
0.990889788836284,0.987739559362111,0.987486127973996)))
REPRESENTATION_ITEM('')
SURFACE()
);
#3243=(
BOUNDED_SURFACE()
B_SPLINE_SURFACE(1,2,((#149407,#149408,#149409,#149410,#149411),(#149412,
#149413,#149414,#149415,#149416)),.UNSPECIFIED.,.F.,.F.,.F.)
B_SPLINE_SURFACE_WITH_KNOTS((2,2),(3,2,3),(0.,0.28968108435992),(0.556108173865716,
0.571428571428571,0.573654350219911),.UNSPECIFIED.)
GEOMETRIC_REPRESENTATION_ITEM()
RATIONAL_B_SPLINE_SURFACE(((0.991551633675927,0.994622399056526,1.,0.999218731101516,
0.99848615229188),(0.991551633675927,0.994622399056526,1.,0.999218731101516,
0.99848615229188)))
REPRESENTATION_ITEM('')
SURFACE()
);
#3244=(
BOUNDED_SURFACE()
B_SPLINE_SURFACE(1,2,((#149418,#149419,#149420,#149421,#149422),(#149423,
#149424,#149425,#149426,#149427)),.UNSPECIFIED.,.F.,.F.,.F.)
B_SPLINE_SURFACE_WITH_KNOTS((2,2),(3,2,3),(0.,0.290396316321617),(0.159312132614422,
0.159901408087481,0.177069452526137),.UNSPECIFIED.)
GEOMETRIC_REPRESENTATION_ITEM()
RATIONAL_B_SPLINE_SURFACE(((0.990889788836284,0.990889788836284,0.990889788836284,
0.987739559362111,0.987486127973996),(0.990889788836284,0.990889788836284,
0.990889788836284,0.987739559362111,0.987486127973996)))
REPRESENTATION_ITEM('')
SURFACE()
);
#3245=(
BOUNDED_SURFACE()
B_SPLINE_SURFACE(1,2,((#149450,#149451,#149452,#149453,#149454),(#149455,
#149456,#149457,#149458,#149459)),.UNSPECIFIED.,.F.,.F.,.F.)
B_SPLINE_SURFACE_WITH_KNOTS((2,2),(3,2,3),(0.,0.289681084359918),(0.556108173865716,
0.571428571428571,0.573654350219911),.UNSPECIFIED.)
GEOMETRIC_REPRESENTATION_ITEM()
RATIONAL_B_SPLINE_SURFACE(((0.991551633675927,0.994622399056526,1.,0.999218731101516,
0.99848615229188),(0.991551633675927,0.994622399056526,1.,0.999218731101516,
0.99848615229188)))
REPRESENTATION_ITEM('')
SURFACE()
);
#3246=(
BOUNDED_SURFACE()
B_SPLINE_SURFACE(1,2,((#149461,#149462,#149463,#149464,#149465),(#149466,
#149467,#149468,#149469,#149470)),.UNSPECIFIED.,.F.,.F.,.F.)
B_SPLINE_SURFACE_WITH_KNOTS((2,2),(3,2,3),(0.,0.290396316324553),(0.15931213261148,
0.159901408087481,0.177069452526137),.UNSPECIFIED.)
GEOMETRIC_REPRESENTATION_ITEM()
RATIONAL_B_SPLINE_SURFACE(((0.990889788836284,0.990889788836284,0.990889788836284,
0.987739559362111,0.987486127973996),(0.990889788836284,0.990889788836284,
0.990889788836284,0.987739559362111,0.987486127973996)))
REPRESENTATION_ITEM('')
SURFACE()
);
#3247=(
BOUNDED_SURFACE()
B_SPLINE_SURFACE(1,2,((#149481,#149482,#149483,#149484,#149485),(#149486,
#149487,#149488,#149489,#149490)),.UNSPECIFIED.,.F.,.F.,.F.)
B_SPLINE_SURFACE_WITH_KNOTS((2,2),(3,2,3),(0.,0.28968108435992),(0.556108173865716,
0.571428571428571,0.573654350219911),.UNSPECIFIED.)
GEOMETRIC_REPRESENTATION_ITEM()
RATIONAL_B_SPLINE_SURFACE(((0.991551633675927,0.994622399056526,1.,0.999218731101516,
0.99848615229188),(0.991551633675927,0.994622399056526,1.,0.999218731101516,
0.99848615229188)))
REPRESENTATION_ITEM('')
SURFACE()
);
#3248=(
BOUNDED_SURFACE()
B_SPLINE_SURFACE(1,2,((#149504,#149505,#149506,#149507,#149508),(#149509,
#149510,#149511,#149512,#149513)),.UNSPECIFIED.,.F.,.F.,.F.)
B_SPLINE_SURFACE_WITH_KNOTS((2,2),(3,2,3),(0.,0.29039631631159),(0.159312132624448,
0.159901408087475,0.177069452526134),.UNSPECIFIED.)
GEOMETRIC_REPRESENTATION_ITEM()
RATIONAL_B_SPLINE_SURFACE(((0.990889788836286,0.990889788836286,0.990889788836286,
0.987739559362111,0.987486127973996),(0.990889788836286,0.990889788836286,
0.990889788836286,0.987739559362112,0.987486127973996)))
REPRESENTATION_ITEM('')
SURFACE()
);
#3249=(
BOUNDED_SURFACE()
B_SPLINE_SURFACE(1,2,((#149536,#149537,#149538,#149539,#149540),(#149541,
#149542,#149543,#149544,#149545)),.UNSPECIFIED.,.F.,.F.,.F.)
B_SPLINE_SURFACE_WITH_KNOTS((2,2),(3,2,3),(0.,0.289681084360114),(0.556108173865715,
0.571428571428571,0.573654350219913),.UNSPECIFIED.)
GEOMETRIC_REPRESENTATION_ITEM()
RATIONAL_B_SPLINE_SURFACE(((0.991551633675927,0.994622399056526,1.,0.999218731101515,
0.998486152291879),(0.991551633675927,0.994622399056526,1.,0.999218731101515,
0.998486152291879)))
REPRESENTATION_ITEM('')
SURFACE()
);
#3250=(
BOUNDED_SURFACE()
B_SPLINE_SURFACE(1,2,((#149547,#149548,#149549,#149550,#149551),(#149552,
#149553,#149554,#149555,#149556)),.UNSPECIFIED.,.F.,.F.,.F.)
B_SPLINE_SURFACE_WITH_KNOTS((2,2),(3,2,3),(0.,0.290396316325579),(0.159312132610595,
0.159901408087482,0.177069452526135),.UNSPECIFIED.)
GEOMETRIC_REPRESENTATION_ITEM()
RATIONAL_B_SPLINE_SURFACE(((0.990889788836284,0.990889788836284,0.990889788836284,
0.987739559362111,0.987486127973996),(0.990889788836284,0.990889788836284,
0.990889788836284,0.987739559362111,0.987486127973996)))
REPRESENTATION_ITEM('')
SURFACE()
);
#3251=(
BOUNDED_SURFACE()
B_SPLINE_SURFACE(1,2,((#149579,#149580,#149581,#149582,#149583),(#149584,
#149585,#149586,#149587,#149588)),.UNSPECIFIED.,.F.,.F.,.F.)
B_SPLINE_SURFACE_WITH_KNOTS((2,2),(3,2,3),(0.,0.289681084360813),(0.556108173865714,
0.571428571428571,0.573654350219921),.UNSPECIFIED.)
GEOMETRIC_REPRESENTATION_ITEM()
RATIONAL_B_SPLINE_SURFACE(((0.991551633675927,0.994622399056525,1.,0.999218731101512,
0.998486152291873),(0.991551633675927,0.994622399056525,1.,0.999218731101512,
0.998486152291873)))
REPRESENTATION_ITEM('')
SURFACE()
);
#3252=(
BOUNDED_SURFACE()
B_SPLINE_SURFACE(1,2,((#149590,#149591,#149592,#149593,#149594),(#149595,
#149596,#149597,#149598,#149599)),.UNSPECIFIED.,.F.,.F.,.F.)
B_SPLINE_SURFACE_WITH_KNOTS((2,2),(3,2,3),(0.,0.290396316336308),(0.159312132599877,
0.159901408087482,0.177069452526135),.UNSPECIFIED.)
GEOMETRIC_REPRESENTATION_ITEM()
RATIONAL_B_SPLINE_SURFACE(((0.990889788836284,0.990889788836284,0.990889788836284,
0.987739559362111,0.987486127973995),(0.990889788836284,0.990889788836284,
0.990889788836284,0.987739559362111,0.987486127973995)))
REPRESENTATION_ITEM('')
SURFACE()
);
#3253=(
BOUNDED_SURFACE()
B_SPLINE_SURFACE(1,2,((#149622,#149623,#149624,#149625,#149626),(#149627,
#149628,#149629,#149630,#149631)),.UNSPECIFIED.,.F.,.F.,.F.)
B_SPLINE_SURFACE_WITH_KNOTS((2,2),(3,2,3),(0.,0.289681084360947),(0.556108173865714,
0.571428571428571,0.57365435021992),.UNSPECIFIED.)
GEOMETRIC_REPRESENTATION_ITEM()
RATIONAL_B_SPLINE_SURFACE(((0.991551633675927,0.994622399056525,1.,0.999218731101513,
0.998486152291874),(0.991551633675927,0.994622399056525,1.,0.999218731101513,
0.998486152291874)))
REPRESENTATION_ITEM('')
SURFACE()
);
#3254=(
BOUNDED_SURFACE()
B_SPLINE_SURFACE(1,2,((#149633,#149634,#149635,#149636,#149637),(#149638,
#149639,#149640,#149641,#149642)),.UNSPECIFIED.,.F.,.F.,.F.)
B_SPLINE_SURFACE_WITH_KNOTS((2,2),(3,2,3),(0.,0.29039631630548),(0.159312132630947,
0.159901408087482,0.177069452526138),.UNSPECIFIED.)
GEOMETRIC_REPRESENTATION_ITEM()
RATIONAL_B_SPLINE_SURFACE(((0.990889788836284,0.990889788836284,0.990889788836284,
0.98773955936211,0.987486127973996),(0.990889788836284,0.990889788836284,
0.990889788836284,0.98773955936211,0.987486127973996)))
REPRESENTATION_ITEM('')
SURFACE()
);
#3255=(
BOUNDED_SURFACE()
B_SPLINE_SURFACE(1,2,((#149665,#149666,#149667,#149668,#149669),(#149670,
#149671,#149672,#149673,#149674)),.UNSPECIFIED.,.F.,.F.,.F.)
B_SPLINE_SURFACE_WITH_KNOTS((2,2),(3,2,3),(0.,0.289681084360913),(0.556108173865715,
0.571428571428571,0.573654350219922),.UNSPECIFIED.)
GEOMETRIC_REPRESENTATION_ITEM()
RATIONAL_B_SPLINE_SURFACE(((0.991551633675927,0.994622399056525,1.,0.999218731101512,
0.998486152291872),(0.991551633675927,0.994622399056525,1.,0.999218731101512,
0.998486152291872)))
REPRESENTATION_ITEM('')
SURFACE()
);
#3256=(
BOUNDED_SURFACE()
B_SPLINE_SURFACE(1,2,((#149676,#149677,#149678,#149679,#149680),(#149681,
#149682,#149683,#149684,#149685)),.UNSPECIFIED.,.F.,.F.,.F.)
B_SPLINE_SURFACE_WITH_KNOTS((2,2),(3,2,3),(0.,0.290396316326519),(0.159312132611315,
0.159901408087482,0.177069452526135),.UNSPECIFIED.)
GEOMETRIC_REPRESENTATION_ITEM()
RATIONAL_B_SPLINE_SURFACE(((0.990889788836284,0.990889788836284,0.990889788836284,
0.987739559362111,0.987486127973996),(0.990889788836284,0.990889788836284,
0.990889788836284,0.987739559362111,0.987486127973996)))
REPRESENTATION_ITEM('')
SURFACE()
);
#3257=(
BOUNDED_SURFACE()
B_SPLINE_SURFACE(1,2,((#149708,#149709,#149710,#149711,#149712),(#149713,
#149714,#149715,#149716,#149717)),.UNSPECIFIED.,.F.,.F.,.F.)
B_SPLINE_SURFACE_WITH_KNOTS((2,2),(3,2,3),(0.,0.289681084360124),(0.556108173865714,
0.571428571428571,0.57365435021991),.UNSPECIFIED.)
GEOMETRIC_REPRESENTATION_ITEM()
RATIONAL_B_SPLINE_SURFACE(((0.991551633675927,0.994622399056525,1.,0.999218731101516,
0.99848615229188),(0.991551633675927,0.994622399056525,1.,0.999218731101516,
0.99848615229188)))
REPRESENTATION_ITEM('')
SURFACE()
);
#3258=(
BOUNDED_SURFACE()
B_SPLINE_SURFACE(1,2,((#149719,#149720,#149721,#149722,#149723),(#149724,
#149725,#149726,#149727,#149728)),.UNSPECIFIED.,.F.,.F.,.F.)
B_SPLINE_SURFACE_WITH_KNOTS((2,2),(3,2,3),(0.,0.290396316316441),(0.159312132620063,
0.159901408087455,0.177069452526135),.UNSPECIFIED.)
GEOMETRIC_REPRESENTATION_ITEM()
RATIONAL_B_SPLINE_SURFACE(((0.990889788836294,0.990889788836294,0.990889788836294,
0.987739559362111,0.987486127973996),(0.990889788836294,0.990889788836294,
0.990889788836294,0.987739559362111,0.987486127973996)))
REPRESENTATION_ITEM('')
SURFACE()
);
#3259=(
BOUNDED_SURFACE()
B_SPLINE_SURFACE(1,2,((#149751,#149752,#149753,#149754,#149755),(#149756,
#149757,#149758,#149759,#149760)),.UNSPECIFIED.,.F.,.F.,.F.)
B_SPLINE_SURFACE_WITH_KNOTS((2,2),(3,2,3),(0.,0.289681084359929),(0.556108173865714,
0.571428571428571,0.57365435021991),.UNSPECIFIED.)
GEOMETRIC_REPRESENTATION_ITEM()
RATIONAL_B_SPLINE_SURFACE(((0.991551633675927,0.994622399056525,1.,0.999218731101516,
0.99848615229188),(0.991551633675927,0.994622399056525,1.,0.999218731101516,
0.99848615229188)))
REPRESENTATION_ITEM('')
SURFACE()
);
#3260=(
BOUNDED_SURFACE()
B_SPLINE_SURFACE(1,2,((#149762,#149763,#149764,#149765,#149766),(#149767,
#149768,#149769,#149770,#149771)),.UNSPECIFIED.,.F.,.F.,.F.)
B_SPLINE_SURFACE_WITH_KNOTS((2,2),(3,2,3),(0.,0.29039631630902),(0.159312132627105,
0.159901408087482,0.177069452526138),.UNSPECIFIED.)
GEOMETRIC_REPRESENTATION_ITEM()
RATIONAL_B_SPLINE_SURFACE(((0.990889788836284,0.990889788836284,0.990889788836284,
0.98773955936211,0.987486127973996),(0.990889788836284,0.990889788836284,
0.990889788836284,0.98773955936211,0.987486127973996)))
REPRESENTATION_ITEM('')
SURFACE()
);
#3261=(
BOUNDED_SURFACE()
B_SPLINE_SURFACE(1,2,((#149794,#149795,#149796,#149797,#149798),(#149799,
#149800,#149801,#149802,#149803)),.UNSPECIFIED.,.F.,.F.,.F.)
B_SPLINE_SURFACE_WITH_KNOTS((2,2),(3,2,3),(0.,0.289681084359923),(0.556108173865714,
0.571428571428571,0.57365435021991),.UNSPECIFIED.)
GEOMETRIC_REPRESENTATION_ITEM()
RATIONAL_B_SPLINE_SURFACE(((0.991551633675927,0.994622399056525,1.,0.999218731101516,
0.99848615229188),(0.991551633675927,0.994622399056525,1.,0.999218731101516,
0.99848615229188)))
REPRESENTATION_ITEM('')
SURFACE()
);
#3262=(
BOUNDED_SURFACE()
B_SPLINE_SURFACE(1,2,((#149805,#149806,#149807,#149808,#149809),(#149810,
#149811,#149812,#149813,#149814)),.UNSPECIFIED.,.F.,.F.,.F.)
B_SPLINE_SURFACE_WITH_KNOTS((2,2),(3,2,3),(0.,0.290396316315867),(0.159312132620248,
0.159901408087482,0.177069452526135),.UNSPECIFIED.)
GEOMETRIC_REPRESENTATION_ITEM()
RATIONAL_B_SPLINE_SURFACE(((0.990889788836284,0.990889788836284,0.990889788836284,
0.987739559362111,0.987486127973996),(0.990889788836284,0.990889788836284,
0.990889788836284,0.987739559362111,0.987486127973996)))
REPRESENTATION_ITEM('')
SURFACE()
);
#3263=(
BOUNDED_SURFACE()
B_SPLINE_SURFACE(1,2,((#149837,#149838,#149839,#149840,#149841),(#149842,
#149843,#149844,#149845,#149846)),.UNSPECIFIED.,.F.,.F.,.F.)
B_SPLINE_SURFACE_WITH_KNOTS((2,2),(3,2,3),(0.,0.289681084359919),(0.556108173865714,
0.571428571428571,0.57365435021991),.UNSPECIFIED.)
GEOMETRIC_REPRESENTATION_ITEM()
RATIONAL_B_SPLINE_SURFACE(((0.991551633675927,0.994622399056525,1.,0.999218731101516,
0.99848615229188),(0.991551633675927,0.994622399056525,1.,0.999218731101516,
0.99848615229188)))
REPRESENTATION_ITEM('')
SURFACE()
);
#3264=(
BOUNDED_SURFACE()
B_SPLINE_SURFACE(1,2,((#149848,#149849,#149850,#149851,#149852),(#149853,
#149854,#149855,#149856,#149857)),.UNSPECIFIED.,.F.,.F.,.F.)
B_SPLINE_SURFACE_WITH_KNOTS((2,2),(3,2,3),(0.,0.290396316320743),(0.159312132615369,
0.159901408087482,0.177069452526135),.UNSPECIFIED.)
GEOMETRIC_REPRESENTATION_ITEM()
RATIONAL_B_SPLINE_SURFACE(((0.990889788836284,0.990889788836284,0.990889788836284,
0.987739559362111,0.987486127973996),(0.990889788836284,0.990889788836284,
0.990889788836284,0.987739559362111,0.987486127973996)))
REPRESENTATION_ITEM('')
SURFACE()
);
#3265=(
BOUNDED_SURFACE()
B_SPLINE_SURFACE(1,2,((#149880,#149881,#149882,#149883,#149884),(#149885,
#149886,#149887,#149888,#149889)),.UNSPECIFIED.,.F.,.F.,.F.)
B_SPLINE_SURFACE_WITH_KNOTS((2,2),(3,2,3),(0.,0.289681084359923),(0.556108173865714,
0.571428571428571,0.57365435021991),.UNSPECIFIED.)
GEOMETRIC_REPRESENTATION_ITEM()
RATIONAL_B_SPLINE_SURFACE(((0.991551633675927,0.994622399056525,1.,0.999218731101516,
0.99848615229188),(0.991551633675927,0.994622399056525,1.,0.999218731101516,
0.99848615229188)))
REPRESENTATION_ITEM('')
SURFACE()
);
#3266=(
BOUNDED_SURFACE()
B_SPLINE_SURFACE(1,2,((#149891,#149892,#149893,#149894,#149895),(#149896,
#149897,#149898,#149899,#149900)),.UNSPECIFIED.,.F.,.F.,.F.)
B_SPLINE_SURFACE_WITH_KNOTS((2,2),(3,2,3),(0.,0.29039631629488),(0.159312132641506,
0.159901408087428,0.177069452526138),.UNSPECIFIED.)
GEOMETRIC_REPRESENTATION_ITEM()
RATIONAL_B_SPLINE_SURFACE(((0.990889788836304,0.990889788836304,0.990889788836304,
0.987739559362111,0.987486127973996),(0.990889788836304,0.990889788836304,
0.990889788836304,0.987739559362111,0.987486127973996)))
REPRESENTATION_ITEM('')
SURFACE()
);
#3267=(
BOUNDED_SURFACE()
B_SPLINE_SURFACE(1,2,((#149923,#149924,#149925,#149926,#149927),(#149928,
#149929,#149930,#149931,#149932)),.UNSPECIFIED.,.F.,.F.,.F.)
B_SPLINE_SURFACE_WITH_KNOTS((2,2),(3,2,3),(0.,0.289681084359927),(0.556108173865715,
0.571428571428571,0.57365435021991),.UNSPECIFIED.)
GEOMETRIC_REPRESENTATION_ITEM()
RATIONAL_B_SPLINE_SURFACE(((0.991551633675927,0.994622399056525,1.,0.999218731101516,
0.99848615229188),(0.991551633675927,0.994622399056525,1.,0.999218731101516,
0.99848615229188)))
REPRESENTATION_ITEM('')
SURFACE()
);
#3268=(
BOUNDED_SURFACE()
B_SPLINE_SURFACE(1,2,((#149934,#149935,#149936,#149937,#149938),(#149939,
#149940,#149941,#149942,#149943)),.UNSPECIFIED.,.F.,.F.,.F.)
B_SPLINE_SURFACE_WITH_KNOTS((2,2),(3,2,3),(0.709719018626781,1.),(0.607879027750091,
0.625170525609407,0.625770422837593),.UNSPECIFIED.)
GEOMETRIC_REPRESENTATION_ITEM()
RATIONAL_B_SPLINE_SURFACE(((0.987469282487682,0.987594391229382,0.990658108926708,
0.990658108926708,0.990658108926708),(0.987469282487682,0.987594391229382,
0.990658108926708,0.990658108926708,0.990658108926708)))
REPRESENTATION_ITEM('')
SURFACE()
);
#3269=(
BOUNDED_SURFACE()
B_SPLINE_SURFACE(1,2,((#149961,#149962,#149963),(#149964,#149965,#149966)),
 .UNSPECIFIED.,.F.,.F.,.F.)
B_SPLINE_SURFACE_WITH_KNOTS((2,2),(3,3),(0.71019295900798,1.),(0.107982157956012,
0.125273655815329),.UNSPECIFIED.)
GEOMETRIC_REPRESENTATION_ITEM()
RATIONAL_B_SPLINE_SURFACE(((0.987470879370255,0.987613514606721,0.990694758798813),
(0.987470879370256,0.987613514606721,0.990694758798813)))
REPRESENTATION_ITEM('')
SURFACE()
);
#3270=(
BOUNDED_SURFACE()
B_SPLINE_SURFACE(1,2,((#149973,#149974,#149975,#149976,#149977),(#149978,
#149979,#149980,#149981,#149982)),.UNSPECIFIED.,.F.,.F.,.F.)
B_SPLINE_SURFACE_WITH_KNOTS((2,2),(3,2,3),(0.709719018636767,1.),(0.607879027750091,
0.625170525609407,0.625770422827617),.UNSPECIFIED.)
GEOMETRIC_REPRESENTATION_ITEM()
RATIONAL_B_SPLINE_SURFACE(((0.987469282487682,0.987594391229382,0.990658108926708,
0.990658108926708,0.990658108926708),(0.987469282487682,0.987594391229382,
0.990658108926708,0.990658108926708,0.990658108926708)))
REPRESENTATION_ITEM('')
SURFACE()
);
#3271=(
BOUNDED_SURFACE()
B_SPLINE_SURFACE(1,2,((#150000,#150001,#150002),(#150003,#150004,#150005)),
 .UNSPECIFIED.,.F.,.F.,.F.)
B_SPLINE_SURFACE_WITH_KNOTS((2,2),(3,3),(0.710192959007998,1.),(0.107982157956012,
0.125273655815329),.UNSPECIFIED.)
GEOMETRIC_REPRESENTATION_ITEM()
RATIONAL_B_SPLINE_SURFACE(((0.987470879370255,0.987613514606721,0.990694758798813),
(0.987470879370256,0.987613514606721,0.990694758798813)))
REPRESENTATION_ITEM('')
SURFACE()
);
#3272=(
BOUNDED_SURFACE()
B_SPLINE_SURFACE(1,2,((#150012,#150013,#150014,#150015,#150016),(#150017,
#150018,#150019,#150020,#150021)),.UNSPECIFIED.,.F.,.F.,.F.)
B_SPLINE_SURFACE_WITH_KNOTS((2,2),(3,2,3),(0.709719018631378,1.),(0.607879027750091,
0.625170525609407,0.625770422833355),.UNSPECIFIED.)
GEOMETRIC_REPRESENTATION_ITEM()
RATIONAL_B_SPLINE_SURFACE(((0.987469282487682,0.987594391229382,0.990658108926709,
0.990658108926709,0.990658108926709),(0.987469282487682,0.987594391229382,
0.990658108926709,0.990658108926709,0.990658108926709)))
REPRESENTATION_ITEM('')
SURFACE()
);
#3273=(
BOUNDED_SURFACE()
B_SPLINE_SURFACE(1,2,((#150039,#150040,#150041),(#150042,#150043,#150044)),
 .UNSPECIFIED.,.F.,.F.,.F.)
B_SPLINE_SURFACE_WITH_KNOTS((2,2),(3,3),(0.710192959008343,1.),(0.107982157956012,
0.125273655815329),.UNSPECIFIED.)
GEOMETRIC_REPRESENTATION_ITEM()
RATIONAL_B_SPLINE_SURFACE(((0.987470879370255,0.987613514606721,0.990694758798813),
(0.987470879370256,0.987613514606721,0.990694758798813)))
REPRESENTATION_ITEM('')
SURFACE()
);
#3274=(
BOUNDED_SURFACE()
B_SPLINE_SURFACE(1,2,((#150051,#150052,#150053,#150054,#150055),(#150056,
#150057,#150058,#150059,#150060)),.UNSPECIFIED.,.F.,.F.,.F.)
B_SPLINE_SURFACE_WITH_KNOTS((2,2),(3,2,3),(0.709719018649857,1.),(0.607879027750091,
0.625170525609407,0.625770422814865),.UNSPECIFIED.)
GEOMETRIC_REPRESENTATION_ITEM()
RATIONAL_B_SPLINE_SURFACE(((0.987469282487682,0.987594391229382,0.990658108926708,
0.990658108926708,0.990658108926708),(0.987469282487682,0.987594391229382,
0.990658108926708,0.990658108926708,0.990658108926708)))
REPRESENTATION_ITEM('')
SURFACE()
);
#3275=(
BOUNDED_SURFACE()
B_SPLINE_SURFACE(1,2,((#150078,#150079,#150080),(#150081,#150082,#150083)),
 .UNSPECIFIED.,.F.,.F.,.F.)
B_SPLINE_SURFACE_WITH_KNOTS((2,2),(3,3),(0.710192959008336,1.),(0.107982157956012,
0.125273655815329),.UNSPECIFIED.)
GEOMETRIC_REPRESENTATION_ITEM()
RATIONAL_B_SPLINE_SURFACE(((0.987470879370256,0.987613514606721,0.990694758798813),
(0.987470879370256,0.987613514606721,0.990694758798813)))
REPRESENTATION_ITEM('')
SURFACE()
);
#3276=(
BOUNDED_SURFACE()
B_SPLINE_SURFACE(1,2,((#150090,#150091,#150092,#150093,#150094),(#150095,
#150096,#150097,#150098,#150099)),.UNSPECIFIED.,.F.,.F.,.F.)
B_SPLINE_SURFACE_WITH_KNOTS((2,2),(3,2,3),(0.709719018614768,1.),(0.607879027750091,
0.625170525609407,0.625770422849006),.UNSPECIFIED.)
GEOMETRIC_REPRESENTATION_ITEM()
RATIONAL_B_SPLINE_SURFACE(((0.987469282487682,0.987594391229382,0.990658108926709,
0.990658108926709,0.990658108926709),(0.987469282487682,0.987594391229382,
0.990658108926709,0.990658108926709,0.990658108926709)))
REPRESENTATION_ITEM('')
SURFACE()
);
#3277=(
BOUNDED_SURFACE()
B_SPLINE_SURFACE(1,2,((#150117,#150118,#150119),(#150120,#150121,#150122)),
 .UNSPECIFIED.,.F.,.F.,.F.)
B_SPLINE_SURFACE_WITH_KNOTS((2,2),(3,3),(0.710192959007384,1.),(0.107982157956012,
0.125273655815329),.UNSPECIFIED.)
GEOMETRIC_REPRESENTATION_ITEM()
RATIONAL_B_SPLINE_SURFACE(((0.987470879370256,0.987613514606721,0.990694758798813),
(0.987470879370256,0.987613514606721,0.990694758798813)))
REPRESENTATION_ITEM('')
SURFACE()
);
#3278=(
BOUNDED_SURFACE()
B_SPLINE_SURFACE(1,2,((#150129,#150130,#150131,#150132,#150133),(#150134,
#150135,#150136,#150137,#150138)),.UNSPECIFIED.,.F.,.F.,.F.)
B_SPLINE_SURFACE_WITH_KNOTS((2,2),(3,2,3),(0.709719018624158,1.),(0.607879027750091,
0.625170525609407,0.625770422839608),.UNSPECIFIED.)
GEOMETRIC_REPRESENTATION_ITEM()
RATIONAL_B_SPLINE_SURFACE(((0.987469282487682,0.987594391229382,0.990658108926709,
0.990658108926709,0.990658108926709),(0.987469282487682,0.987594391229382,
0.990658108926709,0.990658108926709,0.990658108926709)))
REPRESENTATION_ITEM('')
SURFACE()
);
#3279=(
BOUNDED_SURFACE()
B_SPLINE_SURFACE(1,2,((#150156,#150157,#150158),(#150159,#150160,#150161)),
 .UNSPECIFIED.,.F.,.F.,.F.)
B_SPLINE_SURFACE_WITH_KNOTS((2,2),(3,3),(0.710192959007374,1.),(0.107982157956012,
0.125273655815329),.UNSPECIFIED.)
GEOMETRIC_REPRESENTATION_ITEM()
RATIONAL_B_SPLINE_SURFACE(((0.987470879370255,0.987613514606721,0.990694758798813),
(0.987470879370256,0.987613514606721,0.990694758798813)))
REPRESENTATION_ITEM('')
SURFACE()
);
#3280=(
BOUNDED_SURFACE()
B_SPLINE_SURFACE(1,2,((#150168,#150169,#150170,#150171,#150172),(#150173,
#150174,#150175,#150176,#150177)),.UNSPECIFIED.,.F.,.F.,.F.)
B_SPLINE_SURFACE_WITH_KNOTS((2,2),(3,2,3),(0.709719018629564,1.),(0.607879027750091,
0.625170525609407,0.625770422834208),.UNSPECIFIED.)
GEOMETRIC_REPRESENTATION_ITEM()
RATIONAL_B_SPLINE_SURFACE(((0.987469282487682,0.987594391229382,0.990658108926708,
0.990658108926708,0.990658108926708),(0.987469282487682,0.987594391229382,
0.990658108926709,0.990658108926709,0.990658108926709)))
REPRESENTATION_ITEM('')
SURFACE()
);
#3281=(
BOUNDED_SURFACE()
B_SPLINE_SURFACE(1,2,((#150195,#150196,#150197),(#150198,#150199,#150200)),
 .UNSPECIFIED.,.F.,.F.,.F.)
B_SPLINE_SURFACE_WITH_KNOTS((2,2),(3,3),(0.710192959007377,1.),(0.107982157956012,
0.125273655815329),.UNSPECIFIED.)
GEOMETRIC_REPRESENTATION_ITEM()
RATIONAL_B_SPLINE_SURFACE(((0.987470879370256,0.987613514606721,0.990694758798813),
(0.987470879370256,0.987613514606721,0.990694758798813)))
REPRESENTATION_ITEM('')
SURFACE()
);
#3282=(
BOUNDED_SURFACE()
B_SPLINE_SURFACE(1,2,((#150207,#150208,#150209,#150210,#150211),(#150212,
#150213,#150214,#150215,#150216)),.UNSPECIFIED.,.F.,.F.,.F.)
B_SPLINE_SURFACE_WITH_KNOTS((2,2),(3,2,3),(0.709719018632745,1.),(0.607879027750091,
0.625170525609407,0.625770422830443),.UNSPECIFIED.)
GEOMETRIC_REPRESENTATION_ITEM()
RATIONAL_B_SPLINE_SURFACE(((0.987469282487682,0.987594391229382,0.990658108926709,
0.990658108926709,0.990658108926709),(0.987469282487682,0.987594391229382,
0.990658108926709,0.990658108926709,0.990658108926709)))
REPRESENTATION_ITEM('')
SURFACE()
);
#3283=(
BOUNDED_SURFACE()
B_SPLINE_SURFACE(1,2,((#150234,#150235,#150236),(#150237,#150238,#150239)),
 .UNSPECIFIED.,.F.,.F.,.F.)
B_SPLINE_SURFACE_WITH_KNOTS((2,2),(3,3),(0.710192959006796,1.),(0.107982157956012,
0.125273655815329),.UNSPECIFIED.)
GEOMETRIC_REPRESENTATION_ITEM()
RATIONAL_B_SPLINE_SURFACE(((0.987470879370256,0.987613514606721,0.990694758798813),
(0.987470879370256,0.987613514606721,0.990694758798813)))
REPRESENTATION_ITEM('')
SURFACE()
);
#3284=(
BOUNDED_SURFACE()
B_SPLINE_SURFACE(1,2,((#150246,#150247,#150248,#150249,#150250),(#150251,
#150252,#150253,#150254,#150255)),.UNSPECIFIED.,.F.,.F.,.F.)
B_SPLINE_SURFACE_WITH_KNOTS((2,2),(3,2,3),(0.70971901863244,1.),(0.607879027750091,
0.625170525609407,0.625770422831336),.UNSPECIFIED.)
GEOMETRIC_REPRESENTATION_ITEM()
RATIONAL_B_SPLINE_SURFACE(((0.987469282487682,0.987594391229382,0.990658108926708,
0.990658108926708,0.990658108926708),(0.987469282487682,0.987594391229382,
0.990658108926709,0.990658108926709,0.990658108926709)))
REPRESENTATION_ITEM('')
SURFACE()
);
#3285=(
BOUNDED_SURFACE()
B_SPLINE_SURFACE(1,2,((#150273,#150274,#150275),(#150276,#150277,#150278)),
 .UNSPECIFIED.,.F.,.F.,.F.)
B_SPLINE_SURFACE_WITH_KNOTS((2,2),(3,3),(0.710192959007382,1.),(0.107982157956012,
0.125273655815329),.UNSPECIFIED.)
GEOMETRIC_REPRESENTATION_ITEM()
RATIONAL_B_SPLINE_SURFACE(((0.987470879370256,0.987613514606721,0.990694758798813),
(0.987470879370256,0.987613514606721,0.990694758798813)))
REPRESENTATION_ITEM('')
SURFACE()
);
#3286=(
BOUNDED_SURFACE()
B_SPLINE_SURFACE(1,2,((#150285,#150286,#150287,#150288,#150289),(#150290,
#150291,#150292,#150293,#150294)),.UNSPECIFIED.,.F.,.F.,.F.)
B_SPLINE_SURFACE_WITH_KNOTS((2,2),(3,2,3),(0.709719018613158,1.),(0.607879027750091,
0.625170525609407,0.625770422850059),.UNSPECIFIED.)
GEOMETRIC_REPRESENTATION_ITEM()
RATIONAL_B_SPLINE_SURFACE(((0.987469282487682,0.987594391229382,0.990658108926708,
0.990658108926708,0.990658108926708),(0.987469282487682,0.987594391229382,
0.990658108926708,0.990658108926708,0.990658108926708)))
REPRESENTATION_ITEM('')
SURFACE()
);
#3287=(
BOUNDED_SURFACE()
B_SPLINE_SURFACE(1,2,((#150312,#150313,#150314),(#150315,#150316,#150317)),
 .UNSPECIFIED.,.F.,.F.,.F.)
B_SPLINE_SURFACE_WITH_KNOTS((2,2),(3,3),(0.710192959006824,1.),(0.107982157956012,
0.125273655815329),.UNSPECIFIED.)
GEOMETRIC_REPRESENTATION_ITEM()
RATIONAL_B_SPLINE_SURFACE(((0.987470879370256,0.987613514606721,0.990694758798813),
(0.987470879370256,0.987613514606721,0.990694758798813)))
REPRESENTATION_ITEM('')
SURFACE()
);
#3288=(
BOUNDED_SURFACE()
B_SPLINE_SURFACE(1,2,((#150324,#150325,#150326,#150327,#150328),(#150329,
#150330,#150331,#150332,#150333)),.UNSPECIFIED.,.F.,.F.,.F.)
B_SPLINE_SURFACE_WITH_KNOTS((2,2),(3,2,3),(0.70971901862884,1.),(0.607879027750092,
0.625170525609407,0.625770422834571),.UNSPECIFIED.)
GEOMETRIC_REPRESENTATION_ITEM()
RATIONAL_B_SPLINE_SURFACE(((0.987469282487682,0.987594391229382,0.990658108926708,
0.990658108926708,0.990658108926708),(0.987469282487682,0.987594391229382,
0.990658108926708,0.990658108926708,0.990658108926708)))
REPRESENTATION_ITEM('')
SURFACE()
);
#3289=(
BOUNDED_SURFACE()
B_SPLINE_SURFACE(1,2,((#150351,#150352,#150353),(#150354,#150355,#150356)),
 .UNSPECIFIED.,.F.,.F.,.F.)
B_SPLINE_SURFACE_WITH_KNOTS((2,2),(3,3),(0.710192959007015,1.),(0.107982157956011,
0.125273655815328),.UNSPECIFIED.)
GEOMETRIC_REPRESENTATION_ITEM()
RATIONAL_B_SPLINE_SURFACE(((0.987470879370255,0.98761351460672,0.990694758798812),
(0.987470879370255,0.98761351460672,0.990694758798812)))
REPRESENTATION_ITEM('')
SURFACE()
);
#3290=(
BOUNDED_SURFACE()
B_SPLINE_SURFACE(1,2,((#150363,#150364,#150365,#150366,#150367),(#150368,
#150369,#150370,#150371,#150372)),.UNSPECIFIED.,.F.,.F.,.F.)
B_SPLINE_SURFACE_WITH_KNOTS((2,2),(3,2,3),(0.709719018615787,1.),(0.607879027750092,
0.625170525609408,0.625770422847591),.UNSPECIFIED.)
GEOMETRIC_REPRESENTATION_ITEM()
RATIONAL_B_SPLINE_SURFACE(((0.987469282487682,0.987594391229382,0.990658108926709,
0.990658108926709,0.990658108926709),(0.987469282487682,0.987594391229382,
0.990658108926709,0.990658108926709,0.990658108926709)))
REPRESENTATION_ITEM('')
SURFACE()
);
#3291=(
BOUNDED_SURFACE()
B_SPLINE_SURFACE(1,2,((#150390,#150391,#150392),(#150393,#150394,#150395)),
 .UNSPECIFIED.,.F.,.F.,.F.)
B_SPLINE_SURFACE_WITH_KNOTS((2,2),(3,3),(0.710192959006983,1.),(0.107982157956011,
0.125273655815328),.UNSPECIFIED.)
GEOMETRIC_REPRESENTATION_ITEM()
RATIONAL_B_SPLINE_SURFACE(((0.987470879370255,0.98761351460672,0.990694758798812),
(0.987470879370255,0.98761351460672,0.990694758798812)))
REPRESENTATION_ITEM('')
SURFACE()
);
#3292=(
BOUNDED_SURFACE()
B_SPLINE_SURFACE(1,2,((#150402,#150403,#150404,#150405,#150406),(#150407,
#150408,#150409,#150410,#150411)),.UNSPECIFIED.,.F.,.F.,.F.)
B_SPLINE_SURFACE_WITH_KNOTS((2,2),(3,2,3),(0.70971901861887,1.),(0.607879027750092,
0.625170525609408,0.625770422844231),.UNSPECIFIED.)
GEOMETRIC_REPRESENTATION_ITEM()
RATIONAL_B_SPLINE_SURFACE(((0.987469282487682,0.987594391229382,0.990658108926709,
0.990658108926709,0.990658108926709),(0.987469282487682,0.987594391229382,
0.990658108926709,0.990658108926709,0.990658108926709)))
REPRESENTATION_ITEM('')
SURFACE()
);
#3293=(
BOUNDED_SURFACE()
B_SPLINE_SURFACE(1,2,((#150429,#150430,#150431),(#150432,#150433,#150434)),
 .UNSPECIFIED.,.F.,.F.,.F.)
B_SPLINE_SURFACE_WITH_KNOTS((2,2),(3,3),(0.710192959006704,1.),(0.107982157956011,
0.125273655815328),.UNSPECIFIED.)
GEOMETRIC_REPRESENTATION_ITEM()
RATIONAL_B_SPLINE_SURFACE(((0.987470879370255,0.98761351460672,0.990694758798812),
(0.987470879370255,0.98761351460672,0.990694758798812)))
REPRESENTATION_ITEM('')
SURFACE()
);
#3294=(
BOUNDED_SURFACE()
B_SPLINE_SURFACE(1,2,((#150441,#150442,#150443,#150444,#150445),(#150446,
#150447,#150448,#150449,#150450)),.UNSPECIFIED.,.F.,.F.,.F.)
B_SPLINE_SURFACE_WITH_KNOTS((2,2),(3,2,3),(0.709719018626216,1.),(0.607879027750092,
0.625170525609408,0.625770422837466),.UNSPECIFIED.)
GEOMETRIC_REPRESENTATION_ITEM()
RATIONAL_B_SPLINE_SURFACE(((0.987469282487682,0.987594391229382,0.990658108926709,
0.990658108926709,0.990658108926709),(0.987469282487682,0.987594391229382,
0.990658108926709,0.990658108926709,0.990658108926709)))
REPRESENTATION_ITEM('')
SURFACE()
);
#3295=(
BOUNDED_SURFACE()
B_SPLINE_SURFACE(1,2,((#150468,#150469,#150470),(#150471,#150472,#150473)),
 .UNSPECIFIED.,.F.,.F.,.F.)
B_SPLINE_SURFACE_WITH_KNOTS((2,2),(3,3),(0.710192959007287,1.),(0.107982157956011,
0.125273655815328),.UNSPECIFIED.)
GEOMETRIC_REPRESENTATION_ITEM()
RATIONAL_B_SPLINE_SURFACE(((0.987470879370255,0.98761351460672,0.990694758798812),
(0.987470879370255,0.98761351460672,0.990694758798812)))
REPRESENTATION_ITEM('')
SURFACE()
);
#3296=(
BOUNDED_SURFACE()
B_SPLINE_SURFACE(1,2,((#150480,#150481,#150482,#150483,#150484),(#150485,
#150486,#150487,#150488,#150489)),.UNSPECIFIED.,.F.,.F.,.F.)
B_SPLINE_SURFACE_WITH_KNOTS((2,2),(3,2,3),(0.709719018626252,1.),(0.607879027750092,
0.625170525609409,0.625770422836598),.UNSPECIFIED.)
GEOMETRIC_REPRESENTATION_ITEM()
RATIONAL_B_SPLINE_SURFACE(((0.987469282487682,0.987594391229382,0.990658108926709,
0.990658108926709,0.990658108926709),(0.987469282487682,0.987594391229382,
0.990658108926709,0.990658108926709,0.990658108926709)))
REPRESENTATION_ITEM('')
SURFACE()
);
#3297=(
BOUNDED_SURFACE()
B_SPLINE_SURFACE(1,2,((#150507,#150508,#150509),(#150510,#150511,#150512)),
 .UNSPECIFIED.,.F.,.F.,.F.)
B_SPLINE_SURFACE_WITH_KNOTS((2,2),(3,3),(0.710192959006458,1.),(0.107982157956011,
0.125273655815328),.UNSPECIFIED.)
GEOMETRIC_REPRESENTATION_ITEM()
RATIONAL_B_SPLINE_SURFACE(((0.987470879370255,0.98761351460672,0.990694758798812),
(0.987470879370255,0.98761351460672,0.990694758798812)))
REPRESENTATION_ITEM('')
SURFACE()
);
#3298=(
BOUNDED_SURFACE()
B_SPLINE_SURFACE(1,2,((#150519,#150520,#150521,#150522,#150523),(#150524,
#150525,#150526,#150527,#150528)),.UNSPECIFIED.,.F.,.F.,.F.)
B_SPLINE_SURFACE_WITH_KNOTS((2,2),(3,2,3),(0.709719018614626,1.),(0.607879027750092,
0.625170525609408,0.625770422848724),.UNSPECIFIED.)
GEOMETRIC_REPRESENTATION_ITEM()
RATIONAL_B_SPLINE_SURFACE(((0.987469282487682,0.987594391229382,0.990658108926709,
0.990658108926709,0.990658108926709),(0.987469282487682,0.987594391229382,
0.990658108926709,0.990658108926709,0.990658108926709)))
REPRESENTATION_ITEM('')
SURFACE()
);
#3299=(
BOUNDED_SURFACE()
B_SPLINE_SURFACE(1,2,((#150546,#150547,#150548),(#150549,#150550,#150551)),
 .UNSPECIFIED.,.F.,.F.,.F.)
B_SPLINE_SURFACE_WITH_KNOTS((2,2),(3,3),(0.710192959006957,1.),(0.107982157956011,
0.125273655815328),.UNSPECIFIED.)
GEOMETRIC_REPRESENTATION_ITEM()
RATIONAL_B_SPLINE_SURFACE(((0.987470879370255,0.98761351460672,0.990694758798812),
(0.987470879370255,0.98761351460672,0.990694758798812)))
REPRESENTATION_ITEM('')
SURFACE()
);
#3300=(
BOUNDED_SURFACE()
B_SPLINE_SURFACE(1,2,((#150558,#150559,#150560,#150561,#150562),(#150563,
#150564,#150565,#150566,#150567)),.UNSPECIFIED.,.F.,.F.,.F.)
B_SPLINE_SURFACE_WITH_KNOTS((2,2),(3,2,3),(0.709719018620996,1.),(0.607879027750092,
0.625170525609408,0.625770422841884),.UNSPECIFIED.)
GEOMETRIC_REPRESENTATION_ITEM()
RATIONAL_B_SPLINE_SURFACE(((0.987469282487682,0.987594391229382,0.990658108926709,
0.990658108926709,0.990658108926709),(0.987469282487682,0.987594391229382,
0.990658108926709,0.990658108926709,0.990658108926709)))
REPRESENTATION_ITEM('')
SURFACE()
);
#3301=(
BOUNDED_SURFACE()
B_SPLINE_SURFACE(1,2,((#150585,#150586,#150587),(#150588,#150589,#150590)),
 .UNSPECIFIED.,.F.,.F.,.F.)
B_SPLINE_SURFACE_WITH_KNOTS((2,2),(3,3),(0.710192959006483,1.),(0.107982157956011,
0.125273655815328),.UNSPECIFIED.)
GEOMETRIC_REPRESENTATION_ITEM()
RATIONAL_B_SPLINE_SURFACE(((0.987470879370255,0.98761351460672,0.990694758798812),
(0.987470879370255,0.98761351460672,0.990694758798812)))
REPRESENTATION_ITEM('')
SURFACE()
);
#3302=(
BOUNDED_SURFACE()
B_SPLINE_SURFACE(1,2,((#150597,#150598,#150599,#150600,#150601),(#150602,
#150603,#150604,#150605,#150606)),.UNSPECIFIED.,.F.,.F.,.F.)
B_SPLINE_SURFACE_WITH_KNOTS((2,2),(3,2,3),(0.709719018617797,1.),(0.607879027750092,
0.625170525609408,0.625770422845335),.UNSPECIFIED.)
GEOMETRIC_REPRESENTATION_ITEM()
RATIONAL_B_SPLINE_SURFACE(((0.987469282487682,0.987594391229382,0.990658108926709,
0.990658108926709,0.990658108926709),(0.987469282487682,0.987594391229382,
0.990658108926709,0.990658108926709,0.990658108926709)))
REPRESENTATION_ITEM('')
SURFACE()
);
#3303=(
BOUNDED_SURFACE()
B_SPLINE_SURFACE(1,2,((#150624,#150625,#150626),(#150627,#150628,#150629)),
 .UNSPECIFIED.,.F.,.F.,.F.)
B_SPLINE_SURFACE_WITH_KNOTS((2,2),(3,3),(0.710192959006736,1.),(0.107982157956011,
0.125273655815328),.UNSPECIFIED.)
GEOMETRIC_REPRESENTATION_ITEM()
RATIONAL_B_SPLINE_SURFACE(((0.987470879370255,0.98761351460672,0.990694758798812),
(0.987470879370255,0.98761351460672,0.990694758798812)))
REPRESENTATION_ITEM('')
SURFACE()
);
#3304=(
BOUNDED_SURFACE()
B_SPLINE_SURFACE(1,2,((#150636,#150637,#150638,#150639,#150640),(#150641,
#150642,#150643,#150644,#150645)),.UNSPECIFIED.,.F.,.F.,.F.)
B_SPLINE_SURFACE_WITH_KNOTS((2,2),(3,2,3),(0.70971901862028,1.),(0.607879027750092,
0.625170525609408,0.625770422841692),.UNSPECIFIED.)
GEOMETRIC_REPRESENTATION_ITEM()
RATIONAL_B_SPLINE_SURFACE(((0.987469282487682,0.987594391229382,0.990658108926709,
0.990658108926709,0.990658108926709),(0.987469282487682,0.987594391229382,
0.990658108926709,0.990658108926709,0.990658108926709)))
REPRESENTATION_ITEM('')
SURFACE()
);
#3305=(
BOUNDED_SURFACE()
B_SPLINE_SURFACE(1,2,((#150663,#150664,#150665),(#150666,#150667,#150668)),
 .UNSPECIFIED.,.F.,.F.,.F.)
B_SPLINE_SURFACE_WITH_KNOTS((2,2),(3,3),(0.710192959005573,1.),(0.107982157956011,
0.125273655815328),.UNSPECIFIED.)
GEOMETRIC_REPRESENTATION_ITEM()
RATIONAL_B_SPLINE_SURFACE(((0.987470879370255,0.98761351460672,0.990694758798812),
(0.987470879370255,0.98761351460672,0.990694758798812)))
REPRESENTATION_ITEM('')
SURFACE()
);
#3306=(
BOUNDED_SURFACE()
B_SPLINE_SURFACE(1,2,((#150675,#150676,#150677,#150678,#150679),(#150680,
#150681,#150682,#150683,#150684)),.UNSPECIFIED.,.F.,.F.,.F.)
B_SPLINE_SURFACE_WITH_KNOTS((2,2),(3,2,3),(0.709719018631225,1.),(0.607879027750092,
0.625170525609408,0.625770422832408),.UNSPECIFIED.)
GEOMETRIC_REPRESENTATION_ITEM()
RATIONAL_B_SPLINE_SURFACE(((0.987469282487682,0.987594391229382,0.990658108926709,
0.990658108926709,0.990658108926709),(0.987469282487682,0.987594391229382,
0.990658108926709,0.990658108926709,0.990658108926709)))
REPRESENTATION_ITEM('')
SURFACE()
);
#3307=(
BOUNDED_SURFACE()
B_SPLINE_SURFACE(1,2,((#150702,#150703,#150704),(#150705,#150706,#150707)),
 .UNSPECIFIED.,.F.,.F.,.F.)
B_SPLINE_SURFACE_WITH_KNOTS((2,2),(3,3),(0.710192959007235,1.),(0.107982157956011,
0.125273655815328),.UNSPECIFIED.)
GEOMETRIC_REPRESENTATION_ITEM()
RATIONAL_B_SPLINE_SURFACE(((0.987470879370255,0.98761351460672,0.990694758798812),
(0.987470879370255,0.98761351460672,0.990694758798812)))
REPRESENTATION_ITEM('')
SURFACE()
);
#3308=(
BOUNDED_SURFACE()
B_SPLINE_SURFACE(1,2,((#150714,#150715,#150716,#150717,#150718),(#150719,
#150720,#150721,#150722,#150723)),.UNSPECIFIED.,.F.,.F.,.F.)
B_SPLINE_SURFACE_WITH_KNOTS((2,2),(3,2,3),(0.709719018614688,1.),(0.607879027750092,
0.625170525609408,0.625770422849057),.UNSPECIFIED.)
GEOMETRIC_REPRESENTATION_ITEM()
RATIONAL_B_SPLINE_SURFACE(((0.987469282487682,0.987594391229382,0.990658108926709,
0.990658108926709,0.990658108926709),(0.987469282487682,0.987594391229382,
0.990658108926709,0.990658108926709,0.990658108926709)))
REPRESENTATION_ITEM('')
SURFACE()
);
#3309=(
BOUNDED_SURFACE()
B_SPLINE_SURFACE(1,2,((#150741,#150742,#150743),(#150744,#150745,#150746)),
 .UNSPECIFIED.,.F.,.F.,.F.)
B_SPLINE_SURFACE_WITH_KNOTS((2,2),(3,3),(0.710192959007356,1.),(0.107982157956011,
0.125273655815328),.UNSPECIFIED.)
GEOMETRIC_REPRESENTATION_ITEM()
RATIONAL_B_SPLINE_SURFACE(((0.987470879370255,0.98761351460672,0.990694758798812),
(0.987470879370255,0.98761351460672,0.990694758798812)))
REPRESENTATION_ITEM('')
SURFACE()
);
#3310=(
BOUNDED_SURFACE()
B_SPLINE_SURFACE(1,2,((#150753,#150754,#150755,#150756,#150757),(#150758,
#150759,#150760,#150761,#150762)),.UNSPECIFIED.,.F.,.F.,.F.)
B_SPLINE_SURFACE_WITH_KNOTS((2,2),(3,2,3),(0.710057850970234,1.),(0.607879027750092,
0.625170525609408,0.625431590492668),.UNSPECIFIED.)
GEOMETRIC_REPRESENTATION_ITEM()
RATIONAL_B_SPLINE_SURFACE(((0.987469282487682,0.987594391229382,0.990658108926709,
0.990658108926709,0.990658108926709),(0.987469282487682,0.987594391229382,
0.990658108926709,0.990658108926709,0.990658108926709)))
REPRESENTATION_ITEM('')
SURFACE()
);
#3311=(
BOUNDED_SURFACE()
B_SPLINE_SURFACE(1,2,((#150770,#150771,#150772),(#150773,#150774,#150775)),
 .UNSPECIFIED.,.F.,.F.,.F.)
B_SPLINE_SURFACE_WITH_KNOTS((2,2),(3,3),(0.710192959006505,1.),(0.107982157956011,
0.125273655815328),.UNSPECIFIED.)
GEOMETRIC_REPRESENTATION_ITEM()
RATIONAL_B_SPLINE_SURFACE(((0.987470879370255,0.987613514606721,0.990694758798812),
(0.987470879370255,0.98761351460672,0.990694758798812)))
REPRESENTATION_ITEM('')
SURFACE()
);
#3312=(
BOUNDED_SURFACE()
B_SPLINE_SURFACE(1,2,((#150777,#150778,#150779,#150780,#150781),(#150782,
#150783,#150784,#150785,#150786)),.UNSPECIFIED.,.F.,.F.,.F.)
B_SPLINE_SURFACE_WITH_KNOTS((2,2),(3,2,3),(0.709719018638398,1.),(0.607879027750092,
0.62517052560941,0.625770422825979),.UNSPECIFIED.)
GEOMETRIC_REPRESENTATION_ITEM()
RATIONAL_B_SPLINE_SURFACE(((0.987469282487682,0.987594391229382,0.990658108926709,
0.990658108926709,0.990658108926709),(0.987469282487682,0.987594391229382,
0.990658108926709,0.990658108926709,0.990658108926709)))
REPRESENTATION_ITEM('')
SURFACE()
);
#3313=(
BOUNDED_SURFACE()
B_SPLINE_SURFACE(1,2,((#150804,#150805,#150806),(#150807,#150808,#150809)),
 .UNSPECIFIED.,.F.,.F.,.F.)
B_SPLINE_SURFACE_WITH_KNOTS((2,2),(3,3),(0.710192959007984,1.),(0.107982157956011,
0.125273655815332),.UNSPECIFIED.)
GEOMETRIC_REPRESENTATION_ITEM()
RATIONAL_B_SPLINE_SURFACE(((0.987470879370255,0.987613514606721,0.990694758798814),
(0.987470879370255,0.987613514606721,0.990694758798814)))
REPRESENTATION_ITEM('')
SURFACE()
);
#3314=(
BOUNDED_SURFACE()
B_SPLINE_SURFACE(1,2,((#150816,#150817,#150818,#150819,#150820),(#150821,
#150822,#150823,#150824,#150825)),.UNSPECIFIED.,.F.,.F.,.F.)
B_SPLINE_SURFACE_WITH_KNOTS((2,2),(3,2,3),(0.709719018635918,1.),(0.607879027750092,
0.625170525609409,0.625770422827588),.UNSPECIFIED.)
GEOMETRIC_REPRESENTATION_ITEM()
RATIONAL_B_SPLINE_SURFACE(((0.987469282487682,0.987594391229382,0.990658108926709,
0.990658108926709,0.990658108926709),(0.987469282487682,0.987594391229382,
0.990658108926709,0.990658108926709,0.990658108926709)))
REPRESENTATION_ITEM('')
SURFACE()
);
#3315=(
BOUNDED_SURFACE()
B_SPLINE_SURFACE(1,2,((#150843,#150844,#150845),(#150846,#150847,#150848)),
 .UNSPECIFIED.,.F.,.F.,.F.)
B_SPLINE_SURFACE_WITH_KNOTS((2,2),(3,3),(0.710192959007116,1.),(0.107982157956011,
0.125273655815328),.UNSPECIFIED.)
GEOMETRIC_REPRESENTATION_ITEM()
RATIONAL_B_SPLINE_SURFACE(((0.987470879370255,0.98761351460672,0.990694758798812),
(0.987470879370255,0.98761351460672,0.990694758798812)))
REPRESENTATION_ITEM('')
SURFACE()
);
#3316=(
BOUNDED_SURFACE()
B_SPLINE_SURFACE(1,2,((#150855,#150856,#150857,#150858,#150859),(#150860,
#150861,#150862,#150863,#150864)),.UNSPECIFIED.,.F.,.F.,.F.)
B_SPLINE_SURFACE_WITH_KNOTS((2,2),(3,2,3),(0.709719018610881,1.),(0.607879027750092,
0.625170525609408,0.625770422852824),.UNSPECIFIED.)
GEOMETRIC_REPRESENTATION_ITEM()
RATIONAL_B_SPLINE_SURFACE(((0.987469282487682,0.987594391229382,0.990658108926709,
0.990658108926709,0.990658108926709),(0.987469282487682,0.987594391229382,
0.990658108926709,0.990658108926709,0.990658108926709)))
REPRESENTATION_ITEM('')
SURFACE()
);
#3317=(
BOUNDED_SURFACE()
B_SPLINE_SURFACE(1,2,((#150882,#150883,#150884),(#150885,#150886,#150887)),
 .UNSPECIFIED.,.F.,.F.,.F.)
B_SPLINE_SURFACE_WITH_KNOTS((2,2),(3,3),(0.71019295900731,1.),(0.107982157956012,
0.125273655815328),.UNSPECIFIED.)
GEOMETRIC_REPRESENTATION_ITEM()
RATIONAL_B_SPLINE_SURFACE(((0.987470879370256,0.987613514606721,0.990694758798813),
(0.987470879370256,0.987613514606721,0.990694758798813)))
REPRESENTATION_ITEM('')
SURFACE()
);
#3318=(
BOUNDED_SURFACE()
B_SPLINE_SURFACE(1,2,((#150894,#150895,#150896,#150897,#150898),(#150899,
#150900,#150901,#150902,#150903)),.UNSPECIFIED.,.F.,.F.,.F.)
B_SPLINE_SURFACE_WITH_KNOTS((2,2),(3,2,3),(0.709719018631712,1.),(0.607879027750091,
0.625170525609408,0.625770422833119),.UNSPECIFIED.)
GEOMETRIC_REPRESENTATION_ITEM()
RATIONAL_B_SPLINE_SURFACE(((0.987469282487682,0.987594391229382,0.990658108926708,
0.990658108926708,0.990658108926708),(0.987469282487682,0.987594391229382,
0.990658108926708,0.990658108926708,0.990658108926708)))
REPRESENTATION_ITEM('')
SURFACE()
);
#3319=(
BOUNDED_SURFACE()
B_SPLINE_SURFACE(1,2,((#150921,#150922,#150923),(#150924,#150925,#150926)),
 .UNSPECIFIED.,.F.,.F.,.F.)
B_SPLINE_SURFACE_WITH_KNOTS((2,2),(3,3),(0.710192959008443,1.),(0.107982157956012,
0.125273655815329),.UNSPECIFIED.)
GEOMETRIC_REPRESENTATION_ITEM()
RATIONAL_B_SPLINE_SURFACE(((0.987470879370256,0.987613514606721,0.990694758798813),
(0.987470879370256,0.987613514606721,0.990694758798813)))
REPRESENTATION_ITEM('')
SURFACE()
);
#3320=(
BOUNDED_SURFACE()
B_SPLINE_SURFACE(1,2,((#150933,#150934,#150935,#150936,#150937),(#150938,
#150939,#150940,#150941,#150942)),.UNSPECIFIED.,.F.,.F.,.F.)
B_SPLINE_SURFACE_WITH_KNOTS((2,2),(3,2,3),(0.709719018622383,1.),(0.607879027750091,
0.625170525609407,0.625770422842453),.UNSPECIFIED.)
GEOMETRIC_REPRESENTATION_ITEM()
RATIONAL_B_SPLINE_SURFACE(((0.987469282487682,0.987594391229382,0.990658108926708,
0.990658108926708,0.990658108926708),(0.987469282487682,0.987594391229382,
0.990658108926709,0.990658108926709,0.990658108926709)))
REPRESENTATION_ITEM('')
SURFACE()
);
#3321=(
BOUNDED_SURFACE()
B_SPLINE_SURFACE(1,2,((#150960,#150961,#150962),(#150963,#150964,#150965)),
 .UNSPECIFIED.,.F.,.F.,.F.)
B_SPLINE_SURFACE_WITH_KNOTS((2,2),(3,3),(0.710192959008445,1.),(0.107982157956012,
0.125273655815329),.UNSPECIFIED.)
GEOMETRIC_REPRESENTATION_ITEM()
RATIONAL_B_SPLINE_SURFACE(((0.987470879370256,0.987613514606721,0.990694758798813),
(0.987470879370256,0.987613514606721,0.990694758798813)))
REPRESENTATION_ITEM('')
SURFACE()
);
#3322=(
BOUNDED_SURFACE()
B_SPLINE_SURFACE(1,2,((#150972,#150973,#150974,#150975,#150976),(#150977,
#150978,#150979,#150980,#150981)),.UNSPECIFIED.,.F.,.F.,.F.)
B_SPLINE_SURFACE_WITH_KNOTS((2,2),(3,2,3),(0.70971901863218,1.),(0.607879027750091,
0.625170525609407,0.62577042283265),.UNSPECIFIED.)
GEOMETRIC_REPRESENTATION_ITEM()
RATIONAL_B_SPLINE_SURFACE(((0.987469282487682,0.987594391229382,0.990658108926708,
0.990658108926708,0.990658108926708),(0.987469282487682,0.987594391229382,
0.990658108926709,0.990658108926709,0.990658108926709)))
REPRESENTATION_ITEM('')
SURFACE()
);
#3323=(
BOUNDED_SURFACE()
B_SPLINE_SURFACE(1,2,((#150999,#151000,#151001),(#151002,#151003,#151004)),
 .UNSPECIFIED.,.F.,.F.,.F.)
B_SPLINE_SURFACE_WITH_KNOTS((2,2),(3,3),(0.710192959008444,1.),(0.107982157956012,
0.125273655815329),.UNSPECIFIED.)
GEOMETRIC_REPRESENTATION_ITEM()
RATIONAL_B_SPLINE_SURFACE(((0.987470879370256,0.987613514606721,0.990694758798813),
(0.987470879370256,0.987613514606721,0.990694758798813)))
REPRESENTATION_ITEM('')
SURFACE()
);
#3324=(
BOUNDED_SURFACE()
B_SPLINE_SURFACE(1,2,((#151011,#151012,#151013,#151014,#151015),(#151016,
#151017,#151018,#151019,#151020)),.UNSPECIFIED.,.F.,.F.,.F.)
B_SPLINE_SURFACE_WITH_KNOTS((2,2),(3,2,3),(0.70971901862027,1.),(0.607879027750091,
0.625170525609407,0.625770422844233),.UNSPECIFIED.)
GEOMETRIC_REPRESENTATION_ITEM()
RATIONAL_B_SPLINE_SURFACE(((0.987469282487682,0.987594391229382,0.990658108926708,
0.990658108926708,0.990658108926708),(0.987469282487682,0.987594391229382,
0.990658108926709,0.990658108926709,0.990658108926709)))
REPRESENTATION_ITEM('')
SURFACE()
);
#3325=(
BOUNDED_SURFACE()
B_SPLINE_SURFACE(1,2,((#151038,#151039,#151040),(#151041,#151042,#151043)),
 .UNSPECIFIED.,.F.,.F.,.F.)
B_SPLINE_SURFACE_WITH_KNOTS((2,2),(3,3),(0.710192959008112,1.),(0.107982157956012,
0.125273655815329),.UNSPECIFIED.)
GEOMETRIC_REPRESENTATION_ITEM()
RATIONAL_B_SPLINE_SURFACE(((0.987470879370256,0.987613514606721,0.990694758798813),
(0.987470879370256,0.987613514606721,0.990694758798813)))
REPRESENTATION_ITEM('')
SURFACE()
);
#3326=(
BOUNDED_SURFACE()
B_SPLINE_SURFACE(1,2,((#151050,#151051,#151052,#151053,#151054),(#151055,
#151056,#151057,#151058,#151059)),.UNSPECIFIED.,.F.,.F.,.F.)
B_SPLINE_SURFACE_WITH_KNOTS((2,2),(3,2,3),(0.709590617367083,1.),(0.573052008420699,
0.573654350219791,0.591014490232052),.UNSPECIFIED.)
GEOMETRIC_REPRESENTATION_ITEM()
RATIONAL_B_SPLINE_SURFACE(((0.998486152291959,0.998486152291959,0.998486152291959,
0.99277234517203,0.990020524139833),(0.998486152291959,0.998486152291959,
0.998486152291959,0.99277234517203,0.990020524139833)))
REPRESENTATION_ITEM('')
SURFACE()
);
#3327=(
BOUNDED_SURFACE()
B_SPLINE_SURFACE(1,2,((#151068,#151069,#151070,#151071,#151072),(#151073,
#151074,#151075,#151076,#151077)),.UNSPECIFIED.,.F.,.F.,.F.)
B_SPLINE_SURFACE_WITH_KNOTS((2,2),(3,2,3),(0.710318915640075,1.),(0.142474614281353,
0.142857142857143,0.159901408087482),.UNSPECIFIED.)
GEOMETRIC_REPRESENTATION_ITEM()
RATIONAL_B_SPLINE_SURFACE(((0.999732896029228,0.999865728939368,1.,0.994017305594881,
0.990889788836284),(0.999732896029228,0.999865728939368,1.,0.994017305594881,
0.990889788836284)))
REPRESENTATION_ITEM('')
SURFACE()
);
#3328=(
BOUNDED_SURFACE()
B_SPLINE_SURFACE(1,2,((#151079,#151080,#151081,#151082,#151083),(#151084,
#151085,#151086,#151087,#151088)),.UNSPECIFIED.,.F.,.F.,.F.)
B_SPLINE_SURFACE_WITH_KNOTS((2,2),(3,2,3),(0.709590617386171,1.),(0.573052008439665,
0.573654350219722,0.591014490232053),.UNSPECIFIED.)
GEOMETRIC_REPRESENTATION_ITEM()
RATIONAL_B_SPLINE_SURFACE(((0.998486152292004,0.998486152292004,0.998486152292004,
0.992772345172041,0.990020524139833),(0.998486152292004,0.998486152292004,
0.998486152292004,0.992772345172041,0.990020524139833)))
REPRESENTATION_ITEM('')
SURFACE()
);
#3329=(
BOUNDED_SURFACE()
B_SPLINE_SURFACE(1,2,((#151097,#151098,#151099,#151100,#151101),(#151102,
#151103,#151104,#151105,#151106)),.UNSPECIFIED.,.F.,.F.,.F.)
B_SPLINE_SURFACE_WITH_KNOTS((2,2),(3,2,3),(0.710318915640081,1.),(0.142474614281357,
0.142857142857143,0.159901408087483),.UNSPECIFIED.)
GEOMETRIC_REPRESENTATION_ITEM()
RATIONAL_B_SPLINE_SURFACE(((0.999732896029231,0.999865728939369,1.,0.994017305594881,
0.990889788836284),(0.999732896029231,0.999865728939369,1.,0.994017305594881,
0.990889788836284)))
REPRESENTATION_ITEM('')
SURFACE()
);
#3330=(
BOUNDED_SURFACE()
B_SPLINE_SURFACE(1,2,((#151108,#151109,#151110,#151111,#151112),(#151113,
#151114,#151115,#151116,#151117)),.UNSPECIFIED.,.F.,.F.,.F.)
B_SPLINE_SURFACE_WITH_KNOTS((2,2),(3,2,3),(0.709590617383039,1.),(0.573052008436687,
0.57365435021991,0.591014490232044),.UNSPECIFIED.)
GEOMETRIC_REPRESENTATION_ITEM()
RATIONAL_B_SPLINE_SURFACE(((0.99848615229188,0.99848615229188,0.99848615229188,
0.992772345172014,0.990020524139836),(0.99848615229188,0.99848615229188,
0.99848615229188,0.992772345172014,0.990020524139836)))
REPRESENTATION_ITEM('')
SURFACE()
);
#3331=(
BOUNDED_SURFACE()
B_SPLINE_SURFACE(1,2,((#151126,#151127,#151128,#151129,#151130),(#151131,
#151132,#151133,#151134,#151135)),.UNSPECIFIED.,.F.,.F.,.F.)
B_SPLINE_SURFACE_WITH_KNOTS((2,2),(3,2,3),(0.710318915640083,1.),(0.142474614281355,
0.142857142857143,0.159901408087481),.UNSPECIFIED.)
GEOMETRIC_REPRESENTATION_ITEM()
RATIONAL_B_SPLINE_SURFACE(((0.999732896029229,0.999865728939368,1.,0.994017305594881,
0.990889788836284),(0.999732896029229,0.999865728939368,1.,0.994017305594881,
0.990889788836284)))
REPRESENTATION_ITEM('')
SURFACE()
);
#3332=(
BOUNDED_SURFACE()
B_SPLINE_SURFACE(1,2,((#151137,#151138,#151139,#151140,#151141),(#151142,
#151143,#151144,#151145,#151146)),.UNSPECIFIED.,.F.,.F.,.F.)
B_SPLINE_SURFACE_WITH_KNOTS((2,2),(3,2,3),(0.709590617387445,1.),(0.573052008441487,
0.573654350219663,0.591014490232054),.UNSPECIFIED.)
GEOMETRIC_REPRESENTATION_ITEM()
RATIONAL_B_SPLINE_SURFACE(((0.998486152292043,0.998486152292043,0.998486152292043,
0.99277234517205,0.990020524139832),(0.998486152292043,0.998486152292043,
0.998486152292043,0.99277234517205,0.990020524139832)))
REPRESENTATION_ITEM('')
SURFACE()
);
#3333=(
BOUNDED_SURFACE()
B_SPLINE_SURFACE(1,2,((#151155,#151156,#151157,#151158,#151159),(#151160,
#151161,#151162,#151163,#151164),(#151165,#151166,#151167,#151168,#151169)),
 .UNSPECIFIED.,.F.,.F.,.F.)
B_SPLINE_SURFACE_WITH_KNOTS((2,1,2),(3,2,3),(0.710318915640077,1.,1.0028968108436),
(0.14247461428136,0.142857142857143,0.159901408087481),.UNSPECIFIED.)
GEOMETRIC_REPRESENTATION_ITEM()
RATIONAL_B_SPLINE_SURFACE(((0.999732896029233,0.99986572893937,1.,0.994017305594881,
0.990889788836284),(0.999732896029233,0.99986572893937,1.,0.994017305594881,
0.990889788836284),(0.999732896029233,0.99986572893937,1.,0.994017305594881,
0.990889788836284)))
REPRESENTATION_ITEM('')
SURFACE()
);
#3334=(
BOUNDED_SURFACE()
B_SPLINE_SURFACE(1,2,((#151171,#151172,#151173,#151174,#151175),(#151176,
#151177,#151178,#151179,#151180)),.UNSPECIFIED.,.F.,.F.,.F.)
B_SPLINE_SURFACE_WITH_KNOTS((2,2),(3,2,3),(0.710192959008438,1.),(0.573480748819672,
0.573654350219794,0.59101449023205),.UNSPECIFIED.)
GEOMETRIC_REPRESENTATION_ITEM()
RATIONAL_B_SPLINE_SURFACE(((0.998486152291957,0.998486152291957,0.998486152291957,
0.992772345172031,0.990020524139834),(0.998486152291957,0.998486152291957,
0.998486152291957,0.992772345172031,0.990020524139834)))
REPRESENTATION_ITEM('')
SURFACE()
);
#3335=(
BOUNDED_SURFACE()
B_SPLINE_SURFACE(1,2,((#151189,#151190,#151191,#151192,#151193),(#151194,
#151195,#151196,#151197,#151198),(#151199,#151200,#151201,#151202,#151203)),
 .UNSPECIFIED.,.F.,.F.,.F.)
B_SPLINE_SURFACE_WITH_KNOTS((2,1,2),(3,2,3),(0.710318915640083,1.,1.0028968108436),
(0.142474614281359,0.142857142857143,0.159901408087481),.UNSPECIFIED.)
GEOMETRIC_REPRESENTATION_ITEM()
RATIONAL_B_SPLINE_SURFACE(((0.999732896029232,0.99986572893937,1.,0.994017305594881,
0.990889788836284),(0.999732896029232,0.99986572893937,1.,0.994017305594881,
0.990889788836284),(0.999732896029232,0.99986572893937,1.,0.994017305594881,
0.990889788836284)))
REPRESENTATION_ITEM('')
SURFACE()
);
#3336=(
BOUNDED_SURFACE()
B_SPLINE_SURFACE(1,2,((#151205,#151206,#151207,#151208,#151209),(#151210,
#151211,#151212,#151213,#151214)),.UNSPECIFIED.,.F.,.F.,.F.)
B_SPLINE_SURFACE_WITH_KNOTS((2,2),(3,2,3),(0.71019295900844,1.),(0.57348074881979,
0.573654350219911,0.591014490232053),.UNSPECIFIED.)
GEOMETRIC_REPRESENTATION_ITEM()
RATIONAL_B_SPLINE_SURFACE(((0.99848615229188,0.99848615229188,0.99848615229188,
0.992772345172011,0.990020524139833),(0.99848615229188,0.99848615229188,
0.99848615229188,0.992772345172011,0.990020524139833)))
REPRESENTATION_ITEM('')
SURFACE()
);
#3337=(
BOUNDED_SURFACE()
B_SPLINE_SURFACE(1,2,((#151223,#151224,#151225,#151226,#151227),(#151228,
#151229,#151230,#151231,#151232)),.UNSPECIFIED.,.F.,.F.,.F.)
B_SPLINE_SURFACE_WITH_KNOTS((2,2),(3,2,3),(0.710318915640079,1.),(0.142474614281366,
0.142857142857143,0.159901408087481),.UNSPECIFIED.)
GEOMETRIC_REPRESENTATION_ITEM()
RATIONAL_B_SPLINE_SURFACE(((0.999732896029237,0.999865728939372,1.,0.994017305594881,
0.990889788836284),(0.999732896029237,0.999865728939372,1.,0.994017305594881,
0.990889788836284)))
REPRESENTATION_ITEM('')
SURFACE()
);
#3338=(
BOUNDED_SURFACE()
B_SPLINE_SURFACE(1,2,((#151234,#151235,#151236,#151237,#151238),(#151239,
#151240,#151241,#151242,#151243)),.UNSPECIFIED.,.F.,.F.,.F.)
B_SPLINE_SURFACE_WITH_KNOTS((2,2),(3,2,3),(0.709590617369615,1.),(0.573052008423653,
0.573654350219911,0.591014490232053),.UNSPECIFIED.)
GEOMETRIC_REPRESENTATION_ITEM()
RATIONAL_B_SPLINE_SURFACE(((0.99848615229188,0.99848615229188,0.99848615229188,
0.992772345172011,0.990020524139833),(0.99848615229188,0.99848615229188,
0.99848615229188,0.992772345172011,0.990020524139833)))
REPRESENTATION_ITEM('')
SURFACE()
);
#3339=(
BOUNDED_SURFACE()
B_SPLINE_SURFACE(1,2,((#151252,#151253,#151254,#151255,#151256),(#151257,
#151258,#151259,#151260,#151261)),.UNSPECIFIED.,.F.,.F.,.F.)
B_SPLINE_SURFACE_WITH_KNOTS((2,2),(3,2,3),(0.710318915640074,1.),(0.142474614281351,
0.142857142857143,0.159901408087481),.UNSPECIFIED.)
GEOMETRIC_REPRESENTATION_ITEM()
RATIONAL_B_SPLINE_SURFACE(((0.999732896029227,0.999865728939367,1.,0.994017305594881,
0.990889788836284),(0.999732896029227,0.999865728939367,1.,0.994017305594881,
0.990889788836284)))
REPRESENTATION_ITEM('')
SURFACE()
);
#3340=(
BOUNDED_SURFACE()
B_SPLINE_SURFACE(1,2,((#151263,#151264,#151265,#151266,#151267),(#151268,
#151269,#151270,#151271,#151272)),.UNSPECIFIED.,.F.,.F.,.F.)
B_SPLINE_SURFACE_WITH_KNOTS((2,2),(3,2,3),(0.709590617376943,1.),(0.57305200846928,
0.573654350219911,0.591014490232042),.UNSPECIFIED.)
GEOMETRIC_REPRESENTATION_ITEM()
RATIONAL_B_SPLINE_SURFACE(((0.99848615229188,0.99848615229188,0.99848615229188,
0.992772345172015,0.990020524139836),(0.99848615229188,0.99848615229188,
0.99848615229188,0.992772345172015,0.990020524139836)))
REPRESENTATION_ITEM('')
SURFACE()
);
#3341=(
BOUNDED_SURFACE()
B_SPLINE_SURFACE(1,2,((#151281,#151282,#151283,#151284,#151285),(#151286,
#151287,#151288,#151289,#151290)),.UNSPECIFIED.,.F.,.F.,.F.)
B_SPLINE_SURFACE_WITH_KNOTS((2,2),(3,2,3),(0.71031891564008,1.),(0.14247461428135,
0.142857142857143,0.159901408087481),.UNSPECIFIED.)
GEOMETRIC_REPRESENTATION_ITEM()
RATIONAL_B_SPLINE_SURFACE(((0.999732896029226,0.999865728939367,1.,0.994017305594881,
0.990889788836284),(0.999732896029226,0.999865728939367,1.,0.994017305594881,
0.990889788836284)))
REPRESENTATION_ITEM('')
SURFACE()
);
#3342=(
BOUNDED_SURFACE()
B_SPLINE_SURFACE(1,2,((#151292,#151293,#151294,#151295,#151296),(#151297,
#151298,#151299,#151300,#151301)),.UNSPECIFIED.,.F.,.F.,.F.)
B_SPLINE_SURFACE_WITH_KNOTS((2,2),(3,2,3),(0.70959061736192,1.),(0.573052008416099,
0.573654350219911,0.591014490232053),.UNSPECIFIED.)
GEOMETRIC_REPRESENTATION_ITEM()
RATIONAL_B_SPLINE_SURFACE(((0.99848615229188,0.99848615229188,0.99848615229188,
0.992772345172011,0.990020524139833),(0.99848615229188,0.99848615229188,
0.99848615229188,0.992772345172011,0.990020524139833)))
REPRESENTATION_ITEM('')
SURFACE()
);
#3343=(
BOUNDED_SURFACE()
B_SPLINE_SURFACE(1,2,((#151310,#151311,#151312,#151313,#151314),(#151315,
#151316,#151317,#151318,#151319)),.UNSPECIFIED.,.F.,.F.,.F.)
B_SPLINE_SURFACE_WITH_KNOTS((2,2),(3,2,3),(0.710318915640078,1.),(0.142474614281354,
0.142857142857143,0.159901408087481),.UNSPECIFIED.)
GEOMETRIC_REPRESENTATION_ITEM()
RATIONAL_B_SPLINE_SURFACE(((0.999732896029229,0.999865728939368,1.,0.994017305594881,
0.990889788836284),(0.999732896029229,0.999865728939368,1.,0.994017305594881,
0.990889788836284)))
REPRESENTATION_ITEM('')
SURFACE()
);
#3344=(
BOUNDED_SURFACE()
B_SPLINE_SURFACE(1,2,((#151321,#151322,#151323,#151324,#151325),(#151326,
#151327,#151328,#151329,#151330)),.UNSPECIFIED.,.F.,.F.,.F.)
B_SPLINE_SURFACE_WITH_KNOTS((2,2),(3,2,3),(0.709590617385339,1.),(0.573052008438801,
0.573654350219911,0.591014490232053),.UNSPECIFIED.)
GEOMETRIC_REPRESENTATION_ITEM()
RATIONAL_B_SPLINE_SURFACE(((0.99848615229188,0.99848615229188,0.99848615229188,
0.992772345172011,0.990020524139833),(0.99848615229188,0.99848615229188,
0.99848615229188,0.992772345172011,0.990020524139833)))
REPRESENTATION_ITEM('')
SURFACE()
);
#3345=(
BOUNDED_SURFACE()
B_SPLINE_SURFACE(1,2,((#151339,#151340,#151341,#151342,#151343),(#151344,
#151345,#151346,#151347,#151348)),.UNSPECIFIED.,.F.,.F.,.F.)
B_SPLINE_SURFACE_WITH_KNOTS((2,2),(3,2,3),(0.710318915640077,1.),(0.142474614281367,
0.142857142857143,0.159901408087482),.UNSPECIFIED.)
GEOMETRIC_REPRESENTATION_ITEM()
RATIONAL_B_SPLINE_SURFACE(((0.999732896029237,0.999865728939372,1.,0.994017305594881,
0.990889788836284),(0.999732896029237,0.999865728939372,1.,0.994017305594881,
0.990889788836284)))
REPRESENTATION_ITEM('')
SURFACE()
);
#3346=(
BOUNDED_SURFACE()
B_SPLINE_SURFACE(1,2,((#151350,#151351,#151352,#151353,#151354),(#151355,
#151356,#151357,#151358,#151359)),.UNSPECIFIED.,.F.,.F.,.F.)
B_SPLINE_SURFACE_WITH_KNOTS((2,2),(3,2,3),(0.709590617381935,1.),(0.573052008435693,
0.573654350219837,0.591014490232053),.UNSPECIFIED.)
GEOMETRIC_REPRESENTATION_ITEM()
RATIONAL_B_SPLINE_SURFACE(((0.998486152291929,0.998486152291929,0.998486152291929,
0.992772345172023,0.990020524139833),(0.998486152291929,0.998486152291929,
0.998486152291929,0.992772345172023,0.990020524139833)))
REPRESENTATION_ITEM('')
SURFACE()
);
#3347=(
BOUNDED_SURFACE()
B_SPLINE_SURFACE(1,2,((#151368,#151369,#151370,#151371,#151372),(#151373,
#151374,#151375,#151376,#151377),(#151378,#151379,#151380,#151381,#151382)),
 .UNSPECIFIED.,.F.,.F.,.F.)
B_SPLINE_SURFACE_WITH_KNOTS((2,1,2),(3,2,3),(0.710318915640078,1.,1.0028968108436),
(0.142474614281367,0.142857142857143,0.159901408087481),.UNSPECIFIED.)
GEOMETRIC_REPRESENTATION_ITEM()
RATIONAL_B_SPLINE_SURFACE(((0.999732896029237,0.999865728939372,1.,0.994017305594881,
0.990889788836284),(0.999732896029237,0.999865728939372,1.,0.994017305594881,
0.990889788836284),(0.999732896029237,0.999865728939372,1.,0.994017305594881,
0.990889788836284)))
REPRESENTATION_ITEM('')
SURFACE()
);
#3348=(
BOUNDED_SURFACE()
B_SPLINE_SURFACE(1,2,((#151384,#151385,#151386,#151387,#151388),(#151389,
#151390,#151391,#151392,#151393)),.UNSPECIFIED.,.F.,.F.,.F.)
B_SPLINE_SURFACE_WITH_KNOTS((2,2),(3,2,3),(0.709590617367086,1.),(0.573052008457203,
0.573654350219911,0.591014490232053),.UNSPECIFIED.)
GEOMETRIC_REPRESENTATION_ITEM()
RATIONAL_B_SPLINE_SURFACE(((0.99848615229188,0.99848615229188,0.99848615229188,
0.992772345172011,0.990020524139833),(0.99848615229188,0.99848615229188,
0.99848615229188,0.992772345172011,0.990020524139833)))
REPRESENTATION_ITEM('')
SURFACE()
);
#3349=(
BOUNDED_SURFACE()
B_SPLINE_SURFACE(1,2,((#151402,#151403,#151404,#151405,#151406),(#151407,
#151408,#151409,#151410,#151411)),.UNSPECIFIED.,.F.,.F.,.F.)
B_SPLINE_SURFACE_WITH_KNOTS((2,2),(3,2,3),(0.710318915640077,1.),(0.142474614281296,
0.142857142857143,0.159901408087481),.UNSPECIFIED.)
GEOMETRIC_REPRESENTATION_ITEM()
RATIONAL_B_SPLINE_SURFACE(((0.999732896029188,0.999865728939348,1.,0.994017305594881,
0.990889788836284),(0.999732896029188,0.999865728939348,1.,0.994017305594881,
0.990889788836284)))
REPRESENTATION_ITEM('')
SURFACE()
);
#3350=(
BOUNDED_SURFACE()
B_SPLINE_SURFACE(1,2,((#151413,#151414,#151415,#151416,#151417),(#151418,
#151419,#151420,#151421,#151422)),.UNSPECIFIED.,.F.,.F.,.F.)
B_SPLINE_SURFACE_WITH_KNOTS((2,2),(3,2,3),(0.709590617387075,1.),(0.573052008477772,
0.573654350219911,0.591014490232053),.UNSPECIFIED.)
GEOMETRIC_REPRESENTATION_ITEM()
RATIONAL_B_SPLINE_SURFACE(((0.99848615229188,0.99848615229188,0.99848615229188,
0.992772345172011,0.990020524139833),(0.99848615229188,0.99848615229188,
0.99848615229188,0.992772345172011,0.990020524139833)))
REPRESENTATION_ITEM('')
SURFACE()
);
#3351=(
BOUNDED_SURFACE()
B_SPLINE_SURFACE(1,2,((#151431,#151432,#151433,#151434,#151435),(#151436,
#151437,#151438,#151439,#151440)),.UNSPECIFIED.,.F.,.F.,.F.)
B_SPLINE_SURFACE_WITH_KNOTS((2,2),(3,2,3),(0.710318915640081,1.),(0.142474614281367,
0.142857142857143,0.159901408087481),.UNSPECIFIED.)
GEOMETRIC_REPRESENTATION_ITEM()
RATIONAL_B_SPLINE_SURFACE(((0.999732896029237,0.999865728939372,1.,0.994017305594881,
0.990889788836284),(0.999732896029237,0.999865728939372,1.,0.994017305594881,
0.990889788836284)))
REPRESENTATION_ITEM('')
SURFACE()
);
#3352=(
BOUNDED_SURFACE()
B_SPLINE_SURFACE(1,2,((#151442,#151443,#151444,#151445,#151446),(#151447,
#151448,#151449,#151450,#151451)),.UNSPECIFIED.,.F.,.F.,.F.)
B_SPLINE_SURFACE_WITH_KNOTS((2,2),(3,2,3),(0.710192959008437,1.),(0.57348074881979,
0.573654350219911,0.591014490232053),.UNSPECIFIED.)
GEOMETRIC_REPRESENTATION_ITEM()
RATIONAL_B_SPLINE_SURFACE(((0.99848615229188,0.99848615229188,0.99848615229188,
0.992772345172011,0.990020524139833),(0.99848615229188,0.99848615229188,
0.99848615229188,0.992772345172011,0.990020524139833)))
REPRESENTATION_ITEM('')
SURFACE()
);
#3353=(
BOUNDED_SURFACE()
B_SPLINE_SURFACE(1,2,((#151460,#151461,#151462,#151463,#151464),(#151465,
#151466,#151467,#151468,#151469)),.UNSPECIFIED.,.F.,.F.,.F.)
B_SPLINE_SURFACE_WITH_KNOTS((2,2),(3,2,3),(0.710318915640077,1.),(0.142474614281367,
0.142857142857143,0.159901408087482),.UNSPECIFIED.)
GEOMETRIC_REPRESENTATION_ITEM()
RATIONAL_B_SPLINE_SURFACE(((0.999732896029237,0.999865728939372,1.,0.994017305594881,
0.990889788836284),(0.999732896029237,0.999865728939372,1.,0.994017305594881,
0.990889788836284)))
REPRESENTATION_ITEM('')
SURFACE()
);
#3354=(
BOUNDED_SURFACE()
B_SPLINE_SURFACE(1,2,((#151471,#151472,#151473,#151474,#151475),(#151476,
#151477,#151478,#151479,#151480)),.UNSPECIFIED.,.F.,.F.,.F.)
B_SPLINE_SURFACE_WITH_KNOTS((2,2),(3,2,3),(0.709968463042327,1.),(0.573429854103688,
0.573654350219911,0.591014490232053),.UNSPECIFIED.)
GEOMETRIC_REPRESENTATION_ITEM()
RATIONAL_B_SPLINE_SURFACE(((0.99848615229188,0.99848615229188,0.99848615229188,
0.992772345172011,0.990020524139833),(0.99848615229188,0.99848615229188,
0.99848615229188,0.992772345172011,0.990020524139833)))
REPRESENTATION_ITEM('')
SURFACE()
);
#3355=(
BOUNDED_SURFACE()
B_SPLINE_SURFACE(1,2,((#151489,#151490,#151491,#151492,#151493),(#151494,
#151495,#151496,#151497,#151498),(#151499,#151500,#151501,#151502,#151503)),
 .UNSPECIFIED.,.F.,.F.,.F.)
B_SPLINE_SURFACE_WITH_KNOTS((2,1,2),(3,2,3),(0.710318915640081,1.,1.0028968108436),
(0.142474614281367,0.142857142857143,0.159901408087482),.UNSPECIFIED.)
GEOMETRIC_REPRESENTATION_ITEM()
RATIONAL_B_SPLINE_SURFACE(((0.999732896029237,0.999865728939372,1.,0.994017305594881,
0.990889788836284),(0.999732896029237,0.999865728939372,1.,0.994017305594881,
0.990889788836284),(0.999732896029237,0.999865728939372,1.,0.994017305594881,
0.990889788836284)))
REPRESENTATION_ITEM('')
SURFACE()
);
#3356=(
BOUNDED_SURFACE()
B_SPLINE_SURFACE(1,2,((#151505,#151506,#151507,#151508,#151509),(#151510,
#151511,#151512,#151513,#151514)),.UNSPECIFIED.,.F.,.F.,.F.)
B_SPLINE_SURFACE_WITH_KNOTS((2,2),(3,2,3),(0.709590617371185,1.),(0.573052008461026,
0.573654350219911,0.591014490232053),.UNSPECIFIED.)
GEOMETRIC_REPRESENTATION_ITEM()
RATIONAL_B_SPLINE_SURFACE(((0.99848615229188,0.99848615229188,0.99848615229188,
0.992772345172011,0.990020524139833),(0.99848615229188,0.99848615229188,
0.99848615229188,0.992772345172011,0.990020524139833)))
REPRESENTATION_ITEM('')
SURFACE()
);
#3357=(
BOUNDED_SURFACE()
B_SPLINE_SURFACE(1,2,((#151523,#151524,#151525,#151526,#151527),(#151528,
#151529,#151530,#151531,#151532)),.UNSPECIFIED.,.F.,.F.,.F.)
B_SPLINE_SURFACE_WITH_KNOTS((2,2),(3,2,3),(0.71031891564008,1.),(0.142474614281085,
0.142857142857143,0.159901408087482),.UNSPECIFIED.)
GEOMETRIC_REPRESENTATION_ITEM()
RATIONAL_B_SPLINE_SURFACE(((0.999732896029042,0.999865728939274,1.,0.994017305594881,
0.990889788836284),(0.999732896029042,0.999865728939274,1.,0.994017305594881,
0.990889788836284)))
REPRESENTATION_ITEM('')
SURFACE()
);
#3358=(
BOUNDED_SURFACE()
B_SPLINE_SURFACE(1,2,((#151534,#151535,#151536,#151537,#151538),(#151539,
#151540,#151541,#151542,#151543)),.UNSPECIFIED.,.F.,.F.,.F.)
B_SPLINE_SURFACE_WITH_KNOTS((2,2),(3,2,3),(0.709590617399634,1.),(0.573052008453065,
0.573654350219911,0.591014490232053),.UNSPECIFIED.)
GEOMETRIC_REPRESENTATION_ITEM()
RATIONAL_B_SPLINE_SURFACE(((0.99848615229188,0.99848615229188,0.99848615229188,
0.992772345172011,0.990020524139833),(0.99848615229188,0.99848615229188,
0.99848615229188,0.992772345172011,0.990020524139833)))
REPRESENTATION_ITEM('')
SURFACE()
);
#3359=(
BOUNDED_SURFACE()
B_SPLINE_SURFACE(1,2,((#151552,#151553,#151554,#151555,#151556),(#151557,
#151558,#151559,#151560,#151561)),.UNSPECIFIED.,.F.,.F.,.F.)
B_SPLINE_SURFACE_WITH_KNOTS((2,2),(3,2,3),(0.710318915640076,1.),(0.142474614280958,
0.142857142857143,0.159901408087482),.UNSPECIFIED.)
GEOMETRIC_REPRESENTATION_ITEM()
RATIONAL_B_SPLINE_SURFACE(((0.999732896028954,0.999865728939229,1.,0.994017305594881,
0.990889788836284),(0.999732896028954,0.999865728939229,1.,0.994017305594881,
0.990889788836284)))
REPRESENTATION_ITEM('')
SURFACE()
);
#3360=(
BOUNDED_SURFACE()
B_SPLINE_SURFACE(1,2,((#151563,#151564,#151565,#151566,#151567),(#151568,
#151569,#151570,#151571,#151572)),.UNSPECIFIED.,.F.,.F.,.F.)
B_SPLINE_SURFACE_WITH_KNOTS((2,2),(3,2,3),(0.709590617387241,1.),(0.573052008440968,
0.573654350219911,0.591014490232053),.UNSPECIFIED.)
GEOMETRIC_REPRESENTATION_ITEM()
RATIONAL_B_SPLINE_SURFACE(((0.99848615229188,0.99848615229188,0.99848615229188,
0.992772345172011,0.990020524139833),(0.99848615229188,0.99848615229188,
0.99848615229188,0.992772345172011,0.990020524139833)))
REPRESENTATION_ITEM('')
SURFACE()
);
#3361=(
BOUNDED_SURFACE()
B_SPLINE_SURFACE(1,2,((#151581,#151582,#151583,#151584,#151585),(#151586,
#151587,#151588,#151589,#151590)),.UNSPECIFIED.,.F.,.F.,.F.)
B_SPLINE_SURFACE_WITH_KNOTS((2,2),(3,2,3),(0.710318915640086,1.),(0.142474614281367,
0.142857142857143,0.159901408087481),.UNSPECIFIED.)
GEOMETRIC_REPRESENTATION_ITEM()
RATIONAL_B_SPLINE_SURFACE(((0.999732896029237,0.999865728939372,1.,0.994017305594881,
0.990889788836284),(0.999732896029237,0.999865728939372,1.,0.994017305594881,
0.990889788836284)))
REPRESENTATION_ITEM('')
SURFACE()
);
#3362=(
BOUNDED_SURFACE()
B_SPLINE_SURFACE(1,2,((#151592,#151593,#151594,#151595,#151596),(#151597,
#151598,#151599,#151600,#151601)),.UNSPECIFIED.,.F.,.F.,.F.)
B_SPLINE_SURFACE_WITH_KNOTS((2,2),(3,2,3),(0.709590617385605,1.),(0.573052008476401,
0.573654350219911,0.591014490232053),.UNSPECIFIED.)
GEOMETRIC_REPRESENTATION_ITEM()
RATIONAL_B_SPLINE_SURFACE(((0.99848615229188,0.99848615229188,0.99848615229188,
0.992772345172011,0.990020524139833),(0.99848615229188,0.99848615229188,
0.99848615229188,0.992772345172011,0.990020524139833)))
REPRESENTATION_ITEM('')
SURFACE()
);
#3363=(
BOUNDED_SURFACE()
B_SPLINE_SURFACE(1,2,((#151610,#151611,#151612,#151613,#151614),(#151615,
#151616,#151617,#151618,#151619)),.UNSPECIFIED.,.F.,.F.,.F.)
B_SPLINE_SURFACE_WITH_KNOTS((2,2),(3,2,3),(0.710318915640079,1.),(0.142474614281367,
0.142857142857143,0.159901408087481),.UNSPECIFIED.)
GEOMETRIC_REPRESENTATION_ITEM()
RATIONAL_B_SPLINE_SURFACE(((0.999732896029237,0.999865728939372,1.,0.994017305594881,
0.990889788836284),(0.999732896029237,0.999865728939372,1.,0.994017305594881,
0.990889788836284)))
REPRESENTATION_ITEM('')
SURFACE()
);
#3364=(
BOUNDED_SURFACE()
B_SPLINE_SURFACE(1,2,((#151621,#151622,#151623,#151624,#151625),(#151626,
#151627,#151628,#151629,#151630)),.UNSPECIFIED.,.F.,.F.,.F.)
B_SPLINE_SURFACE_WITH_KNOTS((2,2),(3,2,3),(0.709590617380986,1.),(0.573052008470953,
0.573654350219905,0.591014490232052),.UNSPECIFIED.)
GEOMETRIC_REPRESENTATION_ITEM()
RATIONAL_B_SPLINE_SURFACE(((0.998486152291883,0.998486152291883,0.998486152291883,
0.992772345172012,0.990020524139833),(0.998486152291883,0.998486152291883,
0.998486152291883,0.992772345172012,0.990020524139833)))
REPRESENTATION_ITEM('')
SURFACE()
);
#3365=(
BOUNDED_SURFACE()
B_SPLINE_SURFACE(1,2,((#151639,#151640,#151641,#151642,#151643),(#151644,
#151645,#151646,#151647,#151648)),.UNSPECIFIED.,.F.,.F.,.F.)
B_SPLINE_SURFACE_WITH_KNOTS((2,2),(3,2,3),(0.710318915639879,1.),(0.142474614281367,
0.142857142857143,0.159901408087485),.UNSPECIFIED.)
GEOMETRIC_REPRESENTATION_ITEM()
RATIONAL_B_SPLINE_SURFACE(((0.999732896029238,0.999865728939373,1.,0.99401730559488,
0.990889788836283),(0.999732896029238,0.999865728939373,1.,0.99401730559488,
0.990889788836283)))
REPRESENTATION_ITEM('')
SURFACE()
);
#3366=(
BOUNDED_SURFACE()
B_SPLINE_SURFACE(1,2,((#151650,#151651,#151652,#151653,#151654),(#151655,
#151656,#151657,#151658,#151659)),.UNSPECIFIED.,.F.,.F.,.F.)
B_SPLINE_SURFACE_WITH_KNOTS((2,2),(3,2,3),(0.709590617360321,1.),(0.573052008450992,
0.57365435021991,0.591014490232052),.UNSPECIFIED.)
GEOMETRIC_REPRESENTATION_ITEM()
RATIONAL_B_SPLINE_SURFACE(((0.998486152291881,0.998486152291881,0.998486152291881,
0.992772345172012,0.990020524139833),(0.998486152291881,0.998486152291881,
0.998486152291881,0.992772345172012,0.990020524139833)))
REPRESENTATION_ITEM('')
SURFACE()
);
#3367=(
BOUNDED_SURFACE()
B_SPLINE_SURFACE(1,2,((#151668,#151669,#151670,#151671,#151672),(#151673,
#151674,#151675,#151676,#151677)),.UNSPECIFIED.,.F.,.F.,.F.)
B_SPLINE_SURFACE_WITH_KNOTS((2,2),(3,2,3),(0.710318915639129,1.),(0.142474614281368,
0.142857142857143,0.159901408087494),.UNSPECIFIED.)
GEOMETRIC_REPRESENTATION_ITEM()
RATIONAL_B_SPLINE_SURFACE(((0.999732896029238,0.999865728939373,1.,0.994017305594877,
0.990889788836279),(0.999732896029238,0.999865728939373,1.,0.994017305594877,
0.990889788836279)))
REPRESENTATION_ITEM('')
SURFACE()
);
#3368=(
BOUNDED_SURFACE()
B_SPLINE_SURFACE(1,2,((#151679,#151680,#151681,#151682,#151683),(#151684,
#151685,#151686,#151687,#151688)),.UNSPECIFIED.,.F.,.F.,.F.)
B_SPLINE_SURFACE_WITH_KNOTS((2,2),(3,2,3),(0.710192959008292,1.),(0.573480748819789,
0.57365435021991,0.591014490232053),.UNSPECIFIED.)
GEOMETRIC_REPRESENTATION_ITEM()
RATIONAL_B_SPLINE_SURFACE(((0.99848615229188,0.99848615229188,0.99848615229188,
0.992772345172011,0.990020524139833),(0.99848615229188,0.99848615229188,
0.99848615229188,0.992772345172011,0.990020524139833)))
REPRESENTATION_ITEM('')
SURFACE()
);
#3369=(
BOUNDED_SURFACE()
B_SPLINE_SURFACE(1,2,((#151697,#151698,#151699,#151700,#151701),(#151702,
#151703,#151704,#151705,#151706)),.UNSPECIFIED.,.F.,.F.,.F.)
B_SPLINE_SURFACE_WITH_KNOTS((2,2),(3,2,3),(0.710318915638992,1.),(0.142474614281365,
0.142857142857143,0.159901408087493),.UNSPECIFIED.)
GEOMETRIC_REPRESENTATION_ITEM()
RATIONAL_B_SPLINE_SURFACE(((0.999732896029236,0.999865728939372,1.,0.994017305594877,
0.99088978883628),(0.999732896029236,0.999865728939372,1.,0.994017305594877,
0.99088978883628)))
REPRESENTATION_ITEM('')
SURFACE()
);
#3370=(
BOUNDED_SURFACE()
B_SPLINE_SURFACE(1,2,((#151708,#151709,#151710,#151711,#151712),(#151713,
#151714,#151715,#151716,#151717)),.UNSPECIFIED.,.F.,.F.,.F.)
B_SPLINE_SURFACE_WITH_KNOTS((2,2),(3,2,3),(0.709590617378624,1.),(0.573052008469533,
0.57365435021991,0.591014490232052),.UNSPECIFIED.)
GEOMETRIC_REPRESENTATION_ITEM()
RATIONAL_B_SPLINE_SURFACE(((0.99848615229188,0.99848615229188,0.99848615229188,
0.992772345172011,0.990020524139833),(0.99848615229188,0.99848615229188,
0.99848615229188,0.992772345172011,0.990020524139833)))
REPRESENTATION_ITEM('')
SURFACE()
);
#3371=(
BOUNDED_SURFACE()
B_SPLINE_SURFACE(1,2,((#151726,#151727,#151728,#151729,#151730),(#151731,
#151732,#151733,#151734,#151735)),.UNSPECIFIED.,.F.,.F.,.F.)
B_SPLINE_SURFACE_WITH_KNOTS((2,2),(3,2,3),(0.710318915639023,1.),(0.142474614281365,
0.142857142857143,0.159901408087496),.UNSPECIFIED.)
GEOMETRIC_REPRESENTATION_ITEM()
RATIONAL_B_SPLINE_SURFACE(((0.999732896029237,0.999865728939372,1.,0.994017305594876,
0.990889788836279),(0.999732896029237,0.999865728939372,1.,0.994017305594876,
0.990889788836279)))
REPRESENTATION_ITEM('')
SURFACE()
);
#3372=(
BOUNDED_SURFACE()
B_SPLINE_SURFACE(1,2,((#151737,#151738,#151739,#151740,#151741),(#151742,
#151743,#151744,#151745,#151746)),.UNSPECIFIED.,.F.,.F.,.F.)
B_SPLINE_SURFACE_WITH_KNOTS((2,2),(3,2,3),(0.709590617379361,1.),(0.573052008435022,
0.57365435021991,0.591014490232051),.UNSPECIFIED.)
GEOMETRIC_REPRESENTATION_ITEM()
RATIONAL_B_SPLINE_SURFACE(((0.99848615229188,0.99848615229188,0.99848615229188,
0.992772345172012,0.990020524139833),(0.99848615229188,0.99848615229188,
0.99848615229188,0.992772345172012,0.990020524139833)))
REPRESENTATION_ITEM('')
SURFACE()
);
#3373=(
BOUNDED_SURFACE()
B_SPLINE_SURFACE(1,2,((#151755,#151756,#151757,#151758,#151759),(#151760,
#151761,#151762,#151763,#151764),(#151765,#151766,#151767,#151768,#151769)),
 .UNSPECIFIED.,.F.,.F.,.F.)
B_SPLINE_SURFACE_WITH_KNOTS((2,1,2),(3,2,3),(0.710318915638281,1.,1.00289681084362),
(0.142474614281367,0.142857142857143,0.159901408087482),.UNSPECIFIED.)
GEOMETRIC_REPRESENTATION_ITEM()
RATIONAL_B_SPLINE_SURFACE(((0.999732896029237,0.999865728939372,1.,0.994017305594881,
0.990889788836284),(0.999732896029237,0.999865728939372,1.,0.994017305594881,
0.990889788836284),(0.999732896029237,0.999865728939372,1.,0.994017305594881,
0.990889788836284)))
REPRESENTATION_ITEM('')
SURFACE()
);
#3374=(
BOUNDED_SURFACE()
B_SPLINE_SURFACE(1,2,((#151771,#151772,#151773,#151774,#151775),(#151776,
#151777,#151778,#151779,#151780)),.UNSPECIFIED.,.F.,.F.,.F.)
B_SPLINE_SURFACE_WITH_KNOTS((2,2),(3,2,3),(0.7095906173851,1.),(0.573052008439701,
0.573654350219884,0.591014490232052),.UNSPECIFIED.)
GEOMETRIC_REPRESENTATION_ITEM()
RATIONAL_B_SPLINE_SURFACE(((0.998486152291898,0.998486152291898,0.998486152291898,
0.992772345172016,0.990020524139833),(0.998486152291898,0.998486152291898,
0.998486152291898,0.992772345172016,0.990020524139833)))
REPRESENTATION_ITEM('')
SURFACE()
);
#3375=(
BOUNDED_SURFACE()
B_SPLINE_SURFACE(1,2,((#151789,#151790,#151791,#151792,#151793),(#151794,
#151795,#151796,#151797,#151798)),.UNSPECIFIED.,.F.,.F.,.F.)
B_SPLINE_SURFACE_WITH_KNOTS((2,2),(3,2,3),(0.710318915639621,1.),(0.14247461428136,
0.142857142857143,0.159901408087483),.UNSPECIFIED.)
GEOMETRIC_REPRESENTATION_ITEM()
RATIONAL_B_SPLINE_SURFACE(((0.999732896029233,0.99986572893937,1.,0.994017305594881,
0.990889788836283),(0.999732896029233,0.99986572893937,1.,0.994017305594881,
0.990889788836283)))
REPRESENTATION_ITEM('')
SURFACE()
);
#3376=(
BOUNDED_SURFACE()
B_SPLINE_SURFACE(1,2,((#151800,#151801,#151802,#151803,#151804),(#151805,
#151806,#151807,#151808,#151809)),.UNSPECIFIED.,.F.,.F.,.F.)
B_SPLINE_SURFACE_WITH_KNOTS((2,2),(3,2,3),(0.709590617367967,1.),(0.573052008421813,
0.57365435021991,0.591014490232046),.UNSPECIFIED.)
GEOMETRIC_REPRESENTATION_ITEM()
RATIONAL_B_SPLINE_SURFACE(((0.99848615229188,0.99848615229188,0.99848615229188,
0.992772345172013,0.990020524139835),(0.99848615229188,0.99848615229188,
0.99848615229188,0.992772345172013,0.990020524139835)))
REPRESENTATION_ITEM('')
SURFACE()
);
#3377=(
BOUNDED_SURFACE()
B_SPLINE_SURFACE(1,2,((#151818,#151819,#151820,#151821,#151822),(#151823,
#151824,#151825,#151826,#151827)),.UNSPECIFIED.,.F.,.F.,.F.)
B_SPLINE_SURFACE_WITH_KNOTS((2,2),(3,2,3),(0.71031891564,1.),(0.14247461428136,
0.142857142857143,0.159901408087483),.UNSPECIFIED.)
GEOMETRIC_REPRESENTATION_ITEM()
RATIONAL_B_SPLINE_SURFACE(((0.999732896029233,0.99986572893937,1.,0.994017305594881,
0.990889788836283),(0.999732896029233,0.99986572893937,1.,0.994017305594881,
0.990889788836283)))
REPRESENTATION_ITEM('')
SURFACE()
);
#3378=(
BOUNDED_SURFACE()
B_SPLINE_SURFACE(1,2,((#151829,#151830,#151831,#151832,#151833),(#151834,
#151835,#151836,#151837,#151838)),.UNSPECIFIED.,.F.,.F.,.F.)
B_SPLINE_SURFACE_WITH_KNOTS((2,2),(3,2,3),(0.71019295900836,1.),(0.573480748819789,
0.57365435021991,0.591014490232052),.UNSPECIFIED.)
GEOMETRIC_REPRESENTATION_ITEM()
RATIONAL_B_SPLINE_SURFACE(((0.99848615229188,0.99848615229188,0.99848615229188,
0.992772345172012,0.990020524139833),(0.99848615229188,0.99848615229188,
0.99848615229188,0.992772345172012,0.990020524139833)))
REPRESENTATION_ITEM('')
SURFACE()
);
#3379=(
BOUNDED_SURFACE()
B_SPLINE_SURFACE(1,2,((#151847,#151848,#151849,#151850,#151851),(#151852,
#151853,#151854,#151855,#151856)),.UNSPECIFIED.,.F.,.F.,.F.)
B_SPLINE_SURFACE_WITH_KNOTS((2,2),(3,2,3),(0.710318915640007,1.),(0.142474614281363,
0.142857142857143,0.159901408087482),.UNSPECIFIED.)
GEOMETRIC_REPRESENTATION_ITEM()
RATIONAL_B_SPLINE_SURFACE(((0.999732896029235,0.999865728939371,1.,0.994017305594881,
0.990889788836284),(0.999732896029235,0.999865728939371,1.,0.994017305594881,
0.990889788836284)))
REPRESENTATION_ITEM('')
SURFACE()
);
#3380=(
BOUNDED_SURFACE()
B_SPLINE_SURFACE(1,2,((#151858,#151859,#151860,#151861,#151862),(#151863,
#151864,#151865,#151866,#151867)),.UNSPECIFIED.,.F.,.F.,.F.)
B_SPLINE_SURFACE_WITH_KNOTS((2,2),(3,2,3),(0.710192959008365,1.),(0.573480748819789,
0.57365435021991,0.591014490232052),.UNSPECIFIED.)
GEOMETRIC_REPRESENTATION_ITEM()
RATIONAL_B_SPLINE_SURFACE(((0.99848615229188,0.99848615229188,0.99848615229188,
0.992772345172012,0.990020524139833),(0.99848615229188,0.99848615229188,
0.99848615229188,0.992772345172012,0.990020524139833)))
REPRESENTATION_ITEM('')
SURFACE()
);
#3381=(
BOUNDED_SURFACE()
B_SPLINE_SURFACE(1,2,((#151876,#151877,#151878,#151879,#151880),(#151881,
#151882,#151883,#151884,#151885)),.UNSPECIFIED.,.F.,.F.,.F.)
B_SPLINE_SURFACE_WITH_KNOTS((2,2),(3,2,3),(0.710318915640009,1.),(0.142474614281368,
0.142857142857143,0.159901408087482),.UNSPECIFIED.)
GEOMETRIC_REPRESENTATION_ITEM()
RATIONAL_B_SPLINE_SURFACE(((0.999732896029238,0.999865728939373,1.,0.994017305594881,
0.990889788836284),(0.999732896029238,0.999865728939373,1.,0.994017305594881,
0.990889788836284)))
REPRESENTATION_ITEM('')
SURFACE()
);
#3382=(
BOUNDED_SURFACE()
B_SPLINE_SURFACE(1,2,((#151887,#151888,#151889,#151890,#151891),(#151892,
#151893,#151894,#151895,#151896)),.UNSPECIFIED.,.F.,.F.,.F.)
B_SPLINE_SURFACE_WITH_KNOTS((2,2),(3,2,3),(0.710192959008085,1.),(0.573480748819736,
0.573654350219858,0.591014490232052),.UNSPECIFIED.)
GEOMETRIC_REPRESENTATION_ITEM()
RATIONAL_B_SPLINE_SURFACE(((0.998486152291915,0.998486152291915,0.998486152291915,
0.99277234517202,0.990020524139833),(0.998486152291915,0.998486152291915,
0.998486152291915,0.99277234517202,0.990020524139833)))
REPRESENTATION_ITEM('')
SURFACE()
);
#3383=(
BOUNDED_SURFACE()
B_SPLINE_SURFACE(1,2,((#151905,#151906,#151907,#151908,#151909),(#151910,
#151911,#151912,#151913,#151914),(#151915,#151916,#151917,#151918,#151919)),
 .UNSPECIFIED.,.F.,.F.,.F.)
B_SPLINE_SURFACE_WITH_KNOTS((2,1,2),(3,2,3),(0.710318915639726,1.,1.0028968108436),
(0.142474614281368,0.142857142857143,0.159901408087482),.UNSPECIFIED.)
GEOMETRIC_REPRESENTATION_ITEM()
RATIONAL_B_SPLINE_SURFACE(((0.999732896029238,0.999865728939373,1.,0.994017305594881,
0.990889788836284),(0.999732896029238,0.999865728939373,1.,0.994017305594881,
0.990889788836284),(0.999732896029238,0.999865728939373,1.,0.994017305594881,
0.990889788836284)))
REPRESENTATION_ITEM('')
SURFACE()
);
#3384=(
BOUNDED_SURFACE()
B_SPLINE_SURFACE(1,2,((#151921,#151922,#151923,#151924,#151925),(#151926,
#151927,#151928,#151929,#151930)),.UNSPECIFIED.,.F.,.F.,.F.)
B_SPLINE_SURFACE_WITH_KNOTS((2,2),(3,2,3),(0.,0.289940743966858),(0.0908085233856358,
0.107982157956012,0.108241818529102),.UNSPECIFIED.)
GEOMETRIC_REPRESENTATION_ITEM()
RATIONAL_B_SPLINE_SURFACE(((0.990086238235256,0.987329216372183,0.987470879370256,
0.987470879370256,0.987470879370256),(0.990086238235256,0.987329216372183,
0.987470879370256,0.987470879370256,0.987470879370256)))
REPRESENTATION_ITEM('')
SURFACE()
);
#3385=(
BOUNDED_SURFACE()
B_SPLINE_SURFACE(1,2,((#151934,#151935,#151936),(#151937,#151938,#151939)),
 .UNSPECIFIED.,.F.,.F.,.F.)
B_SPLINE_SURFACE_WITH_KNOTS((2,2),(3,3),(0.,0.289807040992019),(0.625170525609407,
0.642682999576235),.UNSPECIFIED.)
GEOMETRIC_REPRESENTATION_ITEM()
RATIONAL_B_SPLINE_SURFACE(((0.990658108926708,0.993760979299921,0.999878046252916),
(0.990658108926708,0.993760979299921,0.999878046252916)))
REPRESENTATION_ITEM('')
SURFACE()
);
#3386=(
BOUNDED_SURFACE()
B_SPLINE_SURFACE(1,2,((#151941,#151942,#151943,#151944,#151945),(#151946,
#151947,#151948,#151949,#151950)),.UNSPECIFIED.,.F.,.F.,.F.)
B_SPLINE_SURFACE_WITH_KNOTS((2,2),(3,2,3),(0.,0.289940743918361),(0.0908085233856356,
0.107982157956012,0.10824181848113),.UNSPECIFIED.)
GEOMETRIC_REPRESENTATION_ITEM()
RATIONAL_B_SPLINE_SURFACE(((0.990086238235256,0.987329216372183,0.987470879370255,
0.987470879370255,0.987470879370255),(0.990086238235256,0.987329216372183,
0.987470879370255,0.987470879370255,0.987470879370255)))
REPRESENTATION_ITEM('')
SURFACE()
);
#3387=(
BOUNDED_SURFACE()
B_SPLINE_SURFACE(1,2,((#151954,#151955,#151956),(#151957,#151958,#151959)),
 .UNSPECIFIED.,.F.,.F.,.F.)
B_SPLINE_SURFACE_WITH_KNOTS((2,2),(3,3),(0.,0.289807040992003),(0.625170525609407,
0.642682999576235),.UNSPECIFIED.)
GEOMETRIC_REPRESENTATION_ITEM()
RATIONAL_B_SPLINE_SURFACE(((0.990658108926708,0.993760979299921,0.999878046252916),
(0.990658108926708,0.993760979299921,0.999878046252916)))
REPRESENTATION_ITEM('')
SURFACE()
);
#3388=(
BOUNDED_SURFACE()
B_SPLINE_SURFACE(1,2,((#151961,#151962,#151963,#151964,#151965),(#151966,
#151967,#151968,#151969,#151970)),.UNSPECIFIED.,.F.,.F.,.F.)
B_SPLINE_SURFACE_WITH_KNOTS((2,2),(3,2,3),(0.,0.289940743918459),(0.0908085233856357,
0.107982157956012,0.108241818481194),.UNSPECIFIED.)
GEOMETRIC_REPRESENTATION_ITEM()
RATIONAL_B_SPLINE_SURFACE(((0.990086238235256,0.987329216372183,0.987470879370256,
0.987470879370256,0.987470879370256),(0.990086238235256,0.987329216372183,
0.987470879370256,0.987470879370256,0.987470879370256)))
REPRESENTATION_ITEM('')
SURFACE()
);
#3389=(
BOUNDED_SURFACE()
B_SPLINE_SURFACE(1,2,((#151974,#151975,#151976),(#151977,#151978,#151979)),
 .UNSPECIFIED.,.F.,.F.,.F.)
B_SPLINE_SURFACE_WITH_KNOTS((2,2),(3,3),(0.,0.289807040991873),(0.625170525609407,
0.642682999576235),.UNSPECIFIED.)
GEOMETRIC_REPRESENTATION_ITEM()
RATIONAL_B_SPLINE_SURFACE(((0.990658108926708,0.993760979299921,0.999878046252916),
(0.990658108926708,0.993760979299921,0.999878046252916)))
REPRESENTATION_ITEM('')
SURFACE()
);
#3390=(
BOUNDED_SURFACE()
B_SPLINE_SURFACE(1,2,((#151981,#151982,#151983,#151984,#151985),(#151986,
#151987,#151988,#151989,#151990)),.UNSPECIFIED.,.F.,.F.,.F.)
B_SPLINE_SURFACE_WITH_KNOTS((2,2),(3,2,3),(0.,0.289940743934797),(0.0908085233856346,
0.107982157956012,0.10824181849756),.UNSPECIFIED.)
GEOMETRIC_REPRESENTATION_ITEM()
RATIONAL_B_SPLINE_SURFACE(((0.990086238235256,0.987329216372183,0.987470879370255,
0.987470879370255,0.987470879370255),(0.990086238235257,0.987329216372183,
0.987470879370256,0.987470879370256,0.987470879370256)))
REPRESENTATION_ITEM('')
SURFACE()
);
#3391=(
BOUNDED_SURFACE()
B_SPLINE_SURFACE(1,2,((#151994,#151995,#151996),(#151997,#151998,#151999)),
 .UNSPECIFIED.,.F.,.F.,.F.)
B_SPLINE_SURFACE_WITH_KNOTS((2,2),(3,3),(0.,0.289807040991872),(0.625170525609407,
0.642682999576234),.UNSPECIFIED.)
GEOMETRIC_REPRESENTATION_ITEM()
RATIONAL_B_SPLINE_SURFACE(((0.990658108926708,0.993760979299921,0.999878046252915),
(0.990658108926708,0.993760979299921,0.999878046252915)))
REPRESENTATION_ITEM('')
SURFACE()
);
#3392=(
BOUNDED_SURFACE()
B_SPLINE_SURFACE(1,2,((#152001,#152002,#152003,#152004,#152005),(#152006,
#152007,#152008,#152009,#152010)),.UNSPECIFIED.,.F.,.F.,.F.)
B_SPLINE_SURFACE_WITH_KNOTS((2,2),(3,2,3),(0.,0.289940743974797),(0.0908085233856356,
0.107982157956012,0.108241818491054),.UNSPECIFIED.)
GEOMETRIC_REPRESENTATION_ITEM()
RATIONAL_B_SPLINE_SURFACE(((0.990086238235256,0.987329216372183,0.987470879370255,
0.987470879370255,0.987470879370255),(0.990086238235256,0.987329216372183,
0.987470879370255,0.987470879370255,0.987470879370255)))
REPRESENTATION_ITEM('')
SURFACE()
);
#3393=(
BOUNDED_SURFACE()
B_SPLINE_SURFACE(1,2,((#152014,#152015,#152016),(#152017,#152018,#152019)),
 .UNSPECIFIED.,.F.,.F.,.F.)
B_SPLINE_SURFACE_WITH_KNOTS((2,2),(3,3),(0.,0.289807040992622),(0.625170525609407,
0.642682999576235),.UNSPECIFIED.)
GEOMETRIC_REPRESENTATION_ITEM()
RATIONAL_B_SPLINE_SURFACE(((0.990658108926708,0.993760979299921,0.999878046252915),
(0.990658108926708,0.993760979299921,0.999878046252915)))
REPRESENTATION_ITEM('')
SURFACE()
);
#3394=(
BOUNDED_SURFACE()
B_SPLINE_SURFACE(1,2,((#152021,#152022,#152023,#152024,#152025),(#152026,
#152027,#152028,#152029,#152030)),.UNSPECIFIED.,.F.,.F.,.F.)
B_SPLINE_SURFACE_WITH_KNOTS((2,2),(3,2,3),(0.,0.289940743935406),(0.0908085233856344,
0.107982157956012,0.108241818452283),.UNSPECIFIED.)
GEOMETRIC_REPRESENTATION_ITEM()
RATIONAL_B_SPLINE_SURFACE(((0.990086238235257,0.987329216372183,0.987470879370256,
0.987470879370256,0.987470879370256),(0.990086238235257,0.987329216372183,
0.987470879370255,0.987470879370255,0.987470879370255)))
REPRESENTATION_ITEM('')
SURFACE()
);
#3395=(
BOUNDED_SURFACE()
B_SPLINE_SURFACE(1,2,((#152034,#152035,#152036),(#152037,#152038,#152039)),
 .UNSPECIFIED.,.F.,.F.,.F.)
B_SPLINE_SURFACE_WITH_KNOTS((2,2),(3,3),(0.,0.289807040992624),(0.625170525609407,
0.642682999576233),.UNSPECIFIED.)
GEOMETRIC_REPRESENTATION_ITEM()
RATIONAL_B_SPLINE_SURFACE(((0.990658108926708,0.99376097929992,0.999878046252915),
(0.990658108926708,0.99376097929992,0.999878046252915)))
REPRESENTATION_ITEM('')
SURFACE()
);
#3396=(
BOUNDED_SURFACE()
B_SPLINE_SURFACE(1,2,((#152041,#152042,#152043,#152044,#152045),(#152046,
#152047,#152048,#152049,#152050)),.UNSPECIFIED.,.F.,.F.,.F.)
B_SPLINE_SURFACE_WITH_KNOTS((2,2),(3,2,3),(0.,0.289940743989111),(0.0908085233856356,
0.107982157956012,0.108241818505293),.UNSPECIFIED.)
GEOMETRIC_REPRESENTATION_ITEM()
RATIONAL_B_SPLINE_SURFACE(((0.990086238235256,0.987329216372183,0.987470879370255,
0.987470879370255,0.987470879370255),(0.990086238235256,0.987329216372183,
0.987470879370255,0.987470879370255,0.987470879370255)))
REPRESENTATION_ITEM('')
SURFACE()
);
#3397=(
BOUNDED_SURFACE()
B_SPLINE_SURFACE(1,2,((#152054,#152055,#152056),(#152057,#152058,#152059)),
 .UNSPECIFIED.,.F.,.F.,.F.)
B_SPLINE_SURFACE_WITH_KNOTS((2,2),(3,3),(0.,0.289807040992625),(0.625170525609407,
0.642682999576235),.UNSPECIFIED.)
GEOMETRIC_REPRESENTATION_ITEM()
RATIONAL_B_SPLINE_SURFACE(((0.990658108926708,0.993760979299921,0.999878046252916),
(0.990658108926708,0.993760979299921,0.999878046252916)))
REPRESENTATION_ITEM('')
SURFACE()
);
#3398=(
BOUNDED_SURFACE()
B_SPLINE_SURFACE(1,2,((#152061,#152062,#152063,#152064,#152065),(#152066,
#152067,#152068,#152069,#152070)),.UNSPECIFIED.,.F.,.F.,.F.)
B_SPLINE_SURFACE_WITH_KNOTS((2,2),(3,2,3),(0.,0.28994074403715),(0.0908085233856358,
0.107982157956012,0.108241818553818),.UNSPECIFIED.)
GEOMETRIC_REPRESENTATION_ITEM()
RATIONAL_B_SPLINE_SURFACE(((0.990086238235256,0.987329216372183,0.987470879370255,
0.987470879370255,0.987470879370255),(0.990086238235256,0.987329216372183,
0.987470879370255,0.987470879370255,0.987470879370255)))
REPRESENTATION_ITEM('')
SURFACE()
);
#3399=(
BOUNDED_SURFACE()
B_SPLINE_SURFACE(1,2,((#152074,#152075,#152076),(#152077,#152078,#152079)),
 .UNSPECIFIED.,.F.,.F.,.F.)
B_SPLINE_SURFACE_WITH_KNOTS((2,2),(3,3),(0.,0.289807040993206),(0.625170525609407,
0.642682999576235),.UNSPECIFIED.)
GEOMETRIC_REPRESENTATION_ITEM()
RATIONAL_B_SPLINE_SURFACE(((0.990658108926708,0.993760979299921,0.999878046252916),
(0.990658108926708,0.993760979299921,0.999878046252916)))
REPRESENTATION_ITEM('')
SURFACE()
);
#3400=(
BOUNDED_SURFACE()
B_SPLINE_SURFACE(1,2,((#152081,#152082,#152083,#152084,#152085),(#152086,
#152087,#152088,#152089,#152090)),.UNSPECIFIED.,.F.,.F.,.F.)
B_SPLINE_SURFACE_WITH_KNOTS((2,2),(3,2,3),(0.,0.289940743903119),(0.0908085233856344,
0.107982157956012,0.108241818465865),.UNSPECIFIED.)
GEOMETRIC_REPRESENTATION_ITEM()
RATIONAL_B_SPLINE_SURFACE(((0.990086238235257,0.987329216372183,0.987470879370255,
0.987470879370255,0.987470879370255),(0.990086238235257,0.987329216372183,
0.987470879370255,0.987470879370255,0.987470879370255)))
REPRESENTATION_ITEM('')
SURFACE()
);
#3401=(
BOUNDED_SURFACE()
B_SPLINE_SURFACE(1,2,((#152094,#152095,#152096),(#152097,#152098,#152099)),
 .UNSPECIFIED.,.F.,.F.,.F.)
B_SPLINE_SURFACE_WITH_KNOTS((2,2),(3,3),(0.,0.289807040992615),(0.625170525609407,
0.642682999576234),.UNSPECIFIED.)
GEOMETRIC_REPRESENTATION_ITEM()
RATIONAL_B_SPLINE_SURFACE(((0.990658108926708,0.99376097929992,0.999878046252915),
(0.990658108926708,0.99376097929992,0.999878046252915)))
REPRESENTATION_ITEM('')
SURFACE()
);
#3402=(
BOUNDED_SURFACE()
B_SPLINE_SURFACE(1,2,((#152101,#152102,#152103,#152104,#152105),(#152106,
#152107,#152108,#152109,#152110)),.UNSPECIFIED.,.F.,.F.,.F.)
B_SPLINE_SURFACE_WITH_KNOTS((2,2),(3,2,3),(0.,0.289940743947236),(0.0908085233856345,
0.107982157956012,0.108241818509775),.UNSPECIFIED.)
GEOMETRIC_REPRESENTATION_ITEM()
RATIONAL_B_SPLINE_SURFACE(((0.990086238235257,0.987329216372183,0.987470879370255,
0.987470879370255,0.987470879370255),(0.990086238235257,0.987329216372183,
0.987470879370255,0.987470879370255,0.987470879370255)))
REPRESENTATION_ITEM('')
SURFACE()
);
#3403=(
BOUNDED_SURFACE()
B_SPLINE_SURFACE(1,2,((#152114,#152115,#152116),(#152117,#152118,#152119)),
 .UNSPECIFIED.,.F.,.F.,.F.)
B_SPLINE_SURFACE_WITH_KNOTS((2,2),(3,3),(0.,0.289807040993176),(0.625170525609407,
0.642682999576233),.UNSPECIFIED.)
GEOMETRIC_REPRESENTATION_ITEM()
RATIONAL_B_SPLINE_SURFACE(((0.990658108926708,0.99376097929992,0.999878046252915),
(0.990658108926708,0.99376097929992,0.999878046252915)))
REPRESENTATION_ITEM('')
SURFACE()
);
#3404=(
BOUNDED_SURFACE()
B_SPLINE_SURFACE(1,2,((#152121,#152122,#152123,#152124,#152125),(#152126,
#152127,#152128,#152129,#152130)),.UNSPECIFIED.,.F.,.F.,.F.)
B_SPLINE_SURFACE_WITH_KNOTS((2,2),(3,2,3),(0.,0.28994074392508),(0.0908085233856357,
0.107982157956012,0.10824181848765),.UNSPECIFIED.)
GEOMETRIC_REPRESENTATION_ITEM()
RATIONAL_B_SPLINE_SURFACE(((0.990086238235256,0.987329216372183,0.987470879370256,
0.987470879370256,0.987470879370256),(0.990086238235256,0.987329216372183,
0.987470879370256,0.987470879370256,0.987470879370256)))
REPRESENTATION_ITEM('')
SURFACE()
);
#3405=(
BOUNDED_SURFACE()
B_SPLINE_SURFACE(1,2,((#152134,#152135,#152136),(#152137,#152138,#152139)),
 .UNSPECIFIED.,.F.,.F.,.F.)
B_SPLINE_SURFACE_WITH_KNOTS((2,2),(3,3),(0.,0.289807040992982),(0.625170525609408,
0.642682999576235),.UNSPECIFIED.)
GEOMETRIC_REPRESENTATION_ITEM()
RATIONAL_B_SPLINE_SURFACE(((0.990658108926709,0.993760979299921,0.999878046252916),
(0.990658108926709,0.993760979299921,0.999878046252916)))
REPRESENTATION_ITEM('')
SURFACE()
);
#3406=(
BOUNDED_SURFACE()
B_SPLINE_SURFACE(1,2,((#152141,#152142,#152143,#152144,#152145),(#152146,
#152147,#152148,#152149,#152150)),.UNSPECIFIED.,.F.,.F.,.F.)
B_SPLINE_SURFACE_WITH_KNOTS((2,2),(3,2,3),(0.,0.289940743933188),(0.0908085233856345,
0.107982157956011,0.108241818495526),.UNSPECIFIED.)
GEOMETRIC_REPRESENTATION_ITEM()
RATIONAL_B_SPLINE_SURFACE(((0.990086238235257,0.987329216372183,0.987470879370255,
0.987470879370255,0.987470879370255),(0.990086238235257,0.987329216372183,
0.987470879370255,0.987470879370255,0.987470879370255)))
REPRESENTATION_ITEM('')
SURFACE()
);
#3407=(
BOUNDED_SURFACE()
B_SPLINE_SURFACE(1,2,((#152154,#152155,#152156),(#152157,#152158,#152159)),
 .UNSPECIFIED.,.F.,.F.,.F.)
B_SPLINE_SURFACE_WITH_KNOTS((2,2),(3,3),(0.,0.289807040993016),(0.625170525609408,
0.642682999576236),.UNSPECIFIED.)
GEOMETRIC_REPRESENTATION_ITEM()
RATIONAL_B_SPLINE_SURFACE(((0.990658108926709,0.993760979299921,0.999878046252916),
(0.990658108926709,0.993760979299921,0.999878046252916)))
REPRESENTATION_ITEM('')
SURFACE()
);
#3408=(
BOUNDED_SURFACE()
B_SPLINE_SURFACE(1,2,((#152161,#152162,#152163,#152164,#152165),(#152166,
#152167,#152168,#152169,#152170)),.UNSPECIFIED.,.F.,.F.,.F.)
B_SPLINE_SURFACE_WITH_KNOTS((2,2),(3,2,3),(0.,0.289940743982799),(0.0908085233856346,
0.107982157956011,0.108241818499096),.UNSPECIFIED.)
GEOMETRIC_REPRESENTATION_ITEM()
RATIONAL_B_SPLINE_SURFACE(((0.990086238235257,0.987329216372183,0.987470879370256,
0.987470879370256,0.987470879370256),(0.990086238235256,0.987329216372183,
0.987470879370255,0.987470879370255,0.987470879370255)))
REPRESENTATION_ITEM('')
SURFACE()
);
#3409=(
BOUNDED_SURFACE()
B_SPLINE_SURFACE(1,2,((#152174,#152175,#152176),(#152177,#152178,#152179)),
 .UNSPECIFIED.,.F.,.F.,.F.)
B_SPLINE_SURFACE_WITH_KNOTS((2,2),(3,3),(0.,0.289807040993292),(0.625170525609408,
0.642682999576236),.UNSPECIFIED.)
GEOMETRIC_REPRESENTATION_ITEM()
RATIONAL_B_SPLINE_SURFACE(((0.990658108926709,0.993760979299921,0.999878046252916),
(0.990658108926709,0.993760979299921,0.999878046252916)))
REPRESENTATION_ITEM('')
SURFACE()
);
#3410=(
BOUNDED_SURFACE()
B_SPLINE_SURFACE(1,2,((#152181,#152182,#152183,#152184,#152185),(#152186,
#152187,#152188,#152189,#152190)),.UNSPECIFIED.,.F.,.F.,.F.)
B_SPLINE_SURFACE_WITH_KNOTS((2,2),(3,2,3),(0.,0.289940743772721),(0.0908085233856349,
0.107982157956011,0.108241818334936),.UNSPECIFIED.)
GEOMETRIC_REPRESENTATION_ITEM()
RATIONAL_B_SPLINE_SURFACE(((0.990086238235256,0.987329216372183,0.987470879370256,
0.987470879370256,0.987470879370256),(0.990086238235256,0.987329216372183,
0.987470879370256,0.987470879370256,0.987470879370256)))
REPRESENTATION_ITEM('')
SURFACE()
);
#3411=(
BOUNDED_SURFACE()
B_SPLINE_SURFACE(1,2,((#152194,#152195,#152196),(#152197,#152198,#152199)),
 .UNSPECIFIED.,.F.,.F.,.F.)
B_SPLINE_SURFACE_WITH_KNOTS((2,2),(3,3),(0.,0.289807040992714),(0.625170525609408,
0.642682999576236),.UNSPECIFIED.)
GEOMETRIC_REPRESENTATION_ITEM()
RATIONAL_B_SPLINE_SURFACE(((0.990658108926709,0.993760979299922,0.999878046252917),
(0.990658108926709,0.993760979299922,0.999878046252917)))
REPRESENTATION_ITEM('')
SURFACE()
);
#3412=(
BOUNDED_SURFACE()
B_SPLINE_SURFACE(1,2,((#152201,#152202,#152203,#152204,#152205),(#152206,
#152207,#152208,#152209,#152210)),.UNSPECIFIED.,.F.,.F.,.F.)
B_SPLINE_SURFACE_WITH_KNOTS((2,2),(3,2,3),(0.,0.289940743946678),(0.0908085233856334,
0.107982157956011,0.108241818509224),.UNSPECIFIED.)
GEOMETRIC_REPRESENTATION_ITEM()
RATIONAL_B_SPLINE_SURFACE(((0.990086238235257,0.987329216372183,0.987470879370256,
0.987470879370256,0.987470879370256),(0.990086238235257,0.987329216372183,
0.987470879370255,0.987470879370255,0.987470879370255)))
REPRESENTATION_ITEM('')
SURFACE()
);
#3413=(
BOUNDED_SURFACE()
B_SPLINE_SURFACE(1,2,((#152214,#152215,#152216),(#152217,#152218,#152219)),
 .UNSPECIFIED.,.F.,.F.,.F.)
B_SPLINE_SURFACE_WITH_KNOTS((2,2),(3,3),(0.,0.289807040993543),(0.625170525609408,
0.642682999576235),.UNSPECIFIED.)
GEOMETRIC_REPRESENTATION_ITEM()
RATIONAL_B_SPLINE_SURFACE(((0.990658108926709,0.993760979299921,0.999878046252916),
(0.990658108926709,0.993760979299921,0.999878046252916)))
REPRESENTATION_ITEM('')
SURFACE()
);
#3414=(
BOUNDED_SURFACE()
B_SPLINE_SURFACE(1,2,((#152221,#152222,#152223,#152224,#152225),(#152226,
#152227,#152228,#152229,#152230)),.UNSPECIFIED.,.F.,.F.,.F.)
B_SPLINE_SURFACE_WITH_KNOTS((2,2),(3,2,3),(0.,0.289940744094116),(0.0908085233856345,
0.107982157956011,0.108241818911241),.UNSPECIFIED.)
GEOMETRIC_REPRESENTATION_ITEM()
RATIONAL_B_SPLINE_SURFACE(((0.990086238235257,0.987329216372183,0.987470879370255,
0.987470879370255,0.987470879370255),(0.990086238235257,0.987329216372183,
0.987470879370255,0.987470879370255,0.987470879370255)))
REPRESENTATION_ITEM('')
SURFACE()
);
#3415=(
BOUNDED_SURFACE()
B_SPLINE_SURFACE(1,2,((#152234,#152235,#152236),(#152237,#152238,#152239)),
 .UNSPECIFIED.,.F.,.F.,.F.)
B_SPLINE_SURFACE_WITH_KNOTS((2,2),(3,3),(0.,0.289807040993038),(0.625170525609408,
0.642682999576236),.UNSPECIFIED.)
GEOMETRIC_REPRESENTATION_ITEM()
RATIONAL_B_SPLINE_SURFACE(((0.990658108926709,0.993760979299921,0.999878046252916),
(0.990658108926709,0.993760979299921,0.999878046252916)))
REPRESENTATION_ITEM('')
SURFACE()
);
#3416=(
BOUNDED_SURFACE()
B_SPLINE_SURFACE(1,2,((#152241,#152242,#152243,#152244,#152245),(#152246,
#152247,#152248,#152249,#152250)),.UNSPECIFIED.,.F.,.F.,.F.)
B_SPLINE_SURFACE_WITH_KNOTS((2,2),(3,2,3),(0.,0.289940743912886),(0.0908085233856345,
0.107982157956011,0.108241818475653),.UNSPECIFIED.)
GEOMETRIC_REPRESENTATION_ITEM()
RATIONAL_B_SPLINE_SURFACE(((0.990086238235257,0.987329216372183,0.987470879370255,
0.987470879370255,0.987470879370255),(0.990086238235257,0.987329216372183,
0.987470879370255,0.987470879370255,0.987470879370255)))
REPRESENTATION_ITEM('')
SURFACE()
);
#3417=(
BOUNDED_SURFACE()
B_SPLINE_SURFACE(1,2,((#152254,#152255,#152256),(#152257,#152258,#152259)),
 .UNSPECIFIED.,.F.,.F.,.F.)
B_SPLINE_SURFACE_WITH_KNOTS((2,2),(3,3),(0.,0.289807040993515),(0.625170525609408,
0.642682999576236),.UNSPECIFIED.)
GEOMETRIC_REPRESENTATION_ITEM()
RATIONAL_B_SPLINE_SURFACE(((0.990658108926709,0.993760979299921,0.999878046252916),
(0.990658108926709,0.993760979299921,0.999878046252916)))
REPRESENTATION_ITEM('')
SURFACE()
);
#3418=(
BOUNDED_SURFACE()
B_SPLINE_SURFACE(1,2,((#152261,#152262,#152263,#152264,#152265),(#152266,
#152267,#152268,#152269,#152270)),.UNSPECIFIED.,.F.,.F.,.F.)
B_SPLINE_SURFACE_WITH_KNOTS((2,2),(3,2,3),(0.,0.289940743945347),(0.0908085233856346,
0.107982157956011,0.108241818507535),.UNSPECIFIED.)
GEOMETRIC_REPRESENTATION_ITEM()
RATIONAL_B_SPLINE_SURFACE(((0.990086238235257,0.987329216372183,0.987470879370255,
0.987470879370255,0.987470879370255),(0.990086238235257,0.987329216372183,
0.987470879370255,0.987470879370255,0.987470879370255)))
REPRESENTATION_ITEM('')
SURFACE()
);
#3419=(
BOUNDED_SURFACE()
B_SPLINE_SURFACE(1,2,((#152274,#152275,#152276),(#152277,#152278,#152279)),
 .UNSPECIFIED.,.F.,.F.,.F.)
B_SPLINE_SURFACE_WITH_KNOTS((2,2),(3,3),(0.,0.289807040993259),(0.625170525609408,
0.642682999576236),.UNSPECIFIED.)
GEOMETRIC_REPRESENTATION_ITEM()
RATIONAL_B_SPLINE_SURFACE(((0.990658108926709,0.993760979299922,0.999878046252917),
(0.990658108926709,0.993760979299921,0.999878046252917)))
REPRESENTATION_ITEM('')
SURFACE()
);
#3420=(
BOUNDED_SURFACE()
B_SPLINE_SURFACE(1,2,((#152281,#152282,#152283,#152284,#152285),(#152286,
#152287,#152288,#152289,#152290)),.UNSPECIFIED.,.F.,.F.,.F.)
B_SPLINE_SURFACE_WITH_KNOTS((2,2),(3,2,3),(0.,0.289940743920806),(0.0908085233856334,
0.107982157956011,0.108241818483558),.UNSPECIFIED.)
GEOMETRIC_REPRESENTATION_ITEM()
RATIONAL_B_SPLINE_SURFACE(((0.990086238235257,0.987329216372183,0.987470879370256,
0.987470879370256,0.987470879370256),(0.990086238235257,0.987329216372183,
0.987470879370256,0.987470879370256,0.987470879370256)))
REPRESENTATION_ITEM('')
SURFACE()
);
#3421=(
BOUNDED_SURFACE()
B_SPLINE_SURFACE(1,2,((#152294,#152295,#152296),(#152297,#152298,#152299)),
 .UNSPECIFIED.,.F.,.F.,.F.)
B_SPLINE_SURFACE_WITH_KNOTS((2,2),(3,3),(0.,0.289807040994425),(0.625170525609408,
0.642682999576235),.UNSPECIFIED.)
GEOMETRIC_REPRESENTATION_ITEM()
RATIONAL_B_SPLINE_SURFACE(((0.990658108926709,0.993760979299921,0.999878046252915),
(0.990658108926709,0.993760979299921,0.999878046252915)))
REPRESENTATION_ITEM('')
SURFACE()
);
#3422=(
BOUNDED_SURFACE()
B_SPLINE_SURFACE(1,2,((#152301,#152302,#152303,#152304,#152305),(#152306,
#152307,#152308,#152309,#152310)),.UNSPECIFIED.,.F.,.F.,.F.)
B_SPLINE_SURFACE_WITH_KNOTS((2,2),(3,2,3),(0.,0.289940743934633),(0.0908085233856309,
0.107982157956011,0.108241818497391),.UNSPECIFIED.)
GEOMETRIC_REPRESENTATION_ITEM()
RATIONAL_B_SPLINE_SURFACE(((0.990086238235258,0.987329216372183,0.987470879370255,
0.987470879370255,0.987470879370255),(0.990086238235258,0.987329216372183,
0.987470879370255,0.987470879370255,0.987470879370255)))
REPRESENTATION_ITEM('')
SURFACE()
);
#3423=(
BOUNDED_SURFACE()
B_SPLINE_SURFACE(1,2,((#152314,#152315,#152316),(#152317,#152318,#152319)),
 .UNSPECIFIED.,.F.,.F.,.F.)
B_SPLINE_SURFACE_WITH_KNOTS((2,2),(3,3),(0.,0.289807040992766),(0.625170525609408,
0.642682999576236),.UNSPECIFIED.)
GEOMETRIC_REPRESENTATION_ITEM()
RATIONAL_B_SPLINE_SURFACE(((0.990658108926709,0.993760979299921,0.999878046252916),
(0.990658108926709,0.993760979299921,0.999878046252916)))
REPRESENTATION_ITEM('')
SURFACE()
);
#3424=(
BOUNDED_SURFACE()
B_SPLINE_SURFACE(1,2,((#152321,#152322,#152323,#152324,#152325),(#152326,
#152327,#152328,#152329,#152330)),.UNSPECIFIED.,.F.,.F.,.F.)
B_SPLINE_SURFACE_WITH_KNOTS((2,2),(3,2,3),(0.,0.289940743936486),(0.0908085233856343,
0.107982157956011,0.108241818453102),.UNSPECIFIED.)
GEOMETRIC_REPRESENTATION_ITEM()
RATIONAL_B_SPLINE_SURFACE(((0.990086238235257,0.987329216372183,0.987470879370255,
0.987470879370255,0.987470879370255),(0.990086238235257,0.987329216372183,
0.987470879370255,0.987470879370255,0.987470879370255)))
REPRESENTATION_ITEM('')
SURFACE()
);
#3425=(
BOUNDED_SURFACE()
B_SPLINE_SURFACE(1,2,((#152334,#152335,#152336),(#152337,#152338,#152339)),
 .UNSPECIFIED.,.F.,.F.,.F.)
B_SPLINE_SURFACE_WITH_KNOTS((2,2),(3,3),(0.,0.289807040992644),(0.625170525609408,
0.642682999576236),.UNSPECIFIED.)
GEOMETRIC_REPRESENTATION_ITEM()
RATIONAL_B_SPLINE_SURFACE(((0.990658108926709,0.993760979299921,0.999878046252916),
(0.990658108926709,0.993760979299921,0.999878046252916)))
REPRESENTATION_ITEM('')
SURFACE()
);
#3426=(
BOUNDED_SURFACE()
B_SPLINE_SURFACE(1,2,((#152341,#152342,#152343,#152344,#152345),(#152346,
#152347,#152348,#152349,#152350)),.UNSPECIFIED.,.F.,.F.,.F.)
B_SPLINE_SURFACE_WITH_KNOTS((2,2),(3,2,3),(0.,0.289940743784212),(0.0908085233856346,
0.107982157956011,0.10824181860138),.UNSPECIFIED.)
GEOMETRIC_REPRESENTATION_ITEM()
RATIONAL_B_SPLINE_SURFACE(((0.990086238235256,0.987329216372183,0.987470879370255,
0.987470879370255,0.987470879370255),(0.990086238235256,0.987329216372183,
0.987470879370255,0.987470879370255,0.987470879370255)))
REPRESENTATION_ITEM('')
SURFACE()
);
#3427=(
BOUNDED_SURFACE()
B_SPLINE_SURFACE(1,2,((#152354,#152355,#152356),(#152357,#152358,#152359)),
 .UNSPECIFIED.,.F.,.F.,.F.)
B_SPLINE_SURFACE_WITH_KNOTS((2,2),(3,3),(0.,0.289807040993496),(0.625170525609408,
0.642682999576236),.UNSPECIFIED.)
GEOMETRIC_REPRESENTATION_ITEM()
RATIONAL_B_SPLINE_SURFACE(((0.990658108926709,0.993760979299921,0.999878046252916),
(0.990658108926709,0.993760979299921,0.999878046252916)))
REPRESENTATION_ITEM('')
SURFACE()
);
#3428=(
BOUNDED_SURFACE()
B_SPLINE_SURFACE(1,2,((#152361,#152362,#152363,#152364,#152365),(#152366,
#152367,#152368,#152369,#152370)),.UNSPECIFIED.,.F.,.F.,.F.)
B_SPLINE_SURFACE_WITH_KNOTS((2,2),(3,2,3),(0.,0.289940743940566),(0.0908085233856347,
0.107982157956012,0.108241818503291),.UNSPECIFIED.)
GEOMETRIC_REPRESENTATION_ITEM()
RATIONAL_B_SPLINE_SURFACE(((0.990086238235256,0.987329216372183,0.987470879370255,
0.987470879370255,0.987470879370255),(0.990086238235256,0.987329216372183,
0.987470879370255,0.987470879370255,0.987470879370255)))
REPRESENTATION_ITEM('')
SURFACE()
);
#3429=(
BOUNDED_SURFACE()
B_SPLINE_SURFACE(1,2,((#152374,#152375,#152376),(#152377,#152378,#152379)),
 .UNSPECIFIED.,.F.,.F.,.F.)
B_SPLINE_SURFACE_WITH_KNOTS((2,2),(3,3),(0.,0.289807040992018),(0.625170525609408,
0.642682999576236),.UNSPECIFIED.)
GEOMETRIC_REPRESENTATION_ITEM()
RATIONAL_B_SPLINE_SURFACE(((0.990658108926709,0.993760979299921,0.999878046252917),
(0.990658108926709,0.993760979299921,0.999878046252917)))
REPRESENTATION_ITEM('')
SURFACE()
);
#3430=(
BOUNDED_SURFACE()
B_SPLINE_SURFACE(1,2,((#152381,#152382,#152383,#152384,#152385),(#152386,
#152387,#152388,#152389,#152390)),.UNSPECIFIED.,.F.,.F.,.F.)
B_SPLINE_SURFACE_WITH_KNOTS((2,2),(3,2,3),(0.,0.289940743943495),(0.0908085233856345,
0.107982157956011,0.108241818506614),.UNSPECIFIED.)
GEOMETRIC_REPRESENTATION_ITEM()
RATIONAL_B_SPLINE_SURFACE(((0.990086238235257,0.987329216372183,0.987470879370256,
0.987470879370256,0.987470879370256),(0.990086238235257,0.987329216372183,
0.987470879370256,0.987470879370256,0.987470879370256)))
REPRESENTATION_ITEM('')
SURFACE()
);
#3431=(
BOUNDED_SURFACE()
B_SPLINE_SURFACE(1,2,((#152394,#152395,#152396),(#152397,#152398,#152399)),
 .UNSPECIFIED.,.F.,.F.,.F.)
B_SPLINE_SURFACE_WITH_KNOTS((2,2),(3,3),(0.,0.289807040992885),(0.625170525609408,
0.642682999576236),.UNSPECIFIED.)
GEOMETRIC_REPRESENTATION_ITEM()
RATIONAL_B_SPLINE_SURFACE(((0.990658108926709,0.993760979299921,0.999878046252916),
(0.990658108926709,0.993760979299921,0.999878046252916)))
REPRESENTATION_ITEM('')
SURFACE()
);
#3432=(
BOUNDED_SURFACE()
B_SPLINE_SURFACE(1,2,((#152401,#152402,#152403,#152404,#152405),(#152406,
#152407,#152408,#152409,#152410)),.UNSPECIFIED.,.F.,.F.,.F.)
B_SPLINE_SURFACE_WITH_KNOTS((2,2),(3,2,3),(0.,0.289940743905968),(0.0908085233856358,
0.107982157956011,0.108241818468637),.UNSPECIFIED.)
GEOMETRIC_REPRESENTATION_ITEM()
RATIONAL_B_SPLINE_SURFACE(((0.990086238235256,0.987329216372183,0.987470879370255,
0.987470879370255,0.987470879370255),(0.990086238235256,0.987329216372183,
0.987470879370255,0.987470879370255,0.987470879370255)))
REPRESENTATION_ITEM('')
SURFACE()
);
#3433=(
BOUNDED_SURFACE()
B_SPLINE_SURFACE(1,2,((#152414,#152415,#152416),(#152417,#152418,#152419)),
 .UNSPECIFIED.,.F.,.F.,.F.)
B_SPLINE_SURFACE_WITH_KNOTS((2,2),(3,3),(0.,0.289807040991562),(0.625170525609407,
0.642682999576235),.UNSPECIFIED.)
GEOMETRIC_REPRESENTATION_ITEM()
RATIONAL_B_SPLINE_SURFACE(((0.990658108926708,0.993760979299921,0.999878046252916),
(0.990658108926708,0.993760979299921,0.999878046252916)))
REPRESENTATION_ITEM('')
SURFACE()
);
#3434=(
BOUNDED_SURFACE()
B_SPLINE_SURFACE(1,2,((#152421,#152422,#152423,#152424,#152425),(#152426,
#152427,#152428,#152429,#152430)),.UNSPECIFIED.,.F.,.F.,.F.)
B_SPLINE_SURFACE_WITH_KNOTS((2,2),(3,2,3),(0.,0.289940743934749),(0.0908085233856343,
0.107982157956012,0.108241818497582),.UNSPECIFIED.)
GEOMETRIC_REPRESENTATION_ITEM()
RATIONAL_B_SPLINE_SURFACE(((0.990086238235257,0.987329216372183,0.987470879370256,
0.987470879370256,0.987470879370256),(0.990086238235257,0.987329216372183,
0.987470879370256,0.987470879370256,0.987470879370256)))
REPRESENTATION_ITEM('')
SURFACE()
);
#3435=(
BOUNDED_SURFACE()
B_SPLINE_SURFACE(1,2,((#152434,#152435,#152436),(#152437,#152438,#152439)),
 .UNSPECIFIED.,.F.,.F.,.F.)
B_SPLINE_SURFACE_WITH_KNOTS((2,2),(3,3),(0.,0.289807040991874),(0.625170525609407,
0.642682999576234),.UNSPECIFIED.)
GEOMETRIC_REPRESENTATION_ITEM()
RATIONAL_B_SPLINE_SURFACE(((0.990658108926708,0.993760979299921,0.999878046252915),
(0.990658108926708,0.993760979299921,0.999878046252915)))
REPRESENTATION_ITEM('')
SURFACE()
);
#3436=(
BOUNDED_SURFACE()
B_SPLINE_SURFACE(1,2,((#152441,#152442,#152443,#152444,#152445),(#152446,
#152447,#152448,#152449,#152450)),.UNSPECIFIED.,.F.,.F.,.F.)
B_SPLINE_SURFACE_WITH_KNOTS((2,2),(3,2,3),(0.,0.289940744047752),(0.0908085233856344,
0.107982157956012,0.10824181886488),.UNSPECIFIED.)
GEOMETRIC_REPRESENTATION_ITEM()
RATIONAL_B_SPLINE_SURFACE(((0.990086238235257,0.987329216372183,0.987470879370255,
0.987470879370255,0.987470879370255),(0.990086238235257,0.987329216372183,
0.987470879370255,0.987470879370255,0.987470879370255)))
REPRESENTATION_ITEM('')
SURFACE()
);
#3437=(
BOUNDED_SURFACE()
B_SPLINE_SURFACE(1,2,((#152454,#152455,#152456),(#152457,#152458,#152459)),
 .UNSPECIFIED.,.F.,.F.,.F.)
B_SPLINE_SURFACE_WITH_KNOTS((2,2),(3,3),(0.,0.289807040991878),(0.625170525609407,
0.642682999576233),.UNSPECIFIED.)
GEOMETRIC_REPRESENTATION_ITEM()
RATIONAL_B_SPLINE_SURFACE(((0.990658108926708,0.99376097929992,0.999878046252915),
(0.990658108926708,0.99376097929992,0.999878046252915)))
REPRESENTATION_ITEM('')
SURFACE()
);
#3438=(
BOUNDED_SURFACE()
B_SPLINE_SURFACE(1,2,((#152461,#152462,#152463,#152464,#152465),(#152466,
#152467,#152468,#152469,#152470)),.UNSPECIFIED.,.F.,.F.,.F.)
B_SPLINE_SURFACE_WITH_KNOTS((2,2),(3,2,3),(0.,0.28994074393988),(0.0908085233856346,
0.107982157956012,0.108241818456526),.UNSPECIFIED.)
GEOMETRIC_REPRESENTATION_ITEM()
RATIONAL_B_SPLINE_SURFACE(((0.990086238235256,0.987329216372183,0.987470879370255,
0.987470879370255,0.987470879370255),(0.990086238235256,0.987329216372183,
0.987470879370255,0.987470879370255,0.987470879370255)))
REPRESENTATION_ITEM('')
SURFACE()
);
#3439=(
BOUNDED_SURFACE()
B_SPLINE_SURFACE(1,2,((#152474,#152475,#152476),(#152477,#152478,#152479)),
 .UNSPECIFIED.,.F.,.F.,.F.)
B_SPLINE_SURFACE_WITH_KNOTS((2,2),(3,3),(0.,0.28980704099187),(0.625170525609407,
0.642682999576234),.UNSPECIFIED.)
GEOMETRIC_REPRESENTATION_ITEM()
RATIONAL_B_SPLINE_SURFACE(((0.990658108926708,0.993760979299921,0.999878046252915),
(0.990658108926708,0.993760979299921,0.999878046252915)))
REPRESENTATION_ITEM('')
SURFACE()
);
#3440=(
BOUNDED_SURFACE()
B_SPLINE_SURFACE(1,2,((#152481,#152482,#152483,#152484,#152485),(#152486,
#152487,#152488,#152489,#152490)),.UNSPECIFIED.,.F.,.F.,.F.)
B_SPLINE_SURFACE_WITH_KNOTS((2,2),(3,2,3),(0.,0.289940743950375),(0.0908085233856344,
0.107982157956012,0.108241818466931),.UNSPECIFIED.)
GEOMETRIC_REPRESENTATION_ITEM()
RATIONAL_B_SPLINE_SURFACE(((0.990086238235257,0.987329216372183,0.987470879370255,
0.987470879370255,0.987470879370255),(0.990086238235256,0.987329216372183,
0.987470879370255,0.987470879370255,0.987470879370255)))
REPRESENTATION_ITEM('')
SURFACE()
);
#3441=(
BOUNDED_SURFACE()
B_SPLINE_SURFACE(1,2,((#152494,#152495,#152496),(#152497,#152498,#152499)),
 .UNSPECIFIED.,.F.,.F.,.F.)
B_SPLINE_SURFACE_WITH_KNOTS((2,2),(3,3),(0.,0.289807040991884),(0.625170525609407,
0.642682999576233),.UNSPECIFIED.)
GEOMETRIC_REPRESENTATION_ITEM()
RATIONAL_B_SPLINE_SURFACE(((0.990658108926708,0.99376097929992,0.999878046252915),
(0.990658108926708,0.99376097929992,0.999878046252915)))
REPRESENTATION_ITEM('')
SURFACE()
);
#3442=(
BOUNDED_SURFACE()
B_SPLINE_SURFACE(1,2,((#152501,#152502,#152503,#152504,#152505),(#152506,
#152507,#152508,#152509,#152510)),.UNSPECIFIED.,.F.,.F.,.F.)
B_SPLINE_SURFACE_WITH_KNOTS((2,2),(3,2,3),(0.,0.289681084359931),(0.573550810617332,
0.590910950629594,0.591084552029717),.UNSPECIFIED.)
GEOMETRIC_REPRESENTATION_ITEM()
RATIONAL_B_SPLINE_SURFACE(((0.998554414400274,0.992822941359345,0.990053454406147,
0.990053454406147,0.990053454406147),(0.998554414400274,0.992822941359345,
0.990053454406148,0.990053454406148,0.990053454406148)))
REPRESENTATION_ITEM('')
SURFACE()
);
#3443=(
BOUNDED_SURFACE()
B_SPLINE_SURFACE(1,2,((#152521,#152522,#152523,#152524,#152525,#152526,
#152527),(#152528,#152529,#152530,#152531,#152532,#152533,#152534)),
 .UNSPECIFIED.,.F.,.F.,.F.)
B_SPLINE_SURFACE_WITH_KNOTS((2,2),(3,2,2,3),(0.,0.289807040991565),(0.142404283483303,
0.142578551421364,0.142857142857143,0.160005345227479),.UNSPECIFIED.)
GEOMETRIC_REPRESENTATION_ITEM()
RATIONAL_B_SPLINE_SURFACE(((0.999805186472059,0.999805186472059,0.999805186472059,
0.999902211834795,1.,0.993980822699459,0.990851751371591),(0.999805186472059,
0.999805186472059,0.999805186472059,0.999902211834795,1.,0.993980822699459,
0.990851751371591)))
REPRESENTATION_ITEM('')
SURFACE()
);
#3444=(
BOUNDED_SURFACE()
B_SPLINE_SURFACE(1,2,((#152551,#152552,#152553,#152554,#152555),(#152556,
#152557,#152558,#152559,#152560)),.UNSPECIFIED.,.F.,.F.,.F.)
B_SPLINE_SURFACE_WITH_KNOTS((2,2),(3,2,3),(0.,0.289681084359923),(0.573550810617263,
0.590910950629593,0.591084552029716),.UNSPECIFIED.)
GEOMETRIC_REPRESENTATION_ITEM()
RATIONAL_B_SPLINE_SURFACE(((0.99855441440032,0.992822941359356,0.990053454406147,
0.990053454406147,0.990053454406147),(0.99855441440032,0.992822941359356,
0.990053454406147,0.990053454406147,0.990053454406147)))
REPRESENTATION_ITEM('')
SURFACE()
);
#3445=(
BOUNDED_SURFACE()
B_SPLINE_SURFACE(1,2,((#152562,#152563,#152564,#152565,#152566,#152567,
#152568),(#152569,#152570,#152571,#152572,#152573,#152574,#152575)),
 .UNSPECIFIED.,.F.,.F.,.F.)
B_SPLINE_SURFACE_WITH_KNOTS((2,2),(3,2,2,3),(0.,0.289807040991559),(0.142404283483179,
0.142578551421241,0.142857142857143,0.16000534522748),.UNSPECIFIED.)
GEOMETRIC_REPRESENTATION_ITEM()
RATIONAL_B_SPLINE_SURFACE(((0.999805186471973,0.999805186471973,0.999805186471973,
0.999902211834752,1.,0.993980822699459,0.990851751371591),(0.999805186471973,
0.999805186471973,0.999805186471973,0.999902211834752,1.,0.993980822699459,
0.990851751371591)))
REPRESENTATION_ITEM('')
SURFACE()
);
#3446=(
BOUNDED_SURFACE()
B_SPLINE_SURFACE(1,2,((#152592,#152593,#152594,#152595,#152596),(#152597,
#152598,#152599,#152600,#152601)),.UNSPECIFIED.,.F.,.F.,.F.)
B_SPLINE_SURFACE_WITH_KNOTS((2,2),(3,2,3),(0.,0.289681084359933),(0.573550810617452,
0.590910950629594,0.591084552029715),.UNSPECIFIED.)
GEOMETRIC_REPRESENTATION_ITEM()
RATIONAL_B_SPLINE_SURFACE(((0.998554414400195,0.992822941359326,0.990053454406148,
0.990053454406148,0.990053454406148),(0.998554414400195,0.992822941359326,
0.990053454406148,0.990053454406148,0.990053454406148)))
REPRESENTATION_ITEM('')
SURFACE()
);
#3447=(
BOUNDED_SURFACE()
B_SPLINE_SURFACE(1,2,((#152603,#152604,#152605,#152606,#152607,#152608,
#152609),(#152610,#152611,#152612,#152613,#152614,#152615,#152616)),
 .UNSPECIFIED.,.F.,.F.,.F.)
B_SPLINE_SURFACE_WITH_KNOTS((2,2),(3,2,2,3),(0.,0.289807040991559),(0.142404283483291,
0.142578551421352,0.142857142857143,0.160005345227478),.UNSPECIFIED.)
GEOMETRIC_REPRESENTATION_ITEM()
RATIONAL_B_SPLINE_SURFACE(((0.99980518647205,0.99980518647205,0.99980518647205,
0.99990221183479,1.,0.993980822699459,0.990851751371592),(0.99980518647205,
0.99980518647205,0.99980518647205,0.99990221183479,1.,0.993980822699459,
0.990851751371592)))
REPRESENTATION_ITEM('')
SURFACE()
);
#3448=(
BOUNDED_SURFACE()
B_SPLINE_SURFACE(1,2,((#152633,#152634,#152635,#152636,#152637),(#152638,
#152639,#152640,#152641,#152642)),.UNSPECIFIED.,.F.,.F.,.F.)
B_SPLINE_SURFACE_WITH_KNOTS((2,2),(3,2,3),(0.,0.289681084359915),(0.573550810617204,
0.590910950629595,0.591084552029719),.UNSPECIFIED.)
GEOMETRIC_REPRESENTATION_ITEM()
RATIONAL_B_SPLINE_SURFACE(((0.998554414400359,0.992822941359365,0.990053454406147,
0.990053454406147,0.990053454406147),(0.998554414400359,0.992822941359365,
0.990053454406147,0.990053454406147,0.990053454406147)))
REPRESENTATION_ITEM('')
SURFACE()
);
#3449=(
BOUNDED_SURFACE()
B_SPLINE_SURFACE(1,2,((#152644,#152645,#152646,#152647,#152648,#152649,
#152650),(#152651,#152652,#152653,#152654,#152655,#152656,#152657)),
 .UNSPECIFIED.,.F.,.F.,.F.)
B_SPLINE_SURFACE_WITH_KNOTS((2,2),(3,2,2,3),(0.,0.289807040991563),(0.142404283483062,
0.142578551421126,0.142857142857143,0.160005345227473),.UNSPECIFIED.)
GEOMETRIC_REPRESENTATION_ITEM()
RATIONAL_B_SPLINE_SURFACE(((0.999805186471894,0.999805186471894,0.999805186471894,
0.999902211834711,1.,0.993980822699461,0.990851751371593),(0.999805186471894,
0.999805186471894,0.999805186471894,0.999902211834711,1.,0.993980822699461,
0.990851751371593)))
REPRESENTATION_ITEM('')
SURFACE()
);
#3450=(
BOUNDED_SURFACE()
B_SPLINE_SURFACE(1,2,((#152674,#152675,#152676,#152677,#152678),(#152679,
#152680,#152681,#152682,#152683)),.UNSPECIFIED.,.F.,.F.,.F.)
B_SPLINE_SURFACE_WITH_KNOTS((2,2),(3,2,3),(0.,0.289681084359931),(0.573550810617335,
0.590910950629595,0.591084552029718),.UNSPECIFIED.)
GEOMETRIC_REPRESENTATION_ITEM()
RATIONAL_B_SPLINE_SURFACE(((0.998554414400272,0.992822941359344,0.990053454406147,
0.990053454406147,0.990053454406147),(0.998554414400272,0.992822941359344,
0.990053454406147,0.990053454406147,0.990053454406147)))
REPRESENTATION_ITEM('')
SURFACE()
);
#3451=(
BOUNDED_SURFACE()
B_SPLINE_SURFACE(1,2,((#152685,#152686,#152687,#152688,#152689,#152690,
#152691),(#152692,#152693,#152694,#152695,#152696,#152697,#152698)),
 .UNSPECIFIED.,.F.,.F.,.F.)
B_SPLINE_SURFACE_WITH_KNOTS((2,2),(3,2,2,3),(0.,0.289807040991561),(0.142404283483294,
0.142578551421355,0.142857142857143,0.160005345227478),.UNSPECIFIED.)
GEOMETRIC_REPRESENTATION_ITEM()
RATIONAL_B_SPLINE_SURFACE(((0.999805186472053,0.999805186472053,0.999805186472053,
0.999902211834792,1.,0.993980822699459,0.990851751371591),(0.999805186472053,
0.999805186472053,0.999805186472053,0.999902211834792,1.,0.993980822699459,
0.990851751371591)))
REPRESENTATION_ITEM('')
SURFACE()
);
#3452=(
BOUNDED_SURFACE()
B_SPLINE_SURFACE(1,2,((#152715,#152716,#152717,#152718,#152719),(#152720,
#152721,#152722,#152723,#152724)),.UNSPECIFIED.,.F.,.F.,.F.)
B_SPLINE_SURFACE_WITH_KNOTS((2,2),(3,2,3),(0.,0.289681084359922),(0.573550810617453,
0.590910950629595,0.591084552029716),.UNSPECIFIED.)
GEOMETRIC_REPRESENTATION_ITEM()
RATIONAL_B_SPLINE_SURFACE(((0.998554414400194,0.992822941359325,0.990053454406147,
0.990053454406147,0.990053454406147),(0.998554414400194,0.992822941359325,
0.990053454406147,0.990053454406147,0.990053454406147)))
REPRESENTATION_ITEM('')
SURFACE()
);
#3453=(
BOUNDED_SURFACE()
B_SPLINE_SURFACE(1,2,((#152726,#152727,#152728,#152729,#152730,#152731,
#152732),(#152733,#152734,#152735,#152736,#152737,#152738,#152739)),
 .UNSPECIFIED.,.F.,.F.,.F.)
B_SPLINE_SURFACE_WITH_KNOTS((2,2),(3,2,2,3),(0.,0.28980704099156),(0.142404283482878,
0.142578551420943,0.142857142857143,0.160005345227481),.UNSPECIFIED.)
GEOMETRIC_REPRESENTATION_ITEM()
RATIONAL_B_SPLINE_SURFACE(((0.999805186471766,0.999805186471766,0.999805186471766,
0.999902211834647,1.,0.993980822699458,0.99085175137159),(0.999805186471766,
0.999805186471766,0.999805186471766,0.999902211834647,1.,0.993980822699458,
0.99085175137159)))
REPRESENTATION_ITEM('')
SURFACE()
);
#3454=(
BOUNDED_SURFACE()
B_SPLINE_SURFACE(1,2,((#152756,#152757,#152758,#152759,#152760),(#152761,
#152762,#152763,#152764,#152765)),.UNSPECIFIED.,.F.,.F.,.F.)
B_SPLINE_SURFACE_WITH_KNOTS((2,2),(3,2,3),(0.,0.289681084359927),(0.573550810617453,
0.590910950629595,0.591084552029716),.UNSPECIFIED.)
GEOMETRIC_REPRESENTATION_ITEM()
RATIONAL_B_SPLINE_SURFACE(((0.998554414400194,0.992822941359325,0.990053454406147,
0.990053454406147,0.990053454406147),(0.998554414400194,0.992822941359325,
0.990053454406147,0.990053454406147,0.990053454406147)))
REPRESENTATION_ITEM('')
SURFACE()
);
#3455=(
BOUNDED_SURFACE()
B_SPLINE_SURFACE(1,2,((#152767,#152768,#152769,#152770,#152771,#152772,
#152773),(#152774,#152775,#152776,#152777,#152778,#152779,#152780)),
 .UNSPECIFIED.,.F.,.F.,.F.)
B_SPLINE_SURFACE_WITH_KNOTS((2,2),(3,2,2,3),(0.,0.289807040991564),(0.142404283483302,
0.142578551421363,0.142857142857143,0.160005345227478),.UNSPECIFIED.)
GEOMETRIC_REPRESENTATION_ITEM()
RATIONAL_B_SPLINE_SURFACE(((0.999805186472059,0.999805186472059,0.999805186472059,
0.999902211834794,1.,0.993980822699459,0.990851751371591),(0.999805186472059,
0.999805186472059,0.999805186472059,0.999902211834794,1.,0.993980822699459,
0.990851751371591)))
REPRESENTATION_ITEM('')
SURFACE()
);
#3456=(
BOUNDED_SURFACE()
B_SPLINE_SURFACE(1,2,((#152788,#152789,#152790,#152791,#152792),(#152793,
#152794,#152795,#152796,#152797)),.UNSPECIFIED.,.F.,.F.,.F.)
B_SPLINE_SURFACE_WITH_KNOTS((2,2),(3,2,3),(0.,0.289681084359926),(0.573550810617453,
0.590910950629595,0.591084552029716),.UNSPECIFIED.)
GEOMETRIC_REPRESENTATION_ITEM()
RATIONAL_B_SPLINE_SURFACE(((0.998554414400194,0.992822941359325,0.990053454406147,
0.990053454406147,0.990053454406147),(0.998554414400194,0.992822941359325,
0.990053454406147,0.990053454406147,0.990053454406147)))
REPRESENTATION_ITEM('')
SURFACE()
);
#3457=(
BOUNDED_SURFACE()
B_SPLINE_SURFACE(1,2,((#152799,#152800,#152801,#152802,#152803,#152804,
#152805),(#152806,#152807,#152808,#152809,#152810,#152811,#152812)),
 .UNSPECIFIED.,.F.,.F.,.F.)
B_SPLINE_SURFACE_WITH_KNOTS((2,2),(3,2,2,3),(0.,0.289807040991561),(0.142404283483292,
0.142578551421353,0.142857142857143,0.160005345227478),.UNSPECIFIED.)
GEOMETRIC_REPRESENTATION_ITEM()
RATIONAL_B_SPLINE_SURFACE(((0.999805186472051,0.999805186472051,0.999805186472051,
0.999902211834791,1.,0.993980822699459,0.990851751371592),(0.999805186472051,
0.999805186472051,0.999805186472051,0.999902211834791,1.,0.993980822699459,
0.990851751371592)))
REPRESENTATION_ITEM('')
SURFACE()
);
#3458=(
BOUNDED_SURFACE()
B_SPLINE_SURFACE(1,2,((#152829,#152830,#152831,#152832,#152833),(#152834,
#152835,#152836,#152837,#152838)),.UNSPECIFIED.,.F.,.F.,.F.)
B_SPLINE_SURFACE_WITH_KNOTS((2,2),(3,2,3),(0.,0.289681084359916),(0.573550810617453,
0.590910950629595,0.591084552029716),.UNSPECIFIED.)
GEOMETRIC_REPRESENTATION_ITEM()
RATIONAL_B_SPLINE_SURFACE(((0.998554414400194,0.992822941359325,0.990053454406147,
0.990053454406147,0.990053454406147),(0.998554414400194,0.992822941359325,
0.990053454406147,0.990053454406147,0.990053454406147)))
REPRESENTATION_ITEM('')
SURFACE()
);
#3459=(
BOUNDED_SURFACE()
B_SPLINE_SURFACE(1,2,((#152840,#152841,#152842,#152843,#152844,#152845,
#152846),(#152847,#152848,#152849,#152850,#152851,#152852,#152853)),
 .UNSPECIFIED.,.F.,.F.,.F.)
B_SPLINE_SURFACE_WITH_KNOTS((2,2),(3,2,2,3),(0.,0.289807040991557),(0.142404283483302,
0.142578551421363,0.142857142857143,0.160005345227478),.UNSPECIFIED.)
GEOMETRIC_REPRESENTATION_ITEM()
RATIONAL_B_SPLINE_SURFACE(((0.999805186472059,0.999805186472059,0.999805186472059,
0.999902211834794,1.,0.993980822699459,0.990851751371592),(0.999805186472059,
0.999805186472059,0.999805186472059,0.999902211834794,1.,0.993980822699459,
0.990851751371592)))
REPRESENTATION_ITEM('')
SURFACE()
);
#3460=(
BOUNDED_SURFACE()
B_SPLINE_SURFACE(1,2,((#152870,#152871,#152872,#152873,#152874),(#152875,
#152876,#152877,#152878,#152879)),.UNSPECIFIED.,.F.,.F.,.F.)
B_SPLINE_SURFACE_WITH_KNOTS((2,2),(3,2,3),(0.,0.289681084359915),(0.573550810617453,
0.590910950629595,0.591084552029716),.UNSPECIFIED.)
GEOMETRIC_REPRESENTATION_ITEM()
RATIONAL_B_SPLINE_SURFACE(((0.998554414400194,0.992822941359325,0.990053454406147,
0.990053454406147,0.990053454406147),(0.998554414400194,0.992822941359325,
0.990053454406147,0.990053454406147,0.990053454406147)))
REPRESENTATION_ITEM('')
SURFACE()
);
#3461=(
BOUNDED_SURFACE()
B_SPLINE_SURFACE(1,2,((#152881,#152882,#152883,#152884,#152885,#152886,
#152887),(#152888,#152889,#152890,#152891,#152892,#152893,#152894)),
 .UNSPECIFIED.,.F.,.F.,.F.)
B_SPLINE_SURFACE_WITH_KNOTS((2,2),(3,2,2,3),(0.,0.289807040991559),(0.142404283482981,
0.142578551421045,0.142857142857143,0.16000534522748),.UNSPECIFIED.)
GEOMETRIC_REPRESENTATION_ITEM()
RATIONAL_B_SPLINE_SURFACE(((0.999805186471836,0.999805186471836,0.999805186471836,
0.999902211834683,1.,0.993980822699459,0.990851751371591),(0.999805186471836,
0.999805186471836,0.999805186471836,0.999902211834683,1.,0.993980822699459,
0.990851751371591)))
REPRESENTATION_ITEM('')
SURFACE()
);
#3462=(
BOUNDED_SURFACE()
B_SPLINE_SURFACE(1,2,((#152911,#152912,#152913,#152914,#152915),(#152916,
#152917,#152918,#152919,#152920)),.UNSPECIFIED.,.F.,.F.,.F.)
B_SPLINE_SURFACE_WITH_KNOTS((2,2),(3,2,3),(0.,0.289681084359914),(0.573550810617378,
0.590910950629595,0.591084552029717),.UNSPECIFIED.)
GEOMETRIC_REPRESENTATION_ITEM()
RATIONAL_B_SPLINE_SURFACE(((0.998554414400244,0.992822941359337,0.990053454406147,
0.990053454406147,0.990053454406147),(0.998554414400244,0.992822941359337,
0.990053454406147,0.990053454406147,0.990053454406147)))
REPRESENTATION_ITEM('')
SURFACE()
);
#3463=(
BOUNDED_SURFACE()
B_SPLINE_SURFACE(1,2,((#152922,#152923,#152924,#152925,#152926,#152927,
#152928),(#152929,#152930,#152931,#152932,#152933,#152934,#152935)),
 .UNSPECIFIED.,.F.,.F.,.F.)
B_SPLINE_SURFACE_WITH_KNOTS((2,2),(3,2,2,3),(0.,0.289807040991562),(0.142404283483302,
0.142578551421363,0.142857142857143,0.160005345227478),.UNSPECIFIED.)
GEOMETRIC_REPRESENTATION_ITEM()
RATIONAL_B_SPLINE_SURFACE(((0.999805186472058,0.999805186472058,0.999805186472058,
0.999902211834794,1.,0.993980822699459,0.990851751371592),(0.999805186472058,
0.999805186472058,0.999805186472058,0.999902211834794,1.,0.993980822699459,
0.990851751371592)))
REPRESENTATION_ITEM('')
SURFACE()
);
#3464=(
BOUNDED_SURFACE()
B_SPLINE_SURFACE(1,2,((#152952,#152953,#152954,#152955,#152956),(#152957,
#152958,#152959,#152960,#152961)),.UNSPECIFIED.,.F.,.F.,.F.)
B_SPLINE_SURFACE_WITH_KNOTS((2,2),(3,2,3),(0.,0.289681084359919),(0.573550810617453,
0.590910950629595,0.591084552029716),.UNSPECIFIED.)
GEOMETRIC_REPRESENTATION_ITEM()
RATIONAL_B_SPLINE_SURFACE(((0.998554414400194,0.992822941359325,0.990053454406147,
0.990053454406147,0.990053454406147),(0.998554414400194,0.992822941359325,
0.990053454406147,0.990053454406147,0.990053454406147)))
REPRESENTATION_ITEM('')
SURFACE()
);
#3465=(
BOUNDED_SURFACE()
B_SPLINE_SURFACE(1,2,((#152963,#152964,#152965,#152966,#152967,#152968,
#152969),(#152970,#152971,#152972,#152973,#152974,#152975,#152976)),
 .UNSPECIFIED.,.F.,.F.,.F.)
B_SPLINE_SURFACE_WITH_KNOTS((2,2),(3,2,2,3),(0.,0.289807040991563),(0.142404283483231,
0.142578551421293,0.142857142857143,0.160005345227479),.UNSPECIFIED.)
GEOMETRIC_REPRESENTATION_ITEM()
RATIONAL_B_SPLINE_SURFACE(((0.999805186472009,0.999805186472009,0.999805186472009,
0.99990221183477,1.,0.993980822699459,0.990851751371591),(0.999805186472009,
0.999805186472009,0.999805186472009,0.99990221183477,1.,0.993980822699459,
0.990851751371591)))
REPRESENTATION_ITEM('')
SURFACE()
);
#3466=(
BOUNDED_SURFACE()
B_SPLINE_SURFACE(1,2,((#152993,#152994,#152995,#152996,#152997),(#152998,
#152999,#153000,#153001,#153002)),.UNSPECIFIED.,.F.,.F.,.F.)
B_SPLINE_SURFACE_WITH_KNOTS((2,2),(3,2,3),(0.,0.28968108435992),(0.573550810617453,
0.590910950629595,0.591084552029716),.UNSPECIFIED.)
GEOMETRIC_REPRESENTATION_ITEM()
RATIONAL_B_SPLINE_SURFACE(((0.998554414400194,0.992822941359325,0.990053454406147,
0.990053454406147,0.990053454406147),(0.998554414400194,0.992822941359325,
0.990053454406147,0.990053454406147,0.990053454406147)))
REPRESENTATION_ITEM('')
SURFACE()
);
#3467=(
BOUNDED_SURFACE()
B_SPLINE_SURFACE(1,2,((#153004,#153005,#153006,#153007,#153008,#153009,
#153010),(#153011,#153012,#153013,#153014,#153015,#153016,#153017)),
 .UNSPECIFIED.,.F.,.F.,.F.)
B_SPLINE_SURFACE_WITH_KNOTS((2,2),(3,2,2,3),(0.,0.28980704099156),(0.142404283483302,
0.142578551421363,0.142857142857143,0.160005345227478),.UNSPECIFIED.)
GEOMETRIC_REPRESENTATION_ITEM()
RATIONAL_B_SPLINE_SURFACE(((0.999805186472059,0.999805186472059,0.999805186472059,
0.999902211834794,1.,0.993980822699459,0.990851751371591),(0.999805186472059,
0.999805186472059,0.999805186472059,0.999902211834794,1.,0.993980822699459,
0.990851751371591)))
REPRESENTATION_ITEM('')
SURFACE()
);
#3468=(
BOUNDED_SURFACE()
B_SPLINE_SURFACE(1,2,((#153034,#153035,#153036,#153037,#153038),(#153039,
#153040,#153041,#153042,#153043)),.UNSPECIFIED.,.F.,.F.,.F.)
B_SPLINE_SURFACE_WITH_KNOTS((2,2),(3,2,3),(0.,0.28968108435992),(0.573550810617453,
0.590910950629595,0.591084552029716),.UNSPECIFIED.)
GEOMETRIC_REPRESENTATION_ITEM()
RATIONAL_B_SPLINE_SURFACE(((0.998554414400194,0.992822941359325,0.990053454406147,
0.990053454406147,0.990053454406147),(0.998554414400194,0.992822941359325,
0.990053454406147,0.990053454406147,0.990053454406147)))
REPRESENTATION_ITEM('')
SURFACE()
);
#3469=(
BOUNDED_SURFACE()
B_SPLINE_SURFACE(1,2,((#153045,#153046,#153047,#153048,#153049,#153050,
#153051),(#153052,#153053,#153054,#153055,#153056,#153057,#153058)),
 .UNSPECIFIED.,.F.,.F.,.F.)
B_SPLINE_SURFACE_WITH_KNOTS((2,2),(3,2,2,3),(0.,0.289807040991565),(0.142404283483023,
0.142578551421087,0.142857142857143,0.16000534522748),.UNSPECIFIED.)
GEOMETRIC_REPRESENTATION_ITEM()
RATIONAL_B_SPLINE_SURFACE(((0.999805186471866,0.999805186471866,0.999805186471866,
0.999902211834697,1.,0.993980822699459,0.990851751371591),(0.999805186471866,
0.999805186471866,0.999805186471866,0.999902211834697,1.,0.993980822699459,
0.990851751371591)))
REPRESENTATION_ITEM('')
SURFACE()
);
#3470=(
BOUNDED_SURFACE()
B_SPLINE_SURFACE(1,2,((#153075,#153076,#153077,#153078,#153079),(#153080,
#153081,#153082,#153083,#153084)),.UNSPECIFIED.,.F.,.F.,.F.)
B_SPLINE_SURFACE_WITH_KNOTS((2,2),(3,2,3),(0.,0.289681084359922),(0.573550810617453,
0.590910950629595,0.591084552029716),.UNSPECIFIED.)
GEOMETRIC_REPRESENTATION_ITEM()
RATIONAL_B_SPLINE_SURFACE(((0.998554414400194,0.992822941359325,0.990053454406147,
0.990053454406147,0.990053454406147),(0.998554414400194,0.992822941359325,
0.990053454406147,0.990053454406147,0.990053454406147)))
REPRESENTATION_ITEM('')
SURFACE()
);
#3471=(
BOUNDED_SURFACE()
B_SPLINE_SURFACE(1,2,((#153086,#153087,#153088,#153089,#153090,#153091,
#153092),(#153093,#153094,#153095,#153096,#153097,#153098,#153099)),
 .UNSPECIFIED.,.F.,.F.,.F.)
B_SPLINE_SURFACE_WITH_KNOTS((2,2),(3,2,2,3),(0.,0.289807040991562),(0.142404283483302,
0.142578551421363,0.142857142857143,0.160005345227478),.UNSPECIFIED.)
GEOMETRIC_REPRESENTATION_ITEM()
RATIONAL_B_SPLINE_SURFACE(((0.999805186472058,0.999805186472058,0.999805186472058,
0.999902211834794,1.,0.993980822699459,0.990851751371591),(0.999805186472058,
0.999805186472058,0.999805186472058,0.999902211834794,1.,0.993980822699459,
0.990851751371591)))
REPRESENTATION_ITEM('')
SURFACE()
);
#3472=(
BOUNDED_SURFACE()
B_SPLINE_SURFACE(1,2,((#153116,#153117,#153118,#153119,#153120),(#153121,
#153122,#153123,#153124,#153125)),.UNSPECIFIED.,.F.,.F.,.F.)
B_SPLINE_SURFACE_WITH_KNOTS((2,2),(3,2,3),(0.,0.289681084359919),(0.573550810617453,
0.590910950629595,0.591084552029716),.UNSPECIFIED.)
GEOMETRIC_REPRESENTATION_ITEM()
RATIONAL_B_SPLINE_SURFACE(((0.998554414400194,0.992822941359325,0.990053454406147,
0.990053454406147,0.990053454406147),(0.998554414400194,0.992822941359325,
0.990053454406147,0.990053454406147,0.990053454406147)))
REPRESENTATION_ITEM('')
SURFACE()
);
#3473=(
BOUNDED_SURFACE()
B_SPLINE_SURFACE(1,2,((#153127,#153128,#153129,#153130,#153131,#153132,
#153133),(#153134,#153135,#153136,#153137,#153138,#153139,#153140)),
 .UNSPECIFIED.,.F.,.F.,.F.)
B_SPLINE_SURFACE_WITH_KNOTS((2,2),(3,2,2,3),(0.,0.289807040991558),(0.142404283483302,
0.142578551421363,0.142857142857143,0.160005345227478),.UNSPECIFIED.)
GEOMETRIC_REPRESENTATION_ITEM()
RATIONAL_B_SPLINE_SURFACE(((0.999805186472058,0.999805186472058,0.999805186472058,
0.999902211834794,1.,0.993980822699459,0.990851751371591),(0.999805186472058,
0.999805186472058,0.999805186472058,0.999902211834794,1.,0.993980822699459,
0.990851751371591)))
REPRESENTATION_ITEM('')
SURFACE()
);
#3474=(
BOUNDED_SURFACE()
B_SPLINE_SURFACE(1,2,((#153157,#153158,#153159,#153160,#153161),(#153162,
#153163,#153164,#153165,#153166)),.UNSPECIFIED.,.F.,.F.,.F.)
B_SPLINE_SURFACE_WITH_KNOTS((2,2),(3,2,3),(0.,0.289681084359915),(0.573550810617453,
0.590910950629595,0.591084552029716),.UNSPECIFIED.)
GEOMETRIC_REPRESENTATION_ITEM()
RATIONAL_B_SPLINE_SURFACE(((0.998554414400194,0.992822941359325,0.990053454406147,
0.990053454406147,0.990053454406147),(0.998554414400194,0.992822941359325,
0.990053454406147,0.990053454406147,0.990053454406147)))
REPRESENTATION_ITEM('')
SURFACE()
);
#3475=(
BOUNDED_SURFACE()
B_SPLINE_SURFACE(1,2,((#153168,#153169,#153170,#153171,#153172,#153173,
#153174),(#153175,#153176,#153177,#153178,#153179,#153180,#153181)),
 .UNSPECIFIED.,.F.,.F.,.F.)
B_SPLINE_SURFACE_WITH_KNOTS((2,2),(3,2,2,3),(0.,0.289807040991559),(0.142404283483302,
0.142578551421363,0.142857142857143,0.160005345227478),.UNSPECIFIED.)
GEOMETRIC_REPRESENTATION_ITEM()
RATIONAL_B_SPLINE_SURFACE(((0.999805186472058,0.999805186472058,0.999805186472058,
0.999902211834794,1.,0.993980822699459,0.990851751371592),(0.999805186472058,
0.999805186472058,0.999805186472058,0.999902211834794,1.,0.993980822699459,
0.990851751371592)))
REPRESENTATION_ITEM('')
SURFACE()
);
#3476=(
BOUNDED_SURFACE()
B_SPLINE_SURFACE(1,2,((#153198,#153199,#153200,#153201,#153202),(#153203,
#153204,#153205,#153206,#153207)),.UNSPECIFIED.,.F.,.F.,.F.)
B_SPLINE_SURFACE_WITH_KNOTS((2,2),(3,2,3),(0.,0.289681084359918),(0.573550810617453,
0.590910950629595,0.591084552029716),.UNSPECIFIED.)
GEOMETRIC_REPRESENTATION_ITEM()
RATIONAL_B_SPLINE_SURFACE(((0.998554414400194,0.992822941359325,0.990053454406147,
0.990053454406147,0.990053454406147),(0.998554414400194,0.992822941359325,
0.990053454406147,0.990053454406147,0.990053454406147)))
REPRESENTATION_ITEM('')
SURFACE()
);
#3477=(
BOUNDED_SURFACE()
B_SPLINE_SURFACE(1,2,((#153209,#153210,#153211,#153212,#153213,#153214,
#153215),(#153216,#153217,#153218,#153219,#153220,#153221,#153222)),
 .UNSPECIFIED.,.F.,.F.,.F.)
B_SPLINE_SURFACE_WITH_KNOTS((2,2),(3,2,2,3),(0.,0.289807040991562),(0.142404283483302,
0.142578551421363,0.142857142857143,0.160005345227478),.UNSPECIFIED.)
GEOMETRIC_REPRESENTATION_ITEM()
RATIONAL_B_SPLINE_SURFACE(((0.999805186472059,0.999805186472059,0.999805186472059,
0.999902211834794,1.,0.993980822699459,0.990851751371591),(0.999805186472059,
0.999805186472059,0.999805186472059,0.999902211834794,1.,0.993980822699459,
0.990851751371591)))
REPRESENTATION_ITEM('')
SURFACE()
);
#3478=(
BOUNDED_SURFACE()
B_SPLINE_SURFACE(1,2,((#153233,#153234,#153235,#153236,#153237),(#153238,
#153239,#153240,#153241,#153242)),.UNSPECIFIED.,.F.,.F.,.F.)
B_SPLINE_SURFACE_WITH_KNOTS((2,2),(3,2,3),(0.,0.289681084360141),(0.573550810617453,
0.590910950629595,0.591084552029716),.UNSPECIFIED.)
GEOMETRIC_REPRESENTATION_ITEM()
RATIONAL_B_SPLINE_SURFACE(((0.998554414400194,0.992822941359325,0.990053454406147,
0.990053454406147,0.990053454406147),(0.998554414400194,0.992822941359325,
0.990053454406147,0.990053454406147,0.990053454406147)))
REPRESENTATION_ITEM('')
SURFACE()
);
#3479=(
BOUNDED_SURFACE()
B_SPLINE_SURFACE(1,2,((#153250,#153251,#153252,#153253,#153254,#153255,
#153256),(#153257,#153258,#153259,#153260,#153261,#153262,#153263)),
 .UNSPECIFIED.,.F.,.F.,.F.)
B_SPLINE_SURFACE_WITH_KNOTS((2,2),(3,2,2,3),(0.,0.289807040991562),(0.142404283483302,
0.142578551421363,0.142857142857143,0.160005345227478),.UNSPECIFIED.)
GEOMETRIC_REPRESENTATION_ITEM()
RATIONAL_B_SPLINE_SURFACE(((0.999805186472059,0.999805186472059,0.999805186472059,
0.999902211834794,1.,0.993980822699459,0.990851751371591),(0.999805186472059,
0.999805186472059,0.999805186472059,0.999902211834794,1.,0.993980822699459,
0.990851751371591)))
REPRESENTATION_ITEM('')
SURFACE()
);
#3480=(
BOUNDED_SURFACE()
B_SPLINE_SURFACE(1,2,((#153280,#153281,#153282,#153283,#153284),(#153285,
#153286,#153287,#153288,#153289)),.UNSPECIFIED.,.F.,.F.,.F.)
B_SPLINE_SURFACE_WITH_KNOTS((2,2),(3,2,3),(0.,0.289681084359929),(0.573550810617453,
0.590910950629594,0.591084552029715),.UNSPECIFIED.)
GEOMETRIC_REPRESENTATION_ITEM()
RATIONAL_B_SPLINE_SURFACE(((0.998554414400194,0.992822941359326,0.990053454406147,
0.990053454406147,0.990053454406147),(0.998554414400194,0.992822941359326,
0.990053454406147,0.990053454406147,0.990053454406147)))
REPRESENTATION_ITEM('')
SURFACE()
);
#3481=(
BOUNDED_SURFACE()
B_SPLINE_SURFACE(1,2,((#153291,#153292,#153293,#153294,#153295,#153296,
#153297),(#153298,#153299,#153300,#153301,#153302,#153303,#153304)),
 .UNSPECIFIED.,.F.,.F.,.F.)
B_SPLINE_SURFACE_WITH_KNOTS((2,2),(3,2,2,3),(0.,0.289807040991557),(0.142404283483303,
0.142578551421364,0.142857142857143,0.160005345227479),.UNSPECIFIED.)
GEOMETRIC_REPRESENTATION_ITEM()
RATIONAL_B_SPLINE_SURFACE(((0.999805186472059,0.999805186472059,0.999805186472059,
0.999902211834795,1.,0.993980822699459,0.990851751371591),(0.999805186472059,
0.999805186472059,0.999805186472059,0.999902211834795,1.,0.993980822699459,
0.990851751371591)))
REPRESENTATION_ITEM('')
SURFACE()
);
#3482=(
BOUNDED_SURFACE()
B_SPLINE_SURFACE(1,2,((#153321,#153322,#153323,#153324,#153325),(#153326,
#153327,#153328,#153329,#153330)),.UNSPECIFIED.,.F.,.F.,.F.)
B_SPLINE_SURFACE_WITH_KNOTS((2,2),(3,2,3),(0.,0.289681084359923),(0.573550810617443,
0.590910950629593,0.591084552029714),.UNSPECIFIED.)
GEOMETRIC_REPRESENTATION_ITEM()
RATIONAL_B_SPLINE_SURFACE(((0.998554414400201,0.992822941359327,0.990053454406148,
0.990053454406148,0.990053454406148),(0.998554414400201,0.992822941359327,
0.990053454406148,0.990053454406148,0.990053454406148)))
REPRESENTATION_ITEM('')
SURFACE()
);
#3483=(
BOUNDED_SURFACE()
B_SPLINE_SURFACE(1,2,((#153332,#153333,#153334,#153335,#153336,#153337,
#153338),(#153339,#153340,#153341,#153342,#153343,#153344,#153345)),
 .UNSPECIFIED.,.F.,.F.,.F.)
B_SPLINE_SURFACE_WITH_KNOTS((2,2),(3,2,2,3),(0.,0.289807040991565),(0.142404283483237,
0.142578551421299,0.142857142857143,0.16000534522748),.UNSPECIFIED.)
GEOMETRIC_REPRESENTATION_ITEM()
RATIONAL_B_SPLINE_SURFACE(((0.999805186472013,0.999805186472013,0.999805186472013,
0.999902211834772,1.,0.993980822699459,0.990851751371591),(0.999805186472013,
0.999805186472013,0.999805186472013,0.999902211834772,1.,0.993980822699459,
0.990851751371591)))
REPRESENTATION_ITEM('')
SURFACE()
);
#3484=(
BOUNDED_SURFACE()
B_SPLINE_SURFACE(1,2,((#153362,#153363,#153364,#153365,#153366),(#153367,
#153368,#153369,#153370,#153371)),.UNSPECIFIED.,.F.,.F.,.F.)
B_SPLINE_SURFACE_WITH_KNOTS((2,2),(3,2,3),(0.,0.289681084359925),(0.573550810617452,
0.590910950629595,0.591084552029716),.UNSPECIFIED.)
GEOMETRIC_REPRESENTATION_ITEM()
RATIONAL_B_SPLINE_SURFACE(((0.998554414400195,0.992822941359326,0.990053454406147,
0.990053454406147,0.990053454406147),(0.998554414400195,0.992822941359326,
0.990053454406147,0.990053454406147,0.990053454406147)))
REPRESENTATION_ITEM('')
SURFACE()
);
#3485=(
BOUNDED_SURFACE()
B_SPLINE_SURFACE(1,2,((#153373,#153374,#153375,#153376,#153377,#153378,
#153379),(#153380,#153381,#153382,#153383,#153384,#153385,#153386)),
 .UNSPECIFIED.,.F.,.F.,.F.)
B_SPLINE_SURFACE_WITH_KNOTS((2,2),(3,2,2,3),(0.,0.28980704099157),(0.142404283483249,
0.142578551421311,0.142857142857143,0.160005345227479),.UNSPECIFIED.)
GEOMETRIC_REPRESENTATION_ITEM()
RATIONAL_B_SPLINE_SURFACE(((0.999805186472022,0.999805186472022,0.999805186472022,
0.999902211834776,1.,0.993980822699459,0.990851751371591),(0.999805186472022,
0.999805186472022,0.999805186472022,0.999902211834776,1.,0.993980822699459,
0.990851751371591)))
REPRESENTATION_ITEM('')
SURFACE()
);
#3486=(
BOUNDED_SURFACE()
B_SPLINE_SURFACE(1,2,((#153403,#153404,#153405,#153406,#153407),(#153408,
#153409,#153410,#153411,#153412)),.UNSPECIFIED.,.F.,.F.,.F.)
B_SPLINE_SURFACE_WITH_KNOTS((2,2),(3,2,3),(0.,0.289681084359923),(0.573550810617452,
0.590910950629593,0.591084552029714),.UNSPECIFIED.)
GEOMETRIC_REPRESENTATION_ITEM()
RATIONAL_B_SPLINE_SURFACE(((0.998554414400195,0.992822941359326,0.990053454406148,
0.990053454406148,0.990053454406148),(0.998554414400195,0.992822941359326,
0.990053454406148,0.990053454406148,0.990053454406148)))
REPRESENTATION_ITEM('')
SURFACE()
);
#3487=(
BOUNDED_SURFACE()
B_SPLINE_SURFACE(1,2,((#153414,#153415,#153416,#153417,#153418,#153419,
#153420),(#153421,#153422,#153423,#153424,#153425,#153426,#153427)),
 .UNSPECIFIED.,.F.,.F.,.F.)
B_SPLINE_SURFACE_WITH_KNOTS((2,2),(3,2,2,3),(0.,0.289807040991713),(0.142404283483303,
0.142578551421364,0.142857142857143,0.160005345227479),.UNSPECIFIED.)
GEOMETRIC_REPRESENTATION_ITEM()
RATIONAL_B_SPLINE_SURFACE(((0.999805186472059,0.999805186472059,0.999805186472059,
0.999902211834795,1.,0.993980822699459,0.990851751371591),(0.999805186472059,
0.999805186472059,0.999805186472059,0.999902211834795,1.,0.993980822699459,
0.990851751371591)))
REPRESENTATION_ITEM('')
SURFACE()
);
#3488=(
BOUNDED_SURFACE()
B_SPLINE_SURFACE(1,2,((#153444,#153445,#153446,#153447,#153448),(#153449,
#153450,#153451,#153452,#153453)),.UNSPECIFIED.,.F.,.F.,.F.)
B_SPLINE_SURFACE_WITH_KNOTS((2,2),(3,2,3),(0.,0.289681084359918),(0.573550810617382,
0.590910950629593,0.591084552029715),.UNSPECIFIED.)
GEOMETRIC_REPRESENTATION_ITEM()
RATIONAL_B_SPLINE_SURFACE(((0.998554414400241,0.992822941359337,0.990053454406148,
0.990053454406148,0.990053454406148),(0.998554414400241,0.992822941359337,
0.990053454406148,0.990053454406148,0.990053454406148)))
REPRESENTATION_ITEM('')
SURFACE()
);
#3489=(
BOUNDED_SURFACE()
B_SPLINE_SURFACE(1,2,((#153455,#153456,#153457,#153458,#153459,#153460,
#153461),(#153462,#153463,#153464,#153465,#153466,#153467,#153468)),
 .UNSPECIFIED.,.F.,.F.,.F.)
B_SPLINE_SURFACE_WITH_KNOTS((2,2),(3,2,2,3),(0.,0.289807040993087),(0.142404283483302,
0.142578551421363,0.142857142857143,0.160005345227479),.UNSPECIFIED.)
GEOMETRIC_REPRESENTATION_ITEM()
RATIONAL_B_SPLINE_SURFACE(((0.999805186472059,0.999805186472059,0.999805186472059,
0.999902211834794,1.,0.993980822699459,0.990851751371591),(0.999805186472059,
0.999805186472059,0.999805186472059,0.999902211834794,1.,0.993980822699459,
0.990851751371591)))
REPRESENTATION_ITEM('')
SURFACE()
);
#3490=(
BOUNDED_SURFACE()
B_SPLINE_SURFACE(1,2,((#153485,#153486,#153487,#153488,#153489),(#153490,
#153491,#153492,#153493,#153494)),.UNSPECIFIED.,.F.,.F.,.F.)
B_SPLINE_SURFACE_WITH_KNOTS((2,2),(3,2,3),(0.,0.289681084360127),(0.573550810617425,
0.590910950629593,0.591084552029715),.UNSPECIFIED.)
GEOMETRIC_REPRESENTATION_ITEM()
RATIONAL_B_SPLINE_SURFACE(((0.998554414400213,0.99282294135933,0.990053454406148,
0.990053454406148,0.990053454406148),(0.998554414400213,0.99282294135933,
0.990053454406147,0.990053454406147,0.990053454406147)))
REPRESENTATION_ITEM('')
SURFACE()
);
#3491=(
BOUNDED_SURFACE()
B_SPLINE_SURFACE(1,2,((#153496,#153497,#153498,#153499,#153500,#153501,
#153502),(#153503,#153504,#153505,#153506,#153507,#153508,#153509)),
 .UNSPECIFIED.,.F.,.F.,.F.)
B_SPLINE_SURFACE_WITH_KNOTS((2,2),(3,2,2,3),(0.,0.289807040991616),(0.142404283483146,
0.142578551421209,0.142857142857143,0.16000534522748),.UNSPECIFIED.)
GEOMETRIC_REPRESENTATION_ITEM()
RATIONAL_B_SPLINE_SURFACE(((0.999805186471951,0.999805186471951,0.999805186471951,
0.99990221183474,1.,0.993980822699459,0.990851751371591),(0.999805186471951,
0.999805186471951,0.999805186471951,0.99990221183474,1.,0.993980822699459,
0.990851751371591)))
REPRESENTATION_ITEM('')
SURFACE()
);
#3492=(
BOUNDED_SURFACE()
B_SPLINE_SURFACE(1,2,((#153526,#153527,#153528,#153529,#153530),(#153531,
#153532,#153533,#153534,#153535)),.UNSPECIFIED.,.F.,.F.,.F.)
B_SPLINE_SURFACE_WITH_KNOTS((2,2),(3,2,3),(0.,0.289681084359932),(0.573550810617452,
0.590910950629593,0.591084552029714),.UNSPECIFIED.)
GEOMETRIC_REPRESENTATION_ITEM()
RATIONAL_B_SPLINE_SURFACE(((0.998554414400195,0.992822941359326,0.990053454406148,
0.990053454406148,0.990053454406148),(0.998554414400195,0.992822941359326,
0.990053454406148,0.990053454406148,0.990053454406148)))
REPRESENTATION_ITEM('')
SURFACE()
);
#3493=(
BOUNDED_SURFACE()
B_SPLINE_SURFACE(1,2,((#153537,#153538,#153539,#153540,#153541,#153542,
#153543),(#153544,#153545,#153546,#153547,#153548,#153549,#153550)),
 .UNSPECIFIED.,.F.,.F.,.F.)
B_SPLINE_SURFACE_WITH_KNOTS((2,2),(3,2,2,3),(0.,0.289807040991645),(0.142404283483298,
0.142578551421359,0.142857142857143,0.160005345227479),.UNSPECIFIED.)
GEOMETRIC_REPRESENTATION_ITEM()
RATIONAL_B_SPLINE_SURFACE(((0.999805186472056,0.999805186472056,0.999805186472056,
0.999902211834793,1.,0.993980822699459,0.990851751371591),(0.999805186472056,
0.999805186472056,0.999805186472056,0.999902211834793,1.,0.993980822699459,
0.990851751371591)))
REPRESENTATION_ITEM('')
SURFACE()
);
#3494=(
BOUNDED_SURFACE()
B_SPLINE_SURFACE(1,2,((#153567,#153568,#153569,#153570,#153571),(#153572,
#153573,#153574,#153575,#153576)),.UNSPECIFIED.,.F.,.F.,.F.)
B_SPLINE_SURFACE_WITH_KNOTS((2,2),(3,2,3),(0.,0.289681084359924),(0.573550810617452,
0.590910950629593,0.591084552029714),.UNSPECIFIED.)
GEOMETRIC_REPRESENTATION_ITEM()
RATIONAL_B_SPLINE_SURFACE(((0.998554414400195,0.992822941359326,0.990053454406148,
0.990053454406148,0.990053454406148),(0.998554414400195,0.992822941359326,
0.990053454406147,0.990053454406147,0.990053454406147)))
REPRESENTATION_ITEM('')
SURFACE()
);
#3495=(
BOUNDED_SURFACE()
B_SPLINE_SURFACE(1,2,((#153578,#153579,#153580,#153581,#153582,#153583,
#153584),(#153585,#153586,#153587,#153588,#153589,#153590,#153591)),
 .UNSPECIFIED.,.F.,.F.,.F.)
B_SPLINE_SURFACE_WITH_KNOTS((2,2),(3,2,2,3),(0.,0.289807040991634),(0.142404283483303,
0.142578551421364,0.142857142857143,0.160005345227479),.UNSPECIFIED.)
GEOMETRIC_REPRESENTATION_ITEM()
RATIONAL_B_SPLINE_SURFACE(((0.999805186472059,0.999805186472059,0.999805186472059,
0.999902211834795,1.,0.993980822699459,0.990851751371591),(0.999805186472059,
0.999805186472059,0.999805186472059,0.999902211834795,1.,0.993980822699459,
0.990851751371591)))
REPRESENTATION_ITEM('')
SURFACE()
);
#3496=(
BOUNDED_SURFACE()
B_SPLINE_SURFACE(1,2,((#153608,#153609,#153610,#153611,#153612),(#153613,
#153614,#153615,#153616,#153617)),.UNSPECIFIED.,.F.,.F.,.F.)
B_SPLINE_SURFACE_WITH_KNOTS((2,2),(3,2,3),(0.,0.289681084359921),(0.573550810617452,
0.590910950629593,0.591084552029714),.UNSPECIFIED.)
GEOMETRIC_REPRESENTATION_ITEM()
RATIONAL_B_SPLINE_SURFACE(((0.998554414400195,0.992822941359326,0.990053454406147,
0.990053454406147,0.990053454406147),(0.998554414400195,0.992822941359326,
0.990053454406147,0.990053454406147,0.990053454406147)))
REPRESENTATION_ITEM('')
SURFACE()
);
#3497=(
BOUNDED_SURFACE()
B_SPLINE_SURFACE(1,2,((#153619,#153620,#153621,#153622,#153623,#153624,
#153625),(#153626,#153627,#153628,#153629,#153630,#153631,#153632)),
 .UNSPECIFIED.,.F.,.F.,.F.)
B_SPLINE_SURFACE_WITH_KNOTS((2,2),(3,2,2,3),(0.,0.289807040991559),(0.142404283483175,
0.142578551421237,0.142857142857143,0.16000534522748),.UNSPECIFIED.)
GEOMETRIC_REPRESENTATION_ITEM()
RATIONAL_B_SPLINE_SURFACE(((0.999805186471971,0.999805186471971,0.999805186471971,
0.99990221183475,1.,0.993980822699459,0.990851751371591),(0.999805186471971,
0.999805186471971,0.999805186471971,0.99990221183475,1.,0.993980822699459,
0.990851751371591)))
REPRESENTATION_ITEM('')
SURFACE()
);
#3498=(
BOUNDED_SURFACE()
B_SPLINE_SURFACE(1,2,((#153649,#153650,#153651,#153652,#153653),(#153654,
#153655,#153656,#153657,#153658)),.UNSPECIFIED.,.F.,.F.,.F.)
B_SPLINE_SURFACE_WITH_KNOTS((2,2),(3,2,3),(0.,0.289681084359924),(0.5735508106174,
0.590910950629593,0.591084552029715),.UNSPECIFIED.)
GEOMETRIC_REPRESENTATION_ITEM()
RATIONAL_B_SPLINE_SURFACE(((0.998554414400229,0.992822941359334,0.990053454406148,
0.990053454406148,0.990053454406148),(0.998554414400229,0.992822941359334,
0.990053454406148,0.990053454406148,0.990053454406148)))
REPRESENTATION_ITEM('')
SURFACE()
);
#3499=(
BOUNDED_SURFACE()
B_SPLINE_SURFACE(1,2,((#153666,#153667,#153668,#153669,#153670,#153671,
#153672),(#153673,#153674,#153675,#153676,#153677,#153678,#153679)),
 .UNSPECIFIED.,.F.,.F.,.F.)
B_SPLINE_SURFACE_WITH_KNOTS((2,2),(3,2,2,3),(0.,0.289807040991565),(0.142404283483079,
0.142578551421142,0.142857142857143,0.160005345227427),.UNSPECIFIED.)
GEOMETRIC_REPRESENTATION_ITEM()
RATIONAL_B_SPLINE_SURFACE(((0.999805186471905,0.999805186471905,0.999805186471905,
0.999902211834717,1.,0.993980822699477,0.99085175137161),(0.999805186471905,
0.999805186471905,0.999805186471905,0.999902211834717,1.,0.993980822699477,
0.99085175137161)))
REPRESENTATION_ITEM('')
SURFACE()
);
#3500=(
BOUNDED_SURFACE()
B_SPLINE_SURFACE(1,2,((#153681,#153682,#153683),(#153684,#153685,#153686),
(#153687,#153688,#153689)),.UNSPECIFIED.,.F.,.F.,.F.)
B_SPLINE_SURFACE_WITH_KNOTS((2,1,2),(3,3),(0.688417832139402,0.710192959008107,
1.),(0.0909109506295426,0.108084585199971),.UNSPECIFIED.)
GEOMETRIC_REPRESENTATION_ITEM()
RATIONAL_B_SPLINE_SURFACE(((0.990053454406164,0.987313720921967,0.987472672298934),
(0.990053454406164,0.987313720921967,0.987472672298934),(0.990053454406164,
0.987313720921967,0.987472672298934)))
REPRESENTATION_ITEM('')
SURFACE()
);
#3501=(
BOUNDED_SURFACE()
B_SPLINE_SURFACE(1,2,((#153705,#153706,#153707),(#153708,#153709,#153710),
(#153711,#153712,#153713)),.UNSPECIFIED.,.F.,.F.,.F.)
B_SPLINE_SURFACE_WITH_KNOTS((2,1,2),(3,3),(0.688516410643263,0.71031891563962,
1.),(0.625066077454535,0.642578551421363),.UNSPECIFIED.)
GEOMETRIC_REPRESENTATION_ITEM()
RATIONAL_B_SPLINE_SURFACE(((0.990621203777021,0.993706096834649,0.999805186472059),
(0.990621203777021,0.993706096834649,0.999805186472059),(0.990621203777021,
0.993706096834649,0.999805186472059)))
REPRESENTATION_ITEM('')
SURFACE()
);
#3502=(
BOUNDED_SURFACE()
B_SPLINE_SURFACE(1,2,((#153754,#153755,#153756),(#153757,#153758,#153759),
(#153760,#153761,#153762)),.UNSPECIFIED.,.F.,.F.,.F.)
B_SPLINE_SURFACE_WITH_KNOTS((2,1,2),(3,3),(0.688417834114171,0.710192959007975,
1.),(0.0909109506295457,0.108084585199971),.UNSPECIFIED.)
GEOMETRIC_REPRESENTATION_ITEM()
RATIONAL_B_SPLINE_SURFACE(((0.990053454406163,0.987313720921967,0.987472672298934),
(0.990053454406163,0.987313720921967,0.987472672298934),(0.990053454406163,
0.987313720921967,0.987472672298934)))
REPRESENTATION_ITEM('')
SURFACE()
);
#3503=(
BOUNDED_SURFACE()
B_SPLINE_SURFACE(1,2,((#153764,#153765,#153766),(#153767,#153768,#153769),
(#153770,#153771,#153772)),.UNSPECIFIED.,.F.,.F.,.F.)
B_SPLINE_SURFACE_WITH_KNOTS((2,1,2),(3,3),(0.688516410654661,0.710318915639632,
1.),(0.625066077454535,0.642578551421363),.UNSPECIFIED.)
GEOMETRIC_REPRESENTATION_ITEM()
RATIONAL_B_SPLINE_SURFACE(((0.990621203777021,0.993706096834649,0.999805186472059),
(0.990621203777021,0.993706096834649,0.999805186472059),(0.990621203777021,
0.993706096834649,0.999805186472059)))
REPRESENTATION_ITEM('')
SURFACE()
);
#3504=(
BOUNDED_SURFACE()
B_SPLINE_SURFACE(1,2,((#153813,#153814,#153815),(#153816,#153817,#153818),
(#153819,#153820,#153821)),.UNSPECIFIED.,.F.,.F.,.F.)
B_SPLINE_SURFACE_WITH_KNOTS((2,1,2),(3,3),(0.688417833968987,0.710192959007994,
1.),(0.0909109506295942,0.10808458519997),.UNSPECIFIED.)
GEOMETRIC_REPRESENTATION_ITEM()
RATIONAL_B_SPLINE_SURFACE(((0.990053454406147,0.987313720921968,0.987472672298934),
(0.990053454406147,0.987313720921968,0.987472672298934),(0.990053454406147,
0.987313720921968,0.987472672298934)))
REPRESENTATION_ITEM('')
SURFACE()
);
#3505=(
BOUNDED_SURFACE()
B_SPLINE_SURFACE(1,2,((#153823,#153824,#153825),(#153826,#153827,#153828),
(#153829,#153830,#153831)),.UNSPECIFIED.,.F.,.F.,.F.)
B_SPLINE_SURFACE_WITH_KNOTS((2,1,2),(3,3),(0.688516410790942,0.71031891563998,
1.),(0.625066077454535,0.642578551421363),.UNSPECIFIED.)
GEOMETRIC_REPRESENTATION_ITEM()
RATIONAL_B_SPLINE_SURFACE(((0.990621203777021,0.993706096834649,0.999805186472059),
(0.990621203777021,0.993706096834649,0.999805186472059),(0.990621203777021,
0.993706096834649,0.999805186472059)))
REPRESENTATION_ITEM('')
SURFACE()
);
#3506=(
BOUNDED_SURFACE()
B_SPLINE_SURFACE(1,2,((#153872,#153873,#153874),(#153875,#153876,#153877),
(#153878,#153879,#153880)),.UNSPECIFIED.,.F.,.F.,.F.)
B_SPLINE_SURFACE_WITH_KNOTS((2,1,2),(3,3),(0.68841783381541,0.710192959008345,
1.),(0.090910950629593,0.10808458519997),.UNSPECIFIED.)
GEOMETRIC_REPRESENTATION_ITEM()
RATIONAL_B_SPLINE_SURFACE(((0.990053454406147,0.987313720921968,0.987472672298934),
(0.990053454406147,0.987313720921968,0.987472672298934),(0.990053454406147,
0.987313720921968,0.987472672298934)))
REPRESENTATION_ITEM('')
SURFACE()
);
#3507=(
BOUNDED_SURFACE()
B_SPLINE_SURFACE(1,2,((#153882,#153883,#153884),(#153885,#153886,#153887),
(#153888,#153889,#153890)),.UNSPECIFIED.,.F.,.F.,.F.)
B_SPLINE_SURFACE_WITH_KNOTS((2,1,2),(3,3),(0.688516410355011,0.710318915639971,
1.),(0.625066077454535,0.642578551421363),.UNSPECIFIED.)
GEOMETRIC_REPRESENTATION_ITEM()
RATIONAL_B_SPLINE_SURFACE(((0.990621203777021,0.993706096834649,0.999805186472059),
(0.990621203777021,0.993706096834649,0.999805186472059),(0.990621203777021,
0.993706096834649,0.999805186472059)))
REPRESENTATION_ITEM('')
SURFACE()
);
#3508=(
BOUNDED_SURFACE()
B_SPLINE_SURFACE(1,2,((#153931,#153932,#153933),(#153934,#153935,#153936),
(#153937,#153938,#153939)),.UNSPECIFIED.,.F.,.F.,.F.)
B_SPLINE_SURFACE_WITH_KNOTS((2,1,2),(3,3),(0.688417834222182,0.710192959008331,
1.),(0.0909109506295941,0.10808458519997),.UNSPECIFIED.)
GEOMETRIC_REPRESENTATION_ITEM()
RATIONAL_B_SPLINE_SURFACE(((0.990053454406147,0.987313720921968,0.987472672298934),
(0.990053454406147,0.987313720921968,0.987472672298934),(0.990053454406147,
0.987313720921968,0.987472672298934)))
REPRESENTATION_ITEM('')
SURFACE()
);
#3509=(
BOUNDED_SURFACE()
B_SPLINE_SURFACE(1,2,((#153941,#153942,#153943),(#153944,#153945,#153946),
(#153947,#153948,#153949)),.UNSPECIFIED.,.F.,.F.,.F.)
B_SPLINE_SURFACE_WITH_KNOTS((2,1,2),(3,3),(0.688516410538964,0.710318915639015,
1.),(0.625066077454535,0.642578551421363),.UNSPECIFIED.)
GEOMETRIC_REPRESENTATION_ITEM()
RATIONAL_B_SPLINE_SURFACE(((0.990621203777021,0.993706096834649,0.999805186472059),
(0.990621203777021,0.993706096834649,0.999805186472059),(0.990621203777021,
0.993706096834649,0.999805186472059)))
REPRESENTATION_ITEM('')
SURFACE()
);
#3510=(
BOUNDED_SURFACE()
B_SPLINE_SURFACE(1,2,((#153990,#153991,#153992),(#153993,#153994,#153995),
(#153996,#153997,#153998)),.UNSPECIFIED.,.F.,.F.,.F.)
B_SPLINE_SURFACE_WITH_KNOTS((2,1,2),(3,3),(0.688417834370893,0.710192959007374,
1.),(0.0909109506295929,0.10808458519997),.UNSPECIFIED.)
GEOMETRIC_REPRESENTATION_ITEM()
RATIONAL_B_SPLINE_SURFACE(((0.990053454406148,0.987313720921968,0.987472672298934),
(0.990053454406148,0.987313720921968,0.987472672298934),(0.990053454406148,
0.987313720921968,0.987472672298934)))
REPRESENTATION_ITEM('')
SURFACE()
);
#3511=(
BOUNDED_SURFACE()
B_SPLINE_SURFACE(1,2,((#154000,#154001,#154002),(#154003,#154004,#154005),
(#154006,#154007,#154008)),.UNSPECIFIED.,.F.,.F.,.F.)
B_SPLINE_SURFACE_WITH_KNOTS((2,1,2),(3,3),(0.688516410279689,0.710318915639017,
1.),(0.625066077454535,0.642578551421363),.UNSPECIFIED.)
GEOMETRIC_REPRESENTATION_ITEM()
RATIONAL_B_SPLINE_SURFACE(((0.990621203777021,0.993706096834649,0.999805186472059),
(0.990621203777021,0.993706096834649,0.999805186472059),(0.990621203777021,
0.993706096834649,0.999805186472059)))
REPRESENTATION_ITEM('')
SURFACE()
);
#3512=(
BOUNDED_SURFACE()
B_SPLINE_SURFACE(1,2,((#154049,#154050,#154051),(#154052,#154053,#154054),
(#154055,#154056,#154057)),.UNSPECIFIED.,.F.,.F.,.F.)
B_SPLINE_SURFACE_WITH_KNOTS((2,1,2),(3,3),(0.688417834245439,0.710192959007374,
1.),(0.0909109506295555,0.108084585199971),.UNSPECIFIED.)
GEOMETRIC_REPRESENTATION_ITEM()
RATIONAL_B_SPLINE_SURFACE(((0.99005345440616,0.987313720921967,0.987472672298934),
(0.99005345440616,0.987313720921967,0.987472672298934),(0.99005345440616,
0.987313720921967,0.987472672298934)))
REPRESENTATION_ITEM('')
SURFACE()
);
#3513=(
BOUNDED_SURFACE()
B_SPLINE_SURFACE(1,2,((#154059,#154060,#154061),(#154062,#154063,#154064),
(#154065,#154066,#154067)),.UNSPECIFIED.,.F.,.F.,.F.)
B_SPLINE_SURFACE_WITH_KNOTS((2,1,2),(3,3),(0.688516410179556,0.710318915639016,
1.),(0.625066077454535,0.642578551421363),.UNSPECIFIED.)
GEOMETRIC_REPRESENTATION_ITEM()
RATIONAL_B_SPLINE_SURFACE(((0.990621203777021,0.993706096834649,0.999805186472059),
(0.990621203777021,0.993706096834649,0.999805186472059),(0.990621203777021,
0.993706096834649,0.999805186472059)))
REPRESENTATION_ITEM('')
SURFACE()
);
#3514=(
BOUNDED_SURFACE()
B_SPLINE_SURFACE(1,2,((#154108,#154109,#154110),(#154111,#154112,#154113),
(#154114,#154115,#154116)),.UNSPECIFIED.,.F.,.F.,.F.)
B_SPLINE_SURFACE_WITH_KNOTS((2,1,2),(3,3),(0.688417833993896,0.710192959007378,
1.),(0.0909109506295549,0.108084585199971),.UNSPECIFIED.)
GEOMETRIC_REPRESENTATION_ITEM()
RATIONAL_B_SPLINE_SURFACE(((0.99005345440616,0.987313720921967,0.987472672298934),
(0.99005345440616,0.987313720921967,0.987472672298934),(0.99005345440616,
0.987313720921967,0.987472672298934)))
REPRESENTATION_ITEM('')
SURFACE()
);
#3515=(
BOUNDED_SURFACE()
B_SPLINE_SURFACE(1,2,((#154118,#154119,#154120),(#154121,#154122,#154123),
(#154124,#154125,#154126)),.UNSPECIFIED.,.F.,.F.,.F.)
B_SPLINE_SURFACE_WITH_KNOTS((2,1,2),(3,3),(0.68851641069385,0.710318915638436,
1.),(0.625066077454535,0.642578551421363),.UNSPECIFIED.)
GEOMETRIC_REPRESENTATION_ITEM()
RATIONAL_B_SPLINE_SURFACE(((0.990621203777021,0.993706096834649,0.999805186472059),
(0.990621203777021,0.993706096834649,0.999805186472059),(0.990621203777021,
0.993706096834649,0.999805186472059)))
REPRESENTATION_ITEM('')
SURFACE()
);
#3516=(
BOUNDED_SURFACE()
B_SPLINE_SURFACE(1,2,((#154167,#154168,#154169),(#154170,#154171,#154172),
(#154173,#154174,#154175)),.UNSPECIFIED.,.F.,.F.,.F.)
B_SPLINE_SURFACE_WITH_KNOTS((2,1,2),(3,3),(0.688417834521045,0.710192959006796,
1.),(0.0909109506295929,0.10808458519997),.UNSPECIFIED.)
GEOMETRIC_REPRESENTATION_ITEM()
RATIONAL_B_SPLINE_SURFACE(((0.990053454406148,0.987313720921968,0.987472672298934),
(0.990053454406148,0.987313720921968,0.987472672298934),(0.990053454406148,
0.987313720921968,0.987472672298934)))
REPRESENTATION_ITEM('')
SURFACE()
);
#3517=(
BOUNDED_SURFACE()
B_SPLINE_SURFACE(1,2,((#154177,#154178,#154179),(#154180,#154181,#154182),
(#154183,#154184,#154185)),.UNSPECIFIED.,.F.,.F.,.F.)
B_SPLINE_SURFACE_WITH_KNOTS((2,1,2),(3,3),(0.688516410378158,0.71031891563903,
1.),(0.625066077454535,0.642578551421363),.UNSPECIFIED.)
GEOMETRIC_REPRESENTATION_ITEM()
RATIONAL_B_SPLINE_SURFACE(((0.990621203777021,0.993706096834649,0.999805186472059),
(0.990621203777021,0.993706096834649,0.999805186472059),(0.990621203777021,
0.993706096834649,0.999805186472059)))
REPRESENTATION_ITEM('')
SURFACE()
);
#3518=(
BOUNDED_SURFACE()
B_SPLINE_SURFACE(1,2,((#154226,#154227,#154228),(#154229,#154230,#154231),
(#154232,#154233,#154234)),.UNSPECIFIED.,.F.,.F.,.F.)
B_SPLINE_SURFACE_WITH_KNOTS((2,1,2),(3,3),(0.688417834350685,0.710192959007387,
1.),(0.090910950629593,0.10808458519997),.UNSPECIFIED.)
GEOMETRIC_REPRESENTATION_ITEM()
RATIONAL_B_SPLINE_SURFACE(((0.990053454406148,0.987313720921968,0.987472672298934),
(0.990053454406148,0.987313720921968,0.987472672298934),(0.990053454406148,
0.987313720921968,0.987472672298934)))
REPRESENTATION_ITEM('')
SURFACE()
);
#3519=(
BOUNDED_SURFACE()
B_SPLINE_SURFACE(1,2,((#154236,#154237,#154238),(#154239,#154240,#154241),
(#154242,#154243,#154244)),.UNSPECIFIED.,.F.,.F.,.F.)
B_SPLINE_SURFACE_WITH_KNOTS((2,1,2),(3,3),(0.688516410525766,0.710318915638467,
1.),(0.625066077454535,0.642578551421363),.UNSPECIFIED.)
GEOMETRIC_REPRESENTATION_ITEM()
RATIONAL_B_SPLINE_SURFACE(((0.990621203777021,0.993706096834649,0.999805186472058),
(0.990621203777021,0.993706096834649,0.999805186472058),(0.990621203777021,
0.993706096834649,0.999805186472058)))
REPRESENTATION_ITEM('')
SURFACE()
);
#3520=(
BOUNDED_SURFACE()
B_SPLINE_SURFACE(1,2,((#154285,#154286,#154287),(#154288,#154289,#154290),
(#154291,#154292,#154293)),.UNSPECIFIED.,.F.,.F.,.F.)
B_SPLINE_SURFACE_WITH_KNOTS((2,1,2),(3,3),(0.688417834091111,0.710192959006829,
1.),(0.0909109506295647,0.108084585199971),.UNSPECIFIED.)
GEOMETRIC_REPRESENTATION_ITEM()
RATIONAL_B_SPLINE_SURFACE(((0.990053454406157,0.987313720921967,0.987472672298934),
(0.990053454406157,0.987313720921967,0.987472672298934),(0.990053454406157,
0.987313720921967,0.987472672298934)))
REPRESENTATION_ITEM('')
SURFACE()
);
#3521=(
BOUNDED_SURFACE()
B_SPLINE_SURFACE(1,2,((#154295,#154296,#154297),(#154298,#154299,#154300),
(#154301,#154302,#154303)),.UNSPECIFIED.,.F.,.F.,.F.)
B_SPLINE_SURFACE_WITH_KNOTS((2,1,2),(3,3),(0.688516410404015,0.710318915638657,
1.),(0.625066077454536,0.642578551421363),.UNSPECIFIED.)
GEOMETRIC_REPRESENTATION_ITEM()
RATIONAL_B_SPLINE_SURFACE(((0.990621203777022,0.993706096834649,0.999805186472059),
(0.990621203777022,0.993706096834649,0.999805186472059),(0.990621203777022,
0.993706096834649,0.999805186472059)))
REPRESENTATION_ITEM('')
SURFACE()
);
#3522=(
BOUNDED_SURFACE()
B_SPLINE_SURFACE(1,2,((#154344,#154345,#154346),(#154347,#154348,#154349),
(#154350,#154351,#154352)),.UNSPECIFIED.,.F.,.F.,.F.)
B_SPLINE_SURFACE_WITH_KNOTS((2,1,2),(3,3),(0.688417834498563,0.710192959007008,
1.),(0.090910950629561,0.10808458519997),.UNSPECIFIED.)
GEOMETRIC_REPRESENTATION_ITEM()
RATIONAL_B_SPLINE_SURFACE(((0.990053454406158,0.987313720921967,0.987472672298934),
(0.990053454406158,0.987313720921967,0.987472672298934),(0.990053454406158,
0.987313720921967,0.987472672298934)))
REPRESENTATION_ITEM('')
SURFACE()
);
#3523=(
BOUNDED_SURFACE()
B_SPLINE_SURFACE(1,2,((#154354,#154355,#154356),(#154357,#154358,#154359),
(#154360,#154361,#154362)),.UNSPECIFIED.,.F.,.F.,.F.)
B_SPLINE_SURFACE_WITH_KNOTS((2,1,2),(3,3),(0.688516410316575,0.710318915638622,
1.),(0.625066077454536,0.642578551421364),.UNSPECIFIED.)
GEOMETRIC_REPRESENTATION_ITEM()
RATIONAL_B_SPLINE_SURFACE(((0.990621203777022,0.993706096834649,0.999805186472059),
(0.990621203777022,0.993706096834649,0.999805186472059),(0.990621203777022,
0.993706096834649,0.999805186472059)))
REPRESENTATION_ITEM('')
SURFACE()
);
#3524=(
BOUNDED_SURFACE()
B_SPLINE_SURFACE(1,2,((#154403,#154404,#154405),(#154406,#154407,#154408),
(#154409,#154410,#154411)),.UNSPECIFIED.,.F.,.F.,.F.)
B_SPLINE_SURFACE_WITH_KNOTS((2,1,2),(3,3),(0.688417834508433,0.710192959006985,
1.),(0.0909109506295931,0.108084585199969),.UNSPECIFIED.)
GEOMETRIC_REPRESENTATION_ITEM()
RATIONAL_B_SPLINE_SURFACE(((0.990053454406148,0.987313720921968,0.987472672298934),
(0.990053454406148,0.987313720921968,0.987472672298934),(0.990053454406148,
0.987313720921968,0.987472672298934)))
REPRESENTATION_ITEM('')
SURFACE()
);
#3525=(
BOUNDED_SURFACE()
B_SPLINE_SURFACE(1,2,((#154413,#154414,#154415),(#154416,#154417,#154418),
(#154419,#154420,#154421)),.UNSPECIFIED.,.F.,.F.,.F.)
B_SPLINE_SURFACE_WITH_KNOTS((2,1,2),(3,3),(0.688516410725903,0.710318915638348,
1.),(0.625066077454536,0.642578551421364),.UNSPECIFIED.)
GEOMETRIC_REPRESENTATION_ITEM()
RATIONAL_B_SPLINE_SURFACE(((0.990621203777022,0.993706096834649,0.999805186472059),
(0.990621203777022,0.993706096834649,0.999805186472059),(0.990621203777022,
0.993706096834649,0.999805186472059)))
REPRESENTATION_ITEM('')
SURFACE()
);
#3526=(
BOUNDED_SURFACE()
B_SPLINE_SURFACE(1,2,((#154462,#154463,#154464),(#154465,#154466,#154467),
(#154468,#154469,#154470)),.UNSPECIFIED.,.F.,.F.,.F.)
B_SPLINE_SURFACE_WITH_KNOTS((2,1,2),(3,3),(0.688417834372287,0.710192959006701,
1.),(0.0909109506295633,0.108084585199969),.UNSPECIFIED.)
GEOMETRIC_REPRESENTATION_ITEM()
RATIONAL_B_SPLINE_SURFACE(((0.990053454406157,0.987313720921968,0.987472672298934),
(0.990053454406157,0.987313720921968,0.987472672298934),(0.990053454406157,
0.987313720921968,0.987472672298934)))
REPRESENTATION_ITEM('')
SURFACE()
);
#3527=(
BOUNDED_SURFACE()
B_SPLINE_SURFACE(1,2,((#154472,#154473,#154474),(#154475,#154476,#154477),
(#154478,#154479,#154480)),.UNSPECIFIED.,.F.,.F.,.F.)
B_SPLINE_SURFACE_WITH_KNOTS((2,1,2),(3,3),(0.688516410487827,0.710318915638921,
1.),(0.625066077454536,0.642578551421365),.UNSPECIFIED.)
GEOMETRIC_REPRESENTATION_ITEM()
RATIONAL_B_SPLINE_SURFACE(((0.990621203777022,0.993706096834649,0.999805186472059),
(0.990621203777022,0.993706096834649,0.999805186472059),(0.990621203777022,
0.993706096834649,0.999805186472059)))
REPRESENTATION_ITEM('')
SURFACE()
);
#3528=(
BOUNDED_SURFACE()
B_SPLINE_SURFACE(1,2,((#154488,#154489,#154490),(#154491,#154492,#154493),
(#154494,#154495,#154496)),.UNSPECIFIED.,.F.,.F.,.F.)
B_SPLINE_SURFACE_WITH_KNOTS((2,1,2),(3,3),(0.688417834510296,0.710192959007285,
1.),(0.0909109506295919,0.108084585199969),.UNSPECIFIED.)
GEOMETRIC_REPRESENTATION_ITEM()
RATIONAL_B_SPLINE_SURFACE(((0.990053454406148,0.987313720921968,0.987472672298934),
(0.990053454406148,0.987313720921968,0.987472672298934),(0.990053454406148,
0.987313720921968,0.987472672298934)))
REPRESENTATION_ITEM('')
SURFACE()
);
#3529=(
BOUNDED_SURFACE()
B_SPLINE_SURFACE(1,2,((#154498,#154499,#154500),(#154501,#154502,#154503),
(#154504,#154505,#154506)),.UNSPECIFIED.,.F.,.F.,.F.)
B_SPLINE_SURFACE_WITH_KNOTS((2,1,2),(3,3),(0.68851641049287,0.710318915638097,
1.),(0.625066077454536,0.642578551421364),.UNSPECIFIED.)
GEOMETRIC_REPRESENTATION_ITEM()
RATIONAL_B_SPLINE_SURFACE(((0.990621203777022,0.993706096834649,0.999805186472059),
(0.990621203777022,0.993706096834649,0.999805186472059),(0.990621203777022,
0.993706096834649,0.999805186472059)))
REPRESENTATION_ITEM('')
SURFACE()
);
#3530=(
BOUNDED_SURFACE()
B_SPLINE_SURFACE(1,2,((#154547,#154548,#154549),(#154550,#154551,#154552),
(#154553,#154554,#154555)),.UNSPECIFIED.,.F.,.F.,.F.)
B_SPLINE_SURFACE_WITH_KNOTS((2,1,2),(3,3),(0.688417834553386,0.710192959006459,
1.),(0.0909109506295633,0.10808458519997),.UNSPECIFIED.)
GEOMETRIC_REPRESENTATION_ITEM()
RATIONAL_B_SPLINE_SURFACE(((0.990053454406157,0.987313720921968,0.987472672298934),
(0.990053454406157,0.987313720921968,0.987472672298934),(0.990053454406157,
0.987313720921968,0.987472672298934)))
REPRESENTATION_ITEM('')
SURFACE()
);
#3531=(
BOUNDED_SURFACE()
B_SPLINE_SURFACE(1,2,((#154557,#154558,#154559),(#154560,#154561,#154562),
(#154563,#154564,#154565)),.UNSPECIFIED.,.F.,.F.,.F.)
B_SPLINE_SURFACE_WITH_KNOTS((2,1,2),(3,3),(0.688516410521495,0.710318915638601,
1.),(0.625066077454536,0.642578551421364),.UNSPECIFIED.)
GEOMETRIC_REPRESENTATION_ITEM()
RATIONAL_B_SPLINE_SURFACE(((0.990621203777022,0.993706096834649,0.999805186472059),
(0.990621203777022,0.993706096834649,0.999805186472059),(0.990621203777022,
0.993706096834649,0.999805186472059)))
REPRESENTATION_ITEM('')
SURFACE()
);
#3532=(
BOUNDED_SURFACE()
B_SPLINE_SURFACE(1,2,((#154606,#154607,#154608),(#154609,#154610,#154611),
(#154612,#154613,#154614)),.UNSPECIFIED.,.F.,.F.,.F.)
B_SPLINE_SURFACE_WITH_KNOTS((2,1,2),(3,3),(0.688417834311866,0.710192959006958,
1.),(0.0909109506295619,0.108084585199969),.UNSPECIFIED.)
GEOMETRIC_REPRESENTATION_ITEM()
RATIONAL_B_SPLINE_SURFACE(((0.990053454406157,0.987313720921967,0.987472672298933),
(0.990053454406157,0.987313720921967,0.987472672298933),(0.990053454406157,
0.987313720921967,0.987472672298933)))
REPRESENTATION_ITEM('')
SURFACE()
);
#3533=(
BOUNDED_SURFACE()
B_SPLINE_SURFACE(1,2,((#154616,#154617,#154618),(#154619,#154620,#154621),
(#154622,#154623,#154624)),.UNSPECIFIED.,.F.,.F.,.F.)
B_SPLINE_SURFACE_WITH_KNOTS((2,1,2),(3,3),(0.688516410815659,0.710318915638127,
1.),(0.625066077454536,0.642578551421364),.UNSPECIFIED.)
GEOMETRIC_REPRESENTATION_ITEM()
RATIONAL_B_SPLINE_SURFACE(((0.990621203777022,0.993706096834649,0.999805186472059),
(0.990621203777022,0.993706096834649,0.999805186472059),(0.990621203777022,
0.993706096834649,0.999805186472059)))
REPRESENTATION_ITEM('')
SURFACE()
);
#3534=(
BOUNDED_SURFACE()
B_SPLINE_SURFACE(1,2,((#154665,#154666,#154667),(#154668,#154669,#154670),
(#154671,#154672,#154673)),.UNSPECIFIED.,.F.,.F.,.F.)
B_SPLINE_SURFACE_WITH_KNOTS((2,1,2),(3,3),(0.688417834306651,0.71019295900648,
1.),(0.0909109506295634,0.108084585199969),.UNSPECIFIED.)
GEOMETRIC_REPRESENTATION_ITEM()
RATIONAL_B_SPLINE_SURFACE(((0.990053454406157,0.987313720921968,0.987472672298934),
(0.990053454406157,0.987313720921968,0.987472672298934),(0.990053454406157,
0.987313720921968,0.987472672298934)))
REPRESENTATION_ITEM('')
SURFACE()
);
#3535=(
BOUNDED_SURFACE()
B_SPLINE_SURFACE(1,2,((#154675,#154676,#154677),(#154678,#154679,#154680),
(#154681,#154682,#154683)),.UNSPECIFIED.,.F.,.F.,.F.)
B_SPLINE_SURFACE_WITH_KNOTS((2,1,2),(3,3),(0.688516410441904,0.710318915638384,
1.),(0.625066077454536,0.642578551421365),.UNSPECIFIED.)
GEOMETRIC_REPRESENTATION_ITEM()
RATIONAL_B_SPLINE_SURFACE(((0.990621203777022,0.993706096834649,0.999805186472059),
(0.990621203777022,0.993706096834649,0.999805186472059),(0.990621203777022,
0.993706096834649,0.999805186472059)))
REPRESENTATION_ITEM('')
SURFACE()
);
#3536=(
BOUNDED_SURFACE()
B_SPLINE_SURFACE(1,2,((#154724,#154725,#154726),(#154727,#154728,#154729),
(#154730,#154731,#154732)),.UNSPECIFIED.,.F.,.F.,.F.)
B_SPLINE_SURFACE_WITH_KNOTS((2,1,2),(3,3),(0.688417834456928,0.710192959006737,
1.),(0.0909109506295919,0.108084585199969),.UNSPECIFIED.)
GEOMETRIC_REPRESENTATION_ITEM()
RATIONAL_B_SPLINE_SURFACE(((0.990053454406148,0.987313720921968,0.987472672298934),
(0.990053454406148,0.987313720921968,0.987472672298934),(0.990053454406148,
0.987313720921968,0.987472672298934)))
REPRESENTATION_ITEM('')
SURFACE()
);
#3537=(
BOUNDED_SURFACE()
B_SPLINE_SURFACE(1,2,((#154734,#154735,#154736),(#154737,#154738,#154739),
(#154740,#154741,#154742)),.UNSPECIFIED.,.F.,.F.,.F.)
B_SPLINE_SURFACE_WITH_KNOTS((2,1,2),(3,3),(0.688516410585266,0.710318915637217,
1.),(0.625066077454536,0.642578551421364),.UNSPECIFIED.)
GEOMETRIC_REPRESENTATION_ITEM()
RATIONAL_B_SPLINE_SURFACE(((0.990621203777022,0.993706096834649,0.999805186472059),
(0.990621203777022,0.993706096834649,0.999805186472059),(0.990621203777022,
0.993706096834649,0.999805186472059)))
REPRESENTATION_ITEM('')
SURFACE()
);
#3538=(
BOUNDED_SURFACE()
B_SPLINE_SURFACE(1,2,((#154783,#154784,#154785),(#154786,#154787,#154788),
(#154789,#154790,#154791)),.UNSPECIFIED.,.F.,.F.,.F.)
B_SPLINE_SURFACE_WITH_KNOTS((2,1,2),(3,3),(0.688417834295043,0.710192959005572,
1.),(0.0909109506295583,0.10808458519997),.UNSPECIFIED.)
GEOMETRIC_REPRESENTATION_ITEM()
RATIONAL_B_SPLINE_SURFACE(((0.990053454406159,0.987313720921968,0.987472672298934),
(0.990053454406159,0.987313720921968,0.987472672298934),(0.990053454406159,
0.987313720921968,0.987472672298934)))
REPRESENTATION_ITEM('')
SURFACE()
);
#3539=(
BOUNDED_SURFACE()
B_SPLINE_SURFACE(1,2,((#154793,#154794,#154795),(#154796,#154797,#154798),
(#154799,#154800,#154801)),.UNSPECIFIED.,.F.,.F.,.F.)
B_SPLINE_SURFACE_WITH_KNOTS((2,1,2),(3,3),(0.688516410846974,0.710318915638875,
1.),(0.625066077454536,0.642578551421364),.UNSPECIFIED.)
GEOMETRIC_REPRESENTATION_ITEM()
RATIONAL_B_SPLINE_SURFACE(((0.990621203777022,0.993706096834649,0.999805186472059),
(0.990621203777022,0.993706096834649,0.999805186472059),(0.990621203777022,
0.993706096834649,0.999805186472059)))
REPRESENTATION_ITEM('')
SURFACE()
);
#3540=(
BOUNDED_SURFACE()
B_SPLINE_SURFACE(1,2,((#154842,#154843,#154844),(#154845,#154846,#154847),
(#154848,#154849,#154850)),.UNSPECIFIED.,.F.,.F.,.F.)
B_SPLINE_SURFACE_WITH_KNOTS((2,1,2),(3,3),(0.688417834346889,0.710192959007236,
1.),(0.0909109506295931,0.108084585199969),.UNSPECIFIED.)
GEOMETRIC_REPRESENTATION_ITEM()
RATIONAL_B_SPLINE_SURFACE(((0.990053454406148,0.987313720921968,0.987472672298934),
(0.990053454406148,0.987313720921968,0.987472672298934),(0.990053454406148,
0.987313720921968,0.987472672298934)))
REPRESENTATION_ITEM('')
SURFACE()
);
#3541=(
BOUNDED_SURFACE()
B_SPLINE_SURFACE(1,2,((#154852,#154853,#154854),(#154855,#154856,#154857),
(#154858,#154859,#154860)),.UNSPECIFIED.,.F.,.F.,.F.)
B_SPLINE_SURFACE_WITH_KNOTS((2,1,2),(3,3),(0.688516410539477,0.710318915638995,
1.),(0.625066077454536,0.642578551421364),.UNSPECIFIED.)
GEOMETRIC_REPRESENTATION_ITEM()
RATIONAL_B_SPLINE_SURFACE(((0.990621203777022,0.993706096834649,0.999805186472059),
(0.990621203777022,0.993706096834649,0.999805186472059),(0.990621203777022,
0.993706096834649,0.999805186472059)))
REPRESENTATION_ITEM('')
SURFACE()
);
#3542=(
BOUNDED_SURFACE()
B_SPLINE_SURFACE(1,2,((#154868,#154869,#154870),(#154871,#154872,#154873),
(#154874,#154875,#154876)),.UNSPECIFIED.,.F.,.F.,.F.)
B_SPLINE_SURFACE_WITH_KNOTS((2,1,2),(3,3),(0.688417834323998,0.710192959007358,
1.),(0.0909109506295931,0.108084585199969),.UNSPECIFIED.)
GEOMETRIC_REPRESENTATION_ITEM()
RATIONAL_B_SPLINE_SURFACE(((0.990053454406148,0.987313720921968,0.987472672298934),
(0.990053454406148,0.987313720921968,0.987472672298934),(0.990053454406148,
0.987313720921968,0.987472672298934)))
REPRESENTATION_ITEM('')
SURFACE()
);
#3543=(
BOUNDED_SURFACE()
B_SPLINE_SURFACE(1,2,((#154878,#154879,#154880),(#154881,#154882,#154883),
(#154884,#154885,#154886)),.UNSPECIFIED.,.F.,.F.,.F.)
B_SPLINE_SURFACE_WITH_KNOTS((2,1,2),(3,3),(0.688516410871803,0.710318915638144,
1.),(0.625066077454538,0.642578551421364),.UNSPECIFIED.)
GEOMETRIC_REPRESENTATION_ITEM()
RATIONAL_B_SPLINE_SURFACE(((0.990621203777022,0.99370609683465,0.999805186472059),
(0.990621203777022,0.99370609683465,0.999805186472059),(0.990621203777022,
0.99370609683465,0.999805186472059)))
REPRESENTATION_ITEM('')
SURFACE()
);
#3544=(
BOUNDED_SURFACE()
B_SPLINE_SURFACE(1,2,((#154927,#154928,#154929),(#154930,#154931,#154932),
(#154933,#154934,#154935)),.UNSPECIFIED.,.F.,.F.,.F.)
B_SPLINE_SURFACE_WITH_KNOTS((2,1,2),(3,3),(0.688417834386786,0.710192959006501,
1.),(0.0909109506295578,0.108084585199971),.UNSPECIFIED.)
GEOMETRIC_REPRESENTATION_ITEM()
RATIONAL_B_SPLINE_SURFACE(((0.990053454406159,0.987313720921967,0.987472672298934),
(0.990053454406159,0.987313720921967,0.987472672298934),(0.990053454406159,
0.987313720921967,0.987472672298934)))
REPRESENTATION_ITEM('')
SURFACE()
);
#3545=(
BOUNDED_SURFACE()
B_SPLINE_SURFACE(1,2,((#154937,#154938,#154939),(#154940,#154941,#154942),
(#154943,#154944,#154945)),.UNSPECIFIED.,.F.,.F.,.F.)
B_SPLINE_SURFACE_WITH_KNOTS((2,1,2),(3,3),(0.688516410587137,0.710318915639622,
1.),(0.625066077454536,0.642578551421365),.UNSPECIFIED.)
GEOMETRIC_REPRESENTATION_ITEM()
RATIONAL_B_SPLINE_SURFACE(((0.990621203777022,0.993706096834649,0.999805186472059),
(0.990621203777022,0.993706096834649,0.999805186472059),(0.990621203777022,
0.993706096834649,0.999805186472059)))
REPRESENTATION_ITEM('')
SURFACE()
);
#3546=(
BOUNDED_SURFACE()
B_SPLINE_SURFACE(1,2,((#154986,#154987,#154988),(#154989,#154990,#154991),
(#154992,#154993,#154994)),.UNSPECIFIED.,.F.,.F.,.F.)
B_SPLINE_SURFACE_WITH_KNOTS((2,1,2),(3,3),(0.688417834258306,0.710192959007977,
1.),(0.090910950629593,0.108084585199969),.UNSPECIFIED.)
GEOMETRIC_REPRESENTATION_ITEM()
RATIONAL_B_SPLINE_SURFACE(((0.990053454406148,0.987313720921968,0.987472672298934),
(0.990053454406148,0.987313720921968,0.987472672298934),(0.990053454406148,
0.987313720921968,0.987472672298934)))
REPRESENTATION_ITEM('')
SURFACE()
);
#3547=(
BOUNDED_SURFACE()
B_SPLINE_SURFACE(1,2,((#154996,#154997,#154998),(#154999,#155000,#155001),
(#155002,#155003,#155004)),.UNSPECIFIED.,.F.,.F.,.F.)
B_SPLINE_SURFACE_WITH_KNOTS((2,1,2),(3,3),(0.688516410278139,0.710318915638757,
1.),(0.625066077454536,0.642578551421365),.UNSPECIFIED.)
GEOMETRIC_REPRESENTATION_ITEM()
RATIONAL_B_SPLINE_SURFACE(((0.990621203777022,0.993706096834649,0.999805186472059),
(0.990621203777022,0.993706096834649,0.999805186472059),(0.990621203777022,
0.993706096834649,0.999805186472059)))
REPRESENTATION_ITEM('')
SURFACE()
);
#3548=(
BOUNDED_SURFACE()
B_SPLINE_SURFACE(1,2,((#155045,#155046,#155047),(#155048,#155049,#155050),
(#155051,#155052,#155053)),.UNSPECIFIED.,.F.,.F.,.F.)
B_SPLINE_SURFACE_WITH_KNOTS((2,1,2),(3,3),(0.68841783418438,0.710192959007111,
1.),(0.0909109506295945,0.108084585199969),.UNSPECIFIED.)
GEOMETRIC_REPRESENTATION_ITEM()
RATIONAL_B_SPLINE_SURFACE(((0.990053454406147,0.987313720921968,0.987472672298934),
(0.990053454406147,0.987313720921968,0.987472672298934),(0.990053454406147,
0.987313720921968,0.987472672298934)))
REPRESENTATION_ITEM('')
SURFACE()
);
#3549=(
BOUNDED_SURFACE()
B_SPLINE_SURFACE(1,2,((#155055,#155056,#155057),(#155058,#155059,#155060),
(#155061,#155062,#155063)),.UNSPECIFIED.,.F.,.F.,.F.)
B_SPLINE_SURFACE_WITH_KNOTS((2,1,2),(3,3),(0.688516410418622,0.710318915639854,
1.),(0.625066077454535,0.642578551421364),.UNSPECIFIED.)
GEOMETRIC_REPRESENTATION_ITEM()
RATIONAL_B_SPLINE_SURFACE(((0.990621203777021,0.993706096834649,0.999805186472059),
(0.990621203777021,0.993706096834649,0.999805186472059),(0.990621203777021,
0.993706096834649,0.999805186472059)))
REPRESENTATION_ITEM('')
SURFACE()
);
#3550=(
BOUNDED_SURFACE()
B_SPLINE_SURFACE(1,2,((#155104,#155105,#155106),(#155107,#155108,#155109),
(#155110,#155111,#155112)),.UNSPECIFIED.,.F.,.F.,.F.)
B_SPLINE_SURFACE_WITH_KNOTS((2,1,2),(3,3),(0.688417834637952,0.710192959008443,
1.),(0.0909109506295929,0.10808458519997),.UNSPECIFIED.)
GEOMETRIC_REPRESENTATION_ITEM()
RATIONAL_B_SPLINE_SURFACE(((0.990053454406148,0.987313720921968,0.987472672298934),
(0.990053454406148,0.987313720921968,0.987472672298934),(0.990053454406148,
0.987313720921968,0.987472672298934)))
REPRESENTATION_ITEM('')
SURFACE()
);
#3551=(
BOUNDED_SURFACE()
B_SPLINE_SURFACE(1,2,((#155114,#155115,#155116),(#155117,#155118,#155119),
(#155120,#155121,#155122)),.UNSPECIFIED.,.F.,.F.,.F.)
B_SPLINE_SURFACE_WITH_KNOTS((2,1,2),(3,3),(0.688516410561936,0.710318915640085,
1.),(0.625066077454535,0.642578551421364),.UNSPECIFIED.)
GEOMETRIC_REPRESENTATION_ITEM()
RATIONAL_B_SPLINE_SURFACE(((0.990621203777021,0.993706096834649,0.999805186472059),
(0.990621203777021,0.993706096834649,0.999805186472059),(0.990621203777021,
0.993706096834649,0.999805186472059)))
REPRESENTATION_ITEM('')
SURFACE()
);
#3552=(
BOUNDED_SURFACE()
B_SPLINE_SURFACE(1,2,((#155163,#155164,#155165),(#155166,#155167,#155168),
(#155169,#155170,#155171)),.UNSPECIFIED.,.F.,.F.,.F.)
B_SPLINE_SURFACE_WITH_KNOTS((2,1,2),(3,3),(0.688417833994755,0.71019295900844,
1.),(0.0909109506295929,0.10808458519997),.UNSPECIFIED.)
GEOMETRIC_REPRESENTATION_ITEM()
RATIONAL_B_SPLINE_SURFACE(((0.990053454406148,0.987313720921968,0.987472672298934),
(0.990053454406148,0.987313720921968,0.987472672298934),(0.990053454406148,
0.987313720921968,0.987472672298934)))
REPRESENTATION_ITEM('')
SURFACE()
);
#3553=(
BOUNDED_SURFACE()
B_SPLINE_SURFACE(1,2,((#155173,#155174,#155175),(#155176,#155177,#155178),
(#155179,#155180,#155181)),.UNSPECIFIED.,.F.,.F.,.F.)
B_SPLINE_SURFACE_WITH_KNOTS((2,1,2),(3,3),(0.688516410541635,0.710318915640077,
1.),(0.625066077454535,0.642578551421363),.UNSPECIFIED.)
GEOMETRIC_REPRESENTATION_ITEM()
RATIONAL_B_SPLINE_SURFACE(((0.990621203777021,0.993706096834649,0.999805186472059),
(0.990621203777021,0.993706096834649,0.999805186472059),(0.990621203777021,
0.993706096834649,0.999805186472059)))
REPRESENTATION_ITEM('')
SURFACE()
);
#3554=(
BOUNDED_SURFACE()
B_SPLINE_SURFACE(1,2,((#155222,#155223,#155224),(#155225,#155226,#155227),
(#155228,#155229,#155230)),.UNSPECIFIED.,.F.,.F.,.F.)
B_SPLINE_SURFACE_WITH_KNOTS((2,1,2),(3,3),(0.688417834118971,0.710192959008438,
1.),(0.0909109506295931,0.10808458519997),.UNSPECIFIED.)
GEOMETRIC_REPRESENTATION_ITEM()
RATIONAL_B_SPLINE_SURFACE(((0.990053454406148,0.987313720921968,0.987472672298933),
(0.990053454406148,0.987313720921968,0.987472672298933),(0.990053454406148,
0.987313720921968,0.987472672298933)))
REPRESENTATION_ITEM('')
SURFACE()
);
#3555=(
BOUNDED_SURFACE()
B_SPLINE_SURFACE(1,2,((#155232,#155233,#155234),(#155235,#155236,#155237),
(#155238,#155239,#155240)),.UNSPECIFIED.,.F.,.F.,.F.)
B_SPLINE_SURFACE_WITH_KNOTS((2,1,2),(3,3),(0.688516410622233,0.710318915640076,
1.),(0.625066077454535,0.642578551421363),.UNSPECIFIED.)
GEOMETRIC_REPRESENTATION_ITEM()
RATIONAL_B_SPLINE_SURFACE(((0.990621203777021,0.993706096834649,0.999805186472059),
(0.990621203777021,0.993706096834649,0.999805186472059),(0.990621203777021,
0.993706096834649,0.999805186472059)))
REPRESENTATION_ITEM('')
SURFACE()
);
#3556=(
BOUNDED_SURFACE()
B_SPLINE_SURFACE(1,2,((#155281,#155282,#155283),(#155284,#155285,#155286),
(#155287,#155288,#155289)),.UNSPECIFIED.,.F.,.F.,.F.)
B_SPLINE_SURFACE_WITH_KNOTS((2,1,2),(3,3),(0.688417834145499,0.710192959008441,
1.),(0.090910950629593,0.10808458519997),.UNSPECIFIED.)
GEOMETRIC_REPRESENTATION_ITEM()
RATIONAL_B_SPLINE_SURFACE(((0.990053454406148,0.987313720921968,0.987472672298934),
(0.990053454406148,0.987313720921968,0.987472672298934),(0.990053454406148,
0.987313720921968,0.987472672298934)))
REPRESENTATION_ITEM('')
SURFACE()
);
#3557=(
BOUNDED_SURFACE()
B_SPLINE_SURFACE(1,2,((#155316,#155317,#155318),(#155319,#155320,#155321),
(#155322,#155323,#155324)),.UNSPECIFIED.,.F.,.F.,.F.)
B_SPLINE_SURFACE_WITH_KNOTS((2,1,2),(3,3),(0.688516412901942,0.710318915639752,
1.),(0.625066077454535,0.642578551421363),.UNSPECIFIED.)
GEOMETRIC_REPRESENTATION_ITEM()
RATIONAL_B_SPLINE_SURFACE(((0.990621203777021,0.993706096834649,0.999805186472059),
(0.990621203777021,0.993706096834649,0.999805186472059),(0.990621203777021,
0.993706096834649,0.999805186472059)))
REPRESENTATION_ITEM('')
SURFACE()
);
#3558=(
BOUNDED_SURFACE()
B_SPLINE_SURFACE(1,2,((#155326,#155327,#155328),(#155329,#155330,#155331)),
 .UNSPECIFIED.,.F.,.F.,.F.)
B_SPLINE_SURFACE_WITH_KNOTS((2,2),(3,3),(0.71031891564007,1.),(0.125066077454536,
0.142578551421365),.UNSPECIFIED.)
GEOMETRIC_REPRESENTATION_ITEM()
RATIONAL_B_SPLINE_SURFACE(((0.990621203777022,0.993706096834649,0.999805186472059),
(0.990621203777022,0.993706096834649,0.999805186472059)))
REPRESENTATION_ITEM('')
SURFACE()
);
#3559=(
BOUNDED_SURFACE()
B_SPLINE_SURFACE(1,2,((#155340,#155341,#155342),(#155343,#155344,#155345)),
 .UNSPECIFIED.,.F.,.F.,.F.)
B_SPLINE_SURFACE_WITH_KNOTS((2,2),(3,3),(0.710192959008436,1.),(0.590910950629593,
0.608084585199969),.UNSPECIFIED.)
GEOMETRIC_REPRESENTATION_ITEM()
RATIONAL_B_SPLINE_SURFACE(((0.990053454406147,0.987313720921968,0.987472672298934),
(0.990053454406147,0.987313720921968,0.987472672298934)))
REPRESENTATION_ITEM('')
SURFACE()
);
#3560=(
BOUNDED_SURFACE()
B_SPLINE_SURFACE(1,2,((#155354,#155355,#155356),(#155357,#155358,#155359)),
 .UNSPECIFIED.,.F.,.F.,.F.)
B_SPLINE_SURFACE_WITH_KNOTS((2,2),(3,3),(0.71031891564008,1.),(0.125066077454536,
0.142578551421364),.UNSPECIFIED.)
GEOMETRIC_REPRESENTATION_ITEM()
RATIONAL_B_SPLINE_SURFACE(((0.990621203777022,0.993706096834649,0.999805186472059),
(0.990621203777022,0.993706096834649,0.999805186472059)))
REPRESENTATION_ITEM('')
SURFACE()
);
#3561=(
BOUNDED_SURFACE()
B_SPLINE_SURFACE(1,2,((#155361,#155362,#155363),(#155364,#155365,#155366)),
 .UNSPECIFIED.,.F.,.F.,.F.)
B_SPLINE_SURFACE_WITH_KNOTS((2,2),(3,3),(0.710192959008444,1.),(0.590910950629471,
0.60808458519997),.UNSPECIFIED.)
GEOMETRIC_REPRESENTATION_ITEM()
RATIONAL_B_SPLINE_SURFACE(((0.990053454406186,0.987313720921966,0.987472672298933),
(0.990053454406186,0.987313720921966,0.987472672298933)))
REPRESENTATION_ITEM('')
SURFACE()
);
#3562=(
BOUNDED_SURFACE()
B_SPLINE_SURFACE(1,2,((#155375,#155376,#155377),(#155378,#155379,#155380)),
 .UNSPECIFIED.,.F.,.F.,.F.)
B_SPLINE_SURFACE_WITH_KNOTS((2,2),(3,3),(0.710318915640072,1.),(0.125066077454536,
0.142578551421364),.UNSPECIFIED.)
GEOMETRIC_REPRESENTATION_ITEM()
RATIONAL_B_SPLINE_SURFACE(((0.990621203777022,0.993706096834649,0.999805186472059),
(0.990621203777022,0.993706096834649,0.999805186472059)))
REPRESENTATION_ITEM('')
SURFACE()
);
#3563=(
BOUNDED_SURFACE()
B_SPLINE_SURFACE(1,2,((#155382,#155383,#155384),(#155385,#155386,#155387)),
 .UNSPECIFIED.,.F.,.F.,.F.)
B_SPLINE_SURFACE_WITH_KNOTS((2,2),(3,3),(0.710192959008435,1.),(0.590910950629581,
0.60808458519997),.UNSPECIFIED.)
GEOMETRIC_REPRESENTATION_ITEM()
RATIONAL_B_SPLINE_SURFACE(((0.990053454406151,0.987313720921968,0.987472672298934),
(0.990053454406151,0.987313720921968,0.987472672298934)))
REPRESENTATION_ITEM('')
SURFACE()
);
#3564=(
BOUNDED_SURFACE()
B_SPLINE_SURFACE(1,2,((#155396,#155397,#155398),(#155399,#155400,#155401)),
 .UNSPECIFIED.,.F.,.F.,.F.)
B_SPLINE_SURFACE_WITH_KNOTS((2,2),(3,3),(0.710318915640081,1.),(0.125066077454536,
0.142578551421363),.UNSPECIFIED.)
GEOMETRIC_REPRESENTATION_ITEM()
RATIONAL_B_SPLINE_SURFACE(((0.990621203777022,0.993706096834649,0.999805186472059),
(0.990621203777022,0.993706096834649,0.999805186472059)))
REPRESENTATION_ITEM('')
SURFACE()
);
#3565=(
BOUNDED_SURFACE()
B_SPLINE_SURFACE(1,2,((#155403,#155404,#155405),(#155406,#155407,#155408)),
 .UNSPECIFIED.,.F.,.F.,.F.)
B_SPLINE_SURFACE_WITH_KNOTS((2,2),(3,3),(0.710192959008441,1.),(0.59091095062936,
0.608084585199972),.UNSPECIFIED.)
GEOMETRIC_REPRESENTATION_ITEM()
RATIONAL_B_SPLINE_SURFACE(((0.990053454406222,0.987313720921965,0.987472672298933),
(0.990053454406222,0.987313720921965,0.987472672298933)))
REPRESENTATION_ITEM('')
SURFACE()
);
#3566=(
BOUNDED_SURFACE()
B_SPLINE_SURFACE(1,2,((#155417,#155418,#155419),(#155420,#155421,#155422)),
 .UNSPECIFIED.,.F.,.F.,.F.)
B_SPLINE_SURFACE_WITH_KNOTS((2,2),(3,3),(0.710318915640076,1.),(0.125066077454535,
0.142578551421363),.UNSPECIFIED.)
GEOMETRIC_REPRESENTATION_ITEM()
RATIONAL_B_SPLINE_SURFACE(((0.990621203777021,0.993706096834649,0.999805186472058),
(0.990621203777021,0.993706096834649,0.999805186472058)))
REPRESENTATION_ITEM('')
SURFACE()
);
#3567=(
BOUNDED_SURFACE()
B_SPLINE_SURFACE(1,2,((#155424,#155425,#155426),(#155427,#155428,#155429)),
 .UNSPECIFIED.,.F.,.F.,.F.)
B_SPLINE_SURFACE_WITH_KNOTS((2,2),(3,3),(0.71019295900844,1.),(0.590910950629587,
0.608084585199971),.UNSPECIFIED.)
GEOMETRIC_REPRESENTATION_ITEM()
RATIONAL_B_SPLINE_SURFACE(((0.99005345440615,0.987313720921968,0.987472672298934),
(0.990053454406149,0.987313720921967,0.987472672298933)))
REPRESENTATION_ITEM('')
SURFACE()
);
#3568=(
BOUNDED_SURFACE()
B_SPLINE_SURFACE(1,2,((#155438,#155439,#155440),(#155441,#155442,#155443)),
 .UNSPECIFIED.,.F.,.F.,.F.)
B_SPLINE_SURFACE_WITH_KNOTS((2,2),(3,3),(0.710318915640084,1.),(0.125066077454535,
0.142578551421363),.UNSPECIFIED.)
GEOMETRIC_REPRESENTATION_ITEM()
RATIONAL_B_SPLINE_SURFACE(((0.990621203777021,0.993706096834649,0.999805186472059),
(0.990621203777021,0.993706096834649,0.999805186472059)))
REPRESENTATION_ITEM('')
SURFACE()
);
#3569=(
BOUNDED_SURFACE()
B_SPLINE_SURFACE(1,2,((#155445,#155446,#155447),(#155448,#155449,#155450)),
 .UNSPECIFIED.,.F.,.F.,.F.)
B_SPLINE_SURFACE_WITH_KNOTS((2,2),(3,3),(0.71019295900844,1.),(0.590910950629178,
0.608084585199973),.UNSPECIFIED.)
GEOMETRIC_REPRESENTATION_ITEM()
RATIONAL_B_SPLINE_SURFACE(((0.99005345440628,0.987313720921964,0.987472672298934),
(0.99005345440628,0.987313720921964,0.987472672298934)))
REPRESENTATION_ITEM('')
SURFACE()
);
#3570=(
BOUNDED_SURFACE()
B_SPLINE_SURFACE(1,2,((#155459,#155460,#155461),(#155462,#155463,#155464)),
 .UNSPECIFIED.,.F.,.F.,.F.)
B_SPLINE_SURFACE_WITH_KNOTS((2,2),(3,3),(0.710318915640074,1.),(0.125066077454535,
0.142578551421363),.UNSPECIFIED.)
GEOMETRIC_REPRESENTATION_ITEM()
RATIONAL_B_SPLINE_SURFACE(((0.990621203777021,0.993706096834649,0.999805186472059),
(0.990621203777021,0.993706096834649,0.999805186472059)))
REPRESENTATION_ITEM('')
SURFACE()
);
#3571=(
BOUNDED_SURFACE()
B_SPLINE_SURFACE(1,2,((#155466,#155467,#155468),(#155469,#155470,#155471)),
 .UNSPECIFIED.,.F.,.F.,.F.)
B_SPLINE_SURFACE_WITH_KNOTS((2,2),(3,3),(0.71019295900844,1.),(0.590910950629594,
0.60808458519997),.UNSPECIFIED.)
GEOMETRIC_REPRESENTATION_ITEM()
RATIONAL_B_SPLINE_SURFACE(((0.990053454406147,0.987313720921968,0.987472672298933),
(0.990053454406147,0.987313720921968,0.987472672298933)))
REPRESENTATION_ITEM('')
SURFACE()
);
#3572=(
BOUNDED_SURFACE()
B_SPLINE_SURFACE(1,2,((#155480,#155481,#155482),(#155483,#155484,#155485)),
 .UNSPECIFIED.,.F.,.F.,.F.)
B_SPLINE_SURFACE_WITH_KNOTS((2,2),(3,3),(0.710318915640075,1.),(0.125066077454535,
0.142578551421363),.UNSPECIFIED.)
GEOMETRIC_REPRESENTATION_ITEM()
RATIONAL_B_SPLINE_SURFACE(((0.990621203777021,0.993706096834649,0.999805186472059),
(0.990621203777021,0.993706096834649,0.999805186472059)))
REPRESENTATION_ITEM('')
SURFACE()
);
#3573=(
BOUNDED_SURFACE()
B_SPLINE_SURFACE(1,2,((#155487,#155488,#155489),(#155490,#155491,#155492)),
 .UNSPECIFIED.,.F.,.F.,.F.)
B_SPLINE_SURFACE_WITH_KNOTS((2,2),(3,3),(0.71019295900844,1.),(0.590910950629584,
0.608084585199971),.UNSPECIFIED.)
GEOMETRIC_REPRESENTATION_ITEM()
RATIONAL_B_SPLINE_SURFACE(((0.99005345440615,0.987313720921968,0.987472672298934),
(0.99005345440615,0.987313720921968,0.987472672298934)))
REPRESENTATION_ITEM('')
SURFACE()
);
#3574=(
BOUNDED_SURFACE()
B_SPLINE_SURFACE(1,2,((#155501,#155502,#155503),(#155504,#155505,#155506)),
 .UNSPECIFIED.,.F.,.F.,.F.)
B_SPLINE_SURFACE_WITH_KNOTS((2,2),(3,3),(0.710318915640083,1.),(0.125066077454536,
0.142578551421363),.UNSPECIFIED.)
GEOMETRIC_REPRESENTATION_ITEM()
RATIONAL_B_SPLINE_SURFACE(((0.990621203777021,0.993706096834649,0.999805186472059),
(0.990621203777021,0.993706096834649,0.999805186472059)))
REPRESENTATION_ITEM('')
SURFACE()
);
#3575=(
BOUNDED_SURFACE()
B_SPLINE_SURFACE(1,2,((#155508,#155509,#155510),(#155511,#155512,#155513)),
 .UNSPECIFIED.,.F.,.F.,.F.)
B_SPLINE_SURFACE_WITH_KNOTS((2,2),(3,3),(0.710192959008443,1.),(0.590910950629594,
0.608084585199971),.UNSPECIFIED.)
GEOMETRIC_REPRESENTATION_ITEM()
RATIONAL_B_SPLINE_SURFACE(((0.990053454406147,0.987313720921968,0.987472672298934),
(0.990053454406147,0.987313720921968,0.987472672298934)))
REPRESENTATION_ITEM('')
SURFACE()
);
#3576=(
BOUNDED_SURFACE()
B_SPLINE_SURFACE(1,2,((#155522,#155523,#155524),(#155525,#155526,#155527)),
 .UNSPECIFIED.,.F.,.F.,.F.)
B_SPLINE_SURFACE_WITH_KNOTS((2,2),(3,3),(0.710318915640079,1.),(0.125066077454535,
0.142578551421363),.UNSPECIFIED.)
GEOMETRIC_REPRESENTATION_ITEM()
RATIONAL_B_SPLINE_SURFACE(((0.990621203777021,0.993706096834649,0.999805186472059),
(0.990621203777021,0.993706096834649,0.999805186472059)))
REPRESENTATION_ITEM('')
SURFACE()
);
#3577=(
BOUNDED_SURFACE()
B_SPLINE_SURFACE(1,2,((#155529,#155530,#155531),(#155532,#155533,#155534)),
 .UNSPECIFIED.,.F.,.F.,.F.)
B_SPLINE_SURFACE_WITH_KNOTS((2,2),(3,3),(0.710192959008436,1.),(0.590910950629279,
0.608084585199973),.UNSPECIFIED.)
GEOMETRIC_REPRESENTATION_ITEM()
RATIONAL_B_SPLINE_SURFACE(((0.990053454406248,0.987313720921964,0.987472672298934),
(0.990053454406248,0.987313720921964,0.987472672298934)))
REPRESENTATION_ITEM('')
SURFACE()
);
#3578=(
BOUNDED_SURFACE()
B_SPLINE_SURFACE(1,2,((#155543,#155544,#155545),(#155546,#155547,#155548)),
 .UNSPECIFIED.,.F.,.F.,.F.)
B_SPLINE_SURFACE_WITH_KNOTS((2,2),(3,3),(0.710318915640077,1.),(0.125066077454535,
0.142578551421363),.UNSPECIFIED.)
GEOMETRIC_REPRESENTATION_ITEM()
RATIONAL_B_SPLINE_SURFACE(((0.990621203777021,0.993706096834649,0.999805186472059),
(0.990621203777021,0.993706096834649,0.999805186472059)))
REPRESENTATION_ITEM('')
SURFACE()
);
#3579=(
BOUNDED_SURFACE()
B_SPLINE_SURFACE(1,2,((#155550,#155551,#155552),(#155553,#155554,#155555)),
 .UNSPECIFIED.,.F.,.F.,.F.)
B_SPLINE_SURFACE_WITH_KNOTS((2,2),(3,3),(0.710192959008443,1.),(0.590910950629594,
0.608084585199971),.UNSPECIFIED.)
GEOMETRIC_REPRESENTATION_ITEM()
RATIONAL_B_SPLINE_SURFACE(((0.990053454406147,0.987313720921967,0.987472672298933),
(0.990053454406147,0.987313720921967,0.987472672298933)))
REPRESENTATION_ITEM('')
SURFACE()
);
#3580=(
BOUNDED_SURFACE()
B_SPLINE_SURFACE(1,2,((#155564,#155565,#155566),(#155567,#155568,#155569)),
 .UNSPECIFIED.,.F.,.F.,.F.)
B_SPLINE_SURFACE_WITH_KNOTS((2,2),(3,3),(0.710318915640078,1.),(0.125066077454536,
0.142578551421364),.UNSPECIFIED.)
GEOMETRIC_REPRESENTATION_ITEM()
RATIONAL_B_SPLINE_SURFACE(((0.990621203777021,0.993706096834649,0.999805186472059),
(0.990621203777021,0.993706096834649,0.999805186472059)))
REPRESENTATION_ITEM('')
SURFACE()
);
#3581=(
BOUNDED_SURFACE()
B_SPLINE_SURFACE(1,2,((#155571,#155572,#155573),(#155574,#155575,#155576)),
 .UNSPECIFIED.,.F.,.F.,.F.)
B_SPLINE_SURFACE_WITH_KNOTS((2,2),(3,3),(0.710192959008436,1.),(0.590910950629528,
0.608084585199971),.UNSPECIFIED.)
GEOMETRIC_REPRESENTATION_ITEM()
RATIONAL_B_SPLINE_SURFACE(((0.990053454406168,0.987313720921967,0.987472672298934),
(0.990053454406168,0.987313720921967,0.987472672298934)))
REPRESENTATION_ITEM('')
SURFACE()
);
#3582=(
BOUNDED_SURFACE()
B_SPLINE_SURFACE(1,2,((#155585,#155586,#155587),(#155588,#155589,#155590)),
 .UNSPECIFIED.,.F.,.F.,.F.)
B_SPLINE_SURFACE_WITH_KNOTS((2,2),(3,3),(0.710318915640075,1.),(0.125066077454535,
0.142578551421363),.UNSPECIFIED.)
GEOMETRIC_REPRESENTATION_ITEM()
RATIONAL_B_SPLINE_SURFACE(((0.990621203777021,0.993706096834648,0.999805186472059),
(0.990621203777021,0.993706096834648,0.999805186472059)))
REPRESENTATION_ITEM('')
SURFACE()
);
#3583=(
BOUNDED_SURFACE()
B_SPLINE_SURFACE(1,2,((#155592,#155593,#155594),(#155595,#155596,#155597)),
 .UNSPECIFIED.,.F.,.F.,.F.)
B_SPLINE_SURFACE_WITH_KNOTS((2,2),(3,3),(0.710192959008441,1.),(0.590910950629594,
0.60808458519997),.UNSPECIFIED.)
GEOMETRIC_REPRESENTATION_ITEM()
RATIONAL_B_SPLINE_SURFACE(((0.990053454406147,0.987313720921967,0.987472672298933),
(0.990053454406147,0.987313720921968,0.987472672298933)))
REPRESENTATION_ITEM('')
SURFACE()
);
#3584=(
BOUNDED_SURFACE()
B_SPLINE_SURFACE(1,2,((#155606,#155607,#155608),(#155609,#155610,#155611)),
 .UNSPECIFIED.,.F.,.F.,.F.)
B_SPLINE_SURFACE_WITH_KNOTS((2,2),(3,3),(0.71031891564008,1.),(0.125066077454535,
0.142578551421364),.UNSPECIFIED.)
GEOMETRIC_REPRESENTATION_ITEM()
RATIONAL_B_SPLINE_SURFACE(((0.990621203777021,0.993706096834649,0.999805186472059),
(0.990621203777021,0.993706096834649,0.999805186472059)))
REPRESENTATION_ITEM('')
SURFACE()
);
#3585=(
BOUNDED_SURFACE()
B_SPLINE_SURFACE(1,2,((#155613,#155614,#155615),(#155616,#155617,#155618)),
 .UNSPECIFIED.,.F.,.F.,.F.)
B_SPLINE_SURFACE_WITH_KNOTS((2,2),(3,3),(0.710192959008435,1.),(0.590910950629321,
0.608084585199972),.UNSPECIFIED.)
GEOMETRIC_REPRESENTATION_ITEM()
RATIONAL_B_SPLINE_SURFACE(((0.990053454406234,0.987313720921965,0.987472672298934),
(0.990053454406234,0.987313720921965,0.987472672298934)))
REPRESENTATION_ITEM('')
SURFACE()
);
#3586=(
BOUNDED_SURFACE()
B_SPLINE_SURFACE(1,2,((#155627,#155628,#155629),(#155630,#155631,#155632)),
 .UNSPECIFIED.,.F.,.F.,.F.)
B_SPLINE_SURFACE_WITH_KNOTS((2,2),(3,3),(0.710318915640079,1.),(0.125066077454536,
0.142578551421363),.UNSPECIFIED.)
GEOMETRIC_REPRESENTATION_ITEM()
RATIONAL_B_SPLINE_SURFACE(((0.990621203777021,0.993706096834649,0.999805186472059),
(0.990621203777021,0.993706096834649,0.999805186472059)))
REPRESENTATION_ITEM('')
SURFACE()
);
#3587=(
BOUNDED_SURFACE()
B_SPLINE_SURFACE(1,2,((#155634,#155635,#155636),(#155637,#155638,#155639)),
 .UNSPECIFIED.,.F.,.F.,.F.)
B_SPLINE_SURFACE_WITH_KNOTS((2,2),(3,3),(0.710192959008445,1.),(0.590910950629594,
0.60808458519997),.UNSPECIFIED.)
GEOMETRIC_REPRESENTATION_ITEM()
RATIONAL_B_SPLINE_SURFACE(((0.990053454406147,0.987313720921968,0.987472672298933),
(0.990053454406147,0.987313720921968,0.987472672298933)))
REPRESENTATION_ITEM('')
SURFACE()
);
#3588=(
BOUNDED_SURFACE()
B_SPLINE_SURFACE(1,2,((#155648,#155649,#155650),(#155651,#155652,#155653)),
 .UNSPECIFIED.,.F.,.F.,.F.)
B_SPLINE_SURFACE_WITH_KNOTS((2,2),(3,3),(0.71031891564008,1.),(0.125066077454535,
0.142578551421363),.UNSPECIFIED.)
GEOMETRIC_REPRESENTATION_ITEM()
RATIONAL_B_SPLINE_SURFACE(((0.990621203777021,0.993706096834649,0.999805186472059),
(0.990621203777021,0.993706096834649,0.999805186472059)))
REPRESENTATION_ITEM('')
SURFACE()
);
#3589=(
BOUNDED_SURFACE()
B_SPLINE_SURFACE(1,2,((#155655,#155656,#155657),(#155658,#155659,#155660)),
 .UNSPECIFIED.,.F.,.F.,.F.)
B_SPLINE_SURFACE_WITH_KNOTS((2,2),(3,3),(0.710192959008442,1.),(0.590910950629594,
0.60808458519997),.UNSPECIFIED.)
GEOMETRIC_REPRESENTATION_ITEM()
RATIONAL_B_SPLINE_SURFACE(((0.990053454406147,0.987313720921968,0.987472672298933),
(0.990053454406147,0.987313720921968,0.987472672298933)))
REPRESENTATION_ITEM('')
SURFACE()
);
#3590=(
BOUNDED_SURFACE()
B_SPLINE_SURFACE(1,2,((#155669,#155670,#155671),(#155672,#155673,#155674)),
 .UNSPECIFIED.,.F.,.F.,.F.)
B_SPLINE_SURFACE_WITH_KNOTS((2,2),(3,3),(0.71031891564008,1.),(0.125066077454535,
0.142578551421363),.UNSPECIFIED.)
GEOMETRIC_REPRESENTATION_ITEM()
RATIONAL_B_SPLINE_SURFACE(((0.990621203777021,0.993706096834649,0.999805186472059),
(0.990621203777021,0.993706096834649,0.999805186472059)))
REPRESENTATION_ITEM('')
SURFACE()
);
#3591=(
BOUNDED_SURFACE()
B_SPLINE_SURFACE(1,2,((#155676,#155677,#155678),(#155679,#155680,#155681)),
 .UNSPECIFIED.,.F.,.F.,.F.)
B_SPLINE_SURFACE_WITH_KNOTS((2,2),(3,3),(0.710192959008445,1.),(0.590910950629594,
0.608084585199971),.UNSPECIFIED.)
GEOMETRIC_REPRESENTATION_ITEM()
RATIONAL_B_SPLINE_SURFACE(((0.990053454406147,0.987313720921968,0.987472672298934),
(0.990053454406147,0.987313720921968,0.987472672298934)))
REPRESENTATION_ITEM('')
SURFACE()
);
#3592=(
BOUNDED_SURFACE()
B_SPLINE_SURFACE(1,2,((#155690,#155691,#155692),(#155693,#155694,#155695)),
 .UNSPECIFIED.,.F.,.F.,.F.)
B_SPLINE_SURFACE_WITH_KNOTS((2,2),(3,3),(0.710318915640083,1.),(0.125066077454535,
0.142578551421363),.UNSPECIFIED.)
GEOMETRIC_REPRESENTATION_ITEM()
RATIONAL_B_SPLINE_SURFACE(((0.990621203777021,0.993706096834649,0.999805186472059),
(0.990621203777021,0.993706096834649,0.999805186472059)))
REPRESENTATION_ITEM('')
SURFACE()
);
#3593=(
BOUNDED_SURFACE()
B_SPLINE_SURFACE(1,2,((#155697,#155698,#155699),(#155700,#155701,#155702)),
 .UNSPECIFIED.,.F.,.F.,.F.)
B_SPLINE_SURFACE_WITH_KNOTS((2,2),(3,3),(0.710192959008439,1.),(0.590910950629594,
0.60808458519997),.UNSPECIFIED.)
GEOMETRIC_REPRESENTATION_ITEM()
RATIONAL_B_SPLINE_SURFACE(((0.990053454406147,0.987313720921968,0.987472672298933),
(0.990053454406147,0.987313720921968,0.987472672298933)))
REPRESENTATION_ITEM('')
SURFACE()
);
#3594=(
BOUNDED_SURFACE()
B_SPLINE_SURFACE(1,2,((#155711,#155712,#155713),(#155714,#155715,#155716)),
 .UNSPECIFIED.,.F.,.F.,.F.)
B_SPLINE_SURFACE_WITH_KNOTS((2,2),(3,3),(0.710318915639847,1.),(0.125066077454535,
0.142578551421363),.UNSPECIFIED.)
GEOMETRIC_REPRESENTATION_ITEM()
RATIONAL_B_SPLINE_SURFACE(((0.990621203777021,0.993706096834649,0.999805186472059),
(0.990621203777021,0.993706096834649,0.999805186472059)))
REPRESENTATION_ITEM('')
SURFACE()
);
#3595=(
BOUNDED_SURFACE()
B_SPLINE_SURFACE(1,2,((#155718,#155719,#155720),(#155721,#155722,#155723)),
 .UNSPECIFIED.,.F.,.F.,.F.)
B_SPLINE_SURFACE_WITH_KNOTS((2,2),(3,3),(0.710192959008435,1.),(0.590910950629594,
0.60808458519997),.UNSPECIFIED.)
GEOMETRIC_REPRESENTATION_ITEM()
RATIONAL_B_SPLINE_SURFACE(((0.990053454406147,0.987313720921968,0.987472672298933),
(0.990053454406147,0.987313720921968,0.987472672298933)))
REPRESENTATION_ITEM('')
SURFACE()
);
#3596=(
BOUNDED_SURFACE()
B_SPLINE_SURFACE(1,2,((#155732,#155733,#155734),(#155735,#155736,#155737)),
 .UNSPECIFIED.,.F.,.F.,.F.)
B_SPLINE_SURFACE_WITH_KNOTS((2,2),(3,3),(0.710318915640079,1.),(0.125066077454536,
0.142578551421364),.UNSPECIFIED.)
GEOMETRIC_REPRESENTATION_ITEM()
RATIONAL_B_SPLINE_SURFACE(((0.990621203777022,0.993706096834649,0.999805186472059),
(0.990621203777022,0.993706096834649,0.999805186472059)))
REPRESENTATION_ITEM('')
SURFACE()
);
#3597=(
BOUNDED_SURFACE()
B_SPLINE_SURFACE(1,2,((#155739,#155740,#155741),(#155742,#155743,#155744)),
 .UNSPECIFIED.,.F.,.F.,.F.)
B_SPLINE_SURFACE_WITH_KNOTS((2,2),(3,3),(0.71019295900844,1.),(0.590910950629593,
0.608084585199969),.UNSPECIFIED.)
GEOMETRIC_REPRESENTATION_ITEM()
RATIONAL_B_SPLINE_SURFACE(((0.990053454406147,0.987313720921968,0.987472672298934),
(0.990053454406147,0.987313720921968,0.987472672298934)))
REPRESENTATION_ITEM('')
SURFACE()
);
#3598=(
BOUNDED_SURFACE()
B_SPLINE_SURFACE(1,2,((#155753,#155754,#155755),(#155756,#155757,#155758)),
 .UNSPECIFIED.,.F.,.F.,.F.)
B_SPLINE_SURFACE_WITH_KNOTS((2,2),(3,3),(0.710318915640078,1.),(0.125066077454536,
0.142578551421364),.UNSPECIFIED.)
GEOMETRIC_REPRESENTATION_ITEM()
RATIONAL_B_SPLINE_SURFACE(((0.990621203777022,0.993706096834649,0.999805186472059),
(0.990621203777022,0.993706096834649,0.999805186472059)))
REPRESENTATION_ITEM('')
SURFACE()
);
#3599=(
BOUNDED_SURFACE()
B_SPLINE_SURFACE(1,2,((#155760,#155761,#155762),(#155763,#155764,#155765)),
 .UNSPECIFIED.,.F.,.F.,.F.)
B_SPLINE_SURFACE_WITH_KNOTS((2,2),(3,3),(0.710192959008301,1.),(0.590910950629528,
0.60808458519997),.UNSPECIFIED.)
GEOMETRIC_REPRESENTATION_ITEM()
RATIONAL_B_SPLINE_SURFACE(((0.990053454406168,0.987313720921967,0.987472672298934),
(0.990053454406168,0.987313720921967,0.987472672298934)))
REPRESENTATION_ITEM('')
SURFACE()
);
#3600=(
BOUNDED_SURFACE()
B_SPLINE_SURFACE(1,2,((#155774,#155775,#155776),(#155777,#155778,#155779)),
 .UNSPECIFIED.,.F.,.F.,.F.)
B_SPLINE_SURFACE_WITH_KNOTS((2,2),(3,3),(0.710318915639942,1.),(0.125066077454536,
0.142578551421366),.UNSPECIFIED.)
GEOMETRIC_REPRESENTATION_ITEM()
RATIONAL_B_SPLINE_SURFACE(((0.990621203777022,0.993706096834649,0.99980518647206),
(0.990621203777022,0.99370609683465,0.99980518647206)))
REPRESENTATION_ITEM('')
SURFACE()
);
#3601=(
BOUNDED_SURFACE()
B_SPLINE_SURFACE(1,2,((#155781,#155782,#155783),(#155784,#155785,#155786)),
 .UNSPECIFIED.,.F.,.F.,.F.)
B_SPLINE_SURFACE_WITH_KNOTS((2,2),(3,3),(0.710192959008294,1.),(0.590910950629541,
0.60808458519997),.UNSPECIFIED.)
GEOMETRIC_REPRESENTATION_ITEM()
RATIONAL_B_SPLINE_SURFACE(((0.990053454406164,0.987313720921967,0.987472672298934),
(0.990053454406164,0.987313720921967,0.987472672298934)))
REPRESENTATION_ITEM('')
SURFACE()
);
#3602=(
BOUNDED_SURFACE()
B_SPLINE_SURFACE(1,2,((#155795,#155796,#155797),(#155798,#155799,#155800)),
 .UNSPECIFIED.,.F.,.F.,.F.)
B_SPLINE_SURFACE_WITH_KNOTS((2,2),(3,3),(0.710318915639933,1.),(0.125066077454536,
0.142578551421364),.UNSPECIFIED.)
GEOMETRIC_REPRESENTATION_ITEM()
RATIONAL_B_SPLINE_SURFACE(((0.990621203777022,0.993706096834649,0.999805186472059),
(0.990621203777022,0.993706096834649,0.999805186472059)))
REPRESENTATION_ITEM('')
SURFACE()
);
#3603=(
BOUNDED_SURFACE()
B_SPLINE_SURFACE(1,2,((#155802,#155803,#155804),(#155805,#155806,#155807)),
 .UNSPECIFIED.,.F.,.F.,.F.)
B_SPLINE_SURFACE_WITH_KNOTS((2,2),(3,3),(0.710192959008284,1.),(0.590910950629593,
0.60808458519997),.UNSPECIFIED.)
GEOMETRIC_REPRESENTATION_ITEM()
RATIONAL_B_SPLINE_SURFACE(((0.990053454406147,0.987313720921968,0.987472672298934),
(0.990053454406147,0.987313720921968,0.987472672298934)))
REPRESENTATION_ITEM('')
SURFACE()
);
#3604=(
BOUNDED_SURFACE()
B_SPLINE_SURFACE(1,2,((#155816,#155817,#155818),(#155819,#155820,#155821)),
 .UNSPECIFIED.,.F.,.F.,.F.)
B_SPLINE_SURFACE_WITH_KNOTS((2,2),(3,3),(0.710318915639924,1.),(0.125066077454536,
0.142578551421364),.UNSPECIFIED.)
GEOMETRIC_REPRESENTATION_ITEM()
RATIONAL_B_SPLINE_SURFACE(((0.990621203777022,0.993706096834649,0.999805186472059),
(0.990621203777022,0.993706096834649,0.999805186472059)))
REPRESENTATION_ITEM('')
SURFACE()
);
#3605=(
BOUNDED_SURFACE()
B_SPLINE_SURFACE(1,2,((#155823,#155824,#155825),(#155826,#155827,#155828)),
 .UNSPECIFIED.,.F.,.F.,.F.)
B_SPLINE_SURFACE_WITH_KNOTS((2,2),(3,3),(0.71019295900691,1.),(0.590910950629592,
0.608084585199969),.UNSPECIFIED.)
GEOMETRIC_REPRESENTATION_ITEM()
RATIONAL_B_SPLINE_SURFACE(((0.990053454406148,0.987313720921968,0.987472672298934),
(0.990053454406148,0.987313720921968,0.987472672298934)))
REPRESENTATION_ITEM('')
SURFACE()
);
#3606=(
BOUNDED_SURFACE()
B_SPLINE_SURFACE(1,2,((#155837,#155838,#155839),(#155840,#155841,#155842)),
 .UNSPECIFIED.,.F.,.F.,.F.)
B_SPLINE_SURFACE_WITH_KNOTS((2,2),(3,3),(0.710318915638558,1.),(0.125066077454536,
0.142578551421364),.UNSPECIFIED.)
GEOMETRIC_REPRESENTATION_ITEM()
RATIONAL_B_SPLINE_SURFACE(((0.990621203777022,0.993706096834649,0.999805186472059),
(0.990621203777022,0.993706096834649,0.999805186472059)))
REPRESENTATION_ITEM('')
SURFACE()
);
#3607=(
BOUNDED_SURFACE()
B_SPLINE_SURFACE(1,2,((#155844,#155845,#155846),(#155847,#155848,#155849)),
 .UNSPECIFIED.,.F.,.F.,.F.)
B_SPLINE_SURFACE_WITH_KNOTS((2,2),(3,3),(0.710192959007976,1.),(0.59091095062944,
0.60808458519997),.UNSPECIFIED.)
GEOMETRIC_REPRESENTATION_ITEM()
RATIONAL_B_SPLINE_SURFACE(((0.990053454406197,0.987313720921966,0.987472672298934),
(0.990053454406197,0.987313720921966,0.987472672298934)))
REPRESENTATION_ITEM('')
SURFACE()
);
#3608=(
BOUNDED_SURFACE()
B_SPLINE_SURFACE(1,2,((#155858,#155859,#155860),(#155861,#155862,#155863)),
 .UNSPECIFIED.,.F.,.F.,.F.)
B_SPLINE_SURFACE_WITH_KNOTS((2,2),(3,3),(0.710318915639623,1.),(0.125066077454536,
0.142578551421364),.UNSPECIFIED.)
GEOMETRIC_REPRESENTATION_ITEM()
RATIONAL_B_SPLINE_SURFACE(((0.990621203777022,0.993706096834649,0.999805186472059),
(0.990621203777022,0.993706096834649,0.999805186472059)))
REPRESENTATION_ITEM('')
SURFACE()
);
#3609=(
BOUNDED_SURFACE()
B_SPLINE_SURFACE(1,2,((#155865,#155866,#155867),(#155868,#155869,#155870)),
 .UNSPECIFIED.,.F.,.F.,.F.)
B_SPLINE_SURFACE_WITH_KNOTS((2,2),(3,3),(0.710192959008351,1.),(0.590910950629588,
0.608084585199969),.UNSPECIFIED.)
GEOMETRIC_REPRESENTATION_ITEM()
RATIONAL_B_SPLINE_SURFACE(((0.990053454406149,0.987313720921968,0.987472672298934),
(0.990053454406149,0.987313720921968,0.987472672298934)))
REPRESENTATION_ITEM('')
SURFACE()
);
#3610=(
BOUNDED_SURFACE()
B_SPLINE_SURFACE(1,2,((#155879,#155880,#155881),(#155882,#155883,#155884)),
 .UNSPECIFIED.,.F.,.F.,.F.)
B_SPLINE_SURFACE_WITH_KNOTS((2,2),(3,3),(0.710318915639997,1.),(0.125066077454536,
0.142578551421364),.UNSPECIFIED.)
GEOMETRIC_REPRESENTATION_ITEM()
RATIONAL_B_SPLINE_SURFACE(((0.990621203777022,0.993706096834649,0.999805186472059),
(0.990621203777022,0.993706096834649,0.999805186472059)))
REPRESENTATION_ITEM('')
SURFACE()
);
#3611=(
BOUNDED_SURFACE()
B_SPLINE_SURFACE(1,2,((#155886,#155887,#155888),(#155889,#155890,#155891)),
 .UNSPECIFIED.,.F.,.F.,.F.)
B_SPLINE_SURFACE_WITH_KNOTS((2,2),(3,3),(0.71019295900836,1.),(0.590910950629593,
0.608084585199969),.UNSPECIFIED.)
GEOMETRIC_REPRESENTATION_ITEM()
RATIONAL_B_SPLINE_SURFACE(((0.990053454406147,0.987313720921968,0.987472672298934),
(0.990053454406147,0.987313720921968,0.987472672298934)))
REPRESENTATION_ITEM('')
SURFACE()
);
#3612=(
BOUNDED_SURFACE()
B_SPLINE_SURFACE(1,2,((#155900,#155901,#155902),(#155903,#155904,#155905)),
 .UNSPECIFIED.,.F.,.F.,.F.)
B_SPLINE_SURFACE_WITH_KNOTS((2,2),(3,3),(0.710318915640007,1.),(0.125066077454536,
0.142578551421364),.UNSPECIFIED.)
GEOMETRIC_REPRESENTATION_ITEM()
RATIONAL_B_SPLINE_SURFACE(((0.990621203777022,0.993706096834649,0.999805186472059),
(0.990621203777022,0.993706096834649,0.999805186472059)))
REPRESENTATION_ITEM('')
SURFACE()
);
#3613=(
BOUNDED_SURFACE()
B_SPLINE_SURFACE(1,2,((#155907,#155908,#155909),(#155910,#155911,#155912)),
 .UNSPECIFIED.,.F.,.F.,.F.)
B_SPLINE_SURFACE_WITH_KNOTS((2,2),(3,3),(0.710192959008365,1.),(0.590910950629467,
0.60808458519997),.UNSPECIFIED.)
GEOMETRIC_REPRESENTATION_ITEM()
RATIONAL_B_SPLINE_SURFACE(((0.990053454406188,0.987313720921966,0.987472672298934),
(0.990053454406188,0.987313720921966,0.987472672298934)))
REPRESENTATION_ITEM('')
SURFACE()
);
#3614=(
BOUNDED_SURFACE()
B_SPLINE_SURFACE(1,2,((#155921,#155922,#155923),(#155924,#155925,#155926)),
 .UNSPECIFIED.,.F.,.F.,.F.)
B_SPLINE_SURFACE_WITH_KNOTS((2,2),(3,3),(0.710318915640004,1.),(0.125066077454536,
0.142578551421364),.UNSPECIFIED.)
GEOMETRIC_REPRESENTATION_ITEM()
RATIONAL_B_SPLINE_SURFACE(((0.990621203777022,0.993706096834649,0.999805186472059),
(0.990621203777022,0.993706096834649,0.999805186472059)))
REPRESENTATION_ITEM('')
SURFACE()
);
#3615=(
BOUNDED_SURFACE()
B_SPLINE_SURFACE(1,2,((#155928,#155929,#155930),(#155931,#155932,#155933)),
 .UNSPECIFIED.,.F.,.F.,.F.)
B_SPLINE_SURFACE_WITH_KNOTS((2,2),(3,3),(0.71019295900844,1.),(0.590910950629373,
0.608084585199971),.UNSPECIFIED.)
GEOMETRIC_REPRESENTATION_ITEM()
RATIONAL_B_SPLINE_SURFACE(((0.990053454406218,0.987313720921966,0.987472672298934),
(0.990053454406218,0.987313720921966,0.987472672298934)))
REPRESENTATION_ITEM('')
SURFACE()
);
#3616=(
BOUNDED_SURFACE()
B_SPLINE_SURFACE(1,2,((#155935,#155936,#155937,#155938,#155939,#155940,
#155941),(#155942,#155943,#155944,#155945,#155946,#155947,#155948)),
 .UNSPECIFIED.,.F.,.F.,.F.)
B_SPLINE_SURFACE_WITH_KNOTS((2,2),(3,2,2,3),(0.,0.211537324447063),(0.642404283483249,
0.642578551421311,0.642857142857143,0.660005345227472),.UNSPECIFIED.)
GEOMETRIC_REPRESENTATION_ITEM()
RATIONAL_B_SPLINE_SURFACE(((0.999805186472022,0.999805186472022,0.999805186472022,
0.999902211834776,1.,0.993980822699462,0.990851751371594),(0.999805186472022,
0.999805186472022,0.999805186472022,0.999902211834776,1.,0.993980822699462,
0.990851751371594)))
REPRESENTATION_ITEM('')
SURFACE()
);
#3617=(
BOUNDED_SURFACE()
B_SPLINE_SURFACE(1,2,((#155955,#155956,#155957,#155958,#155959),(#155960,
#155961,#155962,#155963,#155964),(#155965,#155966,#155967,#155968,#155969)),
 .UNSPECIFIED.,.F.,.F.,.F.)
B_SPLINE_SURFACE_WITH_KNOTS((2,1,2),(3,2,3),(-0.00211445385587017,0.,0.211445385587017),
(0.0724436332512423,0.0909109506295946,0.0921216909780094),
 .UNSPECIFIED.)
GEOMETRIC_REPRESENTATION_ITEM()
RATIONAL_B_SPLINE_SURFACE(((0.999297534414571,0.992999570883536,0.990053454406147,
0.990053454406147,0.990053454406147),(0.999297534414571,0.992999570883536,
0.990053454406147,0.990053454406147,0.990053454406147),(0.999297534414571,
0.992999570883536,0.990053454406147,0.990053454406147,0.990053454406147)))
REPRESENTATION_ITEM('')
SURFACE()
);
#3618=(
BOUNDED_SURFACE()
B_SPLINE_SURFACE(1,2,((#155976,#155977,#155978,#155979,#155980,#155981,
#155982),(#155983,#155984,#155985,#155986,#155987,#155988,#155989),(#155990,
#155991,#155992,#155993,#155994,#155995,#155996)),.UNSPECIFIED.,.F.,.F.,
 .F.)
B_SPLINE_SURFACE_WITH_KNOTS((2,1,2),(3,2,2,3),(-0.00211537324447033,0.,
0.211537324447033),(0.642404283483253,0.642578551421314,0.642857142857143,
0.660005345227463),.UNSPECIFIED.)
GEOMETRIC_REPRESENTATION_ITEM()
RATIONAL_B_SPLINE_SURFACE(((0.999805186472024,0.999805186472024,0.999805186472024,
0.999902211834777,1.,0.993980822699465,0.990851751371597),(0.999805186472024,
0.999805186472024,0.999805186472024,0.999902211834777,1.,0.993980822699465,
0.990851751371597),(0.999805186472024,0.999805186472024,0.999805186472024,
0.999902211834777,1.,0.993980822699465,0.990851751371597)))
REPRESENTATION_ITEM('')
SURFACE()
);
#3619=(
BOUNDED_SURFACE()
B_SPLINE_SURFACE(1,2,((#155998,#155999,#156000,#156001,#156002),(#156003,
#156004,#156005,#156006,#156007),(#156008,#156009,#156010,#156011,#156012)),
 .UNSPECIFIED.,.F.,.F.,.F.)
B_SPLINE_SURFACE_WITH_KNOTS((2,1,2),(3,2,3),(-0.00211445385587015,0.,0.211445385587015),
(0.0724436330381796,0.0909109506295945,0.0921216911828342),
 .UNSPECIFIED.)
GEOMETRIC_REPRESENTATION_ITEM()
RATIONAL_B_SPLINE_SURFACE(((0.999297534559893,0.992999570917526,0.990053454406147,
0.990053454406147,0.990053454406147),(0.999297534559893,0.992999570917526,
0.990053454406147,0.990053454406147,0.990053454406147),(0.999297534559893,
0.992999570917527,0.990053454406147,0.990053454406147,0.990053454406147)))
REPRESENTATION_ITEM('')
SURFACE()
);
#3620=(
BOUNDED_SURFACE()
B_SPLINE_SURFACE(1,2,((#156019,#156020,#156021,#156022,#156023,#156024,
#156025),(#156026,#156027,#156028,#156029,#156030,#156031,#156032),(#156033,
#156034,#156035,#156036,#156037,#156038,#156039)),.UNSPECIFIED.,.F.,.F.,
 .F.)
B_SPLINE_SURFACE_WITH_KNOTS((2,1,2),(3,2,2,3),(-0.00211537324446618,0.,
0.211537324446618),(0.642404283483302,0.642578551421363,0.642857142857143,
0.660005345227472),.UNSPECIFIED.)
GEOMETRIC_REPRESENTATION_ITEM()
RATIONAL_B_SPLINE_SURFACE(((0.999805186472058,0.999805186472058,0.999805186472058,
0.999902211834794,1.,0.993980822699462,0.990851751371594),(0.999805186472058,
0.999805186472058,0.999805186472058,0.999902211834794,1.,0.993980822699462,
0.990851751371594),(0.999805186472058,0.999805186472058,0.999805186472058,
0.999902211834794,1.,0.993980822699462,0.990851751371594)))
REPRESENTATION_ITEM('')
SURFACE()
);
#3621=(
BOUNDED_SURFACE()
B_SPLINE_SURFACE(1,2,((#156041,#156042,#156043,#156044,#156045),(#156046,
#156047,#156048,#156049,#156050),(#156051,#156052,#156053,#156054,#156055)),
 .UNSPECIFIED.,.F.,.F.,.F.)
B_SPLINE_SURFACE_WITH_KNOTS((2,1,2),(3,2,3),(-0.00211445385587009,0.,0.211445385587009),
(0.0724436337108673,0.0909109506295944,0.0921216910718328),
 .UNSPECIFIED.)
GEOMETRIC_REPRESENTATION_ITEM()
RATIONAL_B_SPLINE_SURFACE(((0.999297534101077,0.992999570810212,0.990053454406147,
0.990053454406147,0.990053454406147),(0.999297534101077,0.992999570810212,
0.990053454406147,0.990053454406147,0.990053454406147),(0.999297534101077,
0.992999570810212,0.990053454406147,0.990053454406147,0.990053454406147)))
REPRESENTATION_ITEM('')
SURFACE()
);
#3622=(
BOUNDED_SURFACE()
B_SPLINE_SURFACE(1,2,((#156062,#156063,#156064,#156065,#156066,#156067,
#156068),(#156069,#156070,#156071,#156072,#156073,#156074,#156075),(#156076,
#156077,#156078,#156079,#156080,#156081,#156082)),.UNSPECIFIED.,.F.,.F.,
 .F.)
B_SPLINE_SURFACE_WITH_KNOTS((2,1,2),(3,2,2,3),(-0.0021153732444663,0.,0.21153732444663),
(0.642404283483301,0.642578551421362,0.642857142857143,0.660005345227463),
 .UNSPECIFIED.)
GEOMETRIC_REPRESENTATION_ITEM()
RATIONAL_B_SPLINE_SURFACE(((0.999805186472057,0.999805186472057,0.999805186472057,
0.999902211834794,1.,0.993980822699465,0.990851751371597),(0.999805186472057,
0.999805186472057,0.999805186472057,0.999902211834794,1.,0.993980822699465,
0.990851751371597),(0.999805186472057,0.999805186472057,0.999805186472057,
0.999902211834794,1.,0.993980822699465,0.990851751371597)))
REPRESENTATION_ITEM('')
SURFACE()
);
#3623=(
BOUNDED_SURFACE()
B_SPLINE_SURFACE(1,2,((#156084,#156085,#156086,#156087,#156088),(#156089,
#156090,#156091,#156092,#156093),(#156094,#156095,#156096,#156097,#156098)),
 .UNSPECIFIED.,.F.,.F.,.F.)
B_SPLINE_SURFACE_WITH_KNOTS((2,1,2),(3,2,3),(-0.00211445385587011,0.,0.211445385587011),
(0.0724436338120045,0.0909109506295944,0.0921216909413642),
 .UNSPECIFIED.)
GEOMETRIC_REPRESENTATION_ITEM()
RATIONAL_B_SPLINE_SURFACE(((0.999297534032094,0.992999570794077,0.990053454406147,
0.990053454406147,0.990053454406147),(0.999297534032094,0.992999570794077,
0.990053454406147,0.990053454406147,0.990053454406147),(0.999297534032094,
0.992999570794077,0.990053454406147,0.990053454406147,0.990053454406147)))
REPRESENTATION_ITEM('')
SURFACE()
);
#3624=(
BOUNDED_SURFACE()
B_SPLINE_SURFACE(1,2,((#156105,#156106,#156107,#156108,#156109,#156110,
#156111),(#156112,#156113,#156114,#156115,#156116,#156117,#156118),(#156119,
#156120,#156121,#156122,#156123,#156124,#156125)),.UNSPECIFIED.,.F.,.F.,
 .F.)
B_SPLINE_SURFACE_WITH_KNOTS((2,1,2),(3,2,2,3),(-0.00211537324446619,0.,
0.211537324446619),(0.642404283483302,0.642578551421363,0.642857142857143,
0.660005345227463),.UNSPECIFIED.)
GEOMETRIC_REPRESENTATION_ITEM()
RATIONAL_B_SPLINE_SURFACE(((0.999805186472058,0.999805186472058,0.999805186472058,
0.999902211834794,1.,0.993980822699465,0.990851751371597),(0.999805186472058,
0.999805186472058,0.999805186472058,0.999902211834794,1.,0.993980822699465,
0.990851751371597),(0.999805186472058,0.999805186472058,0.999805186472058,
0.999902211834794,1.,0.993980822699465,0.990851751371597)))
REPRESENTATION_ITEM('')
SURFACE()
);
#3625=(
BOUNDED_SURFACE()
B_SPLINE_SURFACE(1,2,((#156127,#156128,#156129,#156130,#156131),(#156132,
#156133,#156134,#156135,#156136),(#156137,#156138,#156139,#156140,#156141)),
 .UNSPECIFIED.,.F.,.F.,.F.)
B_SPLINE_SURFACE_WITH_KNOTS((2,1,2),(3,2,3),(-0.00211445385587008,0.,0.211445385587008),
(0.0724436337233711,0.0909109506295944,0.092121691069622),.UNSPECIFIED.)
GEOMETRIC_REPRESENTATION_ITEM()
RATIONAL_B_SPLINE_SURFACE(((0.999297534092548,0.992999570808217,0.990053454406147,
0.990053454406147,0.990053454406147),(0.999297534092548,0.992999570808217,
0.990053454406147,0.990053454406147,0.990053454406147),(0.999297534092548,
0.992999570808217,0.990053454406147,0.990053454406147,0.990053454406147)))
REPRESENTATION_ITEM('')
SURFACE()
);
#3626=(
BOUNDED_SURFACE()
B_SPLINE_SURFACE(1,2,((#156148,#156149,#156150,#156151,#156152,#156153,
#156154),(#156155,#156156,#156157,#156158,#156159,#156160,#156161),(#156162,
#156163,#156164,#156165,#156166,#156167,#156168)),.UNSPECIFIED.,.F.,.F.,
 .F.)
B_SPLINE_SURFACE_WITH_KNOTS((2,1,2),(3,2,2,3),(-0.00211537324446629,0.,
0.211537324446629),(0.642404283483301,0.642578551421362,0.642857142857143,
0.660005345227463),.UNSPECIFIED.)
GEOMETRIC_REPRESENTATION_ITEM()
RATIONAL_B_SPLINE_SURFACE(((0.999805186472057,0.999805186472057,0.999805186472057,
0.999902211834794,1.,0.993980822699465,0.990851751371597),(0.999805186472057,
0.999805186472057,0.999805186472057,0.999902211834794,1.,0.993980822699465,
0.990851751371597),(0.999805186472057,0.999805186472057,0.999805186472057,
0.999902211834794,1.,0.993980822699465,0.990851751371597)))
REPRESENTATION_ITEM('')
SURFACE()
);
#3627=(
BOUNDED_SURFACE()
B_SPLINE_SURFACE(1,2,((#156170,#156171,#156172,#156173,#156174),(#156175,
#156176,#156177,#156178,#156179),(#156180,#156181,#156182,#156183,#156184)),
 .UNSPECIFIED.,.F.,.F.,.F.)
B_SPLINE_SURFACE_WITH_KNOTS((2,1,2),(3,2,3),(-0.0021144538558701,0.,0.21144538558701),
(0.0724436329521793,0.0909109506295945,0.092121691285746),.UNSPECIFIED.)
GEOMETRIC_REPRESENTATION_ITEM()
RATIONAL_B_SPLINE_SURFACE(((0.999297534618552,0.992999570931246,0.990053454406147,
0.990053454406147,0.990053454406147),(0.999297534618552,0.992999570931246,
0.990053454406147,0.990053454406147,0.990053454406147),(0.999297534618552,
0.992999570931246,0.990053454406147,0.990053454406147,0.990053454406147)))
REPRESENTATION_ITEM('')
SURFACE()
);
#3628=(
BOUNDED_SURFACE()
B_SPLINE_SURFACE(1,2,((#156191,#156192,#156193,#156194,#156195,#156196,
#156197),(#156198,#156199,#156200,#156201,#156202,#156203,#156204),(#156205,
#156206,#156207,#156208,#156209,#156210,#156211)),.UNSPECIFIED.,.F.,.F.,
 .F.)
B_SPLINE_SURFACE_WITH_KNOTS((2,1,2),(3,2,2,3),(-0.00211537324446949,0.,
0.211537324446949),(0.642404283483263,0.642578551421324,0.642857142857143,
0.660005345227463),.UNSPECIFIED.)
GEOMETRIC_REPRESENTATION_ITEM()
RATIONAL_B_SPLINE_SURFACE(((0.999805186472031,0.999805186472031,0.999805186472031,
0.999902211834781,1.,0.993980822699465,0.990851751371597),(0.999805186472031,
0.999805186472031,0.999805186472031,0.999902211834781,1.,0.993980822699465,
0.990851751371597),(0.999805186472031,0.999805186472031,0.999805186472031,
0.999902211834781,1.,0.993980822699465,0.990851751371597)))
REPRESENTATION_ITEM('')
SURFACE()
);
#3629=(
BOUNDED_SURFACE()
B_SPLINE_SURFACE(1,2,((#156213,#156214,#156215,#156216,#156217),(#156218,
#156219,#156220,#156221,#156222),(#156223,#156224,#156225,#156226,#156227)),
 .UNSPECIFIED.,.F.,.F.,.F.)
B_SPLINE_SURFACE_WITH_KNOTS((2,1,2),(3,2,3),(-0.00211445385587014,0.,0.211445385587014),
(0.0724436336432635,0.0909109506295945,0.0921216911046539),
 .UNSPECIFIED.)
GEOMETRIC_REPRESENTATION_ITEM()
RATIONAL_B_SPLINE_SURFACE(((0.999297534147187,0.992999570820996,0.990053454406147,
0.990053454406147,0.990053454406147),(0.999297534147187,0.992999570820996,
0.990053454406147,0.990053454406147,0.990053454406147),(0.999297534147187,
0.992999570820996,0.990053454406147,0.990053454406147,0.990053454406147)))
REPRESENTATION_ITEM('')
SURFACE()
);
#3630=(
BOUNDED_SURFACE()
B_SPLINE_SURFACE(1,2,((#156234,#156235,#156236,#156237,#156238,#156239,
#156240),(#156241,#156242,#156243,#156244,#156245,#156246,#156247),(#156248,
#156249,#156250,#156251,#156252,#156253,#156254)),.UNSPECIFIED.,.F.,.F.,
 .F.)
B_SPLINE_SURFACE_WITH_KNOTS((2,1,2),(3,2,2,3),(-0.00211537324446956,0.,
0.211537324446956),(0.642404283483262,0.642578551421323,0.642857142857143,
0.660005345227472),.UNSPECIFIED.)
GEOMETRIC_REPRESENTATION_ITEM()
RATIONAL_B_SPLINE_SURFACE(((0.999805186472031,0.999805186472031,0.999805186472031,
0.99990221183478,1.,0.993980822699462,0.990851751371594),(0.999805186472031,
0.999805186472031,0.999805186472031,0.99990221183478,1.,0.993980822699462,
0.990851751371594),(0.999805186472031,0.999805186472031,0.999805186472031,
0.99990221183478,1.,0.993980822699462,0.990851751371594)))
REPRESENTATION_ITEM('')
SURFACE()
);
#3631=(
BOUNDED_SURFACE()
B_SPLINE_SURFACE(1,2,((#156256,#156257,#156258,#156259,#156260),(#156261,
#156262,#156263,#156264,#156265),(#156266,#156267,#156268,#156269,#156270)),
 .UNSPECIFIED.,.F.,.F.,.F.)
B_SPLINE_SURFACE_WITH_KNOTS((2,1,2),(3,2,3),(-0.00211445385587015,0.,0.211445385587015),
(0.0724436332002964,0.0909109506295945,0.0921216910412671),
 .UNSPECIFIED.)
GEOMETRIC_REPRESENTATION_ITEM()
RATIONAL_B_SPLINE_SURFACE(((0.99929753444932,0.992999570891664,0.990053454406147,
0.990053454406147,0.990053454406147),(0.99929753444932,0.992999570891664,
0.990053454406147,0.990053454406147,0.990053454406147),(0.99929753444932,
0.992999570891664,0.990053454406147,0.990053454406147,0.990053454406147)))
REPRESENTATION_ITEM('')
SURFACE()
);
#3632=(
BOUNDED_SURFACE()
B_SPLINE_SURFACE(1,2,((#156277,#156278,#156279,#156280,#156281,#156282,
#156283),(#156284,#156285,#156286,#156287,#156288,#156289,#156290),(#156291,
#156292,#156293,#156294,#156295,#156296,#156297)),.UNSPECIFIED.,.F.,.F.,
 .F.)
B_SPLINE_SURFACE_WITH_KNOTS((2,1,2),(3,2,2,3),(-0.00211537324446625,0.,
0.211537324446625),(0.642404283483301,0.642578551421362,0.642857142857143,
0.660005345227463),.UNSPECIFIED.)
GEOMETRIC_REPRESENTATION_ITEM()
RATIONAL_B_SPLINE_SURFACE(((0.999805186472057,0.999805186472057,0.999805186472057,
0.999902211834794,1.,0.993980822699465,0.990851751371597),(0.999805186472057,
0.999805186472057,0.999805186472057,0.999902211834794,1.,0.993980822699465,
0.990851751371597),(0.999805186472057,0.999805186472057,0.999805186472057,
0.999902211834794,1.,0.993980822699465,0.990851751371597)))
REPRESENTATION_ITEM('')
SURFACE()
);
#3633=(
BOUNDED_SURFACE()
B_SPLINE_SURFACE(1,2,((#156299,#156300,#156301,#156302,#156303),(#156304,
#156305,#156306,#156307,#156308),(#156309,#156310,#156311,#156312,#156313)),
 .UNSPECIFIED.,.F.,.F.,.F.)
B_SPLINE_SURFACE_WITH_KNOTS((2,1,2),(3,2,3),(-0.00211445385587014,0.,0.211445385587014),
(0.0724436338901995,0.0909109506295945,0.0921216908675382),
 .UNSPECIFIED.)
GEOMETRIC_REPRESENTATION_ITEM()
RATIONAL_B_SPLINE_SURFACE(((0.99929753397876,0.992999570781603,0.990053454406147,
0.990053454406147,0.990053454406147),(0.99929753397876,0.992999570781603,
0.990053454406147,0.990053454406147,0.990053454406147),(0.99929753397876,
0.992999570781603,0.990053454406147,0.990053454406147,0.990053454406147)))
REPRESENTATION_ITEM('')
SURFACE()
);
#3634=(
BOUNDED_SURFACE()
B_SPLINE_SURFACE(1,2,((#156320,#156321,#156322,#156323,#156324,#156325,
#156326),(#156327,#156328,#156329,#156330,#156331,#156332,#156333),(#156334,
#156335,#156336,#156337,#156338,#156339,#156340)),.UNSPECIFIED.,.F.,.F.,
 .F.)
B_SPLINE_SURFACE_WITH_KNOTS((2,1,2),(3,2,2,3),(-0.00211537324446629,0.,
0.211537324446629),(0.642404283483301,0.642578551421362,0.642857142857143,
0.660005345227463),.UNSPECIFIED.)
GEOMETRIC_REPRESENTATION_ITEM()
RATIONAL_B_SPLINE_SURFACE(((0.999805186472057,0.999805186472057,0.999805186472057,
0.999902211834794,1.,0.993980822699465,0.990851751371597),(0.999805186472057,
0.999805186472057,0.999805186472057,0.999902211834794,1.,0.993980822699465,
0.990851751371597),(0.999805186472057,0.999805186472057,0.999805186472057,
0.999902211834794,1.,0.993980822699465,0.990851751371597)))
REPRESENTATION_ITEM('')
SURFACE()
);
#3635=(
BOUNDED_SURFACE()
B_SPLINE_SURFACE(1,2,((#156342,#156343,#156344,#156345,#156346),(#156347,
#156348,#156349,#156350,#156351),(#156352,#156353,#156354,#156355,#156356)),
 .UNSPECIFIED.,.F.,.F.,.F.)
B_SPLINE_SURFACE_WITH_KNOTS((2,1,2),(3,2,3),(-0.00211445385587012,0.,0.211445385587012),
(0.0724436330728422,0.0909109506295943,0.092121691180342),.UNSPECIFIED.)
GEOMETRIC_REPRESENTATION_ITEM()
RATIONAL_B_SPLINE_SURFACE(((0.999297534536251,0.992999570911997,0.990053454406147,
0.990053454406147,0.990053454406147),(0.999297534536251,0.992999570911997,
0.990053454406147,0.990053454406147,0.990053454406147),(0.999297534536251,
0.992999570911997,0.990053454406147,0.990053454406147,0.990053454406147)))
REPRESENTATION_ITEM('')
SURFACE()
);
#3636=(
BOUNDED_SURFACE()
B_SPLINE_SURFACE(1,2,((#156363,#156364,#156365,#156366,#156367,#156368,
#156369),(#156370,#156371,#156372,#156373,#156374,#156375,#156376),(#156377,
#156378,#156379,#156380,#156381,#156382,#156383)),.UNSPECIFIED.,.F.,.F.,
 .F.)
B_SPLINE_SURFACE_WITH_KNOTS((2,1,2),(3,2,2,3),(-0.00211537324446862,0.,
0.211537324446862),(0.642404283483273,0.642578551421334,0.642857142857143,
0.660005345227463),.UNSPECIFIED.)
GEOMETRIC_REPRESENTATION_ITEM()
RATIONAL_B_SPLINE_SURFACE(((0.999805186472038,0.999805186472038,0.999805186472038,
0.999902211834784,1.,0.993980822699465,0.990851751371597),(0.999805186472038,
0.999805186472038,0.999805186472038,0.999902211834784,1.,0.993980822699465,
0.990851751371597),(0.999805186472038,0.999805186472038,0.999805186472038,
0.999902211834784,1.,0.993980822699465,0.990851751371597)))
REPRESENTATION_ITEM('')
SURFACE()
);
#3637=(
BOUNDED_SURFACE()
B_SPLINE_SURFACE(1,2,((#156385,#156386,#156387,#156388,#156389),(#156390,
#156391,#156392,#156393,#156394),(#156395,#156396,#156397,#156398,#156399)),
 .UNSPECIFIED.,.F.,.F.,.F.)
B_SPLINE_SURFACE_WITH_KNOTS((2,1,2),(3,2,3),(-0.00211445385587008,0.,0.211445385587008),
(0.0724436334874632,0.0909109506295944,0.0921216912916598),
 .UNSPECIFIED.)
GEOMETRIC_REPRESENTATION_ITEM()
RATIONAL_B_SPLINE_SURFACE(((0.999297534253452,0.992999570845852,0.990053454406147,
0.990053454406147,0.990053454406147),(0.999297534253452,0.992999570845852,
0.990053454406147,0.990053454406147,0.990053454406147),(0.999297534253452,
0.992999570845852,0.990053454406147,0.990053454406147,0.990053454406147)))
REPRESENTATION_ITEM('')
SURFACE()
);
#3638=(
BOUNDED_SURFACE()
B_SPLINE_SURFACE(1,2,((#156406,#156407,#156408,#156409,#156410,#156411,
#156412),(#156413,#156414,#156415,#156416,#156417,#156418,#156419),(#156420,
#156421,#156422,#156423,#156424,#156425,#156426)),.UNSPECIFIED.,.F.,.F.,
 .F.)
B_SPLINE_SURFACE_WITH_KNOTS((2,1,2),(3,2,2,3),(-0.00211537324446876,0.,
0.211537324446876),(0.642404283483271,0.642578551421332,0.642857142857143,
0.660005345227463),.UNSPECIFIED.)
GEOMETRIC_REPRESENTATION_ITEM()
RATIONAL_B_SPLINE_SURFACE(((0.999805186472037,0.999805186472037,0.999805186472037,
0.999902211834783,1.,0.993980822699465,0.990851751371597),(0.999805186472037,
0.999805186472037,0.999805186472037,0.999902211834783,1.,0.993980822699465,
0.990851751371597),(0.999805186472037,0.999805186472037,0.999805186472037,
0.999902211834783,1.,0.993980822699465,0.990851751371597)))
REPRESENTATION_ITEM('')
SURFACE()
);
#3639=(
BOUNDED_SURFACE()
B_SPLINE_SURFACE(1,2,((#156428,#156429,#156430,#156431,#156432),(#156433,
#156434,#156435,#156436,#156437),(#156438,#156439,#156440,#156441,#156442)),
 .UNSPECIFIED.,.F.,.F.,.F.)
B_SPLINE_SURFACE_WITH_KNOTS((2,1,2),(3,2,3),(-0.00211445385587004,0.,0.211445385587004),
(0.072443633212248,0.0909109506295932,0.0921216910014061),.UNSPECIFIED.)
GEOMETRIC_REPRESENTATION_ITEM()
RATIONAL_B_SPLINE_SURFACE(((0.999297534441168,0.992999570889758,0.990053454406148,
0.990053454406149,0.990053454406149),(0.999297534441168,0.992999570889758,
0.990053454406148,0.990053454406149,0.990053454406149),(0.999297534441168,
0.992999570889758,0.990053454406148,0.990053454406149,0.990053454406149)))
REPRESENTATION_ITEM('')
SURFACE()
);
#3640=(
BOUNDED_SURFACE()
B_SPLINE_SURFACE(1,2,((#156449,#156450,#156451,#156452,#156453,#156454,
#156455),(#156456,#156457,#156458,#156459,#156460,#156461,#156462),(#156463,
#156464,#156465,#156466,#156467,#156468,#156469)),.UNSPECIFIED.,.F.,.F.,
 .F.)
B_SPLINE_SURFACE_WITH_KNOTS((2,1,2),(3,2,2,3),(-0.00211537324446606,0.,
0.211537324446606),(0.642404283483303,0.642578551421364,0.642857142857143,
0.660005345227464),.UNSPECIFIED.)
GEOMETRIC_REPRESENTATION_ITEM()
RATIONAL_B_SPLINE_SURFACE(((0.999805186472059,0.999805186472059,0.999805186472059,
0.999902211834795,1.,0.993980822699464,0.990851751371597),(0.999805186472059,
0.999805186472059,0.999805186472059,0.999902211834795,1.,0.993980822699464,
0.990851751371597),(0.999805186472059,0.999805186472059,0.999805186472059,
0.999902211834795,1.,0.993980822699464,0.990851751371597)))
REPRESENTATION_ITEM('')
SURFACE()
);
#3641=(
BOUNDED_SURFACE()
B_SPLINE_SURFACE(1,2,((#156471,#156472,#156473,#156474,#156475),(#156476,
#156477,#156478,#156479,#156480),(#156481,#156482,#156483,#156484,#156485)),
 .UNSPECIFIED.,.F.,.F.,.F.)
B_SPLINE_SURFACE_WITH_KNOTS((2,1,2),(3,2,3),(-0.00211445385586999,0.,0.211445385586999),
(0.0724436332301871,0.0909109506295932,0.0921216910227852),
 .UNSPECIFIED.)
GEOMETRIC_REPRESENTATION_ITEM()
RATIONAL_B_SPLINE_SURFACE(((0.999297534428931,0.992999570886895,0.990053454406147,
0.990053454406147,0.990053454406147),(0.999297534428931,0.992999570886895,
0.990053454406147,0.990053454406147,0.990053454406147),(0.999297534428931,
0.992999570886895,0.990053454406147,0.990053454406147,0.990053454406147)))
REPRESENTATION_ITEM('')
SURFACE()
);
#3642=(
BOUNDED_SURFACE()
B_SPLINE_SURFACE(1,2,((#156492,#156493,#156494,#156495,#156496,#156497,
#156498),(#156499,#156500,#156501,#156502,#156503,#156504,#156505),(#156506,
#156507,#156508,#156509,#156510,#156511,#156512)),.UNSPECIFIED.,.F.,.F.,
 .F.)
B_SPLINE_SURFACE_WITH_KNOTS((2,1,2),(3,2,2,3),(-0.00211537324446848,0.,
0.211537324446848),(0.642404283483275,0.642578551421336,0.642857142857143,
0.660005345227473),.UNSPECIFIED.)
GEOMETRIC_REPRESENTATION_ITEM()
RATIONAL_B_SPLINE_SURFACE(((0.99980518647204,0.99980518647204,0.99980518647204,
0.999902211834785,1.,0.993980822699461,0.990851751371593),(0.99980518647204,
0.99980518647204,0.99980518647204,0.999902211834785,1.,0.993980822699461,
0.990851751371593),(0.99980518647204,0.99980518647204,0.99980518647204,
0.999902211834785,1.,0.993980822699461,0.990851751371593)))
REPRESENTATION_ITEM('')
SURFACE()
);
#3643=(
BOUNDED_SURFACE()
B_SPLINE_SURFACE(1,2,((#156514,#156515,#156516,#156517,#156518),(#156519,
#156520,#156521,#156522,#156523),(#156524,#156525,#156526,#156527,#156528)),
 .UNSPECIFIED.,.F.,.F.,.F.)
B_SPLINE_SURFACE_WITH_KNOTS((2,1,2),(3,2,3),(-0.00211445385587003,0.,0.211445385587003),
(0.0724436338956014,0.0909109506295934,0.0921216908414379),
 .UNSPECIFIED.)
GEOMETRIC_REPRESENTATION_ITEM()
RATIONAL_B_SPLINE_SURFACE(((0.999297533975076,0.992999570780741,0.990053454406147,
0.990053454406147,0.990053454406147),(0.999297533975076,0.992999570780741,
0.990053454406147,0.990053454406147,0.990053454406147),(0.999297533975076,
0.992999570780741,0.990053454406147,0.990053454406147,0.990053454406147)))
REPRESENTATION_ITEM('')
SURFACE()
);
#3644=(
BOUNDED_SURFACE()
B_SPLINE_SURFACE(1,2,((#156535,#156536,#156537,#156538,#156539,#156540,
#156541),(#156542,#156543,#156544,#156545,#156546,#156547,#156548),(#156549,
#156550,#156551,#156552,#156553,#156554,#156555)),.UNSPECIFIED.,.F.,.F.,
 .F.)
B_SPLINE_SURFACE_WITH_KNOTS((2,1,2),(3,2,2,3),(-0.0021153732444662,0.,0.21153732444662),
(0.642404283483302,0.642578551421363,0.642857142857143,0.660005345227473),
 .UNSPECIFIED.)
GEOMETRIC_REPRESENTATION_ITEM()
RATIONAL_B_SPLINE_SURFACE(((0.999805186472058,0.999805186472058,0.999805186472058,
0.999902211834794,1.,0.993980822699461,0.990851751371594),(0.999805186472058,
0.999805186472058,0.999805186472058,0.999902211834794,1.,0.993980822699461,
0.990851751371594),(0.999805186472058,0.999805186472058,0.999805186472058,
0.999902211834794,1.,0.993980822699461,0.990851751371594)))
REPRESENTATION_ITEM('')
SURFACE()
);
#3645=(
BOUNDED_SURFACE()
B_SPLINE_SURFACE(1,2,((#156557,#156558,#156559,#156560,#156561),(#156562,
#156563,#156564,#156565,#156566),(#156567,#156568,#156569,#156570,#156571)),
 .UNSPECIFIED.,.F.,.F.,.F.)
B_SPLINE_SURFACE_WITH_KNOTS((2,1,2),(3,2,3),(-0.00211445385587001,0.,0.211445385587001),
(0.0724436337408151,0.0909109506295932,0.0921216910221661),
 .UNSPECIFIED.)
GEOMETRIC_REPRESENTATION_ITEM()
RATIONAL_B_SPLINE_SURFACE(((0.999297534080651,0.992999570805435,0.990053454406148,
0.990053454406148,0.990053454406148),(0.999297534080651,0.992999570805435,
0.990053454406148,0.990053454406148,0.990053454406148),(0.999297534080651,
0.992999570805435,0.990053454406148,0.990053454406148,0.990053454406148)))
REPRESENTATION_ITEM('')
SURFACE()
);
#3646=(
BOUNDED_SURFACE()
B_SPLINE_SURFACE(1,2,((#156578,#156579,#156580,#156581,#156582,#156583,
#156584),(#156585,#156586,#156587,#156588,#156589,#156590,#156591),(#156592,
#156593,#156594,#156595,#156596,#156597,#156598)),.UNSPECIFIED.,.F.,.F.,
 .F.)
B_SPLINE_SURFACE_WITH_KNOTS((2,1,2),(3,2,2,3),(-0.00211537324446836,0.,
0.211537324446836),(0.642404283483276,0.642578551421337,0.642857142857143,
0.660005345227464),.UNSPECIFIED.)
GEOMETRIC_REPRESENTATION_ITEM()
RATIONAL_B_SPLINE_SURFACE(((0.99980518647204,0.99980518647204,0.99980518647204,
0.999902211834785,1.,0.993980822699464,0.990851751371596),(0.99980518647204,
0.99980518647204,0.99980518647204,0.999902211834785,1.,0.993980822699464,
0.990851751371596),(0.99980518647204,0.99980518647204,0.99980518647204,
0.999902211834785,1.,0.993980822699464,0.990851751371596)))
REPRESENTATION_ITEM('')
SURFACE()
);
#3647=(
BOUNDED_SURFACE()
B_SPLINE_SURFACE(1,2,((#156600,#156601,#156602,#156603,#156604),(#156605,
#156606,#156607,#156608,#156609),(#156610,#156611,#156612,#156613,#156614)),
 .UNSPECIFIED.,.F.,.F.,.F.)
B_SPLINE_SURFACE_WITH_KNOTS((2,1,2),(3,2,3),(-0.00211445385587002,0.,0.211445385587002),
(0.0724436332573611,0.0909109506295931,0.0921216909806424),
 .UNSPECIFIED.)
GEOMETRIC_REPRESENTATION_ITEM()
RATIONAL_B_SPLINE_SURFACE(((0.999297534410397,0.992999570882561,0.990053454406148,
0.990053454406148,0.990053454406148),(0.999297534410397,0.992999570882561,
0.990053454406148,0.990053454406148,0.990053454406148),(0.999297534410397,
0.992999570882561,0.990053454406148,0.990053454406148,0.990053454406148)))
REPRESENTATION_ITEM('')
SURFACE()
);
#3648=(
BOUNDED_SURFACE()
B_SPLINE_SURFACE(1,2,((#156621,#156622,#156623,#156624,#156625,#156626,
#156627),(#156628,#156629,#156630,#156631,#156632,#156633,#156634),(#156635,
#156636,#156637,#156638,#156639,#156640,#156641)),.UNSPECIFIED.,.F.,.F.,
 .F.)
B_SPLINE_SURFACE_WITH_KNOTS((2,1,2),(3,2,2,3),(-0.00211537324446873,0.,
0.211537324446873),(0.642404283483272,0.642578551421333,0.642857142857143,
0.660005345227464),.UNSPECIFIED.)
GEOMETRIC_REPRESENTATION_ITEM()
RATIONAL_B_SPLINE_SURFACE(((0.999805186472037,0.999805186472037,0.999805186472037,
0.999902211834784,1.,0.993980822699464,0.990851751371597),(0.999805186472037,
0.999805186472037,0.999805186472037,0.999902211834784,1.,0.993980822699464,
0.990851751371597),(0.999805186472037,0.999805186472037,0.999805186472037,
0.999902211834784,1.,0.993980822699464,0.990851751371596)))
REPRESENTATION_ITEM('')
SURFACE()
);
#3649=(
BOUNDED_SURFACE()
B_SPLINE_SURFACE(1,2,((#156643,#156644,#156645,#156646,#156647),(#156648,
#156649,#156650,#156651,#156652),(#156653,#156654,#156655,#156656,#156657)),
 .UNSPECIFIED.,.F.,.F.,.F.)
B_SPLINE_SURFACE_WITH_KNOTS((2,1,2),(3,2,3),(-0.00211445385587002,0.,0.211445385587002),
(0.0724436333091787,0.0909109506295932,0.0921216909179953),
 .UNSPECIFIED.)
GEOMETRIC_REPRESENTATION_ITEM()
RATIONAL_B_SPLINE_SURFACE(((0.999297534375055,0.992999570874294,0.990053454406148,
0.990053454406148,0.990053454406148),(0.999297534375055,0.992999570874294,
0.990053454406148,0.990053454406148,0.990053454406148),(0.999297534375055,
0.992999570874294,0.990053454406148,0.990053454406148,0.990053454406148)))
REPRESENTATION_ITEM('')
SURFACE()
);
#3650=(
BOUNDED_SURFACE()
B_SPLINE_SURFACE(1,2,((#156664,#156665,#156666,#156667,#156668,#156669,
#156670),(#156671,#156672,#156673,#156674,#156675,#156676,#156677),(#156678,
#156679,#156680,#156681,#156682,#156683,#156684)),.UNSPECIFIED.,.F.,.F.,
 .F.)
B_SPLINE_SURFACE_WITH_KNOTS((2,1,2),(3,2,2,3),(-0.00211537324446836,0.,
0.211537324446836),(0.642404283483276,0.642578551421337,0.642857142857143,
0.660005345227473),.UNSPECIFIED.)
GEOMETRIC_REPRESENTATION_ITEM()
RATIONAL_B_SPLINE_SURFACE(((0.99980518647204,0.99980518647204,0.99980518647204,
0.999902211834785,1.,0.993980822699461,0.990851751371593),(0.99980518647204,
0.99980518647204,0.99980518647204,0.999902211834785,1.,0.993980822699461,
0.990851751371593),(0.99980518647204,0.99980518647204,0.99980518647204,
0.999902211834785,1.,0.993980822699461,0.990851751371593)))
REPRESENTATION_ITEM('')
SURFACE()
);
#3651=(
BOUNDED_SURFACE()
B_SPLINE_SURFACE(1,2,((#156686,#156687,#156688,#156689,#156690),(#156691,
#156692,#156693,#156694,#156695),(#156696,#156697,#156698,#156699,#156700)),
 .UNSPECIFIED.,.F.,.F.,.F.)
B_SPLINE_SURFACE_WITH_KNOTS((2,1,2),(3,2,3),(-0.00211445385587004,0.,0.211445385587004),
(0.0724436339056056,0.0909109506295934,0.0921216908356061),
 .UNSPECIFIED.)
GEOMETRIC_REPRESENTATION_ITEM()
RATIONAL_B_SPLINE_SURFACE(((0.999297533968253,0.992999570779146,0.990053454406148,
0.990053454406148,0.990053454406148),(0.999297533968253,0.992999570779146,
0.990053454406148,0.990053454406148,0.990053454406148),(0.999297533968253,
0.992999570779145,0.990053454406148,0.990053454406148,0.990053454406148)))
REPRESENTATION_ITEM('')
SURFACE()
);
#3652=(
BOUNDED_SURFACE()
B_SPLINE_SURFACE(1,2,((#156707,#156708,#156709,#156710,#156711,#156712,
#156713),(#156714,#156715,#156716,#156717,#156718,#156719,#156720),(#156721,
#156722,#156723,#156724,#156725,#156726,#156727)),.UNSPECIFIED.,.F.,.F.,
 .F.)
B_SPLINE_SURFACE_WITH_KNOTS((2,1,2),(3,2,2,3),(-0.00211537324446615,0.,
0.211537324446615),(0.642404283483302,0.642578551421363,0.642857142857143,
0.660005345227464),.UNSPECIFIED.)
GEOMETRIC_REPRESENTATION_ITEM()
RATIONAL_B_SPLINE_SURFACE(((0.999805186472058,0.999805186472058,0.999805186472058,
0.999902211834794,1.,0.993980822699464,0.990851751371597),(0.999805186472058,
0.999805186472058,0.999805186472058,0.999902211834794,1.,0.993980822699464,
0.990851751371597),(0.999805186472058,0.999805186472058,0.999805186472058,
0.999902211834794,1.,0.993980822699464,0.990851751371597)))
REPRESENTATION_ITEM('')
SURFACE()
);
#3653=(
BOUNDED_SURFACE()
B_SPLINE_SURFACE(1,2,((#156729,#156730,#156731,#156732,#156733),(#156734,
#156735,#156736,#156737,#156738),(#156739,#156740,#156741,#156742,#156743)),
 .UNSPECIFIED.,.F.,.F.,.F.)
B_SPLINE_SURFACE_WITH_KNOTS((2,1,2),(3,2,3),(-0.00211445385587003,0.,0.211445385587003),
(0.0724436330770667,0.0909109506295932,0.0921216911365676),
 .UNSPECIFIED.)
GEOMETRIC_REPRESENTATION_ITEM()
RATIONAL_B_SPLINE_SURFACE(((0.99929753453337,0.992999570911323,0.990053454406148,
0.990053454406149,0.990053454406149),(0.99929753453337,0.992999570911323,
0.990053454406148,0.990053454406149,0.990053454406149),(0.99929753453337,
0.992999570911323,0.990053454406148,0.990053454406149,0.990053454406149)))
REPRESENTATION_ITEM('')
SURFACE()
);
#3654=(
BOUNDED_SURFACE()
B_SPLINE_SURFACE(1,2,((#156750,#156751,#156752,#156753,#156754,#156755,
#156756),(#156757,#156758,#156759,#156760,#156761,#156762,#156763),(#156764,
#156765,#156766,#156767,#156768,#156769,#156770)),.UNSPECIFIED.,.F.,.F.,
 .F.)
B_SPLINE_SURFACE_WITH_KNOTS((2,1,2),(3,2,2,3),(-0.00211537324446882,0.,
0.211537324446882),(0.642404283483271,0.642578551421332,0.642857142857143,
0.660005345227473),.UNSPECIFIED.)
GEOMETRIC_REPRESENTATION_ITEM()
RATIONAL_B_SPLINE_SURFACE(((0.999805186472037,0.999805186472037,0.999805186472037,
0.999902211834783,1.,0.993980822699461,0.990851751371593),(0.999805186472037,
0.999805186472037,0.999805186472037,0.999902211834783,1.,0.993980822699461,
0.990851751371593),(0.999805186472037,0.999805186472037,0.999805186472037,
0.999902211834783,1.,0.993980822699461,0.990851751371593)))
REPRESENTATION_ITEM('')
SURFACE()
);
#3655=(
BOUNDED_SURFACE()
B_SPLINE_SURFACE(1,2,((#156772,#156773,#156774,#156775,#156776),(#156777,
#156778,#156779,#156780,#156781),(#156782,#156783,#156784,#156785,#156786)),
 .UNSPECIFIED.,.F.,.F.,.F.)
B_SPLINE_SURFACE_WITH_KNOTS((2,1,2),(3,2,3),(-0.00211445385587001,0.,0.211445385587001),
(0.0724436338307542,0.0909109506295933,0.0921216909422942),
 .UNSPECIFIED.)
GEOMETRIC_REPRESENTATION_ITEM()
RATIONAL_B_SPLINE_SURFACE(((0.999297534019306,0.992999570791086,0.990053454406148,
0.990053454406148,0.990053454406148),(0.999297534019306,0.992999570791086,
0.990053454406148,0.990053454406148,0.990053454406148),(0.999297534019306,
0.992999570791086,0.990053454406148,0.990053454406148,0.990053454406148)))
REPRESENTATION_ITEM('')
SURFACE()
);
#3656=(
BOUNDED_SURFACE()
B_SPLINE_SURFACE(1,2,((#156793,#156794,#156795,#156796,#156797,#156798,
#156799),(#156800,#156801,#156802,#156803,#156804,#156805,#156806),(#156807,
#156808,#156809,#156810,#156811,#156812,#156813)),.UNSPECIFIED.,.F.,.F.,
 .F.)
B_SPLINE_SURFACE_WITH_KNOTS((2,1,2),(3,2,2,3),(-0.00211537324446608,0.,
0.211537324446608),(0.642404283483303,0.642578551421364,0.642857142857143,
0.660005345227473),.UNSPECIFIED.)
GEOMETRIC_REPRESENTATION_ITEM()
RATIONAL_B_SPLINE_SURFACE(((0.999805186472059,0.999805186472059,0.999805186472059,
0.999902211834795,1.,0.993980822699461,0.990851751371594),(0.999805186472059,
0.999805186472059,0.999805186472059,0.999902211834795,1.,0.993980822699461,
0.990851751371594),(0.999805186472059,0.999805186472059,0.999805186472059,
0.999902211834795,1.,0.993980822699461,0.990851751371593)))
REPRESENTATION_ITEM('')
SURFACE()
);
#3657=(
BOUNDED_SURFACE()
B_SPLINE_SURFACE(1,2,((#156815,#156816,#156817,#156818,#156819),(#156820,
#156821,#156822,#156823,#156824),(#156825,#156826,#156827,#156828,#156829)),
 .UNSPECIFIED.,.F.,.F.,.F.)
B_SPLINE_SURFACE_WITH_KNOTS((2,1,2),(3,2,3),(-0.00211445385587005,0.,0.211445385587005),
(0.0724436337011242,0.0909109506295933,0.0921216910686723),
 .UNSPECIFIED.)
GEOMETRIC_REPRESENTATION_ITEM()
RATIONAL_B_SPLINE_SURFACE(((0.999297534107722,0.992999570811766,0.990053454406148,
0.990053454406148,0.990053454406148),(0.999297534107722,0.992999570811766,
0.990053454406148,0.990053454406148,0.990053454406148),(0.999297534107722,
0.992999570811766,0.990053454406148,0.990053454406148,0.990053454406148)))
REPRESENTATION_ITEM('')
SURFACE()
);
#3658=(
BOUNDED_SURFACE()
B_SPLINE_SURFACE(1,2,((#156836,#156837,#156838,#156839,#156840,#156841,
#156842),(#156843,#156844,#156845,#156846,#156847,#156848,#156849),(#156850,
#156851,#156852,#156853,#156854,#156855,#156856)),.UNSPECIFIED.,.F.,.F.,
 .F.)
B_SPLINE_SURFACE_WITH_KNOTS((2,1,2),(3,2,2,3),(-0.00211537324446611,0.,
0.211537324446611),(0.642404283483303,0.642578551421364,0.642857142857143,
0.660005345227473),.UNSPECIFIED.)
GEOMETRIC_REPRESENTATION_ITEM()
RATIONAL_B_SPLINE_SURFACE(((0.999805186472059,0.999805186472059,0.999805186472059,
0.999902211834795,1.,0.993980822699461,0.990851751371594),(0.999805186472059,
0.999805186472059,0.999805186472059,0.999902211834795,1.,0.993980822699461,
0.990851751371594),(0.999805186472059,0.999805186472059,0.999805186472059,
0.999902211834795,1.,0.993980822699461,0.990851751371594)))
REPRESENTATION_ITEM('')
SURFACE()
);
#3659=(
BOUNDED_SURFACE()
B_SPLINE_SURFACE(1,2,((#156858,#156859,#156860,#156861,#156862),(#156863,
#156864,#156865,#156866,#156867),(#156868,#156869,#156870,#156871,#156872)),
 .UNSPECIFIED.,.F.,.F.,.F.)
B_SPLINE_SURFACE_WITH_KNOTS((2,1,2),(3,2,3),(-0.00211445385587002,0.,0.211445385587002),
(0.0724436337261546,0.0909109506295934,0.0921216910594916),
 .UNSPECIFIED.)
GEOMETRIC_REPRESENTATION_ITEM()
RATIONAL_B_SPLINE_SURFACE(((0.999297534090649,0.992999570807773,0.990053454406148,
0.990053454406148,0.990053454406148),(0.999297534090649,0.992999570807773,
0.990053454406148,0.990053454406148,0.990053454406148),(0.999297534090649,
0.992999570807773,0.990053454406148,0.990053454406148,0.990053454406148)))
REPRESENTATION_ITEM('')
SURFACE()
);
#3660=(
BOUNDED_SURFACE()
B_SPLINE_SURFACE(1,2,((#156879,#156880,#156881,#156882,#156883,#156884,
#156885),(#156886,#156887,#156888,#156889,#156890,#156891,#156892),(#156893,
#156894,#156895,#156896,#156897,#156898,#156899)),.UNSPECIFIED.,.F.,.F.,
 .F.)
B_SPLINE_SURFACE_WITH_KNOTS((2,1,2),(3,2,2,3),(-0.00211537324446904,0.,
0.211537324446904),(0.642404283483268,0.642578551421329,0.642857142857143,
0.660005345227479),.UNSPECIFIED.)
GEOMETRIC_REPRESENTATION_ITEM()
RATIONAL_B_SPLINE_SURFACE(((0.999805186472035,0.999805186472035,0.999805186472035,
0.999902211834783,1.,0.993980822699459,0.990851751371591),(0.999805186472035,
0.999805186472035,0.999805186472035,0.999902211834783,1.,0.993980822699459,
0.990851751371591),(0.999805186472035,0.999805186472035,0.999805186472035,
0.999902211834783,1.,0.993980822699459,0.990851751371591)))
REPRESENTATION_ITEM('')
SURFACE()
);
#3661=(
BOUNDED_SURFACE()
B_SPLINE_SURFACE(1,2,((#156901,#156902,#156903,#156904,#156905),(#156906,
#156907,#156908,#156909,#156910),(#156911,#156912,#156913,#156914,#156915)),
 .UNSPECIFIED.,.F.,.F.,.F.)
B_SPLINE_SURFACE_WITH_KNOTS((2,1,2),(3,2,3),(-0.00211445385587009,0.,0.211445385587009),
(0.0724436336683128,0.0909109506295935,0.0921216910852292),
 .UNSPECIFIED.)
GEOMETRIC_REPRESENTATION_ITEM()
RATIONAL_B_SPLINE_SURFACE(((0.999297534130102,0.992999570817001,0.990053454406147,
0.990053454406147,0.990053454406147),(0.999297534130102,0.992999570817001,
0.990053454406147,0.990053454406147,0.990053454406147),(0.999297534130102,
0.992999570817001,0.990053454406147,0.990053454406147,0.990053454406147)))
REPRESENTATION_ITEM('')
SURFACE()
);
#3662=(
BOUNDED_SURFACE()
B_SPLINE_SURFACE(1,2,((#156922,#156923,#156924,#156925,#156926,#156927,
#156928),(#156929,#156930,#156931,#156932,#156933,#156934,#156935),(#156936,
#156937,#156938,#156939,#156940,#156941,#156942)),.UNSPECIFIED.,.F.,.F.,
 .F.)
B_SPLINE_SURFACE_WITH_KNOTS((2,1,2),(3,2,2,3),(-0.00211537324446607,0.,
0.211537324446607),(0.642404283483303,0.642578551421364,0.642857142857143,
0.660005345227472),.UNSPECIFIED.)
GEOMETRIC_REPRESENTATION_ITEM()
RATIONAL_B_SPLINE_SURFACE(((0.999805186472059,0.999805186472059,0.999805186472059,
0.999902211834795,1.,0.993980822699462,0.990851751371594),(0.999805186472059,
0.999805186472059,0.999805186472059,0.999902211834795,1.,0.993980822699462,
0.990851751371594),(0.999805186472059,0.999805186472059,0.999805186472059,
0.999902211834795,1.,0.993980822699462,0.990851751371594)))
REPRESENTATION_ITEM('')
SURFACE()
);
#3663=(
BOUNDED_SURFACE()
B_SPLINE_SURFACE(1,2,((#156944,#156945,#156946,#156947,#156948),(#156949,
#156950,#156951,#156952,#156953),(#156954,#156955,#156956,#156957,#156958)),
 .UNSPECIFIED.,.F.,.F.,.F.)
B_SPLINE_SURFACE_WITH_KNOTS((2,1,2),(3,2,3),(-0.00211445385587004,0.,0.211445385587004),
(0.0724436331381984,0.0909109506295934,0.0921216910780853),
 .UNSPECIFIED.)
GEOMETRIC_REPRESENTATION_ITEM()
RATIONAL_B_SPLINE_SURFACE(((0.999297534491675,0.992999570901571,0.990053454406148,
0.990053454406148,0.990053454406148),(0.999297534491675,0.992999570901571,
0.990053454406148,0.990053454406148,0.990053454406148),(0.999297534491675,
0.992999570901571,0.990053454406148,0.990053454406148,0.990053454406148)))
REPRESENTATION_ITEM('')
SURFACE()
);
#3664=(
BOUNDED_SURFACE()
B_SPLINE_SURFACE(1,2,((#156965,#156966,#156967,#156968,#156969,#156970,
#156971),(#156972,#156973,#156974,#156975,#156976,#156977,#156978),(#156979,
#156980,#156981,#156982,#156983,#156984,#156985)),.UNSPECIFIED.,.F.,.F.,
 .F.)
B_SPLINE_SURFACE_WITH_KNOTS((2,1,2),(3,2,2,3),(-0.00211537324446616,0.,
0.211537324446616),(0.642404283483302,0.642578551421363,0.642857142857143,
0.660005345227471),.UNSPECIFIED.)
GEOMETRIC_REPRESENTATION_ITEM()
RATIONAL_B_SPLINE_SURFACE(((0.999805186472059,0.999805186472059,0.999805186472059,
0.999902211834794,1.,0.993980822699462,0.990851751371594),(0.999805186472059,
0.999805186472059,0.999805186472059,0.999902211834794,1.,0.993980822699462,
0.990851751371594),(0.999805186472059,0.999805186472059,0.999805186472059,
0.999902211834794,1.,0.993980822699462,0.990851751371594)))
REPRESENTATION_ITEM('')
SURFACE()
);
#3665=(
BOUNDED_SURFACE()
B_SPLINE_SURFACE(1,2,((#156987,#156988,#156989,#156990,#156991),(#156992,
#156993,#156994,#156995,#156996),(#156997,#156998,#156999,#157000,#157001)),
 .UNSPECIFIED.,.F.,.F.,.F.)
B_SPLINE_SURFACE_WITH_KNOTS((2,1,2),(3,2,3),(-0.00211445385587011,0.,0.211445385587011),
(0.0724436338486829,0.0909109506295947,0.0921216908958231),
 .UNSPECIFIED.)
GEOMETRIC_REPRESENTATION_ITEM()
RATIONAL_B_SPLINE_SURFACE(((0.999297534007077,0.992999570788226,0.990053454406147,
0.990053454406147,0.990053454406147),(0.999297534007077,0.992999570788226,
0.990053454406147,0.990053454406147,0.990053454406147),(0.999297534007077,
0.992999570788226,0.990053454406147,0.990053454406147,0.990053454406147)))
REPRESENTATION_ITEM('')
SURFACE()
);
#3666=(
BOUNDED_SURFACE()
B_SPLINE_SURFACE(1,2,((#157008,#157009,#157010,#157011,#157012,#157013,
#157014),(#157015,#157016,#157017,#157018,#157019,#157020,#157021),(#157022,
#157023,#157024,#157025,#157026,#157027,#157028)),.UNSPECIFIED.,.F.,.F.,
 .F.)
B_SPLINE_SURFACE_WITH_KNOTS((2,1,2),(3,2,2,3),(-0.00211537324446625,0.,
0.211537324446625),(0.642404283483301,0.642578551421362,0.642857142857143,
0.660005345227463),.UNSPECIFIED.)
GEOMETRIC_REPRESENTATION_ITEM()
RATIONAL_B_SPLINE_SURFACE(((0.999805186472057,0.999805186472057,0.999805186472057,
0.999902211834794,1.,0.993980822699465,0.990851751371597),(0.999805186472057,
0.999805186472057,0.999805186472057,0.999902211834794,1.,0.993980822699465,
0.990851751371597),(0.999805186472057,0.999805186472057,0.999805186472057,
0.999902211834794,1.,0.993980822699465,0.990851751371597)))
REPRESENTATION_ITEM('')
SURFACE()
);
#3667=(
BOUNDED_SURFACE()
B_SPLINE_SURFACE(1,2,((#157030,#157031,#157032,#157033,#157034),(#157035,
#157036,#157037,#157038,#157039),(#157040,#157041,#157042,#157043,#157044)),
 .UNSPECIFIED.,.F.,.F.,.F.)
B_SPLINE_SURFACE_WITH_KNOTS((2,1,2),(3,2,3),(-0.0021144538558701,0.,0.21144538558701),
(0.0724436336675499,0.0909109506295944,0.0921216910926114),
 .UNSPECIFIED.)
GEOMETRIC_REPRESENTATION_ITEM()
RATIONAL_B_SPLINE_SURFACE(((0.999297534130622,0.992999570817122,0.990053454406147,
0.990053454406147,0.990053454406147),(0.999297534130622,0.992999570817122,
0.990053454406147,0.990053454406147,0.990053454406147),(0.999297534130622,
0.992999570817122,0.990053454406147,0.990053454406147,0.990053454406147)))
REPRESENTATION_ITEM('')
SURFACE()
);
#3668=(
BOUNDED_SURFACE()
B_SPLINE_SURFACE(1,2,((#157051,#157052,#157053,#157054,#157055,#157056,
#157057),(#157058,#157059,#157060,#157061,#157062,#157063,#157064),(#157065,
#157066,#157067,#157068,#157069,#157070,#157071)),.UNSPECIFIED.,.F.,.F.,
 .F.)
B_SPLINE_SURFACE_WITH_KNOTS((2,1,2),(3,2,2,3),(-0.0021153732444663,0.,0.21153732444663),
(0.642404283483301,0.642578551421362,0.642857142857143,0.660005345227463),
 .UNSPECIFIED.)
GEOMETRIC_REPRESENTATION_ITEM()
RATIONAL_B_SPLINE_SURFACE(((0.999805186472057,0.999805186472057,0.999805186472057,
0.999902211834794,1.,0.993980822699465,0.990851751371597),(0.999805186472057,
0.999805186472057,0.999805186472057,0.999902211834794,1.,0.993980822699465,
0.990851751371597),(0.999805186472057,0.999805186472057,0.999805186472057,
0.999902211834794,1.,0.993980822699465,0.990851751371597)))
REPRESENTATION_ITEM('')
SURFACE()
);
#3669=(
BOUNDED_SURFACE()
B_SPLINE_SURFACE(1,2,((#157073,#157074,#157075,#157076,#157077),(#157078,
#157079,#157080,#157081,#157082),(#157083,#157084,#157085,#157086,#157087)),
 .UNSPECIFIED.,.F.,.F.,.F.)
B_SPLINE_SURFACE_WITH_KNOTS((2,1,2),(3,2,3),(-0.0021144538558701,0.,0.21144538558701),
(0.0724436336107497,0.0909109506295944,0.0921216911633498),
 .UNSPECIFIED.)
GEOMETRIC_REPRESENTATION_ITEM()
RATIONAL_B_SPLINE_SURFACE(((0.999297534169364,0.992999570826184,0.990053454406147,
0.990053454406147,0.990053454406147),(0.999297534169364,0.992999570826184,
0.990053454406147,0.990053454406147,0.990053454406147),(0.999297534169364,
0.992999570826184,0.990053454406147,0.990053454406147,0.990053454406147)))
REPRESENTATION_ITEM('')
SURFACE()
);
#3670=(
BOUNDED_SURFACE()
B_SPLINE_SURFACE(1,2,((#157094,#157095,#157096,#157097,#157098,#157099,
#157100),(#157101,#157102,#157103,#157104,#157105,#157106,#157107),(#157108,
#157109,#157110,#157111,#157112,#157113,#157114)),.UNSPECIFIED.,.F.,.F.,
 .F.)
B_SPLINE_SURFACE_WITH_KNOTS((2,1,2),(3,2,2,3),(-0.0021153732444663,0.,0.21153732444663),
(0.642404283483301,0.642578551421362,0.642857142857143,0.660005345227463),
 .UNSPECIFIED.)
GEOMETRIC_REPRESENTATION_ITEM()
RATIONAL_B_SPLINE_SURFACE(((0.999805186472057,0.999805186472057,0.999805186472057,
0.999902211834794,1.,0.993980822699465,0.990851751371597),(0.999805186472057,
0.999805186472057,0.999805186472057,0.999902211834794,1.,0.993980822699465,
0.990851751371597),(0.999805186472057,0.999805186472057,0.999805186472057,
0.999902211834794,1.,0.993980822699465,0.990851751371597)))
REPRESENTATION_ITEM('')
SURFACE()
);
#3671=(
BOUNDED_SURFACE()
B_SPLINE_SURFACE(1,2,((#157116,#157117,#157118,#157119,#157120),(#157121,
#157122,#157123,#157124,#157125),(#157126,#157127,#157128,#157129,#157130)),
 .UNSPECIFIED.,.F.,.F.,.F.)
B_SPLINE_SURFACE_WITH_KNOTS((2,1,2),(3,2,3),(-0.00211445385587009,0.,0.211445385587009),
(0.0724436336951236,0.0909109506295944,0.0921216910686102),
 .UNSPECIFIED.)
GEOMETRIC_REPRESENTATION_ITEM()
RATIONAL_B_SPLINE_SURFACE(((0.999297534111815,0.992999570812723,0.990053454406147,
0.990053454406147,0.990053454406147),(0.999297534111815,0.992999570812723,
0.990053454406147,0.990053454406147,0.990053454406147),(0.999297534111815,
0.992999570812723,0.990053454406147,0.990053454406147,0.990053454406147)))
REPRESENTATION_ITEM('')
SURFACE()
);
#3672=(
BOUNDED_SURFACE()
B_SPLINE_SURFACE(1,2,((#157137,#157138,#157139,#157140,#157141,#157142,
#157143),(#157144,#157145,#157146,#157147,#157148,#157149,#157150),(#157151,
#157152,#157153,#157154,#157155,#157156,#157157)),.UNSPECIFIED.,.F.,.F.,
 .F.)
B_SPLINE_SURFACE_WITH_KNOTS((2,1,2),(3,2,2,3),(-0.00211537324446626,0.,
0.211537324446626),(0.642404283483301,0.642578551421362,0.642857142857143,
0.660005345227463),.UNSPECIFIED.)
GEOMETRIC_REPRESENTATION_ITEM()
RATIONAL_B_SPLINE_SURFACE(((0.999805186472057,0.999805186472057,0.999805186472057,
0.999902211834794,1.,0.993980822699465,0.990851751371597),(0.999805186472057,
0.999805186472057,0.999805186472057,0.999902211834794,1.,0.993980822699465,
0.990851751371597),(0.999805186472057,0.999805186472057,0.999805186472057,
0.999902211834794,1.,0.993980822699465,0.990851751371597)))
REPRESENTATION_ITEM('')
SURFACE()
);
#3673=(
BOUNDED_SURFACE()
B_SPLINE_SURFACE(1,2,((#157159,#157160,#157161,#157162,#157163),(#157164,
#157165,#157166,#157167,#157168)),.UNSPECIFIED.,.F.,.F.,.F.)
B_SPLINE_SURFACE_WITH_KNOTS((2,2),(3,2,3),(0.,0.211445385587011),(0.073550810617375,
0.0909109506295944,0.0910845520297166),.UNSPECIFIED.)
GEOMETRIC_REPRESENTATION_ITEM()
RATIONAL_B_SPLINE_SURFACE(((0.998554414400246,0.992822941359338,0.990053454406147,
0.990053454406147,0.990053454406147),(0.998554414400246,0.992822941359338,
0.990053454406147,0.990053454406147,0.990053454406147)))
REPRESENTATION_ITEM('')
SURFACE()
);
#3674=(
BOUNDED_SURFACE()
B_SPLINE_SURFACE(1,2,((#157170,#157171,#157172),(#157173,#157174,#157175)),
 .UNSPECIFIED.,.F.,.F.,.F.)
B_SPLINE_SURFACE_WITH_KNOTS((2,2),(3,3),(0.,0.28980704099168),(0.125170525609408,
0.142682999576236),.UNSPECIFIED.)
GEOMETRIC_REPRESENTATION_ITEM()
RATIONAL_B_SPLINE_SURFACE(((0.990658108926709,0.993760979299921,0.999878046252917),
(0.990658108926709,0.993760979299921,0.999878046252917)))
REPRESENTATION_ITEM('')
SURFACE()
);
#3675=(
BOUNDED_SURFACE()
B_SPLINE_SURFACE(1,2,((#157192,#157193,#157194,#157195,#157196),(#157197,
#157198,#157199,#157200,#157201)),.UNSPECIFIED.,.F.,.F.,.F.)
B_SPLINE_SURFACE_WITH_KNOTS((2,2),(3,2,3),(0.,0.290271444040998),(0.590808523385635,
0.607982157956011,0.608572517835734),.UNSPECIFIED.)
GEOMETRIC_REPRESENTATION_ITEM()
RATIONAL_B_SPLINE_SURFACE(((0.990086238235256,0.987329216372183,0.987470879370255,
0.987470879370255,0.987470879370255),(0.990086238235256,0.987329216372183,
0.987470879370255,0.987470879370255,0.987470879370255)))
REPRESENTATION_ITEM('')
SURFACE()
);
#3676=(
BOUNDED_SURFACE()
B_SPLINE_SURFACE(1,2,((#157203,#157204,#157205),(#157206,#157207,#157208)),
 .UNSPECIFIED.,.F.,.F.,.F.)
B_SPLINE_SURFACE_WITH_KNOTS((2,2),(3,3),(0.,0.289807040991667),(0.125170525609408,
0.142682999576236),.UNSPECIFIED.)
GEOMETRIC_REPRESENTATION_ITEM()
RATIONAL_B_SPLINE_SURFACE(((0.990658108926709,0.993760979299921,0.999878046252917),
(0.990658108926709,0.993760979299921,0.999878046252917)))
REPRESENTATION_ITEM('')
SURFACE()
);
#3677=(
BOUNDED_SURFACE()
B_SPLINE_SURFACE(1,2,((#157225,#157226,#157227,#157228,#157229),(#157230,
#157231,#157232,#157233,#157234)),.UNSPECIFIED.,.F.,.F.,.F.)
B_SPLINE_SURFACE_WITH_KNOTS((2,2),(3,2,3),(0.,0.290271444029068),(0.590808523385632,
0.607982157956011,0.608572517823816),.UNSPECIFIED.)
GEOMETRIC_REPRESENTATION_ITEM()
RATIONAL_B_SPLINE_SURFACE(((0.990086238235257,0.987329216372183,0.987470879370255,
0.987470879370255,0.987470879370255),(0.990086238235257,0.987329216372183,
0.987470879370255,0.987470879370255,0.987470879370255)))
REPRESENTATION_ITEM('')
SURFACE()
);
#3678=(
BOUNDED_SURFACE()
B_SPLINE_SURFACE(1,2,((#157236,#157237,#157238),(#157239,#157240,#157241)),
 .UNSPECIFIED.,.F.,.F.,.F.)
B_SPLINE_SURFACE_WITH_KNOTS((2,2),(3,3),(0.,0.289807040991662),(0.125170525609408,
0.14268299957623),.UNSPECIFIED.)
GEOMETRIC_REPRESENTATION_ITEM()
RATIONAL_B_SPLINE_SURFACE(((0.990658108926709,0.99376097929992,0.999878046252913),
(0.990658108926709,0.99376097929992,0.999878046252913)))
REPRESENTATION_ITEM('')
SURFACE()
);
#3679=(
BOUNDED_SURFACE()
B_SPLINE_SURFACE(1,2,((#157258,#157259,#157260,#157261,#157262),(#157263,
#157264,#157265,#157266,#157267)),.UNSPECIFIED.,.F.,.F.,.F.)
B_SPLINE_SURFACE_WITH_KNOTS((2,2),(3,2,3),(0.,0.29027144404043),(0.590808523385623,
0.607982157956011,0.608572517835178),.UNSPECIFIED.)
GEOMETRIC_REPRESENTATION_ITEM()
RATIONAL_B_SPLINE_SURFACE(((0.99008623823526,0.987329216372183,0.987470879370255,
0.987470879370255,0.987470879370255),(0.99008623823526,0.987329216372183,
0.987470879370255,0.987470879370255,0.987470879370255)))
REPRESENTATION_ITEM('')
SURFACE()
);
#3680=(
BOUNDED_SURFACE()
B_SPLINE_SURFACE(1,2,((#157269,#157270,#157271),(#157272,#157273,#157274)),
 .UNSPECIFIED.,.F.,.F.,.F.)
B_SPLINE_SURFACE_WITH_KNOTS((2,2),(3,3),(0.,0.289807040991601),(0.125170525609408,
0.142682999576235),.UNSPECIFIED.)
GEOMETRIC_REPRESENTATION_ITEM()
RATIONAL_B_SPLINE_SURFACE(((0.990658108926709,0.993760979299921,0.999878046252916),
(0.990658108926709,0.993760979299921,0.999878046252916)))
REPRESENTATION_ITEM('')
SURFACE()
);
#3681=(
BOUNDED_SURFACE()
B_SPLINE_SURFACE(1,2,((#157291,#157292,#157293,#157294,#157295),(#157296,
#157297,#157298,#157299,#157300)),.UNSPECIFIED.,.F.,.F.,.F.)
B_SPLINE_SURFACE_WITH_KNOTS((2,2),(3,2,3),(0.,0.290271444033733),(0.590808523385632,
0.607982157956012,0.608572517870902),.UNSPECIFIED.)
GEOMETRIC_REPRESENTATION_ITEM()
RATIONAL_B_SPLINE_SURFACE(((0.990086238235257,0.987329216372183,0.987470879370255,
0.987470879370255,0.987470879370255),(0.990086238235257,0.987329216372183,
0.987470879370255,0.987470879370255,0.987470879370255)))
REPRESENTATION_ITEM('')
SURFACE()
);
#3682=(
BOUNDED_SURFACE()
B_SPLINE_SURFACE(1,2,((#157302,#157303,#157304),(#157305,#157306,#157307)),
 .UNSPECIFIED.,.F.,.F.,.F.)
B_SPLINE_SURFACE_WITH_KNOTS((2,2),(3,3),(0.,0.289807040991605),(0.125170525609407,
0.142682999576233),.UNSPECIFIED.)
GEOMETRIC_REPRESENTATION_ITEM()
RATIONAL_B_SPLINE_SURFACE(((0.990658108926708,0.99376097929992,0.999878046252915),
(0.990658108926708,0.99376097929992,0.999878046252915)))
REPRESENTATION_ITEM('')
SURFACE()
);
#3683=(
BOUNDED_SURFACE()
B_SPLINE_SURFACE(1,2,((#157324,#157325,#157326,#157327,#157328),(#157329,
#157330,#157331,#157332,#157333)),.UNSPECIFIED.,.F.,.F.,.F.)
B_SPLINE_SURFACE_WITH_KNOTS((2,2),(3,2,3),(0.,0.290271444020211),(0.590808523385629,
0.607982157956012,0.60857251785743),.UNSPECIFIED.)
GEOMETRIC_REPRESENTATION_ITEM()
RATIONAL_B_SPLINE_SURFACE(((0.990086238235258,0.987329216372183,0.987470879370255,
0.987470879370255,0.987470879370255),(0.990086238235258,0.987329216372183,
0.987470879370255,0.987470879370255,0.987470879370255)))
REPRESENTATION_ITEM('')
SURFACE()
);
#3684=(
BOUNDED_SURFACE()
B_SPLINE_SURFACE(1,2,((#157335,#157336,#157337),(#157338,#157339,#157340)),
 .UNSPECIFIED.,.F.,.F.,.F.)
B_SPLINE_SURFACE_WITH_KNOTS((2,2),(3,3),(0.,0.289807040991593),(0.125170525609407,
0.142682999576235),.UNSPECIFIED.)
GEOMETRIC_REPRESENTATION_ITEM()
RATIONAL_B_SPLINE_SURFACE(((0.990658108926708,0.993760979299921,0.999878046252916),
(0.990658108926708,0.993760979299921,0.999878046252916)))
REPRESENTATION_ITEM('')
SURFACE()
);
#3685=(
BOUNDED_SURFACE()
B_SPLINE_SURFACE(1,2,((#157357,#157358,#157359,#157360,#157361),(#157362,
#157363,#157364,#157365,#157366)),.UNSPECIFIED.,.F.,.F.,.F.)
B_SPLINE_SURFACE_WITH_KNOTS((2,2),(3,2,3),(0.,0.290271444018325),(0.590808523385636,
0.607982157956012,0.608572517813142),.UNSPECIFIED.)
GEOMETRIC_REPRESENTATION_ITEM()
RATIONAL_B_SPLINE_SURFACE(((0.990086238235256,0.987329216372183,0.987470879370255,
0.987470879370255,0.987470879370255),(0.990086238235256,0.987329216372183,
0.987470879370255,0.987470879370255,0.987470879370255)))
REPRESENTATION_ITEM('')
SURFACE()
);
#3686=(
BOUNDED_SURFACE()
B_SPLINE_SURFACE(1,2,((#157368,#157369,#157370),(#157371,#157372,#157373)),
 .UNSPECIFIED.,.F.,.F.,.F.)
B_SPLINE_SURFACE_WITH_KNOTS((2,2),(3,3),(0.,0.289807040991612),(0.125170525609407,
0.142682999576235),.UNSPECIFIED.)
GEOMETRIC_REPRESENTATION_ITEM()
RATIONAL_B_SPLINE_SURFACE(((0.990658108926708,0.993760979299921,0.999878046252916),
(0.990658108926708,0.993760979299921,0.999878046252916)))
REPRESENTATION_ITEM('')
SURFACE()
);
#3687=(
BOUNDED_SURFACE()
B_SPLINE_SURFACE(1,2,((#157390,#157391,#157392,#157393,#157394),(#157395,
#157396,#157397,#157398,#157399)),.UNSPECIFIED.,.F.,.F.,.F.)
B_SPLINE_SURFACE_WITH_KNOTS((2,2),(3,2,3),(0.,0.290271444050794),(0.590808523385632,
0.607982157956012,0.608572517845598),.UNSPECIFIED.)
GEOMETRIC_REPRESENTATION_ITEM()
RATIONAL_B_SPLINE_SURFACE(((0.990086238235257,0.987329216372183,0.987470879370256,
0.987470879370256,0.987470879370256),(0.990086238235257,0.987329216372183,
0.987470879370256,0.987470879370256,0.987470879370256)))
REPRESENTATION_ITEM('')
SURFACE()
);
#3688=(
BOUNDED_SURFACE()
B_SPLINE_SURFACE(1,2,((#157401,#157402,#157403),(#157404,#157405,#157406)),
 .UNSPECIFIED.,.F.,.F.,.F.)
B_SPLINE_SURFACE_WITH_KNOTS((2,2),(3,3),(0.,0.289807040991564),(0.125170525609407,
0.142682999576235),.UNSPECIFIED.)
GEOMETRIC_REPRESENTATION_ITEM()
RATIONAL_B_SPLINE_SURFACE(((0.990658108926708,0.993760979299921,0.999878046252916),
(0.990658108926708,0.993760979299921,0.999878046252916)))
REPRESENTATION_ITEM('')
SURFACE()
);
#3689=(
BOUNDED_SURFACE()
B_SPLINE_SURFACE(1,2,((#157423,#157424,#157425,#157426,#157427),(#157428,
#157429,#157430,#157431,#157432)),.UNSPECIFIED.,.F.,.F.,.F.)
B_SPLINE_SURFACE_WITH_KNOTS((2,2),(3,2,3),(0.,0.290271444021746),(0.590808523385626,
0.607982157956012,0.608572517858504),.UNSPECIFIED.)
GEOMETRIC_REPRESENTATION_ITEM()
RATIONAL_B_SPLINE_SURFACE(((0.990086238235259,0.987329216372183,0.987470879370255,
0.987470879370255,0.987470879370255),(0.990086238235259,0.987329216372183,
0.987470879370255,0.987470879370255,0.987470879370255)))
REPRESENTATION_ITEM('')
SURFACE()
);
#3690=(
BOUNDED_SURFACE()
B_SPLINE_SURFACE(1,2,((#157434,#157435,#157436),(#157437,#157438,#157439)),
 .UNSPECIFIED.,.F.,.F.,.F.)
B_SPLINE_SURFACE_WITH_KNOTS((2,2),(3,3),(0.,0.289807040991559),(0.125170525609407,
0.142682999576235),.UNSPECIFIED.)
GEOMETRIC_REPRESENTATION_ITEM()
RATIONAL_B_SPLINE_SURFACE(((0.990658108926708,0.993760979299921,0.999878046252916),
(0.990658108926708,0.993760979299921,0.999878046252916)))
REPRESENTATION_ITEM('')
SURFACE()
);
#3691=(
BOUNDED_SURFACE()
B_SPLINE_SURFACE(1,2,((#157456,#157457,#157458,#157459,#157460),(#157461,
#157462,#157463,#157464,#157465)),.UNSPECIFIED.,.F.,.F.,.F.)
B_SPLINE_SURFACE_WITH_KNOTS((2,2),(3,2,3),(0.,0.290271444051793),(0.590808523385636,
0.607982157956012,0.608572517846652),.UNSPECIFIED.)
GEOMETRIC_REPRESENTATION_ITEM()
RATIONAL_B_SPLINE_SURFACE(((0.990086238235256,0.987329216372183,0.987470879370255,
0.987470879370255,0.987470879370255),(0.990086238235256,0.987329216372183,
0.987470879370255,0.987470879370255,0.987470879370255)))
REPRESENTATION_ITEM('')
SURFACE()
);
#3692=(
BOUNDED_SURFACE()
B_SPLINE_SURFACE(1,2,((#157467,#157468,#157469),(#157470,#157471,#157472)),
 .UNSPECIFIED.,.F.,.F.,.F.)
B_SPLINE_SURFACE_WITH_KNOTS((2,2),(3,3),(0.,0.289807040991559),(0.125170525609407,
0.142682999576235),.UNSPECIFIED.)
GEOMETRIC_REPRESENTATION_ITEM()
RATIONAL_B_SPLINE_SURFACE(((0.990658108926708,0.993760979299921,0.999878046252916),
(0.990658108926708,0.993760979299921,0.999878046252916)))
REPRESENTATION_ITEM('')
SURFACE()
);
#3693=(
BOUNDED_SURFACE()
B_SPLINE_SURFACE(1,2,((#157489,#157490,#157491,#157492,#157493),(#157494,
#157495,#157496,#157497,#157498)),.UNSPECIFIED.,.F.,.F.,.F.)
B_SPLINE_SURFACE_WITH_KNOTS((2,2),(3,2,3),(0.,0.290271444048056),(0.590808523385636,
0.607982157956012,0.608572517842917),.UNSPECIFIED.)
GEOMETRIC_REPRESENTATION_ITEM()
RATIONAL_B_SPLINE_SURFACE(((0.990086238235256,0.987329216372183,0.987470879370255,
0.987470879370255,0.987470879370255),(0.990086238235256,0.987329216372183,
0.987470879370255,0.987470879370255,0.987470879370255)))
REPRESENTATION_ITEM('')
SURFACE()
);
#3694=(
BOUNDED_SURFACE()
B_SPLINE_SURFACE(1,2,((#157500,#157501,#157502),(#157503,#157504,#157505)),
 .UNSPECIFIED.,.F.,.F.,.F.)
B_SPLINE_SURFACE_WITH_KNOTS((2,2),(3,3),(0.,0.289807040991562),(0.125170525609407,
0.142682999576235),.UNSPECIFIED.)
GEOMETRIC_REPRESENTATION_ITEM()
RATIONAL_B_SPLINE_SURFACE(((0.990658108926708,0.993760979299921,0.999878046252916),
(0.990658108926708,0.993760979299921,0.999878046252916)))
REPRESENTATION_ITEM('')
SURFACE()
);
#3695=(
BOUNDED_SURFACE()
B_SPLINE_SURFACE(1,2,((#157522,#157523,#157524,#157525,#157526),(#157527,
#157528,#157529,#157530,#157531)),.UNSPECIFIED.,.F.,.F.,.F.)
B_SPLINE_SURFACE_WITH_KNOTS((2,2),(3,2,3),(0.,0.29027144400483),(0.590808523385636,
0.607982157956012,0.60857251784236),.UNSPECIFIED.)
GEOMETRIC_REPRESENTATION_ITEM()
RATIONAL_B_SPLINE_SURFACE(((0.990086238235256,0.987329216372183,0.987470879370255,
0.987470879370255,0.987470879370255),(0.990086238235256,0.987329216372183,
0.987470879370255,0.987470879370255,0.987470879370255)))
REPRESENTATION_ITEM('')
SURFACE()
);
#3696=(
BOUNDED_SURFACE()
B_SPLINE_SURFACE(1,2,((#157533,#157534,#157535),(#157536,#157537,#157538)),
 .UNSPECIFIED.,.F.,.F.,.F.)
B_SPLINE_SURFACE_WITH_KNOTS((2,2),(3,3),(0.,0.289807040991561),(0.125170525609407,
0.142682999576235),.UNSPECIFIED.)
GEOMETRIC_REPRESENTATION_ITEM()
RATIONAL_B_SPLINE_SURFACE(((0.990658108926708,0.993760979299921,0.999878046252916),
(0.990658108926708,0.993760979299921,0.999878046252916)))
REPRESENTATION_ITEM('')
SURFACE()
);
#3697=(
BOUNDED_SURFACE()
B_SPLINE_SURFACE(1,2,((#157555,#157556,#157557,#157558,#157559),(#157560,
#157561,#157562,#157563,#157564)),.UNSPECIFIED.,.F.,.F.,.F.)
B_SPLINE_SURFACE_WITH_KNOTS((2,2),(3,2,3),(0.,0.290271443966874),(0.59080852338557,
0.607982157956012,0.608572517804365),.UNSPECIFIED.)
GEOMETRIC_REPRESENTATION_ITEM()
RATIONAL_B_SPLINE_SURFACE(((0.990086238235277,0.987329216372182,0.987470879370255,
0.987470879370255,0.987470879370255),(0.990086238235277,0.987329216372182,
0.987470879370255,0.987470879370255,0.987470879370255)))
REPRESENTATION_ITEM('')
SURFACE()
);
#3698=(
BOUNDED_SURFACE()
B_SPLINE_SURFACE(1,2,((#157566,#157567,#157568),(#157569,#157570,#157571)),
 .UNSPECIFIED.,.F.,.F.,.F.)
B_SPLINE_SURFACE_WITH_KNOTS((2,2),(3,3),(0.,0.289807040991565),(0.125170525609406,
0.142682999576235),.UNSPECIFIED.)
GEOMETRIC_REPRESENTATION_ITEM()
RATIONAL_B_SPLINE_SURFACE(((0.990658108926708,0.99376097929992,0.999878046252916),
(0.990658108926708,0.993760979299921,0.999878046252916)))
REPRESENTATION_ITEM('')
SURFACE()
);
#3699=(
BOUNDED_SURFACE()
B_SPLINE_SURFACE(1,2,((#157588,#157589,#157590,#157591,#157592),(#157593,
#157594,#157595,#157596,#157597)),.UNSPECIFIED.,.F.,.F.,.F.)
B_SPLINE_SURFACE_WITH_KNOTS((2,2),(3,2,3),(0.,0.290271444008694),(0.590808523385636,
0.607982157956012,0.608572517846246),.UNSPECIFIED.)
GEOMETRIC_REPRESENTATION_ITEM()
RATIONAL_B_SPLINE_SURFACE(((0.990086238235256,0.987329216372183,0.987470879370255,
0.987470879370255,0.987470879370255),(0.990086238235256,0.987329216372183,
0.987470879370255,0.987470879370255,0.987470879370255)))
REPRESENTATION_ITEM('')
SURFACE()
);
#3700=(
BOUNDED_SURFACE()
B_SPLINE_SURFACE(1,2,((#157599,#157600,#157601),(#157602,#157603,#157604)),
 .UNSPECIFIED.,.F.,.F.,.F.)
B_SPLINE_SURFACE_WITH_KNOTS((2,2),(3,3),(0.,0.289807040991559),(0.125170525609407,
0.142682999576235),.UNSPECIFIED.)
GEOMETRIC_REPRESENTATION_ITEM()
RATIONAL_B_SPLINE_SURFACE(((0.990658108926708,0.993760979299921,0.999878046252916),
(0.990658108926708,0.993760979299921,0.999878046252916)))
REPRESENTATION_ITEM('')
SURFACE()
);
#3701=(
BOUNDED_SURFACE()
B_SPLINE_SURFACE(1,2,((#157621,#157622,#157623,#157624,#157625),(#157626,
#157627,#157628,#157629,#157630)),.UNSPECIFIED.,.F.,.F.,.F.)
B_SPLINE_SURFACE_WITH_KNOTS((2,2),(3,2,3),(0.,0.290271444064358),(0.590808523385636,
0.607982157956012,0.608572517859214),.UNSPECIFIED.)
GEOMETRIC_REPRESENTATION_ITEM()
RATIONAL_B_SPLINE_SURFACE(((0.990086238235256,0.987329216372183,0.987470879370255,
0.987470879370255,0.987470879370255),(0.990086238235256,0.987329216372183,
0.987470879370255,0.987470879370255,0.987470879370255)))
REPRESENTATION_ITEM('')
SURFACE()
);
#3702=(
BOUNDED_SURFACE()
B_SPLINE_SURFACE(1,2,((#157632,#157633,#157634),(#157635,#157636,#157637)),
 .UNSPECIFIED.,.F.,.F.,.F.)
B_SPLINE_SURFACE_WITH_KNOTS((2,2),(3,3),(0.,0.289807040991563),(0.125170525609407,
0.142682999576235),.UNSPECIFIED.)
GEOMETRIC_REPRESENTATION_ITEM()
RATIONAL_B_SPLINE_SURFACE(((0.990658108926708,0.993760979299921,0.999878046252916),
(0.990658108926708,0.993760979299921,0.999878046252916)))
REPRESENTATION_ITEM('')
SURFACE()
);
#3703=(
BOUNDED_SURFACE()
B_SPLINE_SURFACE(1,2,((#157645,#157646,#157647,#157648,#157649),(#157650,
#157651,#157652,#157653,#157654)),.UNSPECIFIED.,.F.,.F.,.F.)
B_SPLINE_SURFACE_WITH_KNOTS((2,2),(3,2,3),(0.,0.290271444031163),(0.590808523385636,
0.607982157956012,0.608572517826022),.UNSPECIFIED.)
GEOMETRIC_REPRESENTATION_ITEM()
RATIONAL_B_SPLINE_SURFACE(((0.990086238235256,0.987329216372183,0.987470879370255,
0.987470879370255,0.987470879370255),(0.990086238235256,0.987329216372183,
0.987470879370255,0.987470879370255,0.987470879370255)))
REPRESENTATION_ITEM('')
SURFACE()
);
#3704=(
BOUNDED_SURFACE()
B_SPLINE_SURFACE(1,2,((#157656,#157657,#157658),(#157659,#157660,#157661)),
 .UNSPECIFIED.,.F.,.F.,.F.)
B_SPLINE_SURFACE_WITH_KNOTS((2,2),(3,3),(0.,0.289807040991562),(0.125170525609407,
0.142682999576235),.UNSPECIFIED.)
GEOMETRIC_REPRESENTATION_ITEM()
RATIONAL_B_SPLINE_SURFACE(((0.990658108926708,0.993760979299921,0.999878046252916),
(0.990658108926708,0.993760979299921,0.999878046252916)))
REPRESENTATION_ITEM('')
SURFACE()
);
#3705=(
BOUNDED_SURFACE()
B_SPLINE_SURFACE(1,2,((#157678,#157679,#157680,#157681,#157682),(#157683,
#157684,#157685,#157686,#157687)),.UNSPECIFIED.,.F.,.F.,.F.)
B_SPLINE_SURFACE_WITH_KNOTS((2,2),(3,2,3),(0.,0.290271444056828),(0.590808523385636,
0.607982157956012,0.608572517851688),.UNSPECIFIED.)
GEOMETRIC_REPRESENTATION_ITEM()
RATIONAL_B_SPLINE_SURFACE(((0.990086238235256,0.987329216372183,0.987470879370255,
0.987470879370255,0.987470879370255),(0.990086238235256,0.987329216372183,
0.987470879370255,0.987470879370255,0.987470879370255)))
REPRESENTATION_ITEM('')
SURFACE()
);
#3706=(
BOUNDED_SURFACE()
B_SPLINE_SURFACE(1,2,((#157689,#157690,#157691),(#157692,#157693,#157694)),
 .UNSPECIFIED.,.F.,.F.,.F.)
B_SPLINE_SURFACE_WITH_KNOTS((2,2),(3,3),(0.,0.289807040991562),(0.125170525609407,
0.142682999576235),.UNSPECIFIED.)
GEOMETRIC_REPRESENTATION_ITEM()
RATIONAL_B_SPLINE_SURFACE(((0.990658108926708,0.993760979299921,0.999878046252916),
(0.990658108926708,0.993760979299921,0.999878046252916)))
REPRESENTATION_ITEM('')
SURFACE()
);
#3707=(
BOUNDED_SURFACE()
B_SPLINE_SURFACE(1,2,((#157711,#157712,#157713,#157714,#157715),(#157716,
#157717,#157718,#157719,#157720)),.UNSPECIFIED.,.F.,.F.,.F.)
B_SPLINE_SURFACE_WITH_KNOTS((2,2),(3,2,3),(0.,0.290271444018615),(0.590808523385636,
0.607982157956012,0.60857251785571),.UNSPECIFIED.)
GEOMETRIC_REPRESENTATION_ITEM()
RATIONAL_B_SPLINE_SURFACE(((0.990086238235256,0.987329216372183,0.987470879370255,
0.987470879370255,0.987470879370255),(0.990086238235256,0.987329216372183,
0.987470879370255,0.987470879370255,0.987470879370255)))
REPRESENTATION_ITEM('')
SURFACE()
);
#3708=(
BOUNDED_SURFACE()
B_SPLINE_SURFACE(1,2,((#157722,#157723,#157724),(#157725,#157726,#157727)),
 .UNSPECIFIED.,.F.,.F.,.F.)
B_SPLINE_SURFACE_WITH_KNOTS((2,2),(3,3),(0.,0.289807040991559),(0.125170525609407,
0.142682999576235),.UNSPECIFIED.)
GEOMETRIC_REPRESENTATION_ITEM()
RATIONAL_B_SPLINE_SURFACE(((0.990658108926708,0.993760979299921,0.999878046252916),
(0.990658108926708,0.993760979299921,0.999878046252916)))
REPRESENTATION_ITEM('')
SURFACE()
);
#3709=(
BOUNDED_SURFACE()
B_SPLINE_SURFACE(1,2,((#157738,#157739,#157740,#157741,#157742),(#157743,
#157744,#157745,#157746,#157747)),.UNSPECIFIED.,.F.,.F.,.F.)
B_SPLINE_SURFACE_WITH_KNOTS((2,2),(3,2,3),(0.,0.290271444082965),(0.590808523385636,
0.607982157956012,0.608572517823633),.UNSPECIFIED.)
GEOMETRIC_REPRESENTATION_ITEM()
RATIONAL_B_SPLINE_SURFACE(((0.990086238235256,0.987329216372183,0.987470879370255,
0.987470879370255,0.987470879370255),(0.990086238235256,0.987329216372183,
0.987470879370255,0.987470879370255,0.987470879370255)))
REPRESENTATION_ITEM('')
SURFACE()
);
#3710=(
BOUNDED_SURFACE()
B_SPLINE_SURFACE(1,2,((#157755,#157756,#157757),(#157758,#157759,#157760)),
 .UNSPECIFIED.,.F.,.F.,.F.)
B_SPLINE_SURFACE_WITH_KNOTS((2,2),(3,3),(0.,0.289807040991562),(0.125170525609398,
0.142682999576235),.UNSPECIFIED.)
GEOMETRIC_REPRESENTATION_ITEM()
RATIONAL_B_SPLINE_SURFACE(((0.990658108926705,0.993760979299918,0.999878046252916),
(0.990658108926705,0.993760979299918,0.999878046252916)))
REPRESENTATION_ITEM('')
SURFACE()
);
#3711=(
BOUNDED_SURFACE()
B_SPLINE_SURFACE(1,2,((#157777,#157778,#157779,#157780,#157781),(#157782,
#157783,#157784,#157785,#157786)),.UNSPECIFIED.,.F.,.F.,.F.)
B_SPLINE_SURFACE_WITH_KNOTS((2,2),(3,2,3),(0.,0.290271443996391),(0.590808523385636,
0.607982157956011,0.608572517833416),.UNSPECIFIED.)
GEOMETRIC_REPRESENTATION_ITEM()
RATIONAL_B_SPLINE_SURFACE(((0.990086238235256,0.987329216372183,0.987470879370255,
0.987470879370255,0.987470879370255),(0.990086238235256,0.987329216372183,
0.987470879370255,0.987470879370255,0.987470879370255)))
REPRESENTATION_ITEM('')
SURFACE()
);
#3712=(
BOUNDED_SURFACE()
B_SPLINE_SURFACE(1,2,((#157788,#157789,#157790),(#157791,#157792,#157793)),
 .UNSPECIFIED.,.F.,.F.,.F.)
B_SPLINE_SURFACE_WITH_KNOTS((2,2),(3,3),(0.,0.289807040991562),(0.125170525609408,
0.142682999576236),.UNSPECIFIED.)
GEOMETRIC_REPRESENTATION_ITEM()
RATIONAL_B_SPLINE_SURFACE(((0.990658108926709,0.993760979299921,0.999878046252917),
(0.990658108926709,0.993760979299921,0.999878046252917)))
REPRESENTATION_ITEM('')
SURFACE()
);
#3713=(
BOUNDED_SURFACE()
B_SPLINE_SURFACE(1,2,((#157810,#157811,#157812,#157813,#157814),(#157815,
#157816,#157817,#157818,#157819)),.UNSPECIFIED.,.F.,.F.,.F.)
B_SPLINE_SURFACE_WITH_KNOTS((2,2),(3,2,3),(0.,0.290271443980373),(0.590808523385635,
0.607982157956011,0.608572517817981),.UNSPECIFIED.)
GEOMETRIC_REPRESENTATION_ITEM()
RATIONAL_B_SPLINE_SURFACE(((0.990086238235256,0.987329216372183,0.987470879370256,
0.987470879370256,0.987470879370256),(0.990086238235256,0.987329216372183,
0.987470879370255,0.987470879370255,0.987470879370255)))
REPRESENTATION_ITEM('')
SURFACE()
);
#3714=(
BOUNDED_SURFACE()
B_SPLINE_SURFACE(1,2,((#157821,#157822,#157823),(#157824,#157825,#157826)),
 .UNSPECIFIED.,.F.,.F.,.F.)
B_SPLINE_SURFACE_WITH_KNOTS((2,2),(3,3),(0.,0.289807040991884),(0.125170525609408,
0.142682999576236),.UNSPECIFIED.)
GEOMETRIC_REPRESENTATION_ITEM()
RATIONAL_B_SPLINE_SURFACE(((0.990658108926709,0.993760979299921,0.999878046252917),
(0.990658108926709,0.993760979299921,0.999878046252917)))
REPRESENTATION_ITEM('')
SURFACE()
);
#3715=(
BOUNDED_SURFACE()
B_SPLINE_SURFACE(1,2,((#157843,#157844,#157845,#157846,#157847),(#157848,
#157849,#157850,#157851,#157852)),.UNSPECIFIED.,.F.,.F.,.F.)
B_SPLINE_SURFACE_WITH_KNOTS((2,2),(3,2,3),(0.,0.290271444022386),(0.590808523385635,
0.607982157956011,0.608572517816915),.UNSPECIFIED.)
GEOMETRIC_REPRESENTATION_ITEM()
RATIONAL_B_SPLINE_SURFACE(((0.990086238235256,0.987329216372183,0.987470879370256,
0.987470879370256,0.987470879370256),(0.990086238235256,0.987329216372183,
0.987470879370256,0.987470879370256,0.987470879370256)))
REPRESENTATION_ITEM('')
SURFACE()
);
#3716=(
BOUNDED_SURFACE()
B_SPLINE_SURFACE(1,2,((#157854,#157855,#157856),(#157857,#157858,#157859)),
 .UNSPECIFIED.,.F.,.F.,.F.)
B_SPLINE_SURFACE_WITH_KNOTS((2,2),(3,3),(0.,0.28980704099189),(0.125170525609408,
0.142682999576237),.UNSPECIFIED.)
GEOMETRIC_REPRESENTATION_ITEM()
RATIONAL_B_SPLINE_SURFACE(((0.990658108926709,0.993760979299922,0.999878046252918),
(0.990658108926709,0.993760979299922,0.999878046252918)))
REPRESENTATION_ITEM('')
SURFACE()
);
#3717=(
BOUNDED_SURFACE()
B_SPLINE_SURFACE(1,2,((#157876,#157877,#157878,#157879,#157880),(#157881,
#157882,#157883,#157884,#157885)),.UNSPECIFIED.,.F.,.F.,.F.)
B_SPLINE_SURFACE_WITH_KNOTS((2,2),(3,2,3),(0.,0.290271444028045),(0.590808523385635,
0.607982157956011,0.608572517822572),.UNSPECIFIED.)
GEOMETRIC_REPRESENTATION_ITEM()
RATIONAL_B_SPLINE_SURFACE(((0.990086238235256,0.987329216372183,0.987470879370255,
0.987470879370255,0.987470879370255),(0.990086238235256,0.987329216372183,
0.987470879370255,0.987470879370255,0.987470879370255)))
REPRESENTATION_ITEM('')
SURFACE()
);
#3718=(
BOUNDED_SURFACE()
B_SPLINE_SURFACE(1,2,((#157887,#157888,#157889),(#157890,#157891,#157892)),
 .UNSPECIFIED.,.F.,.F.,.F.)
B_SPLINE_SURFACE_WITH_KNOTS((2,2),(3,3),(0.,0.289807040991888),(0.125170525609408,
0.142682999576236),.UNSPECIFIED.)
GEOMETRIC_REPRESENTATION_ITEM()
RATIONAL_B_SPLINE_SURFACE(((0.990658108926709,0.993760979299921,0.999878046252917),
(0.990658108926709,0.993760979299921,0.999878046252917)))
REPRESENTATION_ITEM('')
SURFACE()
);
#3719=(
BOUNDED_SURFACE()
B_SPLINE_SURFACE(1,2,((#157909,#157910,#157911,#157912,#157913),(#157914,
#157915,#157916,#157917,#157918)),.UNSPECIFIED.,.F.,.F.,.F.)
B_SPLINE_SURFACE_WITH_KNOTS((2,2),(3,2,3),(0.,0.290271444049221),(0.590808523385635,
0.607982157956011,0.608572517843748),.UNSPECIFIED.)
GEOMETRIC_REPRESENTATION_ITEM()
RATIONAL_B_SPLINE_SURFACE(((0.990086238235256,0.987329216372183,0.987470879370255,
0.987470879370255,0.987470879370255),(0.990086238235256,0.987329216372183,
0.987470879370255,0.987470879370255,0.987470879370255)))
REPRESENTATION_ITEM('')
SURFACE()
);
#3720=(
BOUNDED_SURFACE()
B_SPLINE_SURFACE(1,2,((#157920,#157921,#157922),(#157923,#157924,#157925)),
 .UNSPECIFIED.,.F.,.F.,.F.)
B_SPLINE_SURFACE_WITH_KNOTS((2,2),(3,3),(0.,0.289807040991882),(0.125170525609408,
0.142682999576236),.UNSPECIFIED.)
GEOMETRIC_REPRESENTATION_ITEM()
RATIONAL_B_SPLINE_SURFACE(((0.990658108926709,0.993760979299921,0.999878046252917),
(0.990658108926709,0.993760979299921,0.999878046252917)))
REPRESENTATION_ITEM('')
SURFACE()
);
#3721=(
BOUNDED_SURFACE()
B_SPLINE_SURFACE(1,2,((#157942,#157943,#157944,#157945,#157946),(#157947,
#157948,#157949,#157950,#157951)),.UNSPECIFIED.,.F.,.F.,.F.)
B_SPLINE_SURFACE_WITH_KNOTS((2,2),(3,2,3),(0.,0.290271444045601),(0.590808523385634,
0.607982157956011,0.608572517840137),.UNSPECIFIED.)
GEOMETRIC_REPRESENTATION_ITEM()
RATIONAL_B_SPLINE_SURFACE(((0.990086238235257,0.987329216372183,0.987470879370255,
0.987470879370255,0.987470879370255),(0.990086238235256,0.987329216372183,
0.987470879370255,0.987470879370255,0.987470879370255)))
REPRESENTATION_ITEM('')
SURFACE()
);
#3722=(
BOUNDED_SURFACE()
B_SPLINE_SURFACE(1,2,((#157953,#157954,#157955),(#157956,#157957,#157958)),
 .UNSPECIFIED.,.F.,.F.,.F.)
B_SPLINE_SURFACE_WITH_KNOTS((2,2),(3,3),(0.,0.289807040993083),(0.125170525609408,
0.142682999576236),.UNSPECIFIED.)
GEOMETRIC_REPRESENTATION_ITEM()
RATIONAL_B_SPLINE_SURFACE(((0.990658108926709,0.993760979299921,0.999878046252917),
(0.990658108926709,0.993760979299921,0.999878046252917)))
REPRESENTATION_ITEM('')
SURFACE()
);
#3723=(
BOUNDED_SURFACE()
B_SPLINE_SURFACE(1,2,((#157975,#157976,#157977,#157978,#157979),(#157980,
#157981,#157982,#157983,#157984)),.UNSPECIFIED.,.F.,.F.,.F.)
B_SPLINE_SURFACE_WITH_KNOTS((2,2),(3,2,3),(0.,0.290271444054627),(0.590808523385635,
0.607982157956011,0.608572517849008),.UNSPECIFIED.)
GEOMETRIC_REPRESENTATION_ITEM()
RATIONAL_B_SPLINE_SURFACE(((0.990086238235256,0.987329216372183,0.987470879370255,
0.987470879370255,0.987470879370255),(0.990086238235256,0.987329216372183,
0.987470879370255,0.987470879370255,0.987470879370255)))
REPRESENTATION_ITEM('')
SURFACE()
);
#3724=(
BOUNDED_SURFACE()
B_SPLINE_SURFACE(1,2,((#157986,#157987,#157988),(#157989,#157990,#157991)),
 .UNSPECIFIED.,.F.,.F.,.F.)
B_SPLINE_SURFACE_WITH_KNOTS((2,2),(3,3),(0.,0.289807040991932),(0.125170525609408,
0.142682999576236),.UNSPECIFIED.)
GEOMETRIC_REPRESENTATION_ITEM()
RATIONAL_B_SPLINE_SURFACE(((0.990658108926709,0.993760979299921,0.999878046252917),
(0.990658108926709,0.993760979299921,0.999878046252917)))
REPRESENTATION_ITEM('')
SURFACE()
);
#3725=(
BOUNDED_SURFACE()
B_SPLINE_SURFACE(1,2,((#158008,#158009,#158010,#158011,#158012),(#158013,
#158014,#158015,#158016,#158017)),.UNSPECIFIED.,.F.,.F.,.F.)
B_SPLINE_SURFACE_WITH_KNOTS((2,2),(3,2,3),(0.,0.290271444013195),(0.59080852338563,
0.607982157956011,0.608572517849775),.UNSPECIFIED.)
GEOMETRIC_REPRESENTATION_ITEM()
RATIONAL_B_SPLINE_SURFACE(((0.990086238235258,0.987329216372183,0.987470879370255,
0.987470879370255,0.987470879370255),(0.990086238235258,0.987329216372183,
0.987470879370255,0.987470879370255,0.987470879370255)))
REPRESENTATION_ITEM('')
SURFACE()
);
#3726=(
BOUNDED_SURFACE()
B_SPLINE_SURFACE(1,2,((#158019,#158020,#158021),(#158022,#158023,#158024)),
 .UNSPECIFIED.,.F.,.F.,.F.)
B_SPLINE_SURFACE_WITH_KNOTS((2,2),(3,3),(0.,0.289807040991816),(0.125170525609408,
0.142682999576236),.UNSPECIFIED.)
GEOMETRIC_REPRESENTATION_ITEM()
RATIONAL_B_SPLINE_SURFACE(((0.990658108926709,0.993760979299921,0.999878046252917),
(0.990658108926709,0.993760979299921,0.999878046252917)))
REPRESENTATION_ITEM('')
SURFACE()
);
#3727=(
BOUNDED_SURFACE()
B_SPLINE_SURFACE(1,2,((#158041,#158042,#158043,#158044,#158045),(#158046,
#158047,#158048,#158049,#158050)),.UNSPECIFIED.,.F.,.F.,.F.)
B_SPLINE_SURFACE_WITH_KNOTS((2,2),(3,2,3),(0.,0.290271443990268),(0.590808523385635,
0.607982157956011,0.608572517827565),.UNSPECIFIED.)
GEOMETRIC_REPRESENTATION_ITEM()
RATIONAL_B_SPLINE_SURFACE(((0.990086238235256,0.987329216372183,0.987470879370255,
0.987470879370255,0.987470879370255),(0.990086238235256,0.987329216372183,
0.987470879370255,0.987470879370255,0.987470879370255)))
REPRESENTATION_ITEM('')
SURFACE()
);
#3728=(
BOUNDED_SURFACE()
B_SPLINE_SURFACE(1,2,((#158052,#158053,#158054),(#158055,#158056,#158057)),
 .UNSPECIFIED.,.F.,.F.,.F.)
B_SPLINE_SURFACE_WITH_KNOTS((2,2),(3,3),(0.,0.289807040991841),(0.125170525609408,
0.142682999576236),.UNSPECIFIED.)
GEOMETRIC_REPRESENTATION_ITEM()
RATIONAL_B_SPLINE_SURFACE(((0.990658108926709,0.993760979299921,0.999878046252917),
(0.990658108926709,0.993760979299921,0.999878046252917)))
REPRESENTATION_ITEM('')
SURFACE()
);
#3729=(
BOUNDED_SURFACE()
B_SPLINE_SURFACE(1,2,((#158074,#158075,#158076,#158077,#158078),(#158079,
#158080,#158081,#158082,#158083)),.UNSPECIFIED.,.F.,.F.,.F.)
B_SPLINE_SURFACE_WITH_KNOTS((2,2),(3,2,3),(0.,0.290271444010518),(0.590808523385628,
0.607982157956011,0.608572517847049),.UNSPECIFIED.)
GEOMETRIC_REPRESENTATION_ITEM()
RATIONAL_B_SPLINE_SURFACE(((0.990086238235258,0.987329216372183,0.987470879370255,
0.987470879370255,0.987470879370255),(0.990086238235258,0.987329216372183,
0.987470879370255,0.987470879370255,0.987470879370255)))
REPRESENTATION_ITEM('')
SURFACE()
);
#3730=(
BOUNDED_SURFACE()
B_SPLINE_SURFACE(1,2,((#158085,#158086,#158087),(#158088,#158089,#158090)),
 .UNSPECIFIED.,.F.,.F.,.F.)
B_SPLINE_SURFACE_WITH_KNOTS((2,2),(3,3),(0.,0.289807040991684),(0.125170525609408,
0.142682999576236),.UNSPECIFIED.)
GEOMETRIC_REPRESENTATION_ITEM()
RATIONAL_B_SPLINE_SURFACE(((0.990658108926709,0.993760979299921,0.999878046252917),
(0.990658108926709,0.993760979299921,0.999878046252917)))
REPRESENTATION_ITEM('')
SURFACE()
);
#3731=(
BOUNDED_SURFACE()
B_SPLINE_SURFACE(1,2,((#158107,#158108,#158109,#158110,#158111),(#158112,
#158113,#158114,#158115,#158116)),.UNSPECIFIED.,.F.,.F.,.F.)
B_SPLINE_SURFACE_WITH_KNOTS((2,2),(3,2,3),(0.,0.290271444030255),(0.590808523385629,
0.607982157956011,0.608572517824984),.UNSPECIFIED.)
GEOMETRIC_REPRESENTATION_ITEM()
RATIONAL_B_SPLINE_SURFACE(((0.990086238235258,0.987329216372183,0.987470879370256,
0.987470879370256,0.987470879370256),(0.990086238235258,0.987329216372183,
0.987470879370256,0.987470879370256,0.987470879370256)))
REPRESENTATION_ITEM('')
SURFACE()
);
#3732=(
BOUNDED_SURFACE()
B_SPLINE_SURFACE(1,2,((#158118,#158119,#158120,#158121,#158122),(#158123,
#158124,#158125,#158126,#158127)),.UNSPECIFIED.,.F.,.F.,.F.)
B_SPLINE_SURFACE_WITH_KNOTS((2,2),(3,2,3),(-1.00825488574708E-5,0.0614498483524471),
(0.659832011354081,0.659901408087475,0.666841081426897),.UNSPECIFIED.)
GEOMETRIC_REPRESENTATION_ITEM()
RATIONAL_B_SPLINE_SURFACE(((0.990889788836286,0.990889788836286,0.990889788836286,
0.989616401900861,0.988816334712145),(0.990889788836286,0.990889788836286,
0.990889788836286,0.989616401900861,0.988816334712145)))
REPRESENTATION_ITEM('')
SURFACE()
);
#3733=(
BOUNDED_SURFACE()
B_SPLINE_SURFACE(1,2,((#158130,#158131,#158132),(#158133,#158134,#158135)),
 .UNSPECIFIED.,.F.,.F.,.F.)
B_SPLINE_SURFACE_WITH_KNOTS((2,2),(3,3),(0.947118453120166,1.),(0.659860018385649,
0.666841081426897),.UNSPECIFIED.)
GEOMETRIC_REPRESENTATION_ITEM()
RATIONAL_B_SPLINE_SURFACE(((0.990904995179337,0.989621173673358,0.988816334712145),
(0.990904995179337,0.989621173673358,0.988816334712145)))
REPRESENTATION_ITEM('')
SURFACE()
);
#3734=(
BOUNDED_SURFACE()
B_SPLINE_SURFACE(1,2,((#158146,#158147,#158148,#158149,#158150),(#158151,
#158152,#158153,#158154,#158155)),.UNSPECIFIED.,.F.,.F.,.F.)
B_SPLINE_SURFACE_WITH_KNOTS((2,2),(3,2,3),(0.947095459621871,1.),(0.0665257254736561,
0.0714285714285714,0.0736968668684971),.UNSPECIFIED.)
GEOMETRIC_REPRESENTATION_ITEM()
RATIONAL_B_SPLINE_SURFACE(((0.996794362316491,0.998279055819231,1.,0.999203807365457,
0.998458182734336),(0.996794362316491,0.998279055819231,1.,0.999203807365457,
0.998458182734336)))
REPRESENTATION_ITEM('')
SURFACE()
);
#3735=(
BOUNDED_SURFACE()
B_SPLINE_SURFACE(1,2,((#158163,#158164,#158165,#158166,#158167),(#158168,
#158169,#158170,#158171,#158172)),.UNSPECIFIED.,.F.,.F.,.F.)
B_SPLINE_SURFACE_WITH_KNOTS((2,2),(3,2,3),(0.,0.0614231408718267),(0.0665257254736561,
0.0714285714285714,0.0736543502199108),.UNSPECIFIED.)
GEOMETRIC_REPRESENTATION_ITEM()
RATIONAL_B_SPLINE_SURFACE(((0.996794362316491,0.998279055819231,1.,0.999218731101516,
0.99848615229188),(0.996794362316491,0.998279055819231,1.,0.999218731101516,
0.99848615229188)))
REPRESENTATION_ITEM('')
SURFACE()
);
#3736=(
BOUNDED_SURFACE()
B_SPLINE_SURFACE(1,2,((#158174,#158175,#158176,#158177,#158178),(#158179,
#158180,#158181,#158182,#158183)),.UNSPECIFIED.,.F.,.F.,.F.)
B_SPLINE_SURFACE_WITH_KNOTS((2,2),(3,2,3),(0.817194107660842,1.),(0.642474614281367,
0.642857142857143,0.659901408087504),.UNSPECIFIED.)
GEOMETRIC_REPRESENTATION_ITEM()
RATIONAL_B_SPLINE_SURFACE(((0.999732896029237,0.999865728939372,1.,0.994017305594873,
0.990889788836276),(0.999732896029237,0.999865728939372,1.,0.994017305594873,
0.990889788836276)))
REPRESENTATION_ITEM('')
SURFACE()
);
#3737=(
BOUNDED_SURFACE()
B_SPLINE_SURFACE(1,2,((#158194,#158195,#158196,#158197,#158198),(#158199,
#158200,#158201,#158202,#158203)),.UNSPECIFIED.,.F.,.F.,.F.)
B_SPLINE_SURFACE_WITH_KNOTS((2,2),(3,2,3),(0.817114621578809,1.),(0.0734807488197752,
0.0736543502198967,0.0910144902320528),.UNSPECIFIED.)
GEOMETRIC_REPRESENTATION_ITEM()
RATIONAL_B_SPLINE_SURFACE(((0.998486152291889,0.998486152291889,0.998486152291889,
0.992772345172013,0.990020524139833),(0.998486152291889,0.998486152291889,
0.998486152291889,0.992772345172013,0.990020524139833)))
REPRESENTATION_ITEM('')
SURFACE()
);
#3738=(
BOUNDED_SURFACE()
B_SPLINE_SURFACE(1,2,((#158205,#158206,#158207,#158208,#158209),(#158210,
#158211,#158212,#158213,#158214)),.UNSPECIFIED.,.F.,.F.,.F.)
B_SPLINE_SURFACE_WITH_KNOTS((2,2),(3,2,3),(0.,0.0614498483525203),(0.659832011354072,
0.659901408087466,0.666841081426897),.UNSPECIFIED.)
GEOMETRIC_REPRESENTATION_ITEM()
RATIONAL_B_SPLINE_SURFACE(((0.99088978883629,0.99088978883629,0.99088978883629,
0.989616401900862,0.988816334712145),(0.990889788836289,0.990889788836289,
0.990889788836289,0.989616401900862,0.988816334712145)))
REPRESENTATION_ITEM('')
SURFACE()
);
#3739=(
BOUNDED_SURFACE()
B_SPLINE_SURFACE(1,2,((#158216,#158217,#158218),(#158219,#158220,#158221)),
 .UNSPECIFIED.,.F.,.F.,.F.)
B_SPLINE_SURFACE_WITH_KNOTS((2,2),(3,3),(0.947118453120169,1.),(0.659860018385515,
0.666841081426898),.UNSPECIFIED.)
GEOMETRIC_REPRESENTATION_ITEM()
RATIONAL_B_SPLINE_SURFACE(((0.990904995179386,0.989621173673374,0.988816334712145),
(0.990904995179386,0.989621173673374,0.988816334712145)))
REPRESENTATION_ITEM('')
SURFACE()
);
#3740=(
BOUNDED_SURFACE()
B_SPLINE_SURFACE(1,2,((#158232,#158233,#158234,#158235,#158236),(#158237,
#158238,#158239,#158240,#158241)),.UNSPECIFIED.,.F.,.F.,.F.)
B_SPLINE_SURFACE_WITH_KNOTS((2,2),(3,2,3),(0.947095459621871,1.),(0.066525725473656,
0.0714285714285714,0.0736968668684826),.UNSPECIFIED.)
GEOMETRIC_REPRESENTATION_ITEM()
RATIONAL_B_SPLINE_SURFACE(((0.996794362316491,0.998279055819231,1.,0.999203807365462,
0.998458182734345),(0.996794362316491,0.998279055819231,1.,0.999203807365462,
0.998458182734345)))
REPRESENTATION_ITEM('')
SURFACE()
);
#3741=(
BOUNDED_SURFACE()
B_SPLINE_SURFACE(1,2,((#158249,#158250,#158251,#158252,#158253),(#158254,
#158255,#158256,#158257,#158258)),.UNSPECIFIED.,.F.,.F.,.F.)
B_SPLINE_SURFACE_WITH_KNOTS((2,2),(3,2,3),(0.,0.0614231408718294),(0.0665257254736559,
0.0714285714285714,0.073654350219911),.UNSPECIFIED.)
GEOMETRIC_REPRESENTATION_ITEM()
RATIONAL_B_SPLINE_SURFACE(((0.996794362316491,0.998279055819231,1.,0.999218731101516,
0.99848615229188),(0.996794362316491,0.998279055819231,1.,0.999218731101516,
0.99848615229188)))
REPRESENTATION_ITEM('')
SURFACE()
);
#3742=(
BOUNDED_SURFACE()
B_SPLINE_SURFACE(1,2,((#158260,#158261,#158262,#158263,#158264),(#158265,
#158266,#158267,#158268,#158269)),.UNSPECIFIED.,.F.,.F.,.F.)
B_SPLINE_SURFACE_WITH_KNOTS((2,2),(3,2,3),(0.817194107660843,1.),(0.642474614281366,
0.642857142857143,0.659901408087509),.UNSPECIFIED.)
GEOMETRIC_REPRESENTATION_ITEM()
RATIONAL_B_SPLINE_SURFACE(((0.999732896029237,0.999865728939372,1.,0.994017305594872,
0.990889788836274),(0.999732896029237,0.999865728939372,1.,0.994017305594872,
0.990889788836274)))
REPRESENTATION_ITEM('')
SURFACE()
);
#3743=(
BOUNDED_SURFACE()
B_SPLINE_SURFACE(1,2,((#158280,#158281,#158282,#158283,#158284),(#158285,
#158286,#158287,#158288,#158289)),.UNSPECIFIED.,.F.,.F.,.F.)
B_SPLINE_SURFACE_WITH_KNOTS((2,2),(3,2,3),(0.817114621578807,1.),(0.0734807488197834,
0.0736543502199049,0.0910144902320525),.UNSPECIFIED.)
GEOMETRIC_REPRESENTATION_ITEM()
RATIONAL_B_SPLINE_SURFACE(((0.998486152291884,0.998486152291884,0.998486152291884,
0.992772345172012,0.990020524139833),(0.998486152291884,0.998486152291884,
0.998486152291884,0.992772345172012,0.990020524139833)))
REPRESENTATION_ITEM('')
SURFACE()
);
#3744=(
BOUNDED_SURFACE()
B_SPLINE_SURFACE(1,2,((#158291,#158292,#158293,#158294,#158295),(#158296,
#158297,#158298,#158299,#158300)),.UNSPECIFIED.,.F.,.F.,.F.)
B_SPLINE_SURFACE_WITH_KNOTS((2,2),(3,2,3),(0.,0.0614498483524406),(0.659832011354081,
0.659901408087475,0.666841081426897),.UNSPECIFIED.)
GEOMETRIC_REPRESENTATION_ITEM()
RATIONAL_B_SPLINE_SURFACE(((0.990889788836286,0.990889788836286,0.990889788836286,
0.989616401900861,0.988816334712145),(0.990889788836286,0.990889788836286,
0.990889788836286,0.989616401900861,0.988816334712145)))
REPRESENTATION_ITEM('')
SURFACE()
);
#3745=(
BOUNDED_SURFACE()
B_SPLINE_SURFACE(1,2,((#158302,#158303,#158304),(#158305,#158306,#158307)),
 .UNSPECIFIED.,.F.,.F.,.F.)
B_SPLINE_SURFACE_WITH_KNOTS((2,2),(3,3),(0.947118453120167,1.),(0.659860018385649,
0.666841081426897),.UNSPECIFIED.)
GEOMETRIC_REPRESENTATION_ITEM()
RATIONAL_B_SPLINE_SURFACE(((0.990904995179337,0.989621173673358,0.988816334712146),
(0.990904995179337,0.989621173673358,0.988816334712146)))
REPRESENTATION_ITEM('')
SURFACE()
);
#3746=(
BOUNDED_SURFACE()
B_SPLINE_SURFACE(1,2,((#158318,#158319,#158320,#158321,#158322),(#158323,
#158324,#158325,#158326,#158327)),.UNSPECIFIED.,.F.,.F.,.F.)
B_SPLINE_SURFACE_WITH_KNOTS((2,2),(3,2,3),(0.947095459621869,1.),(0.0665257254736559,
0.0714285714285714,0.0736968668684971),.UNSPECIFIED.)
GEOMETRIC_REPRESENTATION_ITEM()
RATIONAL_B_SPLINE_SURFACE(((0.996794362316491,0.998279055819231,1.,0.999203807365457,
0.998458182734336),(0.996794362316491,0.998279055819231,1.,0.999203807365457,
0.998458182734336)))
REPRESENTATION_ITEM('')
SURFACE()
);
#3747=(
BOUNDED_SURFACE()
B_SPLINE_SURFACE(1,2,((#158334,#158335,#158336,#158337,#158338),(#158339,
#158340,#158341,#158342,#158343)),.UNSPECIFIED.,.F.,.F.,.F.)
B_SPLINE_SURFACE_WITH_KNOTS((2,2),(3,2,3),(0.,0.0614231408718315),(0.0665257254736559,
0.0714285714285714,0.0736543502199111),.UNSPECIFIED.)
GEOMETRIC_REPRESENTATION_ITEM()
RATIONAL_B_SPLINE_SURFACE(((0.996794362316491,0.998279055819231,1.,0.999218731101516,
0.99848615229188),(0.996794362316491,0.998279055819231,1.,0.999218731101516,
0.99848615229188)))
REPRESENTATION_ITEM('')
SURFACE()
);
#3748=(
BOUNDED_SURFACE()
B_SPLINE_SURFACE(1,2,((#158345,#158346,#158347,#158348,#158349),(#158350,
#158351,#158352,#158353,#158354)),.UNSPECIFIED.,.F.,.F.,.F.)
B_SPLINE_SURFACE_WITH_KNOTS((2,2),(3,2,3),(0.817194107660842,1.),(0.642474614281366,
0.642857142857143,0.659901408087507),.UNSPECIFIED.)
GEOMETRIC_REPRESENTATION_ITEM()
RATIONAL_B_SPLINE_SURFACE(((0.999732896029237,0.999865728939372,1.,0.994017305594872,
0.990889788836274),(0.999732896029237,0.999865728939372,1.,0.994017305594872,
0.990889788836274)))
REPRESENTATION_ITEM('')
SURFACE()
);
#3749=(
BOUNDED_SURFACE()
B_SPLINE_SURFACE(1,2,((#158365,#158366,#158367,#158368,#158369),(#158370,
#158371,#158372,#158373,#158374)),.UNSPECIFIED.,.F.,.F.,.F.)
B_SPLINE_SURFACE_WITH_KNOTS((2,2),(3,2,3),(0.817114621578812,1.),(0.0734807488197752,
0.0736543502198967,0.0910144902320527),.UNSPECIFIED.)
GEOMETRIC_REPRESENTATION_ITEM()
RATIONAL_B_SPLINE_SURFACE(((0.998486152291889,0.998486152291889,0.998486152291889,
0.992772345172013,0.990020524139833),(0.998486152291889,0.998486152291889,
0.998486152291889,0.992772345172013,0.990020524139833)))
REPRESENTATION_ITEM('')
SURFACE()
);
#3750=(
BOUNDED_SURFACE()
B_SPLINE_SURFACE(1,2,((#158376,#158377,#158378,#158379,#158380),(#158381,
#158382,#158383,#158384,#158385)),.UNSPECIFIED.,.F.,.F.,.F.)
B_SPLINE_SURFACE_WITH_KNOTS((2,2),(3,2,3),(0.,0.0614498483525165),(0.659832011354072,
0.659901408087466,0.666841081426897),.UNSPECIFIED.)
GEOMETRIC_REPRESENTATION_ITEM()
RATIONAL_B_SPLINE_SURFACE(((0.99088978883629,0.99088978883629,0.99088978883629,
0.989616401900862,0.988816334712146),(0.99088978883629,0.99088978883629,
0.99088978883629,0.989616401900862,0.988816334712146)))
REPRESENTATION_ITEM('')
SURFACE()
);
#3751=(
BOUNDED_SURFACE()
B_SPLINE_SURFACE(1,2,((#158387,#158388,#158389),(#158390,#158391,#158392)),
 .UNSPECIFIED.,.F.,.F.,.F.)
B_SPLINE_SURFACE_WITH_KNOTS((2,2),(3,3),(0.947118453120169,1.),(0.659860018385517,
0.666841081426898),.UNSPECIFIED.)
GEOMETRIC_REPRESENTATION_ITEM()
RATIONAL_B_SPLINE_SURFACE(((0.990904995179385,0.989621173673373,0.988816334712145),
(0.990904995179385,0.989621173673373,0.988816334712145)))
REPRESENTATION_ITEM('')
SURFACE()
);
#3752=(
BOUNDED_SURFACE()
B_SPLINE_SURFACE(1,2,((#158403,#158404,#158405,#158406,#158407),(#158408,
#158409,#158410,#158411,#158412)),.UNSPECIFIED.,.F.,.F.,.F.)
B_SPLINE_SURFACE_WITH_KNOTS((2,2),(3,2,3),(0.947095459621873,1.),(0.0665257254736564,
0.0714285714285714,0.0736968668684826),.UNSPECIFIED.)
GEOMETRIC_REPRESENTATION_ITEM()
RATIONAL_B_SPLINE_SURFACE(((0.996794362316492,0.998279055819231,1.,0.999203807365462,
0.998458182734346),(0.996794362316492,0.998279055819231,1.,0.999203807365462,
0.998458182734346)))
REPRESENTATION_ITEM('')
SURFACE()
);
#3753=(
BOUNDED_SURFACE()
B_SPLINE_SURFACE(1,2,((#158420,#158421,#158422,#158423,#158424),(#158425,
#158426,#158427,#158428,#158429)),.UNSPECIFIED.,.F.,.F.,.F.)
B_SPLINE_SURFACE_WITH_KNOTS((2,2),(3,2,3),(0.,0.0614231408718255),(0.0665257254736564,
0.0714285714285714,0.073654350219911),.UNSPECIFIED.)
GEOMETRIC_REPRESENTATION_ITEM()
RATIONAL_B_SPLINE_SURFACE(((0.996794362316491,0.998279055819231,1.,0.999218731101516,
0.99848615229188),(0.996794362316491,0.998279055819231,1.,0.999218731101516,
0.99848615229188)))
REPRESENTATION_ITEM('')
SURFACE()
);
#3754=(
BOUNDED_SURFACE()
B_SPLINE_SURFACE(1,2,((#158431,#158432,#158433,#158434,#158435),(#158436,
#158437,#158438,#158439,#158440)),.UNSPECIFIED.,.F.,.F.,.F.)
B_SPLINE_SURFACE_WITH_KNOTS((2,2),(3,2,3),(0.817194107660841,1.),(0.642474614281365,
0.642857142857143,0.659901408087507),.UNSPECIFIED.)
GEOMETRIC_REPRESENTATION_ITEM()
RATIONAL_B_SPLINE_SURFACE(((0.999732896029236,0.999865728939372,1.,0.994017305594872,
0.990889788836274),(0.999732896029236,0.999865728939372,1.,0.994017305594872,
0.990889788836274)))
REPRESENTATION_ITEM('')
SURFACE()
);
#3755=(
BOUNDED_SURFACE()
B_SPLINE_SURFACE(1,2,((#158451,#158452,#158453,#158454,#158455),(#158456,
#158457,#158458,#158459,#158460)),.UNSPECIFIED.,.F.,.F.,.F.)
B_SPLINE_SURFACE_WITH_KNOTS((2,2),(3,2,3),(0.817114621578807,1.),(0.073480748819775,
0.0736543502198966,0.0910144902320526),.UNSPECIFIED.)
GEOMETRIC_REPRESENTATION_ITEM()
RATIONAL_B_SPLINE_SURFACE(((0.998486152291889,0.998486152291889,0.998486152291889,
0.992772345172014,0.990020524139833),(0.998486152291889,0.998486152291889,
0.998486152291889,0.992772345172014,0.990020524139833)))
REPRESENTATION_ITEM('')
SURFACE()
);
#3756=(
BOUNDED_SURFACE()
B_SPLINE_SURFACE(1,2,((#158462,#158463,#158464,#158465,#158466),(#158467,
#158468,#158469,#158470,#158471)),.UNSPECIFIED.,.F.,.F.,.F.)
B_SPLINE_SURFACE_WITH_KNOTS((2,2),(3,2,3),(0.,0.0614498483525202),(0.659832011354072,
0.659901408087466,0.666841081426897),.UNSPECIFIED.)
GEOMETRIC_REPRESENTATION_ITEM()
RATIONAL_B_SPLINE_SURFACE(((0.99088978883629,0.99088978883629,0.99088978883629,
0.989616401900862,0.988816334712146),(0.99088978883629,0.99088978883629,
0.99088978883629,0.989616401900862,0.988816334712146)))
REPRESENTATION_ITEM('')
SURFACE()
);
#3757=(
BOUNDED_SURFACE()
B_SPLINE_SURFACE(1,2,((#158473,#158474,#158475),(#158476,#158477,#158478)),
 .UNSPECIFIED.,.F.,.F.,.F.)
B_SPLINE_SURFACE_WITH_KNOTS((2,2),(3,3),(0.947118453120166,1.),(0.659860018385517,
0.666841081426898),.UNSPECIFIED.)
GEOMETRIC_REPRESENTATION_ITEM()
RATIONAL_B_SPLINE_SURFACE(((0.990904995179385,0.989621173673373,0.988816334712145),
(0.990904995179385,0.989621173673373,0.988816334712145)))
REPRESENTATION_ITEM('')
SURFACE()
);
#3758=(
BOUNDED_SURFACE()
B_SPLINE_SURFACE(1,2,((#158489,#158490,#158491,#158492,#158493),(#158494,
#158495,#158496,#158497,#158498)),.UNSPECIFIED.,.F.,.F.,.F.)
B_SPLINE_SURFACE_WITH_KNOTS((2,2),(3,2,3),(0.94741099344175,1.),(0.0665682420727563,
0.0714285714285714,0.0736543913087671),.UNSPECIFIED.)
GEOMETRIC_REPRESENTATION_ITEM()
RATIONAL_B_SPLINE_SURFACE(((0.996820130073177,0.99829397953792,1.,0.999218716678948,
0.998486125244442),(0.996820130073177,0.99829397953792,1.,0.999218716678948,
0.998486125244442)))
REPRESENTATION_ITEM('')
SURFACE()
);
#3759=(
BOUNDED_SURFACE()
B_SPLINE_SURFACE(1,2,((#158504,#158505,#158506,#158507,#158508),(#158509,
#158510,#158511,#158512,#158513)),.UNSPECIFIED.,.F.,.F.,.F.)
B_SPLINE_SURFACE_WITH_KNOTS((2,2),(3,2,3),(0.,0.0614231408718235),(0.0665257254736563,
0.0714285714285714,0.073654350219911),.UNSPECIFIED.)
GEOMETRIC_REPRESENTATION_ITEM()
RATIONAL_B_SPLINE_SURFACE(((0.996794362316491,0.998279055819231,1.,0.999218731101516,
0.99848615229188),(0.996794362316491,0.998279055819231,1.,0.999218731101516,
0.99848615229188)))
REPRESENTATION_ITEM('')
SURFACE()
);
#3760=(
BOUNDED_SURFACE()
B_SPLINE_SURFACE(1,2,((#158515,#158516,#158517,#158518,#158519),(#158520,
#158521,#158522,#158523,#158524)),.UNSPECIFIED.,.F.,.F.,.F.)
B_SPLINE_SURFACE_WITH_KNOTS((2,2),(3,2,3),(0.817194107660847,1.),(0.642474614281366,
0.642857142857143,0.659901408087507),.UNSPECIFIED.)
GEOMETRIC_REPRESENTATION_ITEM()
RATIONAL_B_SPLINE_SURFACE(((0.999732896029237,0.999865728939372,1.,0.994017305594872,
0.990889788836274),(0.999732896029237,0.999865728939372,1.,0.994017305594872,
0.990889788836274)))
REPRESENTATION_ITEM('')
SURFACE()
);
#3761=(
BOUNDED_SURFACE()
B_SPLINE_SURFACE(1,2,((#158535,#158536,#158537,#158538,#158539),(#158540,
#158541,#158542,#158543,#158544)),.UNSPECIFIED.,.F.,.F.,.F.)
B_SPLINE_SURFACE_WITH_KNOTS((2,2),(3,2,3),(0.817114621578816,1.),(0.073480748819775,
0.0736543502198966,0.0910144902320526),.UNSPECIFIED.)
GEOMETRIC_REPRESENTATION_ITEM()
RATIONAL_B_SPLINE_SURFACE(((0.998486152291889,0.998486152291889,0.998486152291889,
0.992772345172013,0.990020524139833),(0.998486152291889,0.998486152291889,
0.998486152291889,0.992772345172013,0.990020524139833)))
REPRESENTATION_ITEM('')
SURFACE()
);
#3762=(
BOUNDED_SURFACE()
B_SPLINE_SURFACE(1,2,((#158546,#158547,#158548,#158549,#158550),(#158551,
#158552,#158553,#158554,#158555)),.UNSPECIFIED.,.F.,.F.,.F.)
B_SPLINE_SURFACE_WITH_KNOTS((2,2),(3,2,3),(0.,0.06144984835252),(0.659832011354072,
0.659901408087466,0.666841081426897),.UNSPECIFIED.)
GEOMETRIC_REPRESENTATION_ITEM()
RATIONAL_B_SPLINE_SURFACE(((0.99088978883629,0.99088978883629,0.99088978883629,
0.989616401900862,0.988816334712146),(0.99088978883629,0.99088978883629,
0.99088978883629,0.989616401900862,0.988816334712146)))
REPRESENTATION_ITEM('')
SURFACE()
);
#3763=(
BOUNDED_SURFACE()
B_SPLINE_SURFACE(1,2,((#158557,#158558,#158559),(#158560,#158561,#158562)),
 .UNSPECIFIED.,.F.,.F.,.F.)
B_SPLINE_SURFACE_WITH_KNOTS((2,2),(3,3),(0.947118453120172,1.),(0.659860018385641,
0.666841081426897),.UNSPECIFIED.)
GEOMETRIC_REPRESENTATION_ITEM()
RATIONAL_B_SPLINE_SURFACE(((0.99090499517934,0.989621173673359,0.988816334712146),
(0.99090499517934,0.989621173673359,0.988816334712146)))
REPRESENTATION_ITEM('')
SURFACE()
);
#3764=(
BOUNDED_SURFACE()
B_SPLINE_SURFACE(1,2,((#158573,#158574,#158575,#158576,#158577),(#158578,
#158579,#158580,#158581,#158582)),.UNSPECIFIED.,.F.,.F.,.F.)
B_SPLINE_SURFACE_WITH_KNOTS((2,2),(3,2,3),(0.947095459621874,1.),(0.0665257254736566,
0.0714285714285714,0.0736968668684971),.UNSPECIFIED.)
GEOMETRIC_REPRESENTATION_ITEM()
RATIONAL_B_SPLINE_SURFACE(((0.996794362316492,0.998279055819231,1.,0.999203807365457,
0.998458182734336),(0.996794362316492,0.998279055819231,1.,0.999203807365457,
0.998458182734336)))
REPRESENTATION_ITEM('')
SURFACE()
);
#3765=(
BOUNDED_SURFACE()
B_SPLINE_SURFACE(1,2,((#158590,#158591,#158592,#158593,#158594),(#158595,
#158596,#158597,#158598,#158599)),.UNSPECIFIED.,.F.,.F.,.F.)
B_SPLINE_SURFACE_WITH_KNOTS((2,2),(3,2,3),(0.,0.0614231408718235),(0.0665257254736566,
0.0714285714285714,0.0736543502199111),.UNSPECIFIED.)
GEOMETRIC_REPRESENTATION_ITEM()
RATIONAL_B_SPLINE_SURFACE(((0.996794362316492,0.998279055819231,1.,0.999218731101516,
0.99848615229188),(0.996794362316492,0.998279055819231,1.,0.999218731101516,
0.99848615229188)))
REPRESENTATION_ITEM('')
SURFACE()
);
#3766=(
BOUNDED_SURFACE()
B_SPLINE_SURFACE(1,2,((#158601,#158602,#158603,#158604,#158605),(#158606,
#158607,#158608,#158609,#158610)),.UNSPECIFIED.,.F.,.F.,.F.)
B_SPLINE_SURFACE_WITH_KNOTS((2,2),(3,2,3),(0.817194107660845,1.),(0.642474614281363,
0.642857142857143,0.659901408087508),.UNSPECIFIED.)
GEOMETRIC_REPRESENTATION_ITEM()
RATIONAL_B_SPLINE_SURFACE(((0.999732896029235,0.999865728939371,1.,0.994017305594872,
0.990889788836274),(0.999732896029235,0.999865728939371,1.,0.994017305594872,
0.990889788836274)))
REPRESENTATION_ITEM('')
SURFACE()
);
#3767=(
BOUNDED_SURFACE()
B_SPLINE_SURFACE(1,2,((#158621,#158622,#158623,#158624,#158625),(#158626,
#158627,#158628,#158629,#158630)),.UNSPECIFIED.,.F.,.F.,.F.)
B_SPLINE_SURFACE_WITH_KNOTS((2,2),(3,2,3),(0.817114621578811,1.),(0.0734807488197752,
0.0736543502198967,0.0910144902320511),.UNSPECIFIED.)
GEOMETRIC_REPRESENTATION_ITEM()
RATIONAL_B_SPLINE_SURFACE(((0.998486152291889,0.998486152291889,0.998486152291889,
0.992772345172014,0.990020524139833),(0.998486152291889,0.998486152291889,
0.998486152291889,0.992772345172014,0.990020524139833)))
REPRESENTATION_ITEM('')
SURFACE()
);
#3768=(
BOUNDED_SURFACE()
B_SPLINE_SURFACE(1,2,((#158632,#158633,#158634,#158635,#158636),(#158637,
#158638,#158639,#158640,#158641)),.UNSPECIFIED.,.F.,.F.,.F.)
B_SPLINE_SURFACE_WITH_KNOTS((2,2),(3,2,3),(0.,0.0614498483525208),(0.659832011354072,
0.659901408087466,0.666841081426897),.UNSPECIFIED.)
GEOMETRIC_REPRESENTATION_ITEM()
RATIONAL_B_SPLINE_SURFACE(((0.990889788836289,0.990889788836289,0.990889788836289,
0.989616401900862,0.988816334712145),(0.990889788836289,0.990889788836289,
0.990889788836289,0.989616401900862,0.988816334712145)))
REPRESENTATION_ITEM('')
SURFACE()
);
#3769=(
BOUNDED_SURFACE()
B_SPLINE_SURFACE(1,2,((#158643,#158644,#158645),(#158646,#158647,#158648)),
 .UNSPECIFIED.,.F.,.F.,.F.)
B_SPLINE_SURFACE_WITH_KNOTS((2,2),(3,3),(0.947118453120167,1.),(0.659860018385514,
0.666841081426898),.UNSPECIFIED.)
GEOMETRIC_REPRESENTATION_ITEM()
RATIONAL_B_SPLINE_SURFACE(((0.990904995179386,0.989621173673373,0.988816334712145),
(0.990904995179386,0.989621173673373,0.988816334712145)))
REPRESENTATION_ITEM('')
SURFACE()
);
#3770=(
BOUNDED_SURFACE()
B_SPLINE_SURFACE(1,2,((#158659,#158660,#158661,#158662,#158663),(#158664,
#158665,#158666,#158667,#158668)),.UNSPECIFIED.,.F.,.F.,.F.)
B_SPLINE_SURFACE_WITH_KNOTS((2,2),(3,2,3),(0.947095459621876,1.),(0.0665257254736565,
0.0714285714285714,0.0736968668684827),.UNSPECIFIED.)
GEOMETRIC_REPRESENTATION_ITEM()
RATIONAL_B_SPLINE_SURFACE(((0.996794362316492,0.998279055819231,1.,0.999203807365462,
0.998458182734345),(0.996794362316492,0.998279055819231,1.,0.999203807365462,
0.998458182734345)))
REPRESENTATION_ITEM('')
SURFACE()
);
#3771=(
BOUNDED_SURFACE()
B_SPLINE_SURFACE(1,2,((#158675,#158676,#158677,#158678,#158679),(#158680,
#158681,#158682,#158683,#158684)),.UNSPECIFIED.,.F.,.F.,.F.)
B_SPLINE_SURFACE_WITH_KNOTS((2,2),(3,2,3),(0.,0.0614231408718282),(0.0665257254736563,
0.0714285714285714,0.0736543502199112),.UNSPECIFIED.)
GEOMETRIC_REPRESENTATION_ITEM()
RATIONAL_B_SPLINE_SURFACE(((0.996794362316491,0.998279055819231,1.,0.999218731101516,
0.99848615229188),(0.996794362316491,0.998279055819231,1.,0.999218731101516,
0.99848615229188)))
REPRESENTATION_ITEM('')
SURFACE()
);
#3772=(
BOUNDED_SURFACE()
B_SPLINE_SURFACE(1,2,((#158686,#158687,#158688,#158689,#158690),(#158691,
#158692,#158693,#158694,#158695)),.UNSPECIFIED.,.F.,.F.,.F.)
B_SPLINE_SURFACE_WITH_KNOTS((2,2),(3,2,3),(0.817194107660841,1.),(0.642474614281363,
0.642857142857143,0.659901408087504),.UNSPECIFIED.)
GEOMETRIC_REPRESENTATION_ITEM()
RATIONAL_B_SPLINE_SURFACE(((0.999732896029235,0.999865728939371,1.,0.994017305594873,
0.990889788836276),(0.999732896029235,0.999865728939371,1.,0.994017305594873,
0.990889788836276)))
REPRESENTATION_ITEM('')
SURFACE()
);
#3773=(
BOUNDED_SURFACE()
B_SPLINE_SURFACE(1,2,((#158706,#158707,#158708,#158709,#158710),(#158711,
#158712,#158713,#158714,#158715)),.UNSPECIFIED.,.F.,.F.,.F.)
B_SPLINE_SURFACE_WITH_KNOTS((2,2),(3,2,3),(0.817114621578807,1.),(0.0734807488197835,
0.073654350219905,0.0910144902320526),.UNSPECIFIED.)
GEOMETRIC_REPRESENTATION_ITEM()
RATIONAL_B_SPLINE_SURFACE(((0.998486152291884,0.998486152291884,0.998486152291884,
0.992772345172012,0.990020524139833),(0.998486152291884,0.998486152291884,
0.998486152291884,0.992772345172012,0.990020524139833)))
REPRESENTATION_ITEM('')
SURFACE()
);
#3774=(
BOUNDED_SURFACE()
B_SPLINE_SURFACE(1,2,((#158717,#158718,#158719,#158720,#158721),(#158722,
#158723,#158724,#158725,#158726)),.UNSPECIFIED.,.F.,.F.,.F.)
B_SPLINE_SURFACE_WITH_KNOTS((2,2),(3,2,3),(0.,0.0614498483524431),(0.659832011354081,
0.659901408087475,0.666841081426897),.UNSPECIFIED.)
GEOMETRIC_REPRESENTATION_ITEM()
RATIONAL_B_SPLINE_SURFACE(((0.990889788836286,0.990889788836286,0.990889788836286,
0.989616401900861,0.988816334712145),(0.990889788836286,0.990889788836286,
0.990889788836286,0.989616401900861,0.988816334712145)))
REPRESENTATION_ITEM('')
SURFACE()
);
#3775=(
BOUNDED_SURFACE()
B_SPLINE_SURFACE(1,2,((#158728,#158729,#158730),(#158731,#158732,#158733)),
 .UNSPECIFIED.,.F.,.F.,.F.)
B_SPLINE_SURFACE_WITH_KNOTS((2,2),(3,3),(0.94711845312017,1.),(0.659860018385515,
0.666841081426897),.UNSPECIFIED.)
GEOMETRIC_REPRESENTATION_ITEM()
RATIONAL_B_SPLINE_SURFACE(((0.990904995179386,0.989621173673373,0.988816334712145),
(0.990904995179386,0.989621173673373,0.988816334712145)))
REPRESENTATION_ITEM('')
SURFACE()
);
#3776=(
BOUNDED_SURFACE()
B_SPLINE_SURFACE(1,2,((#158744,#158745,#158746,#158747,#158748),(#158749,
#158750,#158751,#158752,#158753)),.UNSPECIFIED.,.F.,.F.,.F.)
B_SPLINE_SURFACE_WITH_KNOTS((2,2),(3,2,3),(0.947095459621868,1.),(0.0665257254736558,
0.0714285714285714,0.0736968668684909),.UNSPECIFIED.)
GEOMETRIC_REPRESENTATION_ITEM()
RATIONAL_B_SPLINE_SURFACE(((0.996794362316491,0.998279055819231,1.,0.999203807365459,
0.99845818273434),(0.996794362316491,0.998279055819231,1.,0.999203807365459,
0.99845818273434)))
REPRESENTATION_ITEM('')
SURFACE()
);
#3777=(
BOUNDED_SURFACE()
B_SPLINE_SURFACE(1,2,((#158761,#158762,#158763,#158764,#158765),(#158766,
#158767,#158768,#158769,#158770)),.UNSPECIFIED.,.F.,.F.,.F.)
B_SPLINE_SURFACE_WITH_KNOTS((2,2),(3,2,3),(0.,0.0614231408718295),(0.0665257254736558,
0.0714285714285714,0.0736543502199111),.UNSPECIFIED.)
GEOMETRIC_REPRESENTATION_ITEM()
RATIONAL_B_SPLINE_SURFACE(((0.996794362316491,0.998279055819231,1.,0.999218731101516,
0.99848615229188),(0.996794362316491,0.998279055819231,1.,0.999218731101516,
0.99848615229188)))
REPRESENTATION_ITEM('')
SURFACE()
);
#3778=(
BOUNDED_SURFACE()
B_SPLINE_SURFACE(1,2,((#158772,#158773,#158774,#158775,#158776),(#158777,
#158778,#158779,#158780,#158781)),.UNSPECIFIED.,.F.,.F.,.F.)
B_SPLINE_SURFACE_WITH_KNOTS((2,2),(3,2,3),(0.817194107660844,1.),(0.642474614281363,
0.642857142857143,0.659901408087509),.UNSPECIFIED.)
GEOMETRIC_REPRESENTATION_ITEM()
RATIONAL_B_SPLINE_SURFACE(((0.999732896029235,0.999865728939371,1.,0.994017305594872,
0.990889788836274),(0.999732896029235,0.999865728939371,1.,0.994017305594872,
0.990889788836274)))
REPRESENTATION_ITEM('')
SURFACE()
);
#3779=(
BOUNDED_SURFACE()
B_SPLINE_SURFACE(1,2,((#158792,#158793,#158794,#158795,#158796),(#158797,
#158798,#158799,#158800,#158801)),.UNSPECIFIED.,.F.,.F.,.F.)
B_SPLINE_SURFACE_WITH_KNOTS((2,2),(3,2,3),(0.817114621578811,1.),(0.073480748819775,
0.0736543502198966,0.0910144902320527),.UNSPECIFIED.)
GEOMETRIC_REPRESENTATION_ITEM()
RATIONAL_B_SPLINE_SURFACE(((0.998486152291889,0.998486152291889,0.998486152291889,
0.992772345172014,0.990020524139833),(0.998486152291889,0.998486152291889,
0.998486152291889,0.992772345172014,0.990020524139833)))
REPRESENTATION_ITEM('')
SURFACE()
);
#3780=(
BOUNDED_SURFACE()
B_SPLINE_SURFACE(1,2,((#158803,#158804,#158805,#158806,#158807),(#158808,
#158809,#158810,#158811,#158812)),.UNSPECIFIED.,.F.,.F.,.F.)
B_SPLINE_SURFACE_WITH_KNOTS((2,2),(3,2,3),(0.,0.0614498483525196),(0.659832011354072,
0.659901408087466,0.666841081426896),.UNSPECIFIED.)
GEOMETRIC_REPRESENTATION_ITEM()
RATIONAL_B_SPLINE_SURFACE(((0.99088978883629,0.99088978883629,0.99088978883629,
0.989616401900862,0.988816334712146),(0.990889788836289,0.990889788836289,
0.990889788836289,0.989616401900862,0.988816334712146)))
REPRESENTATION_ITEM('')
SURFACE()
);
#3781=(
BOUNDED_SURFACE()
B_SPLINE_SURFACE(1,2,((#158814,#158815,#158816),(#158817,#158818,#158819)),
 .UNSPECIFIED.,.F.,.F.,.F.)
B_SPLINE_SURFACE_WITH_KNOTS((2,2),(3,3),(0.947118453120172,1.),(0.659860018385514,
0.666841081426897),.UNSPECIFIED.)
GEOMETRIC_REPRESENTATION_ITEM()
RATIONAL_B_SPLINE_SURFACE(((0.990904995179386,0.989621173673374,0.988816334712145),
(0.990904995179386,0.989621173673374,0.988816334712145)))
REPRESENTATION_ITEM('')
SURFACE()
);
#3782=(
BOUNDED_SURFACE()
B_SPLINE_SURFACE(1,2,((#158830,#158831,#158832,#158833,#158834),(#158835,
#158836,#158837,#158838,#158839)),.UNSPECIFIED.,.F.,.F.,.F.)
B_SPLINE_SURFACE_WITH_KNOTS((2,2),(3,2,3),(0.94709545962187,1.),(0.0665257254736561,
0.0714285714285714,0.0736968668684826),.UNSPECIFIED.)
GEOMETRIC_REPRESENTATION_ITEM()
RATIONAL_B_SPLINE_SURFACE(((0.996794362316491,0.998279055819231,1.,0.999203807365462,
0.998458182734345),(0.996794362316491,0.998279055819231,1.,0.999203807365462,
0.998458182734345)))
REPRESENTATION_ITEM('')
SURFACE()
);
#3783=(
BOUNDED_SURFACE()
B_SPLINE_SURFACE(1,2,((#158846,#158847,#158848,#158849,#158850),(#158851,
#158852,#158853,#158854,#158855)),.UNSPECIFIED.,.F.,.F.,.F.)
B_SPLINE_SURFACE_WITH_KNOTS((2,2),(3,2,3),(0.,0.0614231408718267),(0.066525725473656,
0.0714285714285714,0.073654350219911),.UNSPECIFIED.)
GEOMETRIC_REPRESENTATION_ITEM()
RATIONAL_B_SPLINE_SURFACE(((0.996794362316491,0.998279055819231,1.,0.999218731101516,
0.99848615229188),(0.996794362316491,0.998279055819231,1.,0.999218731101516,
0.99848615229188)))
REPRESENTATION_ITEM('')
SURFACE()
);
#3784=(
BOUNDED_SURFACE()
B_SPLINE_SURFACE(1,2,((#158857,#158858,#158859,#158860,#158861),(#158862,
#158863,#158864,#158865,#158866)),.UNSPECIFIED.,.F.,.F.,.F.)
B_SPLINE_SURFACE_WITH_KNOTS((2,2),(3,2,3),(0.817194107660851,1.),(0.642474614281365,
0.642857142857143,0.659901408087504),.UNSPECIFIED.)
GEOMETRIC_REPRESENTATION_ITEM()
RATIONAL_B_SPLINE_SURFACE(((0.999732896029236,0.999865728939372,1.,0.994017305594874,
0.990889788836276),(0.999732896029236,0.999865728939372,1.,0.994017305594874,
0.990889788836276)))
REPRESENTATION_ITEM('')
SURFACE()
);
#3785=(
BOUNDED_SURFACE()
B_SPLINE_SURFACE(1,2,((#158877,#158878,#158879,#158880,#158881),(#158882,
#158883,#158884,#158885,#158886)),.UNSPECIFIED.,.F.,.F.,.F.)
B_SPLINE_SURFACE_WITH_KNOTS((2,2),(3,2,3),(0.81711462157881,1.),(0.073480748819775,
0.0736543502198966,0.0910144902320525),.UNSPECIFIED.)
GEOMETRIC_REPRESENTATION_ITEM()
RATIONAL_B_SPLINE_SURFACE(((0.998486152291889,0.998486152291889,0.998486152291889,
0.992772345172014,0.990020524139833),(0.998486152291889,0.998486152291889,
0.998486152291889,0.992772345172013,0.990020524139833)))
REPRESENTATION_ITEM('')
SURFACE()
);
#3786=(
BOUNDED_SURFACE()
B_SPLINE_SURFACE(1,2,((#158888,#158889,#158890,#158891,#158892),(#158893,
#158894,#158895,#158896,#158897)),.UNSPECIFIED.,.F.,.F.,.F.)
B_SPLINE_SURFACE_WITH_KNOTS((2,2),(3,2,3),(0.,0.0614498483525191),(0.659832011354072,
0.659901408087466,0.666841081426896),.UNSPECIFIED.)
GEOMETRIC_REPRESENTATION_ITEM()
RATIONAL_B_SPLINE_SURFACE(((0.99088978883629,0.99088978883629,0.99088978883629,
0.989616401900862,0.988816334712146),(0.99088978883629,0.99088978883629,
0.99088978883629,0.989616401900862,0.988816334712146)))
REPRESENTATION_ITEM('')
SURFACE()
);
#3787=(
BOUNDED_SURFACE()
B_SPLINE_SURFACE(1,2,((#158899,#158900,#158901),(#158902,#158903,#158904)),
 .UNSPECIFIED.,.F.,.F.,.F.)
B_SPLINE_SURFACE_WITH_KNOTS((2,2),(3,3),(0.947118453120174,1.),(0.659860018385517,
0.666841081426897),.UNSPECIFIED.)
GEOMETRIC_REPRESENTATION_ITEM()
RATIONAL_B_SPLINE_SURFACE(((0.990904995179385,0.989621173673373,0.988816334712145),
(0.990904995179385,0.989621173673373,0.988816334712145)))
REPRESENTATION_ITEM('')
SURFACE()
);
#3788=(
BOUNDED_SURFACE()
B_SPLINE_SURFACE(1,2,((#158915,#158916,#158917,#158918,#158919),(#158920,
#158921,#158922,#158923,#158924)),.UNSPECIFIED.,.F.,.F.,.F.)
B_SPLINE_SURFACE_WITH_KNOTS((2,2),(3,2,3),(0.94709545962187,1.),(0.066525725473656,
0.0714285714285714,0.0736968668684825),.UNSPECIFIED.)
GEOMETRIC_REPRESENTATION_ITEM()
RATIONAL_B_SPLINE_SURFACE(((0.996794362316491,0.998279055819231,1.,0.999203807365462,
0.998458182734346),(0.996794362316491,0.998279055819231,1.,0.999203807365462,
0.998458182734346)))
REPRESENTATION_ITEM('')
SURFACE()
);
#3789=(
BOUNDED_SURFACE()
B_SPLINE_SURFACE(1,2,((#158932,#158933,#158934,#158935,#158936),(#158937,
#158938,#158939,#158940,#158941)),.UNSPECIFIED.,.F.,.F.,.F.)
B_SPLINE_SURFACE_WITH_KNOTS((2,2),(3,2,3),(0.,0.0614231408718213),(0.0665257254736561,
0.0714285714285714,0.0736543502199202),.UNSPECIFIED.)
GEOMETRIC_REPRESENTATION_ITEM()
RATIONAL_B_SPLINE_SURFACE(((0.996794362316491,0.998279055819231,1.,0.999218731101513,
0.998486152291874),(0.996794362316491,0.998279055819231,1.,0.999218731101513,
0.998486152291874)))
REPRESENTATION_ITEM('')
SURFACE()
);
#3790=(
BOUNDED_SURFACE()
B_SPLINE_SURFACE(1,2,((#158943,#158944,#158945,#158946,#158947),(#158948,
#158949,#158950,#158951,#158952)),.UNSPECIFIED.,.F.,.F.,.F.)
B_SPLINE_SURFACE_WITH_KNOTS((2,2),(3,2,3),(0.81719410766085,1.),(0.642474614281365,
0.642857142857143,0.659901408087502),.UNSPECIFIED.)
GEOMETRIC_REPRESENTATION_ITEM()
RATIONAL_B_SPLINE_SURFACE(((0.999732896029236,0.999865728939372,1.,0.994017305594874,
0.990889788836276),(0.999732896029236,0.999865728939372,1.,0.994017305594874,
0.990889788836276)))
REPRESENTATION_ITEM('')
SURFACE()
);
#3791=(
BOUNDED_SURFACE()
B_SPLINE_SURFACE(1,2,((#158963,#158964,#158965,#158966,#158967),(#158968,
#158969,#158970,#158971,#158972)),.UNSPECIFIED.,.F.,.F.,.F.)
B_SPLINE_SURFACE_WITH_KNOTS((2,2),(3,2,3),(0.817114621578809,1.),(0.0734807488197752,
0.0736543502198967,0.0910144902320525),.UNSPECIFIED.)
GEOMETRIC_REPRESENTATION_ITEM()
RATIONAL_B_SPLINE_SURFACE(((0.998486152291889,0.998486152291889,0.998486152291889,
0.992772345172014,0.990020524139833),(0.998486152291889,0.998486152291889,
0.998486152291889,0.992772345172014,0.990020524139833)))
REPRESENTATION_ITEM('')
SURFACE()
);
#3792=(
BOUNDED_SURFACE()
B_SPLINE_SURFACE(1,2,((#158974,#158975,#158976,#158977,#158978),(#158979,
#158980,#158981,#158982,#158983)),.UNSPECIFIED.,.F.,.F.,.F.)
B_SPLINE_SURFACE_WITH_KNOTS((2,2),(3,2,3),(0.,0.0614498483525196),(0.659832011354072,
0.659901408087466,0.666841081426897),.UNSPECIFIED.)
GEOMETRIC_REPRESENTATION_ITEM()
RATIONAL_B_SPLINE_SURFACE(((0.99088978883629,0.99088978883629,0.99088978883629,
0.989616401900862,0.988816334712146),(0.99088978883629,0.99088978883629,
0.99088978883629,0.989616401900862,0.988816334712146)))
REPRESENTATION_ITEM('')
SURFACE()
);
#3793=(
BOUNDED_SURFACE()
B_SPLINE_SURFACE(1,2,((#158985,#158986,#158987),(#158988,#158989,#158990)),
 .UNSPECIFIED.,.F.,.F.,.F.)
B_SPLINE_SURFACE_WITH_KNOTS((2,2),(3,3),(0.947118453120175,1.),(0.659860018385517,
0.666841081426897),.UNSPECIFIED.)
GEOMETRIC_REPRESENTATION_ITEM()
RATIONAL_B_SPLINE_SURFACE(((0.990904995179386,0.989621173673373,0.988816334712145),
(0.990904995179386,0.989621173673373,0.988816334712145)))
REPRESENTATION_ITEM('')
SURFACE()
);
#3794=(
BOUNDED_SURFACE()
B_SPLINE_SURFACE(1,2,((#159001,#159002,#159003,#159004,#159005),(#159006,
#159007,#159008,#159009,#159010)),.UNSPECIFIED.,.F.,.F.,.F.)
B_SPLINE_SURFACE_WITH_KNOTS((2,2),(3,2,3),(0.947095459621871,1.),(0.0665257254736559,
0.0714285714285714,0.0736968668684826),.UNSPECIFIED.)
GEOMETRIC_REPRESENTATION_ITEM()
RATIONAL_B_SPLINE_SURFACE(((0.996794362316491,0.998279055819231,1.,0.999203807365462,
0.998458182734345),(0.996794362316491,0.998279055819231,1.,0.999203807365462,
0.998458182734345)))
REPRESENTATION_ITEM('')
SURFACE()
);
#3795=(
BOUNDED_SURFACE()
B_SPLINE_SURFACE(1,2,((#159018,#159019,#159020,#159021,#159022),(#159023,
#159024,#159025,#159026,#159027)),.UNSPECIFIED.,.F.,.F.,.F.)
B_SPLINE_SURFACE_WITH_KNOTS((2,2),(3,2,3),(0.,0.0614231408718263),(0.0665257254736557,
0.0714285714285714,0.0736543502199203),.UNSPECIFIED.)
GEOMETRIC_REPRESENTATION_ITEM()
RATIONAL_B_SPLINE_SURFACE(((0.996794362316491,0.998279055819231,1.,0.999218731101513,
0.998486152291874),(0.996794362316491,0.998279055819231,1.,0.999218731101513,
0.998486152291874)))
REPRESENTATION_ITEM('')
SURFACE()
);
#3796=(
BOUNDED_SURFACE()
B_SPLINE_SURFACE(1,2,((#159029,#159030,#159031,#159032,#159033),(#159034,
#159035,#159036,#159037,#159038)),.UNSPECIFIED.,.F.,.F.,.F.)
B_SPLINE_SURFACE_WITH_KNOTS((2,2),(3,2,3),(0.817194107660848,1.),(0.642474614281366,
0.642857142857143,0.659901408087502),.UNSPECIFIED.)
GEOMETRIC_REPRESENTATION_ITEM()
RATIONAL_B_SPLINE_SURFACE(((0.999732896029237,0.999865728939372,1.,0.994017305594874,
0.990889788836277),(0.999732896029237,0.999865728939372,1.,0.994017305594874,
0.990889788836277)))
REPRESENTATION_ITEM('')
SURFACE()
);
#3797=(
BOUNDED_SURFACE()
B_SPLINE_SURFACE(1,2,((#159049,#159050,#159051,#159052,#159053),(#159054,
#159055,#159056,#159057,#159058)),.UNSPECIFIED.,.F.,.F.,.F.)
B_SPLINE_SURFACE_WITH_KNOTS((2,2),(3,2,3),(0.817114621578814,1.),(0.0734807488197752,
0.0736543502198967,0.0910144902320526),.UNSPECIFIED.)
GEOMETRIC_REPRESENTATION_ITEM()
RATIONAL_B_SPLINE_SURFACE(((0.998486152291889,0.998486152291889,0.998486152291889,
0.992772345172013,0.990020524139833),(0.998486152291889,0.998486152291889,
0.998486152291889,0.992772345172013,0.990020524139833)))
REPRESENTATION_ITEM('')
SURFACE()
);
#3798=(
BOUNDED_SURFACE()
B_SPLINE_SURFACE(1,2,((#159060,#159061,#159062,#159063,#159064),(#159065,
#159066,#159067,#159068,#159069)),.UNSPECIFIED.,.F.,.F.,.F.)
B_SPLINE_SURFACE_WITH_KNOTS((2,2),(3,2,3),(0.,0.0614498483525172),(0.659832011354072,
0.659901408087466,0.666841081426896),.UNSPECIFIED.)
GEOMETRIC_REPRESENTATION_ITEM()
RATIONAL_B_SPLINE_SURFACE(((0.99088978883629,0.99088978883629,0.99088978883629,
0.989616401900862,0.988816334712146),(0.99088978883629,0.99088978883629,
0.99088978883629,0.989616401900862,0.988816334712146)))
REPRESENTATION_ITEM('')
SURFACE()
);
#3799=(
BOUNDED_SURFACE()
B_SPLINE_SURFACE(1,2,((#159071,#159072,#159073),(#159074,#159075,#159076)),
 .UNSPECIFIED.,.F.,.F.,.F.)
B_SPLINE_SURFACE_WITH_KNOTS((2,2),(3,3),(0.947118453120173,1.),(0.659860018385517,
0.666841081426897),.UNSPECIFIED.)
GEOMETRIC_REPRESENTATION_ITEM()
RATIONAL_B_SPLINE_SURFACE(((0.990904995179385,0.989621173673373,0.988816334712145),
(0.990904995179385,0.989621173673373,0.988816334712145)))
REPRESENTATION_ITEM('')
SURFACE()
);
#3800=(
BOUNDED_SURFACE()
B_SPLINE_SURFACE(1,2,((#159087,#159088,#159089,#159090,#159091),(#159092,
#159093,#159094,#159095,#159096)),.UNSPECIFIED.,.F.,.F.,.F.)
B_SPLINE_SURFACE_WITH_KNOTS((2,2),(3,2,3),(0.947095459621873,1.),(0.0665257254736566,
0.0714285714285714,0.0736968668684826),.UNSPECIFIED.)
GEOMETRIC_REPRESENTATION_ITEM()
RATIONAL_B_SPLINE_SURFACE(((0.996794362316492,0.998279055819231,1.,0.999203807365462,
0.998458182734345),(0.996794362316492,0.998279055819231,1.,0.999203807365462,
0.998458182734345)))
REPRESENTATION_ITEM('')
SURFACE()
);
#3801=(
BOUNDED_SURFACE()
B_SPLINE_SURFACE(1,2,((#159104,#159105,#159106,#159107,#159108),(#159109,
#159110,#159111,#159112,#159113)),.UNSPECIFIED.,.F.,.F.,.F.)
B_SPLINE_SURFACE_WITH_KNOTS((2,2),(3,2,3),(0.,0.0614231408718205),(0.0665257254736566,
0.0714285714285714,0.0736543502199202),.UNSPECIFIED.)
GEOMETRIC_REPRESENTATION_ITEM()
RATIONAL_B_SPLINE_SURFACE(((0.996794362316492,0.998279055819231,1.,0.999218731101513,
0.998486152291874),(0.996794362316492,0.998279055819231,1.,0.999218731101513,
0.998486152291874)))
REPRESENTATION_ITEM('')
SURFACE()
);
#3802=(
BOUNDED_SURFACE()
B_SPLINE_SURFACE(1,2,((#159115,#159116,#159117,#159118,#159119),(#159120,
#159121,#159122,#159123,#159124)),.UNSPECIFIED.,.F.,.F.,.F.)
B_SPLINE_SURFACE_WITH_KNOTS((2,2),(3,2,3),(0.817194107660853,1.),(0.642474614281367,
0.642857142857143,0.659901408087502),.UNSPECIFIED.)
GEOMETRIC_REPRESENTATION_ITEM()
RATIONAL_B_SPLINE_SURFACE(((0.999732896029238,0.999865728939373,1.,0.994017305594874,
0.990889788836276),(0.999732896029238,0.999865728939373,1.,0.994017305594874,
0.990889788836276)))
REPRESENTATION_ITEM('')
SURFACE()
);
#3803=(
BOUNDED_SURFACE()
B_SPLINE_SURFACE(1,2,((#159135,#159136,#159137,#159138,#159139),(#159140,
#159141,#159142,#159143,#159144)),.UNSPECIFIED.,.F.,.F.,.F.)
B_SPLINE_SURFACE_WITH_KNOTS((2,2),(3,2,3),(0.817114621578814,1.),(0.0734807488197738,
0.0736543502198954,0.0910144902320515),.UNSPECIFIED.)
GEOMETRIC_REPRESENTATION_ITEM()
RATIONAL_B_SPLINE_SURFACE(((0.99848615229189,0.99848615229189,0.99848615229189,
0.992772345172014,0.990020524139833),(0.99848615229189,0.99848615229189,
0.99848615229189,0.992772345172014,0.990020524139833)))
REPRESENTATION_ITEM('')
SURFACE()
);
#3804=(
BOUNDED_SURFACE()
B_SPLINE_SURFACE(1,2,((#159146,#159147,#159148,#159149,#159150),(#159151,
#159152,#159153,#159154,#159155)),.UNSPECIFIED.,.F.,.F.,.F.)
B_SPLINE_SURFACE_WITH_KNOTS((2,2),(3,2,3),(0.,0.061449848352509),(0.659832011354073,
0.659901408087467,0.666841081426896),.UNSPECIFIED.)
GEOMETRIC_REPRESENTATION_ITEM()
RATIONAL_B_SPLINE_SURFACE(((0.990889788836289,0.990889788836289,0.990889788836289,
0.989616401900862,0.988816334712146),(0.990889788836289,0.990889788836289,
0.990889788836289,0.989616401900862,0.988816334712146)))
REPRESENTATION_ITEM('')
SURFACE()
);
#3805=(
BOUNDED_SURFACE()
B_SPLINE_SURFACE(1,2,((#159157,#159158,#159159),(#159160,#159161,#159162)),
 .UNSPECIFIED.,.F.,.F.,.F.)
B_SPLINE_SURFACE_WITH_KNOTS((2,2),(3,3),(0.947118453120178,1.),(0.659860018385642,
0.666841081426896),.UNSPECIFIED.)
GEOMETRIC_REPRESENTATION_ITEM()
RATIONAL_B_SPLINE_SURFACE(((0.990904995179339,0.989621173673359,0.988816334712145),
(0.990904995179339,0.989621173673359,0.988816334712145)))
REPRESENTATION_ITEM('')
SURFACE()
);
#3806=(
BOUNDED_SURFACE()
B_SPLINE_SURFACE(1,2,((#159173,#159174,#159175,#159176,#159177),(#159178,
#159179,#159180,#159181,#159182)),.UNSPECIFIED.,.F.,.F.,.F.)
B_SPLINE_SURFACE_WITH_KNOTS((2,2),(3,2,3),(0.947095459621874,1.),(0.0665257254736559,
0.0714285714285714,0.073696866868496),.UNSPECIFIED.)
GEOMETRIC_REPRESENTATION_ITEM()
RATIONAL_B_SPLINE_SURFACE(((0.996794362316491,0.998279055819231,1.,0.999203807365457,
0.998458182734337),(0.996794362316491,0.998279055819231,1.,0.999203807365457,
0.998458182734337)))
REPRESENTATION_ITEM('')
SURFACE()
);
#3807=(
BOUNDED_SURFACE()
B_SPLINE_SURFACE(1,2,((#159189,#159190,#159191,#159192,#159193),(#159194,
#159195,#159196,#159197,#159198)),.UNSPECIFIED.,.F.,.F.,.F.)
B_SPLINE_SURFACE_WITH_KNOTS((2,2),(3,2,3),(0.,0.0614231408718213),(0.0665257254736558,
0.0714285714285714,0.0736543502199218),.UNSPECIFIED.)
GEOMETRIC_REPRESENTATION_ITEM()
RATIONAL_B_SPLINE_SURFACE(((0.996794362316491,0.998279055819231,1.,0.999218731101512,
0.998486152291873),(0.996794362316491,0.998279055819231,1.,0.999218731101512,
0.998486152291873)))
REPRESENTATION_ITEM('')
SURFACE()
);
#3808=(
BOUNDED_SURFACE()
B_SPLINE_SURFACE(1,2,((#159200,#159201,#159202,#159203,#159204),(#159205,
#159206,#159207,#159208,#159209)),.UNSPECIFIED.,.F.,.F.,.F.)
B_SPLINE_SURFACE_WITH_KNOTS((2,2),(3,2,3),(0.817194107660858,1.),(0.642474614281364,
0.642857142857143,0.659901408087509),.UNSPECIFIED.)
GEOMETRIC_REPRESENTATION_ITEM()
RATIONAL_B_SPLINE_SURFACE(((0.999732896029236,0.999865728939372,1.,0.994017305594872,
0.990889788836274),(0.999732896029236,0.999865728939372,1.,0.994017305594872,
0.990889788836274)))
REPRESENTATION_ITEM('')
SURFACE()
);
#3809=(
BOUNDED_SURFACE()
B_SPLINE_SURFACE(1,2,((#159220,#159221,#159222,#159223,#159224),(#159225,
#159226,#159227,#159228,#159229)),.UNSPECIFIED.,.F.,.F.,.F.)
B_SPLINE_SURFACE_WITH_KNOTS((2,2),(3,2,3),(0.817114621578823,1.),(0.0734807488197823,
0.0736543502199038,0.0910144902320512),.UNSPECIFIED.)
GEOMETRIC_REPRESENTATION_ITEM()
RATIONAL_B_SPLINE_SURFACE(((0.998486152291885,0.998486152291885,0.998486152291885,
0.992772345172013,0.990020524139833),(0.998486152291885,0.998486152291885,
0.998486152291885,0.992772345172013,0.990020524139833)))
REPRESENTATION_ITEM('')
SURFACE()
);
#3810=(
BOUNDED_SURFACE()
B_SPLINE_SURFACE(1,2,((#159231,#159232,#159233,#159234,#159235),(#159236,
#159237,#159238,#159239,#159240)),.UNSPECIFIED.,.F.,.F.,.F.)
B_SPLINE_SURFACE_WITH_KNOTS((2,2),(3,2,3),(0.,0.061449848352437),(0.659832011354082,
0.659901408087476,0.666841081426897),.UNSPECIFIED.)
GEOMETRIC_REPRESENTATION_ITEM()
RATIONAL_B_SPLINE_SURFACE(((0.990889788836286,0.990889788836286,0.990889788836286,
0.989616401900861,0.988816334712145),(0.990889788836286,0.990889788836286,
0.990889788836286,0.989616401900861,0.988816334712145)))
REPRESENTATION_ITEM('')
SURFACE()
);
#3811=(
BOUNDED_SURFACE()
B_SPLINE_SURFACE(1,2,((#159242,#159243,#159244),(#159245,#159246,#159247)),
 .UNSPECIFIED.,.F.,.F.,.F.)
B_SPLINE_SURFACE_WITH_KNOTS((2,2),(3,3),(0.947118453120176,1.),(0.659860018385516,
0.666841081426898),.UNSPECIFIED.)
GEOMETRIC_REPRESENTATION_ITEM()
RATIONAL_B_SPLINE_SURFACE(((0.990904995179386,0.989621173673373,0.988816334712145),
(0.990904995179386,0.989621173673373,0.988816334712145)))
REPRESENTATION_ITEM('')
SURFACE()
);
#3812=(
BOUNDED_SURFACE()
B_SPLINE_SURFACE(1,2,((#159258,#159259,#159260,#159261,#159262),(#159263,
#159264,#159265,#159266,#159267)),.UNSPECIFIED.,.F.,.F.,.F.)
B_SPLINE_SURFACE_WITH_KNOTS((2,2),(3,2,3),(0.947095459621877,1.),(0.0665257254736565,
0.0714285714285714,0.0736968668684898),.UNSPECIFIED.)
GEOMETRIC_REPRESENTATION_ITEM()
RATIONAL_B_SPLINE_SURFACE(((0.996794362316492,0.998279055819231,1.,0.999203807365459,
0.998458182734341),(0.996794362316492,0.998279055819231,1.,0.999203807365459,
0.998458182734341)))
REPRESENTATION_ITEM('')
SURFACE()
);
#3813=(
BOUNDED_SURFACE()
B_SPLINE_SURFACE(1,2,((#159274,#159275,#159276,#159277,#159278),(#159279,
#159280,#159281,#159282,#159283)),.UNSPECIFIED.,.F.,.F.,.F.)
B_SPLINE_SURFACE_WITH_KNOTS((2,2),(3,2,3),(0.,0.0614231408718177),(0.0665257254736564,
0.0714285714285714,0.0736543502199223),.UNSPECIFIED.)
GEOMETRIC_REPRESENTATION_ITEM()
RATIONAL_B_SPLINE_SURFACE(((0.996794362316491,0.998279055819231,1.,0.999218731101512,
0.998486152291872),(0.996794362316491,0.998279055819231,1.,0.999218731101512,
0.998486152291872)))
REPRESENTATION_ITEM('')
SURFACE()
);
#3814=(
BOUNDED_SURFACE()
B_SPLINE_SURFACE(1,2,((#159285,#159286,#159287,#159288,#159289),(#159290,
#159291,#159292,#159293,#159294)),.UNSPECIFIED.,.F.,.F.,.F.)
B_SPLINE_SURFACE_WITH_KNOTS((2,2),(3,2,3),(0.81719410766085,1.),(0.642474614281364,
0.642857142857143,0.65990140808751),.UNSPECIFIED.)
GEOMETRIC_REPRESENTATION_ITEM()
RATIONAL_B_SPLINE_SURFACE(((0.999732896029236,0.999865728939372,1.,0.994017305594871,
0.990889788836273),(0.999732896029236,0.999865728939372,1.,0.994017305594871,
0.990889788836273)))
REPRESENTATION_ITEM('')
SURFACE()
);
#3815=(
BOUNDED_SURFACE()
B_SPLINE_SURFACE(1,2,((#159305,#159306,#159307,#159308,#159309),(#159310,
#159311,#159312,#159313,#159314)),.UNSPECIFIED.,.F.,.F.,.F.)
B_SPLINE_SURFACE_WITH_KNOTS((2,2),(3,2,3),(0.817114621578814,1.),(0.0734807488197824,
0.0736543502199039,0.0910144902320515),.UNSPECIFIED.)
GEOMETRIC_REPRESENTATION_ITEM()
RATIONAL_B_SPLINE_SURFACE(((0.998486152291885,0.998486152291885,0.998486152291885,
0.992772345172013,0.990020524139833),(0.998486152291885,0.998486152291885,
0.998486152291885,0.992772345172013,0.990020524139833)))
REPRESENTATION_ITEM('')
SURFACE()
);
#3816=(
BOUNDED_SURFACE()
B_SPLINE_SURFACE(1,2,((#159316,#159317,#159318,#159319,#159320),(#159321,
#159322,#159323,#159324,#159325)),.UNSPECIFIED.,.F.,.F.,.F.)
B_SPLINE_SURFACE_WITH_KNOTS((2,2),(3,2,3),(0.,0.0614498483524338),(0.659832011354082,
0.659901408087476,0.666841081426897),.UNSPECIFIED.)
GEOMETRIC_REPRESENTATION_ITEM()
RATIONAL_B_SPLINE_SURFACE(((0.990889788836286,0.990889788836286,0.990889788836286,
0.989616401900861,0.988816334712145),(0.990889788836286,0.990889788836286,
0.990889788836286,0.989616401900861,0.988816334712145)))
REPRESENTATION_ITEM('')
SURFACE()
);
#3817=(
BOUNDED_SURFACE()
B_SPLINE_SURFACE(1,2,((#159327,#159328,#159329),(#159330,#159331,#159332)),
 .UNSPECIFIED.,.F.,.F.,.F.)
B_SPLINE_SURFACE_WITH_KNOTS((2,2),(3,3),(0.947118453120174,1.),(0.65986001838565,
0.666841081426897),.UNSPECIFIED.)
GEOMETRIC_REPRESENTATION_ITEM()
RATIONAL_B_SPLINE_SURFACE(((0.990904995179336,0.989621173673358,0.988816334712146),
(0.990904995179336,0.989621173673358,0.988816334712146)))
REPRESENTATION_ITEM('')
SURFACE()
);
#3818=(
BOUNDED_SURFACE()
B_SPLINE_SURFACE(1,2,((#159343,#159344,#159345,#159346,#159347),(#159348,
#159349,#159350,#159351,#159352)),.UNSPECIFIED.,.F.,.F.,.F.)
B_SPLINE_SURFACE_WITH_KNOTS((2,2),(3,2,3),(0.947095459621875,1.),(0.066525725473656,
0.0714285714285714,0.0736968668684961),.UNSPECIFIED.)
GEOMETRIC_REPRESENTATION_ITEM()
RATIONAL_B_SPLINE_SURFACE(((0.996794362316491,0.998279055819231,1.,0.999203807365457,
0.998458182734336),(0.996794362316491,0.998279055819231,1.,0.999203807365457,
0.998458182734336)))
REPRESENTATION_ITEM('')
SURFACE()
);
#3819=(
BOUNDED_SURFACE()
B_SPLINE_SURFACE(1,2,((#159360,#159361,#159362,#159363,#159364),(#159365,
#159366,#159367,#159368,#159369)),.UNSPECIFIED.,.F.,.F.,.F.)
B_SPLINE_SURFACE_WITH_KNOTS((2,2),(3,2,3),(0.,0.0614231408718178),(0.0665257254736559,
0.0714285714285714,0.0736543502199197),.UNSPECIFIED.)
GEOMETRIC_REPRESENTATION_ITEM()
RATIONAL_B_SPLINE_SURFACE(((0.996794362316491,0.998279055819231,1.,0.999218731101513,
0.998486152291874),(0.996794362316491,0.998279055819231,1.,0.999218731101513,
0.998486152291874)))
REPRESENTATION_ITEM('')
SURFACE()
);
#3820=(
BOUNDED_SURFACE()
B_SPLINE_SURFACE(1,2,((#159371,#159372,#159373,#159374,#159375),(#159376,
#159377,#159378,#159379,#159380)),.UNSPECIFIED.,.F.,.F.,.F.)
B_SPLINE_SURFACE_WITH_KNOTS((2,2),(3,2,3),(0.817194107660853,1.),(0.642474614281364,
0.642857142857143,0.659901408087504),.UNSPECIFIED.)
GEOMETRIC_REPRESENTATION_ITEM()
RATIONAL_B_SPLINE_SURFACE(((0.999732896029236,0.999865728939372,1.,0.994017305594873,
0.990889788836276),(0.999732896029236,0.999865728939372,1.,0.994017305594873,
0.990889788836276)))
REPRESENTATION_ITEM('')
SURFACE()
);
#3821=(
BOUNDED_SURFACE()
B_SPLINE_SURFACE(1,2,((#159391,#159392,#159393,#159394,#159395),(#159396,
#159397,#159398,#159399,#159400)),.UNSPECIFIED.,.F.,.F.,.F.)
B_SPLINE_SURFACE_WITH_KNOTS((2,2),(3,2,3),(0.817114621578816,1.),(0.0734807488197741,
0.0736543502198956,0.09101449023205),.UNSPECIFIED.)
GEOMETRIC_REPRESENTATION_ITEM()
RATIONAL_B_SPLINE_SURFACE(((0.99848615229189,0.99848615229189,0.99848615229189,
0.992772345172014,0.990020524139834),(0.99848615229189,0.99848615229189,
0.99848615229189,0.992772345172014,0.990020524139834)))
REPRESENTATION_ITEM('')
SURFACE()
);
#3822=(
BOUNDED_SURFACE()
B_SPLINE_SURFACE(1,2,((#159402,#159403,#159404,#159405,#159406),(#159407,
#159408,#159409,#159410,#159411)),.UNSPECIFIED.,.F.,.F.,.F.)
B_SPLINE_SURFACE_WITH_KNOTS((2,2),(3,2,3),(0.,0.0614498483525083),(0.659832011354073,
0.659901408087467,0.666841081426896),.UNSPECIFIED.)
GEOMETRIC_REPRESENTATION_ITEM()
RATIONAL_B_SPLINE_SURFACE(((0.990889788836289,0.990889788836289,0.990889788836289,
0.989616401900862,0.988816334712146),(0.990889788836289,0.990889788836289,
0.990889788836289,0.989616401900862,0.988816334712146)))
REPRESENTATION_ITEM('')
SURFACE()
);
#3823=(
BOUNDED_SURFACE()
B_SPLINE_SURFACE(1,2,((#159413,#159414,#159415),(#159416,#159417,#159418)),
 .UNSPECIFIED.,.F.,.F.,.F.)
B_SPLINE_SURFACE_WITH_KNOTS((2,2),(3,3),(0.947118453120185,1.),(0.659860018385516,
0.666841081426897),.UNSPECIFIED.)
GEOMETRIC_REPRESENTATION_ITEM()
RATIONAL_B_SPLINE_SURFACE(((0.990904995179386,0.989621173673373,0.988816334712145),
(0.990904995179386,0.989621173673373,0.988816334712145)))
REPRESENTATION_ITEM('')
SURFACE()
);
#3824=(
BOUNDED_SURFACE()
B_SPLINE_SURFACE(1,2,((#159429,#159430,#159431,#159432,#159433),(#159434,
#159435,#159436,#159437,#159438)),.UNSPECIFIED.,.F.,.F.,.F.)
B_SPLINE_SURFACE_WITH_KNOTS((2,2),(3,2,3),(0.947095459621886,1.),(0.0665257254736562,
0.0714285714285714,0.0736968668684815),.UNSPECIFIED.)
GEOMETRIC_REPRESENTATION_ITEM()
RATIONAL_B_SPLINE_SURFACE(((0.996794362316491,0.998279055819231,1.,0.999203807365462,
0.998458182734346),(0.996794362316491,0.998279055819231,1.,0.999203807365462,
0.998458182734346)))
REPRESENTATION_ITEM('')
SURFACE()
);
#3825=(
BOUNDED_SURFACE()
B_SPLINE_SURFACE(1,2,((#159446,#159447,#159448,#159449,#159450),(#159451,
#159452,#159453,#159454,#159455)),.UNSPECIFIED.,.F.,.F.,.F.)
B_SPLINE_SURFACE_WITH_KNOTS((2,2),(3,2,3),(0.,0.0614231408718172),(0.0665257254736562,
0.0714285714285714,0.07365435021992),.UNSPECIFIED.)
GEOMETRIC_REPRESENTATION_ITEM()
RATIONAL_B_SPLINE_SURFACE(((0.996794362316491,0.998279055819231,1.,0.999218731101513,
0.998486152291874),(0.996794362316491,0.998279055819231,1.,0.999218731101513,
0.998486152291874)))
REPRESENTATION_ITEM('')
SURFACE()
);
#3826=(
BOUNDED_SURFACE()
B_SPLINE_SURFACE(1,2,((#159457,#159458,#159459,#159460,#159461),(#159462,
#159463,#159464,#159465,#159466)),.UNSPECIFIED.,.F.,.F.,.F.)
B_SPLINE_SURFACE_WITH_KNOTS((2,2),(3,2,3),(0.817194107660859,1.),(0.642474614281367,
0.642857142857143,0.659901408087505),.UNSPECIFIED.)
GEOMETRIC_REPRESENTATION_ITEM()
RATIONAL_B_SPLINE_SURFACE(((0.999732896029238,0.999865728939373,1.,0.994017305594873,
0.990889788836275),(0.999732896029238,0.999865728939373,1.,0.994017305594873,
0.990889788836275)))
REPRESENTATION_ITEM('')
SURFACE()
);
#3827=(
BOUNDED_SURFACE()
B_SPLINE_SURFACE(1,2,((#159477,#159478,#159479,#159480,#159481),(#159482,
#159483,#159484,#159485,#159486)),.UNSPECIFIED.,.F.,.F.,.F.)
B_SPLINE_SURFACE_WITH_KNOTS((2,2),(3,2,3),(0.817114621578821,1.),(0.0734807488197739,
0.0736543502198955,0.0910144902320515),.UNSPECIFIED.)
GEOMETRIC_REPRESENTATION_ITEM()
RATIONAL_B_SPLINE_SURFACE(((0.99848615229189,0.99848615229189,0.99848615229189,
0.992772345172014,0.990020524139833),(0.99848615229189,0.99848615229189,
0.99848615229189,0.992772345172014,0.990020524139833)))
REPRESENTATION_ITEM('')
SURFACE()
);
#3828=(
BOUNDED_SURFACE()
B_SPLINE_SURFACE(1,2,((#159488,#159489,#159490,#159491,#159492),(#159493,
#159494,#159495,#159496,#159497)),.UNSPECIFIED.,.F.,.F.,.F.)
B_SPLINE_SURFACE_WITH_KNOTS((2,2),(3,2,3),(0.,0.0614498483525092),(0.659832011354073,
0.659901408087467,0.666841081426896),.UNSPECIFIED.)
GEOMETRIC_REPRESENTATION_ITEM()
RATIONAL_B_SPLINE_SURFACE(((0.990889788836289,0.990889788836289,0.990889788836289,
0.989616401900862,0.988816334712146),(0.990889788836289,0.990889788836289,
0.990889788836289,0.989616401900862,0.988816334712146)))
REPRESENTATION_ITEM('')
SURFACE()
);
#3829=(
BOUNDED_SURFACE()
B_SPLINE_SURFACE(1,2,((#159499,#159500,#159501),(#159502,#159503,#159504)),
 .UNSPECIFIED.,.F.,.F.,.F.)
B_SPLINE_SURFACE_WITH_KNOTS((2,2),(3,3),(0.947118453120178,1.),(0.659860018385642,
0.666841081426896),.UNSPECIFIED.)
GEOMETRIC_REPRESENTATION_ITEM()
RATIONAL_B_SPLINE_SURFACE(((0.990904995179339,0.989621173673359,0.988816334712145),
(0.990904995179339,0.989621173673359,0.988816334712145)))
REPRESENTATION_ITEM('')
SURFACE()
);
#3830=(
BOUNDED_SURFACE()
B_SPLINE_SURFACE(1,2,((#159515,#159516,#159517,#159518,#159519),(#159520,
#159521,#159522,#159523,#159524)),.UNSPECIFIED.,.F.,.F.,.F.)
B_SPLINE_SURFACE_WITH_KNOTS((2,2),(3,2,3),(0.947095459621876,1.),(0.0665257254736561,
0.0714285714285714,0.073696866868496),.UNSPECIFIED.)
GEOMETRIC_REPRESENTATION_ITEM()
RATIONAL_B_SPLINE_SURFACE(((0.996794362316491,0.998279055819231,1.,0.999203807365457,
0.998458182734337),(0.996794362316491,0.998279055819231,1.,0.999203807365457,
0.998458182734337)))
REPRESENTATION_ITEM('')
SURFACE()
);
#3831=(
BOUNDED_SURFACE()
B_SPLINE_SURFACE(1,2,((#159531,#159532,#159533,#159534,#159535),(#159536,
#159537,#159538,#159539,#159540)),.UNSPECIFIED.,.F.,.F.,.F.)
B_SPLINE_SURFACE_WITH_KNOTS((2,2),(3,2,3),(0.,0.0614231408718195),(0.066525725473656,
0.0714285714285714,0.0736543502199191),.UNSPECIFIED.)
GEOMETRIC_REPRESENTATION_ITEM()
RATIONAL_B_SPLINE_SURFACE(((0.996794362316491,0.998279055819231,1.,0.999218731101513,
0.998486152291874),(0.996794362316491,0.998279055819231,1.,0.999218731101513,
0.998486152291874)))
REPRESENTATION_ITEM('')
SURFACE()
);
#3832=(
BOUNDED_SURFACE()
B_SPLINE_SURFACE(1,2,((#159542,#159543,#159544,#159545,#159546),(#159547,
#159548,#159549,#159550,#159551)),.UNSPECIFIED.,.F.,.F.,.F.)
B_SPLINE_SURFACE_WITH_KNOTS((2,2),(3,2,3),(0.817194107660853,1.),(0.642474614281367,
0.642857142857143,0.659901408087503),.UNSPECIFIED.)
GEOMETRIC_REPRESENTATION_ITEM()
RATIONAL_B_SPLINE_SURFACE(((0.999732896029238,0.999865728939373,1.,0.994017305594874,
0.990889788836276),(0.999732896029238,0.999865728939373,1.,0.994017305594874,
0.990889788836276)))
REPRESENTATION_ITEM('')
SURFACE()
);
#3833=(
BOUNDED_SURFACE()
B_SPLINE_SURFACE(1,2,((#159562,#159563,#159564,#159565,#159566),(#159567,
#159568,#159569,#159570,#159571)),.UNSPECIFIED.,.F.,.F.,.F.)
B_SPLINE_SURFACE_WITH_KNOTS((2,2),(3,2,3),(0.817114621578811,1.),(0.0734807488197823,
0.0736543502199038,0.0910144902320515),.UNSPECIFIED.)
GEOMETRIC_REPRESENTATION_ITEM()
RATIONAL_B_SPLINE_SURFACE(((0.998486152291884,0.998486152291884,0.998486152291884,
0.992772345172013,0.990020524139833),(0.998486152291884,0.998486152291884,
0.998486152291884,0.992772345172013,0.990020524139833)))
REPRESENTATION_ITEM('')
SURFACE()
);
#3834=(
BOUNDED_SURFACE()
B_SPLINE_SURFACE(1,2,((#159573,#159574,#159575,#159576,#159577),(#159578,
#159579,#159580,#159581,#159582)),.UNSPECIFIED.,.F.,.F.,.F.)
B_SPLINE_SURFACE_WITH_KNOTS((2,2),(3,2,3),(0.,0.0614498483524293),(0.659832011354082,
0.659901408087476,0.666841081426896),.UNSPECIFIED.)
GEOMETRIC_REPRESENTATION_ITEM()
RATIONAL_B_SPLINE_SURFACE(((0.990889788836286,0.990889788836286,0.990889788836286,
0.989616401900861,0.988816334712146),(0.990889788836286,0.990889788836286,
0.990889788836286,0.989616401900861,0.988816334712146)))
REPRESENTATION_ITEM('')
SURFACE()
);
#3835=(
BOUNDED_SURFACE()
B_SPLINE_SURFACE(1,2,((#159584,#159585,#159586),(#159587,#159588,#159589)),
 .UNSPECIFIED.,.F.,.F.,.F.)
B_SPLINE_SURFACE_WITH_KNOTS((2,2),(3,3),(0.947118453120178,1.),(0.65986001838565,
0.666841081426896),.UNSPECIFIED.)
GEOMETRIC_REPRESENTATION_ITEM()
RATIONAL_B_SPLINE_SURFACE(((0.990904995179336,0.989621173673358,0.988816334712146),
(0.990904995179336,0.989621173673358,0.988816334712146)))
REPRESENTATION_ITEM('')
SURFACE()
);
#3836=(
BOUNDED_SURFACE()
B_SPLINE_SURFACE(1,2,((#159600,#159601,#159602,#159603,#159604),(#159605,
#159606,#159607,#159608,#159609)),.UNSPECIFIED.,.F.,.F.,.F.)
B_SPLINE_SURFACE_WITH_KNOTS((2,2),(3,2,3),(0.947095459621872,1.),(0.0665257254736559,
0.0714285714285714,0.0736968668684958),.UNSPECIFIED.)
GEOMETRIC_REPRESENTATION_ITEM()
RATIONAL_B_SPLINE_SURFACE(((0.996794362316491,0.998279055819231,1.,0.999203807365457,
0.998458182734337),(0.996794362316491,0.998279055819231,1.,0.999203807365457,
0.998458182734337)))
REPRESENTATION_ITEM('')
SURFACE()
);
#3837=(
BOUNDED_SURFACE()
B_SPLINE_SURFACE(1,2,((#159616,#159617,#159618,#159619,#159620),(#159621,
#159622,#159623,#159624,#159625)),.UNSPECIFIED.,.F.,.F.,.F.)
B_SPLINE_SURFACE_WITH_KNOTS((2,2),(3,2,3),(0.,0.0614231408718199),(0.066525725473656,
0.0714285714285714,0.0736543502199191),.UNSPECIFIED.)
GEOMETRIC_REPRESENTATION_ITEM()
RATIONAL_B_SPLINE_SURFACE(((0.996794362316491,0.998279055819231,1.,0.999218731101513,
0.998486152291874),(0.996794362316491,0.998279055819231,1.,0.999218731101513,
0.998486152291874)))
REPRESENTATION_ITEM('')
SURFACE()
);
#3838=(
BOUNDED_SURFACE()
B_SPLINE_SURFACE(1,2,((#159627,#159628,#159629,#159630,#159631),(#159632,
#159633,#159634,#159635,#159636)),.UNSPECIFIED.,.F.,.F.,.F.)
B_SPLINE_SURFACE_WITH_KNOTS((2,2),(3,2,3),(0.817194107660855,1.),(0.642474614281364,
0.642857142857143,0.659901408087503),.UNSPECIFIED.)
GEOMETRIC_REPRESENTATION_ITEM()
RATIONAL_B_SPLINE_SURFACE(((0.999732896029236,0.999865728939372,1.,0.994017305594874,
0.990889788836276),(0.999732896029236,0.999865728939372,1.,0.994017305594874,
0.990889788836276)))
REPRESENTATION_ITEM('')
SURFACE()
);
#3839=(
BOUNDED_SURFACE()
B_SPLINE_SURFACE(1,2,((#159647,#159648,#159649,#159650,#159651),(#159652,
#159653,#159654,#159655,#159656)),.UNSPECIFIED.,.F.,.F.,.F.)
B_SPLINE_SURFACE_WITH_KNOTS((2,2),(3,2,3),(0.817114621578814,1.),(0.0734807488197738,
0.0736543502198954,0.0910144902320515),.UNSPECIFIED.)
GEOMETRIC_REPRESENTATION_ITEM()
RATIONAL_B_SPLINE_SURFACE(((0.99848615229189,0.99848615229189,0.99848615229189,
0.992772345172014,0.990020524139833),(0.99848615229189,0.99848615229189,
0.99848615229189,0.992772345172014,0.990020524139833)))
REPRESENTATION_ITEM('')
SURFACE()
);
#3840=(
BOUNDED_SURFACE()
B_SPLINE_SURFACE(1,2,((#159658,#159659,#159660,#159661,#159662),(#159663,
#159664,#159665,#159666,#159667)),.UNSPECIFIED.,.F.,.F.,.F.)
B_SPLINE_SURFACE_WITH_KNOTS((2,2),(3,2,3),(0.,0.0614498483525101),(0.659832011354073,
0.659901408087467,0.666841081426897),.UNSPECIFIED.)
GEOMETRIC_REPRESENTATION_ITEM()
RATIONAL_B_SPLINE_SURFACE(((0.990889788836289,0.990889788836289,0.990889788836289,
0.989616401900862,0.988816334712145),(0.990889788836289,0.990889788836289,
0.990889788836289,0.989616401900862,0.988816334712145)))
REPRESENTATION_ITEM('')
SURFACE()
);
#3841=(
BOUNDED_SURFACE()
B_SPLINE_SURFACE(1,2,((#159669,#159670,#159671),(#159672,#159673,#159674)),
 .UNSPECIFIED.,.F.,.F.,.F.)
B_SPLINE_SURFACE_WITH_KNOTS((2,2),(3,3),(0.947118453120179,1.),(0.659860018385518,
0.666841081426897),.UNSPECIFIED.)
GEOMETRIC_REPRESENTATION_ITEM()
RATIONAL_B_SPLINE_SURFACE(((0.990904995179385,0.989621173673373,0.988816334712145),
(0.990904995179385,0.989621173673373,0.988816334712145)))
REPRESENTATION_ITEM('')
SURFACE()
);
#3842=(
BOUNDED_SURFACE()
B_SPLINE_SURFACE(1,2,((#159685,#159686,#159687,#159688,#159689),(#159690,
#159691,#159692,#159693,#159694)),.UNSPECIFIED.,.F.,.F.,.F.)
B_SPLINE_SURFACE_WITH_KNOTS((2,2),(3,2,3),(0.947095459621877,1.),(0.0665257254736561,
0.0714285714285714,0.0736968668684814),.UNSPECIFIED.)
GEOMETRIC_REPRESENTATION_ITEM()
RATIONAL_B_SPLINE_SURFACE(((0.996794362316491,0.998279055819231,1.,0.999203807365462,
0.998458182734346),(0.996794362316491,0.998279055819231,1.,0.999203807365462,
0.998458182734346)))
REPRESENTATION_ITEM('')
SURFACE()
);
#3843=(
BOUNDED_SURFACE()
B_SPLINE_SURFACE(1,2,((#159702,#159703,#159704,#159705,#159706),(#159707,
#159708,#159709,#159710,#159711)),.UNSPECIFIED.,.F.,.F.,.F.)
B_SPLINE_SURFACE_WITH_KNOTS((2,2),(3,2,3),(0.,0.0614231408718166),(0.066525725473656,
0.0714285714285714,0.0736543502199191),.UNSPECIFIED.)
GEOMETRIC_REPRESENTATION_ITEM()
RATIONAL_B_SPLINE_SURFACE(((0.996794362316491,0.998279055819231,1.,0.999218731101513,
0.998486152291874),(0.996794362316491,0.998279055819231,1.,0.999218731101513,
0.998486152291874)))
REPRESENTATION_ITEM('')
SURFACE()
);
#3844=(
BOUNDED_SURFACE()
B_SPLINE_SURFACE(1,2,((#159713,#159714,#159715,#159716,#159717),(#159718,
#159719,#159720,#159721,#159722)),.UNSPECIFIED.,.F.,.F.,.F.)
B_SPLINE_SURFACE_WITH_KNOTS((2,2),(3,2,3),(0.817194107660858,1.),(0.642474614281366,
0.642857142857143,0.659901408087503),.UNSPECIFIED.)
GEOMETRIC_REPRESENTATION_ITEM()
RATIONAL_B_SPLINE_SURFACE(((0.999732896029237,0.999865728939372,1.,0.994017305594874,
0.990889788836276),(0.999732896029237,0.999865728939372,1.,0.994017305594874,
0.990889788836276)))
REPRESENTATION_ITEM('')
SURFACE()
);
#3845=(
BOUNDED_SURFACE()
B_SPLINE_SURFACE(1,2,((#159733,#159734,#159735,#159736,#159737),(#159738,
#159739,#159740,#159741,#159742)),.UNSPECIFIED.,.F.,.F.,.F.)
B_SPLINE_SURFACE_WITH_KNOTS((2,2),(3,2,3),(0.817114621578819,1.),(0.0734807488197824,
0.0736543502199039,0.0910144902320514),.UNSPECIFIED.)
GEOMETRIC_REPRESENTATION_ITEM()
RATIONAL_B_SPLINE_SURFACE(((0.998486152291884,0.998486152291884,0.998486152291884,
0.992772345172013,0.990020524139833),(0.998486152291884,0.998486152291884,
0.998486152291884,0.992772345172013,0.990020524139833)))
REPRESENTATION_ITEM('')
SURFACE()
);
#3846=(
BOUNDED_SURFACE()
B_SPLINE_SURFACE(1,2,((#159744,#159745,#159746,#159747,#159748),(#159749,
#159750,#159751,#159752,#159753)),.UNSPECIFIED.,.F.,.F.,.F.)
B_SPLINE_SURFACE_WITH_KNOTS((2,2),(3,2,3),(0.,0.0614498483524375),(0.659832011354082,
0.659901408087476,0.666841081426897),.UNSPECIFIED.)
GEOMETRIC_REPRESENTATION_ITEM()
RATIONAL_B_SPLINE_SURFACE(((0.990889788836286,0.990889788836286,0.990889788836286,
0.989616401900861,0.988816334712146),(0.990889788836286,0.990889788836286,
0.990889788836286,0.989616401900861,0.988816334712146)))
REPRESENTATION_ITEM('')
SURFACE()
);
#3847=(
BOUNDED_SURFACE()
B_SPLINE_SURFACE(1,2,((#159755,#159756,#159757),(#159758,#159759,#159760)),
 .UNSPECIFIED.,.F.,.F.,.F.)
B_SPLINE_SURFACE_WITH_KNOTS((2,2),(3,3),(0.947118453120176,1.),(0.65986001838565,
0.666841081426897),.UNSPECIFIED.)
GEOMETRIC_REPRESENTATION_ITEM()
RATIONAL_B_SPLINE_SURFACE(((0.990904995179336,0.989621173673358,0.988816334712145),
(0.990904995179336,0.989621173673358,0.988816334712145)))
REPRESENTATION_ITEM('')
SURFACE()
);
#3848=(
BOUNDED_SURFACE()
B_SPLINE_SURFACE(1,2,((#159771,#159772,#159773,#159774,#159775),(#159776,
#159777,#159778,#159779,#159780)),.UNSPECIFIED.,.F.,.F.,.F.)
B_SPLINE_SURFACE_WITH_KNOTS((2,2),(3,2,3),(0.947095459621878,1.),(0.0665257254736558,
0.0714285714285714,0.0736968668684962),.UNSPECIFIED.)
GEOMETRIC_REPRESENTATION_ITEM()
RATIONAL_B_SPLINE_SURFACE(((0.996794362316491,0.998279055819231,1.,0.999203807365457,
0.998458182734337),(0.996794362316491,0.998279055819231,1.,0.999203807365457,
0.998458182734337)))
REPRESENTATION_ITEM('')
SURFACE()
);
#3849=(
BOUNDED_SURFACE()
B_SPLINE_SURFACE(1,2,((#159787,#159788,#159789,#159790,#159791),(#159792,
#159793,#159794,#159795,#159796)),.UNSPECIFIED.,.F.,.F.,.F.)
B_SPLINE_SURFACE_WITH_KNOTS((2,2),(3,2,3),(0.,0.0614231408718161),(0.0665257254736557,
0.0714285714285714,0.0736543502199191),.UNSPECIFIED.)
GEOMETRIC_REPRESENTATION_ITEM()
RATIONAL_B_SPLINE_SURFACE(((0.996794362316491,0.998279055819231,1.,0.999218731101513,
0.998486152291874),(0.996794362316491,0.998279055819231,1.,0.999218731101513,
0.998486152291874)))
REPRESENTATION_ITEM('')
SURFACE()
);
#3850=(
BOUNDED_SURFACE()
B_SPLINE_SURFACE(1,2,((#159798,#159799,#159800,#159801,#159802),(#159803,
#159804,#159805,#159806,#159807)),.UNSPECIFIED.,.F.,.F.,.F.)
B_SPLINE_SURFACE_WITH_KNOTS((2,2),(3,2,3),(0.817194107660851,1.),(0.642474614281365,
0.642857142857143,0.659901408087503),.UNSPECIFIED.)
GEOMETRIC_REPRESENTATION_ITEM()
RATIONAL_B_SPLINE_SURFACE(((0.999732896029236,0.999865728939372,1.,0.994017305594874,
0.990889788836276),(0.999732896029236,0.999865728939372,1.,0.994017305594874,
0.990889788836276)))
REPRESENTATION_ITEM('')
SURFACE()
);
#3851=(
BOUNDED_SURFACE()
B_SPLINE_SURFACE(1,2,((#159818,#159819,#159820,#159821,#159822),(#159823,
#159824,#159825,#159826,#159827)),.UNSPECIFIED.,.F.,.F.,.F.)
B_SPLINE_SURFACE_WITH_KNOTS((2,2),(3,2,3),(0.817114621578816,1.),(0.0734807488197823,
0.0736543502199038,0.0910144902320513),.UNSPECIFIED.)
GEOMETRIC_REPRESENTATION_ITEM()
RATIONAL_B_SPLINE_SURFACE(((0.998486152291884,0.998486152291884,0.998486152291884,
0.992772345172013,0.990020524139833),(0.998486152291884,0.998486152291884,
0.998486152291884,0.992772345172013,0.990020524139833)))
REPRESENTATION_ITEM('')
SURFACE()
);
#3852=(
BOUNDED_SURFACE()
B_SPLINE_SURFACE(1,2,((#159829,#159830,#159831,#159832,#159833),(#159834,
#159835,#159836,#159837,#159838)),.UNSPECIFIED.,.F.,.F.,.F.)
B_SPLINE_SURFACE_WITH_KNOTS((2,2),(3,2,3),(0.,0.0614498483524345),(0.659832011354082,
0.659901408087476,0.666841081426897),.UNSPECIFIED.)
GEOMETRIC_REPRESENTATION_ITEM()
RATIONAL_B_SPLINE_SURFACE(((0.990889788836286,0.990889788836286,0.990889788836286,
0.989616401900861,0.988816334712145),(0.990889788836286,0.990889788836286,
0.990889788836286,0.989616401900861,0.988816334712145)))
REPRESENTATION_ITEM('')
SURFACE()
);
#3853=(
BOUNDED_SURFACE()
B_SPLINE_SURFACE(1,2,((#159840,#159841,#159842),(#159843,#159844,#159845)),
 .UNSPECIFIED.,.F.,.F.,.F.)
B_SPLINE_SURFACE_WITH_KNOTS((2,2),(3,3),(0.947118453120174,1.),(0.659860018385524,
0.666841081426897),.UNSPECIFIED.)
GEOMETRIC_REPRESENTATION_ITEM()
RATIONAL_B_SPLINE_SURFACE(((0.990904995179383,0.989621173673372,0.988816334712145),
(0.990904995179383,0.989621173673372,0.988816334712145)))
REPRESENTATION_ITEM('')
SURFACE()
);
#3854=(
BOUNDED_SURFACE()
B_SPLINE_SURFACE(1,2,((#159856,#159857,#159858,#159859,#159860),(#159861,
#159862,#159863,#159864,#159865)),.UNSPECIFIED.,.F.,.F.,.F.)
B_SPLINE_SURFACE_WITH_KNOTS((2,2),(3,2,3),(0.947095459621876,1.),(0.066525725473656,
0.0714285714285714,0.0736968668684898),.UNSPECIFIED.)
GEOMETRIC_REPRESENTATION_ITEM()
RATIONAL_B_SPLINE_SURFACE(((0.996794362316491,0.998279055819231,1.,0.999203807365459,
0.998458182734341),(0.996794362316491,0.998279055819231,1.,0.999203807365459,
0.998458182734341)))
REPRESENTATION_ITEM('')
SURFACE()
);
#3855=(
BOUNDED_SURFACE()
B_SPLINE_SURFACE(1,2,((#159873,#159874,#159875,#159876,#159877),(#159878,
#159879,#159880,#159881,#159882)),.UNSPECIFIED.,.F.,.F.,.F.)
B_SPLINE_SURFACE_WITH_KNOTS((2,2),(3,2,3),(0.,0.061423140871819),(0.0665257254736559,
0.0714285714285714,0.0736543502199201),.UNSPECIFIED.)
GEOMETRIC_REPRESENTATION_ITEM()
RATIONAL_B_SPLINE_SURFACE(((0.996794362316491,0.998279055819231,1.,0.999218731101513,
0.998486152291874),(0.996794362316491,0.998279055819231,1.,0.999218731101513,
0.998486152291874)))
REPRESENTATION_ITEM('')
SURFACE()
);
#3856=(
BOUNDED_SURFACE()
B_SPLINE_SURFACE(1,2,((#159884,#159885,#159886,#159887,#159888),(#159889,
#159890,#159891,#159892,#159893)),.UNSPECIFIED.,.F.,.F.,.F.)
B_SPLINE_SURFACE_WITH_KNOTS((2,2),(3,2,3),(0.817194107660853,1.),(0.642474614281365,
0.642857142857143,0.659901408087505),.UNSPECIFIED.)
GEOMETRIC_REPRESENTATION_ITEM()
RATIONAL_B_SPLINE_SURFACE(((0.999732896029237,0.999865728939372,1.,0.994017305594873,
0.990889788836275),(0.999732896029237,0.999865728939372,1.,0.994017305594873,
0.990889788836275)))
REPRESENTATION_ITEM('')
SURFACE()
);
#3857=(
BOUNDED_SURFACE()
B_SPLINE_SURFACE(1,2,((#159904,#159905,#159906,#159907,#159908),(#159909,
#159910,#159911,#159912,#159913)),.UNSPECIFIED.,.F.,.F.,.F.)
B_SPLINE_SURFACE_WITH_KNOTS((2,2),(3,2,3),(0.817114621578814,1.),(0.0734807488197823,
0.0736543502199038,0.0910144902320513),.UNSPECIFIED.)
GEOMETRIC_REPRESENTATION_ITEM()
RATIONAL_B_SPLINE_SURFACE(((0.998486152291885,0.998486152291885,0.998486152291885,
0.992772345172013,0.990020524139833),(0.998486152291885,0.998486152291885,
0.998486152291885,0.992772345172013,0.990020524139833)))
REPRESENTATION_ITEM('')
SURFACE()
);
#3858=(
BOUNDED_SURFACE()
B_SPLINE_SURFACE(1,2,((#159915,#159916,#159917,#159918,#159919),(#159920,
#159921,#159922,#159923,#159924)),.UNSPECIFIED.,.F.,.F.,.F.)
B_SPLINE_SURFACE_WITH_KNOTS((2,2),(3,2,3),(0.,0.0614498483524357),(0.659832011354082,
0.659901408087476,0.666841081426897),.UNSPECIFIED.)
GEOMETRIC_REPRESENTATION_ITEM()
RATIONAL_B_SPLINE_SURFACE(((0.990889788836286,0.990889788836286,0.990889788836286,
0.989616401900861,0.988816334712146),(0.990889788836286,0.990889788836286,
0.990889788836286,0.989616401900861,0.988816334712146)))
REPRESENTATION_ITEM('')
SURFACE()
);
#3859=(
BOUNDED_SURFACE()
B_SPLINE_SURFACE(1,2,((#159926,#159927,#159928),(#159929,#159930,#159931)),
 .UNSPECIFIED.,.F.,.F.,.F.)
B_SPLINE_SURFACE_WITH_KNOTS((2,2),(3,3),(0.947118453120176,1.),(0.659860018385401,
0.666841081426898),.UNSPECIFIED.)
GEOMETRIC_REPRESENTATION_ITEM()
RATIONAL_B_SPLINE_SURFACE(((0.990904995179428,0.989621173673386,0.988816334712145),
(0.990904995179428,0.989621173673386,0.988816334712145)))
REPRESENTATION_ITEM('')
SURFACE()
);
#3860=(
BOUNDED_SURFACE()
B_SPLINE_SURFACE(1,2,((#159942,#159943,#159944,#159945,#159946),(#159947,
#159948,#159949,#159950,#159951)),.UNSPECIFIED.,.F.,.F.,.F.)
B_SPLINE_SURFACE_WITH_KNOTS((2,2),(3,2,3),(0.947095459621873,1.),(0.0665257254736559,
0.0714285714285714,0.0736968668684897),.UNSPECIFIED.)
GEOMETRIC_REPRESENTATION_ITEM()
RATIONAL_B_SPLINE_SURFACE(((0.996794362316491,0.998279055819231,1.,0.999203807365459,
0.998458182734341),(0.996794362316491,0.998279055819231,1.,0.999203807365459,
0.998458182734341)))
REPRESENTATION_ITEM('')
SURFACE()
);
#3861=(
BOUNDED_SURFACE()
B_SPLINE_SURFACE(1,2,((#159959,#159960,#159961,#159962,#159963),(#159964,
#159965,#159966,#159967,#159968)),.UNSPECIFIED.,.F.,.F.,.F.)
B_SPLINE_SURFACE_WITH_KNOTS((2,2),(3,2,3),(0.,0.0614231408718203),(0.0665257254736559,
0.0714285714285714,0.0736543502199224),.UNSPECIFIED.)
GEOMETRIC_REPRESENTATION_ITEM()
RATIONAL_B_SPLINE_SURFACE(((0.996794362316491,0.998279055819231,1.,0.999218731101512,
0.998486152291872),(0.996794362316491,0.998279055819231,1.,0.999218731101512,
0.998486152291872)))
REPRESENTATION_ITEM('')
SURFACE()
);
#3862=(
BOUNDED_SURFACE()
B_SPLINE_SURFACE(1,2,((#159970,#159971,#159972,#159973,#159974),(#159975,
#159976,#159977,#159978,#159979)),.UNSPECIFIED.,.F.,.F.,.F.)
B_SPLINE_SURFACE_WITH_KNOTS((2,2),(3,2,3),(0.817194107660857,1.),(0.642474614281367,
0.642857142857143,0.65990140808751),.UNSPECIFIED.)
GEOMETRIC_REPRESENTATION_ITEM()
RATIONAL_B_SPLINE_SURFACE(((0.999732896029238,0.999865728939373,1.,0.994017305594871,
0.990889788836273),(0.999732896029238,0.999865728939373,1.,0.994017305594871,
0.990889788836273)))
REPRESENTATION_ITEM('')
SURFACE()
);
#3863=(
BOUNDED_SURFACE()
B_SPLINE_SURFACE(1,2,((#159990,#159991,#159992,#159993,#159994),(#159995,
#159996,#159997,#159998,#159999)),.UNSPECIFIED.,.F.,.F.,.F.)
B_SPLINE_SURFACE_WITH_KNOTS((2,2),(3,2,3),(0.817114621578821,1.),(0.073480748819731,
0.073654350219853,0.0910144902320518),.UNSPECIFIED.)
GEOMETRIC_REPRESENTATION_ITEM()
RATIONAL_B_SPLINE_SURFACE(((0.998486152291918,0.998486152291918,0.998486152291918,
0.992772345172021,0.990020524139833),(0.998486152291918,0.998486152291918,
0.998486152291918,0.992772345172021,0.990020524139833)))
REPRESENTATION_ITEM('')
SURFACE()
);
#3864=(
BOUNDED_SURFACE()
B_SPLINE_SURFACE(1,2,((#160001,#160002,#160003,#160004,#160005),(#160006,
#160007,#160008,#160009,#160010)),.UNSPECIFIED.,.F.,.F.,.F.)
B_SPLINE_SURFACE_WITH_KNOTS((2,2),(3,2,3),(0.,0.0614498483528877),(0.65983201135403,
0.659901408087425,0.666841081426897),.UNSPECIFIED.)
GEOMETRIC_REPRESENTATION_ITEM()
RATIONAL_B_SPLINE_SURFACE(((0.990889788836305,0.990889788836305,0.990889788836305,
0.989616401900867,0.988816334712145),(0.990889788836305,0.990889788836305,
0.990889788836305,0.989616401900867,0.988816334712145)))
REPRESENTATION_ITEM('')
SURFACE()
);
#3865=(
BOUNDED_SURFACE()
B_SPLINE_SURFACE(1,2,((#160012,#160013,#160014),(#160015,#160016,#160017)),
 .UNSPECIFIED.,.F.,.F.,.F.)
B_SPLINE_SURFACE_WITH_KNOTS((2,2),(3,3),(0.947118453120172,1.),(0.659860018385599,
0.666841081426897),.UNSPECIFIED.)
GEOMETRIC_REPRESENTATION_ITEM()
RATIONAL_B_SPLINE_SURFACE(((0.990904995179355,0.989621173673364,0.988816334712145),
(0.990904995179355,0.989621173673364,0.988816334712145)))
REPRESENTATION_ITEM('')
SURFACE()
);
#3866=(
BOUNDED_SURFACE()
B_SPLINE_SURFACE(1,2,((#160028,#160029,#160030,#160031,#160032),(#160033,
#160034,#160035,#160036,#160037)),.UNSPECIFIED.,.F.,.F.,.F.)
B_SPLINE_SURFACE_WITH_KNOTS((2,2),(3,2,3),(0.947095459621873,1.),(0.066525725473656,
0.0714285714285714,0.073696866868496),.UNSPECIFIED.)
GEOMETRIC_REPRESENTATION_ITEM()
RATIONAL_B_SPLINE_SURFACE(((0.996794362316491,0.998279055819231,1.,0.999203807365457,
0.998458182734337),(0.996794362316491,0.998279055819231,1.,0.999203807365457,
0.998458182734337)))
REPRESENTATION_ITEM('')
SURFACE()
);
#3867=(
BOUNDED_SURFACE()
B_SPLINE_SURFACE(1,2,((#160045,#160046,#160047,#160048,#160049),(#160050,
#160051,#160052,#160053,#160054)),.UNSPECIFIED.,.F.,.F.,.F.)
B_SPLINE_SURFACE_WITH_KNOTS((2,2),(3,2,3),(0.,0.0614231408718192),(0.0665257254736563,
0.0714285714285714,0.073654350219921),.UNSPECIFIED.)
GEOMETRIC_REPRESENTATION_ITEM()
RATIONAL_B_SPLINE_SURFACE(((0.996794362316491,0.998279055819231,1.,0.999218731101512,
0.998486152291873),(0.996794362316491,0.998279055819231,1.,0.999218731101512,
0.998486152291873)))
REPRESENTATION_ITEM('')
SURFACE()
);
#3868=(
BOUNDED_SURFACE()
B_SPLINE_SURFACE(1,2,((#160056,#160057,#160058,#160059,#160060),(#160061,
#160062,#160063,#160064,#160065)),.UNSPECIFIED.,.F.,.F.,.F.)
B_SPLINE_SURFACE_WITH_KNOTS((2,2),(3,2,3),(0.817194107660852,1.),(0.642474614281367,
0.642857142857143,0.659901408087507),.UNSPECIFIED.)
GEOMETRIC_REPRESENTATION_ITEM()
RATIONAL_B_SPLINE_SURFACE(((0.999732896029238,0.999865728939373,1.,0.994017305594872,
0.990889788836274),(0.999732896029238,0.999865728939373,1.,0.994017305594872,
0.990889788836274)))
REPRESENTATION_ITEM('')
SURFACE()
);
#3869=(
BOUNDED_SURFACE()
B_SPLINE_SURFACE(1,2,((#160076,#160077,#160078,#160079,#160080),(#160081,
#160082,#160083,#160084,#160085)),.UNSPECIFIED.,.F.,.F.,.F.)
B_SPLINE_SURFACE_WITH_KNOTS((2,2),(3,2,3),(0.817114621578816,1.),(0.0734807488197815,
0.073654350219903,0.0910144902320514),.UNSPECIFIED.)
GEOMETRIC_REPRESENTATION_ITEM()
RATIONAL_B_SPLINE_SURFACE(((0.998486152291885,0.998486152291885,0.998486152291885,
0.992772345172013,0.990020524139833),(0.998486152291885,0.998486152291885,
0.998486152291885,0.992772345172013,0.990020524139833)))
REPRESENTATION_ITEM('')
SURFACE()
);
#3870=(
BOUNDED_SURFACE()
B_SPLINE_SURFACE(1,2,((#160087,#160088,#160089,#160090,#160091),(#160092,
#160093,#160094,#160095,#160096)),.UNSPECIFIED.,.F.,.F.,.F.)
B_SPLINE_SURFACE_WITH_KNOTS((2,2),(3,2,3),(0.,0.0614498483524432),(0.659832011354081,
0.659901408087475,0.666841081426896),.UNSPECIFIED.)
GEOMETRIC_REPRESENTATION_ITEM()
RATIONAL_B_SPLINE_SURFACE(((0.990889788836286,0.990889788836286,0.990889788836286,
0.989616401900861,0.988816334712146),(0.990889788836286,0.990889788836286,
0.990889788836286,0.989616401900861,0.988816334712146)))
REPRESENTATION_ITEM('')
SURFACE()
);
#3871=(
BOUNDED_SURFACE()
B_SPLINE_SURFACE(1,2,((#160098,#160099,#160100),(#160101,#160102,#160103)),
 .UNSPECIFIED.,.F.,.F.,.F.)
B_SPLINE_SURFACE_WITH_KNOTS((2,2),(3,3),(0.94711845312018,1.),(0.65986001838565,
0.666841081426896),.UNSPECIFIED.)
GEOMETRIC_REPRESENTATION_ITEM()
RATIONAL_B_SPLINE_SURFACE(((0.990904995179337,0.989621173673358,0.988816334712145),
(0.990904995179337,0.989621173673358,0.988816334712145)))
REPRESENTATION_ITEM('')
SURFACE()
);
#3872=(
BOUNDED_SURFACE()
B_SPLINE_SURFACE(1,2,((#160114,#160115,#160116,#160117,#160118),(#160119,
#160120,#160121,#160122,#160123)),.UNSPECIFIED.,.F.,.F.,.F.)
B_SPLINE_SURFACE_WITH_KNOTS((2,2),(3,2,3),(0.947095459621876,1.),(0.0665257254736558,
0.0714285714285714,0.0736968668684959),.UNSPECIFIED.)
GEOMETRIC_REPRESENTATION_ITEM()
RATIONAL_B_SPLINE_SURFACE(((0.996794362316491,0.998279055819231,1.,0.999203807365457,
0.998458182734337),(0.996794362316491,0.998279055819231,1.,0.999203807365457,
0.998458182734337)))
REPRESENTATION_ITEM('')
SURFACE()
);
#3873=(
BOUNDED_SURFACE()
B_SPLINE_SURFACE(1,2,((#160131,#160132,#160133,#160134,#160135),(#160136,
#160137,#160138,#160139,#160140)),.UNSPECIFIED.,.F.,.F.,.F.)
B_SPLINE_SURFACE_WITH_KNOTS((2,2),(3,2,3),(0.,0.0614231408718359),(0.0665257254736558,
0.0714285714285714,0.0736543502199115),.UNSPECIFIED.)
GEOMETRIC_REPRESENTATION_ITEM()
RATIONAL_B_SPLINE_SURFACE(((0.996794362316491,0.998279055819231,1.,0.999218731101516,
0.99848615229188),(0.996794362316491,0.998279055819231,1.,0.999218731101516,
0.99848615229188)))
REPRESENTATION_ITEM('')
SURFACE()
);
#3874=(
BOUNDED_SURFACE()
B_SPLINE_SURFACE(1,2,((#160142,#160143,#160144,#160145,#160146),(#160147,
#160148,#160149,#160150,#160151)),.UNSPECIFIED.,.F.,.F.,.F.)
B_SPLINE_SURFACE_WITH_KNOTS((2,2),(3,2,3),(0.817194107660858,1.),(0.642474614281367,
0.642857142857143,0.659901408087488),.UNSPECIFIED.)
GEOMETRIC_REPRESENTATION_ITEM()
RATIONAL_B_SPLINE_SURFACE(((0.999732896029238,0.999865728939373,1.,0.994017305594879,
0.990889788836282),(0.999732896029238,0.999865728939373,1.,0.994017305594879,
0.990889788836282)))
REPRESENTATION_ITEM('')
SURFACE()
);
#3875=(
BOUNDED_SURFACE()
B_SPLINE_SURFACE(1,2,((#160162,#160163,#160164,#160165,#160166),(#160167,
#160168,#160169,#160170,#160171)),.UNSPECIFIED.,.F.,.F.,.F.)
B_SPLINE_SURFACE_WITH_KNOTS((2,2),(3,2,3),(0.817114621578819,1.),(0.0734807488197832,
0.0736543502199047,0.0910144902320511),.UNSPECIFIED.)
GEOMETRIC_REPRESENTATION_ITEM()
RATIONAL_B_SPLINE_SURFACE(((0.998486152291884,0.998486152291884,0.998486152291884,
0.992772345172013,0.990020524139834),(0.998486152291884,0.998486152291884,
0.998486152291884,0.992772345172013,0.990020524139834)))
REPRESENTATION_ITEM('')
SURFACE()
);
#3876=(
BOUNDED_SURFACE()
B_SPLINE_SURFACE(1,2,((#160173,#160174,#160175,#160176,#160177),(#160178,
#160179,#160180,#160181,#160182)),.UNSPECIFIED.,.F.,.F.,.F.)
B_SPLINE_SURFACE_WITH_KNOTS((2,2),(3,2,3),(0.,0.0614498483524474),(0.659832011354081,
0.659901408087475,0.666841081426896),.UNSPECIFIED.)
GEOMETRIC_REPRESENTATION_ITEM()
RATIONAL_B_SPLINE_SURFACE(((0.990889788836286,0.990889788836286,0.990889788836286,
0.989616401900861,0.988816334712146),(0.990889788836286,0.990889788836286,
0.990889788836286,0.989616401900861,0.988816334712146)))
REPRESENTATION_ITEM('')
SURFACE()
);
#3877=(
BOUNDED_SURFACE()
B_SPLINE_SURFACE(1,2,((#160184,#160185,#160186),(#160187,#160188,#160189)),
 .UNSPECIFIED.,.F.,.F.,.F.)
B_SPLINE_SURFACE_WITH_KNOTS((2,2),(3,3),(0.947118453120166,1.),(0.659860018385649,
0.666841081426897),.UNSPECIFIED.)
GEOMETRIC_REPRESENTATION_ITEM()
RATIONAL_B_SPLINE_SURFACE(((0.990904995179337,0.989621173673358,0.988816334712146),
(0.990904995179337,0.989621173673358,0.988816334712146)))
REPRESENTATION_ITEM('')
SURFACE()
);
#3878=(
BOUNDED_SURFACE()
B_SPLINE_SURFACE(1,2,((#160200,#160201,#160202,#160203,#160204),(#160205,
#160206,#160207,#160208,#160209)),.UNSPECIFIED.,.F.,.F.,.F.)
B_SPLINE_SURFACE_WITH_KNOTS((2,2),(3,2,3),(0.947095459621867,1.),(0.066525725473656,
0.0714285714285714,0.073696866868497),.UNSPECIFIED.)
GEOMETRIC_REPRESENTATION_ITEM()
RATIONAL_B_SPLINE_SURFACE(((0.996794362316491,0.998279055819231,1.,0.999203807365457,
0.998458182734336),(0.996794362316491,0.998279055819231,1.,0.999203807365457,
0.998458182734336)))
REPRESENTATION_ITEM('')
SURFACE()
);
#3879=(
BOUNDED_SURFACE()
B_SPLINE_SURFACE(1,2,((#160216,#160217,#160218,#160219,#160220),(#160221,
#160222,#160223,#160224,#160225)),.UNSPECIFIED.,.F.,.F.,.F.)
B_SPLINE_SURFACE_WITH_KNOTS((2,2),(3,2,3),(0.,0.0614231408718302),(0.066525725473656,
0.0714285714285714,0.0736543502199111),.UNSPECIFIED.)
GEOMETRIC_REPRESENTATION_ITEM()
RATIONAL_B_SPLINE_SURFACE(((0.996794362316491,0.998279055819231,1.,0.999218731101516,
0.99848615229188),(0.996794362316491,0.998279055819231,1.,0.999218731101516,
0.99848615229188)))
REPRESENTATION_ITEM('')
SURFACE()
);
#3880=(
BOUNDED_SURFACE()
B_SPLINE_SURFACE(1,2,((#160227,#160228,#160229,#160230,#160231),(#160232,
#160233,#160234,#160235,#160236)),.UNSPECIFIED.,.F.,.F.,.F.)
B_SPLINE_SURFACE_WITH_KNOTS((2,2),(3,2,3),(0.817194107660843,1.),(0.642474614281367,
0.642857142857143,0.659901408087482),.UNSPECIFIED.)
GEOMETRIC_REPRESENTATION_ITEM()
RATIONAL_B_SPLINE_SURFACE(((0.999732896029238,0.999865728939373,1.,0.994017305594881,
0.990889788836284),(0.999732896029238,0.999865728939373,1.,0.994017305594881,
0.990889788836284)))
REPRESENTATION_ITEM('')
SURFACE()
);
#3881=(
BOUNDED_SURFACE()
B_SPLINE_SURFACE(1,2,((#160247,#160248,#160249,#160250,#160251),(#160252,
#160253,#160254,#160255,#160256)),.UNSPECIFIED.,.F.,.F.,.F.)
B_SPLINE_SURFACE_WITH_KNOTS((2,2),(3,2,3),(0.817114621578812,1.),(0.073480748819775,
0.0736543502198966,0.0910144902320529),.UNSPECIFIED.)
GEOMETRIC_REPRESENTATION_ITEM()
RATIONAL_B_SPLINE_SURFACE(((0.998486152291889,0.998486152291889,0.998486152291889,
0.992772345172014,0.990020524139833),(0.998486152291889,0.998486152291889,
0.998486152291889,0.992772345172014,0.990020524139833)))
REPRESENTATION_ITEM('')
SURFACE()
);
#3882=(
BOUNDED_SURFACE()
B_SPLINE_SURFACE(1,2,((#160258,#160259,#160260,#160261,#160262),(#160263,
#160264,#160265,#160266,#160267)),.UNSPECIFIED.,.F.,.F.,.F.)
B_SPLINE_SURFACE_WITH_KNOTS((2,2),(3,2,3),(0.,0.0614498483525183),(0.659832011354072,
0.659901408087466,0.666841081426896),.UNSPECIFIED.)
GEOMETRIC_REPRESENTATION_ITEM()
RATIONAL_B_SPLINE_SURFACE(((0.99088978883629,0.99088978883629,0.99088978883629,
0.989616401900862,0.988816334712146),(0.99088978883629,0.99088978883629,
0.99088978883629,0.989616401900862,0.988816334712146)))
REPRESENTATION_ITEM('')
SURFACE()
);
#3883=(
BOUNDED_SURFACE()
B_SPLINE_SURFACE(1,2,((#160269,#160270,#160271),(#160272,#160273,#160274)),
 .UNSPECIFIED.,.F.,.F.,.F.)
B_SPLINE_SURFACE_WITH_KNOTS((2,2),(3,3),(0.947118453120172,1.),(0.659860018385517,
0.666841081426897),.UNSPECIFIED.)
GEOMETRIC_REPRESENTATION_ITEM()
RATIONAL_B_SPLINE_SURFACE(((0.990904995179385,0.989621173673373,0.988816334712145),
(0.990904995179385,0.989621173673373,0.988816334712145)))
REPRESENTATION_ITEM('')
SURFACE()
);
#3884=(
BOUNDED_SURFACE()
B_SPLINE_SURFACE(1,2,((#160285,#160286,#160287,#160288,#160289),(#160290,
#160291,#160292,#160293,#160294)),.UNSPECIFIED.,.F.,.F.,.F.)
B_SPLINE_SURFACE_WITH_KNOTS((2,2),(3,2,3),(0.94709545962187,1.),(0.0665257254736565,
0.0714285714285714,0.0736968668684826),.UNSPECIFIED.)
GEOMETRIC_REPRESENTATION_ITEM()
RATIONAL_B_SPLINE_SURFACE(((0.996794362316492,0.998279055819231,1.,0.999203807365462,
0.998458182734345),(0.996794362316492,0.998279055819231,1.,0.999203807365462,
0.998458182734345)))
REPRESENTATION_ITEM('')
SURFACE()
);
#3885=(
BOUNDED_SURFACE()
B_SPLINE_SURFACE(1,2,((#160302,#160303,#160304,#160305,#160306),(#160307,
#160308,#160309,#160310,#160311)),.UNSPECIFIED.,.F.,.F.,.F.)
B_SPLINE_SURFACE_WITH_KNOTS((2,2),(3,2,3),(0.,0.0614231408718237),(0.0665257254736564,
0.0714285714285714,0.0736543502199109),.UNSPECIFIED.)
GEOMETRIC_REPRESENTATION_ITEM()
RATIONAL_B_SPLINE_SURFACE(((0.996794362316491,0.998279055819231,1.,0.999218731101516,
0.99848615229188),(0.996794362316491,0.998279055819231,1.,0.999218731101516,
0.99848615229188)))
REPRESENTATION_ITEM('')
SURFACE()
);
#3886=(
BOUNDED_SURFACE()
B_SPLINE_SURFACE(1,2,((#160313,#160314,#160315,#160316,#160317),(#160318,
#160319,#160320,#160321,#160322)),.UNSPECIFIED.,.F.,.F.,.F.)
B_SPLINE_SURFACE_WITH_KNOTS((2,2),(3,2,3),(0.817194107660847,1.),(0.642474614281365,
0.642857142857143,0.659901408087502),.UNSPECIFIED.)
GEOMETRIC_REPRESENTATION_ITEM()
RATIONAL_B_SPLINE_SURFACE(((0.999732896029236,0.999865728939372,1.,0.994017305594874,
0.990889788836277),(0.999732896029236,0.999865728939372,1.,0.994017305594874,
0.990889788836277)))
REPRESENTATION_ITEM('')
SURFACE()
);
#3887=(
BOUNDED_SURFACE()
B_SPLINE_SURFACE(1,2,((#160333,#160334,#160335,#160336,#160337),(#160338,
#160339,#160340,#160341,#160342)),.UNSPECIFIED.,.F.,.F.,.F.)
B_SPLINE_SURFACE_WITH_KNOTS((2,2),(3,2,3),(0.81711462157881,1.),(0.073480748819775,
0.0736543502198966,0.0910144902320526),.UNSPECIFIED.)
GEOMETRIC_REPRESENTATION_ITEM()
RATIONAL_B_SPLINE_SURFACE(((0.998486152291889,0.998486152291889,0.998486152291889,
0.992772345172013,0.990020524139833),(0.998486152291889,0.998486152291889,
0.998486152291889,0.992772345172013,0.990020524139833)))
REPRESENTATION_ITEM('')
SURFACE()
);
#3888=(
BOUNDED_SURFACE()
B_SPLINE_SURFACE(1,2,((#160344,#160345,#160346,#160347,#160348),(#160349,
#160350,#160351,#160352,#160353)),.UNSPECIFIED.,.F.,.F.,.F.)
B_SPLINE_SURFACE_WITH_KNOTS((2,2),(3,2,3),(0.,0.0614498483525201),(0.659832011354072,
0.659901408087466,0.666841081426897),.UNSPECIFIED.)
GEOMETRIC_REPRESENTATION_ITEM()
RATIONAL_B_SPLINE_SURFACE(((0.99088978883629,0.99088978883629,0.99088978883629,
0.989616401900862,0.988816334712146),(0.990889788836289,0.990889788836289,
0.990889788836289,0.989616401900862,0.988816334712146)))
REPRESENTATION_ITEM('')
SURFACE()
);
#3889=(
BOUNDED_SURFACE()
B_SPLINE_SURFACE(1,2,((#160355,#160356,#160357),(#160358,#160359,#160360)),
 .UNSPECIFIED.,.F.,.F.,.F.)
B_SPLINE_SURFACE_WITH_KNOTS((2,2),(3,3),(0.94711845312017,1.),(0.659860018385641,
0.666841081426897),.UNSPECIFIED.)
GEOMETRIC_REPRESENTATION_ITEM()
RATIONAL_B_SPLINE_SURFACE(((0.99090499517934,0.989621173673359,0.988816334712145),
(0.99090499517934,0.989621173673359,0.988816334712145)))
REPRESENTATION_ITEM('')
SURFACE()
);
#3890=(
BOUNDED_SURFACE()
B_SPLINE_SURFACE(1,2,((#160371,#160372,#160373,#160374,#160375),(#160376,
#160377,#160378,#160379,#160380)),.UNSPECIFIED.,.F.,.F.,.F.)
B_SPLINE_SURFACE_WITH_KNOTS((2,2),(3,2,3),(0.947095459621873,1.),(0.0665257254736562,
0.0714285714285714,0.0736968668684971),.UNSPECIFIED.)
GEOMETRIC_REPRESENTATION_ITEM()
RATIONAL_B_SPLINE_SURFACE(((0.996794362316491,0.998279055819231,1.,0.999203807365457,
0.998458182734336),(0.996794362316491,0.998279055819231,1.,0.999203807365457,
0.998458182734336)))
REPRESENTATION_ITEM('')
SURFACE()
);
#3891=(
BOUNDED_SURFACE()
B_SPLINE_SURFACE(1,2,((#160388,#160389,#160390,#160391,#160392),(#160393,
#160394,#160395,#160396,#160397)),.UNSPECIFIED.,.F.,.F.,.F.)
B_SPLINE_SURFACE_WITH_KNOTS((2,2),(3,2,3),(0.,0.0614231408718238),(0.0665257254736562,
0.0714285714285714,0.073654350219911),.UNSPECIFIED.)
GEOMETRIC_REPRESENTATION_ITEM()
RATIONAL_B_SPLINE_SURFACE(((0.996794362316491,0.998279055819231,1.,0.999218731101516,
0.99848615229188),(0.996794362316491,0.998279055819231,1.,0.999218731101516,
0.99848615229188)))
REPRESENTATION_ITEM('')
SURFACE()
);
#3892=(
BOUNDED_SURFACE()
B_SPLINE_SURFACE(1,2,((#160399,#160400,#160401,#160402,#160403),(#160404,
#160405,#160406,#160407,#160408)),.UNSPECIFIED.,.F.,.F.,.F.)
B_SPLINE_SURFACE_WITH_KNOTS((2,2),(3,2,3),(0.817194107660843,1.),(0.642474614281365,
0.642857142857143,0.659901408087508),.UNSPECIFIED.)
GEOMETRIC_REPRESENTATION_ITEM()
RATIONAL_B_SPLINE_SURFACE(((0.999732896029236,0.999865728939372,1.,0.994017305594872,
0.990889788836274),(0.999732896029236,0.999865728939372,1.,0.994017305594872,
0.990889788836274)))
REPRESENTATION_ITEM('')
SURFACE()
);
#3893=(
BOUNDED_SURFACE()
B_SPLINE_SURFACE(1,2,((#160419,#160420,#160421,#160422,#160423),(#160424,
#160425,#160426,#160427,#160428)),.UNSPECIFIED.,.F.,.F.,.F.)
B_SPLINE_SURFACE_WITH_KNOTS((2,2),(3,2,3),(0.817114621578812,1.),(0.0734807488197753,
0.0736543502198968,0.0910144902320527),.UNSPECIFIED.)
GEOMETRIC_REPRESENTATION_ITEM()
RATIONAL_B_SPLINE_SURFACE(((0.998486152291889,0.998486152291889,0.998486152291889,
0.992772345172013,0.990020524139833),(0.998486152291889,0.998486152291889,
0.998486152291889,0.992772345172013,0.990020524139833)))
REPRESENTATION_ITEM('')
SURFACE()
);
#3894=(
BOUNDED_SURFACE()
B_SPLINE_SURFACE(1,2,((#160430,#160431,#160432,#160433,#160434),(#160435,
#160436,#160437,#160438,#160439)),.UNSPECIFIED.,.F.,.F.,.F.)
B_SPLINE_SURFACE_WITH_KNOTS((2,2),(3,2,3),(0.,0.0614498483525222),(0.659832011354072,
0.659901408087466,0.666841081426897),.UNSPECIFIED.)
GEOMETRIC_REPRESENTATION_ITEM()
RATIONAL_B_SPLINE_SURFACE(((0.99088978883629,0.99088978883629,0.99088978883629,
0.989616401900862,0.988816334712145),(0.99088978883629,0.99088978883629,
0.99088978883629,0.989616401900862,0.988816334712145)))
REPRESENTATION_ITEM('')
SURFACE()
);
#3895=(
BOUNDED_SURFACE()
B_SPLINE_SURFACE(1,2,((#160441,#160442,#160443),(#160444,#160445,#160446)),
 .UNSPECIFIED.,.F.,.F.,.F.)
B_SPLINE_SURFACE_WITH_KNOTS((2,2),(3,3),(0.94711845312017,1.),(0.659860018385515,
0.666841081426897),.UNSPECIFIED.)
GEOMETRIC_REPRESENTATION_ITEM()
RATIONAL_B_SPLINE_SURFACE(((0.990904995179386,0.989621173673373,0.988816334712145),
(0.990904995179386,0.989621173673373,0.988816334712145)))
REPRESENTATION_ITEM('')
SURFACE()
);
#3896=(
BOUNDED_SURFACE()
B_SPLINE_SURFACE(1,2,((#160457,#160458,#160459,#160460,#160461),(#160462,
#160463,#160464,#160465,#160466)),.UNSPECIFIED.,.F.,.F.,.F.)
B_SPLINE_SURFACE_WITH_KNOTS((2,2),(3,2,3),(0.947095459621873,1.),(0.0665257254736565,
0.0714285714285714,0.0736968668684827),.UNSPECIFIED.)
GEOMETRIC_REPRESENTATION_ITEM()
RATIONAL_B_SPLINE_SURFACE(((0.996794362316492,0.998279055819231,1.,0.999203807365462,
0.998458182734345),(0.996794362316492,0.998279055819231,1.,0.999203807365462,
0.998458182734345)))
REPRESENTATION_ITEM('')
SURFACE()
);
#3897=(
BOUNDED_SURFACE()
B_SPLINE_SURFACE(1,2,((#160474,#160475,#160476,#160477,#160478),(#160479,
#160480,#160481,#160482,#160483)),.UNSPECIFIED.,.F.,.F.,.F.)
B_SPLINE_SURFACE_WITH_KNOTS((2,2),(3,2,3),(0.,0.0614231408718247),(0.0665257254736564,
0.0714285714285714,0.073654350219911),.UNSPECIFIED.)
GEOMETRIC_REPRESENTATION_ITEM()
RATIONAL_B_SPLINE_SURFACE(((0.996794362316491,0.998279055819231,1.,0.999218731101516,
0.99848615229188),(0.996794362316491,0.998279055819231,1.,0.999218731101516,
0.99848615229188)))
REPRESENTATION_ITEM('')
SURFACE()
);
#3898=(
BOUNDED_SURFACE()
B_SPLINE_SURFACE(1,2,((#160485,#160486,#160487,#160488,#160489),(#160490,
#160491,#160492,#160493,#160494)),.UNSPECIFIED.,.F.,.F.,.F.)
B_SPLINE_SURFACE_WITH_KNOTS((2,2),(3,2,3),(0.817194107660843,1.),(0.642474614281365,
0.642857142857143,0.659901408087509),.UNSPECIFIED.)
GEOMETRIC_REPRESENTATION_ITEM()
RATIONAL_B_SPLINE_SURFACE(((0.999732896029236,0.999865728939372,1.,0.994017305594872,
0.990889788836274),(0.999732896029236,0.999865728939372,1.,0.994017305594872,
0.990889788836274)))
REPRESENTATION_ITEM('')
SURFACE()
);
#3899=(
BOUNDED_SURFACE()
B_SPLINE_SURFACE(1,2,((#160505,#160506,#160507,#160508,#160509),(#160510,
#160511,#160512,#160513,#160514)),.UNSPECIFIED.,.F.,.F.,.F.)
B_SPLINE_SURFACE_WITH_KNOTS((2,2),(3,2,3),(0.817114621578811,1.),(0.0734807488197753,
0.0736543502198968,0.0910144902320527),.UNSPECIFIED.)
GEOMETRIC_REPRESENTATION_ITEM()
RATIONAL_B_SPLINE_SURFACE(((0.998486152291889,0.998486152291889,0.998486152291889,
0.992772345172013,0.990020524139833),(0.998486152291889,0.998486152291889,
0.998486152291889,0.992772345172013,0.990020524139833)))
REPRESENTATION_ITEM('')
SURFACE()
);
#3900=(
BOUNDED_SURFACE()
B_SPLINE_SURFACE(1,2,((#160516,#160517,#160518,#160519,#160520),(#160521,
#160522,#160523,#160524,#160525)),.UNSPECIFIED.,.F.,.F.,.F.)
B_SPLINE_SURFACE_WITH_KNOTS((2,2),(3,2,3),(0.,0.061449848352517),(0.659832011354072,
0.659901408087466,0.666841081426897),.UNSPECIFIED.)
GEOMETRIC_REPRESENTATION_ITEM()
RATIONAL_B_SPLINE_SURFACE(((0.990889788836289,0.990889788836289,0.990889788836289,
0.989616401900862,0.988816334712145),(0.99088978883629,0.99088978883629,
0.99088978883629,0.989616401900862,0.988816334712146)))
REPRESENTATION_ITEM('')
SURFACE()
);
#3901=(
BOUNDED_SURFACE()
B_SPLINE_SURFACE(1,2,((#160527,#160528,#160529),(#160530,#160531,#160532)),
 .UNSPECIFIED.,.F.,.F.,.F.)
B_SPLINE_SURFACE_WITH_KNOTS((2,2),(3,3),(0.947118453120168,1.),(0.659860018385514,
0.666841081426898),.UNSPECIFIED.)
GEOMETRIC_REPRESENTATION_ITEM()
RATIONAL_B_SPLINE_SURFACE(((0.990904995179386,0.989621173673373,0.988816334712145),
(0.990904995179386,0.989621173673373,0.988816334712145)))
REPRESENTATION_ITEM('')
SURFACE()
);
#3902=(
BOUNDED_SURFACE()
B_SPLINE_SURFACE(1,2,((#160543,#160544,#160545,#160546,#160547),(#160548,
#160549,#160550,#160551,#160552)),.UNSPECIFIED.,.F.,.F.,.F.)
B_SPLINE_SURFACE_WITH_KNOTS((2,2),(3,2,3),(0.947095459621871,1.),(0.0665257254736566,
0.0714285714285714,0.0736968668684827),.UNSPECIFIED.)
GEOMETRIC_REPRESENTATION_ITEM()
RATIONAL_B_SPLINE_SURFACE(((0.996794362316492,0.998279055819231,1.,0.999203807365462,
0.998458182734345),(0.996794362316492,0.998279055819231,1.,0.999203807365462,
0.998458182734345)))
REPRESENTATION_ITEM('')
SURFACE()
);
#3903=(
BOUNDED_SURFACE()
B_SPLINE_SURFACE(1,2,((#160560,#160561,#160562,#160563,#160564),(#160565,
#160566,#160567,#160568,#160569)),.UNSPECIFIED.,.F.,.F.,.F.)
B_SPLINE_SURFACE_WITH_KNOTS((2,2),(3,2,3),(0.,0.0614231408718261),(0.0665257254736565,
0.0714285714285714,0.073654350219911),.UNSPECIFIED.)
GEOMETRIC_REPRESENTATION_ITEM()
RATIONAL_B_SPLINE_SURFACE(((0.996794362316492,0.998279055819231,1.,0.999218731101516,
0.99848615229188),(0.996794362316492,0.998279055819231,1.,0.999218731101516,
0.99848615229188)))
REPRESENTATION_ITEM('')
SURFACE()
);
#3904=(
BOUNDED_SURFACE()
B_SPLINE_SURFACE(1,2,((#160571,#160572,#160573,#160574,#160575),(#160576,
#160577,#160578,#160579,#160580)),.UNSPECIFIED.,.F.,.F.,.F.)
B_SPLINE_SURFACE_WITH_KNOTS((2,2),(3,2,3),(0.817194107660846,1.),(0.642474614281365,
0.642857142857143,0.659901408087504),.UNSPECIFIED.)
GEOMETRIC_REPRESENTATION_ITEM()
RATIONAL_B_SPLINE_SURFACE(((0.999732896029236,0.999865728939372,1.,0.994017305594873,
0.990889788836276),(0.999732896029236,0.999865728939372,1.,0.994017305594873,
0.990889788836276)))
REPRESENTATION_ITEM('')
SURFACE()
);
#3905=(
BOUNDED_SURFACE()
B_SPLINE_SURFACE(1,2,((#160591,#160592,#160593,#160594,#160595),(#160596,
#160597,#160598,#160599,#160600)),.UNSPECIFIED.,.F.,.F.,.F.)
B_SPLINE_SURFACE_WITH_KNOTS((2,2),(3,2,3),(0.817114621578813,1.),(0.0734807488197834,
0.0736543502199049,0.0910144902320528),.UNSPECIFIED.)
GEOMETRIC_REPRESENTATION_ITEM()
RATIONAL_B_SPLINE_SURFACE(((0.998486152291884,0.998486152291884,0.998486152291884,
0.992772345172012,0.990020524139833),(0.998486152291884,0.998486152291884,
0.998486152291884,0.992772345172012,0.990020524139833)))
REPRESENTATION_ITEM('')
SURFACE()
);
#3906=(
BOUNDED_SURFACE()
B_SPLINE_SURFACE(1,2,((#160601,#160602,#160603),(#160604,#160605,#160606)),
 .UNSPECIFIED.,.F.,.F.,.F.)
B_SPLINE_SURFACE_WITH_KNOTS((2,2),(3,3),(0.710192959008443,1.),(0.607982157956011,
0.625273655815328),.UNSPECIFIED.)
GEOMETRIC_REPRESENTATION_ITEM()
RATIONAL_B_SPLINE_SURFACE(((0.987470879370255,0.98761351460672,0.990694758798812),
(0.987470879370255,0.98761351460672,0.990694758798812)))
REPRESENTATION_ITEM('')
SURFACE()
);
#3907=(
BOUNDED_SURFACE()
B_SPLINE_SURFACE(1,2,((#160615,#160616,#160617,#160618,#160619),(#160620,
#160621,#160622,#160623,#160624)),.UNSPECIFIED.,.F.,.F.,.F.)
B_SPLINE_SURFACE_WITH_KNOTS((2,2),(3,2,3),(0.709719018660168,1.),(0.107879027750092,
0.125170525609408,0.125770422804668),.UNSPECIFIED.)
GEOMETRIC_REPRESENTATION_ITEM()
RATIONAL_B_SPLINE_SURFACE(((0.987469282487682,0.987594391229382,0.990658108926709,
0.990658108926709,0.990658108926709),(0.987469282487682,0.987594391229382,
0.990658108926709,0.990658108926709,0.990658108926709)))
REPRESENTATION_ITEM('')
SURFACE()
);
#3908=(
BOUNDED_SURFACE()
B_SPLINE_SURFACE(1,2,((#160626,#160627,#160628),(#160629,#160630,#160631)),
 .UNSPECIFIED.,.F.,.F.,.F.)
B_SPLINE_SURFACE_WITH_KNOTS((2,2),(3,3),(0.710192959008439,1.),(0.607982157956011,
0.625273655815328),.UNSPECIFIED.)
GEOMETRIC_REPRESENTATION_ITEM()
RATIONAL_B_SPLINE_SURFACE(((0.987470879370255,0.98761351460672,0.990694758798812),
(0.987470879370255,0.98761351460672,0.990694758798812)))
REPRESENTATION_ITEM('')
SURFACE()
);
#3909=(
BOUNDED_SURFACE()
B_SPLINE_SURFACE(1,2,((#160640,#160641,#160642,#160643,#160644),(#160645,
#160646,#160647,#160648,#160649)),.UNSPECIFIED.,.F.,.F.,.F.)
B_SPLINE_SURFACE_WITH_KNOTS((2,2),(3,2,3),(0.709719018657229,1.),(0.107879027750092,
0.125170525609408,0.125770422807604),.UNSPECIFIED.)
GEOMETRIC_REPRESENTATION_ITEM()
RATIONAL_B_SPLINE_SURFACE(((0.987469282487682,0.987594391229382,0.990658108926709,
0.990658108926709,0.990658108926709),(0.987469282487682,0.987594391229382,
0.990658108926709,0.990658108926709,0.990658108926709)))
REPRESENTATION_ITEM('')
SURFACE()
);
#3910=(
BOUNDED_SURFACE()
B_SPLINE_SURFACE(1,2,((#160651,#160652,#160653),(#160654,#160655,#160656)),
 .UNSPECIFIED.,.F.,.F.,.F.)
B_SPLINE_SURFACE_WITH_KNOTS((2,2),(3,3),(0.710192959008444,1.),(0.607982157956011,
0.625273655815328),.UNSPECIFIED.)
GEOMETRIC_REPRESENTATION_ITEM()
RATIONAL_B_SPLINE_SURFACE(((0.987470879370255,0.98761351460672,0.990694758798812),
(0.987470879370255,0.98761351460672,0.990694758798812)))
REPRESENTATION_ITEM('')
SURFACE()
);
#3911=(
BOUNDED_SURFACE()
B_SPLINE_SURFACE(1,2,((#160665,#160666,#160667,#160668,#160669),(#160670,
#160671,#160672,#160673,#160674)),.UNSPECIFIED.,.F.,.F.,.F.)
B_SPLINE_SURFACE_WITH_KNOTS((2,2),(3,2,3),(0.709719018653174,1.),(0.107879027750092,
0.125170525609408,0.12577042281166),.UNSPECIFIED.)
GEOMETRIC_REPRESENTATION_ITEM()
RATIONAL_B_SPLINE_SURFACE(((0.987469282487682,0.987594391229382,0.990658108926709,
0.990658108926709,0.990658108926709),(0.987469282487682,0.987594391229382,
0.990658108926709,0.990658108926709,0.990658108926709)))
REPRESENTATION_ITEM('')
SURFACE()
);
#3912=(
BOUNDED_SURFACE()
B_SPLINE_SURFACE(1,2,((#160676,#160677,#160678),(#160679,#160680,#160681)),
 .UNSPECIFIED.,.F.,.F.,.F.)
B_SPLINE_SURFACE_WITH_KNOTS((2,2),(3,3),(0.710192959008439,1.),(0.607982157956011,
0.625273655815328),.UNSPECIFIED.)
GEOMETRIC_REPRESENTATION_ITEM()
RATIONAL_B_SPLINE_SURFACE(((0.987470879370255,0.98761351460672,0.990694758798812),
(0.987470879370255,0.98761351460672,0.990694758798812)))
REPRESENTATION_ITEM('')
SURFACE()
);
#3913=(
BOUNDED_SURFACE()
B_SPLINE_SURFACE(1,2,((#160690,#160691,#160692,#160693,#160694),(#160695,
#160696,#160697,#160698,#160699)),.UNSPECIFIED.,.F.,.F.,.F.)
B_SPLINE_SURFACE_WITH_KNOTS((2,2),(3,2,3),(0.709719018660876,1.),(0.107879027750092,
0.125170525609407,0.125770422844536),.UNSPECIFIED.)
GEOMETRIC_REPRESENTATION_ITEM()
RATIONAL_B_SPLINE_SURFACE(((0.987469282487682,0.987594391229382,0.990658108926709,
0.990658108926709,0.990658108926709),(0.987469282487682,0.987594391229382,
0.990658108926709,0.990658108926709,0.990658108926709)))
REPRESENTATION_ITEM('')
SURFACE()
);
#3914=(
BOUNDED_SURFACE()
B_SPLINE_SURFACE(1,2,((#160701,#160702,#160703),(#160704,#160705,#160706)),
 .UNSPECIFIED.,.F.,.F.,.F.)
B_SPLINE_SURFACE_WITH_KNOTS((2,2),(3,3),(0.710192959008442,1.),(0.607982157956012,
0.625273655815329),.UNSPECIFIED.)
GEOMETRIC_REPRESENTATION_ITEM()
RATIONAL_B_SPLINE_SURFACE(((0.987470879370256,0.987613514606721,0.990694758798813),
(0.987470879370256,0.987613514606721,0.990694758798813)))
REPRESENTATION_ITEM('')
SURFACE()
);
#3915=(
BOUNDED_SURFACE()
B_SPLINE_SURFACE(1,2,((#160715,#160716,#160717,#160718,#160719),(#160720,
#160721,#160722,#160723,#160724)),.UNSPECIFIED.,.F.,.F.,.F.)
B_SPLINE_SURFACE_WITH_KNOTS((2,2),(3,2,3),(0.709719018647908,1.),(0.10787902775009,
0.125170525609407,0.125770422857558),.UNSPECIFIED.)
GEOMETRIC_REPRESENTATION_ITEM()
RATIONAL_B_SPLINE_SURFACE(((0.987469282487682,0.987594391229382,0.990658108926708,
0.990658108926708,0.990658108926708),(0.987469282487682,0.987594391229382,
0.990658108926708,0.990658108926708,0.990658108926708)))
REPRESENTATION_ITEM('')
SURFACE()
);
#3916=(
BOUNDED_SURFACE()
B_SPLINE_SURFACE(1,2,((#160726,#160727,#160728),(#160729,#160730,#160731)),
 .UNSPECIFIED.,.F.,.F.,.F.)
B_SPLINE_SURFACE_WITH_KNOTS((2,2),(3,3),(0.710192959008439,1.),(0.607982157956012,
0.625273655815329),.UNSPECIFIED.)
GEOMETRIC_REPRESENTATION_ITEM()
RATIONAL_B_SPLINE_SURFACE(((0.987470879370256,0.987613514606721,0.990694758798813),
(0.987470879370256,0.987613514606721,0.990694758798813)))
REPRESENTATION_ITEM('')
SURFACE()
);
#3917=(
BOUNDED_SURFACE()
B_SPLINE_SURFACE(1,2,((#160740,#160741,#160742,#160743,#160744),(#160745,
#160746,#160747,#160748,#160749)),.UNSPECIFIED.,.F.,.F.,.F.)
B_SPLINE_SURFACE_WITH_KNOTS((2,2),(3,2,3),(0.709719018670347,1.),(0.10787902775009,
0.125170525609407,0.125770422794484),.UNSPECIFIED.)
GEOMETRIC_REPRESENTATION_ITEM()
RATIONAL_B_SPLINE_SURFACE(((0.987469282487682,0.987594391229382,0.990658108926708,
0.990658108926708,0.990658108926708),(0.987469282487682,0.987594391229382,
0.990658108926708,0.990658108926708,0.990658108926708)))
REPRESENTATION_ITEM('')
SURFACE()
);
#3918=(
BOUNDED_SURFACE()
B_SPLINE_SURFACE(1,2,((#160751,#160752,#160753),(#160754,#160755,#160756)),
 .UNSPECIFIED.,.F.,.F.,.F.)
B_SPLINE_SURFACE_WITH_KNOTS((2,2),(3,3),(0.710192959008438,1.),(0.607982157956012,
0.625273655815329),.UNSPECIFIED.)
GEOMETRIC_REPRESENTATION_ITEM()
RATIONAL_B_SPLINE_SURFACE(((0.987470879370255,0.987613514606721,0.990694758798813),
(0.987470879370255,0.987613514606721,0.990694758798813)))
REPRESENTATION_ITEM('')
SURFACE()
);
#3919=(
BOUNDED_SURFACE()
B_SPLINE_SURFACE(1,2,((#160765,#160766,#160767,#160768,#160769),(#160770,
#160771,#160772,#160773,#160774)),.UNSPECIFIED.,.F.,.F.,.F.)
B_SPLINE_SURFACE_WITH_KNOTS((2,2),(3,2,3),(0.709719018669977,1.),(0.10787902775009,
0.125170525609407,0.125770422794847),.UNSPECIFIED.)
GEOMETRIC_REPRESENTATION_ITEM()
RATIONAL_B_SPLINE_SURFACE(((0.987469282487682,0.987594391229382,0.990658108926708,
0.990658108926708,0.990658108926708),(0.987469282487682,0.987594391229382,
0.990658108926708,0.990658108926708,0.990658108926708)))
REPRESENTATION_ITEM('')
SURFACE()
);
#3920=(
BOUNDED_SURFACE()
B_SPLINE_SURFACE(1,2,((#160776,#160777,#160778),(#160779,#160780,#160781)),
 .UNSPECIFIED.,.F.,.F.,.F.)
B_SPLINE_SURFACE_WITH_KNOTS((2,2),(3,3),(0.710192959008442,1.),(0.607982157956012,
0.625273655815329),.UNSPECIFIED.)
GEOMETRIC_REPRESENTATION_ITEM()
RATIONAL_B_SPLINE_SURFACE(((0.987470879370256,0.987613514606721,0.990694758798813),
(0.987470879370256,0.987613514606721,0.990694758798813)))
REPRESENTATION_ITEM('')
SURFACE()
);
#3921=(
BOUNDED_SURFACE()
B_SPLINE_SURFACE(1,2,((#160790,#160791,#160792,#160793,#160794),(#160795,
#160796,#160797,#160798,#160799)),.UNSPECIFIED.,.F.,.F.,.F.)
B_SPLINE_SURFACE_WITH_KNOTS((2,2),(3,2,3),(0.709719018661188,1.),(0.10787902775009,
0.125170525609407,0.125770422843774),.UNSPECIFIED.)
GEOMETRIC_REPRESENTATION_ITEM()
RATIONAL_B_SPLINE_SURFACE(((0.987469282487682,0.987594391229382,0.990658108926708,
0.990658108926708,0.990658108926708),(0.987469282487682,0.987594391229382,
0.990658108926708,0.990658108926708,0.990658108926708)))
REPRESENTATION_ITEM('')
SURFACE()
);
#3922=(
BOUNDED_SURFACE()
B_SPLINE_SURFACE(1,2,((#160801,#160802,#160803),(#160804,#160805,#160806)),
 .UNSPECIFIED.,.F.,.F.,.F.)
B_SPLINE_SURFACE_WITH_KNOTS((2,2),(3,3),(0.71019295900844,1.),(0.607982157956012,
0.625273655815329),.UNSPECIFIED.)
GEOMETRIC_REPRESENTATION_ITEM()
RATIONAL_B_SPLINE_SURFACE(((0.987470879370256,0.987613514606721,0.990694758798813),
(0.987470879370256,0.987613514606721,0.990694758798813)))
REPRESENTATION_ITEM('')
SURFACE()
);
#3923=(
BOUNDED_SURFACE()
B_SPLINE_SURFACE(1,2,((#160815,#160816,#160817,#160818,#160819),(#160820,
#160821,#160822,#160823,#160824)),.UNSPECIFIED.,.F.,.F.,.F.)
B_SPLINE_SURFACE_WITH_KNOTS((2,2),(3,2,3),(0.709719018663442,1.),(0.107879027750091,
0.125170525609407,0.125770422801386),.UNSPECIFIED.)
GEOMETRIC_REPRESENTATION_ITEM()
RATIONAL_B_SPLINE_SURFACE(((0.987469282487682,0.987594391229382,0.990658108926709,
0.990658108926709,0.990658108926709),(0.987469282487682,0.987594391229382,
0.990658108926709,0.990658108926709,0.990658108926709)))
REPRESENTATION_ITEM('')
SURFACE()
);
#3924=(
BOUNDED_SURFACE()
B_SPLINE_SURFACE(1,2,((#160826,#160827,#160828),(#160829,#160830,#160831)),
 .UNSPECIFIED.,.F.,.F.,.F.)
B_SPLINE_SURFACE_WITH_KNOTS((2,2),(3,3),(0.710192959008444,1.),(0.607982157956012,
0.625273655815329),.UNSPECIFIED.)
GEOMETRIC_REPRESENTATION_ITEM()
RATIONAL_B_SPLINE_SURFACE(((0.987470879370255,0.987613514606721,0.990694758798813),
(0.987470879370255,0.987613514606721,0.990694758798813)))
REPRESENTATION_ITEM('')
SURFACE()
);
#3925=(
BOUNDED_SURFACE()
B_SPLINE_SURFACE(1,2,((#160840,#160841,#160842,#160843,#160844),(#160845,
#160846,#160847,#160848,#160849)),.UNSPECIFIED.,.F.,.F.,.F.)
B_SPLINE_SURFACE_WITH_KNOTS((2,2),(3,2,3),(0.709719018653236,1.),(0.107879027750091,
0.125170525609407,0.125770422811596),.UNSPECIFIED.)
GEOMETRIC_REPRESENTATION_ITEM()
RATIONAL_B_SPLINE_SURFACE(((0.987469282487682,0.987594391229382,0.990658108926708,
0.990658108926708,0.990658108926708),(0.987469282487682,0.987594391229382,
0.990658108926708,0.990658108926708,0.990658108926708)))
REPRESENTATION_ITEM('')
SURFACE()
);
#3926=(
BOUNDED_SURFACE()
B_SPLINE_SURFACE(1,2,((#160851,#160852,#160853),(#160854,#160855,#160856)),
 .UNSPECIFIED.,.F.,.F.,.F.)
B_SPLINE_SURFACE_WITH_KNOTS((2,2),(3,3),(0.71019295900844,1.),(0.607982157956012,
0.625273655815329),.UNSPECIFIED.)
GEOMETRIC_REPRESENTATION_ITEM()
RATIONAL_B_SPLINE_SURFACE(((0.987470879370255,0.987613514606721,0.990694758798813),
(0.987470879370255,0.987613514606721,0.990694758798813)))
REPRESENTATION_ITEM('')
SURFACE()
);
#3927=(
BOUNDED_SURFACE()
B_SPLINE_SURFACE(1,2,((#160865,#160866,#160867,#160868,#160869),(#160870,
#160871,#160872,#160873,#160874)),.UNSPECIFIED.,.F.,.F.,.F.)
B_SPLINE_SURFACE_WITH_KNOTS((2,2),(3,2,3),(0.709719018681401,1.),(0.107879027750091,
0.125170525609407,0.125770422824321),.UNSPECIFIED.)
GEOMETRIC_REPRESENTATION_ITEM()
RATIONAL_B_SPLINE_SURFACE(((0.987469282487682,0.987594391229382,0.990658108926708,
0.990658108926708,0.990658108926708),(0.987469282487682,0.987594391229382,
0.990658108926708,0.990658108926708,0.990658108926708)))
REPRESENTATION_ITEM('')
SURFACE()
);
#3928=(
BOUNDED_SURFACE()
B_SPLINE_SURFACE(1,2,((#160876,#160877,#160878),(#160879,#160880,#160881)),
 .UNSPECIFIED.,.F.,.F.,.F.)
B_SPLINE_SURFACE_WITH_KNOTS((2,2),(3,3),(0.710192959008443,1.),(0.607982157956012,
0.625273655815329),.UNSPECIFIED.)
GEOMETRIC_REPRESENTATION_ITEM()
RATIONAL_B_SPLINE_SURFACE(((0.987470879370255,0.987613514606721,0.990694758798813),
(0.987470879370255,0.987613514606721,0.990694758798813)))
REPRESENTATION_ITEM('')
SURFACE()
);
#3929=(
BOUNDED_SURFACE()
B_SPLINE_SURFACE(1,2,((#160890,#160891,#160892,#160893,#160894),(#160895,
#160896,#160897,#160898,#160899)),.UNSPECIFIED.,.F.,.F.,.F.)
B_SPLINE_SURFACE_WITH_KNOTS((2,2),(3,2,3),(0.709719018663075,1.),(0.107879027750091,
0.125170525609407,0.125770422842613),.UNSPECIFIED.)
GEOMETRIC_REPRESENTATION_ITEM()
RATIONAL_B_SPLINE_SURFACE(((0.987469282487682,0.987594391229382,0.990658108926709,
0.990658108926709,0.990658108926709),(0.987469282487682,0.987594391229382,
0.990658108926708,0.990658108926708,0.990658108926708)))
REPRESENTATION_ITEM('')
SURFACE()
);
#3930=(
BOUNDED_SURFACE()
B_SPLINE_SURFACE(1,2,((#160901,#160902,#160903),(#160904,#160905,#160906)),
 .UNSPECIFIED.,.F.,.F.,.F.)
B_SPLINE_SURFACE_WITH_KNOTS((2,2),(3,3),(0.710192959008438,1.),(0.607982157956011,
0.625273655815329),.UNSPECIFIED.)
GEOMETRIC_REPRESENTATION_ITEM()
RATIONAL_B_SPLINE_SURFACE(((0.987470879370256,0.987613514606721,0.990694758798813),
(0.987470879370256,0.987613514606721,0.990694758798813)))
REPRESENTATION_ITEM('')
SURFACE()
);
#3931=(
BOUNDED_SURFACE()
B_SPLINE_SURFACE(1,2,((#160915,#160916,#160917,#160918,#160919),(#160920,
#160921,#160922,#160923,#160924)),.UNSPECIFIED.,.F.,.F.,.F.)
B_SPLINE_SURFACE_WITH_KNOTS((2,2),(3,2,3),(0.709719018666025,1.),(0.107879027750091,
0.125170525609407,0.125770422839723),.UNSPECIFIED.)
GEOMETRIC_REPRESENTATION_ITEM()
RATIONAL_B_SPLINE_SURFACE(((0.987469282487682,0.987594391229382,0.990658108926708,
0.990658108926708,0.990658108926708),(0.987469282487682,0.987594391229382,
0.990658108926708,0.990658108926708,0.990658108926708)))
REPRESENTATION_ITEM('')
SURFACE()
);
#3932=(
BOUNDED_SURFACE()
B_SPLINE_SURFACE(1,2,((#160926,#160927,#160928),(#160929,#160930,#160931)),
 .UNSPECIFIED.,.F.,.F.,.F.)
B_SPLINE_SURFACE_WITH_KNOTS((2,2),(3,3),(0.710192959008441,1.),(0.607982157956012,
0.625273655815329),.UNSPECIFIED.)
GEOMETRIC_REPRESENTATION_ITEM()
RATIONAL_B_SPLINE_SURFACE(((0.987470879370256,0.987613514606721,0.990694758798813),
(0.987470879370256,0.987613514606721,0.990694758798813)))
REPRESENTATION_ITEM('')
SURFACE()
);
#3933=(
BOUNDED_SURFACE()
B_SPLINE_SURFACE(1,2,((#160940,#160941,#160942,#160943,#160944),(#160945,
#160946,#160947,#160948,#160949)),.UNSPECIFIED.,.F.,.F.,.F.)
B_SPLINE_SURFACE_WITH_KNOTS((2,2),(3,2,3),(0.709719018663549,1.),(0.10787902775009,
0.125170525609407,0.125770422801283),.UNSPECIFIED.)
GEOMETRIC_REPRESENTATION_ITEM()
RATIONAL_B_SPLINE_SURFACE(((0.987469282487682,0.987594391229382,0.990658108926708,
0.990658108926708,0.990658108926708),(0.987469282487682,0.987594391229382,
0.990658108926708,0.990658108926708,0.990658108926708)))
REPRESENTATION_ITEM('')
SURFACE()
);
#3934=(
BOUNDED_SURFACE()
B_SPLINE_SURFACE(1,2,((#160951,#160952,#160953),(#160954,#160955,#160956)),
 .UNSPECIFIED.,.F.,.F.,.F.)
B_SPLINE_SURFACE_WITH_KNOTS((2,2),(3,3),(0.710192959008435,1.),(0.607982157956012,
0.625273655815329),.UNSPECIFIED.)
GEOMETRIC_REPRESENTATION_ITEM()
RATIONAL_B_SPLINE_SURFACE(((0.987470879370255,0.987613514606721,0.990694758798813),
(0.987470879370255,0.987613514606721,0.990694758798813)))
REPRESENTATION_ITEM('')
SURFACE()
);
#3935=(
BOUNDED_SURFACE()
B_SPLINE_SURFACE(1,2,((#160965,#160966,#160967,#160968,#160969),(#160970,
#160971,#160972,#160973,#160974)),.UNSPECIFIED.,.F.,.F.,.F.)
B_SPLINE_SURFACE_WITH_KNOTS((2,2),(3,2,3),(0.709719018657777,1.),(0.107879027750091,
0.125170525609407,0.125770422807052),.UNSPECIFIED.)
GEOMETRIC_REPRESENTATION_ITEM()
RATIONAL_B_SPLINE_SURFACE(((0.987469282487682,0.987594391229382,0.990658108926708,
0.990658108926708,0.990658108926708),(0.987469282487682,0.987594391229382,
0.990658108926708,0.990658108926708,0.990658108926708)))
REPRESENTATION_ITEM('')
SURFACE()
);
#3936=(
BOUNDED_SURFACE()
B_SPLINE_SURFACE(1,2,((#160976,#160977,#160978),(#160979,#160980,#160981)),
 .UNSPECIFIED.,.F.,.F.,.F.)
B_SPLINE_SURFACE_WITH_KNOTS((2,2),(3,3),(0.710192959008442,1.),(0.607982157956012,
0.625273655815329),.UNSPECIFIED.)
GEOMETRIC_REPRESENTATION_ITEM()
RATIONAL_B_SPLINE_SURFACE(((0.987470879370255,0.987613514606721,0.990694758798813),
(0.987470879370255,0.987613514606721,0.990694758798813)))
REPRESENTATION_ITEM('')
SURFACE()
);
#3937=(
BOUNDED_SURFACE()
B_SPLINE_SURFACE(1,2,((#160990,#160991,#160992,#160993,#160994),(#160995,
#160996,#160997,#160998,#160999)),.UNSPECIFIED.,.F.,.F.,.F.)
B_SPLINE_SURFACE_WITH_KNOTS((2,2),(3,2,3),(0.709719018667416,1.),(0.107879027750091,
0.125170525609407,0.125770422797416),.UNSPECIFIED.)
GEOMETRIC_REPRESENTATION_ITEM()
RATIONAL_B_SPLINE_SURFACE(((0.987469282487682,0.987594391229382,0.990658108926708,
0.990658108926708,0.990658108926708),(0.987469282487682,0.987594391229382,
0.990658108926708,0.990658108926708,0.990658108926708)))
REPRESENTATION_ITEM('')
SURFACE()
);
#3938=(
BOUNDED_SURFACE()
B_SPLINE_SURFACE(1,2,((#161001,#161002,#161003),(#161004,#161005,#161006)),
 .UNSPECIFIED.,.F.,.F.,.F.)
B_SPLINE_SURFACE_WITH_KNOTS((2,2),(3,3),(0.710192959008442,1.),(0.607982157956012,
0.625273655815329),.UNSPECIFIED.)
GEOMETRIC_REPRESENTATION_ITEM()
RATIONAL_B_SPLINE_SURFACE(((0.987470879370256,0.987613514606721,0.990694758798813),
(0.987470879370256,0.987613514606721,0.990694758798813)))
REPRESENTATION_ITEM('')
SURFACE()
);
#3939=(
BOUNDED_SURFACE()
B_SPLINE_SURFACE(1,2,((#161015,#161016,#161017,#161018,#161019),(#161020,
#161021,#161022,#161023,#161024)),.UNSPECIFIED.,.F.,.F.,.F.)
B_SPLINE_SURFACE_WITH_KNOTS((2,2),(3,2,3),(0.70971901865264,1.),(0.107879027750091,
0.125170525609407,0.125770422852652),.UNSPECIFIED.)
GEOMETRIC_REPRESENTATION_ITEM()
RATIONAL_B_SPLINE_SURFACE(((0.987469282487682,0.987594391229382,0.990658108926708,
0.990658108926708,0.990658108926708),(0.987469282487682,0.987594391229382,
0.990658108926708,0.990658108926708,0.990658108926708)))
REPRESENTATION_ITEM('')
SURFACE()
);
#3940=(
BOUNDED_SURFACE()
B_SPLINE_SURFACE(1,2,((#161026,#161027,#161028),(#161029,#161030,#161031)),
 .UNSPECIFIED.,.F.,.F.,.F.)
B_SPLINE_SURFACE_WITH_KNOTS((2,2),(3,3),(0.710192959008445,1.),(0.607982157956012,
0.625273655815329),.UNSPECIFIED.)
GEOMETRIC_REPRESENTATION_ITEM()
RATIONAL_B_SPLINE_SURFACE(((0.987470879370255,0.987613514606721,0.990694758798813),
(0.987470879370255,0.987613514606721,0.990694758798813)))
REPRESENTATION_ITEM('')
SURFACE()
);
#3941=(
BOUNDED_SURFACE()
B_SPLINE_SURFACE(1,2,((#161040,#161041,#161042,#161043,#161044),(#161045,
#161046,#161047,#161048,#161049)),.UNSPECIFIED.,.F.,.F.,.F.)
B_SPLINE_SURFACE_WITH_KNOTS((2,2),(3,2,3),(0.709719018677328,1.),(0.107879027750091,
0.125170525609407,0.125770422723825),.UNSPECIFIED.)
GEOMETRIC_REPRESENTATION_ITEM()
RATIONAL_B_SPLINE_SURFACE(((0.987469282487682,0.987594391229382,0.990658108926708,
0.990658108926708,0.990658108926708),(0.987469282487682,0.987594391229382,
0.990658108926708,0.990658108926708,0.990658108926708)))
REPRESENTATION_ITEM('')
SURFACE()
);
#3942=(
BOUNDED_SURFACE()
B_SPLINE_SURFACE(1,2,((#161051,#161052,#161053),(#161054,#161055,#161056)),
 .UNSPECIFIED.,.F.,.F.,.F.)
B_SPLINE_SURFACE_WITH_KNOTS((2,2),(3,3),(0.710192959008401,1.),(0.607982157956004,
0.625273655815328),.UNSPECIFIED.)
GEOMETRIC_REPRESENTATION_ITEM()
RATIONAL_B_SPLINE_SURFACE(((0.987470879370255,0.987613514606719,0.990694758798812),
(0.987470879370255,0.987613514606719,0.990694758798812)))
REPRESENTATION_ITEM('')
SURFACE()
);
#3943=(
BOUNDED_SURFACE()
B_SPLINE_SURFACE(1,2,((#161065,#161066,#161067,#161068,#161069),(#161070,
#161071,#161072,#161073,#161074)),.UNSPECIFIED.,.F.,.F.,.F.)
B_SPLINE_SURFACE_WITH_KNOTS((2,2),(3,2,3),(0.709719018645982,1.),(0.107879027750092,
0.125170525609408,0.125770422859206),.UNSPECIFIED.)
GEOMETRIC_REPRESENTATION_ITEM()
RATIONAL_B_SPLINE_SURFACE(((0.987469282487682,0.987594391229382,0.990658108926709,
0.990658108926709,0.990658108926709),(0.987469282487682,0.987594391229382,
0.990658108926709,0.990658108926709,0.990658108926709)))
REPRESENTATION_ITEM('')
SURFACE()
);
#3944=(
BOUNDED_SURFACE()
B_SPLINE_SURFACE(1,2,((#161076,#161077,#161078),(#161079,#161080,#161081)),
 .UNSPECIFIED.,.F.,.F.,.F.)
B_SPLINE_SURFACE_WITH_KNOTS((2,2),(3,3),(0.710192959008439,1.),(0.607982157956011,
0.625273655815328),.UNSPECIFIED.)
GEOMETRIC_REPRESENTATION_ITEM()
RATIONAL_B_SPLINE_SURFACE(((0.987470879370255,0.98761351460672,0.990694758798812),
(0.987470879370255,0.98761351460672,0.990694758798812)))
REPRESENTATION_ITEM('')
SURFACE()
);
#3945=(
BOUNDED_SURFACE()
B_SPLINE_SURFACE(1,2,((#161090,#161091,#161092,#161093,#161094),(#161095,
#161096,#161097,#161098,#161099)),.UNSPECIFIED.,.F.,.F.,.F.)
B_SPLINE_SURFACE_WITH_KNOTS((2,2),(3,2,3),(0.709719018671277,1.),(0.107879027750092,
0.125170525609409,0.125770422834533),.UNSPECIFIED.)
GEOMETRIC_REPRESENTATION_ITEM()
RATIONAL_B_SPLINE_SURFACE(((0.987469282487682,0.987594391229382,0.990658108926709,
0.990658108926709,0.990658108926709),(0.987469282487682,0.987594391229382,
0.990658108926709,0.990658108926709,0.990658108926709)))
REPRESENTATION_ITEM('')
SURFACE()
);
#3946=(
BOUNDED_SURFACE()
B_SPLINE_SURFACE(1,2,((#161101,#161102,#161103),(#161104,#161105,#161106)),
 .UNSPECIFIED.,.F.,.F.,.F.)
B_SPLINE_SURFACE_WITH_KNOTS((2,2),(3,3),(0.710192959008442,1.),(0.607982157956011,
0.625273655815328),.UNSPECIFIED.)
GEOMETRIC_REPRESENTATION_ITEM()
RATIONAL_B_SPLINE_SURFACE(((0.987470879370255,0.98761351460672,0.990694758798812),
(0.987470879370255,0.98761351460672,0.990694758798812)))
REPRESENTATION_ITEM('')
SURFACE()
);
#3947=(
BOUNDED_SURFACE()
B_SPLINE_SURFACE(1,2,((#161115,#161116,#161117,#161118,#161119),(#161120,
#161121,#161122,#161123,#161124)),.UNSPECIFIED.,.F.,.F.,.F.)
B_SPLINE_SURFACE_WITH_KNOTS((2,2),(3,2,3),(0.709719018674124,1.),(0.107879027750092,
0.125170525609408,0.125770422790709),.UNSPECIFIED.)
GEOMETRIC_REPRESENTATION_ITEM()
RATIONAL_B_SPLINE_SURFACE(((0.987469282487682,0.987594391229382,0.990658108926709,
0.990658108926709,0.990658108926709),(0.987469282487682,0.987594391229382,
0.990658108926709,0.990658108926709,0.990658108926709)))
REPRESENTATION_ITEM('')
SURFACE()
);
#3948=(
BOUNDED_SURFACE()
B_SPLINE_SURFACE(1,2,((#161126,#161127,#161128),(#161129,#161130,#161131)),
 .UNSPECIFIED.,.F.,.F.,.F.)
B_SPLINE_SURFACE_WITH_KNOTS((2,2),(3,3),(0.710192959008299,1.),(0.607982157956011,
0.625273655815328),.UNSPECIFIED.)
GEOMETRIC_REPRESENTATION_ITEM()
RATIONAL_B_SPLINE_SURFACE(((0.987470879370255,0.98761351460672,0.990694758798812),
(0.987470879370255,0.98761351460672,0.990694758798812)))
REPRESENTATION_ITEM('')
SURFACE()
);
#3949=(
BOUNDED_SURFACE()
B_SPLINE_SURFACE(1,2,((#161140,#161141,#161142,#161143,#161144),(#161145,
#161146,#161147,#161148,#161149)),.UNSPECIFIED.,.F.,.F.,.F.)
B_SPLINE_SURFACE_WITH_KNOTS((2,2),(3,2,3),(0.709719018668243,1.),(0.107879027750092,
0.125170525609408,0.125770422796449),.UNSPECIFIED.)
GEOMETRIC_REPRESENTATION_ITEM()
RATIONAL_B_SPLINE_SURFACE(((0.987469282487682,0.987594391229382,0.990658108926709,
0.990658108926709,0.990658108926709),(0.987469282487682,0.987594391229382,
0.990658108926709,0.990658108926709,0.990658108926709)))
REPRESENTATION_ITEM('')
SURFACE()
);
#3950=(
BOUNDED_SURFACE()
B_SPLINE_SURFACE(1,2,((#161151,#161152,#161153),(#161154,#161155,#161156)),
 .UNSPECIFIED.,.F.,.F.,.F.)
B_SPLINE_SURFACE_WITH_KNOTS((2,2),(3,3),(0.710192959008295,1.),(0.607982157956011,
0.625273655815328),.UNSPECIFIED.)
GEOMETRIC_REPRESENTATION_ITEM()
RATIONAL_B_SPLINE_SURFACE(((0.987470879370255,0.98761351460672,0.990694758798812),
(0.987470879370255,0.98761351460672,0.990694758798812)))
REPRESENTATION_ITEM('')
SURFACE()
);
#3951=(
BOUNDED_SURFACE()
B_SPLINE_SURFACE(1,2,((#161165,#161166,#161167,#161168,#161169),(#161170,
#161171,#161172,#161173,#161174)),.UNSPECIFIED.,.F.,.F.,.F.)
B_SPLINE_SURFACE_WITH_KNOTS((2,2),(3,2,3),(0.709719018652826,1.),(0.107879027750092,
0.125170525609408,0.125770422811858),.UNSPECIFIED.)
GEOMETRIC_REPRESENTATION_ITEM()
RATIONAL_B_SPLINE_SURFACE(((0.987469282487682,0.987594391229382,0.990658108926709,
0.990658108926709,0.990658108926709),(0.987469282487682,0.987594391229382,
0.990658108926709,0.990658108926709,0.990658108926709)))
REPRESENTATION_ITEM('')
SURFACE()
);
#3952=(
BOUNDED_SURFACE()
B_SPLINE_SURFACE(1,2,((#161176,#161177,#161178),(#161179,#161180,#161181)),
 .UNSPECIFIED.,.F.,.F.,.F.)
B_SPLINE_SURFACE_WITH_KNOTS((2,2),(3,3),(0.710192959008283,1.),(0.607982157956011,
0.625273655815328),.UNSPECIFIED.)
GEOMETRIC_REPRESENTATION_ITEM()
RATIONAL_B_SPLINE_SURFACE(((0.987470879370255,0.98761351460672,0.990694758798812),
(0.987470879370255,0.98761351460672,0.990694758798812)))
REPRESENTATION_ITEM('')
SURFACE()
);
#3953=(
BOUNDED_SURFACE()
B_SPLINE_SURFACE(1,2,((#161190,#161191,#161192,#161193,#161194),(#161195,
#161196,#161197,#161198,#161199)),.UNSPECIFIED.,.F.,.F.,.F.)
B_SPLINE_SURFACE_WITH_KNOTS((2,2),(3,2,3),(0.709719018665039,1.),(0.107879027750092,
0.125170525609408,0.125770422799641),.UNSPECIFIED.)
GEOMETRIC_REPRESENTATION_ITEM()
RATIONAL_B_SPLINE_SURFACE(((0.987469282487682,0.987594391229382,0.990658108926709,
0.990658108926709,0.990658108926709),(0.987469282487682,0.987594391229382,
0.990658108926709,0.990658108926709,0.990658108926709)))
REPRESENTATION_ITEM('')
SURFACE()
);
#3954=(
BOUNDED_SURFACE()
B_SPLINE_SURFACE(1,2,((#161201,#161202,#161203),(#161204,#161205,#161206)),
 .UNSPECIFIED.,.F.,.F.,.F.)
B_SPLINE_SURFACE_WITH_KNOTS((2,2),(3,3),(0.710192959006913,1.),(0.607982157956011,
0.625273655815328),.UNSPECIFIED.)
GEOMETRIC_REPRESENTATION_ITEM()
RATIONAL_B_SPLINE_SURFACE(((0.987470879370255,0.98761351460672,0.990694758798812),
(0.987470879370255,0.98761351460672,0.990694758798812)))
REPRESENTATION_ITEM('')
SURFACE()
);
#3955=(
BOUNDED_SURFACE()
B_SPLINE_SURFACE(1,2,((#161215,#161216,#161217,#161218,#161219),(#161220,
#161221,#161222,#161223,#161224)),.UNSPECIFIED.,.F.,.F.,.F.)
B_SPLINE_SURFACE_WITH_KNOTS((2,2),(3,2,3),(0.709719018659893,1.),(0.107879027750092,
0.125170525609408,0.12577042280342),.UNSPECIFIED.)
GEOMETRIC_REPRESENTATION_ITEM()
RATIONAL_B_SPLINE_SURFACE(((0.987469282487682,0.987594391229382,0.990658108926709,
0.990658108926709,0.990658108926709),(0.987469282487682,0.987594391229382,
0.990658108926709,0.990658108926709,0.990658108926709)))
REPRESENTATION_ITEM('')
SURFACE()
);
#3956=(
BOUNDED_SURFACE()
B_SPLINE_SURFACE(1,2,((#161226,#161227,#161228),(#161229,#161230,#161231)),
 .UNSPECIFIED.,.F.,.F.,.F.)
B_SPLINE_SURFACE_WITH_KNOTS((2,2),(3,3),(0.710192959008063,1.),(0.607982157956011,
0.625273655815328),.UNSPECIFIED.)
GEOMETRIC_REPRESENTATION_ITEM()
RATIONAL_B_SPLINE_SURFACE(((0.987470879370255,0.98761351460672,0.990694758798812),
(0.987470879370255,0.98761351460672,0.990694758798812)))
REPRESENTATION_ITEM('')
SURFACE()
);
#3957=(
BOUNDED_SURFACE()
B_SPLINE_SURFACE(1,2,((#161240,#161241,#161242,#161243,#161244),(#161245,
#161246,#161247,#161248,#161249)),.UNSPECIFIED.,.F.,.F.,.F.)
B_SPLINE_SURFACE_WITH_KNOTS((2,2),(3,2,3),(0.709719018652961,1.),(0.107879027750092,
0.125170525609408,0.125770422851709),.UNSPECIFIED.)
GEOMETRIC_REPRESENTATION_ITEM()
RATIONAL_B_SPLINE_SURFACE(((0.987469282487682,0.987594391229382,0.990658108926709,
0.990658108926709,0.990658108926709),(0.987469282487682,0.987594391229382,
0.990658108926709,0.990658108926709,0.990658108926709)))
REPRESENTATION_ITEM('')
SURFACE()
);
#3958=(
BOUNDED_SURFACE()
B_SPLINE_SURFACE(1,2,((#161251,#161252,#161253),(#161254,#161255,#161256)),
 .UNSPECIFIED.,.F.,.F.,.F.)
B_SPLINE_SURFACE_WITH_KNOTS((2,2),(3,3),(0.710192959008438,1.),(0.607982157956011,
0.625273655815328),.UNSPECIFIED.)
GEOMETRIC_REPRESENTATION_ITEM()
RATIONAL_B_SPLINE_SURFACE(((0.987470879370255,0.98761351460672,0.990694758798812),
(0.987470879370255,0.98761351460672,0.990694758798812)))
REPRESENTATION_ITEM('')
SURFACE()
);
#3959=(
BOUNDED_SURFACE()
B_SPLINE_SURFACE(1,2,((#161265,#161266,#161267,#161268,#161269),(#161270,
#161271,#161272,#161273,#161274)),.UNSPECIFIED.,.F.,.F.,.F.)
B_SPLINE_SURFACE_WITH_KNOTS((2,2),(3,2,3),(0.709719018650375,1.),(0.107879027750092,
0.125170525609408,0.125770422855389),.UNSPECIFIED.)
GEOMETRIC_REPRESENTATION_ITEM()
RATIONAL_B_SPLINE_SURFACE(((0.987469282487682,0.987594391229382,0.990658108926709,
0.990658108926709,0.990658108926709),(0.987469282487682,0.987594391229382,
0.990658108926709,0.990658108926709,0.990658108926709)))
REPRESENTATION_ITEM('')
SURFACE()
);
#3960=(
BOUNDED_SURFACE()
B_SPLINE_SURFACE(1,2,((#161276,#161277,#161278),(#161279,#161280,#161281)),
 .UNSPECIFIED.,.F.,.F.,.F.)
B_SPLINE_SURFACE_WITH_KNOTS((2,2),(3,3),(0.71019295900844,1.),(0.607982157956011,
0.625273655815328),.UNSPECIFIED.)
GEOMETRIC_REPRESENTATION_ITEM()
RATIONAL_B_SPLINE_SURFACE(((0.987470879370255,0.987613514606721,0.990694758798812),
(0.987470879370255,0.98761351460672,0.990694758798812)))
REPRESENTATION_ITEM('')
SURFACE()
);
#3961=(
BOUNDED_SURFACE()
B_SPLINE_SURFACE(1,2,((#161290,#161291,#161292,#161293,#161294),(#161295,
#161296,#161297,#161298,#161299)),.UNSPECIFIED.,.F.,.F.,.F.)
B_SPLINE_SURFACE_WITH_KNOTS((2,2),(3,2,3),(0.709719018647816,1.),(0.107879027750092,
0.125170525609408,0.125770422857201),.UNSPECIFIED.)
GEOMETRIC_REPRESENTATION_ITEM()
RATIONAL_B_SPLINE_SURFACE(((0.987469282487682,0.987594391229382,0.990658108926709,
0.990658108926709,0.990658108926709),(0.987469282487682,0.987594391229382,
0.990658108926709,0.990658108926709,0.990658108926709)))
REPRESENTATION_ITEM('')
SURFACE()
);
#3962=(
BOUNDED_SURFACE()
B_SPLINE_SURFACE(1,2,((#161301,#161302,#161303),(#161304,#161305,#161306)),
 .UNSPECIFIED.,.F.,.F.,.F.)
B_SPLINE_SURFACE_WITH_KNOTS((2,2),(3,3),(0.710192959008442,1.),(0.607982157956011,
0.625273655815328),.UNSPECIFIED.)
GEOMETRIC_REPRESENTATION_ITEM()
RATIONAL_B_SPLINE_SURFACE(((0.987470879370255,0.98761351460672,0.990694758798812),
(0.987470879370255,0.98761351460672,0.990694758798812)))
REPRESENTATION_ITEM('')
SURFACE()
);
#3963=(
BOUNDED_SURFACE()
B_SPLINE_SURFACE(1,2,((#161315,#161316,#161317,#161318,#161319),(#161320,
#161321,#161322,#161323,#161324)),.UNSPECIFIED.,.F.,.F.,.F.)
B_SPLINE_SURFACE_WITH_KNOTS((2,2),(3,2,3),(0.709719018663423,1.),(0.107879027750092,
0.125170525609408,0.125770422801407),.UNSPECIFIED.)
GEOMETRIC_REPRESENTATION_ITEM()
RATIONAL_B_SPLINE_SURFACE(((0.987469282487682,0.987594391229382,0.990658108926709,
0.990658108926709,0.990658108926709),(0.987469282487682,0.987594391229382,
0.990658108926709,0.990658108926709,0.990658108926709)))
REPRESENTATION_ITEM('')
SURFACE()
);
#3964=(
BOUNDED_SURFACE()
B_SPLINE_SURFACE(1,2,((#161326,#161327,#161328,#161329,#161330),(#161331,
#161332,#161333,#161334,#161335)),.UNSPECIFIED.,.F.,.F.,.F.)
B_SPLINE_SURFACE_WITH_KNOTS((2,2),(3,2,3),(0.,0.290280981336755),(0.607879027750091,
0.625170525609408,0.625770422759447),.UNSPECIFIED.)
GEOMETRIC_REPRESENTATION_ITEM()
RATIONAL_B_SPLINE_SURFACE(((0.987469282487682,0.987594391229382,0.990658108926708,
0.990658108926708,0.990658108926708),(0.987469282487682,0.987594391229382,
0.990658108926708,0.990658108926708,0.990658108926708)))
REPRESENTATION_ITEM('')
SURFACE()
);
#3965=(
BOUNDED_SURFACE()
B_SPLINE_SURFACE(1,2,((#161346,#161347,#161348),(#161349,#161350,#161351)),
 .UNSPECIFIED.,.F.,.F.,.F.)
B_SPLINE_SURFACE_WITH_KNOTS((2,2),(3,3),(0.,0.289807040991561),(0.107982157956012,
0.125273655815329),.UNSPECIFIED.)
GEOMETRIC_REPRESENTATION_ITEM()
RATIONAL_B_SPLINE_SURFACE(((0.987470879370255,0.987613514606721,0.990694758798813),
(0.987470879370255,0.987613514606721,0.990694758798813)))
REPRESENTATION_ITEM('')
SURFACE()
);
#3966=(
BOUNDED_SURFACE()
B_SPLINE_SURFACE(1,2,((#161369,#161370,#161371,#161372,#161373),(#161374,
#161375,#161376,#161377,#161378)),.UNSPECIFIED.,.F.,.F.,.F.)
B_SPLINE_SURFACE_WITH_KNOTS((2,2),(3,2,3),(0.,0.290280981329489),(0.607879027750091,
0.625170525609407,0.625770422752178),.UNSPECIFIED.)
GEOMETRIC_REPRESENTATION_ITEM()
RATIONAL_B_SPLINE_SURFACE(((0.987469282487682,0.987594391229382,0.990658108926708,
0.990658108926708,0.990658108926708),(0.987469282487682,0.987594391229382,
0.990658108926708,0.990658108926708,0.990658108926708)))
REPRESENTATION_ITEM('')
SURFACE()
);
#3967=(
BOUNDED_SURFACE()
B_SPLINE_SURFACE(1,2,((#161385,#161386,#161387),(#161388,#161389,#161390)),
 .UNSPECIFIED.,.F.,.F.,.F.)
B_SPLINE_SURFACE_WITH_KNOTS((2,2),(3,3),(0.,0.289807040991559),(0.107982157956012,
0.125273655815329),.UNSPECIFIED.)
GEOMETRIC_REPRESENTATION_ITEM()
RATIONAL_B_SPLINE_SURFACE(((0.987470879370256,0.987613514606721,0.990694758798813),
(0.987470879370255,0.987613514606721,0.990694758798813)))
REPRESENTATION_ITEM('')
SURFACE()
);
#3968=(
BOUNDED_SURFACE()
B_SPLINE_SURFACE(1,2,((#161408,#161409,#161410,#161411,#161412),(#161413,
#161414,#161415,#161416,#161417)),.UNSPECIFIED.,.F.,.F.,.F.)
B_SPLINE_SURFACE_WITH_KNOTS((2,2),(3,2,3),(0.,0.290280981342653),(0.607879027750091,
0.625170525609407,0.625770422765346),.UNSPECIFIED.)
GEOMETRIC_REPRESENTATION_ITEM()
RATIONAL_B_SPLINE_SURFACE(((0.987469282487682,0.987594391229382,0.990658108926708,
0.990658108926708,0.990658108926708),(0.987469282487682,0.987594391229382,
0.990658108926708,0.990658108926708,0.990658108926708)))
REPRESENTATION_ITEM('')
SURFACE()
);
#3969=(
BOUNDED_SURFACE()
B_SPLINE_SURFACE(1,2,((#161424,#161425,#161426),(#161427,#161428,#161429)),
 .UNSPECIFIED.,.F.,.F.,.F.)
B_SPLINE_SURFACE_WITH_KNOTS((2,2),(3,3),(0.,0.289807040991559),(0.107982157956012,
0.125273655815329),.UNSPECIFIED.)
GEOMETRIC_REPRESENTATION_ITEM()
RATIONAL_B_SPLINE_SURFACE(((0.987470879370255,0.987613514606721,0.990694758798813),
(0.987470879370255,0.987613514606721,0.990694758798813)))
REPRESENTATION_ITEM('')
SURFACE()
);
#3970=(
BOUNDED_SURFACE()
B_SPLINE_SURFACE(1,2,((#161447,#161448,#161449,#161450,#161451),(#161452,
#161453,#161454,#161455,#161456)),.UNSPECIFIED.,.F.,.F.,.F.)
B_SPLINE_SURFACE_WITH_KNOTS((2,2),(3,2,3),(0.,0.290280981329113),(0.607879027750091,
0.625170525609408,0.625770422751802),.UNSPECIFIED.)
GEOMETRIC_REPRESENTATION_ITEM()
RATIONAL_B_SPLINE_SURFACE(((0.987469282487682,0.987594391229382,0.990658108926708,
0.990658108926708,0.990658108926708),(0.987469282487682,0.987594391229382,
0.990658108926708,0.990658108926708,0.990658108926708)))
REPRESENTATION_ITEM('')
SURFACE()
);
#3971=(
BOUNDED_SURFACE()
B_SPLINE_SURFACE(1,2,((#161463,#161464,#161465),(#161466,#161467,#161468)),
 .UNSPECIFIED.,.F.,.F.,.F.)
B_SPLINE_SURFACE_WITH_KNOTS((2,2),(3,3),(0.,0.289807040991557),(0.107982157956012,
0.125273655815328),.UNSPECIFIED.)
GEOMETRIC_REPRESENTATION_ITEM()
RATIONAL_B_SPLINE_SURFACE(((0.987470879370256,0.987613514606721,0.990694758798812),
(0.987470879370256,0.987613514606721,0.990694758798812)))
REPRESENTATION_ITEM('')
SURFACE()
);
#3972=(
BOUNDED_SURFACE()
B_SPLINE_SURFACE(1,2,((#161486,#161487,#161488,#161489,#161490),(#161491,
#161492,#161493,#161494,#161495)),.UNSPECIFIED.,.F.,.F.,.F.)
B_SPLINE_SURFACE_WITH_KNOTS((2,2),(3,2,3),(0.,0.290280981348175),(0.607879027750092,
0.625170525609408,0.625770422770872),.UNSPECIFIED.)
GEOMETRIC_REPRESENTATION_ITEM()
RATIONAL_B_SPLINE_SURFACE(((0.987469282487682,0.987594391229382,0.990658108926709,
0.990658108926709,0.990658108926709),(0.987469282487682,0.987594391229382,
0.990658108926709,0.990658108926709,0.990658108926709)))
REPRESENTATION_ITEM('')
SURFACE()
);
#3973=(
BOUNDED_SURFACE()
B_SPLINE_SURFACE(1,2,((#161502,#161503,#161504),(#161505,#161506,#161507)),
 .UNSPECIFIED.,.F.,.F.,.F.)
B_SPLINE_SURFACE_WITH_KNOTS((2,2),(3,3),(0.,0.289807040991561),(0.107982157956011,
0.125273655815328),.UNSPECIFIED.)
GEOMETRIC_REPRESENTATION_ITEM()
RATIONAL_B_SPLINE_SURFACE(((0.987470879370255,0.98761351460672,0.990694758798812),
(0.987470879370255,0.98761351460672,0.990694758798812)))
REPRESENTATION_ITEM('')
SURFACE()
);
#3974=(
BOUNDED_SURFACE()
B_SPLINE_SURFACE(1,2,((#161525,#161526,#161527,#161528,#161529),(#161530,
#161531,#161532,#161533,#161534)),.UNSPECIFIED.,.F.,.F.,.F.)
B_SPLINE_SURFACE_WITH_KNOTS((2,2),(3,2,3),(0.,0.290280981322439),(0.607879027750092,
0.625170525609409,0.625770422745125),.UNSPECIFIED.)
GEOMETRIC_REPRESENTATION_ITEM()
RATIONAL_B_SPLINE_SURFACE(((0.987469282487682,0.987594391229382,0.990658108926709,
0.990658108926709,0.990658108926709),(0.987469282487682,0.987594391229382,
0.990658108926709,0.990658108926709,0.990658108926709)))
REPRESENTATION_ITEM('')
SURFACE()
);
#3975=(
BOUNDED_SURFACE()
B_SPLINE_SURFACE(1,2,((#161541,#161542,#161543),(#161544,#161545,#161546)),
 .UNSPECIFIED.,.F.,.F.,.F.)
B_SPLINE_SURFACE_WITH_KNOTS((2,2),(3,3),(0.,0.289807040991559),(0.107982157956011,
0.125273655815328),.UNSPECIFIED.)
GEOMETRIC_REPRESENTATION_ITEM()
RATIONAL_B_SPLINE_SURFACE(((0.987470879370255,0.98761351460672,0.990694758798812),
(0.987470879370255,0.98761351460672,0.990694758798812)))
REPRESENTATION_ITEM('')
SURFACE()
);
#3976=(
BOUNDED_SURFACE()
B_SPLINE_SURFACE(1,2,((#161564,#161565,#161566,#161567,#161568),(#161569,
#161570,#161571,#161572,#161573)),.UNSPECIFIED.,.F.,.F.,.F.)
B_SPLINE_SURFACE_WITH_KNOTS((2,2),(3,2,3),(0.,0.290280981323384),(0.607879027750092,
0.625170525609408,0.625770422746075),.UNSPECIFIED.)
GEOMETRIC_REPRESENTATION_ITEM()
RATIONAL_B_SPLINE_SURFACE(((0.987469282487682,0.987594391229382,0.990658108926709,
0.990658108926709,0.990658108926709),(0.987469282487682,0.987594391229382,
0.990658108926709,0.990658108926709,0.990658108926709)))
REPRESENTATION_ITEM('')
SURFACE()
);
#3977=(
BOUNDED_SURFACE()
B_SPLINE_SURFACE(1,2,((#161580,#161581,#161582),(#161583,#161584,#161585)),
 .UNSPECIFIED.,.F.,.F.,.F.)
B_SPLINE_SURFACE_WITH_KNOTS((2,2),(3,3),(0.,0.289807040991564),(0.107982157956011,
0.125273655815328),.UNSPECIFIED.)
GEOMETRIC_REPRESENTATION_ITEM()
RATIONAL_B_SPLINE_SURFACE(((0.987470879370255,0.98761351460672,0.990694758798812),
(0.987470879370255,0.98761351460672,0.990694758798812)))
REPRESENTATION_ITEM('')
SURFACE()
);
#3978=(
BOUNDED_SURFACE()
B_SPLINE_SURFACE(1,2,((#161597,#161598,#161599,#161600,#161601),(#161602,
#161603,#161604,#161605,#161606)),.UNSPECIFIED.,.F.,.F.,.F.)
B_SPLINE_SURFACE_WITH_KNOTS((2,2),(3,2,3),(0.,0.289942149041009),(0.607879027750092,
0.625170525609408,0.625431590463695),.UNSPECIFIED.)
GEOMETRIC_REPRESENTATION_ITEM()
RATIONAL_B_SPLINE_SURFACE(((0.987469282487682,0.987594391229382,0.990658108926709,
0.990658108926709,0.990658108926709),(0.987469282487682,0.987594391229382,
0.990658108926709,0.990658108926709,0.990658108926709)))
REPRESENTATION_ITEM('')
SURFACE()
);
#3979=(
BOUNDED_SURFACE()
B_SPLINE_SURFACE(1,2,((#161608,#161609,#161610),(#161611,#161612,#161613)),
 .UNSPECIFIED.,.F.,.F.,.F.)
B_SPLINE_SURFACE_WITH_KNOTS((2,2),(3,3),(0.,0.289807040991559),(0.107982157956011,
0.125273655815328),.UNSPECIFIED.)
GEOMETRIC_REPRESENTATION_ITEM()
RATIONAL_B_SPLINE_SURFACE(((0.987470879370255,0.98761351460672,0.990694758798812),
(0.987470879370255,0.98761351460672,0.990694758798812)))
REPRESENTATION_ITEM('')
SURFACE()
);
#3980=(
BOUNDED_SURFACE()
B_SPLINE_SURFACE(1,2,((#161631,#161632,#161633,#161634,#161635),(#161636,
#161637,#161638,#161639,#161640)),.UNSPECIFIED.,.F.,.F.,.F.)
B_SPLINE_SURFACE_WITH_KNOTS((2,2),(3,2,3),(0.,0.290280981345223),(0.607879027750092,
0.625170525609409,0.625770422767914),.UNSPECIFIED.)
GEOMETRIC_REPRESENTATION_ITEM()
RATIONAL_B_SPLINE_SURFACE(((0.987469282487682,0.987594391229382,0.990658108926709,
0.990658108926709,0.990658108926709),(0.987469282487682,0.987594391229382,
0.990658108926709,0.990658108926709,0.990658108926709)))
REPRESENTATION_ITEM('')
SURFACE()
);
#3981=(
BOUNDED_SURFACE()
B_SPLINE_SURFACE(1,2,((#161647,#161648,#161649),(#161650,#161651,#161652)),
 .UNSPECIFIED.,.F.,.F.,.F.)
B_SPLINE_SURFACE_WITH_KNOTS((2,2),(3,3),(0.,0.289807040991563),(0.107982157956011,
0.125273655815328),.UNSPECIFIED.)
GEOMETRIC_REPRESENTATION_ITEM()
RATIONAL_B_SPLINE_SURFACE(((0.987470879370255,0.987613514606721,0.990694758798812),
(0.987470879370255,0.987613514606721,0.990694758798812)))
REPRESENTATION_ITEM('')
SURFACE()
);
#3982=(
BOUNDED_SURFACE()
B_SPLINE_SURFACE(1,2,((#161670,#161671,#161672,#161673,#161674),(#161675,
#161676,#161677,#161678,#161679)),.UNSPECIFIED.,.F.,.F.,.F.)
B_SPLINE_SURFACE_WITH_KNOTS((2,2),(3,2,3),(0.,0.290280981333581),(0.607879027750092,
0.625170525609408,0.625770422756274),.UNSPECIFIED.)
GEOMETRIC_REPRESENTATION_ITEM()
RATIONAL_B_SPLINE_SURFACE(((0.987469282487682,0.987594391229382,0.990658108926709,
0.990658108926709,0.990658108926709),(0.987469282487682,0.987594391229382,
0.990658108926709,0.990658108926709,0.990658108926709)))
REPRESENTATION_ITEM('')
SURFACE()
);
#3983=(
BOUNDED_SURFACE()
B_SPLINE_SURFACE(1,2,((#161686,#161687,#161688),(#161689,#161690,#161691)),
 .UNSPECIFIED.,.F.,.F.,.F.)
B_SPLINE_SURFACE_WITH_KNOTS((2,2),(3,3),(0.,0.28980704099156),(0.107982157956011,
0.125273655815328),.UNSPECIFIED.)
GEOMETRIC_REPRESENTATION_ITEM()
RATIONAL_B_SPLINE_SURFACE(((0.987470879370255,0.98761351460672,0.990694758798812),
(0.987470879370256,0.987613514606721,0.990694758798812)))
REPRESENTATION_ITEM('')
SURFACE()
);
#3984=(
BOUNDED_SURFACE()
B_SPLINE_SURFACE(1,2,((#161709,#161710,#161711,#161712,#161713),(#161714,
#161715,#161716,#161717,#161718)),.UNSPECIFIED.,.F.,.F.,.F.)
B_SPLINE_SURFACE_WITH_KNOTS((2,2),(3,2,3),(0.,0.290280981337563),(0.607879027750092,
0.625170525609408,0.625770422760259),.UNSPECIFIED.)
GEOMETRIC_REPRESENTATION_ITEM()
RATIONAL_B_SPLINE_SURFACE(((0.987469282487682,0.987594391229382,0.990658108926709,
0.990658108926709,0.990658108926709),(0.987469282487682,0.987594391229382,
0.990658108926709,0.990658108926709,0.990658108926709)))
REPRESENTATION_ITEM('')
SURFACE()
);
#3985=(
BOUNDED_SURFACE()
B_SPLINE_SURFACE(1,2,((#161725,#161726,#161727),(#161728,#161729,#161730)),
 .UNSPECIFIED.,.F.,.F.,.F.)
B_SPLINE_SURFACE_WITH_KNOTS((2,2),(3,3),(0.,0.289807040991559),(0.107982157956011,
0.125273655815328),.UNSPECIFIED.)
GEOMETRIC_REPRESENTATION_ITEM()
RATIONAL_B_SPLINE_SURFACE(((0.987470879370255,0.98761351460672,0.990694758798812),
(0.987470879370255,0.98761351460672,0.990694758798812)))
REPRESENTATION_ITEM('')
SURFACE()
);
#3986=(
BOUNDED_SURFACE()
B_SPLINE_SURFACE(1,2,((#161748,#161749,#161750,#161751,#161752),(#161753,
#161754,#161755,#161756,#161757)),.UNSPECIFIED.,.F.,.F.,.F.)
B_SPLINE_SURFACE_WITH_KNOTS((2,2),(3,2,3),(0.,0.290280981340732),(0.607879027750092,
0.625170525609409,0.62577042276343),.UNSPECIFIED.)
GEOMETRIC_REPRESENTATION_ITEM()
RATIONAL_B_SPLINE_SURFACE(((0.987469282487682,0.987594391229382,0.990658108926709,
0.990658108926709,0.990658108926709),(0.987469282487682,0.987594391229382,
0.990658108926709,0.990658108926709,0.990658108926709)))
REPRESENTATION_ITEM('')
SURFACE()
);
#3987=(
BOUNDED_SURFACE()
B_SPLINE_SURFACE(1,2,((#161764,#161765,#161766),(#161767,#161768,#161769)),
 .UNSPECIFIED.,.F.,.F.,.F.)
B_SPLINE_SURFACE_WITH_KNOTS((2,2),(3,3),(0.,0.289807040991564),(0.107982157956011,
0.125273655815328),.UNSPECIFIED.)
GEOMETRIC_REPRESENTATION_ITEM()
RATIONAL_B_SPLINE_SURFACE(((0.987470879370255,0.98761351460672,0.990694758798812),
(0.987470879370255,0.98761351460672,0.990694758798812)))
REPRESENTATION_ITEM('')
SURFACE()
);
#3988=(
BOUNDED_SURFACE()
B_SPLINE_SURFACE(1,2,((#161787,#161788,#161789,#161790,#161791),(#161792,
#161793,#161794,#161795,#161796)),.UNSPECIFIED.,.F.,.F.,.F.)
B_SPLINE_SURFACE_WITH_KNOTS((2,2),(3,2,3),(0.,0.290280981343082),(0.607879027750091,
0.625170525609408,0.625770422765774),.UNSPECIFIED.)
GEOMETRIC_REPRESENTATION_ITEM()
RATIONAL_B_SPLINE_SURFACE(((0.987469282487682,0.987594391229382,0.990658108926709,
0.990658108926709,0.990658108926709),(0.987469282487682,0.987594391229382,
0.990658108926709,0.990658108926709,0.990658108926709)))
REPRESENTATION_ITEM('')
SURFACE()
);
#3989=(
BOUNDED_SURFACE()
B_SPLINE_SURFACE(1,2,((#161803,#161804,#161805),(#161806,#161807,#161808)),
 .UNSPECIFIED.,.F.,.F.,.F.)
B_SPLINE_SURFACE_WITH_KNOTS((2,2),(3,3),(0.,0.289807040991561),(0.107982157956011,
0.125273655815328),.UNSPECIFIED.)
GEOMETRIC_REPRESENTATION_ITEM()
RATIONAL_B_SPLINE_SURFACE(((0.987470879370255,0.98761351460672,0.990694758798812),
(0.987470879370256,0.987613514606721,0.990694758798812)))
REPRESENTATION_ITEM('')
SURFACE()
);
#3990=(
BOUNDED_SURFACE()
B_SPLINE_SURFACE(1,2,((#161826,#161827,#161828,#161829,#161830),(#161831,
#161832,#161833,#161834,#161835)),.UNSPECIFIED.,.F.,.F.,.F.)
B_SPLINE_SURFACE_WITH_KNOTS((2,2),(3,2,3),(0.,0.290280981344683),(0.607879027750092,
0.625170525609408,0.625770422767375),.UNSPECIFIED.)
GEOMETRIC_REPRESENTATION_ITEM()
RATIONAL_B_SPLINE_SURFACE(((0.987469282487682,0.987594391229382,0.990658108926709,
0.990658108926709,0.990658108926709),(0.987469282487682,0.987594391229382,
0.990658108926709,0.990658108926709,0.990658108926709)))
REPRESENTATION_ITEM('')
SURFACE()
);
#3991=(
BOUNDED_SURFACE()
B_SPLINE_SURFACE(1,2,((#161842,#161843,#161844),(#161845,#161846,#161847)),
 .UNSPECIFIED.,.F.,.F.,.F.)
B_SPLINE_SURFACE_WITH_KNOTS((2,2),(3,3),(0.,0.289807040991559),(0.107982157956011,
0.125273655815328),.UNSPECIFIED.)
GEOMETRIC_REPRESENTATION_ITEM()
RATIONAL_B_SPLINE_SURFACE(((0.987470879370255,0.98761351460672,0.990694758798812),
(0.987470879370255,0.98761351460672,0.990694758798812)))
REPRESENTATION_ITEM('')
SURFACE()
);
#3992=(
BOUNDED_SURFACE()
B_SPLINE_SURFACE(1,2,((#161865,#161866,#161867,#161868,#161869),(#161870,
#161871,#161872,#161873,#161874)),.UNSPECIFIED.,.F.,.F.,.F.)
B_SPLINE_SURFACE_WITH_KNOTS((2,2),(3,2,3),(0.,0.290280981333494),(0.607879027750092,
0.625170525609409,0.625770422756186),.UNSPECIFIED.)
GEOMETRIC_REPRESENTATION_ITEM()
RATIONAL_B_SPLINE_SURFACE(((0.987469282487682,0.987594391229382,0.990658108926709,
0.990658108926709,0.990658108926709),(0.987469282487682,0.987594391229382,
0.990658108926709,0.990658108926709,0.990658108926709)))
REPRESENTATION_ITEM('')
SURFACE()
);
#3993=(
BOUNDED_SURFACE()
B_SPLINE_SURFACE(1,2,((#161881,#161882,#161883),(#161884,#161885,#161886)),
 .UNSPECIFIED.,.F.,.F.,.F.)
B_SPLINE_SURFACE_WITH_KNOTS((2,2),(3,3),(0.,0.289807040991563),(0.107982157956011,
0.125273655815328),.UNSPECIFIED.)
GEOMETRIC_REPRESENTATION_ITEM()
RATIONAL_B_SPLINE_SURFACE(((0.987470879370255,0.98761351460672,0.990694758798812),
(0.987470879370255,0.98761351460672,0.990694758798812)))
REPRESENTATION_ITEM('')
SURFACE()
);
#3994=(
BOUNDED_SURFACE()
B_SPLINE_SURFACE(1,2,((#161904,#161905,#161906,#161907,#161908),(#161909,
#161910,#161911,#161912,#161913)),.UNSPECIFIED.,.F.,.F.,.F.)
B_SPLINE_SURFACE_WITH_KNOTS((2,2),(3,2,3),(0.,0.290280981335216),(0.607879027750091,
0.625170525609408,0.625770422757911),.UNSPECIFIED.)
GEOMETRIC_REPRESENTATION_ITEM()
RATIONAL_B_SPLINE_SURFACE(((0.987469282487682,0.987594391229382,0.990658108926709,
0.990658108926709,0.990658108926709),(0.987469282487682,0.987594391229382,
0.990658108926709,0.990658108926709,0.990658108926709)))
REPRESENTATION_ITEM('')
SURFACE()
);
#3995=(
BOUNDED_SURFACE()
B_SPLINE_SURFACE(1,2,((#161920,#161921,#161922),(#161923,#161924,#161925)),
 .UNSPECIFIED.,.F.,.F.,.F.)
B_SPLINE_SURFACE_WITH_KNOTS((2,2),(3,3),(0.,0.289807040991561),(0.107982157956011,
0.125273655815328),.UNSPECIFIED.)
GEOMETRIC_REPRESENTATION_ITEM()
RATIONAL_B_SPLINE_SURFACE(((0.987470879370255,0.98761351460672,0.990694758798812),
(0.987470879370255,0.98761351460672,0.990694758798812)))
REPRESENTATION_ITEM('')
SURFACE()
);
#3996=(
BOUNDED_SURFACE()
B_SPLINE_SURFACE(1,2,((#161943,#161944,#161945,#161946,#161947),(#161948,
#161949,#161950,#161951,#161952)),.UNSPECIFIED.,.F.,.F.,.F.)
B_SPLINE_SURFACE_WITH_KNOTS((2,2),(3,2,3),(0.,0.290280981343155),(0.607879027750092,
0.625170525609409,0.625770422765852),.UNSPECIFIED.)
GEOMETRIC_REPRESENTATION_ITEM()
RATIONAL_B_SPLINE_SURFACE(((0.987469282487682,0.987594391229382,0.990658108926709,
0.990658108926709,0.990658108926709),(0.987469282487682,0.987594391229382,
0.990658108926709,0.990658108926709,0.990658108926709)))
REPRESENTATION_ITEM('')
SURFACE()
);
#3997=(
BOUNDED_SURFACE()
B_SPLINE_SURFACE(1,2,((#161959,#161960,#161961),(#161962,#161963,#161964)),
 .UNSPECIFIED.,.F.,.F.,.F.)
B_SPLINE_SURFACE_WITH_KNOTS((2,2),(3,3),(0.,0.289807040991557),(0.107982157956011,
0.125273655815328),.UNSPECIFIED.)
GEOMETRIC_REPRESENTATION_ITEM()
RATIONAL_B_SPLINE_SURFACE(((0.987470879370255,0.98761351460672,0.990694758798812),
(0.987470879370255,0.98761351460672,0.990694758798812)))
REPRESENTATION_ITEM('')
SURFACE()
);
#3998=(
BOUNDED_SURFACE()
B_SPLINE_SURFACE(1,2,((#161982,#161983,#161984,#161985,#161986),(#161987,
#161988,#161989,#161990,#161991)),.UNSPECIFIED.,.F.,.F.,.F.)
B_SPLINE_SURFACE_WITH_KNOTS((2,2),(3,2,3),(0.,0.290280981344033),(0.607879027750092,
0.625170525609408,0.625770422766729),.UNSPECIFIED.)
GEOMETRIC_REPRESENTATION_ITEM()
RATIONAL_B_SPLINE_SURFACE(((0.987469282487682,0.987594391229382,0.990658108926709,
0.990658108926709,0.990658108926709),(0.987469282487682,0.987594391229382,
0.990658108926709,0.990658108926709,0.990658108926709)))
REPRESENTATION_ITEM('')
SURFACE()
);
#3999=(
BOUNDED_SURFACE()
B_SPLINE_SURFACE(1,2,((#161998,#161999,#162000),(#162001,#162002,#162003)),
 .UNSPECIFIED.,.F.,.F.,.F.)
B_SPLINE_SURFACE_WITH_KNOTS((2,2),(3,3),(0.,0.28980704099156),(0.107982157956006,
0.125273655815328),.UNSPECIFIED.)
GEOMETRIC_REPRESENTATION_ITEM()
RATIONAL_B_SPLINE_SURFACE(((0.987470879370255,0.98761351460672,0.990694758798812),
(0.987470879370255,0.98761351460672,0.990694758798812)))
REPRESENTATION_ITEM('')
SURFACE()
);
#4000=(
BOUNDED_SURFACE()
B_SPLINE_SURFACE(1,2,((#162021,#162022,#162023,#162024,#162025),(#162026,
#162027,#162028,#162029,#162030)),.UNSPECIFIED.,.F.,.F.,.F.)
B_SPLINE_SURFACE_WITH_KNOTS((2,2),(3,2,3),(0.,0.290280981330619),(0.607879027750092,
0.625170525609407,0.625770422753314),.UNSPECIFIED.)
GEOMETRIC_REPRESENTATION_ITEM()
RATIONAL_B_SPLINE_SURFACE(((0.987469282487682,0.987594391229382,0.990658108926708,
0.990658108926708,0.990658108926708),(0.987469282487682,0.987594391229382,
0.990658108926708,0.990658108926708,0.990658108926708)))
REPRESENTATION_ITEM('')
SURFACE()
);
#4001=(
BOUNDED_SURFACE()
B_SPLINE_SURFACE(1,2,((#162037,#162038,#162039),(#162040,#162041,#162042)),
 .UNSPECIFIED.,.F.,.F.,.F.)
B_SPLINE_SURFACE_WITH_KNOTS((2,2),(3,3),(0.,0.289807040991596),(0.107982157956012,
0.125273655815329),.UNSPECIFIED.)
GEOMETRIC_REPRESENTATION_ITEM()
RATIONAL_B_SPLINE_SURFACE(((0.987470879370256,0.987613514606721,0.990694758798813),
(0.987470879370256,0.987613514606721,0.990694758798813)))
REPRESENTATION_ITEM('')
SURFACE()
);
#4002=(
BOUNDED_SURFACE()
B_SPLINE_SURFACE(1,2,((#162060,#162061,#162062,#162063,#162064),(#162065,
#162066,#162067,#162068,#162069)),.UNSPECIFIED.,.F.,.F.,.F.)
B_SPLINE_SURFACE_WITH_KNOTS((2,2),(3,2,3),(0.,0.290280981345742),(0.607879027750091,
0.625170525609407,0.625770422768438),.UNSPECIFIED.)
GEOMETRIC_REPRESENTATION_ITEM()
RATIONAL_B_SPLINE_SURFACE(((0.987469282487682,0.987594391229382,0.990658108926708,
0.990658108926708,0.990658108926708),(0.987469282487682,0.987594391229382,
0.990658108926708,0.990658108926708,0.990658108926708)))
REPRESENTATION_ITEM('')
SURFACE()
);
#4003=(
BOUNDED_SURFACE()
B_SPLINE_SURFACE(1,2,((#162076,#162077,#162078),(#162079,#162080,#162081)),
 .UNSPECIFIED.,.F.,.F.,.F.)
B_SPLINE_SURFACE_WITH_KNOTS((2,2),(3,3),(0.,0.289807040991564),(0.107982157956012,
0.125273655815329),.UNSPECIFIED.)
GEOMETRIC_REPRESENTATION_ITEM()
RATIONAL_B_SPLINE_SURFACE(((0.987470879370256,0.987613514606721,0.990694758798813),
(0.987470879370255,0.987613514606721,0.990694758798813)))
REPRESENTATION_ITEM('')
SURFACE()
);
#4004=(
BOUNDED_SURFACE()
B_SPLINE_SURFACE(1,2,((#162099,#162100,#162101,#162102,#162103),(#162104,
#162105,#162106,#162107,#162108)),.UNSPECIFIED.,.F.,.F.,.F.)
B_SPLINE_SURFACE_WITH_KNOTS((2,2),(3,2,3),(0.,0.290280981329602),(0.607879027750091,
0.625170525609407,0.625770422752291),.UNSPECIFIED.)
GEOMETRIC_REPRESENTATION_ITEM()
RATIONAL_B_SPLINE_SURFACE(((0.987469282487682,0.987594391229382,0.990658108926708,
0.990658108926708,0.990658108926708),(0.987469282487682,0.987594391229382,
0.990658108926708,0.990658108926708,0.990658108926708)))
REPRESENTATION_ITEM('')
SURFACE()
);
#4005=(
BOUNDED_SURFACE()
B_SPLINE_SURFACE(1,2,((#162115,#162116,#162117),(#162118,#162119,#162120)),
 .UNSPECIFIED.,.F.,.F.,.F.)
B_SPLINE_SURFACE_WITH_KNOTS((2,2),(3,3),(0.,0.289807040991561),(0.107982157956012,
0.125273655815329),.UNSPECIFIED.)
GEOMETRIC_REPRESENTATION_ITEM()
RATIONAL_B_SPLINE_SURFACE(((0.987470879370255,0.987613514606721,0.990694758798813),
(0.987470879370255,0.987613514606721,0.990694758798813)))
REPRESENTATION_ITEM('')
SURFACE()
);
#4006=(
BOUNDED_SURFACE()
B_SPLINE_SURFACE(1,2,((#162138,#162139,#162140,#162141,#162142),(#162143,
#162144,#162145,#162146,#162147)),.UNSPECIFIED.,.F.,.F.,.F.)
B_SPLINE_SURFACE_WITH_KNOTS((2,2),(3,2,3),(0.,0.290280981329769),(0.607879027750091,
0.625170525609408,0.625770422752459),.UNSPECIFIED.)
GEOMETRIC_REPRESENTATION_ITEM()
RATIONAL_B_SPLINE_SURFACE(((0.987469282487682,0.987594391229382,0.990658108926708,
0.990658108926708,0.990658108926708),(0.987469282487682,0.987594391229382,
0.990658108926708,0.990658108926708,0.990658108926708)))
REPRESENTATION_ITEM('')
SURFACE()
);
#4007=(
BOUNDED_SURFACE()
B_SPLINE_SURFACE(1,2,((#162154,#162155,#162156),(#162157,#162158,#162159)),
 .UNSPECIFIED.,.F.,.F.,.F.)
B_SPLINE_SURFACE_WITH_KNOTS((2,2),(3,3),(0.,0.289807040991696),(0.107982157956012,
0.125273655815329),.UNSPECIFIED.)
GEOMETRIC_REPRESENTATION_ITEM()
RATIONAL_B_SPLINE_SURFACE(((0.987470879370256,0.987613514606721,0.990694758798813),
(0.987470879370255,0.987613514606721,0.990694758798813)))
REPRESENTATION_ITEM('')
SURFACE()
);
#4008=(
BOUNDED_SURFACE()
B_SPLINE_SURFACE(1,2,((#162177,#162178,#162179,#162180,#162181),(#162182,
#162183,#162184,#162185,#162186)),.UNSPECIFIED.,.F.,.F.,.F.)
B_SPLINE_SURFACE_WITH_KNOTS((2,2),(3,2,3),(0.,0.290280981331014),(0.607879027750091,
0.625170525609407,0.625770422753705),.UNSPECIFIED.)
GEOMETRIC_REPRESENTATION_ITEM()
RATIONAL_B_SPLINE_SURFACE(((0.987469282487682,0.987594391229382,0.990658108926708,
0.990658108926708,0.990658108926708),(0.987469282487682,0.987594391229382,
0.990658108926708,0.990658108926708,0.990658108926708)))
REPRESENTATION_ITEM('')
SURFACE()
);
#4009=(
BOUNDED_SURFACE()
B_SPLINE_SURFACE(1,2,((#162193,#162194,#162195),(#162196,#162197,#162198)),
 .UNSPECIFIED.,.F.,.F.,.F.)
B_SPLINE_SURFACE_WITH_KNOTS((2,2),(3,3),(0.,0.289807040991704),(0.107982157956012,
0.125273655815329),.UNSPECIFIED.)
GEOMETRIC_REPRESENTATION_ITEM()
RATIONAL_B_SPLINE_SURFACE(((0.987470879370256,0.987613514606721,0.990694758798813),
(0.987470879370256,0.987613514606721,0.990694758798813)))
REPRESENTATION_ITEM('')
SURFACE()
);
#4010=(
BOUNDED_SURFACE()
B_SPLINE_SURFACE(1,2,((#162216,#162217,#162218,#162219,#162220),(#162221,
#162222,#162223,#162224,#162225)),.UNSPECIFIED.,.F.,.F.,.F.)
B_SPLINE_SURFACE_WITH_KNOTS((2,2),(3,2,3),(0.,0.290280981334896),(0.607879027750091,
0.625170525609407,0.625770422757586),.UNSPECIFIED.)
GEOMETRIC_REPRESENTATION_ITEM()
RATIONAL_B_SPLINE_SURFACE(((0.987469282487682,0.987594391229382,0.990658108926708,
0.990658108926708,0.990658108926708),(0.987469282487682,0.987594391229382,
0.990658108926709,0.990658108926709,0.990658108926709)))
REPRESENTATION_ITEM('')
SURFACE()
);
#4011=(
BOUNDED_SURFACE()
B_SPLINE_SURFACE(1,2,((#162232,#162233,#162234),(#162235,#162236,#162237)),
 .UNSPECIFIED.,.F.,.F.,.F.)
B_SPLINE_SURFACE_WITH_KNOTS((2,2),(3,3),(0.,0.289807040991712),(0.107982157956012,
0.125273655815329),.UNSPECIFIED.)
GEOMETRIC_REPRESENTATION_ITEM()
RATIONAL_B_SPLINE_SURFACE(((0.987470879370256,0.987613514606721,0.990694758798813),
(0.987470879370256,0.987613514606721,0.990694758798813)))
REPRESENTATION_ITEM('')
SURFACE()
);
#4012=(
BOUNDED_SURFACE()
B_SPLINE_SURFACE(1,2,((#162255,#162256,#162257,#162258,#162259),(#162260,
#162261,#162262,#162263,#162264)),.UNSPECIFIED.,.F.,.F.,.F.)
B_SPLINE_SURFACE_WITH_KNOTS((2,2),(3,2,3),(0.,0.290280981346236),(0.607879027750091,
0.625170525609407,0.62577042276893),.UNSPECIFIED.)
GEOMETRIC_REPRESENTATION_ITEM()
RATIONAL_B_SPLINE_SURFACE(((0.987469282487682,0.987594391229382,0.990658108926708,
0.990658108926708,0.990658108926708),(0.987469282487682,0.987594391229382,
0.990658108926708,0.990658108926708,0.990658108926708)))
REPRESENTATION_ITEM('')
SURFACE()
);
#4013=(
BOUNDED_SURFACE()
B_SPLINE_SURFACE(1,2,((#162271,#162272,#162273),(#162274,#162275,#162276)),
 .UNSPECIFIED.,.F.,.F.,.F.)
B_SPLINE_SURFACE_WITH_KNOTS((2,2),(3,3),(0.,0.289807040993084),(0.107982157956012,
0.125273655815329),.UNSPECIFIED.)
GEOMETRIC_REPRESENTATION_ITEM()
RATIONAL_B_SPLINE_SURFACE(((0.987470879370255,0.987613514606721,0.990694758798813),
(0.987470879370255,0.987613514606721,0.990694758798813)))
REPRESENTATION_ITEM('')
SURFACE()
);
#4014=(
BOUNDED_SURFACE()
B_SPLINE_SURFACE(1,2,((#162294,#162295,#162296,#162297,#162298),(#162299,
#162300,#162301,#162302,#162303)),.UNSPECIFIED.,.F.,.F.,.F.)
B_SPLINE_SURFACE_WITH_KNOTS((2,2),(3,2,3),(0.,0.290280981314508),(0.607879027750091,
0.625170525609407,0.625770422736998),.UNSPECIFIED.)
GEOMETRIC_REPRESENTATION_ITEM()
RATIONAL_B_SPLINE_SURFACE(((0.987469282487682,0.987594391229382,0.990658108926708,
0.990658108926708,0.990658108926708),(0.987469282487682,0.987594391229382,
0.990658108926708,0.990658108926708,0.990658108926708)))
REPRESENTATION_ITEM('')
SURFACE()
);
#4015=(
BOUNDED_SURFACE()
B_SPLINE_SURFACE(1,2,((#162310,#162311,#162312),(#162313,#162314,#162315)),
 .UNSPECIFIED.,.F.,.F.,.F.)
B_SPLINE_SURFACE_WITH_KNOTS((2,2),(3,3),(0.,0.289807040991928),(0.107982157956012,
0.125273655815329),.UNSPECIFIED.)
GEOMETRIC_REPRESENTATION_ITEM()
RATIONAL_B_SPLINE_SURFACE(((0.987470879370256,0.987613514606721,0.990694758798813),
(0.987470879370256,0.987613514606721,0.990694758798813)))
REPRESENTATION_ITEM('')
SURFACE()
);
#4016=(
BOUNDED_SURFACE()
B_SPLINE_SURFACE(1,2,((#162333,#162334,#162335,#162336,#162337),(#162338,
#162339,#162340,#162341,#162342)),.UNSPECIFIED.,.F.,.F.,.F.)
B_SPLINE_SURFACE_WITH_KNOTS((2,2),(3,2,3),(0.,0.290280981329288),(0.607879027750091,
0.625170525609407,0.625770422751973),.UNSPECIFIED.)
GEOMETRIC_REPRESENTATION_ITEM()
RATIONAL_B_SPLINE_SURFACE(((0.987469282487682,0.987594391229382,0.990658108926708,
0.990658108926708,0.990658108926708),(0.987469282487682,0.987594391229382,
0.990658108926709,0.990658108926709,0.990658108926709)))
REPRESENTATION_ITEM('')
SURFACE()
);
#4017=(
BOUNDED_SURFACE()
B_SPLINE_SURFACE(1,2,((#162349,#162350,#162351),(#162352,#162353,#162354)),
 .UNSPECIFIED.,.F.,.F.,.F.)
B_SPLINE_SURFACE_WITH_KNOTS((2,2),(3,3),(0.,0.289807040991557),(0.107982157956012,
0.125273655815329),.UNSPECIFIED.)
GEOMETRIC_REPRESENTATION_ITEM()
RATIONAL_B_SPLINE_SURFACE(((0.987470879370255,0.987613514606721,0.990694758798813),
(0.987470879370255,0.987613514606721,0.990694758798813)))
REPRESENTATION_ITEM('')
SURFACE()
);
#4018=(
BOUNDED_SURFACE()
B_SPLINE_SURFACE(1,2,((#162372,#162373,#162374,#162375,#162376),(#162377,
#162378,#162379,#162380,#162381)),.UNSPECIFIED.,.F.,.F.,.F.)
B_SPLINE_SURFACE_WITH_KNOTS((2,2),(3,2,3),(0.,0.290280981324863),(0.607879027750091,
0.625170525609408,0.625770422747553),.UNSPECIFIED.)
GEOMETRIC_REPRESENTATION_ITEM()
RATIONAL_B_SPLINE_SURFACE(((0.987469282487682,0.987594391229382,0.990658108926708,
0.990658108926708,0.990658108926708),(0.987469282487682,0.987594391229382,
0.990658108926708,0.990658108926708,0.990658108926708)))
REPRESENTATION_ITEM('')
SURFACE()
);
#4019=(
BOUNDED_SURFACE()
B_SPLINE_SURFACE(1,2,((#162388,#162389,#162390),(#162391,#162392,#162393)),
 .UNSPECIFIED.,.F.,.F.,.F.)
B_SPLINE_SURFACE_WITH_KNOTS((2,2),(3,3),(0.,0.289807040991562),(0.107982157956012,
0.125273655815329),.UNSPECIFIED.)
GEOMETRIC_REPRESENTATION_ITEM()
RATIONAL_B_SPLINE_SURFACE(((0.987470879370256,0.987613514606721,0.990694758798813),
(0.987470879370255,0.987613514606721,0.990694758798813)))
REPRESENTATION_ITEM('')
SURFACE()
);
#4020=(
BOUNDED_SURFACE()
B_SPLINE_SURFACE(1,2,((#162411,#162412,#162413,#162414,#162415),(#162416,
#162417,#162418,#162419,#162420)),.UNSPECIFIED.,.F.,.F.,.F.)
B_SPLINE_SURFACE_WITH_KNOTS((2,2),(3,2,3),(0.,0.290280981331528),(0.607879027750091,
0.625170525609407,0.625770422754222),.UNSPECIFIED.)
GEOMETRIC_REPRESENTATION_ITEM()
RATIONAL_B_SPLINE_SURFACE(((0.987469282487682,0.987594391229382,0.990658108926708,
0.990658108926708,0.990658108926708),(0.987469282487682,0.987594391229382,
0.990658108926709,0.990658108926709,0.990658108926709)))
REPRESENTATION_ITEM('')
SURFACE()
);
#4021=(
BOUNDED_SURFACE()
B_SPLINE_SURFACE(1,2,((#162439,#162440,#162441),(#162442,#162443,#162444)),
 .UNSPECIFIED.,.F.,.F.,.F.)
B_SPLINE_SURFACE_WITH_KNOTS((2,2),(3,3),(0.,0.289807040991564),(0.107982157956012,
0.125273655815329),.UNSPECIFIED.)
GEOMETRIC_REPRESENTATION_ITEM()
RATIONAL_B_SPLINE_SURFACE(((0.987470879370255,0.987613514606721,0.990694758798813),
(0.987470879370255,0.987613514606721,0.990694758798813)))
REPRESENTATION_ITEM('')
SURFACE()
);
#4022=(
BOUNDED_SURFACE()
B_SPLINE_SURFACE(1,2,((#162447,#162448,#162449,#162450,#162451),(#162452,
#162453,#162454,#162455,#162456)),.UNSPECIFIED.,.F.,.F.,.F.)
B_SPLINE_SURFACE_WITH_KNOTS((2,2),(3,2,3),(0.71005925781061,1.),(0.0908085233856358,
0.107982157956013,0.108241816694656),.UNSPECIFIED.)
GEOMETRIC_REPRESENTATION_ITEM()
RATIONAL_B_SPLINE_SURFACE(((0.990086238235256,0.987329216372183,0.987470879370256,
0.987470879370256,0.987470879370256),(0.990086238235256,0.987329216372183,
0.987470879370256,0.987470879370256,0.987470879370256)))
REPRESENTATION_ITEM('')
SURFACE()
);
#4023=(
BOUNDED_SURFACE()
B_SPLINE_SURFACE(1,2,((#162460,#162461,#162462),(#162463,#162464,#162465)),
 .UNSPECIFIED.,.F.,.F.,.F.)
B_SPLINE_SURFACE_WITH_KNOTS((2,2),(3,3),(0.710192959008442,1.),(0.625170525609407,
0.642682999576235),.UNSPECIFIED.)
GEOMETRIC_REPRESENTATION_ITEM()
RATIONAL_B_SPLINE_SURFACE(((0.990658108926708,0.993760979299921,0.999878046252916),
(0.990658108926708,0.993760979299921,0.999878046252916)))
REPRESENTATION_ITEM('')
SURFACE()
);
#4024=(
BOUNDED_SURFACE()
B_SPLINE_SURFACE(1,2,((#162469,#162470,#162471,#162472,#162473),(#162474,
#162475,#162476,#162477,#162478)),.UNSPECIFIED.,.F.,.F.,.F.)
B_SPLINE_SURFACE_WITH_KNOTS((2,2),(3,2,3),(0.710059257949577,1.),(0.0908085233856358,
0.107982157956012,0.10824181686735),.UNSPECIFIED.)
GEOMETRIC_REPRESENTATION_ITEM()
RATIONAL_B_SPLINE_SURFACE(((0.990086238235256,0.987329216372183,0.987470879370255,
0.987470879370255,0.987470879370255),(0.990086238235256,0.987329216372183,
0.987470879370255,0.987470879370255,0.987470879370255)))
REPRESENTATION_ITEM('')
SURFACE()
);
#4025=(
BOUNDED_SURFACE()
B_SPLINE_SURFACE(1,2,((#162480,#162481,#162482),(#162483,#162484,#162485)),
 .UNSPECIFIED.,.F.,.F.,.F.)
B_SPLINE_SURFACE_WITH_KNOTS((2,2),(3,3),(0.710192959008438,1.),(0.625170525609407,
0.642682999576235),.UNSPECIFIED.)
GEOMETRIC_REPRESENTATION_ITEM()
RATIONAL_B_SPLINE_SURFACE(((0.990658108926708,0.993760979299921,0.999878046252916),
(0.990658108926708,0.993760979299921,0.999878046252916)))
REPRESENTATION_ITEM('')
SURFACE()
);
#4026=(
BOUNDED_SURFACE()
B_SPLINE_SURFACE(1,2,((#162489,#162490,#162491,#162492,#162493),(#162494,
#162495,#162496,#162497,#162498)),.UNSPECIFIED.,.F.,.F.,.F.)
B_SPLINE_SURFACE_WITH_KNOTS((2,2),(3,2,3),(0.710059257875638,1.),(0.0908085233856357,
0.107982157956012,0.108241816941263),.UNSPECIFIED.)
GEOMETRIC_REPRESENTATION_ITEM()
RATIONAL_B_SPLINE_SURFACE(((0.990086238235256,0.987329216372183,0.987470879370255,
0.987470879370255,0.987470879370255),(0.990086238235256,0.987329216372183,
0.987470879370255,0.987470879370255,0.987470879370255)))
REPRESENTATION_ITEM('')
SURFACE()
);
#4027=(
BOUNDED_SURFACE()
B_SPLINE_SURFACE(1,2,((#162500,#162501,#162502),(#162503,#162504,#162505)),
 .UNSPECIFIED.,.F.,.F.,.F.)
B_SPLINE_SURFACE_WITH_KNOTS((2,2),(3,3),(0.710192959008443,1.),(0.625170525609407,
0.642682999576235),.UNSPECIFIED.)
GEOMETRIC_REPRESENTATION_ITEM()
RATIONAL_B_SPLINE_SURFACE(((0.990658108926708,0.993760979299921,0.999878046252916),
(0.990658108926708,0.993760979299921,0.999878046252916)))
REPRESENTATION_ITEM('')
SURFACE()
);
#4028=(
BOUNDED_SURFACE()
B_SPLINE_SURFACE(1,2,((#162509,#162510,#162511,#162512,#162513),(#162514,
#162515,#162516,#162517,#162518)),.UNSPECIFIED.,.F.,.F.,.F.)
B_SPLINE_SURFACE_WITH_KNOTS((2,2),(3,2,3),(0.710059257951385,1.),(0.0908085233856357,
0.107982157956012,0.10824181686549),.UNSPECIFIED.)
GEOMETRIC_REPRESENTATION_ITEM()
RATIONAL_B_SPLINE_SURFACE(((0.990086238235256,0.987329216372183,0.987470879370255,
0.987470879370255,0.987470879370255),(0.990086238235256,0.987329216372183,
0.987470879370255,0.987470879370255,0.987470879370255)))
REPRESENTATION_ITEM('')
SURFACE()
);
#4029=(
BOUNDED_SURFACE()
B_SPLINE_SURFACE(1,2,((#162520,#162521,#162522),(#162523,#162524,#162525)),
 .UNSPECIFIED.,.F.,.F.,.F.)
B_SPLINE_SURFACE_WITH_KNOTS((2,2),(3,3),(0.710192959008438,1.),(0.625170525609407,
0.642682999576235),.UNSPECIFIED.)
GEOMETRIC_REPRESENTATION_ITEM()
RATIONAL_B_SPLINE_SURFACE(((0.990658108926708,0.993760979299921,0.999878046252916),
(0.990658108926708,0.993760979299921,0.999878046252916)))
REPRESENTATION_ITEM('')
SURFACE()
);
#4030=(
BOUNDED_SURFACE()
B_SPLINE_SURFACE(1,2,((#162529,#162530,#162531,#162532,#162533),(#162534,
#162535,#162536,#162537,#162538)),.UNSPECIFIED.,.F.,.F.,.F.)
B_SPLINE_SURFACE_WITH_KNOTS((2,2),(3,2,3),(0.71005925795596,1.),(0.0908085233856358,
0.107982157956011,0.108241816860967),.UNSPECIFIED.)
GEOMETRIC_REPRESENTATION_ITEM()
RATIONAL_B_SPLINE_SURFACE(((0.990086238235256,0.987329216372183,0.987470879370255,
0.987470879370255,0.987470879370255),(0.990086238235256,0.987329216372183,
0.987470879370255,0.987470879370255,0.987470879370255)))
REPRESENTATION_ITEM('')
SURFACE()
);
#4031=(
BOUNDED_SURFACE()
B_SPLINE_SURFACE(1,2,((#162540,#162541,#162542),(#162543,#162544,#162545)),
 .UNSPECIFIED.,.F.,.F.,.F.)
B_SPLINE_SURFACE_WITH_KNOTS((2,2),(3,3),(0.710192959008441,1.),(0.625170525609408,
0.642682999576236),.UNSPECIFIED.)
GEOMETRIC_REPRESENTATION_ITEM()
RATIONAL_B_SPLINE_SURFACE(((0.990658108926709,0.993760979299921,0.999878046252917),
(0.990658108926709,0.993760979299922,0.999878046252917)))
REPRESENTATION_ITEM('')
SURFACE()
);
#4032=(
BOUNDED_SURFACE()
B_SPLINE_SURFACE(1,2,((#162549,#162550,#162551,#162552,#162553),(#162554,
#162555,#162556,#162557,#162558)),.UNSPECIFIED.,.F.,.F.,.F.)
B_SPLINE_SURFACE_WITH_KNOTS((2,2),(3,2,3),(0.710059258013954,1.),(0.0908085233856347,
0.107982157956011,0.10824181680298),.UNSPECIFIED.)
GEOMETRIC_REPRESENTATION_ITEM()
RATIONAL_B_SPLINE_SURFACE(((0.990086238235256,0.987329216372183,0.987470879370256,
0.987470879370256,0.987470879370256),(0.990086238235256,0.987329216372183,
0.987470879370256,0.987470879370256,0.987470879370256)))
REPRESENTATION_ITEM('')
SURFACE()
);
#4033=(
BOUNDED_SURFACE()
B_SPLINE_SURFACE(1,2,((#162560,#162561,#162562),(#162563,#162564,#162565)),
 .UNSPECIFIED.,.F.,.F.,.F.)
B_SPLINE_SURFACE_WITH_KNOTS((2,2),(3,3),(0.710192959008439,1.),(0.625170525609408,
0.642682999576236),.UNSPECIFIED.)
GEOMETRIC_REPRESENTATION_ITEM()
RATIONAL_B_SPLINE_SURFACE(((0.990658108926709,0.993760979299921,0.999878046252917),
(0.990658108926709,0.993760979299921,0.999878046252917)))
REPRESENTATION_ITEM('')
SURFACE()
);
#4034=(
BOUNDED_SURFACE()
B_SPLINE_SURFACE(1,2,((#162569,#162570,#162571,#162572,#162573),(#162574,
#162575,#162576,#162577,#162578)),.UNSPECIFIED.,.F.,.F.,.F.)
B_SPLINE_SURFACE_WITH_KNOTS((2,2),(3,2,3),(0.710059257951645,1.),(0.0908085233856347,
0.107982157956011,0.108241816865274),.UNSPECIFIED.)
GEOMETRIC_REPRESENTATION_ITEM()
RATIONAL_B_SPLINE_SURFACE(((0.990086238235256,0.987329216372183,0.987470879370255,
0.987470879370255,0.987470879370255),(0.990086238235256,0.987329216372183,
0.987470879370255,0.987470879370255,0.987470879370255)))
REPRESENTATION_ITEM('')
SURFACE()
);
#4035=(
BOUNDED_SURFACE()
B_SPLINE_SURFACE(1,2,((#162580,#162581,#162582),(#162583,#162584,#162585)),
 .UNSPECIFIED.,.F.,.F.,.F.)
B_SPLINE_SURFACE_WITH_KNOTS((2,2),(3,3),(0.710192959008438,1.),(0.625170525609408,
0.642682999576236),.UNSPECIFIED.)
GEOMETRIC_REPRESENTATION_ITEM()
RATIONAL_B_SPLINE_SURFACE(((0.990658108926709,0.993760979299921,0.999878046252917),
(0.990658108926709,0.993760979299921,0.999878046252917)))
REPRESENTATION_ITEM('')
SURFACE()
);
#4036=(
BOUNDED_SURFACE()
B_SPLINE_SURFACE(1,2,((#162589,#162590,#162591,#162592,#162593),(#162594,
#162595,#162596,#162597,#162598)),.UNSPECIFIED.,.F.,.F.,.F.)
B_SPLINE_SURFACE_WITH_KNOTS((2,2),(3,2,3),(0.710059257776109,1.),(0.0908085233856348,
0.107982157956011,0.108241816729418),.UNSPECIFIED.)
GEOMETRIC_REPRESENTATION_ITEM()
RATIONAL_B_SPLINE_SURFACE(((0.990086238235256,0.987329216372183,0.987470879370255,
0.987470879370255,0.987470879370255),(0.990086238235256,0.987329216372183,
0.987470879370255,0.987470879370255,0.987470879370255)))
REPRESENTATION_ITEM('')
SURFACE()
);
#4037=(
BOUNDED_SURFACE()
B_SPLINE_SURFACE(1,2,((#162600,#162601,#162602),(#162603,#162604,#162605)),
 .UNSPECIFIED.,.F.,.F.,.F.)
B_SPLINE_SURFACE_WITH_KNOTS((2,2),(3,3),(0.710192959008441,1.),(0.625170525609408,
0.642682999576236),.UNSPECIFIED.)
GEOMETRIC_REPRESENTATION_ITEM()
RATIONAL_B_SPLINE_SURFACE(((0.990658108926709,0.993760979299921,0.999878046252917),
(0.990658108926709,0.993760979299921,0.999878046252917)))
REPRESENTATION_ITEM('')
SURFACE()
);
#4038=(
BOUNDED_SURFACE()
B_SPLINE_SURFACE(1,2,((#162609,#162610,#162611,#162612,#162613),(#162614,
#162615,#162616,#162617,#162618)),.UNSPECIFIED.,.F.,.F.,.F.)
B_SPLINE_SURFACE_WITH_KNOTS((2,2),(3,2,3),(0.710059257948746,1.),(0.0908085233856347,
0.107982157956011,0.108241816868152),.UNSPECIFIED.)
GEOMETRIC_REPRESENTATION_ITEM()
RATIONAL_B_SPLINE_SURFACE(((0.990086238235257,0.987329216372183,0.987470879370256,
0.987470879370256,0.987470879370256),(0.990086238235257,0.987329216372183,
0.987470879370256,0.987470879370256,0.987470879370256)))
REPRESENTATION_ITEM('')
SURFACE()
);
#4039=(
BOUNDED_SURFACE()
B_SPLINE_SURFACE(1,2,((#162620,#162621,#162622),(#162623,#162624,#162625)),
 .UNSPECIFIED.,.F.,.F.,.F.)
B_SPLINE_SURFACE_WITH_KNOTS((2,2),(3,3),(0.71019295900844,1.),(0.625170525609408,
0.642682999576236),.UNSPECIFIED.)
GEOMETRIC_REPRESENTATION_ITEM()
RATIONAL_B_SPLINE_SURFACE(((0.990658108926709,0.993760979299921,0.999878046252917),
(0.990658108926709,0.993760979299921,0.999878046252917)))
REPRESENTATION_ITEM('')
SURFACE()
);
#4040=(
BOUNDED_SURFACE()
B_SPLINE_SURFACE(1,2,((#162629,#162630,#162631,#162632,#162633),(#162634,
#162635,#162636,#162637,#162638)),.UNSPECIFIED.,.F.,.F.,.F.)
B_SPLINE_SURFACE_WITH_KNOTS((2,2),(3,2,3),(0.710059257948785,1.),(0.0908085233856347,
0.107982157956011,0.108241816868058),.UNSPECIFIED.)
GEOMETRIC_REPRESENTATION_ITEM()
RATIONAL_B_SPLINE_SURFACE(((0.990086238235256,0.987329216372183,0.987470879370255,
0.987470879370255,0.987470879370255),(0.990086238235256,0.987329216372183,
0.987470879370255,0.987470879370255,0.987470879370255)))
REPRESENTATION_ITEM('')
SURFACE()
);
#4041=(
BOUNDED_SURFACE()
B_SPLINE_SURFACE(1,2,((#162640,#162641,#162642),(#162643,#162644,#162645)),
 .UNSPECIFIED.,.F.,.F.,.F.)
B_SPLINE_SURFACE_WITH_KNOTS((2,2),(3,3),(0.710192959008442,1.),(0.625170525609408,
0.642682999576236),.UNSPECIFIED.)
GEOMETRIC_REPRESENTATION_ITEM()
RATIONAL_B_SPLINE_SURFACE(((0.990658108926709,0.993760979299921,0.999878046252917),
(0.990658108926709,0.993760979299921,0.999878046252917)))
REPRESENTATION_ITEM('')
SURFACE()
);
#4042=(
BOUNDED_SURFACE()
B_SPLINE_SURFACE(1,2,((#162649,#162650,#162651,#162652,#162653),(#162654,
#162655,#162656,#162657,#162658)),.UNSPECIFIED.,.F.,.F.,.F.)
B_SPLINE_SURFACE_WITH_KNOTS((2,2),(3,2,3),(0.710059257952301,1.),(0.0908085233856347,
0.107982157956011,0.108241816864594),.UNSPECIFIED.)
GEOMETRIC_REPRESENTATION_ITEM()
RATIONAL_B_SPLINE_SURFACE(((0.990086238235257,0.987329216372183,0.987470879370255,
0.987470879370255,0.987470879370255),(0.990086238235257,0.987329216372183,
0.987470879370255,0.987470879370255,0.987470879370255)))
REPRESENTATION_ITEM('')
SURFACE()
);
#4043=(
BOUNDED_SURFACE()
B_SPLINE_SURFACE(1,2,((#162660,#162661,#162662),(#162663,#162664,#162665)),
 .UNSPECIFIED.,.F.,.F.,.F.)
B_SPLINE_SURFACE_WITH_KNOTS((2,2),(3,3),(0.710192959008441,1.),(0.625170525609408,
0.642682999576236),.UNSPECIFIED.)
GEOMETRIC_REPRESENTATION_ITEM()
RATIONAL_B_SPLINE_SURFACE(((0.990658108926709,0.993760979299921,0.999878046252917),
(0.990658108926709,0.993760979299921,0.999878046252917)))
REPRESENTATION_ITEM('')
SURFACE()
);
#4044=(
BOUNDED_SURFACE()
B_SPLINE_SURFACE(1,2,((#162669,#162670,#162671,#162672,#162673),(#162674,
#162675,#162676,#162677,#162678)),.UNSPECIFIED.,.F.,.F.,.F.)
B_SPLINE_SURFACE_WITH_KNOTS((2,2),(3,2,3),(0.710059257867479,1.),(0.0908085233856346,
0.107982157956011,0.108241816949409),.UNSPECIFIED.)
GEOMETRIC_REPRESENTATION_ITEM()
RATIONAL_B_SPLINE_SURFACE(((0.990086238235256,0.987329216372183,0.987470879370255,
0.987470879370255,0.987470879370255),(0.990086238235256,0.987329216372183,
0.987470879370255,0.987470879370255,0.987470879370255)))
REPRESENTATION_ITEM('')
SURFACE()
);
#4045=(
BOUNDED_SURFACE()
B_SPLINE_SURFACE(1,2,((#162680,#162681,#162682),(#162683,#162684,#162685)),
 .UNSPECIFIED.,.F.,.F.,.F.)
B_SPLINE_SURFACE_WITH_KNOTS((2,2),(3,3),(0.710192959008446,1.),(0.625170525609408,
0.642682999576237),.UNSPECIFIED.)
GEOMETRIC_REPRESENTATION_ITEM()
RATIONAL_B_SPLINE_SURFACE(((0.990658108926709,0.993760979299922,0.999878046252917),
(0.990658108926709,0.993760979299922,0.999878046252917)))
REPRESENTATION_ITEM('')
SURFACE()
);
#4046=(
BOUNDED_SURFACE()
B_SPLINE_SURFACE(1,2,((#162689,#162690,#162691,#162692,#162693),(#162694,
#162695,#162696,#162697,#162698)),.UNSPECIFIED.,.F.,.F.,.F.)
B_SPLINE_SURFACE_WITH_KNOTS((2,2),(3,2,3),(0.710059257964262,1.),(0.0908085233856348,
0.107982157956011,0.108241816852688),.UNSPECIFIED.)
GEOMETRIC_REPRESENTATION_ITEM()
RATIONAL_B_SPLINE_SURFACE(((0.990086238235256,0.987329216372183,0.987470879370255,
0.987470879370255,0.987470879370255),(0.990086238235256,0.987329216372183,
0.987470879370255,0.987470879370255,0.987470879370255)))
REPRESENTATION_ITEM('')
SURFACE()
);
#4047=(
BOUNDED_SURFACE()
B_SPLINE_SURFACE(1,2,((#162700,#162701,#162702),(#162703,#162704,#162705)),
 .UNSPECIFIED.,.F.,.F.,.F.)
B_SPLINE_SURFACE_WITH_KNOTS((2,2),(3,3),(0.710192959008443,1.),(0.625170525609408,
0.642682999576236),.UNSPECIFIED.)
GEOMETRIC_REPRESENTATION_ITEM()
RATIONAL_B_SPLINE_SURFACE(((0.990658108926709,0.993760979299921,0.999878046252917),
(0.990658108926709,0.993760979299921,0.999878046252917)))
REPRESENTATION_ITEM('')
SURFACE()
);
#4048=(
BOUNDED_SURFACE()
B_SPLINE_SURFACE(1,2,((#162709,#162710,#162711,#162712,#162713),(#162714,
#162715,#162716,#162717,#162718)),.UNSPECIFIED.,.F.,.F.,.F.)
B_SPLINE_SURFACE_WITH_KNOTS((2,2),(3,2,3),(0.710059257941329,1.),(0.0908085233856347,
0.107982157956011,0.108241816875574),.UNSPECIFIED.)
GEOMETRIC_REPRESENTATION_ITEM()
RATIONAL_B_SPLINE_SURFACE(((0.990086238235256,0.987329216372183,0.987470879370256,
0.987470879370256,0.987470879370256),(0.990086238235256,0.987329216372183,
0.987470879370256,0.987470879370256,0.987470879370256)))
REPRESENTATION_ITEM('')
SURFACE()
);
#4049=(
BOUNDED_SURFACE()
B_SPLINE_SURFACE(1,2,((#162720,#162721,#162722),(#162723,#162724,#162725)),
 .UNSPECIFIED.,.F.,.F.,.F.)
B_SPLINE_SURFACE_WITH_KNOTS((2,2),(3,3),(0.710192959008441,1.),(0.625170525609408,
0.642682999576236),.UNSPECIFIED.)
GEOMETRIC_REPRESENTATION_ITEM()
RATIONAL_B_SPLINE_SURFACE(((0.990658108926709,0.993760979299921,0.999878046252917),
(0.990658108926709,0.993760979299921,0.999878046252917)))
REPRESENTATION_ITEM('')
SURFACE()
);
#4050=(
BOUNDED_SURFACE()
B_SPLINE_SURFACE(1,2,((#162729,#162730,#162731,#162732,#162733),(#162734,
#162735,#162736,#162737,#162738)),.UNSPECIFIED.,.F.,.F.,.F.)
B_SPLINE_SURFACE_WITH_KNOTS((2,2),(3,2,3),(0.710059257942299,1.),(0.0908085233856346,
0.107982157956011,0.108241816874653),.UNSPECIFIED.)
GEOMETRIC_REPRESENTATION_ITEM()
RATIONAL_B_SPLINE_SURFACE(((0.990086238235257,0.987329216372183,0.987470879370256,
0.987470879370256,0.987470879370256),(0.990086238235257,0.987329216372183,
0.987470879370256,0.987470879370256,0.987470879370256)))
REPRESENTATION_ITEM('')
SURFACE()
);
#4051=(
BOUNDED_SURFACE()
B_SPLINE_SURFACE(1,2,((#162740,#162741,#162742),(#162743,#162744,#162745)),
 .UNSPECIFIED.,.F.,.F.,.F.)
B_SPLINE_SURFACE_WITH_KNOTS((2,2),(3,3),(0.710192959008435,1.),(0.625170525609408,
0.642682999576236),.UNSPECIFIED.)
GEOMETRIC_REPRESENTATION_ITEM()
RATIONAL_B_SPLINE_SURFACE(((0.990658108926709,0.993760979299922,0.999878046252917),
(0.990658108926709,0.993760979299922,0.999878046252917)))
REPRESENTATION_ITEM('')
SURFACE()
);
#4052=(
BOUNDED_SURFACE()
B_SPLINE_SURFACE(1,2,((#162749,#162750,#162751,#162752,#162753),(#162754,
#162755,#162756,#162757,#162758)),.UNSPECIFIED.,.F.,.F.,.F.)
B_SPLINE_SURFACE_WITH_KNOTS((2,2),(3,2,3),(0.710059258506232,1.),(0.0908085233856347,
0.107982157956011,0.108241816310694),.UNSPECIFIED.)
GEOMETRIC_REPRESENTATION_ITEM()
RATIONAL_B_SPLINE_SURFACE(((0.990086238235256,0.987329216372183,0.987470879370255,
0.987470879370255,0.987470879370255),(0.990086238235256,0.987329216372183,
0.987470879370255,0.987470879370255,0.987470879370255)))
REPRESENTATION_ITEM('')
SURFACE()
);
#4053=(
BOUNDED_SURFACE()
B_SPLINE_SURFACE(1,2,((#162760,#162761,#162762),(#162763,#162764,#162765)),
 .UNSPECIFIED.,.F.,.F.,.F.)
B_SPLINE_SURFACE_WITH_KNOTS((2,2),(3,3),(0.71019295900844,1.),(0.625170525609408,
0.642682999576236),.UNSPECIFIED.)
GEOMETRIC_REPRESENTATION_ITEM()
RATIONAL_B_SPLINE_SURFACE(((0.990658108926709,0.993760979299922,0.999878046252917),
(0.990658108926709,0.993760979299922,0.999878046252917)))
REPRESENTATION_ITEM('')
SURFACE()
);
#4054=(
BOUNDED_SURFACE()
B_SPLINE_SURFACE(1,2,((#162769,#162770,#162771,#162772,#162773),(#162774,
#162775,#162776,#162777,#162778)),.UNSPECIFIED.,.F.,.F.,.F.)
B_SPLINE_SURFACE_WITH_KNOTS((2,2),(3,2,3),(0.71005925774851,1.),(0.0908085233856347,
0.107982157956011,0.108241817068402),.UNSPECIFIED.)
GEOMETRIC_REPRESENTATION_ITEM()
RATIONAL_B_SPLINE_SURFACE(((0.990086238235256,0.987329216372183,0.987470879370255,
0.987470879370255,0.987470879370255),(0.990086238235256,0.987329216372183,
0.987470879370255,0.987470879370255,0.987470879370255)))
REPRESENTATION_ITEM('')
SURFACE()
);
#4055=(
BOUNDED_SURFACE()
B_SPLINE_SURFACE(1,2,((#162780,#162781,#162782),(#162783,#162784,#162785)),
 .UNSPECIFIED.,.F.,.F.,.F.)
B_SPLINE_SURFACE_WITH_KNOTS((2,2),(3,3),(0.710192959008443,1.),(0.625170525609409,
0.642682999576236),.UNSPECIFIED.)
GEOMETRIC_REPRESENTATION_ITEM()
RATIONAL_B_SPLINE_SURFACE(((0.990658108926709,0.993760979299921,0.999878046252917),
(0.990658108926709,0.993760979299921,0.999878046252917)))
REPRESENTATION_ITEM('')
SURFACE()
);
#4056=(
BOUNDED_SURFACE()
B_SPLINE_SURFACE(1,2,((#162789,#162790,#162791,#162792,#162793),(#162794,
#162795,#162796,#162797,#162798)),.UNSPECIFIED.,.F.,.F.,.F.)
B_SPLINE_SURFACE_WITH_KNOTS((2,2),(3,2,3),(0.710059257944843,1.),(0.0908085233856348,
0.107982157956011,0.108241816872063),.UNSPECIFIED.)
GEOMETRIC_REPRESENTATION_ITEM()
RATIONAL_B_SPLINE_SURFACE(((0.990086238235256,0.987329216372183,0.987470879370255,
0.987470879370255,0.987470879370255),(0.990086238235256,0.987329216372183,
0.987470879370255,0.987470879370255,0.987470879370255)))
REPRESENTATION_ITEM('')
SURFACE()
);
#4057=(
BOUNDED_SURFACE()
B_SPLINE_SURFACE(1,2,((#162800,#162801,#162802),(#162803,#162804,#162805)),
 .UNSPECIFIED.,.F.,.F.,.F.)
B_SPLINE_SURFACE_WITH_KNOTS((2,2),(3,3),(0.710192959008253,1.),(0.625170525609404,
0.642682999576235),.UNSPECIFIED.)
GEOMETRIC_REPRESENTATION_ITEM()
RATIONAL_B_SPLINE_SURFACE(((0.990658108926707,0.99376097929992,0.999878046252916),
(0.990658108926707,0.99376097929992,0.999878046252916)))
REPRESENTATION_ITEM('')
SURFACE()
);
#4058=(
BOUNDED_SURFACE()
B_SPLINE_SURFACE(1,2,((#162809,#162810,#162811,#162812,#162813),(#162814,
#162815,#162816,#162817,#162818)),.UNSPECIFIED.,.F.,.F.,.F.)
B_SPLINE_SURFACE_WITH_KNOTS((2,2),(3,2,3),(0.710059257864338,1.),(0.0908085233856356,
0.107982157956012,0.108241816952354),.UNSPECIFIED.)
GEOMETRIC_REPRESENTATION_ITEM()
RATIONAL_B_SPLINE_SURFACE(((0.990086238235256,0.987329216372183,0.987470879370256,
0.987470879370256,0.987470879370256),(0.990086238235256,0.987329216372183,
0.987470879370256,0.987470879370256,0.987470879370256)))
REPRESENTATION_ITEM('')
SURFACE()
);
#4059=(
BOUNDED_SURFACE()
B_SPLINE_SURFACE(1,2,((#162820,#162821,#162822),(#162823,#162824,#162825)),
 .UNSPECIFIED.,.F.,.F.,.F.)
B_SPLINE_SURFACE_WITH_KNOTS((2,2),(3,3),(0.710192959008401,1.),(0.625170525609407,
0.642682999576235),.UNSPECIFIED.)
GEOMETRIC_REPRESENTATION_ITEM()
RATIONAL_B_SPLINE_SURFACE(((0.990658108926708,0.993760979299921,0.999878046252916),
(0.990658108926708,0.993760979299921,0.999878046252916)))
REPRESENTATION_ITEM('')
SURFACE()
);
#4060=(
BOUNDED_SURFACE()
B_SPLINE_SURFACE(1,2,((#162829,#162830,#162831,#162832,#162833),(#162834,
#162835,#162836,#162837,#162838)),.UNSPECIFIED.,.F.,.F.,.F.)
B_SPLINE_SURFACE_WITH_KNOTS((2,2),(3,2,3),(0.710059257951225,1.),(0.0908085233856358,
0.107982157956012,0.108241816865715),.UNSPECIFIED.)
GEOMETRIC_REPRESENTATION_ITEM()
RATIONAL_B_SPLINE_SURFACE(((0.990086238235256,0.987329216372183,0.987470879370255,
0.987470879370255,0.987470879370255),(0.990086238235256,0.987329216372183,
0.987470879370255,0.987470879370255,0.987470879370255)))
REPRESENTATION_ITEM('')
SURFACE()
);
#4061=(
BOUNDED_SURFACE()
B_SPLINE_SURFACE(1,2,((#162840,#162841,#162842),(#162843,#162844,#162845)),
 .UNSPECIFIED.,.F.,.F.,.F.)
B_SPLINE_SURFACE_WITH_KNOTS((2,2),(3,3),(0.71019295900844,1.),(0.625170525609407,
0.642682999576235),.UNSPECIFIED.)
GEOMETRIC_REPRESENTATION_ITEM()
RATIONAL_B_SPLINE_SURFACE(((0.990658108926708,0.993760979299921,0.999878046252916),
(0.990658108926708,0.993760979299921,0.999878046252916)))
REPRESENTATION_ITEM('')
SURFACE()
);
#4062=(
BOUNDED_SURFACE()
B_SPLINE_SURFACE(1,2,((#162849,#162850,#162851,#162852,#162853),(#162854,
#162855,#162856,#162857,#162858)),.UNSPECIFIED.,.F.,.F.,.F.)
B_SPLINE_SURFACE_WITH_KNOTS((2,2),(3,2,3),(0.710059258002317,1.),(0.0908085233856358,
0.107982157956012,0.108241816814637),.UNSPECIFIED.)
GEOMETRIC_REPRESENTATION_ITEM()
RATIONAL_B_SPLINE_SURFACE(((0.990086238235256,0.987329216372183,0.987470879370256,
0.987470879370256,0.987470879370256),(0.990086238235256,0.987329216372183,
0.987470879370256,0.987470879370256,0.987470879370256)))
REPRESENTATION_ITEM('')
SURFACE()
);
#4063=(
BOUNDED_SURFACE()
B_SPLINE_SURFACE(1,2,((#162860,#162861,#162862),(#162863,#162864,#162865)),
 .UNSPECIFIED.,.F.,.F.,.F.)
B_SPLINE_SURFACE_WITH_KNOTS((2,2),(3,3),(0.71019295900844,1.),(0.625170525609407,
0.642682999576235),.UNSPECIFIED.)
GEOMETRIC_REPRESENTATION_ITEM()
RATIONAL_B_SPLINE_SURFACE(((0.990658108926708,0.993760979299921,0.999878046252916),
(0.990658108926708,0.993760979299921,0.999878046252916)))
REPRESENTATION_ITEM('')
SURFACE()
);
#4064=(
BOUNDED_SURFACE()
B_SPLINE_SURFACE(1,2,((#162869,#162870,#162871,#162872,#162873),(#162874,
#162875,#162876,#162877,#162878)),.UNSPECIFIED.,.F.,.F.,.F.)
B_SPLINE_SURFACE_WITH_KNOTS((2,2),(3,2,3),(0.710059257948496,1.),(0.0908085233856358,
0.107982157956012,0.108241816868451),.UNSPECIFIED.)
GEOMETRIC_REPRESENTATION_ITEM()
RATIONAL_B_SPLINE_SURFACE(((0.990086238235256,0.987329216372183,0.987470879370256,
0.987470879370256,0.987470879370256),(0.990086238235256,0.987329216372183,
0.987470879370256,0.987470879370256,0.987470879370256)))
REPRESENTATION_ITEM('')
SURFACE()
);
#4065=(
BOUNDED_SURFACE()
B_SPLINE_SURFACE(1,2,((#162880,#162881,#162882),(#162883,#162884,#162885)),
 .UNSPECIFIED.,.F.,.F.,.F.)
B_SPLINE_SURFACE_WITH_KNOTS((2,2),(3,3),(0.7101929590083,1.),(0.625170525609407,
0.642682999576235),.UNSPECIFIED.)
GEOMETRIC_REPRESENTATION_ITEM()
RATIONAL_B_SPLINE_SURFACE(((0.990658108926708,0.993760979299921,0.999878046252916),
(0.990658108926708,0.993760979299921,0.999878046252916)))
REPRESENTATION_ITEM('')
SURFACE()
);
#4066=(
BOUNDED_SURFACE()
B_SPLINE_SURFACE(1,2,((#162889,#162890,#162891,#162892,#162893),(#162894,
#162895,#162896,#162897,#162898)),.UNSPECIFIED.,.F.,.F.,.F.)
B_SPLINE_SURFACE_WITH_KNOTS((2,2),(3,2,3),(0.710059258485914,1.),(0.0908085233856358,
0.107982157956012,0.108241816330897),.UNSPECIFIED.)
GEOMETRIC_REPRESENTATION_ITEM()
RATIONAL_B_SPLINE_SURFACE(((0.990086238235256,0.987329216372183,0.987470879370256,
0.987470879370256,0.987470879370256),(0.990086238235256,0.987329216372183,
0.987470879370256,0.987470879370256,0.987470879370256)))
REPRESENTATION_ITEM('')
SURFACE()
);
#4067=(
BOUNDED_SURFACE()
B_SPLINE_SURFACE(1,2,((#162900,#162901,#162902),(#162903,#162904,#162905)),
 .UNSPECIFIED.,.F.,.F.,.F.)
B_SPLINE_SURFACE_WITH_KNOTS((2,2),(3,3),(0.710192959008298,1.),(0.625170525609407,
0.642682999576235),.UNSPECIFIED.)
GEOMETRIC_REPRESENTATION_ITEM()
RATIONAL_B_SPLINE_SURFACE(((0.990658108926708,0.993760979299921,0.999878046252916),
(0.990658108926708,0.993760979299921,0.999878046252916)))
REPRESENTATION_ITEM('')
SURFACE()
);
#4068=(
BOUNDED_SURFACE()
B_SPLINE_SURFACE(1,2,((#162909,#162910,#162911,#162912,#162913),(#162914,
#162915,#162916,#162917,#162918)),.UNSPECIFIED.,.F.,.F.,.F.)
B_SPLINE_SURFACE_WITH_KNOTS((2,2),(3,2,3),(0.710059257984503,1.),(0.0908085233856357,
0.107982157956012,0.108241816832277),.UNSPECIFIED.)
GEOMETRIC_REPRESENTATION_ITEM()
RATIONAL_B_SPLINE_SURFACE(((0.990086238235256,0.987329216372183,0.987470879370256,
0.987470879370256,0.987470879370256),(0.990086238235256,0.987329216372183,
0.987470879370256,0.987470879370256,0.987470879370256)))
REPRESENTATION_ITEM('')
SURFACE()
);
#4069=(
BOUNDED_SURFACE()
B_SPLINE_SURFACE(1,2,((#162920,#162921,#162922),(#162923,#162924,#162925)),
 .UNSPECIFIED.,.F.,.F.,.F.)
B_SPLINE_SURFACE_WITH_KNOTS((2,2),(3,3),(0.710192959008281,1.),(0.625170525609407,
0.642682999576235),.UNSPECIFIED.)
GEOMETRIC_REPRESENTATION_ITEM()
RATIONAL_B_SPLINE_SURFACE(((0.990658108926708,0.993760979299921,0.999878046252916),
(0.990658108926708,0.993760979299921,0.999878046252916)))
REPRESENTATION_ITEM('')
SURFACE()
);
#4070=(
BOUNDED_SURFACE()
B_SPLINE_SURFACE(1,2,((#162929,#162930,#162931,#162932,#162933),(#162934,
#162935,#162936,#162937,#162938)),.UNSPECIFIED.,.F.,.F.,.F.)
B_SPLINE_SURFACE_WITH_KNOTS((2,2),(3,2,3),(0.710059257931992,1.),(0.0908085233856358,
0.107982157956012,0.108241816884714),.UNSPECIFIED.)
GEOMETRIC_REPRESENTATION_ITEM()
RATIONAL_B_SPLINE_SURFACE(((0.990086238235256,0.987329216372183,0.987470879370256,
0.987470879370256,0.987470879370256),(0.990086238235256,0.987329216372183,
0.987470879370256,0.987470879370256,0.987470879370256)))
REPRESENTATION_ITEM('')
SURFACE()
);
#4071=(
BOUNDED_SURFACE()
B_SPLINE_SURFACE(1,2,((#162940,#162941,#162942),(#162943,#162944,#162945)),
 .UNSPECIFIED.,.F.,.F.,.F.)
B_SPLINE_SURFACE_WITH_KNOTS((2,2),(3,3),(0.71019295900691,1.),(0.625170525609407,
0.642682999576235),.UNSPECIFIED.)
GEOMETRIC_REPRESENTATION_ITEM()
RATIONAL_B_SPLINE_SURFACE(((0.990658108926708,0.993760979299921,0.999878046252916),
(0.990658108926708,0.993760979299921,0.999878046252916)))
REPRESENTATION_ITEM('')
SURFACE()
);
#4072=(
BOUNDED_SURFACE()
B_SPLINE_SURFACE(1,2,((#162949,#162950,#162951,#162952,#162953),(#162954,
#162955,#162956,#162957,#162958)),.UNSPECIFIED.,.F.,.F.,.F.)
B_SPLINE_SURFACE_WITH_KNOTS((2,2),(3,2,3),(0.71005925787149,1.),(0.0908085233856358,
0.107982157956012,0.108241816944409),.UNSPECIFIED.)
GEOMETRIC_REPRESENTATION_ITEM()
RATIONAL_B_SPLINE_SURFACE(((0.990086238235256,0.987329216372183,0.987470879370256,
0.987470879370256,0.987470879370256),(0.990086238235256,0.987329216372183,
0.987470879370255,0.987470879370255,0.987470879370255)))
REPRESENTATION_ITEM('')
SURFACE()
);
#4073=(
BOUNDED_SURFACE()
B_SPLINE_SURFACE(1,2,((#162960,#162961,#162962),(#162963,#162964,#162965)),
 .UNSPECIFIED.,.F.,.F.,.F.)
B_SPLINE_SURFACE_WITH_KNOTS((2,2),(3,3),(0.710192959008067,1.),(0.625170525609407,
0.642682999576233),.UNSPECIFIED.)
GEOMETRIC_REPRESENTATION_ITEM()
RATIONAL_B_SPLINE_SURFACE(((0.990658108926708,0.99376097929992,0.999878046252914),
(0.990658108926708,0.99376097929992,0.999878046252914)))
REPRESENTATION_ITEM('')
SURFACE()
);
#4074=(
BOUNDED_SURFACE()
B_SPLINE_SURFACE(1,2,((#162969,#162970,#162971,#162972,#162973),(#162974,
#162975,#162976,#162977,#162978)),.UNSPECIFIED.,.F.,.F.,.F.)
B_SPLINE_SURFACE_WITH_KNOTS((2,2),(3,2,3),(0.710059258140776,1.),(0.0908085233856304,
0.107982157956012,0.108241816675822),.UNSPECIFIED.)
GEOMETRIC_REPRESENTATION_ITEM()
RATIONAL_B_SPLINE_SURFACE(((0.990086238235258,0.987329216372183,0.987470879370256,
0.987470879370256,0.987470879370256),(0.990086238235258,0.987329216372183,
0.987470879370255,0.987470879370255,0.987470879370255)))
REPRESENTATION_ITEM('')
SURFACE()
);
#4075=(
BOUNDED_SURFACE()
B_SPLINE_SURFACE(1,2,((#162980,#162981,#162982),(#162983,#162984,#162985)),
 .UNSPECIFIED.,.F.,.F.,.F.)
B_SPLINE_SURFACE_WITH_KNOTS((2,2),(3,3),(0.71019295900844,1.),(0.625170525609407,
0.642682999576235),.UNSPECIFIED.)
GEOMETRIC_REPRESENTATION_ITEM()
RATIONAL_B_SPLINE_SURFACE(((0.990658108926708,0.993760979299921,0.999878046252916),
(0.990658108926708,0.993760979299921,0.999878046252916)))
REPRESENTATION_ITEM('')
SURFACE()
);
#4076=(
BOUNDED_SURFACE()
B_SPLINE_SURFACE(1,2,((#162989,#162990,#162991,#162992,#162993),(#162994,
#162995,#162996,#162997,#162998)),.UNSPECIFIED.,.F.,.F.,.F.)
B_SPLINE_SURFACE_WITH_KNOTS((2,2),(3,2,3),(0.710059257748965,1.),(0.0908085233856358,
0.107982157956012,0.108241817067853),.UNSPECIFIED.)
GEOMETRIC_REPRESENTATION_ITEM()
RATIONAL_B_SPLINE_SURFACE(((0.990086238235256,0.987329216372183,0.987470879370256,
0.987470879370256,0.987470879370256),(0.990086238235256,0.987329216372183,
0.987470879370256,0.987470879370256,0.987470879370256)))
REPRESENTATION_ITEM('')
SURFACE()
);
#4077=(
BOUNDED_SURFACE()
B_SPLINE_SURFACE(1,2,((#163000,#163001,#163002),(#163003,#163004,#163005)),
 .UNSPECIFIED.,.F.,.F.,.F.)
B_SPLINE_SURFACE_WITH_KNOTS((2,2),(3,3),(0.710192959008438,1.),(0.625170525609407,
0.642682999576235),.UNSPECIFIED.)
GEOMETRIC_REPRESENTATION_ITEM()
RATIONAL_B_SPLINE_SURFACE(((0.990658108926708,0.993760979299921,0.999878046252916),
(0.990658108926708,0.993760979299921,0.999878046252916)))
REPRESENTATION_ITEM('')
SURFACE()
);
#4078=(
BOUNDED_SURFACE()
B_SPLINE_SURFACE(1,2,((#163009,#163010,#163011,#163012,#163013),(#163014,
#163015,#163016,#163017,#163018)),.UNSPECIFIED.,.F.,.F.,.F.)
B_SPLINE_SURFACE_WITH_KNOTS((2,2),(3,2,3),(0.710059257935878,1.),(0.0908085233856358,
0.107982157956012,0.108241816880996),.UNSPECIFIED.)
GEOMETRIC_REPRESENTATION_ITEM()
RATIONAL_B_SPLINE_SURFACE(((0.990086238235256,0.987329216372183,0.987470879370255,
0.987470879370255,0.987470879370255),(0.990086238235256,0.987329216372183,
0.987470879370255,0.987470879370255,0.987470879370255)))
REPRESENTATION_ITEM('')
SURFACE()
);
#4079=(
BOUNDED_SURFACE()
B_SPLINE_SURFACE(1,2,((#163020,#163021,#163022),(#163023,#163024,#163025)),
 .UNSPECIFIED.,.F.,.F.,.F.)
B_SPLINE_SURFACE_WITH_KNOTS((2,2),(3,3),(0.710192959008437,1.),(0.625170525609407,
0.642682999576235),.UNSPECIFIED.)
GEOMETRIC_REPRESENTATION_ITEM()
RATIONAL_B_SPLINE_SURFACE(((0.990658108926708,0.993760979299921,0.999878046252916),
(0.990658108926708,0.993760979299921,0.999878046252916)))
REPRESENTATION_ITEM('')
SURFACE()
);
#4080=(
BOUNDED_SURFACE()
B_SPLINE_SURFACE(1,2,((#163027,#163028,#163029),(#163030,#163031,#163032),
(#163033,#163034,#163035)),.UNSPECIFIED.,.F.,.F.,.F.)
B_SPLINE_SURFACE_WITH_KNOTS((2,1,2),(3,3),(0.,0.289807040991559,0.311582168299949),
(0.0909109506295943,0.108084585199971),.UNSPECIFIED.)
GEOMETRIC_REPRESENTATION_ITEM()
RATIONAL_B_SPLINE_SURFACE(((0.990053454406147,0.987313720921968,0.987472672298934),
(0.990053454406147,0.987313720921967,0.987472672298933),(0.990053454406147,
0.987313720921967,0.987472672298933)))
REPRESENTATION_ITEM('')
SURFACE()
);
#4081=(
BOUNDED_SURFACE()
B_SPLINE_SURFACE(1,2,((#163076,#163077,#163078),(#163079,#163080,#163081),
(#163082,#163083,#163084)),.UNSPECIFIED.,.F.,.F.,.F.)
B_SPLINE_SURFACE_WITH_KNOTS((2,1,2),(3,3),(0.,0.289681084359918,0.311483586954517),
(0.625066077454536,0.642578551421363),.UNSPECIFIED.)
GEOMETRIC_REPRESENTATION_ITEM()
RATIONAL_B_SPLINE_SURFACE(((0.990621203777021,0.993706096834649,0.999805186472059),
(0.990621203777021,0.993706096834649,0.999805186472059),(0.990621203777021,
0.993706096834649,0.999805186472059)))
REPRESENTATION_ITEM('')
SURFACE()
);
#4082=(
BOUNDED_SURFACE()
B_SPLINE_SURFACE(1,2,((#163086,#163087,#163088),(#163089,#163090,#163091),
(#163092,#163093,#163094)),.UNSPECIFIED.,.F.,.F.,.F.)
B_SPLINE_SURFACE_WITH_KNOTS((2,1,2),(3,3),(0.,0.289807040991555,0.311582168338885),
(0.0909109506295943,0.108084585199971),.UNSPECIFIED.)
GEOMETRIC_REPRESENTATION_ITEM()
RATIONAL_B_SPLINE_SURFACE(((0.990053454406147,0.987313720921968,0.987472672298934),
(0.990053454406147,0.987313720921968,0.987472672298934),(0.990053454406147,
0.987313720921968,0.987472672298934)))
REPRESENTATION_ITEM('')
SURFACE()
);
#4083=(
BOUNDED_SURFACE()
B_SPLINE_SURFACE(1,2,((#163135,#163136,#163137),(#163138,#163139,#163140),
(#163141,#163142,#163143)),.UNSPECIFIED.,.F.,.F.,.F.)
B_SPLINE_SURFACE_WITH_KNOTS((2,1,2),(3,3),(0.,0.289681084359919,0.311483587022812),
(0.625066077454535,0.642578551421363),.UNSPECIFIED.)
GEOMETRIC_REPRESENTATION_ITEM()
RATIONAL_B_SPLINE_SURFACE(((0.990621203777021,0.993706096834649,0.999805186472059),
(0.990621203777021,0.993706096834649,0.999805186472059),(0.990621203777021,
0.993706096834649,0.999805186472059)))
REPRESENTATION_ITEM('')
SURFACE()
);
#4084=(
BOUNDED_SURFACE()
B_SPLINE_SURFACE(1,2,((#163145,#163146,#163147),(#163148,#163149,#163150),
(#163151,#163152,#163153)),.UNSPECIFIED.,.F.,.F.,.F.)
B_SPLINE_SURFACE_WITH_KNOTS((2,1,2),(3,3),(0.,0.289807040991561,0.311582168422346),
(0.0909109506295943,0.108084585199971),.UNSPECIFIED.)
GEOMETRIC_REPRESENTATION_ITEM()
RATIONAL_B_SPLINE_SURFACE(((0.990053454406147,0.987313720921968,0.987472672298934),
(0.990053454406147,0.987313720921968,0.987472672298934),(0.990053454406147,
0.987313720921968,0.987472672298934)))
REPRESENTATION_ITEM('')
SURFACE()
);
#4085=(
BOUNDED_SURFACE()
B_SPLINE_SURFACE(1,2,((#163194,#163195,#163196),(#163197,#163198,#163199),
(#163200,#163201,#163202)),.UNSPECIFIED.,.F.,.F.,.F.)
B_SPLINE_SURFACE_WITH_KNOTS((2,1,2),(3,3),(0.,0.289681084359919,0.31148358704291),
(0.625066077454535,0.642578551421363),.UNSPECIFIED.)
GEOMETRIC_REPRESENTATION_ITEM()
RATIONAL_B_SPLINE_SURFACE(((0.990621203777021,0.993706096834649,0.999805186472059),
(0.990621203777021,0.993706096834649,0.999805186472059),(0.990621203777021,
0.993706096834649,0.999805186472059)))
REPRESENTATION_ITEM('')
SURFACE()
);
#4086=(
BOUNDED_SURFACE()
B_SPLINE_SURFACE(1,2,((#163204,#163205,#163206),(#163207,#163208,#163209),
(#163210,#163211,#163212)),.UNSPECIFIED.,.F.,.F.,.F.)
B_SPLINE_SURFACE_WITH_KNOTS((2,1,2),(3,3),(0.,0.289807040991562,0.311582167804269),
(0.0909109506295943,0.10808458519997),.UNSPECIFIED.)
GEOMETRIC_REPRESENTATION_ITEM()
RATIONAL_B_SPLINE_SURFACE(((0.990053454406147,0.987313720921968,0.987472672298934),
(0.990053454406147,0.987313720921967,0.987472672298933),(0.990053454406147,
0.987313720921967,0.987472672298933)))
REPRESENTATION_ITEM('')
SURFACE()
);
#4087=(
BOUNDED_SURFACE()
B_SPLINE_SURFACE(1,2,((#163253,#163254,#163255),(#163256,#163257,#163258),
(#163259,#163260,#163261)),.UNSPECIFIED.,.F.,.F.,.F.)
B_SPLINE_SURFACE_WITH_KNOTS((2,1,2),(3,3),(0.,0.289681084359921,0.311483587161093),
(0.625066077454535,0.642578551421363),.UNSPECIFIED.)
GEOMETRIC_REPRESENTATION_ITEM()
RATIONAL_B_SPLINE_SURFACE(((0.990621203777021,0.993706096834649,0.999805186472059),
(0.990621203777021,0.993706096834649,0.999805186472059),(0.990621203777021,
0.993706096834649,0.999805186472059)))
REPRESENTATION_ITEM('')
SURFACE()
);
#4088=(
BOUNDED_SURFACE()
B_SPLINE_SURFACE(1,2,((#163263,#163264,#163265),(#163266,#163267,#163268),
(#163269,#163270,#163271)),.UNSPECIFIED.,.F.,.F.,.F.)
B_SPLINE_SURFACE_WITH_KNOTS((2,1,2),(3,3),(0.,0.289807040991556,0.3115821682498),
(0.0909109506295943,0.108084585199969),.UNSPECIFIED.)
GEOMETRIC_REPRESENTATION_ITEM()
RATIONAL_B_SPLINE_SURFACE(((0.990053454406147,0.987313720921968,0.987472672298934),
(0.990053454406147,0.987313720921968,0.987472672298934),(0.990053454406147,
0.987313720921968,0.987472672298934)))
REPRESENTATION_ITEM('')
SURFACE()
);
#4089=(
BOUNDED_SURFACE()
B_SPLINE_SURFACE(1,2,((#163312,#163313,#163314),(#163315,#163316,#163317),
(#163318,#163319,#163320)),.UNSPECIFIED.,.F.,.F.,.F.)
B_SPLINE_SURFACE_WITH_KNOTS((2,1,2),(3,3),(0.,0.289681084359916,0.311483587306944),
(0.625066077454536,0.642578551421364),.UNSPECIFIED.)
GEOMETRIC_REPRESENTATION_ITEM()
RATIONAL_B_SPLINE_SURFACE(((0.990621203777022,0.993706096834649,0.999805186472059),
(0.990621203777022,0.993706096834649,0.999805186472059),(0.990621203777022,
0.993706096834649,0.999805186472059)))
REPRESENTATION_ITEM('')
SURFACE()
);
#4090=(
BOUNDED_SURFACE()
B_SPLINE_SURFACE(1,2,((#163322,#163323,#163324),(#163325,#163326,#163327),
(#163328,#163329,#163330)),.UNSPECIFIED.,.F.,.F.,.F.)
B_SPLINE_SURFACE_WITH_KNOTS((2,1,2),(3,3),(0.,0.289807040991564,0.311582168172586),
(0.0909109506295932,0.108084585199969),.UNSPECIFIED.)
GEOMETRIC_REPRESENTATION_ITEM()
RATIONAL_B_SPLINE_SURFACE(((0.990053454406148,0.987313720921968,0.987472672298934),
(0.990053454406147,0.987313720921968,0.987472672298934),(0.990053454406147,
0.987313720921968,0.987472672298934)))
REPRESENTATION_ITEM('')
SURFACE()
);
#4091=(
BOUNDED_SURFACE()
B_SPLINE_SURFACE(1,2,((#163371,#163372,#163373),(#163374,#163375,#163376),
(#163377,#163378,#163379)),.UNSPECIFIED.,.F.,.F.,.F.)
B_SPLINE_SURFACE_WITH_KNOTS((2,1,2),(3,3),(0.,0.289681084359926,0.311483587003064),
(0.625066077454536,0.642578551421364),.UNSPECIFIED.)
GEOMETRIC_REPRESENTATION_ITEM()
RATIONAL_B_SPLINE_SURFACE(((0.990621203777022,0.993706096834649,0.999805186472059),
(0.990621203777022,0.993706096834649,0.999805186472059),(0.990621203777022,
0.993706096834649,0.999805186472059)))
REPRESENTATION_ITEM('')
SURFACE()
);
#4092=(
BOUNDED_SURFACE()
B_SPLINE_SURFACE(1,2,((#163381,#163382,#163383),(#163384,#163385,#163386),
(#163387,#163388,#163389)),.UNSPECIFIED.,.F.,.F.,.F.)
B_SPLINE_SURFACE_WITH_KNOTS((2,1,2),(3,3),(0.,0.289807040991566,0.311582168018321),
(0.0909109506295932,0.108084585199969),.UNSPECIFIED.)
GEOMETRIC_REPRESENTATION_ITEM()
RATIONAL_B_SPLINE_SURFACE(((0.990053454406148,0.987313720921968,0.987472672298934),
(0.990053454406148,0.987313720921968,0.987472672298934),(0.990053454406148,
0.987313720921968,0.987472672298934)))
REPRESENTATION_ITEM('')
SURFACE()
);
#4093=(
BOUNDED_SURFACE()
B_SPLINE_SURFACE(1,2,((#163430,#163431,#163432),(#163433,#163434,#163435),
(#163436,#163437,#163438)),.UNSPECIFIED.,.F.,.F.,.F.)
B_SPLINE_SURFACE_WITH_KNOTS((2,1,2),(3,3),(0.,0.289681084359925,0.311483586740803),
(0.625066077454536,0.642578551421364),.UNSPECIFIED.)
GEOMETRIC_REPRESENTATION_ITEM()
RATIONAL_B_SPLINE_SURFACE(((0.990621203777022,0.993706096834649,0.999805186472059),
(0.990621203777022,0.993706096834649,0.999805186472059),(0.990621203777022,
0.993706096834649,0.999805186472059)))
REPRESENTATION_ITEM('')
SURFACE()
);
#4094=(
BOUNDED_SURFACE()
B_SPLINE_SURFACE(1,2,((#163440,#163441,#163442),(#163443,#163444,#163445),
(#163446,#163447,#163448)),.UNSPECIFIED.,.F.,.F.,.F.)
B_SPLINE_SURFACE_WITH_KNOTS((2,1,2),(3,3),(0.,0.289807040991568,0.311582168115042),
(0.0909109506295933,0.10808458519997),.UNSPECIFIED.)
GEOMETRIC_REPRESENTATION_ITEM()
RATIONAL_B_SPLINE_SURFACE(((0.990053454406148,0.987313720921968,0.987472672298934),
(0.990053454406148,0.987313720921968,0.987472672298934),(0.990053454406148,
0.987313720921968,0.987472672298934)))
REPRESENTATION_ITEM('')
SURFACE()
);
#4095=(
BOUNDED_SURFACE()
B_SPLINE_SURFACE(1,2,((#163489,#163490,#163491),(#163492,#163493,#163494),
(#163495,#163496,#163497)),.UNSPECIFIED.,.F.,.F.,.F.)
B_SPLINE_SURFACE_WITH_KNOTS((2,1,2),(3,3),(0.,0.289681084359926,0.31148358704133),
(0.625066077454536,0.642578551421364),.UNSPECIFIED.)
GEOMETRIC_REPRESENTATION_ITEM()
RATIONAL_B_SPLINE_SURFACE(((0.990621203777022,0.993706096834649,0.999805186472059),
(0.990621203777022,0.993706096834649,0.999805186472059),(0.990621203777022,
0.993706096834649,0.999805186472059)))
REPRESENTATION_ITEM('')
SURFACE()
);
#4096=(
BOUNDED_SURFACE()
B_SPLINE_SURFACE(1,2,((#163499,#163500,#163501),(#163502,#163503,#163504),
(#163505,#163506,#163507)),.UNSPECIFIED.,.F.,.F.,.F.)
B_SPLINE_SURFACE_WITH_KNOTS((2,1,2),(3,3),(0.,0.289807040991563,0.311582168082872),
(0.0909109506295932,0.10808458519997),.UNSPECIFIED.)
GEOMETRIC_REPRESENTATION_ITEM()
RATIONAL_B_SPLINE_SURFACE(((0.990053454406148,0.987313720921968,0.987472672298934),
(0.990053454406147,0.987313720921968,0.987472672298933),(0.990053454406147,
0.987313720921968,0.987472672298933)))
REPRESENTATION_ITEM('')
SURFACE()
);
#4097=(
BOUNDED_SURFACE()
B_SPLINE_SURFACE(1,2,((#163548,#163549,#163550),(#163551,#163552,#163553),
(#163554,#163555,#163556)),.UNSPECIFIED.,.F.,.F.,.F.)
B_SPLINE_SURFACE_WITH_KNOTS((2,1,2),(3,3),(0.,0.289681084359922,0.311483586742761),
(0.625066077454537,0.642578551421364),.UNSPECIFIED.)
GEOMETRIC_REPRESENTATION_ITEM()
RATIONAL_B_SPLINE_SURFACE(((0.990621203777022,0.993706096834649,0.999805186472059),
(0.990621203777022,0.993706096834649,0.999805186472059),(0.990621203777022,
0.993706096834649,0.999805186472059)))
REPRESENTATION_ITEM('')
SURFACE()
);
#4098=(
BOUNDED_SURFACE()
B_SPLINE_SURFACE(1,2,((#163558,#163559,#163560),(#163561,#163562,#163563),
(#163564,#163565,#163566)),.UNSPECIFIED.,.F.,.F.,.F.)
B_SPLINE_SURFACE_WITH_KNOTS((2,1,2),(3,3),(0.,0.289807040991562,0.311582168130035),
(0.0909109506295931,0.108084585199969),.UNSPECIFIED.)
GEOMETRIC_REPRESENTATION_ITEM()
RATIONAL_B_SPLINE_SURFACE(((0.990053454406148,0.987313720921968,0.987472672298934),
(0.990053454406147,0.987313720921968,0.987472672298933),(0.990053454406147,
0.987313720921968,0.987472672298933)))
REPRESENTATION_ITEM('')
SURFACE()
);
#4099=(
BOUNDED_SURFACE()
B_SPLINE_SURFACE(1,2,((#163607,#163608,#163609),(#163610,#163611,#163612),
(#163613,#163614,#163615)),.UNSPECIFIED.,.F.,.F.,.F.)
B_SPLINE_SURFACE_WITH_KNOTS((2,1,2),(3,3),(0.,0.289681084359916,0.311483587005553),
(0.625066077454537,0.642578551421365),.UNSPECIFIED.)
GEOMETRIC_REPRESENTATION_ITEM()
RATIONAL_B_SPLINE_SURFACE(((0.990621203777022,0.993706096834649,0.999805186472059),
(0.990621203777022,0.993706096834649,0.999805186472059),(0.990621203777022,
0.993706096834649,0.999805186472059)))
REPRESENTATION_ITEM('')
SURFACE()
);
#4100=(
BOUNDED_SURFACE()
B_SPLINE_SURFACE(1,2,((#163617,#163618,#163619),(#163620,#163621,#163622),
(#163623,#163624,#163625)),.UNSPECIFIED.,.F.,.F.,.F.)
B_SPLINE_SURFACE_WITH_KNOTS((2,1,2),(3,3),(0.,0.289807040991561,0.311582167973507),
(0.0909109506295932,0.10808458519997),.UNSPECIFIED.)
GEOMETRIC_REPRESENTATION_ITEM()
RATIONAL_B_SPLINE_SURFACE(((0.990053454406147,0.987313720921968,0.987472672298934),
(0.990053454406147,0.987313720921968,0.987472672298934),(0.990053454406147,
0.987313720921968,0.987472672298934)))
REPRESENTATION_ITEM('')
SURFACE()
);
#4101=(
BOUNDED_SURFACE()
B_SPLINE_SURFACE(1,2,((#163666,#163667,#163668),(#163669,#163670,#163671),
(#163672,#163673,#163674)),.UNSPECIFIED.,.F.,.F.,.F.)
B_SPLINE_SURFACE_WITH_KNOTS((2,1,2),(3,3),(0.,0.289681084359914,0.311483587146096),
(0.625066077454537,0.642578551421365),.UNSPECIFIED.)
GEOMETRIC_REPRESENTATION_ITEM()
RATIONAL_B_SPLINE_SURFACE(((0.990621203777022,0.993706096834649,0.999805186472059),
(0.990621203777022,0.993706096834649,0.999805186472059),(0.990621203777022,
0.993706096834649,0.999805186472059)))
REPRESENTATION_ITEM('')
SURFACE()
);
#4102=(
BOUNDED_SURFACE()
B_SPLINE_SURFACE(1,2,((#163676,#163677,#163678),(#163679,#163680,#163681),
(#163682,#163683,#163684)),.UNSPECIFIED.,.F.,.F.,.F.)
B_SPLINE_SURFACE_WITH_KNOTS((2,1,2),(3,3),(0.,0.289807040991563,0.311582168117811),
(0.090910950629593,0.10808458519997),.UNSPECIFIED.)
GEOMETRIC_REPRESENTATION_ITEM()
RATIONAL_B_SPLINE_SURFACE(((0.990053454406148,0.987313720921968,0.987472672298934),
(0.990053454406148,0.987313720921968,0.987472672298934),(0.990053454406148,
0.987313720921968,0.987472672298934)))
REPRESENTATION_ITEM('')
SURFACE()
);
#4103=(
BOUNDED_SURFACE()
B_SPLINE_SURFACE(1,2,((#163725,#163726,#163727),(#163728,#163729,#163730),
(#163731,#163732,#163733)),.UNSPECIFIED.,.F.,.F.,.F.)
B_SPLINE_SURFACE_WITH_KNOTS((2,1,2),(3,3),(0.,0.289681084359914,0.311483586777713),
(0.625066077454537,0.642578551421365),.UNSPECIFIED.)
GEOMETRIC_REPRESENTATION_ITEM()
RATIONAL_B_SPLINE_SURFACE(((0.990621203777022,0.99370609683465,0.99980518647206),
(0.990621203777022,0.99370609683465,0.99980518647206),(0.990621203777022,
0.99370609683465,0.99980518647206)))
REPRESENTATION_ITEM('')
SURFACE()
);
#4104=(
BOUNDED_SURFACE()
B_SPLINE_SURFACE(1,2,((#163735,#163736,#163737),(#163738,#163739,#163740),
(#163741,#163742,#163743)),.UNSPECIFIED.,.F.,.F.,.F.)
B_SPLINE_SURFACE_WITH_KNOTS((2,1,2),(3,3),(0.,0.289807040991564,0.311582168145372),
(0.0909109506295933,0.108084585199969),.UNSPECIFIED.)
GEOMETRIC_REPRESENTATION_ITEM()
RATIONAL_B_SPLINE_SURFACE(((0.990053454406148,0.987313720921968,0.987472672298934),
(0.990053454406148,0.987313720921968,0.987472672298934),(0.990053454406148,
0.987313720921968,0.987472672298934)))
REPRESENTATION_ITEM('')
SURFACE()
);
#4105=(
BOUNDED_SURFACE()
B_SPLINE_SURFACE(1,2,((#163784,#163785,#163786),(#163787,#163788,#163789),
(#163790,#163791,#163792)),.UNSPECIFIED.,.F.,.F.,.F.)
B_SPLINE_SURFACE_WITH_KNOTS((2,1,2),(3,3),(0.,0.289681084359918,0.311483587040421),
(0.625066077454537,0.642578551421364),.UNSPECIFIED.)
GEOMETRIC_REPRESENTATION_ITEM()
RATIONAL_B_SPLINE_SURFACE(((0.990621203777022,0.993706096834649,0.999805186472059),
(0.990621203777022,0.993706096834649,0.999805186472059),(0.990621203777022,
0.993706096834649,0.999805186472059)))
REPRESENTATION_ITEM('')
SURFACE()
);
#4106=(
BOUNDED_SURFACE()
B_SPLINE_SURFACE(1,2,((#163794,#163795,#163796),(#163797,#163798,#163799),
(#163800,#163801,#163802)),.UNSPECIFIED.,.F.,.F.,.F.)
B_SPLINE_SURFACE_WITH_KNOTS((2,1,2),(3,3),(0.,0.289807040991562,0.311582167901583),
(0.0909109506295932,0.108084585199969),.UNSPECIFIED.)
GEOMETRIC_REPRESENTATION_ITEM()
RATIONAL_B_SPLINE_SURFACE(((0.990053454406148,0.987313720921968,0.987472672298934),
(0.990053454406148,0.987313720921968,0.987472672298934),(0.990053454406148,
0.987313720921968,0.987472672298934)))
REPRESENTATION_ITEM('')
SURFACE()
);
#4107=(
BOUNDED_SURFACE()
B_SPLINE_SURFACE(1,2,((#163843,#163844,#163845),(#163846,#163847,#163848),
(#163849,#163850,#163851)),.UNSPECIFIED.,.F.,.F.,.F.)
B_SPLINE_SURFACE_WITH_KNOTS((2,1,2),(3,3),(0.,0.28968108435992,0.311483587070223),
(0.625066077454536,0.642578551421364),.UNSPECIFIED.)
GEOMETRIC_REPRESENTATION_ITEM()
RATIONAL_B_SPLINE_SURFACE(((0.990621203777022,0.993706096834649,0.999805186472059),
(0.990621203777022,0.993706096834649,0.999805186472059),(0.990621203777022,
0.993706096834649,0.999805186472059)))
REPRESENTATION_ITEM('')
SURFACE()
);
#4108=(
BOUNDED_SURFACE()
B_SPLINE_SURFACE(1,2,((#163853,#163854,#163855),(#163856,#163857,#163858),
(#163859,#163860,#163861)),.UNSPECIFIED.,.F.,.F.,.F.)
B_SPLINE_SURFACE_WITH_KNOTS((2,1,2),(3,3),(0.,0.28980704099156,0.311582167938859),
(0.0909109506295931,0.10808458519997),.UNSPECIFIED.)
GEOMETRIC_REPRESENTATION_ITEM()
RATIONAL_B_SPLINE_SURFACE(((0.990053454406148,0.987313720921968,0.987472672298934),
(0.990053454406148,0.987313720921968,0.987472672298934),(0.990053454406148,
0.987313720921968,0.987472672298934)))
REPRESENTATION_ITEM('')
SURFACE()
);
#4109=(
BOUNDED_SURFACE()
B_SPLINE_SURFACE(1,2,((#163902,#163903,#163904),(#163905,#163906,#163907),
(#163908,#163909,#163910)),.UNSPECIFIED.,.F.,.F.,.F.)
B_SPLINE_SURFACE_WITH_KNOTS((2,1,2),(3,3),(0.,0.289681084359922,0.311483587082788),
(0.625066077454537,0.642578551421364),.UNSPECIFIED.)
GEOMETRIC_REPRESENTATION_ITEM()
RATIONAL_B_SPLINE_SURFACE(((0.990621203777022,0.993706096834649,0.999805186472059),
(0.990621203777022,0.993706096834649,0.999805186472059),(0.990621203777022,
0.993706096834649,0.999805186472059)))
REPRESENTATION_ITEM('')
SURFACE()
);
#4110=(
BOUNDED_SURFACE()
B_SPLINE_SURFACE(1,2,((#163912,#163913,#163914),(#163915,#163916,#163917),
(#163918,#163919,#163920)),.UNSPECIFIED.,.F.,.F.,.F.)
B_SPLINE_SURFACE_WITH_KNOTS((2,1,2),(3,3),(0.,0.289807040991562,0.311582168075301),
(0.0909109506295932,0.108084585199969),.UNSPECIFIED.)
GEOMETRIC_REPRESENTATION_ITEM()
RATIONAL_B_SPLINE_SURFACE(((0.990053454406147,0.987313720921968,0.987472672298934),
(0.990053454406147,0.987313720921968,0.987472672298934),(0.990053454406147,
0.987313720921968,0.987472672298934)))
REPRESENTATION_ITEM('')
SURFACE()
);
#4111=(
BOUNDED_SURFACE()
B_SPLINE_SURFACE(1,2,((#163961,#163962,#163963),(#163964,#163965,#163966),
(#163967,#163968,#163969)),.UNSPECIFIED.,.F.,.F.,.F.)
B_SPLINE_SURFACE_WITH_KNOTS((2,1,2),(3,3),(0.,0.289681084359918,0.31148358684503),
(0.625066077454536,0.642578551421364),.UNSPECIFIED.)
GEOMETRIC_REPRESENTATION_ITEM()
RATIONAL_B_SPLINE_SURFACE(((0.990621203777022,0.993706096834649,0.999805186472059),
(0.990621203777022,0.993706096834649,0.999805186472059),(0.990621203777022,
0.993706096834649,0.999805186472059)))
REPRESENTATION_ITEM('')
SURFACE()
);
#4112=(
BOUNDED_SURFACE()
B_SPLINE_SURFACE(1,2,((#163971,#163972,#163973),(#163974,#163975,#163976),
(#163977,#163978,#163979)),.UNSPECIFIED.,.F.,.F.,.F.)
B_SPLINE_SURFACE_WITH_KNOTS((2,1,2),(3,3),(0.,0.289807040991558,0.311582167912575),
(0.0909109506295932,0.10808458519997),.UNSPECIFIED.)
GEOMETRIC_REPRESENTATION_ITEM()
RATIONAL_B_SPLINE_SURFACE(((0.990053454406148,0.987313720921968,0.987472672298934),
(0.990053454406148,0.987313720921968,0.987472672298934),(0.990053454406148,
0.987313720921968,0.987472672298934)))
REPRESENTATION_ITEM('')
SURFACE()
);
#4113=(
BOUNDED_SURFACE()
B_SPLINE_SURFACE(1,2,((#164020,#164021,#164022),(#164023,#164024,#164025),
(#164026,#164027,#164028)),.UNSPECIFIED.,.F.,.F.,.F.)
B_SPLINE_SURFACE_WITH_KNOTS((2,1,2),(3,3),(0.,0.289681084359916,0.311483587281286),
(0.625066077454537,0.642578551421364),.UNSPECIFIED.)
GEOMETRIC_REPRESENTATION_ITEM()
RATIONAL_B_SPLINE_SURFACE(((0.990621203777022,0.993706096834649,0.999805186472059),
(0.990621203777022,0.993706096834649,0.999805186472059),(0.990621203777022,
0.993706096834649,0.999805186472059)))
REPRESENTATION_ITEM('')
SURFACE()
);
#4114=(
BOUNDED_SURFACE()
B_SPLINE_SURFACE(1,2,((#164030,#164031,#164032),(#164033,#164034,#164035),
(#164036,#164037,#164038)),.UNSPECIFIED.,.F.,.F.,.F.)
B_SPLINE_SURFACE_WITH_KNOTS((2,1,2),(3,3),(0.,0.28980704099156,0.31158216795133),
(0.0909109506295932,0.10808458519997),.UNSPECIFIED.)
GEOMETRIC_REPRESENTATION_ITEM()
RATIONAL_B_SPLINE_SURFACE(((0.990053454406148,0.987313720921968,0.987472672298934),
(0.990053454406148,0.987313720921968,0.987472672298934),(0.990053454406148,
0.987313720921968,0.987472672298934)))
REPRESENTATION_ITEM('')
SURFACE()
);
#4115=(
BOUNDED_SURFACE()
B_SPLINE_SURFACE(1,2,((#164079,#164080,#164081),(#164082,#164083,#164084),
(#164085,#164086,#164087)),.UNSPECIFIED.,.F.,.F.,.F.)
B_SPLINE_SURFACE_WITH_KNOTS((2,1,2),(3,3),(0.,0.289681084359915,0.31148358716528),
(0.625066077454537,0.642578551421363),.UNSPECIFIED.)
GEOMETRIC_REPRESENTATION_ITEM()
RATIONAL_B_SPLINE_SURFACE(((0.990621203777022,0.993706096834649,0.999805186472059),
(0.990621203777022,0.993706096834649,0.999805186472059),(0.990621203777022,
0.993706096834649,0.999805186472059)))
REPRESENTATION_ITEM('')
SURFACE()
);
#4116=(
BOUNDED_SURFACE()
B_SPLINE_SURFACE(1,2,((#164089,#164090,#164091),(#164092,#164093,#164094),
(#164095,#164096,#164097)),.UNSPECIFIED.,.F.,.F.,.F.)
B_SPLINE_SURFACE_WITH_KNOTS((2,1,2),(3,3),(0.,0.289807040991637,0.311582168368617),
(0.0909109506295941,0.10808458519997),.UNSPECIFIED.)
GEOMETRIC_REPRESENTATION_ITEM()
RATIONAL_B_SPLINE_SURFACE(((0.990053454406147,0.987313720921968,0.987472672298934),
(0.990053454406147,0.987313720921968,0.987472672298934),(0.990053454406147,
0.987313720921968,0.987472672298934)))
REPRESENTATION_ITEM('')
SURFACE()
);
#4117=(
BOUNDED_SURFACE()
B_SPLINE_SURFACE(1,2,((#164138,#164139,#164140),(#164141,#164142,#164143),
(#164144,#164145,#164146)),.UNSPECIFIED.,.F.,.F.,.F.)
B_SPLINE_SURFACE_WITH_KNOTS((2,1,2),(3,3),(0.,0.289681084359918,0.311483587033473),
(0.625066077454535,0.642578551421363),.UNSPECIFIED.)
GEOMETRIC_REPRESENTATION_ITEM()
RATIONAL_B_SPLINE_SURFACE(((0.990621203777021,0.993706096834649,0.999805186472059),
(0.990621203777021,0.993706096834649,0.999805186472059),(0.990621203777021,
0.993706096834649,0.999805186472059)))
REPRESENTATION_ITEM('')
SURFACE()
);
#4118=(
BOUNDED_SURFACE()
B_SPLINE_SURFACE(1,2,((#164148,#164149,#164150),(#164151,#164152,#164153),
(#164154,#164155,#164156)),.UNSPECIFIED.,.F.,.F.,.F.)
B_SPLINE_SURFACE_WITH_KNOTS((2,1,2),(3,3),(0.,0.289807040991563,0.31158216809578),
(0.0909109506295943,0.108084585199971),.UNSPECIFIED.)
GEOMETRIC_REPRESENTATION_ITEM()
RATIONAL_B_SPLINE_SURFACE(((0.990053454406147,0.987313720921968,0.987472672298934),
(0.990053454406147,0.987313720921968,0.987472672298934),(0.990053454406147,
0.987313720921968,0.987472672298934)))
REPRESENTATION_ITEM('')
SURFACE()
);
#4119=(
BOUNDED_SURFACE()
B_SPLINE_SURFACE(1,2,((#164197,#164198,#164199),(#164200,#164201,#164202),
(#164203,#164204,#164205)),.UNSPECIFIED.,.F.,.F.,.F.)
B_SPLINE_SURFACE_WITH_KNOTS((2,1,2),(3,3),(0.,0.289681084359918,0.311483587195346),
(0.625066077454535,0.642578551421363),.UNSPECIFIED.)
GEOMETRIC_REPRESENTATION_ITEM()
RATIONAL_B_SPLINE_SURFACE(((0.990621203777021,0.993706096834649,0.999805186472059),
(0.990621203777021,0.993706096834649,0.999805186472059),(0.990621203777021,
0.993706096834649,0.999805186472059)))
REPRESENTATION_ITEM('')
SURFACE()
);
#4120=(
BOUNDED_SURFACE()
B_SPLINE_SURFACE(1,2,((#164207,#164208,#164209),(#164210,#164211,#164212),
(#164213,#164214,#164215)),.UNSPECIFIED.,.F.,.F.,.F.)
B_SPLINE_SURFACE_WITH_KNOTS((2,1,2),(3,3),(0.,0.289807040991564,0.31158216794018),
(0.0909109506295943,0.108084585199971),.UNSPECIFIED.)
GEOMETRIC_REPRESENTATION_ITEM()
RATIONAL_B_SPLINE_SURFACE(((0.990053454406147,0.987313720921968,0.987472672298934),
(0.990053454406147,0.987313720921968,0.987472672298934),(0.990053454406147,
0.987313720921968,0.987472672298934)))
REPRESENTATION_ITEM('')
SURFACE()
);
#4121=(
BOUNDED_SURFACE()
B_SPLINE_SURFACE(1,2,((#164256,#164257,#164258),(#164259,#164260,#164261),
(#164262,#164263,#164264)),.UNSPECIFIED.,.F.,.F.,.F.)
B_SPLINE_SURFACE_WITH_KNOTS((2,1,2),(3,3),(0.,0.289681084359924,0.311483586863778),
(0.625066077454535,0.642578551421363),.UNSPECIFIED.)
GEOMETRIC_REPRESENTATION_ITEM()
RATIONAL_B_SPLINE_SURFACE(((0.990621203777021,0.993706096834649,0.999805186472059),
(0.990621203777021,0.993706096834649,0.999805186472059),(0.990621203777021,
0.993706096834649,0.999805186472059)))
REPRESENTATION_ITEM('')
SURFACE()
);
#4122=(
BOUNDED_SURFACE()
B_SPLINE_SURFACE(1,2,((#164266,#164267,#164268),(#164269,#164270,#164271),
(#164272,#164273,#164274)),.UNSPECIFIED.,.F.,.F.,.F.)
B_SPLINE_SURFACE_WITH_KNOTS((2,1,2),(3,3),(0.,0.289807040991559,0.311582168493806),
(0.0909109506295943,0.108084585199971),.UNSPECIFIED.)
GEOMETRIC_REPRESENTATION_ITEM()
RATIONAL_B_SPLINE_SURFACE(((0.990053454406147,0.987313720921968,0.987472672298934),
(0.990053454406147,0.987313720921967,0.987472672298933),(0.990053454406147,
0.987313720921967,0.987472672298933)))
REPRESENTATION_ITEM('')
SURFACE()
);
#4123=(
BOUNDED_SURFACE()
B_SPLINE_SURFACE(1,2,((#164282,#164283,#164284),(#164285,#164286,#164287),
(#164288,#164289,#164290)),.UNSPECIFIED.,.F.,.F.,.F.)
B_SPLINE_SURFACE_WITH_KNOTS((2,1,2),(3,3),(0.,0.289681084359921,0.311483587353062),
(0.625066077454535,0.642578551421364),.UNSPECIFIED.)
GEOMETRIC_REPRESENTATION_ITEM()
RATIONAL_B_SPLINE_SURFACE(((0.990621203777021,0.993706096834649,0.999805186472059),
(0.990621203777021,0.993706096834649,0.999805186472059),(0.990621203777021,
0.993706096834649,0.999805186472059)))
REPRESENTATION_ITEM('')
SURFACE()
);
#4124=(
BOUNDED_SURFACE()
B_SPLINE_SURFACE(1,2,((#164292,#164293,#164294),(#164295,#164296,#164297),
(#164298,#164299,#164300)),.UNSPECIFIED.,.F.,.F.,.F.)
B_SPLINE_SURFACE_WITH_KNOTS((2,1,2),(3,3),(0.,0.289807040991592,0.311582168185893),
(0.0909109506295943,0.108084585199971),.UNSPECIFIED.)
GEOMETRIC_REPRESENTATION_ITEM()
RATIONAL_B_SPLINE_SURFACE(((0.990053454406147,0.987313720921968,0.987472672298934),
(0.990053454406147,0.987313720921968,0.987472672298934),(0.990053454406147,
0.987313720921968,0.987472672298934)))
REPRESENTATION_ITEM('')
SURFACE()
);
#4125=(
BOUNDED_SURFACE()
B_SPLINE_SURFACE(1,2,((#164341,#164342,#164343),(#164344,#164345,#164346),
(#164347,#164348,#164349)),.UNSPECIFIED.,.F.,.F.,.F.)
B_SPLINE_SURFACE_WITH_KNOTS((2,1,2),(3,3),(0.,0.28968108435992,0.311483587308824),
(0.625066077454535,0.642578551421363),.UNSPECIFIED.)
GEOMETRIC_REPRESENTATION_ITEM()
RATIONAL_B_SPLINE_SURFACE(((0.990621203777021,0.993706096834649,0.999805186472059),
(0.990621203777021,0.993706096834649,0.999805186472059),(0.990621203777021,
0.993706096834649,0.999805186472059)))
REPRESENTATION_ITEM('')
SURFACE()
);
#4126=(
BOUNDED_SURFACE()
B_SPLINE_SURFACE(1,2,((#164351,#164352,#164353),(#164354,#164355,#164356),
(#164357,#164358,#164359)),.UNSPECIFIED.,.F.,.F.,.F.)
B_SPLINE_SURFACE_WITH_KNOTS((2,1,2),(3,3),(0.,0.289807040991593,0.311582168106922),
(0.0909109506295942,0.10808458519997),.UNSPECIFIED.)
GEOMETRIC_REPRESENTATION_ITEM()
RATIONAL_B_SPLINE_SURFACE(((0.990053454406147,0.987313720921968,0.987472672298934),
(0.990053454406147,0.987313720921968,0.987472672298934),(0.990053454406147,
0.987313720921968,0.987472672298934)))
REPRESENTATION_ITEM('')
SURFACE()
);
#4127=(
BOUNDED_SURFACE()
B_SPLINE_SURFACE(1,2,((#164400,#164401,#164402),(#164403,#164404,#164405),
(#164406,#164407,#164408)),.UNSPECIFIED.,.F.,.F.,.F.)
B_SPLINE_SURFACE_WITH_KNOTS((2,1,2),(3,3),(0.,0.289681084359921,0.31148358700348),
(0.625066077454535,0.642578551421363),.UNSPECIFIED.)
GEOMETRIC_REPRESENTATION_ITEM()
RATIONAL_B_SPLINE_SURFACE(((0.990621203777021,0.993706096834649,0.999805186472059),
(0.990621203777021,0.993706096834649,0.999805186472059),(0.990621203777021,
0.993706096834649,0.999805186472059)))
REPRESENTATION_ITEM('')
SURFACE()
);
#4128=(
BOUNDED_SURFACE()
B_SPLINE_SURFACE(1,2,((#164410,#164411,#164412),(#164413,#164414,#164415),
(#164416,#164417,#164418)),.UNSPECIFIED.,.F.,.F.,.F.)
B_SPLINE_SURFACE_WITH_KNOTS((2,1,2),(3,3),(0.,0.289807040991604,0.311582168205773),
(0.0909109506295943,0.108084585199971),.UNSPECIFIED.)
GEOMETRIC_REPRESENTATION_ITEM()
RATIONAL_B_SPLINE_SURFACE(((0.990053454406147,0.987313720921968,0.987472672298934),
(0.990053454406147,0.987313720921968,0.987472672298934),(0.990053454406147,
0.987313720921968,0.987472672298934)))
REPRESENTATION_ITEM('')
SURFACE()
);
#4129=(
BOUNDED_SURFACE()
B_SPLINE_SURFACE(1,2,((#164459,#164460,#164461),(#164462,#164463,#164464),
(#164465,#164466,#164467)),.UNSPECIFIED.,.F.,.F.,.F.)
B_SPLINE_SURFACE_WITH_KNOTS((2,1,2),(3,3),(0.,0.289681084359918,0.311483587238885),
(0.625066077454535,0.642578551421363),.UNSPECIFIED.)
GEOMETRIC_REPRESENTATION_ITEM()
RATIONAL_B_SPLINE_SURFACE(((0.990621203777021,0.993706096834649,0.999805186472059),
(0.990621203777021,0.993706096834649,0.999805186472059),(0.990621203777021,
0.993706096834649,0.999805186472059)))
REPRESENTATION_ITEM('')
SURFACE()
);
#4130=(
BOUNDED_SURFACE()
B_SPLINE_SURFACE(1,2,((#164469,#164470,#164471),(#164472,#164473,#164474),
(#164475,#164476,#164477)),.UNSPECIFIED.,.F.,.F.,.F.)
B_SPLINE_SURFACE_WITH_KNOTS((2,1,2),(3,3),(0.,0.289807040992979,0.311582168660763),
(0.0909109506295943,0.10808458519997),.UNSPECIFIED.)
GEOMETRIC_REPRESENTATION_ITEM()
RATIONAL_B_SPLINE_SURFACE(((0.990053454406147,0.987313720921968,0.987472672298934),
(0.990053454406147,0.987313720921968,0.987472672298934),(0.990053454406147,
0.987313720921968,0.987472672298934)))
REPRESENTATION_ITEM('')
SURFACE()
);
#4131=(
BOUNDED_SURFACE()
B_SPLINE_SURFACE(1,2,((#164518,#164519,#164520),(#164521,#164522,#164523),
(#164524,#164525,#164526)),.UNSPECIFIED.,.F.,.F.,.F.)
B_SPLINE_SURFACE_WITH_KNOTS((2,1,2),(3,3),(0.,0.289681084360127,0.31148358675689),
(0.625066077454535,0.642578551421363),.UNSPECIFIED.)
GEOMETRIC_REPRESENTATION_ITEM()
RATIONAL_B_SPLINE_SURFACE(((0.990621203777021,0.993706096834649,0.999805186472059),
(0.990621203777021,0.993706096834649,0.999805186472059),(0.990621203777021,
0.993706096834649,0.999805186472059)))
REPRESENTATION_ITEM('')
SURFACE()
);
#4132=(
BOUNDED_SURFACE()
B_SPLINE_SURFACE(1,2,((#164528,#164529,#164530),(#164531,#164532,#164533),
(#164534,#164535,#164536)),.UNSPECIFIED.,.F.,.F.,.F.)
B_SPLINE_SURFACE_WITH_KNOTS((2,1,2),(3,3),(0.,0.289807040991931,0.311582168479859),
(0.0909109506295922,0.108084585199971),.UNSPECIFIED.)
GEOMETRIC_REPRESENTATION_ITEM()
RATIONAL_B_SPLINE_SURFACE(((0.990053454406148,0.987313720921968,0.987472672298933),
(0.990053454406148,0.987313720921968,0.987472672298933),(0.990053454406148,
0.987313720921968,0.987472672298933)))
REPRESENTATION_ITEM('')
SURFACE()
);
#4133=(
BOUNDED_SURFACE()
B_SPLINE_SURFACE(1,2,((#164577,#164578,#164579),(#164580,#164581,#164582),
(#164583,#164584,#164585)),.UNSPECIFIED.,.F.,.F.,.F.)
B_SPLINE_SURFACE_WITH_KNOTS((2,1,2),(3,3),(0.,0.289681084359922,0.311483586918173),
(0.625066077454535,0.642578551421363),.UNSPECIFIED.)
GEOMETRIC_REPRESENTATION_ITEM()
RATIONAL_B_SPLINE_SURFACE(((0.990621203777021,0.993706096834649,0.999805186472059),
(0.990621203777021,0.993706096834649,0.999805186472059),(0.990621203777021,
0.993706096834649,0.999805186472059)))
REPRESENTATION_ITEM('')
SURFACE()
);
#4134=(
BOUNDED_SURFACE()
B_SPLINE_SURFACE(1,2,((#164587,#164588,#164589),(#164590,#164591,#164592),
(#164593,#164594,#164595)),.UNSPECIFIED.,.F.,.F.,.F.)
B_SPLINE_SURFACE_WITH_KNOTS((2,1,2),(3,3),(0.,0.289807040991561,0.311582168314643),
(0.0909109506295943,0.108084585199971),.UNSPECIFIED.)
GEOMETRIC_REPRESENTATION_ITEM()
RATIONAL_B_SPLINE_SURFACE(((0.990053454406147,0.987313720921968,0.987472672298934),
(0.990053454406147,0.987313720921968,0.987472672298934),(0.990053454406147,
0.987313720921968,0.987472672298934)))
REPRESENTATION_ITEM('')
SURFACE()
);
#4135=(
BOUNDED_SURFACE()
B_SPLINE_SURFACE(1,2,((#164636,#164637,#164638),(#164639,#164640,#164641),
(#164642,#164643,#164644)),.UNSPECIFIED.,.F.,.F.,.F.)
B_SPLINE_SURFACE_WITH_KNOTS((2,1,2),(3,3),(0.,0.289681084359922,0.311483586948988),
(0.625066077454535,0.642578551421363),.UNSPECIFIED.)
GEOMETRIC_REPRESENTATION_ITEM()
RATIONAL_B_SPLINE_SURFACE(((0.990621203777021,0.993706096834649,0.999805186472059),
(0.990621203777021,0.993706096834649,0.999805186472059),(0.990621203777021,
0.993706096834649,0.999805186472059)))
REPRESENTATION_ITEM('')
SURFACE()
);
#4136=(
BOUNDED_SURFACE()
B_SPLINE_SURFACE(1,2,((#164646,#164647,#164648),(#164649,#164650,#164651),
(#164652,#164653,#164654)),.UNSPECIFIED.,.F.,.F.,.F.)
B_SPLINE_SURFACE_WITH_KNOTS((2,1,2),(3,3),(0.,0.289807040991561,0.311582167860186),
(0.0909109506295943,0.108084585199971),.UNSPECIFIED.)
GEOMETRIC_REPRESENTATION_ITEM()
RATIONAL_B_SPLINE_SURFACE(((0.990053454406147,0.987313720921968,0.987472672298934),
(0.990053454406147,0.987313720921968,0.987472672298934),(0.990053454406147,
0.987313720921968,0.987472672298934)))
REPRESENTATION_ITEM('')
SURFACE()
);
#4137=(
BOUNDED_SURFACE()
B_SPLINE_SURFACE(1,2,((#164662,#164663,#164664),(#164665,#164666,#164667),
(#164668,#164669,#164670)),.UNSPECIFIED.,.F.,.F.,.F.)
B_SPLINE_SURFACE_WITH_KNOTS((2,1,2),(3,3),(0.,0.289681084359917,0.311483587097765),
(0.625066077454535,0.642578551421363),.UNSPECIFIED.)
GEOMETRIC_REPRESENTATION_ITEM()
RATIONAL_B_SPLINE_SURFACE(((0.990621203777021,0.993706096834649,0.999805186472059),
(0.990621203777021,0.993706096834649,0.999805186472059),(0.990621203777021,
0.993706096834649,0.999805186472059)))
REPRESENTATION_ITEM('')
SURFACE()
);
#4138=(
BOUNDED_SURFACE()
B_SPLINE_SURFACE(1,2,((#164672,#164673,#164674,#164675,#164676,#164677,
#164678),(#164679,#164680,#164681,#164682,#164683,#164684,#164685)),
 .UNSPECIFIED.,.F.,.F.,.F.)
B_SPLINE_SURFACE_WITH_KNOTS((2,2),(3,2,2,3),(0.788462675553386,1.),(0.642404283483305,
0.642578551421363,0.642857142857143,0.660005345227123),.UNSPECIFIED.)
GEOMETRIC_REPRESENTATION_ITEM()
RATIONAL_B_SPLINE_SURFACE(((0.999805186472058,0.999805186472058,0.999805186472058,
0.999902211834794,1.,0.993980822699584,0.990851751371721),(0.999805186472058,
0.999805186472058,0.999805186472058,0.999902211834794,1.,0.993980822699584,
0.990851751371721)))
REPRESENTATION_ITEM('')
SURFACE()
);
#4139=(
BOUNDED_SURFACE()
B_SPLINE_SURFACE(1,2,((#164689,#164690,#164691,#164692,#164693),(#164694,
#164695,#164696,#164697,#164698)),.UNSPECIFIED.,.F.,.F.,.F.)
B_SPLINE_SURFACE_WITH_KNOTS((2,2),(3,2,3),(0.788554614412989,1.),(0.0735508106170104,
0.0909109506295944,0.0910845520297202),.UNSPECIFIED.)
GEOMETRIC_REPRESENTATION_ITEM()
RATIONAL_B_SPLINE_SURFACE(((0.998554414400487,0.992822941359396,0.990053454406147,
0.990053454406147,0.990053454406147),(0.998554414400487,0.992822941359396,
0.990053454406147,0.990053454406147,0.990053454406147)))
REPRESENTATION_ITEM('')
SURFACE()
);
#4140=(
BOUNDED_SURFACE()
B_SPLINE_SURFACE(1,2,((#164700,#164701,#164702,#164703,#164704,#164705,
#164706),(#164707,#164708,#164709,#164710,#164711,#164712,#164713),(#164714,
#164715,#164716,#164717,#164718,#164719,#164720)),.UNSPECIFIED.,.F.,.F.,
 .F.)
B_SPLINE_SURFACE_WITH_KNOTS((2,1,2),(3,2,2,3),(0.788462675553383,1.,1.00211537324447),
(0.642404283483302,0.642578551421363,0.642857142857143,0.660005345227478),
 .UNSPECIFIED.)
GEOMETRIC_REPRESENTATION_ITEM()
RATIONAL_B_SPLINE_SURFACE(((0.999805186472058,0.999805186472058,0.999805186472058,
0.999902211834794,1.,0.993980822699459,0.990851751371591),(0.999805186472058,
0.999805186472058,0.999805186472058,0.999902211834794,1.,0.993980822699459,
0.990851751371591),(0.999805186472058,0.999805186472058,0.999805186472058,
0.999902211834794,1.,0.993980822699459,0.990851751371591)))
REPRESENTATION_ITEM('')
SURFACE()
);
#4141=(
BOUNDED_SURFACE()
B_SPLINE_SURFACE(1,2,((#164727,#164728,#164729,#164730,#164731),(#164732,
#164733,#164734,#164735,#164736)),.UNSPECIFIED.,.F.,.F.,.F.)
B_SPLINE_SURFACE_WITH_KNOTS((2,2),(3,2,3),(0.788554614412989,1.00000106324376),
(0.0735508106169813,0.0909109506295944,0.0910845520297205),
 .UNSPECIFIED.)
GEOMETRIC_REPRESENTATION_ITEM()
RATIONAL_B_SPLINE_SURFACE(((0.998554414400506,0.992822941359401,0.990053454406147,
0.990053454406147,0.990053454406147),(0.998554414400506,0.992822941359401,
0.990053454406147,0.990053454406147,0.990053454406147)))
REPRESENTATION_ITEM('')
SURFACE()
);
#4142=(
BOUNDED_SURFACE()
B_SPLINE_SURFACE(1,2,((#164738,#164739,#164740,#164741,#164742,#164743,
#164744),(#164745,#164746,#164747,#164748,#164749,#164750,#164751)),
 .UNSPECIFIED.,.F.,.F.,.F.)
B_SPLINE_SURFACE_WITH_KNOTS((2,2),(3,2,2,3),(0.78846267555338,1.),(0.642404283483302,
0.642578551421363,0.642857142857143,0.660005345227478),.UNSPECIFIED.)
GEOMETRIC_REPRESENTATION_ITEM()
RATIONAL_B_SPLINE_SURFACE(((0.999805186472058,0.999805186472058,0.999805186472058,
0.999902211834794,1.,0.993980822699459,0.990851751371591),(0.999805186472058,
0.999805186472058,0.999805186472058,0.999902211834794,1.,0.993980822699459,
0.990851751371591)))
REPRESENTATION_ITEM('')
SURFACE()
);
#4143=(
BOUNDED_SURFACE()
B_SPLINE_SURFACE(1,2,((#164755,#164756,#164757,#164758,#164759),(#164760,
#164761,#164762,#164763,#164764)),.UNSPECIFIED.,.F.,.F.,.F.)
B_SPLINE_SURFACE_WITH_KNOTS((2,2),(3,2,3),(0.788554614412984,1.00000106320563),
(0.0735508106171715,0.0909109506295945,0.0910845520297187),
 .UNSPECIFIED.)
GEOMETRIC_REPRESENTATION_ITEM()
RATIONAL_B_SPLINE_SURFACE(((0.99855441440038,0.99282294135937,0.990053454406147,
0.990053454406147,0.990053454406147),(0.99855441440038,0.99282294135937,
0.990053454406147,0.990053454406147,0.990053454406147)))
REPRESENTATION_ITEM('')
SURFACE()
);
#4144=(
BOUNDED_SURFACE()
B_SPLINE_SURFACE(1,2,((#164766,#164767,#164768,#164769,#164770,#164771,
#164772),(#164773,#164774,#164775,#164776,#164777,#164778,#164779)),
 .UNSPECIFIED.,.F.,.F.,.F.)
B_SPLINE_SURFACE_WITH_KNOTS((2,2),(3,2,2,3),(0.788462675553387,1.),(0.642404283483302,
0.642578551421363,0.642857142857143,0.660005345227478),.UNSPECIFIED.)
GEOMETRIC_REPRESENTATION_ITEM()
RATIONAL_B_SPLINE_SURFACE(((0.999805186472058,0.999805186472058,0.999805186472058,
0.999902211834794,1.,0.993980822699459,0.990851751371592),(0.999805186472058,
0.999805186472058,0.999805186472058,0.999902211834794,1.,0.993980822699459,
0.990851751371592)))
REPRESENTATION_ITEM('')
SURFACE()
);
#4145=(
BOUNDED_SURFACE()
B_SPLINE_SURFACE(1,2,((#164783,#164784,#164785,#164786,#164787),(#164788,
#164789,#164790,#164791,#164792)),.UNSPECIFIED.,.F.,.F.,.F.)
B_SPLINE_SURFACE_WITH_KNOTS((2,2),(3,2,3),(0.788554614412988,1.),(0.0735508106173321,
0.0909109506295944,0.091084552029717),.UNSPECIFIED.)
GEOMETRIC_REPRESENTATION_ITEM()
RATIONAL_B_SPLINE_SURFACE(((0.998554414400274,0.992822941359345,0.990053454406147,
0.990053454406147,0.990053454406147),(0.998554414400274,0.992822941359345,
0.990053454406147,0.990053454406147,0.990053454406147)))
REPRESENTATION_ITEM('')
SURFACE()
);
#4146=(
BOUNDED_SURFACE()
B_SPLINE_SURFACE(1,2,((#164794,#164795,#164796,#164797,#164798,#164799,
#164800),(#164801,#164802,#164803,#164804,#164805,#164806,#164807)),
 .UNSPECIFIED.,.F.,.F.,.F.)
B_SPLINE_SURFACE_WITH_KNOTS((2,2),(3,2,2,3),(0.78846267555338,1.),(0.642404283483302,
0.642578551421363,0.642857142857143,0.660005345227478),.UNSPECIFIED.)
GEOMETRIC_REPRESENTATION_ITEM()
RATIONAL_B_SPLINE_SURFACE(((0.999805186472058,0.999805186472058,0.999805186472058,
0.999902211834794,1.,0.993980822699459,0.990851751371591),(0.999805186472058,
0.999805186472058,0.999805186472058,0.999902211834794,1.,0.993980822699459,
0.990851751371591)))
REPRESENTATION_ITEM('')
SURFACE()
);
#4147=(
BOUNDED_SURFACE()
B_SPLINE_SURFACE(1,2,((#164811,#164812,#164813,#164814,#164815),(#164816,
#164817,#164818,#164819,#164820)),.UNSPECIFIED.,.F.,.F.,.F.)
B_SPLINE_SURFACE_WITH_KNOTS((2,2),(3,2,3),(0.788554614412994,1.00000106310531),
(0.073550810617453,0.0909109506295934,0.0910845520297148),.UNSPECIFIED.)
GEOMETRIC_REPRESENTATION_ITEM()
RATIONAL_B_SPLINE_SURFACE(((0.998554414400194,0.992822941359326,0.990053454406148,
0.990053454406148,0.990053454406148),(0.998554414400194,0.992822941359326,
0.990053454406148,0.990053454406148,0.990053454406148)))
REPRESENTATION_ITEM('')
SURFACE()
);
#4148=(
BOUNDED_SURFACE()
B_SPLINE_SURFACE(1,2,((#164822,#164823,#164824,#164825,#164826,#164827,
#164828),(#164829,#164830,#164831,#164832,#164833,#164834,#164835)),
 .UNSPECIFIED.,.F.,.F.,.F.)
B_SPLINE_SURFACE_WITH_KNOTS((2,2),(3,2,2,3),(0.788462675553394,1.),(0.642404283483303,
0.642578551421364,0.642857142857143,0.660005345227479),.UNSPECIFIED.)
GEOMETRIC_REPRESENTATION_ITEM()
RATIONAL_B_SPLINE_SURFACE(((0.999805186472059,0.999805186472059,0.999805186472059,
0.999902211834795,1.,0.993980822699459,0.990851751371591),(0.999805186472059,
0.999805186472059,0.999805186472059,0.999902211834795,1.,0.993980822699459,
0.990851751371591)))
REPRESENTATION_ITEM('')
SURFACE()
);
#4149=(
BOUNDED_SURFACE()
B_SPLINE_SURFACE(1,2,((#164839,#164840,#164841,#164842,#164843),(#164844,
#164845,#164846,#164847,#164848)),.UNSPECIFIED.,.F.,.F.,.F.)
B_SPLINE_SURFACE_WITH_KNOTS((2,2),(3,2,3),(0.788554614412994,1.00000106321494),
(0.0735508106174518,0.0909109506295933,0.0910845520297147),
 .UNSPECIFIED.)
GEOMETRIC_REPRESENTATION_ITEM()
RATIONAL_B_SPLINE_SURFACE(((0.998554414400195,0.992822941359326,0.990053454406148,
0.990053454406148,0.990053454406148),(0.998554414400195,0.992822941359326,
0.990053454406148,0.990053454406148,0.990053454406148)))
REPRESENTATION_ITEM('')
SURFACE()
);
#4150=(
BOUNDED_SURFACE()
B_SPLINE_SURFACE(1,2,((#164850,#164851,#164852,#164853,#164854,#164855,
#164856),(#164857,#164858,#164859,#164860,#164861,#164862,#164863)),
 .UNSPECIFIED.,.F.,.F.,.F.)
B_SPLINE_SURFACE_WITH_KNOTS((2,2),(3,2,2,3),(0.78846267555339,1.),(0.642404283483303,
0.642578551421364,0.642857142857143,0.660005345227479),.UNSPECIFIED.)
GEOMETRIC_REPRESENTATION_ITEM()
RATIONAL_B_SPLINE_SURFACE(((0.999805186472059,0.999805186472059,0.999805186472059,
0.999902211834795,1.,0.993980822699459,0.990851751371591),(0.999805186472059,
0.999805186472059,0.999805186472059,0.999902211834795,1.,0.993980822699459,
0.990851751371591)))
REPRESENTATION_ITEM('')
SURFACE()
);
#4151=(
BOUNDED_SURFACE()
B_SPLINE_SURFACE(1,2,((#164867,#164868,#164869,#164870,#164871),(#164872,
#164873,#164874,#164875,#164876)),.UNSPECIFIED.,.F.,.F.,.F.)
B_SPLINE_SURFACE_WITH_KNOTS((2,2),(3,2,3),(0.788554614412996,1.00000106338885),
(0.0735508106174519,0.0909109506295934,0.0910845520297148),
 .UNSPECIFIED.)
GEOMETRIC_REPRESENTATION_ITEM()
RATIONAL_B_SPLINE_SURFACE(((0.998554414400195,0.992822941359326,0.990053454406148,
0.990053454406148,0.990053454406148),(0.998554414400195,0.992822941359326,
0.990053454406148,0.990053454406148,0.990053454406148)))
REPRESENTATION_ITEM('')
SURFACE()
);
#4152=(
BOUNDED_SURFACE()
B_SPLINE_SURFACE(1,2,((#164878,#164879,#164880,#164881,#164882,#164883,
#164884),(#164885,#164886,#164887,#164888,#164889,#164890,#164891),(#164892,
#164893,#164894,#164895,#164896,#164897,#164898)),.UNSPECIFIED.,.F.,.F.,
 .F.)
B_SPLINE_SURFACE_WITH_KNOTS((2,1,2),(3,2,2,3),(0.788462675553393,1.,1.00211537324447),
(0.642404283483303,0.642578551421364,0.642857142857143,0.660005345227479),
 .UNSPECIFIED.)
GEOMETRIC_REPRESENTATION_ITEM()
RATIONAL_B_SPLINE_SURFACE(((0.999805186472059,0.999805186472059,0.999805186472059,
0.999902211834795,1.,0.993980822699459,0.990851751371591),(0.999805186472059,
0.999805186472059,0.999805186472059,0.999902211834795,1.,0.993980822699459,
0.990851751371591),(0.999805186472059,0.999805186472059,0.999805186472059,
0.999902211834795,1.,0.993980822699459,0.990851751371591)))
REPRESENTATION_ITEM('')
SURFACE()
);
#4153=(
BOUNDED_SURFACE()
B_SPLINE_SURFACE(1,2,((#164905,#164906,#164907,#164908,#164909),(#164910,
#164911,#164912,#164913,#164914)),.UNSPECIFIED.,.F.,.F.,.F.)
B_SPLINE_SURFACE_WITH_KNOTS((2,2),(3,2,3),(0.788554614412992,1.),(0.0735508106174519,
0.0909109506295934,0.0910845520297148),.UNSPECIFIED.)
GEOMETRIC_REPRESENTATION_ITEM()
RATIONAL_B_SPLINE_SURFACE(((0.998554414400195,0.992822941359326,0.990053454406148,
0.990053454406148,0.990053454406148),(0.998554414400195,0.992822941359326,
0.990053454406148,0.990053454406148,0.990053454406148)))
REPRESENTATION_ITEM('')
SURFACE()
);
#4154=(
BOUNDED_SURFACE()
B_SPLINE_SURFACE(1,2,((#164916,#164917,#164918,#164919,#164920,#164921,
#164922),(#164923,#164924,#164925,#164926,#164927,#164928,#164929)),
 .UNSPECIFIED.,.F.,.F.,.F.)
B_SPLINE_SURFACE_WITH_KNOTS((2,2),(3,2,2,3),(0.788462675553392,1.),(0.642404283483303,
0.642578551421364,0.642857142857143,0.660005345227479),.UNSPECIFIED.)
GEOMETRIC_REPRESENTATION_ITEM()
RATIONAL_B_SPLINE_SURFACE(((0.999805186472059,0.999805186472059,0.999805186472059,
0.999902211834795,1.,0.993980822699459,0.990851751371591),(0.999805186472059,
0.999805186472059,0.999805186472059,0.999902211834795,1.,0.993980822699459,
0.990851751371591)))
REPRESENTATION_ITEM('')
SURFACE()
);
#4155=(
BOUNDED_SURFACE()
B_SPLINE_SURFACE(1,2,((#164933,#164934,#164935,#164936,#164937),(#164938,
#164939,#164940,#164941,#164942)),.UNSPECIFIED.,.F.,.F.,.F.)
B_SPLINE_SURFACE_WITH_KNOTS((2,2),(3,2,3),(0.788554614412995,1.00000106564244),
(0.0735508106174519,0.0909109506295934,0.0910845520297148),
 .UNSPECIFIED.)
GEOMETRIC_REPRESENTATION_ITEM()
RATIONAL_B_SPLINE_SURFACE(((0.998554414400195,0.992822941359326,0.990053454406148,
0.990053454406148,0.990053454406148),(0.998554414400195,0.992822941359326,
0.990053454406148,0.990053454406148,0.990053454406148)))
REPRESENTATION_ITEM('')
SURFACE()
);
#4156=(
BOUNDED_SURFACE()
B_SPLINE_SURFACE(1,2,((#164944,#164945,#164946,#164947,#164948,#164949,
#164950),(#164951,#164952,#164953,#164954,#164955,#164956,#164957)),
 .UNSPECIFIED.,.F.,.F.,.F.)
B_SPLINE_SURFACE_WITH_KNOTS((2,2),(3,2,2,3),(0.78846267555339,1.),(0.642404283483303,
0.642578551421364,0.642857142857143,0.660005345227479),.UNSPECIFIED.)
GEOMETRIC_REPRESENTATION_ITEM()
RATIONAL_B_SPLINE_SURFACE(((0.999805186472059,0.999805186472059,0.999805186472059,
0.999902211834795,1.,0.993980822699459,0.990851751371591),(0.999805186472059,
0.999805186472059,0.999805186472059,0.999902211834795,1.,0.993980822699459,
0.990851751371591)))
REPRESENTATION_ITEM('')
SURFACE()
);
#4157=(
BOUNDED_SURFACE()
B_SPLINE_SURFACE(1,2,((#164961,#164962,#164963,#164964,#164965),(#164966,
#164967,#164968,#164969,#164970)),.UNSPECIFIED.,.F.,.F.,.F.)
B_SPLINE_SURFACE_WITH_KNOTS((2,2),(3,2,3),(0.788554614412993,1.00000106557312),
(0.0735508106174519,0.0909109506295933,0.0910845520297147),
 .UNSPECIFIED.)
GEOMETRIC_REPRESENTATION_ITEM()
RATIONAL_B_SPLINE_SURFACE(((0.998554414400195,0.992822941359326,0.990053454406148,
0.990053454406148,0.990053454406148),(0.998554414400195,0.992822941359326,
0.990053454406148,0.990053454406148,0.990053454406148)))
REPRESENTATION_ITEM('')
SURFACE()
);
#4158=(
BOUNDED_SURFACE()
B_SPLINE_SURFACE(1,2,((#164972,#164973,#164974,#164975,#164976,#164977,
#164978),(#164979,#164980,#164981,#164982,#164983,#164984,#164985)),
 .UNSPECIFIED.,.F.,.F.,.F.)
B_SPLINE_SURFACE_WITH_KNOTS((2,2),(3,2,2,3),(0.788462675553395,1.),(0.642404283483303,
0.642578551421364,0.642857142857143,0.660005345227479),.UNSPECIFIED.)
GEOMETRIC_REPRESENTATION_ITEM()
RATIONAL_B_SPLINE_SURFACE(((0.999805186472059,0.999805186472059,0.999805186472059,
0.999902211834795,1.,0.993980822699459,0.990851751371591),(0.999805186472059,
0.999805186472059,0.999805186472059,0.999902211834795,1.,0.993980822699459,
0.990851751371591)))
REPRESENTATION_ITEM('')
SURFACE()
);
#4159=(
BOUNDED_SURFACE()
B_SPLINE_SURFACE(1,2,((#164989,#164990,#164991,#164992,#164993),(#164994,
#164995,#164996,#164997,#164998)),.UNSPECIFIED.,.F.,.F.,.F.)
B_SPLINE_SURFACE_WITH_KNOTS((2,2),(3,2,3),(0.788554614412993,1.),(0.0735508106174519,
0.0909109506295934,0.0910845520297148),.UNSPECIFIED.)
GEOMETRIC_REPRESENTATION_ITEM()
RATIONAL_B_SPLINE_SURFACE(((0.998554414400195,0.992822941359326,0.990053454406147,
0.990053454406147,0.990053454406147),(0.998554414400195,0.992822941359326,
0.990053454406147,0.990053454406147,0.990053454406147)))
REPRESENTATION_ITEM('')
SURFACE()
);
#4160=(
BOUNDED_SURFACE()
B_SPLINE_SURFACE(1,2,((#165000,#165001,#165002,#165003,#165004,#165005,
#165006),(#165007,#165008,#165009,#165010,#165011,#165012,#165013)),
 .UNSPECIFIED.,.F.,.F.,.F.)
B_SPLINE_SURFACE_WITH_KNOTS((2,2),(3,2,2,3),(0.788462675553396,1.),(0.642404283483303,
0.642578551421364,0.642857142857143,0.660005345227478),.UNSPECIFIED.)
GEOMETRIC_REPRESENTATION_ITEM()
RATIONAL_B_SPLINE_SURFACE(((0.999805186472059,0.999805186472059,0.999805186472059,
0.999902211834795,1.,0.993980822699459,0.990851751371591),(0.999805186472059,
0.999805186472059,0.999805186472059,0.999902211834795,1.,0.993980822699459,
0.990851751371591)))
REPRESENTATION_ITEM('')
SURFACE()
);
#4161=(
BOUNDED_SURFACE()
B_SPLINE_SURFACE(1,2,((#165017,#165018,#165019,#165020,#165021),(#165022,
#165023,#165024,#165025,#165026)),.UNSPECIFIED.,.F.,.F.,.F.)
B_SPLINE_SURFACE_WITH_KNOTS((2,2),(3,2,3),(0.788554614412983,1.00000106566568),
(0.0735508106174511,0.0909109506295945,0.0910845520297159),
 .UNSPECIFIED.)
GEOMETRIC_REPRESENTATION_ITEM()
RATIONAL_B_SPLINE_SURFACE(((0.998554414400196,0.992822941359326,0.990053454406147,
0.990053454406147,0.990053454406147),(0.998554414400196,0.992822941359326,
0.990053454406147,0.990053454406147,0.990053454406147)))
REPRESENTATION_ITEM('')
SURFACE()
);
#4162=(
BOUNDED_SURFACE()
B_SPLINE_SURFACE(1,2,((#165028,#165029,#165030,#165031,#165032,#165033,
#165034),(#165035,#165036,#165037,#165038,#165039,#165040,#165041),(#165042,
#165043,#165044,#165045,#165046,#165047,#165048)),.UNSPECIFIED.,.F.,.F.,
 .F.)
B_SPLINE_SURFACE_WITH_KNOTS((2,1,2),(3,2,2,3),(0.788462675553396,1.,1.00211537324447),
(0.642404283483303,0.642578551421364,0.642857142857143,0.660005345227479),
 .UNSPECIFIED.)
GEOMETRIC_REPRESENTATION_ITEM()
RATIONAL_B_SPLINE_SURFACE(((0.999805186472059,0.999805186472059,0.999805186472059,
0.999902211834795,1.,0.993980822699459,0.990851751371591),(0.999805186472059,
0.999805186472059,0.999805186472059,0.999902211834795,1.,0.993980822699459,
0.990851751371591),(0.999805186472059,0.999805186472059,0.999805186472059,
0.999902211834795,1.,0.993980822699459,0.990851751371591)))
REPRESENTATION_ITEM('')
SURFACE()
);
#4163=(
BOUNDED_SURFACE()
B_SPLINE_SURFACE(1,2,((#165055,#165056,#165057,#165058,#165059),(#165060,
#165061,#165062,#165063,#165064)),.UNSPECIFIED.,.F.,.F.,.F.)
B_SPLINE_SURFACE_WITH_KNOTS((2,2),(3,2,3),(0.788554614412996,1.),(0.0735508106174261,
0.0909109506295933,0.091084552029715),.UNSPECIFIED.)
GEOMETRIC_REPRESENTATION_ITEM()
RATIONAL_B_SPLINE_SURFACE(((0.998554414400212,0.99282294135933,0.990053454406147,
0.990053454406147,0.990053454406147),(0.998554414400212,0.99282294135933,
0.990053454406147,0.990053454406147,0.990053454406147)))
REPRESENTATION_ITEM('')
SURFACE()
);
#4164=(
BOUNDED_SURFACE()
B_SPLINE_SURFACE(1,2,((#165066,#165067,#165068,#165069,#165070,#165071,
#165072),(#165073,#165074,#165075,#165076,#165077,#165078,#165079)),
 .UNSPECIFIED.,.F.,.F.,.F.)
B_SPLINE_SURFACE_WITH_KNOTS((2,2),(3,2,2,3),(0.788462675553396,1.),(0.642404283483303,
0.642578551421364,0.642857142857143,0.660005345227479),.UNSPECIFIED.)
GEOMETRIC_REPRESENTATION_ITEM()
RATIONAL_B_SPLINE_SURFACE(((0.999805186472059,0.999805186472059,0.999805186472059,
0.999902211834795,1.,0.993980822699459,0.990851751371591),(0.999805186472059,
0.999805186472059,0.999805186472059,0.999902211834795,1.,0.993980822699459,
0.990851751371591)))
REPRESENTATION_ITEM('')
SURFACE()
);
#4165=(
BOUNDED_SURFACE()
B_SPLINE_SURFACE(1,2,((#165083,#165084,#165085,#165086,#165087),(#165088,
#165089,#165090,#165091,#165092)),.UNSPECIFIED.,.F.,.F.,.F.)
B_SPLINE_SURFACE_WITH_KNOTS((2,2),(3,2,3),(0.788554614412993,1.00000106321825),
(0.0735508106174518,0.0909109506295934,0.0910845520297148),
 .UNSPECIFIED.)
GEOMETRIC_REPRESENTATION_ITEM()
RATIONAL_B_SPLINE_SURFACE(((0.998554414400195,0.992822941359326,0.990053454406148,
0.990053454406148,0.990053454406148),(0.998554414400195,0.992822941359326,
0.990053454406148,0.990053454406148,0.990053454406148)))
REPRESENTATION_ITEM('')
SURFACE()
);
#4166=(
BOUNDED_SURFACE()
B_SPLINE_SURFACE(1,2,((#165094,#165095,#165096,#165097,#165098,#165099,
#165100),(#165101,#165102,#165103,#165104,#165105,#165106,#165107)),
 .UNSPECIFIED.,.F.,.F.,.F.)
B_SPLINE_SURFACE_WITH_KNOTS((2,2),(3,2,2,3),(0.788462675553389,1.),(0.642404283483303,
0.642578551421364,0.642857142857143,0.660005345227479),.UNSPECIFIED.)
GEOMETRIC_REPRESENTATION_ITEM()
RATIONAL_B_SPLINE_SURFACE(((0.999805186472059,0.999805186472059,0.999805186472059,
0.999902211834795,1.,0.993980822699459,0.990851751371591),(0.999805186472059,
0.999805186472059,0.999805186472059,0.999902211834795,1.,0.993980822699459,
0.990851751371591)))
REPRESENTATION_ITEM('')
SURFACE()
);
#4167=(
BOUNDED_SURFACE()
B_SPLINE_SURFACE(1,2,((#165111,#165112,#165113,#165114,#165115),(#165116,
#165117,#165118,#165119,#165120)),.UNSPECIFIED.,.F.,.F.,.F.)
B_SPLINE_SURFACE_WITH_KNOTS((2,2),(3,2,3),(0.788554614412994,1.),(0.0735508106174519,
0.0909109506295933,0.0910845520297147),.UNSPECIFIED.)
GEOMETRIC_REPRESENTATION_ITEM()
RATIONAL_B_SPLINE_SURFACE(((0.998554414400195,0.992822941359326,0.990053454406147,
0.990053454406147,0.990053454406147),(0.998554414400195,0.992822941359326,
0.990053454406147,0.990053454406147,0.990053454406147)))
REPRESENTATION_ITEM('')
SURFACE()
);
#4168=(
BOUNDED_SURFACE()
B_SPLINE_SURFACE(1,2,((#165122,#165123,#165124,#165125,#165126,#165127,
#165128),(#165129,#165130,#165131,#165132,#165133,#165134,#165135),(#165136,
#165137,#165138,#165139,#165140,#165141,#165142)),.UNSPECIFIED.,.F.,.F.,
 .F.)
B_SPLINE_SURFACE_WITH_KNOTS((2,1,2),(3,2,2,3),(0.78846267555339,1.,1.00211537324447),
(0.642404283483303,0.642578551421364,0.642857142857143,0.660005345227479),
 .UNSPECIFIED.)
GEOMETRIC_REPRESENTATION_ITEM()
RATIONAL_B_SPLINE_SURFACE(((0.999805186472059,0.999805186472059,0.999805186472059,
0.999902211834795,1.,0.993980822699459,0.990851751371591),(0.999805186472059,
0.999805186472059,0.999805186472059,0.999902211834795,1.,0.993980822699459,
0.990851751371591),(0.999805186472059,0.999805186472059,0.999805186472059,
0.999902211834795,1.,0.993980822699459,0.990851751371591)))
REPRESENTATION_ITEM('')
SURFACE()
);
#4169=(
BOUNDED_SURFACE()
B_SPLINE_SURFACE(1,2,((#165149,#165150,#165151,#165152,#165153),(#165154,
#165155,#165156,#165157,#165158)),.UNSPECIFIED.,.F.,.F.,.F.)
B_SPLINE_SURFACE_WITH_KNOTS((2,2),(3,2,3),(0.788554614412998,1.),(0.0735508106174519,
0.0909109506295934,0.0910845520297148),.UNSPECIFIED.)
GEOMETRIC_REPRESENTATION_ITEM()
RATIONAL_B_SPLINE_SURFACE(((0.998554414400195,0.992822941359326,0.990053454406148,
0.990053454406148,0.990053454406148),(0.998554414400195,0.992822941359326,
0.990053454406148,0.990053454406148,0.990053454406148)))
REPRESENTATION_ITEM('')
SURFACE()
);
#4170=(
BOUNDED_SURFACE()
B_SPLINE_SURFACE(1,2,((#165160,#165161,#165162,#165163,#165164,#165165,
#165166),(#165167,#165168,#165169,#165170,#165171,#165172,#165173)),
 .UNSPECIFIED.,.F.,.F.,.F.)
B_SPLINE_SURFACE_WITH_KNOTS((2,2),(3,2,2,3),(0.788462675553395,1.),(0.642404283483303,
0.642578551421364,0.642857142857143,0.660005345227479),.UNSPECIFIED.)
GEOMETRIC_REPRESENTATION_ITEM()
RATIONAL_B_SPLINE_SURFACE(((0.999805186472059,0.999805186472059,0.999805186472059,
0.999902211834795,1.,0.993980822699459,0.990851751371591),(0.999805186472059,
0.999805186472059,0.999805186472059,0.999902211834795,1.,0.993980822699459,
0.990851751371591)))
REPRESENTATION_ITEM('')
SURFACE()
);
#4171=(
BOUNDED_SURFACE()
B_SPLINE_SURFACE(1,2,((#165177,#165178,#165179,#165180,#165181),(#165182,
#165183,#165184,#165185,#165186)),.UNSPECIFIED.,.F.,.F.,.F.)
B_SPLINE_SURFACE_WITH_KNOTS((2,2),(3,2,3),(0.78855461441299,1.),(0.0735508106174519,
0.0909109506295936,0.091084552029715),.UNSPECIFIED.)
GEOMETRIC_REPRESENTATION_ITEM()
RATIONAL_B_SPLINE_SURFACE(((0.998554414400195,0.992822941359326,0.990053454406148,
0.990053454406148,0.990053454406148),(0.998554414400195,0.992822941359326,
0.990053454406147,0.990053454406147,0.990053454406147)))
REPRESENTATION_ITEM('')
SURFACE()
);
#4172=(
BOUNDED_SURFACE()
B_SPLINE_SURFACE(1,2,((#165188,#165189,#165190,#165191,#165192,#165193,
#165194),(#165195,#165196,#165197,#165198,#165199,#165200,#165201),(#165202,
#165203,#165204,#165205,#165206,#165207,#165208)),.UNSPECIFIED.,.F.,.F.,
 .F.)
B_SPLINE_SURFACE_WITH_KNOTS((2,1,2),(3,2,2,3),(0.788462675553397,1.,1.00211537324447),
(0.642404283483303,0.642578551421364,0.642857142857143,0.660005345227478),
 .UNSPECIFIED.)
GEOMETRIC_REPRESENTATION_ITEM()
RATIONAL_B_SPLINE_SURFACE(((0.999805186472059,0.999805186472059,0.999805186472059,
0.999902211834795,1.,0.993980822699459,0.990851751371591),(0.999805186472059,
0.999805186472059,0.999805186472059,0.999902211834795,1.,0.993980822699459,
0.990851751371591),(0.999805186472059,0.999805186472059,0.999805186472059,
0.999902211834795,1.,0.993980822699459,0.990851751371591)))
REPRESENTATION_ITEM('')
SURFACE()
);
#4173=(
BOUNDED_SURFACE()
B_SPLINE_SURFACE(1,2,((#165215,#165216,#165217,#165218,#165219),(#165220,
#165221,#165222,#165223,#165224)),.UNSPECIFIED.,.F.,.F.,.F.)
B_SPLINE_SURFACE_WITH_KNOTS((2,2),(3,2,3),(0.788554614412988,1.),(0.0735508106174229,
0.0909109506295945,0.0910845520297162),.UNSPECIFIED.)
GEOMETRIC_REPRESENTATION_ITEM()
RATIONAL_B_SPLINE_SURFACE(((0.998554414400214,0.99282294135933,0.990053454406147,
0.990053454406147,0.990053454406147),(0.998554414400214,0.99282294135933,
0.990053454406147,0.990053454406147,0.990053454406147)))
REPRESENTATION_ITEM('')
SURFACE()
);
#4174=(
BOUNDED_SURFACE()
B_SPLINE_SURFACE(1,2,((#165226,#165227,#165228,#165229,#165230,#165231,
#165232),(#165233,#165234,#165235,#165236,#165237,#165238,#165239)),
 .UNSPECIFIED.,.F.,.F.,.F.)
B_SPLINE_SURFACE_WITH_KNOTS((2,2),(3,2,2,3),(0.788462675553383,1.),(0.642404283483302,
0.642578551421363,0.642857142857143,0.660005345227478),.UNSPECIFIED.)
GEOMETRIC_REPRESENTATION_ITEM()
RATIONAL_B_SPLINE_SURFACE(((0.999805186472058,0.999805186472058,0.999805186472058,
0.999902211834794,1.,0.993980822699459,0.990851751371592),(0.999805186472058,
0.999805186472058,0.999805186472058,0.999902211834794,1.,0.993980822699459,
0.990851751371592)))
REPRESENTATION_ITEM('')
SURFACE()
);
#4175=(
BOUNDED_SURFACE()
B_SPLINE_SURFACE(1,2,((#165243,#165244,#165245,#165246,#165247),(#165248,
#165249,#165250,#165251,#165252)),.UNSPECIFIED.,.F.,.F.,.F.)
B_SPLINE_SURFACE_WITH_KNOTS((2,2),(3,2,3),(0.788554614412982,1.0000010632625),
(0.0735508106174268,0.0909109506295945,0.0910845520297162),
 .UNSPECIFIED.)
GEOMETRIC_REPRESENTATION_ITEM()
RATIONAL_B_SPLINE_SURFACE(((0.998554414400211,0.99282294135933,0.990053454406147,
0.990053454406147,0.990053454406147),(0.998554414400211,0.99282294135933,
0.990053454406147,0.990053454406147,0.990053454406147)))
REPRESENTATION_ITEM('')
SURFACE()
);
#4176=(
BOUNDED_SURFACE()
B_SPLINE_SURFACE(1,2,((#165254,#165255,#165256,#165257,#165258,#165259,
#165260),(#165261,#165262,#165263,#165264,#165265,#165266,#165267)),
 .UNSPECIFIED.,.F.,.F.,.F.)
B_SPLINE_SURFACE_WITH_KNOTS((2,2),(3,2,2,3),(0.788462675553384,1.),(0.642404283483302,
0.642578551421363,0.642857142857143,0.660005345227479),.UNSPECIFIED.)
GEOMETRIC_REPRESENTATION_ITEM()
RATIONAL_B_SPLINE_SURFACE(((0.999805186472058,0.999805186472058,0.999805186472058,
0.999902211834794,1.,0.993980822699459,0.990851751371591),(0.999805186472058,
0.999805186472058,0.999805186472058,0.999902211834794,1.,0.993980822699459,
0.990851751371591)))
REPRESENTATION_ITEM('')
SURFACE()
);
#4177=(
BOUNDED_SURFACE()
B_SPLINE_SURFACE(1,2,((#165271,#165272,#165273,#165274,#165275),(#165276,
#165277,#165278,#165279,#165280)),.UNSPECIFIED.,.F.,.F.,.F.)
B_SPLINE_SURFACE_WITH_KNOTS((2,2),(3,2,3),(0.788554614412984,1.00000106568131),
(0.0735508106174531,0.0909109506295944,0.0910845520297158),
 .UNSPECIFIED.)
GEOMETRIC_REPRESENTATION_ITEM()
RATIONAL_B_SPLINE_SURFACE(((0.998554414400194,0.992822941359325,0.990053454406147,
0.990053454406147,0.990053454406147),(0.998554414400194,0.992822941359325,
0.990053454406147,0.990053454406147,0.990053454406147)))
REPRESENTATION_ITEM('')
SURFACE()
);
#4178=(
BOUNDED_SURFACE()
B_SPLINE_SURFACE(1,2,((#165282,#165283,#165284,#165285,#165286,#165287,
#165288),(#165289,#165290,#165291,#165292,#165293,#165294,#165295),(#165296,
#165297,#165298,#165299,#165300,#165301,#165302)),.UNSPECIFIED.,.F.,.F.,
 .F.)
B_SPLINE_SURFACE_WITH_KNOTS((2,1,2),(3,2,2,3),(0.788462675553387,1.,1.00211537324447),
(0.642404283483302,0.642578551421363,0.642857142857143,0.660005345227478),
 .UNSPECIFIED.)
GEOMETRIC_REPRESENTATION_ITEM()
RATIONAL_B_SPLINE_SURFACE(((0.999805186472058,0.999805186472058,0.999805186472058,
0.999902211834794,1.,0.993980822699459,0.990851751371591),(0.999805186472058,
0.999805186472058,0.999805186472058,0.999902211834794,1.,0.993980822699459,
0.990851751371591),(0.999805186472058,0.999805186472058,0.999805186472058,
0.999902211834794,1.,0.993980822699459,0.990851751371591)))
REPRESENTATION_ITEM('')
SURFACE()
);
#4179=(
BOUNDED_SURFACE()
B_SPLINE_SURFACE(1,2,((#165309,#165310,#165311,#165312,#165313),(#165314,
#165315,#165316,#165317,#165318)),.UNSPECIFIED.,.F.,.F.,.F.)
B_SPLINE_SURFACE_WITH_KNOTS((2,2),(3,2,3),(0.788554614412982,1.),(0.073550810617453,
0.0909109506295945,0.0910845520297159),.UNSPECIFIED.)
GEOMETRIC_REPRESENTATION_ITEM()
RATIONAL_B_SPLINE_SURFACE(((0.998554414400194,0.992822941359326,0.990053454406147,
0.990053454406147,0.990053454406147),(0.998554414400194,0.992822941359326,
0.990053454406147,0.990053454406147,0.990053454406147)))
REPRESENTATION_ITEM('')
SURFACE()
);
#4180=(
BOUNDED_SURFACE()
B_SPLINE_SURFACE(1,2,((#165320,#165321,#165322,#165323,#165324,#165325,
#165326),(#165327,#165328,#165329,#165330,#165331,#165332,#165333),(#165334,
#165335,#165336,#165337,#165338,#165339,#165340)),.UNSPECIFIED.,.F.,.F.,
 .F.)
B_SPLINE_SURFACE_WITH_KNOTS((2,1,2),(3,2,2,3),(0.788462675553383,1.,1.00211537324447),
(0.642404283483302,0.642578551421363,0.642857142857143,0.660005345227478),
 .UNSPECIFIED.)
GEOMETRIC_REPRESENTATION_ITEM()
RATIONAL_B_SPLINE_SURFACE(((0.999805186472058,0.999805186472058,0.999805186472058,
0.999902211834794,1.,0.993980822699459,0.990851751371591),(0.999805186472058,
0.999805186472058,0.999805186472058,0.999902211834794,1.,0.993980822699459,
0.990851751371591),(0.999805186472058,0.999805186472058,0.999805186472058,
0.999902211834794,1.,0.993980822699459,0.990851751371591)))
REPRESENTATION_ITEM('')
SURFACE()
);
#4181=(
BOUNDED_SURFACE()
B_SPLINE_SURFACE(1,2,((#165347,#165348,#165349,#165350,#165351),(#165352,
#165353,#165354,#165355,#165356)),.UNSPECIFIED.,.F.,.F.,.F.)
B_SPLINE_SURFACE_WITH_KNOTS((2,2),(3,2,3),(0.78855461441298,1.),(0.0735508106173347,
0.0909109506295947,0.0910845520297173),.UNSPECIFIED.)
GEOMETRIC_REPRESENTATION_ITEM()
RATIONAL_B_SPLINE_SURFACE(((0.998554414400272,0.992822941359344,0.990053454406147,
0.990053454406147,0.990053454406147),(0.998554414400272,0.992822941359344,
0.990053454406147,0.990053454406147,0.990053454406147)))
REPRESENTATION_ITEM('')
SURFACE()
);
#4182=(
BOUNDED_SURFACE()
B_SPLINE_SURFACE(1,2,((#165358,#165359,#165360,#165361,#165362,#165363,
#165364),(#165365,#165366,#165367,#165368,#165369,#165370,#165371)),
 .UNSPECIFIED.,.F.,.F.,.F.)
B_SPLINE_SURFACE_WITH_KNOTS((2,2),(3,2,2,3),(0.788462675553384,1.),(0.642404283483302,
0.642578551421363,0.642857142857143,0.660005345227478),.UNSPECIFIED.)
GEOMETRIC_REPRESENTATION_ITEM()
RATIONAL_B_SPLINE_SURFACE(((0.999805186472059,0.999805186472059,0.999805186472059,
0.999902211834794,1.,0.993980822699459,0.990851751371591),(0.999805186472059,
0.999805186472059,0.999805186472059,0.999902211834794,1.,0.993980822699459,
0.990851751371591)))
REPRESENTATION_ITEM('')
SURFACE()
);
#4183=(
BOUNDED_SURFACE()
B_SPLINE_SURFACE(1,2,((#165375,#165376,#165377,#165378,#165379),(#165380,
#165381,#165382,#165383,#165384)),.UNSPECIFIED.,.F.,.F.,.F.)
B_SPLINE_SURFACE_WITH_KNOTS((2,2),(3,2,3),(0.788554614412986,1.),(0.073550810617453,
0.0909109506295945,0.0910845520297159),.UNSPECIFIED.)
GEOMETRIC_REPRESENTATION_ITEM()
RATIONAL_B_SPLINE_SURFACE(((0.998554414400194,0.992822941359325,0.990053454406147,
0.990053454406147,0.990053454406147),(0.998554414400194,0.992822941359325,
0.990053454406147,0.990053454406147,0.990053454406147)))
REPRESENTATION_ITEM('')
SURFACE()
);
#4184=(
BOUNDED_SURFACE()
B_SPLINE_SURFACE(1,2,((#165386,#165387,#165388,#165389,#165390,#165391,
#165392),(#165393,#165394,#165395,#165396,#165397,#165398,#165399)),
 .UNSPECIFIED.,.F.,.F.,.F.)
B_SPLINE_SURFACE_WITH_KNOTS((2,2),(3,2,2,3),(0.788462675553381,1.),(0.642404283483302,
0.642578551421363,0.642857142857143,0.660005345227479),.UNSPECIFIED.)
GEOMETRIC_REPRESENTATION_ITEM()
RATIONAL_B_SPLINE_SURFACE(((0.999805186472058,0.999805186472058,0.999805186472058,
0.999902211834794,1.,0.993980822699459,0.990851751371591),(0.999805186472058,
0.999805186472058,0.999805186472058,0.999902211834794,1.,0.993980822699459,
0.990851751371591)))
REPRESENTATION_ITEM('')
SURFACE()
);
#4185=(
BOUNDED_SURFACE()
B_SPLINE_SURFACE(1,2,((#165403,#165404,#165405,#165406,#165407),(#165408,
#165409,#165410,#165411,#165412)),.UNSPECIFIED.,.F.,.F.,.F.)
B_SPLINE_SURFACE_WITH_KNOTS((2,2),(3,2,3),(0.788554614412988,1.00000106334399),
(0.0735508106174531,0.0909109506295945,0.0910845520297159),
 .UNSPECIFIED.)
GEOMETRIC_REPRESENTATION_ITEM()
RATIONAL_B_SPLINE_SURFACE(((0.998554414400194,0.992822941359326,0.990053454406147,
0.990053454406147,0.990053454406147),(0.998554414400194,0.992822941359326,
0.990053454406147,0.990053454406147,0.990053454406147)))
REPRESENTATION_ITEM('')
SURFACE()
);
#4186=(
BOUNDED_SURFACE()
B_SPLINE_SURFACE(1,2,((#165414,#165415,#165416,#165417,#165418,#165419,
#165420),(#165421,#165422,#165423,#165424,#165425,#165426,#165427)),
 .UNSPECIFIED.,.F.,.F.,.F.)
B_SPLINE_SURFACE_WITH_KNOTS((2,2),(3,2,2,3),(0.788462675553238,1.),(0.642404283483285,
0.642578551421346,0.642857142857143,0.660005345227478),.UNSPECIFIED.)
GEOMETRIC_REPRESENTATION_ITEM()
RATIONAL_B_SPLINE_SURFACE(((0.999805186472047,0.999805186472047,0.999805186472047,
0.999902211834788,1.,0.993980822699459,0.990851751371591),(0.999805186472047,
0.999805186472047,0.999805186472047,0.999902211834788,1.,0.993980822699459,
0.990851751371591)))
REPRESENTATION_ITEM('')
SURFACE()
);
#4187=(
BOUNDED_SURFACE()
B_SPLINE_SURFACE(1,2,((#165431,#165432,#165433,#165434,#165435),(#165436,
#165437,#165438,#165439,#165440)),.UNSPECIFIED.,.F.,.F.,.F.)
B_SPLINE_SURFACE_WITH_KNOTS((2,2),(3,2,3),(0.788554614412988,1.00000106562849),
(0.073550810617453,0.0909109506295944,0.0910845520297158),.UNSPECIFIED.)
GEOMETRIC_REPRESENTATION_ITEM()
RATIONAL_B_SPLINE_SURFACE(((0.998554414400194,0.992822941359325,0.990053454406147,
0.990053454406147,0.990053454406147),(0.998554414400194,0.992822941359325,
0.990053454406147,0.990053454406147,0.990053454406147)))
REPRESENTATION_ITEM('')
SURFACE()
);
#4188=(
BOUNDED_SURFACE()
B_SPLINE_SURFACE(1,2,((#165442,#165443,#165444,#165445,#165446,#165447,
#165448),(#165449,#165450,#165451,#165452,#165453,#165454,#165455)),
 .UNSPECIFIED.,.F.,.F.,.F.)
B_SPLINE_SURFACE_WITH_KNOTS((2,2),(3,2,2,3),(0.788462675553159,1.),(0.642404283483276,
0.642578551421337,0.642857142857143,0.660005345227478),.UNSPECIFIED.)
GEOMETRIC_REPRESENTATION_ITEM()
RATIONAL_B_SPLINE_SURFACE(((0.99980518647204,0.99980518647204,0.99980518647204,
0.999902211834785,1.,0.993980822699459,0.990851751371591),(0.99980518647204,
0.99980518647204,0.99980518647204,0.999902211834785,1.,0.993980822699459,
0.990851751371591)))
REPRESENTATION_ITEM('')
SURFACE()
);
#4189=(
BOUNDED_SURFACE()
B_SPLINE_SURFACE(1,2,((#165459,#165460,#165461,#165462,#165463),(#165464,
#165465,#165466,#165467,#165468)),.UNSPECIFIED.,.F.,.F.,.F.)
B_SPLINE_SURFACE_WITH_KNOTS((2,2),(3,2,3),(0.788554614412984,1.00000106325674),
(0.0735508106174531,0.0909109506295946,0.091084552029716),.UNSPECIFIED.)
GEOMETRIC_REPRESENTATION_ITEM()
RATIONAL_B_SPLINE_SURFACE(((0.998554414400194,0.992822941359325,0.990053454406147,
0.990053454406147,0.990053454406147),(0.998554414400194,0.992822941359325,
0.990053454406147,0.990053454406147,0.990053454406147)))
REPRESENTATION_ITEM('')
SURFACE()
);
#4190=(
BOUNDED_SURFACE()
B_SPLINE_SURFACE(1,2,((#165470,#165471,#165472,#165473,#165474,#165475,
#165476),(#165477,#165478,#165479,#165480,#165481,#165482,#165483)),
 .UNSPECIFIED.,.F.,.F.,.F.)
B_SPLINE_SURFACE_WITH_KNOTS((2,2),(3,2,2,3),(0.788462675553045,1.),(0.642404283483262,
0.642578551421323,0.642857142857143,0.660005345227478),.UNSPECIFIED.)
GEOMETRIC_REPRESENTATION_ITEM()
RATIONAL_B_SPLINE_SURFACE(((0.999805186472031,0.999805186472031,0.999805186472031,
0.99990221183478,1.,0.993980822699459,0.990851751371591),(0.999805186472031,
0.999805186472031,0.999805186472031,0.99990221183478,1.,0.993980822699459,
0.990851751371591)))
REPRESENTATION_ITEM('')
SURFACE()
);
#4191=(
BOUNDED_SURFACE()
B_SPLINE_SURFACE(1,2,((#165487,#165488,#165489,#165490,#165491),(#165492,
#165493,#165494,#165495,#165496)),.UNSPECIFIED.,.F.,.F.,.F.)
B_SPLINE_SURFACE_WITH_KNOTS((2,2),(3,2,3),(0.788554614412981,1.00000106317919),
(0.073550810617453,0.0909109506295945,0.0910845520297159),.UNSPECIFIED.)
GEOMETRIC_REPRESENTATION_ITEM()
RATIONAL_B_SPLINE_SURFACE(((0.998554414400194,0.992822941359325,0.990053454406147,
0.990053454406147,0.990053454406147),(0.998554414400194,0.992822941359325,
0.990053454406147,0.990053454406147,0.990053454406147)))
REPRESENTATION_ITEM('')
SURFACE()
);
#4192=(
BOUNDED_SURFACE()
B_SPLINE_SURFACE(1,2,((#165498,#165499,#165500,#165501,#165502,#165503,
#165504),(#165505,#165506,#165507,#165508,#165509,#165510,#165511)),
 .UNSPECIFIED.,.F.,.F.,.F.)
B_SPLINE_SURFACE_WITH_KNOTS((2,2),(3,2,2,3),(0.788462675552883,1.),(0.642404283483242,
0.642578551421304,0.642857142857143,0.660005345227478),.UNSPECIFIED.)
GEOMETRIC_REPRESENTATION_ITEM()
RATIONAL_B_SPLINE_SURFACE(((0.999805186472017,0.999805186472017,0.999805186472017,
0.999902211834774,1.,0.993980822699459,0.990851751371591),(0.999805186472017,
0.999805186472017,0.999805186472017,0.999902211834774,1.,0.993980822699459,
0.990851751371591)))
REPRESENTATION_ITEM('')
SURFACE()
);
#4193=(
BOUNDED_SURFACE()
B_SPLINE_SURFACE(1,2,((#165515,#165516,#165517,#165518,#165519),(#165520,
#165521,#165522,#165523,#165524)),.UNSPECIFIED.,.F.,.F.,.F.)
B_SPLINE_SURFACE_WITH_KNOTS((2,2),(3,2,3),(0.788554614412985,1.00000106576408),
(0.073550810617453,0.0909109506295944,0.0910845520297158),.UNSPECIFIED.)
GEOMETRIC_REPRESENTATION_ITEM()
RATIONAL_B_SPLINE_SURFACE(((0.998554414400194,0.992822941359326,0.990053454406147,
0.990053454406147,0.990053454406147),(0.998554414400194,0.992822941359326,
0.990053454406147,0.990053454406147,0.990053454406147)))
REPRESENTATION_ITEM('')
SURFACE()
);
#4194=(
BOUNDED_SURFACE()
B_SPLINE_SURFACE(1,2,((#165526,#165527,#165528,#165529,#165530,#165531,
#165532),(#165533,#165534,#165535,#165536,#165537,#165538,#165539)),
 .UNSPECIFIED.,.F.,.F.,.F.)
B_SPLINE_SURFACE_WITH_KNOTS((2,2),(3,2,2,3),(0.788462675552653,1.),(0.642404283483215,
0.642578551421277,0.642857142857143,0.660005345227479),.UNSPECIFIED.)
GEOMETRIC_REPRESENTATION_ITEM()
RATIONAL_B_SPLINE_SURFACE(((0.999805186471999,0.999805186471999,0.999805186471999,
0.999902211834764,1.,0.993980822699459,0.990851751371591),(0.999805186471999,
0.999805186471999,0.999805186471999,0.999902211834764,1.,0.993980822699459,
0.990851751371591)))
REPRESENTATION_ITEM('')
SURFACE()
);
#4195=(
BOUNDED_SURFACE()
B_SPLINE_SURFACE(1,2,((#165543,#165544,#165545,#165546,#165547),(#165548,
#165549,#165550,#165551,#165552),(#165553,#165554,#165555,#165556,#165557)),
 .UNSPECIFIED.,.F.,.F.,.F.)
B_SPLINE_SURFACE_WITH_KNOTS((2,1,2),(3,2,3),(0.776713355992017,0.788554614412987,
1.),(0.073550810617453,0.0909109506295944,0.0910845520297158),
 .UNSPECIFIED.)
GEOMETRIC_REPRESENTATION_ITEM()
RATIONAL_B_SPLINE_SURFACE(((0.998554414400194,0.992822941359326,0.990053454406147,
0.990053454406147,0.990053454406147),(0.998554414400194,0.992822941359326,
0.990053454406147,0.990053454406147,0.990053454406147),(0.998554414400194,
0.992822941359326,0.990053454406147,0.990053454406147,0.990053454406147)))
REPRESENTATION_ITEM('')
SURFACE()
);
#4196=(
BOUNDED_SURFACE()
B_SPLINE_SURFACE(1,2,((#165560,#165561,#165562,#165563,#165564),(#165565,
#165566,#165567,#165568,#165569)),.UNSPECIFIED.,.F.,.F.,.F.)
B_SPLINE_SURFACE_WITH_KNOTS((2,2),(3,2,3),(0.,0.182805892339156),(0.642474614281366,
0.642857142857143,0.659901408087481),.UNSPECIFIED.)
GEOMETRIC_REPRESENTATION_ITEM()
RATIONAL_B_SPLINE_SURFACE(((0.999732896029237,0.999865728939372,1.,0.994017305594881,
0.990889788836284),(0.999732896029237,0.999865728939372,1.,0.994017305594881,
0.990889788836284)))
REPRESENTATION_ITEM('')
SURFACE()
);
#4197=(
BOUNDED_SURFACE()
B_SPLINE_SURFACE(1,2,((#165581,#165582,#165583,#165584,#165585),(#165586,
#165587,#165588,#165589,#165590)),.UNSPECIFIED.,.F.,.F.,.F.)
B_SPLINE_SURFACE_WITH_KNOTS((2,2),(3,2,3),(0.938576859128175,1.),(0.0665257254736565,
0.0714285714285714,0.0736543502199111),.UNSPECIFIED.)
GEOMETRIC_REPRESENTATION_ITEM()
RATIONAL_B_SPLINE_SURFACE(((0.996794362316492,0.998279055819231,1.,0.999218731101516,
0.99848615229188),(0.996794362316492,0.998279055819231,1.,0.999218731101516,
0.99848615229188)))
REPRESENTATION_ITEM('')
SURFACE()
);
#4198=(
BOUNDED_SURFACE()
B_SPLINE_SURFACE(1,2,((#165598,#165599,#165600,#165601,#165602),(#165603,
#165604,#165605,#165606,#165607)),.UNSPECIFIED.,.F.,.F.,.F.)
B_SPLINE_SURFACE_WITH_KNOTS((2,2),(3,2,3),(0.,0.0529045403781329),(0.0665257254736577,
0.0714285714285714,0.0736968668682836),.UNSPECIFIED.)
GEOMETRIC_REPRESENTATION_ITEM()
RATIONAL_B_SPLINE_SURFACE(((0.996794362316492,0.998279055819232,1.,0.999203807365532,
0.998458182734476),(0.996794362316492,0.998279055819232,1.,0.999203807365532,
0.998458182734476)))
REPRESENTATION_ITEM('')
SURFACE()
);
#4199=(
BOUNDED_SURFACE()
B_SPLINE_SURFACE(1,2,((#165618,#165619,#165620),(#165621,#165622,#165623)),
 .UNSPECIFIED.,.F.,.F.,.F.)
B_SPLINE_SURFACE_WITH_KNOTS((2,2),(3,3),(0.,0.052881546879832),(0.659860018385301,
0.666841081426899),.UNSPECIFIED.)
GEOMETRIC_REPRESENTATION_ITEM()
RATIONAL_B_SPLINE_SURFACE(((0.990904995179465,0.989621173673398,0.988816334712145),
(0.990904995179465,0.989621173673398,0.988816334712145)))
REPRESENTATION_ITEM('')
SURFACE()
);
#4200=(
BOUNDED_SURFACE()
B_SPLINE_SURFACE(1,2,((#165625,#165626,#165627,#165628,#165629),(#165630,
#165631,#165632,#165633,#165634)),.UNSPECIFIED.,.F.,.F.,.F.)
B_SPLINE_SURFACE_WITH_KNOTS((2,2),(3,2,3),(0.938550151644316,1.0000100824887),
(0.65983201135371,0.659901408087108,0.666841081426899),.UNSPECIFIED.)
GEOMETRIC_REPRESENTATION_ITEM()
RATIONAL_B_SPLINE_SURFACE(((0.990889788836421,0.990889788836421,0.990889788836421,
0.989616401900903,0.988816334712145),(0.990889788836421,0.990889788836421,
0.990889788836421,0.989616401900903,0.988816334712145)))
REPRESENTATION_ITEM('')
SURFACE()
);
#4201=(
BOUNDED_SURFACE()
B_SPLINE_SURFACE(1,2,((#165636,#165637,#165638,#165639,#165640),(#165641,
#165642,#165643,#165644,#165645)),.UNSPECIFIED.,.F.,.F.,.F.)
B_SPLINE_SURFACE_WITH_KNOTS((2,2),(3,2,3),(0.,0.182885378421189),(0.0734807488194108,
0.073654350219536,0.0910144902320546),.UNSPECIFIED.)
GEOMETRIC_REPRESENTATION_ITEM()
RATIONAL_B_SPLINE_SURFACE(((0.998486152292127,0.998486152292127,0.998486152292127,
0.99277234517207,0.990020524139832),(0.998486152292127,0.998486152292127,
0.998486152292127,0.99277234517207,0.990020524139832)))
REPRESENTATION_ITEM('')
SURFACE()
);
#4202=(
BOUNDED_SURFACE()
B_SPLINE_SURFACE(1,2,((#165656,#165657,#165658,#165659,#165660),(#165661,
#165662,#165663,#165664,#165665)),.UNSPECIFIED.,.F.,.F.,.F.)
B_SPLINE_SURFACE_WITH_KNOTS((2,2),(3,2,3),(0.,0.182805892339158),(0.642474614281361,
0.642857142857143,0.659901408087481),.UNSPECIFIED.)
GEOMETRIC_REPRESENTATION_ITEM()
RATIONAL_B_SPLINE_SURFACE(((0.999732896029233,0.99986572893937,1.,0.994017305594881,
0.990889788836284),(0.999732896029233,0.99986572893937,1.,0.994017305594881,
0.990889788836284)))
REPRESENTATION_ITEM('')
SURFACE()
);
#4203=(
BOUNDED_SURFACE()
B_SPLINE_SURFACE(1,2,((#165667,#165668,#165669,#165670,#165671),(#165672,
#165673,#165674,#165675,#165676)),.UNSPECIFIED.,.F.,.F.,.F.)
B_SPLINE_SURFACE_WITH_KNOTS((2,2),(3,2,3),(0.938576859128175,1.),(0.0665257254736565,
0.0714285714285714,0.0736543502199112),.UNSPECIFIED.)
GEOMETRIC_REPRESENTATION_ITEM()
RATIONAL_B_SPLINE_SURFACE(((0.996794362316492,0.998279055819231,1.,0.999218731101516,
0.99848615229188),(0.996794362316492,0.998279055819231,1.,0.999218731101516,
0.99848615229188)))
REPRESENTATION_ITEM('')
SURFACE()
);
#4204=(
BOUNDED_SURFACE()
B_SPLINE_SURFACE(1,2,((#165684,#165685,#165686,#165687,#165688),(#165689,
#165690,#165691,#165692,#165693)),.UNSPECIFIED.,.F.,.F.,.F.)
B_SPLINE_SURFACE_WITH_KNOTS((2,2),(3,2,3),(0.,0.052904540378128),(0.0665257254736564,
0.0714285714285714,0.0736968668684972),.UNSPECIFIED.)
GEOMETRIC_REPRESENTATION_ITEM()
RATIONAL_B_SPLINE_SURFACE(((0.996794362316492,0.998279055819231,1.,0.999203807365457,
0.998458182734336),(0.996794362316492,0.998279055819231,1.,0.999203807365457,
0.998458182734336)))
REPRESENTATION_ITEM('')
SURFACE()
);
#4205=(
BOUNDED_SURFACE()
B_SPLINE_SURFACE(1,2,((#165704,#165705,#165706),(#165707,#165708,#165709)),
 .UNSPECIFIED.,.F.,.F.,.F.)
B_SPLINE_SURFACE_WITH_KNOTS((2,2),(3,3),(0.,0.0528815468798315),(0.659860018385656,
0.666841081426896),.UNSPECIFIED.)
GEOMETRIC_REPRESENTATION_ITEM()
RATIONAL_B_SPLINE_SURFACE(((0.990904995179334,0.989621173673357,0.988816334712145),
(0.990904995179334,0.989621173673357,0.988816334712145)))
REPRESENTATION_ITEM('')
SURFACE()
);
#4206=(
BOUNDED_SURFACE()
B_SPLINE_SURFACE(1,2,((#165711,#165712,#165713,#165714,#165715),(#165716,
#165717,#165718,#165719,#165720)),.UNSPECIFIED.,.F.,.F.,.F.)
B_SPLINE_SURFACE_WITH_KNOTS((2,2),(3,2,3),(0.938550151647612,1.00001008246538),
(0.659832011354087,0.659901408087481,0.666841081426897),.UNSPECIFIED.)
GEOMETRIC_REPRESENTATION_ITEM()
RATIONAL_B_SPLINE_SURFACE(((0.990889788836284,0.990889788836284,0.990889788836284,
0.98961640190086,0.988816334712146),(0.990889788836284,0.990889788836284,
0.990889788836284,0.98961640190086,0.988816334712146)))
REPRESENTATION_ITEM('')
SURFACE()
);
#4207=(
BOUNDED_SURFACE()
B_SPLINE_SURFACE(1,2,((#165722,#165723,#165724,#165725,#165726),(#165727,
#165728,#165729,#165730,#165731)),.UNSPECIFIED.,.F.,.F.,.F.)
B_SPLINE_SURFACE_WITH_KNOTS((2,2),(3,2,3),(-1.0691269832958E-6,0.182885378421193),
(0.0734807488197898,0.0736543502199112,0.0910144902320524),
 .UNSPECIFIED.)
GEOMETRIC_REPRESENTATION_ITEM()
RATIONAL_B_SPLINE_SURFACE(((0.99848615229188,0.99848615229188,0.99848615229188,
0.992772345172011,0.990020524139833),(0.99848615229188,0.99848615229188,
0.99848615229188,0.992772345172011,0.990020524139833)))
REPRESENTATION_ITEM('')
SURFACE()
);
#4208=(
BOUNDED_SURFACE()
B_SPLINE_SURFACE(1,2,((#165742,#165743,#165744,#165745,#165746),(#165747,
#165748,#165749,#165750,#165751)),.UNSPECIFIED.,.F.,.F.,.F.)
B_SPLINE_SURFACE_WITH_KNOTS((2,2),(3,2,3),(0.,0.18280589233916),(0.642474614281366,
0.642857142857143,0.659901408087481),.UNSPECIFIED.)
GEOMETRIC_REPRESENTATION_ITEM()
RATIONAL_B_SPLINE_SURFACE(((0.999732896029237,0.999865728939372,1.,0.994017305594881,
0.990889788836284),(0.999732896029237,0.999865728939372,1.,0.994017305594881,
0.990889788836284)))
REPRESENTATION_ITEM('')
SURFACE()
);
#4209=(
BOUNDED_SURFACE()
B_SPLINE_SURFACE(1,2,((#165753,#165754,#165755,#165756,#165757),(#165758,
#165759,#165760,#165761,#165762)),.UNSPECIFIED.,.F.,.F.,.F.)
B_SPLINE_SURFACE_WITH_KNOTS((2,2),(3,2,3),(0.938576859128171,1.),(0.0665257254736565,
0.0714285714285714,0.0736543502199113),.UNSPECIFIED.)
GEOMETRIC_REPRESENTATION_ITEM()
RATIONAL_B_SPLINE_SURFACE(((0.996794362316492,0.998279055819231,1.,0.999218731101516,
0.99848615229188),(0.996794362316492,0.998279055819231,1.,0.999218731101516,
0.99848615229188)))
REPRESENTATION_ITEM('')
SURFACE()
);
#4210=(
BOUNDED_SURFACE()
B_SPLINE_SURFACE(1,2,((#165770,#165771,#165772,#165773,#165774),(#165775,
#165776,#165777,#165778,#165779)),.UNSPECIFIED.,.F.,.F.,.F.)
B_SPLINE_SURFACE_WITH_KNOTS((2,2),(3,2,3),(0.,0.0529045403781295),(0.0665257254736562,
0.0714285714285714,0.0736968668684972),.UNSPECIFIED.)
GEOMETRIC_REPRESENTATION_ITEM()
RATIONAL_B_SPLINE_SURFACE(((0.996794362316491,0.998279055819231,1.,0.999203807365457,
0.998458182734336),(0.996794362316491,0.998279055819231,1.,0.999203807365457,
0.998458182734336)))
REPRESENTATION_ITEM('')
SURFACE()
);
#4211=(
BOUNDED_SURFACE()
B_SPLINE_SURFACE(1,2,((#165790,#165791,#165792),(#165793,#165794,#165795)),
 .UNSPECIFIED.,.F.,.F.,.F.)
B_SPLINE_SURFACE_WITH_KNOTS((2,2),(3,3),(0.,0.0528815468798302),(0.659860018385514,
0.666841081426898),.UNSPECIFIED.)
GEOMETRIC_REPRESENTATION_ITEM()
RATIONAL_B_SPLINE_SURFACE(((0.990904995179386,0.989621173673374,0.988816334712145),
(0.990904995179386,0.989621173673374,0.988816334712145)))
REPRESENTATION_ITEM('')
SURFACE()
);
#4212=(
BOUNDED_SURFACE()
B_SPLINE_SURFACE(1,2,((#165797,#165798,#165799,#165800,#165801),(#165802,
#165803,#165804,#165805,#165806)),.UNSPECIFIED.,.F.,.F.,.F.)
B_SPLINE_SURFACE_WITH_KNOTS((2,2),(3,2,3),(0.93855015164761,1.00001008255567),
(0.659832011354087,0.659901408087481,0.666841081426897),.UNSPECIFIED.)
GEOMETRIC_REPRESENTATION_ITEM()
RATIONAL_B_SPLINE_SURFACE(((0.990889788836284,0.990889788836284,0.990889788836284,
0.98961640190086,0.988816334712146),(0.990889788836284,0.990889788836284,
0.990889788836284,0.98961640190086,0.988816334712146)))
REPRESENTATION_ITEM('')
SURFACE()
);
#4213=(
BOUNDED_SURFACE()
B_SPLINE_SURFACE(1,2,((#165808,#165809,#165810,#165811,#165812),(#165813,
#165814,#165815,#165816,#165817)),.UNSPECIFIED.,.F.,.F.,.F.)
B_SPLINE_SURFACE_WITH_KNOTS((2,2),(3,2,3),(-1.0690240066242E-6,0.182885378421191),
(0.0734807488197898,0.0736543502199112,0.0910144902320524),
 .UNSPECIFIED.)
GEOMETRIC_REPRESENTATION_ITEM()
RATIONAL_B_SPLINE_SURFACE(((0.99848615229188,0.99848615229188,0.99848615229188,
0.992772345172011,0.990020524139833),(0.99848615229188,0.99848615229188,
0.99848615229188,0.992772345172011,0.990020524139833)))
REPRESENTATION_ITEM('')
SURFACE()
);
#4214=(
BOUNDED_SURFACE()
B_SPLINE_SURFACE(1,2,((#165828,#165829,#165830,#165831,#165832),(#165833,
#165834,#165835,#165836,#165837)),.UNSPECIFIED.,.F.,.F.,.F.)
B_SPLINE_SURFACE_WITH_KNOTS((2,2),(3,2,3),(0.,0.182805892339153),(0.642474614281367,
0.642857142857143,0.659901408087481),.UNSPECIFIED.)
GEOMETRIC_REPRESENTATION_ITEM()
RATIONAL_B_SPLINE_SURFACE(((0.999732896029237,0.999865728939372,1.,0.994017305594881,
0.990889788836284),(0.999732896029237,0.999865728939372,1.,0.994017305594881,
0.990889788836284)))
REPRESENTATION_ITEM('')
SURFACE()
);
#4215=(
BOUNDED_SURFACE()
B_SPLINE_SURFACE(1,2,((#165839,#165840,#165841,#165842,#165843),(#165844,
#165845,#165846,#165847,#165848)),.UNSPECIFIED.,.F.,.F.,.F.)
B_SPLINE_SURFACE_WITH_KNOTS((2,2),(3,2,3),(0.938576859128174,1.),(0.0665257254736565,
0.0714285714285714,0.0736543502199112),.UNSPECIFIED.)
GEOMETRIC_REPRESENTATION_ITEM()
RATIONAL_B_SPLINE_SURFACE(((0.996794362316492,0.998279055819231,1.,0.999218731101516,
0.99848615229188),(0.996794362316492,0.998279055819231,1.,0.999218731101516,
0.99848615229188)))
REPRESENTATION_ITEM('')
SURFACE()
);
#4216=(
BOUNDED_SURFACE()
B_SPLINE_SURFACE(1,2,((#165856,#165857,#165858,#165859,#165860),(#165861,
#165862,#165863,#165864,#165865)),.UNSPECIFIED.,.F.,.F.,.F.)
B_SPLINE_SURFACE_WITH_KNOTS((2,2),(3,2,3),(0.,0.0529045403781288),(0.0665257254736565,
0.0714285714285714,0.0736968668684971),.UNSPECIFIED.)
GEOMETRIC_REPRESENTATION_ITEM()
RATIONAL_B_SPLINE_SURFACE(((0.996794362316492,0.998279055819231,1.,0.999203807365457,
0.998458182734336),(0.996794362316492,0.998279055819231,1.,0.999203807365457,
0.998458182734336)))
REPRESENTATION_ITEM('')
SURFACE()
);
#4217=(
BOUNDED_SURFACE()
B_SPLINE_SURFACE(1,2,((#165876,#165877,#165878),(#165879,#165880,#165881)),
 .UNSPECIFIED.,.F.,.F.,.F.)
B_SPLINE_SURFACE_WITH_KNOTS((2,2),(3,3),(0.,0.0528815468798279),(0.659860018385542,
0.666841081426897),.UNSPECIFIED.)
GEOMETRIC_REPRESENTATION_ITEM()
RATIONAL_B_SPLINE_SURFACE(((0.990904995179376,0.98962117367337,0.988816334712146),
(0.990904995179376,0.98962117367337,0.988816334712146)))
REPRESENTATION_ITEM('')
SURFACE()
);
#4218=(
BOUNDED_SURFACE()
B_SPLINE_SURFACE(1,2,((#165883,#165884,#165885,#165886,#165887),(#165888,
#165889,#165890,#165891,#165892)),.UNSPECIFIED.,.F.,.F.,.F.)
B_SPLINE_SURFACE_WITH_KNOTS((2,2),(3,2,3),(0.93855015164656,1.00001008245209),
(0.659832011353967,0.659901408087362,0.666841081426897),.UNSPECIFIED.)
GEOMETRIC_REPRESENTATION_ITEM()
RATIONAL_B_SPLINE_SURFACE(((0.990889788836328,0.990889788836328,0.990889788836328,
0.989616401900874,0.988816334712145),(0.990889788836328,0.990889788836328,
0.990889788836328,0.989616401900874,0.988816334712145)))
REPRESENTATION_ITEM('')
SURFACE()
);
#4219=(
BOUNDED_SURFACE()
B_SPLINE_SURFACE(1,2,((#165894,#165895,#165896,#165897,#165898),(#165899,
#165900,#165901,#165902,#165903)),.UNSPECIFIED.,.F.,.F.,.F.)
B_SPLINE_SURFACE_WITH_KNOTS((2,2),(3,2,3),(0.,0.182885378421188),(0.0734807488196683,
0.0736543502197909,0.0910144902320531),.UNSPECIFIED.)
GEOMETRIC_REPRESENTATION_ITEM()
RATIONAL_B_SPLINE_SURFACE(((0.998486152291959,0.998486152291959,0.998486152291959,
0.99277234517203,0.990020524139833),(0.998486152291959,0.998486152291959,
0.998486152291959,0.99277234517203,0.990020524139833)))
REPRESENTATION_ITEM('')
SURFACE()
);
#4220=(
BOUNDED_SURFACE()
B_SPLINE_SURFACE(1,2,((#165914,#165915,#165916,#165917,#165918),(#165919,
#165920,#165921,#165922,#165923)),.UNSPECIFIED.,.F.,.F.,.F.)
B_SPLINE_SURFACE_WITH_KNOTS((2,2),(3,2,3),(0.,0.182805892339156),(0.642474614281367,
0.642857142857143,0.659901408087481),.UNSPECIFIED.)
GEOMETRIC_REPRESENTATION_ITEM()
RATIONAL_B_SPLINE_SURFACE(((0.999732896029237,0.999865728939372,1.,0.994017305594881,
0.990889788836284),(0.999732896029237,0.999865728939372,1.,0.994017305594881,
0.990889788836284)))
REPRESENTATION_ITEM('')
SURFACE()
);
#4221=(
BOUNDED_SURFACE()
B_SPLINE_SURFACE(1,2,((#165925,#165926,#165927,#165928,#165929),(#165930,
#165931,#165932,#165933,#165934)),.UNSPECIFIED.,.F.,.F.,.F.)
B_SPLINE_SURFACE_WITH_KNOTS((2,2),(3,2,3),(0.938576859128168,1.),(0.066525725473656,
0.0714285714285714,0.0736543502199112),.UNSPECIFIED.)
GEOMETRIC_REPRESENTATION_ITEM()
RATIONAL_B_SPLINE_SURFACE(((0.996794362316491,0.998279055819231,1.,0.999218731101516,
0.99848615229188),(0.996794362316491,0.998279055819231,1.,0.999218731101516,
0.99848615229188)))
REPRESENTATION_ITEM('')
SURFACE()
);
#4222=(
BOUNDED_SURFACE()
B_SPLINE_SURFACE(1,2,((#165941,#165942,#165943,#165944,#165945),(#165946,
#165947,#165948,#165949,#165950)),.UNSPECIFIED.,.F.,.F.,.F.)
B_SPLINE_SURFACE_WITH_KNOTS((2,2),(3,2,3),(0.,0.0529045403781274),(0.066525725473656,
0.0714285714285714,0.0736968668684972),.UNSPECIFIED.)
GEOMETRIC_REPRESENTATION_ITEM()
RATIONAL_B_SPLINE_SURFACE(((0.996794362316491,0.998279055819231,1.,0.999203807365457,
0.998458182734336),(0.996794362316491,0.998279055819231,1.,0.999203807365457,
0.998458182734336)))
REPRESENTATION_ITEM('')
SURFACE()
);
#4223=(
BOUNDED_SURFACE()
B_SPLINE_SURFACE(1,2,((#165961,#165962,#165963),(#165964,#165965,#165966)),
 .UNSPECIFIED.,.F.,.F.,.F.)
B_SPLINE_SURFACE_WITH_KNOTS((2,2),(3,3),(0.,0.0528815468798305),(0.659860018385656,
0.666841081426897),.UNSPECIFIED.)
GEOMETRIC_REPRESENTATION_ITEM()
RATIONAL_B_SPLINE_SURFACE(((0.990904995179334,0.989621173673357,0.988816334712145),
(0.990904995179334,0.989621173673357,0.988816334712145)))
REPRESENTATION_ITEM('')
SURFACE()
);
#4224=(
BOUNDED_SURFACE()
B_SPLINE_SURFACE(1,2,((#165968,#165969,#165970,#165971,#165972),(#165973,
#165974,#165975,#165976,#165977)),.UNSPECIFIED.,.F.,.F.,.F.)
B_SPLINE_SURFACE_WITH_KNOTS((2,2),(3,2,3),(0.938550151647609,1.00001008248703),
(0.659832011354087,0.659901408087481,0.666841081426897),.UNSPECIFIED.)
GEOMETRIC_REPRESENTATION_ITEM()
RATIONAL_B_SPLINE_SURFACE(((0.990889788836284,0.990889788836284,0.990889788836284,
0.98961640190086,0.988816334712146),(0.990889788836284,0.990889788836284,
0.990889788836284,0.98961640190086,0.988816334712146)))
REPRESENTATION_ITEM('')
SURFACE()
);
#4225=(
BOUNDED_SURFACE()
B_SPLINE_SURFACE(1,2,((#165979,#165980,#165981,#165982,#165983),(#165984,
#165985,#165986,#165987,#165988)),.UNSPECIFIED.,.F.,.F.,.F.)
B_SPLINE_SURFACE_WITH_KNOTS((2,2),(3,2,3),(-1.06890081270921E-6,0.182885378421181),
(0.0734807488197897,0.0736543502199111,0.0910144902320513),
 .UNSPECIFIED.)
GEOMETRIC_REPRESENTATION_ITEM()
RATIONAL_B_SPLINE_SURFACE(((0.99848615229188,0.99848615229188,0.99848615229188,
0.992772345172012,0.990020524139833),(0.99848615229188,0.99848615229188,
0.99848615229188,0.992772345172012,0.990020524139833)))
REPRESENTATION_ITEM('')
SURFACE()
);
#4226=(
BOUNDED_SURFACE()
B_SPLINE_SURFACE(1,2,((#165999,#166000,#166001,#166002,#166003),(#166004,
#166005,#166006,#166007,#166008)),.UNSPECIFIED.,.F.,.F.,.F.)
B_SPLINE_SURFACE_WITH_KNOTS((2,2),(3,2,3),(0.,0.182805892339142),(0.642474614281368,
0.642857142857143,0.659901408087482),.UNSPECIFIED.)
GEOMETRIC_REPRESENTATION_ITEM()
RATIONAL_B_SPLINE_SURFACE(((0.999732896029238,0.999865728939373,1.,0.994017305594881,
0.990889788836284),(0.999732896029238,0.999865728939373,1.,0.994017305594881,
0.990889788836284)))
REPRESENTATION_ITEM('')
SURFACE()
);
#4227=(
BOUNDED_SURFACE()
B_SPLINE_SURFACE(1,2,((#166010,#166011,#166012,#166013,#166014),(#166015,
#166016,#166017,#166018,#166019)),.UNSPECIFIED.,.F.,.F.,.F.)
B_SPLINE_SURFACE_WITH_KNOTS((2,2),(3,2,3),(0.938576859128178,1.),(0.0665257254736559,
0.0714285714285714,0.0736543502199103),.UNSPECIFIED.)
GEOMETRIC_REPRESENTATION_ITEM()
RATIONAL_B_SPLINE_SURFACE(((0.996794362316491,0.998279055819231,1.,0.999218731101516,
0.99848615229188),(0.996794362316491,0.998279055819231,1.,0.999218731101516,
0.99848615229188)))
REPRESENTATION_ITEM('')
SURFACE()
);
#4228=(
BOUNDED_SURFACE()
B_SPLINE_SURFACE(1,2,((#166027,#166028,#166029,#166030,#166031),(#166032,
#166033,#166034,#166035,#166036)),.UNSPECIFIED.,.F.,.F.,.F.)
B_SPLINE_SURFACE_WITH_KNOTS((2,2),(3,2,3),(0.,0.0529045403781231),(0.0665257254736559,
0.0714285714285714,0.0736968668684961),.UNSPECIFIED.)
GEOMETRIC_REPRESENTATION_ITEM()
RATIONAL_B_SPLINE_SURFACE(((0.996794362316491,0.998279055819231,1.,0.999203807365457,
0.998458182734337),(0.996794362316491,0.998279055819231,1.,0.999203807365457,
0.998458182734337)))
REPRESENTATION_ITEM('')
SURFACE()
);
#4229=(
BOUNDED_SURFACE()
B_SPLINE_SURFACE(1,2,((#166047,#166048,#166049),(#166050,#166051,#166052)),
 .UNSPECIFIED.,.F.,.F.,.F.)
B_SPLINE_SURFACE_WITH_KNOTS((2,2),(3,3),(0.,0.0528815468798204),(0.659860018385657,
0.666841081426896),.UNSPECIFIED.)
GEOMETRIC_REPRESENTATION_ITEM()
RATIONAL_B_SPLINE_SURFACE(((0.990904995179334,0.989621173673357,0.988816334712146),
(0.990904995179334,0.989621173673357,0.988816334712146)))
REPRESENTATION_ITEM('')
SURFACE()
);
#4230=(
BOUNDED_SURFACE()
B_SPLINE_SURFACE(1,2,((#166054,#166055,#166056,#166057,#166058),(#166059,
#166060,#166061,#166062,#166063)),.UNSPECIFIED.,.F.,.F.,.F.)
B_SPLINE_SURFACE_WITH_KNOTS((2,2),(3,2,3),(0.938550151647352,1.00001008247331),
(0.659832011354058,0.659901408087452,0.666841081426896),.UNSPECIFIED.)
GEOMETRIC_REPRESENTATION_ITEM()
RATIONAL_B_SPLINE_SURFACE(((0.990889788836295,0.990889788836295,0.990889788836295,
0.989616401900864,0.988816334712146),(0.990889788836295,0.990889788836295,
0.990889788836295,0.989616401900864,0.988816334712146)))
REPRESENTATION_ITEM('')
SURFACE()
);
#4231=(
BOUNDED_SURFACE()
B_SPLINE_SURFACE(1,2,((#166065,#166066,#166067,#166068,#166069),(#166070,
#166071,#166072,#166073,#166074)),.UNSPECIFIED.,.F.,.F.,.F.)
B_SPLINE_SURFACE_WITH_KNOTS((2,2),(3,2,3),(-1.0690222232507E-6,0.182885378421185),
(0.0734807488197886,0.07365435021991,0.0910144902320513),.UNSPECIFIED.)
GEOMETRIC_REPRESENTATION_ITEM()
RATIONAL_B_SPLINE_SURFACE(((0.99848615229188,0.99848615229188,0.99848615229188,
0.992772345172012,0.990020524139833),(0.99848615229188,0.99848615229188,
0.99848615229188,0.992772345172012,0.990020524139833)))
REPRESENTATION_ITEM('')
SURFACE()
);
#4232=(
BOUNDED_SURFACE()
B_SPLINE_SURFACE(1,2,((#166085,#166086,#166087,#166088,#166089),(#166090,
#166091,#166092,#166093,#166094)),.UNSPECIFIED.,.F.,.F.,.F.)
B_SPLINE_SURFACE_WITH_KNOTS((2,2),(3,2,3),(0.,0.182805892339149),(0.642474614281368,
0.642857142857143,0.659901408087483),.UNSPECIFIED.)
GEOMETRIC_REPRESENTATION_ITEM()
RATIONAL_B_SPLINE_SURFACE(((0.999732896029238,0.999865728939373,1.,0.994017305594881,
0.990889788836284),(0.999732896029238,0.999865728939373,1.,0.994017305594881,
0.990889788836284)))
REPRESENTATION_ITEM('')
SURFACE()
);
#4233=(
BOUNDED_SURFACE()
B_SPLINE_SURFACE(1,2,((#166096,#166097,#166098,#166099,#166100),(#166101,
#166102,#166103,#166104,#166105)),.UNSPECIFIED.,.F.,.F.,.F.)
B_SPLINE_SURFACE_WITH_KNOTS((2,2),(3,2,3),(0.93857685912818,1.),(0.0665257254736559,
0.0714285714285714,0.0736543502199101),.UNSPECIFIED.)
GEOMETRIC_REPRESENTATION_ITEM()
RATIONAL_B_SPLINE_SURFACE(((0.996794362316491,0.998279055819231,1.,0.999218731101516,
0.99848615229188),(0.996794362316491,0.998279055819231,1.,0.999218731101516,
0.99848615229188)))
REPRESENTATION_ITEM('')
SURFACE()
);
#4234=(
BOUNDED_SURFACE()
B_SPLINE_SURFACE(1,2,((#166113,#166114,#166115,#166116,#166117),(#166118,
#166119,#166120,#166121,#166122)),.UNSPECIFIED.,.F.,.F.,.F.)
B_SPLINE_SURFACE_WITH_KNOTS((2,2),(3,2,3),(0.,0.0529045403781231),(0.0665257254736559,
0.0714285714285714,0.073696866868496),.UNSPECIFIED.)
GEOMETRIC_REPRESENTATION_ITEM()
RATIONAL_B_SPLINE_SURFACE(((0.996794362316491,0.998279055819231,1.,0.999203807365457,
0.998458182734337),(0.996794362316491,0.998279055819231,1.,0.999203807365457,
0.998458182734337)))
REPRESENTATION_ITEM('')
SURFACE()
);
#4235=(
BOUNDED_SURFACE()
B_SPLINE_SURFACE(1,2,((#166133,#166134,#166135),(#166136,#166137,#166138)),
 .UNSPECIFIED.,.F.,.F.,.F.)
B_SPLINE_SURFACE_WITH_KNOTS((2,2),(3,3),(0.,0.0528815468798243),(0.659860018385657,
0.666841081426897),.UNSPECIFIED.)
GEOMETRIC_REPRESENTATION_ITEM()
RATIONAL_B_SPLINE_SURFACE(((0.990904995179334,0.989621173673357,0.988816334712146),
(0.990904995179334,0.989621173673357,0.988816334712146)))
REPRESENTATION_ITEM('')
SURFACE()
);
#4236=(
BOUNDED_SURFACE()
B_SPLINE_SURFACE(1,2,((#166140,#166141,#166142,#166143,#166144),(#166145,
#166146,#166147,#166148,#166149)),.UNSPECIFIED.,.F.,.F.,.F.)
B_SPLINE_SURFACE_WITH_KNOTS((2,2),(3,2,3),(0.938550151647345,1.00001008244498),
(0.659832011354057,0.659901408087451,0.666841081426897),.UNSPECIFIED.)
GEOMETRIC_REPRESENTATION_ITEM()
RATIONAL_B_SPLINE_SURFACE(((0.990889788836295,0.990889788836295,0.990889788836295,
0.989616401900863,0.988816334712145),(0.990889788836295,0.990889788836295,
0.990889788836295,0.989616401900863,0.988816334712145)))
REPRESENTATION_ITEM('')
SURFACE()
);
#4237=(
BOUNDED_SURFACE()
B_SPLINE_SURFACE(1,2,((#166151,#166152,#166153,#166154,#166155),(#166156,
#166157,#166158,#166159,#166160)),.UNSPECIFIED.,.F.,.F.,.F.)
B_SPLINE_SURFACE_WITH_KNOTS((2,2),(3,2,3),(-1.06898485868802E-6,0.182885378421184),
(0.0734807488197886,0.07365435021991,0.0910144902320514),.UNSPECIFIED.)
GEOMETRIC_REPRESENTATION_ITEM()
RATIONAL_B_SPLINE_SURFACE(((0.998486152291881,0.998486152291881,0.998486152291881,
0.992772345172012,0.990020524139834),(0.998486152291881,0.998486152291881,
0.998486152291881,0.992772345172012,0.990020524139834)))
REPRESENTATION_ITEM('')
SURFACE()
);
#4238=(
BOUNDED_SURFACE()
B_SPLINE_SURFACE(1,2,((#166171,#166172,#166173,#166174,#166175),(#166176,
#166177,#166178,#166179,#166180)),.UNSPECIFIED.,.F.,.F.,.F.)
B_SPLINE_SURFACE_WITH_KNOTS((2,2),(3,2,3),(0.,0.182805892339149),(0.642474614281368,
0.642857142857143,0.659901408087482),.UNSPECIFIED.)
GEOMETRIC_REPRESENTATION_ITEM()
RATIONAL_B_SPLINE_SURFACE(((0.999732896029238,0.999865728939373,1.,0.994017305594881,
0.990889788836284),(0.999732896029238,0.999865728939373,1.,0.994017305594881,
0.990889788836284)))
REPRESENTATION_ITEM('')
SURFACE()
);
#4239=(
BOUNDED_SURFACE()
B_SPLINE_SURFACE(1,2,((#166182,#166183,#166184,#166185,#166186),(#166187,
#166188,#166189,#166190,#166191)),.UNSPECIFIED.,.F.,.F.,.F.)
B_SPLINE_SURFACE_WITH_KNOTS((2,2),(3,2,3),(0.938576859128178,1.),(0.0665257254736558,
0.0714285714285714,0.0736543502199101),.UNSPECIFIED.)
GEOMETRIC_REPRESENTATION_ITEM()
RATIONAL_B_SPLINE_SURFACE(((0.996794362316491,0.998279055819231,1.,0.999218731101516,
0.99848615229188),(0.996794362316491,0.998279055819231,1.,0.999218731101516,
0.99848615229188)))
REPRESENTATION_ITEM('')
SURFACE()
);
#4240=(
BOUNDED_SURFACE()
B_SPLINE_SURFACE(1,2,((#166199,#166200,#166201,#166202,#166203),(#166204,
#166205,#166206,#166207,#166208)),.UNSPECIFIED.,.F.,.F.,.F.)
B_SPLINE_SURFACE_WITH_KNOTS((2,2),(3,2,3),(0.,0.0529045403781231),(0.0665257254736558,
0.0714285714285714,0.073696866868496),.UNSPECIFIED.)
GEOMETRIC_REPRESENTATION_ITEM()
RATIONAL_B_SPLINE_SURFACE(((0.996794362316491,0.998279055819231,1.,0.999203807365457,
0.998458182734336),(0.996794362316491,0.998279055819231,1.,0.999203807365457,
0.998458182734336)))
REPRESENTATION_ITEM('')
SURFACE()
);
#4241=(
BOUNDED_SURFACE()
B_SPLINE_SURFACE(1,2,((#166219,#166220,#166221),(#166222,#166223,#166224)),
 .UNSPECIFIED.,.F.,.F.,.F.)
B_SPLINE_SURFACE_WITH_KNOTS((2,2),(3,3),(0.,0.0528815468798209),(0.659860018385657,
0.666841081426897),.UNSPECIFIED.)
GEOMETRIC_REPRESENTATION_ITEM()
RATIONAL_B_SPLINE_SURFACE(((0.990904995179334,0.989621173673357,0.988816334712146),
(0.990904995179334,0.989621173673357,0.988816334712146)))
REPRESENTATION_ITEM('')
SURFACE()
);
#4242=(
BOUNDED_SURFACE()
B_SPLINE_SURFACE(1,2,((#166226,#166227,#166228,#166229,#166230),(#166231,
#166232,#166233,#166234,#166235)),.UNSPECIFIED.,.F.,.F.,.F.)
B_SPLINE_SURFACE_WITH_KNOTS((2,2),(3,2,3),(0.938550151647348,1.00001008248998),
(0.659832011354058,0.659901408087452,0.666841081426897),.UNSPECIFIED.)
GEOMETRIC_REPRESENTATION_ITEM()
RATIONAL_B_SPLINE_SURFACE(((0.990889788836295,0.990889788836295,0.990889788836295,
0.989616401900863,0.988816334712145),(0.990889788836295,0.990889788836295,
0.990889788836295,0.989616401900863,0.988816334712145)))
REPRESENTATION_ITEM('')
SURFACE()
);
#4243=(
BOUNDED_SURFACE()
B_SPLINE_SURFACE(1,2,((#166237,#166238,#166239,#166240,#166241),(#166242,
#166243,#166244,#166245,#166246)),.UNSPECIFIED.,.F.,.F.,.F.)
B_SPLINE_SURFACE_WITH_KNOTS((2,2),(3,2,3),(0.,0.182885378421184),(0.0734807488197886,
0.07365435021991,0.0910144902320513),.UNSPECIFIED.)
GEOMETRIC_REPRESENTATION_ITEM()
RATIONAL_B_SPLINE_SURFACE(((0.99848615229188,0.99848615229188,0.99848615229188,
0.992772345172012,0.990020524139833),(0.99848615229188,0.99848615229188,
0.99848615229188,0.992772345172012,0.990020524139833)))
REPRESENTATION_ITEM('')
SURFACE()
);
#4244=(
BOUNDED_SURFACE()
B_SPLINE_SURFACE(1,2,((#166257,#166258,#166259,#166260,#166261),(#166262,
#166263,#166264,#166265,#166266)),.UNSPECIFIED.,.F.,.F.,.F.)
B_SPLINE_SURFACE_WITH_KNOTS((2,2),(3,2,3),(0.,0.182805892339146),(0.642474614281368,
0.642857142857143,0.659901408087482),.UNSPECIFIED.)
GEOMETRIC_REPRESENTATION_ITEM()
RATIONAL_B_SPLINE_SURFACE(((0.999732896029238,0.999865728939373,1.,0.994017305594881,
0.990889788836284),(0.999732896029238,0.999865728939373,1.,0.994017305594881,
0.990889788836284)))
REPRESENTATION_ITEM('')
SURFACE()
);
#4245=(
BOUNDED_SURFACE()
B_SPLINE_SURFACE(1,2,((#166268,#166269,#166270,#166271,#166272),(#166273,
#166274,#166275,#166276,#166277)),.UNSPECIFIED.,.F.,.F.,.F.)
B_SPLINE_SURFACE_WITH_KNOTS((2,2),(3,2,3),(0.93857685912818,1.),(0.0665257254736559,
0.0714285714285714,0.07365435021991),.UNSPECIFIED.)
GEOMETRIC_REPRESENTATION_ITEM()
RATIONAL_B_SPLINE_SURFACE(((0.996794362316491,0.998279055819231,1.,0.999218731101516,
0.99848615229188),(0.996794362316491,0.998279055819231,1.,0.999218731101516,
0.99848615229188)))
REPRESENTATION_ITEM('')
SURFACE()
);
#4246=(
BOUNDED_SURFACE()
B_SPLINE_SURFACE(1,2,((#166285,#166286,#166287,#166288,#166289),(#166290,
#166291,#166292,#166293,#166294)),.UNSPECIFIED.,.F.,.F.,.F.)
B_SPLINE_SURFACE_WITH_KNOTS((2,2),(3,2,3),(0.,0.0529045403781213),(0.0665257254736559,
0.0714285714285714,0.073696866868496),.UNSPECIFIED.)
GEOMETRIC_REPRESENTATION_ITEM()
RATIONAL_B_SPLINE_SURFACE(((0.996794362316491,0.998279055819231,1.,0.999203807365457,
0.998458182734337),(0.996794362316491,0.998279055819231,1.,0.999203807365457,
0.998458182734337)))
REPRESENTATION_ITEM('')
SURFACE()
);
#4247=(
BOUNDED_SURFACE()
B_SPLINE_SURFACE(1,2,((#166305,#166306,#166307),(#166308,#166309,#166310)),
 .UNSPECIFIED.,.F.,.F.,.F.)
B_SPLINE_SURFACE_WITH_KNOTS((2,2),(3,3),(0.,0.0528815468798213),(0.659860018385657,
0.666841081426897),.UNSPECIFIED.)
GEOMETRIC_REPRESENTATION_ITEM()
RATIONAL_B_SPLINE_SURFACE(((0.990904995179334,0.989621173673357,0.988816334712145),
(0.990904995179334,0.989621173673357,0.988816334712145)))
REPRESENTATION_ITEM('')
SURFACE()
);
#4248=(
BOUNDED_SURFACE()
B_SPLINE_SURFACE(1,2,((#166312,#166313,#166314,#166315,#166316),(#166317,
#166318,#166319,#166320,#166321)),.UNSPECIFIED.,.F.,.F.,.F.)
B_SPLINE_SURFACE_WITH_KNOTS((2,2),(3,2,3),(0.93855015164735,1.00001008250064),
(0.659832011354058,0.659901408087452,0.666841081426897),.UNSPECIFIED.)
GEOMETRIC_REPRESENTATION_ITEM()
RATIONAL_B_SPLINE_SURFACE(((0.990889788836295,0.990889788836295,0.990889788836295,
0.989616401900864,0.988816334712146),(0.990889788836295,0.990889788836295,
0.990889788836295,0.989616401900864,0.988816334712146)))
REPRESENTATION_ITEM('')
SURFACE()
);
#4249=(
BOUNDED_SURFACE()
B_SPLINE_SURFACE(1,2,((#166323,#166324,#166325,#166326,#166327),(#166328,
#166329,#166330,#166331,#166332)),.UNSPECIFIED.,.F.,.F.,.F.)
B_SPLINE_SURFACE_WITH_KNOTS((2,2),(3,2,3),(-1.07111455693367E-6,0.182885378421183),
(0.0734807488197886,0.07365435021991,0.0910144902320513),.UNSPECIFIED.)
GEOMETRIC_REPRESENTATION_ITEM()
RATIONAL_B_SPLINE_SURFACE(((0.99848615229188,0.99848615229188,0.99848615229188,
0.992772345172012,0.990020524139833),(0.99848615229188,0.99848615229188,
0.99848615229188,0.992772345172012,0.990020524139833)))
REPRESENTATION_ITEM('')
SURFACE()
);
#4250=(
BOUNDED_SURFACE()
B_SPLINE_SURFACE(1,2,((#166343,#166344,#166345,#166346,#166347),(#166348,
#166349,#166350,#166351,#166352)),.UNSPECIFIED.,.F.,.F.,.F.)
B_SPLINE_SURFACE_WITH_KNOTS((2,2),(3,2,3),(0.,0.182805892339148),(0.642474614281367,
0.642857142857143,0.659901408087482),.UNSPECIFIED.)
GEOMETRIC_REPRESENTATION_ITEM()
RATIONAL_B_SPLINE_SURFACE(((0.999732896029238,0.999865728939373,1.,0.994017305594881,
0.990889788836284),(0.999732896029238,0.999865728939373,1.,0.994017305594881,
0.990889788836284)))
REPRESENTATION_ITEM('')
SURFACE()
);
#4251=(
BOUNDED_SURFACE()
B_SPLINE_SURFACE(1,2,((#166354,#166355,#166356,#166357,#166358),(#166359,
#166360,#166361,#166362,#166363)),.UNSPECIFIED.,.F.,.F.,.F.)
B_SPLINE_SURFACE_WITH_KNOTS((2,2),(3,2,3),(0.938576859128178,1.),(0.0665257254736559,
0.0714285714285714,0.0736543502199101),.UNSPECIFIED.)
GEOMETRIC_REPRESENTATION_ITEM()
RATIONAL_B_SPLINE_SURFACE(((0.996794362316491,0.998279055819231,1.,0.999218731101516,
0.99848615229188),(0.996794362316491,0.998279055819231,1.,0.999218731101516,
0.99848615229188)))
REPRESENTATION_ITEM('')
SURFACE()
);
#4252=(
BOUNDED_SURFACE()
B_SPLINE_SURFACE(1,2,((#166370,#166371,#166372,#166373,#166374),(#166375,
#166376,#166377,#166378,#166379)),.UNSPECIFIED.,.F.,.F.,.F.)
B_SPLINE_SURFACE_WITH_KNOTS((2,2),(3,2,3),(0.,0.0529045403781227),(0.0665257254736559,
0.0714285714285714,0.073696866868496),.UNSPECIFIED.)
GEOMETRIC_REPRESENTATION_ITEM()
RATIONAL_B_SPLINE_SURFACE(((0.996794362316491,0.998279055819231,1.,0.999203807365457,
0.998458182734337),(0.996794362316491,0.998279055819231,1.,0.999203807365457,
0.998458182734337)))
REPRESENTATION_ITEM('')
SURFACE()
);
#4253=(
BOUNDED_SURFACE()
B_SPLINE_SURFACE(1,2,((#166390,#166391,#166392),(#166393,#166394,#166395)),
 .UNSPECIFIED.,.F.,.F.,.F.)
B_SPLINE_SURFACE_WITH_KNOTS((2,2),(3,3),(0.,0.0528815468798243),(0.659860018385657,
0.666841081426897),.UNSPECIFIED.)
GEOMETRIC_REPRESENTATION_ITEM()
RATIONAL_B_SPLINE_SURFACE(((0.990904995179334,0.989621173673357,0.988816334712146),
(0.990904995179334,0.989621173673357,0.988816334712145)))
REPRESENTATION_ITEM('')
SURFACE()
);
#4254=(
BOUNDED_SURFACE()
B_SPLINE_SURFACE(1,2,((#166397,#166398,#166399,#166400,#166401),(#166402,
#166403,#166404,#166405,#166406)),.UNSPECIFIED.,.F.,.F.,.F.)
B_SPLINE_SURFACE_WITH_KNOTS((2,2),(3,2,3),(0.938550151647349,1.00001008247581),
(0.659832011354058,0.659901408087452,0.666841081426897),.UNSPECIFIED.)
GEOMETRIC_REPRESENTATION_ITEM()
RATIONAL_B_SPLINE_SURFACE(((0.990889788836295,0.990889788836295,0.990889788836295,
0.989616401900864,0.988816334712146),(0.990889788836295,0.990889788836295,
0.990889788836295,0.989616401900864,0.988816334712146)))
REPRESENTATION_ITEM('')
SURFACE()
);
#4255=(
BOUNDED_SURFACE()
B_SPLINE_SURFACE(1,2,((#166408,#166409,#166410,#166411,#166412),(#166413,
#166414,#166415,#166416,#166417)),.UNSPECIFIED.,.F.,.F.,.F.)
B_SPLINE_SURFACE_WITH_KNOTS((2,2),(3,2,3),(-1.07080442310849E-6,0.182885378421184),
(0.0734807488197886,0.07365435021991,0.0910144902320513),.UNSPECIFIED.)
GEOMETRIC_REPRESENTATION_ITEM()
RATIONAL_B_SPLINE_SURFACE(((0.99848615229188,0.99848615229188,0.99848615229188,
0.992772345172012,0.990020524139833),(0.99848615229188,0.99848615229188,
0.99848615229188,0.992772345172012,0.990020524139833)))
REPRESENTATION_ITEM('')
SURFACE()
);
#4256=(
BOUNDED_SURFACE()
B_SPLINE_SURFACE(1,2,((#166428,#166429,#166430,#166431,#166432),(#166433,
#166434,#166435,#166436,#166437)),.UNSPECIFIED.,.F.,.F.,.F.)
B_SPLINE_SURFACE_WITH_KNOTS((2,2),(3,2,3),(0.,0.182805892339143),(0.642474614281368,
0.642857142857143,0.659901408087482),.UNSPECIFIED.)
GEOMETRIC_REPRESENTATION_ITEM()
RATIONAL_B_SPLINE_SURFACE(((0.999732896029238,0.999865728939373,1.,0.994017305594881,
0.990889788836284),(0.999732896029238,0.999865728939373,1.,0.994017305594881,
0.990889788836284)))
REPRESENTATION_ITEM('')
SURFACE()
);
#4257=(
BOUNDED_SURFACE()
B_SPLINE_SURFACE(1,2,((#166439,#166440,#166441,#166442,#166443),(#166444,
#166445,#166446,#166447,#166448)),.UNSPECIFIED.,.F.,.F.,.F.)
B_SPLINE_SURFACE_WITH_KNOTS((2,2),(3,2,3),(0.938576859128179,1.),(0.0665257254736559,
0.0714285714285714,0.07365435021991),.UNSPECIFIED.)
GEOMETRIC_REPRESENTATION_ITEM()
RATIONAL_B_SPLINE_SURFACE(((0.996794362316491,0.998279055819231,1.,0.999218731101516,
0.99848615229188),(0.996794362316491,0.998279055819231,1.,0.999218731101516,
0.99848615229188)))
REPRESENTATION_ITEM('')
SURFACE()
);
#4258=(
BOUNDED_SURFACE()
B_SPLINE_SURFACE(1,2,((#166456,#166457,#166458,#166459,#166460),(#166461,
#166462,#166463,#166464,#166465)),.UNSPECIFIED.,.F.,.F.,.F.)
B_SPLINE_SURFACE_WITH_KNOTS((2,2),(3,2,3),(0.,0.0529045403781224),(0.066525725473656,
0.0714285714285714,0.073696866868496),.UNSPECIFIED.)
GEOMETRIC_REPRESENTATION_ITEM()
RATIONAL_B_SPLINE_SURFACE(((0.996794362316491,0.998279055819231,1.,0.999203807365457,
0.998458182734337),(0.996794362316491,0.998279055819231,1.,0.999203807365457,
0.998458182734337)))
REPRESENTATION_ITEM('')
SURFACE()
);
#4259=(
BOUNDED_SURFACE()
B_SPLINE_SURFACE(1,2,((#166476,#166477,#166478),(#166479,#166480,#166481)),
 .UNSPECIFIED.,.F.,.F.,.F.)
B_SPLINE_SURFACE_WITH_KNOTS((2,2),(3,3),(0.,0.0528815468798206),(0.659860018385657,
0.666841081426896),.UNSPECIFIED.)
GEOMETRIC_REPRESENTATION_ITEM()
RATIONAL_B_SPLINE_SURFACE(((0.990904995179334,0.989621173673357,0.988816334712146),
(0.990904995179334,0.989621173673357,0.988816334712145)))
REPRESENTATION_ITEM('')
SURFACE()
);
#4260=(
BOUNDED_SURFACE()
B_SPLINE_SURFACE(1,2,((#166483,#166484,#166485,#166486,#166487),(#166488,
#166489,#166490,#166491,#166492)),.UNSPECIFIED.,.F.,.F.,.F.)
B_SPLINE_SURFACE_WITH_KNOTS((2,2),(3,2,3),(0.938550151647356,1.0000100824502),
(0.659832011354058,0.659901408087452,0.666841081426897),.UNSPECIFIED.)
GEOMETRIC_REPRESENTATION_ITEM()
RATIONAL_B_SPLINE_SURFACE(((0.990889788836295,0.990889788836295,0.990889788836295,
0.989616401900864,0.988816334712146),(0.990889788836295,0.990889788836295,
0.990889788836295,0.989616401900864,0.988816334712146)))
REPRESENTATION_ITEM('')
SURFACE()
);
#4261=(
BOUNDED_SURFACE()
B_SPLINE_SURFACE(1,2,((#166494,#166495,#166496,#166497,#166498),(#166499,
#166500,#166501,#166502,#166503)),.UNSPECIFIED.,.F.,.F.,.F.)
B_SPLINE_SURFACE_WITH_KNOTS((2,2),(3,2,3),(0.,0.182885378421178),(0.0734807488197886,
0.07365435021991,0.0910144902320512),.UNSPECIFIED.)
GEOMETRIC_REPRESENTATION_ITEM()
RATIONAL_B_SPLINE_SURFACE(((0.998486152291881,0.998486152291881,0.998486152291881,
0.992772345172012,0.990020524139834),(0.998486152291881,0.998486152291881,
0.998486152291881,0.992772345172012,0.990020524139834)))
REPRESENTATION_ITEM('')
SURFACE()
);
#4262=(
BOUNDED_SURFACE()
B_SPLINE_SURFACE(1,2,((#166514,#166515,#166516,#166517,#166518),(#166519,
#166520,#166521,#166522,#166523)),.UNSPECIFIED.,.F.,.F.,.F.)
B_SPLINE_SURFACE_WITH_KNOTS((2,2),(3,2,3),(0.,0.182805892339139),(0.642474614281368,
0.642857142857143,0.659901408087483),.UNSPECIFIED.)
GEOMETRIC_REPRESENTATION_ITEM()
RATIONAL_B_SPLINE_SURFACE(((0.999732896029238,0.999865728939373,1.,0.994017305594881,
0.990889788836284),(0.999732896029238,0.999865728939373,1.,0.994017305594881,
0.990889788836284)))
REPRESENTATION_ITEM('')
SURFACE()
);
#4263=(
BOUNDED_SURFACE()
B_SPLINE_SURFACE(1,2,((#166525,#166526,#166527,#166528,#166529),(#166530,
#166531,#166532,#166533,#166534)),.UNSPECIFIED.,.F.,.F.,.F.)
B_SPLINE_SURFACE_WITH_KNOTS((2,2),(3,2,3),(0.938576859128171,1.),(0.0665257254736558,
0.0714285714285714,0.0736543502199103),.UNSPECIFIED.)
GEOMETRIC_REPRESENTATION_ITEM()
RATIONAL_B_SPLINE_SURFACE(((0.996794362316491,0.998279055819231,1.,0.999218731101516,
0.99848615229188),(0.996794362316491,0.998279055819231,1.,0.999218731101516,
0.99848615229188)))
REPRESENTATION_ITEM('')
SURFACE()
);
#4264=(
BOUNDED_SURFACE()
B_SPLINE_SURFACE(1,2,((#166541,#166542,#166543,#166544,#166545),(#166546,
#166547,#166548,#166549,#166550)),.UNSPECIFIED.,.F.,.F.,.F.)
B_SPLINE_SURFACE_WITH_KNOTS((2,2),(3,2,3),(0.,0.0529045403781233),(0.0665257254736558,
0.0714285714285714,0.0736968668684958),.UNSPECIFIED.)
GEOMETRIC_REPRESENTATION_ITEM()
RATIONAL_B_SPLINE_SURFACE(((0.996794362316491,0.998279055819231,1.,0.999203807365457,
0.998458182734337),(0.996794362316491,0.998279055819231,1.,0.999203807365457,
0.998458182734337)))
REPRESENTATION_ITEM('')
SURFACE()
);
#4265=(
BOUNDED_SURFACE()
B_SPLINE_SURFACE(1,2,((#166561,#166562,#166563),(#166564,#166565,#166566)),
 .UNSPECIFIED.,.F.,.F.,.F.)
B_SPLINE_SURFACE_WITH_KNOTS((2,2),(3,3),(0.,0.052881546879817),(0.659860018385656,
0.666841081426896),.UNSPECIFIED.)
GEOMETRIC_REPRESENTATION_ITEM()
RATIONAL_B_SPLINE_SURFACE(((0.990904995179334,0.989621173673357,0.988816334712146),
(0.990904995179334,0.989621173673357,0.988816334712146)))
REPRESENTATION_ITEM('')
SURFACE()
);
#4266=(
BOUNDED_SURFACE()
B_SPLINE_SURFACE(1,2,((#166568,#166569,#166570,#166571,#166572),(#166573,
#166574,#166575,#166576,#166577)),.UNSPECIFIED.,.F.,.F.,.F.)
B_SPLINE_SURFACE_WITH_KNOTS((2,2),(3,2,3),(0.938550151647354,1.00001008250033),
(0.659832011354058,0.659901408087452,0.666841081426896),.UNSPECIFIED.)
GEOMETRIC_REPRESENTATION_ITEM()
RATIONAL_B_SPLINE_SURFACE(((0.990889788836295,0.990889788836295,0.990889788836295,
0.989616401900864,0.988816334712146),(0.990889788836295,0.990889788836295,
0.990889788836295,0.989616401900864,0.988816334712146)))
REPRESENTATION_ITEM('')
SURFACE()
);
#4267=(
BOUNDED_SURFACE()
B_SPLINE_SURFACE(1,2,((#166579,#166580,#166581,#166582,#166583),(#166584,
#166585,#166586,#166587,#166588)),.UNSPECIFIED.,.F.,.F.,.F.)
B_SPLINE_SURFACE_WITH_KNOTS((2,2),(3,2,3),(-1.07087661006151E-6,0.182885378421182),
(0.0734807488197878,0.0736543502199092,0.0910144902320526),
 .UNSPECIFIED.)
GEOMETRIC_REPRESENTATION_ITEM()
RATIONAL_B_SPLINE_SURFACE(((0.998486152291881,0.998486152291881,0.998486152291881,
0.992772345172012,0.990020524139833),(0.998486152291881,0.998486152291881,
0.998486152291881,0.992772345172012,0.990020524139833)))
REPRESENTATION_ITEM('')
SURFACE()
);
#4268=(
BOUNDED_SURFACE()
B_SPLINE_SURFACE(1,2,((#166599,#166600,#166601,#166602,#166603),(#166604,
#166605,#166606,#166607,#166608)),.UNSPECIFIED.,.F.,.F.,.F.)
B_SPLINE_SURFACE_WITH_KNOTS((2,2),(3,2,3),(0.,0.182805892339143),(0.642474614281368,
0.642857142857143,0.659901408087483),.UNSPECIFIED.)
GEOMETRIC_REPRESENTATION_ITEM()
RATIONAL_B_SPLINE_SURFACE(((0.999732896029238,0.999865728939373,1.,0.994017305594881,
0.990889788836284),(0.999732896029238,0.999865728939373,1.,0.994017305594881,
0.990889788836284)))
REPRESENTATION_ITEM('')
SURFACE()
);
#4269=(
BOUNDED_SURFACE()
B_SPLINE_SURFACE(1,2,((#166610,#166611,#166612,#166613,#166614),(#166615,
#166616,#166617,#166618,#166619)),.UNSPECIFIED.,.F.,.F.,.F.)
B_SPLINE_SURFACE_WITH_KNOTS((2,2),(3,2,3),(0.938576859128179,1.),(0.066525725473656,
0.0714285714285714,0.0736543502199102),.UNSPECIFIED.)
GEOMETRIC_REPRESENTATION_ITEM()
RATIONAL_B_SPLINE_SURFACE(((0.996794362316491,0.998279055819231,1.,0.999218731101516,
0.99848615229188),(0.996794362316491,0.998279055819231,1.,0.999218731101516,
0.99848615229188)))
REPRESENTATION_ITEM('')
SURFACE()
);
#4270=(
BOUNDED_SURFACE()
B_SPLINE_SURFACE(1,2,((#166626,#166627,#166628,#166629,#166630),(#166631,
#166632,#166633,#166634,#166635)),.UNSPECIFIED.,.F.,.F.,.F.)
B_SPLINE_SURFACE_WITH_KNOTS((2,2),(3,2,3),(0.,0.05290454037812),(0.066525725473656,
0.0714285714285714,0.0736968668684962),.UNSPECIFIED.)
GEOMETRIC_REPRESENTATION_ITEM()
RATIONAL_B_SPLINE_SURFACE(((0.996794362316491,0.998279055819231,1.,0.999203807365457,
0.998458182734337),(0.996794362316491,0.998279055819231,1.,0.999203807365457,
0.998458182734337)))
REPRESENTATION_ITEM('')
SURFACE()
);
#4271=(
BOUNDED_SURFACE()
B_SPLINE_SURFACE(1,2,((#166646,#166647,#166648),(#166649,#166650,#166651)),
 .UNSPECIFIED.,.F.,.F.,.F.)
B_SPLINE_SURFACE_WITH_KNOTS((2,2),(3,3),(0.,0.0528815468798192),(0.659860018385657,
0.666841081426896),.UNSPECIFIED.)
GEOMETRIC_REPRESENTATION_ITEM()
RATIONAL_B_SPLINE_SURFACE(((0.990904995179334,0.989621173673357,0.988816334712146),
(0.990904995179334,0.989621173673357,0.988816334712146)))
REPRESENTATION_ITEM('')
SURFACE()
);
#4272=(
BOUNDED_SURFACE()
B_SPLINE_SURFACE(1,2,((#166653,#166654,#166655,#166656,#166657),(#166658,
#166659,#166660,#166661,#166662)),.UNSPECIFIED.,.F.,.F.,.F.)
B_SPLINE_SURFACE_WITH_KNOTS((2,2),(3,2,3),(0.938550151647622,1.00001008251049),
(0.659832011354088,0.659901408087482,0.666841081426896),.UNSPECIFIED.)
GEOMETRIC_REPRESENTATION_ITEM()
RATIONAL_B_SPLINE_SURFACE(((0.990889788836284,0.990889788836284,0.990889788836284,
0.98961640190086,0.988816334712146),(0.990889788836284,0.990889788836284,
0.990889788836284,0.98961640190086,0.988816334712146)))
REPRESENTATION_ITEM('')
SURFACE()
);
#4273=(
BOUNDED_SURFACE()
B_SPLINE_SURFACE(1,2,((#166664,#166665,#166666,#166667,#166668),(#166669,
#166670,#166671,#166672,#166673)),.UNSPECIFIED.,.F.,.F.,.F.)
B_SPLINE_SURFACE_WITH_KNOTS((2,2),(3,2,3),(0.,0.182885378421183),(0.0734807488197887,
0.0736543502199101,0.0910144902320514),.UNSPECIFIED.)
GEOMETRIC_REPRESENTATION_ITEM()
RATIONAL_B_SPLINE_SURFACE(((0.998486152291881,0.998486152291881,0.998486152291881,
0.992772345172012,0.990020524139833),(0.998486152291881,0.998486152291881,
0.998486152291881,0.992772345172012,0.990020524139833)))
REPRESENTATION_ITEM('')
SURFACE()
);
#4274=(
BOUNDED_SURFACE()
B_SPLINE_SURFACE(1,2,((#166684,#166685,#166686,#166687,#166688),(#166689,
#166690,#166691,#166692,#166693)),.UNSPECIFIED.,.F.,.F.,.F.)
B_SPLINE_SURFACE_WITH_KNOTS((2,2),(3,2,3),(0.,0.182805892339143),(0.642474614281368,
0.642857142857143,0.659901408087483),.UNSPECIFIED.)
GEOMETRIC_REPRESENTATION_ITEM()
RATIONAL_B_SPLINE_SURFACE(((0.999732896029238,0.999865728939373,1.,0.994017305594881,
0.990889788836284),(0.999732896029238,0.999865728939373,1.,0.994017305594881,
0.990889788836284)))
REPRESENTATION_ITEM('')
SURFACE()
);
#4275=(
BOUNDED_SURFACE()
B_SPLINE_SURFACE(1,2,((#166695,#166696,#166697,#166698,#166699),(#166700,
#166701,#166702,#166703,#166704)),.UNSPECIFIED.,.F.,.F.,.F.)
B_SPLINE_SURFACE_WITH_KNOTS((2,2),(3,2,3),(0.938576859128176,1.),(0.0665257254736562,
0.0714285714285714,0.0736543502199103),.UNSPECIFIED.)
GEOMETRIC_REPRESENTATION_ITEM()
RATIONAL_B_SPLINE_SURFACE(((0.996794362316491,0.998279055819231,1.,0.999218731101516,
0.99848615229188),(0.996794362316491,0.998279055819231,1.,0.999218731101516,
0.99848615229188)))
REPRESENTATION_ITEM('')
SURFACE()
);
#4276=(
BOUNDED_SURFACE()
B_SPLINE_SURFACE(1,2,((#166712,#166713,#166714,#166715,#166716),(#166717,
#166718,#166719,#166720,#166721)),.UNSPECIFIED.,.F.,.F.,.F.)
B_SPLINE_SURFACE_WITH_KNOTS((2,2),(3,2,3),(0.,0.0529045403781185),(0.0665257254736562,
0.0714285714285714,0.073696866868496),.UNSPECIFIED.)
GEOMETRIC_REPRESENTATION_ITEM()
RATIONAL_B_SPLINE_SURFACE(((0.996794362316491,0.998279055819231,1.,0.999203807365457,
0.998458182734336),(0.996794362316491,0.998279055819231,1.,0.999203807365457,
0.998458182734336)))
REPRESENTATION_ITEM('')
SURFACE()
);
#4277=(
BOUNDED_SURFACE()
B_SPLINE_SURFACE(1,2,((#166732,#166733,#166734),(#166735,#166736,#166737)),
 .UNSPECIFIED.,.F.,.F.,.F.)
B_SPLINE_SURFACE_WITH_KNOTS((2,2),(3,3),(0.,0.0528815468798166),(0.659860018385657,
0.666841081426896),.UNSPECIFIED.)
GEOMETRIC_REPRESENTATION_ITEM()
RATIONAL_B_SPLINE_SURFACE(((0.990904995179334,0.989621173673357,0.988816334712146),
(0.990904995179334,0.989621173673357,0.988816334712146)))
REPRESENTATION_ITEM('')
SURFACE()
);
#4278=(
BOUNDED_SURFACE()
B_SPLINE_SURFACE(1,2,((#166739,#166740,#166741,#166742,#166743),(#166744,
#166745,#166746,#166747,#166748)),.UNSPECIFIED.,.F.,.F.,.F.)
B_SPLINE_SURFACE_WITH_KNOTS((2,2),(3,2,3),(0.938550151647625,1.00001008244618),
(0.659832011354088,0.659901408087482,0.666841081426896),.UNSPECIFIED.)
GEOMETRIC_REPRESENTATION_ITEM()
RATIONAL_B_SPLINE_SURFACE(((0.990889788836284,0.990889788836284,0.990889788836284,
0.98961640190086,0.988816334712146),(0.990889788836284,0.990889788836284,
0.990889788836284,0.98961640190086,0.988816334712146)))
REPRESENTATION_ITEM('')
SURFACE()
);
#4279=(
BOUNDED_SURFACE()
B_SPLINE_SURFACE(1,2,((#166750,#166751,#166752,#166753,#166754),(#166755,
#166756,#166757,#166758,#166759)),.UNSPECIFIED.,.F.,.F.,.F.)
B_SPLINE_SURFACE_WITH_KNOTS((2,2),(3,2,3),(-1.06918541742082E-6,0.182885378421186),
(0.0734807488197885,0.0736543502199099,0.0910144902320512),
 .UNSPECIFIED.)
GEOMETRIC_REPRESENTATION_ITEM()
RATIONAL_B_SPLINE_SURFACE(((0.99848615229188,0.99848615229188,0.99848615229188,
0.992772345172012,0.990020524139833),(0.99848615229188,0.99848615229188,
0.99848615229188,0.992772345172012,0.990020524139833)))
REPRESENTATION_ITEM('')
SURFACE()
);
#4280=(
BOUNDED_SURFACE()
B_SPLINE_SURFACE(1,2,((#166770,#166771,#166772,#166773,#166774),(#166775,
#166776,#166777,#166778,#166779)),.UNSPECIFIED.,.F.,.F.,.F.)
B_SPLINE_SURFACE_WITH_KNOTS((2,2),(3,2,3),(0.,0.182805892339149),(0.642474614281367,
0.642857142857143,0.659901408087483),.UNSPECIFIED.)
GEOMETRIC_REPRESENTATION_ITEM()
RATIONAL_B_SPLINE_SURFACE(((0.999732896029238,0.999865728939373,1.,0.994017305594881,
0.990889788836284),(0.999732896029238,0.999865728939373,1.,0.994017305594881,
0.990889788836284)))
REPRESENTATION_ITEM('')
SURFACE()
);
#4281=(
BOUNDED_SURFACE()
B_SPLINE_SURFACE(1,2,((#166781,#166782,#166783,#166784,#166785),(#166786,
#166787,#166788,#166789,#166790)),.UNSPECIFIED.,.F.,.F.,.F.)
B_SPLINE_SURFACE_WITH_KNOTS((2,2),(3,2,3),(0.938576859128177,1.),(0.0665257254736559,
0.0714285714285714,0.0736543502199103),.UNSPECIFIED.)
GEOMETRIC_REPRESENTATION_ITEM()
RATIONAL_B_SPLINE_SURFACE(((0.996794362316491,0.998279055819231,1.,0.999218731101516,
0.99848615229188),(0.996794362316491,0.998279055819231,1.,0.999218731101516,
0.99848615229188)))
REPRESENTATION_ITEM('')
SURFACE()
);
#4282=(
BOUNDED_SURFACE()
B_SPLINE_SURFACE(1,2,((#166798,#166799,#166800,#166801,#166802),(#166803,
#166804,#166805,#166806,#166807)),.UNSPECIFIED.,.F.,.F.,.F.)
B_SPLINE_SURFACE_WITH_KNOTS((2,2),(3,2,3),(0.,0.0529045403781202),(0.0665257254736559,
0.0714285714285714,0.0736968668684961),.UNSPECIFIED.)
GEOMETRIC_REPRESENTATION_ITEM()
RATIONAL_B_SPLINE_SURFACE(((0.996794362316491,0.998279055819231,1.,0.999203807365457,
0.998458182734336),(0.996794362316491,0.998279055819231,1.,0.999203807365457,
0.998458182734336)))
REPRESENTATION_ITEM('')
SURFACE()
);
#4283=(
BOUNDED_SURFACE()
B_SPLINE_SURFACE(1,2,((#166818,#166819,#166820),(#166821,#166822,#166823)),
 .UNSPECIFIED.,.F.,.F.,.F.)
B_SPLINE_SURFACE_WITH_KNOTS((2,2),(3,3),(0.,0.052881546879819),(0.659860018385657,
0.666841081426897),.UNSPECIFIED.)
GEOMETRIC_REPRESENTATION_ITEM()
RATIONAL_B_SPLINE_SURFACE(((0.990904995179334,0.989621173673357,0.988816334712145),
(0.990904995179334,0.989621173673357,0.988816334712145)))
REPRESENTATION_ITEM('')
SURFACE()
);
#4284=(
BOUNDED_SURFACE()
B_SPLINE_SURFACE(1,2,((#166825,#166826,#166827,#166828,#166829),(#166830,
#166831,#166832,#166833,#166834)),.UNSPECIFIED.,.F.,.F.,.F.)
B_SPLINE_SURFACE_WITH_KNOTS((2,2),(3,2,3),(0.938550151647619,1.00001008245349),
(0.659832011354088,0.659901408087482,0.666841081426897),.UNSPECIFIED.)
GEOMETRIC_REPRESENTATION_ITEM()
RATIONAL_B_SPLINE_SURFACE(((0.990889788836284,0.990889788836284,0.990889788836284,
0.98961640190086,0.988816334712146),(0.990889788836284,0.990889788836284,
0.990889788836284,0.98961640190086,0.988816334712146)))
REPRESENTATION_ITEM('')
SURFACE()
);
#4285=(
BOUNDED_SURFACE()
B_SPLINE_SURFACE(1,2,((#166836,#166837,#166838,#166839,#166840),(#166841,
#166842,#166843,#166844,#166845)),.UNSPECIFIED.,.F.,.F.,.F.)
B_SPLINE_SURFACE_WITH_KNOTS((2,2),(3,2,3),(0.,0.182885378421186),(0.0734807488197886,
0.07365435021991,0.0910144902320513),.UNSPECIFIED.)
GEOMETRIC_REPRESENTATION_ITEM()
RATIONAL_B_SPLINE_SURFACE(((0.99848615229188,0.99848615229188,0.99848615229188,
0.992772345172012,0.990020524139833),(0.99848615229188,0.99848615229188,
0.99848615229188,0.992772345172012,0.990020524139833)))
REPRESENTATION_ITEM('')
SURFACE()
);
#4286=(
BOUNDED_SURFACE()
B_SPLINE_SURFACE(1,2,((#166856,#166857,#166858,#166859,#166860),(#166861,
#166862,#166863,#166864,#166865)),.UNSPECIFIED.,.F.,.F.,.F.)
B_SPLINE_SURFACE_WITH_KNOTS((2,2),(3,2,3),(0.,0.182805892339151),(0.642474614281368,
0.642857142857143,0.659901408087483),.UNSPECIFIED.)
GEOMETRIC_REPRESENTATION_ITEM()
RATIONAL_B_SPLINE_SURFACE(((0.999732896029238,0.999865728939373,1.,0.994017305594881,
0.990889788836284),(0.999732896029238,0.999865728939373,1.,0.994017305594881,
0.990889788836284)))
REPRESENTATION_ITEM('')
SURFACE()
);
#4287=(
BOUNDED_SURFACE()
B_SPLINE_SURFACE(1,2,((#166867,#166868,#166869,#166870,#166871),(#166872,
#166873,#166874,#166875,#166876)),.UNSPECIFIED.,.F.,.F.,.F.)
B_SPLINE_SURFACE_WITH_KNOTS((2,2),(3,2,3),(0.938576859128184,1.),(0.0665257254736563,
0.0714285714285714,0.07365435021991),.UNSPECIFIED.)
GEOMETRIC_REPRESENTATION_ITEM()
RATIONAL_B_SPLINE_SURFACE(((0.996794362316491,0.998279055819231,1.,0.999218731101516,
0.99848615229188),(0.996794362316491,0.998279055819231,1.,0.999218731101516,
0.99848615229188)))
REPRESENTATION_ITEM('')
SURFACE()
);
#4288=(
BOUNDED_SURFACE()
B_SPLINE_SURFACE(1,2,((#166883,#166884,#166885,#166886,#166887),(#166888,
#166889,#166890,#166891,#166892)),.UNSPECIFIED.,.F.,.F.,.F.)
B_SPLINE_SURFACE_WITH_KNOTS((2,2),(3,2,3),(0.,0.0529045403781217),(0.0665257254736563,
0.0714285714285714,0.073696866868496),.UNSPECIFIED.)
GEOMETRIC_REPRESENTATION_ITEM()
RATIONAL_B_SPLINE_SURFACE(((0.996794362316491,0.998279055819231,1.,0.999203807365457,
0.998458182734337),(0.996794362316491,0.998279055819231,1.,0.999203807365457,
0.998458182734337)))
REPRESENTATION_ITEM('')
SURFACE()
);
#4289=(
BOUNDED_SURFACE()
B_SPLINE_SURFACE(1,2,((#166903,#166904,#166905),(#166906,#166907,#166908)),
 .UNSPECIFIED.,.F.,.F.,.F.)
B_SPLINE_SURFACE_WITH_KNOTS((2,2),(3,3),(0.,0.0528815468798244),(0.659860018385657,
0.666841081426897),.UNSPECIFIED.)
GEOMETRIC_REPRESENTATION_ITEM()
RATIONAL_B_SPLINE_SURFACE(((0.990904995179334,0.989621173673357,0.988816334712146),
(0.990904995179334,0.989621173673357,0.988816334712146)))
REPRESENTATION_ITEM('')
SURFACE()
);
#4290=(
BOUNDED_SURFACE()
B_SPLINE_SURFACE(1,2,((#166910,#166911,#166912,#166913,#166914),(#166915,
#166916,#166917,#166918,#166919)),.UNSPECIFIED.,.F.,.F.,.F.)
B_SPLINE_SURFACE_WITH_KNOTS((2,2),(3,2,3),(0.93855015164762,1.0000100824797),
(0.659832011354088,0.659901408087482,0.666841081426897),.UNSPECIFIED.)
GEOMETRIC_REPRESENTATION_ITEM()
RATIONAL_B_SPLINE_SURFACE(((0.990889788836284,0.990889788836284,0.990889788836284,
0.98961640190086,0.988816334712146),(0.990889788836284,0.990889788836284,
0.990889788836284,0.98961640190086,0.988816334712146)))
REPRESENTATION_ITEM('')
SURFACE()
);
#4291=(
BOUNDED_SURFACE()
B_SPLINE_SURFACE(1,2,((#166921,#166922,#166923,#166924,#166925),(#166926,
#166927,#166928,#166929,#166930)),.UNSPECIFIED.,.F.,.F.,.F.)
B_SPLINE_SURFACE_WITH_KNOTS((2,2),(3,2,3),(0.,0.182885378421181),(0.0734807488197886,
0.07365435021991,0.0910144902320513),.UNSPECIFIED.)
GEOMETRIC_REPRESENTATION_ITEM()
RATIONAL_B_SPLINE_SURFACE(((0.998486152291881,0.998486152291881,0.998486152291881,
0.992772345172012,0.990020524139833),(0.998486152291881,0.998486152291881,
0.998486152291881,0.992772345172012,0.990020524139833)))
REPRESENTATION_ITEM('')
SURFACE()
);
#4292=(
BOUNDED_SURFACE()
B_SPLINE_SURFACE(1,2,((#166941,#166942,#166943,#166944,#166945),(#166946,
#166947,#166948,#166949,#166950)),.UNSPECIFIED.,.F.,.F.,.F.)
B_SPLINE_SURFACE_WITH_KNOTS((2,2),(3,2,3),(0.,0.182805892339142),(0.642474614281368,
0.642857142857143,0.659901408087482),.UNSPECIFIED.)
GEOMETRIC_REPRESENTATION_ITEM()
RATIONAL_B_SPLINE_SURFACE(((0.999732896029238,0.999865728939373,1.,0.994017305594881,
0.990889788836284),(0.999732896029238,0.999865728939373,1.,0.994017305594881,
0.990889788836284)))
REPRESENTATION_ITEM('')
SURFACE()
);
#4293=(
BOUNDED_SURFACE()
B_SPLINE_SURFACE(1,2,((#166952,#166953,#166954,#166955,#166956),(#166957,
#166958,#166959,#166960,#166961)),.UNSPECIFIED.,.F.,.F.,.F.)
B_SPLINE_SURFACE_WITH_KNOTS((2,2),(3,2,3),(0.938576859128179,1.),(0.0665257254736559,
0.0714285714285714,0.0736543502199101),.UNSPECIFIED.)
GEOMETRIC_REPRESENTATION_ITEM()
RATIONAL_B_SPLINE_SURFACE(((0.996794362316491,0.998279055819231,1.,0.999218731101516,
0.99848615229188),(0.996794362316491,0.998279055819231,1.,0.999218731101516,
0.99848615229188)))
REPRESENTATION_ITEM('')
SURFACE()
);
#4294=(
BOUNDED_SURFACE()
B_SPLINE_SURFACE(1,2,((#166968,#166969,#166970,#166971,#166972),(#166973,
#166974,#166975,#166976,#166977)),.UNSPECIFIED.,.F.,.F.,.F.)
B_SPLINE_SURFACE_WITH_KNOTS((2,2),(3,2,3),(0.,0.0529045403781215),(0.0665257254736559,
0.0714285714285714,0.073696866868496),.UNSPECIFIED.)
GEOMETRIC_REPRESENTATION_ITEM()
RATIONAL_B_SPLINE_SURFACE(((0.996794362316491,0.998279055819231,1.,0.999203807365457,
0.998458182734337),(0.996794362316491,0.998279055819231,1.,0.999203807365457,
0.998458182734337)))
REPRESENTATION_ITEM('')
SURFACE()
);
#4295=(
BOUNDED_SURFACE()
B_SPLINE_SURFACE(1,2,((#166988,#166989,#166990),(#166991,#166992,#166993)),
 .UNSPECIFIED.,.F.,.F.,.F.)
B_SPLINE_SURFACE_WITH_KNOTS((2,2),(3,3),(0.,0.0528815468798181),(0.659860018385657,
0.666841081426896),.UNSPECIFIED.)
GEOMETRIC_REPRESENTATION_ITEM()
RATIONAL_B_SPLINE_SURFACE(((0.990904995179334,0.989621173673357,0.988816334712146),
(0.990904995179334,0.989621173673357,0.988816334712146)))
REPRESENTATION_ITEM('')
SURFACE()
);
#4296=(
BOUNDED_SURFACE()
B_SPLINE_SURFACE(1,2,((#166995,#166996,#166997,#166998,#166999),(#167000,
#167001,#167002,#167003,#167004)),.UNSPECIFIED.,.F.,.F.,.F.)
B_SPLINE_SURFACE_WITH_KNOTS((2,2),(3,2,3),(0.938550151647624,1.00001008245332),
(0.659832011354088,0.659901408087482,0.666841081426896),.UNSPECIFIED.)
GEOMETRIC_REPRESENTATION_ITEM()
RATIONAL_B_SPLINE_SURFACE(((0.990889788836284,0.990889788836284,0.990889788836284,
0.98961640190086,0.988816334712146),(0.990889788836284,0.990889788836284,
0.990889788836284,0.98961640190086,0.988816334712146)))
REPRESENTATION_ITEM('')
SURFACE()
);
#4297=(
BOUNDED_SURFACE()
B_SPLINE_SURFACE(1,2,((#167006,#167007,#167008,#167009,#167010),(#167011,
#167012,#167013,#167014,#167015)),.UNSPECIFIED.,.F.,.F.,.F.)
B_SPLINE_SURFACE_WITH_KNOTS((2,2),(3,2,3),(0.,0.182885378421185),(0.0734807488197886,
0.07365435021991,0.0910144902320514),.UNSPECIFIED.)
GEOMETRIC_REPRESENTATION_ITEM()
RATIONAL_B_SPLINE_SURFACE(((0.998486152291881,0.998486152291881,0.998486152291881,
0.992772345172012,0.990020524139834),(0.998486152291881,0.998486152291881,
0.998486152291881,0.992772345172012,0.990020524139834)))
REPRESENTATION_ITEM('')
SURFACE()
);
#4298=(
BOUNDED_SURFACE()
B_SPLINE_SURFACE(1,2,((#167026,#167027,#167028,#167029,#167030),(#167031,
#167032,#167033,#167034,#167035)),.UNSPECIFIED.,.F.,.F.,.F.)
B_SPLINE_SURFACE_WITH_KNOTS((2,2),(3,2,3),(0.,0.182805892339144),(0.642474614281367,
0.642857142857143,0.659901408087591),.UNSPECIFIED.)
GEOMETRIC_REPRESENTATION_ITEM()
RATIONAL_B_SPLINE_SURFACE(((0.999732896029238,0.999865728939373,1.,0.994017305594843,
0.990889788836244),(0.999732896029238,0.999865728939373,1.,0.994017305594843,
0.990889788836244)))
REPRESENTATION_ITEM('')
SURFACE()
);
#4299=(
BOUNDED_SURFACE()
B_SPLINE_SURFACE(1,2,((#167037,#167038,#167039,#167040,#167041),(#167042,
#167043,#167044,#167045,#167046)),.UNSPECIFIED.,.F.,.F.,.F.)
B_SPLINE_SURFACE_WITH_KNOTS((2,2),(3,2,3),(0.938576859127265,1.),(0.0665257254736557,
0.0714285714285714,0.0736543502200163),.UNSPECIFIED.)
GEOMETRIC_REPRESENTATION_ITEM()
RATIONAL_B_SPLINE_SURFACE(((0.996794362316491,0.998279055819231,1.,0.999218731101479,
0.998486152291811),(0.996794362316491,0.998279055819231,1.,0.999218731101479,
0.998486152291811)))
REPRESENTATION_ITEM('')
SURFACE()
);
#4300=(
BOUNDED_SURFACE()
B_SPLINE_SURFACE(1,2,((#167054,#167055,#167056,#167057,#167058),(#167059,
#167060,#167061,#167062,#167063)),.UNSPECIFIED.,.F.,.F.,.F.)
B_SPLINE_SURFACE_WITH_KNOTS((2,2),(3,2,3),(0.,0.0529045403781241),(0.0665257254736563,
0.0714285714285714,0.0736968668684971),.UNSPECIFIED.)
GEOMETRIC_REPRESENTATION_ITEM()
RATIONAL_B_SPLINE_SURFACE(((0.996794362316491,0.998279055819231,1.,0.999203807365457,
0.998458182734336),(0.996794362316491,0.998279055819231,1.,0.999203807365457,
0.998458182734336)))
REPRESENTATION_ITEM('')
SURFACE()
);
#4301=(
BOUNDED_SURFACE()
B_SPLINE_SURFACE(1,2,((#167074,#167075,#167076),(#167077,#167078,#167079)),
 .UNSPECIFIED.,.F.,.F.,.F.)
B_SPLINE_SURFACE_WITH_KNOTS((2,2),(3,3),(0.,0.0528815468798234),(0.65986001838565,
0.666841081426896),.UNSPECIFIED.)
GEOMETRIC_REPRESENTATION_ITEM()
RATIONAL_B_SPLINE_SURFACE(((0.990904995179336,0.989621173673358,0.988816334712146),
(0.990904995179336,0.989621173673358,0.988816334712146)))
REPRESENTATION_ITEM('')
SURFACE()
);
#4302=(
BOUNDED_SURFACE()
B_SPLINE_SURFACE(1,2,((#167081,#167082,#167083,#167084,#167085),(#167086,
#167087,#167088,#167089,#167090)),.UNSPECIFIED.,.F.,.F.,.F.)
B_SPLINE_SURFACE_WITH_KNOTS((2,2),(3,2,3),(0.938550151647616,1.00001008250531),
(0.659832011354087,0.659901408087481,0.666841081426896),.UNSPECIFIED.)
GEOMETRIC_REPRESENTATION_ITEM()
RATIONAL_B_SPLINE_SURFACE(((0.990889788836284,0.990889788836284,0.990889788836284,
0.98961640190086,0.988816334712146),(0.990889788836284,0.990889788836284,
0.990889788836284,0.98961640190086,0.988816334712146)))
REPRESENTATION_ITEM('')
SURFACE()
);
#4303=(
BOUNDED_SURFACE()
B_SPLINE_SURFACE(1,2,((#167092,#167093,#167094,#167095,#167096),(#167097,
#167098,#167099,#167100,#167101)),.UNSPECIFIED.,.F.,.F.,.F.)
B_SPLINE_SURFACE_WITH_KNOTS((2,2),(3,2,3),(0.,0.182885378421189),(0.0734807488197897,
0.0736543502199111,0.0910144902320522),.UNSPECIFIED.)
GEOMETRIC_REPRESENTATION_ITEM()
RATIONAL_B_SPLINE_SURFACE(((0.99848615229188,0.99848615229188,0.99848615229188,
0.992772345172011,0.990020524139833),(0.99848615229188,0.99848615229188,
0.99848615229188,0.992772345172011,0.990020524139833)))
REPRESENTATION_ITEM('')
SURFACE()
);
#4304=(
BOUNDED_SURFACE()
B_SPLINE_SURFACE(1,2,((#167112,#167113,#167114,#167115,#167116),(#167117,
#167118,#167119,#167120,#167121)),.UNSPECIFIED.,.F.,.F.,.F.)
B_SPLINE_SURFACE_WITH_KNOTS((2,2),(3,2,3),(0.,0.182805892339155),(0.642474614281366,
0.642857142857143,0.659901408087481),.UNSPECIFIED.)
GEOMETRIC_REPRESENTATION_ITEM()
RATIONAL_B_SPLINE_SURFACE(((0.999732896029237,0.999865728939372,1.,0.994017305594881,
0.990889788836284),(0.999732896029237,0.999865728939372,1.,0.994017305594881,
0.990889788836284)))
REPRESENTATION_ITEM('')
SURFACE()
);
#4305=(
BOUNDED_SURFACE()
B_SPLINE_SURFACE(1,2,((#167123,#167124,#167125,#167126,#167127),(#167128,
#167129,#167130,#167131,#167132)),.UNSPECIFIED.,.F.,.F.,.F.)
B_SPLINE_SURFACE_WITH_KNOTS((2,2),(3,2,3),(0.938576859128167,1.),(0.0665257254736558,
0.0714285714285714,0.0736543502199113),.UNSPECIFIED.)
GEOMETRIC_REPRESENTATION_ITEM()
RATIONAL_B_SPLINE_SURFACE(((0.996794362316491,0.998279055819231,1.,0.999218731101516,
0.99848615229188),(0.996794362316491,0.998279055819231,1.,0.999218731101516,
0.99848615229188)))
REPRESENTATION_ITEM('')
SURFACE()
);
#4306=(
BOUNDED_SURFACE()
B_SPLINE_SURFACE(1,2,((#167140,#167141,#167142,#167143,#167144),(#167145,
#167146,#167147,#167148,#167149)),.UNSPECIFIED.,.F.,.F.,.F.)
B_SPLINE_SURFACE_WITH_KNOTS((2,2),(3,2,3),(0.,0.0529045403781334),(0.0665257254736558,
0.0714285714285714,0.0736968668684969),.UNSPECIFIED.)
GEOMETRIC_REPRESENTATION_ITEM()
RATIONAL_B_SPLINE_SURFACE(((0.996794362316491,0.998279055819231,1.,0.999203807365457,
0.998458182734336),(0.996794362316491,0.998279055819231,1.,0.999203807365457,
0.998458182734336)))
REPRESENTATION_ITEM('')
SURFACE()
);
#4307=(
BOUNDED_SURFACE()
B_SPLINE_SURFACE(1,2,((#167160,#167161,#167162),(#167163,#167164,#167165)),
 .UNSPECIFIED.,.F.,.F.,.F.)
B_SPLINE_SURFACE_WITH_KNOTS((2,2),(3,3),(0.,0.0528815468798287),(0.659860018385631,
0.666841081426896),.UNSPECIFIED.)
GEOMETRIC_REPRESENTATION_ITEM()
RATIONAL_B_SPLINE_SURFACE(((0.990904995179343,0.98962117367336,0.988816334712146),
(0.990904995179343,0.98962117367336,0.988816334712146)))
REPRESENTATION_ITEM('')
SURFACE()
);
#4308=(
BOUNDED_SURFACE()
B_SPLINE_SURFACE(1,2,((#167167,#167168,#167169,#167170,#167171),(#167172,
#167173,#167174,#167175,#167176)),.UNSPECIFIED.,.F.,.F.,.F.)
B_SPLINE_SURFACE_WITH_KNOTS((2,2),(3,2,3),(0.938550151647388,1.00001008248308),
(0.659832011354062,0.659901408087456,0.666841081426896),.UNSPECIFIED.)
GEOMETRIC_REPRESENTATION_ITEM()
RATIONAL_B_SPLINE_SURFACE(((0.990889788836293,0.990889788836293,0.990889788836293,
0.989616401900863,0.988816334712145),(0.990889788836293,0.990889788836293,
0.990889788836293,0.989616401900863,0.988816334712145)))
REPRESENTATION_ITEM('')
SURFACE()
);
#4309=(
BOUNDED_SURFACE()
B_SPLINE_SURFACE(1,2,((#167178,#167179,#167180,#167181,#167182),(#167183,
#167184,#167185,#167186,#167187)),.UNSPECIFIED.,.F.,.F.,.F.)
B_SPLINE_SURFACE_WITH_KNOTS((2,2),(3,2,3),(-1.06915738063826E-6,0.182885378421192),
(0.0734807488197634,0.0736543502198851,0.0910144902320526),
 .UNSPECIFIED.)
GEOMETRIC_REPRESENTATION_ITEM()
RATIONAL_B_SPLINE_SURFACE(((0.998486152291897,0.998486152291897,0.998486152291897,
0.992772345172015,0.990020524139833),(0.998486152291897,0.998486152291897,
0.998486152291897,0.992772345172015,0.990020524139833)))
REPRESENTATION_ITEM('')
SURFACE()
);
#4310=(
BOUNDED_SURFACE()
B_SPLINE_SURFACE(1,2,((#167198,#167199,#167200,#167201,#167202),(#167203,
#167204,#167205,#167206,#167207)),.UNSPECIFIED.,.F.,.F.,.F.)
B_SPLINE_SURFACE_WITH_KNOTS((2,2),(3,2,3),(0.,0.182805892339151),(0.642474614281366,
0.642857142857143,0.659901408087483),.UNSPECIFIED.)
GEOMETRIC_REPRESENTATION_ITEM()
RATIONAL_B_SPLINE_SURFACE(((0.999732896029237,0.999865728939372,1.,0.994017305594881,
0.990889788836284),(0.999732896029237,0.999865728939372,1.,0.994017305594881,
0.990889788836284)))
REPRESENTATION_ITEM('')
SURFACE()
);
#4311=(
BOUNDED_SURFACE()
B_SPLINE_SURFACE(1,2,((#167209,#167210,#167211,#167212,#167213),(#167214,
#167215,#167216,#167217,#167218)),.UNSPECIFIED.,.F.,.F.,.F.)
B_SPLINE_SURFACE_WITH_KNOTS((2,2),(3,2,3),(0.938576859128156,1.),(0.0665257254736561,
0.0714285714285714,0.0736543502199126),.UNSPECIFIED.)
GEOMETRIC_REPRESENTATION_ITEM()
RATIONAL_B_SPLINE_SURFACE(((0.996794362316491,0.998279055819231,1.,0.999218731101515,
0.998486152291879),(0.996794362316491,0.998279055819231,1.,0.999218731101515,
0.998486152291879)))
REPRESENTATION_ITEM('')
SURFACE()
);
#4312=(
BOUNDED_SURFACE()
B_SPLINE_SURFACE(1,2,((#167226,#167227,#167228,#167229,#167230),(#167231,
#167232,#167233,#167234,#167235)),.UNSPECIFIED.,.F.,.F.,.F.)
B_SPLINE_SURFACE_WITH_KNOTS((2,2),(3,2,3),(0.,0.0529045403781322),(0.066525725473656,
0.0714285714285714,0.0736968668684985),.UNSPECIFIED.)
GEOMETRIC_REPRESENTATION_ITEM()
RATIONAL_B_SPLINE_SURFACE(((0.996794362316491,0.998279055819231,1.,0.999203807365456,
0.998458182734335),(0.996794362316491,0.998279055819231,1.,0.999203807365456,
0.998458182734335)))
REPRESENTATION_ITEM('')
SURFACE()
);
#4313=(
BOUNDED_SURFACE()
B_SPLINE_SURFACE(1,2,((#167246,#167247,#167248),(#167249,#167250,#167251)),
 .UNSPECIFIED.,.F.,.F.,.F.)
B_SPLINE_SURFACE_WITH_KNOTS((2,2),(3,3),(0.,0.0528815468798286),(0.659860018385641,
0.666841081426896),.UNSPECIFIED.)
GEOMETRIC_REPRESENTATION_ITEM()
RATIONAL_B_SPLINE_SURFACE(((0.99090499517934,0.989621173673359,0.988816334712146),
(0.99090499517934,0.989621173673359,0.988816334712146)))
REPRESENTATION_ITEM('')
SURFACE()
);
#4314=(
BOUNDED_SURFACE()
B_SPLINE_SURFACE(1,2,((#167253,#167254,#167255,#167256,#167257),(#167258,
#167259,#167260,#167261,#167262)),.UNSPECIFIED.,.F.,.F.,.F.)
B_SPLINE_SURFACE_WITH_KNOTS((2,2),(3,2,3),(0.938550151647614,1.00001008252413),
(0.659832011354087,0.659901408087481,0.666841081426896),.UNSPECIFIED.)
GEOMETRIC_REPRESENTATION_ITEM()
RATIONAL_B_SPLINE_SURFACE(((0.990889788836284,0.990889788836284,0.990889788836284,
0.98961640190086,0.988816334712146),(0.990889788836284,0.990889788836284,
0.990889788836284,0.98961640190086,0.988816334712146)))
REPRESENTATION_ITEM('')
SURFACE()
);
#4315=(
BOUNDED_SURFACE()
B_SPLINE_SURFACE(1,2,((#167264,#167265,#167266,#167267,#167268),(#167269,
#167270,#167271,#167272,#167273)),.UNSPECIFIED.,.F.,.F.,.F.)
B_SPLINE_SURFACE_WITH_KNOTS((2,2),(3,2,3),(-1.07114226772793E-6,0.18288537842119),
(0.0734807488197897,0.0736543502199111,0.0910144902320524),
 .UNSPECIFIED.)
GEOMETRIC_REPRESENTATION_ITEM()
RATIONAL_B_SPLINE_SURFACE(((0.99848615229188,0.99848615229188,0.99848615229188,
0.992772345172011,0.990020524139833),(0.99848615229188,0.99848615229188,
0.99848615229188,0.992772345172011,0.990020524139833)))
REPRESENTATION_ITEM('')
SURFACE()
);
#4316=(
BOUNDED_SURFACE()
B_SPLINE_SURFACE(1,2,((#167284,#167285,#167286,#167287,#167288),(#167289,
#167290,#167291,#167292,#167293)),.UNSPECIFIED.,.F.,.F.,.F.)
B_SPLINE_SURFACE_WITH_KNOTS((2,2),(3,2,3),(0.,0.18280589233915),(0.642474614281367,
0.642857142857143,0.659901408087481),.UNSPECIFIED.)
GEOMETRIC_REPRESENTATION_ITEM()
RATIONAL_B_SPLINE_SURFACE(((0.999732896029237,0.999865728939372,1.,0.994017305594881,
0.990889788836284),(0.999732896029237,0.999865728939372,1.,0.994017305594881,
0.990889788836284)))
REPRESENTATION_ITEM('')
SURFACE()
);
#4317=(
BOUNDED_SURFACE()
B_SPLINE_SURFACE(1,2,((#167295,#167296,#167297,#167298,#167299),(#167300,
#167301,#167302,#167303,#167304)),.UNSPECIFIED.,.F.,.F.,.F.)
B_SPLINE_SURFACE_WITH_KNOTS((2,2),(3,2,3),(0.938576859128171,1.),(0.0665257254736561,
0.0714285714285714,0.0736543502199112),.UNSPECIFIED.)
GEOMETRIC_REPRESENTATION_ITEM()
RATIONAL_B_SPLINE_SURFACE(((0.996794362316491,0.998279055819231,1.,0.999218731101516,
0.99848615229188),(0.996794362316491,0.998279055819231,1.,0.999218731101516,
0.99848615229188)))
REPRESENTATION_ITEM('')
SURFACE()
);
#4318=(
BOUNDED_SURFACE()
B_SPLINE_SURFACE(1,2,((#167311,#167312,#167313,#167314,#167315),(#167316,
#167317,#167318,#167319,#167320)),.UNSPECIFIED.,.F.,.F.,.F.)
B_SPLINE_SURFACE_WITH_KNOTS((2,2),(3,2,3),(0.,0.0529045403781285),(0.0665257254736561,
0.0714285714285714,0.0736968668684971),.UNSPECIFIED.)
GEOMETRIC_REPRESENTATION_ITEM()
RATIONAL_B_SPLINE_SURFACE(((0.996794362316491,0.998279055819231,1.,0.999203807365457,
0.998458182734336),(0.996794362316491,0.998279055819231,1.,0.999203807365457,
0.998458182734336)))
REPRESENTATION_ITEM('')
SURFACE()
);
#4319=(
BOUNDED_SURFACE()
B_SPLINE_SURFACE(1,2,((#167331,#167332,#167333),(#167334,#167335,#167336)),
 .UNSPECIFIED.,.F.,.F.,.F.)
B_SPLINE_SURFACE_WITH_KNOTS((2,2),(3,3),(0.,0.0528815468798285),(0.659860018385656,
0.666841081426896),.UNSPECIFIED.)
GEOMETRIC_REPRESENTATION_ITEM()
RATIONAL_B_SPLINE_SURFACE(((0.990904995179334,0.989621173673357,0.988816334712145),
(0.990904995179334,0.989621173673357,0.988816334712145)))
REPRESENTATION_ITEM('')
SURFACE()
);
#4320=(
BOUNDED_SURFACE()
B_SPLINE_SURFACE(1,2,((#167338,#167339,#167340,#167341,#167342),(#167343,
#167344,#167345,#167346,#167347)),.UNSPECIFIED.,.F.,.F.,.F.)
B_SPLINE_SURFACE_WITH_KNOTS((2,2),(3,2,3),(0.938550151647616,1.00001008244981),
(0.659832011354087,0.659901408087481,0.666841081426896),.UNSPECIFIED.)
GEOMETRIC_REPRESENTATION_ITEM()
RATIONAL_B_SPLINE_SURFACE(((0.990889788836284,0.990889788836284,0.990889788836284,
0.98961640190086,0.988816334712146),(0.990889788836284,0.990889788836284,
0.990889788836284,0.98961640190086,0.988816334712146)))
REPRESENTATION_ITEM('')
SURFACE()
);
#4321=(
BOUNDED_SURFACE()
B_SPLINE_SURFACE(1,2,((#167349,#167350,#167351,#167352,#167353),(#167354,
#167355,#167356,#167357,#167358)),.UNSPECIFIED.,.F.,.F.,.F.)
B_SPLINE_SURFACE_WITH_KNOTS((2,2),(3,2,3),(0.,0.182885378421189),(0.0734807488197897,
0.0736543502199111,0.0910144902320524),.UNSPECIFIED.)
GEOMETRIC_REPRESENTATION_ITEM()
RATIONAL_B_SPLINE_SURFACE(((0.99848615229188,0.99848615229188,0.99848615229188,
0.992772345172011,0.990020524139833),(0.99848615229188,0.99848615229188,
0.99848615229188,0.992772345172011,0.990020524139833)))
REPRESENTATION_ITEM('')
SURFACE()
);
#4322=(
BOUNDED_SURFACE()
B_SPLINE_SURFACE(1,2,((#167369,#167370,#167371,#167372,#167373),(#167374,
#167375,#167376,#167377,#167378)),.UNSPECIFIED.,.F.,.F.,.F.)
B_SPLINE_SURFACE_WITH_KNOTS((2,2),(3,2,3),(0.,0.182805892339155),(0.642474614281366,
0.642857142857143,0.659901408087482),.UNSPECIFIED.)
GEOMETRIC_REPRESENTATION_ITEM()
RATIONAL_B_SPLINE_SURFACE(((0.999732896029237,0.999865728939372,1.,0.994017305594881,
0.990889788836284),(0.999732896029237,0.999865728939372,1.,0.994017305594881,
0.990889788836284)))
REPRESENTATION_ITEM('')
SURFACE()
);
#4323=(
BOUNDED_SURFACE()
B_SPLINE_SURFACE(1,2,((#167380,#167381,#167382,#167383,#167384),(#167385,
#167386,#167387,#167388,#167389)),.UNSPECIFIED.,.F.,.F.,.F.)
B_SPLINE_SURFACE_WITH_KNOTS((2,2),(3,2,3),(0.938576859128165,1.),(0.0665257254736557,
0.0714285714285714,0.0736543502199114),.UNSPECIFIED.)
GEOMETRIC_REPRESENTATION_ITEM()
RATIONAL_B_SPLINE_SURFACE(((0.996794362316491,0.998279055819231,1.,0.999218731101516,
0.99848615229188),(0.996794362316491,0.998279055819231,1.,0.999218731101516,
0.99848615229188)))
REPRESENTATION_ITEM('')
SURFACE()
);
#4324=(
BOUNDED_SURFACE()
B_SPLINE_SURFACE(1,2,((#167397,#167398,#167399,#167400,#167401),(#167402,
#167403,#167404,#167405,#167406)),.UNSPECIFIED.,.F.,.F.,.F.)
B_SPLINE_SURFACE_WITH_KNOTS((2,2),(3,2,3),(0.,0.0529045403781337),(0.0665257254736557,
0.0714285714285714,0.0736968668684971),.UNSPECIFIED.)
GEOMETRIC_REPRESENTATION_ITEM()
RATIONAL_B_SPLINE_SURFACE(((0.996794362316491,0.998279055819231,1.,0.999203807365457,
0.998458182734336),(0.996794362316491,0.998279055819231,1.,0.999203807365457,
0.998458182734336)))
REPRESENTATION_ITEM('')
SURFACE()
);
#4325=(
BOUNDED_SURFACE()
B_SPLINE_SURFACE(1,2,((#167417,#167418,#167419),(#167420,#167421,#167422)),
 .UNSPECIFIED.,.F.,.F.,.F.)
B_SPLINE_SURFACE_WITH_KNOTS((2,2),(3,3),(0.,0.0528815468798329),(0.659860018385558,
0.666841081426897),.UNSPECIFIED.)
GEOMETRIC_REPRESENTATION_ITEM()
RATIONAL_B_SPLINE_SURFACE(((0.99090499517937,0.989621173673368,0.988816334712145),
(0.99090499517937,0.989621173673368,0.988816334712145)))
REPRESENTATION_ITEM('')
SURFACE()
);
#4326=(
BOUNDED_SURFACE()
B_SPLINE_SURFACE(1,2,((#167424,#167425,#167426,#167427,#167428),(#167429,
#167430,#167431,#167432,#167433)),.UNSPECIFIED.,.F.,.F.,.F.)
B_SPLINE_SURFACE_WITH_KNOTS((2,2),(3,2,3),(0.938550151647612,1.00001008245693),
(0.659832011354087,0.659901408087481,0.666841081426897),.UNSPECIFIED.)
GEOMETRIC_REPRESENTATION_ITEM()
RATIONAL_B_SPLINE_SURFACE(((0.990889788836284,0.990889788836284,0.990889788836284,
0.98961640190086,0.988816334712146),(0.990889788836284,0.990889788836284,
0.990889788836284,0.98961640190086,0.988816334712146)))
REPRESENTATION_ITEM('')
SURFACE()
);
#4327=(
BOUNDED_SURFACE()
B_SPLINE_SURFACE(1,2,((#167435,#167436,#167437,#167438,#167439),(#167440,
#167441,#167442,#167443,#167444)),.UNSPECIFIED.,.F.,.F.,.F.)
B_SPLINE_SURFACE_WITH_KNOTS((2,2),(3,2,3),(0.,0.182885378421192),(0.0734807488197897,
0.0736543502199111,0.0910144902320528),.UNSPECIFIED.)
GEOMETRIC_REPRESENTATION_ITEM()
RATIONAL_B_SPLINE_SURFACE(((0.99848615229188,0.99848615229188,0.99848615229188,
0.992772345172011,0.990020524139833),(0.99848615229188,0.99848615229188,
0.99848615229188,0.992772345172011,0.990020524139833)))
REPRESENTATION_ITEM('')
SURFACE()
);
#4328=(
BOUNDED_SURFACE()
B_SPLINE_SURFACE(1,2,((#167455,#167456,#167457,#167458,#167459),(#167460,
#167461,#167462,#167463,#167464)),.UNSPECIFIED.,.F.,.F.,.F.)
B_SPLINE_SURFACE_WITH_KNOTS((2,2),(3,2,3),(0.,0.182805892339158),(0.642474614281367,
0.642857142857143,0.659901408087481),.UNSPECIFIED.)
GEOMETRIC_REPRESENTATION_ITEM()
RATIONAL_B_SPLINE_SURFACE(((0.999732896029238,0.999865728939373,1.,0.994017305594881,
0.990889788836284),(0.999732896029238,0.999865728939373,1.,0.994017305594881,
0.990889788836284)))
REPRESENTATION_ITEM('')
SURFACE()
);
#4329=(
BOUNDED_SURFACE()
B_SPLINE_SURFACE(1,2,((#167466,#167467,#167468,#167469,#167470),(#167471,
#167472,#167473,#167474,#167475)),.UNSPECIFIED.,.F.,.F.,.F.)
B_SPLINE_SURFACE_WITH_KNOTS((2,2),(3,2,3),(0.938576859128171,1.),(0.0665257254736564,
0.0714285714285714,0.0736543502199112),.UNSPECIFIED.)
GEOMETRIC_REPRESENTATION_ITEM()
RATIONAL_B_SPLINE_SURFACE(((0.996794362316492,0.998279055819231,1.,0.999218731101516,
0.99848615229188),(0.996794362316492,0.998279055819231,1.,0.999218731101516,
0.99848615229188)))
REPRESENTATION_ITEM('')
SURFACE()
);
#4330=(
BOUNDED_SURFACE()
B_SPLINE_SURFACE(1,2,((#167482,#167483,#167484,#167485,#167486),(#167487,
#167488,#167489,#167490,#167491)),.UNSPECIFIED.,.F.,.F.,.F.)
B_SPLINE_SURFACE_WITH_KNOTS((2,2),(3,2,3),(0.,0.052904540378125),(0.0665257254736564,
0.0714285714285714,0.0736968668684972),.UNSPECIFIED.)
GEOMETRIC_REPRESENTATION_ITEM()
RATIONAL_B_SPLINE_SURFACE(((0.996794362316492,0.998279055819231,1.,0.999203807365457,
0.998458182734336),(0.996794362316492,0.998279055819231,1.,0.999203807365457,
0.998458182734336)))
REPRESENTATION_ITEM('')
SURFACE()
);
#4331=(
BOUNDED_SURFACE()
B_SPLINE_SURFACE(1,2,((#167502,#167503,#167504),(#167505,#167506,#167507)),
 .UNSPECIFIED.,.F.,.F.,.F.)
B_SPLINE_SURFACE_WITH_KNOTS((2,2),(3,3),(0.,0.0528815468798311),(0.659860018385656,
0.666841081426897),.UNSPECIFIED.)
GEOMETRIC_REPRESENTATION_ITEM()
RATIONAL_B_SPLINE_SURFACE(((0.990904995179334,0.989621173673357,0.988816334712145),
(0.990904995179334,0.989621173673357,0.988816334712145)))
REPRESENTATION_ITEM('')
SURFACE()
);
#4332=(
BOUNDED_SURFACE()
B_SPLINE_SURFACE(1,2,((#167509,#167510,#167511,#167512,#167513),(#167514,
#167515,#167516,#167517,#167518)),.UNSPECIFIED.,.F.,.F.,.F.)
B_SPLINE_SURFACE_WITH_KNOTS((2,2),(3,2,3),(0.938550151647611,1.00001008249664),
(0.659832011354087,0.659901408087481,0.666841081426897),.UNSPECIFIED.)
GEOMETRIC_REPRESENTATION_ITEM()
RATIONAL_B_SPLINE_SURFACE(((0.990889788836284,0.990889788836284,0.990889788836284,
0.98961640190086,0.988816334712146),(0.990889788836284,0.990889788836284,
0.990889788836284,0.98961640190086,0.988816334712146)))
REPRESENTATION_ITEM('')
SURFACE()
);
#4333=(
BOUNDED_SURFACE()
B_SPLINE_SURFACE(1,2,((#167520,#167521,#167522,#167523,#167524),(#167525,
#167526,#167527,#167528,#167529)),.UNSPECIFIED.,.F.,.F.,.F.)
B_SPLINE_SURFACE_WITH_KNOTS((2,2),(3,2,3),(-1.06908625210514E-6,0.182885378421192),
(0.0734807488197897,0.0736543502199111,0.0910144902320523),
 .UNSPECIFIED.)
GEOMETRIC_REPRESENTATION_ITEM()
RATIONAL_B_SPLINE_SURFACE(((0.99848615229188,0.99848615229188,0.99848615229188,
0.992772345172011,0.990020524139833),(0.99848615229188,0.99848615229188,
0.99848615229188,0.992772345172011,0.990020524139833)))
REPRESENTATION_ITEM('')
SURFACE()
);
#4334=(
BOUNDED_SURFACE()
B_SPLINE_SURFACE(1,2,((#167540,#167541,#167542,#167543,#167544),(#167545,
#167546,#167547,#167548,#167549)),.UNSPECIFIED.,.F.,.F.,.F.)
B_SPLINE_SURFACE_WITH_KNOTS((2,2),(3,2,3),(0.,0.182805892339156),(0.642474614281366,
0.642857142857143,0.659901408087482),.UNSPECIFIED.)
GEOMETRIC_REPRESENTATION_ITEM()
RATIONAL_B_SPLINE_SURFACE(((0.999732896029237,0.999865728939372,1.,0.994017305594881,
0.990889788836284),(0.999732896029237,0.999865728939372,1.,0.994017305594881,
0.990889788836284)))
REPRESENTATION_ITEM('')
SURFACE()
);
#4335=(
BOUNDED_SURFACE()
B_SPLINE_SURFACE(1,2,((#167551,#167552,#167553,#167554,#167555),(#167556,
#167557,#167558,#167559,#167560)),.UNSPECIFIED.,.F.,.F.,.F.)
B_SPLINE_SURFACE_WITH_KNOTS((2,2),(3,2,3),(0.938576859128167,1.),(0.0665257254736567,
0.0714285714285714,0.0736543502199119),.UNSPECIFIED.)
GEOMETRIC_REPRESENTATION_ITEM()
RATIONAL_B_SPLINE_SURFACE(((0.996794362316492,0.998279055819231,1.,0.999218731101515,
0.998486152291879),(0.996794362316492,0.998279055819231,1.,0.999218731101515,
0.998486152291879)))
REPRESENTATION_ITEM('')
SURFACE()
);
#4336=(
BOUNDED_SURFACE()
B_SPLINE_SURFACE(1,2,((#167568,#167569,#167570,#167571,#167572),(#167573,
#167574,#167575,#167576,#167577)),.UNSPECIFIED.,.F.,.F.,.F.)
B_SPLINE_SURFACE_WITH_KNOTS((2,2),(3,2,3),(0.,0.0529045403781293),(0.0665257254736565,
0.0714285714285714,0.0736968668684979),.UNSPECIFIED.)
GEOMETRIC_REPRESENTATION_ITEM()
RATIONAL_B_SPLINE_SURFACE(((0.996794362316492,0.998279055819231,1.,0.999203807365456,
0.998458182734335),(0.996794362316492,0.998279055819231,1.,0.999203807365456,
0.998458182734335)))
REPRESENTATION_ITEM('')
SURFACE()
);
#4337=(
BOUNDED_SURFACE()
B_SPLINE_SURFACE(1,2,((#167588,#167589,#167590),(#167591,#167592,#167593)),
 .UNSPECIFIED.,.F.,.F.,.F.)
B_SPLINE_SURFACE_WITH_KNOTS((2,2),(3,3),(0.,0.0528815468798305),(0.659860018385656,
0.666841081426896),.UNSPECIFIED.)
GEOMETRIC_REPRESENTATION_ITEM()
RATIONAL_B_SPLINE_SURFACE(((0.990904995179334,0.989621173673357,0.988816334712145),
(0.990904995179334,0.989621173673357,0.988816334712145)))
REPRESENTATION_ITEM('')
SURFACE()
);
#4338=(
BOUNDED_SURFACE()
B_SPLINE_SURFACE(1,2,((#167595,#167596,#167597,#167598,#167599),(#167600,
#167601,#167602,#167603,#167604)),.UNSPECIFIED.,.F.,.F.,.F.)
B_SPLINE_SURFACE_WITH_KNOTS((2,2),(3,2,3),(0.938550151643589,1.00001008249256),
(0.659832011353627,0.659901408087026,0.666841081426899),.UNSPECIFIED.)
GEOMETRIC_REPRESENTATION_ITEM()
RATIONAL_B_SPLINE_SURFACE(((0.990889788836451,0.990889788836451,0.990889788836451,
0.989616401900912,0.988816334712145),(0.990889788836451,0.990889788836451,
0.990889788836451,0.989616401900912,0.988816334712145)))
REPRESENTATION_ITEM('')
SURFACE()
);
#4339=(
BOUNDED_SURFACE()
B_SPLINE_SURFACE(1,2,((#167606,#167607,#167608,#167609,#167610),(#167611,
#167612,#167613,#167614,#167615)),.UNSPECIFIED.,.F.,.F.,.F.)
B_SPLINE_SURFACE_WITH_KNOTS((2,2),(3,2,3),(-1.06896686295104E-6,0.18288537842119),
(0.0734807488195811,0.0736543502197046,0.0910144902320537),
 .UNSPECIFIED.)
GEOMETRIC_REPRESENTATION_ITEM()
RATIONAL_B_SPLINE_SURFACE(((0.998486152292016,0.998486152292016,0.998486152292016,
0.992772345172043,0.990020524139833),(0.998486152292016,0.998486152292016,
0.998486152292016,0.992772345172043,0.990020524139833)))
REPRESENTATION_ITEM('')
SURFACE()
);
#4340=(
BOUNDED_SURFACE()
B_SPLINE_SURFACE(1,2,((#167626,#167627,#167628,#167629,#167630),(#167631,
#167632,#167633,#167634,#167635)),.UNSPECIFIED.,.F.,.F.,.F.)
B_SPLINE_SURFACE_WITH_KNOTS((2,2),(3,2,3),(0.,0.182805892339159),(0.642474614281366,
0.642857142857143,0.659901408087481),.UNSPECIFIED.)
GEOMETRIC_REPRESENTATION_ITEM()
RATIONAL_B_SPLINE_SURFACE(((0.999732896029237,0.999865728939372,1.,0.994017305594881,
0.990889788836284),(0.999732896029237,0.999865728939372,1.,0.994017305594881,
0.990889788836284)))
REPRESENTATION_ITEM('')
SURFACE()
);
#4341=(
BOUNDED_SURFACE()
B_SPLINE_SURFACE(1,2,((#167637,#167638,#167639,#167640,#167641),(#167642,
#167643,#167644,#167645,#167646)),.UNSPECIFIED.,.F.,.F.,.F.)
B_SPLINE_SURFACE_WITH_KNOTS((2,2),(3,2,3),(0.938576859128175,1.),(0.0665257254736565,
0.0714285714285714,0.0736543502199112),.UNSPECIFIED.)
GEOMETRIC_REPRESENTATION_ITEM()
RATIONAL_B_SPLINE_SURFACE(((0.996794362316492,0.998279055819231,1.,0.999218731101516,
0.99848615229188),(0.996794362316492,0.998279055819231,1.,0.999218731101516,
0.99848615229188)))
REPRESENTATION_ITEM('')
SURFACE()
);
#4342=(
BOUNDED_SURFACE()
B_SPLINE_SURFACE(1,2,((#167652,#167653,#167654,#167655,#167656),(#167657,
#167658,#167659,#167660,#167661)),.UNSPECIFIED.,.F.,.F.,.F.)
B_SPLINE_SURFACE_WITH_KNOTS((2,2),(3,2,3),(0.,0.0525890063985138),(0.0665682420727563,
0.0714285714285714,0.0736543503731481),.UNSPECIFIED.)
GEOMETRIC_REPRESENTATION_ITEM()
RATIONAL_B_SPLINE_SURFACE(((0.996820130073177,0.99829397953792,1.,0.999218731047729,
0.998486152191009),(0.996820130073177,0.99829397953792,1.,0.999218731047729,
0.998486152191009)))
REPRESENTATION_ITEM('')
SURFACE()
);
#4343=(
BOUNDED_SURFACE()
B_SPLINE_SURFACE(1,2,((#167672,#167673,#167674),(#167675,#167676,#167677)),
 .UNSPECIFIED.,.F.,.F.,.F.)
B_SPLINE_SURFACE_WITH_KNOTS((2,2),(3,3),(0.,0.0528815468798306),(0.659860018385656,
0.666841081426897),.UNSPECIFIED.)
GEOMETRIC_REPRESENTATION_ITEM()
RATIONAL_B_SPLINE_SURFACE(((0.990904995179334,0.989621173673357,0.988816334712145),
(0.990904995179334,0.989621173673357,0.988816334712146)))
REPRESENTATION_ITEM('')
SURFACE()
);
#4344=(
BOUNDED_SURFACE()
B_SPLINE_SURFACE(1,2,((#167679,#167680,#167681,#167682,#167683),(#167684,
#167685,#167686,#167687,#167688)),.UNSPECIFIED.,.F.,.F.,.F.)
B_SPLINE_SURFACE_WITH_KNOTS((2,2),(3,2,3),(0.938550151647611,1.00001008245607),
(0.659832011354087,0.659901408087481,0.666841081426897),.UNSPECIFIED.)
GEOMETRIC_REPRESENTATION_ITEM()
RATIONAL_B_SPLINE_SURFACE(((0.990889788836284,0.990889788836284,0.990889788836284,
0.98961640190086,0.988816334712146),(0.990889788836284,0.990889788836284,
0.990889788836284,0.98961640190086,0.988816334712146)))
REPRESENTATION_ITEM('')
SURFACE()
);
#4345=(
BOUNDED_SURFACE()
B_SPLINE_SURFACE(1,2,((#167690,#167691,#167692,#167693,#167694),(#167695,
#167696,#167697,#167698,#167699)),.UNSPECIFIED.,.F.,.F.,.F.)
B_SPLINE_SURFACE_WITH_KNOTS((2,2),(3,2,3),(-1.07106247283029E-6,0.182885378421187),
(0.0734807488197897,0.0736543502199111,0.0910144902320524),
 .UNSPECIFIED.)
GEOMETRIC_REPRESENTATION_ITEM()
RATIONAL_B_SPLINE_SURFACE(((0.99848615229188,0.99848615229188,0.99848615229188,
0.992772345172011,0.990020524139833),(0.99848615229188,0.99848615229188,
0.99848615229188,0.992772345172011,0.990020524139833)))
REPRESENTATION_ITEM('')
SURFACE()
);
#4346=(
BOUNDED_SURFACE()
B_SPLINE_SURFACE(1,2,((#167710,#167711,#167712,#167713,#167714),(#167715,
#167716,#167717,#167718,#167719)),.UNSPECIFIED.,.F.,.F.,.F.)
B_SPLINE_SURFACE_WITH_KNOTS((2,2),(3,2,3),(0.,0.182805892339153),(0.642474614281367,
0.642857142857143,0.659901408087481),.UNSPECIFIED.)
GEOMETRIC_REPRESENTATION_ITEM()
RATIONAL_B_SPLINE_SURFACE(((0.999732896029237,0.999865728939372,1.,0.994017305594881,
0.990889788836284),(0.999732896029237,0.999865728939372,1.,0.994017305594881,
0.990889788836284)))
REPRESENTATION_ITEM('')
SURFACE()
);
#4347=(
BOUNDED_SURFACE()
B_SPLINE_SURFACE(1,2,((#167721,#167722,#167723,#167724,#167725),(#167726,
#167727,#167728,#167729,#167730)),.UNSPECIFIED.,.F.,.F.,.F.)
B_SPLINE_SURFACE_WITH_KNOTS((2,2),(3,2,3),(0.938576859128174,1.),(0.0665257254736566,
0.0714285714285714,0.0736543502199112),.UNSPECIFIED.)
GEOMETRIC_REPRESENTATION_ITEM()
RATIONAL_B_SPLINE_SURFACE(((0.996794362316492,0.998279055819231,1.,0.999218731101516,
0.99848615229188),(0.996794362316492,0.998279055819231,1.,0.999218731101516,
0.99848615229188)))
REPRESENTATION_ITEM('')
SURFACE()
);
#4348=(
BOUNDED_SURFACE()
B_SPLINE_SURFACE(1,2,((#167738,#167739,#167740,#167741,#167742),(#167743,
#167744,#167745,#167746,#167747)),.UNSPECIFIED.,.F.,.F.,.F.)
B_SPLINE_SURFACE_WITH_KNOTS((2,2),(3,2,3),(0.,0.0529045403781294),(0.0665257254736564,
0.0714285714285714,0.0736968668684973),.UNSPECIFIED.)
GEOMETRIC_REPRESENTATION_ITEM()
RATIONAL_B_SPLINE_SURFACE(((0.996794362316492,0.998279055819231,1.,0.999203807365457,
0.998458182734336),(0.996794362316492,0.998279055819231,1.,0.999203807365457,
0.998458182734336)))
REPRESENTATION_ITEM('')
SURFACE()
);
#4349=(
BOUNDED_SURFACE()
B_SPLINE_SURFACE(1,2,((#167758,#167759,#167760),(#167761,#167762,#167763)),
 .UNSPECIFIED.,.F.,.F.,.F.)
B_SPLINE_SURFACE_WITH_KNOTS((2,2),(3,3),(0.,0.0528815468798319),(0.659860018385656,
0.666841081426897),.UNSPECIFIED.)
GEOMETRIC_REPRESENTATION_ITEM()
RATIONAL_B_SPLINE_SURFACE(((0.990904995179334,0.989621173673357,0.988816334712146),
(0.990904995179334,0.989621173673357,0.988816334712146)))
REPRESENTATION_ITEM('')
SURFACE()
);
#4350=(
BOUNDED_SURFACE()
B_SPLINE_SURFACE(1,2,((#167765,#167766,#167767,#167768,#167769),(#167770,
#167771,#167772,#167773,#167774)),.UNSPECIFIED.,.F.,.F.,.F.)
B_SPLINE_SURFACE_WITH_KNOTS((2,2),(3,2,3),(0.938550151647611,1.00001008245706),
(0.659832011354087,0.659901408087481,0.666841081426897),.UNSPECIFIED.)
GEOMETRIC_REPRESENTATION_ITEM()
RATIONAL_B_SPLINE_SURFACE(((0.990889788836284,0.990889788836284,0.990889788836284,
0.98961640190086,0.988816334712145),(0.990889788836284,0.990889788836284,
0.990889788836284,0.98961640190086,0.988816334712145)))
REPRESENTATION_ITEM('')
SURFACE()
);
#4351=(
BOUNDED_SURFACE()
B_SPLINE_SURFACE(1,2,((#167776,#167777,#167778,#167779,#167780),(#167781,
#167782,#167783,#167784,#167785)),.UNSPECIFIED.,.F.,.F.,.F.)
B_SPLINE_SURFACE_WITH_KNOTS((2,2),(3,2,3),(-1.06904910472764E-6,0.182885378421189),
(0.0734807488197898,0.0736543502199112,0.0910144902320519),
 .UNSPECIFIED.)
GEOMETRIC_REPRESENTATION_ITEM()
RATIONAL_B_SPLINE_SURFACE(((0.99848615229188,0.99848615229188,0.99848615229188,
0.992772345172011,0.990020524139833),(0.99848615229188,0.99848615229188,
0.99848615229188,0.992772345172011,0.990020524139833)))
REPRESENTATION_ITEM('')
SURFACE()
);
#4352=(
BOUNDED_SURFACE()
B_SPLINE_SURFACE(1,2,((#167796,#167797,#167798,#167799,#167800),(#167801,
#167802,#167803,#167804,#167805)),.UNSPECIFIED.,.F.,.F.,.F.)
B_SPLINE_SURFACE_WITH_KNOTS((2,2),(3,2,3),(0.,0.18280589233916),(0.642474614281364,
0.642857142857143,0.659901408087481),.UNSPECIFIED.)
GEOMETRIC_REPRESENTATION_ITEM()
RATIONAL_B_SPLINE_SURFACE(((0.999732896029236,0.999865728939372,1.,0.994017305594881,
0.990889788836284),(0.999732896029236,0.999865728939372,1.,0.994017305594881,
0.990889788836284)))
REPRESENTATION_ITEM('')
SURFACE()
);
#4353=(
BOUNDED_SURFACE()
B_SPLINE_SURFACE(1,2,((#167807,#167808,#167809,#167810,#167811),(#167812,
#167813,#167814,#167815,#167816)),.UNSPECIFIED.,.F.,.F.,.F.)
B_SPLINE_SURFACE_WITH_KNOTS((2,2),(3,2,3),(0.938576859128167,1.),(0.066525725473656,
0.0714285714285714,0.0736543502199112),.UNSPECIFIED.)
GEOMETRIC_REPRESENTATION_ITEM()
RATIONAL_B_SPLINE_SURFACE(((0.996794362316491,0.998279055819231,1.,0.999218731101516,
0.99848615229188),(0.996794362316491,0.998279055819231,1.,0.999218731101516,
0.99848615229188)))
REPRESENTATION_ITEM('')
SURFACE()
);
#4354=(
BOUNDED_SURFACE()
B_SPLINE_SURFACE(1,2,((#167823,#167824,#167825,#167826,#167827),(#167828,
#167829,#167830,#167831,#167832)),.UNSPECIFIED.,.F.,.F.,.F.)
B_SPLINE_SURFACE_WITH_KNOTS((2,2),(3,2,3),(0.,0.0529045403781331),(0.0665257254736559,
0.0714285714285714,0.0736968668684971),.UNSPECIFIED.)
GEOMETRIC_REPRESENTATION_ITEM()
RATIONAL_B_SPLINE_SURFACE(((0.996794362316491,0.998279055819231,1.,0.999203807365457,
0.998458182734336),(0.996794362316491,0.998279055819231,1.,0.999203807365457,
0.998458182734336)))
REPRESENTATION_ITEM('')
SURFACE()
);
#4355=(
BOUNDED_SURFACE()
B_SPLINE_SURFACE(1,2,((#167843,#167844,#167845),(#167846,#167847,#167848)),
 .UNSPECIFIED.,.F.,.F.,.F.)
B_SPLINE_SURFACE_WITH_KNOTS((2,2),(3,3),(0.,0.0528815468798318),(0.659860018385434,
0.666841081426898),.UNSPECIFIED.)
GEOMETRIC_REPRESENTATION_ITEM()
RATIONAL_B_SPLINE_SURFACE(((0.990904995179416,0.989621173673383,0.988816334712145),
(0.990904995179416,0.989621173673383,0.988816334712145)))
REPRESENTATION_ITEM('')
SURFACE()
);
#4356=(
BOUNDED_SURFACE()
B_SPLINE_SURFACE(1,2,((#167850,#167851,#167852,#167853,#167854),(#167855,
#167856,#167857,#167858,#167859)),.UNSPECIFIED.,.F.,.F.,.F.)
B_SPLINE_SURFACE_WITH_KNOTS((2,2),(3,2,3),(0.938550151647612,1.00001008240785),
(0.659832011354087,0.659901408087481,0.666841081426897),.UNSPECIFIED.)
GEOMETRIC_REPRESENTATION_ITEM()
RATIONAL_B_SPLINE_SURFACE(((0.990889788836284,0.990889788836284,0.990889788836284,
0.98961640190086,0.988816334712145),(0.990889788836284,0.990889788836284,
0.990889788836284,0.98961640190086,0.988816334712145)))
REPRESENTATION_ITEM('')
SURFACE()
);
#4357=(
BOUNDED_SURFACE()
B_SPLINE_SURFACE(1,2,((#167861,#167862,#167863,#167864,#167865),(#167866,
#167867,#167868,#167869,#167870)),.UNSPECIFIED.,.F.,.F.,.F.)
B_SPLINE_SURFACE_WITH_KNOTS((2,2),(3,2,3),(-1.06888495707795E-6,0.182885378421191),
(0.0734807488197897,0.0736543502199111,0.0910144902320524),
 .UNSPECIFIED.)
GEOMETRIC_REPRESENTATION_ITEM()
RATIONAL_B_SPLINE_SURFACE(((0.99848615229188,0.99848615229188,0.99848615229188,
0.992772345172011,0.990020524139833),(0.99848615229188,0.99848615229188,
0.99848615229188,0.992772345172011,0.990020524139833)))
REPRESENTATION_ITEM('')
SURFACE()
);
#4358=(
BOUNDED_SURFACE()
B_SPLINE_SURFACE(1,2,((#167881,#167882,#167883,#167884,#167885),(#167886,
#167887,#167888,#167889,#167890)),.UNSPECIFIED.,.F.,.F.,.F.)
B_SPLINE_SURFACE_WITH_KNOTS((2,2),(3,2,3),(0.,0.182805892339158),(0.642474614281364,
0.642857142857143,0.659901408087481),.UNSPECIFIED.)
GEOMETRIC_REPRESENTATION_ITEM()
RATIONAL_B_SPLINE_SURFACE(((0.999732896029236,0.999865728939372,1.,0.994017305594881,
0.990889788836284),(0.999732896029236,0.999865728939372,1.,0.994017305594881,
0.990889788836284)))
REPRESENTATION_ITEM('')
SURFACE()
);
#4359=(
BOUNDED_SURFACE()
B_SPLINE_SURFACE(1,2,((#167892,#167893,#167894,#167895,#167896),(#167897,
#167898,#167899,#167900,#167901)),.UNSPECIFIED.,.F.,.F.,.F.)
B_SPLINE_SURFACE_WITH_KNOTS((2,2),(3,2,3),(0.938576859128169,1.),(0.0665257254736559,
0.0714285714285714,0.0736543502199112),.UNSPECIFIED.)
GEOMETRIC_REPRESENTATION_ITEM()
RATIONAL_B_SPLINE_SURFACE(((0.996794362316491,0.998279055819231,1.,0.999218731101516,
0.99848615229188),(0.996794362316491,0.998279055819231,1.,0.999218731101516,
0.99848615229188)))
REPRESENTATION_ITEM('')
SURFACE()
);
#4360=(
BOUNDED_SURFACE()
B_SPLINE_SURFACE(1,2,((#167909,#167910,#167911,#167912,#167913),(#167914,
#167915,#167916,#167917,#167918)),.UNSPECIFIED.,.F.,.F.,.F.)
B_SPLINE_SURFACE_WITH_KNOTS((2,2),(3,2,3),(0.,0.0529045403781336),(0.0665257254736559,
0.0714285714285714,0.0736968668684972),.UNSPECIFIED.)
GEOMETRIC_REPRESENTATION_ITEM()
RATIONAL_B_SPLINE_SURFACE(((0.996794362316491,0.998279055819231,1.,0.999203807365457,
0.998458182734336),(0.996794362316491,0.998279055819231,1.,0.999203807365457,
0.998458182734336)))
REPRESENTATION_ITEM('')
SURFACE()
);
#4361=(
BOUNDED_SURFACE()
B_SPLINE_SURFACE(1,2,((#167929,#167930,#167931),(#167932,#167933,#167934)),
 .UNSPECIFIED.,.F.,.F.,.F.)
B_SPLINE_SURFACE_WITH_KNOTS((2,2),(3,3),(0.,0.0528815468798333),(0.659860018385656,
0.666841081426897),.UNSPECIFIED.)
GEOMETRIC_REPRESENTATION_ITEM()
RATIONAL_B_SPLINE_SURFACE(((0.990904995179334,0.989621173673357,0.988816334712145),
(0.990904995179334,0.989621173673357,0.988816334712145)))
REPRESENTATION_ITEM('')
SURFACE()
);
#4362=(
BOUNDED_SURFACE()
B_SPLINE_SURFACE(1,2,((#167936,#167937,#167938,#167939,#167940),(#167941,
#167942,#167943,#167944,#167945)),.UNSPECIFIED.,.F.,.F.,.F.)
B_SPLINE_SURFACE_WITH_KNOTS((2,2),(3,2,3),(0.938550151647612,1.00001008244309),
(0.659832011354087,0.659901408087481,0.666841081426897),.UNSPECIFIED.)
GEOMETRIC_REPRESENTATION_ITEM()
RATIONAL_B_SPLINE_SURFACE(((0.990889788836284,0.990889788836284,0.990889788836284,
0.98961640190086,0.988816334712146),(0.990889788836284,0.990889788836284,
0.990889788836284,0.98961640190086,0.988816334712146)))
REPRESENTATION_ITEM('')
SURFACE()
);
#4363=(
BOUNDED_SURFACE()
B_SPLINE_SURFACE(1,2,((#167947,#167948,#167949,#167950,#167951),(#167952,
#167953,#167954,#167955,#167956)),.UNSPECIFIED.,.F.,.F.,.F.)
B_SPLINE_SURFACE_WITH_KNOTS((2,2),(3,2,3),(-1.07113328560007E-6,0.182885378421191),
(0.0734807488197897,0.0736543502199111,0.0910144902320524),
 .UNSPECIFIED.)
GEOMETRIC_REPRESENTATION_ITEM()
RATIONAL_B_SPLINE_SURFACE(((0.99848615229188,0.99848615229188,0.99848615229188,
0.992772345172011,0.990020524139833),(0.99848615229188,0.99848615229188,
0.99848615229188,0.992772345172011,0.990020524139833)))
REPRESENTATION_ITEM('')
SURFACE()
);
#4364=(
BOUNDED_SURFACE()
B_SPLINE_SURFACE(1,2,((#167967,#167968,#167969,#167970,#167971),(#167972,
#167973,#167974,#167975,#167976)),.UNSPECIFIED.,.F.,.F.,.F.)
B_SPLINE_SURFACE_WITH_KNOTS((2,2),(3,2,3),(0.,0.182805892339156),(0.642474614281366,
0.642857142857143,0.659901408087481),.UNSPECIFIED.)
GEOMETRIC_REPRESENTATION_ITEM()
RATIONAL_B_SPLINE_SURFACE(((0.999732896029237,0.999865728939372,1.,0.994017305594881,
0.990889788836284),(0.999732896029237,0.999865728939372,1.,0.994017305594881,
0.990889788836284)))
REPRESENTATION_ITEM('')
SURFACE()
);
#4365=(
BOUNDED_SURFACE()
B_SPLINE_SURFACE(1,2,((#167978,#167979,#167980,#167981,#167982),(#167983,
#167984,#167985,#167986,#167987)),.UNSPECIFIED.,.F.,.F.,.F.)
B_SPLINE_SURFACE_WITH_KNOTS((2,2),(3,2,3),(0.938576859128171,1.),(0.0665257254736565,
0.0714285714285714,0.0736543502199112),.UNSPECIFIED.)
GEOMETRIC_REPRESENTATION_ITEM()
RATIONAL_B_SPLINE_SURFACE(((0.996794362316492,0.998279055819231,1.,0.999218731101516,
0.99848615229188),(0.996794362316492,0.998279055819231,1.,0.999218731101516,
0.99848615229188)))
REPRESENTATION_ITEM('')
SURFACE()
);
#4366=(
BOUNDED_SURFACE()
B_SPLINE_SURFACE(1,2,((#167995,#167996,#167997,#167998,#167999),(#168000,
#168001,#168002,#168003,#168004)),.UNSPECIFIED.,.F.,.F.,.F.)
B_SPLINE_SURFACE_WITH_KNOTS((2,2),(3,2,3),(0.,0.052904540378127),(0.0665257254736564,
0.0714285714285714,0.0736968668684973),.UNSPECIFIED.)
GEOMETRIC_REPRESENTATION_ITEM()
RATIONAL_B_SPLINE_SURFACE(((0.996794362316492,0.998279055819231,1.,0.999203807365457,
0.998458182734336),(0.996794362316492,0.998279055819231,1.,0.999203807365457,
0.998458182734336)))
REPRESENTATION_ITEM('')
SURFACE()
);
#4367=(
BOUNDED_SURFACE()
B_SPLINE_SURFACE(1,2,((#168015,#168016,#168017),(#168018,#168019,#168020)),
 .UNSPECIFIED.,.F.,.F.,.F.)
B_SPLINE_SURFACE_WITH_KNOTS((2,2),(3,3),(0.,0.0528815468798321),(0.659860018385656,
0.666841081426897),.UNSPECIFIED.)
GEOMETRIC_REPRESENTATION_ITEM()
RATIONAL_B_SPLINE_SURFACE(((0.990904995179334,0.989621173673357,0.988816334712145),
(0.990904995179334,0.989621173673357,0.988816334712145)))
REPRESENTATION_ITEM('')
SURFACE()
);
#4368=(
BOUNDED_SURFACE()
B_SPLINE_SURFACE(1,2,((#168022,#168023,#168024,#168025,#168026),(#168027,
#168028,#168029,#168030,#168031)),.UNSPECIFIED.,.F.,.F.,.F.)
B_SPLINE_SURFACE_WITH_KNOTS((2,2),(3,2,3),(0.938550151647611,1.00001008251789),
(0.659832011354087,0.659901408087481,0.666841081426897),.UNSPECIFIED.)
GEOMETRIC_REPRESENTATION_ITEM()
RATIONAL_B_SPLINE_SURFACE(((0.990889788836284,0.990889788836284,0.990889788836284,
0.98961640190086,0.988816334712145),(0.990889788836284,0.990889788836284,
0.990889788836284,0.98961640190086,0.988816334712145)))
REPRESENTATION_ITEM('')
SURFACE()
);
#4369=(
BOUNDED_SURFACE()
B_SPLINE_SURFACE(1,2,((#168033,#168034,#168035,#168036,#168037),(#168038,
#168039,#168040,#168041,#168042)),.UNSPECIFIED.,.F.,.F.,.F.)
B_SPLINE_SURFACE_WITH_KNOTS((2,2),(3,2,3),(0.,0.182885378421188),(0.0734807488197898,
0.0736543502199112,0.0910144902320524),.UNSPECIFIED.)
GEOMETRIC_REPRESENTATION_ITEM()
RATIONAL_B_SPLINE_SURFACE(((0.99848615229188,0.99848615229188,0.99848615229188,
0.992772345172011,0.990020524139833),(0.99848615229188,0.99848615229188,
0.99848615229188,0.992772345172011,0.990020524139833)))
REPRESENTATION_ITEM('')
SURFACE()
);
#4375=(
BOUNDED_CURVE()
B_SPLINE_CURVE(2,(#95475,#95476,#95477,#95478,#95479),.UNSPECIFIED.,.F.,
 .F.)
B_SPLINE_CURVE_WITH_KNOTS((3,2,3),(0.418312080773434,0.428571428571429,
0.430498434992938),.UNSPECIFIED.)
CURVE()
GEOMETRIC_REPRESENTATION_ITEM()
RATIONAL_B_SPLINE_CURVE((0.99383221411677,0.996398874234721,1.,0.999323602960832,
0.998683701721927))
REPRESENTATION_ITEM('')
);
#4376=(
BOUNDED_CURVE()
B_SPLINE_CURVE(2,(#98022,#98023,#98024,#98025,#98026),.UNSPECIFIED.,.F.,
 .F.)
B_SPLINE_CURVE_WITH_KNOTS((3,2,3),(0.349440546437696,0.359118183105575,
0.366891343982437),.UNSPECIFIED.)
CURVE()
GEOMETRIC_REPRESENTATION_ITEM()
RATIONAL_B_SPLINE_CURVE((0.994126602224873,0.996603060231146,1.,0.997271548790187,
0.995136940905933))
REPRESENTATION_ITEM('')
);
#4377=(
BOUNDED_CURVE()
B_SPLINE_CURVE(2,(#98055,#98056,#98057,#98058,#98059),.UNSPECIFIED.,.F.,
 .F.)
B_SPLINE_CURVE_WITH_KNOTS((3,2,3),(0.349440546446772,0.359118183105576,
0.366891343971801),.UNSPECIFIED.)
CURVE()
GEOMETRIC_REPRESENTATION_ITEM()
RATIONAL_B_SPLINE_CURVE((0.994126602224872,0.996603060231146,1.,0.99727154879392,
0.995136940911775))
REPRESENTATION_ITEM('')
);
#4378=(
BOUNDED_CURVE()
B_SPLINE_CURVE(2,(#98088,#98089,#98090,#98091,#98092),.UNSPECIFIED.,.F.,
 .F.)
B_SPLINE_CURVE_WITH_KNOTS((3,2,3),(0.349440546433574,0.359118183105575,
0.366891343991316),.UNSPECIFIED.)
CURVE()
GEOMETRIC_REPRESENTATION_ITEM()
RATIONAL_B_SPLINE_CURVE((0.994126602224873,0.996603060231146,1.,0.99727154878707,
0.995136940901056))
REPRESENTATION_ITEM('')
);
#4379=(
BOUNDED_CURVE()
B_SPLINE_CURVE(2,(#98121,#98122,#98123,#98124,#98125),.UNSPECIFIED.,.F.,
 .F.)
B_SPLINE_CURVE_WITH_KNOTS((3,2,3),(0.349440546441033,0.359118183105575,
0.36689134396703),.UNSPECIFIED.)
CURVE()
GEOMETRIC_REPRESENTATION_ITEM()
RATIONAL_B_SPLINE_CURVE((0.994126602224873,0.996603060231146,1.,0.997271548795594,
0.995136940914395))
REPRESENTATION_ITEM('')
);
#4380=(
BOUNDED_CURVE()
B_SPLINE_CURVE(2,(#98154,#98155,#98156,#98157,#98158),.UNSPECIFIED.,.F.,
 .F.)
B_SPLINE_CURVE_WITH_KNOTS((3,2,3),(0.349440546416899,0.359118183105575,
0.366891343982081),.UNSPECIFIED.)
CURVE()
GEOMETRIC_REPRESENTATION_ITEM()
RATIONAL_B_SPLINE_CURVE((0.994126602224873,0.996603060231146,1.,0.997271548790312,
0.995136940906129))
REPRESENTATION_ITEM('')
);
#4381=(
BOUNDED_CURVE()
B_SPLINE_CURVE(2,(#98187,#98188,#98189,#98190,#98191),.UNSPECIFIED.,.F.,
 .F.)
B_SPLINE_CURVE_WITH_KNOTS((3,2,3),(0.349440546419126,0.359118183105565,
0.366891343966471),.UNSPECIFIED.)
CURVE()
GEOMETRIC_REPRESENTATION_ITEM()
RATIONAL_B_SPLINE_CURVE((0.994126602224873,0.996603060231146,1.,0.997271548795788,
0.995136940914697))
REPRESENTATION_ITEM('')
);
#4382=(
BOUNDED_CURVE()
B_SPLINE_CURVE(2,(#98220,#98221,#98222,#98223,#98224),.UNSPECIFIED.,.F.,
 .F.)
B_SPLINE_CURVE_WITH_KNOTS((3,2,3),(0.349440546426667,0.359118183105575,
0.366891343970343),.UNSPECIFIED.)
CURVE()
GEOMETRIC_REPRESENTATION_ITEM()
RATIONAL_B_SPLINE_CURVE((0.994126602224873,0.996603060231146,1.,0.997271548794432,
0.995136940912576))
REPRESENTATION_ITEM('')
);
#4383=(
BOUNDED_CURVE()
B_SPLINE_CURVE(2,(#98288,#98289,#98290,#98291,#98292),.UNSPECIFIED.,.F.,
 .F.)
B_SPLINE_CURVE_WITH_KNOTS((3,2,3),(0.349440546445551,0.359118183105575,
0.366891343984427),.UNSPECIFIED.)
CURVE()
GEOMETRIC_REPRESENTATION_ITEM()
RATIONAL_B_SPLINE_CURVE((0.994126602224873,0.996603060231146,1.,0.997271548789488,
0.99513694090484))
REPRESENTATION_ITEM('')
);
#4384=(
BOUNDED_CURVE()
B_SPLINE_CURVE(2,(#98321,#98322,#98323,#98324,#98325),.UNSPECIFIED.,.F.,
 .F.)
B_SPLINE_CURVE_WITH_KNOTS((3,2,3),(0.349440546417489,0.359118183105584,
0.366891343969882),.UNSPECIFIED.)
CURVE()
GEOMETRIC_REPRESENTATION_ITEM()
RATIONAL_B_SPLINE_CURVE((0.994126602224868,0.996603060231143,1.,0.997271548794597,
0.995136940912833))
REPRESENTATION_ITEM('')
);
#4385=(
BOUNDED_CURVE()
B_SPLINE_CURVE(2,(#98354,#98355,#98356,#98357,#98358),.UNSPECIFIED.,.F.,
 .F.)
B_SPLINE_CURVE_WITH_KNOTS((3,2,3),(0.349440546409791,0.359118183105584,
0.366891343977855),.UNSPECIFIED.)
CURVE()
GEOMETRIC_REPRESENTATION_ITEM()
RATIONAL_B_SPLINE_CURVE((0.994126602224868,0.996603060231143,1.,0.997271548791798,
0.995136940908454))
REPRESENTATION_ITEM('')
);
#4386=(
BOUNDED_CURVE()
B_SPLINE_CURVE(2,(#98387,#98388,#98389,#98390,#98391),.UNSPECIFIED.,.F.,
 .F.)
B_SPLINE_CURVE_WITH_KNOTS((3,2,3),(0.349440546428452,0.359118183105584,
0.366891343978224),.UNSPECIFIED.)
CURVE()
GEOMETRIC_REPRESENTATION_ITEM()
RATIONAL_B_SPLINE_CURVE((0.994126602224868,0.996603060231143,1.,0.997271548791668,
0.995136940908252))
REPRESENTATION_ITEM('')
);
#4387=(
BOUNDED_CURVE()
B_SPLINE_CURVE(2,(#98490,#98491,#98492,#98493,#98494),.UNSPECIFIED.,.F.,
 .F.)
B_SPLINE_CURVE_WITH_KNOTS((3,2,3),(0.349440546425061,0.359118183105584,
0.366891343989552),.UNSPECIFIED.)
CURVE()
GEOMETRIC_REPRESENTATION_ITEM()
RATIONAL_B_SPLINE_CURVE((0.994126602224868,0.996603060231143,1.,0.997271548787692,
0.99513694090203))
REPRESENTATION_ITEM('')
);
#4388=(
BOUNDED_CURVE()
B_SPLINE_CURVE(2,(#98523,#98524,#98525,#98526,#98527),.UNSPECIFIED.,.F.,
 .F.)
B_SPLINE_CURVE_WITH_KNOTS((3,2,3),(0.349440546442563,0.359118183105584,
0.366891343973804),.UNSPECIFIED.)
CURVE()
GEOMETRIC_REPRESENTATION_ITEM()
RATIONAL_B_SPLINE_CURVE((0.994126602224868,0.996603060231143,1.,0.99727154879322,
0.995136940910679))
REPRESENTATION_ITEM('')
);
#4389=(
BOUNDED_CURVE()
B_SPLINE_CURVE(2,(#98591,#98592,#98593,#98594,#98595),.UNSPECIFIED.,.F.,
 .F.)
B_SPLINE_CURVE_WITH_KNOTS((3,2,3),(0.349440546416269,0.359118183105584,
0.366891343964705),.UNSPECIFIED.)
CURVE()
GEOMETRIC_REPRESENTATION_ITEM()
RATIONAL_B_SPLINE_CURVE((0.994126602224868,0.996603060231143,1.,0.997271548796414,
0.995136940915677))
REPRESENTATION_ITEM('')
);
#4390=(
BOUNDED_CURVE()
B_SPLINE_CURVE(2,(#98624,#98625,#98626,#98627,#98628),.UNSPECIFIED.,.F.,
 .F.)
B_SPLINE_CURVE_WITH_KNOTS((3,2,3),(0.349440546439546,0.359118183105584,
0.366891343987011),.UNSPECIFIED.)
CURVE()
GEOMETRIC_REPRESENTATION_ITEM()
RATIONAL_B_SPLINE_CURVE((0.994126602224868,0.996603060231143,1.,0.997271548788584,
0.995136940903426))
REPRESENTATION_ITEM('')
);
#4391=(
BOUNDED_CURVE()
B_SPLINE_CURVE(2,(#98657,#98658,#98659,#98660,#98661),.UNSPECIFIED.,.F.,
 .F.)
B_SPLINE_CURVE_WITH_KNOTS((3,2,3),(0.349440546419593,0.359118183105584,
0.366891343980483),.UNSPECIFIED.)
CURVE()
GEOMETRIC_REPRESENTATION_ITEM()
RATIONAL_B_SPLINE_CURVE((0.994126602224868,0.996603060231143,1.,0.997271548790876,
0.995136940907011))
REPRESENTATION_ITEM('')
);
#4392=(
BOUNDED_CURVE()
B_SPLINE_CURVE(2,(#98690,#98691,#98692,#98693,#98694),.UNSPECIFIED.,.F.,
 .F.)
B_SPLINE_CURVE_WITH_KNOTS((3,2,3),(0.349440546448491,0.359118183105584,
0.366891343972737),.UNSPECIFIED.)
CURVE()
GEOMETRIC_REPRESENTATION_ITEM()
RATIONAL_B_SPLINE_CURVE((0.994126602224868,0.996603060231143,1.,0.997271548793594,
0.995136940911266))
REPRESENTATION_ITEM('')
);
#4393=(
BOUNDED_CURVE()
B_SPLINE_CURVE(2,(#98723,#98724,#98725,#98726,#98727),.UNSPECIFIED.,.F.,
 .F.)
B_SPLINE_CURVE_WITH_KNOTS((3,2,3),(0.349440546424786,0.359118183105584,
0.366891343966157),.UNSPECIFIED.)
CURVE()
GEOMETRIC_REPRESENTATION_ITEM()
RATIONAL_B_SPLINE_CURVE((0.994126602224868,0.996603060231143,1.,0.997271548795904,
0.995136940914879))
REPRESENTATION_ITEM('')
);
#4394=(
BOUNDED_CURVE()
B_SPLINE_CURVE(2,(#98861,#98862,#98863,#98864,#98865),.UNSPECIFIED.,.F.,
 .F.)
B_SPLINE_CURVE_WITH_KNOTS((3,2,3),(0.349440546437349,0.359118183105576,
0.366891343969567),.UNSPECIFIED.)
CURVE()
GEOMETRIC_REPRESENTATION_ITEM()
RATIONAL_B_SPLINE_CURVE((0.994126602224873,0.996603060231146,1.,0.997271548794705,
0.995136940913002))
REPRESENTATION_ITEM('')
);
#4395=(
BOUNDED_CURVE()
B_SPLINE_CURVE(2,(#98894,#98895,#98896,#98897,#98898),.UNSPECIFIED.,.F.,
 .F.)
B_SPLINE_CURVE_WITH_KNOTS((3,2,3),(0.349440546418518,0.359118183105575,
0.366891343970643),.UNSPECIFIED.)
CURVE()
GEOMETRIC_REPRESENTATION_ITEM()
RATIONAL_B_SPLINE_CURVE((0.994126602224873,0.996603060231146,1.,0.997271548794326,
0.99513694091241))
REPRESENTATION_ITEM('')
);
#4396=(
BOUNDED_CURVE()
B_SPLINE_CURVE(2,(#98927,#98928,#98929,#98930,#98931),.UNSPECIFIED.,.F.,
 .F.)
B_SPLINE_CURVE_WITH_KNOTS((3,2,3),(0.349440546437857,0.359118183105575,
0.366891343981114),.UNSPECIFIED.)
CURVE()
GEOMETRIC_REPRESENTATION_ITEM()
RATIONAL_B_SPLINE_CURVE((0.994126602224873,0.996603060231146,1.,0.997271548790651,
0.99513694090666))
REPRESENTATION_ITEM('')
);
#4397=(
BOUNDED_CURVE()
B_SPLINE_CURVE(2,(#101127,#101128,#101129,#101130,#101131),
 .UNSPECIFIED.,.F.,.F.)
B_SPLINE_CURVE_WITH_KNOTS((3,2,3),(0.418312080773434,0.428571428571429,
0.430498434990588),.UNSPECIFIED.)
CURVE()
GEOMETRIC_REPRESENTATION_ITEM()
RATIONAL_B_SPLINE_CURVE((0.99383221411677,0.99639887423472,1.,0.999323602961657,
0.998683701723488))
REPRESENTATION_ITEM('')
);
#4398=(
BOUNDED_CURVE()
B_SPLINE_CURVE(2,(#101168,#101169,#101170,#101171,#101172),
 .UNSPECIFIED.,.F.,.F.)
B_SPLINE_CURVE_WITH_KNOTS((3,2,3),(0.418312080773433,0.428571428571429,
0.430498434989605),.UNSPECIFIED.)
CURVE()
GEOMETRIC_REPRESENTATION_ITEM()
RATIONAL_B_SPLINE_CURVE((0.993832214116769,0.99639887423472,1.,0.999323602962002,
0.99868370172414))
REPRESENTATION_ITEM('')
);
#4399=(
BOUNDED_CURVE()
B_SPLINE_CURVE(2,(#101209,#101210,#101211,#101212,#101213),
 .UNSPECIFIED.,.F.,.F.)
B_SPLINE_CURVE_WITH_KNOTS((3,2,3),(0.418312080773433,0.428571428571429,
0.430498434990323),.UNSPECIFIED.)
CURVE()
GEOMETRIC_REPRESENTATION_ITEM()
RATIONAL_B_SPLINE_CURVE((0.993832214116769,0.99639887423472,1.,0.99932360296175,
0.998683701723664))
REPRESENTATION_ITEM('')
);
#4400=(
BOUNDED_CURVE()
B_SPLINE_CURVE(2,(#101250,#101251,#101252,#101253,#101254),
 .UNSPECIFIED.,.F.,.F.)
B_SPLINE_CURVE_WITH_KNOTS((3,2,3),(0.418312080773433,0.428571428571429,
0.430498434985288),.UNSPECIFIED.)
CURVE()
GEOMETRIC_REPRESENTATION_ITEM()
RATIONAL_B_SPLINE_CURVE((0.993832214116769,0.99639887423472,1.,0.999323602963517,
0.998683701727008))
REPRESENTATION_ITEM('')
);
#4401=(
BOUNDED_CURVE()
B_SPLINE_CURVE(2,(#101291,#101292,#101293,#101294,#101295),
 .UNSPECIFIED.,.F.,.F.)
B_SPLINE_CURVE_WITH_KNOTS((3,2,3),(0.418312080773434,0.428571428571429,
0.430498434986539),.UNSPECIFIED.)
CURVE()
GEOMETRIC_REPRESENTATION_ITEM()
RATIONAL_B_SPLINE_CURVE((0.99383221411677,0.99639887423472,1.,0.999323602963078,
0.998683701726177))
REPRESENTATION_ITEM('')
);
#4402=(
BOUNDED_CURVE()
B_SPLINE_CURVE(2,(#101332,#101333,#101334,#101335,#101336),
 .UNSPECIFIED.,.F.,.F.)
B_SPLINE_CURVE_WITH_KNOTS((3,2,3),(0.418312080773434,0.428571428571429,
0.430498434990513),.UNSPECIFIED.)
CURVE()
GEOMETRIC_REPRESENTATION_ITEM()
RATIONAL_B_SPLINE_CURVE((0.99383221411677,0.996398874234721,1.,0.999323602961683,
0.998683701723538))
REPRESENTATION_ITEM('')
);
#4403=(
BOUNDED_CURVE()
B_SPLINE_CURVE(2,(#101373,#101374,#101375,#101376,#101377),
 .UNSPECIFIED.,.F.,.F.)
B_SPLINE_CURVE_WITH_KNOTS((3,2,3),(0.418312080773434,0.428571428571429,
0.430498434985252),.UNSPECIFIED.)
CURVE()
GEOMETRIC_REPRESENTATION_ITEM()
RATIONAL_B_SPLINE_CURVE((0.99383221411677,0.99639887423472,1.,0.99932360296353,
0.998683701727032))
REPRESENTATION_ITEM('')
);
#4404=(
BOUNDED_CURVE()
B_SPLINE_CURVE(2,(#101414,#101415,#101416,#101417,#101418),
 .UNSPECIFIED.,.F.,.F.)
B_SPLINE_CURVE_WITH_KNOTS((3,2,3),(0.418312080773434,0.428571428571429,
0.430498434984252),.UNSPECIFIED.)
CURVE()
GEOMETRIC_REPRESENTATION_ITEM()
RATIONAL_B_SPLINE_CURVE((0.99383221411677,0.996398874234721,1.,0.999323602963881,
0.998683701727696))
REPRESENTATION_ITEM('')
);
#4405=(
BOUNDED_CURVE()
B_SPLINE_CURVE(2,(#101455,#101456,#101457,#101458,#101459),
 .UNSPECIFIED.,.F.,.F.)
B_SPLINE_CURVE_WITH_KNOTS((3,2,3),(0.418312080773434,0.428571428571429,
0.430498434987172),.UNSPECIFIED.)
CURVE()
GEOMETRIC_REPRESENTATION_ITEM()
RATIONAL_B_SPLINE_CURVE((0.99383221411677,0.996398874234721,1.,0.999323602962856,
0.998683701725757))
REPRESENTATION_ITEM('')
);
#4406=(
BOUNDED_CURVE()
B_SPLINE_CURVE(2,(#101496,#101497,#101498,#101499,#101500),
 .UNSPECIFIED.,.F.,.F.)
B_SPLINE_CURVE_WITH_KNOTS((3,2,3),(0.418312080773434,0.428571428571429,
0.43049843498926),.UNSPECIFIED.)
CURVE()
GEOMETRIC_REPRESENTATION_ITEM()
RATIONAL_B_SPLINE_CURVE((0.99383221411677,0.996398874234721,1.,0.999323602962123,
0.99868370172437))
REPRESENTATION_ITEM('')
);
#4407=(
BOUNDED_CURVE()
B_SPLINE_CURVE(2,(#101537,#101538,#101539,#101540,#101541),
 .UNSPECIFIED.,.F.,.F.)
B_SPLINE_CURVE_WITH_KNOTS((3,2,3),(0.418312080773434,0.428571428571429,
0.43049843498763),.UNSPECIFIED.)
CURVE()
GEOMETRIC_REPRESENTATION_ITEM()
RATIONAL_B_SPLINE_CURVE((0.99383221411677,0.99639887423472,1.,0.999323602962695,
0.998683701725452))
REPRESENTATION_ITEM('')
);
#4408=(
BOUNDED_CURVE()
B_SPLINE_CURVE(2,(#101578,#101579,#101580,#101581,#101582),
 .UNSPECIFIED.,.F.,.F.)
B_SPLINE_CURVE_WITH_KNOTS((3,2,3),(0.418312080773434,0.428571428571429,
0.430498434990192),.UNSPECIFIED.)
CURVE()
GEOMETRIC_REPRESENTATION_ITEM()
RATIONAL_B_SPLINE_CURVE((0.99383221411677,0.996398874234721,1.,0.999323602961796,
0.998683701723751))
REPRESENTATION_ITEM('')
);
#4409=(
BOUNDED_CURVE()
B_SPLINE_CURVE(2,(#101619,#101620,#101621,#101622,#101623),
 .UNSPECIFIED.,.F.,.F.)
B_SPLINE_CURVE_WITH_KNOTS((3,2,3),(0.418312080773434,0.428571428571429,
0.430498434989795),.UNSPECIFIED.)
CURVE()
GEOMETRIC_REPRESENTATION_ITEM()
RATIONAL_B_SPLINE_CURVE((0.99383221411677,0.996398874234721,1.,0.999323602961935,
0.998683701724015))
REPRESENTATION_ITEM('')
);
#4410=(
BOUNDED_CURVE()
B_SPLINE_CURVE(2,(#101660,#101661,#101662,#101663,#101664),
 .UNSPECIFIED.,.F.,.F.)
B_SPLINE_CURVE_WITH_KNOTS((3,2,3),(0.418312080773434,0.428571428571429,
0.430498434986927),.UNSPECIFIED.)
CURVE()
GEOMETRIC_REPRESENTATION_ITEM()
RATIONAL_B_SPLINE_CURVE((0.99383221411677,0.99639887423472,1.,0.999323602962942,
0.998683701725919))
REPRESENTATION_ITEM('')
);
#4411=(
BOUNDED_CURVE()
B_SPLINE_CURVE(2,(#101701,#101702,#101703,#101704,#101705),
 .UNSPECIFIED.,.F.,.F.)
B_SPLINE_CURVE_WITH_KNOTS((3,2,3),(0.418312080773433,0.428571428571429,
0.430498434988302),.UNSPECIFIED.)
CURVE()
GEOMETRIC_REPRESENTATION_ITEM()
RATIONAL_B_SPLINE_CURVE((0.99383221411677,0.99639887423472,1.,0.999323602962459,
0.998683701725006))
REPRESENTATION_ITEM('')
);
#4412=(
BOUNDED_CURVE()
B_SPLINE_CURVE(2,(#101742,#101743,#101744,#101745,#101746),
 .UNSPECIFIED.,.F.,.F.)
B_SPLINE_CURVE_WITH_KNOTS((3,2,3),(0.418312080773434,0.428571428571429,
0.430498434993456),.UNSPECIFIED.)
CURVE()
GEOMETRIC_REPRESENTATION_ITEM()
RATIONAL_B_SPLINE_CURVE((0.99383221411677,0.996398874234721,1.,0.99932360296065,
0.998683701721583))
REPRESENTATION_ITEM('')
);
#4413=(
BOUNDED_CURVE()
B_SPLINE_CURVE(2,(#101783,#101784,#101785,#101786,#101787),
 .UNSPECIFIED.,.F.,.F.)
B_SPLINE_CURVE_WITH_KNOTS((3,2,3),(0.418312080773434,0.428571428571429,
0.430498434990347),.UNSPECIFIED.)
CURVE()
GEOMETRIC_REPRESENTATION_ITEM()
RATIONAL_B_SPLINE_CURVE((0.99383221411677,0.996398874234721,1.,0.999323602961742,
0.998683701723649))
REPRESENTATION_ITEM('')
);
#4414=(
BOUNDED_CURVE()
B_SPLINE_CURVE(2,(#101824,#101825,#101826,#101827,#101828),
 .UNSPECIFIED.,.F.,.F.)
B_SPLINE_CURVE_WITH_KNOTS((3,2,3),(0.418312080773434,0.428571428571429,
0.430498434990058),.UNSPECIFIED.)
CURVE()
GEOMETRIC_REPRESENTATION_ITEM()
RATIONAL_B_SPLINE_CURVE((0.99383221411677,0.996398874234721,1.,0.999323602961843,
0.99868370172384))
REPRESENTATION_ITEM('')
);
#4415=(
BOUNDED_CURVE()
B_SPLINE_CURVE(2,(#101865,#101866,#101867,#101868,#101869),
 .UNSPECIFIED.,.F.,.F.)
B_SPLINE_CURVE_WITH_KNOTS((3,2,3),(0.418312080773434,0.428571428571429,
0.43049843498816),.UNSPECIFIED.)
CURVE()
GEOMETRIC_REPRESENTATION_ITEM()
RATIONAL_B_SPLINE_CURVE((0.99383221411677,0.996398874234721,1.,0.999323602962509,
0.998683701725101))
REPRESENTATION_ITEM('')
);
#4416=(
BOUNDED_CURVE()
B_SPLINE_CURVE(2,(#101906,#101907,#101908,#101909,#101910),
 .UNSPECIFIED.,.F.,.F.)
B_SPLINE_CURVE_WITH_KNOTS((3,2,3),(0.418312080773434,0.428571428571429,
0.430498434988028),.UNSPECIFIED.)
CURVE()
GEOMETRIC_REPRESENTATION_ITEM()
RATIONAL_B_SPLINE_CURVE((0.99383221411677,0.996398874234721,1.,0.999323602962556,
0.998683701725188))
REPRESENTATION_ITEM('')
);
#4417=(
BOUNDED_CURVE()
B_SPLINE_CURVE(2,(#101947,#101948,#101949,#101950,#101951),
 .UNSPECIFIED.,.F.,.F.)
B_SPLINE_CURVE_WITH_KNOTS((3,2,3),(0.418312080773434,0.428571428571429,
0.430498434991989),.UNSPECIFIED.)
CURVE()
GEOMETRIC_REPRESENTATION_ITEM()
RATIONAL_B_SPLINE_CURVE((0.99383221411677,0.996398874234721,1.,0.999323602961165,
0.998683701722558))
REPRESENTATION_ITEM('')
);
#4418=(
BOUNDED_CURVE()
B_SPLINE_CURVE(2,(#102016,#102017,#102018,#102019,#102020),
 .UNSPECIFIED.,.F.,.F.)
B_SPLINE_CURVE_WITH_KNOTS((3,2,3),(0.418312080773434,0.428571428571429,
0.430498434989518),.UNSPECIFIED.)
CURVE()
GEOMETRIC_REPRESENTATION_ITEM()
RATIONAL_B_SPLINE_CURVE((0.99383221411677,0.99639887423472,1.,0.999323602962032,
0.998683701724199))
REPRESENTATION_ITEM('')
);
#4419=(
BOUNDED_CURVE()
B_SPLINE_CURVE(2,(#102057,#102058,#102059,#102060,#102061),
 .UNSPECIFIED.,.F.,.F.)
B_SPLINE_CURVE_WITH_KNOTS((3,2,3),(0.418312080773434,0.428571428571429,
0.430498434994573),.UNSPECIFIED.)
CURVE()
GEOMETRIC_REPRESENTATION_ITEM()
RATIONAL_B_SPLINE_CURVE((0.99383221411677,0.996398874234721,1.,0.999323602960258,
0.998683701720842))
REPRESENTATION_ITEM('')
);
#4420=(
BOUNDED_CURVE()
B_SPLINE_CURVE(2,(#102098,#102099,#102100,#102101,#102102),
 .UNSPECIFIED.,.F.,.F.)
B_SPLINE_CURVE_WITH_KNOTS((3,2,3),(0.418312080773434,0.428571428571429,
0.430498434990144),.UNSPECIFIED.)
CURVE()
GEOMETRIC_REPRESENTATION_ITEM()
RATIONAL_B_SPLINE_CURVE((0.99383221411677,0.996398874234721,1.,0.999323602961813,
0.998683701723783))
REPRESENTATION_ITEM('')
);
#4421=(
BOUNDED_CURVE()
B_SPLINE_CURVE(2,(#102139,#102140,#102141,#102142,#102143),
 .UNSPECIFIED.,.F.,.F.)
B_SPLINE_CURVE_WITH_KNOTS((3,2,3),(0.418312080773434,0.428571428571429,
0.430498434989385),.UNSPECIFIED.)
CURVE()
GEOMETRIC_REPRESENTATION_ITEM()
RATIONAL_B_SPLINE_CURVE((0.99383221411677,0.99639887423472,1.,0.999323602962079,
0.998683701724287))
REPRESENTATION_ITEM('')
);
#4422=(
BOUNDED_CURVE()
B_SPLINE_CURVE(2,(#102180,#102181,#102182,#102183,#102184),
 .UNSPECIFIED.,.F.,.F.)
B_SPLINE_CURVE_WITH_KNOTS((3,2,3),(0.418312080773434,0.428571428571429,
0.430498434988894),.UNSPECIFIED.)
CURVE()
GEOMETRIC_REPRESENTATION_ITEM()
RATIONAL_B_SPLINE_CURVE((0.99383221411677,0.996398874234721,1.,0.999323602962252,
0.998683701724613))
REPRESENTATION_ITEM('')
);
#4423=(
BOUNDED_CURVE()
B_SPLINE_CURVE(2,(#102221,#102222,#102223,#102224,#102225),
 .UNSPECIFIED.,.F.,.F.)
B_SPLINE_CURVE_WITH_KNOTS((3,2,3),(0.418312080773434,0.428571428571429,
0.430498434988829),.UNSPECIFIED.)
CURVE()
GEOMETRIC_REPRESENTATION_ITEM()
RATIONAL_B_SPLINE_CURVE((0.99383221411677,0.99639887423472,1.,0.999323602962274,
0.998683701724656))
REPRESENTATION_ITEM('')
);
#4424=(
BOUNDED_CURVE()
B_SPLINE_CURVE(2,(#102262,#102263,#102264,#102265,#102266),
 .UNSPECIFIED.,.F.,.F.)
B_SPLINE_CURVE_WITH_KNOTS((3,2,3),(0.418312080773434,0.428571428571429,
0.430498434986823),.UNSPECIFIED.)
CURVE()
GEOMETRIC_REPRESENTATION_ITEM()
RATIONAL_B_SPLINE_CURVE((0.99383221411677,0.99639887423472,1.,0.999323602962978,
0.998683701725988))
REPRESENTATION_ITEM('')
);
#4425=(
BOUNDED_CURVE()
B_SPLINE_CURVE(2,(#108607,#108608,#108609,#108610,#108611),
 .UNSPECIFIED.,.F.,.F.)
B_SPLINE_CURVE_WITH_KNOTS((3,2,3),(0.280433083113984,0.285714285714286,
0.297856505249078),.UNSPECIFIED.)
CURVE()
GEOMETRIC_REPRESENTATION_ITEM()
RATIONAL_B_SPLINE_CURVE((0.996566619267863,0.998146249162903,1.,0.995737968877225,
0.992924952246043))
REPRESENTATION_ITEM('')
);
#4426=(
BOUNDED_CURVE()
B_SPLINE_CURVE(2,(#123888,#123889,#123890,#123891,#123892),
 .UNSPECIFIED.,.F.,.F.)
B_SPLINE_CURVE_WITH_KNOTS((3,2,3),(0.211502584834065,0.214285714285714,
0.228883374865518),.UNSPECIFIED.)
CURVE()
GEOMETRIC_REPRESENTATION_ITEM()
RATIONAL_B_SPLINE_CURVE((0.998122319569323,0.999023095875705,1.,0.994876086408045,
0.991846493056848))
REPRESENTATION_ITEM('')
);
#4427=(
BOUNDED_CURVE()
B_SPLINE_CURVE(2,(#123929,#123930,#123931,#123932,#123933),
 .UNSPECIFIED.,.F.,.F.)
B_SPLINE_CURVE_WITH_KNOTS((3,2,3),(0.211502584834065,0.214285714285714,
0.228883374853505),.UNSPECIFIED.)
CURVE()
GEOMETRIC_REPRESENTATION_ITEM()
RATIONAL_B_SPLINE_CURVE((0.998122319569323,0.999023095875705,1.,0.994876086412262,
0.991846493061834))
REPRESENTATION_ITEM('')
);
#4428=(
BOUNDED_CURVE()
B_SPLINE_CURVE(2,(#124062,#124063,#124064,#124065,#124066),
 .UNSPECIFIED.,.F.,.F.)
B_SPLINE_CURVE_WITH_KNOTS((3,2,3),(0.211502584834065,0.214285714285714,
0.228883374851655),.UNSPECIFIED.)
CURVE()
GEOMETRIC_REPRESENTATION_ITEM()
RATIONAL_B_SPLINE_CURVE((0.998122319569323,0.999023095875705,1.,0.994876086412911,
0.991846493062601))
REPRESENTATION_ITEM('')
);
#4429=(
BOUNDED_CURVE()
B_SPLINE_CURVE(2,(#124103,#124104,#124105,#124106,#124107),
 .UNSPECIFIED.,.F.,.F.)
B_SPLINE_CURVE_WITH_KNOTS((3,2,3),(0.211502584834065,0.214285714285714,
0.228883374862862),.UNSPECIFIED.)
CURVE()
GEOMETRIC_REPRESENTATION_ITEM()
RATIONAL_B_SPLINE_CURVE((0.998122319569323,0.999023095875705,1.,0.994876086408978,
0.99184649305795))
REPRESENTATION_ITEM('')
);
#4430=(
BOUNDED_CURVE()
B_SPLINE_CURVE(2,(#124144,#124145,#124146,#124147,#124148),
 .UNSPECIFIED.,.F.,.F.)
B_SPLINE_CURVE_WITH_KNOTS((3,2,3),(0.211502584834064,0.214285714285714,
0.228883374863024),.UNSPECIFIED.)
CURVE()
GEOMETRIC_REPRESENTATION_ITEM()
RATIONAL_B_SPLINE_CURVE((0.998122319569322,0.999023095875704,1.,0.994876086408921,
0.991846493057883))
REPRESENTATION_ITEM('')
);
#4431=(
BOUNDED_CURVE()
B_SPLINE_CURVE(2,(#124185,#124186,#124187,#124188,#124189),
 .UNSPECIFIED.,.F.,.F.)
B_SPLINE_CURVE_WITH_KNOTS((3,2,3),(0.211502584834064,0.214285714285714,
0.228883374860444),.UNSPECIFIED.)
CURVE()
GEOMETRIC_REPRESENTATION_ITEM()
RATIONAL_B_SPLINE_CURVE((0.998122319569322,0.999023095875704,1.,0.994876086409827,
0.991846493058953))
REPRESENTATION_ITEM('')
);
#4432=(
BOUNDED_CURVE()
B_SPLINE_CURVE(2,(#124272,#124273,#124274,#124275,#124276),
 .UNSPECIFIED.,.F.,.F.)
B_SPLINE_CURVE_WITH_KNOTS((3,2,3),(0.211502584834064,0.214285714285714,
0.228883374854438),.UNSPECIFIED.)
CURVE()
GEOMETRIC_REPRESENTATION_ITEM()
RATIONAL_B_SPLINE_CURVE((0.998122319569322,0.999023095875704,1.,0.994876086411935,
0.991846493061446))
REPRESENTATION_ITEM('')
);
#4433=(
BOUNDED_CURVE()
B_SPLINE_CURVE(2,(#124313,#124314,#124315,#124316,#124317),
 .UNSPECIFIED.,.F.,.F.)
B_SPLINE_CURVE_WITH_KNOTS((3,2,3),(0.211502584834064,0.214285714285714,
0.228883374860568),.UNSPECIFIED.)
CURVE()
GEOMETRIC_REPRESENTATION_ITEM()
RATIONAL_B_SPLINE_CURVE((0.998122319569322,0.999023095875704,1.,0.994876086409783,
0.991846493058902))
REPRESENTATION_ITEM('')
);
#4434=(
BOUNDED_CURVE()
B_SPLINE_CURVE(2,(#124354,#124355,#124356,#124357,#124358),
 .UNSPECIFIED.,.F.,.F.)
B_SPLINE_CURVE_WITH_KNOTS((3,2,3),(0.211502584834064,0.214285714285714,
0.228883374858422),.UNSPECIFIED.)
CURVE()
GEOMETRIC_REPRESENTATION_ITEM()
RATIONAL_B_SPLINE_CURVE((0.998122319569322,0.999023095875704,1.,0.994876086410537,
0.991846493059793))
REPRESENTATION_ITEM('')
);
#4435=(
BOUNDED_CURVE()
B_SPLINE_CURVE(2,(#124545,#124546,#124547,#124548,#124549),
 .UNSPECIFIED.,.F.,.F.)
B_SPLINE_CURVE_WITH_KNOTS((3,2,3),(0.211502584834062,0.214285714285714,
0.228883374860236),.UNSPECIFIED.)
CURVE()
GEOMETRIC_REPRESENTATION_ITEM()
RATIONAL_B_SPLINE_CURVE((0.998122319569321,0.999023095875703,1.,0.9948760864099,
0.99184649305904))
REPRESENTATION_ITEM('')
);
#4436=(
BOUNDED_CURVE()
B_SPLINE_CURVE(2,(#124586,#124587,#124588,#124589,#124590),
 .UNSPECIFIED.,.F.,.F.)
B_SPLINE_CURVE_WITH_KNOTS((3,2,3),(0.211502584834064,0.214285714285714,
0.228883374861132),.UNSPECIFIED.)
CURVE()
GEOMETRIC_REPRESENTATION_ITEM()
RATIONAL_B_SPLINE_CURVE((0.998122319569322,0.999023095875704,1.,0.994876086409585,
0.991846493058668))
REPRESENTATION_ITEM('')
);
#4437=(
BOUNDED_CURVE()
B_SPLINE_CURVE(2,(#124673,#124674,#124675,#124676,#124677),
 .UNSPECIFIED.,.F.,.F.)
B_SPLINE_CURVE_WITH_KNOTS((3,2,3),(0.211502584834063,0.214285714285714,
0.228883374855239),.UNSPECIFIED.)
CURVE()
GEOMETRIC_REPRESENTATION_ITEM()
RATIONAL_B_SPLINE_CURVE((0.998122319569321,0.999023095875704,1.,0.994876086411653,
0.991846493061113))
REPRESENTATION_ITEM('')
);
#4438=(
BOUNDED_CURVE()
B_SPLINE_CURVE(2,(#124714,#124715,#124716,#124717,#124718),
 .UNSPECIFIED.,.F.,.F.)
B_SPLINE_CURVE_WITH_KNOTS((3,2,3),(0.21150258483406,0.214285714285714,0.228883374855733),
 .UNSPECIFIED.)
CURVE()
GEOMETRIC_REPRESENTATION_ITEM()
RATIONAL_B_SPLINE_CURVE((0.998122319569319,0.999023095875703,1.,0.99487608641148,
0.991846493060909))
REPRESENTATION_ITEM('')
);
#4439=(
BOUNDED_CURVE()
B_SPLINE_CURVE(2,(#124851,#124852,#124853,#124854,#124855),
 .UNSPECIFIED.,.F.,.F.)
B_SPLINE_CURVE_WITH_KNOTS((3,2,3),(0.211502584834064,0.214285714285714,
0.22888337485822),.UNSPECIFIED.)
CURVE()
GEOMETRIC_REPRESENTATION_ITEM()
RATIONAL_B_SPLINE_CURVE((0.998122319569322,0.999023095875704,1.,0.994876086410607,
0.991846493059876))
REPRESENTATION_ITEM('')
);
#4440=(
BOUNDED_CURVE()
B_SPLINE_CURVE(2,(#124892,#124893,#124894,#124895,#124896),
 .UNSPECIFIED.,.F.,.F.)
B_SPLINE_CURVE_WITH_KNOTS((3,2,3),(0.211502584834064,0.214285714285714,
0.22888337485685),.UNSPECIFIED.)
CURVE()
GEOMETRIC_REPRESENTATION_ITEM()
RATIONAL_B_SPLINE_CURVE((0.998122319569322,0.999023095875704,1.,0.994876086411088,
0.991846493060445))
REPRESENTATION_ITEM('')
);
#4441=(
BOUNDED_CURVE()
B_SPLINE_CURVE(2,(#124933,#124934,#124935,#124936,#124937),
 .UNSPECIFIED.,.F.,.F.)
B_SPLINE_CURVE_WITH_KNOTS((3,2,3),(0.211502584834064,0.214285714285714,
0.22888337486731),.UNSPECIFIED.)
CURVE()
GEOMETRIC_REPRESENTATION_ITEM()
RATIONAL_B_SPLINE_CURVE((0.998122319569322,0.999023095875704,1.,0.994876086407416,
0.991846493056104))
REPRESENTATION_ITEM('')
);
#4442=(
BOUNDED_CURVE()
B_SPLINE_CURVE(2,(#132970,#132971,#132972,#132973,#132974),
 .UNSPECIFIED.,.F.,.F.)
B_SPLINE_CURVE_WITH_KNOTS((3,2,3),(0.492524364190421,0.5,0.504719756176228),
 .UNSPECIFIED.)
CURVE()
GEOMETRIC_REPRESENTATION_ITEM()
RATIONAL_B_SPLINE_CURVE((0.995301219176778,0.997375982834797,1.,0.998343322021369,
0.996905579294145))
REPRESENTATION_ITEM('')
);
#4443=(
BOUNDED_CURVE()
B_SPLINE_CURVE(2,(#136465,#136466,#136467,#136468,#136469),
 .UNSPECIFIED.,.F.,.F.)
B_SPLINE_CURVE_WITH_KNOTS((3,2,3),(0.556212823134607,0.571428571428571,
0.573654350147172),.UNSPECIFIED.)
CURVE()
GEOMETRIC_REPRESENTATION_ITEM()
RATIONAL_B_SPLINE_CURVE((0.991593692355873,0.994659131915763,1.,0.999218731127048,
0.998486152339761))
REPRESENTATION_ITEM('')
);
#4444=(
BOUNDED_CURVE()
B_SPLINE_CURVE(2,(#136506,#136507,#136508,#136509,#136510),
 .UNSPECIFIED.,.F.,.F.)
B_SPLINE_CURVE_WITH_KNOTS((3,2,3),(0.556212830495791,0.571428571428571,
0.573654350219911),.UNSPECIFIED.)
CURVE()
GEOMETRIC_REPRESENTATION_ITEM()
RATIONAL_B_SPLINE_CURVE((0.991593695321915,0.994659134499606,1.,0.999218731101516,
0.99848615229188))
REPRESENTATION_ITEM('')
);
#4445=(
BOUNDED_CURVE()
B_SPLINE_CURVE(2,(#136692,#136693,#136694,#136695,#136696),
 .UNSPECIFIED.,.F.,.F.)
B_SPLINE_CURVE_WITH_KNOTS((3,2,3),(0.55621283049301,0.571428571428571,0.573654350219911),
 .UNSPECIFIED.)
CURVE()
GEOMETRIC_REPRESENTATION_ITEM()
RATIONAL_B_SPLINE_CURVE((0.991593695320794,0.99465913449863,1.,0.999218731101516,
0.99848615229188))
REPRESENTATION_ITEM('')
);
#4446=(
BOUNDED_CURVE()
B_SPLINE_CURVE(2,(#136783,#136784,#136785,#136786,#136787),
 .UNSPECIFIED.,.F.,.F.)
B_SPLINE_CURVE_WITH_KNOTS((3,2,3),(0.556212830496133,0.571428571428571,
0.573654350219911),.UNSPECIFIED.)
CURVE()
GEOMETRIC_REPRESENTATION_ITEM()
RATIONAL_B_SPLINE_CURVE((0.991593695322053,0.994659134499726,1.,0.999218731101516,
0.99848615229188))
REPRESENTATION_ITEM('')
);
#4447=(
BOUNDED_CURVE()
B_SPLINE_CURVE(2,(#137072,#137073,#137074,#137075,#137076),
 .UNSPECIFIED.,.F.,.F.)
B_SPLINE_CURVE_WITH_KNOTS((3,2,3),(0.556212830497704,0.571428571428571,
0.573654350219911),.UNSPECIFIED.)
CURVE()
GEOMETRIC_REPRESENTATION_ITEM()
RATIONAL_B_SPLINE_CURVE((0.991593695322685,0.994659134500278,1.,0.999218731101516,
0.99848615229188))
REPRESENTATION_ITEM('')
);
#4448=(
BOUNDED_CURVE()
B_SPLINE_CURVE(2,(#137113,#137114,#137115,#137116,#137117),
 .UNSPECIFIED.,.F.,.F.)
B_SPLINE_CURVE_WITH_KNOTS((3,2,3),(0.556212830496801,0.571428571428571,
0.573654350219911),.UNSPECIFIED.)
CURVE()
GEOMETRIC_REPRESENTATION_ITEM()
RATIONAL_B_SPLINE_CURVE((0.991593695322322,0.994659134499961,1.,0.999218731101516,
0.99848615229188))
REPRESENTATION_ITEM('')
);
#4449=(
BOUNDED_CURVE()
B_SPLINE_CURVE(2,(#137204,#137205,#137206,#137207,#137208),
 .UNSPECIFIED.,.F.,.F.)
B_SPLINE_CURVE_WITH_KNOTS((3,2,3),(0.556212830500266,0.571428571428571,
0.57365435021991),.UNSPECIFIED.)
CURVE()
GEOMETRIC_REPRESENTATION_ITEM()
RATIONAL_B_SPLINE_CURVE((0.991593695323718,0.994659134501177,1.,0.999218731101516,
0.99848615229188))
REPRESENTATION_ITEM('')
);
#4450=(
BOUNDED_CURVE()
B_SPLINE_CURVE(2,(#146696,#146697,#146698,#146699,#146700),
 .UNSPECIFIED.,.F.,.F.)
B_SPLINE_CURVE_WITH_KNOTS((3,2,3),(0.556108173865715,0.558333952657054,
0.573549700888524),.UNSPECIFIED.)
CURVE()
GEOMETRIC_REPRESENTATION_ITEM()
RATIONAL_B_SPLINE_CURVE((0.99848615229188,0.999218731101516,1.,0.994659131937698,
0.991593692381054))
REPRESENTATION_ITEM('')
);
#4451=(
BOUNDED_CURVE()
B_SPLINE_CURVE(2,(#146787,#146788,#146789,#146790,#146791),
 .UNSPECIFIED.,.F.,.F.)
B_SPLINE_CURVE_WITH_KNOTS((3,2,3),(0.556108173865715,0.558333952657055,
0.573549700890172),.UNSPECIFIED.)
CURVE()
GEOMETRIC_REPRESENTATION_ITEM()
RATIONAL_B_SPLINE_CURVE((0.99848615229188,0.999218731101516,1.,0.994659131937121,
0.991593692380391))
REPRESENTATION_ITEM('')
);
#4452=(
BOUNDED_CURVE()
B_SPLINE_CURVE(2,(#146828,#146829,#146830,#146831,#146832),
 .UNSPECIFIED.,.F.,.F.)
B_SPLINE_CURVE_WITH_KNOTS((3,2,3),(0.556108173865716,0.558333952657056,
0.573549700892252),.UNSPECIFIED.)
CURVE()
GEOMETRIC_REPRESENTATION_ITEM()
RATIONAL_B_SPLINE_CURVE((0.99848615229188,0.999218731101516,1.,0.994659131936391,
0.991593692379553))
REPRESENTATION_ITEM('')
);
#4453=(
BOUNDED_CURVE()
B_SPLINE_CURVE(2,(#147117,#147118,#147119,#147120,#147121),
 .UNSPECIFIED.,.F.,.F.)
B_SPLINE_CURVE_WITH_KNOTS((3,2,3),(0.556108173865716,0.558333952657056,
0.57354970089628),.UNSPECIFIED.)
CURVE()
GEOMETRIC_REPRESENTATION_ITEM()
RATIONAL_B_SPLINE_CURVE((0.99848615229188,0.999218731101516,1.,0.994659131934977,
0.99159369237793))
REPRESENTATION_ITEM('')
);
#4454=(
BOUNDED_CURVE()
B_SPLINE_CURVE(2,(#147208,#147209,#147210,#147211,#147212),
 .UNSPECIFIED.,.F.,.F.)
B_SPLINE_CURVE_WITH_KNOTS((3,2,3),(0.556108173865715,0.558333952657055,
0.573549700896557),.UNSPECIFIED.)
CURVE()
GEOMETRIC_REPRESENTATION_ITEM()
RATIONAL_B_SPLINE_CURVE((0.99848615229188,0.999218731101516,1.,0.994659131934879,
0.991593692377818))
REPRESENTATION_ITEM('')
);
#4455=(
BOUNDED_CURVE()
B_SPLINE_CURVE(2,(#147394,#147395,#147396,#147397,#147398),
 .UNSPECIFIED.,.F.,.F.)
B_SPLINE_CURVE_WITH_KNOTS((3,2,3),(0.556108173865716,0.558333952657056,
0.573549700888435),.UNSPECIFIED.)
CURVE()
GEOMETRIC_REPRESENTATION_ITEM()
RATIONAL_B_SPLINE_CURVE((0.99848615229188,0.999218731101516,1.,0.99465913193773,
0.99159369238109))
REPRESENTATION_ITEM('')
);
#4456=(
BOUNDED_CURVE()
B_SPLINE_CURVE(2,(#158499,#158500,#158501,#158502,#158503),
 .UNSPECIFIED.,.F.,.F.)
B_SPLINE_CURVE_WITH_KNOTS((3,2,3),(-0.0736543716039549,-0.0714285714285714,
-0.0665682420727563),.UNSPECIFIED.)
CURVE()
GEOMETRIC_REPRESENTATION_ITEM()
RATIONAL_B_SPLINE_CURVE((0.998486138215465,0.999218723595519,1.,0.99829397953792,
0.996820130073177))
REPRESENTATION_ITEM('')
);
#4457=(
BOUNDED_CURVE()
B_SPLINE_CURVE(2,(#167647,#167648,#167649,#167650,#167651),
 .UNSPECIFIED.,.F.,.F.)
B_SPLINE_CURVE_WITH_KNOTS((3,2,3),(-0.0736543503731481,-0.0714285714285714,
-0.0665682420727563),.UNSPECIFIED.)
CURVE()
GEOMETRIC_REPRESENTATION_ITEM()
RATIONAL_B_SPLINE_CURVE((0.998486152191009,0.999218731047729,1.,0.99829397953792,
0.996820130073177))
REPRESENTATION_ITEM('')
);
#4459=CYLINDRICAL_SURFACE('',#71533,3.25);
#4460=CYLINDRICAL_SURFACE('',#71537,7.);
#4461=CYLINDRICAL_SURFACE('',#71540,6.125);
#4462=CYLINDRICAL_SURFACE('',#71611,7.5000000000019);
#4463=CYLINDRICAL_SURFACE('',#71616,7.50000000000249);
#4464=CYLINDRICAL_SURFACE('',#71623,7.49999999999896);
#4465=CYLINDRICAL_SURFACE('',#71626,7.50000000000045);
#4466=CYLINDRICAL_SURFACE('',#71633,7.49999999999779);
#4467=CYLINDRICAL_SURFACE('',#71635,7.50000000000013);
#4468=CYLINDRICAL_SURFACE('',#71638,7.50000000000107);
#4469=CYLINDRICAL_SURFACE('',#71641,7.5);
#4470=CYLINDRICAL_SURFACE('',#71644,7.50000000000042);
#4471=CYLINDRICAL_SURFACE('',#71647,7.49999999999967);
#4472=CYLINDRICAL_SURFACE('',#71649,7.50000000000012);
#4473=CYLINDRICAL_SURFACE('',#71651,7.49999999999917);
#4474=CYLINDRICAL_SURFACE('',#71653,7.49999999999998);
#4475=CYLINDRICAL_SURFACE('',#71656,7.49999999999897);
#4476=CYLINDRICAL_SURFACE('',#71659,7.50000000000024);
#4477=CYLINDRICAL_SURFACE('',#71661,7.5000000000015);
#4478=CYLINDRICAL_SURFACE('',#71664,7.49999999999738);
#4479=CYLINDRICAL_SURFACE('',#71666,7.50000000000006);
#4480=CYLINDRICAL_SURFACE('',#71668,7.49999999999942);
#4481=CYLINDRICAL_SURFACE('',#71671,7.50000000000151);
#4482=CYLINDRICAL_SURFACE('',#71673,7.50000000000047);
#4483=CYLINDRICAL_SURFACE('',#71676,7.50000000000012);
#4484=CYLINDRICAL_SURFACE('',#71678,7.50000000000129);
#4485=CYLINDRICAL_SURFACE('',#71681,7.49999999999964);
#4486=CYLINDRICAL_SURFACE('',#71683,7.50000000000003);
#4487=CYLINDRICAL_SURFACE('',#71685,7.50000000000029);
#4488=CYLINDRICAL_SURFACE('',#71687,7.50000000000047);
#4489=CYLINDRICAL_SURFACE('',#71688,7.49999999999994);
#4490=CYLINDRICAL_SURFACE('',#71691,7.50000000000153);
#4491=CYLINDRICAL_SURFACE('',#71697,7.49999999999978);
#4492=CYLINDRICAL_SURFACE('',#71703,7.50000000000036);
#4493=CYLINDRICAL_SURFACE('',#71709,7.49999999999827);
#4494=CYLINDRICAL_SURFACE('',#71715,7.50000000000059);
#4495=CYLINDRICAL_SURFACE('',#71721,7.50000000000016);
#4496=CYLINDRICAL_SURFACE('',#71727,7.50000000000111);
#4497=CYLINDRICAL_SURFACE('',#71735,7.50000000000021);
#4498=CYLINDRICAL_SURFACE('',#71741,7.49999999999943);
#4499=CYLINDRICAL_SURFACE('',#71747,7.49999999999932);
#4500=CYLINDRICAL_SURFACE('',#71753,7.50000000000055);
#4501=CYLINDRICAL_SURFACE('',#71759,7.50000000000016);
#4502=CYLINDRICAL_SURFACE('',#71765,7.49999999999825);
#4503=CYLINDRICAL_SURFACE('',#71771,7.49999999999844);
#4504=CYLINDRICAL_SURFACE('',#71777,7.49999999999911);
#4505=CYLINDRICAL_SURFACE('',#71783,7.50000000000129);
#4506=CYLINDRICAL_SURFACE('',#71789,7.49999999999985);
#4507=CYLINDRICAL_SURFACE('',#71795,7.49999999999989);
#4508=CYLINDRICAL_SURFACE('',#71801,7.49999999999936);
#4509=CYLINDRICAL_SURFACE('',#71807,7.5000000000015);
#4510=CYLINDRICAL_SURFACE('',#71813,7.49999999999907);
#4511=CYLINDRICAL_SURFACE('',#71819,7.49999999999943);
#4512=CYLINDRICAL_SURFACE('',#71825,7.49999999999939);
#4513=CYLINDRICAL_SURFACE('',#71831,7.49999999999972);
#4514=CYLINDRICAL_SURFACE('',#71839,7.49999999999887);
#4515=CYLINDRICAL_SURFACE('',#71843,7.50000000000122);
#4516=CYLINDRICAL_SURFACE('',#71849,7.49999999999991);
#4517=CYLINDRICAL_SURFACE('',#71855,7.49999999999911);
#4518=CYLINDRICAL_SURFACE('',#71859,7.49999999999879);
#4519=CYLINDRICAL_SURFACE('',#71866,7.49999999999953);
#4520=CYLINDRICAL_SURFACE('',#71871,7.49999999999775);
#4521=CYLINDRICAL_SURFACE('',#71876,7.50000000000054);
#4522=CYLINDRICAL_SURFACE('',#71881,7.49999999999899);
#4523=CYLINDRICAL_SURFACE('',#71886,7.49999999999925);
#4524=CYLINDRICAL_SURFACE('',#71891,7.49999999999932);
#4525=CYLINDRICAL_SURFACE('',#71896,7.50000000000172);
#4526=CYLINDRICAL_SURFACE('',#71901,7.50000000000026);
#4527=CYLINDRICAL_SURFACE('',#71906,7.50000000000139);
#4528=CYLINDRICAL_SURFACE('',#71911,7.50000000000019);
#4529=CYLINDRICAL_SURFACE('',#71916,7.49999999999962);
#4530=CYLINDRICAL_SURFACE('',#71921,7.49999999999975);
#4531=CYLINDRICAL_SURFACE('',#71926,7.49999999999885);
#4532=CYLINDRICAL_SURFACE('',#71931,7.50000000000064);
#4533=CYLINDRICAL_SURFACE('',#71936,7.49999999999907);
#4534=CYLINDRICAL_SURFACE('',#71941,7.49999999999931);
#4535=CYLINDRICAL_SURFACE('',#71946,7.5000000000005);
#4536=CYLINDRICAL_SURFACE('',#71951,7.50000000000094);
#4537=CYLINDRICAL_SURFACE('',#71956,7.50000000000172);
#4538=CYLINDRICAL_SURFACE('',#71961,7.50000000000123);
#4539=CYLINDRICAL_SURFACE('',#71966,7.50000000000139);
#4540=CYLINDRICAL_SURFACE('',#71971,7.49999999999962);
#4541=CYLINDRICAL_SURFACE('',#71976,7.49999999999967);
#4542=CYLINDRICAL_SURFACE('',#71981,7.50000000000006);
#4543=CYLINDRICAL_SURFACE('',#71986,7.49999999999917);
#4544=CYLINDRICAL_SURFACE('',#71991,7.49999999999949);
#4545=CYLINDRICAL_SURFACE('',#71996,7.49999999999865);
#4546=CYLINDRICAL_SURFACE('',#71999,7.50000000000002);
#4547=CYLINDRICAL_SURFACE('',#72091,7.49999999999856);
#4548=CYLINDRICAL_SURFACE('',#72094,7.49999999999898);
#4549=CYLINDRICAL_SURFACE('',#72097,7.49999999999979);
#4550=CYLINDRICAL_SURFACE('',#72100,7.49999999999998);
#4551=CYLINDRICAL_SURFACE('',#72103,7.49999999999804);
#4552=CYLINDRICAL_SURFACE('',#72106,7.50000000000217);
#4553=CYLINDRICAL_SURFACE('',#72109,7.50000000000047);
#4554=CYLINDRICAL_SURFACE('',#72112,7.49999999999995);
#4555=CYLINDRICAL_SURFACE('',#72115,7.49999999999997);
#4556=CYLINDRICAL_SURFACE('',#72118,7.50000000000076);
#4557=CYLINDRICAL_SURFACE('',#72121,7.50000000000068);
#4558=CYLINDRICAL_SURFACE('',#72124,7.50000000000021);
#4559=CYLINDRICAL_SURFACE('',#72127,7.49999999999918);
#4560=CYLINDRICAL_SURFACE('',#72130,7.50000000000134);
#4561=CYLINDRICAL_SURFACE('',#72133,7.5000000000009);
#4562=CYLINDRICAL_SURFACE('',#72136,7.49999999999987);
#4563=CYLINDRICAL_SURFACE('',#72139,7.49999999999943);
#4564=CYLINDRICAL_SURFACE('',#72142,7.5);
#4565=CYLINDRICAL_SURFACE('',#72145,7.49999999999884);
#4566=CYLINDRICAL_SURFACE('',#72148,7.50000000000024);
#4567=CYLINDRICAL_SURFACE('',#72151,7.50000000000066);
#4568=CYLINDRICAL_SURFACE('',#72154,7.50000000000124);
#4569=CYLINDRICAL_SURFACE('',#72157,7.49999999999855);
#4570=CYLINDRICAL_SURFACE('',#72160,7.50000000000082);
#4571=CYLINDRICAL_SURFACE('',#72163,7.4999999999996);
#4572=CYLINDRICAL_SURFACE('',#72166,7.50000000000008);
#4573=CYLINDRICAL_SURFACE('',#72169,7.50000000000191);
#4574=CYLINDRICAL_SURFACE('',#72172,7.50000000000073);
#4575=CYLINDRICAL_SURFACE('',#72176,7.5000000000004);
#4576=CYLINDRICAL_SURFACE('',#72180,7.49999999999908);
#4577=CYLINDRICAL_SURFACE('',#72184,7.50000000000109);
#4578=CYLINDRICAL_SURFACE('',#72188,7.49999999999915);
#4579=CYLINDRICAL_SURFACE('',#72192,7.49999999999946);
#4580=CYLINDRICAL_SURFACE('',#72196,7.50000000000006);
#4581=CYLINDRICAL_SURFACE('',#72200,7.49999999999995);
#4582=CYLINDRICAL_SURFACE('',#72204,7.49999999999935);
#4583=CYLINDRICAL_SURFACE('',#72208,7.4999999999993);
#4584=CYLINDRICAL_SURFACE('',#72212,7.49999999999968);
#4585=CYLINDRICAL_SURFACE('',#72216,7.50000000000123);
#4586=CYLINDRICAL_SURFACE('',#72220,7.50000000000104);
#4587=CYLINDRICAL_SURFACE('',#72224,7.49999999999961);
#4588=CYLINDRICAL_SURFACE('',#72228,7.50000000000035);
#4589=CYLINDRICAL_SURFACE('',#72232,7.4999999999982);
#4590=CYLINDRICAL_SURFACE('',#72236,7.50000000000075);
#4591=CYLINDRICAL_SURFACE('',#72240,7.50000000000173);
#4592=CYLINDRICAL_SURFACE('',#72244,7.49999999999834);
#4593=CYLINDRICAL_SURFACE('',#72248,7.49999999999941);
#4594=CYLINDRICAL_SURFACE('',#72252,7.49999999999971);
#4595=CYLINDRICAL_SURFACE('',#72256,7.50000000000052);
#4596=CYLINDRICAL_SURFACE('',#72260,7.49999999999878);
#4597=CYLINDRICAL_SURFACE('',#72264,7.50000000000034);
#4598=CYLINDRICAL_SURFACE('',#72268,7.50000000000112);
#4599=CYLINDRICAL_SURFACE('',#72272,7.50000000000131);
#4600=CYLINDRICAL_SURFACE('',#72276,7.49999999999987);
#4601=CYLINDRICAL_SURFACE('',#72280,7.50000000000044);
#4602=CYLINDRICAL_SURFACE('',#72284,7.50000000000073);
#4603=CYLINDRICAL_SURFACE('',#72345,7.5000000000005);
#4604=CYLINDRICAL_SURFACE('',#72349,7.50000000000059);
#4605=CYLINDRICAL_SURFACE('',#72353,7.50000000000095);
#4606=CYLINDRICAL_SURFACE('',#72357,7.49999999999793);
#4607=CYLINDRICAL_SURFACE('',#72361,7.49999999999914);
#4608=CYLINDRICAL_SURFACE('',#72365,7.50000000000072);
#4609=CYLINDRICAL_SURFACE('',#72369,7.49999999999963);
#4610=CYLINDRICAL_SURFACE('',#72373,7.49999999999949);
#4611=CYLINDRICAL_SURFACE('',#72377,7.50000000000053);
#4612=CYLINDRICAL_SURFACE('',#72381,7.50000000000013);
#4613=CYLINDRICAL_SURFACE('',#72385,7.50000000000036);
#4614=CYLINDRICAL_SURFACE('',#72389,7.50000000000167);
#4615=CYLINDRICAL_SURFACE('',#72393,7.49999999999751);
#4616=CYLINDRICAL_SURFACE('',#72397,7.49999999999885);
#4617=CYLINDRICAL_SURFACE('',#72401,7.50000000000097);
#4618=CYLINDRICAL_SURFACE('',#72405,7.49999999999976);
#4619=CYLINDRICAL_SURFACE('',#72409,7.49999999999933);
#4620=CYLINDRICAL_SURFACE('',#72413,7.49999999999933);
#4621=CYLINDRICAL_SURFACE('',#72417,7.49999999999827);
#4622=CYLINDRICAL_SURFACE('',#72421,7.50000000000131);
#4623=CYLINDRICAL_SURFACE('',#72425,7.50000000000009);
#4624=CYLINDRICAL_SURFACE('',#72429,7.50000000000029);
#4625=CYLINDRICAL_SURFACE('',#72434,7.49999999999913);
#4626=CYLINDRICAL_SURFACE('',#72437,7.50000000000064);
#4627=CYLINDRICAL_SURFACE('',#72441,7.50000000000118);
#4628=CYLINDRICAL_SURFACE('',#72445,7.49999999999926);
#4629=CYLINDRICAL_SURFACE('',#72449,7.49999999999923);
#4630=CYLINDRICAL_SURFACE('',#72453,7.50000000000082);
#4631=CYLINDRICAL_SURFACE('',#72458,7.49999999999976);
#4632=CYLINDRICAL_SURFACE('',#72462,7.49999999999993);
#4633=CYLINDRICAL_SURFACE('',#72466,7.50000000000046);
#4634=CYLINDRICAL_SURFACE('',#72470,7.50000000000008);
#4635=CYLINDRICAL_SURFACE('',#72474,7.49999999999994);
#4636=CYLINDRICAL_SURFACE('',#72478,7.50000000000125);
#4637=CYLINDRICAL_SURFACE('',#72482,7.49999999999926);
#4638=CYLINDRICAL_SURFACE('',#72486,7.49999999999853);
#4639=CYLINDRICAL_SURFACE('',#72490,7.49999999999969);
#4640=CYLINDRICAL_SURFACE('',#72494,7.49999999999989);
#4641=CYLINDRICAL_SURFACE('',#72498,7.50000000000173);
#4642=CYLINDRICAL_SURFACE('',#72502,7.4999999999987);
#4643=CYLINDRICAL_SURFACE('',#72506,7.50000000000052);
#4644=CYLINDRICAL_SURFACE('',#72510,7.50000000000042);
#4645=CYLINDRICAL_SURFACE('',#72514,7.5000000000004);
#4646=CYLINDRICAL_SURFACE('',#72518,7.50000000000212);
#4647=CYLINDRICAL_SURFACE('',#72522,7.50000000000009);
#4648=CYLINDRICAL_SURFACE('',#72526,7.50000000000025);
#4649=CYLINDRICAL_SURFACE('',#72530,7.4999999999998);
#4650=CYLINDRICAL_SURFACE('',#72534,7.50000000000038);
#4651=CYLINDRICAL_SURFACE('',#72538,7.49999999999992);
#4652=CYLINDRICAL_SURFACE('',#72542,7.49999999999992);
#4653=CYLINDRICAL_SURFACE('',#72546,7.50000000000101);
#4654=CYLINDRICAL_SURFACE('',#72550,7.49999999999969);
#4655=CYLINDRICAL_SURFACE('',#72554,7.50000000000117);
#4656=CYLINDRICAL_SURFACE('',#72558,7.4999999999993);
#4657=CYLINDRICAL_SURFACE('',#72562,7.49999999999926);
#4658=CYLINDRICAL_SURFACE('',#72565,7.49999999999808);
#4659=CYLINDRICAL_SURFACE('',#72656,7.49999999999972);
#4660=CYLINDRICAL_SURFACE('',#72661,7.49999999999782);
#4661=CYLINDRICAL_SURFACE('',#72666,7.49999999999986);
#4662=CYLINDRICAL_SURFACE('',#72671,7.50000000000091);
#4663=CYLINDRICAL_SURFACE('',#72676,7.49999999999878);
#4664=CYLINDRICAL_SURFACE('',#72681,7.50000000000178);
#4665=CYLINDRICAL_SURFACE('',#72686,7.49999999999909);
#4666=CYLINDRICAL_SURFACE('',#72691,7.5000000000006);
#4667=CYLINDRICAL_SURFACE('',#72696,7.4999999999991);
#4668=CYLINDRICAL_SURFACE('',#72701,7.4999999999995);
#4669=CYLINDRICAL_SURFACE('',#72706,7.49999999999992);
#4670=CYLINDRICAL_SURFACE('',#72711,7.49999999999957);
#4671=CYLINDRICAL_SURFACE('',#72716,7.5000000000003);
#4672=CYLINDRICAL_SURFACE('',#72721,7.49999999999944);
#4673=CYLINDRICAL_SURFACE('',#72726,7.50000000000098);
#4674=CYLINDRICAL_SURFACE('',#72731,7.5000000000002);
#4675=CYLINDRICAL_SURFACE('',#72736,7.50000000000003);
#4676=CYLINDRICAL_SURFACE('',#72741,7.50000000000008);
#4677=CYLINDRICAL_SURFACE('',#72746,7.49999999999799);
#4678=CYLINDRICAL_SURFACE('',#72751,7.49999999999937);
#4679=CYLINDRICAL_SURFACE('',#72756,7.5000000000009);
#4680=CYLINDRICAL_SURFACE('',#72761,7.50000000000057);
#4681=CYLINDRICAL_SURFACE('',#72767,7.49999999999968);
#4682=CYLINDRICAL_SURFACE('',#72771,7.50000000000128);
#4683=CYLINDRICAL_SURFACE('',#72776,7.49999999999952);
#4684=CYLINDRICAL_SURFACE('',#72781,7.5);
#4685=CYLINDRICAL_SURFACE('',#72786,7.50000000000135);
#4686=CYLINDRICAL_SURFACE('',#72791,7.4999999999995);
#4687=CYLINDRICAL_SURFACE('',#72796,7.50000000000061);
#4688=CYLINDRICAL_SURFACE('',#72800,7.4999999999991);
#4689=CYLINDRICAL_SURFACE('',#72804,7.49999999999952);
#4690=CYLINDRICAL_SURFACE('',#72808,7.50000000000152);
#4691=CYLINDRICAL_SURFACE('',#72812,7.49999999999977);
#4692=CYLINDRICAL_SURFACE('',#72816,7.50000000000048);
#4693=CYLINDRICAL_SURFACE('',#72820,7.50000000000133);
#4694=CYLINDRICAL_SURFACE('',#72824,7.49999999999992);
#4695=CYLINDRICAL_SURFACE('',#72828,7.50000000000004);
#4696=CYLINDRICAL_SURFACE('',#72832,7.49999999999888);
#4697=CYLINDRICAL_SURFACE('',#72836,7.49999999999974);
#4698=CYLINDRICAL_SURFACE('',#72840,7.50000000000138);
#4699=CYLINDRICAL_SURFACE('',#72844,7.49999999999858);
#4700=CYLINDRICAL_SURFACE('',#72848,7.5000000000013);
#4701=CYLINDRICAL_SURFACE('',#72852,7.50000000000192);
#4702=CYLINDRICAL_SURFACE('',#72856,7.50000000000123);
#4703=CYLINDRICAL_SURFACE('',#72860,7.50000000000003);
#4704=CYLINDRICAL_SURFACE('',#72864,7.50000000000171);
#4705=CYLINDRICAL_SURFACE('',#72868,7.49999999999925);
#4706=CYLINDRICAL_SURFACE('',#72872,7.49999999999916);
#4707=CYLINDRICAL_SURFACE('',#72876,7.5000000000006);
#4708=CYLINDRICAL_SURFACE('',#72880,7.49999999999937);
#4709=CYLINDRICAL_SURFACE('',#72884,7.49999999999992);
#4710=CYLINDRICAL_SURFACE('',#72888,7.50000000000151);
#4711=CYLINDRICAL_SURFACE('',#72892,7.50000000000037);
#4712=CYLINDRICAL_SURFACE('',#72896,7.50000000000052);
#4713=CYLINDRICAL_SURFACE('',#72900,7.50000000000022);
#4714=CYLINDRICAL_SURFACE('',#72904,7.50000000000124);
#4715=CYLINDRICAL_SURFACE('',#72908,7.49999999999967);
#4716=CYLINDRICAL_SURFACE('',#73029,7.49999999999918);
#4717=CYLINDRICAL_SURFACE('',#73033,7.49999999999899);
#4718=CYLINDRICAL_SURFACE('',#73037,7.49999999999804);
#4719=CYLINDRICAL_SURFACE('',#73041,7.49999999999938);
#4720=CYLINDRICAL_SURFACE('',#73045,7.49999999999996);
#4721=CYLINDRICAL_SURFACE('',#73049,7.50000000000072);
#4722=CYLINDRICAL_SURFACE('',#73053,7.49999999999797);
#4723=CYLINDRICAL_SURFACE('',#73057,7.50000000000107);
#4724=CYLINDRICAL_SURFACE('',#73061,7.49999999999992);
#4725=CYLINDRICAL_SURFACE('',#73065,7.49999999999948);
#4726=CYLINDRICAL_SURFACE('',#73069,7.50000000000065);
#4727=CYLINDRICAL_SURFACE('',#73073,7.500000000001);
#4728=CYLINDRICAL_SURFACE('',#73077,7.50000000000035);
#4729=CYLINDRICAL_SURFACE('',#73081,7.49999999999899);
#4730=CYLINDRICAL_SURFACE('',#73085,7.49999999999896);
#4731=CYLINDRICAL_SURFACE('',#73089,7.49999999999911);
#4732=CYLINDRICAL_SURFACE('',#73093,7.49999999999864);
#4733=CYLINDRICAL_SURFACE('',#73097,7.50000000000138);
#4734=CYLINDRICAL_SURFACE('',#73101,7.50000000000113);
#4735=CYLINDRICAL_SURFACE('',#73105,7.49999999999821);
#4736=CYLINDRICAL_SURFACE('',#73109,7.49999999999997);
#4737=CYLINDRICAL_SURFACE('',#73114,7.50000000000013);
#4738=CYLINDRICAL_SURFACE('',#73117,7.4999999999984);
#4739=CYLINDRICAL_SURFACE('',#73121,7.49999999999845);
#4740=CYLINDRICAL_SURFACE('',#73125,7.49999999999939);
#4741=CYLINDRICAL_SURFACE('',#73129,7.5000000000014);
#4742=CYLINDRICAL_SURFACE('',#73133,7.49999999999944);
#4743=CYLINDRICAL_SURFACE('',#73136,7.50000000000009);
#4744=CYLINDRICAL_SURFACE('',#73142,7.50000000000093);
#4745=CYLINDRICAL_SURFACE('',#73147,7.50000000000101);
#4746=CYLINDRICAL_SURFACE('',#73152,7.50000000000019);
#4747=CYLINDRICAL_SURFACE('',#73157,7.50000000000078);
#4748=CYLINDRICAL_SURFACE('',#73162,7.49999999999956);
#4749=CYLINDRICAL_SURFACE('',#73167,7.49999999999952);
#4750=CYLINDRICAL_SURFACE('',#73172,7.49999999999875);
#4751=CYLINDRICAL_SURFACE('',#73177,7.50000000000101);
#4752=CYLINDRICAL_SURFACE('',#73182,7.49999999999994);
#4753=CYLINDRICAL_SURFACE('',#73187,7.49999999999869);
#4754=CYLINDRICAL_SURFACE('',#73192,7.50000000000083);
#4755=CYLINDRICAL_SURFACE('',#73197,7.50000000000055);
#4756=CYLINDRICAL_SURFACE('',#73202,7.49999999999946);
#4757=CYLINDRICAL_SURFACE('',#73207,7.49999999999996);
#4758=CYLINDRICAL_SURFACE('',#73212,7.49999999999975);
#4759=CYLINDRICAL_SURFACE('',#73217,7.50000000000033);
#4760=CYLINDRICAL_SURFACE('',#73222,7.49999999999967);
#4761=CYLINDRICAL_SURFACE('',#73227,7.49999999999812);
#4762=CYLINDRICAL_SURFACE('',#73232,7.49999999999913);
#4763=CYLINDRICAL_SURFACE('',#73237,7.50000000000017);
#4764=CYLINDRICAL_SURFACE('',#73242,7.49999999999952);
#4765=CYLINDRICAL_SURFACE('',#73247,7.49999999999948);
#4766=CYLINDRICAL_SURFACE('',#73252,7.49999999999999);
#4767=CYLINDRICAL_SURFACE('',#73257,7.50000000000098);
#4768=CYLINDRICAL_SURFACE('',#73262,7.4999999999991);
#4769=CYLINDRICAL_SURFACE('',#73267,7.49999999999897);
#4770=CYLINDRICAL_SURFACE('',#73272,7.5000000000004);
#4771=CYLINDRICAL_SURFACE('',#73275,7.50000000000016);
#4772=CYLINDRICAL_SURFACE('',#73367,7.50000000000024);
#4773=CYLINDRICAL_SURFACE('',#73371,7.49999999999933);
#4774=CYLINDRICAL_SURFACE('',#73375,7.50000000000075);
#4775=CYLINDRICAL_SURFACE('',#73379,7.50000000000048);
#4776=CYLINDRICAL_SURFACE('',#73383,7.49999999999963);
#4777=CYLINDRICAL_SURFACE('',#73387,7.49999999999864);
#4778=CYLINDRICAL_SURFACE('',#73391,7.50000000000096);
#4779=CYLINDRICAL_SURFACE('',#73395,7.50000000000103);
#4780=CYLINDRICAL_SURFACE('',#73399,7.50000000000109);
#4781=CYLINDRICAL_SURFACE('',#73403,7.50000000000174);
#4782=CYLINDRICAL_SURFACE('',#73407,7.50000000000068);
#4783=CYLINDRICAL_SURFACE('',#73411,7.49999999999957);
#4784=CYLINDRICAL_SURFACE('',#73415,7.49999999999931);
#4785=CYLINDRICAL_SURFACE('',#73419,7.49999999999943);
#4786=CYLINDRICAL_SURFACE('',#73423,7.50000000000114);
#4787=CYLINDRICAL_SURFACE('',#73427,7.49999999999958);
#4788=CYLINDRICAL_SURFACE('',#73431,7.50000000000009);
#4789=CYLINDRICAL_SURFACE('',#73435,7.49999999999893);
#4790=CYLINDRICAL_SURFACE('',#73439,7.499999999999);
#4791=CYLINDRICAL_SURFACE('',#73443,7.50000000000161);
#4792=CYLINDRICAL_SURFACE('',#73447,7.50000000000002);
#4793=CYLINDRICAL_SURFACE('',#73451,7.499999999999);
#4794=CYLINDRICAL_SURFACE('',#73455,7.50000000000037);
#4795=CYLINDRICAL_SURFACE('',#73459,7.50000000000065);
#4796=CYLINDRICAL_SURFACE('',#73463,7.50000000000121);
#4797=CYLINDRICAL_SURFACE('',#73467,7.49999999999954);
#4798=CYLINDRICAL_SURFACE('',#73471,7.5000000000004);
#4799=CYLINDRICAL_SURFACE('',#73475,7.49999999999934);
#4800=CYLINDRICAL_SURFACE('',#73480,7.5000000000006);
#4801=CYLINDRICAL_SURFACE('',#73485,7.50000000000082);
#4802=CYLINDRICAL_SURFACE('',#73490,7.5000000000001);
#4803=CYLINDRICAL_SURFACE('',#73495,7.49999999999925);
#4804=CYLINDRICAL_SURFACE('',#73500,7.49999999999948);
#4805=CYLINDRICAL_SURFACE('',#73505,7.50000000000036);
#4806=CYLINDRICAL_SURFACE('',#73510,7.50000000000125);
#4807=CYLINDRICAL_SURFACE('',#73515,7.50000000000139);
#4808=CYLINDRICAL_SURFACE('',#73520,7.49999999999891);
#4809=CYLINDRICAL_SURFACE('',#73525,7.50000000000095);
#4810=CYLINDRICAL_SURFACE('',#73530,7.5000000000018);
#4811=CYLINDRICAL_SURFACE('',#73535,7.50000000000146);
#4812=CYLINDRICAL_SURFACE('',#73540,7.50000000000031);
#4813=CYLINDRICAL_SURFACE('',#73545,7.50000000000054);
#4814=CYLINDRICAL_SURFACE('',#73550,7.49999999999982);
#4815=CYLINDRICAL_SURFACE('',#73555,7.50000000000102);
#4816=CYLINDRICAL_SURFACE('',#73560,7.49999999999954);
#4817=CYLINDRICAL_SURFACE('',#73565,7.50000000000099);
#4818=CYLINDRICAL_SURFACE('',#73570,7.50000000000137);
#4819=CYLINDRICAL_SURFACE('',#73575,7.50000000000115);
#4820=CYLINDRICAL_SURFACE('',#73580,7.49999999999994);
#4821=CYLINDRICAL_SURFACE('',#73585,7.4999999999994);
#4822=CYLINDRICAL_SURFACE('',#73590,7.50000000000148);
#4823=CYLINDRICAL_SURFACE('',#73595,7.49999999999962);
#4824=CYLINDRICAL_SURFACE('',#73600,7.4999999999996);
#4825=CYLINDRICAL_SURFACE('',#73605,7.4999999999989);
#4826=CYLINDRICAL_SURFACE('',#73610,7.49999999999878);
#4827=CYLINDRICAL_SURFACE('',#73615,7.49999999999946);
#4828=CYLINDRICAL_SURFACE('',#73677,7.49999999999873);
#4829=CYLINDRICAL_SURFACE('',#73681,7.4999999999998);
#4830=CYLINDRICAL_SURFACE('',#73685,7.50000000000156);
#4831=CYLINDRICAL_SURFACE('',#73689,7.49999999999997);
#4832=CYLINDRICAL_SURFACE('',#73693,7.50000000000053);
#4833=CYLINDRICAL_SURFACE('',#73697,7.5000000000006);
#4834=CYLINDRICAL_SURFACE('',#73701,7.50000000000044);
#4835=CYLINDRICAL_SURFACE('',#73705,7.50000000000109);
#4836=CYLINDRICAL_SURFACE('',#73709,7.50000000000118);
#4837=CYLINDRICAL_SURFACE('',#73713,7.49999999999971);
#4838=CYLINDRICAL_SURFACE('',#73717,7.49999999999824);
#4839=CYLINDRICAL_SURFACE('',#73721,7.49999999999969);
#4840=CYLINDRICAL_SURFACE('',#73725,7.50000000000001);
#4841=CYLINDRICAL_SURFACE('',#73729,7.50000000000027);
#4842=CYLINDRICAL_SURFACE('',#73733,7.50000000000108);
#4843=CYLINDRICAL_SURFACE('',#73737,7.50000000000155);
#4844=CYLINDRICAL_SURFACE('',#73741,7.49999999999977);
#4845=CYLINDRICAL_SURFACE('',#73745,7.49999999999988);
#4846=CYLINDRICAL_SURFACE('',#73749,7.49999999999933);
#4847=CYLINDRICAL_SURFACE('',#73753,7.49999999999938);
#4848=CYLINDRICAL_SURFACE('',#73758,7.50000000000141);
#4849=CYLINDRICAL_SURFACE('',#73761,7.49999999999987);
#4850=CYLINDRICAL_SURFACE('',#73765,7.49999999999894);
#4851=CYLINDRICAL_SURFACE('',#73769,7.50000000000072);
#4852=CYLINDRICAL_SURFACE('',#73773,7.50000000000035);
#4853=CYLINDRICAL_SURFACE('',#73777,7.50000000000078);
#4854=CYLINDRICAL_SURFACE('',#73781,7.5000000000011);
#4855=CYLINDRICAL_SURFACE('',#73785,7.49999999999968);
#4856=CYLINDRICAL_SURFACE('',#73790,7.50000000000073);
#4857=CYLINDRICAL_SURFACE('',#73794,7.49999999999964);
#4858=CYLINDRICAL_SURFACE('',#73798,7.50000000000016);
#4859=CYLINDRICAL_SURFACE('',#73802,7.50000000000077);
#4860=CYLINDRICAL_SURFACE('',#73806,7.49999999999883);
#4861=CYLINDRICAL_SURFACE('',#73810,7.49999999999898);
#4862=CYLINDRICAL_SURFACE('',#73814,7.50000000000104);
#4863=CYLINDRICAL_SURFACE('',#73818,7.49999999999999);
#4864=CYLINDRICAL_SURFACE('',#73822,7.4999999999997);
#4865=CYLINDRICAL_SURFACE('',#73826,7.50000000000055);
#4866=CYLINDRICAL_SURFACE('',#73830,7.5000000000011);
#4867=CYLINDRICAL_SURFACE('',#73834,7.49999999999919);
#4868=CYLINDRICAL_SURFACE('',#73838,7.50000000000024);
#4869=CYLINDRICAL_SURFACE('',#73842,7.4999999999999);
#4870=CYLINDRICAL_SURFACE('',#73846,7.4999999999998);
#4871=CYLINDRICAL_SURFACE('',#73850,7.50000000000136);
#4872=CYLINDRICAL_SURFACE('',#73854,7.49999999999837);
#4873=CYLINDRICAL_SURFACE('',#73858,7.4999999999993);
#4874=CYLINDRICAL_SURFACE('',#73862,7.50000000000194);
#4875=CYLINDRICAL_SURFACE('',#73866,7.50000000000107);
#4876=CYLINDRICAL_SURFACE('',#73870,7.49999999999828);
#4877=CYLINDRICAL_SURFACE('',#73874,7.50000000000107);
#4878=CYLINDRICAL_SURFACE('',#73878,7.50000000000048);
#4879=CYLINDRICAL_SURFACE('',#73882,7.49999999999992);
#4880=CYLINDRICAL_SURFACE('',#73886,7.49999999999992);
#4881=CYLINDRICAL_SURFACE('',#73890,7.49999999999964);
#4882=CYLINDRICAL_SURFACE('',#73894,7.49999999999907);
#4883=CYLINDRICAL_SURFACE('',#73897,7.49999999999886);
#4884=CYLINDRICAL_SURFACE('',#73988,7.50000000000108);
#4885=CYLINDRICAL_SURFACE('',#73993,7.49999999999884);
#4886=CYLINDRICAL_SURFACE('',#73998,7.50000000000104);
#4887=CYLINDRICAL_SURFACE('',#74003,7.49999999999938);
#4888=CYLINDRICAL_SURFACE('',#74008,7.49999999999986);
#4889=CYLINDRICAL_SURFACE('',#74013,7.5000000000004);
#4890=CYLINDRICAL_SURFACE('',#74018,7.49999999999964);
#4891=CYLINDRICAL_SURFACE('',#74023,7.50000000000035);
#4892=CYLINDRICAL_SURFACE('',#74028,7.50000000000071);
#4893=CYLINDRICAL_SURFACE('',#74033,7.49999999999945);
#4894=CYLINDRICAL_SURFACE('',#74038,7.50000000000004);
#4895=CYLINDRICAL_SURFACE('',#74043,7.49999999999904);
#4896=CYLINDRICAL_SURFACE('',#74048,7.49999999999924);
#4897=CYLINDRICAL_SURFACE('',#74053,7.50000000000149);
#4898=CYLINDRICAL_SURFACE('',#74058,7.49999999999987);
#4899=CYLINDRICAL_SURFACE('',#74063,7.50000000000046);
#4900=CYLINDRICAL_SURFACE('',#74068,7.49999999999963);
#4901=CYLINDRICAL_SURFACE('',#74073,7.49999999999954);
#4902=CYLINDRICAL_SURFACE('',#74078,7.49999999999914);
#4903=CYLINDRICAL_SURFACE('',#74083,7.50000000000008);
#4904=CYLINDRICAL_SURFACE('',#74089,7.50000000000167);
#4905=CYLINDRICAL_SURFACE('',#74093,7.50000000000075);
#4906=CYLINDRICAL_SURFACE('',#74098,7.50000000000071);
#4907=CYLINDRICAL_SURFACE('',#74103,7.5000000000001);
#4908=CYLINDRICAL_SURFACE('',#74108,7.49999999999912);
#4909=CYLINDRICAL_SURFACE('',#74113,7.49999999999949);
#4910=CYLINDRICAL_SURFACE('',#74118,7.49999999999822);
#4911=CYLINDRICAL_SURFACE('',#74123,7.50000000000116);
#4912=CYLINDRICAL_SURFACE('',#74128,7.50000000000107);
#4913=CYLINDRICAL_SURFACE('',#74132,7.500000000001);
#4914=CYLINDRICAL_SURFACE('',#74136,7.49999999999867);
#4915=CYLINDRICAL_SURFACE('',#74140,7.50000000000072);
#4916=CYLINDRICAL_SURFACE('',#74144,7.50000000000002);
#4917=CYLINDRICAL_SURFACE('',#74148,7.50000000000016);
#4918=CYLINDRICAL_SURFACE('',#74152,7.4999999999977);
#4919=CYLINDRICAL_SURFACE('',#74156,7.50000000000075);
#4920=CYLINDRICAL_SURFACE('',#74160,7.50000000000128);
#4921=CYLINDRICAL_SURFACE('',#74164,7.50000000000007);
#4922=CYLINDRICAL_SURFACE('',#74168,7.49999999999968);
#4923=CYLINDRICAL_SURFACE('',#74172,7.49999999999942);
#4924=CYLINDRICAL_SURFACE('',#74176,7.49999999999947);
#4925=CYLINDRICAL_SURFACE('',#74180,7.49999999999886);
#4926=CYLINDRICAL_SURFACE('',#74184,7.49999999999996);
#4927=CYLINDRICAL_SURFACE('',#74188,7.49999999999863);
#4928=CYLINDRICAL_SURFACE('',#74192,7.49999999999905);
#4929=CYLINDRICAL_SURFACE('',#74196,7.49999999999839);
#4930=CYLINDRICAL_SURFACE('',#74200,7.50000000000018);
#4931=CYLINDRICAL_SURFACE('',#74204,7.50000000000139);
#4932=CYLINDRICAL_SURFACE('',#74208,7.50000000000011);
#4933=CYLINDRICAL_SURFACE('',#74212,7.49999999999936);
#4934=CYLINDRICAL_SURFACE('',#74216,7.49999999999924);
#4935=CYLINDRICAL_SURFACE('',#74220,7.49999999999896);
#4936=CYLINDRICAL_SURFACE('',#74224,7.50000000000106);
#4937=CYLINDRICAL_SURFACE('',#74228,7.49999999999841);
#4938=CYLINDRICAL_SURFACE('',#74232,7.5000000000007);
#4939=CYLINDRICAL_SURFACE('',#74236,7.49999999999929);
#4940=CYLINDRICAL_SURFACE('',#74357,7.49999999999838);
#4941=CYLINDRICAL_SURFACE('',#74362,7.49999999999869);
#4942=CYLINDRICAL_SURFACE('',#74367,7.50000000000082);
#4943=CYLINDRICAL_SURFACE('',#74372,7.50000000000171);
#4944=CYLINDRICAL_SURFACE('',#74377,7.49999999999838);
#4945=CYLINDRICAL_SURFACE('',#74382,7.49999999999738);
#4946=CYLINDRICAL_SURFACE('',#74387,7.49999999999968);
#4947=CYLINDRICAL_SURFACE('',#74392,7.49999999999915);
#4948=CYLINDRICAL_SURFACE('',#74397,7.50000000000115);
#4949=CYLINDRICAL_SURFACE('',#74402,7.49999999999923);
#4950=CYLINDRICAL_SURFACE('',#74407,7.49999999999971);
#4951=CYLINDRICAL_SURFACE('',#74412,7.50000000000045);
#4952=CYLINDRICAL_SURFACE('',#74417,7.4999999999983);
#4953=CYLINDRICAL_SURFACE('',#74422,7.49999999999974);
#4954=CYLINDRICAL_SURFACE('',#74427,7.50000000000059);
#4955=CYLINDRICAL_SURFACE('',#74432,7.49999999999865);
#4956=CYLINDRICAL_SURFACE('',#74437,7.5000000000016);
#4957=CYLINDRICAL_SURFACE('',#74442,7.49999999999936);
#4958=CYLINDRICAL_SURFACE('',#74447,7.49999999999902);
#4959=CYLINDRICAL_SURFACE('',#74453,7.5000000000002);
#4960=CYLINDRICAL_SURFACE('',#74457,7.50000000000014);
#4961=CYLINDRICAL_SURFACE('',#74462,7.50000000000037);
#4962=CYLINDRICAL_SURFACE('',#74467,7.5000000000016);
#4963=CYLINDRICAL_SURFACE('',#74472,7.49999999999911);
#4964=CYLINDRICAL_SURFACE('',#74477,7.49999999999995);
#4965=CYLINDRICAL_SURFACE('',#74482,7.50000000000142);
#4966=CYLINDRICAL_SURFACE('',#74487,7.50000000000018);
#4967=CYLINDRICAL_SURFACE('',#74491,7.49999999999995);
#4968=CYLINDRICAL_SURFACE('',#74498,7.49999999999969);
#4969=CYLINDRICAL_SURFACE('',#74503,7.50000000000032);
#4970=CYLINDRICAL_SURFACE('',#74508,7.50000000000134);
#4971=CYLINDRICAL_SURFACE('',#74513,7.50000000000005);
#4972=CYLINDRICAL_SURFACE('',#74518,7.50000000000026);
#4973=CYLINDRICAL_SURFACE('',#74523,7.5000000000011);
#4974=CYLINDRICAL_SURFACE('',#74528,7.50000000000166);
#4975=CYLINDRICAL_SURFACE('',#74533,7.49999999999912);
#4976=CYLINDRICAL_SURFACE('',#74538,7.50000000000039);
#4977=CYLINDRICAL_SURFACE('',#74543,7.49999999999916);
#4978=CYLINDRICAL_SURFACE('',#74548,7.49999999999987);
#4979=CYLINDRICAL_SURFACE('',#74553,7.49999999999992);
#4980=CYLINDRICAL_SURFACE('',#74558,7.49999999999871);
#4981=CYLINDRICAL_SURFACE('',#74563,7.5000000000005);
#4982=CYLINDRICAL_SURFACE('',#74568,7.50000000000091);
#4983=CYLINDRICAL_SURFACE('',#74573,7.50000000000126);
#4984=CYLINDRICAL_SURFACE('',#74578,7.50000000000107);
#4985=CYLINDRICAL_SURFACE('',#74583,7.50000000000023);
#4986=CYLINDRICAL_SURFACE('',#74588,7.49999999999994);
#4987=CYLINDRICAL_SURFACE('',#74593,7.50000000000013);
#4988=CYLINDRICAL_SURFACE('',#74598,7.50000000000086);
#4989=CYLINDRICAL_SURFACE('',#74603,7.50000000000015);
#4990=CYLINDRICAL_SURFACE('',#74608,7.50000000000103);
#4991=CYLINDRICAL_SURFACE('',#74613,7.50000000000045);
#4992=CYLINDRICAL_SURFACE('',#74618,7.50000000000103);
#4993=CYLINDRICAL_SURFACE('',#74623,7.49999999999952);
#4994=CYLINDRICAL_SURFACE('',#74628,7.50000000000068);
#4995=CYLINDRICAL_SURFACE('',#74631,7.49999999999993);
#4996=CYLINDRICAL_SURFACE('',#74723,7.49999999999987);
#4997=CYLINDRICAL_SURFACE('',#74727,7.49999999999988);
#4998=CYLINDRICAL_SURFACE('',#74731,7.49999999999856);
#4999=CYLINDRICAL_SURFACE('',#74735,7.50000000000064);
#5000=CYLINDRICAL_SURFACE('',#74739,7.50000000000078);
#5001=CYLINDRICAL_SURFACE('',#74743,7.50000000000074);
#5002=CYLINDRICAL_SURFACE('',#74747,7.49999999999937);
#5003=CYLINDRICAL_SURFACE('',#74751,7.50000000000038);
#5004=CYLINDRICAL_SURFACE('',#74755,7.50000000000138);
#5005=CYLINDRICAL_SURFACE('',#74759,7.50000000000087);
#5006=CYLINDRICAL_SURFACE('',#74763,7.50000000000108);
#5007=CYLINDRICAL_SURFACE('',#74767,7.49999999999908);
#5008=CYLINDRICAL_SURFACE('',#74771,7.49999999999961);
#5009=CYLINDRICAL_SURFACE('',#74775,7.50000000000016);
#5010=CYLINDRICAL_SURFACE('',#74779,7.4999999999995);
#5011=CYLINDRICAL_SURFACE('',#74783,7.50000000000142);
#5012=CYLINDRICAL_SURFACE('',#74787,7.50000000000107);
#5013=CYLINDRICAL_SURFACE('',#74791,7.50000000000045);
#5014=CYLINDRICAL_SURFACE('',#74795,7.49999999999951);
#5015=CYLINDRICAL_SURFACE('',#74799,7.4999999999989);
#5016=CYLINDRICAL_SURFACE('',#74803,7.49999999999918);
#5017=CYLINDRICAL_SURFACE('',#74807,7.50000000000033);
#5018=CYLINDRICAL_SURFACE('',#74811,7.49999999999982);
#5019=CYLINDRICAL_SURFACE('',#74815,7.49999999999988);
#5020=CYLINDRICAL_SURFACE('',#74819,7.50000000000107);
#5021=CYLINDRICAL_SURFACE('',#74823,7.50000000000036);
#5022=CYLINDRICAL_SURFACE('',#74827,7.50000000000041);
#5023=CYLINDRICAL_SURFACE('',#74831,7.50000000000068);
#5024=CYLINDRICAL_SURFACE('',#74836,7.50000000000055);
#5025=CYLINDRICAL_SURFACE('',#74841,7.49999999999906);
#5026=CYLINDRICAL_SURFACE('',#74846,7.49999999999978);
#5027=CYLINDRICAL_SURFACE('',#74851,7.50000000000051);
#5028=CYLINDRICAL_SURFACE('',#74856,7.50000000000021);
#5029=CYLINDRICAL_SURFACE('',#74861,7.50000000000068);
#5030=CYLINDRICAL_SURFACE('',#74866,7.50000000000086);
#5031=CYLINDRICAL_SURFACE('',#74871,7.50000000000036);
#5032=CYLINDRICAL_SURFACE('',#74876,7.50000000000095);
#5033=CYLINDRICAL_SURFACE('',#74881,7.50000000000105);
#5034=CYLINDRICAL_SURFACE('',#74886,7.50000000000114);
#5035=CYLINDRICAL_SURFACE('',#74891,7.5000000000009);
#5036=CYLINDRICAL_SURFACE('',#74896,7.50000000000006);
#5037=CYLINDRICAL_SURFACE('',#74901,7.49999999999887);
#5038=CYLINDRICAL_SURFACE('',#74906,7.49999999999948);
#5039=CYLINDRICAL_SURFACE('',#74911,7.5000000000009);
#5040=CYLINDRICAL_SURFACE('',#74916,7.49999999999928);
#5041=CYLINDRICAL_SURFACE('',#74921,7.50000000000024);
#5042=CYLINDRICAL_SURFACE('',#74926,7.50000000000052);
#5043=CYLINDRICAL_SURFACE('',#74931,7.49999999999965);
#5044=CYLINDRICAL_SURFACE('',#74936,7.50000000000169);
#5045=CYLINDRICAL_SURFACE('',#74941,7.50000000000101);
#5046=CYLINDRICAL_SURFACE('',#74946,7.49999999999905);
#5047=CYLINDRICAL_SURFACE('',#74951,7.49999999999969);
#5048=CYLINDRICAL_SURFACE('',#74956,7.50000000000003);
#5049=CYLINDRICAL_SURFACE('',#74961,7.49999999999982);
#5050=CYLINDRICAL_SURFACE('',#74966,7.4999999999998);
#5051=CYLINDRICAL_SURFACE('',#74971,7.50000000000035);
#5052=CYLINDRICAL_SURFACE('',#74976,7.4999999999998);
#5053=CYLINDRICAL_SURFACE('',#75038,7.50000000000103);
#5054=CYLINDRICAL_SURFACE('',#75042,7.49999999999921);
#5055=CYLINDRICAL_SURFACE('',#75046,7.50000000000047);
#5056=CYLINDRICAL_SURFACE('',#75050,7.49999999999861);
#5057=CYLINDRICAL_SURFACE('',#75054,7.49999999999951);
#5058=CYLINDRICAL_SURFACE('',#75058,7.4999999999994);
#5059=CYLINDRICAL_SURFACE('',#75062,7.49999999999855);
#5060=CYLINDRICAL_SURFACE('',#75066,7.50000000000025);
#5061=CYLINDRICAL_SURFACE('',#75070,7.50000000000009);
#5062=CYLINDRICAL_SURFACE('',#75074,7.49999999999832);
#5063=CYLINDRICAL_SURFACE('',#75078,7.49999999999923);
#5064=CYLINDRICAL_SURFACE('',#75082,7.49999999999844);
#5065=CYLINDRICAL_SURFACE('',#75086,7.49999999999893);
#5066=CYLINDRICAL_SURFACE('',#75090,7.50000000000281);
#5067=CYLINDRICAL_SURFACE('',#75094,7.50000000000082);
#5068=CYLINDRICAL_SURFACE('',#75098,7.5);
#5069=CYLINDRICAL_SURFACE('',#75102,7.50000000000082);
#5070=CYLINDRICAL_SURFACE('',#75106,7.50000000000095);
#5071=CYLINDRICAL_SURFACE('',#75111,7.50000000000097);
#5072=CYLINDRICAL_SURFACE('',#75114,7.50000000000035);
#5073=CYLINDRICAL_SURFACE('',#75118,7.49999999999909);
#5074=CYLINDRICAL_SURFACE('',#75122,7.5000000000005);
#5075=CYLINDRICAL_SURFACE('',#75126,7.49999999999976);
#5076=CYLINDRICAL_SURFACE('',#75130,7.49999999999953);
#5077=CYLINDRICAL_SURFACE('',#75134,7.49999999999916);
#5078=CYLINDRICAL_SURFACE('',#75138,7.5000000000001);
#5079=CYLINDRICAL_SURFACE('',#75142,7.50000000000193);
#5080=CYLINDRICAL_SURFACE('',#75146,7.49999999999949);
#5081=CYLINDRICAL_SURFACE('',#75151,7.4999999999997);
#5082=CYLINDRICAL_SURFACE('',#75155,7.49999999999984);
#5083=CYLINDRICAL_SURFACE('',#75159,7.50000000000064);
#5084=CYLINDRICAL_SURFACE('',#75163,7.49999999999956);
#5085=CYLINDRICAL_SURFACE('',#75167,7.50000000000121);
#5086=CYLINDRICAL_SURFACE('',#75171,7.49999999999886);
#5087=CYLINDRICAL_SURFACE('',#75175,7.49999999999906);
#5088=CYLINDRICAL_SURFACE('',#75179,7.49999999999926);
#5089=CYLINDRICAL_SURFACE('',#75183,7.49999999999995);
#5090=CYLINDRICAL_SURFACE('',#75187,7.49999999999959);
#5091=CYLINDRICAL_SURFACE('',#75191,7.49999999999962);
#5092=CYLINDRICAL_SURFACE('',#75195,7.50000000000058);
#5093=CYLINDRICAL_SURFACE('',#75199,7.49999999999953);
#5094=CYLINDRICAL_SURFACE('',#75203,7.49999999999982);
#5095=CYLINDRICAL_SURFACE('',#75207,7.49999999999959);
#5096=CYLINDRICAL_SURFACE('',#75211,7.50000000000001);
#5097=CYLINDRICAL_SURFACE('',#75215,7.49999999999972);
#5098=CYLINDRICAL_SURFACE('',#75219,7.50000000000012);
#5099=CYLINDRICAL_SURFACE('',#75223,7.49999999999998);
#5100=CYLINDRICAL_SURFACE('',#75227,7.49999999999767);
#5101=CYLINDRICAL_SURFACE('',#75231,7.50000000000083);
#5102=CYLINDRICAL_SURFACE('',#75235,7.49999999999857);
#5103=CYLINDRICAL_SURFACE('',#75239,7.50000000000065);
#5104=CYLINDRICAL_SURFACE('',#75243,7.49999999999904);
#5105=CYLINDRICAL_SURFACE('',#75247,7.50000000000149);
#5106=CYLINDRICAL_SURFACE('',#75251,7.49999999999998);
#5107=CYLINDRICAL_SURFACE('',#75255,7.50000000000078);
#5108=CYLINDRICAL_SURFACE('',#75258,7.49999999999895);
#5109=CYLINDRICAL_SURFACE('',#75378,7.50000000000086);
#5110=CYLINDRICAL_SURFACE('',#75383,7.50000000000024);
#5111=CYLINDRICAL_SURFACE('',#75388,7.49999999999883);
#5112=CYLINDRICAL_SURFACE('',#75393,7.50000000000074);
#5113=CYLINDRICAL_SURFACE('',#75398,7.49999999999952);
#5114=CYLINDRICAL_SURFACE('',#75403,7.49999999999914);
#5115=CYLINDRICAL_SURFACE('',#75408,7.49999999999965);
#5116=CYLINDRICAL_SURFACE('',#75413,7.50000000000115);
#5117=CYLINDRICAL_SURFACE('',#75418,7.49999999999992);
#5118=CYLINDRICAL_SURFACE('',#75423,7.49999999999906);
#5119=CYLINDRICAL_SURFACE('',#75428,7.50000000000055);
#5120=CYLINDRICAL_SURFACE('',#75433,7.50000000000195);
#5121=CYLINDRICAL_SURFACE('',#75438,7.49999999999956);
#5122=CYLINDRICAL_SURFACE('',#75443,7.49999999999863);
#5123=CYLINDRICAL_SURFACE('',#75448,7.49999999999977);
#5124=CYLINDRICAL_SURFACE('',#75453,7.5000000000016);
#5125=CYLINDRICAL_SURFACE('',#75458,7.50000000000047);
#5126=CYLINDRICAL_SURFACE('',#75463,7.50000000000125);
#5127=CYLINDRICAL_SURFACE('',#75469,7.50000000000031);
#5128=CYLINDRICAL_SURFACE('',#75473,7.50000000000031);
#5129=CYLINDRICAL_SURFACE('',#75478,7.49999999999752);
#5130=CYLINDRICAL_SURFACE('',#75483,7.49999999999966);
#5131=CYLINDRICAL_SURFACE('',#75488,7.50000000000105);
#5132=CYLINDRICAL_SURFACE('',#75493,7.50000000000112);
#5133=CYLINDRICAL_SURFACE('',#75498,7.5000000000005);
#5134=CYLINDRICAL_SURFACE('',#75503,7.49999999999953);
#5135=CYLINDRICAL_SURFACE('',#75508,7.50000000000087);
#5136=CYLINDRICAL_SURFACE('',#75513,7.49999999999993);
#5137=CYLINDRICAL_SURFACE('',#75519,7.5000000000018);
#5138=CYLINDRICAL_SURFACE('',#75524,7.50000000000045);
#5139=CYLINDRICAL_SURFACE('',#75529,7.49999999999987);
#5140=CYLINDRICAL_SURFACE('',#75534,7.5000000000015);
#5141=CYLINDRICAL_SURFACE('',#75539,7.50000000000095);
#5142=CYLINDRICAL_SURFACE('',#75544,7.50000000000098);
#5143=CYLINDRICAL_SURFACE('',#75549,7.50000000000068);
#5144=CYLINDRICAL_SURFACE('',#75554,7.49999999999984);
#5145=CYLINDRICAL_SURFACE('',#75559,7.50000000000035);
#5146=CYLINDRICAL_SURFACE('',#75564,7.49999999999952);
#5147=CYLINDRICAL_SURFACE('',#75569,7.50000000000135);
#5148=CYLINDRICAL_SURFACE('',#75574,7.49999999999964);
#5149=CYLINDRICAL_SURFACE('',#75579,7.50000000000069);
#5150=CYLINDRICAL_SURFACE('',#75584,7.50000000000112);
#5151=CYLINDRICAL_SURFACE('',#75589,7.50000000000045);
#5152=CYLINDRICAL_SURFACE('',#75594,7.500000000003);
#5153=CYLINDRICAL_SURFACE('',#75599,7.50000000000051);
#5154=CYLINDRICAL_SURFACE('',#75604,7.50000000000022);
#5155=CYLINDRICAL_SURFACE('',#75609,7.49999999999907);
#5156=CYLINDRICAL_SURFACE('',#75614,7.49999999999984);
#5157=CYLINDRICAL_SURFACE('',#75619,7.50000000000031);
#5158=CYLINDRICAL_SURFACE('',#75624,7.50000000000036);
#5159=CYLINDRICAL_SURFACE('',#75629,7.49999999999868);
#5160=CYLINDRICAL_SURFACE('',#75634,7.49999999999904);
#5161=CYLINDRICAL_SURFACE('',#75639,7.49999999999943);
#5162=CYLINDRICAL_SURFACE('',#75644,7.49999999999986);
#5163=CYLINDRICAL_SURFACE('',#75649,7.50000000000246);
#5164=CYLINDRICAL_SURFACE('',#75654,7.50000000000062);
#5165=CYLINDRICAL_SURFACE('',#75775,7.49999999999993);
#5166=CYLINDRICAL_SURFACE('',#75780,7.50000000000008);
#5167=CYLINDRICAL_SURFACE('',#75785,7.50000000000149);
#5168=CYLINDRICAL_SURFACE('',#75790,7.50000000000108);
#5169=CYLINDRICAL_SURFACE('',#75795,7.50000000000101);
#5170=CYLINDRICAL_SURFACE('',#75800,7.49999999999874);
#5171=CYLINDRICAL_SURFACE('',#75805,7.50000000000018);
#5172=CYLINDRICAL_SURFACE('',#75810,7.50000000000006);
#5173=CYLINDRICAL_SURFACE('',#75815,7.5000000000002);
#5174=CYLINDRICAL_SURFACE('',#75820,7.50000000000027);
#5175=CYLINDRICAL_SURFACE('',#75825,7.50000000000002);
#5176=CYLINDRICAL_SURFACE('',#75830,7.49999999999989);
#5177=CYLINDRICAL_SURFACE('',#75835,7.50000000000097);
#5178=CYLINDRICAL_SURFACE('',#75840,7.50000000000115);
#5179=CYLINDRICAL_SURFACE('',#75845,7.50000000000046);
#5180=CYLINDRICAL_SURFACE('',#75850,7.49999999999974);
#5181=CYLINDRICAL_SURFACE('',#75855,7.50000000000165);
#5182=CYLINDRICAL_SURFACE('',#75861,7.50000000000142);
#5183=CYLINDRICAL_SURFACE('',#75865,7.50000000000104);
#5184=CYLINDRICAL_SURFACE('',#75870,7.49999999999953);
#5185=CYLINDRICAL_SURFACE('',#75875,7.50000000000099);
#5186=CYLINDRICAL_SURFACE('',#75880,7.50000000000091);
#5187=CYLINDRICAL_SURFACE('',#75885,7.49999999999943);
#5188=CYLINDRICAL_SURFACE('',#75890,7.50000000000072);
#5189=CYLINDRICAL_SURFACE('',#75895,7.49999999999811);
#5190=CYLINDRICAL_SURFACE('',#75900,7.50000000000036);
#5191=CYLINDRICAL_SURFACE('',#75905,7.49999999999855);
#5192=CYLINDRICAL_SURFACE('',#75909,7.49999999999989);
#5193=CYLINDRICAL_SURFACE('',#75916,7.49999999999854);
#5194=CYLINDRICAL_SURFACE('',#75921,7.4999999999983);
#5195=CYLINDRICAL_SURFACE('',#75926,7.49999999999806);
#5196=CYLINDRICAL_SURFACE('',#75931,7.49999999999984);
#5197=CYLINDRICAL_SURFACE('',#75936,7.49999999999986);
#5198=CYLINDRICAL_SURFACE('',#75941,7.50000000000069);
#5199=CYLINDRICAL_SURFACE('',#75946,7.49999999999977);
#5200=CYLINDRICAL_SURFACE('',#75951,7.49999999999974);
#5201=CYLINDRICAL_SURFACE('',#75956,7.49999999999927);
#5202=CYLINDRICAL_SURFACE('',#75961,7.50000000000063);
#5203=CYLINDRICAL_SURFACE('',#75966,7.4999999999996);
#5204=CYLINDRICAL_SURFACE('',#75971,7.49999999999951);
#5205=CYLINDRICAL_SURFACE('',#75976,7.50000000000091);
#5206=CYLINDRICAL_SURFACE('',#75981,7.49999999999948);
#5207=CYLINDRICAL_SURFACE('',#75986,7.49999999999928);
#5208=CYLINDRICAL_SURFACE('',#75991,7.49999999999904);
#5209=CYLINDRICAL_SURFACE('',#75996,7.49999999999936);
#5210=CYLINDRICAL_SURFACE('',#76001,7.50000000000108);
#5211=CYLINDRICAL_SURFACE('',#76006,7.5000000000006);
#5212=CYLINDRICAL_SURFACE('',#76011,7.50000000000072);
#5213=CYLINDRICAL_SURFACE('',#76016,7.49999999999886);
#5214=CYLINDRICAL_SURFACE('',#76021,7.49999999999831);
#5215=CYLINDRICAL_SURFACE('',#76026,7.50000000000101);
#5216=CYLINDRICAL_SURFACE('',#76031,7.49999999999924);
#5217=CYLINDRICAL_SURFACE('',#76036,7.49999999999796);
#5218=CYLINDRICAL_SURFACE('',#76041,7.49999999999881);
#5219=CYLINDRICAL_SURFACE('',#76046,7.49999999999965);
#5220=CYLINDRICAL_SURFACE('',#76049,7.50000000000054);
#5221=CYLINDRICAL_SURFACE('',#76141,7.49999999999829);
#5222=CYLINDRICAL_SURFACE('',#76145,7.50000000000136);
#5223=CYLINDRICAL_SURFACE('',#76149,7.50000000000038);
#5224=CYLINDRICAL_SURFACE('',#76153,7.50000000000154);
#5225=CYLINDRICAL_SURFACE('',#76157,7.50000000000029);
#5226=CYLINDRICAL_SURFACE('',#76161,7.49999999999914);
#5227=CYLINDRICAL_SURFACE('',#76165,7.49999999999986);
#5228=CYLINDRICAL_SURFACE('',#76169,7.5000000000006);
#5229=CYLINDRICAL_SURFACE('',#76173,7.50000000000089);
#5230=CYLINDRICAL_SURFACE('',#76177,7.50000000000173);
#5231=CYLINDRICAL_SURFACE('',#76181,7.49999999999671);
#5232=CYLINDRICAL_SURFACE('',#76185,7.50000000000107);
#5233=CYLINDRICAL_SURFACE('',#76189,7.50000000000124);
#5234=CYLINDRICAL_SURFACE('',#76193,7.4999999999985);
#5235=CYLINDRICAL_SURFACE('',#76197,7.49999999999936);
#5236=CYLINDRICAL_SURFACE('',#76201,7.50000000000132);
#5237=CYLINDRICAL_SURFACE('',#76205,7.50000000000063);
#5238=CYLINDRICAL_SURFACE('',#76209,7.49999999999944);
#5239=CYLINDRICAL_SURFACE('',#76213,7.50000000000154);
#5240=CYLINDRICAL_SURFACE('',#76217,7.49999999999982);
#5241=CYLINDRICAL_SURFACE('',#76221,7.49999999999879);
#5242=CYLINDRICAL_SURFACE('',#76225,7.49999999999893);
#5243=CYLINDRICAL_SURFACE('',#76229,7.49999999999837);
#5244=CYLINDRICAL_SURFACE('',#76233,7.49999999999956);
#5245=CYLINDRICAL_SURFACE('',#76237,7.50000000000076);
#5246=CYLINDRICAL_SURFACE('',#76241,7.49999999999921);
#5247=CYLINDRICAL_SURFACE('',#76245,7.49999999999933);
#5248=CYLINDRICAL_SURFACE('',#76249,7.5000000000015);
#5249=CYLINDRICAL_SURFACE('',#76258,7.50000000000068);
#5250=CYLINDRICAL_SURFACE('',#76267,7.49999999999906);
#5251=CYLINDRICAL_SURFACE('',#76276,7.50000000000119);
#5252=CYLINDRICAL_SURFACE('',#76285,7.50000000000095);
#5253=CYLINDRICAL_SURFACE('',#76294,7.49999999999979);
#5254=CYLINDRICAL_SURFACE('',#76303,7.49999999999866);
#5255=CYLINDRICAL_SURFACE('',#76312,7.50000000000089);
#5256=CYLINDRICAL_SURFACE('',#76321,7.50000000000142);
#5257=CYLINDRICAL_SURFACE('',#76330,7.49999999999948);
#5258=CYLINDRICAL_SURFACE('',#76339,7.49999999999996);
#5259=CYLINDRICAL_SURFACE('',#76348,7.49999999999837);
#5260=CYLINDRICAL_SURFACE('',#76357,7.50000000000016);
#5261=CYLINDRICAL_SURFACE('',#76366,7.5000000000002);
#5262=CYLINDRICAL_SURFACE('',#76375,7.49999999999976);
#5263=CYLINDRICAL_SURFACE('',#76384,7.50000000000073);
#5264=CYLINDRICAL_SURFACE('',#76393,7.50000000000145);
#5265=CYLINDRICAL_SURFACE('',#76402,7.50000000000033);
#5266=CYLINDRICAL_SURFACE('',#76411,7.50000000000189);
#5267=CYLINDRICAL_SURFACE('',#76420,7.50000000000128);
#5268=CYLINDRICAL_SURFACE('',#76429,7.49999999999988);
#5269=CYLINDRICAL_SURFACE('',#76438,7.50000000000037);
#5270=CYLINDRICAL_SURFACE('',#76447,7.49999999999926);
#5271=CYLINDRICAL_SURFACE('',#76456,7.50000000000009);
#5272=CYLINDRICAL_SURFACE('',#76465,7.49999999999888);
#5273=CYLINDRICAL_SURFACE('',#76474,7.5000000000001);
#5274=CYLINDRICAL_SURFACE('',#76483,7.49999999999936);
#5275=CYLINDRICAL_SURFACE('',#76492,7.49999999999966);
#5276=CYLINDRICAL_SURFACE('',#76501,7.49999999999988);
#5277=CYLINDRICAL_SURFACE('',#76651,7.50000000000019);
#5278=CYLINDRICAL_SURFACE('',#76656,7.50000000000089);
#5279=CYLINDRICAL_SURFACE('',#76661,7.500000000001);
#5280=CYLINDRICAL_SURFACE('',#76666,7.50000000000125);
#5281=CYLINDRICAL_SURFACE('',#76671,7.50000000000063);
#5282=CYLINDRICAL_SURFACE('',#76676,7.49999999999918);
#5283=CYLINDRICAL_SURFACE('',#76681,7.50000000000149);
#5284=CYLINDRICAL_SURFACE('',#76686,7.50000000000101);
#5285=CYLINDRICAL_SURFACE('',#76691,7.49999999999985);
#5286=CYLINDRICAL_SURFACE('',#76696,7.50000000000006);
#5287=CYLINDRICAL_SURFACE('',#76701,7.50000000000201);
#5288=CYLINDRICAL_SURFACE('',#76706,7.5000000000003);
#5289=CYLINDRICAL_SURFACE('',#76711,7.50000000000073);
#5290=CYLINDRICAL_SURFACE('',#76716,7.49999999999934);
#5291=CYLINDRICAL_SURFACE('',#76721,7.49999999999874);
#5292=CYLINDRICAL_SURFACE('',#76726,7.50000000000064);
#5293=CYLINDRICAL_SURFACE('',#76732,7.49999999999973);
#5294=CYLINDRICAL_SURFACE('',#76736,7.49999999999924);
#5295=CYLINDRICAL_SURFACE('',#76741,7.50000000000012);
#5296=CYLINDRICAL_SURFACE('',#76746,7.499999999999);
#5297=CYLINDRICAL_SURFACE('',#76751,7.49999999999987);
#5298=CYLINDRICAL_SURFACE('',#76756,7.50000000000125);
#5299=CYLINDRICAL_SURFACE('',#76761,7.50000000000055);
#5300=CYLINDRICAL_SURFACE('',#76766,7.50000000000049);
#5301=CYLINDRICAL_SURFACE('',#76771,7.49999999999952);
#5302=CYLINDRICAL_SURFACE('',#76776,7.50000000000184);
#5303=CYLINDRICAL_SURFACE('',#76781,7.49999999999831);
#5304=CYLINDRICAL_SURFACE('',#76785,7.50000000000028);
#5305=CYLINDRICAL_SURFACE('',#76933,7.50000000000006);
#5306=CYLINDRICAL_SURFACE('',#76938,7.50000000000193);
#5307=CYLINDRICAL_SURFACE('',#76943,7.50000000000066);
#5308=CYLINDRICAL_SURFACE('',#76948,7.50000000000187);
#5309=CYLINDRICAL_SURFACE('',#76953,7.49999999999954);
#5310=CYLINDRICAL_SURFACE('',#76958,7.49999999999832);
#5311=CYLINDRICAL_SURFACE('',#76963,7.49999999999972);
#5312=CYLINDRICAL_SURFACE('',#76968,7.50000000000133);
#5313=CYLINDRICAL_SURFACE('',#76973,7.50000000000065);
#5314=CYLINDRICAL_SURFACE('',#76978,7.50000000000155);
#5315=CYLINDRICAL_SURFACE('',#76983,7.50000000000083);
#5316=CYLINDRICAL_SURFACE('',#76988,7.50000000000002);
#5317=CYLINDRICAL_SURFACE('',#76993,7.49999999999901);
#5318=CYLINDRICAL_SURFACE('',#76998,7.50000000000075);
#5319=CYLINDRICAL_SURFACE('',#77003,7.50000000000107);
#5320=CYLINDRICAL_SURFACE('',#77008,7.49999999999885);
#5321=CYLINDRICAL_SURFACE('',#77014,7.50000000000039);
#5322=CYLINDRICAL_SURFACE('',#77018,7.49999999999898);
#5323=CYLINDRICAL_SURFACE('',#77023,7.49999999999877);
#5324=CYLINDRICAL_SURFACE('',#77028,7.49999999999893);
#5325=CYLINDRICAL_SURFACE('',#77033,7.4999999999999);
#5326=CYLINDRICAL_SURFACE('',#77038,7.49999999999949);
#5327=CYLINDRICAL_SURFACE('',#77043,7.49999999999888);
#5328=CYLINDRICAL_SURFACE('',#77048,7.50000000000012);
#5329=CYLINDRICAL_SURFACE('',#77053,7.49999999999965);
#5330=CYLINDRICAL_SURFACE('',#77058,7.50000000000049);
#5331=CYLINDRICAL_SURFACE('',#77063,7.49999999999969);
#5332=CYLINDRICAL_SURFACE('',#77068,7.50000000000174);
#5333=CYLINDRICAL_SURFACE('',#77166,7.50000000000002);
#5334=CYLINDRICAL_SURFACE('',#77175,7.50000000000086);
#5335=CYLINDRICAL_SURFACE('',#77184,7.49999999999894);
#5336=CYLINDRICAL_SURFACE('',#77193,7.49999999999968);
#5337=CYLINDRICAL_SURFACE('',#77202,7.49999999999949);
#5338=CYLINDRICAL_SURFACE('',#77211,7.50000000000058);
#5339=CYLINDRICAL_SURFACE('',#77223,7.49999999999883);
#5340=CYLINDRICAL_SURFACE('',#77232,7.50000000000146);
#5341=CYLINDRICAL_SURFACE('',#77241,7.49999999999999);
#5342=CYLINDRICAL_SURFACE('',#77250,7.50000000000032);
#5343=CYLINDRICAL_SURFACE('',#77259,7.49999999999892);
#5344=CYLINDRICAL_SURFACE('',#77268,7.50000000000196);
#5345=CYLINDRICAL_SURFACE('',#77277,7.50000000000019);
#5346=CYLINDRICAL_SURFACE('',#77286,7.50000000000041);
#5347=CYLINDRICAL_SURFACE('',#77295,7.50000000000071);
#5348=CYLINDRICAL_SURFACE('',#77304,7.49999999999975);
#5349=CYLINDRICAL_SURFACE('',#77313,7.49999999999947);
#5350=CYLINDRICAL_SURFACE('',#77322,7.5);
#5351=CYLINDRICAL_SURFACE('',#77331,7.49999999999963);
#5352=CYLINDRICAL_SURFACE('',#77340,7.49999999999951);
#5353=CYLINDRICAL_SURFACE('',#77349,7.50000000000136);
#5354=CYLINDRICAL_SURFACE('',#77358,7.49999999999879);
#5355=CYLINDRICAL_SURFACE('',#77367,7.50000000000127);
#5356=CYLINDRICAL_SURFACE('',#77376,7.50000000000044);
#5357=CYLINDRICAL_SURFACE('',#77385,7.49999999999987);
#5358=CYLINDRICAL_SURFACE('',#77394,7.50000000000078);
#5359=CYLINDRICAL_SURFACE('',#77403,7.50000000000087);
#5360=CYLINDRICAL_SURFACE('',#77410,7.50000000000169);
#5383=FACE_OUTER_BOUND('',#10648,.T.);
#5384=FACE_OUTER_BOUND('',#10649,.T.);
#5385=FACE_OUTER_BOUND('',#10650,.T.);
#5386=FACE_OUTER_BOUND('',#10651,.T.);
#5387=FACE_OUTER_BOUND('',#10652,.T.);
#5388=FACE_OUTER_BOUND('',#10653,.T.);
#5389=FACE_OUTER_BOUND('',#10654,.T.);
#5390=FACE_OUTER_BOUND('',#10655,.T.);
#5391=FACE_OUTER_BOUND('',#10656,.T.);
#5392=FACE_OUTER_BOUND('',#10657,.T.);
#5393=FACE_OUTER_BOUND('',#10658,.T.);
#5394=FACE_OUTER_BOUND('',#10659,.T.);
#5395=FACE_OUTER_BOUND('',#10660,.T.);
#5396=FACE_OUTER_BOUND('',#10661,.T.);
#5397=FACE_OUTER_BOUND('',#10662,.T.);
#5398=FACE_OUTER_BOUND('',#10663,.T.);
#5399=FACE_OUTER_BOUND('',#10664,.T.);
#5400=FACE_OUTER_BOUND('',#10665,.T.);
#5401=FACE_OUTER_BOUND('',#10666,.T.);
#5402=FACE_OUTER_BOUND('',#10667,.T.);
#5403=FACE_OUTER_BOUND('',#10668,.T.);
#5404=FACE_OUTER_BOUND('',#10669,.T.);
#5405=FACE_OUTER_BOUND('',#10670,.T.);
#5406=FACE_OUTER_BOUND('',#10671,.T.);
#5407=FACE_OUTER_BOUND('',#10672,.T.);
#5408=FACE_OUTER_BOUND('',#10673,.T.);
#5409=FACE_OUTER_BOUND('',#10674,.T.);
#5410=FACE_OUTER_BOUND('',#10675,.T.);
#5411=FACE_OUTER_BOUND('',#10676,.T.);
#5412=FACE_OUTER_BOUND('',#10677,.T.);
#5413=FACE_OUTER_BOUND('',#10678,.T.);
#5414=FACE_OUTER_BOUND('',#10679,.T.);
#5415=FACE_OUTER_BOUND('',#10680,.T.);
#5416=FACE_OUTER_BOUND('',#10681,.T.);
#5417=FACE_OUTER_BOUND('',#10682,.T.);
#5418=FACE_OUTER_BOUND('',#10683,.T.);
#5419=FACE_OUTER_BOUND('',#10684,.T.);
#5420=FACE_OUTER_BOUND('',#10685,.T.);
#5421=FACE_OUTER_BOUND('',#10686,.T.);
#5422=FACE_OUTER_BOUND('',#10687,.T.);
#5423=FACE_OUTER_BOUND('',#10688,.T.);
#5424=FACE_OUTER_BOUND('',#10689,.T.);
#5425=FACE_OUTER_BOUND('',#10690,.T.);
#5426=FACE_OUTER_BOUND('',#10691,.T.);
#5427=FACE_OUTER_BOUND('',#10692,.T.);
#5428=FACE_OUTER_BOUND('',#10693,.T.);
#5429=FACE_OUTER_BOUND('',#10694,.T.);
#5430=FACE_OUTER_BOUND('',#10695,.T.);
#5431=FACE_OUTER_BOUND('',#10696,.T.);
#5432=FACE_OUTER_BOUND('',#10697,.T.);
#5433=FACE_OUTER_BOUND('',#10698,.T.);
#5434=FACE_OUTER_BOUND('',#10699,.T.);
#5435=FACE_OUTER_BOUND('',#10700,.T.);
#5436=FACE_OUTER_BOUND('',#10701,.T.);
#5437=FACE_OUTER_BOUND('',#10702,.T.);
#5438=FACE_OUTER_BOUND('',#10703,.T.);
#5439=FACE_OUTER_BOUND('',#10704,.T.);
#5440=FACE_OUTER_BOUND('',#10705,.T.);
#5441=FACE_OUTER_BOUND('',#10706,.T.);
#5442=FACE_OUTER_BOUND('',#10707,.T.);
#5443=FACE_OUTER_BOUND('',#10708,.T.);
#5444=FACE_OUTER_BOUND('',#10709,.T.);
#5445=FACE_OUTER_BOUND('',#10710,.T.);
#5446=FACE_OUTER_BOUND('',#10711,.T.);
#5447=FACE_OUTER_BOUND('',#10712,.T.);
#5448=FACE_OUTER_BOUND('',#10713,.T.);
#5449=FACE_OUTER_BOUND('',#10714,.T.);
#5450=FACE_OUTER_BOUND('',#10715,.T.);
#5451=FACE_OUTER_BOUND('',#10716,.T.);
#5452=FACE_OUTER_BOUND('',#10717,.T.);
#5453=FACE_OUTER_BOUND('',#10718,.T.);
#5454=FACE_OUTER_BOUND('',#10719,.T.);
#5455=FACE_OUTER_BOUND('',#10720,.T.);
#5456=FACE_OUTER_BOUND('',#10721,.T.);
#5457=FACE_OUTER_BOUND('',#10722,.T.);
#5458=FACE_OUTER_BOUND('',#10723,.T.);
#5459=FACE_OUTER_BOUND('',#10724,.T.);
#5460=FACE_OUTER_BOUND('',#10725,.T.);
#5461=FACE_OUTER_BOUND('',#10726,.T.);
#5462=FACE_OUTER_BOUND('',#10727,.T.);
#5463=FACE_OUTER_BOUND('',#10728,.T.);
#5464=FACE_OUTER_BOUND('',#10729,.T.);
#5465=FACE_OUTER_BOUND('',#10730,.T.);
#5466=FACE_OUTER_BOUND('',#10731,.T.);
#5467=FACE_OUTER_BOUND('',#10732,.T.);
#5468=FACE_OUTER_BOUND('',#10733,.T.);
#5469=FACE_OUTER_BOUND('',#10734,.T.);
#5470=FACE_OUTER_BOUND('',#10735,.T.);
#5471=FACE_OUTER_BOUND('',#10736,.T.);
#5472=FACE_OUTER_BOUND('',#10737,.T.);
#5473=FACE_OUTER_BOUND('',#10738,.T.);
#5474=FACE_OUTER_BOUND('',#10739,.T.);
#5475=FACE_OUTER_BOUND('',#10740,.T.);
#5476=FACE_OUTER_BOUND('',#10741,.T.);
#5477=FACE_OUTER_BOUND('',#10742,.T.);
#5478=FACE_OUTER_BOUND('',#10743,.T.);
#5479=FACE_OUTER_BOUND('',#10744,.T.);
#5480=FACE_OUTER_BOUND('',#10745,.T.);
#5481=FACE_OUTER_BOUND('',#10746,.T.);
#5482=FACE_OUTER_BOUND('',#10747,.T.);
#5483=FACE_OUTER_BOUND('',#10748,.T.);
#5484=FACE_OUTER_BOUND('',#10749,.T.);
#5485=FACE_OUTER_BOUND('',#10750,.T.);
#5486=FACE_OUTER_BOUND('',#10751,.T.);
#5487=FACE_OUTER_BOUND('',#10752,.T.);
#5488=FACE_OUTER_BOUND('',#10753,.T.);
#5489=FACE_OUTER_BOUND('',#10754,.T.);
#5490=FACE_OUTER_BOUND('',#10755,.T.);
#5491=FACE_OUTER_BOUND('',#10756,.T.);
#5492=FACE_OUTER_BOUND('',#10757,.T.);
#5493=FACE_OUTER_BOUND('',#10758,.T.);
#5494=FACE_OUTER_BOUND('',#10759,.T.);
#5495=FACE_OUTER_BOUND('',#10760,.T.);
#5496=FACE_OUTER_BOUND('',#10761,.T.);
#5497=FACE_OUTER_BOUND('',#10762,.T.);
#5498=FACE_OUTER_BOUND('',#10763,.T.);
#5499=FACE_OUTER_BOUND('',#10764,.T.);
#5500=FACE_OUTER_BOUND('',#10765,.T.);
#5501=FACE_OUTER_BOUND('',#10766,.T.);
#5502=FACE_OUTER_BOUND('',#10767,.T.);
#5503=FACE_OUTER_BOUND('',#10768,.T.);
#5504=FACE_OUTER_BOUND('',#10769,.T.);
#5505=FACE_OUTER_BOUND('',#10770,.T.);
#5506=FACE_OUTER_BOUND('',#10771,.T.);
#5507=FACE_OUTER_BOUND('',#10772,.T.);
#5508=FACE_OUTER_BOUND('',#10773,.T.);
#5509=FACE_OUTER_BOUND('',#10774,.T.);
#5510=FACE_OUTER_BOUND('',#10775,.T.);
#5511=FACE_OUTER_BOUND('',#10776,.T.);
#5512=FACE_OUTER_BOUND('',#10777,.T.);
#5513=FACE_OUTER_BOUND('',#10778,.T.);
#5514=FACE_OUTER_BOUND('',#10779,.T.);
#5515=FACE_OUTER_BOUND('',#10780,.T.);
#5516=FACE_OUTER_BOUND('',#10781,.T.);
#5517=FACE_OUTER_BOUND('',#10782,.T.);
#5518=FACE_OUTER_BOUND('',#10783,.T.);
#5519=FACE_OUTER_BOUND('',#10784,.T.);
#5520=FACE_OUTER_BOUND('',#10785,.T.);
#5521=FACE_OUTER_BOUND('',#10786,.T.);
#5522=FACE_OUTER_BOUND('',#10787,.T.);
#5523=FACE_OUTER_BOUND('',#10788,.T.);
#5524=FACE_OUTER_BOUND('',#10789,.T.);
#5525=FACE_OUTER_BOUND('',#10790,.T.);
#5526=FACE_OUTER_BOUND('',#10791,.T.);
#5527=FACE_OUTER_BOUND('',#10792,.T.);
#5528=FACE_OUTER_BOUND('',#10793,.T.);
#5529=FACE_OUTER_BOUND('',#10794,.T.);
#5530=FACE_OUTER_BOUND('',#10795,.T.);
#5531=FACE_OUTER_BOUND('',#10796,.T.);
#5532=FACE_OUTER_BOUND('',#10797,.T.);
#5533=FACE_OUTER_BOUND('',#10798,.T.);
#5534=FACE_OUTER_BOUND('',#10799,.T.);
#5535=FACE_OUTER_BOUND('',#10800,.T.);
#5536=FACE_OUTER_BOUND('',#10801,.T.);
#5537=FACE_OUTER_BOUND('',#10802,.T.);
#5538=FACE_OUTER_BOUND('',#10803,.T.);
#5539=FACE_OUTER_BOUND('',#10804,.T.);
#5540=FACE_OUTER_BOUND('',#10805,.T.);
#5541=FACE_OUTER_BOUND('',#10806,.T.);
#5542=FACE_OUTER_BOUND('',#10807,.T.);
#5543=FACE_OUTER_BOUND('',#10808,.T.);
#5544=FACE_OUTER_BOUND('',#10809,.T.);
#5545=FACE_OUTER_BOUND('',#10810,.T.);
#5546=FACE_OUTER_BOUND('',#10811,.T.);
#5547=FACE_OUTER_BOUND('',#10812,.T.);
#5548=FACE_OUTER_BOUND('',#10813,.T.);
#5549=FACE_OUTER_BOUND('',#10814,.T.);
#5550=FACE_OUTER_BOUND('',#10815,.T.);
#5551=FACE_OUTER_BOUND('',#10816,.T.);
#5552=FACE_OUTER_BOUND('',#10817,.T.);
#5553=FACE_OUTER_BOUND('',#10818,.T.);
#5554=FACE_OUTER_BOUND('',#10819,.T.);
#5555=FACE_OUTER_BOUND('',#10820,.T.);
#5556=FACE_OUTER_BOUND('',#10821,.T.);
#5557=FACE_OUTER_BOUND('',#10822,.T.);
#5558=FACE_OUTER_BOUND('',#10823,.T.);
#5559=FACE_OUTER_BOUND('',#10824,.T.);
#5560=FACE_OUTER_BOUND('',#10825,.T.);
#5561=FACE_OUTER_BOUND('',#10826,.T.);
#5562=FACE_OUTER_BOUND('',#10827,.T.);
#5563=FACE_OUTER_BOUND('',#10828,.T.);
#5564=FACE_OUTER_BOUND('',#10829,.T.);
#5565=FACE_OUTER_BOUND('',#10830,.T.);
#5566=FACE_OUTER_BOUND('',#10831,.T.);
#5567=FACE_OUTER_BOUND('',#10832,.T.);
#5568=FACE_OUTER_BOUND('',#10833,.T.);
#5569=FACE_OUTER_BOUND('',#10834,.T.);
#5570=FACE_OUTER_BOUND('',#10835,.T.);
#5571=FACE_OUTER_BOUND('',#10836,.T.);
#5572=FACE_OUTER_BOUND('',#10837,.T.);
#5573=FACE_OUTER_BOUND('',#10838,.T.);
#5574=FACE_OUTER_BOUND('',#10839,.T.);
#5575=FACE_OUTER_BOUND('',#10840,.T.);
#5576=FACE_OUTER_BOUND('',#10841,.T.);
#5577=FACE_OUTER_BOUND('',#10842,.T.);
#5578=FACE_OUTER_BOUND('',#10843,.T.);
#5579=FACE_OUTER_BOUND('',#10844,.T.);
#5580=FACE_OUTER_BOUND('',#10845,.T.);
#5581=FACE_OUTER_BOUND('',#10846,.T.);
#5582=FACE_OUTER_BOUND('',#10847,.T.);
#5583=FACE_OUTER_BOUND('',#10848,.T.);
#5584=FACE_OUTER_BOUND('',#10849,.T.);
#5585=FACE_OUTER_BOUND('',#10850,.T.);
#5586=FACE_OUTER_BOUND('',#10851,.T.);
#5587=FACE_OUTER_BOUND('',#10852,.T.);
#5588=FACE_OUTER_BOUND('',#10853,.T.);
#5589=FACE_OUTER_BOUND('',#10854,.T.);
#5590=FACE_OUTER_BOUND('',#10855,.T.);
#5591=FACE_OUTER_BOUND('',#10856,.T.);
#5592=FACE_OUTER_BOUND('',#10857,.T.);
#5593=FACE_OUTER_BOUND('',#10858,.T.);
#5594=FACE_OUTER_BOUND('',#10859,.T.);
#5595=FACE_OUTER_BOUND('',#10860,.T.);
#5596=FACE_OUTER_BOUND('',#10861,.T.);
#5597=FACE_OUTER_BOUND('',#10862,.T.);
#5598=FACE_OUTER_BOUND('',#10863,.T.);
#5599=FACE_OUTER_BOUND('',#10864,.T.);
#5600=FACE_OUTER_BOUND('',#10865,.T.);
#5601=FACE_OUTER_BOUND('',#10866,.T.);
#5602=FACE_OUTER_BOUND('',#10867,.T.);
#5603=FACE_OUTER_BOUND('',#10868,.T.);
#5604=FACE_OUTER_BOUND('',#10869,.T.);
#5605=FACE_OUTER_BOUND('',#10870,.T.);
#5606=FACE_OUTER_BOUND('',#10871,.T.);
#5607=FACE_OUTER_BOUND('',#10872,.T.);
#5608=FACE_OUTER_BOUND('',#10873,.T.);
#5609=FACE_OUTER_BOUND('',#10874,.T.);
#5610=FACE_OUTER_BOUND('',#10875,.T.);
#5611=FACE_OUTER_BOUND('',#10876,.T.);
#5612=FACE_OUTER_BOUND('',#10877,.T.);
#5613=FACE_OUTER_BOUND('',#10878,.T.);
#5614=FACE_OUTER_BOUND('',#10879,.T.);
#5615=FACE_OUTER_BOUND('',#10880,.T.);
#5616=FACE_OUTER_BOUND('',#10881,.T.);
#5617=FACE_OUTER_BOUND('',#10882,.T.);
#5618=FACE_OUTER_BOUND('',#10883,.T.);
#5619=FACE_OUTER_BOUND('',#10884,.T.);
#5620=FACE_OUTER_BOUND('',#10885,.T.);
#5621=FACE_OUTER_BOUND('',#10886,.T.);
#5622=FACE_OUTER_BOUND('',#10887,.T.);
#5623=FACE_OUTER_BOUND('',#10888,.T.);
#5624=FACE_OUTER_BOUND('',#10889,.T.);
#5625=FACE_OUTER_BOUND('',#10890,.T.);
#5626=FACE_OUTER_BOUND('',#10891,.T.);
#5627=FACE_OUTER_BOUND('',#10892,.T.);
#5628=FACE_OUTER_BOUND('',#10893,.T.);
#5629=FACE_OUTER_BOUND('',#10894,.T.);
#5630=FACE_OUTER_BOUND('',#10895,.T.);
#5631=FACE_OUTER_BOUND('',#10896,.T.);
#5632=FACE_OUTER_BOUND('',#10897,.T.);
#5633=FACE_OUTER_BOUND('',#10898,.T.);
#5634=FACE_OUTER_BOUND('',#10899,.T.);
#5635=FACE_OUTER_BOUND('',#10900,.T.);
#5636=FACE_OUTER_BOUND('',#10901,.T.);
#5637=FACE_OUTER_BOUND('',#10902,.T.);
#5638=FACE_OUTER_BOUND('',#10903,.T.);
#5639=FACE_OUTER_BOUND('',#10904,.T.);
#5640=FACE_OUTER_BOUND('',#10905,.T.);
#5641=FACE_OUTER_BOUND('',#10906,.T.);
#5642=FACE_OUTER_BOUND('',#10907,.T.);
#5643=FACE_OUTER_BOUND('',#10908,.T.);
#5644=FACE_OUTER_BOUND('',#10909,.T.);
#5645=FACE_OUTER_BOUND('',#10910,.T.);
#5646=FACE_OUTER_BOUND('',#10911,.T.);
#5647=FACE_OUTER_BOUND('',#10912,.T.);
#5648=FACE_OUTER_BOUND('',#10913,.T.);
#5649=FACE_OUTER_BOUND('',#10914,.T.);
#5650=FACE_OUTER_BOUND('',#10915,.T.);
#5651=FACE_OUTER_BOUND('',#10916,.T.);
#5652=FACE_OUTER_BOUND('',#10917,.T.);
#5653=FACE_OUTER_BOUND('',#10918,.T.);
#5654=FACE_OUTER_BOUND('',#10919,.T.);
#5655=FACE_OUTER_BOUND('',#10920,.T.);
#5656=FACE_OUTER_BOUND('',#10921,.T.);
#5657=FACE_OUTER_BOUND('',#10922,.T.);
#5658=FACE_OUTER_BOUND('',#10923,.T.);
#5659=FACE_OUTER_BOUND('',#10924,.T.);
#5660=FACE_OUTER_BOUND('',#10925,.T.);
#5661=FACE_OUTER_BOUND('',#10926,.T.);
#5662=FACE_OUTER_BOUND('',#10927,.T.);
#5663=FACE_OUTER_BOUND('',#10928,.T.);
#5664=FACE_OUTER_BOUND('',#10929,.T.);
#5665=FACE_OUTER_BOUND('',#10930,.T.);
#5666=FACE_OUTER_BOUND('',#10931,.T.);
#5667=FACE_OUTER_BOUND('',#10932,.T.);
#5668=FACE_OUTER_BOUND('',#10933,.T.);
#5669=FACE_OUTER_BOUND('',#10934,.T.);
#5670=FACE_OUTER_BOUND('',#10935,.T.);
#5671=FACE_OUTER_BOUND('',#10936,.T.);
#5672=FACE_OUTER_BOUND('',#10937,.T.);
#5673=FACE_OUTER_BOUND('',#10938,.T.);
#5674=FACE_OUTER_BOUND('',#10939,.T.);
#5675=FACE_OUTER_BOUND('',#10940,.T.);
#5676=FACE_OUTER_BOUND('',#10941,.T.);
#5677=FACE_OUTER_BOUND('',#10942,.T.);
#5678=FACE_OUTER_BOUND('',#10943,.T.);
#5679=FACE_OUTER_BOUND('',#10944,.T.);
#5680=FACE_OUTER_BOUND('',#10945,.T.);
#5681=FACE_OUTER_BOUND('',#10946,.T.);
#5682=FACE_OUTER_BOUND('',#10947,.T.);
#5683=FACE_OUTER_BOUND('',#10948,.T.);
#5684=FACE_OUTER_BOUND('',#10949,.T.);
#5685=FACE_OUTER_BOUND('',#10950,.T.);
#5686=FACE_OUTER_BOUND('',#10951,.T.);
#5687=FACE_OUTER_BOUND('',#10952,.T.);
#5688=FACE_OUTER_BOUND('',#10953,.T.);
#5689=FACE_OUTER_BOUND('',#10954,.T.);
#5690=FACE_OUTER_BOUND('',#10955,.T.);
#5691=FACE_OUTER_BOUND('',#10956,.T.);
#5692=FACE_OUTER_BOUND('',#10957,.T.);
#5693=FACE_OUTER_BOUND('',#10958,.T.);
#5694=FACE_OUTER_BOUND('',#10959,.T.);
#5695=FACE_OUTER_BOUND('',#10960,.T.);
#5696=FACE_OUTER_BOUND('',#10961,.T.);
#5697=FACE_OUTER_BOUND('',#10962,.T.);
#5698=FACE_OUTER_BOUND('',#10963,.T.);
#5699=FACE_OUTER_BOUND('',#10964,.T.);
#5700=FACE_OUTER_BOUND('',#10965,.T.);
#5701=FACE_OUTER_BOUND('',#10966,.T.);
#5702=FACE_OUTER_BOUND('',#10967,.T.);
#5703=FACE_OUTER_BOUND('',#10968,.T.);
#5704=FACE_OUTER_BOUND('',#10969,.T.);
#5705=FACE_OUTER_BOUND('',#10970,.T.);
#5706=FACE_OUTER_BOUND('',#10971,.T.);
#5707=FACE_OUTER_BOUND('',#10972,.T.);
#5708=FACE_OUTER_BOUND('',#10973,.T.);
#5709=FACE_OUTER_BOUND('',#10974,.T.);
#5710=FACE_OUTER_BOUND('',#10975,.T.);
#5711=FACE_OUTER_BOUND('',#10976,.T.);
#5712=FACE_OUTER_BOUND('',#10977,.T.);
#5713=FACE_OUTER_BOUND('',#10978,.T.);
#5714=FACE_OUTER_BOUND('',#10979,.T.);
#5715=FACE_OUTER_BOUND('',#10980,.T.);
#5716=FACE_OUTER_BOUND('',#10981,.T.);
#5717=FACE_OUTER_BOUND('',#10982,.T.);
#5718=FACE_OUTER_BOUND('',#10983,.T.);
#5719=FACE_OUTER_BOUND('',#10984,.T.);
#5720=FACE_OUTER_BOUND('',#10985,.T.);
#5721=FACE_OUTER_BOUND('',#10986,.T.);
#5722=FACE_OUTER_BOUND('',#10987,.T.);
#5723=FACE_OUTER_BOUND('',#10988,.T.);
#5724=FACE_OUTER_BOUND('',#10989,.T.);
#5725=FACE_OUTER_BOUND('',#10990,.T.);
#5726=FACE_OUTER_BOUND('',#10991,.T.);
#5727=FACE_OUTER_BOUND('',#10992,.T.);
#5728=FACE_OUTER_BOUND('',#10993,.T.);
#5729=FACE_OUTER_BOUND('',#10994,.T.);
#5730=FACE_OUTER_BOUND('',#10995,.T.);
#5731=FACE_OUTER_BOUND('',#10996,.T.);
#5732=FACE_OUTER_BOUND('',#10997,.T.);
#5733=FACE_OUTER_BOUND('',#10998,.T.);
#5734=FACE_OUTER_BOUND('',#10999,.T.);
#5735=FACE_OUTER_BOUND('',#11000,.T.);
#5736=FACE_OUTER_BOUND('',#11001,.T.);
#5737=FACE_OUTER_BOUND('',#11002,.T.);
#5738=FACE_OUTER_BOUND('',#11003,.T.);
#5739=FACE_OUTER_BOUND('',#11004,.T.);
#5740=FACE_OUTER_BOUND('',#11005,.T.);
#5741=FACE_OUTER_BOUND('',#11006,.T.);
#5742=FACE_OUTER_BOUND('',#11007,.T.);
#5743=FACE_OUTER_BOUND('',#11008,.T.);
#5744=FACE_OUTER_BOUND('',#11009,.T.);
#5745=FACE_OUTER_BOUND('',#11010,.T.);
#5746=FACE_OUTER_BOUND('',#11011,.T.);
#5747=FACE_OUTER_BOUND('',#11012,.T.);
#5748=FACE_OUTER_BOUND('',#11013,.T.);
#5749=FACE_OUTER_BOUND('',#11014,.T.);
#5750=FACE_OUTER_BOUND('',#11015,.T.);
#5751=FACE_OUTER_BOUND('',#11016,.T.);
#5752=FACE_OUTER_BOUND('',#11017,.T.);
#5753=FACE_OUTER_BOUND('',#11018,.T.);
#5754=FACE_OUTER_BOUND('',#11019,.T.);
#5755=FACE_OUTER_BOUND('',#11020,.T.);
#5756=FACE_OUTER_BOUND('',#11021,.T.);
#5757=FACE_OUTER_BOUND('',#11022,.T.);
#5758=FACE_OUTER_BOUND('',#11023,.T.);
#5759=FACE_OUTER_BOUND('',#11024,.T.);
#5760=FACE_OUTER_BOUND('',#11025,.T.);
#5761=FACE_OUTER_BOUND('',#11026,.T.);
#5762=FACE_OUTER_BOUND('',#11027,.T.);
#5763=FACE_OUTER_BOUND('',#11028,.T.);
#5764=FACE_OUTER_BOUND('',#11029,.T.);
#5765=FACE_OUTER_BOUND('',#11030,.T.);
#5766=FACE_OUTER_BOUND('',#11031,.T.);
#5767=FACE_OUTER_BOUND('',#11032,.T.);
#5768=FACE_OUTER_BOUND('',#11033,.T.);
#5769=FACE_OUTER_BOUND('',#11034,.T.);
#5770=FACE_OUTER_BOUND('',#11035,.T.);
#5771=FACE_OUTER_BOUND('',#11036,.T.);
#5772=FACE_OUTER_BOUND('',#11037,.T.);
#5773=FACE_OUTER_BOUND('',#11038,.T.);
#5774=FACE_OUTER_BOUND('',#11039,.T.);
#5775=FACE_OUTER_BOUND('',#11040,.T.);
#5776=FACE_OUTER_BOUND('',#11041,.T.);
#5777=FACE_OUTER_BOUND('',#11042,.T.);
#5778=FACE_OUTER_BOUND('',#11043,.T.);
#5779=FACE_OUTER_BOUND('',#11044,.T.);
#5780=FACE_OUTER_BOUND('',#11045,.T.);
#5781=FACE_OUTER_BOUND('',#11046,.T.);
#5782=FACE_OUTER_BOUND('',#11047,.T.);
#5783=FACE_OUTER_BOUND('',#11048,.T.);
#5784=FACE_OUTER_BOUND('',#11049,.T.);
#5785=FACE_OUTER_BOUND('',#11050,.T.);
#5786=FACE_OUTER_BOUND('',#11051,.T.);
#5787=FACE_OUTER_BOUND('',#11052,.T.);
#5788=FACE_OUTER_BOUND('',#11053,.T.);
#5789=FACE_OUTER_BOUND('',#11054,.T.);
#5790=FACE_OUTER_BOUND('',#11055,.T.);
#5791=FACE_OUTER_BOUND('',#11056,.T.);
#5792=FACE_OUTER_BOUND('',#11057,.T.);
#5793=FACE_OUTER_BOUND('',#11058,.T.);
#5794=FACE_OUTER_BOUND('',#11059,.T.);
#5795=FACE_OUTER_BOUND('',#11060,.T.);
#5796=FACE_OUTER_BOUND('',#11061,.T.);
#5797=FACE_OUTER_BOUND('',#11062,.T.);
#5798=FACE_OUTER_BOUND('',#11063,.T.);
#5799=FACE_OUTER_BOUND('',#11064,.T.);
#5800=FACE_OUTER_BOUND('',#11065,.T.);
#5801=FACE_OUTER_BOUND('',#11066,.T.);
#5802=FACE_OUTER_BOUND('',#11067,.T.);
#5803=FACE_OUTER_BOUND('',#11068,.T.);
#5804=FACE_OUTER_BOUND('',#11069,.T.);
#5805=FACE_OUTER_BOUND('',#11070,.T.);
#5806=FACE_OUTER_BOUND('',#11071,.T.);
#5807=FACE_OUTER_BOUND('',#11072,.T.);
#5808=FACE_OUTER_BOUND('',#11073,.T.);
#5809=FACE_OUTER_BOUND('',#11074,.T.);
#5810=FACE_OUTER_BOUND('',#11075,.T.);
#5811=FACE_OUTER_BOUND('',#11076,.T.);
#5812=FACE_OUTER_BOUND('',#11077,.T.);
#5813=FACE_OUTER_BOUND('',#11078,.T.);
#5814=FACE_OUTER_BOUND('',#11079,.T.);
#5815=FACE_OUTER_BOUND('',#11080,.T.);
#5816=FACE_OUTER_BOUND('',#11081,.T.);
#5817=FACE_OUTER_BOUND('',#11082,.T.);
#5818=FACE_OUTER_BOUND('',#11083,.T.);
#5819=FACE_OUTER_BOUND('',#11084,.T.);
#5820=FACE_OUTER_BOUND('',#11085,.T.);
#5821=FACE_OUTER_BOUND('',#11086,.T.);
#5822=FACE_OUTER_BOUND('',#11087,.T.);
#5823=FACE_OUTER_BOUND('',#11088,.T.);
#5824=FACE_OUTER_BOUND('',#11089,.T.);
#5825=FACE_OUTER_BOUND('',#11090,.T.);
#5826=FACE_OUTER_BOUND('',#11091,.T.);
#5827=FACE_OUTER_BOUND('',#11092,.T.);
#5828=FACE_OUTER_BOUND('',#11093,.T.);
#5829=FACE_OUTER_BOUND('',#11094,.T.);
#5830=FACE_OUTER_BOUND('',#11095,.T.);
#5831=FACE_OUTER_BOUND('',#11096,.T.);
#5832=FACE_OUTER_BOUND('',#11097,.T.);
#5833=FACE_OUTER_BOUND('',#11098,.T.);
#5834=FACE_OUTER_BOUND('',#11099,.T.);
#5835=FACE_OUTER_BOUND('',#11100,.T.);
#5836=FACE_OUTER_BOUND('',#11101,.T.);
#5837=FACE_OUTER_BOUND('',#11102,.T.);
#5838=FACE_OUTER_BOUND('',#11103,.T.);
#5839=FACE_OUTER_BOUND('',#11104,.T.);
#5840=FACE_OUTER_BOUND('',#11105,.T.);
#5841=FACE_OUTER_BOUND('',#11106,.T.);
#5842=FACE_OUTER_BOUND('',#11107,.T.);
#5843=FACE_OUTER_BOUND('',#11108,.T.);
#5844=FACE_OUTER_BOUND('',#11109,.T.);
#5845=FACE_OUTER_BOUND('',#11110,.T.);
#5846=FACE_OUTER_BOUND('',#11111,.T.);
#5847=FACE_OUTER_BOUND('',#11112,.T.);
#5848=FACE_OUTER_BOUND('',#11113,.T.);
#5849=FACE_OUTER_BOUND('',#11114,.T.);
#5850=FACE_OUTER_BOUND('',#11115,.T.);
#5851=FACE_OUTER_BOUND('',#11116,.T.);
#5852=FACE_OUTER_BOUND('',#11117,.T.);
#5853=FACE_OUTER_BOUND('',#11118,.T.);
#5854=FACE_OUTER_BOUND('',#11119,.T.);
#5855=FACE_OUTER_BOUND('',#11120,.T.);
#5856=FACE_OUTER_BOUND('',#11121,.T.);
#5857=FACE_OUTER_BOUND('',#11122,.T.);
#5858=FACE_OUTER_BOUND('',#11123,.T.);
#5859=FACE_OUTER_BOUND('',#11124,.T.);
#5860=FACE_OUTER_BOUND('',#11125,.T.);
#5861=FACE_OUTER_BOUND('',#11126,.T.);
#5862=FACE_OUTER_BOUND('',#11127,.T.);
#5863=FACE_OUTER_BOUND('',#11128,.T.);
#5864=FACE_OUTER_BOUND('',#11129,.T.);
#5865=FACE_OUTER_BOUND('',#11130,.T.);
#5866=FACE_OUTER_BOUND('',#11131,.T.);
#5867=FACE_OUTER_BOUND('',#11132,.T.);
#5868=FACE_OUTER_BOUND('',#11133,.T.);
#5869=FACE_OUTER_BOUND('',#11134,.T.);
#5870=FACE_OUTER_BOUND('',#11135,.T.);
#5871=FACE_OUTER_BOUND('',#11136,.T.);
#5872=FACE_OUTER_BOUND('',#11137,.T.);
#5873=FACE_OUTER_BOUND('',#11138,.T.);
#5874=FACE_OUTER_BOUND('',#11139,.T.);
#5875=FACE_OUTER_BOUND('',#11140,.T.);
#5876=FACE_OUTER_BOUND('',#11141,.T.);
#5877=FACE_OUTER_BOUND('',#11142,.T.);
#5878=FACE_OUTER_BOUND('',#11143,.T.);
#5879=FACE_OUTER_BOUND('',#11144,.T.);
#5880=FACE_OUTER_BOUND('',#11145,.T.);
#5881=FACE_OUTER_BOUND('',#11146,.T.);
#5882=FACE_OUTER_BOUND('',#11147,.T.);
#5883=FACE_OUTER_BOUND('',#11148,.T.);
#5884=FACE_OUTER_BOUND('',#11149,.T.);
#5885=FACE_OUTER_BOUND('',#11150,.T.);
#5886=FACE_OUTER_BOUND('',#11151,.T.);
#5887=FACE_OUTER_BOUND('',#11152,.T.);
#5888=FACE_OUTER_BOUND('',#11153,.T.);
#5889=FACE_OUTER_BOUND('',#11154,.T.);
#5890=FACE_OUTER_BOUND('',#11155,.T.);
#5891=FACE_OUTER_BOUND('',#11156,.T.);
#5892=FACE_OUTER_BOUND('',#11157,.T.);
#5893=FACE_OUTER_BOUND('',#11158,.T.);
#5894=FACE_OUTER_BOUND('',#11159,.T.);
#5895=FACE_OUTER_BOUND('',#11160,.T.);
#5896=FACE_OUTER_BOUND('',#11161,.T.);
#5897=FACE_OUTER_BOUND('',#11162,.T.);
#5898=FACE_OUTER_BOUND('',#11163,.T.);
#5899=FACE_OUTER_BOUND('',#11164,.T.);
#5900=FACE_OUTER_BOUND('',#11165,.T.);
#5901=FACE_OUTER_BOUND('',#11166,.T.);
#5902=FACE_OUTER_BOUND('',#11167,.T.);
#5903=FACE_OUTER_BOUND('',#11168,.T.);
#5904=FACE_OUTER_BOUND('',#11169,.T.);
#5905=FACE_OUTER_BOUND('',#11170,.T.);
#5906=FACE_OUTER_BOUND('',#11171,.T.);
#5907=FACE_OUTER_BOUND('',#11172,.T.);
#5908=FACE_OUTER_BOUND('',#11173,.T.);
#5909=FACE_OUTER_BOUND('',#11174,.T.);
#5910=FACE_OUTER_BOUND('',#11175,.T.);
#5911=FACE_OUTER_BOUND('',#11176,.T.);
#5912=FACE_OUTER_BOUND('',#11177,.T.);
#5913=FACE_OUTER_BOUND('',#11178,.T.);
#5914=FACE_OUTER_BOUND('',#11179,.T.);
#5915=FACE_OUTER_BOUND('',#11180,.T.);
#5916=FACE_OUTER_BOUND('',#11181,.T.);
#5917=FACE_OUTER_BOUND('',#11182,.T.);
#5918=FACE_OUTER_BOUND('',#11183,.T.);
#5919=FACE_OUTER_BOUND('',#11184,.T.);
#5920=FACE_OUTER_BOUND('',#11185,.T.);
#5921=FACE_OUTER_BOUND('',#11186,.T.);
#5922=FACE_OUTER_BOUND('',#11187,.T.);
#5923=FACE_OUTER_BOUND('',#11188,.T.);
#5924=FACE_OUTER_BOUND('',#11189,.T.);
#5925=FACE_OUTER_BOUND('',#11190,.T.);
#5926=FACE_OUTER_BOUND('',#11191,.T.);
#5927=FACE_OUTER_BOUND('',#11192,.T.);
#5928=FACE_OUTER_BOUND('',#11193,.T.);
#5929=FACE_OUTER_BOUND('',#11194,.T.);
#5930=FACE_OUTER_BOUND('',#11195,.T.);
#5931=FACE_OUTER_BOUND('',#11196,.T.);
#5932=FACE_OUTER_BOUND('',#11197,.T.);
#5933=FACE_OUTER_BOUND('',#11198,.T.);
#5934=FACE_OUTER_BOUND('',#11199,.T.);
#5935=FACE_OUTER_BOUND('',#11200,.T.);
#5936=FACE_OUTER_BOUND('',#11201,.T.);
#5937=FACE_OUTER_BOUND('',#11202,.T.);
#5938=FACE_OUTER_BOUND('',#11203,.T.);
#5939=FACE_OUTER_BOUND('',#11204,.T.);
#5940=FACE_OUTER_BOUND('',#11205,.T.);
#5941=FACE_OUTER_BOUND('',#11206,.T.);
#5942=FACE_OUTER_BOUND('',#11207,.T.);
#5943=FACE_OUTER_BOUND('',#11208,.T.);
#5944=FACE_OUTER_BOUND('',#11209,.T.);
#5945=FACE_OUTER_BOUND('',#11210,.T.);
#5946=FACE_OUTER_BOUND('',#11211,.T.);
#5947=FACE_OUTER_BOUND('',#11212,.T.);
#5948=FACE_OUTER_BOUND('',#11213,.T.);
#5949=FACE_OUTER_BOUND('',#11214,.T.);
#5950=FACE_OUTER_BOUND('',#11215,.T.);
#5951=FACE_OUTER_BOUND('',#11216,.T.);
#5952=FACE_OUTER_BOUND('',#11217,.T.);
#5953=FACE_OUTER_BOUND('',#11218,.T.);
#5954=FACE_OUTER_BOUND('',#11219,.T.);
#5955=FACE_OUTER_BOUND('',#11220,.T.);
#5956=FACE_OUTER_BOUND('',#11221,.T.);
#5957=FACE_OUTER_BOUND('',#11222,.T.);
#5958=FACE_OUTER_BOUND('',#11223,.T.);
#5959=FACE_OUTER_BOUND('',#11224,.T.);
#5960=FACE_OUTER_BOUND('',#11225,.T.);
#5961=FACE_OUTER_BOUND('',#11226,.T.);
#5962=FACE_OUTER_BOUND('',#11227,.T.);
#5963=FACE_OUTER_BOUND('',#11228,.T.);
#5964=FACE_OUTER_BOUND('',#11229,.T.);
#5965=FACE_OUTER_BOUND('',#11230,.T.);
#5966=FACE_OUTER_BOUND('',#11231,.T.);
#5967=FACE_OUTER_BOUND('',#11232,.T.);
#5968=FACE_OUTER_BOUND('',#11233,.T.);
#5969=FACE_OUTER_BOUND('',#11234,.T.);
#5970=FACE_OUTER_BOUND('',#11235,.T.);
#5971=FACE_OUTER_BOUND('',#11236,.T.);
#5972=FACE_OUTER_BOUND('',#11237,.T.);
#5973=FACE_OUTER_BOUND('',#11238,.T.);
#5974=FACE_OUTER_BOUND('',#11239,.T.);
#5975=FACE_OUTER_BOUND('',#11240,.T.);
#5976=FACE_OUTER_BOUND('',#11241,.T.);
#5977=FACE_OUTER_BOUND('',#11242,.T.);
#5978=FACE_OUTER_BOUND('',#11243,.T.);
#5979=FACE_OUTER_BOUND('',#11244,.T.);
#5980=FACE_OUTER_BOUND('',#11245,.T.);
#5981=FACE_OUTER_BOUND('',#11246,.T.);
#5982=FACE_OUTER_BOUND('',#11247,.T.);
#5983=FACE_OUTER_BOUND('',#11248,.T.);
#5984=FACE_OUTER_BOUND('',#11249,.T.);
#5985=FACE_OUTER_BOUND('',#11250,.T.);
#5986=FACE_OUTER_BOUND('',#11251,.T.);
#5987=FACE_OUTER_BOUND('',#11252,.T.);
#5988=FACE_OUTER_BOUND('',#11253,.T.);
#5989=FACE_OUTER_BOUND('',#11254,.T.);
#5990=FACE_OUTER_BOUND('',#11255,.T.);
#5991=FACE_OUTER_BOUND('',#11256,.T.);
#5992=FACE_OUTER_BOUND('',#11257,.T.);
#5993=FACE_OUTER_BOUND('',#11258,.T.);
#5994=FACE_OUTER_BOUND('',#11259,.T.);
#5995=FACE_OUTER_BOUND('',#11260,.T.);
#5996=FACE_OUTER_BOUND('',#11261,.T.);
#5997=FACE_OUTER_BOUND('',#11262,.T.);
#5998=FACE_OUTER_BOUND('',#11263,.T.);
#5999=FACE_OUTER_BOUND('',#11264,.T.);
#6000=FACE_OUTER_BOUND('',#11265,.T.);
#6001=FACE_OUTER_BOUND('',#11266,.T.);
#6002=FACE_OUTER_BOUND('',#11267,.T.);
#6003=FACE_OUTER_BOUND('',#11268,.T.);
#6004=FACE_OUTER_BOUND('',#11269,.T.);
#6005=FACE_OUTER_BOUND('',#11270,.T.);
#6006=FACE_OUTER_BOUND('',#11271,.T.);
#6007=FACE_OUTER_BOUND('',#11272,.T.);
#6008=FACE_OUTER_BOUND('',#11273,.T.);
#6009=FACE_OUTER_BOUND('',#11274,.T.);
#6010=FACE_OUTER_BOUND('',#11275,.T.);
#6011=FACE_OUTER_BOUND('',#11276,.T.);
#6012=FACE_OUTER_BOUND('',#11277,.T.);
#6013=FACE_OUTER_BOUND('',#11278,.T.);
#6014=FACE_OUTER_BOUND('',#11279,.T.);
#6015=FACE_OUTER_BOUND('',#11280,.T.);
#6016=FACE_OUTER_BOUND('',#11281,.T.);
#6017=FACE_OUTER_BOUND('',#11282,.T.);
#6018=FACE_OUTER_BOUND('',#11283,.T.);
#6019=FACE_OUTER_BOUND('',#11284,.T.);
#6020=FACE_OUTER_BOUND('',#11285,.T.);
#6021=FACE_OUTER_BOUND('',#11286,.T.);
#6022=FACE_OUTER_BOUND('',#11287,.T.);
#6023=FACE_OUTER_BOUND('',#11288,.T.);
#6024=FACE_OUTER_BOUND('',#11289,.T.);
#6025=FACE_OUTER_BOUND('',#11290,.T.);
#6026=FACE_OUTER_BOUND('',#11291,.T.);
#6027=FACE_OUTER_BOUND('',#11292,.T.);
#6028=FACE_OUTER_BOUND('',#11293,.T.);
#6029=FACE_OUTER_BOUND('',#11294,.T.);
#6030=FACE_OUTER_BOUND('',#11295,.T.);
#6031=FACE_OUTER_BOUND('',#11296,.T.);
#6032=FACE_OUTER_BOUND('',#11297,.T.);
#6033=FACE_OUTER_BOUND('',#11298,.T.);
#6034=FACE_OUTER_BOUND('',#11299,.T.);
#6035=FACE_OUTER_BOUND('',#11300,.T.);
#6036=FACE_OUTER_BOUND('',#11301,.T.);
#6037=FACE_OUTER_BOUND('',#11302,.T.);
#6038=FACE_OUTER_BOUND('',#11303,.T.);
#6039=FACE_OUTER_BOUND('',#11304,.T.);
#6040=FACE_OUTER_BOUND('',#11305,.T.);
#6041=FACE_OUTER_BOUND('',#11306,.T.);
#6042=FACE_OUTER_BOUND('',#11307,.T.);
#6043=FACE_OUTER_BOUND('',#11308,.T.);
#6044=FACE_OUTER_BOUND('',#11309,.T.);
#6045=FACE_OUTER_BOUND('',#11310,.T.);
#6046=FACE_OUTER_BOUND('',#11311,.T.);
#6047=FACE_OUTER_BOUND('',#11312,.T.);
#6048=FACE_OUTER_BOUND('',#11313,.T.);
#6049=FACE_OUTER_BOUND('',#11314,.T.);
#6050=FACE_OUTER_BOUND('',#11315,.T.);
#6051=FACE_OUTER_BOUND('',#11316,.T.);
#6052=FACE_OUTER_BOUND('',#11317,.T.);
#6053=FACE_OUTER_BOUND('',#11318,.T.);
#6054=FACE_OUTER_BOUND('',#11319,.T.);
#6055=FACE_OUTER_BOUND('',#11320,.T.);
#6056=FACE_OUTER_BOUND('',#11321,.T.);
#6057=FACE_OUTER_BOUND('',#11322,.T.);
#6058=FACE_OUTER_BOUND('',#11323,.T.);
#6059=FACE_OUTER_BOUND('',#11324,.T.);
#6060=FACE_OUTER_BOUND('',#11325,.T.);
#6061=FACE_OUTER_BOUND('',#11326,.T.);
#6062=FACE_OUTER_BOUND('',#11327,.T.);
#6063=FACE_OUTER_BOUND('',#11328,.T.);
#6064=FACE_OUTER_BOUND('',#11329,.T.);
#6065=FACE_OUTER_BOUND('',#11330,.T.);
#6066=FACE_OUTER_BOUND('',#11331,.T.);
#6067=FACE_OUTER_BOUND('',#11332,.T.);
#6068=FACE_OUTER_BOUND('',#11333,.T.);
#6069=FACE_OUTER_BOUND('',#11334,.T.);
#6070=FACE_OUTER_BOUND('',#11335,.T.);
#6071=FACE_OUTER_BOUND('',#11336,.T.);
#6072=FACE_OUTER_BOUND('',#11337,.T.);
#6073=FACE_OUTER_BOUND('',#11338,.T.);
#6074=FACE_OUTER_BOUND('',#11339,.T.);
#6075=FACE_OUTER_BOUND('',#11340,.T.);
#6076=FACE_OUTER_BOUND('',#11341,.T.);
#6077=FACE_OUTER_BOUND('',#11342,.T.);
#6078=FACE_OUTER_BOUND('',#11343,.T.);
#6079=FACE_OUTER_BOUND('',#11344,.T.);
#6080=FACE_OUTER_BOUND('',#11345,.T.);
#6081=FACE_OUTER_BOUND('',#11346,.T.);
#6082=FACE_OUTER_BOUND('',#11347,.T.);
#6083=FACE_OUTER_BOUND('',#11348,.T.);
#6084=FACE_OUTER_BOUND('',#11349,.T.);
#6085=FACE_OUTER_BOUND('',#11350,.T.);
#6086=FACE_OUTER_BOUND('',#11351,.T.);
#6087=FACE_OUTER_BOUND('',#11352,.T.);
#6088=FACE_OUTER_BOUND('',#11353,.T.);
#6089=FACE_OUTER_BOUND('',#11354,.T.);
#6090=FACE_OUTER_BOUND('',#11355,.T.);
#6091=FACE_OUTER_BOUND('',#11356,.T.);
#6092=FACE_OUTER_BOUND('',#11357,.T.);
#6093=FACE_OUTER_BOUND('',#11358,.T.);
#6094=FACE_OUTER_BOUND('',#11359,.T.);
#6095=FACE_OUTER_BOUND('',#11360,.T.);
#6096=FACE_OUTER_BOUND('',#11361,.T.);
#6097=FACE_OUTER_BOUND('',#11362,.T.);
#6098=FACE_OUTER_BOUND('',#11363,.T.);
#6099=FACE_OUTER_BOUND('',#11364,.T.);
#6100=FACE_OUTER_BOUND('',#11365,.T.);
#6101=FACE_OUTER_BOUND('',#11366,.T.);
#6102=FACE_OUTER_BOUND('',#11367,.T.);
#6103=FACE_OUTER_BOUND('',#11368,.T.);
#6104=FACE_OUTER_BOUND('',#11369,.T.);
#6105=FACE_OUTER_BOUND('',#11370,.T.);
#6106=FACE_OUTER_BOUND('',#11371,.T.);
#6107=FACE_OUTER_BOUND('',#11372,.T.);
#6108=FACE_OUTER_BOUND('',#11373,.T.);
#6109=FACE_OUTER_BOUND('',#11374,.T.);
#6110=FACE_OUTER_BOUND('',#11375,.T.);
#6111=FACE_OUTER_BOUND('',#11376,.T.);
#6112=FACE_OUTER_BOUND('',#11377,.T.);
#6113=FACE_OUTER_BOUND('',#11378,.T.);
#6114=FACE_OUTER_BOUND('',#11379,.T.);
#6115=FACE_OUTER_BOUND('',#11380,.T.);
#6116=FACE_OUTER_BOUND('',#11381,.T.);
#6117=FACE_OUTER_BOUND('',#11382,.T.);
#6118=FACE_OUTER_BOUND('',#11383,.T.);
#6119=FACE_OUTER_BOUND('',#11384,.T.);
#6120=FACE_OUTER_BOUND('',#11385,.T.);
#6121=FACE_OUTER_BOUND('',#11386,.T.);
#6122=FACE_OUTER_BOUND('',#11387,.T.);
#6123=FACE_OUTER_BOUND('',#11388,.T.);
#6124=FACE_OUTER_BOUND('',#11389,.T.);
#6125=FACE_OUTER_BOUND('',#11390,.T.);
#6126=FACE_OUTER_BOUND('',#11391,.T.);
#6127=FACE_OUTER_BOUND('',#11392,.T.);
#6128=FACE_OUTER_BOUND('',#11393,.T.);
#6129=FACE_OUTER_BOUND('',#11394,.T.);
#6130=FACE_OUTER_BOUND('',#11395,.T.);
#6131=FACE_OUTER_BOUND('',#11396,.T.);
#6132=FACE_OUTER_BOUND('',#11397,.T.);
#6133=FACE_OUTER_BOUND('',#11398,.T.);
#6134=FACE_OUTER_BOUND('',#11399,.T.);
#6135=FACE_OUTER_BOUND('',#11400,.T.);
#6136=FACE_OUTER_BOUND('',#11401,.T.);
#6137=FACE_OUTER_BOUND('',#11402,.T.);
#6138=FACE_OUTER_BOUND('',#11403,.T.);
#6139=FACE_OUTER_BOUND('',#11404,.T.);
#6140=FACE_OUTER_BOUND('',#11405,.T.);
#6141=FACE_OUTER_BOUND('',#11406,.T.);
#6142=FACE_OUTER_BOUND('',#11407,.T.);
#6143=FACE_OUTER_BOUND('',#11408,.T.);
#6144=FACE_OUTER_BOUND('',#11409,.T.);
#6145=FACE_OUTER_BOUND('',#11410,.T.);
#6146=FACE_OUTER_BOUND('',#11411,.T.);
#6147=FACE_OUTER_BOUND('',#11412,.T.);
#6148=FACE_OUTER_BOUND('',#11413,.T.);
#6149=FACE_OUTER_BOUND('',#11414,.T.);
#6150=FACE_OUTER_BOUND('',#11415,.T.);
#6151=FACE_OUTER_BOUND('',#11416,.T.);
#6152=FACE_OUTER_BOUND('',#11417,.T.);
#6153=FACE_OUTER_BOUND('',#11418,.T.);
#6154=FACE_OUTER_BOUND('',#11419,.T.);
#6155=FACE_OUTER_BOUND('',#11420,.T.);
#6156=FACE_OUTER_BOUND('',#11421,.T.);
#6157=FACE_OUTER_BOUND('',#11422,.T.);
#6158=FACE_OUTER_BOUND('',#11423,.T.);
#6159=FACE_OUTER_BOUND('',#11424,.T.);
#6160=FACE_OUTER_BOUND('',#11425,.T.);
#6161=FACE_OUTER_BOUND('',#11426,.T.);
#6162=FACE_OUTER_BOUND('',#11427,.T.);
#6163=FACE_OUTER_BOUND('',#11428,.T.);
#6164=FACE_OUTER_BOUND('',#11429,.T.);
#6165=FACE_OUTER_BOUND('',#11430,.T.);
#6166=FACE_OUTER_BOUND('',#11431,.T.);
#6167=FACE_OUTER_BOUND('',#11432,.T.);
#6168=FACE_OUTER_BOUND('',#11433,.T.);
#6169=FACE_OUTER_BOUND('',#11434,.T.);
#6170=FACE_OUTER_BOUND('',#11435,.T.);
#6171=FACE_OUTER_BOUND('',#11436,.T.);
#6172=FACE_OUTER_BOUND('',#11437,.T.);
#6173=FACE_OUTER_BOUND('',#11438,.T.);
#6174=FACE_OUTER_BOUND('',#11439,.T.);
#6175=FACE_OUTER_BOUND('',#11440,.T.);
#6176=FACE_OUTER_BOUND('',#11441,.T.);
#6177=FACE_OUTER_BOUND('',#11442,.T.);
#6178=FACE_OUTER_BOUND('',#11443,.T.);
#6179=FACE_OUTER_BOUND('',#11444,.T.);
#6180=FACE_OUTER_BOUND('',#11445,.T.);
#6181=FACE_OUTER_BOUND('',#11446,.T.);
#6182=FACE_OUTER_BOUND('',#11447,.T.);
#6183=FACE_OUTER_BOUND('',#11448,.T.);
#6184=FACE_OUTER_BOUND('',#11449,.T.);
#6185=FACE_OUTER_BOUND('',#11450,.T.);
#6186=FACE_OUTER_BOUND('',#11451,.T.);
#6187=FACE_OUTER_BOUND('',#11452,.T.);
#6188=FACE_OUTER_BOUND('',#11453,.T.);
#6189=FACE_OUTER_BOUND('',#11454,.T.);
#6190=FACE_OUTER_BOUND('',#11455,.T.);
#6191=FACE_OUTER_BOUND('',#11456,.T.);
#6192=FACE_OUTER_BOUND('',#11457,.T.);
#6193=FACE_OUTER_BOUND('',#11458,.T.);
#6194=FACE_OUTER_BOUND('',#11459,.T.);
#6195=FACE_OUTER_BOUND('',#11460,.T.);
#6196=FACE_OUTER_BOUND('',#11461,.T.);
#6197=FACE_OUTER_BOUND('',#11462,.T.);
#6198=FACE_OUTER_BOUND('',#11463,.T.);
#6199=FACE_OUTER_BOUND('',#11464,.T.);
#6200=FACE_OUTER_BOUND('',#11465,.T.);
#6201=FACE_OUTER_BOUND('',#11466,.T.);
#6202=FACE_OUTER_BOUND('',#11467,.T.);
#6203=FACE_OUTER_BOUND('',#11468,.T.);
#6204=FACE_OUTER_BOUND('',#11469,.T.);
#6205=FACE_OUTER_BOUND('',#11470,.T.);
#6206=FACE_OUTER_BOUND('',#11471,.T.);
#6207=FACE_OUTER_BOUND('',#11472,.T.);
#6208=FACE_OUTER_BOUND('',#11473,.T.);
#6209=FACE_OUTER_BOUND('',#11474,.T.);
#6210=FACE_OUTER_BOUND('',#11475,.T.);
#6211=FACE_OUTER_BOUND('',#11476,.T.);
#6212=FACE_OUTER_BOUND('',#11477,.T.);
#6213=FACE_OUTER_BOUND('',#11478,.T.);
#6214=FACE_OUTER_BOUND('',#11479,.T.);
#6215=FACE_OUTER_BOUND('',#11480,.T.);
#6216=FACE_OUTER_BOUND('',#11481,.T.);
#6217=FACE_OUTER_BOUND('',#11482,.T.);
#6218=FACE_OUTER_BOUND('',#11483,.T.);
#6219=FACE_OUTER_BOUND('',#11484,.T.);
#6220=FACE_OUTER_BOUND('',#11485,.T.);
#6221=FACE_OUTER_BOUND('',#11486,.T.);
#6222=FACE_OUTER_BOUND('',#11487,.T.);
#6223=FACE_OUTER_BOUND('',#11488,.T.);
#6224=FACE_OUTER_BOUND('',#11489,.T.);
#6225=FACE_OUTER_BOUND('',#11490,.T.);
#6226=FACE_OUTER_BOUND('',#11491,.T.);
#6227=FACE_OUTER_BOUND('',#11492,.T.);
#6228=FACE_OUTER_BOUND('',#11493,.T.);
#6229=FACE_OUTER_BOUND('',#11494,.T.);
#6230=FACE_OUTER_BOUND('',#11495,.T.);
#6231=FACE_OUTER_BOUND('',#11496,.T.);
#6232=FACE_OUTER_BOUND('',#11497,.T.);
#6233=FACE_OUTER_BOUND('',#11498,.T.);
#6234=FACE_OUTER_BOUND('',#11499,.T.);
#6235=FACE_OUTER_BOUND('',#11500,.T.);
#6236=FACE_OUTER_BOUND('',#11501,.T.);
#6237=FACE_OUTER_BOUND('',#11502,.T.);
#6238=FACE_OUTER_BOUND('',#11503,.T.);
#6239=FACE_OUTER_BOUND('',#11504,.T.);
#6240=FACE_OUTER_BOUND('',#11505,.T.);
#6241=FACE_OUTER_BOUND('',#11506,.T.);
#6242=FACE_OUTER_BOUND('',#11507,.T.);
#6243=FACE_OUTER_BOUND('',#11508,.T.);
#6244=FACE_OUTER_BOUND('',#11509,.T.);
#6245=FACE_OUTER_BOUND('',#11510,.T.);
#6246=FACE_OUTER_BOUND('',#11511,.T.);
#6247=FACE_OUTER_BOUND('',#11512,.T.);
#6248=FACE_OUTER_BOUND('',#11513,.T.);
#6249=FACE_OUTER_BOUND('',#11514,.T.);
#6250=FACE_OUTER_BOUND('',#11515,.T.);
#6251=FACE_OUTER_BOUND('',#11516,.T.);
#6252=FACE_OUTER_BOUND('',#11517,.T.);
#6253=FACE_OUTER_BOUND('',#11518,.T.);
#6254=FACE_OUTER_BOUND('',#11519,.T.);
#6255=FACE_OUTER_BOUND('',#11520,.T.);
#6256=FACE_OUTER_BOUND('',#11521,.T.);
#6257=FACE_OUTER_BOUND('',#11522,.T.);
#6258=FACE_OUTER_BOUND('',#11523,.T.);
#6259=FACE_OUTER_BOUND('',#11524,.T.);
#6260=FACE_OUTER_BOUND('',#11525,.T.);
#6261=FACE_OUTER_BOUND('',#11526,.T.);
#6262=FACE_OUTER_BOUND('',#11527,.T.);
#6263=FACE_OUTER_BOUND('',#11528,.T.);
#6264=FACE_OUTER_BOUND('',#11529,.T.);
#6265=FACE_OUTER_BOUND('',#11530,.T.);
#6266=FACE_OUTER_BOUND('',#11531,.T.);
#6267=FACE_OUTER_BOUND('',#11532,.T.);
#6268=FACE_OUTER_BOUND('',#11533,.T.);
#6269=FACE_OUTER_BOUND('',#11534,.T.);
#6270=FACE_OUTER_BOUND('',#11535,.T.);
#6271=FACE_OUTER_BOUND('',#11536,.T.);
#6272=FACE_OUTER_BOUND('',#11537,.T.);
#6273=FACE_OUTER_BOUND('',#11538,.T.);
#6274=FACE_OUTER_BOUND('',#11539,.T.);
#6275=FACE_OUTER_BOUND('',#11540,.T.);
#6276=FACE_OUTER_BOUND('',#11541,.T.);
#6277=FACE_OUTER_BOUND('',#11542,.T.);
#6278=FACE_OUTER_BOUND('',#11543,.T.);
#6279=FACE_OUTER_BOUND('',#11544,.T.);
#6280=FACE_OUTER_BOUND('',#11545,.T.);
#6281=FACE_OUTER_BOUND('',#11546,.T.);
#6282=FACE_OUTER_BOUND('',#11547,.T.);
#6283=FACE_OUTER_BOUND('',#11548,.T.);
#6284=FACE_OUTER_BOUND('',#11549,.T.);
#6285=FACE_OUTER_BOUND('',#11550,.T.);
#6286=FACE_OUTER_BOUND('',#11551,.T.);
#6287=FACE_OUTER_BOUND('',#11552,.T.);
#6288=FACE_OUTER_BOUND('',#11553,.T.);
#6289=FACE_OUTER_BOUND('',#11554,.T.);
#6290=FACE_OUTER_BOUND('',#11555,.T.);
#6291=FACE_OUTER_BOUND('',#11556,.T.);
#6292=FACE_OUTER_BOUND('',#11557,.T.);
#6293=FACE_OUTER_BOUND('',#11558,.T.);
#6294=FACE_OUTER_BOUND('',#11559,.T.);
#6295=FACE_OUTER_BOUND('',#11560,.T.);
#6296=FACE_OUTER_BOUND('',#11561,.T.);
#6297=FACE_OUTER_BOUND('',#11562,.T.);
#6298=FACE_OUTER_BOUND('',#11563,.T.);
#6299=FACE_OUTER_BOUND('',#11564,.T.);
#6300=FACE_OUTER_BOUND('',#11565,.T.);
#6301=FACE_OUTER_BOUND('',#11566,.T.);
#6302=FACE_OUTER_BOUND('',#11567,.T.);
#6303=FACE_OUTER_BOUND('',#11568,.T.);
#6304=FACE_OUTER_BOUND('',#11569,.T.);
#6305=FACE_OUTER_BOUND('',#11570,.T.);
#6306=FACE_OUTER_BOUND('',#11571,.T.);
#6307=FACE_OUTER_BOUND('',#11572,.T.);
#6308=FACE_OUTER_BOUND('',#11573,.T.);
#6309=FACE_OUTER_BOUND('',#11574,.T.);
#6310=FACE_OUTER_BOUND('',#11575,.T.);
#6311=FACE_OUTER_BOUND('',#11576,.T.);
#6312=FACE_OUTER_BOUND('',#11577,.T.);
#6313=FACE_OUTER_BOUND('',#11578,.T.);
#6314=FACE_OUTER_BOUND('',#11579,.T.);
#6315=FACE_OUTER_BOUND('',#11580,.T.);
#6316=FACE_OUTER_BOUND('',#11581,.T.);
#6317=FACE_OUTER_BOUND('',#11582,.T.);
#6318=FACE_OUTER_BOUND('',#11583,.T.);
#6319=FACE_OUTER_BOUND('',#11584,.T.);
#6320=FACE_OUTER_BOUND('',#11585,.T.);
#6321=FACE_OUTER_BOUND('',#11586,.T.);
#6322=FACE_OUTER_BOUND('',#11587,.T.);
#6323=FACE_OUTER_BOUND('',#11588,.T.);
#6324=FACE_OUTER_BOUND('',#11589,.T.);
#6325=FACE_OUTER_BOUND('',#11590,.T.);
#6326=FACE_OUTER_BOUND('',#11591,.T.);
#6327=FACE_OUTER_BOUND('',#11592,.T.);
#6328=FACE_OUTER_BOUND('',#11593,.T.);
#6329=FACE_OUTER_BOUND('',#11594,.T.);
#6330=FACE_OUTER_BOUND('',#11595,.T.);
#6331=FACE_OUTER_BOUND('',#11596,.T.);
#6332=FACE_OUTER_BOUND('',#11597,.T.);
#6333=FACE_OUTER_BOUND('',#11598,.T.);
#6334=FACE_OUTER_BOUND('',#11599,.T.);
#6335=FACE_OUTER_BOUND('',#11600,.T.);
#6336=FACE_OUTER_BOUND('',#11601,.T.);
#6337=FACE_OUTER_BOUND('',#11602,.T.);
#6338=FACE_OUTER_BOUND('',#11603,.T.);
#6339=FACE_OUTER_BOUND('',#11604,.T.);
#6340=FACE_OUTER_BOUND('',#11605,.T.);
#6341=FACE_OUTER_BOUND('',#11606,.T.);
#6342=FACE_OUTER_BOUND('',#11607,.T.);
#6343=FACE_OUTER_BOUND('',#11608,.T.);
#6344=FACE_OUTER_BOUND('',#11609,.T.);
#6345=FACE_OUTER_BOUND('',#11610,.T.);
#6346=FACE_OUTER_BOUND('',#11611,.T.);
#6347=FACE_OUTER_BOUND('',#11612,.T.);
#6348=FACE_OUTER_BOUND('',#11613,.T.);
#6349=FACE_OUTER_BOUND('',#11614,.T.);
#6350=FACE_OUTER_BOUND('',#11615,.T.);
#6351=FACE_OUTER_BOUND('',#11616,.T.);
#6352=FACE_OUTER_BOUND('',#11617,.T.);
#6353=FACE_OUTER_BOUND('',#11618,.T.);
#6354=FACE_OUTER_BOUND('',#11619,.T.);
#6355=FACE_OUTER_BOUND('',#11620,.T.);
#6356=FACE_OUTER_BOUND('',#11621,.T.);
#6357=FACE_OUTER_BOUND('',#11622,.T.);
#6358=FACE_OUTER_BOUND('',#11623,.T.);
#6359=FACE_OUTER_BOUND('',#11624,.T.);
#6360=FACE_OUTER_BOUND('',#11625,.T.);
#6361=FACE_OUTER_BOUND('',#11626,.T.);
#6362=FACE_OUTER_BOUND('',#11627,.T.);
#6363=FACE_OUTER_BOUND('',#11628,.T.);
#6364=FACE_OUTER_BOUND('',#11629,.T.);
#6365=FACE_OUTER_BOUND('',#11630,.T.);
#6366=FACE_OUTER_BOUND('',#11631,.T.);
#6367=FACE_OUTER_BOUND('',#11632,.T.);
#6368=FACE_OUTER_BOUND('',#11633,.T.);
#6369=FACE_OUTER_BOUND('',#11634,.T.);
#6370=FACE_OUTER_BOUND('',#11635,.T.);
#6371=FACE_OUTER_BOUND('',#11636,.T.);
#6372=FACE_OUTER_BOUND('',#11637,.T.);
#6373=FACE_OUTER_BOUND('',#11638,.T.);
#6374=FACE_OUTER_BOUND('',#11639,.T.);
#6375=FACE_OUTER_BOUND('',#11640,.T.);
#6376=FACE_OUTER_BOUND('',#11641,.T.);
#6377=FACE_OUTER_BOUND('',#11642,.T.);
#6378=FACE_OUTER_BOUND('',#11643,.T.);
#6379=FACE_OUTER_BOUND('',#11644,.T.);
#6380=FACE_OUTER_BOUND('',#11645,.T.);
#6381=FACE_OUTER_BOUND('',#11646,.T.);
#6382=FACE_OUTER_BOUND('',#11647,.T.);
#6383=FACE_OUTER_BOUND('',#11648,.T.);
#6384=FACE_OUTER_BOUND('',#11649,.T.);
#6385=FACE_OUTER_BOUND('',#11650,.T.);
#6386=FACE_OUTER_BOUND('',#11651,.T.);
#6387=FACE_OUTER_BOUND('',#11652,.T.);
#6388=FACE_OUTER_BOUND('',#11653,.T.);
#6389=FACE_OUTER_BOUND('',#11654,.T.);
#6390=FACE_OUTER_BOUND('',#11655,.T.);
#6391=FACE_OUTER_BOUND('',#11656,.T.);
#6392=FACE_OUTER_BOUND('',#11657,.T.);
#6393=FACE_OUTER_BOUND('',#11658,.T.);
#6394=FACE_OUTER_BOUND('',#11659,.T.);
#6395=FACE_OUTER_BOUND('',#11660,.T.);
#6396=FACE_OUTER_BOUND('',#11661,.T.);
#6397=FACE_OUTER_BOUND('',#11662,.T.);
#6398=FACE_OUTER_BOUND('',#11663,.T.);
#6399=FACE_OUTER_BOUND('',#11664,.T.);
#6400=FACE_OUTER_BOUND('',#11665,.T.);
#6401=FACE_OUTER_BOUND('',#11666,.T.);
#6402=FACE_OUTER_BOUND('',#11667,.T.);
#6403=FACE_OUTER_BOUND('',#11668,.T.);
#6404=FACE_OUTER_BOUND('',#11669,.T.);
#6405=FACE_OUTER_BOUND('',#11670,.T.);
#6406=FACE_OUTER_BOUND('',#11671,.T.);
#6407=FACE_OUTER_BOUND('',#11672,.T.);
#6408=FACE_OUTER_BOUND('',#11673,.T.);
#6409=FACE_OUTER_BOUND('',#11674,.T.);
#6410=FACE_OUTER_BOUND('',#11675,.T.);
#6411=FACE_OUTER_BOUND('',#11676,.T.);
#6412=FACE_OUTER_BOUND('',#11677,.T.);
#6413=FACE_OUTER_BOUND('',#11678,.T.);
#6414=FACE_OUTER_BOUND('',#11679,.T.);
#6415=FACE_OUTER_BOUND('',#11680,.T.);
#6416=FACE_OUTER_BOUND('',#11681,.T.);
#6417=FACE_OUTER_BOUND('',#11682,.T.);
#6418=FACE_OUTER_BOUND('',#11683,.T.);
#6419=FACE_OUTER_BOUND('',#11684,.T.);
#6420=FACE_OUTER_BOUND('',#11685,.T.);
#6421=FACE_OUTER_BOUND('',#11686,.T.);
#6422=FACE_OUTER_BOUND('',#11687,.T.);
#6423=FACE_OUTER_BOUND('',#11688,.T.);
#6424=FACE_OUTER_BOUND('',#11689,.T.);
#6425=FACE_OUTER_BOUND('',#11690,.T.);
#6426=FACE_OUTER_BOUND('',#11691,.T.);
#6427=FACE_OUTER_BOUND('',#11692,.T.);
#6428=FACE_OUTER_BOUND('',#11693,.T.);
#6429=FACE_OUTER_BOUND('',#11694,.T.);
#6430=FACE_OUTER_BOUND('',#11695,.T.);
#6431=FACE_OUTER_BOUND('',#11696,.T.);
#6432=FACE_OUTER_BOUND('',#11697,.T.);
#6433=FACE_OUTER_BOUND('',#11698,.T.);
#6434=FACE_OUTER_BOUND('',#11699,.T.);
#6435=FACE_OUTER_BOUND('',#11700,.T.);
#6436=FACE_OUTER_BOUND('',#11701,.T.);
#6437=FACE_OUTER_BOUND('',#11702,.T.);
#6438=FACE_OUTER_BOUND('',#11703,.T.);
#6439=FACE_OUTER_BOUND('',#11704,.T.);
#6440=FACE_OUTER_BOUND('',#11705,.T.);
#6441=FACE_OUTER_BOUND('',#11706,.T.);
#6442=FACE_OUTER_BOUND('',#11707,.T.);
#6443=FACE_OUTER_BOUND('',#11708,.T.);
#6444=FACE_OUTER_BOUND('',#11709,.T.);
#6445=FACE_OUTER_BOUND('',#11710,.T.);
#6446=FACE_OUTER_BOUND('',#11711,.T.);
#6447=FACE_OUTER_BOUND('',#11712,.T.);
#6448=FACE_OUTER_BOUND('',#11713,.T.);
#6449=FACE_OUTER_BOUND('',#11714,.T.);
#6450=FACE_OUTER_BOUND('',#11715,.T.);
#6451=FACE_OUTER_BOUND('',#11716,.T.);
#6452=FACE_OUTER_BOUND('',#11717,.T.);
#6453=FACE_OUTER_BOUND('',#11718,.T.);
#6454=FACE_OUTER_BOUND('',#11719,.T.);
#6455=FACE_OUTER_BOUND('',#11720,.T.);
#6456=FACE_OUTER_BOUND('',#11721,.T.);
#6457=FACE_OUTER_BOUND('',#11722,.T.);
#6458=FACE_OUTER_BOUND('',#11723,.T.);
#6459=FACE_OUTER_BOUND('',#11724,.T.);
#6460=FACE_OUTER_BOUND('',#11725,.T.);
#6461=FACE_OUTER_BOUND('',#11726,.T.);
#6462=FACE_OUTER_BOUND('',#11727,.T.);
#6463=FACE_OUTER_BOUND('',#11728,.T.);
#6464=FACE_OUTER_BOUND('',#11729,.T.);
#6465=FACE_OUTER_BOUND('',#11730,.T.);
#6466=FACE_OUTER_BOUND('',#11731,.T.);
#6467=FACE_OUTER_BOUND('',#11732,.T.);
#6468=FACE_OUTER_BOUND('',#11733,.T.);
#6469=FACE_OUTER_BOUND('',#11734,.T.);
#6470=FACE_OUTER_BOUND('',#11735,.T.);
#6471=FACE_OUTER_BOUND('',#11736,.T.);
#6472=FACE_OUTER_BOUND('',#11737,.T.);
#6473=FACE_OUTER_BOUND('',#11738,.T.);
#6474=FACE_OUTER_BOUND('',#11739,.T.);
#6475=FACE_OUTER_BOUND('',#11740,.T.);
#6476=FACE_OUTER_BOUND('',#11741,.T.);
#6477=FACE_OUTER_BOUND('',#11742,.T.);
#6478=FACE_OUTER_BOUND('',#11743,.T.);
#6479=FACE_OUTER_BOUND('',#11744,.T.);
#6480=FACE_OUTER_BOUND('',#11745,.T.);
#6481=FACE_OUTER_BOUND('',#11746,.T.);
#6482=FACE_OUTER_BOUND('',#11747,.T.);
#6483=FACE_OUTER_BOUND('',#11748,.T.);
#6484=FACE_OUTER_BOUND('',#11749,.T.);
#6485=FACE_OUTER_BOUND('',#11750,.T.);
#6486=FACE_OUTER_BOUND('',#11751,.T.);
#6487=FACE_OUTER_BOUND('',#11752,.T.);
#6488=FACE_OUTER_BOUND('',#11753,.T.);
#6489=FACE_OUTER_BOUND('',#11754,.T.);
#6490=FACE_OUTER_BOUND('',#11755,.T.);
#6491=FACE_OUTER_BOUND('',#11756,.T.);
#6492=FACE_OUTER_BOUND('',#11757,.T.);
#6493=FACE_OUTER_BOUND('',#11758,.T.);
#6494=FACE_OUTER_BOUND('',#11759,.T.);
#6495=FACE_OUTER_BOUND('',#11760,.T.);
#6496=FACE_OUTER_BOUND('',#11761,.T.);
#6497=FACE_OUTER_BOUND('',#11762,.T.);
#6498=FACE_OUTER_BOUND('',#11763,.T.);
#6499=FACE_OUTER_BOUND('',#11764,.T.);
#6500=FACE_OUTER_BOUND('',#11765,.T.);
#6501=FACE_OUTER_BOUND('',#11766,.T.);
#6502=FACE_OUTER_BOUND('',#11767,.T.);
#6503=FACE_OUTER_BOUND('',#11768,.T.);
#6504=FACE_OUTER_BOUND('',#11769,.T.);
#6505=FACE_OUTER_BOUND('',#11770,.T.);
#6506=FACE_OUTER_BOUND('',#11771,.T.);
#6507=FACE_OUTER_BOUND('',#11772,.T.);
#6508=FACE_OUTER_BOUND('',#11773,.T.);
#6509=FACE_OUTER_BOUND('',#11774,.T.);
#6510=FACE_OUTER_BOUND('',#11775,.T.);
#6511=FACE_OUTER_BOUND('',#11776,.T.);
#6512=FACE_OUTER_BOUND('',#11777,.T.);
#6513=FACE_OUTER_BOUND('',#11778,.T.);
#6514=FACE_OUTER_BOUND('',#11779,.T.);
#6515=FACE_OUTER_BOUND('',#11780,.T.);
#6516=FACE_OUTER_BOUND('',#11781,.T.);
#6517=FACE_OUTER_BOUND('',#11782,.T.);
#6518=FACE_OUTER_BOUND('',#11783,.T.);
#6519=FACE_OUTER_BOUND('',#11784,.T.);
#6520=FACE_OUTER_BOUND('',#11785,.T.);
#6521=FACE_OUTER_BOUND('',#11786,.T.);
#6522=FACE_OUTER_BOUND('',#11787,.T.);
#6523=FACE_OUTER_BOUND('',#11788,.T.);
#6524=FACE_OUTER_BOUND('',#11789,.T.);
#6525=FACE_OUTER_BOUND('',#11790,.T.);
#6526=FACE_OUTER_BOUND('',#11791,.T.);
#6527=FACE_OUTER_BOUND('',#11792,.T.);
#6528=FACE_OUTER_BOUND('',#11793,.T.);
#6529=FACE_OUTER_BOUND('',#11794,.T.);
#6530=FACE_OUTER_BOUND('',#11795,.T.);
#6531=FACE_OUTER_BOUND('',#11796,.T.);
#6532=FACE_OUTER_BOUND('',#11797,.T.);
#6533=FACE_OUTER_BOUND('',#11798,.T.);
#6534=FACE_OUTER_BOUND('',#11799,.T.);
#6535=FACE_OUTER_BOUND('',#11800,.T.);
#6536=FACE_OUTER_BOUND('',#11801,.T.);
#6537=FACE_OUTER_BOUND('',#11802,.T.);
#6538=FACE_OUTER_BOUND('',#11803,.T.);
#6539=FACE_OUTER_BOUND('',#11804,.T.);
#6540=FACE_OUTER_BOUND('',#11805,.T.);
#6541=FACE_OUTER_BOUND('',#11806,.T.);
#6542=FACE_OUTER_BOUND('',#11807,.T.);
#6543=FACE_OUTER_BOUND('',#11808,.T.);
#6544=FACE_OUTER_BOUND('',#11809,.T.);
#6545=FACE_OUTER_BOUND('',#11810,.T.);
#6546=FACE_OUTER_BOUND('',#11811,.T.);
#6547=FACE_OUTER_BOUND('',#11812,.T.);
#6548=FACE_OUTER_BOUND('',#11813,.T.);
#6549=FACE_OUTER_BOUND('',#11814,.T.);
#6550=FACE_OUTER_BOUND('',#11815,.T.);
#6551=FACE_OUTER_BOUND('',#11816,.T.);
#6552=FACE_OUTER_BOUND('',#11817,.T.);
#6553=FACE_OUTER_BOUND('',#11818,.T.);
#6554=FACE_OUTER_BOUND('',#11819,.T.);
#6555=FACE_OUTER_BOUND('',#11820,.T.);
#6556=FACE_OUTER_BOUND('',#11821,.T.);
#6557=FACE_OUTER_BOUND('',#11822,.T.);
#6558=FACE_OUTER_BOUND('',#11823,.T.);
#6559=FACE_OUTER_BOUND('',#11824,.T.);
#6560=FACE_OUTER_BOUND('',#11825,.T.);
#6561=FACE_OUTER_BOUND('',#11826,.T.);
#6562=FACE_OUTER_BOUND('',#11827,.T.);
#6563=FACE_OUTER_BOUND('',#11828,.T.);
#6564=FACE_OUTER_BOUND('',#11829,.T.);
#6565=FACE_OUTER_BOUND('',#11830,.T.);
#6566=FACE_OUTER_BOUND('',#11831,.T.);
#6567=FACE_OUTER_BOUND('',#11832,.T.);
#6568=FACE_OUTER_BOUND('',#11833,.T.);
#6569=FACE_OUTER_BOUND('',#11834,.T.);
#6570=FACE_OUTER_BOUND('',#11835,.T.);
#6571=FACE_OUTER_BOUND('',#11836,.T.);
#6572=FACE_OUTER_BOUND('',#11837,.T.);
#6573=FACE_OUTER_BOUND('',#11838,.T.);
#6574=FACE_OUTER_BOUND('',#11839,.T.);
#6575=FACE_OUTER_BOUND('',#11840,.T.);
#6576=FACE_OUTER_BOUND('',#11841,.T.);
#6577=FACE_OUTER_BOUND('',#11842,.T.);
#6578=FACE_OUTER_BOUND('',#11843,.T.);
#6579=FACE_OUTER_BOUND('',#11844,.T.);
#6580=FACE_OUTER_BOUND('',#11845,.T.);
#6581=FACE_OUTER_BOUND('',#11846,.T.);
#6582=FACE_OUTER_BOUND('',#11847,.T.);
#6583=FACE_OUTER_BOUND('',#11848,.T.);
#6584=FACE_OUTER_BOUND('',#11849,.T.);
#6585=FACE_OUTER_BOUND('',#11850,.T.);
#6586=FACE_OUTER_BOUND('',#11851,.T.);
#6587=FACE_OUTER_BOUND('',#11852,.T.);
#6588=FACE_OUTER_BOUND('',#11853,.T.);
#6589=FACE_OUTER_BOUND('',#11854,.T.);
#6590=FACE_OUTER_BOUND('',#11855,.T.);
#6591=FACE_OUTER_BOUND('',#11856,.T.);
#6592=FACE_OUTER_BOUND('',#11857,.T.);
#6593=FACE_OUTER_BOUND('',#11858,.T.);
#6594=FACE_OUTER_BOUND('',#11859,.T.);
#6595=FACE_OUTER_BOUND('',#11860,.T.);
#6596=FACE_OUTER_BOUND('',#11861,.T.);
#6597=FACE_OUTER_BOUND('',#11862,.T.);
#6598=FACE_OUTER_BOUND('',#11863,.T.);
#6599=FACE_OUTER_BOUND('',#11864,.T.);
#6600=FACE_OUTER_BOUND('',#11865,.T.);
#6601=FACE_OUTER_BOUND('',#11866,.T.);
#6602=FACE_OUTER_BOUND('',#11867,.T.);
#6603=FACE_OUTER_BOUND('',#11868,.T.);
#6604=FACE_OUTER_BOUND('',#11869,.T.);
#6605=FACE_OUTER_BOUND('',#11870,.T.);
#6606=FACE_OUTER_BOUND('',#11871,.T.);
#6607=FACE_OUTER_BOUND('',#11872,.T.);
#6608=FACE_OUTER_BOUND('',#11873,.T.);
#6609=FACE_OUTER_BOUND('',#11874,.T.);
#6610=FACE_OUTER_BOUND('',#11875,.T.);
#6611=FACE_OUTER_BOUND('',#11876,.T.);
#6612=FACE_OUTER_BOUND('',#11877,.T.);
#6613=FACE_OUTER_BOUND('',#11878,.T.);
#6614=FACE_OUTER_BOUND('',#11879,.T.);
#6615=FACE_OUTER_BOUND('',#11880,.T.);
#6616=FACE_OUTER_BOUND('',#11881,.T.);
#6617=FACE_OUTER_BOUND('',#11882,.T.);
#6618=FACE_OUTER_BOUND('',#11883,.T.);
#6619=FACE_OUTER_BOUND('',#11884,.T.);
#6620=FACE_OUTER_BOUND('',#11885,.T.);
#6621=FACE_OUTER_BOUND('',#11886,.T.);
#6622=FACE_OUTER_BOUND('',#11887,.T.);
#6623=FACE_OUTER_BOUND('',#11888,.T.);
#6624=FACE_OUTER_BOUND('',#11889,.T.);
#6625=FACE_OUTER_BOUND('',#11890,.T.);
#6626=FACE_OUTER_BOUND('',#11891,.T.);
#6627=FACE_OUTER_BOUND('',#11892,.T.);
#6628=FACE_OUTER_BOUND('',#11893,.T.);
#6629=FACE_OUTER_BOUND('',#11894,.T.);
#6630=FACE_OUTER_BOUND('',#11895,.T.);
#6631=FACE_OUTER_BOUND('',#11896,.T.);
#6632=FACE_OUTER_BOUND('',#11897,.T.);
#6633=FACE_OUTER_BOUND('',#11898,.T.);
#6634=FACE_OUTER_BOUND('',#11899,.T.);
#6635=FACE_OUTER_BOUND('',#11900,.T.);
#6636=FACE_OUTER_BOUND('',#11901,.T.);
#6637=FACE_OUTER_BOUND('',#11902,.T.);
#6638=FACE_OUTER_BOUND('',#11903,.T.);
#6639=FACE_OUTER_BOUND('',#11904,.T.);
#6640=FACE_OUTER_BOUND('',#11905,.T.);
#6641=FACE_OUTER_BOUND('',#11906,.T.);
#6642=FACE_OUTER_BOUND('',#11907,.T.);
#6643=FACE_OUTER_BOUND('',#11908,.T.);
#6644=FACE_OUTER_BOUND('',#11909,.T.);
#6645=FACE_OUTER_BOUND('',#11910,.T.);
#6646=FACE_OUTER_BOUND('',#11911,.T.);
#6647=FACE_OUTER_BOUND('',#11912,.T.);
#6648=FACE_OUTER_BOUND('',#11913,.T.);
#6649=FACE_OUTER_BOUND('',#11914,.T.);
#6650=FACE_OUTER_BOUND('',#11915,.T.);
#6651=FACE_OUTER_BOUND('',#11916,.T.);
#6652=FACE_OUTER_BOUND('',#11917,.T.);
#6653=FACE_OUTER_BOUND('',#11918,.T.);
#6654=FACE_OUTER_BOUND('',#11919,.T.);
#6655=FACE_OUTER_BOUND('',#11920,.T.);
#6656=FACE_OUTER_BOUND('',#11921,.T.);
#6657=FACE_OUTER_BOUND('',#11922,.T.);
#6658=FACE_OUTER_BOUND('',#11923,.T.);
#6659=FACE_OUTER_BOUND('',#11924,.T.);
#6660=FACE_OUTER_BOUND('',#11925,.T.);
#6661=FACE_OUTER_BOUND('',#11926,.T.);
#6662=FACE_OUTER_BOUND('',#11927,.T.);
#6663=FACE_OUTER_BOUND('',#11928,.T.);
#6664=FACE_OUTER_BOUND('',#11929,.T.);
#6665=FACE_OUTER_BOUND('',#11930,.T.);
#6666=FACE_OUTER_BOUND('',#11931,.T.);
#6667=FACE_OUTER_BOUND('',#11932,.T.);
#6668=FACE_OUTER_BOUND('',#11933,.T.);
#6669=FACE_OUTER_BOUND('',#11934,.T.);
#6670=FACE_OUTER_BOUND('',#11935,.T.);
#6671=FACE_OUTER_BOUND('',#11936,.T.);
#6672=FACE_OUTER_BOUND('',#11937,.T.);
#6673=FACE_OUTER_BOUND('',#11938,.T.);
#6674=FACE_OUTER_BOUND('',#11939,.T.);
#6675=FACE_OUTER_BOUND('',#11940,.T.);
#6676=FACE_OUTER_BOUND('',#11941,.T.);
#6677=FACE_OUTER_BOUND('',#11942,.T.);
#6678=FACE_OUTER_BOUND('',#11943,.T.);
#6679=FACE_OUTER_BOUND('',#11944,.T.);
#6680=FACE_OUTER_BOUND('',#11945,.T.);
#6681=FACE_OUTER_BOUND('',#11946,.T.);
#6682=FACE_OUTER_BOUND('',#11947,.T.);
#6683=FACE_OUTER_BOUND('',#11948,.T.);
#6684=FACE_OUTER_BOUND('',#11949,.T.);
#6685=FACE_OUTER_BOUND('',#11950,.T.);
#6686=FACE_OUTER_BOUND('',#11951,.T.);
#6687=FACE_OUTER_BOUND('',#11952,.T.);
#6688=FACE_OUTER_BOUND('',#11953,.T.);
#6689=FACE_OUTER_BOUND('',#11954,.T.);
#6690=FACE_OUTER_BOUND('',#11955,.T.);
#6691=FACE_OUTER_BOUND('',#11956,.T.);
#6692=FACE_OUTER_BOUND('',#11957,.T.);
#6693=FACE_OUTER_BOUND('',#11958,.T.);
#6694=FACE_OUTER_BOUND('',#11959,.T.);
#6695=FACE_OUTER_BOUND('',#11960,.T.);
#6696=FACE_OUTER_BOUND('',#11961,.T.);
#6697=FACE_OUTER_BOUND('',#11962,.T.);
#6698=FACE_OUTER_BOUND('',#11963,.T.);
#6699=FACE_OUTER_BOUND('',#11964,.T.);
#6700=FACE_OUTER_BOUND('',#11965,.T.);
#6701=FACE_OUTER_BOUND('',#11966,.T.);
#6702=FACE_OUTER_BOUND('',#11967,.T.);
#6703=FACE_OUTER_BOUND('',#11968,.T.);
#6704=FACE_OUTER_BOUND('',#11969,.T.);
#6705=FACE_OUTER_BOUND('',#11970,.T.);
#6706=FACE_OUTER_BOUND('',#11971,.T.);
#6707=FACE_OUTER_BOUND('',#11972,.T.);
#6708=FACE_OUTER_BOUND('',#11973,.T.);
#6709=FACE_OUTER_BOUND('',#11974,.T.);
#6710=FACE_OUTER_BOUND('',#11975,.T.);
#6711=FACE_OUTER_BOUND('',#11976,.T.);
#6712=FACE_OUTER_BOUND('',#11977,.T.);
#6713=FACE_OUTER_BOUND('',#11978,.T.);
#6714=FACE_OUTER_BOUND('',#11979,.T.);
#6715=FACE_OUTER_BOUND('',#11980,.T.);
#6716=FACE_OUTER_BOUND('',#11981,.T.);
#6717=FACE_OUTER_BOUND('',#11982,.T.);
#6718=FACE_OUTER_BOUND('',#11983,.T.);
#6719=FACE_OUTER_BOUND('',#11984,.T.);
#6720=FACE_OUTER_BOUND('',#11985,.T.);
#6721=FACE_OUTER_BOUND('',#11986,.T.);
#6722=FACE_OUTER_BOUND('',#11987,.T.);
#6723=FACE_OUTER_BOUND('',#11988,.T.);
#6724=FACE_OUTER_BOUND('',#11989,.T.);
#6725=FACE_OUTER_BOUND('',#11990,.T.);
#6726=FACE_OUTER_BOUND('',#11991,.T.);
#6727=FACE_OUTER_BOUND('',#11992,.T.);
#6728=FACE_OUTER_BOUND('',#11993,.T.);
#6729=FACE_OUTER_BOUND('',#11994,.T.);
#6730=FACE_OUTER_BOUND('',#11995,.T.);
#6731=FACE_OUTER_BOUND('',#11996,.T.);
#6732=FACE_OUTER_BOUND('',#11997,.T.);
#6733=FACE_OUTER_BOUND('',#11998,.T.);
#6734=FACE_OUTER_BOUND('',#11999,.T.);
#6735=FACE_OUTER_BOUND('',#12000,.T.);
#6736=FACE_OUTER_BOUND('',#12001,.T.);
#6737=FACE_OUTER_BOUND('',#12002,.T.);
#6738=FACE_OUTER_BOUND('',#12003,.T.);
#6739=FACE_OUTER_BOUND('',#12004,.T.);
#6740=FACE_OUTER_BOUND('',#12005,.T.);
#6741=FACE_OUTER_BOUND('',#12006,.T.);
#6742=FACE_OUTER_BOUND('',#12007,.T.);
#6743=FACE_OUTER_BOUND('',#12008,.T.);
#6744=FACE_OUTER_BOUND('',#12009,.T.);
#6745=FACE_OUTER_BOUND('',#12010,.T.);
#6746=FACE_OUTER_BOUND('',#12011,.T.);
#6747=FACE_OUTER_BOUND('',#12012,.T.);
#6748=FACE_OUTER_BOUND('',#12013,.T.);
#6749=FACE_OUTER_BOUND('',#12014,.T.);
#6750=FACE_OUTER_BOUND('',#12015,.T.);
#6751=FACE_OUTER_BOUND('',#12016,.T.);
#6752=FACE_OUTER_BOUND('',#12017,.T.);
#6753=FACE_OUTER_BOUND('',#12018,.T.);
#6754=FACE_OUTER_BOUND('',#12019,.T.);
#6755=FACE_OUTER_BOUND('',#12020,.T.);
#6756=FACE_OUTER_BOUND('',#12021,.T.);
#6757=FACE_OUTER_BOUND('',#12022,.T.);
#6758=FACE_OUTER_BOUND('',#12023,.T.);
#6759=FACE_OUTER_BOUND('',#12024,.T.);
#6760=FACE_OUTER_BOUND('',#12025,.T.);
#6761=FACE_OUTER_BOUND('',#12026,.T.);
#6762=FACE_OUTER_BOUND('',#12027,.T.);
#6763=FACE_OUTER_BOUND('',#12028,.T.);
#6764=FACE_OUTER_BOUND('',#12029,.T.);
#6765=FACE_OUTER_BOUND('',#12030,.T.);
#6766=FACE_OUTER_BOUND('',#12031,.T.);
#6767=FACE_OUTER_BOUND('',#12032,.T.);
#6768=FACE_OUTER_BOUND('',#12033,.T.);
#6769=FACE_OUTER_BOUND('',#12034,.T.);
#6770=FACE_OUTER_BOUND('',#12035,.T.);
#6771=FACE_OUTER_BOUND('',#12036,.T.);
#6772=FACE_OUTER_BOUND('',#12037,.T.);
#6773=FACE_OUTER_BOUND('',#12038,.T.);
#6774=FACE_OUTER_BOUND('',#12039,.T.);
#6775=FACE_OUTER_BOUND('',#12040,.T.);
#6776=FACE_OUTER_BOUND('',#12041,.T.);
#6777=FACE_OUTER_BOUND('',#12042,.T.);
#6778=FACE_OUTER_BOUND('',#12043,.T.);
#6779=FACE_OUTER_BOUND('',#12044,.T.);
#6780=FACE_OUTER_BOUND('',#12045,.T.);
#6781=FACE_OUTER_BOUND('',#12046,.T.);
#6782=FACE_OUTER_BOUND('',#12047,.T.);
#6783=FACE_OUTER_BOUND('',#12048,.T.);
#6784=FACE_OUTER_BOUND('',#12049,.T.);
#6785=FACE_OUTER_BOUND('',#12050,.T.);
#6786=FACE_OUTER_BOUND('',#12051,.T.);
#6787=FACE_OUTER_BOUND('',#12052,.T.);
#6788=FACE_OUTER_BOUND('',#12053,.T.);
#6789=FACE_OUTER_BOUND('',#12054,.T.);
#6790=FACE_OUTER_BOUND('',#12055,.T.);
#6791=FACE_OUTER_BOUND('',#12056,.T.);
#6792=FACE_OUTER_BOUND('',#12057,.T.);
#6793=FACE_OUTER_BOUND('',#12058,.T.);
#6794=FACE_OUTER_BOUND('',#12059,.T.);
#6795=FACE_OUTER_BOUND('',#12060,.T.);
#6796=FACE_OUTER_BOUND('',#12061,.T.);
#6797=FACE_OUTER_BOUND('',#12062,.T.);
#6798=FACE_OUTER_BOUND('',#12063,.T.);
#6799=FACE_OUTER_BOUND('',#12064,.T.);
#6800=FACE_OUTER_BOUND('',#12065,.T.);
#6801=FACE_OUTER_BOUND('',#12066,.T.);
#6802=FACE_OUTER_BOUND('',#12067,.T.);
#6803=FACE_OUTER_BOUND('',#12068,.T.);
#6804=FACE_OUTER_BOUND('',#12069,.T.);
#6805=FACE_OUTER_BOUND('',#12070,.T.);
#6806=FACE_OUTER_BOUND('',#12071,.T.);
#6807=FACE_OUTER_BOUND('',#12072,.T.);
#6808=FACE_OUTER_BOUND('',#12073,.T.);
#6809=FACE_OUTER_BOUND('',#12074,.T.);
#6810=FACE_OUTER_BOUND('',#12075,.T.);
#6811=FACE_OUTER_BOUND('',#12076,.T.);
#6812=FACE_OUTER_BOUND('',#12077,.T.);
#6813=FACE_OUTER_BOUND('',#12078,.T.);
#6814=FACE_OUTER_BOUND('',#12079,.T.);
#6815=FACE_OUTER_BOUND('',#12080,.T.);
#6816=FACE_OUTER_BOUND('',#12081,.T.);
#6817=FACE_OUTER_BOUND('',#12082,.T.);
#6818=FACE_OUTER_BOUND('',#12083,.T.);
#6819=FACE_OUTER_BOUND('',#12084,.T.);
#6820=FACE_OUTER_BOUND('',#12085,.T.);
#6821=FACE_OUTER_BOUND('',#12086,.T.);
#6822=FACE_OUTER_BOUND('',#12087,.T.);
#6823=FACE_OUTER_BOUND('',#12088,.T.);
#6824=FACE_OUTER_BOUND('',#12089,.T.);
#6825=FACE_OUTER_BOUND('',#12090,.T.);
#6826=FACE_OUTER_BOUND('',#12091,.T.);
#6827=FACE_OUTER_BOUND('',#12092,.T.);
#6828=FACE_OUTER_BOUND('',#12093,.T.);
#6829=FACE_OUTER_BOUND('',#12094,.T.);
#6830=FACE_OUTER_BOUND('',#12095,.T.);
#6831=FACE_OUTER_BOUND('',#12096,.T.);
#6832=FACE_OUTER_BOUND('',#12097,.T.);
#6833=FACE_OUTER_BOUND('',#12098,.T.);
#6834=FACE_OUTER_BOUND('',#12099,.T.);
#6835=FACE_OUTER_BOUND('',#12100,.T.);
#6836=FACE_OUTER_BOUND('',#12101,.T.);
#6837=FACE_OUTER_BOUND('',#12102,.T.);
#6838=FACE_OUTER_BOUND('',#12103,.T.);
#6839=FACE_OUTER_BOUND('',#12104,.T.);
#6840=FACE_OUTER_BOUND('',#12105,.T.);
#6841=FACE_OUTER_BOUND('',#12106,.T.);
#6842=FACE_OUTER_BOUND('',#12107,.T.);
#6843=FACE_OUTER_BOUND('',#12108,.T.);
#6844=FACE_OUTER_BOUND('',#12109,.T.);
#6845=FACE_OUTER_BOUND('',#12110,.T.);
#6846=FACE_OUTER_BOUND('',#12111,.T.);
#6847=FACE_OUTER_BOUND('',#12112,.T.);
#6848=FACE_OUTER_BOUND('',#12113,.T.);
#6849=FACE_OUTER_BOUND('',#12114,.T.);
#6850=FACE_OUTER_BOUND('',#12115,.T.);
#6851=FACE_OUTER_BOUND('',#12116,.T.);
#6852=FACE_OUTER_BOUND('',#12117,.T.);
#6853=FACE_OUTER_BOUND('',#12118,.T.);
#6854=FACE_OUTER_BOUND('',#12119,.T.);
#6855=FACE_OUTER_BOUND('',#12120,.T.);
#6856=FACE_OUTER_BOUND('',#12121,.T.);
#6857=FACE_OUTER_BOUND('',#12122,.T.);
#6858=FACE_OUTER_BOUND('',#12123,.T.);
#6859=FACE_OUTER_BOUND('',#12124,.T.);
#6860=FACE_OUTER_BOUND('',#12125,.T.);
#6861=FACE_OUTER_BOUND('',#12126,.T.);
#6862=FACE_OUTER_BOUND('',#12127,.T.);
#6863=FACE_OUTER_BOUND('',#12128,.T.);
#6864=FACE_OUTER_BOUND('',#12129,.T.);
#6865=FACE_OUTER_BOUND('',#12130,.T.);
#6866=FACE_OUTER_BOUND('',#12131,.T.);
#6867=FACE_OUTER_BOUND('',#12132,.T.);
#6868=FACE_OUTER_BOUND('',#12133,.T.);
#6869=FACE_OUTER_BOUND('',#12134,.T.);
#6870=FACE_OUTER_BOUND('',#12135,.T.);
#6871=FACE_OUTER_BOUND('',#12136,.T.);
#6872=FACE_OUTER_BOUND('',#12137,.T.);
#6873=FACE_OUTER_BOUND('',#12138,.T.);
#6874=FACE_OUTER_BOUND('',#12139,.T.);
#6875=FACE_OUTER_BOUND('',#12140,.T.);
#6876=FACE_OUTER_BOUND('',#12141,.T.);
#6877=FACE_OUTER_BOUND('',#12142,.T.);
#6878=FACE_OUTER_BOUND('',#12143,.T.);
#6879=FACE_OUTER_BOUND('',#12144,.T.);
#6880=FACE_OUTER_BOUND('',#12145,.T.);
#6881=FACE_OUTER_BOUND('',#12146,.T.);
#6882=FACE_OUTER_BOUND('',#12147,.T.);
#6883=FACE_OUTER_BOUND('',#12148,.T.);
#6884=FACE_OUTER_BOUND('',#12149,.T.);
#6885=FACE_OUTER_BOUND('',#12150,.T.);
#6886=FACE_OUTER_BOUND('',#12151,.T.);
#6887=FACE_OUTER_BOUND('',#12152,.T.);
#6888=FACE_OUTER_BOUND('',#12153,.T.);
#6889=FACE_OUTER_BOUND('',#12154,.T.);
#6890=FACE_OUTER_BOUND('',#12155,.T.);
#6891=FACE_OUTER_BOUND('',#12156,.T.);
#6892=FACE_OUTER_BOUND('',#12157,.T.);
#6893=FACE_OUTER_BOUND('',#12158,.T.);
#6894=FACE_OUTER_BOUND('',#12159,.T.);
#6895=FACE_OUTER_BOUND('',#12160,.T.);
#6896=FACE_OUTER_BOUND('',#12161,.T.);
#6897=FACE_OUTER_BOUND('',#12162,.T.);
#6898=FACE_OUTER_BOUND('',#12163,.T.);
#6899=FACE_OUTER_BOUND('',#12164,.T.);
#6900=FACE_OUTER_BOUND('',#12165,.T.);
#6901=FACE_OUTER_BOUND('',#12166,.T.);
#6902=FACE_OUTER_BOUND('',#12167,.T.);
#6903=FACE_OUTER_BOUND('',#12168,.T.);
#6904=FACE_OUTER_BOUND('',#12169,.T.);
#6905=FACE_OUTER_BOUND('',#12170,.T.);
#6906=FACE_OUTER_BOUND('',#12171,.T.);
#6907=FACE_OUTER_BOUND('',#12172,.T.);
#6908=FACE_OUTER_BOUND('',#12173,.T.);
#6909=FACE_OUTER_BOUND('',#12174,.T.);
#6910=FACE_OUTER_BOUND('',#12175,.T.);
#6911=FACE_OUTER_BOUND('',#12176,.T.);
#6912=FACE_OUTER_BOUND('',#12177,.T.);
#6913=FACE_OUTER_BOUND('',#12178,.T.);
#6914=FACE_OUTER_BOUND('',#12179,.T.);
#6915=FACE_OUTER_BOUND('',#12180,.T.);
#6916=FACE_OUTER_BOUND('',#12181,.T.);
#6917=FACE_OUTER_BOUND('',#12182,.T.);
#6918=FACE_OUTER_BOUND('',#12183,.T.);
#6919=FACE_OUTER_BOUND('',#12184,.T.);
#6920=FACE_OUTER_BOUND('',#12185,.T.);
#6921=FACE_OUTER_BOUND('',#12186,.T.);
#6922=FACE_OUTER_BOUND('',#12187,.T.);
#6923=FACE_OUTER_BOUND('',#12188,.T.);
#6924=FACE_OUTER_BOUND('',#12189,.T.);
#6925=FACE_OUTER_BOUND('',#12190,.T.);
#6926=FACE_OUTER_BOUND('',#12191,.T.);
#6927=FACE_OUTER_BOUND('',#12192,.T.);
#6928=FACE_OUTER_BOUND('',#12193,.T.);
#6929=FACE_OUTER_BOUND('',#12194,.T.);
#6930=FACE_OUTER_BOUND('',#12195,.T.);
#6931=FACE_OUTER_BOUND('',#12196,.T.);
#6932=FACE_OUTER_BOUND('',#12197,.T.);
#6933=FACE_OUTER_BOUND('',#12198,.T.);
#6934=FACE_OUTER_BOUND('',#12199,.T.);
#6935=FACE_OUTER_BOUND('',#12200,.T.);
#6936=FACE_OUTER_BOUND('',#12201,.T.);
#6937=FACE_OUTER_BOUND('',#12202,.T.);
#6938=FACE_OUTER_BOUND('',#12203,.T.);
#6939=FACE_OUTER_BOUND('',#12204,.T.);
#6940=FACE_OUTER_BOUND('',#12205,.T.);
#6941=FACE_OUTER_BOUND('',#12206,.T.);
#6942=FACE_OUTER_BOUND('',#12207,.T.);
#6943=FACE_OUTER_BOUND('',#12208,.T.);
#6944=FACE_OUTER_BOUND('',#12209,.T.);
#6945=FACE_OUTER_BOUND('',#12210,.T.);
#6946=FACE_OUTER_BOUND('',#12211,.T.);
#6947=FACE_OUTER_BOUND('',#12212,.T.);
#6948=FACE_OUTER_BOUND('',#12213,.T.);
#6949=FACE_OUTER_BOUND('',#12214,.T.);
#6950=FACE_OUTER_BOUND('',#12215,.T.);
#6951=FACE_OUTER_BOUND('',#12216,.T.);
#6952=FACE_OUTER_BOUND('',#12217,.T.);
#6953=FACE_OUTER_BOUND('',#12218,.T.);
#6954=FACE_OUTER_BOUND('',#12219,.T.);
#6955=FACE_OUTER_BOUND('',#12220,.T.);
#6956=FACE_OUTER_BOUND('',#12221,.T.);
#6957=FACE_OUTER_BOUND('',#12222,.T.);
#6958=FACE_OUTER_BOUND('',#12223,.T.);
#6959=FACE_OUTER_BOUND('',#12224,.T.);
#6960=FACE_OUTER_BOUND('',#12225,.T.);
#6961=FACE_OUTER_BOUND('',#12226,.T.);
#6962=FACE_OUTER_BOUND('',#12227,.T.);
#6963=FACE_OUTER_BOUND('',#12228,.T.);
#6964=FACE_OUTER_BOUND('',#12229,.T.);
#6965=FACE_OUTER_BOUND('',#12230,.T.);
#6966=FACE_OUTER_BOUND('',#12231,.T.);
#6967=FACE_OUTER_BOUND('',#12232,.T.);
#6968=FACE_OUTER_BOUND('',#12233,.T.);
#6969=FACE_OUTER_BOUND('',#12234,.T.);
#6970=FACE_OUTER_BOUND('',#12235,.T.);
#6971=FACE_OUTER_BOUND('',#12236,.T.);
#6972=FACE_OUTER_BOUND('',#12237,.T.);
#6973=FACE_OUTER_BOUND('',#12238,.T.);
#6974=FACE_OUTER_BOUND('',#12239,.T.);
#6975=FACE_OUTER_BOUND('',#12240,.T.);
#6976=FACE_OUTER_BOUND('',#12241,.T.);
#6977=FACE_OUTER_BOUND('',#12242,.T.);
#6978=FACE_OUTER_BOUND('',#12243,.T.);
#6979=FACE_OUTER_BOUND('',#12244,.T.);
#6980=FACE_OUTER_BOUND('',#12245,.T.);
#6981=FACE_OUTER_BOUND('',#12246,.T.);
#6982=FACE_OUTER_BOUND('',#12247,.T.);
#6983=FACE_OUTER_BOUND('',#12248,.T.);
#6984=FACE_OUTER_BOUND('',#12249,.T.);
#6985=FACE_OUTER_BOUND('',#12250,.T.);
#6986=FACE_OUTER_BOUND('',#12251,.T.);
#6987=FACE_OUTER_BOUND('',#12252,.T.);
#6988=FACE_OUTER_BOUND('',#12253,.T.);
#6989=FACE_OUTER_BOUND('',#12254,.T.);
#6990=FACE_OUTER_BOUND('',#12255,.T.);
#6991=FACE_OUTER_BOUND('',#12256,.T.);
#6992=FACE_OUTER_BOUND('',#12257,.T.);
#6993=FACE_OUTER_BOUND('',#12258,.T.);
#6994=FACE_OUTER_BOUND('',#12259,.T.);
#6995=FACE_OUTER_BOUND('',#12260,.T.);
#6996=FACE_OUTER_BOUND('',#12261,.T.);
#6997=FACE_OUTER_BOUND('',#12262,.T.);
#6998=FACE_OUTER_BOUND('',#12263,.T.);
#6999=FACE_OUTER_BOUND('',#12264,.T.);
#7000=FACE_OUTER_BOUND('',#12265,.T.);
#7001=FACE_OUTER_BOUND('',#12266,.T.);
#7002=FACE_OUTER_BOUND('',#12267,.T.);
#7003=FACE_OUTER_BOUND('',#12268,.T.);
#7004=FACE_OUTER_BOUND('',#12269,.T.);
#7005=FACE_OUTER_BOUND('',#12270,.T.);
#7006=FACE_OUTER_BOUND('',#12271,.T.);
#7007=FACE_OUTER_BOUND('',#12272,.T.);
#7008=FACE_OUTER_BOUND('',#12273,.T.);
#7009=FACE_OUTER_BOUND('',#12274,.T.);
#7010=FACE_OUTER_BOUND('',#12275,.T.);
#7011=FACE_OUTER_BOUND('',#12276,.T.);
#7012=FACE_OUTER_BOUND('',#12277,.T.);
#7013=FACE_OUTER_BOUND('',#12278,.T.);
#7014=FACE_OUTER_BOUND('',#12279,.T.);
#7015=FACE_OUTER_BOUND('',#12280,.T.);
#7016=FACE_OUTER_BOUND('',#12281,.T.);
#7017=FACE_OUTER_BOUND('',#12282,.T.);
#7018=FACE_OUTER_BOUND('',#12283,.T.);
#7019=FACE_OUTER_BOUND('',#12284,.T.);
#7020=FACE_OUTER_BOUND('',#12285,.T.);
#7021=FACE_OUTER_BOUND('',#12286,.T.);
#7022=FACE_OUTER_BOUND('',#12287,.T.);
#7023=FACE_OUTER_BOUND('',#12288,.T.);
#7024=FACE_OUTER_BOUND('',#12289,.T.);
#7025=FACE_OUTER_BOUND('',#12290,.T.);
#7026=FACE_OUTER_BOUND('',#12291,.T.);
#7027=FACE_OUTER_BOUND('',#12292,.T.);
#7028=FACE_OUTER_BOUND('',#12293,.T.);
#7029=FACE_OUTER_BOUND('',#12294,.T.);
#7030=FACE_OUTER_BOUND('',#12295,.T.);
#7031=FACE_OUTER_BOUND('',#12296,.T.);
#7032=FACE_OUTER_BOUND('',#12297,.T.);
#7033=FACE_OUTER_BOUND('',#12298,.T.);
#7034=FACE_OUTER_BOUND('',#12299,.T.);
#7035=FACE_OUTER_BOUND('',#12300,.T.);
#7036=FACE_OUTER_BOUND('',#12301,.T.);
#7037=FACE_OUTER_BOUND('',#12302,.T.);
#7038=FACE_OUTER_BOUND('',#12303,.T.);
#7039=FACE_OUTER_BOUND('',#12304,.T.);
#7040=FACE_OUTER_BOUND('',#12305,.T.);
#7041=FACE_OUTER_BOUND('',#12306,.T.);
#7042=FACE_OUTER_BOUND('',#12307,.T.);
#7043=FACE_OUTER_BOUND('',#12308,.T.);
#7044=FACE_OUTER_BOUND('',#12309,.T.);
#7045=FACE_OUTER_BOUND('',#12310,.T.);
#7046=FACE_OUTER_BOUND('',#12311,.T.);
#7047=FACE_OUTER_BOUND('',#12312,.T.);
#7048=FACE_OUTER_BOUND('',#12313,.T.);
#7049=FACE_OUTER_BOUND('',#12314,.T.);
#7050=FACE_OUTER_BOUND('',#12315,.T.);
#7051=FACE_OUTER_BOUND('',#12316,.T.);
#7052=FACE_OUTER_BOUND('',#12317,.T.);
#7053=FACE_OUTER_BOUND('',#12318,.T.);
#7054=FACE_OUTER_BOUND('',#12319,.T.);
#7055=FACE_OUTER_BOUND('',#12320,.T.);
#7056=FACE_OUTER_BOUND('',#12321,.T.);
#7057=FACE_OUTER_BOUND('',#12322,.T.);
#7058=FACE_OUTER_BOUND('',#12323,.T.);
#7059=FACE_OUTER_BOUND('',#12324,.T.);
#7060=FACE_OUTER_BOUND('',#12325,.T.);
#7061=FACE_OUTER_BOUND('',#12326,.T.);
#7062=FACE_OUTER_BOUND('',#12327,.T.);
#7063=FACE_OUTER_BOUND('',#12328,.T.);
#7064=FACE_OUTER_BOUND('',#12329,.T.);
#7065=FACE_OUTER_BOUND('',#12330,.T.);
#7066=FACE_OUTER_BOUND('',#12331,.T.);
#7067=FACE_OUTER_BOUND('',#12332,.T.);
#7068=FACE_OUTER_BOUND('',#12333,.T.);
#7069=FACE_OUTER_BOUND('',#12334,.T.);
#7070=FACE_OUTER_BOUND('',#12335,.T.);
#7071=FACE_OUTER_BOUND('',#12336,.T.);
#7072=FACE_OUTER_BOUND('',#12337,.T.);
#7073=FACE_OUTER_BOUND('',#12338,.T.);
#7074=FACE_OUTER_BOUND('',#12339,.T.);
#7075=FACE_OUTER_BOUND('',#12340,.T.);
#7076=FACE_OUTER_BOUND('',#12341,.T.);
#7077=FACE_OUTER_BOUND('',#12342,.T.);
#7078=FACE_OUTER_BOUND('',#12343,.T.);
#7079=FACE_OUTER_BOUND('',#12344,.T.);
#7080=FACE_OUTER_BOUND('',#12345,.T.);
#7081=FACE_OUTER_BOUND('',#12346,.T.);
#7082=FACE_OUTER_BOUND('',#12347,.T.);
#7083=FACE_OUTER_BOUND('',#12348,.T.);
#7084=FACE_OUTER_BOUND('',#12349,.T.);
#7085=FACE_OUTER_BOUND('',#12350,.T.);
#7086=FACE_OUTER_BOUND('',#12351,.T.);
#7087=FACE_OUTER_BOUND('',#12352,.T.);
#7088=FACE_OUTER_BOUND('',#12353,.T.);
#7089=FACE_OUTER_BOUND('',#12354,.T.);
#7090=FACE_OUTER_BOUND('',#12355,.T.);
#7091=FACE_OUTER_BOUND('',#12356,.T.);
#7092=FACE_OUTER_BOUND('',#12357,.T.);
#7093=FACE_OUTER_BOUND('',#12358,.T.);
#7094=FACE_OUTER_BOUND('',#12359,.T.);
#7095=FACE_OUTER_BOUND('',#12360,.T.);
#7096=FACE_OUTER_BOUND('',#12361,.T.);
#7097=FACE_OUTER_BOUND('',#12362,.T.);
#7098=FACE_OUTER_BOUND('',#12363,.T.);
#7099=FACE_OUTER_BOUND('',#12364,.T.);
#7100=FACE_OUTER_BOUND('',#12365,.T.);
#7101=FACE_OUTER_BOUND('',#12366,.T.);
#7102=FACE_OUTER_BOUND('',#12367,.T.);
#7103=FACE_OUTER_BOUND('',#12368,.T.);
#7104=FACE_OUTER_BOUND('',#12369,.T.);
#7105=FACE_OUTER_BOUND('',#12370,.T.);
#7106=FACE_OUTER_BOUND('',#12371,.T.);
#7107=FACE_OUTER_BOUND('',#12372,.T.);
#7108=FACE_OUTER_BOUND('',#12373,.T.);
#7109=FACE_OUTER_BOUND('',#12374,.T.);
#7110=FACE_OUTER_BOUND('',#12375,.T.);
#7111=FACE_OUTER_BOUND('',#12376,.T.);
#7112=FACE_OUTER_BOUND('',#12377,.T.);
#7113=FACE_OUTER_BOUND('',#12378,.T.);
#7114=FACE_OUTER_BOUND('',#12379,.T.);
#7115=FACE_OUTER_BOUND('',#12380,.T.);
#7116=FACE_OUTER_BOUND('',#12381,.T.);
#7117=FACE_OUTER_BOUND('',#12382,.T.);
#7118=FACE_OUTER_BOUND('',#12383,.T.);
#7119=FACE_OUTER_BOUND('',#12384,.T.);
#7120=FACE_OUTER_BOUND('',#12385,.T.);
#7121=FACE_OUTER_BOUND('',#12386,.T.);
#7122=FACE_OUTER_BOUND('',#12387,.T.);
#7123=FACE_OUTER_BOUND('',#12388,.T.);
#7124=FACE_OUTER_BOUND('',#12389,.T.);
#7125=FACE_OUTER_BOUND('',#12390,.T.);
#7126=FACE_OUTER_BOUND('',#12391,.T.);
#7127=FACE_OUTER_BOUND('',#12392,.T.);
#7128=FACE_OUTER_BOUND('',#12393,.T.);
#7129=FACE_OUTER_BOUND('',#12394,.T.);
#7130=FACE_OUTER_BOUND('',#12395,.T.);
#7131=FACE_OUTER_BOUND('',#12396,.T.);
#7132=FACE_OUTER_BOUND('',#12397,.T.);
#7133=FACE_OUTER_BOUND('',#12398,.T.);
#7134=FACE_OUTER_BOUND('',#12399,.T.);
#7135=FACE_OUTER_BOUND('',#12400,.T.);
#7136=FACE_OUTER_BOUND('',#12401,.T.);
#7137=FACE_OUTER_BOUND('',#12402,.T.);
#7138=FACE_OUTER_BOUND('',#12403,.T.);
#7139=FACE_OUTER_BOUND('',#12404,.T.);
#7140=FACE_OUTER_BOUND('',#12405,.T.);
#7141=FACE_OUTER_BOUND('',#12406,.T.);
#7142=FACE_OUTER_BOUND('',#12407,.T.);
#7143=FACE_OUTER_BOUND('',#12408,.T.);
#7144=FACE_OUTER_BOUND('',#12409,.T.);
#7145=FACE_OUTER_BOUND('',#12410,.T.);
#7146=FACE_OUTER_BOUND('',#12411,.T.);
#7147=FACE_OUTER_BOUND('',#12412,.T.);
#7148=FACE_OUTER_BOUND('',#12413,.T.);
#7149=FACE_OUTER_BOUND('',#12414,.T.);
#7150=FACE_OUTER_BOUND('',#12415,.T.);
#7151=FACE_OUTER_BOUND('',#12416,.T.);
#7152=FACE_OUTER_BOUND('',#12417,.T.);
#7153=FACE_OUTER_BOUND('',#12418,.T.);
#7154=FACE_OUTER_BOUND('',#12419,.T.);
#7155=FACE_OUTER_BOUND('',#12420,.T.);
#7156=FACE_OUTER_BOUND('',#12421,.T.);
#7157=FACE_OUTER_BOUND('',#12422,.T.);
#7158=FACE_OUTER_BOUND('',#12423,.T.);
#7159=FACE_OUTER_BOUND('',#12424,.T.);
#7160=FACE_OUTER_BOUND('',#12425,.T.);
#7161=FACE_OUTER_BOUND('',#12426,.T.);
#7162=FACE_OUTER_BOUND('',#12427,.T.);
#7163=FACE_OUTER_BOUND('',#12428,.T.);
#7164=FACE_OUTER_BOUND('',#12429,.T.);
#7165=FACE_OUTER_BOUND('',#12430,.T.);
#7166=FACE_OUTER_BOUND('',#12431,.T.);
#7167=FACE_OUTER_BOUND('',#12432,.T.);
#7168=FACE_OUTER_BOUND('',#12433,.T.);
#7169=FACE_OUTER_BOUND('',#12434,.T.);
#7170=FACE_OUTER_BOUND('',#12435,.T.);
#7171=FACE_OUTER_BOUND('',#12436,.T.);
#7172=FACE_OUTER_BOUND('',#12437,.T.);
#7173=FACE_OUTER_BOUND('',#12438,.T.);
#7174=FACE_OUTER_BOUND('',#12439,.T.);
#7175=FACE_OUTER_BOUND('',#12440,.T.);
#7176=FACE_OUTER_BOUND('',#12441,.T.);
#7177=FACE_OUTER_BOUND('',#12442,.T.);
#7178=FACE_OUTER_BOUND('',#12443,.T.);
#7179=FACE_OUTER_BOUND('',#12444,.T.);
#7180=FACE_OUTER_BOUND('',#12445,.T.);
#7181=FACE_OUTER_BOUND('',#12446,.T.);
#7182=FACE_OUTER_BOUND('',#12447,.T.);
#7183=FACE_OUTER_BOUND('',#12448,.T.);
#7184=FACE_OUTER_BOUND('',#12449,.T.);
#7185=FACE_OUTER_BOUND('',#12450,.T.);
#7186=FACE_OUTER_BOUND('',#12451,.T.);
#7187=FACE_OUTER_BOUND('',#12452,.T.);
#7188=FACE_OUTER_BOUND('',#12453,.T.);
#7189=FACE_OUTER_BOUND('',#12454,.T.);
#7190=FACE_OUTER_BOUND('',#12455,.T.);
#7191=FACE_OUTER_BOUND('',#12456,.T.);
#7192=FACE_OUTER_BOUND('',#12457,.T.);
#7193=FACE_OUTER_BOUND('',#12458,.T.);
#7194=FACE_OUTER_BOUND('',#12459,.T.);
#7195=FACE_OUTER_BOUND('',#12460,.T.);
#7196=FACE_OUTER_BOUND('',#12461,.T.);
#7197=FACE_OUTER_BOUND('',#12462,.T.);
#7198=FACE_OUTER_BOUND('',#12463,.T.);
#7199=FACE_OUTER_BOUND('',#12464,.T.);
#7200=FACE_OUTER_BOUND('',#12465,.T.);
#7201=FACE_OUTER_BOUND('',#12466,.T.);
#7202=FACE_OUTER_BOUND('',#12467,.T.);
#7203=FACE_OUTER_BOUND('',#12468,.T.);
#7204=FACE_OUTER_BOUND('',#12469,.T.);
#7205=FACE_OUTER_BOUND('',#12470,.T.);
#7206=FACE_OUTER_BOUND('',#12471,.T.);
#7207=FACE_OUTER_BOUND('',#12472,.T.);
#7208=FACE_OUTER_BOUND('',#12473,.T.);
#7209=FACE_OUTER_BOUND('',#12474,.T.);
#7210=FACE_OUTER_BOUND('',#12475,.T.);
#7211=FACE_OUTER_BOUND('',#12476,.T.);
#7212=FACE_OUTER_BOUND('',#12477,.T.);
#7213=FACE_OUTER_BOUND('',#12478,.T.);
#7214=FACE_OUTER_BOUND('',#12479,.T.);
#7215=FACE_OUTER_BOUND('',#12480,.T.);
#7216=FACE_OUTER_BOUND('',#12481,.T.);
#7217=FACE_OUTER_BOUND('',#12482,.T.);
#7218=FACE_OUTER_BOUND('',#12483,.T.);
#7219=FACE_OUTER_BOUND('',#12484,.T.);
#7220=FACE_OUTER_BOUND('',#12485,.T.);
#7221=FACE_OUTER_BOUND('',#12486,.T.);
#7222=FACE_OUTER_BOUND('',#12487,.T.);
#7223=FACE_OUTER_BOUND('',#12488,.T.);
#7224=FACE_OUTER_BOUND('',#12489,.T.);
#7225=FACE_OUTER_BOUND('',#12490,.T.);
#7226=FACE_OUTER_BOUND('',#12491,.T.);
#7227=FACE_OUTER_BOUND('',#12492,.T.);
#7228=FACE_OUTER_BOUND('',#12493,.T.);
#7229=FACE_OUTER_BOUND('',#12494,.T.);
#7230=FACE_OUTER_BOUND('',#12495,.T.);
#7231=FACE_OUTER_BOUND('',#12496,.T.);
#7232=FACE_OUTER_BOUND('',#12497,.T.);
#7233=FACE_OUTER_BOUND('',#12498,.T.);
#7234=FACE_OUTER_BOUND('',#12499,.T.);
#7235=FACE_OUTER_BOUND('',#12500,.T.);
#7236=FACE_OUTER_BOUND('',#12501,.T.);
#7237=FACE_OUTER_BOUND('',#12502,.T.);
#7238=FACE_OUTER_BOUND('',#12503,.T.);
#7239=FACE_OUTER_BOUND('',#12504,.T.);
#7240=FACE_OUTER_BOUND('',#12505,.T.);
#7241=FACE_OUTER_BOUND('',#12506,.T.);
#7242=FACE_OUTER_BOUND('',#12507,.T.);
#7243=FACE_OUTER_BOUND('',#12508,.T.);
#7244=FACE_OUTER_BOUND('',#12509,.T.);
#7245=FACE_OUTER_BOUND('',#12510,.T.);
#7246=FACE_OUTER_BOUND('',#12511,.T.);
#7247=FACE_OUTER_BOUND('',#12512,.T.);
#7248=FACE_OUTER_BOUND('',#12513,.T.);
#7249=FACE_OUTER_BOUND('',#12514,.T.);
#7250=FACE_OUTER_BOUND('',#12515,.T.);
#7251=FACE_OUTER_BOUND('',#12516,.T.);
#7252=FACE_OUTER_BOUND('',#12517,.T.);
#7253=FACE_OUTER_BOUND('',#12518,.T.);
#7254=FACE_OUTER_BOUND('',#12519,.T.);
#7255=FACE_OUTER_BOUND('',#12520,.T.);
#7256=FACE_OUTER_BOUND('',#12521,.T.);
#7257=FACE_OUTER_BOUND('',#12522,.T.);
#7258=FACE_OUTER_BOUND('',#12523,.T.);
#7259=FACE_OUTER_BOUND('',#12524,.T.);
#7260=FACE_OUTER_BOUND('',#12525,.T.);
#7261=FACE_OUTER_BOUND('',#12526,.T.);
#7262=FACE_OUTER_BOUND('',#12527,.T.);
#7263=FACE_OUTER_BOUND('',#12528,.T.);
#7264=FACE_OUTER_BOUND('',#12529,.T.);
#7265=FACE_OUTER_BOUND('',#12530,.T.);
#7266=FACE_OUTER_BOUND('',#12531,.T.);
#7267=FACE_OUTER_BOUND('',#12532,.T.);
#7268=FACE_OUTER_BOUND('',#12533,.T.);
#7269=FACE_OUTER_BOUND('',#12534,.T.);
#7270=FACE_OUTER_BOUND('',#12535,.T.);
#7271=FACE_OUTER_BOUND('',#12536,.T.);
#7272=FACE_OUTER_BOUND('',#12537,.T.);
#7273=FACE_OUTER_BOUND('',#12538,.T.);
#7274=FACE_OUTER_BOUND('',#12539,.T.);
#7275=FACE_OUTER_BOUND('',#12540,.T.);
#7276=FACE_OUTER_BOUND('',#12541,.T.);
#7277=FACE_OUTER_BOUND('',#12542,.T.);
#7278=FACE_OUTER_BOUND('',#12543,.T.);
#7279=FACE_OUTER_BOUND('',#12544,.T.);
#7280=FACE_OUTER_BOUND('',#12545,.T.);
#7281=FACE_OUTER_BOUND('',#12546,.T.);
#7282=FACE_OUTER_BOUND('',#12547,.T.);
#7283=FACE_OUTER_BOUND('',#12548,.T.);
#7284=FACE_OUTER_BOUND('',#12549,.T.);
#7285=FACE_OUTER_BOUND('',#12550,.T.);
#7286=FACE_OUTER_BOUND('',#12551,.T.);
#7287=FACE_OUTER_BOUND('',#12552,.T.);
#7288=FACE_OUTER_BOUND('',#12553,.T.);
#7289=FACE_OUTER_BOUND('',#12554,.T.);
#7290=FACE_OUTER_BOUND('',#12555,.T.);
#7291=FACE_OUTER_BOUND('',#12556,.T.);
#7292=FACE_OUTER_BOUND('',#12557,.T.);
#7293=FACE_OUTER_BOUND('',#12558,.T.);
#7294=FACE_OUTER_BOUND('',#12559,.T.);
#7295=FACE_OUTER_BOUND('',#12560,.T.);
#7296=FACE_OUTER_BOUND('',#12561,.T.);
#7297=FACE_OUTER_BOUND('',#12562,.T.);
#7298=FACE_OUTER_BOUND('',#12563,.T.);
#7299=FACE_OUTER_BOUND('',#12564,.T.);
#7300=FACE_OUTER_BOUND('',#12565,.T.);
#7301=FACE_OUTER_BOUND('',#12566,.T.);
#7302=FACE_OUTER_BOUND('',#12567,.T.);
#7303=FACE_OUTER_BOUND('',#12568,.T.);
#7304=FACE_OUTER_BOUND('',#12569,.T.);
#7305=FACE_OUTER_BOUND('',#12570,.T.);
#7306=FACE_OUTER_BOUND('',#12571,.T.);
#7307=FACE_OUTER_BOUND('',#12572,.T.);
#7308=FACE_OUTER_BOUND('',#12573,.T.);
#7309=FACE_OUTER_BOUND('',#12574,.T.);
#7310=FACE_OUTER_BOUND('',#12575,.T.);
#7311=FACE_OUTER_BOUND('',#12576,.T.);
#7312=FACE_OUTER_BOUND('',#12577,.T.);
#7313=FACE_OUTER_BOUND('',#12578,.T.);
#7314=FACE_OUTER_BOUND('',#12579,.T.);
#7315=FACE_OUTER_BOUND('',#12580,.T.);
#7316=FACE_OUTER_BOUND('',#12581,.T.);
#7317=FACE_OUTER_BOUND('',#12582,.T.);
#7318=FACE_OUTER_BOUND('',#12583,.T.);
#7319=FACE_OUTER_BOUND('',#12584,.T.);
#7320=FACE_OUTER_BOUND('',#12585,.T.);
#7321=FACE_OUTER_BOUND('',#12586,.T.);
#7322=FACE_OUTER_BOUND('',#12587,.T.);
#7323=FACE_OUTER_BOUND('',#12588,.T.);
#7324=FACE_OUTER_BOUND('',#12589,.T.);
#7325=FACE_OUTER_BOUND('',#12590,.T.);
#7326=FACE_OUTER_BOUND('',#12591,.T.);
#7327=FACE_OUTER_BOUND('',#12592,.T.);
#7328=FACE_OUTER_BOUND('',#12593,.T.);
#7329=FACE_OUTER_BOUND('',#12594,.T.);
#7330=FACE_OUTER_BOUND('',#12595,.T.);
#7331=FACE_OUTER_BOUND('',#12596,.T.);
#7332=FACE_OUTER_BOUND('',#12597,.T.);
#7333=FACE_OUTER_BOUND('',#12598,.T.);
#7334=FACE_OUTER_BOUND('',#12599,.T.);
#7335=FACE_OUTER_BOUND('',#12600,.T.);
#7336=FACE_OUTER_BOUND('',#12601,.T.);
#7337=FACE_OUTER_BOUND('',#12602,.T.);
#7338=FACE_OUTER_BOUND('',#12603,.T.);
#7339=FACE_OUTER_BOUND('',#12604,.T.);
#7340=FACE_OUTER_BOUND('',#12605,.T.);
#7341=FACE_OUTER_BOUND('',#12606,.T.);
#7342=FACE_OUTER_BOUND('',#12607,.T.);
#7343=FACE_OUTER_BOUND('',#12608,.T.);
#7344=FACE_OUTER_BOUND('',#12609,.T.);
#7345=FACE_OUTER_BOUND('',#12610,.T.);
#7346=FACE_OUTER_BOUND('',#12611,.T.);
#7347=FACE_OUTER_BOUND('',#12612,.T.);
#7348=FACE_OUTER_BOUND('',#12613,.T.);
#7349=FACE_OUTER_BOUND('',#12614,.T.);
#7350=FACE_OUTER_BOUND('',#12615,.T.);
#7351=FACE_OUTER_BOUND('',#12616,.T.);
#7352=FACE_OUTER_BOUND('',#12617,.T.);
#7353=FACE_OUTER_BOUND('',#12618,.T.);
#7354=FACE_OUTER_BOUND('',#12619,.T.);
#7355=FACE_OUTER_BOUND('',#12620,.T.);
#7356=FACE_OUTER_BOUND('',#12621,.T.);
#7357=FACE_OUTER_BOUND('',#12622,.T.);
#7358=FACE_OUTER_BOUND('',#12623,.T.);
#7359=FACE_OUTER_BOUND('',#12624,.T.);
#7360=FACE_OUTER_BOUND('',#12625,.T.);
#7361=FACE_OUTER_BOUND('',#12626,.T.);
#7362=FACE_OUTER_BOUND('',#12627,.T.);
#7363=FACE_OUTER_BOUND('',#12628,.T.);
#7364=FACE_OUTER_BOUND('',#12629,.T.);
#7365=FACE_OUTER_BOUND('',#12630,.T.);
#7366=FACE_OUTER_BOUND('',#12631,.T.);
#7367=FACE_OUTER_BOUND('',#12632,.T.);
#7368=FACE_OUTER_BOUND('',#12633,.T.);
#7369=FACE_OUTER_BOUND('',#12634,.T.);
#7370=FACE_OUTER_BOUND('',#12635,.T.);
#7371=FACE_OUTER_BOUND('',#12636,.T.);
#7372=FACE_OUTER_BOUND('',#12637,.T.);
#7373=FACE_OUTER_BOUND('',#12638,.T.);
#7374=FACE_OUTER_BOUND('',#12639,.T.);
#7375=FACE_OUTER_BOUND('',#12640,.T.);
#7376=FACE_OUTER_BOUND('',#12641,.T.);
#7377=FACE_OUTER_BOUND('',#12642,.T.);
#7378=FACE_OUTER_BOUND('',#12643,.T.);
#7379=FACE_OUTER_BOUND('',#12644,.T.);
#7380=FACE_OUTER_BOUND('',#12645,.T.);
#7381=FACE_OUTER_BOUND('',#12646,.T.);
#7382=FACE_OUTER_BOUND('',#12647,.T.);
#7383=FACE_OUTER_BOUND('',#12648,.T.);
#7384=FACE_OUTER_BOUND('',#12649,.T.);
#7385=FACE_OUTER_BOUND('',#12650,.T.);
#7386=FACE_OUTER_BOUND('',#12651,.T.);
#7387=FACE_OUTER_BOUND('',#12652,.T.);
#7388=FACE_OUTER_BOUND('',#12653,.T.);
#7389=FACE_OUTER_BOUND('',#12654,.T.);
#7390=FACE_OUTER_BOUND('',#12655,.T.);
#7391=FACE_OUTER_BOUND('',#12656,.T.);
#7392=FACE_OUTER_BOUND('',#12657,.T.);
#7393=FACE_OUTER_BOUND('',#12658,.T.);
#7394=FACE_OUTER_BOUND('',#12659,.T.);
#7395=FACE_OUTER_BOUND('',#12660,.T.);
#7396=FACE_OUTER_BOUND('',#12661,.T.);
#7397=FACE_OUTER_BOUND('',#12662,.T.);
#7398=FACE_OUTER_BOUND('',#12663,.T.);
#7399=FACE_OUTER_BOUND('',#12664,.T.);
#7400=FACE_OUTER_BOUND('',#12665,.T.);
#7401=FACE_OUTER_BOUND('',#12666,.T.);
#7402=FACE_OUTER_BOUND('',#12667,.T.);
#7403=FACE_OUTER_BOUND('',#12668,.T.);
#7404=FACE_OUTER_BOUND('',#12669,.T.);
#7405=FACE_OUTER_BOUND('',#12670,.T.);
#7406=FACE_OUTER_BOUND('',#12671,.T.);
#7407=FACE_OUTER_BOUND('',#12672,.T.);
#7408=FACE_OUTER_BOUND('',#12673,.T.);
#7409=FACE_OUTER_BOUND('',#12674,.T.);
#7410=FACE_OUTER_BOUND('',#12675,.T.);
#7411=FACE_OUTER_BOUND('',#12676,.T.);
#7412=FACE_OUTER_BOUND('',#12677,.T.);
#7413=FACE_OUTER_BOUND('',#12678,.T.);
#7414=FACE_OUTER_BOUND('',#12679,.T.);
#7415=FACE_OUTER_BOUND('',#12680,.T.);
#7416=FACE_OUTER_BOUND('',#12681,.T.);
#7417=FACE_OUTER_BOUND('',#12682,.T.);
#7418=FACE_OUTER_BOUND('',#12683,.T.);
#7419=FACE_OUTER_BOUND('',#12684,.T.);
#7420=FACE_OUTER_BOUND('',#12685,.T.);
#7421=FACE_OUTER_BOUND('',#12686,.T.);
#7422=FACE_OUTER_BOUND('',#12687,.T.);
#7423=FACE_OUTER_BOUND('',#12688,.T.);
#7424=FACE_OUTER_BOUND('',#12689,.T.);
#7425=FACE_OUTER_BOUND('',#12690,.T.);
#7426=FACE_OUTER_BOUND('',#12691,.T.);
#7427=FACE_OUTER_BOUND('',#12692,.T.);
#7428=FACE_OUTER_BOUND('',#12693,.T.);
#7429=FACE_OUTER_BOUND('',#12694,.T.);
#7430=FACE_OUTER_BOUND('',#12695,.T.);
#7431=FACE_OUTER_BOUND('',#12696,.T.);
#7432=FACE_OUTER_BOUND('',#12697,.T.);
#7433=FACE_OUTER_BOUND('',#12698,.T.);
#7434=FACE_OUTER_BOUND('',#12699,.T.);
#7435=FACE_OUTER_BOUND('',#12700,.T.);
#7436=FACE_OUTER_BOUND('',#12701,.T.);
#7437=FACE_OUTER_BOUND('',#12702,.T.);
#7438=FACE_OUTER_BOUND('',#12703,.T.);
#7439=FACE_OUTER_BOUND('',#12704,.T.);
#7440=FACE_OUTER_BOUND('',#12705,.T.);
#7441=FACE_OUTER_BOUND('',#12706,.T.);
#7442=FACE_OUTER_BOUND('',#12707,.T.);
#7443=FACE_OUTER_BOUND('',#12708,.T.);
#7444=FACE_OUTER_BOUND('',#12709,.T.);
#7445=FACE_OUTER_BOUND('',#12710,.T.);
#7446=FACE_OUTER_BOUND('',#12711,.T.);
#7447=FACE_OUTER_BOUND('',#12712,.T.);
#7448=FACE_OUTER_BOUND('',#12713,.T.);
#7449=FACE_OUTER_BOUND('',#12714,.T.);
#7450=FACE_OUTER_BOUND('',#12715,.T.);
#7451=FACE_OUTER_BOUND('',#12716,.T.);
#7452=FACE_OUTER_BOUND('',#12717,.T.);
#7453=FACE_OUTER_BOUND('',#12718,.T.);
#7454=FACE_OUTER_BOUND('',#12719,.T.);
#7455=FACE_OUTER_BOUND('',#12720,.T.);
#7456=FACE_OUTER_BOUND('',#12721,.T.);
#7457=FACE_OUTER_BOUND('',#12722,.T.);
#7458=FACE_OUTER_BOUND('',#12723,.T.);
#7459=FACE_OUTER_BOUND('',#12724,.T.);
#7460=FACE_OUTER_BOUND('',#12725,.T.);
#7461=FACE_OUTER_BOUND('',#12726,.T.);
#7462=FACE_OUTER_BOUND('',#12727,.T.);
#7463=FACE_OUTER_BOUND('',#12728,.T.);
#7464=FACE_OUTER_BOUND('',#12729,.T.);
#7465=FACE_OUTER_BOUND('',#12730,.T.);
#7466=FACE_OUTER_BOUND('',#12731,.T.);
#7467=FACE_OUTER_BOUND('',#12732,.T.);
#7468=FACE_OUTER_BOUND('',#12733,.T.);
#7469=FACE_OUTER_BOUND('',#12734,.T.);
#7470=FACE_OUTER_BOUND('',#12735,.T.);
#7471=FACE_OUTER_BOUND('',#12736,.T.);
#7472=FACE_OUTER_BOUND('',#12737,.T.);
#7473=FACE_OUTER_BOUND('',#12738,.T.);
#7474=FACE_OUTER_BOUND('',#12739,.T.);
#7475=FACE_OUTER_BOUND('',#12740,.T.);
#7476=FACE_OUTER_BOUND('',#12741,.T.);
#7477=FACE_OUTER_BOUND('',#12742,.T.);
#7478=FACE_OUTER_BOUND('',#12743,.T.);
#7479=FACE_OUTER_BOUND('',#12744,.T.);
#7480=FACE_OUTER_BOUND('',#12745,.T.);
#7481=FACE_OUTER_BOUND('',#12746,.T.);
#7482=FACE_OUTER_BOUND('',#12747,.T.);
#7483=FACE_OUTER_BOUND('',#12748,.T.);
#7484=FACE_OUTER_BOUND('',#12749,.T.);
#7485=FACE_OUTER_BOUND('',#12750,.T.);
#7486=FACE_OUTER_BOUND('',#12751,.T.);
#7487=FACE_OUTER_BOUND('',#12752,.T.);
#7488=FACE_OUTER_BOUND('',#12753,.T.);
#7489=FACE_OUTER_BOUND('',#12754,.T.);
#7490=FACE_OUTER_BOUND('',#12755,.T.);
#7491=FACE_OUTER_BOUND('',#12756,.T.);
#7492=FACE_OUTER_BOUND('',#12757,.T.);
#7493=FACE_OUTER_BOUND('',#12758,.T.);
#7494=FACE_OUTER_BOUND('',#12759,.T.);
#7495=FACE_OUTER_BOUND('',#12760,.T.);
#7496=FACE_OUTER_BOUND('',#12761,.T.);
#7497=FACE_OUTER_BOUND('',#12762,.T.);
#7498=FACE_OUTER_BOUND('',#12763,.T.);
#7499=FACE_OUTER_BOUND('',#12764,.T.);
#7500=FACE_OUTER_BOUND('',#12765,.T.);
#7501=FACE_OUTER_BOUND('',#12766,.T.);
#7502=FACE_OUTER_BOUND('',#12767,.T.);
#7503=FACE_OUTER_BOUND('',#12768,.T.);
#7504=FACE_OUTER_BOUND('',#12769,.T.);
#7505=FACE_OUTER_BOUND('',#12770,.T.);
#7506=FACE_OUTER_BOUND('',#12771,.T.);
#7507=FACE_OUTER_BOUND('',#12772,.T.);
#7508=FACE_OUTER_BOUND('',#12773,.T.);
#7509=FACE_OUTER_BOUND('',#12774,.T.);
#7510=FACE_OUTER_BOUND('',#12775,.T.);
#7511=FACE_OUTER_BOUND('',#12776,.T.);
#7512=FACE_OUTER_BOUND('',#12777,.T.);
#7513=FACE_OUTER_BOUND('',#12778,.T.);
#7514=FACE_OUTER_BOUND('',#12779,.T.);
#7515=FACE_OUTER_BOUND('',#12780,.T.);
#7516=FACE_OUTER_BOUND('',#12781,.T.);
#7517=FACE_OUTER_BOUND('',#12782,.T.);
#7518=FACE_OUTER_BOUND('',#12783,.T.);
#7519=FACE_OUTER_BOUND('',#12784,.T.);
#7520=FACE_OUTER_BOUND('',#12785,.T.);
#7521=FACE_OUTER_BOUND('',#12786,.T.);
#7522=FACE_OUTER_BOUND('',#12787,.T.);
#7523=FACE_OUTER_BOUND('',#12788,.T.);
#7524=FACE_OUTER_BOUND('',#12789,.T.);
#7525=FACE_OUTER_BOUND('',#12790,.T.);
#7526=FACE_OUTER_BOUND('',#12791,.T.);
#7527=FACE_OUTER_BOUND('',#12792,.T.);
#7528=FACE_OUTER_BOUND('',#12793,.T.);
#7529=FACE_OUTER_BOUND('',#12794,.T.);
#7530=FACE_OUTER_BOUND('',#12795,.T.);
#7531=FACE_OUTER_BOUND('',#12796,.T.);
#7532=FACE_OUTER_BOUND('',#12797,.T.);
#7533=FACE_OUTER_BOUND('',#12798,.T.);
#7534=FACE_OUTER_BOUND('',#12799,.T.);
#7535=FACE_OUTER_BOUND('',#12800,.T.);
#7536=FACE_OUTER_BOUND('',#12801,.T.);
#7537=FACE_OUTER_BOUND('',#12802,.T.);
#7538=FACE_OUTER_BOUND('',#12803,.T.);
#7539=FACE_OUTER_BOUND('',#12804,.T.);
#7540=FACE_OUTER_BOUND('',#12805,.T.);
#7541=FACE_OUTER_BOUND('',#12806,.T.);
#7542=FACE_OUTER_BOUND('',#12807,.T.);
#7543=FACE_OUTER_BOUND('',#12808,.T.);
#7544=FACE_OUTER_BOUND('',#12809,.T.);
#7545=FACE_OUTER_BOUND('',#12810,.T.);
#7546=FACE_OUTER_BOUND('',#12811,.T.);
#7547=FACE_OUTER_BOUND('',#12812,.T.);
#7548=FACE_OUTER_BOUND('',#12813,.T.);
#7549=FACE_OUTER_BOUND('',#12814,.T.);
#7550=FACE_OUTER_BOUND('',#12815,.T.);
#7551=FACE_OUTER_BOUND('',#12816,.T.);
#7552=FACE_OUTER_BOUND('',#12817,.T.);
#7553=FACE_OUTER_BOUND('',#12818,.T.);
#7554=FACE_OUTER_BOUND('',#12819,.T.);
#7555=FACE_OUTER_BOUND('',#12820,.T.);
#7556=FACE_OUTER_BOUND('',#12821,.T.);
#7557=FACE_OUTER_BOUND('',#12822,.T.);
#7558=FACE_OUTER_BOUND('',#12823,.T.);
#7559=FACE_OUTER_BOUND('',#12824,.T.);
#7560=FACE_OUTER_BOUND('',#12825,.T.);
#7561=FACE_OUTER_BOUND('',#12826,.T.);
#7562=FACE_OUTER_BOUND('',#12827,.T.);
#7563=FACE_OUTER_BOUND('',#12828,.T.);
#7564=FACE_OUTER_BOUND('',#12829,.T.);
#7565=FACE_OUTER_BOUND('',#12830,.T.);
#7566=FACE_OUTER_BOUND('',#12831,.T.);
#7567=FACE_OUTER_BOUND('',#12832,.T.);
#7568=FACE_OUTER_BOUND('',#12833,.T.);
#7569=FACE_OUTER_BOUND('',#12834,.T.);
#7570=FACE_OUTER_BOUND('',#12835,.T.);
#7571=FACE_OUTER_BOUND('',#12836,.T.);
#7572=FACE_OUTER_BOUND('',#12837,.T.);
#7573=FACE_OUTER_BOUND('',#12838,.T.);
#7574=FACE_OUTER_BOUND('',#12839,.T.);
#7575=FACE_OUTER_BOUND('',#12840,.T.);
#7576=FACE_OUTER_BOUND('',#12841,.T.);
#7577=FACE_OUTER_BOUND('',#12842,.T.);
#7578=FACE_OUTER_BOUND('',#12843,.T.);
#7579=FACE_OUTER_BOUND('',#12844,.T.);
#7580=FACE_OUTER_BOUND('',#12845,.T.);
#7581=FACE_OUTER_BOUND('',#12846,.T.);
#7582=FACE_OUTER_BOUND('',#12847,.T.);
#7583=FACE_OUTER_BOUND('',#12848,.T.);
#7584=FACE_OUTER_BOUND('',#12849,.T.);
#7585=FACE_OUTER_BOUND('',#12850,.T.);
#7586=FACE_OUTER_BOUND('',#12851,.T.);
#7587=FACE_OUTER_BOUND('',#12852,.T.);
#7588=FACE_OUTER_BOUND('',#12853,.T.);
#7589=FACE_OUTER_BOUND('',#12854,.T.);
#7590=FACE_OUTER_BOUND('',#12855,.T.);
#7591=FACE_OUTER_BOUND('',#12856,.T.);
#7592=FACE_OUTER_BOUND('',#12857,.T.);
#7593=FACE_OUTER_BOUND('',#12858,.T.);
#7594=FACE_OUTER_BOUND('',#12859,.T.);
#7595=FACE_OUTER_BOUND('',#12860,.T.);
#7596=FACE_OUTER_BOUND('',#12861,.T.);
#7597=FACE_OUTER_BOUND('',#12862,.T.);
#7598=FACE_OUTER_BOUND('',#12863,.T.);
#7599=FACE_OUTER_BOUND('',#12864,.T.);
#7600=FACE_OUTER_BOUND('',#12865,.T.);
#7601=FACE_OUTER_BOUND('',#12866,.T.);
#7602=FACE_OUTER_BOUND('',#12867,.T.);
#7603=FACE_OUTER_BOUND('',#12868,.T.);
#7604=FACE_OUTER_BOUND('',#12869,.T.);
#7605=FACE_OUTER_BOUND('',#12870,.T.);
#7606=FACE_OUTER_BOUND('',#12871,.T.);
#7607=FACE_OUTER_BOUND('',#12872,.T.);
#7608=FACE_OUTER_BOUND('',#12873,.T.);
#7609=FACE_OUTER_BOUND('',#12874,.T.);
#7610=FACE_OUTER_BOUND('',#12875,.T.);
#7611=FACE_OUTER_BOUND('',#12876,.T.);
#7612=FACE_OUTER_BOUND('',#12877,.T.);
#7613=FACE_OUTER_BOUND('',#12878,.T.);
#7614=FACE_OUTER_BOUND('',#12879,.T.);
#7615=FACE_OUTER_BOUND('',#12880,.T.);
#7616=FACE_OUTER_BOUND('',#12881,.T.);
#7617=FACE_OUTER_BOUND('',#12882,.T.);
#7618=FACE_OUTER_BOUND('',#12883,.T.);
#7619=FACE_OUTER_BOUND('',#12884,.T.);
#7620=FACE_OUTER_BOUND('',#12885,.T.);
#7621=FACE_OUTER_BOUND('',#12886,.T.);
#7622=FACE_OUTER_BOUND('',#12887,.T.);
#7623=FACE_OUTER_BOUND('',#12888,.T.);
#7624=FACE_OUTER_BOUND('',#12889,.T.);
#7625=FACE_OUTER_BOUND('',#12890,.T.);
#7626=FACE_OUTER_BOUND('',#12891,.T.);
#7627=FACE_OUTER_BOUND('',#12892,.T.);
#7628=FACE_OUTER_BOUND('',#12893,.T.);
#7629=FACE_OUTER_BOUND('',#12894,.T.);
#7630=FACE_OUTER_BOUND('',#12895,.T.);
#7631=FACE_OUTER_BOUND('',#12896,.T.);
#7632=FACE_OUTER_BOUND('',#12897,.T.);
#7633=FACE_OUTER_BOUND('',#12898,.T.);
#7634=FACE_OUTER_BOUND('',#12899,.T.);
#7635=FACE_OUTER_BOUND('',#12900,.T.);
#7636=FACE_OUTER_BOUND('',#12901,.T.);
#7637=FACE_OUTER_BOUND('',#12902,.T.);
#7638=FACE_OUTER_BOUND('',#12903,.T.);
#7639=FACE_OUTER_BOUND('',#12904,.T.);
#7640=FACE_OUTER_BOUND('',#12905,.T.);
#7641=FACE_OUTER_BOUND('',#12906,.T.);
#7642=FACE_OUTER_BOUND('',#12907,.T.);
#7643=FACE_OUTER_BOUND('',#12908,.T.);
#7644=FACE_OUTER_BOUND('',#12909,.T.);
#7645=FACE_OUTER_BOUND('',#12910,.T.);
#7646=FACE_OUTER_BOUND('',#12911,.T.);
#7647=FACE_OUTER_BOUND('',#12912,.T.);
#7648=FACE_OUTER_BOUND('',#12913,.T.);
#7649=FACE_OUTER_BOUND('',#12914,.T.);
#7650=FACE_OUTER_BOUND('',#12915,.T.);
#7651=FACE_OUTER_BOUND('',#12916,.T.);
#7652=FACE_OUTER_BOUND('',#12917,.T.);
#7653=FACE_OUTER_BOUND('',#12918,.T.);
#7654=FACE_OUTER_BOUND('',#12919,.T.);
#7655=FACE_OUTER_BOUND('',#12920,.T.);
#7656=FACE_OUTER_BOUND('',#12921,.T.);
#7657=FACE_OUTER_BOUND('',#12922,.T.);
#7658=FACE_OUTER_BOUND('',#12923,.T.);
#7659=FACE_OUTER_BOUND('',#12924,.T.);
#7660=FACE_OUTER_BOUND('',#12925,.T.);
#7661=FACE_OUTER_BOUND('',#12926,.T.);
#7662=FACE_OUTER_BOUND('',#12927,.T.);
#7663=FACE_OUTER_BOUND('',#12928,.T.);
#7664=FACE_OUTER_BOUND('',#12929,.T.);
#7665=FACE_OUTER_BOUND('',#12930,.T.);
#7666=FACE_OUTER_BOUND('',#12931,.T.);
#7667=FACE_OUTER_BOUND('',#12932,.T.);
#7668=FACE_OUTER_BOUND('',#12933,.T.);
#7669=FACE_OUTER_BOUND('',#12934,.T.);
#7670=FACE_OUTER_BOUND('',#12935,.T.);
#7671=FACE_OUTER_BOUND('',#12936,.T.);
#7672=FACE_OUTER_BOUND('',#12937,.T.);
#7673=FACE_OUTER_BOUND('',#12938,.T.);
#7674=FACE_OUTER_BOUND('',#12939,.T.);
#7675=FACE_OUTER_BOUND('',#12940,.T.);
#7676=FACE_OUTER_BOUND('',#12941,.T.);
#7677=FACE_OUTER_BOUND('',#12942,.T.);
#7678=FACE_OUTER_BOUND('',#12943,.T.);
#7679=FACE_OUTER_BOUND('',#12944,.T.);
#7680=FACE_OUTER_BOUND('',#12945,.T.);
#7681=FACE_OUTER_BOUND('',#12946,.T.);
#7682=FACE_OUTER_BOUND('',#12947,.T.);
#7683=FACE_OUTER_BOUND('',#12948,.T.);
#7684=FACE_OUTER_BOUND('',#12949,.T.);
#7685=FACE_OUTER_BOUND('',#12950,.T.);
#7686=FACE_OUTER_BOUND('',#12951,.T.);
#7687=FACE_OUTER_BOUND('',#12952,.T.);
#7688=FACE_OUTER_BOUND('',#12953,.T.);
#7689=FACE_OUTER_BOUND('',#12954,.T.);
#7690=FACE_OUTER_BOUND('',#12955,.T.);
#7691=FACE_OUTER_BOUND('',#12956,.T.);
#7692=FACE_OUTER_BOUND('',#12957,.T.);
#7693=FACE_OUTER_BOUND('',#12958,.T.);
#7694=FACE_OUTER_BOUND('',#12959,.T.);
#7695=FACE_OUTER_BOUND('',#12960,.T.);
#7696=FACE_OUTER_BOUND('',#12961,.T.);
#7697=FACE_OUTER_BOUND('',#12962,.T.);
#7698=FACE_OUTER_BOUND('',#12963,.T.);
#7699=FACE_OUTER_BOUND('',#12964,.T.);
#7700=FACE_OUTER_BOUND('',#12965,.T.);
#7701=FACE_OUTER_BOUND('',#12966,.T.);
#7702=FACE_OUTER_BOUND('',#12967,.T.);
#7703=FACE_OUTER_BOUND('',#12968,.T.);
#7704=FACE_OUTER_BOUND('',#12969,.T.);
#7705=FACE_OUTER_BOUND('',#12970,.T.);
#7706=FACE_OUTER_BOUND('',#12971,.T.);
#7707=FACE_OUTER_BOUND('',#12972,.T.);
#7708=FACE_OUTER_BOUND('',#12973,.T.);
#7709=FACE_OUTER_BOUND('',#12974,.T.);
#7710=FACE_OUTER_BOUND('',#12975,.T.);
#7711=FACE_OUTER_BOUND('',#12976,.T.);
#7712=FACE_OUTER_BOUND('',#12977,.T.);
#7713=FACE_OUTER_BOUND('',#12978,.T.);
#7714=FACE_OUTER_BOUND('',#12979,.T.);
#7715=FACE_OUTER_BOUND('',#12980,.T.);
#7716=FACE_OUTER_BOUND('',#12981,.T.);
#7717=FACE_OUTER_BOUND('',#12982,.T.);
#7718=FACE_OUTER_BOUND('',#12983,.T.);
#7719=FACE_OUTER_BOUND('',#12984,.T.);
#7720=FACE_OUTER_BOUND('',#12985,.T.);
#7721=FACE_OUTER_BOUND('',#12986,.T.);
#7722=FACE_OUTER_BOUND('',#12987,.T.);
#7723=FACE_OUTER_BOUND('',#12988,.T.);
#7724=FACE_OUTER_BOUND('',#12989,.T.);
#7725=FACE_OUTER_BOUND('',#12990,.T.);
#7726=FACE_OUTER_BOUND('',#12991,.T.);
#7727=FACE_OUTER_BOUND('',#12992,.T.);
#7728=FACE_OUTER_BOUND('',#12993,.T.);
#7729=FACE_OUTER_BOUND('',#12994,.T.);
#7730=FACE_OUTER_BOUND('',#12995,.T.);
#7731=FACE_OUTER_BOUND('',#12996,.T.);
#7732=FACE_OUTER_BOUND('',#12997,.T.);
#7733=FACE_OUTER_BOUND('',#12998,.T.);
#7734=FACE_OUTER_BOUND('',#12999,.T.);
#7735=FACE_OUTER_BOUND('',#13000,.T.);
#7736=FACE_OUTER_BOUND('',#13001,.T.);
#7737=FACE_OUTER_BOUND('',#13002,.T.);
#7738=FACE_OUTER_BOUND('',#13003,.T.);
#7739=FACE_OUTER_BOUND('',#13004,.T.);
#7740=FACE_OUTER_BOUND('',#13005,.T.);
#7741=FACE_OUTER_BOUND('',#13006,.T.);
#7742=FACE_OUTER_BOUND('',#13007,.T.);
#7743=FACE_OUTER_BOUND('',#13008,.T.);
#7744=FACE_OUTER_BOUND('',#13009,.T.);
#7745=FACE_OUTER_BOUND('',#13010,.T.);
#7746=FACE_OUTER_BOUND('',#13011,.T.);
#7747=FACE_OUTER_BOUND('',#13012,.T.);
#7748=FACE_OUTER_BOUND('',#13013,.T.);
#7749=FACE_OUTER_BOUND('',#13014,.T.);
#7750=FACE_OUTER_BOUND('',#13015,.T.);
#7751=FACE_OUTER_BOUND('',#13016,.T.);
#7752=FACE_OUTER_BOUND('',#13017,.T.);
#7753=FACE_OUTER_BOUND('',#13018,.T.);
#7754=FACE_OUTER_BOUND('',#13019,.T.);
#7755=FACE_OUTER_BOUND('',#13020,.T.);
#7756=FACE_OUTER_BOUND('',#13021,.T.);
#7757=FACE_OUTER_BOUND('',#13022,.T.);
#7758=FACE_OUTER_BOUND('',#13023,.T.);
#7759=FACE_OUTER_BOUND('',#13024,.T.);
#7760=FACE_OUTER_BOUND('',#13025,.T.);
#7761=FACE_OUTER_BOUND('',#13026,.T.);
#7762=FACE_OUTER_BOUND('',#13027,.T.);
#7763=FACE_OUTER_BOUND('',#13028,.T.);
#7764=FACE_OUTER_BOUND('',#13029,.T.);
#7765=FACE_OUTER_BOUND('',#13030,.T.);
#7766=FACE_OUTER_BOUND('',#13031,.T.);
#7767=FACE_OUTER_BOUND('',#13032,.T.);
#7768=FACE_OUTER_BOUND('',#13033,.T.);
#7769=FACE_OUTER_BOUND('',#13034,.T.);
#7770=FACE_OUTER_BOUND('',#13035,.T.);
#7771=FACE_OUTER_BOUND('',#13036,.T.);
#7772=FACE_OUTER_BOUND('',#13037,.T.);
#7773=FACE_OUTER_BOUND('',#13038,.T.);
#7774=FACE_OUTER_BOUND('',#13039,.T.);
#7775=FACE_OUTER_BOUND('',#13040,.T.);
#7776=FACE_OUTER_BOUND('',#13041,.T.);
#7777=FACE_OUTER_BOUND('',#13042,.T.);
#7778=FACE_OUTER_BOUND('',#13043,.T.);
#7779=FACE_OUTER_BOUND('',#13044,.T.);
#7780=FACE_OUTER_BOUND('',#13045,.T.);
#7781=FACE_OUTER_BOUND('',#13046,.T.);
#7782=FACE_OUTER_BOUND('',#13047,.T.);
#7783=FACE_OUTER_BOUND('',#13048,.T.);
#7784=FACE_OUTER_BOUND('',#13049,.T.);
#7785=FACE_OUTER_BOUND('',#13050,.T.);
#7786=FACE_OUTER_BOUND('',#13051,.T.);
#7787=FACE_OUTER_BOUND('',#13052,.T.);
#7788=FACE_OUTER_BOUND('',#13053,.T.);
#7789=FACE_OUTER_BOUND('',#13054,.T.);
#7790=FACE_OUTER_BOUND('',#13055,.T.);
#7791=FACE_OUTER_BOUND('',#13056,.T.);
#7792=FACE_OUTER_BOUND('',#13057,.T.);
#7793=FACE_OUTER_BOUND('',#13058,.T.);
#7794=FACE_OUTER_BOUND('',#13059,.T.);
#7795=FACE_OUTER_BOUND('',#13060,.T.);
#7796=FACE_OUTER_BOUND('',#13061,.T.);
#7797=FACE_OUTER_BOUND('',#13062,.T.);
#7798=FACE_OUTER_BOUND('',#13063,.T.);
#7799=FACE_OUTER_BOUND('',#13064,.T.);
#7800=FACE_OUTER_BOUND('',#13065,.T.);
#7801=FACE_OUTER_BOUND('',#13066,.T.);
#7802=FACE_OUTER_BOUND('',#13067,.T.);
#7803=FACE_OUTER_BOUND('',#13068,.T.);
#7804=FACE_OUTER_BOUND('',#13069,.T.);
#7805=FACE_OUTER_BOUND('',#13070,.T.);
#7806=FACE_OUTER_BOUND('',#13071,.T.);
#7807=FACE_OUTER_BOUND('',#13072,.T.);
#7808=FACE_OUTER_BOUND('',#13073,.T.);
#7809=FACE_OUTER_BOUND('',#13074,.T.);
#7810=FACE_OUTER_BOUND('',#13075,.T.);
#7811=FACE_OUTER_BOUND('',#13076,.T.);
#7812=FACE_OUTER_BOUND('',#13077,.T.);
#7813=FACE_OUTER_BOUND('',#13078,.T.);
#7814=FACE_OUTER_BOUND('',#13079,.T.);
#7815=FACE_OUTER_BOUND('',#13080,.T.);
#7816=FACE_OUTER_BOUND('',#13081,.T.);
#7817=FACE_OUTER_BOUND('',#13082,.T.);
#7818=FACE_OUTER_BOUND('',#13083,.T.);
#7819=FACE_OUTER_BOUND('',#13084,.T.);
#7820=FACE_OUTER_BOUND('',#13085,.T.);
#7821=FACE_OUTER_BOUND('',#13086,.T.);
#7822=FACE_OUTER_BOUND('',#13087,.T.);
#7823=FACE_OUTER_BOUND('',#13088,.T.);
#7824=FACE_OUTER_BOUND('',#13089,.T.);
#7825=FACE_OUTER_BOUND('',#13090,.T.);
#7826=FACE_OUTER_BOUND('',#13091,.T.);
#7827=FACE_OUTER_BOUND('',#13092,.T.);
#7828=FACE_OUTER_BOUND('',#13093,.T.);
#7829=FACE_OUTER_BOUND('',#13094,.T.);
#7830=FACE_OUTER_BOUND('',#13095,.T.);
#7831=FACE_OUTER_BOUND('',#13096,.T.);
#7832=FACE_OUTER_BOUND('',#13097,.T.);
#7833=FACE_OUTER_BOUND('',#13098,.T.);
#7834=FACE_OUTER_BOUND('',#13099,.T.);
#7835=FACE_OUTER_BOUND('',#13100,.T.);
#7836=FACE_OUTER_BOUND('',#13101,.T.);
#7837=FACE_OUTER_BOUND('',#13102,.T.);
#7838=FACE_OUTER_BOUND('',#13103,.T.);
#7839=FACE_OUTER_BOUND('',#13104,.T.);
#7840=FACE_OUTER_BOUND('',#13105,.T.);
#7841=FACE_OUTER_BOUND('',#13106,.T.);
#7842=FACE_OUTER_BOUND('',#13107,.T.);
#7843=FACE_OUTER_BOUND('',#13108,.T.);
#7844=FACE_OUTER_BOUND('',#13109,.T.);
#7845=FACE_OUTER_BOUND('',#13110,.T.);
#7846=FACE_OUTER_BOUND('',#13111,.T.);
#7847=FACE_OUTER_BOUND('',#13112,.T.);
#7848=FACE_OUTER_BOUND('',#13113,.T.);
#7849=FACE_OUTER_BOUND('',#13114,.T.);
#7850=FACE_OUTER_BOUND('',#13115,.T.);
#7851=FACE_OUTER_BOUND('',#13116,.T.);
#7852=FACE_OUTER_BOUND('',#13117,.T.);
#7853=FACE_OUTER_BOUND('',#13118,.T.);
#7854=FACE_OUTER_BOUND('',#13119,.T.);
#7855=FACE_OUTER_BOUND('',#13120,.T.);
#7856=FACE_OUTER_BOUND('',#13121,.T.);
#7857=FACE_OUTER_BOUND('',#13122,.T.);
#7858=FACE_OUTER_BOUND('',#13123,.T.);
#7859=FACE_OUTER_BOUND('',#13124,.T.);
#7860=FACE_OUTER_BOUND('',#13125,.T.);
#7861=FACE_OUTER_BOUND('',#13126,.T.);
#7862=FACE_OUTER_BOUND('',#13127,.T.);
#7863=FACE_OUTER_BOUND('',#13128,.T.);
#7864=FACE_OUTER_BOUND('',#13129,.T.);
#7865=FACE_OUTER_BOUND('',#13130,.T.);
#7866=FACE_OUTER_BOUND('',#13131,.T.);
#7867=FACE_OUTER_BOUND('',#13132,.T.);
#7868=FACE_OUTER_BOUND('',#13133,.T.);
#7869=FACE_OUTER_BOUND('',#13134,.T.);
#7870=FACE_OUTER_BOUND('',#13135,.T.);
#7871=FACE_OUTER_BOUND('',#13136,.T.);
#7872=FACE_OUTER_BOUND('',#13137,.T.);
#7873=FACE_OUTER_BOUND('',#13138,.T.);
#7874=FACE_OUTER_BOUND('',#13139,.T.);
#7875=FACE_OUTER_BOUND('',#13140,.T.);
#7876=FACE_OUTER_BOUND('',#13141,.T.);
#7877=FACE_OUTER_BOUND('',#13142,.T.);
#7878=FACE_OUTER_BOUND('',#13143,.T.);
#7879=FACE_OUTER_BOUND('',#13144,.T.);
#7880=FACE_OUTER_BOUND('',#13145,.T.);
#7881=FACE_OUTER_BOUND('',#13146,.T.);
#7882=FACE_OUTER_BOUND('',#13147,.T.);
#7883=FACE_OUTER_BOUND('',#13148,.T.);
#7884=FACE_OUTER_BOUND('',#13149,.T.);
#7885=FACE_OUTER_BOUND('',#13150,.T.);
#7886=FACE_OUTER_BOUND('',#13151,.T.);
#7887=FACE_OUTER_BOUND('',#13152,.T.);
#7888=FACE_OUTER_BOUND('',#13153,.T.);
#7889=FACE_OUTER_BOUND('',#13154,.T.);
#7890=FACE_OUTER_BOUND('',#13155,.T.);
#7891=FACE_OUTER_BOUND('',#13156,.T.);
#7892=FACE_OUTER_BOUND('',#13157,.T.);
#7893=FACE_OUTER_BOUND('',#13158,.T.);
#7894=FACE_OUTER_BOUND('',#13159,.T.);
#7895=FACE_OUTER_BOUND('',#13160,.T.);
#7896=FACE_OUTER_BOUND('',#13161,.T.);
#7897=FACE_OUTER_BOUND('',#13162,.T.);
#7898=FACE_OUTER_BOUND('',#13163,.T.);
#7899=FACE_OUTER_BOUND('',#13164,.T.);
#7900=FACE_OUTER_BOUND('',#13165,.T.);
#7901=FACE_OUTER_BOUND('',#13166,.T.);
#7902=FACE_OUTER_BOUND('',#13167,.T.);
#7903=FACE_OUTER_BOUND('',#13168,.T.);
#7904=FACE_OUTER_BOUND('',#13169,.T.);
#7905=FACE_OUTER_BOUND('',#13170,.T.);
#7906=FACE_OUTER_BOUND('',#13171,.T.);
#7907=FACE_OUTER_BOUND('',#13172,.T.);
#7908=FACE_OUTER_BOUND('',#13173,.T.);
#7909=FACE_OUTER_BOUND('',#13174,.T.);
#7910=FACE_OUTER_BOUND('',#13175,.T.);
#7911=FACE_OUTER_BOUND('',#13176,.T.);
#7912=FACE_OUTER_BOUND('',#13177,.T.);
#7913=FACE_OUTER_BOUND('',#13178,.T.);
#7914=FACE_OUTER_BOUND('',#13179,.T.);
#7915=FACE_OUTER_BOUND('',#13180,.T.);
#7916=FACE_OUTER_BOUND('',#13181,.T.);
#7917=FACE_OUTER_BOUND('',#13182,.T.);
#7918=FACE_OUTER_BOUND('',#13183,.T.);
#7919=FACE_OUTER_BOUND('',#13184,.T.);
#7920=FACE_OUTER_BOUND('',#13185,.T.);
#7921=FACE_OUTER_BOUND('',#13186,.T.);
#7922=FACE_OUTER_BOUND('',#13187,.T.);
#7923=FACE_OUTER_BOUND('',#13188,.T.);
#7924=FACE_OUTER_BOUND('',#13189,.T.);
#7925=FACE_OUTER_BOUND('',#13190,.T.);
#7926=FACE_OUTER_BOUND('',#13191,.T.);
#7927=FACE_OUTER_BOUND('',#13192,.T.);
#7928=FACE_OUTER_BOUND('',#13193,.T.);
#7929=FACE_OUTER_BOUND('',#13194,.T.);
#7930=FACE_OUTER_BOUND('',#13195,.T.);
#7931=FACE_OUTER_BOUND('',#13196,.T.);
#7932=FACE_OUTER_BOUND('',#13197,.T.);
#7933=FACE_OUTER_BOUND('',#13198,.T.);
#7934=FACE_OUTER_BOUND('',#13199,.T.);
#7935=FACE_OUTER_BOUND('',#13200,.T.);
#7936=FACE_OUTER_BOUND('',#13201,.T.);
#7937=FACE_OUTER_BOUND('',#13202,.T.);
#7938=FACE_OUTER_BOUND('',#13203,.T.);
#7939=FACE_OUTER_BOUND('',#13204,.T.);
#7940=FACE_OUTER_BOUND('',#13205,.T.);
#7941=FACE_OUTER_BOUND('',#13206,.T.);
#7942=FACE_OUTER_BOUND('',#13207,.T.);
#7943=FACE_OUTER_BOUND('',#13208,.T.);
#7944=FACE_OUTER_BOUND('',#13209,.T.);
#7945=FACE_OUTER_BOUND('',#13210,.T.);
#7946=FACE_OUTER_BOUND('',#13211,.T.);
#7947=FACE_OUTER_BOUND('',#13212,.T.);
#7948=FACE_OUTER_BOUND('',#13213,.T.);
#7949=FACE_OUTER_BOUND('',#13214,.T.);
#7950=FACE_OUTER_BOUND('',#13215,.T.);
#7951=FACE_OUTER_BOUND('',#13216,.T.);
#7952=FACE_OUTER_BOUND('',#13217,.T.);
#7953=FACE_OUTER_BOUND('',#13218,.T.);
#7954=FACE_OUTER_BOUND('',#13219,.T.);
#7955=FACE_OUTER_BOUND('',#13220,.T.);
#7956=FACE_OUTER_BOUND('',#13221,.T.);
#7957=FACE_OUTER_BOUND('',#13222,.T.);
#7958=FACE_OUTER_BOUND('',#13223,.T.);
#7959=FACE_OUTER_BOUND('',#13224,.T.);
#7960=FACE_OUTER_BOUND('',#13225,.T.);
#7961=FACE_OUTER_BOUND('',#13226,.T.);
#7962=FACE_OUTER_BOUND('',#13227,.T.);
#7963=FACE_OUTER_BOUND('',#13228,.T.);
#7964=FACE_OUTER_BOUND('',#13229,.T.);
#7965=FACE_OUTER_BOUND('',#13230,.T.);
#7966=FACE_OUTER_BOUND('',#13231,.T.);
#7967=FACE_OUTER_BOUND('',#13232,.T.);
#7968=FACE_OUTER_BOUND('',#13233,.T.);
#7969=FACE_OUTER_BOUND('',#13234,.T.);
#7970=FACE_OUTER_BOUND('',#13235,.T.);
#7971=FACE_OUTER_BOUND('',#13236,.T.);
#7972=FACE_OUTER_BOUND('',#13237,.T.);
#7973=FACE_OUTER_BOUND('',#13238,.T.);
#7974=FACE_OUTER_BOUND('',#13239,.T.);
#7975=FACE_OUTER_BOUND('',#13240,.T.);
#7976=FACE_OUTER_BOUND('',#13241,.T.);
#7977=FACE_OUTER_BOUND('',#13242,.T.);
#7978=FACE_OUTER_BOUND('',#13243,.T.);
#7979=FACE_OUTER_BOUND('',#13244,.T.);
#7980=FACE_OUTER_BOUND('',#13245,.T.);
#7981=FACE_OUTER_BOUND('',#13246,.T.);
#7982=FACE_OUTER_BOUND('',#13247,.T.);
#7983=FACE_OUTER_BOUND('',#13248,.T.);
#7984=FACE_OUTER_BOUND('',#13249,.T.);
#7985=FACE_OUTER_BOUND('',#13250,.T.);
#7986=FACE_OUTER_BOUND('',#13251,.T.);
#7987=FACE_OUTER_BOUND('',#13252,.T.);
#7988=FACE_OUTER_BOUND('',#13253,.T.);
#7989=FACE_OUTER_BOUND('',#13254,.T.);
#7990=FACE_OUTER_BOUND('',#13255,.T.);
#7991=FACE_OUTER_BOUND('',#13256,.T.);
#7992=FACE_OUTER_BOUND('',#13257,.T.);
#7993=FACE_OUTER_BOUND('',#13258,.T.);
#7994=FACE_OUTER_BOUND('',#13259,.T.);
#7995=FACE_OUTER_BOUND('',#13260,.T.);
#7996=FACE_OUTER_BOUND('',#13261,.T.);
#7997=FACE_OUTER_BOUND('',#13262,.T.);
#7998=FACE_OUTER_BOUND('',#13263,.T.);
#7999=FACE_OUTER_BOUND('',#13264,.T.);
#8000=FACE_OUTER_BOUND('',#13265,.T.);
#8001=FACE_OUTER_BOUND('',#13266,.T.);
#8002=FACE_OUTER_BOUND('',#13267,.T.);
#8003=FACE_OUTER_BOUND('',#13268,.T.);
#8004=FACE_OUTER_BOUND('',#13269,.T.);
#8005=FACE_OUTER_BOUND('',#13270,.T.);
#8006=FACE_OUTER_BOUND('',#13271,.T.);
#8007=FACE_OUTER_BOUND('',#13272,.T.);
#8008=FACE_OUTER_BOUND('',#13273,.T.);
#8009=FACE_OUTER_BOUND('',#13274,.T.);
#8010=FACE_OUTER_BOUND('',#13275,.T.);
#8011=FACE_OUTER_BOUND('',#13276,.T.);
#8012=FACE_OUTER_BOUND('',#13277,.T.);
#8013=FACE_OUTER_BOUND('',#13278,.T.);
#8014=FACE_OUTER_BOUND('',#13279,.T.);
#8015=FACE_OUTER_BOUND('',#13280,.T.);
#8016=FACE_OUTER_BOUND('',#13281,.T.);
#8017=FACE_OUTER_BOUND('',#13282,.T.);
#8018=FACE_OUTER_BOUND('',#13283,.T.);
#8019=FACE_OUTER_BOUND('',#13284,.T.);
#8020=FACE_OUTER_BOUND('',#13285,.T.);
#8021=FACE_OUTER_BOUND('',#13286,.T.);
#8022=FACE_OUTER_BOUND('',#13287,.T.);
#8023=FACE_OUTER_BOUND('',#13288,.T.);
#8024=FACE_OUTER_BOUND('',#13289,.T.);
#8025=FACE_OUTER_BOUND('',#13290,.T.);
#8026=FACE_OUTER_BOUND('',#13291,.T.);
#8027=FACE_OUTER_BOUND('',#13292,.T.);
#8028=FACE_OUTER_BOUND('',#13293,.T.);
#8029=FACE_OUTER_BOUND('',#13294,.T.);
#8030=FACE_OUTER_BOUND('',#13295,.T.);
#8031=FACE_OUTER_BOUND('',#13296,.T.);
#8032=FACE_OUTER_BOUND('',#13297,.T.);
#8033=FACE_OUTER_BOUND('',#13298,.T.);
#8034=FACE_OUTER_BOUND('',#13299,.T.);
#8035=FACE_OUTER_BOUND('',#13300,.T.);
#8036=FACE_OUTER_BOUND('',#13301,.T.);
#8037=FACE_OUTER_BOUND('',#13302,.T.);
#8038=FACE_OUTER_BOUND('',#13303,.T.);
#8039=FACE_OUTER_BOUND('',#13304,.T.);
#8040=FACE_OUTER_BOUND('',#13305,.T.);
#8041=FACE_OUTER_BOUND('',#13306,.T.);
#8042=FACE_OUTER_BOUND('',#13307,.T.);
#8043=FACE_OUTER_BOUND('',#13308,.T.);
#8044=FACE_OUTER_BOUND('',#13309,.T.);
#8045=FACE_OUTER_BOUND('',#13310,.T.);
#8046=FACE_OUTER_BOUND('',#13311,.T.);
#8047=FACE_OUTER_BOUND('',#13312,.T.);
#8048=FACE_OUTER_BOUND('',#13313,.T.);
#8049=FACE_OUTER_BOUND('',#13314,.T.);
#8050=FACE_OUTER_BOUND('',#13315,.T.);
#8051=FACE_OUTER_BOUND('',#13316,.T.);
#8052=FACE_OUTER_BOUND('',#13317,.T.);
#8053=FACE_OUTER_BOUND('',#13318,.T.);
#8054=FACE_OUTER_BOUND('',#13319,.T.);
#8055=FACE_OUTER_BOUND('',#13320,.T.);
#8056=FACE_OUTER_BOUND('',#13321,.T.);
#8057=FACE_OUTER_BOUND('',#13322,.T.);
#8058=FACE_OUTER_BOUND('',#13323,.T.);
#8059=FACE_OUTER_BOUND('',#13324,.T.);
#8060=FACE_OUTER_BOUND('',#13325,.T.);
#8061=FACE_OUTER_BOUND('',#13326,.T.);
#8062=FACE_OUTER_BOUND('',#13327,.T.);
#8063=FACE_OUTER_BOUND('',#13328,.T.);
#8064=FACE_OUTER_BOUND('',#13329,.T.);
#8065=FACE_OUTER_BOUND('',#13330,.T.);
#8066=FACE_OUTER_BOUND('',#13331,.T.);
#8067=FACE_OUTER_BOUND('',#13332,.T.);
#8068=FACE_OUTER_BOUND('',#13333,.T.);
#8069=FACE_OUTER_BOUND('',#13334,.T.);
#8070=FACE_OUTER_BOUND('',#13335,.T.);
#8071=FACE_OUTER_BOUND('',#13336,.T.);
#8072=FACE_OUTER_BOUND('',#13337,.T.);
#8073=FACE_OUTER_BOUND('',#13338,.T.);
#8074=FACE_OUTER_BOUND('',#13339,.T.);
#8075=FACE_OUTER_BOUND('',#13340,.T.);
#8076=FACE_OUTER_BOUND('',#13341,.T.);
#8077=FACE_OUTER_BOUND('',#13342,.T.);
#8078=FACE_OUTER_BOUND('',#13343,.T.);
#8079=FACE_OUTER_BOUND('',#13344,.T.);
#8080=FACE_OUTER_BOUND('',#13345,.T.);
#8081=FACE_OUTER_BOUND('',#13346,.T.);
#8082=FACE_OUTER_BOUND('',#13347,.T.);
#8083=FACE_OUTER_BOUND('',#13348,.T.);
#8084=FACE_OUTER_BOUND('',#13349,.T.);
#8085=FACE_OUTER_BOUND('',#13350,.T.);
#8086=FACE_OUTER_BOUND('',#13351,.T.);
#8087=FACE_OUTER_BOUND('',#13352,.T.);
#8088=FACE_OUTER_BOUND('',#13353,.T.);
#8089=FACE_OUTER_BOUND('',#13354,.T.);
#8090=FACE_OUTER_BOUND('',#13355,.T.);
#8091=FACE_OUTER_BOUND('',#13356,.T.);
#8092=FACE_OUTER_BOUND('',#13357,.T.);
#8093=FACE_OUTER_BOUND('',#13358,.T.);
#8094=FACE_OUTER_BOUND('',#13359,.T.);
#8095=FACE_OUTER_BOUND('',#13360,.T.);
#8096=FACE_OUTER_BOUND('',#13361,.T.);
#8097=FACE_OUTER_BOUND('',#13362,.T.);
#8098=FACE_OUTER_BOUND('',#13363,.T.);
#8099=FACE_OUTER_BOUND('',#13364,.T.);
#8100=FACE_OUTER_BOUND('',#13365,.T.);
#8101=FACE_OUTER_BOUND('',#13366,.T.);
#8102=FACE_OUTER_BOUND('',#13367,.T.);
#8103=FACE_OUTER_BOUND('',#13368,.T.);
#8104=FACE_OUTER_BOUND('',#13369,.T.);
#8105=FACE_OUTER_BOUND('',#13370,.T.);
#8106=FACE_OUTER_BOUND('',#13371,.T.);
#8107=FACE_OUTER_BOUND('',#13372,.T.);
#8108=FACE_OUTER_BOUND('',#13373,.T.);
#8109=FACE_OUTER_BOUND('',#13374,.T.);
#8110=FACE_OUTER_BOUND('',#13375,.T.);
#8111=FACE_OUTER_BOUND('',#13376,.T.);
#8112=FACE_OUTER_BOUND('',#13377,.T.);
#8113=FACE_OUTER_BOUND('',#13378,.T.);
#8114=FACE_OUTER_BOUND('',#13379,.T.);
#8115=FACE_OUTER_BOUND('',#13380,.T.);
#8116=FACE_OUTER_BOUND('',#13381,.T.);
#8117=FACE_OUTER_BOUND('',#13382,.T.);
#8118=FACE_OUTER_BOUND('',#13383,.T.);
#8119=FACE_OUTER_BOUND('',#13384,.T.);
#8120=FACE_OUTER_BOUND('',#13385,.T.);
#8121=FACE_OUTER_BOUND('',#13386,.T.);
#8122=FACE_OUTER_BOUND('',#13387,.T.);
#8123=FACE_OUTER_BOUND('',#13388,.T.);
#8124=FACE_OUTER_BOUND('',#13389,.T.);
#8125=FACE_OUTER_BOUND('',#13390,.T.);
#8126=FACE_OUTER_BOUND('',#13391,.T.);
#8127=FACE_OUTER_BOUND('',#13392,.T.);
#8128=FACE_OUTER_BOUND('',#13393,.T.);
#8129=FACE_OUTER_BOUND('',#13394,.T.);
#8130=FACE_OUTER_BOUND('',#13395,.T.);
#8131=FACE_OUTER_BOUND('',#13396,.T.);
#8132=FACE_OUTER_BOUND('',#13397,.T.);
#8133=FACE_OUTER_BOUND('',#13398,.T.);
#8134=FACE_OUTER_BOUND('',#13399,.T.);
#8135=FACE_OUTER_BOUND('',#13400,.T.);
#8136=FACE_OUTER_BOUND('',#13401,.T.);
#8137=FACE_OUTER_BOUND('',#13402,.T.);
#8138=FACE_OUTER_BOUND('',#13403,.T.);
#8139=FACE_OUTER_BOUND('',#13404,.T.);
#8140=FACE_OUTER_BOUND('',#13405,.T.);
#8141=FACE_OUTER_BOUND('',#13406,.T.);
#8142=FACE_OUTER_BOUND('',#13407,.T.);
#8143=FACE_OUTER_BOUND('',#13408,.T.);
#8144=FACE_OUTER_BOUND('',#13409,.T.);
#8145=FACE_OUTER_BOUND('',#13410,.T.);
#8146=FACE_OUTER_BOUND('',#13411,.T.);
#8147=FACE_OUTER_BOUND('',#13412,.T.);
#8148=FACE_OUTER_BOUND('',#13413,.T.);
#8149=FACE_OUTER_BOUND('',#13414,.T.);
#8150=FACE_OUTER_BOUND('',#13415,.T.);
#8151=FACE_OUTER_BOUND('',#13416,.T.);
#8152=FACE_OUTER_BOUND('',#13417,.T.);
#8153=FACE_OUTER_BOUND('',#13418,.T.);
#8154=FACE_OUTER_BOUND('',#13419,.T.);
#8155=FACE_OUTER_BOUND('',#13420,.T.);
#8156=FACE_OUTER_BOUND('',#13421,.T.);
#8157=FACE_OUTER_BOUND('',#13422,.T.);
#8158=FACE_OUTER_BOUND('',#13423,.T.);
#8159=FACE_OUTER_BOUND('',#13424,.T.);
#8160=FACE_OUTER_BOUND('',#13425,.T.);
#8161=FACE_OUTER_BOUND('',#13426,.T.);
#8162=FACE_OUTER_BOUND('',#13427,.T.);
#8163=FACE_OUTER_BOUND('',#13428,.T.);
#8164=FACE_OUTER_BOUND('',#13429,.T.);
#8165=FACE_OUTER_BOUND('',#13430,.T.);
#8166=FACE_OUTER_BOUND('',#13431,.T.);
#8167=FACE_OUTER_BOUND('',#13432,.T.);
#8168=FACE_OUTER_BOUND('',#13433,.T.);
#8169=FACE_OUTER_BOUND('',#13434,.T.);
#8170=FACE_OUTER_BOUND('',#13435,.T.);
#8171=FACE_OUTER_BOUND('',#13436,.T.);
#8172=FACE_OUTER_BOUND('',#13437,.T.);
#8173=FACE_OUTER_BOUND('',#13438,.T.);
#8174=FACE_OUTER_BOUND('',#13439,.T.);
#8175=FACE_OUTER_BOUND('',#13440,.T.);
#8176=FACE_OUTER_BOUND('',#13441,.T.);
#8177=FACE_OUTER_BOUND('',#13442,.T.);
#8178=FACE_OUTER_BOUND('',#13443,.T.);
#8179=FACE_OUTER_BOUND('',#13444,.T.);
#8180=FACE_OUTER_BOUND('',#13445,.T.);
#8181=FACE_OUTER_BOUND('',#13446,.T.);
#8182=FACE_OUTER_BOUND('',#13447,.T.);
#8183=FACE_OUTER_BOUND('',#13448,.T.);
#8184=FACE_OUTER_BOUND('',#13449,.T.);
#8185=FACE_OUTER_BOUND('',#13450,.T.);
#8186=FACE_OUTER_BOUND('',#13451,.T.);
#8187=FACE_OUTER_BOUND('',#13452,.T.);
#8188=FACE_OUTER_BOUND('',#13453,.T.);
#8189=FACE_OUTER_BOUND('',#13454,.T.);
#8190=FACE_OUTER_BOUND('',#13455,.T.);
#8191=FACE_OUTER_BOUND('',#13456,.T.);
#8192=FACE_OUTER_BOUND('',#13457,.T.);
#8193=FACE_OUTER_BOUND('',#13458,.T.);
#8194=FACE_OUTER_BOUND('',#13459,.T.);
#8195=FACE_OUTER_BOUND('',#13460,.T.);
#8196=FACE_OUTER_BOUND('',#13461,.T.);
#8197=FACE_OUTER_BOUND('',#13462,.T.);
#8198=FACE_OUTER_BOUND('',#13463,.T.);
#8199=FACE_OUTER_BOUND('',#13464,.T.);
#8200=FACE_OUTER_BOUND('',#13465,.T.);
#8201=FACE_OUTER_BOUND('',#13466,.T.);
#8202=FACE_OUTER_BOUND('',#13467,.T.);
#8203=FACE_OUTER_BOUND('',#13468,.T.);
#8204=FACE_OUTER_BOUND('',#13469,.T.);
#8205=FACE_OUTER_BOUND('',#13470,.T.);
#8206=FACE_OUTER_BOUND('',#13471,.T.);
#8207=FACE_OUTER_BOUND('',#13472,.T.);
#8208=FACE_OUTER_BOUND('',#13473,.T.);
#8209=FACE_OUTER_BOUND('',#13474,.T.);
#8210=FACE_OUTER_BOUND('',#13475,.T.);
#8211=FACE_OUTER_BOUND('',#13476,.T.);
#8212=FACE_OUTER_BOUND('',#13477,.T.);
#8213=FACE_OUTER_BOUND('',#13478,.T.);
#8214=FACE_OUTER_BOUND('',#13479,.T.);
#8215=FACE_OUTER_BOUND('',#13480,.T.);
#8216=FACE_OUTER_BOUND('',#13481,.T.);
#8217=FACE_OUTER_BOUND('',#13482,.T.);
#8218=FACE_OUTER_BOUND('',#13483,.T.);
#8219=FACE_OUTER_BOUND('',#13484,.T.);
#8220=FACE_OUTER_BOUND('',#13485,.T.);
#8221=FACE_OUTER_BOUND('',#13486,.T.);
#8222=FACE_OUTER_BOUND('',#13487,.T.);
#8223=FACE_OUTER_BOUND('',#13488,.T.);
#8224=FACE_OUTER_BOUND('',#13489,.T.);
#8225=FACE_OUTER_BOUND('',#13490,.T.);
#8226=FACE_OUTER_BOUND('',#13491,.T.);
#8227=FACE_OUTER_BOUND('',#13492,.T.);
#8228=FACE_OUTER_BOUND('',#13493,.T.);
#8229=FACE_OUTER_BOUND('',#13494,.T.);
#8230=FACE_OUTER_BOUND('',#13495,.T.);
#8231=FACE_OUTER_BOUND('',#13496,.T.);
#8232=FACE_OUTER_BOUND('',#13497,.T.);
#8233=FACE_OUTER_BOUND('',#13498,.T.);
#8234=FACE_OUTER_BOUND('',#13499,.T.);
#8235=FACE_OUTER_BOUND('',#13500,.T.);
#8236=FACE_OUTER_BOUND('',#13501,.T.);
#8237=FACE_OUTER_BOUND('',#13502,.T.);
#8238=FACE_OUTER_BOUND('',#13503,.T.);
#8239=FACE_OUTER_BOUND('',#13504,.T.);
#8240=FACE_OUTER_BOUND('',#13505,.T.);
#8241=FACE_OUTER_BOUND('',#13506,.T.);
#8242=FACE_OUTER_BOUND('',#13507,.T.);
#8243=FACE_OUTER_BOUND('',#13508,.T.);
#8244=FACE_OUTER_BOUND('',#13509,.T.);
#8245=FACE_OUTER_BOUND('',#13510,.T.);
#8246=FACE_OUTER_BOUND('',#13511,.T.);
#8247=FACE_OUTER_BOUND('',#13512,.T.);
#8248=FACE_OUTER_BOUND('',#13513,.T.);
#8249=FACE_OUTER_BOUND('',#13514,.T.);
#8250=FACE_OUTER_BOUND('',#13515,.T.);
#8251=FACE_OUTER_BOUND('',#13516,.T.);
#8252=FACE_OUTER_BOUND('',#13517,.T.);
#8253=FACE_OUTER_BOUND('',#13518,.T.);
#8254=FACE_OUTER_BOUND('',#13519,.T.);
#8255=FACE_OUTER_BOUND('',#13520,.T.);
#8256=FACE_OUTER_BOUND('',#13521,.T.);
#8257=FACE_OUTER_BOUND('',#13522,.T.);
#8258=FACE_OUTER_BOUND('',#13523,.T.);
#8259=FACE_OUTER_BOUND('',#13524,.T.);
#8260=FACE_OUTER_BOUND('',#13525,.T.);
#8261=FACE_OUTER_BOUND('',#13526,.T.);
#8262=FACE_OUTER_BOUND('',#13527,.T.);
#8263=FACE_OUTER_BOUND('',#13528,.T.);
#8264=FACE_OUTER_BOUND('',#13529,.T.);
#8265=FACE_OUTER_BOUND('',#13530,.T.);
#8266=FACE_OUTER_BOUND('',#13531,.T.);
#8267=FACE_OUTER_BOUND('',#13532,.T.);
#8268=FACE_OUTER_BOUND('',#13533,.T.);
#8269=FACE_OUTER_BOUND('',#13534,.T.);
#8270=FACE_OUTER_BOUND('',#13535,.T.);
#8271=FACE_OUTER_BOUND('',#13536,.T.);
#8272=FACE_OUTER_BOUND('',#13537,.T.);
#8273=FACE_OUTER_BOUND('',#13538,.T.);
#8274=FACE_OUTER_BOUND('',#13539,.T.);
#8275=FACE_OUTER_BOUND('',#13540,.T.);
#8276=FACE_OUTER_BOUND('',#13541,.T.);
#8277=FACE_OUTER_BOUND('',#13542,.T.);
#8278=FACE_OUTER_BOUND('',#13543,.T.);
#8279=FACE_OUTER_BOUND('',#13544,.T.);
#8280=FACE_OUTER_BOUND('',#13545,.T.);
#8281=FACE_OUTER_BOUND('',#13546,.T.);
#8282=FACE_OUTER_BOUND('',#13547,.T.);
#8283=FACE_OUTER_BOUND('',#13548,.T.);
#8284=FACE_OUTER_BOUND('',#13549,.T.);
#8285=FACE_OUTER_BOUND('',#13550,.T.);
#8286=FACE_OUTER_BOUND('',#13551,.T.);
#8287=FACE_OUTER_BOUND('',#13552,.T.);
#8288=FACE_OUTER_BOUND('',#13553,.T.);
#8289=FACE_OUTER_BOUND('',#13554,.T.);
#8290=FACE_OUTER_BOUND('',#13555,.T.);
#8291=FACE_OUTER_BOUND('',#13556,.T.);
#8292=FACE_OUTER_BOUND('',#13557,.T.);
#8293=FACE_OUTER_BOUND('',#13558,.T.);
#8294=FACE_OUTER_BOUND('',#13559,.T.);
#8295=FACE_OUTER_BOUND('',#13560,.T.);
#8296=FACE_OUTER_BOUND('',#13561,.T.);
#8297=FACE_OUTER_BOUND('',#13562,.T.);
#8298=FACE_OUTER_BOUND('',#13563,.T.);
#8299=FACE_OUTER_BOUND('',#13564,.T.);
#8300=FACE_OUTER_BOUND('',#13565,.T.);
#8301=FACE_OUTER_BOUND('',#13566,.T.);
#8302=FACE_OUTER_BOUND('',#13567,.T.);
#8303=FACE_OUTER_BOUND('',#13568,.T.);
#8304=FACE_OUTER_BOUND('',#13569,.T.);
#8305=FACE_OUTER_BOUND('',#13570,.T.);
#8306=FACE_OUTER_BOUND('',#13571,.T.);
#8307=FACE_OUTER_BOUND('',#13572,.T.);
#8308=FACE_OUTER_BOUND('',#13573,.T.);
#8309=FACE_OUTER_BOUND('',#13574,.T.);
#8310=FACE_OUTER_BOUND('',#13575,.T.);
#8311=FACE_OUTER_BOUND('',#13576,.T.);
#8312=FACE_OUTER_BOUND('',#13577,.T.);
#8313=FACE_OUTER_BOUND('',#13578,.T.);
#8314=FACE_OUTER_BOUND('',#13579,.T.);
#8315=FACE_OUTER_BOUND('',#13580,.T.);
#8316=FACE_OUTER_BOUND('',#13581,.T.);
#8317=FACE_OUTER_BOUND('',#13582,.T.);
#8318=FACE_OUTER_BOUND('',#13583,.T.);
#8319=FACE_OUTER_BOUND('',#13584,.T.);
#8320=FACE_OUTER_BOUND('',#13585,.T.);
#8321=FACE_OUTER_BOUND('',#13586,.T.);
#8322=FACE_OUTER_BOUND('',#13587,.T.);
#8323=FACE_OUTER_BOUND('',#13588,.T.);
#8324=FACE_OUTER_BOUND('',#13589,.T.);
#8325=FACE_OUTER_BOUND('',#13590,.T.);
#8326=FACE_OUTER_BOUND('',#13591,.T.);
#8327=FACE_OUTER_BOUND('',#13592,.T.);
#8328=FACE_OUTER_BOUND('',#13593,.T.);
#8329=FACE_OUTER_BOUND('',#13594,.T.);
#8330=FACE_OUTER_BOUND('',#13595,.T.);
#8331=FACE_OUTER_BOUND('',#13596,.T.);
#8332=FACE_OUTER_BOUND('',#13597,.T.);
#8333=FACE_OUTER_BOUND('',#13598,.T.);
#8334=FACE_OUTER_BOUND('',#13599,.T.);
#8335=FACE_OUTER_BOUND('',#13600,.T.);
#8336=FACE_OUTER_BOUND('',#13601,.T.);
#8337=FACE_OUTER_BOUND('',#13602,.T.);
#8338=FACE_OUTER_BOUND('',#13603,.T.);
#8339=FACE_OUTER_BOUND('',#13604,.T.);
#8340=FACE_OUTER_BOUND('',#13605,.T.);
#8341=FACE_OUTER_BOUND('',#13606,.T.);
#8342=FACE_OUTER_BOUND('',#13607,.T.);
#8343=FACE_OUTER_BOUND('',#13608,.T.);
#8344=FACE_OUTER_BOUND('',#13609,.T.);
#8345=FACE_OUTER_BOUND('',#13610,.T.);
#8346=FACE_OUTER_BOUND('',#13611,.T.);
#8347=FACE_OUTER_BOUND('',#13612,.T.);
#8348=FACE_OUTER_BOUND('',#13613,.T.);
#8349=FACE_OUTER_BOUND('',#13614,.T.);
#8350=FACE_OUTER_BOUND('',#13615,.T.);
#8351=FACE_OUTER_BOUND('',#13616,.T.);
#8352=FACE_OUTER_BOUND('',#13617,.T.);
#8353=FACE_OUTER_BOUND('',#13618,.T.);
#8354=FACE_OUTER_BOUND('',#13619,.T.);
#8355=FACE_OUTER_BOUND('',#13620,.T.);
#8356=FACE_OUTER_BOUND('',#13621,.T.);
#8357=FACE_OUTER_BOUND('',#13622,.T.);
#8358=FACE_OUTER_BOUND('',#13623,.T.);
#8359=FACE_OUTER_BOUND('',#13624,.T.);
#8360=FACE_OUTER_BOUND('',#13625,.T.);
#8361=FACE_OUTER_BOUND('',#13626,.T.);
#8362=FACE_OUTER_BOUND('',#13627,.T.);
#8363=FACE_OUTER_BOUND('',#13628,.T.);
#8364=FACE_OUTER_BOUND('',#13629,.T.);
#8365=FACE_OUTER_BOUND('',#13630,.T.);
#8366=FACE_OUTER_BOUND('',#13631,.T.);
#8367=FACE_OUTER_BOUND('',#13632,.T.);
#8368=FACE_OUTER_BOUND('',#13633,.T.);
#8369=FACE_OUTER_BOUND('',#13634,.T.);
#8370=FACE_OUTER_BOUND('',#13635,.T.);
#8371=FACE_OUTER_BOUND('',#13636,.T.);
#8372=FACE_OUTER_BOUND('',#13637,.T.);
#8373=FACE_OUTER_BOUND('',#13638,.T.);
#8374=FACE_OUTER_BOUND('',#13639,.T.);
#8375=FACE_OUTER_BOUND('',#13640,.T.);
#8376=FACE_OUTER_BOUND('',#13641,.T.);
#8377=FACE_OUTER_BOUND('',#13642,.T.);
#8378=FACE_OUTER_BOUND('',#13643,.T.);
#8379=FACE_OUTER_BOUND('',#13644,.T.);
#8380=FACE_OUTER_BOUND('',#13645,.T.);
#8381=FACE_OUTER_BOUND('',#13646,.T.);
#8382=FACE_OUTER_BOUND('',#13647,.T.);
#8383=FACE_OUTER_BOUND('',#13648,.T.);
#8384=FACE_OUTER_BOUND('',#13649,.T.);
#8385=FACE_OUTER_BOUND('',#13650,.T.);
#8386=FACE_OUTER_BOUND('',#13651,.T.);
#8387=FACE_OUTER_BOUND('',#13652,.T.);
#8388=FACE_OUTER_BOUND('',#13653,.T.);
#8389=FACE_OUTER_BOUND('',#13654,.T.);
#8390=FACE_OUTER_BOUND('',#13655,.T.);
#8391=FACE_OUTER_BOUND('',#13656,.T.);
#8392=FACE_OUTER_BOUND('',#13657,.T.);
#8393=FACE_OUTER_BOUND('',#13658,.T.);
#8394=FACE_OUTER_BOUND('',#13659,.T.);
#8395=FACE_OUTER_BOUND('',#13660,.T.);
#8396=FACE_OUTER_BOUND('',#13661,.T.);
#8397=FACE_OUTER_BOUND('',#13662,.T.);
#8398=FACE_OUTER_BOUND('',#13663,.T.);
#8399=FACE_OUTER_BOUND('',#13664,.T.);
#8400=FACE_OUTER_BOUND('',#13665,.T.);
#8401=FACE_OUTER_BOUND('',#13666,.T.);
#8402=FACE_OUTER_BOUND('',#13667,.T.);
#8403=FACE_OUTER_BOUND('',#13668,.T.);
#8404=FACE_OUTER_BOUND('',#13669,.T.);
#8405=FACE_OUTER_BOUND('',#13670,.T.);
#8406=FACE_OUTER_BOUND('',#13671,.T.);
#8407=FACE_OUTER_BOUND('',#13672,.T.);
#8408=FACE_OUTER_BOUND('',#13673,.T.);
#8409=FACE_OUTER_BOUND('',#13674,.T.);
#8410=FACE_OUTER_BOUND('',#13675,.T.);
#8411=FACE_OUTER_BOUND('',#13676,.T.);
#8412=FACE_OUTER_BOUND('',#13677,.T.);
#8413=FACE_OUTER_BOUND('',#13678,.T.);
#8414=FACE_OUTER_BOUND('',#13679,.T.);
#8415=FACE_OUTER_BOUND('',#13680,.T.);
#8416=FACE_OUTER_BOUND('',#13681,.T.);
#8417=FACE_OUTER_BOUND('',#13682,.T.);
#8418=FACE_OUTER_BOUND('',#13683,.T.);
#8419=FACE_OUTER_BOUND('',#13684,.T.);
#8420=FACE_OUTER_BOUND('',#13685,.T.);
#8421=FACE_OUTER_BOUND('',#13686,.T.);
#8422=FACE_OUTER_BOUND('',#13687,.T.);
#8423=FACE_OUTER_BOUND('',#13688,.T.);
#8424=FACE_OUTER_BOUND('',#13689,.T.);
#8425=FACE_OUTER_BOUND('',#13690,.T.);
#8426=FACE_OUTER_BOUND('',#13691,.T.);
#8427=FACE_OUTER_BOUND('',#13692,.T.);
#8428=FACE_OUTER_BOUND('',#13693,.T.);
#8429=FACE_OUTER_BOUND('',#13694,.T.);
#8430=FACE_OUTER_BOUND('',#13695,.T.);
#8431=FACE_OUTER_BOUND('',#13696,.T.);
#8432=FACE_OUTER_BOUND('',#13697,.T.);
#8433=FACE_OUTER_BOUND('',#13698,.T.);
#8434=FACE_OUTER_BOUND('',#13699,.T.);
#8435=FACE_OUTER_BOUND('',#13700,.T.);
#8436=FACE_OUTER_BOUND('',#13701,.T.);
#8437=FACE_OUTER_BOUND('',#13702,.T.);
#8438=FACE_OUTER_BOUND('',#13703,.T.);
#8439=FACE_OUTER_BOUND('',#13704,.T.);
#8440=FACE_OUTER_BOUND('',#13705,.T.);
#8441=FACE_OUTER_BOUND('',#13706,.T.);
#8442=FACE_OUTER_BOUND('',#13707,.T.);
#8443=FACE_OUTER_BOUND('',#13708,.T.);
#8444=FACE_OUTER_BOUND('',#13709,.T.);
#8445=FACE_OUTER_BOUND('',#13710,.T.);
#8446=FACE_OUTER_BOUND('',#13711,.T.);
#8447=FACE_OUTER_BOUND('',#13712,.T.);
#8448=FACE_OUTER_BOUND('',#13713,.T.);
#8449=FACE_OUTER_BOUND('',#13714,.T.);
#8450=FACE_OUTER_BOUND('',#13715,.T.);
#8451=FACE_OUTER_BOUND('',#13716,.T.);
#8452=FACE_OUTER_BOUND('',#13717,.T.);
#8453=FACE_OUTER_BOUND('',#13718,.T.);
#8454=FACE_OUTER_BOUND('',#13719,.T.);
#8455=FACE_OUTER_BOUND('',#13720,.T.);
#8456=FACE_OUTER_BOUND('',#13721,.T.);
#8457=FACE_OUTER_BOUND('',#13722,.T.);
#8458=FACE_OUTER_BOUND('',#13723,.T.);
#8459=FACE_OUTER_BOUND('',#13724,.T.);
#8460=FACE_OUTER_BOUND('',#13725,.T.);
#8461=FACE_OUTER_BOUND('',#13726,.T.);
#8462=FACE_OUTER_BOUND('',#13727,.T.);
#8463=FACE_OUTER_BOUND('',#13728,.T.);
#8464=FACE_OUTER_BOUND('',#13729,.T.);
#8465=FACE_OUTER_BOUND('',#13730,.T.);
#8466=FACE_OUTER_BOUND('',#13731,.T.);
#8467=FACE_OUTER_BOUND('',#13732,.T.);
#8468=FACE_OUTER_BOUND('',#13733,.T.);
#8469=FACE_OUTER_BOUND('',#13734,.T.);
#8470=FACE_OUTER_BOUND('',#13735,.T.);
#8471=FACE_OUTER_BOUND('',#13736,.T.);
#8472=FACE_OUTER_BOUND('',#13737,.T.);
#8473=FACE_OUTER_BOUND('',#13738,.T.);
#8474=FACE_OUTER_BOUND('',#13739,.T.);
#8475=FACE_OUTER_BOUND('',#13740,.T.);
#8476=FACE_OUTER_BOUND('',#13741,.T.);
#8477=FACE_OUTER_BOUND('',#13742,.T.);
#8478=FACE_OUTER_BOUND('',#13743,.T.);
#8479=FACE_OUTER_BOUND('',#13744,.T.);
#8480=FACE_OUTER_BOUND('',#13745,.T.);
#8481=FACE_OUTER_BOUND('',#13746,.T.);
#8482=FACE_OUTER_BOUND('',#13747,.T.);
#8483=FACE_OUTER_BOUND('',#13748,.T.);
#8484=FACE_OUTER_BOUND('',#13749,.T.);
#8485=FACE_OUTER_BOUND('',#13750,.T.);
#8486=FACE_OUTER_BOUND('',#13751,.T.);
#8487=FACE_OUTER_BOUND('',#13752,.T.);
#8488=FACE_OUTER_BOUND('',#13753,.T.);
#8489=FACE_OUTER_BOUND('',#13754,.T.);
#8490=FACE_OUTER_BOUND('',#13755,.T.);
#8491=FACE_OUTER_BOUND('',#13756,.T.);
#8492=FACE_OUTER_BOUND('',#13757,.T.);
#8493=FACE_OUTER_BOUND('',#13758,.T.);
#8494=FACE_OUTER_BOUND('',#13759,.T.);
#8495=FACE_OUTER_BOUND('',#13760,.T.);
#8496=FACE_OUTER_BOUND('',#13761,.T.);
#8497=FACE_OUTER_BOUND('',#13762,.T.);
#8498=FACE_OUTER_BOUND('',#13763,.T.);
#8499=FACE_OUTER_BOUND('',#13764,.T.);
#8500=FACE_OUTER_BOUND('',#13765,.T.);
#8501=FACE_OUTER_BOUND('',#13766,.T.);
#8502=FACE_OUTER_BOUND('',#13767,.T.);
#8503=FACE_OUTER_BOUND('',#13768,.T.);
#8504=FACE_OUTER_BOUND('',#13769,.T.);
#8505=FACE_OUTER_BOUND('',#13770,.T.);
#8506=FACE_OUTER_BOUND('',#13771,.T.);
#8507=FACE_OUTER_BOUND('',#13772,.T.);
#8508=FACE_OUTER_BOUND('',#13773,.T.);
#8509=FACE_OUTER_BOUND('',#13774,.T.);
#8510=FACE_OUTER_BOUND('',#13775,.T.);
#8511=FACE_OUTER_BOUND('',#13776,.T.);
#8512=FACE_OUTER_BOUND('',#13777,.T.);
#8513=FACE_OUTER_BOUND('',#13778,.T.);
#8514=FACE_OUTER_BOUND('',#13779,.T.);
#8515=FACE_OUTER_BOUND('',#13780,.T.);
#8516=FACE_OUTER_BOUND('',#13781,.T.);
#8517=FACE_OUTER_BOUND('',#13782,.T.);
#8518=FACE_OUTER_BOUND('',#13783,.T.);
#8519=FACE_OUTER_BOUND('',#13784,.T.);
#8520=FACE_OUTER_BOUND('',#13785,.T.);
#8521=FACE_OUTER_BOUND('',#13786,.T.);
#8522=FACE_OUTER_BOUND('',#13787,.T.);
#8523=FACE_OUTER_BOUND('',#13788,.T.);
#8524=FACE_OUTER_BOUND('',#13789,.T.);
#8525=FACE_OUTER_BOUND('',#13790,.T.);
#8526=FACE_OUTER_BOUND('',#13791,.T.);
#8527=FACE_OUTER_BOUND('',#13792,.T.);
#8528=FACE_OUTER_BOUND('',#13793,.T.);
#8529=FACE_OUTER_BOUND('',#13794,.T.);
#8530=FACE_OUTER_BOUND('',#13795,.T.);
#8531=FACE_OUTER_BOUND('',#13796,.T.);
#8532=FACE_OUTER_BOUND('',#13797,.T.);
#8533=FACE_OUTER_BOUND('',#13798,.T.);
#8534=FACE_OUTER_BOUND('',#13799,.T.);
#8535=FACE_OUTER_BOUND('',#13800,.T.);
#8536=FACE_OUTER_BOUND('',#13801,.T.);
#8537=FACE_OUTER_BOUND('',#13802,.T.);
#8538=FACE_OUTER_BOUND('',#13803,.T.);
#8539=FACE_OUTER_BOUND('',#13804,.T.);
#8540=FACE_OUTER_BOUND('',#13805,.T.);
#8541=FACE_OUTER_BOUND('',#13806,.T.);
#8542=FACE_OUTER_BOUND('',#13807,.T.);
#8543=FACE_OUTER_BOUND('',#13808,.T.);
#8544=FACE_OUTER_BOUND('',#13809,.T.);
#8545=FACE_OUTER_BOUND('',#13810,.T.);
#8546=FACE_OUTER_BOUND('',#13811,.T.);
#8547=FACE_OUTER_BOUND('',#13812,.T.);
#8548=FACE_OUTER_BOUND('',#13813,.T.);
#8549=FACE_OUTER_BOUND('',#13814,.T.);
#8550=FACE_OUTER_BOUND('',#13815,.T.);
#8551=FACE_OUTER_BOUND('',#13816,.T.);
#8552=FACE_OUTER_BOUND('',#13817,.T.);
#8553=FACE_OUTER_BOUND('',#13818,.T.);
#8554=FACE_OUTER_BOUND('',#13819,.T.);
#8555=FACE_OUTER_BOUND('',#13820,.T.);
#8556=FACE_OUTER_BOUND('',#13821,.T.);
#8557=FACE_OUTER_BOUND('',#13822,.T.);
#8558=FACE_OUTER_BOUND('',#13823,.T.);
#8559=FACE_OUTER_BOUND('',#13824,.T.);
#8560=FACE_OUTER_BOUND('',#13825,.T.);
#8561=FACE_OUTER_BOUND('',#13826,.T.);
#8562=FACE_OUTER_BOUND('',#13827,.T.);
#8563=FACE_OUTER_BOUND('',#13828,.T.);
#8564=FACE_OUTER_BOUND('',#13829,.T.);
#8565=FACE_OUTER_BOUND('',#13830,.T.);
#8566=FACE_OUTER_BOUND('',#13831,.T.);
#8567=FACE_OUTER_BOUND('',#13832,.T.);
#8568=FACE_OUTER_BOUND('',#13833,.T.);
#8569=FACE_OUTER_BOUND('',#13834,.T.);
#8570=FACE_OUTER_BOUND('',#13835,.T.);
#8571=FACE_OUTER_BOUND('',#13836,.T.);
#8572=FACE_OUTER_BOUND('',#13837,.T.);
#8573=FACE_OUTER_BOUND('',#13838,.T.);
#8574=FACE_OUTER_BOUND('',#13839,.T.);
#8575=FACE_OUTER_BOUND('',#13840,.T.);
#8576=FACE_OUTER_BOUND('',#13841,.T.);
#8577=FACE_OUTER_BOUND('',#13842,.T.);
#8578=FACE_OUTER_BOUND('',#13843,.T.);
#8579=FACE_OUTER_BOUND('',#13844,.T.);
#8580=FACE_OUTER_BOUND('',#13845,.T.);
#8581=FACE_OUTER_BOUND('',#13846,.T.);
#8582=FACE_OUTER_BOUND('',#13847,.T.);
#8583=FACE_OUTER_BOUND('',#13848,.T.);
#8584=FACE_OUTER_BOUND('',#13849,.T.);
#8585=FACE_OUTER_BOUND('',#13850,.T.);
#8586=FACE_OUTER_BOUND('',#13851,.T.);
#8587=FACE_OUTER_BOUND('',#13852,.T.);
#8588=FACE_OUTER_BOUND('',#13853,.T.);
#8589=FACE_OUTER_BOUND('',#13854,.T.);
#8590=FACE_OUTER_BOUND('',#13855,.T.);
#8591=FACE_OUTER_BOUND('',#13856,.T.);
#8592=FACE_OUTER_BOUND('',#13857,.T.);
#8593=FACE_OUTER_BOUND('',#13858,.T.);
#8594=FACE_OUTER_BOUND('',#13859,.T.);
#8595=FACE_OUTER_BOUND('',#13860,.T.);
#8596=FACE_OUTER_BOUND('',#13861,.T.);
#8597=FACE_OUTER_BOUND('',#13862,.T.);
#8598=FACE_OUTER_BOUND('',#13863,.T.);
#8599=FACE_OUTER_BOUND('',#13864,.T.);
#8600=FACE_OUTER_BOUND('',#13865,.T.);
#8601=FACE_OUTER_BOUND('',#13866,.T.);
#8602=FACE_OUTER_BOUND('',#13867,.T.);
#8603=FACE_OUTER_BOUND('',#13868,.T.);
#8604=FACE_OUTER_BOUND('',#13869,.T.);
#8605=FACE_OUTER_BOUND('',#13870,.T.);
#8606=FACE_OUTER_BOUND('',#13871,.T.);
#8607=FACE_OUTER_BOUND('',#13872,.T.);
#8608=FACE_OUTER_BOUND('',#13873,.T.);
#8609=FACE_OUTER_BOUND('',#13874,.T.);
#8610=FACE_OUTER_BOUND('',#13875,.T.);
#8611=FACE_OUTER_BOUND('',#13876,.T.);
#8612=FACE_OUTER_BOUND('',#13877,.T.);
#8613=FACE_OUTER_BOUND('',#13878,.T.);
#8614=FACE_OUTER_BOUND('',#13879,.T.);
#8615=FACE_OUTER_BOUND('',#13880,.T.);
#8616=FACE_OUTER_BOUND('',#13881,.T.);
#8617=FACE_OUTER_BOUND('',#13882,.T.);
#8618=FACE_OUTER_BOUND('',#13883,.T.);
#8619=FACE_OUTER_BOUND('',#13884,.T.);
#8620=FACE_OUTER_BOUND('',#13885,.T.);
#8621=FACE_OUTER_BOUND('',#13886,.T.);
#8622=FACE_OUTER_BOUND('',#13887,.T.);
#8623=FACE_OUTER_BOUND('',#13888,.T.);
#8624=FACE_OUTER_BOUND('',#13889,.T.);
#8625=FACE_OUTER_BOUND('',#13890,.T.);
#8626=FACE_OUTER_BOUND('',#13891,.T.);
#8627=FACE_OUTER_BOUND('',#13892,.T.);
#8628=FACE_OUTER_BOUND('',#13893,.T.);
#8629=FACE_OUTER_BOUND('',#13894,.T.);
#8630=FACE_OUTER_BOUND('',#13895,.T.);
#8631=FACE_OUTER_BOUND('',#13896,.T.);
#8632=FACE_OUTER_BOUND('',#13897,.T.);
#8633=FACE_OUTER_BOUND('',#13898,.T.);
#8634=FACE_OUTER_BOUND('',#13899,.T.);
#8635=FACE_OUTER_BOUND('',#13900,.T.);
#8636=FACE_OUTER_BOUND('',#13901,.T.);
#8637=FACE_OUTER_BOUND('',#13902,.T.);
#8638=FACE_OUTER_BOUND('',#13903,.T.);
#8639=FACE_OUTER_BOUND('',#13904,.T.);
#8640=FACE_OUTER_BOUND('',#13905,.T.);
#8641=FACE_OUTER_BOUND('',#13906,.T.);
#8642=FACE_OUTER_BOUND('',#13907,.T.);
#8643=FACE_OUTER_BOUND('',#13908,.T.);
#8644=FACE_OUTER_BOUND('',#13909,.T.);
#8645=FACE_OUTER_BOUND('',#13910,.T.);
#8646=FACE_OUTER_BOUND('',#13911,.T.);
#8647=FACE_OUTER_BOUND('',#13912,.T.);
#8648=FACE_OUTER_BOUND('',#13913,.T.);
#8649=FACE_OUTER_BOUND('',#13914,.T.);
#8650=FACE_OUTER_BOUND('',#13915,.T.);
#8651=FACE_OUTER_BOUND('',#13916,.T.);
#8652=FACE_OUTER_BOUND('',#13917,.T.);
#8653=FACE_OUTER_BOUND('',#13918,.T.);
#8654=FACE_OUTER_BOUND('',#13919,.T.);
#8655=FACE_OUTER_BOUND('',#13920,.T.);
#8656=FACE_OUTER_BOUND('',#13921,.T.);
#8657=FACE_OUTER_BOUND('',#13922,.T.);
#8658=FACE_OUTER_BOUND('',#13923,.T.);
#8659=FACE_OUTER_BOUND('',#13924,.T.);
#8660=FACE_OUTER_BOUND('',#13925,.T.);
#8661=FACE_OUTER_BOUND('',#13926,.T.);
#8662=FACE_OUTER_BOUND('',#13927,.T.);
#8663=FACE_OUTER_BOUND('',#13928,.T.);
#8664=FACE_OUTER_BOUND('',#13929,.T.);
#8665=FACE_OUTER_BOUND('',#13930,.T.);
#8666=FACE_OUTER_BOUND('',#13931,.T.);
#8667=FACE_OUTER_BOUND('',#13932,.T.);
#8668=FACE_OUTER_BOUND('',#13933,.T.);
#8669=FACE_OUTER_BOUND('',#13934,.T.);
#8670=FACE_OUTER_BOUND('',#13935,.T.);
#8671=FACE_OUTER_BOUND('',#13936,.T.);
#8672=FACE_OUTER_BOUND('',#13937,.T.);
#8673=FACE_OUTER_BOUND('',#13938,.T.);
#8674=FACE_OUTER_BOUND('',#13939,.T.);
#8675=FACE_OUTER_BOUND('',#13940,.T.);
#8676=FACE_OUTER_BOUND('',#13941,.T.);
#8677=FACE_OUTER_BOUND('',#13942,.T.);
#8678=FACE_OUTER_BOUND('',#13943,.T.);
#8679=FACE_OUTER_BOUND('',#13944,.T.);
#8680=FACE_OUTER_BOUND('',#13945,.T.);
#8681=FACE_OUTER_BOUND('',#13946,.T.);
#8682=FACE_OUTER_BOUND('',#13947,.T.);
#8683=FACE_OUTER_BOUND('',#13948,.T.);
#8684=FACE_OUTER_BOUND('',#13949,.T.);
#8685=FACE_OUTER_BOUND('',#13950,.T.);
#8686=FACE_OUTER_BOUND('',#13951,.T.);
#8687=FACE_OUTER_BOUND('',#13952,.T.);
#8688=FACE_OUTER_BOUND('',#13953,.T.);
#8689=FACE_OUTER_BOUND('',#13954,.T.);
#8690=FACE_OUTER_BOUND('',#13955,.T.);
#8691=FACE_OUTER_BOUND('',#13956,.T.);
#8692=FACE_OUTER_BOUND('',#13957,.T.);
#8693=FACE_OUTER_BOUND('',#13958,.T.);
#8694=FACE_OUTER_BOUND('',#13959,.T.);
#8695=FACE_OUTER_BOUND('',#13960,.T.);
#8696=FACE_OUTER_BOUND('',#13961,.T.);
#8697=FACE_OUTER_BOUND('',#13962,.T.);
#8698=FACE_OUTER_BOUND('',#13963,.T.);
#8699=FACE_OUTER_BOUND('',#13964,.T.);
#8700=FACE_OUTER_BOUND('',#13965,.T.);
#8701=FACE_OUTER_BOUND('',#13966,.T.);
#8702=FACE_OUTER_BOUND('',#13967,.T.);
#8703=FACE_OUTER_BOUND('',#13968,.T.);
#8704=FACE_OUTER_BOUND('',#13969,.T.);
#8705=FACE_OUTER_BOUND('',#13970,.T.);
#8706=FACE_OUTER_BOUND('',#13971,.T.);
#8707=FACE_OUTER_BOUND('',#13972,.T.);
#8708=FACE_OUTER_BOUND('',#13973,.T.);
#8709=FACE_OUTER_BOUND('',#13974,.T.);
#8710=FACE_OUTER_BOUND('',#13975,.T.);
#8711=FACE_OUTER_BOUND('',#13976,.T.);
#8712=FACE_OUTER_BOUND('',#13977,.T.);
#8713=FACE_OUTER_BOUND('',#13978,.T.);
#8714=FACE_OUTER_BOUND('',#13979,.T.);
#8715=FACE_OUTER_BOUND('',#13980,.T.);
#8716=FACE_OUTER_BOUND('',#13981,.T.);
#8717=FACE_OUTER_BOUND('',#13982,.T.);
#8718=FACE_OUTER_BOUND('',#13983,.T.);
#8719=FACE_OUTER_BOUND('',#13984,.T.);
#8720=FACE_OUTER_BOUND('',#13985,.T.);
#8721=FACE_OUTER_BOUND('',#13986,.T.);
#8722=FACE_OUTER_BOUND('',#13987,.T.);
#8723=FACE_OUTER_BOUND('',#13988,.T.);
#8724=FACE_OUTER_BOUND('',#13989,.T.);
#8725=FACE_OUTER_BOUND('',#13990,.T.);
#8726=FACE_OUTER_BOUND('',#13991,.T.);
#8727=FACE_OUTER_BOUND('',#13992,.T.);
#8728=FACE_OUTER_BOUND('',#13993,.T.);
#8729=FACE_OUTER_BOUND('',#13994,.T.);
#8730=FACE_OUTER_BOUND('',#13995,.T.);
#8731=FACE_OUTER_BOUND('',#13996,.T.);
#8732=FACE_OUTER_BOUND('',#13997,.T.);
#8733=FACE_OUTER_BOUND('',#13998,.T.);
#8734=FACE_OUTER_BOUND('',#13999,.T.);
#8735=FACE_OUTER_BOUND('',#14000,.T.);
#8736=FACE_OUTER_BOUND('',#14001,.T.);
#8737=FACE_OUTER_BOUND('',#14002,.T.);
#8738=FACE_OUTER_BOUND('',#14003,.T.);
#8739=FACE_OUTER_BOUND('',#14004,.T.);
#8740=FACE_OUTER_BOUND('',#14005,.T.);
#8741=FACE_OUTER_BOUND('',#14006,.T.);
#8742=FACE_OUTER_BOUND('',#14007,.T.);
#8743=FACE_OUTER_BOUND('',#14008,.T.);
#8744=FACE_OUTER_BOUND('',#14009,.T.);
#8745=FACE_OUTER_BOUND('',#14010,.T.);
#8746=FACE_OUTER_BOUND('',#14011,.T.);
#8747=FACE_OUTER_BOUND('',#14012,.T.);
#8748=FACE_OUTER_BOUND('',#14013,.T.);
#8749=FACE_OUTER_BOUND('',#14014,.T.);
#8750=FACE_OUTER_BOUND('',#14015,.T.);
#8751=FACE_OUTER_BOUND('',#14016,.T.);
#8752=FACE_OUTER_BOUND('',#14017,.T.);
#8753=FACE_OUTER_BOUND('',#14018,.T.);
#8754=FACE_OUTER_BOUND('',#14019,.T.);
#8755=FACE_OUTER_BOUND('',#14020,.T.);
#8756=FACE_OUTER_BOUND('',#14021,.T.);
#8757=FACE_OUTER_BOUND('',#14022,.T.);
#8758=FACE_OUTER_BOUND('',#14023,.T.);
#8759=FACE_OUTER_BOUND('',#14024,.T.);
#8760=FACE_OUTER_BOUND('',#14025,.T.);
#8761=FACE_OUTER_BOUND('',#14026,.T.);
#8762=FACE_OUTER_BOUND('',#14027,.T.);
#8763=FACE_OUTER_BOUND('',#14028,.T.);
#8764=FACE_OUTER_BOUND('',#14029,.T.);
#8765=FACE_OUTER_BOUND('',#14030,.T.);
#8766=FACE_OUTER_BOUND('',#14031,.T.);
#8767=FACE_OUTER_BOUND('',#14032,.T.);
#8768=FACE_OUTER_BOUND('',#14033,.T.);
#8769=FACE_OUTER_BOUND('',#14034,.T.);
#8770=FACE_OUTER_BOUND('',#14035,.T.);
#8771=FACE_OUTER_BOUND('',#14036,.T.);
#8772=FACE_OUTER_BOUND('',#14037,.T.);
#8773=FACE_OUTER_BOUND('',#14038,.T.);
#8774=FACE_OUTER_BOUND('',#14039,.T.);
#8775=FACE_OUTER_BOUND('',#14040,.T.);
#8776=FACE_OUTER_BOUND('',#14041,.T.);
#8777=FACE_OUTER_BOUND('',#14042,.T.);
#8778=FACE_OUTER_BOUND('',#14043,.T.);
#8779=FACE_OUTER_BOUND('',#14044,.T.);
#8780=FACE_OUTER_BOUND('',#14045,.T.);
#8781=FACE_OUTER_BOUND('',#14046,.T.);
#8782=FACE_OUTER_BOUND('',#14047,.T.);
#8783=FACE_OUTER_BOUND('',#14048,.T.);
#8784=FACE_OUTER_BOUND('',#14049,.T.);
#8785=FACE_OUTER_BOUND('',#14050,.T.);
#8786=FACE_OUTER_BOUND('',#14051,.T.);
#8787=FACE_OUTER_BOUND('',#14052,.T.);
#8788=FACE_OUTER_BOUND('',#14053,.T.);
#8789=FACE_OUTER_BOUND('',#14054,.T.);
#8790=FACE_OUTER_BOUND('',#14055,.T.);
#8791=FACE_OUTER_BOUND('',#14056,.T.);
#8792=FACE_OUTER_BOUND('',#14057,.T.);
#8793=FACE_OUTER_BOUND('',#14058,.T.);
#8794=FACE_OUTER_BOUND('',#14059,.T.);
#8795=FACE_OUTER_BOUND('',#14060,.T.);
#8796=FACE_OUTER_BOUND('',#14061,.T.);
#8797=FACE_OUTER_BOUND('',#14062,.T.);
#8798=FACE_OUTER_BOUND('',#14063,.T.);
#8799=FACE_OUTER_BOUND('',#14064,.T.);
#8800=FACE_OUTER_BOUND('',#14065,.T.);
#8801=FACE_OUTER_BOUND('',#14066,.T.);
#8802=FACE_OUTER_BOUND('',#14067,.T.);
#8803=FACE_OUTER_BOUND('',#14068,.T.);
#8804=FACE_OUTER_BOUND('',#14069,.T.);
#8805=FACE_OUTER_BOUND('',#14070,.T.);
#8806=FACE_OUTER_BOUND('',#14071,.T.);
#8807=FACE_OUTER_BOUND('',#14072,.T.);
#8808=FACE_OUTER_BOUND('',#14073,.T.);
#8809=FACE_OUTER_BOUND('',#14074,.T.);
#8810=FACE_OUTER_BOUND('',#14075,.T.);
#8811=FACE_OUTER_BOUND('',#14076,.T.);
#8812=FACE_OUTER_BOUND('',#14077,.T.);
#8813=FACE_OUTER_BOUND('',#14078,.T.);
#8814=FACE_OUTER_BOUND('',#14079,.T.);
#8815=FACE_OUTER_BOUND('',#14080,.T.);
#8816=FACE_OUTER_BOUND('',#14081,.T.);
#8817=FACE_OUTER_BOUND('',#14082,.T.);
#8818=FACE_OUTER_BOUND('',#14083,.T.);
#8819=FACE_OUTER_BOUND('',#14084,.T.);
#8820=FACE_OUTER_BOUND('',#14085,.T.);
#8821=FACE_OUTER_BOUND('',#14086,.T.);
#8822=FACE_OUTER_BOUND('',#14087,.T.);
#8823=FACE_OUTER_BOUND('',#14088,.T.);
#8824=FACE_OUTER_BOUND('',#14089,.T.);
#8825=FACE_OUTER_BOUND('',#14090,.T.);
#8826=FACE_OUTER_BOUND('',#14091,.T.);
#8827=FACE_OUTER_BOUND('',#14092,.T.);
#8828=FACE_OUTER_BOUND('',#14093,.T.);
#8829=FACE_OUTER_BOUND('',#14094,.T.);
#8830=FACE_OUTER_BOUND('',#14095,.T.);
#8831=FACE_OUTER_BOUND('',#14096,.T.);
#8832=FACE_OUTER_BOUND('',#14097,.T.);
#8833=FACE_OUTER_BOUND('',#14098,.T.);
#8834=FACE_OUTER_BOUND('',#14099,.T.);
#8835=FACE_OUTER_BOUND('',#14100,.T.);
#8836=FACE_OUTER_BOUND('',#14101,.T.);
#8837=FACE_OUTER_BOUND('',#14102,.T.);
#8838=FACE_OUTER_BOUND('',#14103,.T.);
#8839=FACE_OUTER_BOUND('',#14104,.T.);
#8840=FACE_OUTER_BOUND('',#14105,.T.);
#8841=FACE_OUTER_BOUND('',#14106,.T.);
#8842=FACE_OUTER_BOUND('',#14107,.T.);
#8843=FACE_OUTER_BOUND('',#14108,.T.);
#8844=FACE_OUTER_BOUND('',#14109,.T.);
#8845=FACE_OUTER_BOUND('',#14110,.T.);
#8846=FACE_OUTER_BOUND('',#14111,.T.);
#8847=FACE_OUTER_BOUND('',#14112,.T.);
#8848=FACE_OUTER_BOUND('',#14113,.T.);
#8849=FACE_OUTER_BOUND('',#14114,.T.);
#8850=FACE_OUTER_BOUND('',#14115,.T.);
#8851=FACE_OUTER_BOUND('',#14116,.T.);
#8852=FACE_OUTER_BOUND('',#14117,.T.);
#8853=FACE_OUTER_BOUND('',#14118,.T.);
#8854=FACE_OUTER_BOUND('',#14119,.T.);
#8855=FACE_OUTER_BOUND('',#14120,.T.);
#8856=FACE_OUTER_BOUND('',#14121,.T.);
#8857=FACE_OUTER_BOUND('',#14122,.T.);
#8858=FACE_OUTER_BOUND('',#14123,.T.);
#8859=FACE_OUTER_BOUND('',#14124,.T.);
#8860=FACE_OUTER_BOUND('',#14125,.T.);
#8861=FACE_OUTER_BOUND('',#14126,.T.);
#8862=FACE_OUTER_BOUND('',#14127,.T.);
#8863=FACE_OUTER_BOUND('',#14128,.T.);
#8864=FACE_OUTER_BOUND('',#14129,.T.);
#8865=FACE_OUTER_BOUND('',#14130,.T.);
#8866=FACE_OUTER_BOUND('',#14131,.T.);
#8867=FACE_OUTER_BOUND('',#14132,.T.);
#8868=FACE_OUTER_BOUND('',#14133,.T.);
#8869=FACE_OUTER_BOUND('',#14134,.T.);
#8870=FACE_OUTER_BOUND('',#14135,.T.);
#8871=FACE_OUTER_BOUND('',#14136,.T.);
#8872=FACE_OUTER_BOUND('',#14137,.T.);
#8873=FACE_OUTER_BOUND('',#14138,.T.);
#8874=FACE_OUTER_BOUND('',#14139,.T.);
#8875=FACE_OUTER_BOUND('',#14140,.T.);
#8876=FACE_OUTER_BOUND('',#14141,.T.);
#8877=FACE_OUTER_BOUND('',#14142,.T.);
#8878=FACE_OUTER_BOUND('',#14143,.T.);
#8879=FACE_OUTER_BOUND('',#14144,.T.);
#8880=FACE_OUTER_BOUND('',#14145,.T.);
#8881=FACE_OUTER_BOUND('',#14146,.T.);
#8882=FACE_OUTER_BOUND('',#14147,.T.);
#8883=FACE_OUTER_BOUND('',#14148,.T.);
#8884=FACE_OUTER_BOUND('',#14149,.T.);
#8885=FACE_OUTER_BOUND('',#14150,.T.);
#8886=FACE_OUTER_BOUND('',#14151,.T.);
#8887=FACE_OUTER_BOUND('',#14152,.T.);
#8888=FACE_OUTER_BOUND('',#14153,.T.);
#8889=FACE_OUTER_BOUND('',#14154,.T.);
#8890=FACE_OUTER_BOUND('',#14155,.T.);
#8891=FACE_OUTER_BOUND('',#14156,.T.);
#8892=FACE_OUTER_BOUND('',#14157,.T.);
#8893=FACE_OUTER_BOUND('',#14158,.T.);
#8894=FACE_OUTER_BOUND('',#14159,.T.);
#8895=FACE_OUTER_BOUND('',#14160,.T.);
#8896=FACE_OUTER_BOUND('',#14161,.T.);
#8897=FACE_OUTER_BOUND('',#14162,.T.);
#8898=FACE_OUTER_BOUND('',#14163,.T.);
#8899=FACE_OUTER_BOUND('',#14164,.T.);
#8900=FACE_OUTER_BOUND('',#14165,.T.);
#8901=FACE_OUTER_BOUND('',#14166,.T.);
#8902=FACE_OUTER_BOUND('',#14167,.T.);
#8903=FACE_OUTER_BOUND('',#14168,.T.);
#8904=FACE_OUTER_BOUND('',#14169,.T.);
#8905=FACE_OUTER_BOUND('',#14170,.T.);
#8906=FACE_OUTER_BOUND('',#14171,.T.);
#8907=FACE_OUTER_BOUND('',#14172,.T.);
#8908=FACE_OUTER_BOUND('',#14173,.T.);
#8909=FACE_OUTER_BOUND('',#14174,.T.);
#8910=FACE_OUTER_BOUND('',#14175,.T.);
#8911=FACE_OUTER_BOUND('',#14176,.T.);
#8912=FACE_OUTER_BOUND('',#14177,.T.);
#8913=FACE_OUTER_BOUND('',#14178,.T.);
#8914=FACE_OUTER_BOUND('',#14179,.T.);
#8915=FACE_OUTER_BOUND('',#14180,.T.);
#8916=FACE_OUTER_BOUND('',#14181,.T.);
#8917=FACE_OUTER_BOUND('',#14182,.T.);
#8918=FACE_OUTER_BOUND('',#14183,.T.);
#8919=FACE_OUTER_BOUND('',#14184,.T.);
#8920=FACE_OUTER_BOUND('',#14185,.T.);
#8921=FACE_OUTER_BOUND('',#14186,.T.);
#8922=FACE_OUTER_BOUND('',#14187,.T.);
#8923=FACE_OUTER_BOUND('',#14188,.T.);
#8924=FACE_OUTER_BOUND('',#14189,.T.);
#8925=FACE_OUTER_BOUND('',#14190,.T.);
#8926=FACE_OUTER_BOUND('',#14191,.T.);
#8927=FACE_OUTER_BOUND('',#14192,.T.);
#8928=FACE_OUTER_BOUND('',#14193,.T.);
#8929=FACE_OUTER_BOUND('',#14194,.T.);
#8930=FACE_OUTER_BOUND('',#14195,.T.);
#8931=FACE_OUTER_BOUND('',#14196,.T.);
#8932=FACE_OUTER_BOUND('',#14197,.T.);
#8933=FACE_OUTER_BOUND('',#14198,.T.);
#8934=FACE_OUTER_BOUND('',#14199,.T.);
#8935=FACE_OUTER_BOUND('',#14200,.T.);
#8936=FACE_OUTER_BOUND('',#14201,.T.);
#8937=FACE_OUTER_BOUND('',#14202,.T.);
#8938=FACE_OUTER_BOUND('',#14203,.T.);
#8939=FACE_OUTER_BOUND('',#14204,.T.);
#8940=FACE_OUTER_BOUND('',#14205,.T.);
#8941=FACE_OUTER_BOUND('',#14206,.T.);
#8942=FACE_OUTER_BOUND('',#14207,.T.);
#8943=FACE_OUTER_BOUND('',#14208,.T.);
#8944=FACE_OUTER_BOUND('',#14209,.T.);
#8945=FACE_OUTER_BOUND('',#14210,.T.);
#8946=FACE_OUTER_BOUND('',#14211,.T.);
#8947=FACE_OUTER_BOUND('',#14212,.T.);
#8948=FACE_OUTER_BOUND('',#14213,.T.);
#8949=FACE_OUTER_BOUND('',#14214,.T.);
#8950=FACE_OUTER_BOUND('',#14215,.T.);
#8951=FACE_OUTER_BOUND('',#14216,.T.);
#8952=FACE_OUTER_BOUND('',#14217,.T.);
#8953=FACE_OUTER_BOUND('',#14218,.T.);
#8954=FACE_OUTER_BOUND('',#14219,.T.);
#8955=FACE_OUTER_BOUND('',#14220,.T.);
#8956=FACE_OUTER_BOUND('',#14221,.T.);
#8957=FACE_OUTER_BOUND('',#14222,.T.);
#8958=FACE_OUTER_BOUND('',#14223,.T.);
#8959=FACE_OUTER_BOUND('',#14224,.T.);
#8960=FACE_OUTER_BOUND('',#14225,.T.);
#8961=FACE_OUTER_BOUND('',#14226,.T.);
#8962=FACE_OUTER_BOUND('',#14227,.T.);
#8963=FACE_OUTER_BOUND('',#14228,.T.);
#8964=FACE_OUTER_BOUND('',#14229,.T.);
#8965=FACE_OUTER_BOUND('',#14230,.T.);
#8966=FACE_OUTER_BOUND('',#14231,.T.);
#8967=FACE_OUTER_BOUND('',#14232,.T.);
#8968=FACE_OUTER_BOUND('',#14233,.T.);
#8969=FACE_OUTER_BOUND('',#14234,.T.);
#8970=FACE_OUTER_BOUND('',#14235,.T.);
#8971=FACE_OUTER_BOUND('',#14236,.T.);
#8972=FACE_OUTER_BOUND('',#14237,.T.);
#8973=FACE_OUTER_BOUND('',#14238,.T.);
#8974=FACE_OUTER_BOUND('',#14239,.T.);
#8975=FACE_OUTER_BOUND('',#14240,.T.);
#8976=FACE_OUTER_BOUND('',#14241,.T.);
#8977=FACE_OUTER_BOUND('',#14242,.T.);
#8978=FACE_OUTER_BOUND('',#14243,.T.);
#8979=FACE_OUTER_BOUND('',#14244,.T.);
#8980=FACE_OUTER_BOUND('',#14245,.T.);
#8981=FACE_OUTER_BOUND('',#14246,.T.);
#8982=FACE_OUTER_BOUND('',#14247,.T.);
#8983=FACE_OUTER_BOUND('',#14248,.T.);
#8984=FACE_OUTER_BOUND('',#14249,.T.);
#8985=FACE_OUTER_BOUND('',#14250,.T.);
#8986=FACE_OUTER_BOUND('',#14251,.T.);
#8987=FACE_OUTER_BOUND('',#14252,.T.);
#8988=FACE_OUTER_BOUND('',#14253,.T.);
#8989=FACE_OUTER_BOUND('',#14254,.T.);
#8990=FACE_OUTER_BOUND('',#14255,.T.);
#8991=FACE_OUTER_BOUND('',#14256,.T.);
#8992=FACE_OUTER_BOUND('',#14257,.T.);
#8993=FACE_OUTER_BOUND('',#14258,.T.);
#8994=FACE_OUTER_BOUND('',#14259,.T.);
#8995=FACE_OUTER_BOUND('',#14260,.T.);
#8996=FACE_OUTER_BOUND('',#14261,.T.);
#8997=FACE_OUTER_BOUND('',#14262,.T.);
#8998=FACE_OUTER_BOUND('',#14263,.T.);
#8999=FACE_OUTER_BOUND('',#14264,.T.);
#9000=FACE_OUTER_BOUND('',#14265,.T.);
#9001=FACE_OUTER_BOUND('',#14266,.T.);
#9002=FACE_OUTER_BOUND('',#14267,.T.);
#9003=FACE_OUTER_BOUND('',#14268,.T.);
#9004=FACE_OUTER_BOUND('',#14269,.T.);
#9005=FACE_OUTER_BOUND('',#14270,.T.);
#9006=FACE_OUTER_BOUND('',#14271,.T.);
#9007=FACE_OUTER_BOUND('',#14272,.T.);
#9008=FACE_OUTER_BOUND('',#14273,.T.);
#9009=FACE_OUTER_BOUND('',#14274,.T.);
#9010=FACE_OUTER_BOUND('',#14275,.T.);
#9011=FACE_OUTER_BOUND('',#14276,.T.);
#9012=FACE_OUTER_BOUND('',#14277,.T.);
#9013=FACE_OUTER_BOUND('',#14278,.T.);
#9014=FACE_OUTER_BOUND('',#14279,.T.);
#9015=FACE_OUTER_BOUND('',#14280,.T.);
#9016=FACE_OUTER_BOUND('',#14281,.T.);
#9017=FACE_OUTER_BOUND('',#14282,.T.);
#9018=FACE_OUTER_BOUND('',#14283,.T.);
#9019=FACE_OUTER_BOUND('',#14284,.T.);
#9020=FACE_OUTER_BOUND('',#14285,.T.);
#9021=FACE_OUTER_BOUND('',#14286,.T.);
#9022=FACE_OUTER_BOUND('',#14287,.T.);
#9023=FACE_OUTER_BOUND('',#14288,.T.);
#9024=FACE_OUTER_BOUND('',#14289,.T.);
#9025=FACE_OUTER_BOUND('',#14290,.T.);
#9026=FACE_OUTER_BOUND('',#14291,.T.);
#9027=FACE_OUTER_BOUND('',#14292,.T.);
#9028=FACE_OUTER_BOUND('',#14293,.T.);
#9029=FACE_OUTER_BOUND('',#14294,.T.);
#9030=FACE_OUTER_BOUND('',#14295,.T.);
#9031=FACE_OUTER_BOUND('',#14296,.T.);
#9032=FACE_OUTER_BOUND('',#14297,.T.);
#9033=FACE_OUTER_BOUND('',#14298,.T.);
#9034=FACE_OUTER_BOUND('',#14299,.T.);
#9035=FACE_OUTER_BOUND('',#14300,.T.);
#9036=FACE_OUTER_BOUND('',#14301,.T.);
#9037=FACE_OUTER_BOUND('',#14302,.T.);
#9038=FACE_OUTER_BOUND('',#14303,.T.);
#9039=FACE_OUTER_BOUND('',#14304,.T.);
#9040=FACE_OUTER_BOUND('',#14305,.T.);
#9041=FACE_OUTER_BOUND('',#14306,.T.);
#9042=FACE_OUTER_BOUND('',#14307,.T.);
#9043=FACE_OUTER_BOUND('',#14308,.T.);
#9044=FACE_OUTER_BOUND('',#14309,.T.);
#9045=FACE_OUTER_BOUND('',#14310,.T.);
#9046=FACE_OUTER_BOUND('',#14311,.T.);
#9047=FACE_OUTER_BOUND('',#14312,.T.);
#9048=FACE_OUTER_BOUND('',#14313,.T.);
#9049=FACE_OUTER_BOUND('',#14314,.T.);
#9050=FACE_OUTER_BOUND('',#14315,.T.);
#9051=FACE_OUTER_BOUND('',#14316,.T.);
#9052=FACE_OUTER_BOUND('',#14317,.T.);
#9053=FACE_OUTER_BOUND('',#14318,.T.);
#9054=FACE_OUTER_BOUND('',#14319,.T.);
#9055=FACE_OUTER_BOUND('',#14320,.T.);
#9056=FACE_OUTER_BOUND('',#14321,.T.);
#9057=FACE_OUTER_BOUND('',#14322,.T.);
#9058=FACE_OUTER_BOUND('',#14323,.T.);
#9059=FACE_OUTER_BOUND('',#14324,.T.);
#9060=FACE_OUTER_BOUND('',#14325,.T.);
#9061=FACE_OUTER_BOUND('',#14326,.T.);
#9062=FACE_OUTER_BOUND('',#14327,.T.);
#9063=FACE_OUTER_BOUND('',#14328,.T.);
#9064=FACE_OUTER_BOUND('',#14329,.T.);
#9065=FACE_OUTER_BOUND('',#14330,.T.);
#9066=FACE_OUTER_BOUND('',#14331,.T.);
#9067=FACE_OUTER_BOUND('',#14332,.T.);
#9068=FACE_OUTER_BOUND('',#14333,.T.);
#9069=FACE_OUTER_BOUND('',#14334,.T.);
#9070=FACE_OUTER_BOUND('',#14335,.T.);
#9071=FACE_OUTER_BOUND('',#14336,.T.);
#9072=FACE_OUTER_BOUND('',#14337,.T.);
#9073=FACE_OUTER_BOUND('',#14338,.T.);
#9074=FACE_OUTER_BOUND('',#14339,.T.);
#9075=FACE_OUTER_BOUND('',#14340,.T.);
#9076=FACE_OUTER_BOUND('',#14341,.T.);
#9077=FACE_OUTER_BOUND('',#14342,.T.);
#9078=FACE_OUTER_BOUND('',#14343,.T.);
#9079=FACE_OUTER_BOUND('',#14344,.T.);
#9080=FACE_OUTER_BOUND('',#14345,.T.);
#9081=FACE_OUTER_BOUND('',#14346,.T.);
#9082=FACE_OUTER_BOUND('',#14347,.T.);
#9083=FACE_OUTER_BOUND('',#14348,.T.);
#9084=FACE_OUTER_BOUND('',#14349,.T.);
#9085=FACE_OUTER_BOUND('',#14350,.T.);
#9086=FACE_OUTER_BOUND('',#14351,.T.);
#9087=FACE_OUTER_BOUND('',#14352,.T.);
#9088=FACE_OUTER_BOUND('',#14353,.T.);
#9089=FACE_OUTER_BOUND('',#14354,.T.);
#9090=FACE_OUTER_BOUND('',#14355,.T.);
#9091=FACE_OUTER_BOUND('',#14356,.T.);
#9092=FACE_OUTER_BOUND('',#14357,.T.);
#9093=FACE_OUTER_BOUND('',#14358,.T.);
#9094=FACE_OUTER_BOUND('',#14359,.T.);
#9095=FACE_OUTER_BOUND('',#14360,.T.);
#9096=FACE_OUTER_BOUND('',#14361,.T.);
#9097=FACE_OUTER_BOUND('',#14362,.T.);
#9098=FACE_OUTER_BOUND('',#14363,.T.);
#9099=FACE_OUTER_BOUND('',#14364,.T.);
#9100=FACE_OUTER_BOUND('',#14365,.T.);
#9101=FACE_OUTER_BOUND('',#14366,.T.);
#9102=FACE_OUTER_BOUND('',#14367,.T.);
#9103=FACE_OUTER_BOUND('',#14368,.T.);
#9104=FACE_OUTER_BOUND('',#14369,.T.);
#9105=FACE_OUTER_BOUND('',#14370,.T.);
#9106=FACE_OUTER_BOUND('',#14371,.T.);
#9107=FACE_OUTER_BOUND('',#14372,.T.);
#9108=FACE_OUTER_BOUND('',#14373,.T.);
#9109=FACE_OUTER_BOUND('',#14374,.T.);
#9110=FACE_OUTER_BOUND('',#14375,.T.);
#9111=FACE_OUTER_BOUND('',#14376,.T.);
#9112=FACE_OUTER_BOUND('',#14377,.T.);
#9113=FACE_OUTER_BOUND('',#14378,.T.);
#9114=FACE_OUTER_BOUND('',#14379,.T.);
#9115=FACE_OUTER_BOUND('',#14380,.T.);
#9116=FACE_OUTER_BOUND('',#14381,.T.);
#9117=FACE_OUTER_BOUND('',#14382,.T.);
#9118=FACE_OUTER_BOUND('',#14383,.T.);
#9119=FACE_OUTER_BOUND('',#14384,.T.);
#9120=FACE_OUTER_BOUND('',#14385,.T.);
#9121=FACE_OUTER_BOUND('',#14386,.T.);
#9122=FACE_OUTER_BOUND('',#14387,.T.);
#9123=FACE_OUTER_BOUND('',#14388,.T.);
#9124=FACE_OUTER_BOUND('',#14389,.T.);
#9125=FACE_OUTER_BOUND('',#14390,.T.);
#9126=FACE_OUTER_BOUND('',#14391,.T.);
#9127=FACE_OUTER_BOUND('',#14392,.T.);
#9128=FACE_OUTER_BOUND('',#14393,.T.);
#9129=FACE_OUTER_BOUND('',#14394,.T.);
#9130=FACE_OUTER_BOUND('',#14395,.T.);
#9131=FACE_OUTER_BOUND('',#14396,.T.);
#9132=FACE_OUTER_BOUND('',#14397,.T.);
#9133=FACE_OUTER_BOUND('',#14398,.T.);
#9134=FACE_OUTER_BOUND('',#14399,.T.);
#9135=FACE_OUTER_BOUND('',#14400,.T.);
#9136=FACE_OUTER_BOUND('',#14401,.T.);
#9137=FACE_OUTER_BOUND('',#14402,.T.);
#9138=FACE_OUTER_BOUND('',#14403,.T.);
#9139=FACE_OUTER_BOUND('',#14404,.T.);
#9140=FACE_OUTER_BOUND('',#14405,.T.);
#9141=FACE_OUTER_BOUND('',#14406,.T.);
#9142=FACE_OUTER_BOUND('',#14407,.T.);
#9143=FACE_OUTER_BOUND('',#14408,.T.);
#9144=FACE_OUTER_BOUND('',#14409,.T.);
#9145=FACE_OUTER_BOUND('',#14410,.T.);
#9146=FACE_OUTER_BOUND('',#14411,.T.);
#9147=FACE_OUTER_BOUND('',#14412,.T.);
#9148=FACE_OUTER_BOUND('',#14413,.T.);
#9149=FACE_OUTER_BOUND('',#14414,.T.);
#9150=FACE_OUTER_BOUND('',#14415,.T.);
#9151=FACE_OUTER_BOUND('',#14416,.T.);
#9152=FACE_OUTER_BOUND('',#14417,.T.);
#9153=FACE_OUTER_BOUND('',#14418,.T.);
#9154=FACE_OUTER_BOUND('',#14419,.T.);
#9155=FACE_OUTER_BOUND('',#14420,.T.);
#9156=FACE_OUTER_BOUND('',#14421,.T.);
#9157=FACE_OUTER_BOUND('',#14422,.T.);
#9158=FACE_OUTER_BOUND('',#14423,.T.);
#9159=FACE_OUTER_BOUND('',#14424,.T.);
#9160=FACE_OUTER_BOUND('',#14425,.T.);
#9161=FACE_OUTER_BOUND('',#14426,.T.);
#9162=FACE_OUTER_BOUND('',#14427,.T.);
#9163=FACE_OUTER_BOUND('',#14428,.T.);
#9164=FACE_OUTER_BOUND('',#14429,.T.);
#9165=FACE_OUTER_BOUND('',#14430,.T.);
#9166=FACE_OUTER_BOUND('',#14431,.T.);
#9167=FACE_OUTER_BOUND('',#14432,.T.);
#9168=FACE_OUTER_BOUND('',#14433,.T.);
#9169=FACE_OUTER_BOUND('',#14434,.T.);
#9170=FACE_OUTER_BOUND('',#14435,.T.);
#9171=FACE_OUTER_BOUND('',#14436,.T.);
#9172=FACE_OUTER_BOUND('',#14437,.T.);
#9173=FACE_OUTER_BOUND('',#14438,.T.);
#9174=FACE_OUTER_BOUND('',#14439,.T.);
#9175=FACE_OUTER_BOUND('',#14440,.T.);
#9176=FACE_OUTER_BOUND('',#14441,.T.);
#9177=FACE_OUTER_BOUND('',#14442,.T.);
#9178=FACE_OUTER_BOUND('',#14443,.T.);
#9179=FACE_OUTER_BOUND('',#14444,.T.);
#9180=FACE_OUTER_BOUND('',#14445,.T.);
#9181=FACE_OUTER_BOUND('',#14446,.T.);
#9182=FACE_OUTER_BOUND('',#14447,.T.);
#9183=FACE_OUTER_BOUND('',#14448,.T.);
#9184=FACE_OUTER_BOUND('',#14449,.T.);
#9185=FACE_OUTER_BOUND('',#14450,.T.);
#9186=FACE_OUTER_BOUND('',#14451,.T.);
#9187=FACE_OUTER_BOUND('',#14452,.T.);
#9188=FACE_OUTER_BOUND('',#14453,.T.);
#9189=FACE_OUTER_BOUND('',#14454,.T.);
#9190=FACE_OUTER_BOUND('',#14455,.T.);
#9191=FACE_OUTER_BOUND('',#14456,.T.);
#9192=FACE_OUTER_BOUND('',#14457,.T.);
#9193=FACE_OUTER_BOUND('',#14458,.T.);
#9194=FACE_OUTER_BOUND('',#14459,.T.);
#9195=FACE_OUTER_BOUND('',#14460,.T.);
#9196=FACE_OUTER_BOUND('',#14461,.T.);
#9197=FACE_OUTER_BOUND('',#14462,.T.);
#9198=FACE_OUTER_BOUND('',#14463,.T.);
#9199=FACE_OUTER_BOUND('',#14464,.T.);
#9200=FACE_OUTER_BOUND('',#14465,.T.);
#9201=FACE_OUTER_BOUND('',#14466,.T.);
#9202=FACE_OUTER_BOUND('',#14467,.T.);
#9203=FACE_OUTER_BOUND('',#14468,.T.);
#9204=FACE_OUTER_BOUND('',#14469,.T.);
#9205=FACE_OUTER_BOUND('',#14470,.T.);
#9206=FACE_OUTER_BOUND('',#14471,.T.);
#9207=FACE_OUTER_BOUND('',#14472,.T.);
#9208=FACE_OUTER_BOUND('',#14473,.T.);
#9209=FACE_OUTER_BOUND('',#14474,.T.);
#9210=FACE_OUTER_BOUND('',#14475,.T.);
#9211=FACE_OUTER_BOUND('',#14476,.T.);
#9212=FACE_OUTER_BOUND('',#14477,.T.);
#9213=FACE_OUTER_BOUND('',#14478,.T.);
#9214=FACE_OUTER_BOUND('',#14479,.T.);
#9215=FACE_OUTER_BOUND('',#14480,.T.);
#9216=FACE_OUTER_BOUND('',#14481,.T.);
#9217=FACE_OUTER_BOUND('',#14482,.T.);
#9218=FACE_OUTER_BOUND('',#14483,.T.);
#9219=FACE_OUTER_BOUND('',#14484,.T.);
#9220=FACE_OUTER_BOUND('',#14485,.T.);
#9221=FACE_OUTER_BOUND('',#14486,.T.);
#9222=FACE_OUTER_BOUND('',#14487,.T.);
#9223=FACE_OUTER_BOUND('',#14488,.T.);
#9224=FACE_OUTER_BOUND('',#14489,.T.);
#9225=FACE_OUTER_BOUND('',#14490,.T.);
#9226=FACE_OUTER_BOUND('',#14491,.T.);
#9227=FACE_OUTER_BOUND('',#14492,.T.);
#9228=FACE_OUTER_BOUND('',#14493,.T.);
#9229=FACE_OUTER_BOUND('',#14494,.T.);
#9230=FACE_OUTER_BOUND('',#14495,.T.);
#9231=FACE_OUTER_BOUND('',#14496,.T.);
#9232=FACE_OUTER_BOUND('',#14497,.T.);
#9233=FACE_OUTER_BOUND('',#14498,.T.);
#9234=FACE_OUTER_BOUND('',#14499,.T.);
#9235=FACE_OUTER_BOUND('',#14500,.T.);
#9236=FACE_OUTER_BOUND('',#14501,.T.);
#9237=FACE_OUTER_BOUND('',#14502,.T.);
#9238=FACE_OUTER_BOUND('',#14503,.T.);
#9239=FACE_OUTER_BOUND('',#14504,.T.);
#9240=FACE_OUTER_BOUND('',#14505,.T.);
#9241=FACE_OUTER_BOUND('',#14506,.T.);
#9242=FACE_OUTER_BOUND('',#14507,.T.);
#9243=FACE_OUTER_BOUND('',#14508,.T.);
#9244=FACE_OUTER_BOUND('',#14509,.T.);
#9245=FACE_OUTER_BOUND('',#14510,.T.);
#9246=FACE_OUTER_BOUND('',#14511,.T.);
#9247=FACE_OUTER_BOUND('',#14512,.T.);
#9248=FACE_OUTER_BOUND('',#14513,.T.);
#9249=FACE_OUTER_BOUND('',#14514,.T.);
#9250=FACE_OUTER_BOUND('',#14515,.T.);
#9251=FACE_OUTER_BOUND('',#14516,.T.);
#9252=FACE_OUTER_BOUND('',#14517,.T.);
#9253=FACE_OUTER_BOUND('',#14518,.T.);
#9254=FACE_OUTER_BOUND('',#14519,.T.);
#9255=FACE_OUTER_BOUND('',#14520,.T.);
#9256=FACE_OUTER_BOUND('',#14521,.T.);
#9257=FACE_OUTER_BOUND('',#14522,.T.);
#9258=FACE_OUTER_BOUND('',#14523,.T.);
#9259=FACE_OUTER_BOUND('',#14524,.T.);
#9260=FACE_OUTER_BOUND('',#14525,.T.);
#9261=FACE_OUTER_BOUND('',#14526,.T.);
#9262=FACE_OUTER_BOUND('',#14527,.T.);
#9263=FACE_OUTER_BOUND('',#14528,.T.);
#9264=FACE_OUTER_BOUND('',#14529,.T.);
#9265=FACE_OUTER_BOUND('',#14530,.T.);
#9266=FACE_OUTER_BOUND('',#14531,.T.);
#9267=FACE_OUTER_BOUND('',#14532,.T.);
#9268=FACE_OUTER_BOUND('',#14533,.T.);
#9269=FACE_OUTER_BOUND('',#14534,.T.);
#9270=FACE_OUTER_BOUND('',#14535,.T.);
#9271=FACE_OUTER_BOUND('',#14536,.T.);
#9272=FACE_OUTER_BOUND('',#14537,.T.);
#9273=FACE_OUTER_BOUND('',#14538,.T.);
#9274=FACE_OUTER_BOUND('',#14539,.T.);
#9275=FACE_OUTER_BOUND('',#14540,.T.);
#9276=FACE_OUTER_BOUND('',#14541,.T.);
#9277=FACE_OUTER_BOUND('',#14542,.T.);
#9278=FACE_OUTER_BOUND('',#14543,.T.);
#9279=FACE_OUTER_BOUND('',#14544,.T.);
#9280=FACE_OUTER_BOUND('',#14545,.T.);
#9281=FACE_OUTER_BOUND('',#14546,.T.);
#9282=FACE_OUTER_BOUND('',#14547,.T.);
#9283=FACE_OUTER_BOUND('',#14548,.T.);
#9284=FACE_OUTER_BOUND('',#14549,.T.);
#9285=FACE_OUTER_BOUND('',#14550,.T.);
#9286=FACE_OUTER_BOUND('',#14551,.T.);
#9287=FACE_OUTER_BOUND('',#14552,.T.);
#9288=FACE_OUTER_BOUND('',#14553,.T.);
#9289=FACE_OUTER_BOUND('',#14554,.T.);
#9290=FACE_OUTER_BOUND('',#14555,.T.);
#9291=FACE_OUTER_BOUND('',#14556,.T.);
#9292=FACE_OUTER_BOUND('',#14557,.T.);
#9293=FACE_OUTER_BOUND('',#14558,.T.);
#9294=FACE_OUTER_BOUND('',#14559,.T.);
#9295=FACE_OUTER_BOUND('',#14560,.T.);
#9296=FACE_OUTER_BOUND('',#14561,.T.);
#9297=FACE_OUTER_BOUND('',#14562,.T.);
#9298=FACE_OUTER_BOUND('',#14563,.T.);
#9299=FACE_OUTER_BOUND('',#14564,.T.);
#9300=FACE_OUTER_BOUND('',#14565,.T.);
#9301=FACE_OUTER_BOUND('',#14566,.T.);
#9302=FACE_OUTER_BOUND('',#14567,.T.);
#9303=FACE_OUTER_BOUND('',#14568,.T.);
#9304=FACE_OUTER_BOUND('',#14569,.T.);
#9305=FACE_OUTER_BOUND('',#14570,.T.);
#9306=FACE_OUTER_BOUND('',#14571,.T.);
#9307=FACE_OUTER_BOUND('',#14572,.T.);
#9308=FACE_OUTER_BOUND('',#14573,.T.);
#9309=FACE_OUTER_BOUND('',#14574,.T.);
#9310=FACE_OUTER_BOUND('',#14575,.T.);
#9311=FACE_OUTER_BOUND('',#14576,.T.);
#9312=FACE_OUTER_BOUND('',#14577,.T.);
#9313=FACE_OUTER_BOUND('',#14578,.T.);
#9314=FACE_OUTER_BOUND('',#14579,.T.);
#9315=FACE_OUTER_BOUND('',#14580,.T.);
#9316=FACE_OUTER_BOUND('',#14581,.T.);
#9317=FACE_OUTER_BOUND('',#14582,.T.);
#9318=FACE_OUTER_BOUND('',#14583,.T.);
#9319=FACE_OUTER_BOUND('',#14584,.T.);
#9320=FACE_OUTER_BOUND('',#14585,.T.);
#9321=FACE_OUTER_BOUND('',#14586,.T.);
#9322=FACE_OUTER_BOUND('',#14587,.T.);
#9323=FACE_OUTER_BOUND('',#14588,.T.);
#9324=FACE_OUTER_BOUND('',#14589,.T.);
#9325=FACE_OUTER_BOUND('',#14590,.T.);
#9326=FACE_OUTER_BOUND('',#14591,.T.);
#9327=FACE_OUTER_BOUND('',#14592,.T.);
#9328=FACE_OUTER_BOUND('',#14593,.T.);
#9329=FACE_OUTER_BOUND('',#14594,.T.);
#9330=FACE_OUTER_BOUND('',#14595,.T.);
#9331=FACE_OUTER_BOUND('',#14596,.T.);
#9332=FACE_OUTER_BOUND('',#14597,.T.);
#9333=FACE_OUTER_BOUND('',#14598,.T.);
#9334=FACE_OUTER_BOUND('',#14599,.T.);
#9335=FACE_OUTER_BOUND('',#14600,.T.);
#9336=FACE_OUTER_BOUND('',#14601,.T.);
#9337=FACE_OUTER_BOUND('',#14602,.T.);
#9338=FACE_OUTER_BOUND('',#14603,.T.);
#9339=FACE_OUTER_BOUND('',#14604,.T.);
#9340=FACE_OUTER_BOUND('',#14605,.T.);
#9341=FACE_OUTER_BOUND('',#14606,.T.);
#9342=FACE_OUTER_BOUND('',#14607,.T.);
#9343=FACE_OUTER_BOUND('',#14608,.T.);
#9344=FACE_OUTER_BOUND('',#14609,.T.);
#9345=FACE_OUTER_BOUND('',#14610,.T.);
#9346=FACE_OUTER_BOUND('',#14611,.T.);
#9347=FACE_OUTER_BOUND('',#14612,.T.);
#9348=FACE_OUTER_BOUND('',#14613,.T.);
#9349=FACE_OUTER_BOUND('',#14614,.T.);
#9350=FACE_OUTER_BOUND('',#14615,.T.);
#9351=FACE_OUTER_BOUND('',#14616,.T.);
#9352=FACE_OUTER_BOUND('',#14617,.T.);
#9353=FACE_OUTER_BOUND('',#14618,.T.);
#9354=FACE_OUTER_BOUND('',#14619,.T.);
#9355=FACE_OUTER_BOUND('',#14620,.T.);
#9356=FACE_OUTER_BOUND('',#14621,.T.);
#9357=FACE_OUTER_BOUND('',#14622,.T.);
#9358=FACE_OUTER_BOUND('',#14623,.T.);
#9359=FACE_OUTER_BOUND('',#14624,.T.);
#9360=FACE_OUTER_BOUND('',#14625,.T.);
#9361=FACE_OUTER_BOUND('',#14626,.T.);
#9362=FACE_OUTER_BOUND('',#14627,.T.);
#9363=FACE_OUTER_BOUND('',#14628,.T.);
#9364=FACE_OUTER_BOUND('',#14629,.T.);
#9365=FACE_OUTER_BOUND('',#14630,.T.);
#9366=FACE_OUTER_BOUND('',#14631,.T.);
#9367=FACE_OUTER_BOUND('',#14632,.T.);
#9368=FACE_OUTER_BOUND('',#14633,.T.);
#9369=FACE_OUTER_BOUND('',#14634,.T.);
#9370=FACE_OUTER_BOUND('',#14635,.T.);
#9371=FACE_OUTER_BOUND('',#14636,.T.);
#9372=FACE_OUTER_BOUND('',#14637,.T.);
#9373=FACE_OUTER_BOUND('',#14638,.T.);
#9374=FACE_OUTER_BOUND('',#14639,.T.);
#9375=FACE_OUTER_BOUND('',#14640,.T.);
#9376=FACE_OUTER_BOUND('',#14641,.T.);
#9377=FACE_OUTER_BOUND('',#14642,.T.);
#9378=FACE_OUTER_BOUND('',#14643,.T.);
#9379=FACE_OUTER_BOUND('',#14644,.T.);
#9380=FACE_OUTER_BOUND('',#14645,.T.);
#9381=FACE_OUTER_BOUND('',#14646,.T.);
#9382=FACE_OUTER_BOUND('',#14647,.T.);
#9383=FACE_OUTER_BOUND('',#14648,.T.);
#9384=FACE_OUTER_BOUND('',#14649,.T.);
#9385=FACE_OUTER_BOUND('',#14650,.T.);
#9386=FACE_OUTER_BOUND('',#14651,.T.);
#9387=FACE_OUTER_BOUND('',#14652,.T.);
#9388=FACE_OUTER_BOUND('',#14653,.T.);
#9389=FACE_OUTER_BOUND('',#14654,.T.);
#9390=FACE_OUTER_BOUND('',#14655,.T.);
#9391=FACE_OUTER_BOUND('',#14656,.T.);
#9392=FACE_OUTER_BOUND('',#14657,.T.);
#9393=FACE_OUTER_BOUND('',#14658,.T.);
#9394=FACE_OUTER_BOUND('',#14659,.T.);
#9395=FACE_OUTER_BOUND('',#14660,.T.);
#9396=FACE_OUTER_BOUND('',#14661,.T.);
#9397=FACE_OUTER_BOUND('',#14662,.T.);
#9398=FACE_OUTER_BOUND('',#14663,.T.);
#9399=FACE_OUTER_BOUND('',#14664,.T.);
#9400=FACE_OUTER_BOUND('',#14665,.T.);
#9401=FACE_OUTER_BOUND('',#14666,.T.);
#9402=FACE_OUTER_BOUND('',#14667,.T.);
#9403=FACE_OUTER_BOUND('',#14668,.T.);
#9404=FACE_OUTER_BOUND('',#14669,.T.);
#9405=FACE_OUTER_BOUND('',#14670,.T.);
#9406=FACE_OUTER_BOUND('',#14671,.T.);
#9407=FACE_OUTER_BOUND('',#14672,.T.);
#9408=FACE_OUTER_BOUND('',#14673,.T.);
#9409=FACE_OUTER_BOUND('',#14674,.T.);
#9410=FACE_OUTER_BOUND('',#14675,.T.);
#9411=FACE_OUTER_BOUND('',#14676,.T.);
#9412=FACE_OUTER_BOUND('',#14677,.T.);
#9413=FACE_OUTER_BOUND('',#14678,.T.);
#9414=FACE_OUTER_BOUND('',#14679,.T.);
#9415=FACE_OUTER_BOUND('',#14680,.T.);
#9416=FACE_OUTER_BOUND('',#14681,.T.);
#9417=FACE_OUTER_BOUND('',#14682,.T.);
#9418=FACE_OUTER_BOUND('',#14683,.T.);
#9419=FACE_OUTER_BOUND('',#14684,.T.);
#9420=FACE_OUTER_BOUND('',#14685,.T.);
#9421=FACE_OUTER_BOUND('',#14686,.T.);
#9422=FACE_OUTER_BOUND('',#14687,.T.);
#9423=FACE_OUTER_BOUND('',#14688,.T.);
#9424=FACE_OUTER_BOUND('',#14689,.T.);
#9425=FACE_OUTER_BOUND('',#14690,.T.);
#9426=FACE_OUTER_BOUND('',#14691,.T.);
#9427=FACE_OUTER_BOUND('',#14692,.T.);
#9428=FACE_OUTER_BOUND('',#14693,.T.);
#9429=FACE_OUTER_BOUND('',#14694,.T.);
#9430=FACE_OUTER_BOUND('',#14695,.T.);
#9431=FACE_OUTER_BOUND('',#14696,.T.);
#9432=FACE_OUTER_BOUND('',#14697,.T.);
#9433=FACE_OUTER_BOUND('',#14698,.T.);
#9434=FACE_OUTER_BOUND('',#14699,.T.);
#9435=FACE_OUTER_BOUND('',#14700,.T.);
#9436=FACE_OUTER_BOUND('',#14701,.T.);
#9437=FACE_OUTER_BOUND('',#14702,.T.);
#9438=FACE_OUTER_BOUND('',#14703,.T.);
#9439=FACE_OUTER_BOUND('',#14704,.T.);
#9440=FACE_OUTER_BOUND('',#14705,.T.);
#9441=FACE_OUTER_BOUND('',#14706,.T.);
#9442=FACE_OUTER_BOUND('',#14707,.T.);
#9443=FACE_OUTER_BOUND('',#14708,.T.);
#9444=FACE_OUTER_BOUND('',#14709,.T.);
#9445=FACE_OUTER_BOUND('',#14710,.T.);
#9446=FACE_OUTER_BOUND('',#14711,.T.);
#9447=FACE_OUTER_BOUND('',#14712,.T.);
#9448=FACE_OUTER_BOUND('',#14713,.T.);
#9449=FACE_OUTER_BOUND('',#14714,.T.);
#9450=FACE_OUTER_BOUND('',#14715,.T.);
#9451=FACE_OUTER_BOUND('',#14716,.T.);
#9452=FACE_OUTER_BOUND('',#14717,.T.);
#9453=FACE_OUTER_BOUND('',#14718,.T.);
#9454=FACE_OUTER_BOUND('',#14719,.T.);
#9455=FACE_OUTER_BOUND('',#14720,.T.);
#9456=FACE_OUTER_BOUND('',#14721,.T.);
#9457=FACE_OUTER_BOUND('',#14722,.T.);
#9458=FACE_OUTER_BOUND('',#14723,.T.);
#9459=FACE_OUTER_BOUND('',#14724,.T.);
#9460=FACE_OUTER_BOUND('',#14725,.T.);
#9461=FACE_OUTER_BOUND('',#14726,.T.);
#9462=FACE_OUTER_BOUND('',#14727,.T.);
#9463=FACE_OUTER_BOUND('',#14728,.T.);
#9464=FACE_OUTER_BOUND('',#14729,.T.);
#9465=FACE_OUTER_BOUND('',#14730,.T.);
#9466=FACE_OUTER_BOUND('',#14731,.T.);
#9467=FACE_OUTER_BOUND('',#14732,.T.);
#9468=FACE_OUTER_BOUND('',#14733,.T.);
#9469=FACE_OUTER_BOUND('',#14734,.T.);
#9470=FACE_OUTER_BOUND('',#14735,.T.);
#9471=FACE_OUTER_BOUND('',#14736,.T.);
#9472=FACE_OUTER_BOUND('',#14737,.T.);
#9473=FACE_OUTER_BOUND('',#14738,.T.);
#9474=FACE_OUTER_BOUND('',#14739,.T.);
#9475=FACE_OUTER_BOUND('',#14740,.T.);
#9476=FACE_OUTER_BOUND('',#14741,.T.);
#9477=FACE_OUTER_BOUND('',#14742,.T.);
#9478=FACE_OUTER_BOUND('',#14743,.T.);
#9479=FACE_OUTER_BOUND('',#14744,.T.);
#9480=FACE_OUTER_BOUND('',#14745,.T.);
#9481=FACE_OUTER_BOUND('',#14746,.T.);
#9482=FACE_OUTER_BOUND('',#14747,.T.);
#9483=FACE_OUTER_BOUND('',#14748,.T.);
#9484=FACE_OUTER_BOUND('',#14749,.T.);
#9485=FACE_OUTER_BOUND('',#14750,.T.);
#9486=FACE_OUTER_BOUND('',#14751,.T.);
#9487=FACE_OUTER_BOUND('',#14752,.T.);
#9488=FACE_OUTER_BOUND('',#14753,.T.);
#9489=FACE_OUTER_BOUND('',#14754,.T.);
#9490=FACE_OUTER_BOUND('',#14755,.T.);
#9491=FACE_OUTER_BOUND('',#14756,.T.);
#9492=FACE_OUTER_BOUND('',#14757,.T.);
#9493=FACE_OUTER_BOUND('',#14758,.T.);
#9494=FACE_OUTER_BOUND('',#14759,.T.);
#9495=FACE_OUTER_BOUND('',#14760,.T.);
#9496=FACE_OUTER_BOUND('',#14761,.T.);
#9497=FACE_OUTER_BOUND('',#14762,.T.);
#9498=FACE_OUTER_BOUND('',#14763,.T.);
#9499=FACE_OUTER_BOUND('',#14764,.T.);
#9500=FACE_OUTER_BOUND('',#14765,.T.);
#9501=FACE_OUTER_BOUND('',#14766,.T.);
#9502=FACE_OUTER_BOUND('',#14767,.T.);
#9503=FACE_OUTER_BOUND('',#14768,.T.);
#9504=FACE_OUTER_BOUND('',#14769,.T.);
#9505=FACE_OUTER_BOUND('',#14770,.T.);
#9506=FACE_OUTER_BOUND('',#14771,.T.);
#9507=FACE_OUTER_BOUND('',#14772,.T.);
#9508=FACE_OUTER_BOUND('',#14773,.T.);
#9509=FACE_OUTER_BOUND('',#14774,.T.);
#9510=FACE_OUTER_BOUND('',#14775,.T.);
#9511=FACE_OUTER_BOUND('',#14776,.T.);
#9512=FACE_OUTER_BOUND('',#14777,.T.);
#9513=FACE_OUTER_BOUND('',#14778,.T.);
#9514=FACE_OUTER_BOUND('',#14779,.T.);
#9515=FACE_OUTER_BOUND('',#14780,.T.);
#9516=FACE_OUTER_BOUND('',#14781,.T.);
#9517=FACE_OUTER_BOUND('',#14782,.T.);
#9518=FACE_OUTER_BOUND('',#14783,.T.);
#9519=FACE_OUTER_BOUND('',#14784,.T.);
#9520=FACE_OUTER_BOUND('',#14785,.T.);
#9521=FACE_OUTER_BOUND('',#14786,.T.);
#9522=FACE_OUTER_BOUND('',#14787,.T.);
#9523=FACE_OUTER_BOUND('',#14788,.T.);
#9524=FACE_OUTER_BOUND('',#14789,.T.);
#9525=FACE_OUTER_BOUND('',#14790,.T.);
#9526=FACE_OUTER_BOUND('',#14791,.T.);
#9527=FACE_OUTER_BOUND('',#14792,.T.);
#9528=FACE_OUTER_BOUND('',#14793,.T.);
#9529=FACE_OUTER_BOUND('',#14794,.T.);
#9530=FACE_OUTER_BOUND('',#14795,.T.);
#9531=FACE_OUTER_BOUND('',#14796,.T.);
#9532=FACE_OUTER_BOUND('',#14797,.T.);
#9533=FACE_OUTER_BOUND('',#14798,.T.);
#9534=FACE_OUTER_BOUND('',#14799,.T.);
#9535=FACE_OUTER_BOUND('',#14800,.T.);
#9536=FACE_OUTER_BOUND('',#14801,.T.);
#9537=FACE_OUTER_BOUND('',#14802,.T.);
#9538=FACE_OUTER_BOUND('',#14803,.T.);
#9539=FACE_OUTER_BOUND('',#14804,.T.);
#9540=FACE_OUTER_BOUND('',#14805,.T.);
#9541=FACE_OUTER_BOUND('',#14806,.T.);
#9542=FACE_OUTER_BOUND('',#14807,.T.);
#9543=FACE_OUTER_BOUND('',#14808,.T.);
#9544=FACE_OUTER_BOUND('',#14809,.T.);
#9545=FACE_OUTER_BOUND('',#14810,.T.);
#9546=FACE_OUTER_BOUND('',#14811,.T.);
#9547=FACE_OUTER_BOUND('',#14812,.T.);
#9548=FACE_OUTER_BOUND('',#14813,.T.);
#9549=FACE_OUTER_BOUND('',#14814,.T.);
#9550=FACE_OUTER_BOUND('',#14815,.T.);
#9551=FACE_OUTER_BOUND('',#14816,.T.);
#9552=FACE_OUTER_BOUND('',#14817,.T.);
#9553=FACE_OUTER_BOUND('',#14818,.T.);
#9554=FACE_OUTER_BOUND('',#14819,.T.);
#9555=FACE_OUTER_BOUND('',#14820,.T.);
#9556=FACE_OUTER_BOUND('',#14821,.T.);
#9557=FACE_OUTER_BOUND('',#14822,.T.);
#9558=FACE_OUTER_BOUND('',#14823,.T.);
#9559=FACE_OUTER_BOUND('',#14824,.T.);
#9560=FACE_OUTER_BOUND('',#14825,.T.);
#9561=FACE_OUTER_BOUND('',#14826,.T.);
#9562=FACE_OUTER_BOUND('',#14827,.T.);
#9563=FACE_OUTER_BOUND('',#14828,.T.);
#9564=FACE_OUTER_BOUND('',#14829,.T.);
#9565=FACE_OUTER_BOUND('',#14830,.T.);
#9566=FACE_OUTER_BOUND('',#14831,.T.);
#9567=FACE_OUTER_BOUND('',#14832,.T.);
#9568=FACE_OUTER_BOUND('',#14833,.T.);
#9569=FACE_OUTER_BOUND('',#14834,.T.);
#9570=FACE_OUTER_BOUND('',#14835,.T.);
#9571=FACE_OUTER_BOUND('',#14836,.T.);
#9572=FACE_OUTER_BOUND('',#14837,.T.);
#9573=FACE_OUTER_BOUND('',#14838,.T.);
#9574=FACE_OUTER_BOUND('',#14839,.T.);
#9575=FACE_OUTER_BOUND('',#14840,.T.);
#9576=FACE_OUTER_BOUND('',#14841,.T.);
#9577=FACE_OUTER_BOUND('',#14842,.T.);
#9578=FACE_OUTER_BOUND('',#14843,.T.);
#9579=FACE_OUTER_BOUND('',#14844,.T.);
#9580=FACE_OUTER_BOUND('',#14845,.T.);
#9581=FACE_OUTER_BOUND('',#14846,.T.);
#9582=FACE_OUTER_BOUND('',#14847,.T.);
#9583=FACE_OUTER_BOUND('',#14848,.T.);
#9584=FACE_OUTER_BOUND('',#14849,.T.);
#9585=FACE_OUTER_BOUND('',#14850,.T.);
#9586=FACE_OUTER_BOUND('',#14851,.T.);
#9587=FACE_OUTER_BOUND('',#14852,.T.);
#9588=FACE_OUTER_BOUND('',#14853,.T.);
#9589=FACE_OUTER_BOUND('',#14854,.T.);
#9590=FACE_OUTER_BOUND('',#14855,.T.);
#9591=FACE_OUTER_BOUND('',#14856,.T.);
#9592=FACE_OUTER_BOUND('',#14857,.T.);
#9593=FACE_OUTER_BOUND('',#14858,.T.);
#9594=FACE_OUTER_BOUND('',#14859,.T.);
#9595=FACE_OUTER_BOUND('',#14860,.T.);
#9596=FACE_OUTER_BOUND('',#14861,.T.);
#9597=FACE_OUTER_BOUND('',#14862,.T.);
#9598=FACE_OUTER_BOUND('',#14863,.T.);
#9599=FACE_OUTER_BOUND('',#14864,.T.);
#9600=FACE_OUTER_BOUND('',#14865,.T.);
#9601=FACE_OUTER_BOUND('',#14866,.T.);
#9602=FACE_OUTER_BOUND('',#14867,.T.);
#9603=FACE_OUTER_BOUND('',#14868,.T.);
#9604=FACE_OUTER_BOUND('',#14869,.T.);
#9605=FACE_OUTER_BOUND('',#14870,.T.);
#9606=FACE_OUTER_BOUND('',#14871,.T.);
#9607=FACE_OUTER_BOUND('',#14872,.T.);
#9608=FACE_OUTER_BOUND('',#14873,.T.);
#9609=FACE_OUTER_BOUND('',#14874,.T.);
#9610=FACE_OUTER_BOUND('',#14875,.T.);
#9611=FACE_OUTER_BOUND('',#14876,.T.);
#9612=FACE_OUTER_BOUND('',#14877,.T.);
#9613=FACE_OUTER_BOUND('',#14878,.T.);
#9614=FACE_OUTER_BOUND('',#14879,.T.);
#9615=FACE_OUTER_BOUND('',#14880,.T.);
#9616=FACE_OUTER_BOUND('',#14881,.T.);
#9617=FACE_OUTER_BOUND('',#14882,.T.);
#9618=FACE_OUTER_BOUND('',#14883,.T.);
#9619=FACE_OUTER_BOUND('',#14884,.T.);
#9620=FACE_OUTER_BOUND('',#14885,.T.);
#9621=FACE_OUTER_BOUND('',#14886,.T.);
#9622=FACE_OUTER_BOUND('',#14887,.T.);
#9623=FACE_OUTER_BOUND('',#14888,.T.);
#9624=FACE_OUTER_BOUND('',#14889,.T.);
#9625=FACE_OUTER_BOUND('',#14890,.T.);
#9626=FACE_OUTER_BOUND('',#14891,.T.);
#9627=FACE_OUTER_BOUND('',#14892,.T.);
#9628=FACE_OUTER_BOUND('',#14893,.T.);
#9629=FACE_OUTER_BOUND('',#14894,.T.);
#9630=FACE_OUTER_BOUND('',#14895,.T.);
#9631=FACE_OUTER_BOUND('',#14896,.T.);
#9632=FACE_OUTER_BOUND('',#14897,.T.);
#9633=FACE_OUTER_BOUND('',#14898,.T.);
#9634=FACE_OUTER_BOUND('',#14899,.T.);
#9635=FACE_OUTER_BOUND('',#14900,.T.);
#9636=FACE_OUTER_BOUND('',#14901,.T.);
#9637=FACE_OUTER_BOUND('',#14902,.T.);
#9638=FACE_OUTER_BOUND('',#14903,.T.);
#9639=FACE_OUTER_BOUND('',#14904,.T.);
#9640=FACE_OUTER_BOUND('',#14905,.T.);
#9641=FACE_OUTER_BOUND('',#14906,.T.);
#9642=FACE_OUTER_BOUND('',#14907,.T.);
#9643=FACE_OUTER_BOUND('',#14908,.T.);
#9644=FACE_OUTER_BOUND('',#14909,.T.);
#9645=FACE_OUTER_BOUND('',#14910,.T.);
#9646=FACE_OUTER_BOUND('',#14911,.T.);
#9647=FACE_OUTER_BOUND('',#14912,.T.);
#9648=FACE_OUTER_BOUND('',#14913,.T.);
#9649=FACE_OUTER_BOUND('',#14914,.T.);
#9650=FACE_OUTER_BOUND('',#14915,.T.);
#9651=FACE_OUTER_BOUND('',#14916,.T.);
#9652=FACE_OUTER_BOUND('',#14917,.T.);
#9653=FACE_OUTER_BOUND('',#14918,.T.);
#9654=FACE_OUTER_BOUND('',#14919,.T.);
#9655=FACE_OUTER_BOUND('',#14920,.T.);
#9656=FACE_OUTER_BOUND('',#14921,.T.);
#9657=FACE_OUTER_BOUND('',#14922,.T.);
#9658=FACE_OUTER_BOUND('',#14923,.T.);
#9659=FACE_OUTER_BOUND('',#14924,.T.);
#9660=FACE_OUTER_BOUND('',#14925,.T.);
#9661=FACE_OUTER_BOUND('',#14926,.T.);
#9662=FACE_OUTER_BOUND('',#14927,.T.);
#9663=FACE_OUTER_BOUND('',#14928,.T.);
#9664=FACE_OUTER_BOUND('',#14929,.T.);
#9665=FACE_OUTER_BOUND('',#14930,.T.);
#9666=FACE_OUTER_BOUND('',#14931,.T.);
#9667=FACE_OUTER_BOUND('',#14932,.T.);
#9668=FACE_OUTER_BOUND('',#14933,.T.);
#9669=FACE_OUTER_BOUND('',#14934,.T.);
#9670=FACE_OUTER_BOUND('',#14935,.T.);
#9671=FACE_OUTER_BOUND('',#14936,.T.);
#9672=FACE_OUTER_BOUND('',#14937,.T.);
#9673=FACE_OUTER_BOUND('',#14938,.T.);
#9674=FACE_OUTER_BOUND('',#14939,.T.);
#9675=FACE_OUTER_BOUND('',#14940,.T.);
#9676=FACE_OUTER_BOUND('',#14941,.T.);
#9677=FACE_OUTER_BOUND('',#14942,.T.);
#9678=FACE_OUTER_BOUND('',#14943,.T.);
#9679=FACE_OUTER_BOUND('',#14944,.T.);
#9680=FACE_OUTER_BOUND('',#14945,.T.);
#9681=FACE_OUTER_BOUND('',#14946,.T.);
#9682=FACE_OUTER_BOUND('',#14947,.T.);
#9683=FACE_OUTER_BOUND('',#14948,.T.);
#9684=FACE_OUTER_BOUND('',#14949,.T.);
#9685=FACE_OUTER_BOUND('',#14950,.T.);
#9686=FACE_OUTER_BOUND('',#14951,.T.);
#9687=FACE_OUTER_BOUND('',#14952,.T.);
#9688=FACE_OUTER_BOUND('',#14953,.T.);
#9689=FACE_OUTER_BOUND('',#14954,.T.);
#9690=FACE_OUTER_BOUND('',#14955,.T.);
#9691=FACE_OUTER_BOUND('',#14956,.T.);
#9692=FACE_OUTER_BOUND('',#14957,.T.);
#9693=FACE_OUTER_BOUND('',#14958,.T.);
#9694=FACE_OUTER_BOUND('',#14959,.T.);
#9695=FACE_OUTER_BOUND('',#14960,.T.);
#9696=FACE_OUTER_BOUND('',#14961,.T.);
#9697=FACE_OUTER_BOUND('',#14962,.T.);
#9698=FACE_OUTER_BOUND('',#14963,.T.);
#9699=FACE_OUTER_BOUND('',#14964,.T.);
#9700=FACE_OUTER_BOUND('',#14965,.T.);
#9701=FACE_OUTER_BOUND('',#14966,.T.);
#9702=FACE_OUTER_BOUND('',#14967,.T.);
#9703=FACE_OUTER_BOUND('',#14968,.T.);
#9704=FACE_OUTER_BOUND('',#14969,.T.);
#9705=FACE_OUTER_BOUND('',#14970,.T.);
#9706=FACE_OUTER_BOUND('',#14971,.T.);
#9707=FACE_OUTER_BOUND('',#14972,.T.);
#9708=FACE_OUTER_BOUND('',#14973,.T.);
#9709=FACE_OUTER_BOUND('',#14974,.T.);
#9710=FACE_OUTER_BOUND('',#14975,.T.);
#9711=FACE_OUTER_BOUND('',#14976,.T.);
#9712=FACE_OUTER_BOUND('',#14977,.T.);
#9713=FACE_OUTER_BOUND('',#14978,.T.);
#9714=FACE_OUTER_BOUND('',#14979,.T.);
#9715=FACE_OUTER_BOUND('',#14980,.T.);
#9716=FACE_OUTER_BOUND('',#14981,.T.);
#9717=FACE_OUTER_BOUND('',#14982,.T.);
#9718=FACE_OUTER_BOUND('',#14983,.T.);
#9719=FACE_OUTER_BOUND('',#14984,.T.);
#9720=FACE_OUTER_BOUND('',#14985,.T.);
#9721=FACE_OUTER_BOUND('',#14986,.T.);
#9722=FACE_OUTER_BOUND('',#14987,.T.);
#9723=FACE_OUTER_BOUND('',#14988,.T.);
#9724=FACE_OUTER_BOUND('',#14989,.T.);
#9725=FACE_OUTER_BOUND('',#14990,.T.);
#9726=FACE_OUTER_BOUND('',#14991,.T.);
#9727=FACE_OUTER_BOUND('',#14992,.T.);
#9728=FACE_OUTER_BOUND('',#14993,.T.);
#9729=FACE_OUTER_BOUND('',#14994,.T.);
#9730=FACE_OUTER_BOUND('',#14995,.T.);
#9731=FACE_OUTER_BOUND('',#14996,.T.);
#9732=FACE_OUTER_BOUND('',#14997,.T.);
#9733=FACE_OUTER_BOUND('',#14998,.T.);
#9734=FACE_OUTER_BOUND('',#14999,.T.);
#9735=FACE_OUTER_BOUND('',#15000,.T.);
#9736=FACE_OUTER_BOUND('',#15001,.T.);
#9737=FACE_OUTER_BOUND('',#15002,.T.);
#9738=FACE_OUTER_BOUND('',#15003,.T.);
#9739=FACE_OUTER_BOUND('',#15004,.T.);
#9740=FACE_OUTER_BOUND('',#15005,.T.);
#9741=FACE_OUTER_BOUND('',#15006,.T.);
#9742=FACE_OUTER_BOUND('',#15007,.T.);
#9743=FACE_OUTER_BOUND('',#15008,.T.);
#9744=FACE_OUTER_BOUND('',#15009,.T.);
#9745=FACE_OUTER_BOUND('',#15010,.T.);
#9746=FACE_OUTER_BOUND('',#15011,.T.);
#9747=FACE_OUTER_BOUND('',#15012,.T.);
#9748=FACE_OUTER_BOUND('',#15013,.T.);
#9749=FACE_OUTER_BOUND('',#15014,.T.);
#9750=FACE_OUTER_BOUND('',#15015,.T.);
#9751=FACE_OUTER_BOUND('',#15016,.T.);
#9752=FACE_OUTER_BOUND('',#15017,.T.);
#9753=FACE_OUTER_BOUND('',#15018,.T.);
#9754=FACE_OUTER_BOUND('',#15019,.T.);
#9755=FACE_OUTER_BOUND('',#15020,.T.);
#9756=FACE_OUTER_BOUND('',#15021,.T.);
#9757=FACE_OUTER_BOUND('',#15022,.T.);
#9758=FACE_OUTER_BOUND('',#15023,.T.);
#9759=FACE_OUTER_BOUND('',#15024,.T.);
#9760=FACE_OUTER_BOUND('',#15025,.T.);
#9761=FACE_OUTER_BOUND('',#15026,.T.);
#9762=FACE_OUTER_BOUND('',#15027,.T.);
#9763=FACE_OUTER_BOUND('',#15028,.T.);
#9764=FACE_OUTER_BOUND('',#15029,.T.);
#9765=FACE_OUTER_BOUND('',#15030,.T.);
#9766=FACE_OUTER_BOUND('',#15031,.T.);
#9767=FACE_OUTER_BOUND('',#15032,.T.);
#9768=FACE_OUTER_BOUND('',#15033,.T.);
#9769=FACE_OUTER_BOUND('',#15034,.T.);
#9770=FACE_OUTER_BOUND('',#15035,.T.);
#9771=FACE_OUTER_BOUND('',#15036,.T.);
#9772=FACE_OUTER_BOUND('',#15037,.T.);
#9773=FACE_OUTER_BOUND('',#15038,.T.);
#9774=FACE_OUTER_BOUND('',#15039,.T.);
#9775=FACE_OUTER_BOUND('',#15040,.T.);
#9776=FACE_OUTER_BOUND('',#15041,.T.);
#9777=FACE_OUTER_BOUND('',#15042,.T.);
#9778=FACE_OUTER_BOUND('',#15043,.T.);
#9779=FACE_OUTER_BOUND('',#15044,.T.);
#9780=FACE_OUTER_BOUND('',#15045,.T.);
#9781=FACE_OUTER_BOUND('',#15046,.T.);
#9782=FACE_OUTER_BOUND('',#15047,.T.);
#9783=FACE_OUTER_BOUND('',#15048,.T.);
#9784=FACE_OUTER_BOUND('',#15049,.T.);
#9785=FACE_OUTER_BOUND('',#15050,.T.);
#9786=FACE_OUTER_BOUND('',#15051,.T.);
#9787=FACE_OUTER_BOUND('',#15052,.T.);
#9788=FACE_OUTER_BOUND('',#15053,.T.);
#9789=FACE_OUTER_BOUND('',#15054,.T.);
#9790=FACE_OUTER_BOUND('',#15055,.T.);
#9791=FACE_OUTER_BOUND('',#15056,.T.);
#9792=FACE_OUTER_BOUND('',#15057,.T.);
#9793=FACE_OUTER_BOUND('',#15058,.T.);
#9794=FACE_OUTER_BOUND('',#15059,.T.);
#9795=FACE_OUTER_BOUND('',#15060,.T.);
#9796=FACE_OUTER_BOUND('',#15061,.T.);
#9797=FACE_OUTER_BOUND('',#15062,.T.);
#9798=FACE_OUTER_BOUND('',#15063,.T.);
#9799=FACE_OUTER_BOUND('',#15064,.T.);
#9800=FACE_OUTER_BOUND('',#15065,.T.);
#9801=FACE_OUTER_BOUND('',#15066,.T.);
#9802=FACE_OUTER_BOUND('',#15067,.T.);
#9803=FACE_OUTER_BOUND('',#15068,.T.);
#9804=FACE_OUTER_BOUND('',#15069,.T.);
#9805=FACE_OUTER_BOUND('',#15070,.T.);
#9806=FACE_OUTER_BOUND('',#15071,.T.);
#9807=FACE_OUTER_BOUND('',#15072,.T.);
#9808=FACE_OUTER_BOUND('',#15073,.T.);
#9809=FACE_OUTER_BOUND('',#15074,.T.);
#9810=FACE_OUTER_BOUND('',#15075,.T.);
#9811=FACE_OUTER_BOUND('',#15076,.T.);
#9812=FACE_OUTER_BOUND('',#15077,.T.);
#9813=FACE_OUTER_BOUND('',#15078,.T.);
#9814=FACE_OUTER_BOUND('',#15079,.T.);
#9815=FACE_OUTER_BOUND('',#15080,.T.);
#9816=FACE_OUTER_BOUND('',#15081,.T.);
#9817=FACE_OUTER_BOUND('',#15082,.T.);
#9818=FACE_OUTER_BOUND('',#15083,.T.);
#9819=FACE_OUTER_BOUND('',#15084,.T.);
#9820=FACE_OUTER_BOUND('',#15085,.T.);
#9821=FACE_OUTER_BOUND('',#15086,.T.);
#9822=FACE_OUTER_BOUND('',#15087,.T.);
#9823=FACE_OUTER_BOUND('',#15088,.T.);
#9824=FACE_OUTER_BOUND('',#15089,.T.);
#9825=FACE_OUTER_BOUND('',#15090,.T.);
#9826=FACE_OUTER_BOUND('',#15091,.T.);
#9827=FACE_OUTER_BOUND('',#15092,.T.);
#9828=FACE_OUTER_BOUND('',#15093,.T.);
#9829=FACE_OUTER_BOUND('',#15094,.T.);
#9830=FACE_OUTER_BOUND('',#15095,.T.);
#9831=FACE_OUTER_BOUND('',#15096,.T.);
#9832=FACE_OUTER_BOUND('',#15097,.T.);
#9833=FACE_OUTER_BOUND('',#15098,.T.);
#9834=FACE_OUTER_BOUND('',#15099,.T.);
#9835=FACE_OUTER_BOUND('',#15100,.T.);
#9836=FACE_OUTER_BOUND('',#15101,.T.);
#9837=FACE_OUTER_BOUND('',#15102,.T.);
#9838=FACE_OUTER_BOUND('',#15103,.T.);
#9839=FACE_OUTER_BOUND('',#15104,.T.);
#9840=FACE_OUTER_BOUND('',#15105,.T.);
#9841=FACE_OUTER_BOUND('',#15106,.T.);
#9842=FACE_OUTER_BOUND('',#15107,.T.);
#9843=FACE_OUTER_BOUND('',#15108,.T.);
#9844=FACE_OUTER_BOUND('',#15109,.T.);
#9845=FACE_OUTER_BOUND('',#15110,.T.);
#9846=FACE_OUTER_BOUND('',#15111,.T.);
#9847=FACE_OUTER_BOUND('',#15112,.T.);
#9848=FACE_OUTER_BOUND('',#15113,.T.);
#9849=FACE_OUTER_BOUND('',#15114,.T.);
#9850=FACE_OUTER_BOUND('',#15115,.T.);
#9851=FACE_OUTER_BOUND('',#15116,.T.);
#9852=FACE_OUTER_BOUND('',#15117,.T.);
#9853=FACE_OUTER_BOUND('',#15118,.T.);
#9854=FACE_OUTER_BOUND('',#15119,.T.);
#9855=FACE_OUTER_BOUND('',#15120,.T.);
#9856=FACE_OUTER_BOUND('',#15121,.T.);
#9857=FACE_OUTER_BOUND('',#15122,.T.);
#9858=FACE_OUTER_BOUND('',#15123,.T.);
#9859=FACE_OUTER_BOUND('',#15124,.T.);
#9860=FACE_OUTER_BOUND('',#15125,.T.);
#9861=FACE_OUTER_BOUND('',#15126,.T.);
#9862=FACE_OUTER_BOUND('',#15127,.T.);
#9863=FACE_OUTER_BOUND('',#15128,.T.);
#9864=FACE_OUTER_BOUND('',#15129,.T.);
#9865=FACE_OUTER_BOUND('',#15130,.T.);
#9866=FACE_OUTER_BOUND('',#15131,.T.);
#9867=FACE_OUTER_BOUND('',#15132,.T.);
#9868=FACE_OUTER_BOUND('',#15133,.T.);
#9869=FACE_OUTER_BOUND('',#15134,.T.);
#9870=FACE_OUTER_BOUND('',#15135,.T.);
#9871=FACE_OUTER_BOUND('',#15136,.T.);
#9872=FACE_OUTER_BOUND('',#15137,.T.);
#9873=FACE_OUTER_BOUND('',#15138,.T.);
#9874=FACE_OUTER_BOUND('',#15139,.T.);
#9875=FACE_OUTER_BOUND('',#15140,.T.);
#9876=FACE_OUTER_BOUND('',#15141,.T.);
#9877=FACE_OUTER_BOUND('',#15142,.T.);
#9878=FACE_OUTER_BOUND('',#15143,.T.);
#9879=FACE_OUTER_BOUND('',#15144,.T.);
#9880=FACE_OUTER_BOUND('',#15145,.T.);
#9881=FACE_OUTER_BOUND('',#15146,.T.);
#9882=FACE_OUTER_BOUND('',#15147,.T.);
#9883=FACE_OUTER_BOUND('',#15148,.T.);
#9884=FACE_OUTER_BOUND('',#15149,.T.);
#9885=FACE_OUTER_BOUND('',#15150,.T.);
#9886=FACE_OUTER_BOUND('',#15151,.T.);
#9887=FACE_OUTER_BOUND('',#15152,.T.);
#9888=FACE_OUTER_BOUND('',#15153,.T.);
#9889=FACE_OUTER_BOUND('',#15154,.T.);
#9890=FACE_OUTER_BOUND('',#15155,.T.);
#9891=FACE_OUTER_BOUND('',#15156,.T.);
#9892=FACE_OUTER_BOUND('',#15157,.T.);
#9893=FACE_OUTER_BOUND('',#15158,.T.);
#9894=FACE_OUTER_BOUND('',#15159,.T.);
#9895=FACE_OUTER_BOUND('',#15160,.T.);
#9896=FACE_OUTER_BOUND('',#15161,.T.);
#9897=FACE_OUTER_BOUND('',#15162,.T.);
#9898=FACE_OUTER_BOUND('',#15163,.T.);
#9899=FACE_OUTER_BOUND('',#15164,.T.);
#9900=FACE_OUTER_BOUND('',#15165,.T.);
#9901=FACE_OUTER_BOUND('',#15166,.T.);
#9902=FACE_OUTER_BOUND('',#15167,.T.);
#9903=FACE_OUTER_BOUND('',#15168,.T.);
#9904=FACE_OUTER_BOUND('',#15169,.T.);
#9905=FACE_OUTER_BOUND('',#15170,.T.);
#9906=FACE_OUTER_BOUND('',#15171,.T.);
#9907=FACE_OUTER_BOUND('',#15172,.T.);
#9908=FACE_OUTER_BOUND('',#15173,.T.);
#9909=FACE_OUTER_BOUND('',#15174,.T.);
#9910=FACE_OUTER_BOUND('',#15175,.T.);
#9911=FACE_OUTER_BOUND('',#15176,.T.);
#9912=FACE_OUTER_BOUND('',#15177,.T.);
#9913=FACE_OUTER_BOUND('',#15178,.T.);
#9914=FACE_OUTER_BOUND('',#15179,.T.);
#9915=FACE_OUTER_BOUND('',#15180,.T.);
#9916=FACE_OUTER_BOUND('',#15181,.T.);
#9917=FACE_OUTER_BOUND('',#15182,.T.);
#9918=FACE_OUTER_BOUND('',#15183,.T.);
#9919=FACE_OUTER_BOUND('',#15184,.T.);
#9920=FACE_OUTER_BOUND('',#15185,.T.);
#9921=FACE_OUTER_BOUND('',#15186,.T.);
#9922=FACE_OUTER_BOUND('',#15187,.T.);
#9923=FACE_OUTER_BOUND('',#15188,.T.);
#9924=FACE_OUTER_BOUND('',#15189,.T.);
#9925=FACE_OUTER_BOUND('',#15190,.T.);
#9926=FACE_OUTER_BOUND('',#15191,.T.);
#9927=FACE_OUTER_BOUND('',#15192,.T.);
#9928=FACE_OUTER_BOUND('',#15193,.T.);
#9929=FACE_OUTER_BOUND('',#15194,.T.);
#9930=FACE_OUTER_BOUND('',#15195,.T.);
#9931=FACE_OUTER_BOUND('',#15196,.T.);
#9932=FACE_OUTER_BOUND('',#15197,.T.);
#9933=FACE_OUTER_BOUND('',#15198,.T.);
#9934=FACE_OUTER_BOUND('',#15199,.T.);
#9935=FACE_OUTER_BOUND('',#15200,.T.);
#9936=FACE_OUTER_BOUND('',#15201,.T.);
#9937=FACE_OUTER_BOUND('',#15202,.T.);
#9938=FACE_OUTER_BOUND('',#15203,.T.);
#9939=FACE_OUTER_BOUND('',#15204,.T.);
#9940=FACE_OUTER_BOUND('',#15205,.T.);
#9941=FACE_OUTER_BOUND('',#15206,.T.);
#9942=FACE_OUTER_BOUND('',#15207,.T.);
#9943=FACE_OUTER_BOUND('',#15208,.T.);
#9944=FACE_OUTER_BOUND('',#15209,.T.);
#9945=FACE_OUTER_BOUND('',#15210,.T.);
#9946=FACE_OUTER_BOUND('',#15211,.T.);
#9947=FACE_OUTER_BOUND('',#15212,.T.);
#9948=FACE_OUTER_BOUND('',#15213,.T.);
#9949=FACE_OUTER_BOUND('',#15214,.T.);
#9950=FACE_OUTER_BOUND('',#15215,.T.);
#9951=FACE_OUTER_BOUND('',#15216,.T.);
#9952=FACE_OUTER_BOUND('',#15217,.T.);
#9953=FACE_OUTER_BOUND('',#15218,.T.);
#9954=FACE_OUTER_BOUND('',#15219,.T.);
#9955=FACE_OUTER_BOUND('',#15220,.T.);
#9956=FACE_OUTER_BOUND('',#15221,.T.);
#9957=FACE_OUTER_BOUND('',#15222,.T.);
#9958=FACE_OUTER_BOUND('',#15223,.T.);
#9959=FACE_OUTER_BOUND('',#15224,.T.);
#9960=FACE_OUTER_BOUND('',#15225,.T.);
#9961=FACE_OUTER_BOUND('',#15226,.T.);
#9962=FACE_OUTER_BOUND('',#15227,.T.);
#9963=FACE_OUTER_BOUND('',#15228,.T.);
#9964=FACE_OUTER_BOUND('',#15229,.T.);
#9965=FACE_OUTER_BOUND('',#15230,.T.);
#9966=FACE_OUTER_BOUND('',#15231,.T.);
#9967=FACE_OUTER_BOUND('',#15232,.T.);
#9968=FACE_OUTER_BOUND('',#15233,.T.);
#9969=FACE_OUTER_BOUND('',#15234,.T.);
#9970=FACE_OUTER_BOUND('',#15235,.T.);
#9971=FACE_OUTER_BOUND('',#15236,.T.);
#9972=FACE_OUTER_BOUND('',#15237,.T.);
#9973=FACE_OUTER_BOUND('',#15238,.T.);
#9974=FACE_OUTER_BOUND('',#15239,.T.);
#9975=FACE_OUTER_BOUND('',#15240,.T.);
#9976=FACE_OUTER_BOUND('',#15241,.T.);
#9977=FACE_OUTER_BOUND('',#15242,.T.);
#9978=FACE_OUTER_BOUND('',#15243,.T.);
#9979=FACE_OUTER_BOUND('',#15244,.T.);
#9980=FACE_OUTER_BOUND('',#15245,.T.);
#9981=FACE_OUTER_BOUND('',#15246,.T.);
#9982=FACE_OUTER_BOUND('',#15247,.T.);
#9983=FACE_OUTER_BOUND('',#15248,.T.);
#9984=FACE_OUTER_BOUND('',#15249,.T.);
#9985=FACE_OUTER_BOUND('',#15250,.T.);
#9986=FACE_OUTER_BOUND('',#15251,.T.);
#9987=FACE_OUTER_BOUND('',#15252,.T.);
#9988=FACE_OUTER_BOUND('',#15253,.T.);
#9989=FACE_OUTER_BOUND('',#15254,.T.);
#9990=FACE_OUTER_BOUND('',#15255,.T.);
#9991=FACE_OUTER_BOUND('',#15256,.T.);
#9992=FACE_OUTER_BOUND('',#15257,.T.);
#9993=FACE_OUTER_BOUND('',#15258,.T.);
#9994=FACE_OUTER_BOUND('',#15259,.T.);
#9995=FACE_OUTER_BOUND('',#15260,.T.);
#9996=FACE_OUTER_BOUND('',#15261,.T.);
#9997=FACE_OUTER_BOUND('',#15262,.T.);
#9998=FACE_OUTER_BOUND('',#15263,.T.);
#9999=FACE_OUTER_BOUND('',#15264,.T.);
#10000=FACE_OUTER_BOUND('',#15265,.T.);
#10001=FACE_OUTER_BOUND('',#15266,.T.);
#10002=FACE_OUTER_BOUND('',#15267,.T.);
#10003=FACE_OUTER_BOUND('',#15268,.T.);
#10004=FACE_OUTER_BOUND('',#15269,.T.);
#10005=FACE_OUTER_BOUND('',#15270,.T.);
#10006=FACE_OUTER_BOUND('',#15271,.T.);
#10007=FACE_OUTER_BOUND('',#15272,.T.);
#10008=FACE_OUTER_BOUND('',#15273,.T.);
#10009=FACE_OUTER_BOUND('',#15274,.T.);
#10010=FACE_OUTER_BOUND('',#15275,.T.);
#10011=FACE_OUTER_BOUND('',#15276,.T.);
#10012=FACE_OUTER_BOUND('',#15277,.T.);
#10013=FACE_OUTER_BOUND('',#15278,.T.);
#10014=FACE_OUTER_BOUND('',#15279,.T.);
#10015=FACE_OUTER_BOUND('',#15280,.T.);
#10016=FACE_OUTER_BOUND('',#15281,.T.);
#10017=FACE_OUTER_BOUND('',#15282,.T.);
#10018=FACE_OUTER_BOUND('',#15283,.T.);
#10019=FACE_OUTER_BOUND('',#15284,.T.);
#10020=FACE_OUTER_BOUND('',#15285,.T.);
#10021=FACE_OUTER_BOUND('',#15286,.T.);
#10022=FACE_OUTER_BOUND('',#15287,.T.);
#10023=FACE_OUTER_BOUND('',#15288,.T.);
#10024=FACE_OUTER_BOUND('',#15289,.T.);
#10025=FACE_OUTER_BOUND('',#15290,.T.);
#10026=FACE_OUTER_BOUND('',#15291,.T.);
#10027=FACE_OUTER_BOUND('',#15292,.T.);
#10028=FACE_OUTER_BOUND('',#15293,.T.);
#10029=FACE_OUTER_BOUND('',#15294,.T.);
#10030=FACE_OUTER_BOUND('',#15295,.T.);
#10031=FACE_OUTER_BOUND('',#15296,.T.);
#10032=FACE_OUTER_BOUND('',#15297,.T.);
#10033=FACE_OUTER_BOUND('',#15298,.T.);
#10034=FACE_OUTER_BOUND('',#15299,.T.);
#10035=FACE_OUTER_BOUND('',#15300,.T.);
#10036=FACE_OUTER_BOUND('',#15301,.T.);
#10037=FACE_OUTER_BOUND('',#15302,.T.);
#10038=FACE_OUTER_BOUND('',#15303,.T.);
#10039=FACE_OUTER_BOUND('',#15304,.T.);
#10040=FACE_OUTER_BOUND('',#15305,.T.);
#10041=FACE_OUTER_BOUND('',#15306,.T.);
#10042=FACE_OUTER_BOUND('',#15307,.T.);
#10043=FACE_OUTER_BOUND('',#15308,.T.);
#10044=FACE_OUTER_BOUND('',#15309,.T.);
#10045=FACE_OUTER_BOUND('',#15310,.T.);
#10046=FACE_OUTER_BOUND('',#15311,.T.);
#10047=FACE_OUTER_BOUND('',#15312,.T.);
#10048=FACE_OUTER_BOUND('',#15313,.T.);
#10049=FACE_OUTER_BOUND('',#15314,.T.);
#10050=FACE_OUTER_BOUND('',#15315,.T.);
#10051=FACE_OUTER_BOUND('',#15316,.T.);
#10052=FACE_OUTER_BOUND('',#15317,.T.);
#10053=FACE_OUTER_BOUND('',#15318,.T.);
#10054=FACE_OUTER_BOUND('',#15319,.T.);
#10055=FACE_OUTER_BOUND('',#15320,.T.);
#10056=FACE_OUTER_BOUND('',#15321,.T.);
#10057=FACE_OUTER_BOUND('',#15322,.T.);
#10058=FACE_OUTER_BOUND('',#15323,.T.);
#10059=FACE_OUTER_BOUND('',#15324,.T.);
#10060=FACE_OUTER_BOUND('',#15325,.T.);
#10061=FACE_OUTER_BOUND('',#15326,.T.);
#10062=FACE_OUTER_BOUND('',#15327,.T.);
#10063=FACE_OUTER_BOUND('',#15328,.T.);
#10064=FACE_OUTER_BOUND('',#15329,.T.);
#10065=FACE_OUTER_BOUND('',#15330,.T.);
#10066=FACE_OUTER_BOUND('',#15331,.T.);
#10067=FACE_OUTER_BOUND('',#15332,.T.);
#10068=FACE_OUTER_BOUND('',#15333,.T.);
#10069=FACE_OUTER_BOUND('',#15334,.T.);
#10070=FACE_OUTER_BOUND('',#15335,.T.);
#10071=FACE_OUTER_BOUND('',#15336,.T.);
#10072=FACE_OUTER_BOUND('',#15337,.T.);
#10073=FACE_OUTER_BOUND('',#15338,.T.);
#10074=FACE_OUTER_BOUND('',#15339,.T.);
#10075=FACE_OUTER_BOUND('',#15340,.T.);
#10076=FACE_OUTER_BOUND('',#15341,.T.);
#10077=FACE_OUTER_BOUND('',#15342,.T.);
#10078=FACE_OUTER_BOUND('',#15343,.T.);
#10079=FACE_OUTER_BOUND('',#15344,.T.);
#10080=FACE_OUTER_BOUND('',#15345,.T.);
#10081=FACE_OUTER_BOUND('',#15346,.T.);
#10082=FACE_OUTER_BOUND('',#15347,.T.);
#10083=FACE_OUTER_BOUND('',#15348,.T.);
#10084=FACE_OUTER_BOUND('',#15349,.T.);
#10085=FACE_OUTER_BOUND('',#15350,.T.);
#10086=FACE_OUTER_BOUND('',#15351,.T.);
#10087=FACE_OUTER_BOUND('',#15352,.T.);
#10088=FACE_OUTER_BOUND('',#15353,.T.);
#10089=FACE_OUTER_BOUND('',#15354,.T.);
#10090=FACE_OUTER_BOUND('',#15355,.T.);
#10091=FACE_OUTER_BOUND('',#15356,.T.);
#10092=FACE_OUTER_BOUND('',#15357,.T.);
#10093=FACE_OUTER_BOUND('',#15358,.T.);
#10094=FACE_OUTER_BOUND('',#15359,.T.);
#10095=FACE_OUTER_BOUND('',#15360,.T.);
#10096=FACE_OUTER_BOUND('',#15361,.T.);
#10097=FACE_OUTER_BOUND('',#15362,.T.);
#10098=FACE_OUTER_BOUND('',#15363,.T.);
#10099=FACE_OUTER_BOUND('',#15364,.T.);
#10100=FACE_OUTER_BOUND('',#15365,.T.);
#10101=FACE_OUTER_BOUND('',#15366,.T.);
#10102=FACE_OUTER_BOUND('',#15367,.T.);
#10103=FACE_OUTER_BOUND('',#15368,.T.);
#10104=FACE_OUTER_BOUND('',#15369,.T.);
#10105=FACE_OUTER_BOUND('',#15370,.T.);
#10106=FACE_OUTER_BOUND('',#15371,.T.);
#10107=FACE_OUTER_BOUND('',#15372,.T.);
#10108=FACE_OUTER_BOUND('',#15373,.T.);
#10109=FACE_OUTER_BOUND('',#15374,.T.);
#10110=FACE_OUTER_BOUND('',#15375,.T.);
#10111=FACE_OUTER_BOUND('',#15376,.T.);
#10112=FACE_OUTER_BOUND('',#15377,.T.);
#10113=FACE_OUTER_BOUND('',#15378,.T.);
#10114=FACE_OUTER_BOUND('',#15379,.T.);
#10115=FACE_OUTER_BOUND('',#15380,.T.);
#10116=FACE_OUTER_BOUND('',#15381,.T.);
#10117=FACE_OUTER_BOUND('',#15382,.T.);
#10118=FACE_OUTER_BOUND('',#15383,.T.);
#10119=FACE_OUTER_BOUND('',#15384,.T.);
#10120=FACE_OUTER_BOUND('',#15385,.T.);
#10121=FACE_OUTER_BOUND('',#15386,.T.);
#10122=FACE_OUTER_BOUND('',#15387,.T.);
#10123=FACE_OUTER_BOUND('',#15388,.T.);
#10124=FACE_OUTER_BOUND('',#15389,.T.);
#10125=FACE_OUTER_BOUND('',#15390,.T.);
#10126=FACE_OUTER_BOUND('',#15391,.T.);
#10127=FACE_OUTER_BOUND('',#15392,.T.);
#10128=FACE_OUTER_BOUND('',#15393,.T.);
#10129=FACE_OUTER_BOUND('',#15394,.T.);
#10130=FACE_OUTER_BOUND('',#15395,.T.);
#10131=FACE_OUTER_BOUND('',#15396,.T.);
#10132=FACE_OUTER_BOUND('',#15397,.T.);
#10133=FACE_OUTER_BOUND('',#15398,.T.);
#10134=FACE_OUTER_BOUND('',#15399,.T.);
#10135=FACE_OUTER_BOUND('',#15400,.T.);
#10136=FACE_OUTER_BOUND('',#15401,.T.);
#10137=FACE_OUTER_BOUND('',#15402,.T.);
#10138=FACE_OUTER_BOUND('',#15403,.T.);
#10139=FACE_OUTER_BOUND('',#15404,.T.);
#10140=FACE_OUTER_BOUND('',#15405,.T.);
#10141=FACE_OUTER_BOUND('',#15406,.T.);
#10142=FACE_OUTER_BOUND('',#15407,.T.);
#10143=FACE_OUTER_BOUND('',#15408,.T.);
#10144=FACE_OUTER_BOUND('',#15409,.T.);
#10145=FACE_OUTER_BOUND('',#15410,.T.);
#10146=FACE_OUTER_BOUND('',#15411,.T.);
#10147=FACE_OUTER_BOUND('',#15412,.T.);
#10148=FACE_OUTER_BOUND('',#15413,.T.);
#10149=FACE_OUTER_BOUND('',#15414,.T.);
#10150=FACE_OUTER_BOUND('',#15415,.T.);
#10151=FACE_OUTER_BOUND('',#15416,.T.);
#10152=FACE_OUTER_BOUND('',#15417,.T.);
#10153=FACE_OUTER_BOUND('',#15418,.T.);
#10154=FACE_OUTER_BOUND('',#15419,.T.);
#10155=FACE_OUTER_BOUND('',#15420,.T.);
#10156=FACE_OUTER_BOUND('',#15421,.T.);
#10157=FACE_OUTER_BOUND('',#15422,.T.);
#10158=FACE_OUTER_BOUND('',#15423,.T.);
#10159=FACE_OUTER_BOUND('',#15424,.T.);
#10160=FACE_OUTER_BOUND('',#15425,.T.);
#10161=FACE_OUTER_BOUND('',#15426,.T.);
#10162=FACE_OUTER_BOUND('',#15427,.T.);
#10163=FACE_OUTER_BOUND('',#15428,.T.);
#10164=FACE_OUTER_BOUND('',#15429,.T.);
#10165=FACE_OUTER_BOUND('',#15430,.T.);
#10166=FACE_OUTER_BOUND('',#15431,.T.);
#10167=FACE_OUTER_BOUND('',#15432,.T.);
#10168=FACE_OUTER_BOUND('',#15433,.T.);
#10169=FACE_OUTER_BOUND('',#15434,.T.);
#10170=FACE_OUTER_BOUND('',#15435,.T.);
#10171=FACE_OUTER_BOUND('',#15436,.T.);
#10172=FACE_OUTER_BOUND('',#15437,.T.);
#10173=FACE_OUTER_BOUND('',#15438,.T.);
#10174=FACE_OUTER_BOUND('',#15439,.T.);
#10175=FACE_OUTER_BOUND('',#15440,.T.);
#10176=FACE_OUTER_BOUND('',#15441,.T.);
#10177=FACE_OUTER_BOUND('',#15442,.T.);
#10178=FACE_OUTER_BOUND('',#15443,.T.);
#10179=FACE_OUTER_BOUND('',#15444,.T.);
#10180=FACE_OUTER_BOUND('',#15445,.T.);
#10181=FACE_OUTER_BOUND('',#15446,.T.);
#10182=FACE_OUTER_BOUND('',#15447,.T.);
#10183=FACE_OUTER_BOUND('',#15448,.T.);
#10184=FACE_OUTER_BOUND('',#15449,.T.);
#10185=FACE_OUTER_BOUND('',#15450,.T.);
#10186=FACE_OUTER_BOUND('',#15451,.T.);
#10187=FACE_OUTER_BOUND('',#15452,.T.);
#10188=FACE_OUTER_BOUND('',#15453,.T.);
#10189=FACE_OUTER_BOUND('',#15454,.T.);
#10190=FACE_OUTER_BOUND('',#15455,.T.);
#10191=FACE_OUTER_BOUND('',#15456,.T.);
#10192=FACE_OUTER_BOUND('',#15457,.T.);
#10193=FACE_OUTER_BOUND('',#15458,.T.);
#10194=FACE_OUTER_BOUND('',#15459,.T.);
#10195=FACE_OUTER_BOUND('',#15460,.T.);
#10196=FACE_OUTER_BOUND('',#15461,.T.);
#10197=FACE_OUTER_BOUND('',#15462,.T.);
#10198=FACE_OUTER_BOUND('',#15463,.T.);
#10199=FACE_OUTER_BOUND('',#15464,.T.);
#10200=FACE_OUTER_BOUND('',#15465,.T.);
#10201=FACE_OUTER_BOUND('',#15466,.T.);
#10202=FACE_OUTER_BOUND('',#15467,.T.);
#10203=FACE_OUTER_BOUND('',#15468,.T.);
#10204=FACE_OUTER_BOUND('',#15469,.T.);
#10205=FACE_OUTER_BOUND('',#15470,.T.);
#10206=FACE_OUTER_BOUND('',#15471,.T.);
#10207=FACE_OUTER_BOUND('',#15473,.T.);
#10208=FACE_OUTER_BOUND('',#15474,.T.);
#10209=FACE_OUTER_BOUND('',#15475,.T.);
#10210=FACE_OUTER_BOUND('',#15476,.T.);
#10211=FACE_OUTER_BOUND('',#15477,.T.);
#10212=FACE_OUTER_BOUND('',#15478,.T.);
#10213=FACE_OUTER_BOUND('',#15479,.T.);
#10214=FACE_OUTER_BOUND('',#15480,.T.);
#10215=FACE_OUTER_BOUND('',#15481,.T.);
#10216=FACE_OUTER_BOUND('',#15482,.T.);
#10217=FACE_OUTER_BOUND('',#15483,.T.);
#10218=FACE_OUTER_BOUND('',#15484,.T.);
#10219=FACE_OUTER_BOUND('',#15485,.T.);
#10220=FACE_OUTER_BOUND('',#15486,.T.);
#10221=FACE_OUTER_BOUND('',#15487,.T.);
#10222=FACE_OUTER_BOUND('',#15488,.T.);
#10223=FACE_OUTER_BOUND('',#15489,.T.);
#10224=FACE_OUTER_BOUND('',#15490,.T.);
#10225=FACE_OUTER_BOUND('',#15491,.T.);
#10226=FACE_OUTER_BOUND('',#15492,.T.);
#10227=FACE_OUTER_BOUND('',#15493,.T.);
#10228=FACE_OUTER_BOUND('',#15494,.T.);
#10229=FACE_OUTER_BOUND('',#15495,.T.);
#10230=FACE_OUTER_BOUND('',#15496,.T.);
#10231=FACE_OUTER_BOUND('',#15497,.T.);
#10232=FACE_OUTER_BOUND('',#15498,.T.);
#10233=FACE_OUTER_BOUND('',#15499,.T.);
#10234=FACE_OUTER_BOUND('',#15500,.T.);
#10235=FACE_OUTER_BOUND('',#15501,.T.);
#10236=FACE_OUTER_BOUND('',#15502,.T.);
#10237=FACE_OUTER_BOUND('',#15503,.T.);
#10238=FACE_OUTER_BOUND('',#15504,.T.);
#10239=FACE_OUTER_BOUND('',#15505,.T.);
#10240=FACE_OUTER_BOUND('',#15506,.T.);
#10241=FACE_OUTER_BOUND('',#15507,.T.);
#10242=FACE_OUTER_BOUND('',#15508,.T.);
#10243=FACE_OUTER_BOUND('',#15509,.T.);
#10244=FACE_OUTER_BOUND('',#15510,.T.);
#10245=FACE_OUTER_BOUND('',#15511,.T.);
#10246=FACE_OUTER_BOUND('',#15512,.T.);
#10247=FACE_OUTER_BOUND('',#15513,.T.);
#10248=FACE_OUTER_BOUND('',#15514,.T.);
#10249=FACE_OUTER_BOUND('',#15515,.T.);
#10250=FACE_OUTER_BOUND('',#15516,.T.);
#10251=FACE_OUTER_BOUND('',#15517,.T.);
#10252=FACE_OUTER_BOUND('',#15518,.T.);
#10253=FACE_OUTER_BOUND('',#15519,.T.);
#10254=FACE_OUTER_BOUND('',#15520,.T.);
#10255=FACE_OUTER_BOUND('',#15521,.T.);
#10256=FACE_OUTER_BOUND('',#15522,.T.);
#10257=FACE_OUTER_BOUND('',#15523,.T.);
#10258=FACE_OUTER_BOUND('',#15524,.T.);
#10259=FACE_OUTER_BOUND('',#15525,.T.);
#10260=FACE_OUTER_BOUND('',#15526,.T.);
#10261=FACE_OUTER_BOUND('',#15527,.T.);
#10262=FACE_OUTER_BOUND('',#15528,.T.);
#10263=FACE_OUTER_BOUND('',#15529,.T.);
#10264=FACE_OUTER_BOUND('',#15530,.T.);
#10265=FACE_OUTER_BOUND('',#15531,.T.);
#10266=FACE_OUTER_BOUND('',#15532,.T.);
#10267=FACE_OUTER_BOUND('',#15533,.T.);
#10268=FACE_OUTER_BOUND('',#15534,.T.);
#10269=FACE_OUTER_BOUND('',#15535,.T.);
#10270=FACE_OUTER_BOUND('',#15536,.T.);
#10271=FACE_OUTER_BOUND('',#15537,.T.);
#10272=FACE_OUTER_BOUND('',#15538,.T.);
#10273=FACE_OUTER_BOUND('',#15539,.T.);
#10274=FACE_OUTER_BOUND('',#15540,.T.);
#10275=FACE_OUTER_BOUND('',#15541,.T.);
#10276=FACE_OUTER_BOUND('',#15542,.T.);
#10277=FACE_OUTER_BOUND('',#15543,.T.);
#10278=FACE_OUTER_BOUND('',#15544,.T.);
#10279=FACE_OUTER_BOUND('',#15545,.T.);
#10280=FACE_OUTER_BOUND('',#15546,.T.);
#10281=FACE_OUTER_BOUND('',#15547,.T.);
#10282=FACE_OUTER_BOUND('',#15548,.T.);
#10283=FACE_OUTER_BOUND('',#15549,.T.);
#10284=FACE_OUTER_BOUND('',#15550,.T.);
#10285=FACE_OUTER_BOUND('',#15551,.T.);
#10286=FACE_OUTER_BOUND('',#15552,.T.);
#10287=FACE_OUTER_BOUND('',#15553,.T.);
#10288=FACE_OUTER_BOUND('',#15554,.T.);
#10289=FACE_OUTER_BOUND('',#15555,.T.);
#10290=FACE_OUTER_BOUND('',#15556,.T.);
#10291=FACE_OUTER_BOUND('',#15557,.T.);
#10292=FACE_OUTER_BOUND('',#15558,.T.);
#10293=FACE_OUTER_BOUND('',#15559,.T.);
#10294=FACE_OUTER_BOUND('',#15560,.T.);
#10295=FACE_OUTER_BOUND('',#15561,.T.);
#10296=FACE_OUTER_BOUND('',#15562,.T.);
#10297=FACE_OUTER_BOUND('',#15563,.T.);
#10298=FACE_OUTER_BOUND('',#15564,.T.);
#10299=FACE_OUTER_BOUND('',#15565,.T.);
#10300=FACE_OUTER_BOUND('',#15566,.T.);
#10301=FACE_OUTER_BOUND('',#15567,.T.);
#10302=FACE_OUTER_BOUND('',#15568,.T.);
#10303=FACE_OUTER_BOUND('',#15569,.T.);
#10304=FACE_OUTER_BOUND('',#15570,.T.);
#10305=FACE_OUTER_BOUND('',#15571,.T.);
#10306=FACE_OUTER_BOUND('',#15572,.T.);
#10307=FACE_OUTER_BOUND('',#15573,.T.);
#10308=FACE_OUTER_BOUND('',#15574,.T.);
#10309=FACE_OUTER_BOUND('',#15575,.T.);
#10310=FACE_OUTER_BOUND('',#15576,.T.);
#10311=FACE_OUTER_BOUND('',#15577,.T.);
#10312=FACE_OUTER_BOUND('',#15578,.T.);
#10313=FACE_OUTER_BOUND('',#15579,.T.);
#10314=FACE_OUTER_BOUND('',#15580,.T.);
#10315=FACE_OUTER_BOUND('',#15581,.T.);
#10316=FACE_OUTER_BOUND('',#15582,.T.);
#10317=FACE_OUTER_BOUND('',#15583,.T.);
#10318=FACE_OUTER_BOUND('',#15584,.T.);
#10319=FACE_OUTER_BOUND('',#15585,.T.);
#10320=FACE_OUTER_BOUND('',#15586,.T.);
#10321=FACE_OUTER_BOUND('',#15587,.T.);
#10322=FACE_OUTER_BOUND('',#15588,.T.);
#10323=FACE_OUTER_BOUND('',#15589,.T.);
#10324=FACE_OUTER_BOUND('',#15590,.T.);
#10325=FACE_OUTER_BOUND('',#15591,.T.);
#10326=FACE_OUTER_BOUND('',#15592,.T.);
#10327=FACE_OUTER_BOUND('',#15593,.T.);
#10328=FACE_OUTER_BOUND('',#15594,.T.);
#10329=FACE_OUTER_BOUND('',#15595,.T.);
#10330=FACE_OUTER_BOUND('',#15596,.T.);
#10331=FACE_OUTER_BOUND('',#15597,.T.);
#10332=FACE_OUTER_BOUND('',#15598,.T.);
#10333=FACE_OUTER_BOUND('',#15599,.T.);
#10334=FACE_OUTER_BOUND('',#15600,.T.);
#10335=FACE_OUTER_BOUND('',#15601,.T.);
#10336=FACE_OUTER_BOUND('',#15602,.T.);
#10337=FACE_OUTER_BOUND('',#15603,.T.);
#10338=FACE_OUTER_BOUND('',#15604,.T.);
#10339=FACE_OUTER_BOUND('',#15605,.T.);
#10340=FACE_OUTER_BOUND('',#15606,.T.);
#10341=FACE_OUTER_BOUND('',#15607,.T.);
#10342=FACE_OUTER_BOUND('',#15608,.T.);
#10343=FACE_OUTER_BOUND('',#15609,.T.);
#10344=FACE_OUTER_BOUND('',#15610,.T.);
#10345=FACE_OUTER_BOUND('',#15611,.T.);
#10346=FACE_OUTER_BOUND('',#15612,.T.);
#10347=FACE_OUTER_BOUND('',#15613,.T.);
#10348=FACE_OUTER_BOUND('',#15614,.T.);
#10349=FACE_OUTER_BOUND('',#15615,.T.);
#10350=FACE_OUTER_BOUND('',#15616,.T.);
#10351=FACE_OUTER_BOUND('',#15617,.T.);
#10352=FACE_OUTER_BOUND('',#15618,.T.);
#10353=FACE_OUTER_BOUND('',#15619,.T.);
#10354=FACE_OUTER_BOUND('',#15620,.T.);
#10355=FACE_OUTER_BOUND('',#15621,.T.);
#10356=FACE_OUTER_BOUND('',#15622,.T.);
#10357=FACE_OUTER_BOUND('',#15623,.T.);
#10358=FACE_OUTER_BOUND('',#15624,.T.);
#10359=FACE_OUTER_BOUND('',#15625,.T.);
#10360=FACE_OUTER_BOUND('',#15626,.T.);
#10361=FACE_OUTER_BOUND('',#15627,.T.);
#10362=FACE_OUTER_BOUND('',#15628,.T.);
#10363=FACE_OUTER_BOUND('',#15629,.T.);
#10364=FACE_OUTER_BOUND('',#15630,.T.);
#10365=FACE_OUTER_BOUND('',#15631,.T.);
#10366=FACE_OUTER_BOUND('',#15632,.T.);
#10367=FACE_OUTER_BOUND('',#15633,.T.);
#10368=FACE_OUTER_BOUND('',#15634,.T.);
#10369=FACE_OUTER_BOUND('',#15635,.T.);
#10370=FACE_OUTER_BOUND('',#15636,.T.);
#10371=FACE_OUTER_BOUND('',#15637,.T.);
#10372=FACE_OUTER_BOUND('',#15638,.T.);
#10373=FACE_OUTER_BOUND('',#15639,.T.);
#10374=FACE_OUTER_BOUND('',#15640,.T.);
#10375=FACE_OUTER_BOUND('',#15641,.T.);
#10376=FACE_OUTER_BOUND('',#15642,.T.);
#10377=FACE_OUTER_BOUND('',#15643,.T.);
#10378=FACE_OUTER_BOUND('',#15644,.T.);
#10379=FACE_OUTER_BOUND('',#15645,.T.);
#10380=FACE_OUTER_BOUND('',#15646,.T.);
#10381=FACE_OUTER_BOUND('',#15647,.T.);
#10382=FACE_OUTER_BOUND('',#15648,.T.);
#10383=FACE_OUTER_BOUND('',#15649,.T.);
#10384=FACE_OUTER_BOUND('',#15650,.T.);
#10385=FACE_OUTER_BOUND('',#15651,.T.);
#10386=FACE_OUTER_BOUND('',#15652,.T.);
#10387=FACE_OUTER_BOUND('',#15653,.T.);
#10388=FACE_OUTER_BOUND('',#15654,.T.);
#10389=FACE_OUTER_BOUND('',#15655,.T.);
#10390=FACE_OUTER_BOUND('',#15656,.T.);
#10391=FACE_OUTER_BOUND('',#15657,.T.);
#10392=FACE_OUTER_BOUND('',#15658,.T.);
#10393=FACE_OUTER_BOUND('',#15659,.T.);
#10394=FACE_OUTER_BOUND('',#15660,.T.);
#10395=FACE_OUTER_BOUND('',#15661,.T.);
#10396=FACE_OUTER_BOUND('',#15662,.T.);
#10397=FACE_OUTER_BOUND('',#15663,.T.);
#10398=FACE_OUTER_BOUND('',#15664,.T.);
#10399=FACE_OUTER_BOUND('',#15665,.T.);
#10400=FACE_OUTER_BOUND('',#15666,.T.);
#10401=FACE_OUTER_BOUND('',#15667,.T.);
#10402=FACE_OUTER_BOUND('',#15668,.T.);
#10403=FACE_OUTER_BOUND('',#15669,.T.);
#10404=FACE_OUTER_BOUND('',#15670,.T.);
#10405=FACE_OUTER_BOUND('',#15671,.T.);
#10406=FACE_OUTER_BOUND('',#15672,.T.);
#10407=FACE_OUTER_BOUND('',#15673,.T.);
#10408=FACE_OUTER_BOUND('',#15674,.T.);
#10409=FACE_OUTER_BOUND('',#15676,.T.);
#10410=FACE_OUTER_BOUND('',#15677,.T.);
#10411=FACE_OUTER_BOUND('',#15678,.T.);
#10412=FACE_OUTER_BOUND('',#15679,.T.);
#10413=FACE_OUTER_BOUND('',#15680,.T.);
#10414=FACE_OUTER_BOUND('',#15681,.T.);
#10415=FACE_OUTER_BOUND('',#15682,.T.);
#10416=FACE_OUTER_BOUND('',#15683,.T.);
#10417=FACE_OUTER_BOUND('',#15684,.T.);
#10418=FACE_OUTER_BOUND('',#15685,.T.);
#10419=FACE_OUTER_BOUND('',#15686,.T.);
#10420=FACE_OUTER_BOUND('',#15687,.T.);
#10421=FACE_OUTER_BOUND('',#15688,.T.);
#10422=FACE_OUTER_BOUND('',#15689,.T.);
#10423=FACE_OUTER_BOUND('',#15690,.T.);
#10424=FACE_OUTER_BOUND('',#15691,.T.);
#10425=FACE_OUTER_BOUND('',#15692,.T.);
#10426=FACE_OUTER_BOUND('',#15693,.T.);
#10427=FACE_OUTER_BOUND('',#15694,.T.);
#10428=FACE_OUTER_BOUND('',#15695,.T.);
#10429=FACE_OUTER_BOUND('',#15696,.T.);
#10430=FACE_OUTER_BOUND('',#15697,.T.);
#10431=FACE_OUTER_BOUND('',#15698,.T.);
#10432=FACE_OUTER_BOUND('',#15699,.T.);
#10433=FACE_OUTER_BOUND('',#15700,.T.);
#10434=FACE_OUTER_BOUND('',#15701,.T.);
#10435=FACE_OUTER_BOUND('',#15702,.T.);
#10436=FACE_OUTER_BOUND('',#15703,.T.);
#10437=FACE_OUTER_BOUND('',#15704,.T.);
#10438=FACE_OUTER_BOUND('',#15705,.T.);
#10439=FACE_OUTER_BOUND('',#15706,.T.);
#10440=FACE_OUTER_BOUND('',#15707,.T.);
#10441=FACE_OUTER_BOUND('',#15708,.T.);
#10442=FACE_OUTER_BOUND('',#15709,.T.);
#10443=FACE_OUTER_BOUND('',#15710,.T.);
#10444=FACE_OUTER_BOUND('',#15711,.T.);
#10445=FACE_OUTER_BOUND('',#15712,.T.);
#10446=FACE_OUTER_BOUND('',#15713,.T.);
#10447=FACE_OUTER_BOUND('',#15714,.T.);
#10448=FACE_OUTER_BOUND('',#15715,.T.);
#10449=FACE_OUTER_BOUND('',#15716,.T.);
#10450=FACE_OUTER_BOUND('',#15717,.T.);
#10451=FACE_OUTER_BOUND('',#15718,.T.);
#10452=FACE_OUTER_BOUND('',#15719,.T.);
#10453=FACE_OUTER_BOUND('',#15720,.T.);
#10454=FACE_OUTER_BOUND('',#15721,.T.);
#10455=FACE_OUTER_BOUND('',#15722,.T.);
#10456=FACE_OUTER_BOUND('',#15723,.T.);
#10457=FACE_OUTER_BOUND('',#15724,.T.);
#10458=FACE_OUTER_BOUND('',#15725,.T.);
#10459=FACE_OUTER_BOUND('',#15726,.T.);
#10460=FACE_OUTER_BOUND('',#15727,.T.);
#10461=FACE_OUTER_BOUND('',#15728,.T.);
#10462=FACE_OUTER_BOUND('',#15729,.T.);
#10463=FACE_OUTER_BOUND('',#15730,.T.);
#10464=FACE_OUTER_BOUND('',#15731,.T.);
#10465=FACE_OUTER_BOUND('',#15732,.T.);
#10466=FACE_OUTER_BOUND('',#15733,.T.);
#10467=FACE_OUTER_BOUND('',#15734,.T.);
#10468=FACE_OUTER_BOUND('',#15735,.T.);
#10469=FACE_OUTER_BOUND('',#15736,.T.);
#10470=FACE_OUTER_BOUND('',#15737,.T.);
#10471=FACE_OUTER_BOUND('',#15738,.T.);
#10472=FACE_OUTER_BOUND('',#15739,.T.);
#10473=FACE_OUTER_BOUND('',#15740,.T.);
#10474=FACE_OUTER_BOUND('',#15741,.T.);
#10475=FACE_OUTER_BOUND('',#15742,.T.);
#10476=FACE_OUTER_BOUND('',#15743,.T.);
#10477=FACE_OUTER_BOUND('',#15744,.T.);
#10478=FACE_OUTER_BOUND('',#15745,.T.);
#10479=FACE_OUTER_BOUND('',#15746,.T.);
#10480=FACE_OUTER_BOUND('',#15747,.T.);
#10481=FACE_OUTER_BOUND('',#15748,.T.);
#10482=FACE_OUTER_BOUND('',#15749,.T.);
#10483=FACE_OUTER_BOUND('',#15750,.T.);
#10484=FACE_OUTER_BOUND('',#15751,.T.);
#10485=FACE_OUTER_BOUND('',#15752,.T.);
#10486=FACE_OUTER_BOUND('',#15753,.T.);
#10487=FACE_OUTER_BOUND('',#15754,.T.);
#10488=FACE_OUTER_BOUND('',#15755,.T.);
#10489=FACE_OUTER_BOUND('',#15756,.T.);
#10490=FACE_OUTER_BOUND('',#15757,.T.);
#10491=FACE_OUTER_BOUND('',#15758,.T.);
#10492=FACE_OUTER_BOUND('',#15759,.T.);
#10493=FACE_OUTER_BOUND('',#15760,.T.);
#10494=FACE_OUTER_BOUND('',#15761,.T.);
#10495=FACE_OUTER_BOUND('',#15762,.T.);
#10496=FACE_OUTER_BOUND('',#15763,.T.);
#10497=FACE_OUTER_BOUND('',#15764,.T.);
#10498=FACE_OUTER_BOUND('',#15765,.T.);
#10499=FACE_OUTER_BOUND('',#15766,.T.);
#10500=FACE_OUTER_BOUND('',#15767,.T.);
#10501=FACE_OUTER_BOUND('',#15768,.T.);
#10502=FACE_OUTER_BOUND('',#15769,.T.);
#10503=FACE_OUTER_BOUND('',#15770,.T.);
#10504=FACE_OUTER_BOUND('',#15771,.T.);
#10505=FACE_OUTER_BOUND('',#15772,.T.);
#10506=FACE_OUTER_BOUND('',#15773,.T.);
#10507=FACE_OUTER_BOUND('',#15774,.T.);
#10508=FACE_OUTER_BOUND('',#15775,.T.);
#10509=FACE_OUTER_BOUND('',#15776,.T.);
#10510=FACE_OUTER_BOUND('',#15777,.T.);
#10511=FACE_OUTER_BOUND('',#15778,.T.);
#10512=FACE_OUTER_BOUND('',#15779,.T.);
#10513=FACE_OUTER_BOUND('',#15780,.T.);
#10514=FACE_OUTER_BOUND('',#15781,.T.);
#10515=FACE_OUTER_BOUND('',#15782,.T.);
#10516=FACE_OUTER_BOUND('',#15783,.T.);
#10517=FACE_OUTER_BOUND('',#15784,.T.);
#10518=FACE_OUTER_BOUND('',#15785,.T.);
#10519=FACE_OUTER_BOUND('',#15786,.T.);
#10520=FACE_OUTER_BOUND('',#15787,.T.);
#10521=FACE_OUTER_BOUND('',#15788,.T.);
#10522=FACE_OUTER_BOUND('',#15789,.T.);
#10523=FACE_OUTER_BOUND('',#15790,.T.);
#10524=FACE_OUTER_BOUND('',#15791,.T.);
#10525=FACE_OUTER_BOUND('',#15792,.T.);
#10526=FACE_OUTER_BOUND('',#15793,.T.);
#10527=FACE_OUTER_BOUND('',#15794,.T.);
#10528=FACE_OUTER_BOUND('',#15795,.T.);
#10529=FACE_OUTER_BOUND('',#15796,.T.);
#10530=FACE_OUTER_BOUND('',#15797,.T.);
#10531=FACE_OUTER_BOUND('',#15798,.T.);
#10532=FACE_OUTER_BOUND('',#15799,.T.);
#10533=FACE_OUTER_BOUND('',#15800,.T.);
#10534=FACE_OUTER_BOUND('',#15801,.T.);
#10535=FACE_OUTER_BOUND('',#15802,.T.);
#10536=FACE_OUTER_BOUND('',#15803,.T.);
#10537=FACE_OUTER_BOUND('',#15804,.T.);
#10538=FACE_OUTER_BOUND('',#15805,.T.);
#10539=FACE_OUTER_BOUND('',#15806,.T.);
#10540=FACE_OUTER_BOUND('',#15807,.T.);
#10541=FACE_OUTER_BOUND('',#15808,.T.);
#10542=FACE_OUTER_BOUND('',#15809,.T.);
#10543=FACE_OUTER_BOUND('',#15810,.T.);
#10544=FACE_OUTER_BOUND('',#15811,.T.);
#10545=FACE_OUTER_BOUND('',#15812,.T.);
#10546=FACE_OUTER_BOUND('',#15813,.T.);
#10547=FACE_OUTER_BOUND('',#15814,.T.);
#10548=FACE_OUTER_BOUND('',#15815,.T.);
#10549=FACE_OUTER_BOUND('',#15816,.T.);
#10550=FACE_OUTER_BOUND('',#15817,.T.);
#10551=FACE_OUTER_BOUND('',#15818,.T.);
#10552=FACE_OUTER_BOUND('',#15819,.T.);
#10553=FACE_OUTER_BOUND('',#15820,.T.);
#10554=FACE_OUTER_BOUND('',#15821,.T.);
#10555=FACE_OUTER_BOUND('',#15822,.T.);
#10556=FACE_OUTER_BOUND('',#15823,.T.);
#10557=FACE_OUTER_BOUND('',#15824,.T.);
#10558=FACE_OUTER_BOUND('',#15825,.T.);
#10559=FACE_OUTER_BOUND('',#15826,.T.);
#10560=FACE_OUTER_BOUND('',#15827,.T.);
#10561=FACE_OUTER_BOUND('',#15828,.T.);
#10562=FACE_OUTER_BOUND('',#15829,.T.);
#10563=FACE_OUTER_BOUND('',#15830,.T.);
#10564=FACE_OUTER_BOUND('',#15831,.T.);
#10565=FACE_OUTER_BOUND('',#15832,.T.);
#10566=FACE_OUTER_BOUND('',#15833,.T.);
#10567=FACE_OUTER_BOUND('',#15834,.T.);
#10568=FACE_OUTER_BOUND('',#15835,.T.);
#10569=FACE_OUTER_BOUND('',#15836,.T.);
#10570=FACE_OUTER_BOUND('',#15837,.T.);
#10571=FACE_OUTER_BOUND('',#15838,.T.);
#10572=FACE_OUTER_BOUND('',#15839,.T.);
#10573=FACE_OUTER_BOUND('',#15840,.T.);
#10574=FACE_OUTER_BOUND('',#15841,.T.);
#10575=FACE_OUTER_BOUND('',#15842,.T.);
#10576=FACE_OUTER_BOUND('',#15843,.T.);
#10577=FACE_OUTER_BOUND('',#15844,.T.);
#10578=FACE_OUTER_BOUND('',#15845,.T.);
#10579=FACE_OUTER_BOUND('',#15846,.T.);
#10580=FACE_OUTER_BOUND('',#15847,.T.);
#10581=FACE_OUTER_BOUND('',#15848,.T.);
#10582=FACE_OUTER_BOUND('',#15849,.T.);
#10583=FACE_OUTER_BOUND('',#15850,.T.);
#10584=FACE_OUTER_BOUND('',#15852,.T.);
#10648=EDGE_LOOP('',(#44646,#44647,#44648,#44649,#44650,#44651,#44652,#44653,
#44654,#44655,#44656,#44657,#44658,#44659,#44660,#44661,#44662,#44663,#44664,
#44665,#44666,#44667,#44668,#44669,#44670,#44671,#44672,#44673,#44674,#44675,
#44676,#44677,#44678,#44679,#44680,#44681,#44682,#44683,#44684,#44685,#44686,
#44687,#44688,#44689,#44690,#44691,#44692,#44693,#44694,#44695,#44696,#44697,
#44698,#44699,#44700,#44701,#44702,#44703,#44704,#44705,#44706,#44707,#44708,
#44709,#44710,#44711,#44712,#44713,#44714,#44715,#44716,#44717,#44718,#44719,
#44720,#44721,#44722,#44723,#44724,#44725,#44726,#44727,#44728,#44729,#44730,
#44731,#44732,#44733,#44734,#44735,#44736,#44737,#44738,#44739,#44740,#44741,
#44742,#44743,#44744,#44745,#44746,#44747,#44748,#44749,#44750,#44751,#44752,
#44753,#44754,#44755,#44756,#44757,#44758,#44759,#44760,#44761,#44762,#44763,
#44764,#44765,#44766,#44767,#44768,#44769,#44770,#44771,#44772,#44773,#44774,
#44775,#44776,#44777,#44778,#44779,#44780,#44781,#44782,#44783,#44784,#44785,
#44786,#44787,#44788,#44789,#44790,#44791,#44792,#44793,#44794,#44795,#44796,
#44797,#44798,#44799,#44800,#44801,#44802,#44803,#44804,#44805,#44806,#44807,
#44808,#44809,#44810,#44811,#44812,#44813,#44814,#44815,#44816,#44817,#44818,
#44819,#44820,#44821,#44822,#44823,#44824));
#10649=EDGE_LOOP('',(#44825,#44826,#44827,#44828));
#10650=EDGE_LOOP('',(#44829,#44830,#44831));
#10651=EDGE_LOOP('',(#44832,#44833,#44834,#44835));
#10652=EDGE_LOOP('',(#44836,#44837,#44838,#44839,#44840));
#10653=EDGE_LOOP('',(#44841,#44842,#44843,#44844,#44845));
#10654=EDGE_LOOP('',(#44846,#44847,#44848,#44849,#44850,#44851,#44852,#44853,
#44854,#44855,#44856,#44857,#44858,#44859,#44860,#44861,#44862,#44863,#44864,
#44865,#44866,#44867,#44868,#44869,#44870,#44871,#44872,#44873,#44874,#44875,
#44876,#44877,#44878,#44879,#44880,#44881,#44882,#44883,#44884,#44885,#44886,
#44887,#44888,#44889,#44890,#44891,#44892,#44893,#44894,#44895,#44896,#44897,
#44898,#44899,#44900,#44901,#44902,#44903,#44904,#44905,#44906,#44907,#44908,
#44909,#44910,#44911,#44912,#44913,#44914,#44915,#44916,#44917,#44918,#44919,
#44920,#44921,#44922,#44923,#44924,#44925,#44926,#44927,#44928,#44929,#44930,
#44931,#44932,#44933,#44934,#44935,#44936,#44937,#44938,#44939,#44940,#44941,
#44942,#44943,#44944,#44945,#44946,#44947,#44948,#44949,#44950,#44951,#44952,
#44953,#44954,#44955,#44956,#44957,#44958,#44959,#44960,#44961,#44962,#44963,
#44964,#44965,#44966,#44967,#44968,#44969,#44970,#44971,#44972,#44973,#44974,
#44975,#44976,#44977,#44978,#44979,#44980,#44981,#44982,#44983,#44984,#44985,
#44986,#44987,#44988,#44989,#44990,#44991,#44992,#44993,#44994,#44995,#44996,
#44997,#44998,#44999,#45000,#45001,#45002,#45003,#45004,#45005,#45006,#45007,
#45008,#45009,#45010,#45011,#45012,#45013,#45014,#45015,#45016,#45017,#45018,
#45019,#45020,#45021,#45022,#45023));
#10655=EDGE_LOOP('',(#45024,#45025,#45026,#45027));
#10656=EDGE_LOOP('',(#45028,#45029,#45030,#45031));
#10657=EDGE_LOOP('',(#45032,#45033,#45034,#45035,#45036));
#10658=EDGE_LOOP('',(#45037,#45038,#45039,#45040));
#10659=EDGE_LOOP('',(#45041,#45042,#45043,#45044));
#10660=EDGE_LOOP('',(#45045,#45046,#45047,#45048));
#10661=EDGE_LOOP('',(#45049,#45050,#45051,#45052));
#10662=EDGE_LOOP('',(#45053,#45054,#45055,#45056,#45057));
#10663=EDGE_LOOP('',(#45058,#45059,#45060));
#10664=EDGE_LOOP('',(#45061,#45062,#45063,#45064));
#10665=EDGE_LOOP('',(#45065,#45066,#45067,#45068));
#10666=EDGE_LOOP('',(#45069,#45070,#45071,#45072));
#10667=EDGE_LOOP('',(#45073,#45074,#45075,#45076));
#10668=EDGE_LOOP('',(#45077,#45078,#45079,#45080));
#10669=EDGE_LOOP('',(#45081,#45082,#45083,#45084));
#10670=EDGE_LOOP('',(#45085,#45086,#45087,#45088));
#10671=EDGE_LOOP('',(#45089,#45090,#45091,#45092));
#10672=EDGE_LOOP('',(#45093,#45094,#45095,#45096));
#10673=EDGE_LOOP('',(#45097,#45098,#45099,#45100));
#10674=EDGE_LOOP('',(#45101,#45102,#45103,#45104));
#10675=EDGE_LOOP('',(#45105,#45106,#45107,#45108));
#10676=EDGE_LOOP('',(#45109,#45110,#45111,#45112));
#10677=EDGE_LOOP('',(#45113,#45114,#45115,#45116));
#10678=EDGE_LOOP('',(#45117,#45118,#45119,#45120));
#10679=EDGE_LOOP('',(#45121,#45122,#45123,#45124));
#10680=EDGE_LOOP('',(#45125,#45126,#45127,#45128));
#10681=EDGE_LOOP('',(#45129,#45130,#45131,#45132));
#10682=EDGE_LOOP('',(#45133,#45134,#45135,#45136));
#10683=EDGE_LOOP('',(#45137,#45138,#45139,#45140));
#10684=EDGE_LOOP('',(#45141,#45142,#45143,#45144));
#10685=EDGE_LOOP('',(#45145,#45146,#45147,#45148));
#10686=EDGE_LOOP('',(#45149,#45150,#45151,#45152));
#10687=EDGE_LOOP('',(#45153,#45154,#45155,#45156));
#10688=EDGE_LOOP('',(#45157,#45158,#45159,#45160));
#10689=EDGE_LOOP('',(#45161,#45162,#45163,#45164));
#10690=EDGE_LOOP('',(#45165,#45166,#45167,#45168));
#10691=EDGE_LOOP('',(#45169,#45170,#45171,#45172));
#10692=EDGE_LOOP('',(#45173,#45174,#45175,#45176));
#10693=EDGE_LOOP('',(#45177,#45178,#45179,#45180));
#10694=EDGE_LOOP('',(#45181,#45182,#45183,#45184));
#10695=EDGE_LOOP('',(#45185,#45186,#45187,#45188));
#10696=EDGE_LOOP('',(#45189,#45190,#45191,#45192));
#10697=EDGE_LOOP('',(#45193,#45194,#45195,#45196));
#10698=EDGE_LOOP('',(#45197,#45198,#45199,#45200));
#10699=EDGE_LOOP('',(#45201,#45202,#45203,#45204));
#10700=EDGE_LOOP('',(#45205,#45206,#45207,#45208));
#10701=EDGE_LOOP('',(#45209,#45210,#45211,#45212));
#10702=EDGE_LOOP('',(#45213,#45214,#45215,#45216));
#10703=EDGE_LOOP('',(#45217,#45218,#45219,#45220));
#10704=EDGE_LOOP('',(#45221,#45222,#45223,#45224));
#10705=EDGE_LOOP('',(#45225,#45226,#45227,#45228));
#10706=EDGE_LOOP('',(#45229,#45230,#45231,#45232));
#10707=EDGE_LOOP('',(#45233,#45234,#45235,#45236));
#10708=EDGE_LOOP('',(#45237,#45238,#45239,#45240));
#10709=EDGE_LOOP('',(#45241,#45242,#45243,#45244));
#10710=EDGE_LOOP('',(#45245,#45246,#45247,#45248));
#10711=EDGE_LOOP('',(#45249,#45250,#45251,#45252));
#10712=EDGE_LOOP('',(#45253,#45254,#45255,#45256));
#10713=EDGE_LOOP('',(#45257,#45258,#45259,#45260));
#10714=EDGE_LOOP('',(#45261,#45262,#45263,#45264));
#10715=EDGE_LOOP('',(#45265,#45266,#45267,#45268));
#10716=EDGE_LOOP('',(#45269,#45270,#45271,#45272));
#10717=EDGE_LOOP('',(#45273,#45274,#45275,#45276));
#10718=EDGE_LOOP('',(#45277,#45278,#45279,#45280));
#10719=EDGE_LOOP('',(#45281,#45282,#45283,#45284));
#10720=EDGE_LOOP('',(#45285,#45286,#45287,#45288));
#10721=EDGE_LOOP('',(#45289,#45290,#45291,#45292));
#10722=EDGE_LOOP('',(#45293,#45294,#45295,#45296));
#10723=EDGE_LOOP('',(#45297,#45298,#45299,#45300));
#10724=EDGE_LOOP('',(#45301,#45302,#45303,#45304));
#10725=EDGE_LOOP('',(#45305,#45306,#45307,#45308));
#10726=EDGE_LOOP('',(#45309,#45310,#45311,#45312));
#10727=EDGE_LOOP('',(#45313,#45314,#45315,#45316));
#10728=EDGE_LOOP('',(#45317,#45318,#45319,#45320));
#10729=EDGE_LOOP('',(#45321,#45322,#45323,#45324));
#10730=EDGE_LOOP('',(#45325,#45326,#45327,#45328));
#10731=EDGE_LOOP('',(#45329,#45330,#45331,#45332));
#10732=EDGE_LOOP('',(#45333,#45334,#45335,#45336));
#10733=EDGE_LOOP('',(#45337,#45338,#45339,#45340));
#10734=EDGE_LOOP('',(#45341,#45342,#45343,#45344));
#10735=EDGE_LOOP('',(#45345,#45346,#45347,#45348));
#10736=EDGE_LOOP('',(#45349,#45350,#45351,#45352));
#10737=EDGE_LOOP('',(#45353,#45354,#45355,#45356));
#10738=EDGE_LOOP('',(#45357,#45358,#45359,#45360));
#10739=EDGE_LOOP('',(#45361,#45362,#45363,#45364));
#10740=EDGE_LOOP('',(#45365,#45366,#45367,#45368));
#10741=EDGE_LOOP('',(#45369,#45370,#45371,#45372));
#10742=EDGE_LOOP('',(#45373,#45374,#45375,#45376));
#10743=EDGE_LOOP('',(#45377,#45378,#45379,#45380));
#10744=EDGE_LOOP('',(#45381,#45382,#45383,#45384));
#10745=EDGE_LOOP('',(#45385,#45386,#45387,#45388));
#10746=EDGE_LOOP('',(#45389,#45390,#45391,#45392));
#10747=EDGE_LOOP('',(#45393,#45394,#45395,#45396));
#10748=EDGE_LOOP('',(#45397,#45398,#45399,#45400));
#10749=EDGE_LOOP('',(#45401,#45402,#45403,#45404));
#10750=EDGE_LOOP('',(#45405,#45406,#45407,#45408));
#10751=EDGE_LOOP('',(#45409,#45410,#45411,#45412));
#10752=EDGE_LOOP('',(#45413,#45414,#45415,#45416));
#10753=EDGE_LOOP('',(#45417,#45418,#45419,#45420));
#10754=EDGE_LOOP('',(#45421,#45422,#45423,#45424));
#10755=EDGE_LOOP('',(#45425,#45426,#45427,#45428));
#10756=EDGE_LOOP('',(#45429,#45430,#45431,#45432));
#10757=EDGE_LOOP('',(#45433,#45434,#45435,#45436));
#10758=EDGE_LOOP('',(#45437,#45438,#45439,#45440));
#10759=EDGE_LOOP('',(#45441,#45442,#45443,#45444));
#10760=EDGE_LOOP('',(#45445,#45446,#45447,#45448));
#10761=EDGE_LOOP('',(#45449,#45450,#45451,#45452));
#10762=EDGE_LOOP('',(#45453,#45454,#45455,#45456));
#10763=EDGE_LOOP('',(#45457,#45458,#45459,#45460));
#10764=EDGE_LOOP('',(#45461,#45462,#45463,#45464));
#10765=EDGE_LOOP('',(#45465,#45466,#45467,#45468));
#10766=EDGE_LOOP('',(#45469,#45470,#45471,#45472));
#10767=EDGE_LOOP('',(#45473,#45474,#45475,#45476));
#10768=EDGE_LOOP('',(#45477,#45478,#45479,#45480));
#10769=EDGE_LOOP('',(#45481,#45482,#45483,#45484));
#10770=EDGE_LOOP('',(#45485,#45486,#45487,#45488));
#10771=EDGE_LOOP('',(#45489,#45490,#45491,#45492));
#10772=EDGE_LOOP('',(#45493,#45494,#45495,#45496));
#10773=EDGE_LOOP('',(#45497,#45498,#45499,#45500));
#10774=EDGE_LOOP('',(#45501,#45502,#45503,#45504));
#10775=EDGE_LOOP('',(#45505,#45506,#45507,#45508));
#10776=EDGE_LOOP('',(#45509,#45510,#45511,#45512));
#10777=EDGE_LOOP('',(#45513,#45514,#45515,#45516));
#10778=EDGE_LOOP('',(#45517,#45518,#45519,#45520));
#10779=EDGE_LOOP('',(#45521,#45522,#45523,#45524));
#10780=EDGE_LOOP('',(#45525,#45526,#45527,#45528));
#10781=EDGE_LOOP('',(#45529,#45530,#45531,#45532));
#10782=EDGE_LOOP('',(#45533,#45534,#45535,#45536));
#10783=EDGE_LOOP('',(#45537,#45538,#45539,#45540));
#10784=EDGE_LOOP('',(#45541,#45542,#45543,#45544));
#10785=EDGE_LOOP('',(#45545,#45546,#45547,#45548));
#10786=EDGE_LOOP('',(#45549,#45550,#45551,#45552));
#10787=EDGE_LOOP('',(#45553,#45554,#45555,#45556));
#10788=EDGE_LOOP('',(#45557,#45558,#45559,#45560));
#10789=EDGE_LOOP('',(#45561,#45562,#45563,#45564));
#10790=EDGE_LOOP('',(#45565,#45566,#45567,#45568));
#10791=EDGE_LOOP('',(#45569,#45570,#45571,#45572));
#10792=EDGE_LOOP('',(#45573,#45574,#45575,#45576));
#10793=EDGE_LOOP('',(#45577,#45578,#45579,#45580));
#10794=EDGE_LOOP('',(#45581,#45582,#45583,#45584));
#10795=EDGE_LOOP('',(#45585,#45586,#45587,#45588));
#10796=EDGE_LOOP('',(#45589,#45590,#45591,#45592));
#10797=EDGE_LOOP('',(#45593,#45594,#45595,#45596));
#10798=EDGE_LOOP('',(#45597,#45598,#45599,#45600));
#10799=EDGE_LOOP('',(#45601,#45602,#45603,#45604));
#10800=EDGE_LOOP('',(#45605,#45606,#45607,#45608));
#10801=EDGE_LOOP('',(#45609,#45610,#45611,#45612));
#10802=EDGE_LOOP('',(#45613,#45614,#45615,#45616));
#10803=EDGE_LOOP('',(#45617,#45618,#45619,#45620));
#10804=EDGE_LOOP('',(#45621,#45622,#45623,#45624));
#10805=EDGE_LOOP('',(#45625,#45626,#45627,#45628));
#10806=EDGE_LOOP('',(#45629,#45630,#45631,#45632));
#10807=EDGE_LOOP('',(#45633,#45634,#45635,#45636));
#10808=EDGE_LOOP('',(#45637,#45638,#45639,#45640));
#10809=EDGE_LOOP('',(#45641,#45642,#45643,#45644));
#10810=EDGE_LOOP('',(#45645,#45646,#45647,#45648));
#10811=EDGE_LOOP('',(#45649,#45650,#45651,#45652));
#10812=EDGE_LOOP('',(#45653,#45654,#45655,#45656));
#10813=EDGE_LOOP('',(#45657,#45658,#45659,#45660));
#10814=EDGE_LOOP('',(#45661,#45662,#45663,#45664));
#10815=EDGE_LOOP('',(#45665,#45666,#45667,#45668));
#10816=EDGE_LOOP('',(#45669,#45670,#45671,#45672));
#10817=EDGE_LOOP('',(#45673,#45674,#45675,#45676));
#10818=EDGE_LOOP('',(#45677,#45678,#45679,#45680));
#10819=EDGE_LOOP('',(#45681,#45682,#45683,#45684));
#10820=EDGE_LOOP('',(#45685,#45686,#45687,#45688));
#10821=EDGE_LOOP('',(#45689,#45690,#45691,#45692));
#10822=EDGE_LOOP('',(#45693,#45694,#45695,#45696));
#10823=EDGE_LOOP('',(#45697,#45698,#45699,#45700));
#10824=EDGE_LOOP('',(#45701,#45702,#45703,#45704));
#10825=EDGE_LOOP('',(#45705,#45706,#45707,#45708));
#10826=EDGE_LOOP('',(#45709,#45710,#45711,#45712));
#10827=EDGE_LOOP('',(#45713,#45714,#45715,#45716));
#10828=EDGE_LOOP('',(#45717,#45718,#45719,#45720));
#10829=EDGE_LOOP('',(#45721,#45722,#45723,#45724));
#10830=EDGE_LOOP('',(#45725,#45726,#45727,#45728));
#10831=EDGE_LOOP('',(#45729,#45730,#45731,#45732));
#10832=EDGE_LOOP('',(#45733,#45734,#45735,#45736));
#10833=EDGE_LOOP('',(#45737,#45738,#45739,#45740));
#10834=EDGE_LOOP('',(#45741,#45742,#45743,#45744));
#10835=EDGE_LOOP('',(#45745,#45746,#45747,#45748));
#10836=EDGE_LOOP('',(#45749,#45750,#45751,#45752));
#10837=EDGE_LOOP('',(#45753,#45754,#45755,#45756));
#10838=EDGE_LOOP('',(#45757,#45758,#45759,#45760));
#10839=EDGE_LOOP('',(#45761,#45762,#45763,#45764));
#10840=EDGE_LOOP('',(#45765,#45766,#45767,#45768));
#10841=EDGE_LOOP('',(#45769,#45770,#45771,#45772));
#10842=EDGE_LOOP('',(#45773,#45774,#45775,#45776));
#10843=EDGE_LOOP('',(#45777,#45778,#45779,#45780));
#10844=EDGE_LOOP('',(#45781,#45782,#45783,#45784));
#10845=EDGE_LOOP('',(#45785,#45786,#45787,#45788));
#10846=EDGE_LOOP('',(#45789,#45790,#45791,#45792));
#10847=EDGE_LOOP('',(#45793,#45794,#45795,#45796));
#10848=EDGE_LOOP('',(#45797,#45798,#45799,#45800));
#10849=EDGE_LOOP('',(#45801,#45802,#45803,#45804));
#10850=EDGE_LOOP('',(#45805,#45806,#45807,#45808));
#10851=EDGE_LOOP('',(#45809,#45810,#45811,#45812));
#10852=EDGE_LOOP('',(#45813,#45814,#45815,#45816));
#10853=EDGE_LOOP('',(#45817,#45818,#45819,#45820));
#10854=EDGE_LOOP('',(#45821,#45822,#45823,#45824));
#10855=EDGE_LOOP('',(#45825,#45826,#45827,#45828));
#10856=EDGE_LOOP('',(#45829,#45830,#45831,#45832));
#10857=EDGE_LOOP('',(#45833,#45834,#45835,#45836));
#10858=EDGE_LOOP('',(#45837,#45838,#45839,#45840));
#10859=EDGE_LOOP('',(#45841,#45842,#45843,#45844));
#10860=EDGE_LOOP('',(#45845,#45846,#45847,#45848));
#10861=EDGE_LOOP('',(#45849,#45850,#45851,#45852));
#10862=EDGE_LOOP('',(#45853,#45854,#45855,#45856));
#10863=EDGE_LOOP('',(#45857,#45858,#45859,#45860));
#10864=EDGE_LOOP('',(#45861,#45862,#45863,#45864));
#10865=EDGE_LOOP('',(#45865,#45866,#45867,#45868));
#10866=EDGE_LOOP('',(#45869,#45870,#45871,#45872));
#10867=EDGE_LOOP('',(#45873,#45874,#45875,#45876));
#10868=EDGE_LOOP('',(#45877,#45878,#45879,#45880));
#10869=EDGE_LOOP('',(#45881,#45882,#45883,#45884));
#10870=EDGE_LOOP('',(#45885,#45886,#45887,#45888));
#10871=EDGE_LOOP('',(#45889,#45890,#45891,#45892));
#10872=EDGE_LOOP('',(#45893,#45894,#45895,#45896));
#10873=EDGE_LOOP('',(#45897,#45898,#45899,#45900));
#10874=EDGE_LOOP('',(#45901,#45902,#45903,#45904));
#10875=EDGE_LOOP('',(#45905,#45906,#45907,#45908));
#10876=EDGE_LOOP('',(#45909,#45910,#45911,#45912));
#10877=EDGE_LOOP('',(#45913,#45914,#45915,#45916));
#10878=EDGE_LOOP('',(#45917,#45918,#45919,#45920));
#10879=EDGE_LOOP('',(#45921,#45922,#45923,#45924));
#10880=EDGE_LOOP('',(#45925,#45926,#45927,#45928));
#10881=EDGE_LOOP('',(#45929,#45930,#45931,#45932));
#10882=EDGE_LOOP('',(#45933,#45934,#45935,#45936));
#10883=EDGE_LOOP('',(#45937,#45938,#45939,#45940));
#10884=EDGE_LOOP('',(#45941,#45942,#45943,#45944));
#10885=EDGE_LOOP('',(#45945,#45946,#45947,#45948));
#10886=EDGE_LOOP('',(#45949,#45950,#45951,#45952));
#10887=EDGE_LOOP('',(#45953,#45954,#45955,#45956));
#10888=EDGE_LOOP('',(#45957,#45958,#45959,#45960));
#10889=EDGE_LOOP('',(#45961,#45962,#45963,#45964));
#10890=EDGE_LOOP('',(#45965,#45966,#45967,#45968));
#10891=EDGE_LOOP('',(#45969,#45970,#45971,#45972));
#10892=EDGE_LOOP('',(#45973,#45974,#45975,#45976));
#10893=EDGE_LOOP('',(#45977,#45978,#45979,#45980));
#10894=EDGE_LOOP('',(#45981,#45982,#45983,#45984));
#10895=EDGE_LOOP('',(#45985,#45986,#45987,#45988));
#10896=EDGE_LOOP('',(#45989,#45990,#45991,#45992));
#10897=EDGE_LOOP('',(#45993,#45994,#45995,#45996));
#10898=EDGE_LOOP('',(#45997,#45998,#45999,#46000));
#10899=EDGE_LOOP('',(#46001,#46002,#46003,#46004));
#10900=EDGE_LOOP('',(#46005,#46006,#46007,#46008));
#10901=EDGE_LOOP('',(#46009,#46010,#46011,#46012));
#10902=EDGE_LOOP('',(#46013,#46014,#46015,#46016));
#10903=EDGE_LOOP('',(#46017,#46018,#46019,#46020));
#10904=EDGE_LOOP('',(#46021,#46022,#46023,#46024));
#10905=EDGE_LOOP('',(#46025,#46026,#46027,#46028));
#10906=EDGE_LOOP('',(#46029,#46030,#46031,#46032));
#10907=EDGE_LOOP('',(#46033,#46034,#46035,#46036));
#10908=EDGE_LOOP('',(#46037,#46038,#46039,#46040));
#10909=EDGE_LOOP('',(#46041,#46042,#46043,#46044));
#10910=EDGE_LOOP('',(#46045,#46046,#46047,#46048));
#10911=EDGE_LOOP('',(#46049,#46050,#46051,#46052));
#10912=EDGE_LOOP('',(#46053,#46054,#46055,#46056));
#10913=EDGE_LOOP('',(#46057,#46058,#46059,#46060));
#10914=EDGE_LOOP('',(#46061,#46062,#46063,#46064));
#10915=EDGE_LOOP('',(#46065,#46066,#46067,#46068));
#10916=EDGE_LOOP('',(#46069,#46070,#46071,#46072));
#10917=EDGE_LOOP('',(#46073,#46074,#46075,#46076));
#10918=EDGE_LOOP('',(#46077,#46078,#46079,#46080));
#10919=EDGE_LOOP('',(#46081,#46082,#46083,#46084));
#10920=EDGE_LOOP('',(#46085,#46086,#46087,#46088));
#10921=EDGE_LOOP('',(#46089,#46090,#46091,#46092));
#10922=EDGE_LOOP('',(#46093,#46094,#46095,#46096));
#10923=EDGE_LOOP('',(#46097,#46098,#46099,#46100));
#10924=EDGE_LOOP('',(#46101,#46102,#46103,#46104));
#10925=EDGE_LOOP('',(#46105,#46106,#46107,#46108));
#10926=EDGE_LOOP('',(#46109,#46110,#46111,#46112));
#10927=EDGE_LOOP('',(#46113,#46114,#46115,#46116));
#10928=EDGE_LOOP('',(#46117,#46118,#46119,#46120));
#10929=EDGE_LOOP('',(#46121,#46122,#46123,#46124));
#10930=EDGE_LOOP('',(#46125,#46126,#46127,#46128));
#10931=EDGE_LOOP('',(#46129,#46130,#46131,#46132));
#10932=EDGE_LOOP('',(#46133,#46134,#46135,#46136));
#10933=EDGE_LOOP('',(#46137,#46138,#46139,#46140));
#10934=EDGE_LOOP('',(#46141,#46142,#46143,#46144));
#10935=EDGE_LOOP('',(#46145,#46146,#46147,#46148));
#10936=EDGE_LOOP('',(#46149,#46150,#46151,#46152));
#10937=EDGE_LOOP('',(#46153,#46154,#46155,#46156));
#10938=EDGE_LOOP('',(#46157,#46158,#46159,#46160));
#10939=EDGE_LOOP('',(#46161,#46162,#46163,#46164));
#10940=EDGE_LOOP('',(#46165,#46166,#46167,#46168));
#10941=EDGE_LOOP('',(#46169,#46170,#46171,#46172));
#10942=EDGE_LOOP('',(#46173,#46174,#46175,#46176));
#10943=EDGE_LOOP('',(#46177,#46178,#46179,#46180));
#10944=EDGE_LOOP('',(#46181,#46182,#46183,#46184));
#10945=EDGE_LOOP('',(#46185,#46186,#46187,#46188));
#10946=EDGE_LOOP('',(#46189,#46190,#46191,#46192));
#10947=EDGE_LOOP('',(#46193,#46194,#46195,#46196));
#10948=EDGE_LOOP('',(#46197,#46198,#46199,#46200));
#10949=EDGE_LOOP('',(#46201,#46202,#46203,#46204));
#10950=EDGE_LOOP('',(#46205,#46206,#46207,#46208));
#10951=EDGE_LOOP('',(#46209,#46210,#46211,#46212));
#10952=EDGE_LOOP('',(#46213,#46214,#46215,#46216));
#10953=EDGE_LOOP('',(#46217,#46218,#46219,#46220));
#10954=EDGE_LOOP('',(#46221,#46222,#46223,#46224));
#10955=EDGE_LOOP('',(#46225,#46226,#46227,#46228));
#10956=EDGE_LOOP('',(#46229,#46230,#46231,#46232));
#10957=EDGE_LOOP('',(#46233,#46234,#46235,#46236));
#10958=EDGE_LOOP('',(#46237,#46238,#46239,#46240));
#10959=EDGE_LOOP('',(#46241,#46242,#46243,#46244));
#10960=EDGE_LOOP('',(#46245,#46246,#46247,#46248));
#10961=EDGE_LOOP('',(#46249,#46250,#46251,#46252));
#10962=EDGE_LOOP('',(#46253,#46254,#46255,#46256));
#10963=EDGE_LOOP('',(#46257,#46258,#46259,#46260));
#10964=EDGE_LOOP('',(#46261,#46262,#46263,#46264));
#10965=EDGE_LOOP('',(#46265,#46266,#46267,#46268));
#10966=EDGE_LOOP('',(#46269,#46270,#46271,#46272));
#10967=EDGE_LOOP('',(#46273,#46274,#46275,#46276));
#10968=EDGE_LOOP('',(#46277,#46278,#46279,#46280));
#10969=EDGE_LOOP('',(#46281,#46282,#46283,#46284));
#10970=EDGE_LOOP('',(#46285,#46286,#46287,#46288));
#10971=EDGE_LOOP('',(#46289,#46290,#46291,#46292));
#10972=EDGE_LOOP('',(#46293,#46294,#46295,#46296));
#10973=EDGE_LOOP('',(#46297,#46298,#46299,#46300));
#10974=EDGE_LOOP('',(#46301,#46302,#46303,#46304));
#10975=EDGE_LOOP('',(#46305,#46306,#46307,#46308));
#10976=EDGE_LOOP('',(#46309,#46310,#46311,#46312));
#10977=EDGE_LOOP('',(#46313,#46314,#46315,#46316));
#10978=EDGE_LOOP('',(#46317,#46318,#46319,#46320));
#10979=EDGE_LOOP('',(#46321,#46322,#46323,#46324));
#10980=EDGE_LOOP('',(#46325,#46326,#46327,#46328));
#10981=EDGE_LOOP('',(#46329,#46330,#46331,#46332));
#10982=EDGE_LOOP('',(#46333,#46334,#46335,#46336));
#10983=EDGE_LOOP('',(#46337,#46338,#46339,#46340));
#10984=EDGE_LOOP('',(#46341,#46342,#46343,#46344));
#10985=EDGE_LOOP('',(#46345,#46346,#46347,#46348));
#10986=EDGE_LOOP('',(#46349,#46350,#46351,#46352));
#10987=EDGE_LOOP('',(#46353,#46354,#46355,#46356));
#10988=EDGE_LOOP('',(#46357,#46358,#46359,#46360));
#10989=EDGE_LOOP('',(#46361,#46362,#46363,#46364));
#10990=EDGE_LOOP('',(#46365,#46366,#46367,#46368));
#10991=EDGE_LOOP('',(#46369,#46370,#46371,#46372));
#10992=EDGE_LOOP('',(#46373,#46374,#46375,#46376));
#10993=EDGE_LOOP('',(#46377,#46378,#46379,#46380));
#10994=EDGE_LOOP('',(#46381,#46382,#46383,#46384));
#10995=EDGE_LOOP('',(#46385,#46386,#46387,#46388));
#10996=EDGE_LOOP('',(#46389,#46390,#46391,#46392));
#10997=EDGE_LOOP('',(#46393,#46394,#46395,#46396));
#10998=EDGE_LOOP('',(#46397,#46398,#46399,#46400));
#10999=EDGE_LOOP('',(#46401,#46402,#46403,#46404));
#11000=EDGE_LOOP('',(#46405,#46406,#46407,#46408));
#11001=EDGE_LOOP('',(#46409,#46410,#46411,#46412));
#11002=EDGE_LOOP('',(#46413,#46414,#46415,#46416));
#11003=EDGE_LOOP('',(#46417,#46418,#46419,#46420));
#11004=EDGE_LOOP('',(#46421,#46422,#46423,#46424));
#11005=EDGE_LOOP('',(#46425,#46426,#46427,#46428));
#11006=EDGE_LOOP('',(#46429,#46430,#46431,#46432));
#11007=EDGE_LOOP('',(#46433,#46434,#46435,#46436));
#11008=EDGE_LOOP('',(#46437,#46438,#46439,#46440));
#11009=EDGE_LOOP('',(#46441,#46442,#46443,#46444));
#11010=EDGE_LOOP('',(#46445,#46446,#46447,#46448));
#11011=EDGE_LOOP('',(#46449,#46450,#46451,#46452));
#11012=EDGE_LOOP('',(#46453,#46454,#46455,#46456));
#11013=EDGE_LOOP('',(#46457,#46458,#46459,#46460));
#11014=EDGE_LOOP('',(#46461,#46462,#46463,#46464));
#11015=EDGE_LOOP('',(#46465,#46466,#46467,#46468));
#11016=EDGE_LOOP('',(#46469,#46470,#46471,#46472));
#11017=EDGE_LOOP('',(#46473,#46474,#46475,#46476));
#11018=EDGE_LOOP('',(#46477,#46478,#46479,#46480));
#11019=EDGE_LOOP('',(#46481,#46482,#46483,#46484));
#11020=EDGE_LOOP('',(#46485,#46486,#46487,#46488));
#11021=EDGE_LOOP('',(#46489,#46490,#46491,#46492));
#11022=EDGE_LOOP('',(#46493,#46494,#46495,#46496));
#11023=EDGE_LOOP('',(#46497,#46498,#46499,#46500));
#11024=EDGE_LOOP('',(#46501,#46502,#46503,#46504));
#11025=EDGE_LOOP('',(#46505,#46506,#46507,#46508));
#11026=EDGE_LOOP('',(#46509,#46510,#46511,#46512));
#11027=EDGE_LOOP('',(#46513,#46514,#46515,#46516));
#11028=EDGE_LOOP('',(#46517,#46518,#46519,#46520));
#11029=EDGE_LOOP('',(#46521,#46522,#46523,#46524));
#11030=EDGE_LOOP('',(#46525,#46526,#46527,#46528));
#11031=EDGE_LOOP('',(#46529,#46530,#46531,#46532));
#11032=EDGE_LOOP('',(#46533,#46534,#46535,#46536));
#11033=EDGE_LOOP('',(#46537,#46538,#46539,#46540));
#11034=EDGE_LOOP('',(#46541,#46542,#46543,#46544));
#11035=EDGE_LOOP('',(#46545,#46546,#46547,#46548));
#11036=EDGE_LOOP('',(#46549,#46550,#46551,#46552));
#11037=EDGE_LOOP('',(#46553,#46554,#46555,#46556));
#11038=EDGE_LOOP('',(#46557,#46558,#46559,#46560));
#11039=EDGE_LOOP('',(#46561,#46562,#46563,#46564));
#11040=EDGE_LOOP('',(#46565,#46566,#46567,#46568));
#11041=EDGE_LOOP('',(#46569,#46570,#46571,#46572));
#11042=EDGE_LOOP('',(#46573,#46574,#46575,#46576));
#11043=EDGE_LOOP('',(#46577,#46578,#46579,#46580));
#11044=EDGE_LOOP('',(#46581,#46582,#46583,#46584));
#11045=EDGE_LOOP('',(#46585,#46586,#46587,#46588));
#11046=EDGE_LOOP('',(#46589,#46590,#46591,#46592));
#11047=EDGE_LOOP('',(#46593,#46594,#46595,#46596));
#11048=EDGE_LOOP('',(#46597,#46598,#46599,#46600));
#11049=EDGE_LOOP('',(#46601,#46602,#46603,#46604));
#11050=EDGE_LOOP('',(#46605,#46606,#46607,#46608));
#11051=EDGE_LOOP('',(#46609,#46610,#46611,#46612));
#11052=EDGE_LOOP('',(#46613,#46614,#46615,#46616));
#11053=EDGE_LOOP('',(#46617,#46618,#46619,#46620));
#11054=EDGE_LOOP('',(#46621,#46622,#46623,#46624));
#11055=EDGE_LOOP('',(#46625,#46626,#46627,#46628));
#11056=EDGE_LOOP('',(#46629,#46630,#46631,#46632));
#11057=EDGE_LOOP('',(#46633,#46634,#46635,#46636));
#11058=EDGE_LOOP('',(#46637,#46638,#46639,#46640));
#11059=EDGE_LOOP('',(#46641,#46642,#46643,#46644));
#11060=EDGE_LOOP('',(#46645,#46646,#46647,#46648));
#11061=EDGE_LOOP('',(#46649,#46650,#46651,#46652));
#11062=EDGE_LOOP('',(#46653,#46654,#46655,#46656));
#11063=EDGE_LOOP('',(#46657,#46658,#46659,#46660));
#11064=EDGE_LOOP('',(#46661,#46662,#46663,#46664));
#11065=EDGE_LOOP('',(#46665,#46666,#46667,#46668));
#11066=EDGE_LOOP('',(#46669,#46670,#46671,#46672));
#11067=EDGE_LOOP('',(#46673,#46674,#46675,#46676));
#11068=EDGE_LOOP('',(#46677,#46678,#46679,#46680));
#11069=EDGE_LOOP('',(#46681,#46682,#46683,#46684));
#11070=EDGE_LOOP('',(#46685,#46686,#46687,#46688));
#11071=EDGE_LOOP('',(#46689,#46690,#46691,#46692));
#11072=EDGE_LOOP('',(#46693,#46694,#46695,#46696));
#11073=EDGE_LOOP('',(#46697,#46698,#46699,#46700));
#11074=EDGE_LOOP('',(#46701,#46702,#46703,#46704));
#11075=EDGE_LOOP('',(#46705,#46706,#46707,#46708));
#11076=EDGE_LOOP('',(#46709,#46710,#46711,#46712));
#11077=EDGE_LOOP('',(#46713,#46714,#46715,#46716));
#11078=EDGE_LOOP('',(#46717,#46718,#46719,#46720));
#11079=EDGE_LOOP('',(#46721,#46722,#46723,#46724));
#11080=EDGE_LOOP('',(#46725,#46726,#46727,#46728));
#11081=EDGE_LOOP('',(#46729,#46730,#46731,#46732));
#11082=EDGE_LOOP('',(#46733,#46734,#46735,#46736));
#11083=EDGE_LOOP('',(#46737,#46738,#46739,#46740));
#11084=EDGE_LOOP('',(#46741,#46742,#46743,#46744));
#11085=EDGE_LOOP('',(#46745,#46746,#46747,#46748));
#11086=EDGE_LOOP('',(#46749,#46750,#46751,#46752));
#11087=EDGE_LOOP('',(#46753,#46754,#46755,#46756));
#11088=EDGE_LOOP('',(#46757,#46758,#46759,#46760));
#11089=EDGE_LOOP('',(#46761,#46762,#46763,#46764));
#11090=EDGE_LOOP('',(#46765,#46766,#46767,#46768));
#11091=EDGE_LOOP('',(#46769,#46770,#46771,#46772));
#11092=EDGE_LOOP('',(#46773,#46774,#46775,#46776));
#11093=EDGE_LOOP('',(#46777,#46778,#46779,#46780));
#11094=EDGE_LOOP('',(#46781,#46782,#46783,#46784));
#11095=EDGE_LOOP('',(#46785,#46786,#46787,#46788));
#11096=EDGE_LOOP('',(#46789,#46790,#46791,#46792));
#11097=EDGE_LOOP('',(#46793,#46794,#46795,#46796));
#11098=EDGE_LOOP('',(#46797,#46798,#46799,#46800));
#11099=EDGE_LOOP('',(#46801,#46802,#46803,#46804));
#11100=EDGE_LOOP('',(#46805,#46806,#46807,#46808));
#11101=EDGE_LOOP('',(#46809,#46810,#46811,#46812));
#11102=EDGE_LOOP('',(#46813,#46814,#46815,#46816));
#11103=EDGE_LOOP('',(#46817,#46818,#46819,#46820));
#11104=EDGE_LOOP('',(#46821,#46822,#46823,#46824));
#11105=EDGE_LOOP('',(#46825,#46826,#46827,#46828));
#11106=EDGE_LOOP('',(#46829,#46830,#46831,#46832));
#11107=EDGE_LOOP('',(#46833,#46834,#46835,#46836));
#11108=EDGE_LOOP('',(#46837,#46838,#46839,#46840));
#11109=EDGE_LOOP('',(#46841,#46842,#46843,#46844));
#11110=EDGE_LOOP('',(#46845,#46846,#46847,#46848));
#11111=EDGE_LOOP('',(#46849,#46850,#46851,#46852));
#11112=EDGE_LOOP('',(#46853,#46854,#46855,#46856));
#11113=EDGE_LOOP('',(#46857,#46858,#46859,#46860));
#11114=EDGE_LOOP('',(#46861,#46862,#46863,#46864));
#11115=EDGE_LOOP('',(#46865,#46866,#46867,#46868));
#11116=EDGE_LOOP('',(#46869,#46870,#46871,#46872));
#11117=EDGE_LOOP('',(#46873,#46874,#46875,#46876));
#11118=EDGE_LOOP('',(#46877,#46878,#46879,#46880));
#11119=EDGE_LOOP('',(#46881,#46882,#46883,#46884));
#11120=EDGE_LOOP('',(#46885,#46886,#46887,#46888));
#11121=EDGE_LOOP('',(#46889,#46890,#46891,#46892));
#11122=EDGE_LOOP('',(#46893,#46894,#46895,#46896));
#11123=EDGE_LOOP('',(#46897,#46898,#46899,#46900));
#11124=EDGE_LOOP('',(#46901,#46902,#46903,#46904));
#11125=EDGE_LOOP('',(#46905,#46906,#46907,#46908));
#11126=EDGE_LOOP('',(#46909,#46910,#46911,#46912));
#11127=EDGE_LOOP('',(#46913,#46914,#46915,#46916));
#11128=EDGE_LOOP('',(#46917,#46918,#46919,#46920));
#11129=EDGE_LOOP('',(#46921,#46922,#46923,#46924));
#11130=EDGE_LOOP('',(#46925,#46926,#46927,#46928));
#11131=EDGE_LOOP('',(#46929,#46930,#46931,#46932));
#11132=EDGE_LOOP('',(#46933,#46934,#46935,#46936));
#11133=EDGE_LOOP('',(#46937,#46938,#46939,#46940));
#11134=EDGE_LOOP('',(#46941,#46942,#46943,#46944));
#11135=EDGE_LOOP('',(#46945,#46946,#46947,#46948));
#11136=EDGE_LOOP('',(#46949,#46950,#46951,#46952));
#11137=EDGE_LOOP('',(#46953,#46954,#46955,#46956));
#11138=EDGE_LOOP('',(#46957,#46958,#46959,#46960));
#11139=EDGE_LOOP('',(#46961,#46962,#46963,#46964));
#11140=EDGE_LOOP('',(#46965,#46966,#46967,#46968));
#11141=EDGE_LOOP('',(#46969,#46970,#46971,#46972));
#11142=EDGE_LOOP('',(#46973,#46974,#46975,#46976));
#11143=EDGE_LOOP('',(#46977,#46978,#46979,#46980));
#11144=EDGE_LOOP('',(#46981,#46982,#46983,#46984));
#11145=EDGE_LOOP('',(#46985,#46986,#46987,#46988));
#11146=EDGE_LOOP('',(#46989,#46990,#46991,#46992));
#11147=EDGE_LOOP('',(#46993,#46994,#46995,#46996));
#11148=EDGE_LOOP('',(#46997,#46998,#46999,#47000));
#11149=EDGE_LOOP('',(#47001,#47002,#47003,#47004));
#11150=EDGE_LOOP('',(#47005,#47006,#47007,#47008));
#11151=EDGE_LOOP('',(#47009,#47010,#47011,#47012));
#11152=EDGE_LOOP('',(#47013,#47014,#47015,#47016));
#11153=EDGE_LOOP('',(#47017,#47018,#47019,#47020));
#11154=EDGE_LOOP('',(#47021,#47022,#47023,#47024));
#11155=EDGE_LOOP('',(#47025,#47026,#47027,#47028));
#11156=EDGE_LOOP('',(#47029,#47030,#47031,#47032));
#11157=EDGE_LOOP('',(#47033,#47034,#47035,#47036));
#11158=EDGE_LOOP('',(#47037,#47038,#47039,#47040));
#11159=EDGE_LOOP('',(#47041,#47042,#47043,#47044));
#11160=EDGE_LOOP('',(#47045,#47046,#47047,#47048));
#11161=EDGE_LOOP('',(#47049,#47050,#47051,#47052));
#11162=EDGE_LOOP('',(#47053,#47054,#47055,#47056));
#11163=EDGE_LOOP('',(#47057,#47058,#47059,#47060));
#11164=EDGE_LOOP('',(#47061,#47062,#47063,#47064));
#11165=EDGE_LOOP('',(#47065,#47066,#47067,#47068));
#11166=EDGE_LOOP('',(#47069,#47070,#47071,#47072));
#11167=EDGE_LOOP('',(#47073,#47074,#47075,#47076));
#11168=EDGE_LOOP('',(#47077,#47078,#47079,#47080));
#11169=EDGE_LOOP('',(#47081,#47082,#47083,#47084));
#11170=EDGE_LOOP('',(#47085,#47086,#47087,#47088));
#11171=EDGE_LOOP('',(#47089,#47090,#47091,#47092));
#11172=EDGE_LOOP('',(#47093,#47094,#47095,#47096));
#11173=EDGE_LOOP('',(#47097,#47098,#47099,#47100));
#11174=EDGE_LOOP('',(#47101,#47102,#47103,#47104));
#11175=EDGE_LOOP('',(#47105,#47106,#47107,#47108));
#11176=EDGE_LOOP('',(#47109,#47110,#47111,#47112));
#11177=EDGE_LOOP('',(#47113,#47114,#47115,#47116));
#11178=EDGE_LOOP('',(#47117,#47118,#47119,#47120));
#11179=EDGE_LOOP('',(#47121,#47122,#47123,#47124));
#11180=EDGE_LOOP('',(#47125,#47126,#47127,#47128));
#11181=EDGE_LOOP('',(#47129,#47130,#47131,#47132));
#11182=EDGE_LOOP('',(#47133,#47134,#47135,#47136));
#11183=EDGE_LOOP('',(#47137,#47138,#47139,#47140));
#11184=EDGE_LOOP('',(#47141,#47142,#47143,#47144));
#11185=EDGE_LOOP('',(#47145,#47146,#47147,#47148));
#11186=EDGE_LOOP('',(#47149,#47150,#47151,#47152));
#11187=EDGE_LOOP('',(#47153,#47154,#47155,#47156));
#11188=EDGE_LOOP('',(#47157,#47158,#47159,#47160));
#11189=EDGE_LOOP('',(#47161,#47162,#47163,#47164));
#11190=EDGE_LOOP('',(#47165,#47166,#47167,#47168));
#11191=EDGE_LOOP('',(#47169,#47170,#47171,#47172));
#11192=EDGE_LOOP('',(#47173,#47174,#47175,#47176));
#11193=EDGE_LOOP('',(#47177,#47178,#47179,#47180));
#11194=EDGE_LOOP('',(#47181,#47182,#47183,#47184));
#11195=EDGE_LOOP('',(#47185,#47186,#47187,#47188));
#11196=EDGE_LOOP('',(#47189,#47190,#47191,#47192));
#11197=EDGE_LOOP('',(#47193,#47194,#47195,#47196));
#11198=EDGE_LOOP('',(#47197,#47198,#47199,#47200));
#11199=EDGE_LOOP('',(#47201,#47202,#47203,#47204));
#11200=EDGE_LOOP('',(#47205,#47206,#47207,#47208));
#11201=EDGE_LOOP('',(#47209,#47210,#47211,#47212));
#11202=EDGE_LOOP('',(#47213,#47214,#47215,#47216));
#11203=EDGE_LOOP('',(#47217,#47218,#47219,#47220));
#11204=EDGE_LOOP('',(#47221,#47222,#47223,#47224));
#11205=EDGE_LOOP('',(#47225,#47226,#47227,#47228));
#11206=EDGE_LOOP('',(#47229,#47230,#47231,#47232));
#11207=EDGE_LOOP('',(#47233,#47234,#47235,#47236));
#11208=EDGE_LOOP('',(#47237,#47238,#47239,#47240));
#11209=EDGE_LOOP('',(#47241,#47242,#47243,#47244));
#11210=EDGE_LOOP('',(#47245,#47246,#47247,#47248));
#11211=EDGE_LOOP('',(#47249,#47250,#47251,#47252));
#11212=EDGE_LOOP('',(#47253,#47254,#47255,#47256));
#11213=EDGE_LOOP('',(#47257,#47258,#47259,#47260));
#11214=EDGE_LOOP('',(#47261,#47262,#47263,#47264));
#11215=EDGE_LOOP('',(#47265,#47266,#47267,#47268));
#11216=EDGE_LOOP('',(#47269,#47270,#47271,#47272));
#11217=EDGE_LOOP('',(#47273,#47274,#47275,#47276));
#11218=EDGE_LOOP('',(#47277,#47278,#47279,#47280));
#11219=EDGE_LOOP('',(#47281,#47282,#47283,#47284));
#11220=EDGE_LOOP('',(#47285,#47286,#47287,#47288));
#11221=EDGE_LOOP('',(#47289,#47290,#47291,#47292));
#11222=EDGE_LOOP('',(#47293,#47294,#47295,#47296));
#11223=EDGE_LOOP('',(#47297,#47298,#47299,#47300));
#11224=EDGE_LOOP('',(#47301,#47302,#47303,#47304));
#11225=EDGE_LOOP('',(#47305,#47306,#47307,#47308));
#11226=EDGE_LOOP('',(#47309,#47310,#47311,#47312));
#11227=EDGE_LOOP('',(#47313,#47314,#47315,#47316));
#11228=EDGE_LOOP('',(#47317,#47318,#47319,#47320));
#11229=EDGE_LOOP('',(#47321,#47322,#47323,#47324));
#11230=EDGE_LOOP('',(#47325,#47326,#47327,#47328));
#11231=EDGE_LOOP('',(#47329,#47330,#47331,#47332));
#11232=EDGE_LOOP('',(#47333,#47334,#47335,#47336));
#11233=EDGE_LOOP('',(#47337,#47338,#47339,#47340));
#11234=EDGE_LOOP('',(#47341,#47342,#47343,#47344));
#11235=EDGE_LOOP('',(#47345,#47346,#47347,#47348));
#11236=EDGE_LOOP('',(#47349,#47350,#47351,#47352));
#11237=EDGE_LOOP('',(#47353,#47354,#47355,#47356));
#11238=EDGE_LOOP('',(#47357,#47358,#47359,#47360));
#11239=EDGE_LOOP('',(#47361,#47362,#47363,#47364));
#11240=EDGE_LOOP('',(#47365,#47366,#47367,#47368));
#11241=EDGE_LOOP('',(#47369,#47370,#47371,#47372));
#11242=EDGE_LOOP('',(#47373,#47374,#47375,#47376));
#11243=EDGE_LOOP('',(#47377,#47378,#47379,#47380));
#11244=EDGE_LOOP('',(#47381,#47382,#47383,#47384));
#11245=EDGE_LOOP('',(#47385,#47386,#47387,#47388));
#11246=EDGE_LOOP('',(#47389,#47390,#47391,#47392));
#11247=EDGE_LOOP('',(#47393,#47394,#47395,#47396));
#11248=EDGE_LOOP('',(#47397,#47398,#47399,#47400));
#11249=EDGE_LOOP('',(#47401,#47402,#47403,#47404));
#11250=EDGE_LOOP('',(#47405,#47406,#47407,#47408));
#11251=EDGE_LOOP('',(#47409,#47410,#47411,#47412));
#11252=EDGE_LOOP('',(#47413,#47414,#47415,#47416));
#11253=EDGE_LOOP('',(#47417,#47418,#47419,#47420));
#11254=EDGE_LOOP('',(#47421,#47422,#47423,#47424));
#11255=EDGE_LOOP('',(#47425,#47426,#47427,#47428));
#11256=EDGE_LOOP('',(#47429,#47430,#47431,#47432));
#11257=EDGE_LOOP('',(#47433,#47434,#47435,#47436));
#11258=EDGE_LOOP('',(#47437,#47438,#47439,#47440));
#11259=EDGE_LOOP('',(#47441,#47442,#47443,#47444));
#11260=EDGE_LOOP('',(#47445,#47446,#47447,#47448));
#11261=EDGE_LOOP('',(#47449,#47450,#47451,#47452));
#11262=EDGE_LOOP('',(#47453,#47454,#47455,#47456));
#11263=EDGE_LOOP('',(#47457,#47458,#47459,#47460));
#11264=EDGE_LOOP('',(#47461,#47462,#47463,#47464));
#11265=EDGE_LOOP('',(#47465,#47466,#47467,#47468));
#11266=EDGE_LOOP('',(#47469,#47470,#47471,#47472));
#11267=EDGE_LOOP('',(#47473,#47474,#47475,#47476));
#11268=EDGE_LOOP('',(#47477,#47478,#47479,#47480));
#11269=EDGE_LOOP('',(#47481,#47482,#47483,#47484));
#11270=EDGE_LOOP('',(#47485,#47486,#47487,#47488));
#11271=EDGE_LOOP('',(#47489,#47490,#47491,#47492));
#11272=EDGE_LOOP('',(#47493,#47494,#47495,#47496));
#11273=EDGE_LOOP('',(#47497,#47498,#47499,#47500));
#11274=EDGE_LOOP('',(#47501,#47502,#47503,#47504));
#11275=EDGE_LOOP('',(#47505,#47506,#47507,#47508));
#11276=EDGE_LOOP('',(#47509,#47510,#47511,#47512));
#11277=EDGE_LOOP('',(#47513,#47514,#47515,#47516));
#11278=EDGE_LOOP('',(#47517,#47518,#47519,#47520));
#11279=EDGE_LOOP('',(#47521,#47522,#47523,#47524));
#11280=EDGE_LOOP('',(#47525,#47526,#47527,#47528));
#11281=EDGE_LOOP('',(#47529,#47530,#47531,#47532));
#11282=EDGE_LOOP('',(#47533,#47534,#47535,#47536));
#11283=EDGE_LOOP('',(#47537,#47538,#47539,#47540));
#11284=EDGE_LOOP('',(#47541,#47542,#47543,#47544));
#11285=EDGE_LOOP('',(#47545,#47546,#47547,#47548));
#11286=EDGE_LOOP('',(#47549,#47550,#47551,#47552));
#11287=EDGE_LOOP('',(#47553,#47554,#47555,#47556));
#11288=EDGE_LOOP('',(#47557,#47558,#47559,#47560));
#11289=EDGE_LOOP('',(#47561,#47562,#47563,#47564));
#11290=EDGE_LOOP('',(#47565,#47566,#47567,#47568));
#11291=EDGE_LOOP('',(#47569,#47570,#47571,#47572));
#11292=EDGE_LOOP('',(#47573,#47574,#47575,#47576));
#11293=EDGE_LOOP('',(#47577,#47578,#47579,#47580));
#11294=EDGE_LOOP('',(#47581,#47582,#47583,#47584));
#11295=EDGE_LOOP('',(#47585,#47586,#47587,#47588));
#11296=EDGE_LOOP('',(#47589,#47590,#47591,#47592));
#11297=EDGE_LOOP('',(#47593,#47594,#47595,#47596));
#11298=EDGE_LOOP('',(#47597,#47598,#47599,#47600));
#11299=EDGE_LOOP('',(#47601,#47602,#47603,#47604));
#11300=EDGE_LOOP('',(#47605,#47606,#47607,#47608));
#11301=EDGE_LOOP('',(#47609,#47610,#47611,#47612));
#11302=EDGE_LOOP('',(#47613,#47614,#47615,#47616));
#11303=EDGE_LOOP('',(#47617,#47618,#47619,#47620));
#11304=EDGE_LOOP('',(#47621,#47622,#47623,#47624));
#11305=EDGE_LOOP('',(#47625,#47626,#47627,#47628));
#11306=EDGE_LOOP('',(#47629,#47630,#47631,#47632));
#11307=EDGE_LOOP('',(#47633,#47634,#47635,#47636));
#11308=EDGE_LOOP('',(#47637,#47638,#47639,#47640));
#11309=EDGE_LOOP('',(#47641,#47642,#47643,#47644));
#11310=EDGE_LOOP('',(#47645,#47646,#47647,#47648));
#11311=EDGE_LOOP('',(#47649,#47650,#47651,#47652));
#11312=EDGE_LOOP('',(#47653,#47654,#47655,#47656));
#11313=EDGE_LOOP('',(#47657,#47658,#47659,#47660));
#11314=EDGE_LOOP('',(#47661,#47662,#47663,#47664));
#11315=EDGE_LOOP('',(#47665,#47666,#47667,#47668));
#11316=EDGE_LOOP('',(#47669,#47670,#47671,#47672));
#11317=EDGE_LOOP('',(#47673,#47674,#47675,#47676));
#11318=EDGE_LOOP('',(#47677,#47678,#47679,#47680));
#11319=EDGE_LOOP('',(#47681,#47682,#47683,#47684));
#11320=EDGE_LOOP('',(#47685,#47686,#47687,#47688));
#11321=EDGE_LOOP('',(#47689,#47690,#47691,#47692));
#11322=EDGE_LOOP('',(#47693,#47694,#47695,#47696));
#11323=EDGE_LOOP('',(#47697,#47698,#47699,#47700));
#11324=EDGE_LOOP('',(#47701,#47702,#47703,#47704));
#11325=EDGE_LOOP('',(#47705,#47706,#47707,#47708));
#11326=EDGE_LOOP('',(#47709,#47710,#47711,#47712));
#11327=EDGE_LOOP('',(#47713,#47714,#47715,#47716));
#11328=EDGE_LOOP('',(#47717,#47718,#47719,#47720));
#11329=EDGE_LOOP('',(#47721,#47722,#47723,#47724));
#11330=EDGE_LOOP('',(#47725,#47726,#47727,#47728));
#11331=EDGE_LOOP('',(#47729,#47730,#47731,#47732));
#11332=EDGE_LOOP('',(#47733,#47734,#47735,#47736));
#11333=EDGE_LOOP('',(#47737,#47738,#47739,#47740));
#11334=EDGE_LOOP('',(#47741,#47742,#47743,#47744));
#11335=EDGE_LOOP('',(#47745,#47746,#47747,#47748));
#11336=EDGE_LOOP('',(#47749,#47750,#47751,#47752));
#11337=EDGE_LOOP('',(#47753,#47754,#47755,#47756));
#11338=EDGE_LOOP('',(#47757,#47758,#47759,#47760));
#11339=EDGE_LOOP('',(#47761,#47762,#47763,#47764));
#11340=EDGE_LOOP('',(#47765,#47766,#47767,#47768));
#11341=EDGE_LOOP('',(#47769,#47770,#47771,#47772));
#11342=EDGE_LOOP('',(#47773,#47774,#47775,#47776));
#11343=EDGE_LOOP('',(#47777,#47778,#47779,#47780));
#11344=EDGE_LOOP('',(#47781,#47782,#47783,#47784));
#11345=EDGE_LOOP('',(#47785,#47786,#47787,#47788));
#11346=EDGE_LOOP('',(#47789,#47790,#47791,#47792));
#11347=EDGE_LOOP('',(#47793,#47794,#47795,#47796));
#11348=EDGE_LOOP('',(#47797,#47798,#47799,#47800));
#11349=EDGE_LOOP('',(#47801,#47802,#47803,#47804));
#11350=EDGE_LOOP('',(#47805,#47806,#47807,#47808));
#11351=EDGE_LOOP('',(#47809,#47810,#47811,#47812));
#11352=EDGE_LOOP('',(#47813,#47814,#47815,#47816));
#11353=EDGE_LOOP('',(#47817,#47818,#47819,#47820));
#11354=EDGE_LOOP('',(#47821,#47822,#47823,#47824));
#11355=EDGE_LOOP('',(#47825,#47826,#47827,#47828));
#11356=EDGE_LOOP('',(#47829,#47830,#47831,#47832));
#11357=EDGE_LOOP('',(#47833,#47834,#47835,#47836));
#11358=EDGE_LOOP('',(#47837,#47838,#47839,#47840));
#11359=EDGE_LOOP('',(#47841,#47842,#47843,#47844));
#11360=EDGE_LOOP('',(#47845,#47846,#47847,#47848));
#11361=EDGE_LOOP('',(#47849,#47850,#47851,#47852));
#11362=EDGE_LOOP('',(#47853,#47854,#47855,#47856));
#11363=EDGE_LOOP('',(#47857,#47858,#47859,#47860));
#11364=EDGE_LOOP('',(#47861,#47862,#47863,#47864));
#11365=EDGE_LOOP('',(#47865,#47866,#47867,#47868));
#11366=EDGE_LOOP('',(#47869,#47870,#47871,#47872));
#11367=EDGE_LOOP('',(#47873,#47874,#47875,#47876));
#11368=EDGE_LOOP('',(#47877,#47878,#47879,#47880));
#11369=EDGE_LOOP('',(#47881,#47882,#47883,#47884));
#11370=EDGE_LOOP('',(#47885,#47886,#47887,#47888));
#11371=EDGE_LOOP('',(#47889,#47890,#47891,#47892));
#11372=EDGE_LOOP('',(#47893,#47894,#47895,#47896));
#11373=EDGE_LOOP('',(#47897,#47898,#47899,#47900));
#11374=EDGE_LOOP('',(#47901,#47902,#47903,#47904));
#11375=EDGE_LOOP('',(#47905,#47906,#47907,#47908));
#11376=EDGE_LOOP('',(#47909,#47910,#47911,#47912));
#11377=EDGE_LOOP('',(#47913,#47914,#47915,#47916));
#11378=EDGE_LOOP('',(#47917,#47918,#47919,#47920));
#11379=EDGE_LOOP('',(#47921,#47922,#47923,#47924));
#11380=EDGE_LOOP('',(#47925,#47926,#47927,#47928));
#11381=EDGE_LOOP('',(#47929,#47930,#47931,#47932));
#11382=EDGE_LOOP('',(#47933,#47934,#47935,#47936));
#11383=EDGE_LOOP('',(#47937,#47938,#47939,#47940));
#11384=EDGE_LOOP('',(#47941,#47942,#47943,#47944));
#11385=EDGE_LOOP('',(#47945,#47946,#47947,#47948));
#11386=EDGE_LOOP('',(#47949,#47950,#47951,#47952));
#11387=EDGE_LOOP('',(#47953,#47954,#47955,#47956));
#11388=EDGE_LOOP('',(#47957,#47958,#47959,#47960));
#11389=EDGE_LOOP('',(#47961,#47962,#47963,#47964));
#11390=EDGE_LOOP('',(#47965,#47966,#47967,#47968));
#11391=EDGE_LOOP('',(#47969,#47970,#47971,#47972));
#11392=EDGE_LOOP('',(#47973,#47974,#47975,#47976));
#11393=EDGE_LOOP('',(#47977,#47978,#47979,#47980));
#11394=EDGE_LOOP('',(#47981,#47982,#47983,#47984));
#11395=EDGE_LOOP('',(#47985,#47986,#47987,#47988));
#11396=EDGE_LOOP('',(#47989,#47990,#47991,#47992));
#11397=EDGE_LOOP('',(#47993,#47994,#47995,#47996));
#11398=EDGE_LOOP('',(#47997,#47998,#47999,#48000));
#11399=EDGE_LOOP('',(#48001,#48002,#48003,#48004));
#11400=EDGE_LOOP('',(#48005,#48006,#48007,#48008));
#11401=EDGE_LOOP('',(#48009,#48010,#48011,#48012));
#11402=EDGE_LOOP('',(#48013,#48014,#48015,#48016));
#11403=EDGE_LOOP('',(#48017,#48018,#48019,#48020));
#11404=EDGE_LOOP('',(#48021,#48022,#48023,#48024));
#11405=EDGE_LOOP('',(#48025,#48026,#48027,#48028));
#11406=EDGE_LOOP('',(#48029,#48030,#48031,#48032));
#11407=EDGE_LOOP('',(#48033,#48034,#48035,#48036));
#11408=EDGE_LOOP('',(#48037,#48038,#48039,#48040));
#11409=EDGE_LOOP('',(#48041,#48042,#48043,#48044));
#11410=EDGE_LOOP('',(#48045,#48046,#48047,#48048));
#11411=EDGE_LOOP('',(#48049,#48050,#48051,#48052));
#11412=EDGE_LOOP('',(#48053,#48054,#48055,#48056));
#11413=EDGE_LOOP('',(#48057,#48058,#48059,#48060));
#11414=EDGE_LOOP('',(#48061,#48062,#48063,#48064));
#11415=EDGE_LOOP('',(#48065,#48066,#48067,#48068));
#11416=EDGE_LOOP('',(#48069,#48070,#48071,#48072));
#11417=EDGE_LOOP('',(#48073,#48074,#48075,#48076));
#11418=EDGE_LOOP('',(#48077,#48078,#48079,#48080));
#11419=EDGE_LOOP('',(#48081,#48082,#48083,#48084));
#11420=EDGE_LOOP('',(#48085,#48086,#48087,#48088));
#11421=EDGE_LOOP('',(#48089,#48090,#48091,#48092));
#11422=EDGE_LOOP('',(#48093,#48094,#48095,#48096));
#11423=EDGE_LOOP('',(#48097,#48098,#48099,#48100));
#11424=EDGE_LOOP('',(#48101,#48102,#48103,#48104));
#11425=EDGE_LOOP('',(#48105,#48106,#48107,#48108));
#11426=EDGE_LOOP('',(#48109,#48110,#48111,#48112));
#11427=EDGE_LOOP('',(#48113,#48114,#48115,#48116));
#11428=EDGE_LOOP('',(#48117,#48118,#48119,#48120));
#11429=EDGE_LOOP('',(#48121,#48122,#48123,#48124));
#11430=EDGE_LOOP('',(#48125,#48126,#48127,#48128));
#11431=EDGE_LOOP('',(#48129,#48130,#48131,#48132));
#11432=EDGE_LOOP('',(#48133,#48134,#48135,#48136));
#11433=EDGE_LOOP('',(#48137,#48138,#48139,#48140));
#11434=EDGE_LOOP('',(#48141,#48142,#48143,#48144));
#11435=EDGE_LOOP('',(#48145,#48146,#48147,#48148));
#11436=EDGE_LOOP('',(#48149,#48150,#48151,#48152));
#11437=EDGE_LOOP('',(#48153,#48154,#48155,#48156));
#11438=EDGE_LOOP('',(#48157,#48158,#48159,#48160));
#11439=EDGE_LOOP('',(#48161,#48162,#48163,#48164));
#11440=EDGE_LOOP('',(#48165,#48166,#48167,#48168));
#11441=EDGE_LOOP('',(#48169,#48170,#48171,#48172));
#11442=EDGE_LOOP('',(#48173,#48174,#48175,#48176));
#11443=EDGE_LOOP('',(#48177,#48178,#48179,#48180));
#11444=EDGE_LOOP('',(#48181,#48182,#48183,#48184));
#11445=EDGE_LOOP('',(#48185,#48186,#48187,#48188));
#11446=EDGE_LOOP('',(#48189,#48190,#48191,#48192));
#11447=EDGE_LOOP('',(#48193,#48194,#48195,#48196));
#11448=EDGE_LOOP('',(#48197,#48198,#48199,#48200));
#11449=EDGE_LOOP('',(#48201,#48202,#48203,#48204));
#11450=EDGE_LOOP('',(#48205,#48206,#48207,#48208));
#11451=EDGE_LOOP('',(#48209,#48210,#48211,#48212));
#11452=EDGE_LOOP('',(#48213,#48214,#48215,#48216));
#11453=EDGE_LOOP('',(#48217,#48218,#48219,#48220));
#11454=EDGE_LOOP('',(#48221,#48222,#48223,#48224));
#11455=EDGE_LOOP('',(#48225,#48226,#48227,#48228));
#11456=EDGE_LOOP('',(#48229,#48230,#48231,#48232));
#11457=EDGE_LOOP('',(#48233,#48234,#48235,#48236));
#11458=EDGE_LOOP('',(#48237,#48238,#48239,#48240));
#11459=EDGE_LOOP('',(#48241,#48242,#48243,#48244));
#11460=EDGE_LOOP('',(#48245,#48246,#48247,#48248));
#11461=EDGE_LOOP('',(#48249,#48250,#48251,#48252));
#11462=EDGE_LOOP('',(#48253,#48254,#48255,#48256));
#11463=EDGE_LOOP('',(#48257,#48258,#48259,#48260));
#11464=EDGE_LOOP('',(#48261,#48262,#48263,#48264));
#11465=EDGE_LOOP('',(#48265,#48266,#48267,#48268));
#11466=EDGE_LOOP('',(#48269,#48270,#48271,#48272));
#11467=EDGE_LOOP('',(#48273,#48274,#48275,#48276));
#11468=EDGE_LOOP('',(#48277,#48278,#48279,#48280));
#11469=EDGE_LOOP('',(#48281,#48282,#48283,#48284));
#11470=EDGE_LOOP('',(#48285,#48286,#48287,#48288));
#11471=EDGE_LOOP('',(#48289,#48290,#48291,#48292));
#11472=EDGE_LOOP('',(#48293,#48294,#48295,#48296));
#11473=EDGE_LOOP('',(#48297,#48298,#48299,#48300));
#11474=EDGE_LOOP('',(#48301,#48302,#48303,#48304));
#11475=EDGE_LOOP('',(#48305,#48306,#48307,#48308));
#11476=EDGE_LOOP('',(#48309,#48310,#48311,#48312));
#11477=EDGE_LOOP('',(#48313,#48314,#48315,#48316));
#11478=EDGE_LOOP('',(#48317,#48318,#48319,#48320));
#11479=EDGE_LOOP('',(#48321,#48322,#48323,#48324));
#11480=EDGE_LOOP('',(#48325,#48326,#48327,#48328));
#11481=EDGE_LOOP('',(#48329,#48330,#48331,#48332));
#11482=EDGE_LOOP('',(#48333,#48334,#48335,#48336));
#11483=EDGE_LOOP('',(#48337,#48338,#48339,#48340));
#11484=EDGE_LOOP('',(#48341,#48342,#48343,#48344));
#11485=EDGE_LOOP('',(#48345,#48346,#48347,#48348));
#11486=EDGE_LOOP('',(#48349,#48350,#48351,#48352));
#11487=EDGE_LOOP('',(#48353,#48354,#48355,#48356));
#11488=EDGE_LOOP('',(#48357,#48358,#48359,#48360));
#11489=EDGE_LOOP('',(#48361,#48362,#48363,#48364));
#11490=EDGE_LOOP('',(#48365,#48366,#48367,#48368));
#11491=EDGE_LOOP('',(#48369,#48370,#48371,#48372));
#11492=EDGE_LOOP('',(#48373,#48374,#48375,#48376));
#11493=EDGE_LOOP('',(#48377,#48378,#48379,#48380));
#11494=EDGE_LOOP('',(#48381,#48382,#48383,#48384));
#11495=EDGE_LOOP('',(#48385,#48386,#48387,#48388));
#11496=EDGE_LOOP('',(#48389,#48390,#48391,#48392));
#11497=EDGE_LOOP('',(#48393,#48394,#48395,#48396));
#11498=EDGE_LOOP('',(#48397,#48398,#48399,#48400));
#11499=EDGE_LOOP('',(#48401,#48402,#48403,#48404));
#11500=EDGE_LOOP('',(#48405,#48406,#48407,#48408));
#11501=EDGE_LOOP('',(#48409,#48410,#48411,#48412));
#11502=EDGE_LOOP('',(#48413,#48414,#48415,#48416));
#11503=EDGE_LOOP('',(#48417,#48418,#48419,#48420));
#11504=EDGE_LOOP('',(#48421,#48422,#48423,#48424));
#11505=EDGE_LOOP('',(#48425,#48426,#48427,#48428));
#11506=EDGE_LOOP('',(#48429,#48430,#48431,#48432));
#11507=EDGE_LOOP('',(#48433,#48434,#48435,#48436));
#11508=EDGE_LOOP('',(#48437,#48438,#48439,#48440));
#11509=EDGE_LOOP('',(#48441,#48442,#48443,#48444));
#11510=EDGE_LOOP('',(#48445,#48446,#48447,#48448));
#11511=EDGE_LOOP('',(#48449,#48450,#48451,#48452));
#11512=EDGE_LOOP('',(#48453,#48454,#48455,#48456));
#11513=EDGE_LOOP('',(#48457,#48458,#48459,#48460));
#11514=EDGE_LOOP('',(#48461,#48462,#48463,#48464));
#11515=EDGE_LOOP('',(#48465,#48466,#48467,#48468));
#11516=EDGE_LOOP('',(#48469,#48470,#48471,#48472));
#11517=EDGE_LOOP('',(#48473,#48474,#48475,#48476));
#11518=EDGE_LOOP('',(#48477,#48478,#48479,#48480));
#11519=EDGE_LOOP('',(#48481,#48482,#48483,#48484));
#11520=EDGE_LOOP('',(#48485,#48486,#48487,#48488));
#11521=EDGE_LOOP('',(#48489,#48490,#48491,#48492));
#11522=EDGE_LOOP('',(#48493,#48494,#48495,#48496));
#11523=EDGE_LOOP('',(#48497,#48498,#48499,#48500));
#11524=EDGE_LOOP('',(#48501,#48502,#48503,#48504));
#11525=EDGE_LOOP('',(#48505,#48506,#48507,#48508));
#11526=EDGE_LOOP('',(#48509,#48510,#48511,#48512));
#11527=EDGE_LOOP('',(#48513,#48514,#48515,#48516));
#11528=EDGE_LOOP('',(#48517,#48518,#48519,#48520));
#11529=EDGE_LOOP('',(#48521,#48522,#48523,#48524));
#11530=EDGE_LOOP('',(#48525,#48526,#48527,#48528));
#11531=EDGE_LOOP('',(#48529,#48530,#48531,#48532));
#11532=EDGE_LOOP('',(#48533,#48534,#48535,#48536));
#11533=EDGE_LOOP('',(#48537,#48538,#48539,#48540));
#11534=EDGE_LOOP('',(#48541,#48542,#48543,#48544));
#11535=EDGE_LOOP('',(#48545,#48546,#48547,#48548));
#11536=EDGE_LOOP('',(#48549,#48550,#48551,#48552));
#11537=EDGE_LOOP('',(#48553,#48554,#48555,#48556));
#11538=EDGE_LOOP('',(#48557,#48558,#48559,#48560));
#11539=EDGE_LOOP('',(#48561,#48562,#48563,#48564));
#11540=EDGE_LOOP('',(#48565,#48566,#48567,#48568));
#11541=EDGE_LOOP('',(#48569,#48570,#48571,#48572));
#11542=EDGE_LOOP('',(#48573,#48574,#48575,#48576));
#11543=EDGE_LOOP('',(#48577,#48578,#48579,#48580));
#11544=EDGE_LOOP('',(#48581,#48582,#48583,#48584));
#11545=EDGE_LOOP('',(#48585,#48586,#48587,#48588));
#11546=EDGE_LOOP('',(#48589,#48590,#48591,#48592));
#11547=EDGE_LOOP('',(#48593,#48594,#48595,#48596));
#11548=EDGE_LOOP('',(#48597,#48598,#48599,#48600));
#11549=EDGE_LOOP('',(#48601,#48602,#48603,#48604));
#11550=EDGE_LOOP('',(#48605,#48606,#48607,#48608));
#11551=EDGE_LOOP('',(#48609,#48610,#48611,#48612));
#11552=EDGE_LOOP('',(#48613,#48614,#48615,#48616));
#11553=EDGE_LOOP('',(#48617,#48618,#48619,#48620));
#11554=EDGE_LOOP('',(#48621,#48622,#48623,#48624));
#11555=EDGE_LOOP('',(#48625,#48626,#48627,#48628));
#11556=EDGE_LOOP('',(#48629,#48630,#48631,#48632));
#11557=EDGE_LOOP('',(#48633,#48634,#48635,#48636));
#11558=EDGE_LOOP('',(#48637,#48638,#48639,#48640));
#11559=EDGE_LOOP('',(#48641,#48642,#48643,#48644));
#11560=EDGE_LOOP('',(#48645,#48646,#48647,#48648));
#11561=EDGE_LOOP('',(#48649,#48650,#48651,#48652));
#11562=EDGE_LOOP('',(#48653,#48654,#48655,#48656));
#11563=EDGE_LOOP('',(#48657,#48658,#48659,#48660));
#11564=EDGE_LOOP('',(#48661,#48662,#48663,#48664));
#11565=EDGE_LOOP('',(#48665,#48666,#48667,#48668));
#11566=EDGE_LOOP('',(#48669,#48670,#48671,#48672));
#11567=EDGE_LOOP('',(#48673,#48674,#48675,#48676));
#11568=EDGE_LOOP('',(#48677,#48678,#48679,#48680));
#11569=EDGE_LOOP('',(#48681,#48682,#48683,#48684));
#11570=EDGE_LOOP('',(#48685,#48686,#48687,#48688));
#11571=EDGE_LOOP('',(#48689,#48690,#48691,#48692));
#11572=EDGE_LOOP('',(#48693,#48694,#48695,#48696));
#11573=EDGE_LOOP('',(#48697,#48698,#48699,#48700));
#11574=EDGE_LOOP('',(#48701,#48702,#48703,#48704));
#11575=EDGE_LOOP('',(#48705,#48706,#48707,#48708));
#11576=EDGE_LOOP('',(#48709,#48710,#48711,#48712));
#11577=EDGE_LOOP('',(#48713,#48714,#48715,#48716));
#11578=EDGE_LOOP('',(#48717,#48718,#48719,#48720));
#11579=EDGE_LOOP('',(#48721,#48722,#48723,#48724));
#11580=EDGE_LOOP('',(#48725,#48726,#48727,#48728));
#11581=EDGE_LOOP('',(#48729,#48730,#48731,#48732));
#11582=EDGE_LOOP('',(#48733,#48734,#48735,#48736));
#11583=EDGE_LOOP('',(#48737,#48738,#48739,#48740));
#11584=EDGE_LOOP('',(#48741,#48742,#48743,#48744));
#11585=EDGE_LOOP('',(#48745,#48746,#48747,#48748));
#11586=EDGE_LOOP('',(#48749,#48750,#48751,#48752));
#11587=EDGE_LOOP('',(#48753,#48754,#48755,#48756));
#11588=EDGE_LOOP('',(#48757,#48758,#48759,#48760));
#11589=EDGE_LOOP('',(#48761,#48762,#48763,#48764));
#11590=EDGE_LOOP('',(#48765,#48766,#48767,#48768));
#11591=EDGE_LOOP('',(#48769,#48770,#48771,#48772));
#11592=EDGE_LOOP('',(#48773,#48774,#48775,#48776));
#11593=EDGE_LOOP('',(#48777,#48778,#48779,#48780));
#11594=EDGE_LOOP('',(#48781,#48782,#48783,#48784));
#11595=EDGE_LOOP('',(#48785,#48786,#48787,#48788));
#11596=EDGE_LOOP('',(#48789,#48790,#48791,#48792));
#11597=EDGE_LOOP('',(#48793,#48794,#48795,#48796));
#11598=EDGE_LOOP('',(#48797,#48798,#48799,#48800));
#11599=EDGE_LOOP('',(#48801,#48802,#48803,#48804));
#11600=EDGE_LOOP('',(#48805,#48806,#48807,#48808));
#11601=EDGE_LOOP('',(#48809,#48810,#48811,#48812));
#11602=EDGE_LOOP('',(#48813,#48814,#48815,#48816));
#11603=EDGE_LOOP('',(#48817,#48818,#48819,#48820));
#11604=EDGE_LOOP('',(#48821,#48822,#48823,#48824));
#11605=EDGE_LOOP('',(#48825,#48826,#48827,#48828));
#11606=EDGE_LOOP('',(#48829,#48830,#48831,#48832));
#11607=EDGE_LOOP('',(#48833,#48834,#48835,#48836));
#11608=EDGE_LOOP('',(#48837,#48838,#48839,#48840));
#11609=EDGE_LOOP('',(#48841,#48842,#48843,#48844));
#11610=EDGE_LOOP('',(#48845,#48846,#48847,#48848));
#11611=EDGE_LOOP('',(#48849,#48850,#48851,#48852));
#11612=EDGE_LOOP('',(#48853,#48854,#48855,#48856));
#11613=EDGE_LOOP('',(#48857,#48858,#48859,#48860));
#11614=EDGE_LOOP('',(#48861,#48862,#48863,#48864));
#11615=EDGE_LOOP('',(#48865,#48866,#48867,#48868));
#11616=EDGE_LOOP('',(#48869,#48870,#48871,#48872));
#11617=EDGE_LOOP('',(#48873,#48874,#48875,#48876));
#11618=EDGE_LOOP('',(#48877,#48878,#48879,#48880));
#11619=EDGE_LOOP('',(#48881,#48882,#48883,#48884));
#11620=EDGE_LOOP('',(#48885,#48886,#48887,#48888));
#11621=EDGE_LOOP('',(#48889,#48890,#48891,#48892));
#11622=EDGE_LOOP('',(#48893,#48894,#48895,#48896));
#11623=EDGE_LOOP('',(#48897,#48898,#48899,#48900));
#11624=EDGE_LOOP('',(#48901,#48902,#48903,#48904));
#11625=EDGE_LOOP('',(#48905,#48906,#48907,#48908));
#11626=EDGE_LOOP('',(#48909,#48910,#48911,#48912));
#11627=EDGE_LOOP('',(#48913,#48914,#48915,#48916));
#11628=EDGE_LOOP('',(#48917,#48918,#48919,#48920));
#11629=EDGE_LOOP('',(#48921,#48922,#48923,#48924));
#11630=EDGE_LOOP('',(#48925,#48926,#48927,#48928));
#11631=EDGE_LOOP('',(#48929,#48930,#48931,#48932));
#11632=EDGE_LOOP('',(#48933,#48934,#48935,#48936));
#11633=EDGE_LOOP('',(#48937,#48938,#48939,#48940));
#11634=EDGE_LOOP('',(#48941,#48942,#48943,#48944));
#11635=EDGE_LOOP('',(#48945,#48946,#48947,#48948));
#11636=EDGE_LOOP('',(#48949,#48950,#48951,#48952));
#11637=EDGE_LOOP('',(#48953,#48954,#48955,#48956));
#11638=EDGE_LOOP('',(#48957,#48958,#48959,#48960));
#11639=EDGE_LOOP('',(#48961,#48962,#48963,#48964));
#11640=EDGE_LOOP('',(#48965,#48966,#48967,#48968));
#11641=EDGE_LOOP('',(#48969,#48970,#48971,#48972));
#11642=EDGE_LOOP('',(#48973,#48974,#48975,#48976));
#11643=EDGE_LOOP('',(#48977,#48978,#48979,#48980));
#11644=EDGE_LOOP('',(#48981,#48982,#48983,#48984));
#11645=EDGE_LOOP('',(#48985,#48986,#48987,#48988));
#11646=EDGE_LOOP('',(#48989,#48990,#48991,#48992));
#11647=EDGE_LOOP('',(#48993,#48994,#48995,#48996));
#11648=EDGE_LOOP('',(#48997,#48998,#48999,#49000));
#11649=EDGE_LOOP('',(#49001,#49002,#49003,#49004));
#11650=EDGE_LOOP('',(#49005,#49006,#49007,#49008));
#11651=EDGE_LOOP('',(#49009,#49010,#49011,#49012));
#11652=EDGE_LOOP('',(#49013,#49014,#49015,#49016));
#11653=EDGE_LOOP('',(#49017,#49018,#49019,#49020));
#11654=EDGE_LOOP('',(#49021,#49022,#49023,#49024));
#11655=EDGE_LOOP('',(#49025,#49026,#49027,#49028));
#11656=EDGE_LOOP('',(#49029,#49030,#49031,#49032));
#11657=EDGE_LOOP('',(#49033,#49034,#49035,#49036));
#11658=EDGE_LOOP('',(#49037,#49038,#49039,#49040));
#11659=EDGE_LOOP('',(#49041,#49042,#49043,#49044));
#11660=EDGE_LOOP('',(#49045,#49046,#49047,#49048));
#11661=EDGE_LOOP('',(#49049,#49050,#49051,#49052));
#11662=EDGE_LOOP('',(#49053,#49054,#49055,#49056));
#11663=EDGE_LOOP('',(#49057,#49058,#49059,#49060));
#11664=EDGE_LOOP('',(#49061,#49062,#49063,#49064));
#11665=EDGE_LOOP('',(#49065,#49066,#49067,#49068));
#11666=EDGE_LOOP('',(#49069,#49070,#49071,#49072));
#11667=EDGE_LOOP('',(#49073,#49074,#49075,#49076));
#11668=EDGE_LOOP('',(#49077,#49078,#49079,#49080));
#11669=EDGE_LOOP('',(#49081,#49082,#49083,#49084));
#11670=EDGE_LOOP('',(#49085,#49086,#49087,#49088));
#11671=EDGE_LOOP('',(#49089,#49090,#49091,#49092));
#11672=EDGE_LOOP('',(#49093,#49094,#49095,#49096));
#11673=EDGE_LOOP('',(#49097,#49098,#49099,#49100));
#11674=EDGE_LOOP('',(#49101,#49102,#49103,#49104));
#11675=EDGE_LOOP('',(#49105,#49106,#49107,#49108));
#11676=EDGE_LOOP('',(#49109,#49110,#49111,#49112));
#11677=EDGE_LOOP('',(#49113,#49114,#49115,#49116));
#11678=EDGE_LOOP('',(#49117,#49118,#49119,#49120));
#11679=EDGE_LOOP('',(#49121,#49122,#49123,#49124));
#11680=EDGE_LOOP('',(#49125,#49126,#49127,#49128));
#11681=EDGE_LOOP('',(#49129,#49130,#49131,#49132));
#11682=EDGE_LOOP('',(#49133,#49134,#49135,#49136));
#11683=EDGE_LOOP('',(#49137,#49138,#49139,#49140));
#11684=EDGE_LOOP('',(#49141,#49142,#49143,#49144));
#11685=EDGE_LOOP('',(#49145,#49146,#49147,#49148));
#11686=EDGE_LOOP('',(#49149,#49150,#49151,#49152));
#11687=EDGE_LOOP('',(#49153,#49154,#49155,#49156));
#11688=EDGE_LOOP('',(#49157,#49158,#49159,#49160));
#11689=EDGE_LOOP('',(#49161,#49162,#49163,#49164));
#11690=EDGE_LOOP('',(#49165,#49166,#49167,#49168));
#11691=EDGE_LOOP('',(#49169,#49170,#49171,#49172));
#11692=EDGE_LOOP('',(#49173,#49174,#49175,#49176));
#11693=EDGE_LOOP('',(#49177,#49178,#49179,#49180));
#11694=EDGE_LOOP('',(#49181,#49182,#49183,#49184));
#11695=EDGE_LOOP('',(#49185,#49186,#49187,#49188));
#11696=EDGE_LOOP('',(#49189,#49190,#49191,#49192));
#11697=EDGE_LOOP('',(#49193,#49194,#49195,#49196));
#11698=EDGE_LOOP('',(#49197,#49198,#49199,#49200));
#11699=EDGE_LOOP('',(#49201,#49202,#49203,#49204));
#11700=EDGE_LOOP('',(#49205,#49206,#49207,#49208));
#11701=EDGE_LOOP('',(#49209,#49210,#49211,#49212));
#11702=EDGE_LOOP('',(#49213,#49214,#49215,#49216));
#11703=EDGE_LOOP('',(#49217,#49218,#49219,#49220));
#11704=EDGE_LOOP('',(#49221,#49222,#49223,#49224));
#11705=EDGE_LOOP('',(#49225,#49226,#49227,#49228));
#11706=EDGE_LOOP('',(#49229,#49230,#49231,#49232));
#11707=EDGE_LOOP('',(#49233,#49234,#49235,#49236));
#11708=EDGE_LOOP('',(#49237,#49238,#49239,#49240));
#11709=EDGE_LOOP('',(#49241,#49242,#49243,#49244));
#11710=EDGE_LOOP('',(#49245,#49246,#49247,#49248));
#11711=EDGE_LOOP('',(#49249,#49250,#49251,#49252));
#11712=EDGE_LOOP('',(#49253,#49254,#49255,#49256));
#11713=EDGE_LOOP('',(#49257,#49258,#49259,#49260));
#11714=EDGE_LOOP('',(#49261,#49262,#49263,#49264));
#11715=EDGE_LOOP('',(#49265,#49266,#49267,#49268));
#11716=EDGE_LOOP('',(#49269,#49270,#49271,#49272));
#11717=EDGE_LOOP('',(#49273,#49274,#49275,#49276));
#11718=EDGE_LOOP('',(#49277,#49278,#49279,#49280));
#11719=EDGE_LOOP('',(#49281,#49282,#49283,#49284));
#11720=EDGE_LOOP('',(#49285,#49286,#49287,#49288));
#11721=EDGE_LOOP('',(#49289,#49290,#49291,#49292));
#11722=EDGE_LOOP('',(#49293,#49294,#49295,#49296));
#11723=EDGE_LOOP('',(#49297,#49298,#49299,#49300));
#11724=EDGE_LOOP('',(#49301,#49302,#49303,#49304));
#11725=EDGE_LOOP('',(#49305,#49306,#49307,#49308));
#11726=EDGE_LOOP('',(#49309,#49310,#49311,#49312));
#11727=EDGE_LOOP('',(#49313,#49314,#49315,#49316));
#11728=EDGE_LOOP('',(#49317,#49318,#49319,#49320));
#11729=EDGE_LOOP('',(#49321,#49322,#49323,#49324));
#11730=EDGE_LOOP('',(#49325,#49326,#49327,#49328));
#11731=EDGE_LOOP('',(#49329,#49330,#49331,#49332));
#11732=EDGE_LOOP('',(#49333,#49334,#49335,#49336));
#11733=EDGE_LOOP('',(#49337,#49338,#49339,#49340));
#11734=EDGE_LOOP('',(#49341,#49342,#49343,#49344));
#11735=EDGE_LOOP('',(#49345,#49346,#49347,#49348));
#11736=EDGE_LOOP('',(#49349,#49350,#49351,#49352));
#11737=EDGE_LOOP('',(#49353,#49354,#49355,#49356));
#11738=EDGE_LOOP('',(#49357,#49358,#49359,#49360));
#11739=EDGE_LOOP('',(#49361,#49362,#49363,#49364));
#11740=EDGE_LOOP('',(#49365,#49366,#49367,#49368));
#11741=EDGE_LOOP('',(#49369,#49370,#49371,#49372));
#11742=EDGE_LOOP('',(#49373,#49374,#49375,#49376));
#11743=EDGE_LOOP('',(#49377,#49378,#49379,#49380));
#11744=EDGE_LOOP('',(#49381,#49382,#49383,#49384));
#11745=EDGE_LOOP('',(#49385,#49386,#49387,#49388));
#11746=EDGE_LOOP('',(#49389,#49390,#49391,#49392));
#11747=EDGE_LOOP('',(#49393,#49394,#49395,#49396));
#11748=EDGE_LOOP('',(#49397,#49398,#49399,#49400));
#11749=EDGE_LOOP('',(#49401,#49402,#49403,#49404));
#11750=EDGE_LOOP('',(#49405,#49406,#49407,#49408));
#11751=EDGE_LOOP('',(#49409,#49410,#49411,#49412));
#11752=EDGE_LOOP('',(#49413,#49414,#49415,#49416));
#11753=EDGE_LOOP('',(#49417,#49418,#49419,#49420));
#11754=EDGE_LOOP('',(#49421,#49422,#49423,#49424));
#11755=EDGE_LOOP('',(#49425,#49426,#49427,#49428));
#11756=EDGE_LOOP('',(#49429,#49430,#49431,#49432));
#11757=EDGE_LOOP('',(#49433,#49434,#49435,#49436));
#11758=EDGE_LOOP('',(#49437,#49438,#49439,#49440));
#11759=EDGE_LOOP('',(#49441,#49442,#49443,#49444));
#11760=EDGE_LOOP('',(#49445,#49446,#49447,#49448));
#11761=EDGE_LOOP('',(#49449,#49450,#49451,#49452));
#11762=EDGE_LOOP('',(#49453,#49454,#49455,#49456));
#11763=EDGE_LOOP('',(#49457,#49458,#49459,#49460));
#11764=EDGE_LOOP('',(#49461,#49462,#49463,#49464));
#11765=EDGE_LOOP('',(#49465,#49466,#49467,#49468));
#11766=EDGE_LOOP('',(#49469,#49470,#49471,#49472));
#11767=EDGE_LOOP('',(#49473,#49474,#49475,#49476));
#11768=EDGE_LOOP('',(#49477,#49478,#49479,#49480));
#11769=EDGE_LOOP('',(#49481,#49482,#49483,#49484));
#11770=EDGE_LOOP('',(#49485,#49486,#49487,#49488));
#11771=EDGE_LOOP('',(#49489,#49490,#49491,#49492));
#11772=EDGE_LOOP('',(#49493,#49494,#49495,#49496));
#11773=EDGE_LOOP('',(#49497,#49498,#49499,#49500));
#11774=EDGE_LOOP('',(#49501,#49502,#49503,#49504));
#11775=EDGE_LOOP('',(#49505,#49506,#49507,#49508));
#11776=EDGE_LOOP('',(#49509,#49510,#49511,#49512));
#11777=EDGE_LOOP('',(#49513,#49514,#49515,#49516));
#11778=EDGE_LOOP('',(#49517,#49518,#49519,#49520));
#11779=EDGE_LOOP('',(#49521,#49522,#49523,#49524));
#11780=EDGE_LOOP('',(#49525,#49526,#49527,#49528));
#11781=EDGE_LOOP('',(#49529,#49530,#49531,#49532));
#11782=EDGE_LOOP('',(#49533,#49534,#49535,#49536));
#11783=EDGE_LOOP('',(#49537,#49538,#49539,#49540));
#11784=EDGE_LOOP('',(#49541,#49542,#49543,#49544));
#11785=EDGE_LOOP('',(#49545,#49546,#49547,#49548));
#11786=EDGE_LOOP('',(#49549,#49550,#49551,#49552));
#11787=EDGE_LOOP('',(#49553,#49554,#49555,#49556));
#11788=EDGE_LOOP('',(#49557,#49558,#49559,#49560));
#11789=EDGE_LOOP('',(#49561,#49562,#49563,#49564));
#11790=EDGE_LOOP('',(#49565,#49566,#49567,#49568));
#11791=EDGE_LOOP('',(#49569,#49570,#49571,#49572));
#11792=EDGE_LOOP('',(#49573,#49574,#49575,#49576));
#11793=EDGE_LOOP('',(#49577,#49578,#49579,#49580));
#11794=EDGE_LOOP('',(#49581,#49582,#49583,#49584));
#11795=EDGE_LOOP('',(#49585,#49586,#49587,#49588));
#11796=EDGE_LOOP('',(#49589,#49590,#49591,#49592));
#11797=EDGE_LOOP('',(#49593,#49594,#49595,#49596));
#11798=EDGE_LOOP('',(#49597,#49598,#49599,#49600));
#11799=EDGE_LOOP('',(#49601,#49602,#49603,#49604));
#11800=EDGE_LOOP('',(#49605,#49606,#49607,#49608));
#11801=EDGE_LOOP('',(#49609,#49610,#49611,#49612));
#11802=EDGE_LOOP('',(#49613,#49614,#49615,#49616));
#11803=EDGE_LOOP('',(#49617,#49618,#49619,#49620));
#11804=EDGE_LOOP('',(#49621,#49622,#49623,#49624));
#11805=EDGE_LOOP('',(#49625,#49626,#49627,#49628));
#11806=EDGE_LOOP('',(#49629,#49630,#49631,#49632));
#11807=EDGE_LOOP('',(#49633,#49634,#49635,#49636));
#11808=EDGE_LOOP('',(#49637,#49638,#49639,#49640));
#11809=EDGE_LOOP('',(#49641,#49642,#49643,#49644));
#11810=EDGE_LOOP('',(#49645,#49646,#49647,#49648));
#11811=EDGE_LOOP('',(#49649,#49650,#49651,#49652));
#11812=EDGE_LOOP('',(#49653,#49654,#49655,#49656));
#11813=EDGE_LOOP('',(#49657,#49658,#49659,#49660));
#11814=EDGE_LOOP('',(#49661,#49662,#49663,#49664));
#11815=EDGE_LOOP('',(#49665,#49666,#49667,#49668));
#11816=EDGE_LOOP('',(#49669,#49670,#49671,#49672));
#11817=EDGE_LOOP('',(#49673,#49674,#49675,#49676));
#11818=EDGE_LOOP('',(#49677,#49678,#49679,#49680));
#11819=EDGE_LOOP('',(#49681,#49682,#49683,#49684));
#11820=EDGE_LOOP('',(#49685,#49686,#49687,#49688));
#11821=EDGE_LOOP('',(#49689,#49690,#49691,#49692));
#11822=EDGE_LOOP('',(#49693,#49694,#49695,#49696));
#11823=EDGE_LOOP('',(#49697,#49698,#49699,#49700));
#11824=EDGE_LOOP('',(#49701,#49702,#49703,#49704));
#11825=EDGE_LOOP('',(#49705,#49706,#49707,#49708));
#11826=EDGE_LOOP('',(#49709,#49710,#49711,#49712));
#11827=EDGE_LOOP('',(#49713,#49714,#49715,#49716));
#11828=EDGE_LOOP('',(#49717,#49718,#49719,#49720));
#11829=EDGE_LOOP('',(#49721,#49722,#49723,#49724));
#11830=EDGE_LOOP('',(#49725,#49726,#49727,#49728));
#11831=EDGE_LOOP('',(#49729,#49730,#49731,#49732));
#11832=EDGE_LOOP('',(#49733,#49734,#49735,#49736));
#11833=EDGE_LOOP('',(#49737,#49738,#49739,#49740));
#11834=EDGE_LOOP('',(#49741,#49742,#49743,#49744));
#11835=EDGE_LOOP('',(#49745,#49746,#49747,#49748));
#11836=EDGE_LOOP('',(#49749,#49750,#49751,#49752));
#11837=EDGE_LOOP('',(#49753,#49754,#49755,#49756));
#11838=EDGE_LOOP('',(#49757,#49758,#49759,#49760));
#11839=EDGE_LOOP('',(#49761,#49762,#49763,#49764));
#11840=EDGE_LOOP('',(#49765,#49766,#49767,#49768));
#11841=EDGE_LOOP('',(#49769,#49770,#49771,#49772));
#11842=EDGE_LOOP('',(#49773,#49774,#49775,#49776));
#11843=EDGE_LOOP('',(#49777,#49778,#49779,#49780));
#11844=EDGE_LOOP('',(#49781,#49782,#49783,#49784));
#11845=EDGE_LOOP('',(#49785,#49786,#49787,#49788));
#11846=EDGE_LOOP('',(#49789,#49790,#49791,#49792));
#11847=EDGE_LOOP('',(#49793,#49794,#49795,#49796));
#11848=EDGE_LOOP('',(#49797,#49798,#49799,#49800));
#11849=EDGE_LOOP('',(#49801,#49802,#49803,#49804));
#11850=EDGE_LOOP('',(#49805,#49806,#49807,#49808));
#11851=EDGE_LOOP('',(#49809,#49810,#49811,#49812));
#11852=EDGE_LOOP('',(#49813,#49814,#49815,#49816));
#11853=EDGE_LOOP('',(#49817,#49818,#49819,#49820));
#11854=EDGE_LOOP('',(#49821,#49822,#49823,#49824));
#11855=EDGE_LOOP('',(#49825,#49826,#49827,#49828));
#11856=EDGE_LOOP('',(#49829,#49830,#49831,#49832));
#11857=EDGE_LOOP('',(#49833,#49834,#49835,#49836));
#11858=EDGE_LOOP('',(#49837,#49838,#49839,#49840));
#11859=EDGE_LOOP('',(#49841,#49842,#49843,#49844));
#11860=EDGE_LOOP('',(#49845,#49846,#49847,#49848));
#11861=EDGE_LOOP('',(#49849,#49850,#49851,#49852));
#11862=EDGE_LOOP('',(#49853,#49854,#49855,#49856));
#11863=EDGE_LOOP('',(#49857,#49858,#49859,#49860));
#11864=EDGE_LOOP('',(#49861,#49862,#49863,#49864));
#11865=EDGE_LOOP('',(#49865,#49866,#49867,#49868));
#11866=EDGE_LOOP('',(#49869,#49870,#49871,#49872));
#11867=EDGE_LOOP('',(#49873,#49874,#49875,#49876));
#11868=EDGE_LOOP('',(#49877,#49878,#49879,#49880));
#11869=EDGE_LOOP('',(#49881,#49882,#49883,#49884));
#11870=EDGE_LOOP('',(#49885,#49886,#49887,#49888));
#11871=EDGE_LOOP('',(#49889,#49890,#49891,#49892));
#11872=EDGE_LOOP('',(#49893,#49894,#49895,#49896));
#11873=EDGE_LOOP('',(#49897,#49898,#49899,#49900));
#11874=EDGE_LOOP('',(#49901,#49902,#49903,#49904));
#11875=EDGE_LOOP('',(#49905,#49906,#49907,#49908));
#11876=EDGE_LOOP('',(#49909,#49910,#49911,#49912));
#11877=EDGE_LOOP('',(#49913,#49914,#49915,#49916));
#11878=EDGE_LOOP('',(#49917,#49918,#49919,#49920));
#11879=EDGE_LOOP('',(#49921,#49922,#49923,#49924));
#11880=EDGE_LOOP('',(#49925,#49926,#49927,#49928));
#11881=EDGE_LOOP('',(#49929,#49930,#49931,#49932));
#11882=EDGE_LOOP('',(#49933,#49934,#49935,#49936));
#11883=EDGE_LOOP('',(#49937,#49938,#49939,#49940));
#11884=EDGE_LOOP('',(#49941,#49942,#49943,#49944));
#11885=EDGE_LOOP('',(#49945,#49946,#49947,#49948));
#11886=EDGE_LOOP('',(#49949,#49950,#49951,#49952));
#11887=EDGE_LOOP('',(#49953,#49954,#49955,#49956));
#11888=EDGE_LOOP('',(#49957,#49958,#49959,#49960));
#11889=EDGE_LOOP('',(#49961,#49962,#49963,#49964));
#11890=EDGE_LOOP('',(#49965,#49966,#49967,#49968));
#11891=EDGE_LOOP('',(#49969,#49970,#49971,#49972));
#11892=EDGE_LOOP('',(#49973,#49974,#49975,#49976));
#11893=EDGE_LOOP('',(#49977,#49978,#49979,#49980));
#11894=EDGE_LOOP('',(#49981,#49982,#49983,#49984));
#11895=EDGE_LOOP('',(#49985,#49986,#49987,#49988));
#11896=EDGE_LOOP('',(#49989,#49990,#49991,#49992));
#11897=EDGE_LOOP('',(#49993,#49994,#49995,#49996));
#11898=EDGE_LOOP('',(#49997,#49998,#49999,#50000));
#11899=EDGE_LOOP('',(#50001,#50002,#50003,#50004));
#11900=EDGE_LOOP('',(#50005,#50006,#50007,#50008));
#11901=EDGE_LOOP('',(#50009,#50010,#50011,#50012));
#11902=EDGE_LOOP('',(#50013,#50014,#50015,#50016));
#11903=EDGE_LOOP('',(#50017,#50018,#50019,#50020));
#11904=EDGE_LOOP('',(#50021,#50022,#50023,#50024));
#11905=EDGE_LOOP('',(#50025,#50026,#50027,#50028));
#11906=EDGE_LOOP('',(#50029,#50030,#50031,#50032));
#11907=EDGE_LOOP('',(#50033,#50034,#50035,#50036));
#11908=EDGE_LOOP('',(#50037,#50038,#50039,#50040));
#11909=EDGE_LOOP('',(#50041,#50042,#50043,#50044));
#11910=EDGE_LOOP('',(#50045,#50046,#50047,#50048));
#11911=EDGE_LOOP('',(#50049,#50050,#50051,#50052));
#11912=EDGE_LOOP('',(#50053,#50054,#50055,#50056));
#11913=EDGE_LOOP('',(#50057,#50058,#50059,#50060));
#11914=EDGE_LOOP('',(#50061,#50062,#50063,#50064));
#11915=EDGE_LOOP('',(#50065,#50066,#50067,#50068));
#11916=EDGE_LOOP('',(#50069,#50070,#50071,#50072));
#11917=EDGE_LOOP('',(#50073,#50074,#50075,#50076));
#11918=EDGE_LOOP('',(#50077,#50078,#50079,#50080));
#11919=EDGE_LOOP('',(#50081,#50082,#50083,#50084));
#11920=EDGE_LOOP('',(#50085,#50086,#50087,#50088));
#11921=EDGE_LOOP('',(#50089,#50090,#50091,#50092));
#11922=EDGE_LOOP('',(#50093,#50094,#50095,#50096));
#11923=EDGE_LOOP('',(#50097,#50098,#50099,#50100));
#11924=EDGE_LOOP('',(#50101,#50102,#50103,#50104));
#11925=EDGE_LOOP('',(#50105,#50106,#50107,#50108));
#11926=EDGE_LOOP('',(#50109,#50110,#50111,#50112));
#11927=EDGE_LOOP('',(#50113,#50114,#50115,#50116));
#11928=EDGE_LOOP('',(#50117,#50118,#50119,#50120));
#11929=EDGE_LOOP('',(#50121,#50122,#50123,#50124));
#11930=EDGE_LOOP('',(#50125,#50126,#50127,#50128));
#11931=EDGE_LOOP('',(#50129,#50130,#50131,#50132));
#11932=EDGE_LOOP('',(#50133,#50134,#50135,#50136));
#11933=EDGE_LOOP('',(#50137,#50138,#50139,#50140));
#11934=EDGE_LOOP('',(#50141,#50142,#50143,#50144));
#11935=EDGE_LOOP('',(#50145,#50146,#50147,#50148));
#11936=EDGE_LOOP('',(#50149,#50150,#50151,#50152));
#11937=EDGE_LOOP('',(#50153,#50154,#50155,#50156));
#11938=EDGE_LOOP('',(#50157,#50158,#50159,#50160));
#11939=EDGE_LOOP('',(#50161,#50162,#50163,#50164));
#11940=EDGE_LOOP('',(#50165,#50166,#50167,#50168));
#11941=EDGE_LOOP('',(#50169,#50170,#50171,#50172));
#11942=EDGE_LOOP('',(#50173,#50174,#50175,#50176));
#11943=EDGE_LOOP('',(#50177,#50178,#50179,#50180));
#11944=EDGE_LOOP('',(#50181,#50182,#50183,#50184));
#11945=EDGE_LOOP('',(#50185,#50186,#50187,#50188));
#11946=EDGE_LOOP('',(#50189,#50190,#50191,#50192));
#11947=EDGE_LOOP('',(#50193,#50194,#50195,#50196));
#11948=EDGE_LOOP('',(#50197,#50198,#50199,#50200));
#11949=EDGE_LOOP('',(#50201,#50202,#50203,#50204));
#11950=EDGE_LOOP('',(#50205,#50206,#50207,#50208));
#11951=EDGE_LOOP('',(#50209,#50210,#50211,#50212));
#11952=EDGE_LOOP('',(#50213,#50214,#50215,#50216));
#11953=EDGE_LOOP('',(#50217,#50218,#50219,#50220));
#11954=EDGE_LOOP('',(#50221,#50222,#50223,#50224));
#11955=EDGE_LOOP('',(#50225,#50226,#50227,#50228));
#11956=EDGE_LOOP('',(#50229,#50230,#50231,#50232));
#11957=EDGE_LOOP('',(#50233,#50234,#50235,#50236));
#11958=EDGE_LOOP('',(#50237,#50238,#50239,#50240));
#11959=EDGE_LOOP('',(#50241,#50242,#50243,#50244));
#11960=EDGE_LOOP('',(#50245,#50246,#50247,#50248));
#11961=EDGE_LOOP('',(#50249,#50250,#50251,#50252));
#11962=EDGE_LOOP('',(#50253,#50254,#50255,#50256));
#11963=EDGE_LOOP('',(#50257,#50258,#50259,#50260));
#11964=EDGE_LOOP('',(#50261,#50262,#50263,#50264));
#11965=EDGE_LOOP('',(#50265,#50266,#50267,#50268));
#11966=EDGE_LOOP('',(#50269,#50270,#50271,#50272));
#11967=EDGE_LOOP('',(#50273,#50274,#50275,#50276));
#11968=EDGE_LOOP('',(#50277,#50278,#50279,#50280));
#11969=EDGE_LOOP('',(#50281,#50282,#50283,#50284));
#11970=EDGE_LOOP('',(#50285,#50286,#50287,#50288));
#11971=EDGE_LOOP('',(#50289,#50290,#50291,#50292));
#11972=EDGE_LOOP('',(#50293,#50294,#50295,#50296));
#11973=EDGE_LOOP('',(#50297,#50298,#50299,#50300));
#11974=EDGE_LOOP('',(#50301,#50302,#50303,#50304));
#11975=EDGE_LOOP('',(#50305,#50306,#50307,#50308));
#11976=EDGE_LOOP('',(#50309,#50310,#50311,#50312));
#11977=EDGE_LOOP('',(#50313,#50314,#50315,#50316));
#11978=EDGE_LOOP('',(#50317,#50318,#50319,#50320));
#11979=EDGE_LOOP('',(#50321,#50322,#50323,#50324));
#11980=EDGE_LOOP('',(#50325,#50326,#50327,#50328));
#11981=EDGE_LOOP('',(#50329,#50330,#50331,#50332));
#11982=EDGE_LOOP('',(#50333,#50334,#50335,#50336));
#11983=EDGE_LOOP('',(#50337,#50338,#50339,#50340));
#11984=EDGE_LOOP('',(#50341,#50342,#50343,#50344));
#11985=EDGE_LOOP('',(#50345,#50346,#50347,#50348));
#11986=EDGE_LOOP('',(#50349,#50350,#50351,#50352));
#11987=EDGE_LOOP('',(#50353,#50354,#50355,#50356));
#11988=EDGE_LOOP('',(#50357,#50358,#50359,#50360));
#11989=EDGE_LOOP('',(#50361,#50362,#50363,#50364));
#11990=EDGE_LOOP('',(#50365,#50366,#50367,#50368));
#11991=EDGE_LOOP('',(#50369,#50370,#50371,#50372));
#11992=EDGE_LOOP('',(#50373,#50374,#50375,#50376));
#11993=EDGE_LOOP('',(#50377,#50378,#50379,#50380));
#11994=EDGE_LOOP('',(#50381,#50382,#50383,#50384));
#11995=EDGE_LOOP('',(#50385,#50386,#50387,#50388));
#11996=EDGE_LOOP('',(#50389,#50390,#50391,#50392));
#11997=EDGE_LOOP('',(#50393,#50394,#50395,#50396));
#11998=EDGE_LOOP('',(#50397,#50398,#50399,#50400));
#11999=EDGE_LOOP('',(#50401,#50402,#50403,#50404));
#12000=EDGE_LOOP('',(#50405,#50406,#50407,#50408));
#12001=EDGE_LOOP('',(#50409,#50410,#50411,#50412));
#12002=EDGE_LOOP('',(#50413,#50414,#50415,#50416));
#12003=EDGE_LOOP('',(#50417,#50418,#50419,#50420));
#12004=EDGE_LOOP('',(#50421,#50422,#50423,#50424));
#12005=EDGE_LOOP('',(#50425,#50426,#50427,#50428));
#12006=EDGE_LOOP('',(#50429,#50430,#50431,#50432));
#12007=EDGE_LOOP('',(#50433,#50434,#50435,#50436));
#12008=EDGE_LOOP('',(#50437,#50438,#50439,#50440));
#12009=EDGE_LOOP('',(#50441,#50442,#50443,#50444));
#12010=EDGE_LOOP('',(#50445,#50446,#50447,#50448));
#12011=EDGE_LOOP('',(#50449,#50450,#50451,#50452));
#12012=EDGE_LOOP('',(#50453,#50454,#50455,#50456));
#12013=EDGE_LOOP('',(#50457,#50458,#50459,#50460));
#12014=EDGE_LOOP('',(#50461,#50462,#50463,#50464));
#12015=EDGE_LOOP('',(#50465,#50466,#50467,#50468));
#12016=EDGE_LOOP('',(#50469,#50470,#50471,#50472));
#12017=EDGE_LOOP('',(#50473,#50474,#50475,#50476));
#12018=EDGE_LOOP('',(#50477,#50478,#50479,#50480));
#12019=EDGE_LOOP('',(#50481,#50482,#50483,#50484));
#12020=EDGE_LOOP('',(#50485,#50486,#50487,#50488));
#12021=EDGE_LOOP('',(#50489,#50490,#50491,#50492));
#12022=EDGE_LOOP('',(#50493,#50494,#50495,#50496));
#12023=EDGE_LOOP('',(#50497,#50498,#50499,#50500));
#12024=EDGE_LOOP('',(#50501,#50502,#50503,#50504));
#12025=EDGE_LOOP('',(#50505,#50506,#50507,#50508));
#12026=EDGE_LOOP('',(#50509,#50510,#50511,#50512));
#12027=EDGE_LOOP('',(#50513,#50514,#50515,#50516));
#12028=EDGE_LOOP('',(#50517,#50518,#50519,#50520));
#12029=EDGE_LOOP('',(#50521,#50522,#50523,#50524));
#12030=EDGE_LOOP('',(#50525,#50526,#50527,#50528));
#12031=EDGE_LOOP('',(#50529,#50530,#50531,#50532));
#12032=EDGE_LOOP('',(#50533,#50534,#50535,#50536));
#12033=EDGE_LOOP('',(#50537,#50538,#50539,#50540));
#12034=EDGE_LOOP('',(#50541,#50542,#50543,#50544));
#12035=EDGE_LOOP('',(#50545,#50546,#50547,#50548));
#12036=EDGE_LOOP('',(#50549,#50550,#50551,#50552));
#12037=EDGE_LOOP('',(#50553,#50554,#50555,#50556));
#12038=EDGE_LOOP('',(#50557,#50558,#50559,#50560));
#12039=EDGE_LOOP('',(#50561,#50562,#50563,#50564));
#12040=EDGE_LOOP('',(#50565,#50566,#50567,#50568));
#12041=EDGE_LOOP('',(#50569,#50570,#50571,#50572));
#12042=EDGE_LOOP('',(#50573,#50574,#50575,#50576));
#12043=EDGE_LOOP('',(#50577,#50578,#50579,#50580));
#12044=EDGE_LOOP('',(#50581,#50582,#50583,#50584));
#12045=EDGE_LOOP('',(#50585,#50586,#50587,#50588));
#12046=EDGE_LOOP('',(#50589,#50590,#50591,#50592));
#12047=EDGE_LOOP('',(#50593,#50594,#50595,#50596));
#12048=EDGE_LOOP('',(#50597,#50598,#50599,#50600));
#12049=EDGE_LOOP('',(#50601,#50602,#50603,#50604));
#12050=EDGE_LOOP('',(#50605,#50606,#50607,#50608));
#12051=EDGE_LOOP('',(#50609,#50610,#50611,#50612));
#12052=EDGE_LOOP('',(#50613,#50614,#50615,#50616));
#12053=EDGE_LOOP('',(#50617,#50618,#50619,#50620));
#12054=EDGE_LOOP('',(#50621,#50622,#50623,#50624));
#12055=EDGE_LOOP('',(#50625,#50626,#50627,#50628));
#12056=EDGE_LOOP('',(#50629,#50630,#50631,#50632));
#12057=EDGE_LOOP('',(#50633,#50634,#50635,#50636));
#12058=EDGE_LOOP('',(#50637,#50638,#50639,#50640));
#12059=EDGE_LOOP('',(#50641,#50642,#50643,#50644));
#12060=EDGE_LOOP('',(#50645,#50646,#50647,#50648));
#12061=EDGE_LOOP('',(#50649,#50650,#50651,#50652));
#12062=EDGE_LOOP('',(#50653,#50654,#50655,#50656));
#12063=EDGE_LOOP('',(#50657,#50658,#50659,#50660));
#12064=EDGE_LOOP('',(#50661,#50662,#50663,#50664));
#12065=EDGE_LOOP('',(#50665,#50666,#50667,#50668));
#12066=EDGE_LOOP('',(#50669,#50670,#50671,#50672));
#12067=EDGE_LOOP('',(#50673,#50674,#50675,#50676));
#12068=EDGE_LOOP('',(#50677,#50678,#50679,#50680));
#12069=EDGE_LOOP('',(#50681,#50682,#50683,#50684));
#12070=EDGE_LOOP('',(#50685,#50686,#50687,#50688));
#12071=EDGE_LOOP('',(#50689,#50690,#50691,#50692));
#12072=EDGE_LOOP('',(#50693,#50694,#50695,#50696));
#12073=EDGE_LOOP('',(#50697,#50698,#50699,#50700));
#12074=EDGE_LOOP('',(#50701,#50702,#50703,#50704));
#12075=EDGE_LOOP('',(#50705,#50706,#50707,#50708));
#12076=EDGE_LOOP('',(#50709,#50710,#50711,#50712));
#12077=EDGE_LOOP('',(#50713,#50714,#50715,#50716));
#12078=EDGE_LOOP('',(#50717,#50718,#50719,#50720));
#12079=EDGE_LOOP('',(#50721,#50722,#50723,#50724));
#12080=EDGE_LOOP('',(#50725,#50726,#50727,#50728));
#12081=EDGE_LOOP('',(#50729,#50730,#50731,#50732));
#12082=EDGE_LOOP('',(#50733,#50734,#50735,#50736));
#12083=EDGE_LOOP('',(#50737,#50738,#50739,#50740));
#12084=EDGE_LOOP('',(#50741,#50742,#50743,#50744));
#12085=EDGE_LOOP('',(#50745,#50746,#50747,#50748));
#12086=EDGE_LOOP('',(#50749,#50750,#50751,#50752));
#12087=EDGE_LOOP('',(#50753,#50754,#50755,#50756));
#12088=EDGE_LOOP('',(#50757,#50758,#50759,#50760));
#12089=EDGE_LOOP('',(#50761,#50762,#50763,#50764));
#12090=EDGE_LOOP('',(#50765,#50766,#50767,#50768));
#12091=EDGE_LOOP('',(#50769,#50770,#50771,#50772));
#12092=EDGE_LOOP('',(#50773,#50774,#50775,#50776));
#12093=EDGE_LOOP('',(#50777,#50778,#50779,#50780));
#12094=EDGE_LOOP('',(#50781,#50782,#50783,#50784));
#12095=EDGE_LOOP('',(#50785,#50786,#50787,#50788));
#12096=EDGE_LOOP('',(#50789,#50790,#50791,#50792));
#12097=EDGE_LOOP('',(#50793,#50794,#50795,#50796));
#12098=EDGE_LOOP('',(#50797,#50798,#50799,#50800));
#12099=EDGE_LOOP('',(#50801,#50802,#50803,#50804));
#12100=EDGE_LOOP('',(#50805,#50806,#50807,#50808));
#12101=EDGE_LOOP('',(#50809,#50810,#50811,#50812));
#12102=EDGE_LOOP('',(#50813,#50814,#50815,#50816));
#12103=EDGE_LOOP('',(#50817,#50818,#50819,#50820));
#12104=EDGE_LOOP('',(#50821,#50822,#50823,#50824));
#12105=EDGE_LOOP('',(#50825,#50826,#50827,#50828));
#12106=EDGE_LOOP('',(#50829,#50830,#50831,#50832));
#12107=EDGE_LOOP('',(#50833,#50834,#50835,#50836));
#12108=EDGE_LOOP('',(#50837,#50838,#50839,#50840));
#12109=EDGE_LOOP('',(#50841,#50842,#50843,#50844));
#12110=EDGE_LOOP('',(#50845,#50846,#50847,#50848));
#12111=EDGE_LOOP('',(#50849,#50850,#50851,#50852));
#12112=EDGE_LOOP('',(#50853,#50854,#50855,#50856));
#12113=EDGE_LOOP('',(#50857,#50858,#50859,#50860));
#12114=EDGE_LOOP('',(#50861,#50862,#50863,#50864));
#12115=EDGE_LOOP('',(#50865,#50866,#50867,#50868));
#12116=EDGE_LOOP('',(#50869,#50870,#50871,#50872));
#12117=EDGE_LOOP('',(#50873,#50874,#50875,#50876));
#12118=EDGE_LOOP('',(#50877,#50878,#50879,#50880));
#12119=EDGE_LOOP('',(#50881,#50882,#50883,#50884));
#12120=EDGE_LOOP('',(#50885,#50886,#50887,#50888));
#12121=EDGE_LOOP('',(#50889,#50890,#50891,#50892));
#12122=EDGE_LOOP('',(#50893,#50894,#50895,#50896));
#12123=EDGE_LOOP('',(#50897,#50898,#50899,#50900));
#12124=EDGE_LOOP('',(#50901,#50902,#50903,#50904));
#12125=EDGE_LOOP('',(#50905,#50906,#50907,#50908));
#12126=EDGE_LOOP('',(#50909,#50910,#50911,#50912));
#12127=EDGE_LOOP('',(#50913,#50914,#50915,#50916));
#12128=EDGE_LOOP('',(#50917,#50918,#50919,#50920));
#12129=EDGE_LOOP('',(#50921,#50922,#50923,#50924));
#12130=EDGE_LOOP('',(#50925,#50926,#50927,#50928));
#12131=EDGE_LOOP('',(#50929,#50930,#50931,#50932));
#12132=EDGE_LOOP('',(#50933,#50934,#50935,#50936));
#12133=EDGE_LOOP('',(#50937,#50938,#50939,#50940));
#12134=EDGE_LOOP('',(#50941,#50942,#50943,#50944));
#12135=EDGE_LOOP('',(#50945,#50946,#50947,#50948));
#12136=EDGE_LOOP('',(#50949,#50950,#50951,#50952));
#12137=EDGE_LOOP('',(#50953,#50954,#50955,#50956));
#12138=EDGE_LOOP('',(#50957,#50958,#50959,#50960));
#12139=EDGE_LOOP('',(#50961,#50962,#50963,#50964));
#12140=EDGE_LOOP('',(#50965,#50966,#50967,#50968));
#12141=EDGE_LOOP('',(#50969,#50970,#50971,#50972));
#12142=EDGE_LOOP('',(#50973,#50974,#50975,#50976));
#12143=EDGE_LOOP('',(#50977,#50978,#50979,#50980));
#12144=EDGE_LOOP('',(#50981,#50982,#50983,#50984));
#12145=EDGE_LOOP('',(#50985,#50986,#50987,#50988));
#12146=EDGE_LOOP('',(#50989,#50990,#50991,#50992));
#12147=EDGE_LOOP('',(#50993,#50994,#50995,#50996));
#12148=EDGE_LOOP('',(#50997,#50998,#50999,#51000));
#12149=EDGE_LOOP('',(#51001,#51002,#51003,#51004));
#12150=EDGE_LOOP('',(#51005,#51006,#51007,#51008));
#12151=EDGE_LOOP('',(#51009,#51010,#51011,#51012));
#12152=EDGE_LOOP('',(#51013,#51014,#51015,#51016));
#12153=EDGE_LOOP('',(#51017,#51018,#51019,#51020));
#12154=EDGE_LOOP('',(#51021,#51022,#51023,#51024));
#12155=EDGE_LOOP('',(#51025,#51026,#51027,#51028));
#12156=EDGE_LOOP('',(#51029,#51030,#51031,#51032));
#12157=EDGE_LOOP('',(#51033,#51034,#51035,#51036));
#12158=EDGE_LOOP('',(#51037,#51038,#51039,#51040));
#12159=EDGE_LOOP('',(#51041,#51042,#51043,#51044));
#12160=EDGE_LOOP('',(#51045,#51046,#51047,#51048));
#12161=EDGE_LOOP('',(#51049,#51050,#51051,#51052));
#12162=EDGE_LOOP('',(#51053,#51054,#51055,#51056));
#12163=EDGE_LOOP('',(#51057,#51058,#51059,#51060));
#12164=EDGE_LOOP('',(#51061,#51062,#51063,#51064));
#12165=EDGE_LOOP('',(#51065,#51066,#51067,#51068));
#12166=EDGE_LOOP('',(#51069,#51070,#51071,#51072));
#12167=EDGE_LOOP('',(#51073,#51074,#51075,#51076));
#12168=EDGE_LOOP('',(#51077,#51078,#51079,#51080));
#12169=EDGE_LOOP('',(#51081,#51082,#51083,#51084));
#12170=EDGE_LOOP('',(#51085,#51086,#51087,#51088));
#12171=EDGE_LOOP('',(#51089,#51090,#51091,#51092));
#12172=EDGE_LOOP('',(#51093,#51094,#51095,#51096));
#12173=EDGE_LOOP('',(#51097,#51098,#51099,#51100));
#12174=EDGE_LOOP('',(#51101,#51102,#51103,#51104));
#12175=EDGE_LOOP('',(#51105,#51106,#51107,#51108));
#12176=EDGE_LOOP('',(#51109,#51110,#51111,#51112));
#12177=EDGE_LOOP('',(#51113,#51114,#51115,#51116));
#12178=EDGE_LOOP('',(#51117,#51118,#51119,#51120));
#12179=EDGE_LOOP('',(#51121,#51122,#51123,#51124));
#12180=EDGE_LOOP('',(#51125,#51126,#51127,#51128));
#12181=EDGE_LOOP('',(#51129,#51130,#51131,#51132));
#12182=EDGE_LOOP('',(#51133,#51134,#51135,#51136));
#12183=EDGE_LOOP('',(#51137,#51138,#51139,#51140));
#12184=EDGE_LOOP('',(#51141,#51142,#51143,#51144));
#12185=EDGE_LOOP('',(#51145,#51146,#51147,#51148));
#12186=EDGE_LOOP('',(#51149,#51150,#51151,#51152));
#12187=EDGE_LOOP('',(#51153,#51154,#51155,#51156));
#12188=EDGE_LOOP('',(#51157,#51158,#51159,#51160));
#12189=EDGE_LOOP('',(#51161,#51162,#51163,#51164));
#12190=EDGE_LOOP('',(#51165,#51166,#51167,#51168));
#12191=EDGE_LOOP('',(#51169,#51170,#51171,#51172));
#12192=EDGE_LOOP('',(#51173,#51174,#51175,#51176));
#12193=EDGE_LOOP('',(#51177,#51178,#51179,#51180));
#12194=EDGE_LOOP('',(#51181,#51182,#51183,#51184));
#12195=EDGE_LOOP('',(#51185,#51186,#51187,#51188));
#12196=EDGE_LOOP('',(#51189,#51190,#51191,#51192));
#12197=EDGE_LOOP('',(#51193,#51194,#51195,#51196));
#12198=EDGE_LOOP('',(#51197,#51198,#51199,#51200));
#12199=EDGE_LOOP('',(#51201,#51202,#51203,#51204));
#12200=EDGE_LOOP('',(#51205,#51206,#51207,#51208));
#12201=EDGE_LOOP('',(#51209,#51210,#51211,#51212));
#12202=EDGE_LOOP('',(#51213,#51214,#51215,#51216));
#12203=EDGE_LOOP('',(#51217,#51218,#51219,#51220));
#12204=EDGE_LOOP('',(#51221,#51222,#51223,#51224));
#12205=EDGE_LOOP('',(#51225,#51226,#51227,#51228));
#12206=EDGE_LOOP('',(#51229,#51230,#51231,#51232));
#12207=EDGE_LOOP('',(#51233,#51234,#51235,#51236));
#12208=EDGE_LOOP('',(#51237,#51238,#51239,#51240));
#12209=EDGE_LOOP('',(#51241,#51242,#51243,#51244));
#12210=EDGE_LOOP('',(#51245,#51246,#51247,#51248));
#12211=EDGE_LOOP('',(#51249,#51250,#51251,#51252));
#12212=EDGE_LOOP('',(#51253,#51254,#51255,#51256));
#12213=EDGE_LOOP('',(#51257,#51258,#51259,#51260));
#12214=EDGE_LOOP('',(#51261,#51262,#51263,#51264));
#12215=EDGE_LOOP('',(#51265,#51266,#51267,#51268));
#12216=EDGE_LOOP('',(#51269,#51270,#51271,#51272));
#12217=EDGE_LOOP('',(#51273,#51274,#51275,#51276));
#12218=EDGE_LOOP('',(#51277,#51278,#51279,#51280));
#12219=EDGE_LOOP('',(#51281,#51282,#51283,#51284));
#12220=EDGE_LOOP('',(#51285,#51286,#51287,#51288));
#12221=EDGE_LOOP('',(#51289,#51290,#51291,#51292));
#12222=EDGE_LOOP('',(#51293,#51294,#51295,#51296));
#12223=EDGE_LOOP('',(#51297,#51298,#51299,#51300));
#12224=EDGE_LOOP('',(#51301,#51302,#51303,#51304));
#12225=EDGE_LOOP('',(#51305,#51306,#51307,#51308));
#12226=EDGE_LOOP('',(#51309,#51310,#51311,#51312));
#12227=EDGE_LOOP('',(#51313,#51314,#51315,#51316));
#12228=EDGE_LOOP('',(#51317,#51318,#51319,#51320));
#12229=EDGE_LOOP('',(#51321,#51322,#51323,#51324));
#12230=EDGE_LOOP('',(#51325,#51326,#51327,#51328));
#12231=EDGE_LOOP('',(#51329,#51330,#51331,#51332));
#12232=EDGE_LOOP('',(#51333,#51334,#51335,#51336));
#12233=EDGE_LOOP('',(#51337,#51338,#51339,#51340));
#12234=EDGE_LOOP('',(#51341,#51342,#51343,#51344));
#12235=EDGE_LOOP('',(#51345,#51346,#51347,#51348));
#12236=EDGE_LOOP('',(#51349,#51350,#51351,#51352));
#12237=EDGE_LOOP('',(#51353,#51354,#51355,#51356));
#12238=EDGE_LOOP('',(#51357,#51358,#51359,#51360));
#12239=EDGE_LOOP('',(#51361,#51362,#51363,#51364));
#12240=EDGE_LOOP('',(#51365,#51366,#51367,#51368));
#12241=EDGE_LOOP('',(#51369,#51370,#51371,#51372));
#12242=EDGE_LOOP('',(#51373,#51374,#51375,#51376));
#12243=EDGE_LOOP('',(#51377,#51378,#51379,#51380));
#12244=EDGE_LOOP('',(#51381,#51382,#51383,#51384));
#12245=EDGE_LOOP('',(#51385,#51386,#51387,#51388));
#12246=EDGE_LOOP('',(#51389,#51390,#51391,#51392));
#12247=EDGE_LOOP('',(#51393,#51394,#51395,#51396));
#12248=EDGE_LOOP('',(#51397,#51398,#51399,#51400));
#12249=EDGE_LOOP('',(#51401,#51402,#51403,#51404));
#12250=EDGE_LOOP('',(#51405,#51406,#51407,#51408));
#12251=EDGE_LOOP('',(#51409,#51410,#51411,#51412));
#12252=EDGE_LOOP('',(#51413,#51414,#51415,#51416));
#12253=EDGE_LOOP('',(#51417,#51418,#51419,#51420));
#12254=EDGE_LOOP('',(#51421,#51422,#51423,#51424));
#12255=EDGE_LOOP('',(#51425,#51426,#51427,#51428));
#12256=EDGE_LOOP('',(#51429,#51430,#51431,#51432));
#12257=EDGE_LOOP('',(#51433,#51434,#51435,#51436));
#12258=EDGE_LOOP('',(#51437,#51438,#51439,#51440));
#12259=EDGE_LOOP('',(#51441,#51442,#51443,#51444));
#12260=EDGE_LOOP('',(#51445,#51446,#51447,#51448));
#12261=EDGE_LOOP('',(#51449,#51450,#51451,#51452));
#12262=EDGE_LOOP('',(#51453,#51454,#51455,#51456));
#12263=EDGE_LOOP('',(#51457,#51458,#51459,#51460));
#12264=EDGE_LOOP('',(#51461,#51462,#51463,#51464));
#12265=EDGE_LOOP('',(#51465,#51466,#51467,#51468));
#12266=EDGE_LOOP('',(#51469,#51470,#51471,#51472));
#12267=EDGE_LOOP('',(#51473,#51474,#51475,#51476));
#12268=EDGE_LOOP('',(#51477,#51478,#51479,#51480));
#12269=EDGE_LOOP('',(#51481,#51482,#51483,#51484));
#12270=EDGE_LOOP('',(#51485,#51486,#51487,#51488));
#12271=EDGE_LOOP('',(#51489,#51490,#51491,#51492));
#12272=EDGE_LOOP('',(#51493,#51494,#51495,#51496));
#12273=EDGE_LOOP('',(#51497,#51498,#51499,#51500));
#12274=EDGE_LOOP('',(#51501,#51502,#51503,#51504));
#12275=EDGE_LOOP('',(#51505,#51506,#51507,#51508));
#12276=EDGE_LOOP('',(#51509,#51510,#51511,#51512));
#12277=EDGE_LOOP('',(#51513,#51514,#51515,#51516));
#12278=EDGE_LOOP('',(#51517,#51518,#51519,#51520));
#12279=EDGE_LOOP('',(#51521,#51522,#51523,#51524));
#12280=EDGE_LOOP('',(#51525,#51526,#51527,#51528));
#12281=EDGE_LOOP('',(#51529,#51530,#51531,#51532));
#12282=EDGE_LOOP('',(#51533,#51534,#51535,#51536));
#12283=EDGE_LOOP('',(#51537,#51538,#51539,#51540));
#12284=EDGE_LOOP('',(#51541,#51542,#51543,#51544));
#12285=EDGE_LOOP('',(#51545,#51546,#51547,#51548));
#12286=EDGE_LOOP('',(#51549,#51550,#51551,#51552));
#12287=EDGE_LOOP('',(#51553,#51554,#51555,#51556));
#12288=EDGE_LOOP('',(#51557,#51558,#51559,#51560));
#12289=EDGE_LOOP('',(#51561,#51562,#51563,#51564));
#12290=EDGE_LOOP('',(#51565,#51566,#51567,#51568));
#12291=EDGE_LOOP('',(#51569,#51570,#51571,#51572));
#12292=EDGE_LOOP('',(#51573,#51574,#51575,#51576));
#12293=EDGE_LOOP('',(#51577,#51578,#51579,#51580));
#12294=EDGE_LOOP('',(#51581,#51582,#51583,#51584));
#12295=EDGE_LOOP('',(#51585,#51586,#51587,#51588));
#12296=EDGE_LOOP('',(#51589,#51590,#51591,#51592));
#12297=EDGE_LOOP('',(#51593,#51594,#51595,#51596));
#12298=EDGE_LOOP('',(#51597,#51598,#51599,#51600));
#12299=EDGE_LOOP('',(#51601,#51602,#51603,#51604));
#12300=EDGE_LOOP('',(#51605,#51606,#51607,#51608));
#12301=EDGE_LOOP('',(#51609,#51610,#51611,#51612));
#12302=EDGE_LOOP('',(#51613,#51614,#51615,#51616));
#12303=EDGE_LOOP('',(#51617,#51618,#51619,#51620));
#12304=EDGE_LOOP('',(#51621,#51622,#51623,#51624));
#12305=EDGE_LOOP('',(#51625,#51626,#51627,#51628));
#12306=EDGE_LOOP('',(#51629,#51630,#51631,#51632));
#12307=EDGE_LOOP('',(#51633,#51634,#51635,#51636));
#12308=EDGE_LOOP('',(#51637,#51638,#51639,#51640));
#12309=EDGE_LOOP('',(#51641,#51642,#51643,#51644));
#12310=EDGE_LOOP('',(#51645,#51646,#51647,#51648));
#12311=EDGE_LOOP('',(#51649,#51650,#51651,#51652));
#12312=EDGE_LOOP('',(#51653,#51654,#51655,#51656));
#12313=EDGE_LOOP('',(#51657,#51658,#51659,#51660));
#12314=EDGE_LOOP('',(#51661,#51662,#51663,#51664));
#12315=EDGE_LOOP('',(#51665,#51666,#51667,#51668));
#12316=EDGE_LOOP('',(#51669,#51670,#51671,#51672));
#12317=EDGE_LOOP('',(#51673,#51674,#51675,#51676));
#12318=EDGE_LOOP('',(#51677,#51678,#51679,#51680));
#12319=EDGE_LOOP('',(#51681,#51682,#51683,#51684));
#12320=EDGE_LOOP('',(#51685,#51686,#51687,#51688));
#12321=EDGE_LOOP('',(#51689,#51690,#51691,#51692));
#12322=EDGE_LOOP('',(#51693,#51694,#51695,#51696));
#12323=EDGE_LOOP('',(#51697,#51698,#51699,#51700));
#12324=EDGE_LOOP('',(#51701,#51702,#51703,#51704));
#12325=EDGE_LOOP('',(#51705,#51706,#51707,#51708));
#12326=EDGE_LOOP('',(#51709,#51710,#51711,#51712));
#12327=EDGE_LOOP('',(#51713,#51714,#51715,#51716));
#12328=EDGE_LOOP('',(#51717,#51718,#51719,#51720));
#12329=EDGE_LOOP('',(#51721,#51722,#51723,#51724));
#12330=EDGE_LOOP('',(#51725,#51726,#51727,#51728));
#12331=EDGE_LOOP('',(#51729,#51730,#51731,#51732));
#12332=EDGE_LOOP('',(#51733,#51734,#51735,#51736));
#12333=EDGE_LOOP('',(#51737,#51738,#51739,#51740));
#12334=EDGE_LOOP('',(#51741,#51742,#51743,#51744));
#12335=EDGE_LOOP('',(#51745,#51746,#51747,#51748));
#12336=EDGE_LOOP('',(#51749,#51750,#51751,#51752));
#12337=EDGE_LOOP('',(#51753,#51754,#51755,#51756));
#12338=EDGE_LOOP('',(#51757,#51758,#51759,#51760));
#12339=EDGE_LOOP('',(#51761,#51762,#51763,#51764));
#12340=EDGE_LOOP('',(#51765,#51766,#51767,#51768));
#12341=EDGE_LOOP('',(#51769,#51770,#51771,#51772));
#12342=EDGE_LOOP('',(#51773,#51774,#51775,#51776));
#12343=EDGE_LOOP('',(#51777,#51778,#51779,#51780));
#12344=EDGE_LOOP('',(#51781,#51782,#51783,#51784));
#12345=EDGE_LOOP('',(#51785,#51786,#51787,#51788));
#12346=EDGE_LOOP('',(#51789,#51790,#51791,#51792));
#12347=EDGE_LOOP('',(#51793,#51794,#51795,#51796));
#12348=EDGE_LOOP('',(#51797,#51798,#51799,#51800));
#12349=EDGE_LOOP('',(#51801,#51802,#51803,#51804));
#12350=EDGE_LOOP('',(#51805,#51806,#51807,#51808));
#12351=EDGE_LOOP('',(#51809,#51810,#51811,#51812));
#12352=EDGE_LOOP('',(#51813,#51814,#51815,#51816));
#12353=EDGE_LOOP('',(#51817,#51818,#51819,#51820));
#12354=EDGE_LOOP('',(#51821,#51822,#51823,#51824));
#12355=EDGE_LOOP('',(#51825,#51826,#51827,#51828));
#12356=EDGE_LOOP('',(#51829,#51830,#51831,#51832));
#12357=EDGE_LOOP('',(#51833,#51834,#51835,#51836));
#12358=EDGE_LOOP('',(#51837,#51838,#51839,#51840));
#12359=EDGE_LOOP('',(#51841,#51842,#51843,#51844));
#12360=EDGE_LOOP('',(#51845,#51846,#51847,#51848));
#12361=EDGE_LOOP('',(#51849,#51850,#51851,#51852));
#12362=EDGE_LOOP('',(#51853,#51854,#51855,#51856));
#12363=EDGE_LOOP('',(#51857,#51858,#51859,#51860));
#12364=EDGE_LOOP('',(#51861,#51862,#51863,#51864));
#12365=EDGE_LOOP('',(#51865,#51866,#51867,#51868));
#12366=EDGE_LOOP('',(#51869,#51870,#51871,#51872));
#12367=EDGE_LOOP('',(#51873,#51874,#51875,#51876));
#12368=EDGE_LOOP('',(#51877,#51878,#51879,#51880));
#12369=EDGE_LOOP('',(#51881,#51882,#51883,#51884));
#12370=EDGE_LOOP('',(#51885,#51886,#51887,#51888));
#12371=EDGE_LOOP('',(#51889,#51890,#51891,#51892));
#12372=EDGE_LOOP('',(#51893,#51894,#51895,#51896));
#12373=EDGE_LOOP('',(#51897,#51898,#51899,#51900));
#12374=EDGE_LOOP('',(#51901,#51902,#51903,#51904));
#12375=EDGE_LOOP('',(#51905,#51906,#51907,#51908));
#12376=EDGE_LOOP('',(#51909,#51910,#51911,#51912));
#12377=EDGE_LOOP('',(#51913,#51914,#51915,#51916));
#12378=EDGE_LOOP('',(#51917,#51918,#51919,#51920));
#12379=EDGE_LOOP('',(#51921,#51922,#51923,#51924));
#12380=EDGE_LOOP('',(#51925,#51926,#51927,#51928));
#12381=EDGE_LOOP('',(#51929,#51930,#51931,#51932));
#12382=EDGE_LOOP('',(#51933,#51934,#51935,#51936));
#12383=EDGE_LOOP('',(#51937,#51938,#51939,#51940));
#12384=EDGE_LOOP('',(#51941,#51942,#51943,#51944));
#12385=EDGE_LOOP('',(#51945,#51946,#51947,#51948));
#12386=EDGE_LOOP('',(#51949,#51950,#51951,#51952));
#12387=EDGE_LOOP('',(#51953,#51954,#51955,#51956));
#12388=EDGE_LOOP('',(#51957,#51958,#51959,#51960));
#12389=EDGE_LOOP('',(#51961,#51962,#51963,#51964));
#12390=EDGE_LOOP('',(#51965,#51966,#51967,#51968));
#12391=EDGE_LOOP('',(#51969,#51970,#51971,#51972));
#12392=EDGE_LOOP('',(#51973,#51974,#51975,#51976));
#12393=EDGE_LOOP('',(#51977,#51978,#51979,#51980));
#12394=EDGE_LOOP('',(#51981,#51982,#51983,#51984));
#12395=EDGE_LOOP('',(#51985,#51986,#51987,#51988));
#12396=EDGE_LOOP('',(#51989,#51990,#51991,#51992));
#12397=EDGE_LOOP('',(#51993,#51994,#51995,#51996));
#12398=EDGE_LOOP('',(#51997,#51998,#51999,#52000));
#12399=EDGE_LOOP('',(#52001,#52002,#52003,#52004));
#12400=EDGE_LOOP('',(#52005,#52006,#52007,#52008));
#12401=EDGE_LOOP('',(#52009,#52010,#52011,#52012));
#12402=EDGE_LOOP('',(#52013,#52014,#52015,#52016));
#12403=EDGE_LOOP('',(#52017,#52018,#52019,#52020));
#12404=EDGE_LOOP('',(#52021,#52022,#52023,#52024));
#12405=EDGE_LOOP('',(#52025,#52026,#52027,#52028));
#12406=EDGE_LOOP('',(#52029,#52030,#52031,#52032));
#12407=EDGE_LOOP('',(#52033,#52034,#52035,#52036));
#12408=EDGE_LOOP('',(#52037,#52038,#52039,#52040));
#12409=EDGE_LOOP('',(#52041,#52042,#52043,#52044));
#12410=EDGE_LOOP('',(#52045,#52046,#52047,#52048));
#12411=EDGE_LOOP('',(#52049,#52050,#52051,#52052));
#12412=EDGE_LOOP('',(#52053,#52054,#52055,#52056));
#12413=EDGE_LOOP('',(#52057,#52058,#52059,#52060));
#12414=EDGE_LOOP('',(#52061,#52062,#52063,#52064));
#12415=EDGE_LOOP('',(#52065,#52066,#52067,#52068));
#12416=EDGE_LOOP('',(#52069,#52070,#52071,#52072));
#12417=EDGE_LOOP('',(#52073,#52074,#52075,#52076));
#12418=EDGE_LOOP('',(#52077,#52078,#52079,#52080));
#12419=EDGE_LOOP('',(#52081,#52082,#52083,#52084));
#12420=EDGE_LOOP('',(#52085,#52086,#52087,#52088));
#12421=EDGE_LOOP('',(#52089,#52090,#52091,#52092));
#12422=EDGE_LOOP('',(#52093,#52094,#52095,#52096));
#12423=EDGE_LOOP('',(#52097,#52098,#52099,#52100));
#12424=EDGE_LOOP('',(#52101,#52102,#52103,#52104));
#12425=EDGE_LOOP('',(#52105,#52106,#52107,#52108));
#12426=EDGE_LOOP('',(#52109,#52110,#52111,#52112));
#12427=EDGE_LOOP('',(#52113,#52114,#52115,#52116));
#12428=EDGE_LOOP('',(#52117,#52118,#52119,#52120));
#12429=EDGE_LOOP('',(#52121,#52122,#52123,#52124));
#12430=EDGE_LOOP('',(#52125,#52126,#52127,#52128));
#12431=EDGE_LOOP('',(#52129,#52130,#52131,#52132));
#12432=EDGE_LOOP('',(#52133,#52134,#52135,#52136));
#12433=EDGE_LOOP('',(#52137,#52138,#52139,#52140));
#12434=EDGE_LOOP('',(#52141,#52142,#52143,#52144));
#12435=EDGE_LOOP('',(#52145,#52146,#52147,#52148));
#12436=EDGE_LOOP('',(#52149,#52150,#52151,#52152));
#12437=EDGE_LOOP('',(#52153,#52154,#52155,#52156));
#12438=EDGE_LOOP('',(#52157,#52158,#52159,#52160));
#12439=EDGE_LOOP('',(#52161,#52162,#52163,#52164));
#12440=EDGE_LOOP('',(#52165,#52166,#52167,#52168));
#12441=EDGE_LOOP('',(#52169,#52170,#52171,#52172));
#12442=EDGE_LOOP('',(#52173,#52174,#52175,#52176));
#12443=EDGE_LOOP('',(#52177,#52178,#52179,#52180));
#12444=EDGE_LOOP('',(#52181,#52182,#52183,#52184));
#12445=EDGE_LOOP('',(#52185,#52186,#52187,#52188));
#12446=EDGE_LOOP('',(#52189,#52190,#52191,#52192));
#12447=EDGE_LOOP('',(#52193,#52194,#52195,#52196));
#12448=EDGE_LOOP('',(#52197,#52198,#52199,#52200));
#12449=EDGE_LOOP('',(#52201,#52202,#52203,#52204));
#12450=EDGE_LOOP('',(#52205,#52206,#52207,#52208));
#12451=EDGE_LOOP('',(#52209,#52210,#52211,#52212));
#12452=EDGE_LOOP('',(#52213,#52214,#52215,#52216));
#12453=EDGE_LOOP('',(#52217,#52218,#52219,#52220));
#12454=EDGE_LOOP('',(#52221,#52222,#52223,#52224));
#12455=EDGE_LOOP('',(#52225,#52226,#52227,#52228));
#12456=EDGE_LOOP('',(#52229,#52230,#52231,#52232));
#12457=EDGE_LOOP('',(#52233,#52234,#52235,#52236));
#12458=EDGE_LOOP('',(#52237,#52238,#52239,#52240));
#12459=EDGE_LOOP('',(#52241,#52242,#52243,#52244));
#12460=EDGE_LOOP('',(#52245,#52246,#52247,#52248));
#12461=EDGE_LOOP('',(#52249,#52250,#52251,#52252));
#12462=EDGE_LOOP('',(#52253,#52254,#52255,#52256));
#12463=EDGE_LOOP('',(#52257,#52258,#52259,#52260));
#12464=EDGE_LOOP('',(#52261,#52262,#52263,#52264));
#12465=EDGE_LOOP('',(#52265,#52266,#52267,#52268));
#12466=EDGE_LOOP('',(#52269,#52270,#52271,#52272));
#12467=EDGE_LOOP('',(#52273,#52274,#52275,#52276));
#12468=EDGE_LOOP('',(#52277,#52278,#52279,#52280));
#12469=EDGE_LOOP('',(#52281,#52282,#52283,#52284));
#12470=EDGE_LOOP('',(#52285,#52286,#52287,#52288));
#12471=EDGE_LOOP('',(#52289,#52290,#52291,#52292));
#12472=EDGE_LOOP('',(#52293,#52294,#52295,#52296));
#12473=EDGE_LOOP('',(#52297,#52298,#52299,#52300));
#12474=EDGE_LOOP('',(#52301,#52302,#52303,#52304));
#12475=EDGE_LOOP('',(#52305,#52306,#52307,#52308));
#12476=EDGE_LOOP('',(#52309,#52310,#52311,#52312));
#12477=EDGE_LOOP('',(#52313,#52314,#52315,#52316));
#12478=EDGE_LOOP('',(#52317,#52318,#52319,#52320));
#12479=EDGE_LOOP('',(#52321,#52322,#52323,#52324));
#12480=EDGE_LOOP('',(#52325,#52326,#52327,#52328));
#12481=EDGE_LOOP('',(#52329,#52330,#52331,#52332));
#12482=EDGE_LOOP('',(#52333,#52334,#52335,#52336));
#12483=EDGE_LOOP('',(#52337,#52338,#52339,#52340));
#12484=EDGE_LOOP('',(#52341,#52342,#52343,#52344));
#12485=EDGE_LOOP('',(#52345,#52346,#52347,#52348));
#12486=EDGE_LOOP('',(#52349,#52350,#52351,#52352));
#12487=EDGE_LOOP('',(#52353,#52354,#52355,#52356));
#12488=EDGE_LOOP('',(#52357,#52358,#52359,#52360));
#12489=EDGE_LOOP('',(#52361,#52362,#52363,#52364));
#12490=EDGE_LOOP('',(#52365,#52366,#52367,#52368));
#12491=EDGE_LOOP('',(#52369,#52370,#52371,#52372));
#12492=EDGE_LOOP('',(#52373,#52374,#52375,#52376));
#12493=EDGE_LOOP('',(#52377,#52378,#52379,#52380));
#12494=EDGE_LOOP('',(#52381,#52382,#52383,#52384));
#12495=EDGE_LOOP('',(#52385,#52386,#52387,#52388));
#12496=EDGE_LOOP('',(#52389,#52390,#52391,#52392));
#12497=EDGE_LOOP('',(#52393,#52394,#52395,#52396));
#12498=EDGE_LOOP('',(#52397,#52398,#52399,#52400));
#12499=EDGE_LOOP('',(#52401,#52402,#52403,#52404));
#12500=EDGE_LOOP('',(#52405,#52406,#52407,#52408));
#12501=EDGE_LOOP('',(#52409,#52410,#52411,#52412));
#12502=EDGE_LOOP('',(#52413,#52414,#52415,#52416));
#12503=EDGE_LOOP('',(#52417,#52418,#52419,#52420));
#12504=EDGE_LOOP('',(#52421,#52422,#52423,#52424));
#12505=EDGE_LOOP('',(#52425,#52426,#52427,#52428));
#12506=EDGE_LOOP('',(#52429,#52430,#52431,#52432));
#12507=EDGE_LOOP('',(#52433,#52434,#52435,#52436));
#12508=EDGE_LOOP('',(#52437,#52438,#52439,#52440));
#12509=EDGE_LOOP('',(#52441,#52442,#52443,#52444));
#12510=EDGE_LOOP('',(#52445,#52446,#52447,#52448));
#12511=EDGE_LOOP('',(#52449,#52450,#52451,#52452));
#12512=EDGE_LOOP('',(#52453,#52454,#52455,#52456));
#12513=EDGE_LOOP('',(#52457,#52458,#52459,#52460));
#12514=EDGE_LOOP('',(#52461,#52462,#52463,#52464));
#12515=EDGE_LOOP('',(#52465,#52466,#52467,#52468));
#12516=EDGE_LOOP('',(#52469,#52470,#52471,#52472));
#12517=EDGE_LOOP('',(#52473,#52474,#52475,#52476));
#12518=EDGE_LOOP('',(#52477,#52478,#52479,#52480));
#12519=EDGE_LOOP('',(#52481,#52482,#52483,#52484));
#12520=EDGE_LOOP('',(#52485,#52486,#52487,#52488));
#12521=EDGE_LOOP('',(#52489,#52490,#52491,#52492));
#12522=EDGE_LOOP('',(#52493,#52494,#52495,#52496));
#12523=EDGE_LOOP('',(#52497,#52498,#52499,#52500));
#12524=EDGE_LOOP('',(#52501,#52502,#52503,#52504));
#12525=EDGE_LOOP('',(#52505,#52506,#52507,#52508));
#12526=EDGE_LOOP('',(#52509,#52510,#52511,#52512));
#12527=EDGE_LOOP('',(#52513,#52514,#52515,#52516));
#12528=EDGE_LOOP('',(#52517,#52518,#52519,#52520));
#12529=EDGE_LOOP('',(#52521,#52522,#52523,#52524));
#12530=EDGE_LOOP('',(#52525,#52526,#52527,#52528));
#12531=EDGE_LOOP('',(#52529,#52530,#52531,#52532));
#12532=EDGE_LOOP('',(#52533,#52534,#52535,#52536));
#12533=EDGE_LOOP('',(#52537,#52538,#52539,#52540));
#12534=EDGE_LOOP('',(#52541,#52542,#52543,#52544));
#12535=EDGE_LOOP('',(#52545,#52546,#52547,#52548));
#12536=EDGE_LOOP('',(#52549,#52550,#52551,#52552));
#12537=EDGE_LOOP('',(#52553,#52554,#52555,#52556));
#12538=EDGE_LOOP('',(#52557,#52558,#52559,#52560));
#12539=EDGE_LOOP('',(#52561,#52562,#52563,#52564));
#12540=EDGE_LOOP('',(#52565,#52566,#52567,#52568));
#12541=EDGE_LOOP('',(#52569,#52570,#52571,#52572));
#12542=EDGE_LOOP('',(#52573,#52574,#52575,#52576));
#12543=EDGE_LOOP('',(#52577,#52578,#52579,#52580));
#12544=EDGE_LOOP('',(#52581,#52582,#52583,#52584));
#12545=EDGE_LOOP('',(#52585,#52586,#52587,#52588));
#12546=EDGE_LOOP('',(#52589,#52590,#52591,#52592));
#12547=EDGE_LOOP('',(#52593,#52594,#52595,#52596));
#12548=EDGE_LOOP('',(#52597,#52598,#52599,#52600));
#12549=EDGE_LOOP('',(#52601,#52602,#52603,#52604));
#12550=EDGE_LOOP('',(#52605,#52606,#52607,#52608));
#12551=EDGE_LOOP('',(#52609,#52610,#52611,#52612));
#12552=EDGE_LOOP('',(#52613,#52614,#52615,#52616));
#12553=EDGE_LOOP('',(#52617,#52618,#52619,#52620));
#12554=EDGE_LOOP('',(#52621,#52622,#52623,#52624));
#12555=EDGE_LOOP('',(#52625,#52626,#52627,#52628));
#12556=EDGE_LOOP('',(#52629,#52630,#52631,#52632));
#12557=EDGE_LOOP('',(#52633,#52634,#52635,#52636));
#12558=EDGE_LOOP('',(#52637,#52638,#52639,#52640));
#12559=EDGE_LOOP('',(#52641,#52642,#52643,#52644));
#12560=EDGE_LOOP('',(#52645,#52646,#52647,#52648));
#12561=EDGE_LOOP('',(#52649,#52650,#52651,#52652));
#12562=EDGE_LOOP('',(#52653,#52654,#52655,#52656));
#12563=EDGE_LOOP('',(#52657,#52658,#52659,#52660));
#12564=EDGE_LOOP('',(#52661,#52662,#52663,#52664));
#12565=EDGE_LOOP('',(#52665,#52666,#52667,#52668));
#12566=EDGE_LOOP('',(#52669,#52670,#52671,#52672));
#12567=EDGE_LOOP('',(#52673,#52674,#52675,#52676));
#12568=EDGE_LOOP('',(#52677,#52678,#52679,#52680));
#12569=EDGE_LOOP('',(#52681,#52682,#52683,#52684));
#12570=EDGE_LOOP('',(#52685,#52686,#52687,#52688));
#12571=EDGE_LOOP('',(#52689,#52690,#52691,#52692));
#12572=EDGE_LOOP('',(#52693,#52694,#52695,#52696));
#12573=EDGE_LOOP('',(#52697,#52698,#52699,#52700));
#12574=EDGE_LOOP('',(#52701,#52702,#52703,#52704));
#12575=EDGE_LOOP('',(#52705,#52706,#52707,#52708));
#12576=EDGE_LOOP('',(#52709,#52710,#52711,#52712));
#12577=EDGE_LOOP('',(#52713,#52714,#52715,#52716));
#12578=EDGE_LOOP('',(#52717,#52718,#52719,#52720));
#12579=EDGE_LOOP('',(#52721,#52722,#52723,#52724));
#12580=EDGE_LOOP('',(#52725,#52726,#52727,#52728));
#12581=EDGE_LOOP('',(#52729,#52730,#52731,#52732));
#12582=EDGE_LOOP('',(#52733,#52734,#52735,#52736));
#12583=EDGE_LOOP('',(#52737,#52738,#52739,#52740));
#12584=EDGE_LOOP('',(#52741,#52742,#52743,#52744));
#12585=EDGE_LOOP('',(#52745,#52746,#52747,#52748));
#12586=EDGE_LOOP('',(#52749,#52750,#52751,#52752));
#12587=EDGE_LOOP('',(#52753,#52754,#52755,#52756));
#12588=EDGE_LOOP('',(#52757,#52758,#52759,#52760));
#12589=EDGE_LOOP('',(#52761,#52762,#52763,#52764));
#12590=EDGE_LOOP('',(#52765,#52766,#52767,#52768));
#12591=EDGE_LOOP('',(#52769,#52770,#52771,#52772));
#12592=EDGE_LOOP('',(#52773,#52774,#52775,#52776));
#12593=EDGE_LOOP('',(#52777,#52778,#52779,#52780));
#12594=EDGE_LOOP('',(#52781,#52782,#52783,#52784));
#12595=EDGE_LOOP('',(#52785,#52786,#52787,#52788));
#12596=EDGE_LOOP('',(#52789,#52790,#52791,#52792));
#12597=EDGE_LOOP('',(#52793,#52794,#52795,#52796));
#12598=EDGE_LOOP('',(#52797,#52798,#52799,#52800));
#12599=EDGE_LOOP('',(#52801,#52802,#52803,#52804));
#12600=EDGE_LOOP('',(#52805,#52806,#52807,#52808));
#12601=EDGE_LOOP('',(#52809,#52810,#52811,#52812));
#12602=EDGE_LOOP('',(#52813,#52814,#52815,#52816));
#12603=EDGE_LOOP('',(#52817,#52818,#52819,#52820));
#12604=EDGE_LOOP('',(#52821,#52822,#52823,#52824));
#12605=EDGE_LOOP('',(#52825,#52826,#52827,#52828));
#12606=EDGE_LOOP('',(#52829,#52830,#52831,#52832));
#12607=EDGE_LOOP('',(#52833,#52834,#52835,#52836));
#12608=EDGE_LOOP('',(#52837,#52838,#52839,#52840));
#12609=EDGE_LOOP('',(#52841,#52842,#52843,#52844));
#12610=EDGE_LOOP('',(#52845,#52846,#52847,#52848));
#12611=EDGE_LOOP('',(#52849,#52850,#52851,#52852));
#12612=EDGE_LOOP('',(#52853,#52854,#52855,#52856));
#12613=EDGE_LOOP('',(#52857,#52858,#52859,#52860));
#12614=EDGE_LOOP('',(#52861,#52862,#52863,#52864));
#12615=EDGE_LOOP('',(#52865,#52866,#52867,#52868));
#12616=EDGE_LOOP('',(#52869,#52870,#52871,#52872));
#12617=EDGE_LOOP('',(#52873,#52874,#52875,#52876));
#12618=EDGE_LOOP('',(#52877,#52878,#52879,#52880));
#12619=EDGE_LOOP('',(#52881,#52882,#52883,#52884));
#12620=EDGE_LOOP('',(#52885,#52886,#52887,#52888));
#12621=EDGE_LOOP('',(#52889,#52890,#52891,#52892));
#12622=EDGE_LOOP('',(#52893,#52894,#52895,#52896));
#12623=EDGE_LOOP('',(#52897,#52898,#52899,#52900));
#12624=EDGE_LOOP('',(#52901,#52902,#52903,#52904));
#12625=EDGE_LOOP('',(#52905,#52906,#52907,#52908));
#12626=EDGE_LOOP('',(#52909,#52910,#52911,#52912));
#12627=EDGE_LOOP('',(#52913,#52914,#52915,#52916));
#12628=EDGE_LOOP('',(#52917,#52918,#52919,#52920));
#12629=EDGE_LOOP('',(#52921,#52922,#52923,#52924));
#12630=EDGE_LOOP('',(#52925,#52926,#52927,#52928));
#12631=EDGE_LOOP('',(#52929,#52930,#52931,#52932));
#12632=EDGE_LOOP('',(#52933,#52934,#52935,#52936));
#12633=EDGE_LOOP('',(#52937,#52938,#52939,#52940));
#12634=EDGE_LOOP('',(#52941,#52942,#52943,#52944));
#12635=EDGE_LOOP('',(#52945,#52946,#52947,#52948));
#12636=EDGE_LOOP('',(#52949,#52950,#52951,#52952));
#12637=EDGE_LOOP('',(#52953,#52954,#52955,#52956));
#12638=EDGE_LOOP('',(#52957,#52958,#52959,#52960));
#12639=EDGE_LOOP('',(#52961,#52962,#52963,#52964));
#12640=EDGE_LOOP('',(#52965,#52966,#52967,#52968));
#12641=EDGE_LOOP('',(#52969,#52970,#52971,#52972));
#12642=EDGE_LOOP('',(#52973,#52974,#52975,#52976));
#12643=EDGE_LOOP('',(#52977,#52978,#52979,#52980));
#12644=EDGE_LOOP('',(#52981,#52982,#52983,#52984));
#12645=EDGE_LOOP('',(#52985,#52986,#52987,#52988));
#12646=EDGE_LOOP('',(#52989,#52990,#52991,#52992));
#12647=EDGE_LOOP('',(#52993,#52994,#52995,#52996));
#12648=EDGE_LOOP('',(#52997,#52998,#52999,#53000));
#12649=EDGE_LOOP('',(#53001,#53002,#53003,#53004));
#12650=EDGE_LOOP('',(#53005,#53006,#53007,#53008));
#12651=EDGE_LOOP('',(#53009,#53010,#53011,#53012));
#12652=EDGE_LOOP('',(#53013,#53014,#53015,#53016));
#12653=EDGE_LOOP('',(#53017,#53018,#53019,#53020));
#12654=EDGE_LOOP('',(#53021,#53022,#53023,#53024));
#12655=EDGE_LOOP('',(#53025,#53026,#53027,#53028));
#12656=EDGE_LOOP('',(#53029,#53030,#53031,#53032));
#12657=EDGE_LOOP('',(#53033,#53034,#53035,#53036));
#12658=EDGE_LOOP('',(#53037,#53038,#53039,#53040));
#12659=EDGE_LOOP('',(#53041,#53042,#53043,#53044));
#12660=EDGE_LOOP('',(#53045,#53046,#53047,#53048));
#12661=EDGE_LOOP('',(#53049,#53050,#53051,#53052));
#12662=EDGE_LOOP('',(#53053,#53054,#53055,#53056));
#12663=EDGE_LOOP('',(#53057,#53058,#53059,#53060));
#12664=EDGE_LOOP('',(#53061,#53062,#53063,#53064));
#12665=EDGE_LOOP('',(#53065,#53066,#53067,#53068));
#12666=EDGE_LOOP('',(#53069,#53070,#53071,#53072));
#12667=EDGE_LOOP('',(#53073,#53074,#53075,#53076));
#12668=EDGE_LOOP('',(#53077,#53078,#53079,#53080));
#12669=EDGE_LOOP('',(#53081,#53082,#53083,#53084));
#12670=EDGE_LOOP('',(#53085,#53086,#53087,#53088));
#12671=EDGE_LOOP('',(#53089,#53090,#53091,#53092));
#12672=EDGE_LOOP('',(#53093,#53094,#53095,#53096));
#12673=EDGE_LOOP('',(#53097,#53098,#53099,#53100));
#12674=EDGE_LOOP('',(#53101,#53102,#53103,#53104));
#12675=EDGE_LOOP('',(#53105,#53106,#53107,#53108));
#12676=EDGE_LOOP('',(#53109,#53110,#53111,#53112));
#12677=EDGE_LOOP('',(#53113,#53114,#53115,#53116));
#12678=EDGE_LOOP('',(#53117,#53118,#53119,#53120));
#12679=EDGE_LOOP('',(#53121,#53122,#53123,#53124));
#12680=EDGE_LOOP('',(#53125,#53126,#53127,#53128));
#12681=EDGE_LOOP('',(#53129,#53130,#53131,#53132));
#12682=EDGE_LOOP('',(#53133,#53134,#53135,#53136));
#12683=EDGE_LOOP('',(#53137,#53138,#53139,#53140));
#12684=EDGE_LOOP('',(#53141,#53142,#53143,#53144));
#12685=EDGE_LOOP('',(#53145,#53146,#53147,#53148));
#12686=EDGE_LOOP('',(#53149,#53150,#53151,#53152));
#12687=EDGE_LOOP('',(#53153,#53154,#53155,#53156));
#12688=EDGE_LOOP('',(#53157,#53158,#53159,#53160));
#12689=EDGE_LOOP('',(#53161,#53162,#53163,#53164));
#12690=EDGE_LOOP('',(#53165,#53166,#53167,#53168));
#12691=EDGE_LOOP('',(#53169,#53170,#53171,#53172));
#12692=EDGE_LOOP('',(#53173,#53174,#53175,#53176));
#12693=EDGE_LOOP('',(#53177,#53178,#53179,#53180));
#12694=EDGE_LOOP('',(#53181,#53182,#53183,#53184));
#12695=EDGE_LOOP('',(#53185,#53186,#53187,#53188));
#12696=EDGE_LOOP('',(#53189,#53190,#53191,#53192));
#12697=EDGE_LOOP('',(#53193,#53194,#53195,#53196));
#12698=EDGE_LOOP('',(#53197,#53198,#53199,#53200));
#12699=EDGE_LOOP('',(#53201,#53202,#53203,#53204));
#12700=EDGE_LOOP('',(#53205,#53206,#53207,#53208));
#12701=EDGE_LOOP('',(#53209,#53210,#53211,#53212));
#12702=EDGE_LOOP('',(#53213,#53214,#53215,#53216));
#12703=EDGE_LOOP('',(#53217,#53218,#53219,#53220));
#12704=EDGE_LOOP('',(#53221,#53222,#53223,#53224));
#12705=EDGE_LOOP('',(#53225,#53226,#53227,#53228));
#12706=EDGE_LOOP('',(#53229,#53230,#53231,#53232));
#12707=EDGE_LOOP('',(#53233,#53234,#53235,#53236));
#12708=EDGE_LOOP('',(#53237,#53238,#53239,#53240));
#12709=EDGE_LOOP('',(#53241,#53242,#53243,#53244));
#12710=EDGE_LOOP('',(#53245,#53246,#53247,#53248));
#12711=EDGE_LOOP('',(#53249,#53250,#53251,#53252));
#12712=EDGE_LOOP('',(#53253,#53254,#53255,#53256));
#12713=EDGE_LOOP('',(#53257,#53258,#53259,#53260));
#12714=EDGE_LOOP('',(#53261,#53262,#53263,#53264));
#12715=EDGE_LOOP('',(#53265,#53266,#53267,#53268));
#12716=EDGE_LOOP('',(#53269,#53270,#53271,#53272));
#12717=EDGE_LOOP('',(#53273,#53274,#53275,#53276));
#12718=EDGE_LOOP('',(#53277,#53278,#53279,#53280));
#12719=EDGE_LOOP('',(#53281,#53282,#53283,#53284));
#12720=EDGE_LOOP('',(#53285,#53286,#53287,#53288));
#12721=EDGE_LOOP('',(#53289,#53290,#53291,#53292));
#12722=EDGE_LOOP('',(#53293,#53294,#53295,#53296));
#12723=EDGE_LOOP('',(#53297,#53298,#53299,#53300));
#12724=EDGE_LOOP('',(#53301,#53302,#53303,#53304));
#12725=EDGE_LOOP('',(#53305,#53306,#53307,#53308));
#12726=EDGE_LOOP('',(#53309,#53310,#53311,#53312));
#12727=EDGE_LOOP('',(#53313,#53314,#53315,#53316));
#12728=EDGE_LOOP('',(#53317,#53318,#53319,#53320));
#12729=EDGE_LOOP('',(#53321,#53322,#53323,#53324));
#12730=EDGE_LOOP('',(#53325,#53326,#53327,#53328));
#12731=EDGE_LOOP('',(#53329,#53330,#53331,#53332));
#12732=EDGE_LOOP('',(#53333,#53334,#53335,#53336));
#12733=EDGE_LOOP('',(#53337,#53338,#53339,#53340));
#12734=EDGE_LOOP('',(#53341,#53342,#53343,#53344));
#12735=EDGE_LOOP('',(#53345,#53346,#53347,#53348));
#12736=EDGE_LOOP('',(#53349,#53350,#53351,#53352));
#12737=EDGE_LOOP('',(#53353,#53354,#53355,#53356));
#12738=EDGE_LOOP('',(#53357,#53358,#53359,#53360));
#12739=EDGE_LOOP('',(#53361,#53362,#53363,#53364));
#12740=EDGE_LOOP('',(#53365,#53366,#53367,#53368));
#12741=EDGE_LOOP('',(#53369,#53370,#53371,#53372));
#12742=EDGE_LOOP('',(#53373,#53374,#53375,#53376));
#12743=EDGE_LOOP('',(#53377,#53378,#53379,#53380));
#12744=EDGE_LOOP('',(#53381,#53382,#53383,#53384));
#12745=EDGE_LOOP('',(#53385,#53386,#53387,#53388));
#12746=EDGE_LOOP('',(#53389,#53390,#53391,#53392));
#12747=EDGE_LOOP('',(#53393,#53394,#53395,#53396));
#12748=EDGE_LOOP('',(#53397,#53398,#53399,#53400));
#12749=EDGE_LOOP('',(#53401,#53402,#53403,#53404));
#12750=EDGE_LOOP('',(#53405,#53406,#53407,#53408));
#12751=EDGE_LOOP('',(#53409,#53410,#53411,#53412));
#12752=EDGE_LOOP('',(#53413,#53414,#53415,#53416));
#12753=EDGE_LOOP('',(#53417,#53418,#53419,#53420));
#12754=EDGE_LOOP('',(#53421,#53422,#53423,#53424));
#12755=EDGE_LOOP('',(#53425,#53426,#53427,#53428));
#12756=EDGE_LOOP('',(#53429,#53430,#53431,#53432));
#12757=EDGE_LOOP('',(#53433,#53434,#53435,#53436));
#12758=EDGE_LOOP('',(#53437,#53438,#53439,#53440));
#12759=EDGE_LOOP('',(#53441,#53442,#53443,#53444));
#12760=EDGE_LOOP('',(#53445,#53446,#53447,#53448));
#12761=EDGE_LOOP('',(#53449,#53450,#53451,#53452));
#12762=EDGE_LOOP('',(#53453,#53454,#53455,#53456));
#12763=EDGE_LOOP('',(#53457,#53458,#53459,#53460));
#12764=EDGE_LOOP('',(#53461,#53462,#53463,#53464));
#12765=EDGE_LOOP('',(#53465,#53466,#53467,#53468));
#12766=EDGE_LOOP('',(#53469,#53470,#53471,#53472));
#12767=EDGE_LOOP('',(#53473,#53474,#53475,#53476));
#12768=EDGE_LOOP('',(#53477,#53478,#53479,#53480));
#12769=EDGE_LOOP('',(#53481,#53482,#53483,#53484));
#12770=EDGE_LOOP('',(#53485,#53486,#53487,#53488));
#12771=EDGE_LOOP('',(#53489,#53490,#53491,#53492));
#12772=EDGE_LOOP('',(#53493,#53494,#53495,#53496));
#12773=EDGE_LOOP('',(#53497,#53498,#53499,#53500));
#12774=EDGE_LOOP('',(#53501,#53502,#53503,#53504));
#12775=EDGE_LOOP('',(#53505,#53506,#53507,#53508));
#12776=EDGE_LOOP('',(#53509,#53510,#53511,#53512));
#12777=EDGE_LOOP('',(#53513,#53514,#53515,#53516));
#12778=EDGE_LOOP('',(#53517,#53518,#53519,#53520));
#12779=EDGE_LOOP('',(#53521,#53522,#53523,#53524));
#12780=EDGE_LOOP('',(#53525,#53526,#53527,#53528));
#12781=EDGE_LOOP('',(#53529,#53530,#53531,#53532));
#12782=EDGE_LOOP('',(#53533,#53534,#53535,#53536));
#12783=EDGE_LOOP('',(#53537,#53538,#53539,#53540));
#12784=EDGE_LOOP('',(#53541,#53542,#53543,#53544));
#12785=EDGE_LOOP('',(#53545,#53546,#53547,#53548));
#12786=EDGE_LOOP('',(#53549,#53550,#53551,#53552));
#12787=EDGE_LOOP('',(#53553,#53554,#53555,#53556));
#12788=EDGE_LOOP('',(#53557,#53558,#53559,#53560));
#12789=EDGE_LOOP('',(#53561,#53562,#53563,#53564));
#12790=EDGE_LOOP('',(#53565,#53566,#53567,#53568));
#12791=EDGE_LOOP('',(#53569,#53570,#53571,#53572));
#12792=EDGE_LOOP('',(#53573,#53574,#53575,#53576));
#12793=EDGE_LOOP('',(#53577,#53578,#53579,#53580));
#12794=EDGE_LOOP('',(#53581,#53582,#53583,#53584));
#12795=EDGE_LOOP('',(#53585,#53586,#53587,#53588));
#12796=EDGE_LOOP('',(#53589,#53590,#53591,#53592));
#12797=EDGE_LOOP('',(#53593,#53594,#53595,#53596));
#12798=EDGE_LOOP('',(#53597,#53598,#53599,#53600));
#12799=EDGE_LOOP('',(#53601,#53602,#53603,#53604));
#12800=EDGE_LOOP('',(#53605,#53606,#53607,#53608));
#12801=EDGE_LOOP('',(#53609,#53610,#53611,#53612));
#12802=EDGE_LOOP('',(#53613,#53614,#53615,#53616));
#12803=EDGE_LOOP('',(#53617,#53618,#53619,#53620));
#12804=EDGE_LOOP('',(#53621,#53622,#53623,#53624));
#12805=EDGE_LOOP('',(#53625,#53626,#53627,#53628));
#12806=EDGE_LOOP('',(#53629,#53630,#53631,#53632));
#12807=EDGE_LOOP('',(#53633,#53634,#53635,#53636));
#12808=EDGE_LOOP('',(#53637,#53638,#53639,#53640));
#12809=EDGE_LOOP('',(#53641,#53642,#53643,#53644));
#12810=EDGE_LOOP('',(#53645,#53646,#53647,#53648));
#12811=EDGE_LOOP('',(#53649,#53650,#53651,#53652));
#12812=EDGE_LOOP('',(#53653,#53654,#53655,#53656));
#12813=EDGE_LOOP('',(#53657,#53658,#53659,#53660));
#12814=EDGE_LOOP('',(#53661,#53662,#53663,#53664));
#12815=EDGE_LOOP('',(#53665,#53666,#53667,#53668));
#12816=EDGE_LOOP('',(#53669,#53670,#53671,#53672));
#12817=EDGE_LOOP('',(#53673,#53674,#53675,#53676));
#12818=EDGE_LOOP('',(#53677,#53678,#53679,#53680));
#12819=EDGE_LOOP('',(#53681,#53682,#53683,#53684));
#12820=EDGE_LOOP('',(#53685,#53686,#53687,#53688));
#12821=EDGE_LOOP('',(#53689,#53690,#53691,#53692));
#12822=EDGE_LOOP('',(#53693,#53694,#53695,#53696));
#12823=EDGE_LOOP('',(#53697,#53698,#53699,#53700));
#12824=EDGE_LOOP('',(#53701,#53702,#53703,#53704));
#12825=EDGE_LOOP('',(#53705,#53706,#53707,#53708));
#12826=EDGE_LOOP('',(#53709,#53710,#53711,#53712));
#12827=EDGE_LOOP('',(#53713,#53714,#53715,#53716));
#12828=EDGE_LOOP('',(#53717,#53718,#53719,#53720));
#12829=EDGE_LOOP('',(#53721,#53722,#53723,#53724));
#12830=EDGE_LOOP('',(#53725,#53726,#53727,#53728));
#12831=EDGE_LOOP('',(#53729,#53730,#53731,#53732));
#12832=EDGE_LOOP('',(#53733,#53734,#53735,#53736));
#12833=EDGE_LOOP('',(#53737,#53738,#53739,#53740));
#12834=EDGE_LOOP('',(#53741,#53742,#53743,#53744));
#12835=EDGE_LOOP('',(#53745,#53746,#53747,#53748));
#12836=EDGE_LOOP('',(#53749,#53750,#53751,#53752));
#12837=EDGE_LOOP('',(#53753,#53754,#53755,#53756));
#12838=EDGE_LOOP('',(#53757,#53758,#53759,#53760));
#12839=EDGE_LOOP('',(#53761,#53762,#53763,#53764));
#12840=EDGE_LOOP('',(#53765,#53766,#53767,#53768));
#12841=EDGE_LOOP('',(#53769,#53770,#53771,#53772));
#12842=EDGE_LOOP('',(#53773,#53774,#53775,#53776));
#12843=EDGE_LOOP('',(#53777,#53778,#53779,#53780));
#12844=EDGE_LOOP('',(#53781,#53782,#53783,#53784));
#12845=EDGE_LOOP('',(#53785,#53786,#53787,#53788));
#12846=EDGE_LOOP('',(#53789,#53790,#53791,#53792));
#12847=EDGE_LOOP('',(#53793,#53794,#53795,#53796));
#12848=EDGE_LOOP('',(#53797,#53798,#53799,#53800));
#12849=EDGE_LOOP('',(#53801,#53802,#53803,#53804));
#12850=EDGE_LOOP('',(#53805,#53806,#53807,#53808));
#12851=EDGE_LOOP('',(#53809,#53810,#53811,#53812));
#12852=EDGE_LOOP('',(#53813,#53814,#53815,#53816));
#12853=EDGE_LOOP('',(#53817,#53818,#53819,#53820));
#12854=EDGE_LOOP('',(#53821,#53822,#53823,#53824));
#12855=EDGE_LOOP('',(#53825,#53826,#53827,#53828));
#12856=EDGE_LOOP('',(#53829,#53830,#53831,#53832));
#12857=EDGE_LOOP('',(#53833,#53834,#53835,#53836));
#12858=EDGE_LOOP('',(#53837,#53838,#53839,#53840));
#12859=EDGE_LOOP('',(#53841,#53842,#53843,#53844));
#12860=EDGE_LOOP('',(#53845,#53846,#53847,#53848));
#12861=EDGE_LOOP('',(#53849,#53850,#53851,#53852));
#12862=EDGE_LOOP('',(#53853,#53854,#53855,#53856));
#12863=EDGE_LOOP('',(#53857,#53858,#53859,#53860));
#12864=EDGE_LOOP('',(#53861,#53862,#53863,#53864));
#12865=EDGE_LOOP('',(#53865,#53866,#53867,#53868));
#12866=EDGE_LOOP('',(#53869,#53870,#53871,#53872));
#12867=EDGE_LOOP('',(#53873,#53874,#53875,#53876));
#12868=EDGE_LOOP('',(#53877,#53878,#53879,#53880));
#12869=EDGE_LOOP('',(#53881,#53882,#53883,#53884));
#12870=EDGE_LOOP('',(#53885,#53886,#53887,#53888));
#12871=EDGE_LOOP('',(#53889,#53890,#53891,#53892));
#12872=EDGE_LOOP('',(#53893,#53894,#53895,#53896));
#12873=EDGE_LOOP('',(#53897,#53898,#53899,#53900));
#12874=EDGE_LOOP('',(#53901,#53902,#53903,#53904));
#12875=EDGE_LOOP('',(#53905,#53906,#53907,#53908));
#12876=EDGE_LOOP('',(#53909,#53910,#53911,#53912));
#12877=EDGE_LOOP('',(#53913,#53914,#53915,#53916));
#12878=EDGE_LOOP('',(#53917,#53918,#53919,#53920));
#12879=EDGE_LOOP('',(#53921,#53922,#53923,#53924));
#12880=EDGE_LOOP('',(#53925,#53926,#53927,#53928));
#12881=EDGE_LOOP('',(#53929,#53930,#53931,#53932));
#12882=EDGE_LOOP('',(#53933,#53934,#53935,#53936));
#12883=EDGE_LOOP('',(#53937,#53938,#53939,#53940));
#12884=EDGE_LOOP('',(#53941,#53942,#53943,#53944));
#12885=EDGE_LOOP('',(#53945,#53946,#53947,#53948));
#12886=EDGE_LOOP('',(#53949,#53950,#53951,#53952));
#12887=EDGE_LOOP('',(#53953,#53954,#53955,#53956));
#12888=EDGE_LOOP('',(#53957,#53958,#53959,#53960));
#12889=EDGE_LOOP('',(#53961,#53962,#53963,#53964));
#12890=EDGE_LOOP('',(#53965,#53966,#53967,#53968));
#12891=EDGE_LOOP('',(#53969,#53970,#53971,#53972));
#12892=EDGE_LOOP('',(#53973,#53974,#53975,#53976));
#12893=EDGE_LOOP('',(#53977,#53978,#53979,#53980));
#12894=EDGE_LOOP('',(#53981,#53982,#53983,#53984));
#12895=EDGE_LOOP('',(#53985,#53986,#53987,#53988));
#12896=EDGE_LOOP('',(#53989,#53990,#53991,#53992));
#12897=EDGE_LOOP('',(#53993,#53994,#53995,#53996));
#12898=EDGE_LOOP('',(#53997,#53998,#53999,#54000));
#12899=EDGE_LOOP('',(#54001,#54002,#54003,#54004));
#12900=EDGE_LOOP('',(#54005,#54006,#54007,#54008));
#12901=EDGE_LOOP('',(#54009,#54010,#54011,#54012));
#12902=EDGE_LOOP('',(#54013,#54014,#54015,#54016));
#12903=EDGE_LOOP('',(#54017,#54018,#54019,#54020));
#12904=EDGE_LOOP('',(#54021,#54022,#54023,#54024));
#12905=EDGE_LOOP('',(#54025,#54026,#54027,#54028));
#12906=EDGE_LOOP('',(#54029,#54030,#54031,#54032));
#12907=EDGE_LOOP('',(#54033,#54034,#54035,#54036));
#12908=EDGE_LOOP('',(#54037,#54038,#54039,#54040));
#12909=EDGE_LOOP('',(#54041,#54042,#54043,#54044));
#12910=EDGE_LOOP('',(#54045,#54046,#54047,#54048));
#12911=EDGE_LOOP('',(#54049,#54050,#54051,#54052));
#12912=EDGE_LOOP('',(#54053,#54054,#54055,#54056));
#12913=EDGE_LOOP('',(#54057,#54058,#54059,#54060));
#12914=EDGE_LOOP('',(#54061,#54062,#54063,#54064));
#12915=EDGE_LOOP('',(#54065,#54066,#54067,#54068));
#12916=EDGE_LOOP('',(#54069,#54070,#54071,#54072));
#12917=EDGE_LOOP('',(#54073,#54074,#54075,#54076));
#12918=EDGE_LOOP('',(#54077,#54078,#54079,#54080));
#12919=EDGE_LOOP('',(#54081,#54082,#54083,#54084));
#12920=EDGE_LOOP('',(#54085,#54086,#54087,#54088));
#12921=EDGE_LOOP('',(#54089,#54090,#54091,#54092));
#12922=EDGE_LOOP('',(#54093,#54094,#54095,#54096));
#12923=EDGE_LOOP('',(#54097,#54098,#54099,#54100));
#12924=EDGE_LOOP('',(#54101,#54102,#54103,#54104));
#12925=EDGE_LOOP('',(#54105,#54106,#54107,#54108));
#12926=EDGE_LOOP('',(#54109,#54110,#54111,#54112));
#12927=EDGE_LOOP('',(#54113,#54114,#54115,#54116));
#12928=EDGE_LOOP('',(#54117,#54118,#54119,#54120));
#12929=EDGE_LOOP('',(#54121,#54122,#54123,#54124));
#12930=EDGE_LOOP('',(#54125,#54126,#54127,#54128));
#12931=EDGE_LOOP('',(#54129,#54130,#54131,#54132));
#12932=EDGE_LOOP('',(#54133,#54134,#54135,#54136));
#12933=EDGE_LOOP('',(#54137,#54138,#54139,#54140));
#12934=EDGE_LOOP('',(#54141,#54142,#54143,#54144));
#12935=EDGE_LOOP('',(#54145,#54146,#54147,#54148));
#12936=EDGE_LOOP('',(#54149,#54150,#54151,#54152));
#12937=EDGE_LOOP('',(#54153,#54154,#54155,#54156));
#12938=EDGE_LOOP('',(#54157,#54158,#54159,#54160));
#12939=EDGE_LOOP('',(#54161,#54162,#54163,#54164));
#12940=EDGE_LOOP('',(#54165,#54166,#54167,#54168));
#12941=EDGE_LOOP('',(#54169,#54170,#54171,#54172));
#12942=EDGE_LOOP('',(#54173,#54174,#54175,#54176));
#12943=EDGE_LOOP('',(#54177,#54178,#54179,#54180));
#12944=EDGE_LOOP('',(#54181,#54182,#54183,#54184));
#12945=EDGE_LOOP('',(#54185,#54186,#54187,#54188));
#12946=EDGE_LOOP('',(#54189,#54190,#54191,#54192));
#12947=EDGE_LOOP('',(#54193,#54194,#54195,#54196));
#12948=EDGE_LOOP('',(#54197,#54198,#54199,#54200));
#12949=EDGE_LOOP('',(#54201,#54202,#54203,#54204));
#12950=EDGE_LOOP('',(#54205,#54206,#54207,#54208));
#12951=EDGE_LOOP('',(#54209,#54210,#54211,#54212));
#12952=EDGE_LOOP('',(#54213,#54214,#54215,#54216));
#12953=EDGE_LOOP('',(#54217,#54218,#54219,#54220));
#12954=EDGE_LOOP('',(#54221,#54222,#54223,#54224));
#12955=EDGE_LOOP('',(#54225,#54226,#54227,#54228));
#12956=EDGE_LOOP('',(#54229,#54230,#54231,#54232));
#12957=EDGE_LOOP('',(#54233,#54234,#54235,#54236));
#12958=EDGE_LOOP('',(#54237,#54238,#54239,#54240));
#12959=EDGE_LOOP('',(#54241,#54242,#54243,#54244));
#12960=EDGE_LOOP('',(#54245,#54246,#54247,#54248));
#12961=EDGE_LOOP('',(#54249,#54250,#54251,#54252));
#12962=EDGE_LOOP('',(#54253,#54254,#54255,#54256));
#12963=EDGE_LOOP('',(#54257,#54258,#54259,#54260));
#12964=EDGE_LOOP('',(#54261,#54262,#54263,#54264));
#12965=EDGE_LOOP('',(#54265,#54266,#54267,#54268));
#12966=EDGE_LOOP('',(#54269,#54270,#54271,#54272));
#12967=EDGE_LOOP('',(#54273,#54274,#54275,#54276));
#12968=EDGE_LOOP('',(#54277,#54278,#54279,#54280));
#12969=EDGE_LOOP('',(#54281,#54282,#54283,#54284));
#12970=EDGE_LOOP('',(#54285,#54286,#54287,#54288));
#12971=EDGE_LOOP('',(#54289,#54290,#54291,#54292));
#12972=EDGE_LOOP('',(#54293,#54294,#54295,#54296));
#12973=EDGE_LOOP('',(#54297,#54298,#54299,#54300));
#12974=EDGE_LOOP('',(#54301,#54302,#54303,#54304));
#12975=EDGE_LOOP('',(#54305,#54306,#54307,#54308));
#12976=EDGE_LOOP('',(#54309,#54310,#54311,#54312));
#12977=EDGE_LOOP('',(#54313,#54314,#54315,#54316));
#12978=EDGE_LOOP('',(#54317,#54318,#54319,#54320));
#12979=EDGE_LOOP('',(#54321,#54322,#54323,#54324));
#12980=EDGE_LOOP('',(#54325,#54326,#54327,#54328));
#12981=EDGE_LOOP('',(#54329,#54330,#54331,#54332));
#12982=EDGE_LOOP('',(#54333,#54334,#54335,#54336));
#12983=EDGE_LOOP('',(#54337,#54338,#54339,#54340));
#12984=EDGE_LOOP('',(#54341,#54342,#54343,#54344));
#12985=EDGE_LOOP('',(#54345,#54346,#54347,#54348));
#12986=EDGE_LOOP('',(#54349,#54350,#54351,#54352));
#12987=EDGE_LOOP('',(#54353,#54354,#54355,#54356));
#12988=EDGE_LOOP('',(#54357,#54358,#54359,#54360));
#12989=EDGE_LOOP('',(#54361,#54362,#54363,#54364));
#12990=EDGE_LOOP('',(#54365,#54366,#54367,#54368));
#12991=EDGE_LOOP('',(#54369,#54370,#54371,#54372));
#12992=EDGE_LOOP('',(#54373,#54374,#54375,#54376));
#12993=EDGE_LOOP('',(#54377,#54378,#54379,#54380));
#12994=EDGE_LOOP('',(#54381,#54382,#54383,#54384));
#12995=EDGE_LOOP('',(#54385,#54386,#54387,#54388));
#12996=EDGE_LOOP('',(#54389,#54390,#54391,#54392));
#12997=EDGE_LOOP('',(#54393,#54394,#54395,#54396));
#12998=EDGE_LOOP('',(#54397,#54398,#54399,#54400));
#12999=EDGE_LOOP('',(#54401,#54402,#54403,#54404));
#13000=EDGE_LOOP('',(#54405,#54406,#54407,#54408));
#13001=EDGE_LOOP('',(#54409,#54410,#54411,#54412));
#13002=EDGE_LOOP('',(#54413,#54414,#54415,#54416));
#13003=EDGE_LOOP('',(#54417,#54418,#54419,#54420));
#13004=EDGE_LOOP('',(#54421,#54422,#54423,#54424));
#13005=EDGE_LOOP('',(#54425,#54426,#54427,#54428));
#13006=EDGE_LOOP('',(#54429,#54430,#54431,#54432));
#13007=EDGE_LOOP('',(#54433,#54434,#54435,#54436));
#13008=EDGE_LOOP('',(#54437,#54438,#54439,#54440));
#13009=EDGE_LOOP('',(#54441,#54442,#54443,#54444));
#13010=EDGE_LOOP('',(#54445,#54446,#54447,#54448));
#13011=EDGE_LOOP('',(#54449,#54450,#54451,#54452));
#13012=EDGE_LOOP('',(#54453,#54454,#54455,#54456));
#13013=EDGE_LOOP('',(#54457,#54458,#54459,#54460));
#13014=EDGE_LOOP('',(#54461,#54462,#54463,#54464));
#13015=EDGE_LOOP('',(#54465,#54466,#54467,#54468));
#13016=EDGE_LOOP('',(#54469,#54470,#54471,#54472));
#13017=EDGE_LOOP('',(#54473,#54474,#54475,#54476));
#13018=EDGE_LOOP('',(#54477,#54478,#54479,#54480));
#13019=EDGE_LOOP('',(#54481,#54482,#54483,#54484));
#13020=EDGE_LOOP('',(#54485,#54486,#54487,#54488));
#13021=EDGE_LOOP('',(#54489,#54490,#54491,#54492));
#13022=EDGE_LOOP('',(#54493,#54494,#54495,#54496));
#13023=EDGE_LOOP('',(#54497,#54498,#54499,#54500));
#13024=EDGE_LOOP('',(#54501,#54502,#54503,#54504));
#13025=EDGE_LOOP('',(#54505,#54506,#54507,#54508));
#13026=EDGE_LOOP('',(#54509,#54510,#54511,#54512));
#13027=EDGE_LOOP('',(#54513,#54514,#54515,#54516));
#13028=EDGE_LOOP('',(#54517,#54518,#54519,#54520));
#13029=EDGE_LOOP('',(#54521,#54522,#54523,#54524));
#13030=EDGE_LOOP('',(#54525,#54526,#54527,#54528));
#13031=EDGE_LOOP('',(#54529,#54530,#54531,#54532));
#13032=EDGE_LOOP('',(#54533,#54534,#54535,#54536));
#13033=EDGE_LOOP('',(#54537,#54538,#54539,#54540));
#13034=EDGE_LOOP('',(#54541,#54542,#54543,#54544));
#13035=EDGE_LOOP('',(#54545,#54546,#54547,#54548));
#13036=EDGE_LOOP('',(#54549,#54550,#54551,#54552));
#13037=EDGE_LOOP('',(#54553,#54554,#54555,#54556));
#13038=EDGE_LOOP('',(#54557,#54558,#54559,#54560));
#13039=EDGE_LOOP('',(#54561,#54562,#54563,#54564));
#13040=EDGE_LOOP('',(#54565,#54566,#54567,#54568));
#13041=EDGE_LOOP('',(#54569,#54570,#54571,#54572));
#13042=EDGE_LOOP('',(#54573,#54574,#54575,#54576));
#13043=EDGE_LOOP('',(#54577,#54578,#54579,#54580));
#13044=EDGE_LOOP('',(#54581,#54582,#54583,#54584));
#13045=EDGE_LOOP('',(#54585,#54586,#54587,#54588));
#13046=EDGE_LOOP('',(#54589,#54590,#54591,#54592));
#13047=EDGE_LOOP('',(#54593,#54594,#54595,#54596));
#13048=EDGE_LOOP('',(#54597,#54598,#54599,#54600));
#13049=EDGE_LOOP('',(#54601,#54602,#54603,#54604));
#13050=EDGE_LOOP('',(#54605,#54606,#54607,#54608));
#13051=EDGE_LOOP('',(#54609,#54610,#54611,#54612));
#13052=EDGE_LOOP('',(#54613,#54614,#54615,#54616));
#13053=EDGE_LOOP('',(#54617,#54618,#54619,#54620));
#13054=EDGE_LOOP('',(#54621,#54622,#54623,#54624));
#13055=EDGE_LOOP('',(#54625,#54626,#54627,#54628));
#13056=EDGE_LOOP('',(#54629,#54630,#54631,#54632));
#13057=EDGE_LOOP('',(#54633,#54634,#54635,#54636));
#13058=EDGE_LOOP('',(#54637,#54638,#54639,#54640));
#13059=EDGE_LOOP('',(#54641,#54642,#54643,#54644));
#13060=EDGE_LOOP('',(#54645,#54646,#54647,#54648));
#13061=EDGE_LOOP('',(#54649,#54650,#54651,#54652));
#13062=EDGE_LOOP('',(#54653,#54654,#54655,#54656));
#13063=EDGE_LOOP('',(#54657,#54658,#54659,#54660));
#13064=EDGE_LOOP('',(#54661,#54662,#54663,#54664));
#13065=EDGE_LOOP('',(#54665,#54666,#54667,#54668));
#13066=EDGE_LOOP('',(#54669,#54670,#54671,#54672));
#13067=EDGE_LOOP('',(#54673,#54674,#54675,#54676));
#13068=EDGE_LOOP('',(#54677,#54678,#54679,#54680));
#13069=EDGE_LOOP('',(#54681,#54682,#54683,#54684));
#13070=EDGE_LOOP('',(#54685,#54686,#54687,#54688));
#13071=EDGE_LOOP('',(#54689,#54690,#54691,#54692));
#13072=EDGE_LOOP('',(#54693,#54694,#54695,#54696));
#13073=EDGE_LOOP('',(#54697,#54698,#54699,#54700));
#13074=EDGE_LOOP('',(#54701,#54702,#54703,#54704));
#13075=EDGE_LOOP('',(#54705,#54706,#54707,#54708));
#13076=EDGE_LOOP('',(#54709,#54710,#54711,#54712));
#13077=EDGE_LOOP('',(#54713,#54714,#54715,#54716));
#13078=EDGE_LOOP('',(#54717,#54718,#54719,#54720));
#13079=EDGE_LOOP('',(#54721,#54722,#54723,#54724));
#13080=EDGE_LOOP('',(#54725,#54726,#54727,#54728));
#13081=EDGE_LOOP('',(#54729,#54730,#54731,#54732));
#13082=EDGE_LOOP('',(#54733,#54734,#54735,#54736));
#13083=EDGE_LOOP('',(#54737,#54738,#54739,#54740));
#13084=EDGE_LOOP('',(#54741,#54742,#54743,#54744));
#13085=EDGE_LOOP('',(#54745,#54746,#54747,#54748));
#13086=EDGE_LOOP('',(#54749,#54750,#54751,#54752));
#13087=EDGE_LOOP('',(#54753,#54754,#54755,#54756));
#13088=EDGE_LOOP('',(#54757,#54758,#54759,#54760));
#13089=EDGE_LOOP('',(#54761,#54762,#54763,#54764));
#13090=EDGE_LOOP('',(#54765,#54766,#54767,#54768));
#13091=EDGE_LOOP('',(#54769,#54770,#54771,#54772));
#13092=EDGE_LOOP('',(#54773,#54774,#54775,#54776));
#13093=EDGE_LOOP('',(#54777,#54778,#54779,#54780));
#13094=EDGE_LOOP('',(#54781,#54782,#54783,#54784));
#13095=EDGE_LOOP('',(#54785,#54786,#54787,#54788));
#13096=EDGE_LOOP('',(#54789,#54790,#54791,#54792));
#13097=EDGE_LOOP('',(#54793,#54794,#54795,#54796));
#13098=EDGE_LOOP('',(#54797,#54798,#54799,#54800));
#13099=EDGE_LOOP('',(#54801,#54802,#54803,#54804));
#13100=EDGE_LOOP('',(#54805,#54806,#54807,#54808));
#13101=EDGE_LOOP('',(#54809,#54810,#54811,#54812));
#13102=EDGE_LOOP('',(#54813,#54814,#54815,#54816));
#13103=EDGE_LOOP('',(#54817,#54818,#54819,#54820));
#13104=EDGE_LOOP('',(#54821,#54822,#54823,#54824));
#13105=EDGE_LOOP('',(#54825,#54826,#54827,#54828));
#13106=EDGE_LOOP('',(#54829,#54830,#54831,#54832));
#13107=EDGE_LOOP('',(#54833,#54834,#54835,#54836));
#13108=EDGE_LOOP('',(#54837,#54838,#54839,#54840));
#13109=EDGE_LOOP('',(#54841,#54842,#54843,#54844));
#13110=EDGE_LOOP('',(#54845,#54846,#54847,#54848));
#13111=EDGE_LOOP('',(#54849,#54850,#54851,#54852));
#13112=EDGE_LOOP('',(#54853,#54854,#54855,#54856));
#13113=EDGE_LOOP('',(#54857,#54858,#54859,#54860));
#13114=EDGE_LOOP('',(#54861,#54862,#54863,#54864));
#13115=EDGE_LOOP('',(#54865,#54866,#54867,#54868));
#13116=EDGE_LOOP('',(#54869,#54870,#54871,#54872));
#13117=EDGE_LOOP('',(#54873,#54874,#54875,#54876));
#13118=EDGE_LOOP('',(#54877,#54878,#54879,#54880));
#13119=EDGE_LOOP('',(#54881,#54882,#54883,#54884));
#13120=EDGE_LOOP('',(#54885,#54886,#54887,#54888));
#13121=EDGE_LOOP('',(#54889,#54890,#54891,#54892));
#13122=EDGE_LOOP('',(#54893,#54894,#54895,#54896));
#13123=EDGE_LOOP('',(#54897,#54898,#54899,#54900));
#13124=EDGE_LOOP('',(#54901,#54902,#54903,#54904));
#13125=EDGE_LOOP('',(#54905,#54906,#54907,#54908));
#13126=EDGE_LOOP('',(#54909,#54910,#54911,#54912));
#13127=EDGE_LOOP('',(#54913,#54914,#54915,#54916));
#13128=EDGE_LOOP('',(#54917,#54918,#54919,#54920));
#13129=EDGE_LOOP('',(#54921,#54922,#54923,#54924));
#13130=EDGE_LOOP('',(#54925,#54926,#54927,#54928));
#13131=EDGE_LOOP('',(#54929,#54930,#54931,#54932));
#13132=EDGE_LOOP('',(#54933,#54934,#54935,#54936));
#13133=EDGE_LOOP('',(#54937,#54938,#54939,#54940));
#13134=EDGE_LOOP('',(#54941,#54942,#54943,#54944));
#13135=EDGE_LOOP('',(#54945,#54946,#54947,#54948));
#13136=EDGE_LOOP('',(#54949,#54950,#54951,#54952));
#13137=EDGE_LOOP('',(#54953,#54954,#54955,#54956));
#13138=EDGE_LOOP('',(#54957,#54958,#54959,#54960));
#13139=EDGE_LOOP('',(#54961,#54962,#54963,#54964));
#13140=EDGE_LOOP('',(#54965,#54966,#54967,#54968));
#13141=EDGE_LOOP('',(#54969,#54970,#54971,#54972));
#13142=EDGE_LOOP('',(#54973,#54974,#54975,#54976));
#13143=EDGE_LOOP('',(#54977,#54978,#54979,#54980));
#13144=EDGE_LOOP('',(#54981,#54982,#54983,#54984));
#13145=EDGE_LOOP('',(#54985,#54986,#54987,#54988));
#13146=EDGE_LOOP('',(#54989,#54990,#54991,#54992));
#13147=EDGE_LOOP('',(#54993,#54994,#54995,#54996));
#13148=EDGE_LOOP('',(#54997,#54998,#54999,#55000));
#13149=EDGE_LOOP('',(#55001,#55002,#55003,#55004));
#13150=EDGE_LOOP('',(#55005,#55006,#55007,#55008));
#13151=EDGE_LOOP('',(#55009,#55010,#55011,#55012));
#13152=EDGE_LOOP('',(#55013,#55014,#55015,#55016));
#13153=EDGE_LOOP('',(#55017,#55018,#55019,#55020));
#13154=EDGE_LOOP('',(#55021,#55022,#55023,#55024));
#13155=EDGE_LOOP('',(#55025,#55026,#55027,#55028));
#13156=EDGE_LOOP('',(#55029,#55030,#55031,#55032));
#13157=EDGE_LOOP('',(#55033,#55034,#55035,#55036));
#13158=EDGE_LOOP('',(#55037,#55038,#55039,#55040));
#13159=EDGE_LOOP('',(#55041,#55042,#55043,#55044));
#13160=EDGE_LOOP('',(#55045,#55046,#55047,#55048));
#13161=EDGE_LOOP('',(#55049,#55050,#55051,#55052));
#13162=EDGE_LOOP('',(#55053,#55054,#55055,#55056));
#13163=EDGE_LOOP('',(#55057,#55058,#55059,#55060));
#13164=EDGE_LOOP('',(#55061,#55062,#55063,#55064));
#13165=EDGE_LOOP('',(#55065,#55066,#55067,#55068));
#13166=EDGE_LOOP('',(#55069,#55070,#55071,#55072));
#13167=EDGE_LOOP('',(#55073,#55074,#55075,#55076));
#13168=EDGE_LOOP('',(#55077,#55078,#55079,#55080));
#13169=EDGE_LOOP('',(#55081,#55082,#55083,#55084));
#13170=EDGE_LOOP('',(#55085,#55086,#55087,#55088));
#13171=EDGE_LOOP('',(#55089,#55090,#55091,#55092));
#13172=EDGE_LOOP('',(#55093,#55094,#55095,#55096));
#13173=EDGE_LOOP('',(#55097,#55098,#55099,#55100));
#13174=EDGE_LOOP('',(#55101,#55102,#55103,#55104));
#13175=EDGE_LOOP('',(#55105,#55106,#55107,#55108));
#13176=EDGE_LOOP('',(#55109,#55110,#55111,#55112));
#13177=EDGE_LOOP('',(#55113,#55114,#55115,#55116));
#13178=EDGE_LOOP('',(#55117,#55118,#55119,#55120));
#13179=EDGE_LOOP('',(#55121,#55122,#55123,#55124));
#13180=EDGE_LOOP('',(#55125,#55126,#55127,#55128));
#13181=EDGE_LOOP('',(#55129,#55130,#55131,#55132));
#13182=EDGE_LOOP('',(#55133,#55134,#55135,#55136));
#13183=EDGE_LOOP('',(#55137,#55138,#55139,#55140));
#13184=EDGE_LOOP('',(#55141,#55142,#55143,#55144));
#13185=EDGE_LOOP('',(#55145,#55146,#55147,#55148));
#13186=EDGE_LOOP('',(#55149,#55150,#55151,#55152));
#13187=EDGE_LOOP('',(#55153,#55154,#55155,#55156));
#13188=EDGE_LOOP('',(#55157,#55158,#55159,#55160));
#13189=EDGE_LOOP('',(#55161,#55162,#55163,#55164));
#13190=EDGE_LOOP('',(#55165,#55166,#55167,#55168));
#13191=EDGE_LOOP('',(#55169,#55170,#55171,#55172));
#13192=EDGE_LOOP('',(#55173,#55174,#55175,#55176));
#13193=EDGE_LOOP('',(#55177,#55178,#55179,#55180));
#13194=EDGE_LOOP('',(#55181,#55182,#55183,#55184));
#13195=EDGE_LOOP('',(#55185,#55186,#55187,#55188));
#13196=EDGE_LOOP('',(#55189,#55190,#55191,#55192));
#13197=EDGE_LOOP('',(#55193,#55194,#55195,#55196));
#13198=EDGE_LOOP('',(#55197,#55198,#55199,#55200));
#13199=EDGE_LOOP('',(#55201,#55202,#55203,#55204));
#13200=EDGE_LOOP('',(#55205,#55206,#55207,#55208));
#13201=EDGE_LOOP('',(#55209,#55210,#55211,#55212));
#13202=EDGE_LOOP('',(#55213,#55214,#55215,#55216));
#13203=EDGE_LOOP('',(#55217,#55218,#55219,#55220));
#13204=EDGE_LOOP('',(#55221,#55222,#55223,#55224));
#13205=EDGE_LOOP('',(#55225,#55226,#55227,#55228));
#13206=EDGE_LOOP('',(#55229,#55230,#55231,#55232));
#13207=EDGE_LOOP('',(#55233,#55234,#55235,#55236));
#13208=EDGE_LOOP('',(#55237,#55238,#55239,#55240));
#13209=EDGE_LOOP('',(#55241,#55242,#55243,#55244));
#13210=EDGE_LOOP('',(#55245,#55246,#55247,#55248));
#13211=EDGE_LOOP('',(#55249,#55250,#55251,#55252));
#13212=EDGE_LOOP('',(#55253,#55254,#55255,#55256));
#13213=EDGE_LOOP('',(#55257,#55258,#55259,#55260));
#13214=EDGE_LOOP('',(#55261,#55262,#55263,#55264));
#13215=EDGE_LOOP('',(#55265,#55266,#55267,#55268));
#13216=EDGE_LOOP('',(#55269,#55270,#55271,#55272));
#13217=EDGE_LOOP('',(#55273,#55274,#55275,#55276));
#13218=EDGE_LOOP('',(#55277,#55278,#55279,#55280));
#13219=EDGE_LOOP('',(#55281,#55282,#55283,#55284));
#13220=EDGE_LOOP('',(#55285,#55286,#55287,#55288));
#13221=EDGE_LOOP('',(#55289,#55290,#55291,#55292));
#13222=EDGE_LOOP('',(#55293,#55294,#55295,#55296));
#13223=EDGE_LOOP('',(#55297,#55298,#55299,#55300));
#13224=EDGE_LOOP('',(#55301,#55302,#55303,#55304));
#13225=EDGE_LOOP('',(#55305,#55306,#55307,#55308));
#13226=EDGE_LOOP('',(#55309,#55310,#55311,#55312));
#13227=EDGE_LOOP('',(#55313,#55314,#55315,#55316));
#13228=EDGE_LOOP('',(#55317,#55318,#55319,#55320));
#13229=EDGE_LOOP('',(#55321,#55322,#55323,#55324));
#13230=EDGE_LOOP('',(#55325,#55326,#55327,#55328));
#13231=EDGE_LOOP('',(#55329,#55330,#55331,#55332));
#13232=EDGE_LOOP('',(#55333,#55334,#55335,#55336));
#13233=EDGE_LOOP('',(#55337,#55338,#55339,#55340));
#13234=EDGE_LOOP('',(#55341,#55342,#55343,#55344));
#13235=EDGE_LOOP('',(#55345,#55346,#55347,#55348));
#13236=EDGE_LOOP('',(#55349,#55350,#55351,#55352));
#13237=EDGE_LOOP('',(#55353,#55354,#55355,#55356));
#13238=EDGE_LOOP('',(#55357,#55358,#55359,#55360));
#13239=EDGE_LOOP('',(#55361,#55362,#55363,#55364));
#13240=EDGE_LOOP('',(#55365,#55366,#55367,#55368));
#13241=EDGE_LOOP('',(#55369,#55370,#55371,#55372));
#13242=EDGE_LOOP('',(#55373,#55374,#55375,#55376));
#13243=EDGE_LOOP('',(#55377,#55378,#55379,#55380));
#13244=EDGE_LOOP('',(#55381,#55382,#55383,#55384));
#13245=EDGE_LOOP('',(#55385,#55386,#55387,#55388));
#13246=EDGE_LOOP('',(#55389,#55390,#55391,#55392));
#13247=EDGE_LOOP('',(#55393,#55394,#55395,#55396));
#13248=EDGE_LOOP('',(#55397,#55398,#55399,#55400));
#13249=EDGE_LOOP('',(#55401,#55402,#55403,#55404));
#13250=EDGE_LOOP('',(#55405,#55406,#55407,#55408));
#13251=EDGE_LOOP('',(#55409,#55410,#55411,#55412));
#13252=EDGE_LOOP('',(#55413,#55414,#55415,#55416));
#13253=EDGE_LOOP('',(#55417,#55418,#55419,#55420));
#13254=EDGE_LOOP('',(#55421,#55422,#55423,#55424));
#13255=EDGE_LOOP('',(#55425,#55426,#55427,#55428));
#13256=EDGE_LOOP('',(#55429,#55430,#55431,#55432));
#13257=EDGE_LOOP('',(#55433,#55434,#55435,#55436));
#13258=EDGE_LOOP('',(#55437,#55438,#55439,#55440));
#13259=EDGE_LOOP('',(#55441,#55442,#55443,#55444));
#13260=EDGE_LOOP('',(#55445,#55446,#55447,#55448));
#13261=EDGE_LOOP('',(#55449,#55450,#55451,#55452));
#13262=EDGE_LOOP('',(#55453,#55454,#55455,#55456));
#13263=EDGE_LOOP('',(#55457,#55458,#55459,#55460));
#13264=EDGE_LOOP('',(#55461,#55462,#55463,#55464));
#13265=EDGE_LOOP('',(#55465,#55466,#55467,#55468));
#13266=EDGE_LOOP('',(#55469,#55470,#55471,#55472));
#13267=EDGE_LOOP('',(#55473,#55474,#55475,#55476));
#13268=EDGE_LOOP('',(#55477,#55478,#55479,#55480));
#13269=EDGE_LOOP('',(#55481,#55482,#55483,#55484));
#13270=EDGE_LOOP('',(#55485,#55486,#55487,#55488));
#13271=EDGE_LOOP('',(#55489,#55490,#55491,#55492));
#13272=EDGE_LOOP('',(#55493,#55494,#55495,#55496));
#13273=EDGE_LOOP('',(#55497,#55498,#55499,#55500));
#13274=EDGE_LOOP('',(#55501,#55502,#55503,#55504));
#13275=EDGE_LOOP('',(#55505,#55506,#55507,#55508));
#13276=EDGE_LOOP('',(#55509,#55510,#55511,#55512));
#13277=EDGE_LOOP('',(#55513,#55514,#55515,#55516));
#13278=EDGE_LOOP('',(#55517,#55518,#55519,#55520));
#13279=EDGE_LOOP('',(#55521,#55522,#55523,#55524));
#13280=EDGE_LOOP('',(#55525,#55526,#55527,#55528));
#13281=EDGE_LOOP('',(#55529,#55530,#55531,#55532));
#13282=EDGE_LOOP('',(#55533,#55534,#55535,#55536));
#13283=EDGE_LOOP('',(#55537,#55538,#55539,#55540));
#13284=EDGE_LOOP('',(#55541,#55542,#55543,#55544));
#13285=EDGE_LOOP('',(#55545,#55546,#55547,#55548));
#13286=EDGE_LOOP('',(#55549,#55550,#55551,#55552));
#13287=EDGE_LOOP('',(#55553,#55554,#55555,#55556));
#13288=EDGE_LOOP('',(#55557,#55558,#55559,#55560));
#13289=EDGE_LOOP('',(#55561,#55562,#55563,#55564));
#13290=EDGE_LOOP('',(#55565,#55566,#55567,#55568));
#13291=EDGE_LOOP('',(#55569,#55570,#55571,#55572));
#13292=EDGE_LOOP('',(#55573,#55574,#55575,#55576));
#13293=EDGE_LOOP('',(#55577,#55578,#55579,#55580));
#13294=EDGE_LOOP('',(#55581,#55582,#55583,#55584));
#13295=EDGE_LOOP('',(#55585,#55586,#55587,#55588));
#13296=EDGE_LOOP('',(#55589,#55590,#55591,#55592));
#13297=EDGE_LOOP('',(#55593,#55594,#55595,#55596));
#13298=EDGE_LOOP('',(#55597,#55598,#55599,#55600));
#13299=EDGE_LOOP('',(#55601,#55602,#55603,#55604));
#13300=EDGE_LOOP('',(#55605,#55606,#55607,#55608));
#13301=EDGE_LOOP('',(#55609,#55610,#55611,#55612));
#13302=EDGE_LOOP('',(#55613,#55614,#55615,#55616));
#13303=EDGE_LOOP('',(#55617,#55618,#55619,#55620));
#13304=EDGE_LOOP('',(#55621,#55622,#55623,#55624));
#13305=EDGE_LOOP('',(#55625,#55626,#55627,#55628));
#13306=EDGE_LOOP('',(#55629,#55630,#55631,#55632));
#13307=EDGE_LOOP('',(#55633,#55634,#55635,#55636));
#13308=EDGE_LOOP('',(#55637,#55638,#55639,#55640));
#13309=EDGE_LOOP('',(#55641,#55642,#55643,#55644));
#13310=EDGE_LOOP('',(#55645,#55646,#55647,#55648));
#13311=EDGE_LOOP('',(#55649,#55650,#55651,#55652));
#13312=EDGE_LOOP('',(#55653,#55654,#55655,#55656));
#13313=EDGE_LOOP('',(#55657,#55658,#55659,#55660));
#13314=EDGE_LOOP('',(#55661,#55662,#55663,#55664));
#13315=EDGE_LOOP('',(#55665,#55666,#55667,#55668));
#13316=EDGE_LOOP('',(#55669,#55670,#55671,#55672));
#13317=EDGE_LOOP('',(#55673,#55674,#55675,#55676));
#13318=EDGE_LOOP('',(#55677,#55678,#55679,#55680));
#13319=EDGE_LOOP('',(#55681,#55682,#55683,#55684));
#13320=EDGE_LOOP('',(#55685,#55686,#55687,#55688));
#13321=EDGE_LOOP('',(#55689,#55690,#55691,#55692));
#13322=EDGE_LOOP('',(#55693,#55694,#55695,#55696));
#13323=EDGE_LOOP('',(#55697,#55698,#55699,#55700));
#13324=EDGE_LOOP('',(#55701,#55702,#55703,#55704));
#13325=EDGE_LOOP('',(#55705,#55706,#55707,#55708));
#13326=EDGE_LOOP('',(#55709,#55710,#55711,#55712));
#13327=EDGE_LOOP('',(#55713,#55714,#55715,#55716));
#13328=EDGE_LOOP('',(#55717,#55718,#55719,#55720));
#13329=EDGE_LOOP('',(#55721,#55722,#55723,#55724));
#13330=EDGE_LOOP('',(#55725,#55726,#55727,#55728));
#13331=EDGE_LOOP('',(#55729,#55730,#55731,#55732));
#13332=EDGE_LOOP('',(#55733,#55734,#55735,#55736));
#13333=EDGE_LOOP('',(#55737,#55738,#55739,#55740));
#13334=EDGE_LOOP('',(#55741,#55742,#55743,#55744));
#13335=EDGE_LOOP('',(#55745,#55746,#55747,#55748));
#13336=EDGE_LOOP('',(#55749,#55750,#55751,#55752));
#13337=EDGE_LOOP('',(#55753,#55754,#55755,#55756));
#13338=EDGE_LOOP('',(#55757,#55758,#55759,#55760));
#13339=EDGE_LOOP('',(#55761,#55762,#55763,#55764));
#13340=EDGE_LOOP('',(#55765,#55766,#55767,#55768));
#13341=EDGE_LOOP('',(#55769,#55770,#55771,#55772));
#13342=EDGE_LOOP('',(#55773,#55774,#55775,#55776));
#13343=EDGE_LOOP('',(#55777,#55778,#55779,#55780));
#13344=EDGE_LOOP('',(#55781,#55782,#55783,#55784));
#13345=EDGE_LOOP('',(#55785,#55786,#55787,#55788));
#13346=EDGE_LOOP('',(#55789,#55790,#55791,#55792));
#13347=EDGE_LOOP('',(#55793,#55794,#55795,#55796));
#13348=EDGE_LOOP('',(#55797,#55798,#55799,#55800));
#13349=EDGE_LOOP('',(#55801,#55802,#55803,#55804));
#13350=EDGE_LOOP('',(#55805,#55806,#55807,#55808));
#13351=EDGE_LOOP('',(#55809,#55810,#55811,#55812));
#13352=EDGE_LOOP('',(#55813,#55814,#55815,#55816));
#13353=EDGE_LOOP('',(#55817,#55818,#55819,#55820));
#13354=EDGE_LOOP('',(#55821,#55822,#55823,#55824));
#13355=EDGE_LOOP('',(#55825,#55826,#55827,#55828));
#13356=EDGE_LOOP('',(#55829,#55830,#55831,#55832));
#13357=EDGE_LOOP('',(#55833,#55834,#55835,#55836));
#13358=EDGE_LOOP('',(#55837,#55838,#55839,#55840));
#13359=EDGE_LOOP('',(#55841,#55842,#55843,#55844));
#13360=EDGE_LOOP('',(#55845,#55846,#55847,#55848));
#13361=EDGE_LOOP('',(#55849,#55850,#55851,#55852));
#13362=EDGE_LOOP('',(#55853,#55854,#55855,#55856));
#13363=EDGE_LOOP('',(#55857,#55858,#55859,#55860));
#13364=EDGE_LOOP('',(#55861,#55862,#55863,#55864));
#13365=EDGE_LOOP('',(#55865,#55866,#55867,#55868));
#13366=EDGE_LOOP('',(#55869,#55870,#55871,#55872));
#13367=EDGE_LOOP('',(#55873,#55874,#55875,#55876));
#13368=EDGE_LOOP('',(#55877,#55878,#55879,#55880));
#13369=EDGE_LOOP('',(#55881,#55882,#55883,#55884));
#13370=EDGE_LOOP('',(#55885,#55886,#55887,#55888));
#13371=EDGE_LOOP('',(#55889,#55890,#55891,#55892));
#13372=EDGE_LOOP('',(#55893,#55894,#55895,#55896));
#13373=EDGE_LOOP('',(#55897,#55898,#55899,#55900));
#13374=EDGE_LOOP('',(#55901,#55902,#55903,#55904));
#13375=EDGE_LOOP('',(#55905,#55906,#55907,#55908));
#13376=EDGE_LOOP('',(#55909,#55910,#55911,#55912));
#13377=EDGE_LOOP('',(#55913,#55914,#55915,#55916));
#13378=EDGE_LOOP('',(#55917,#55918,#55919,#55920));
#13379=EDGE_LOOP('',(#55921,#55922,#55923,#55924));
#13380=EDGE_LOOP('',(#55925,#55926,#55927,#55928));
#13381=EDGE_LOOP('',(#55929,#55930,#55931,#55932));
#13382=EDGE_LOOP('',(#55933,#55934,#55935,#55936));
#13383=EDGE_LOOP('',(#55937,#55938,#55939,#55940));
#13384=EDGE_LOOP('',(#55941,#55942,#55943,#55944));
#13385=EDGE_LOOP('',(#55945,#55946,#55947,#55948));
#13386=EDGE_LOOP('',(#55949,#55950,#55951,#55952));
#13387=EDGE_LOOP('',(#55953,#55954,#55955,#55956));
#13388=EDGE_LOOP('',(#55957,#55958,#55959,#55960));
#13389=EDGE_LOOP('',(#55961,#55962,#55963,#55964));
#13390=EDGE_LOOP('',(#55965,#55966,#55967,#55968));
#13391=EDGE_LOOP('',(#55969,#55970,#55971,#55972));
#13392=EDGE_LOOP('',(#55973,#55974,#55975,#55976));
#13393=EDGE_LOOP('',(#55977,#55978,#55979,#55980));
#13394=EDGE_LOOP('',(#55981,#55982,#55983,#55984));
#13395=EDGE_LOOP('',(#55985,#55986,#55987,#55988));
#13396=EDGE_LOOP('',(#55989,#55990,#55991,#55992));
#13397=EDGE_LOOP('',(#55993,#55994,#55995,#55996));
#13398=EDGE_LOOP('',(#55997,#55998,#55999,#56000));
#13399=EDGE_LOOP('',(#56001,#56002,#56003,#56004));
#13400=EDGE_LOOP('',(#56005,#56006,#56007,#56008));
#13401=EDGE_LOOP('',(#56009,#56010,#56011,#56012));
#13402=EDGE_LOOP('',(#56013,#56014,#56015,#56016));
#13403=EDGE_LOOP('',(#56017,#56018,#56019,#56020));
#13404=EDGE_LOOP('',(#56021,#56022,#56023,#56024));
#13405=EDGE_LOOP('',(#56025,#56026,#56027,#56028));
#13406=EDGE_LOOP('',(#56029,#56030,#56031,#56032));
#13407=EDGE_LOOP('',(#56033,#56034,#56035,#56036));
#13408=EDGE_LOOP('',(#56037,#56038,#56039,#56040));
#13409=EDGE_LOOP('',(#56041,#56042,#56043,#56044));
#13410=EDGE_LOOP('',(#56045,#56046,#56047,#56048));
#13411=EDGE_LOOP('',(#56049,#56050,#56051,#56052));
#13412=EDGE_LOOP('',(#56053,#56054,#56055,#56056));
#13413=EDGE_LOOP('',(#56057,#56058,#56059,#56060));
#13414=EDGE_LOOP('',(#56061,#56062,#56063,#56064));
#13415=EDGE_LOOP('',(#56065,#56066,#56067,#56068));
#13416=EDGE_LOOP('',(#56069,#56070,#56071,#56072));
#13417=EDGE_LOOP('',(#56073,#56074,#56075,#56076));
#13418=EDGE_LOOP('',(#56077,#56078,#56079,#56080));
#13419=EDGE_LOOP('',(#56081,#56082,#56083,#56084));
#13420=EDGE_LOOP('',(#56085,#56086,#56087,#56088));
#13421=EDGE_LOOP('',(#56089,#56090,#56091,#56092));
#13422=EDGE_LOOP('',(#56093,#56094,#56095,#56096));
#13423=EDGE_LOOP('',(#56097,#56098,#56099,#56100));
#13424=EDGE_LOOP('',(#56101,#56102,#56103,#56104));
#13425=EDGE_LOOP('',(#56105,#56106,#56107,#56108));
#13426=EDGE_LOOP('',(#56109,#56110,#56111,#56112));
#13427=EDGE_LOOP('',(#56113,#56114,#56115,#56116));
#13428=EDGE_LOOP('',(#56117,#56118,#56119,#56120));
#13429=EDGE_LOOP('',(#56121,#56122,#56123,#56124));
#13430=EDGE_LOOP('',(#56125,#56126,#56127,#56128));
#13431=EDGE_LOOP('',(#56129,#56130,#56131,#56132));
#13432=EDGE_LOOP('',(#56133,#56134,#56135,#56136));
#13433=EDGE_LOOP('',(#56137,#56138,#56139,#56140));
#13434=EDGE_LOOP('',(#56141,#56142,#56143,#56144));
#13435=EDGE_LOOP('',(#56145,#56146,#56147,#56148));
#13436=EDGE_LOOP('',(#56149,#56150,#56151,#56152));
#13437=EDGE_LOOP('',(#56153,#56154,#56155,#56156));
#13438=EDGE_LOOP('',(#56157,#56158,#56159,#56160));
#13439=EDGE_LOOP('',(#56161,#56162,#56163,#56164));
#13440=EDGE_LOOP('',(#56165,#56166,#56167,#56168));
#13441=EDGE_LOOP('',(#56169,#56170,#56171,#56172));
#13442=EDGE_LOOP('',(#56173,#56174,#56175,#56176));
#13443=EDGE_LOOP('',(#56177,#56178,#56179,#56180));
#13444=EDGE_LOOP('',(#56181,#56182,#56183,#56184));
#13445=EDGE_LOOP('',(#56185,#56186,#56187,#56188));
#13446=EDGE_LOOP('',(#56189,#56190,#56191,#56192));
#13447=EDGE_LOOP('',(#56193,#56194,#56195,#56196));
#13448=EDGE_LOOP('',(#56197,#56198,#56199,#56200));
#13449=EDGE_LOOP('',(#56201,#56202,#56203,#56204));
#13450=EDGE_LOOP('',(#56205,#56206,#56207,#56208));
#13451=EDGE_LOOP('',(#56209,#56210,#56211,#56212));
#13452=EDGE_LOOP('',(#56213,#56214,#56215,#56216));
#13453=EDGE_LOOP('',(#56217,#56218,#56219,#56220));
#13454=EDGE_LOOP('',(#56221,#56222,#56223,#56224));
#13455=EDGE_LOOP('',(#56225,#56226,#56227,#56228));
#13456=EDGE_LOOP('',(#56229,#56230,#56231,#56232));
#13457=EDGE_LOOP('',(#56233,#56234,#56235,#56236));
#13458=EDGE_LOOP('',(#56237,#56238,#56239,#56240));
#13459=EDGE_LOOP('',(#56241,#56242,#56243,#56244));
#13460=EDGE_LOOP('',(#56245,#56246,#56247,#56248));
#13461=EDGE_LOOP('',(#56249,#56250,#56251,#56252));
#13462=EDGE_LOOP('',(#56253,#56254,#56255,#56256));
#13463=EDGE_LOOP('',(#56257,#56258,#56259,#56260));
#13464=EDGE_LOOP('',(#56261,#56262,#56263,#56264));
#13465=EDGE_LOOP('',(#56265,#56266,#56267,#56268));
#13466=EDGE_LOOP('',(#56269,#56270,#56271,#56272));
#13467=EDGE_LOOP('',(#56273,#56274,#56275,#56276));
#13468=EDGE_LOOP('',(#56277,#56278,#56279,#56280));
#13469=EDGE_LOOP('',(#56281,#56282,#56283,#56284));
#13470=EDGE_LOOP('',(#56285,#56286,#56287,#56288));
#13471=EDGE_LOOP('',(#56289,#56290,#56291,#56292));
#13472=EDGE_LOOP('',(#56293,#56294,#56295,#56296));
#13473=EDGE_LOOP('',(#56297,#56298,#56299,#56300));
#13474=EDGE_LOOP('',(#56301,#56302,#56303,#56304));
#13475=EDGE_LOOP('',(#56305,#56306,#56307,#56308));
#13476=EDGE_LOOP('',(#56309,#56310,#56311,#56312));
#13477=EDGE_LOOP('',(#56313,#56314,#56315,#56316));
#13478=EDGE_LOOP('',(#56317,#56318,#56319,#56320));
#13479=EDGE_LOOP('',(#56321,#56322,#56323,#56324));
#13480=EDGE_LOOP('',(#56325,#56326,#56327,#56328));
#13481=EDGE_LOOP('',(#56329,#56330,#56331,#56332));
#13482=EDGE_LOOP('',(#56333,#56334,#56335,#56336));
#13483=EDGE_LOOP('',(#56337,#56338,#56339,#56340));
#13484=EDGE_LOOP('',(#56341,#56342,#56343,#56344));
#13485=EDGE_LOOP('',(#56345,#56346,#56347,#56348));
#13486=EDGE_LOOP('',(#56349,#56350,#56351,#56352));
#13487=EDGE_LOOP('',(#56353,#56354,#56355,#56356));
#13488=EDGE_LOOP('',(#56357,#56358,#56359,#56360));
#13489=EDGE_LOOP('',(#56361,#56362,#56363,#56364));
#13490=EDGE_LOOP('',(#56365,#56366,#56367,#56368));
#13491=EDGE_LOOP('',(#56369,#56370,#56371,#56372));
#13492=EDGE_LOOP('',(#56373,#56374,#56375,#56376));
#13493=EDGE_LOOP('',(#56377,#56378,#56379,#56380));
#13494=EDGE_LOOP('',(#56381,#56382,#56383,#56384));
#13495=EDGE_LOOP('',(#56385,#56386,#56387,#56388));
#13496=EDGE_LOOP('',(#56389,#56390,#56391,#56392));
#13497=EDGE_LOOP('',(#56393,#56394,#56395,#56396));
#13498=EDGE_LOOP('',(#56397,#56398,#56399,#56400));
#13499=EDGE_LOOP('',(#56401,#56402,#56403,#56404));
#13500=EDGE_LOOP('',(#56405,#56406,#56407,#56408));
#13501=EDGE_LOOP('',(#56409,#56410,#56411,#56412));
#13502=EDGE_LOOP('',(#56413,#56414,#56415,#56416));
#13503=EDGE_LOOP('',(#56417,#56418,#56419,#56420));
#13504=EDGE_LOOP('',(#56421,#56422,#56423,#56424));
#13505=EDGE_LOOP('',(#56425,#56426,#56427,#56428));
#13506=EDGE_LOOP('',(#56429,#56430,#56431,#56432));
#13507=EDGE_LOOP('',(#56433,#56434,#56435,#56436));
#13508=EDGE_LOOP('',(#56437,#56438,#56439,#56440));
#13509=EDGE_LOOP('',(#56441,#56442,#56443,#56444));
#13510=EDGE_LOOP('',(#56445,#56446,#56447,#56448));
#13511=EDGE_LOOP('',(#56449,#56450,#56451,#56452));
#13512=EDGE_LOOP('',(#56453,#56454,#56455,#56456));
#13513=EDGE_LOOP('',(#56457,#56458,#56459,#56460));
#13514=EDGE_LOOP('',(#56461,#56462,#56463,#56464));
#13515=EDGE_LOOP('',(#56465,#56466,#56467,#56468));
#13516=EDGE_LOOP('',(#56469,#56470,#56471,#56472));
#13517=EDGE_LOOP('',(#56473,#56474,#56475,#56476));
#13518=EDGE_LOOP('',(#56477,#56478,#56479,#56480));
#13519=EDGE_LOOP('',(#56481,#56482,#56483,#56484));
#13520=EDGE_LOOP('',(#56485,#56486,#56487,#56488));
#13521=EDGE_LOOP('',(#56489,#56490,#56491,#56492));
#13522=EDGE_LOOP('',(#56493,#56494,#56495,#56496));
#13523=EDGE_LOOP('',(#56497,#56498,#56499,#56500));
#13524=EDGE_LOOP('',(#56501,#56502,#56503,#56504));
#13525=EDGE_LOOP('',(#56505,#56506,#56507,#56508));
#13526=EDGE_LOOP('',(#56509,#56510,#56511,#56512));
#13527=EDGE_LOOP('',(#56513,#56514,#56515,#56516));
#13528=EDGE_LOOP('',(#56517,#56518,#56519,#56520));
#13529=EDGE_LOOP('',(#56521,#56522,#56523,#56524));
#13530=EDGE_LOOP('',(#56525,#56526,#56527,#56528));
#13531=EDGE_LOOP('',(#56529,#56530,#56531,#56532));
#13532=EDGE_LOOP('',(#56533,#56534,#56535,#56536));
#13533=EDGE_LOOP('',(#56537,#56538,#56539,#56540));
#13534=EDGE_LOOP('',(#56541,#56542,#56543,#56544));
#13535=EDGE_LOOP('',(#56545,#56546,#56547,#56548));
#13536=EDGE_LOOP('',(#56549,#56550,#56551,#56552));
#13537=EDGE_LOOP('',(#56553,#56554,#56555,#56556));
#13538=EDGE_LOOP('',(#56557,#56558,#56559,#56560));
#13539=EDGE_LOOP('',(#56561,#56562,#56563,#56564));
#13540=EDGE_LOOP('',(#56565,#56566,#56567,#56568));
#13541=EDGE_LOOP('',(#56569,#56570,#56571,#56572));
#13542=EDGE_LOOP('',(#56573,#56574,#56575,#56576));
#13543=EDGE_LOOP('',(#56577,#56578,#56579,#56580));
#13544=EDGE_LOOP('',(#56581,#56582,#56583,#56584));
#13545=EDGE_LOOP('',(#56585,#56586,#56587,#56588));
#13546=EDGE_LOOP('',(#56589,#56590,#56591,#56592));
#13547=EDGE_LOOP('',(#56593,#56594,#56595,#56596));
#13548=EDGE_LOOP('',(#56597,#56598,#56599,#56600));
#13549=EDGE_LOOP('',(#56601,#56602,#56603,#56604));
#13550=EDGE_LOOP('',(#56605,#56606,#56607,#56608));
#13551=EDGE_LOOP('',(#56609,#56610,#56611,#56612));
#13552=EDGE_LOOP('',(#56613,#56614,#56615,#56616));
#13553=EDGE_LOOP('',(#56617,#56618,#56619,#56620));
#13554=EDGE_LOOP('',(#56621,#56622,#56623,#56624));
#13555=EDGE_LOOP('',(#56625,#56626,#56627,#56628));
#13556=EDGE_LOOP('',(#56629,#56630,#56631,#56632));
#13557=EDGE_LOOP('',(#56633,#56634,#56635,#56636));
#13558=EDGE_LOOP('',(#56637,#56638,#56639,#56640));
#13559=EDGE_LOOP('',(#56641,#56642,#56643,#56644));
#13560=EDGE_LOOP('',(#56645,#56646,#56647,#56648));
#13561=EDGE_LOOP('',(#56649,#56650,#56651,#56652));
#13562=EDGE_LOOP('',(#56653,#56654,#56655,#56656));
#13563=EDGE_LOOP('',(#56657,#56658,#56659,#56660));
#13564=EDGE_LOOP('',(#56661,#56662,#56663,#56664));
#13565=EDGE_LOOP('',(#56665,#56666,#56667,#56668));
#13566=EDGE_LOOP('',(#56669,#56670,#56671,#56672));
#13567=EDGE_LOOP('',(#56673,#56674,#56675,#56676));
#13568=EDGE_LOOP('',(#56677,#56678,#56679,#56680));
#13569=EDGE_LOOP('',(#56681,#56682,#56683,#56684));
#13570=EDGE_LOOP('',(#56685,#56686,#56687,#56688));
#13571=EDGE_LOOP('',(#56689,#56690,#56691,#56692));
#13572=EDGE_LOOP('',(#56693,#56694,#56695,#56696));
#13573=EDGE_LOOP('',(#56697,#56698,#56699,#56700));
#13574=EDGE_LOOP('',(#56701,#56702,#56703,#56704));
#13575=EDGE_LOOP('',(#56705,#56706,#56707,#56708));
#13576=EDGE_LOOP('',(#56709,#56710,#56711,#56712));
#13577=EDGE_LOOP('',(#56713,#56714,#56715,#56716));
#13578=EDGE_LOOP('',(#56717,#56718,#56719,#56720));
#13579=EDGE_LOOP('',(#56721,#56722,#56723,#56724));
#13580=EDGE_LOOP('',(#56725,#56726,#56727,#56728));
#13581=EDGE_LOOP('',(#56729,#56730,#56731,#56732));
#13582=EDGE_LOOP('',(#56733,#56734,#56735,#56736));
#13583=EDGE_LOOP('',(#56737,#56738,#56739,#56740));
#13584=EDGE_LOOP('',(#56741,#56742,#56743,#56744));
#13585=EDGE_LOOP('',(#56745,#56746,#56747,#56748));
#13586=EDGE_LOOP('',(#56749,#56750,#56751,#56752));
#13587=EDGE_LOOP('',(#56753,#56754,#56755,#56756));
#13588=EDGE_LOOP('',(#56757,#56758,#56759,#56760));
#13589=EDGE_LOOP('',(#56761,#56762,#56763,#56764));
#13590=EDGE_LOOP('',(#56765,#56766,#56767,#56768));
#13591=EDGE_LOOP('',(#56769,#56770,#56771,#56772));
#13592=EDGE_LOOP('',(#56773,#56774,#56775,#56776));
#13593=EDGE_LOOP('',(#56777,#56778,#56779,#56780));
#13594=EDGE_LOOP('',(#56781,#56782,#56783,#56784));
#13595=EDGE_LOOP('',(#56785,#56786,#56787,#56788));
#13596=EDGE_LOOP('',(#56789,#56790,#56791,#56792));
#13597=EDGE_LOOP('',(#56793,#56794,#56795,#56796));
#13598=EDGE_LOOP('',(#56797,#56798,#56799,#56800));
#13599=EDGE_LOOP('',(#56801,#56802,#56803,#56804));
#13600=EDGE_LOOP('',(#56805,#56806,#56807,#56808));
#13601=EDGE_LOOP('',(#56809,#56810,#56811,#56812));
#13602=EDGE_LOOP('',(#56813,#56814,#56815,#56816));
#13603=EDGE_LOOP('',(#56817,#56818,#56819,#56820));
#13604=EDGE_LOOP('',(#56821,#56822,#56823,#56824));
#13605=EDGE_LOOP('',(#56825,#56826,#56827,#56828));
#13606=EDGE_LOOP('',(#56829,#56830,#56831,#56832));
#13607=EDGE_LOOP('',(#56833,#56834,#56835,#56836));
#13608=EDGE_LOOP('',(#56837,#56838,#56839,#56840));
#13609=EDGE_LOOP('',(#56841,#56842,#56843,#56844));
#13610=EDGE_LOOP('',(#56845,#56846,#56847,#56848));
#13611=EDGE_LOOP('',(#56849,#56850,#56851,#56852));
#13612=EDGE_LOOP('',(#56853,#56854,#56855,#56856));
#13613=EDGE_LOOP('',(#56857,#56858,#56859,#56860));
#13614=EDGE_LOOP('',(#56861,#56862,#56863,#56864));
#13615=EDGE_LOOP('',(#56865,#56866,#56867,#56868));
#13616=EDGE_LOOP('',(#56869,#56870,#56871,#56872));
#13617=EDGE_LOOP('',(#56873,#56874,#56875,#56876));
#13618=EDGE_LOOP('',(#56877,#56878,#56879,#56880));
#13619=EDGE_LOOP('',(#56881,#56882,#56883,#56884));
#13620=EDGE_LOOP('',(#56885,#56886,#56887,#56888));
#13621=EDGE_LOOP('',(#56889,#56890,#56891,#56892));
#13622=EDGE_LOOP('',(#56893,#56894,#56895,#56896));
#13623=EDGE_LOOP('',(#56897,#56898,#56899,#56900));
#13624=EDGE_LOOP('',(#56901,#56902,#56903,#56904));
#13625=EDGE_LOOP('',(#56905,#56906,#56907,#56908));
#13626=EDGE_LOOP('',(#56909,#56910,#56911,#56912));
#13627=EDGE_LOOP('',(#56913,#56914,#56915,#56916));
#13628=EDGE_LOOP('',(#56917,#56918,#56919,#56920));
#13629=EDGE_LOOP('',(#56921,#56922,#56923,#56924));
#13630=EDGE_LOOP('',(#56925,#56926,#56927,#56928));
#13631=EDGE_LOOP('',(#56929,#56930,#56931,#56932));
#13632=EDGE_LOOP('',(#56933,#56934,#56935,#56936));
#13633=EDGE_LOOP('',(#56937,#56938,#56939,#56940));
#13634=EDGE_LOOP('',(#56941,#56942,#56943,#56944));
#13635=EDGE_LOOP('',(#56945,#56946,#56947,#56948));
#13636=EDGE_LOOP('',(#56949,#56950,#56951,#56952));
#13637=EDGE_LOOP('',(#56953,#56954,#56955,#56956));
#13638=EDGE_LOOP('',(#56957,#56958,#56959,#56960));
#13639=EDGE_LOOP('',(#56961,#56962,#56963,#56964));
#13640=EDGE_LOOP('',(#56965,#56966,#56967,#56968));
#13641=EDGE_LOOP('',(#56969,#56970,#56971,#56972));
#13642=EDGE_LOOP('',(#56973,#56974,#56975,#56976));
#13643=EDGE_LOOP('',(#56977,#56978,#56979,#56980));
#13644=EDGE_LOOP('',(#56981,#56982,#56983,#56984));
#13645=EDGE_LOOP('',(#56985,#56986,#56987,#56988));
#13646=EDGE_LOOP('',(#56989,#56990,#56991,#56992));
#13647=EDGE_LOOP('',(#56993,#56994,#56995,#56996));
#13648=EDGE_LOOP('',(#56997,#56998,#56999,#57000));
#13649=EDGE_LOOP('',(#57001,#57002,#57003,#57004));
#13650=EDGE_LOOP('',(#57005,#57006,#57007,#57008));
#13651=EDGE_LOOP('',(#57009,#57010,#57011,#57012));
#13652=EDGE_LOOP('',(#57013,#57014,#57015,#57016));
#13653=EDGE_LOOP('',(#57017,#57018,#57019,#57020));
#13654=EDGE_LOOP('',(#57021,#57022,#57023,#57024));
#13655=EDGE_LOOP('',(#57025,#57026,#57027,#57028));
#13656=EDGE_LOOP('',(#57029,#57030,#57031,#57032));
#13657=EDGE_LOOP('',(#57033,#57034,#57035,#57036));
#13658=EDGE_LOOP('',(#57037,#57038,#57039,#57040));
#13659=EDGE_LOOP('',(#57041,#57042,#57043,#57044));
#13660=EDGE_LOOP('',(#57045,#57046,#57047,#57048));
#13661=EDGE_LOOP('',(#57049,#57050,#57051,#57052));
#13662=EDGE_LOOP('',(#57053,#57054,#57055,#57056));
#13663=EDGE_LOOP('',(#57057,#57058,#57059,#57060));
#13664=EDGE_LOOP('',(#57061,#57062,#57063,#57064));
#13665=EDGE_LOOP('',(#57065,#57066,#57067,#57068));
#13666=EDGE_LOOP('',(#57069,#57070,#57071,#57072));
#13667=EDGE_LOOP('',(#57073,#57074,#57075,#57076));
#13668=EDGE_LOOP('',(#57077,#57078,#57079,#57080));
#13669=EDGE_LOOP('',(#57081,#57082,#57083,#57084));
#13670=EDGE_LOOP('',(#57085,#57086,#57087,#57088));
#13671=EDGE_LOOP('',(#57089,#57090,#57091,#57092));
#13672=EDGE_LOOP('',(#57093,#57094,#57095,#57096));
#13673=EDGE_LOOP('',(#57097,#57098,#57099,#57100));
#13674=EDGE_LOOP('',(#57101,#57102,#57103,#57104));
#13675=EDGE_LOOP('',(#57105,#57106,#57107,#57108));
#13676=EDGE_LOOP('',(#57109,#57110,#57111,#57112));
#13677=EDGE_LOOP('',(#57113,#57114,#57115,#57116));
#13678=EDGE_LOOP('',(#57117,#57118,#57119,#57120));
#13679=EDGE_LOOP('',(#57121,#57122,#57123,#57124));
#13680=EDGE_LOOP('',(#57125,#57126,#57127,#57128));
#13681=EDGE_LOOP('',(#57129,#57130,#57131,#57132));
#13682=EDGE_LOOP('',(#57133,#57134,#57135,#57136));
#13683=EDGE_LOOP('',(#57137,#57138,#57139,#57140));
#13684=EDGE_LOOP('',(#57141,#57142,#57143,#57144));
#13685=EDGE_LOOP('',(#57145,#57146,#57147,#57148));
#13686=EDGE_LOOP('',(#57149,#57150,#57151,#57152));
#13687=EDGE_LOOP('',(#57153,#57154,#57155,#57156));
#13688=EDGE_LOOP('',(#57157,#57158,#57159,#57160));
#13689=EDGE_LOOP('',(#57161,#57162,#57163,#57164));
#13690=EDGE_LOOP('',(#57165,#57166,#57167,#57168));
#13691=EDGE_LOOP('',(#57169,#57170,#57171,#57172));
#13692=EDGE_LOOP('',(#57173,#57174,#57175,#57176));
#13693=EDGE_LOOP('',(#57177,#57178,#57179,#57180));
#13694=EDGE_LOOP('',(#57181,#57182,#57183,#57184));
#13695=EDGE_LOOP('',(#57185,#57186,#57187,#57188));
#13696=EDGE_LOOP('',(#57189,#57190,#57191,#57192));
#13697=EDGE_LOOP('',(#57193,#57194,#57195,#57196));
#13698=EDGE_LOOP('',(#57197,#57198,#57199,#57200));
#13699=EDGE_LOOP('',(#57201,#57202,#57203,#57204));
#13700=EDGE_LOOP('',(#57205,#57206,#57207,#57208));
#13701=EDGE_LOOP('',(#57209,#57210,#57211,#57212));
#13702=EDGE_LOOP('',(#57213,#57214,#57215,#57216));
#13703=EDGE_LOOP('',(#57217,#57218,#57219,#57220));
#13704=EDGE_LOOP('',(#57221,#57222,#57223,#57224));
#13705=EDGE_LOOP('',(#57225,#57226,#57227,#57228));
#13706=EDGE_LOOP('',(#57229,#57230,#57231,#57232));
#13707=EDGE_LOOP('',(#57233,#57234,#57235,#57236));
#13708=EDGE_LOOP('',(#57237,#57238,#57239,#57240));
#13709=EDGE_LOOP('',(#57241,#57242,#57243,#57244));
#13710=EDGE_LOOP('',(#57245,#57246,#57247,#57248));
#13711=EDGE_LOOP('',(#57249,#57250,#57251,#57252));
#13712=EDGE_LOOP('',(#57253,#57254,#57255,#57256));
#13713=EDGE_LOOP('',(#57257,#57258,#57259,#57260));
#13714=EDGE_LOOP('',(#57261,#57262,#57263,#57264));
#13715=EDGE_LOOP('',(#57265,#57266,#57267,#57268));
#13716=EDGE_LOOP('',(#57269,#57270,#57271,#57272));
#13717=EDGE_LOOP('',(#57273,#57274,#57275,#57276));
#13718=EDGE_LOOP('',(#57277,#57278,#57279,#57280));
#13719=EDGE_LOOP('',(#57281,#57282,#57283,#57284));
#13720=EDGE_LOOP('',(#57285,#57286,#57287,#57288));
#13721=EDGE_LOOP('',(#57289,#57290,#57291,#57292));
#13722=EDGE_LOOP('',(#57293,#57294,#57295,#57296));
#13723=EDGE_LOOP('',(#57297,#57298,#57299,#57300));
#13724=EDGE_LOOP('',(#57301,#57302,#57303,#57304));
#13725=EDGE_LOOP('',(#57305,#57306,#57307,#57308));
#13726=EDGE_LOOP('',(#57309,#57310,#57311,#57312));
#13727=EDGE_LOOP('',(#57313,#57314,#57315,#57316));
#13728=EDGE_LOOP('',(#57317,#57318,#57319,#57320));
#13729=EDGE_LOOP('',(#57321,#57322,#57323,#57324));
#13730=EDGE_LOOP('',(#57325,#57326,#57327,#57328));
#13731=EDGE_LOOP('',(#57329,#57330,#57331,#57332));
#13732=EDGE_LOOP('',(#57333,#57334,#57335,#57336));
#13733=EDGE_LOOP('',(#57337,#57338,#57339,#57340));
#13734=EDGE_LOOP('',(#57341,#57342,#57343,#57344));
#13735=EDGE_LOOP('',(#57345,#57346,#57347,#57348));
#13736=EDGE_LOOP('',(#57349,#57350,#57351,#57352));
#13737=EDGE_LOOP('',(#57353,#57354,#57355,#57356));
#13738=EDGE_LOOP('',(#57357,#57358,#57359,#57360));
#13739=EDGE_LOOP('',(#57361,#57362,#57363,#57364));
#13740=EDGE_LOOP('',(#57365,#57366,#57367,#57368));
#13741=EDGE_LOOP('',(#57369,#57370,#57371,#57372));
#13742=EDGE_LOOP('',(#57373,#57374,#57375,#57376));
#13743=EDGE_LOOP('',(#57377,#57378,#57379,#57380));
#13744=EDGE_LOOP('',(#57381,#57382,#57383,#57384));
#13745=EDGE_LOOP('',(#57385,#57386,#57387,#57388));
#13746=EDGE_LOOP('',(#57389,#57390,#57391,#57392));
#13747=EDGE_LOOP('',(#57393,#57394,#57395,#57396));
#13748=EDGE_LOOP('',(#57397,#57398,#57399,#57400));
#13749=EDGE_LOOP('',(#57401,#57402,#57403,#57404));
#13750=EDGE_LOOP('',(#57405,#57406,#57407,#57408));
#13751=EDGE_LOOP('',(#57409,#57410,#57411,#57412));
#13752=EDGE_LOOP('',(#57413,#57414,#57415,#57416));
#13753=EDGE_LOOP('',(#57417,#57418,#57419,#57420));
#13754=EDGE_LOOP('',(#57421,#57422,#57423,#57424));
#13755=EDGE_LOOP('',(#57425,#57426,#57427,#57428));
#13756=EDGE_LOOP('',(#57429,#57430,#57431,#57432));
#13757=EDGE_LOOP('',(#57433,#57434,#57435,#57436));
#13758=EDGE_LOOP('',(#57437,#57438,#57439,#57440));
#13759=EDGE_LOOP('',(#57441,#57442,#57443,#57444));
#13760=EDGE_LOOP('',(#57445,#57446,#57447,#57448));
#13761=EDGE_LOOP('',(#57449,#57450,#57451,#57452));
#13762=EDGE_LOOP('',(#57453,#57454,#57455,#57456));
#13763=EDGE_LOOP('',(#57457,#57458,#57459,#57460));
#13764=EDGE_LOOP('',(#57461,#57462,#57463,#57464));
#13765=EDGE_LOOP('',(#57465,#57466,#57467,#57468));
#13766=EDGE_LOOP('',(#57469,#57470,#57471,#57472));
#13767=EDGE_LOOP('',(#57473,#57474,#57475,#57476));
#13768=EDGE_LOOP('',(#57477,#57478,#57479,#57480));
#13769=EDGE_LOOP('',(#57481,#57482,#57483,#57484));
#13770=EDGE_LOOP('',(#57485,#57486,#57487,#57488));
#13771=EDGE_LOOP('',(#57489,#57490,#57491,#57492));
#13772=EDGE_LOOP('',(#57493,#57494,#57495,#57496));
#13773=EDGE_LOOP('',(#57497,#57498,#57499,#57500));
#13774=EDGE_LOOP('',(#57501,#57502,#57503,#57504));
#13775=EDGE_LOOP('',(#57505,#57506,#57507,#57508));
#13776=EDGE_LOOP('',(#57509,#57510,#57511,#57512));
#13777=EDGE_LOOP('',(#57513,#57514,#57515,#57516));
#13778=EDGE_LOOP('',(#57517,#57518,#57519,#57520));
#13779=EDGE_LOOP('',(#57521,#57522,#57523,#57524));
#13780=EDGE_LOOP('',(#57525,#57526,#57527,#57528));
#13781=EDGE_LOOP('',(#57529,#57530,#57531,#57532));
#13782=EDGE_LOOP('',(#57533,#57534,#57535,#57536));
#13783=EDGE_LOOP('',(#57537,#57538,#57539,#57540));
#13784=EDGE_LOOP('',(#57541,#57542,#57543,#57544));
#13785=EDGE_LOOP('',(#57545,#57546,#57547,#57548));
#13786=EDGE_LOOP('',(#57549,#57550,#57551,#57552));
#13787=EDGE_LOOP('',(#57553,#57554,#57555,#57556));
#13788=EDGE_LOOP('',(#57557,#57558,#57559,#57560));
#13789=EDGE_LOOP('',(#57561,#57562,#57563,#57564));
#13790=EDGE_LOOP('',(#57565,#57566,#57567,#57568));
#13791=EDGE_LOOP('',(#57569,#57570,#57571,#57572));
#13792=EDGE_LOOP('',(#57573,#57574,#57575,#57576));
#13793=EDGE_LOOP('',(#57577,#57578,#57579,#57580));
#13794=EDGE_LOOP('',(#57581,#57582,#57583,#57584));
#13795=EDGE_LOOP('',(#57585,#57586,#57587,#57588));
#13796=EDGE_LOOP('',(#57589,#57590,#57591,#57592));
#13797=EDGE_LOOP('',(#57593,#57594,#57595,#57596));
#13798=EDGE_LOOP('',(#57597,#57598,#57599,#57600));
#13799=EDGE_LOOP('',(#57601,#57602,#57603,#57604));
#13800=EDGE_LOOP('',(#57605,#57606,#57607,#57608));
#13801=EDGE_LOOP('',(#57609,#57610,#57611,#57612));
#13802=EDGE_LOOP('',(#57613,#57614,#57615,#57616));
#13803=EDGE_LOOP('',(#57617,#57618,#57619,#57620));
#13804=EDGE_LOOP('',(#57621,#57622,#57623,#57624));
#13805=EDGE_LOOP('',(#57625,#57626,#57627,#57628));
#13806=EDGE_LOOP('',(#57629,#57630,#57631,#57632));
#13807=EDGE_LOOP('',(#57633,#57634,#57635,#57636));
#13808=EDGE_LOOP('',(#57637,#57638,#57639,#57640));
#13809=EDGE_LOOP('',(#57641,#57642,#57643,#57644));
#13810=EDGE_LOOP('',(#57645,#57646,#57647,#57648));
#13811=EDGE_LOOP('',(#57649,#57650,#57651,#57652));
#13812=EDGE_LOOP('',(#57653,#57654,#57655,#57656));
#13813=EDGE_LOOP('',(#57657,#57658,#57659,#57660));
#13814=EDGE_LOOP('',(#57661,#57662,#57663,#57664));
#13815=EDGE_LOOP('',(#57665,#57666,#57667,#57668));
#13816=EDGE_LOOP('',(#57669,#57670,#57671,#57672));
#13817=EDGE_LOOP('',(#57673,#57674,#57675,#57676));
#13818=EDGE_LOOP('',(#57677,#57678,#57679,#57680));
#13819=EDGE_LOOP('',(#57681,#57682,#57683,#57684));
#13820=EDGE_LOOP('',(#57685,#57686,#57687,#57688));
#13821=EDGE_LOOP('',(#57689,#57690,#57691,#57692));
#13822=EDGE_LOOP('',(#57693,#57694,#57695,#57696));
#13823=EDGE_LOOP('',(#57697,#57698,#57699,#57700));
#13824=EDGE_LOOP('',(#57701,#57702,#57703,#57704));
#13825=EDGE_LOOP('',(#57705,#57706,#57707,#57708));
#13826=EDGE_LOOP('',(#57709,#57710,#57711,#57712));
#13827=EDGE_LOOP('',(#57713,#57714,#57715,#57716));
#13828=EDGE_LOOP('',(#57717,#57718,#57719,#57720));
#13829=EDGE_LOOP('',(#57721,#57722,#57723,#57724));
#13830=EDGE_LOOP('',(#57725,#57726,#57727,#57728));
#13831=EDGE_LOOP('',(#57729,#57730,#57731,#57732));
#13832=EDGE_LOOP('',(#57733,#57734,#57735,#57736));
#13833=EDGE_LOOP('',(#57737,#57738,#57739,#57740));
#13834=EDGE_LOOP('',(#57741,#57742,#57743,#57744));
#13835=EDGE_LOOP('',(#57745,#57746,#57747,#57748));
#13836=EDGE_LOOP('',(#57749,#57750,#57751,#57752));
#13837=EDGE_LOOP('',(#57753,#57754,#57755,#57756));
#13838=EDGE_LOOP('',(#57757,#57758,#57759,#57760));
#13839=EDGE_LOOP('',(#57761,#57762,#57763,#57764));
#13840=EDGE_LOOP('',(#57765,#57766,#57767,#57768));
#13841=EDGE_LOOP('',(#57769,#57770,#57771,#57772));
#13842=EDGE_LOOP('',(#57773,#57774,#57775,#57776));
#13843=EDGE_LOOP('',(#57777,#57778,#57779,#57780));
#13844=EDGE_LOOP('',(#57781,#57782,#57783,#57784));
#13845=EDGE_LOOP('',(#57785,#57786,#57787,#57788));
#13846=EDGE_LOOP('',(#57789,#57790,#57791,#57792));
#13847=EDGE_LOOP('',(#57793,#57794,#57795,#57796));
#13848=EDGE_LOOP('',(#57797,#57798,#57799,#57800));
#13849=EDGE_LOOP('',(#57801,#57802,#57803,#57804));
#13850=EDGE_LOOP('',(#57805,#57806,#57807,#57808));
#13851=EDGE_LOOP('',(#57809,#57810,#57811,#57812));
#13852=EDGE_LOOP('',(#57813,#57814,#57815,#57816));
#13853=EDGE_LOOP('',(#57817,#57818,#57819,#57820));
#13854=EDGE_LOOP('',(#57821,#57822,#57823,#57824));
#13855=EDGE_LOOP('',(#57825,#57826,#57827,#57828));
#13856=EDGE_LOOP('',(#57829,#57830,#57831,#57832));
#13857=EDGE_LOOP('',(#57833,#57834,#57835,#57836));
#13858=EDGE_LOOP('',(#57837,#57838,#57839,#57840));
#13859=EDGE_LOOP('',(#57841,#57842,#57843,#57844));
#13860=EDGE_LOOP('',(#57845,#57846,#57847,#57848));
#13861=EDGE_LOOP('',(#57849,#57850,#57851,#57852));
#13862=EDGE_LOOP('',(#57853,#57854,#57855,#57856));
#13863=EDGE_LOOP('',(#57857,#57858,#57859,#57860));
#13864=EDGE_LOOP('',(#57861,#57862,#57863,#57864));
#13865=EDGE_LOOP('',(#57865,#57866,#57867,#57868));
#13866=EDGE_LOOP('',(#57869,#57870,#57871,#57872));
#13867=EDGE_LOOP('',(#57873,#57874,#57875,#57876));
#13868=EDGE_LOOP('',(#57877,#57878,#57879,#57880));
#13869=EDGE_LOOP('',(#57881,#57882,#57883,#57884));
#13870=EDGE_LOOP('',(#57885,#57886,#57887,#57888));
#13871=EDGE_LOOP('',(#57889,#57890,#57891,#57892));
#13872=EDGE_LOOP('',(#57893,#57894,#57895,#57896));
#13873=EDGE_LOOP('',(#57897,#57898,#57899,#57900));
#13874=EDGE_LOOP('',(#57901,#57902,#57903,#57904));
#13875=EDGE_LOOP('',(#57905,#57906,#57907,#57908));
#13876=EDGE_LOOP('',(#57909,#57910,#57911,#57912));
#13877=EDGE_LOOP('',(#57913,#57914,#57915,#57916));
#13878=EDGE_LOOP('',(#57917,#57918,#57919,#57920));
#13879=EDGE_LOOP('',(#57921,#57922,#57923,#57924));
#13880=EDGE_LOOP('',(#57925,#57926,#57927,#57928));
#13881=EDGE_LOOP('',(#57929,#57930,#57931,#57932));
#13882=EDGE_LOOP('',(#57933,#57934,#57935,#57936));
#13883=EDGE_LOOP('',(#57937,#57938,#57939,#57940));
#13884=EDGE_LOOP('',(#57941,#57942,#57943,#57944));
#13885=EDGE_LOOP('',(#57945,#57946,#57947,#57948));
#13886=EDGE_LOOP('',(#57949,#57950,#57951,#57952));
#13887=EDGE_LOOP('',(#57953,#57954,#57955,#57956));
#13888=EDGE_LOOP('',(#57957,#57958,#57959,#57960));
#13889=EDGE_LOOP('',(#57961,#57962,#57963,#57964));
#13890=EDGE_LOOP('',(#57965,#57966,#57967,#57968));
#13891=EDGE_LOOP('',(#57969,#57970,#57971,#57972));
#13892=EDGE_LOOP('',(#57973,#57974,#57975,#57976));
#13893=EDGE_LOOP('',(#57977,#57978,#57979,#57980));
#13894=EDGE_LOOP('',(#57981,#57982,#57983,#57984));
#13895=EDGE_LOOP('',(#57985,#57986,#57987,#57988));
#13896=EDGE_LOOP('',(#57989,#57990,#57991,#57992));
#13897=EDGE_LOOP('',(#57993,#57994,#57995,#57996));
#13898=EDGE_LOOP('',(#57997,#57998,#57999,#58000));
#13899=EDGE_LOOP('',(#58001,#58002,#58003,#58004));
#13900=EDGE_LOOP('',(#58005,#58006,#58007,#58008));
#13901=EDGE_LOOP('',(#58009,#58010,#58011,#58012));
#13902=EDGE_LOOP('',(#58013,#58014,#58015,#58016));
#13903=EDGE_LOOP('',(#58017,#58018,#58019,#58020));
#13904=EDGE_LOOP('',(#58021,#58022,#58023,#58024));
#13905=EDGE_LOOP('',(#58025,#58026,#58027,#58028));
#13906=EDGE_LOOP('',(#58029,#58030,#58031,#58032));
#13907=EDGE_LOOP('',(#58033,#58034,#58035,#58036));
#13908=EDGE_LOOP('',(#58037,#58038,#58039,#58040));
#13909=EDGE_LOOP('',(#58041,#58042,#58043,#58044));
#13910=EDGE_LOOP('',(#58045,#58046,#58047,#58048));
#13911=EDGE_LOOP('',(#58049,#58050,#58051,#58052));
#13912=EDGE_LOOP('',(#58053,#58054,#58055,#58056));
#13913=EDGE_LOOP('',(#58057,#58058,#58059,#58060));
#13914=EDGE_LOOP('',(#58061,#58062,#58063,#58064));
#13915=EDGE_LOOP('',(#58065,#58066,#58067,#58068));
#13916=EDGE_LOOP('',(#58069,#58070,#58071,#58072));
#13917=EDGE_LOOP('',(#58073,#58074,#58075,#58076));
#13918=EDGE_LOOP('',(#58077,#58078,#58079,#58080));
#13919=EDGE_LOOP('',(#58081,#58082,#58083,#58084));
#13920=EDGE_LOOP('',(#58085,#58086,#58087,#58088));
#13921=EDGE_LOOP('',(#58089,#58090,#58091,#58092));
#13922=EDGE_LOOP('',(#58093,#58094,#58095,#58096));
#13923=EDGE_LOOP('',(#58097,#58098,#58099,#58100));
#13924=EDGE_LOOP('',(#58101,#58102,#58103,#58104));
#13925=EDGE_LOOP('',(#58105,#58106,#58107,#58108));
#13926=EDGE_LOOP('',(#58109,#58110,#58111,#58112));
#13927=EDGE_LOOP('',(#58113,#58114,#58115,#58116));
#13928=EDGE_LOOP('',(#58117,#58118,#58119,#58120));
#13929=EDGE_LOOP('',(#58121,#58122,#58123,#58124));
#13930=EDGE_LOOP('',(#58125,#58126,#58127,#58128));
#13931=EDGE_LOOP('',(#58129,#58130,#58131,#58132));
#13932=EDGE_LOOP('',(#58133,#58134,#58135,#58136));
#13933=EDGE_LOOP('',(#58137,#58138,#58139,#58140));
#13934=EDGE_LOOP('',(#58141,#58142,#58143,#58144));
#13935=EDGE_LOOP('',(#58145,#58146,#58147,#58148));
#13936=EDGE_LOOP('',(#58149,#58150,#58151,#58152));
#13937=EDGE_LOOP('',(#58153,#58154,#58155,#58156));
#13938=EDGE_LOOP('',(#58157,#58158,#58159,#58160));
#13939=EDGE_LOOP('',(#58161,#58162,#58163,#58164));
#13940=EDGE_LOOP('',(#58165,#58166,#58167,#58168));
#13941=EDGE_LOOP('',(#58169,#58170,#58171,#58172));
#13942=EDGE_LOOP('',(#58173,#58174,#58175,#58176));
#13943=EDGE_LOOP('',(#58177,#58178,#58179,#58180));
#13944=EDGE_LOOP('',(#58181,#58182,#58183,#58184));
#13945=EDGE_LOOP('',(#58185,#58186,#58187,#58188));
#13946=EDGE_LOOP('',(#58189,#58190,#58191,#58192));
#13947=EDGE_LOOP('',(#58193,#58194,#58195,#58196));
#13948=EDGE_LOOP('',(#58197,#58198,#58199,#58200));
#13949=EDGE_LOOP('',(#58201,#58202,#58203,#58204));
#13950=EDGE_LOOP('',(#58205,#58206,#58207,#58208));
#13951=EDGE_LOOP('',(#58209,#58210,#58211,#58212));
#13952=EDGE_LOOP('',(#58213,#58214,#58215,#58216));
#13953=EDGE_LOOP('',(#58217,#58218,#58219,#58220));
#13954=EDGE_LOOP('',(#58221,#58222,#58223,#58224));
#13955=EDGE_LOOP('',(#58225,#58226,#58227,#58228));
#13956=EDGE_LOOP('',(#58229,#58230,#58231,#58232));
#13957=EDGE_LOOP('',(#58233,#58234,#58235,#58236));
#13958=EDGE_LOOP('',(#58237,#58238,#58239,#58240));
#13959=EDGE_LOOP('',(#58241,#58242,#58243,#58244));
#13960=EDGE_LOOP('',(#58245,#58246,#58247,#58248));
#13961=EDGE_LOOP('',(#58249,#58250,#58251,#58252));
#13962=EDGE_LOOP('',(#58253,#58254,#58255,#58256));
#13963=EDGE_LOOP('',(#58257,#58258,#58259,#58260));
#13964=EDGE_LOOP('',(#58261,#58262,#58263,#58264));
#13965=EDGE_LOOP('',(#58265,#58266,#58267,#58268));
#13966=EDGE_LOOP('',(#58269,#58270,#58271,#58272));
#13967=EDGE_LOOP('',(#58273,#58274,#58275,#58276));
#13968=EDGE_LOOP('',(#58277,#58278,#58279,#58280));
#13969=EDGE_LOOP('',(#58281,#58282,#58283,#58284));
#13970=EDGE_LOOP('',(#58285,#58286,#58287,#58288));
#13971=EDGE_LOOP('',(#58289,#58290,#58291,#58292));
#13972=EDGE_LOOP('',(#58293,#58294,#58295,#58296));
#13973=EDGE_LOOP('',(#58297,#58298,#58299,#58300));
#13974=EDGE_LOOP('',(#58301,#58302,#58303,#58304));
#13975=EDGE_LOOP('',(#58305,#58306,#58307,#58308));
#13976=EDGE_LOOP('',(#58309,#58310,#58311,#58312));
#13977=EDGE_LOOP('',(#58313,#58314,#58315,#58316));
#13978=EDGE_LOOP('',(#58317,#58318,#58319,#58320));
#13979=EDGE_LOOP('',(#58321,#58322,#58323,#58324));
#13980=EDGE_LOOP('',(#58325,#58326,#58327,#58328));
#13981=EDGE_LOOP('',(#58329,#58330,#58331,#58332));
#13982=EDGE_LOOP('',(#58333,#58334,#58335,#58336));
#13983=EDGE_LOOP('',(#58337,#58338,#58339,#58340));
#13984=EDGE_LOOP('',(#58341,#58342,#58343,#58344));
#13985=EDGE_LOOP('',(#58345,#58346,#58347,#58348));
#13986=EDGE_LOOP('',(#58349,#58350,#58351,#58352));
#13987=EDGE_LOOP('',(#58353,#58354,#58355,#58356));
#13988=EDGE_LOOP('',(#58357,#58358,#58359,#58360));
#13989=EDGE_LOOP('',(#58361,#58362,#58363,#58364));
#13990=EDGE_LOOP('',(#58365,#58366,#58367,#58368));
#13991=EDGE_LOOP('',(#58369,#58370,#58371,#58372));
#13992=EDGE_LOOP('',(#58373,#58374,#58375,#58376));
#13993=EDGE_LOOP('',(#58377,#58378,#58379,#58380));
#13994=EDGE_LOOP('',(#58381,#58382,#58383,#58384));
#13995=EDGE_LOOP('',(#58385,#58386,#58387,#58388));
#13996=EDGE_LOOP('',(#58389,#58390,#58391,#58392));
#13997=EDGE_LOOP('',(#58393,#58394,#58395,#58396));
#13998=EDGE_LOOP('',(#58397,#58398,#58399,#58400));
#13999=EDGE_LOOP('',(#58401,#58402,#58403,#58404));
#14000=EDGE_LOOP('',(#58405,#58406,#58407,#58408));
#14001=EDGE_LOOP('',(#58409,#58410,#58411,#58412));
#14002=EDGE_LOOP('',(#58413,#58414,#58415,#58416));
#14003=EDGE_LOOP('',(#58417,#58418,#58419,#58420));
#14004=EDGE_LOOP('',(#58421,#58422,#58423,#58424));
#14005=EDGE_LOOP('',(#58425,#58426,#58427,#58428));
#14006=EDGE_LOOP('',(#58429,#58430,#58431,#58432));
#14007=EDGE_LOOP('',(#58433,#58434,#58435,#58436));
#14008=EDGE_LOOP('',(#58437,#58438,#58439,#58440));
#14009=EDGE_LOOP('',(#58441,#58442,#58443,#58444));
#14010=EDGE_LOOP('',(#58445,#58446,#58447,#58448));
#14011=EDGE_LOOP('',(#58449,#58450,#58451,#58452));
#14012=EDGE_LOOP('',(#58453,#58454,#58455,#58456));
#14013=EDGE_LOOP('',(#58457,#58458,#58459,#58460));
#14014=EDGE_LOOP('',(#58461,#58462,#58463,#58464));
#14015=EDGE_LOOP('',(#58465,#58466,#58467,#58468));
#14016=EDGE_LOOP('',(#58469,#58470,#58471,#58472));
#14017=EDGE_LOOP('',(#58473,#58474,#58475,#58476));
#14018=EDGE_LOOP('',(#58477,#58478,#58479,#58480));
#14019=EDGE_LOOP('',(#58481,#58482,#58483,#58484));
#14020=EDGE_LOOP('',(#58485,#58486,#58487,#58488));
#14021=EDGE_LOOP('',(#58489,#58490,#58491,#58492));
#14022=EDGE_LOOP('',(#58493,#58494,#58495,#58496));
#14023=EDGE_LOOP('',(#58497,#58498,#58499,#58500));
#14024=EDGE_LOOP('',(#58501,#58502,#58503,#58504));
#14025=EDGE_LOOP('',(#58505,#58506,#58507,#58508));
#14026=EDGE_LOOP('',(#58509,#58510,#58511,#58512));
#14027=EDGE_LOOP('',(#58513,#58514,#58515,#58516));
#14028=EDGE_LOOP('',(#58517,#58518,#58519,#58520));
#14029=EDGE_LOOP('',(#58521,#58522,#58523,#58524));
#14030=EDGE_LOOP('',(#58525,#58526,#58527,#58528));
#14031=EDGE_LOOP('',(#58529,#58530,#58531,#58532));
#14032=EDGE_LOOP('',(#58533,#58534,#58535,#58536));
#14033=EDGE_LOOP('',(#58537,#58538,#58539,#58540));
#14034=EDGE_LOOP('',(#58541,#58542,#58543,#58544));
#14035=EDGE_LOOP('',(#58545,#58546,#58547,#58548));
#14036=EDGE_LOOP('',(#58549,#58550,#58551,#58552));
#14037=EDGE_LOOP('',(#58553,#58554,#58555,#58556));
#14038=EDGE_LOOP('',(#58557,#58558,#58559,#58560));
#14039=EDGE_LOOP('',(#58561,#58562,#58563,#58564));
#14040=EDGE_LOOP('',(#58565,#58566,#58567,#58568));
#14041=EDGE_LOOP('',(#58569,#58570,#58571,#58572));
#14042=EDGE_LOOP('',(#58573,#58574,#58575,#58576));
#14043=EDGE_LOOP('',(#58577,#58578,#58579,#58580));
#14044=EDGE_LOOP('',(#58581,#58582,#58583,#58584));
#14045=EDGE_LOOP('',(#58585,#58586,#58587,#58588));
#14046=EDGE_LOOP('',(#58589,#58590,#58591,#58592));
#14047=EDGE_LOOP('',(#58593,#58594,#58595,#58596));
#14048=EDGE_LOOP('',(#58597,#58598,#58599,#58600));
#14049=EDGE_LOOP('',(#58601,#58602,#58603,#58604));
#14050=EDGE_LOOP('',(#58605,#58606,#58607,#58608));
#14051=EDGE_LOOP('',(#58609,#58610,#58611,#58612));
#14052=EDGE_LOOP('',(#58613,#58614,#58615,#58616));
#14053=EDGE_LOOP('',(#58617,#58618,#58619,#58620));
#14054=EDGE_LOOP('',(#58621,#58622,#58623,#58624));
#14055=EDGE_LOOP('',(#58625,#58626,#58627,#58628));
#14056=EDGE_LOOP('',(#58629,#58630,#58631,#58632));
#14057=EDGE_LOOP('',(#58633,#58634,#58635,#58636));
#14058=EDGE_LOOP('',(#58637,#58638,#58639,#58640));
#14059=EDGE_LOOP('',(#58641,#58642,#58643,#58644));
#14060=EDGE_LOOP('',(#58645,#58646,#58647,#58648));
#14061=EDGE_LOOP('',(#58649,#58650,#58651,#58652));
#14062=EDGE_LOOP('',(#58653,#58654,#58655,#58656));
#14063=EDGE_LOOP('',(#58657,#58658,#58659,#58660));
#14064=EDGE_LOOP('',(#58661,#58662,#58663,#58664));
#14065=EDGE_LOOP('',(#58665,#58666,#58667,#58668));
#14066=EDGE_LOOP('',(#58669,#58670,#58671,#58672));
#14067=EDGE_LOOP('',(#58673,#58674,#58675,#58676));
#14068=EDGE_LOOP('',(#58677,#58678,#58679,#58680));
#14069=EDGE_LOOP('',(#58681,#58682,#58683,#58684));
#14070=EDGE_LOOP('',(#58685,#58686,#58687,#58688));
#14071=EDGE_LOOP('',(#58689,#58690,#58691,#58692));
#14072=EDGE_LOOP('',(#58693,#58694,#58695,#58696));
#14073=EDGE_LOOP('',(#58697,#58698,#58699,#58700));
#14074=EDGE_LOOP('',(#58701,#58702,#58703,#58704));
#14075=EDGE_LOOP('',(#58705,#58706,#58707,#58708));
#14076=EDGE_LOOP('',(#58709,#58710,#58711,#58712));
#14077=EDGE_LOOP('',(#58713,#58714,#58715,#58716));
#14078=EDGE_LOOP('',(#58717,#58718,#58719,#58720));
#14079=EDGE_LOOP('',(#58721,#58722,#58723,#58724));
#14080=EDGE_LOOP('',(#58725,#58726,#58727,#58728));
#14081=EDGE_LOOP('',(#58729,#58730,#58731,#58732));
#14082=EDGE_LOOP('',(#58733,#58734,#58735,#58736));
#14083=EDGE_LOOP('',(#58737,#58738,#58739,#58740));
#14084=EDGE_LOOP('',(#58741,#58742,#58743,#58744));
#14085=EDGE_LOOP('',(#58745,#58746,#58747,#58748));
#14086=EDGE_LOOP('',(#58749,#58750,#58751,#58752));
#14087=EDGE_LOOP('',(#58753,#58754,#58755,#58756));
#14088=EDGE_LOOP('',(#58757,#58758,#58759,#58760));
#14089=EDGE_LOOP('',(#58761,#58762,#58763,#58764));
#14090=EDGE_LOOP('',(#58765,#58766,#58767,#58768));
#14091=EDGE_LOOP('',(#58769,#58770,#58771,#58772));
#14092=EDGE_LOOP('',(#58773,#58774,#58775,#58776));
#14093=EDGE_LOOP('',(#58777,#58778,#58779,#58780));
#14094=EDGE_LOOP('',(#58781,#58782,#58783,#58784));
#14095=EDGE_LOOP('',(#58785,#58786,#58787,#58788));
#14096=EDGE_LOOP('',(#58789,#58790,#58791,#58792));
#14097=EDGE_LOOP('',(#58793,#58794,#58795,#58796));
#14098=EDGE_LOOP('',(#58797,#58798,#58799,#58800));
#14099=EDGE_LOOP('',(#58801,#58802,#58803,#58804));
#14100=EDGE_LOOP('',(#58805,#58806,#58807,#58808));
#14101=EDGE_LOOP('',(#58809,#58810,#58811,#58812));
#14102=EDGE_LOOP('',(#58813,#58814,#58815,#58816));
#14103=EDGE_LOOP('',(#58817,#58818,#58819,#58820));
#14104=EDGE_LOOP('',(#58821,#58822,#58823,#58824));
#14105=EDGE_LOOP('',(#58825,#58826,#58827,#58828));
#14106=EDGE_LOOP('',(#58829,#58830,#58831,#58832));
#14107=EDGE_LOOP('',(#58833,#58834,#58835,#58836));
#14108=EDGE_LOOP('',(#58837,#58838,#58839,#58840));
#14109=EDGE_LOOP('',(#58841,#58842,#58843,#58844));
#14110=EDGE_LOOP('',(#58845,#58846,#58847,#58848));
#14111=EDGE_LOOP('',(#58849,#58850,#58851,#58852));
#14112=EDGE_LOOP('',(#58853,#58854,#58855,#58856));
#14113=EDGE_LOOP('',(#58857,#58858,#58859,#58860));
#14114=EDGE_LOOP('',(#58861,#58862,#58863,#58864));
#14115=EDGE_LOOP('',(#58865,#58866,#58867,#58868));
#14116=EDGE_LOOP('',(#58869,#58870,#58871,#58872));
#14117=EDGE_LOOP('',(#58873,#58874,#58875,#58876));
#14118=EDGE_LOOP('',(#58877,#58878,#58879,#58880));
#14119=EDGE_LOOP('',(#58881,#58882,#58883,#58884));
#14120=EDGE_LOOP('',(#58885,#58886,#58887,#58888));
#14121=EDGE_LOOP('',(#58889,#58890,#58891,#58892));
#14122=EDGE_LOOP('',(#58893,#58894,#58895,#58896));
#14123=EDGE_LOOP('',(#58897,#58898,#58899,#58900));
#14124=EDGE_LOOP('',(#58901,#58902,#58903,#58904));
#14125=EDGE_LOOP('',(#58905,#58906,#58907,#58908));
#14126=EDGE_LOOP('',(#58909,#58910,#58911,#58912));
#14127=EDGE_LOOP('',(#58913,#58914,#58915,#58916));
#14128=EDGE_LOOP('',(#58917,#58918,#58919,#58920));
#14129=EDGE_LOOP('',(#58921,#58922,#58923,#58924));
#14130=EDGE_LOOP('',(#58925,#58926,#58927,#58928));
#14131=EDGE_LOOP('',(#58929,#58930,#58931,#58932));
#14132=EDGE_LOOP('',(#58933,#58934,#58935,#58936));
#14133=EDGE_LOOP('',(#58937,#58938,#58939,#58940));
#14134=EDGE_LOOP('',(#58941,#58942,#58943,#58944));
#14135=EDGE_LOOP('',(#58945,#58946,#58947,#58948));
#14136=EDGE_LOOP('',(#58949,#58950,#58951,#58952));
#14137=EDGE_LOOP('',(#58953,#58954,#58955,#58956));
#14138=EDGE_LOOP('',(#58957,#58958,#58959,#58960));
#14139=EDGE_LOOP('',(#58961,#58962,#58963,#58964));
#14140=EDGE_LOOP('',(#58965,#58966,#58967,#58968));
#14141=EDGE_LOOP('',(#58969,#58970,#58971,#58972));
#14142=EDGE_LOOP('',(#58973,#58974,#58975,#58976));
#14143=EDGE_LOOP('',(#58977,#58978,#58979,#58980));
#14144=EDGE_LOOP('',(#58981,#58982,#58983,#58984));
#14145=EDGE_LOOP('',(#58985,#58986,#58987,#58988));
#14146=EDGE_LOOP('',(#58989,#58990,#58991,#58992));
#14147=EDGE_LOOP('',(#58993,#58994,#58995,#58996));
#14148=EDGE_LOOP('',(#58997,#58998,#58999,#59000));
#14149=EDGE_LOOP('',(#59001,#59002,#59003,#59004));
#14150=EDGE_LOOP('',(#59005,#59006,#59007,#59008));
#14151=EDGE_LOOP('',(#59009,#59010,#59011,#59012));
#14152=EDGE_LOOP('',(#59013,#59014,#59015,#59016));
#14153=EDGE_LOOP('',(#59017,#59018,#59019,#59020));
#14154=EDGE_LOOP('',(#59021,#59022,#59023,#59024));
#14155=EDGE_LOOP('',(#59025,#59026,#59027,#59028));
#14156=EDGE_LOOP('',(#59029,#59030,#59031,#59032));
#14157=EDGE_LOOP('',(#59033,#59034,#59035,#59036));
#14158=EDGE_LOOP('',(#59037,#59038,#59039,#59040));
#14159=EDGE_LOOP('',(#59041,#59042,#59043,#59044));
#14160=EDGE_LOOP('',(#59045,#59046,#59047,#59048));
#14161=EDGE_LOOP('',(#59049,#59050,#59051,#59052));
#14162=EDGE_LOOP('',(#59053,#59054,#59055,#59056));
#14163=EDGE_LOOP('',(#59057,#59058,#59059,#59060));
#14164=EDGE_LOOP('',(#59061,#59062,#59063,#59064));
#14165=EDGE_LOOP('',(#59065,#59066,#59067,#59068));
#14166=EDGE_LOOP('',(#59069,#59070,#59071,#59072));
#14167=EDGE_LOOP('',(#59073,#59074,#59075,#59076));
#14168=EDGE_LOOP('',(#59077,#59078,#59079,#59080));
#14169=EDGE_LOOP('',(#59081,#59082,#59083,#59084));
#14170=EDGE_LOOP('',(#59085,#59086,#59087,#59088));
#14171=EDGE_LOOP('',(#59089,#59090,#59091,#59092));
#14172=EDGE_LOOP('',(#59093,#59094,#59095,#59096));
#14173=EDGE_LOOP('',(#59097,#59098,#59099,#59100));
#14174=EDGE_LOOP('',(#59101,#59102,#59103,#59104));
#14175=EDGE_LOOP('',(#59105,#59106,#59107,#59108));
#14176=EDGE_LOOP('',(#59109,#59110,#59111,#59112));
#14177=EDGE_LOOP('',(#59113,#59114,#59115,#59116));
#14178=EDGE_LOOP('',(#59117,#59118,#59119,#59120));
#14179=EDGE_LOOP('',(#59121,#59122,#59123,#59124));
#14180=EDGE_LOOP('',(#59125,#59126,#59127,#59128));
#14181=EDGE_LOOP('',(#59129,#59130,#59131,#59132));
#14182=EDGE_LOOP('',(#59133,#59134,#59135,#59136));
#14183=EDGE_LOOP('',(#59137,#59138,#59139,#59140));
#14184=EDGE_LOOP('',(#59141,#59142,#59143,#59144));
#14185=EDGE_LOOP('',(#59145,#59146,#59147,#59148));
#14186=EDGE_LOOP('',(#59149,#59150,#59151,#59152));
#14187=EDGE_LOOP('',(#59153,#59154,#59155,#59156));
#14188=EDGE_LOOP('',(#59157,#59158,#59159,#59160));
#14189=EDGE_LOOP('',(#59161,#59162,#59163,#59164));
#14190=EDGE_LOOP('',(#59165,#59166,#59167,#59168));
#14191=EDGE_LOOP('',(#59169,#59170,#59171,#59172));
#14192=EDGE_LOOP('',(#59173,#59174,#59175,#59176));
#14193=EDGE_LOOP('',(#59177,#59178,#59179,#59180));
#14194=EDGE_LOOP('',(#59181,#59182,#59183,#59184));
#14195=EDGE_LOOP('',(#59185,#59186,#59187,#59188));
#14196=EDGE_LOOP('',(#59189,#59190,#59191,#59192));
#14197=EDGE_LOOP('',(#59193,#59194,#59195,#59196));
#14198=EDGE_LOOP('',(#59197,#59198,#59199,#59200));
#14199=EDGE_LOOP('',(#59201,#59202,#59203,#59204));
#14200=EDGE_LOOP('',(#59205,#59206,#59207,#59208));
#14201=EDGE_LOOP('',(#59209,#59210,#59211,#59212));
#14202=EDGE_LOOP('',(#59213,#59214,#59215,#59216));
#14203=EDGE_LOOP('',(#59217,#59218,#59219,#59220));
#14204=EDGE_LOOP('',(#59221,#59222,#59223,#59224));
#14205=EDGE_LOOP('',(#59225,#59226,#59227,#59228));
#14206=EDGE_LOOP('',(#59229,#59230,#59231,#59232));
#14207=EDGE_LOOP('',(#59233,#59234,#59235,#59236));
#14208=EDGE_LOOP('',(#59237,#59238,#59239,#59240));
#14209=EDGE_LOOP('',(#59241,#59242,#59243,#59244));
#14210=EDGE_LOOP('',(#59245,#59246,#59247,#59248));
#14211=EDGE_LOOP('',(#59249,#59250,#59251,#59252));
#14212=EDGE_LOOP('',(#59253,#59254,#59255,#59256));
#14213=EDGE_LOOP('',(#59257,#59258,#59259,#59260));
#14214=EDGE_LOOP('',(#59261,#59262,#59263,#59264));
#14215=EDGE_LOOP('',(#59265,#59266,#59267,#59268));
#14216=EDGE_LOOP('',(#59269,#59270,#59271,#59272));
#14217=EDGE_LOOP('',(#59273,#59274,#59275,#59276));
#14218=EDGE_LOOP('',(#59277,#59278,#59279,#59280));
#14219=EDGE_LOOP('',(#59281,#59282,#59283,#59284));
#14220=EDGE_LOOP('',(#59285,#59286,#59287,#59288));
#14221=EDGE_LOOP('',(#59289,#59290,#59291,#59292));
#14222=EDGE_LOOP('',(#59293,#59294,#59295,#59296));
#14223=EDGE_LOOP('',(#59297,#59298,#59299,#59300));
#14224=EDGE_LOOP('',(#59301,#59302,#59303,#59304));
#14225=EDGE_LOOP('',(#59305,#59306,#59307,#59308));
#14226=EDGE_LOOP('',(#59309,#59310,#59311,#59312));
#14227=EDGE_LOOP('',(#59313,#59314,#59315,#59316));
#14228=EDGE_LOOP('',(#59317,#59318,#59319,#59320));
#14229=EDGE_LOOP('',(#59321,#59322,#59323,#59324));
#14230=EDGE_LOOP('',(#59325,#59326,#59327,#59328));
#14231=EDGE_LOOP('',(#59329,#59330,#59331,#59332));
#14232=EDGE_LOOP('',(#59333,#59334,#59335,#59336));
#14233=EDGE_LOOP('',(#59337,#59338,#59339,#59340));
#14234=EDGE_LOOP('',(#59341,#59342,#59343,#59344));
#14235=EDGE_LOOP('',(#59345,#59346,#59347,#59348));
#14236=EDGE_LOOP('',(#59349,#59350,#59351,#59352));
#14237=EDGE_LOOP('',(#59353,#59354,#59355,#59356));
#14238=EDGE_LOOP('',(#59357,#59358,#59359,#59360));
#14239=EDGE_LOOP('',(#59361,#59362,#59363,#59364));
#14240=EDGE_LOOP('',(#59365,#59366,#59367,#59368));
#14241=EDGE_LOOP('',(#59369,#59370,#59371,#59372));
#14242=EDGE_LOOP('',(#59373,#59374,#59375,#59376));
#14243=EDGE_LOOP('',(#59377,#59378,#59379,#59380));
#14244=EDGE_LOOP('',(#59381,#59382,#59383,#59384));
#14245=EDGE_LOOP('',(#59385,#59386,#59387,#59388));
#14246=EDGE_LOOP('',(#59389,#59390,#59391,#59392));
#14247=EDGE_LOOP('',(#59393,#59394,#59395,#59396));
#14248=EDGE_LOOP('',(#59397,#59398,#59399,#59400));
#14249=EDGE_LOOP('',(#59401,#59402,#59403,#59404));
#14250=EDGE_LOOP('',(#59405,#59406,#59407,#59408));
#14251=EDGE_LOOP('',(#59409,#59410,#59411,#59412));
#14252=EDGE_LOOP('',(#59413,#59414,#59415,#59416));
#14253=EDGE_LOOP('',(#59417,#59418,#59419,#59420));
#14254=EDGE_LOOP('',(#59421,#59422,#59423,#59424));
#14255=EDGE_LOOP('',(#59425,#59426,#59427,#59428));
#14256=EDGE_LOOP('',(#59429,#59430,#59431,#59432));
#14257=EDGE_LOOP('',(#59433,#59434,#59435,#59436));
#14258=EDGE_LOOP('',(#59437,#59438,#59439,#59440));
#14259=EDGE_LOOP('',(#59441,#59442,#59443,#59444));
#14260=EDGE_LOOP('',(#59445,#59446,#59447,#59448));
#14261=EDGE_LOOP('',(#59449,#59450,#59451,#59452));
#14262=EDGE_LOOP('',(#59453,#59454,#59455,#59456));
#14263=EDGE_LOOP('',(#59457,#59458,#59459,#59460));
#14264=EDGE_LOOP('',(#59461,#59462,#59463,#59464));
#14265=EDGE_LOOP('',(#59465,#59466,#59467,#59468));
#14266=EDGE_LOOP('',(#59469,#59470,#59471,#59472));
#14267=EDGE_LOOP('',(#59473,#59474,#59475,#59476));
#14268=EDGE_LOOP('',(#59477,#59478,#59479,#59480));
#14269=EDGE_LOOP('',(#59481,#59482,#59483,#59484));
#14270=EDGE_LOOP('',(#59485,#59486,#59487,#59488));
#14271=EDGE_LOOP('',(#59489,#59490,#59491,#59492));
#14272=EDGE_LOOP('',(#59493,#59494,#59495,#59496));
#14273=EDGE_LOOP('',(#59497,#59498,#59499,#59500));
#14274=EDGE_LOOP('',(#59501,#59502,#59503,#59504));
#14275=EDGE_LOOP('',(#59505,#59506,#59507,#59508));
#14276=EDGE_LOOP('',(#59509,#59510,#59511,#59512));
#14277=EDGE_LOOP('',(#59513,#59514,#59515,#59516));
#14278=EDGE_LOOP('',(#59517,#59518,#59519,#59520));
#14279=EDGE_LOOP('',(#59521,#59522,#59523,#59524));
#14280=EDGE_LOOP('',(#59525,#59526,#59527,#59528));
#14281=EDGE_LOOP('',(#59529,#59530,#59531,#59532));
#14282=EDGE_LOOP('',(#59533,#59534,#59535,#59536));
#14283=EDGE_LOOP('',(#59537,#59538,#59539,#59540));
#14284=EDGE_LOOP('',(#59541,#59542,#59543,#59544));
#14285=EDGE_LOOP('',(#59545,#59546,#59547,#59548));
#14286=EDGE_LOOP('',(#59549,#59550,#59551,#59552));
#14287=EDGE_LOOP('',(#59553,#59554,#59555,#59556));
#14288=EDGE_LOOP('',(#59557,#59558,#59559,#59560));
#14289=EDGE_LOOP('',(#59561,#59562,#59563,#59564));
#14290=EDGE_LOOP('',(#59565,#59566,#59567,#59568));
#14291=EDGE_LOOP('',(#59569,#59570,#59571,#59572));
#14292=EDGE_LOOP('',(#59573,#59574,#59575,#59576));
#14293=EDGE_LOOP('',(#59577,#59578,#59579,#59580));
#14294=EDGE_LOOP('',(#59581,#59582,#59583,#59584));
#14295=EDGE_LOOP('',(#59585,#59586,#59587,#59588));
#14296=EDGE_LOOP('',(#59589,#59590,#59591,#59592));
#14297=EDGE_LOOP('',(#59593,#59594,#59595,#59596));
#14298=EDGE_LOOP('',(#59597,#59598,#59599,#59600));
#14299=EDGE_LOOP('',(#59601,#59602,#59603,#59604));
#14300=EDGE_LOOP('',(#59605,#59606,#59607,#59608));
#14301=EDGE_LOOP('',(#59609,#59610,#59611,#59612));
#14302=EDGE_LOOP('',(#59613,#59614,#59615,#59616));
#14303=EDGE_LOOP('',(#59617,#59618,#59619,#59620));
#14304=EDGE_LOOP('',(#59621,#59622,#59623,#59624));
#14305=EDGE_LOOP('',(#59625,#59626,#59627,#59628));
#14306=EDGE_LOOP('',(#59629,#59630,#59631,#59632));
#14307=EDGE_LOOP('',(#59633,#59634,#59635,#59636));
#14308=EDGE_LOOP('',(#59637,#59638,#59639,#59640));
#14309=EDGE_LOOP('',(#59641,#59642,#59643,#59644));
#14310=EDGE_LOOP('',(#59645,#59646,#59647,#59648));
#14311=EDGE_LOOP('',(#59649,#59650,#59651,#59652));
#14312=EDGE_LOOP('',(#59653,#59654,#59655,#59656));
#14313=EDGE_LOOP('',(#59657,#59658,#59659,#59660));
#14314=EDGE_LOOP('',(#59661,#59662,#59663,#59664));
#14315=EDGE_LOOP('',(#59665,#59666,#59667,#59668));
#14316=EDGE_LOOP('',(#59669,#59670,#59671,#59672));
#14317=EDGE_LOOP('',(#59673,#59674,#59675,#59676));
#14318=EDGE_LOOP('',(#59677,#59678,#59679,#59680));
#14319=EDGE_LOOP('',(#59681,#59682,#59683,#59684));
#14320=EDGE_LOOP('',(#59685,#59686,#59687,#59688));
#14321=EDGE_LOOP('',(#59689,#59690,#59691,#59692));
#14322=EDGE_LOOP('',(#59693,#59694,#59695,#59696));
#14323=EDGE_LOOP('',(#59697,#59698,#59699,#59700));
#14324=EDGE_LOOP('',(#59701,#59702,#59703,#59704));
#14325=EDGE_LOOP('',(#59705,#59706,#59707,#59708));
#14326=EDGE_LOOP('',(#59709,#59710,#59711,#59712));
#14327=EDGE_LOOP('',(#59713,#59714,#59715,#59716));
#14328=EDGE_LOOP('',(#59717,#59718,#59719,#59720));
#14329=EDGE_LOOP('',(#59721,#59722,#59723,#59724));
#14330=EDGE_LOOP('',(#59725,#59726,#59727,#59728));
#14331=EDGE_LOOP('',(#59729,#59730,#59731,#59732));
#14332=EDGE_LOOP('',(#59733,#59734,#59735,#59736));
#14333=EDGE_LOOP('',(#59737,#59738,#59739,#59740));
#14334=EDGE_LOOP('',(#59741,#59742,#59743,#59744));
#14335=EDGE_LOOP('',(#59745,#59746,#59747,#59748));
#14336=EDGE_LOOP('',(#59749,#59750,#59751,#59752));
#14337=EDGE_LOOP('',(#59753,#59754,#59755,#59756));
#14338=EDGE_LOOP('',(#59757,#59758,#59759,#59760));
#14339=EDGE_LOOP('',(#59761,#59762,#59763,#59764));
#14340=EDGE_LOOP('',(#59765,#59766,#59767,#59768));
#14341=EDGE_LOOP('',(#59769,#59770,#59771,#59772));
#14342=EDGE_LOOP('',(#59773,#59774,#59775,#59776));
#14343=EDGE_LOOP('',(#59777,#59778,#59779,#59780));
#14344=EDGE_LOOP('',(#59781,#59782,#59783,#59784));
#14345=EDGE_LOOP('',(#59785,#59786,#59787,#59788));
#14346=EDGE_LOOP('',(#59789,#59790,#59791,#59792));
#14347=EDGE_LOOP('',(#59793,#59794,#59795,#59796));
#14348=EDGE_LOOP('',(#59797,#59798,#59799,#59800));
#14349=EDGE_LOOP('',(#59801,#59802,#59803,#59804));
#14350=EDGE_LOOP('',(#59805,#59806,#59807,#59808));
#14351=EDGE_LOOP('',(#59809,#59810,#59811,#59812));
#14352=EDGE_LOOP('',(#59813,#59814,#59815,#59816));
#14353=EDGE_LOOP('',(#59817,#59818,#59819,#59820));
#14354=EDGE_LOOP('',(#59821,#59822,#59823,#59824));
#14355=EDGE_LOOP('',(#59825,#59826,#59827,#59828));
#14356=EDGE_LOOP('',(#59829,#59830,#59831,#59832));
#14357=EDGE_LOOP('',(#59833,#59834,#59835,#59836));
#14358=EDGE_LOOP('',(#59837,#59838,#59839,#59840));
#14359=EDGE_LOOP('',(#59841,#59842,#59843,#59844));
#14360=EDGE_LOOP('',(#59845,#59846,#59847,#59848));
#14361=EDGE_LOOP('',(#59849,#59850,#59851,#59852));
#14362=EDGE_LOOP('',(#59853,#59854,#59855,#59856));
#14363=EDGE_LOOP('',(#59857,#59858,#59859,#59860));
#14364=EDGE_LOOP('',(#59861,#59862,#59863,#59864));
#14365=EDGE_LOOP('',(#59865,#59866,#59867,#59868));
#14366=EDGE_LOOP('',(#59869,#59870,#59871,#59872));
#14367=EDGE_LOOP('',(#59873,#59874,#59875,#59876));
#14368=EDGE_LOOP('',(#59877,#59878,#59879,#59880));
#14369=EDGE_LOOP('',(#59881,#59882,#59883,#59884));
#14370=EDGE_LOOP('',(#59885,#59886,#59887,#59888));
#14371=EDGE_LOOP('',(#59889,#59890,#59891,#59892));
#14372=EDGE_LOOP('',(#59893,#59894,#59895,#59896));
#14373=EDGE_LOOP('',(#59897,#59898,#59899,#59900));
#14374=EDGE_LOOP('',(#59901,#59902,#59903,#59904));
#14375=EDGE_LOOP('',(#59905,#59906,#59907,#59908));
#14376=EDGE_LOOP('',(#59909,#59910,#59911,#59912));
#14377=EDGE_LOOP('',(#59913,#59914,#59915,#59916));
#14378=EDGE_LOOP('',(#59917,#59918,#59919,#59920));
#14379=EDGE_LOOP('',(#59921,#59922,#59923,#59924));
#14380=EDGE_LOOP('',(#59925,#59926,#59927,#59928));
#14381=EDGE_LOOP('',(#59929,#59930,#59931,#59932));
#14382=EDGE_LOOP('',(#59933,#59934,#59935,#59936));
#14383=EDGE_LOOP('',(#59937,#59938,#59939,#59940));
#14384=EDGE_LOOP('',(#59941,#59942,#59943,#59944));
#14385=EDGE_LOOP('',(#59945,#59946,#59947,#59948));
#14386=EDGE_LOOP('',(#59949,#59950,#59951,#59952));
#14387=EDGE_LOOP('',(#59953,#59954,#59955,#59956));
#14388=EDGE_LOOP('',(#59957,#59958,#59959,#59960));
#14389=EDGE_LOOP('',(#59961,#59962,#59963,#59964));
#14390=EDGE_LOOP('',(#59965,#59966,#59967,#59968));
#14391=EDGE_LOOP('',(#59969,#59970,#59971,#59972));
#14392=EDGE_LOOP('',(#59973,#59974,#59975,#59976));
#14393=EDGE_LOOP('',(#59977,#59978,#59979,#59980));
#14394=EDGE_LOOP('',(#59981,#59982,#59983,#59984));
#14395=EDGE_LOOP('',(#59985,#59986,#59987,#59988));
#14396=EDGE_LOOP('',(#59989,#59990,#59991,#59992));
#14397=EDGE_LOOP('',(#59993,#59994,#59995,#59996));
#14398=EDGE_LOOP('',(#59997,#59998,#59999,#60000));
#14399=EDGE_LOOP('',(#60001,#60002,#60003,#60004));
#14400=EDGE_LOOP('',(#60005,#60006,#60007,#60008));
#14401=EDGE_LOOP('',(#60009,#60010,#60011,#60012));
#14402=EDGE_LOOP('',(#60013,#60014,#60015,#60016));
#14403=EDGE_LOOP('',(#60017,#60018,#60019,#60020));
#14404=EDGE_LOOP('',(#60021,#60022,#60023,#60024));
#14405=EDGE_LOOP('',(#60025,#60026,#60027,#60028));
#14406=EDGE_LOOP('',(#60029,#60030,#60031,#60032));
#14407=EDGE_LOOP('',(#60033,#60034,#60035,#60036));
#14408=EDGE_LOOP('',(#60037,#60038,#60039,#60040));
#14409=EDGE_LOOP('',(#60041,#60042,#60043,#60044));
#14410=EDGE_LOOP('',(#60045,#60046,#60047,#60048));
#14411=EDGE_LOOP('',(#60049,#60050,#60051,#60052));
#14412=EDGE_LOOP('',(#60053,#60054,#60055,#60056));
#14413=EDGE_LOOP('',(#60057,#60058,#60059,#60060));
#14414=EDGE_LOOP('',(#60061,#60062,#60063,#60064));
#14415=EDGE_LOOP('',(#60065,#60066,#60067,#60068));
#14416=EDGE_LOOP('',(#60069,#60070,#60071,#60072));
#14417=EDGE_LOOP('',(#60073,#60074,#60075,#60076));
#14418=EDGE_LOOP('',(#60077,#60078,#60079,#60080));
#14419=EDGE_LOOP('',(#60081,#60082,#60083,#60084));
#14420=EDGE_LOOP('',(#60085,#60086,#60087,#60088));
#14421=EDGE_LOOP('',(#60089,#60090,#60091,#60092));
#14422=EDGE_LOOP('',(#60093,#60094,#60095,#60096));
#14423=EDGE_LOOP('',(#60097,#60098,#60099,#60100));
#14424=EDGE_LOOP('',(#60101,#60102,#60103,#60104));
#14425=EDGE_LOOP('',(#60105,#60106,#60107,#60108));
#14426=EDGE_LOOP('',(#60109,#60110,#60111,#60112));
#14427=EDGE_LOOP('',(#60113,#60114,#60115,#60116));
#14428=EDGE_LOOP('',(#60117,#60118,#60119,#60120));
#14429=EDGE_LOOP('',(#60121,#60122,#60123,#60124));
#14430=EDGE_LOOP('',(#60125,#60126,#60127,#60128));
#14431=EDGE_LOOP('',(#60129,#60130,#60131,#60132));
#14432=EDGE_LOOP('',(#60133,#60134,#60135,#60136));
#14433=EDGE_LOOP('',(#60137,#60138,#60139,#60140));
#14434=EDGE_LOOP('',(#60141,#60142,#60143,#60144));
#14435=EDGE_LOOP('',(#60145,#60146,#60147,#60148));
#14436=EDGE_LOOP('',(#60149,#60150,#60151,#60152));
#14437=EDGE_LOOP('',(#60153,#60154,#60155,#60156));
#14438=EDGE_LOOP('',(#60157,#60158,#60159,#60160));
#14439=EDGE_LOOP('',(#60161,#60162,#60163,#60164));
#14440=EDGE_LOOP('',(#60165,#60166,#60167,#60168));
#14441=EDGE_LOOP('',(#60169,#60170,#60171,#60172));
#14442=EDGE_LOOP('',(#60173,#60174,#60175,#60176));
#14443=EDGE_LOOP('',(#60177,#60178,#60179,#60180));
#14444=EDGE_LOOP('',(#60181,#60182,#60183,#60184));
#14445=EDGE_LOOP('',(#60185,#60186,#60187,#60188));
#14446=EDGE_LOOP('',(#60189,#60190,#60191,#60192));
#14447=EDGE_LOOP('',(#60193,#60194,#60195,#60196));
#14448=EDGE_LOOP('',(#60197,#60198,#60199,#60200));
#14449=EDGE_LOOP('',(#60201,#60202,#60203,#60204));
#14450=EDGE_LOOP('',(#60205,#60206,#60207,#60208));
#14451=EDGE_LOOP('',(#60209,#60210,#60211,#60212));
#14452=EDGE_LOOP('',(#60213,#60214,#60215,#60216));
#14453=EDGE_LOOP('',(#60217,#60218,#60219,#60220));
#14454=EDGE_LOOP('',(#60221,#60222,#60223,#60224));
#14455=EDGE_LOOP('',(#60225,#60226,#60227,#60228));
#14456=EDGE_LOOP('',(#60229,#60230,#60231,#60232));
#14457=EDGE_LOOP('',(#60233,#60234,#60235,#60236));
#14458=EDGE_LOOP('',(#60237,#60238,#60239,#60240));
#14459=EDGE_LOOP('',(#60241,#60242,#60243,#60244));
#14460=EDGE_LOOP('',(#60245,#60246,#60247,#60248));
#14461=EDGE_LOOP('',(#60249,#60250,#60251,#60252));
#14462=EDGE_LOOP('',(#60253,#60254,#60255,#60256));
#14463=EDGE_LOOP('',(#60257,#60258,#60259,#60260));
#14464=EDGE_LOOP('',(#60261,#60262,#60263,#60264));
#14465=EDGE_LOOP('',(#60265,#60266,#60267,#60268));
#14466=EDGE_LOOP('',(#60269,#60270,#60271,#60272));
#14467=EDGE_LOOP('',(#60273,#60274,#60275,#60276));
#14468=EDGE_LOOP('',(#60277,#60278,#60279,#60280));
#14469=EDGE_LOOP('',(#60281,#60282,#60283,#60284));
#14470=EDGE_LOOP('',(#60285,#60286,#60287,#60288));
#14471=EDGE_LOOP('',(#60289,#60290,#60291,#60292));
#14472=EDGE_LOOP('',(#60293,#60294,#60295,#60296));
#14473=EDGE_LOOP('',(#60297,#60298,#60299,#60300));
#14474=EDGE_LOOP('',(#60301,#60302,#60303,#60304));
#14475=EDGE_LOOP('',(#60305,#60306,#60307,#60308));
#14476=EDGE_LOOP('',(#60309,#60310,#60311,#60312));
#14477=EDGE_LOOP('',(#60313,#60314,#60315,#60316));
#14478=EDGE_LOOP('',(#60317,#60318,#60319,#60320));
#14479=EDGE_LOOP('',(#60321,#60322,#60323,#60324));
#14480=EDGE_LOOP('',(#60325,#60326,#60327,#60328));
#14481=EDGE_LOOP('',(#60329,#60330,#60331,#60332));
#14482=EDGE_LOOP('',(#60333,#60334,#60335,#60336));
#14483=EDGE_LOOP('',(#60337,#60338,#60339,#60340));
#14484=EDGE_LOOP('',(#60341,#60342,#60343,#60344));
#14485=EDGE_LOOP('',(#60345,#60346,#60347,#60348));
#14486=EDGE_LOOP('',(#60349,#60350,#60351,#60352));
#14487=EDGE_LOOP('',(#60353,#60354,#60355,#60356));
#14488=EDGE_LOOP('',(#60357,#60358,#60359,#60360));
#14489=EDGE_LOOP('',(#60361,#60362,#60363,#60364));
#14490=EDGE_LOOP('',(#60365,#60366,#60367,#60368));
#14491=EDGE_LOOP('',(#60369,#60370,#60371,#60372));
#14492=EDGE_LOOP('',(#60373,#60374,#60375,#60376));
#14493=EDGE_LOOP('',(#60377,#60378,#60379,#60380));
#14494=EDGE_LOOP('',(#60381,#60382,#60383,#60384));
#14495=EDGE_LOOP('',(#60385,#60386,#60387,#60388));
#14496=EDGE_LOOP('',(#60389,#60390,#60391,#60392));
#14497=EDGE_LOOP('',(#60393,#60394,#60395,#60396));
#14498=EDGE_LOOP('',(#60397,#60398,#60399,#60400));
#14499=EDGE_LOOP('',(#60401,#60402,#60403,#60404));
#14500=EDGE_LOOP('',(#60405,#60406,#60407,#60408));
#14501=EDGE_LOOP('',(#60409,#60410,#60411,#60412));
#14502=EDGE_LOOP('',(#60413,#60414,#60415,#60416));
#14503=EDGE_LOOP('',(#60417,#60418,#60419,#60420));
#14504=EDGE_LOOP('',(#60421,#60422,#60423,#60424));
#14505=EDGE_LOOP('',(#60425,#60426,#60427,#60428));
#14506=EDGE_LOOP('',(#60429,#60430,#60431,#60432));
#14507=EDGE_LOOP('',(#60433,#60434,#60435,#60436));
#14508=EDGE_LOOP('',(#60437,#60438,#60439,#60440));
#14509=EDGE_LOOP('',(#60441,#60442,#60443,#60444));
#14510=EDGE_LOOP('',(#60445,#60446,#60447,#60448));
#14511=EDGE_LOOP('',(#60449,#60450,#60451,#60452));
#14512=EDGE_LOOP('',(#60453,#60454,#60455,#60456));
#14513=EDGE_LOOP('',(#60457,#60458,#60459,#60460));
#14514=EDGE_LOOP('',(#60461,#60462,#60463,#60464));
#14515=EDGE_LOOP('',(#60465,#60466,#60467,#60468));
#14516=EDGE_LOOP('',(#60469,#60470,#60471,#60472));
#14517=EDGE_LOOP('',(#60473,#60474,#60475,#60476));
#14518=EDGE_LOOP('',(#60477,#60478,#60479,#60480));
#14519=EDGE_LOOP('',(#60481,#60482,#60483,#60484));
#14520=EDGE_LOOP('',(#60485,#60486,#60487,#60488));
#14521=EDGE_LOOP('',(#60489,#60490,#60491,#60492));
#14522=EDGE_LOOP('',(#60493,#60494,#60495));
#14523=EDGE_LOOP('',(#60496,#60497,#60498,#60499));
#14524=EDGE_LOOP('',(#60500,#60501,#60502,#60503,#60504));
#14525=EDGE_LOOP('',(#60505,#60506,#60507,#60508));
#14526=EDGE_LOOP('',(#60509,#60510,#60511));
#14527=EDGE_LOOP('',(#60512,#60513,#60514,#60515));
#14528=EDGE_LOOP('',(#60516,#60517,#60518,#60519,#60520));
#14529=EDGE_LOOP('',(#60521,#60522,#60523,#60524));
#14530=EDGE_LOOP('',(#60525,#60526,#60527));
#14531=EDGE_LOOP('',(#60528,#60529,#60530,#60531));
#14532=EDGE_LOOP('',(#60532,#60533,#60534,#60535,#60536));
#14533=EDGE_LOOP('',(#60537,#60538,#60539,#60540));
#14534=EDGE_LOOP('',(#60541,#60542,#60543));
#14535=EDGE_LOOP('',(#60544,#60545,#60546,#60547));
#14536=EDGE_LOOP('',(#60548,#60549,#60550,#60551,#60552));
#14537=EDGE_LOOP('',(#60553,#60554,#60555,#60556));
#14538=EDGE_LOOP('',(#60557,#60558,#60559));
#14539=EDGE_LOOP('',(#60560,#60561,#60562,#60563));
#14540=EDGE_LOOP('',(#60564,#60565,#60566,#60567,#60568));
#14541=EDGE_LOOP('',(#60569,#60570,#60571,#60572));
#14542=EDGE_LOOP('',(#60573,#60574,#60575));
#14543=EDGE_LOOP('',(#60576,#60577,#60578,#60579));
#14544=EDGE_LOOP('',(#60580,#60581,#60582,#60583,#60584));
#14545=EDGE_LOOP('',(#60585,#60586,#60587,#60588));
#14546=EDGE_LOOP('',(#60589,#60590,#60591));
#14547=EDGE_LOOP('',(#60592,#60593,#60594,#60595));
#14548=EDGE_LOOP('',(#60596,#60597,#60598,#60599,#60600));
#14549=EDGE_LOOP('',(#60601,#60602,#60603,#60604));
#14550=EDGE_LOOP('',(#60605,#60606,#60607));
#14551=EDGE_LOOP('',(#60608,#60609,#60610,#60611));
#14552=EDGE_LOOP('',(#60612,#60613,#60614,#60615,#60616));
#14553=EDGE_LOOP('',(#60617,#60618,#60619,#60620));
#14554=EDGE_LOOP('',(#60621,#60622,#60623));
#14555=EDGE_LOOP('',(#60624,#60625,#60626,#60627));
#14556=EDGE_LOOP('',(#60628,#60629,#60630,#60631,#60632));
#14557=EDGE_LOOP('',(#60633,#60634,#60635,#60636));
#14558=EDGE_LOOP('',(#60637,#60638,#60639));
#14559=EDGE_LOOP('',(#60640,#60641,#60642,#60643));
#14560=EDGE_LOOP('',(#60644,#60645,#60646,#60647,#60648));
#14561=EDGE_LOOP('',(#60649,#60650,#60651,#60652));
#14562=EDGE_LOOP('',(#60653,#60654,#60655));
#14563=EDGE_LOOP('',(#60656,#60657,#60658,#60659));
#14564=EDGE_LOOP('',(#60660,#60661,#60662,#60663,#60664));
#14565=EDGE_LOOP('',(#60665,#60666,#60667,#60668));
#14566=EDGE_LOOP('',(#60669,#60670,#60671));
#14567=EDGE_LOOP('',(#60672,#60673,#60674,#60675));
#14568=EDGE_LOOP('',(#60676,#60677,#60678,#60679,#60680));
#14569=EDGE_LOOP('',(#60681,#60682,#60683,#60684));
#14570=EDGE_LOOP('',(#60685,#60686,#60687));
#14571=EDGE_LOOP('',(#60688,#60689,#60690,#60691));
#14572=EDGE_LOOP('',(#60692,#60693,#60694,#60695,#60696));
#14573=EDGE_LOOP('',(#60697,#60698,#60699,#60700));
#14574=EDGE_LOOP('',(#60701,#60702,#60703));
#14575=EDGE_LOOP('',(#60704,#60705,#60706,#60707));
#14576=EDGE_LOOP('',(#60708,#60709,#60710,#60711,#60712));
#14577=EDGE_LOOP('',(#60713,#60714,#60715,#60716));
#14578=EDGE_LOOP('',(#60717,#60718,#60719));
#14579=EDGE_LOOP('',(#60720,#60721,#60722,#60723));
#14580=EDGE_LOOP('',(#60724,#60725,#60726,#60727,#60728));
#14581=EDGE_LOOP('',(#60729,#60730,#60731,#60732));
#14582=EDGE_LOOP('',(#60733,#60734,#60735));
#14583=EDGE_LOOP('',(#60736,#60737,#60738,#60739));
#14584=EDGE_LOOP('',(#60740,#60741,#60742,#60743,#60744));
#14585=EDGE_LOOP('',(#60745,#60746,#60747,#60748));
#14586=EDGE_LOOP('',(#60749,#60750,#60751));
#14587=EDGE_LOOP('',(#60752,#60753,#60754,#60755));
#14588=EDGE_LOOP('',(#60756,#60757,#60758,#60759,#60760));
#14589=EDGE_LOOP('',(#60761,#60762,#60763,#60764));
#14590=EDGE_LOOP('',(#60765,#60766,#60767));
#14591=EDGE_LOOP('',(#60768,#60769,#60770,#60771));
#14592=EDGE_LOOP('',(#60772,#60773,#60774,#60775,#60776));
#14593=EDGE_LOOP('',(#60777,#60778,#60779,#60780));
#14594=EDGE_LOOP('',(#60781,#60782,#60783));
#14595=EDGE_LOOP('',(#60784,#60785,#60786,#60787));
#14596=EDGE_LOOP('',(#60788,#60789,#60790,#60791,#60792));
#14597=EDGE_LOOP('',(#60793,#60794,#60795,#60796));
#14598=EDGE_LOOP('',(#60797,#60798,#60799));
#14599=EDGE_LOOP('',(#60800,#60801,#60802,#60803));
#14600=EDGE_LOOP('',(#60804,#60805,#60806,#60807,#60808));
#14601=EDGE_LOOP('',(#60809,#60810,#60811,#60812));
#14602=EDGE_LOOP('',(#60813,#60814,#60815));
#14603=EDGE_LOOP('',(#60816,#60817,#60818,#60819));
#14604=EDGE_LOOP('',(#60820,#60821,#60822,#60823,#60824));
#14605=EDGE_LOOP('',(#60825,#60826,#60827,#60828));
#14606=EDGE_LOOP('',(#60829,#60830,#60831,#60832));
#14607=EDGE_LOOP('',(#60833,#60834,#60835,#60836));
#14608=EDGE_LOOP('',(#60837,#60838,#60839));
#14609=EDGE_LOOP('',(#60840,#60841,#60842,#60843));
#14610=EDGE_LOOP('',(#60844,#60845,#60846,#60847,#60848));
#14611=EDGE_LOOP('',(#60849,#60850,#60851,#60852));
#14612=EDGE_LOOP('',(#60853,#60854,#60855));
#14613=EDGE_LOOP('',(#60856,#60857,#60858,#60859));
#14614=EDGE_LOOP('',(#60860,#60861,#60862,#60863,#60864));
#14615=EDGE_LOOP('',(#60865,#60866,#60867,#60868));
#14616=EDGE_LOOP('',(#60869,#60870,#60871));
#14617=EDGE_LOOP('',(#60872,#60873,#60874,#60875));
#14618=EDGE_LOOP('',(#60876,#60877,#60878,#60879,#60880));
#14619=EDGE_LOOP('',(#60881,#60882,#60883,#60884));
#14620=EDGE_LOOP('',(#60885,#60886,#60887));
#14621=EDGE_LOOP('',(#60888,#60889,#60890,#60891));
#14622=EDGE_LOOP('',(#60892,#60893,#60894,#60895,#60896));
#14623=EDGE_LOOP('',(#60897,#60898,#60899,#60900));
#14624=EDGE_LOOP('',(#60901,#60902,#60903));
#14625=EDGE_LOOP('',(#60904,#60905,#60906,#60907));
#14626=EDGE_LOOP('',(#60908,#60909,#60910,#60911,#60912));
#14627=EDGE_LOOP('',(#60913,#60914,#60915,#60916));
#14628=EDGE_LOOP('',(#60917,#60918,#60919));
#14629=EDGE_LOOP('',(#60920,#60921,#60922,#60923));
#14630=EDGE_LOOP('',(#60924,#60925,#60926,#60927,#60928));
#14631=EDGE_LOOP('',(#60929,#60930,#60931,#60932));
#14632=EDGE_LOOP('',(#60933,#60934,#60935));
#14633=EDGE_LOOP('',(#60936,#60937,#60938,#60939));
#14634=EDGE_LOOP('',(#60940,#60941,#60942,#60943,#60944));
#14635=EDGE_LOOP('',(#60945,#60946,#60947,#60948));
#14636=EDGE_LOOP('',(#60949,#60950,#60951,#60952));
#14637=EDGE_LOOP('',(#60953,#60954,#60955,#60956));
#14638=EDGE_LOOP('',(#60957,#60958,#60959,#60960));
#14639=EDGE_LOOP('',(#60961,#60962,#60963,#60964));
#14640=EDGE_LOOP('',(#60965,#60966,#60967,#60968));
#14641=EDGE_LOOP('',(#60969,#60970,#60971,#60972));
#14642=EDGE_LOOP('',(#60973,#60974,#60975,#60976));
#14643=EDGE_LOOP('',(#60977,#60978,#60979,#60980));
#14644=EDGE_LOOP('',(#60981,#60982,#60983,#60984));
#14645=EDGE_LOOP('',(#60985,#60986,#60987,#60988));
#14646=EDGE_LOOP('',(#60989,#60990,#60991,#60992));
#14647=EDGE_LOOP('',(#60993,#60994,#60995,#60996));
#14648=EDGE_LOOP('',(#60997,#60998,#60999,#61000));
#14649=EDGE_LOOP('',(#61001,#61002,#61003,#61004));
#14650=EDGE_LOOP('',(#61005,#61006,#61007,#61008));
#14651=EDGE_LOOP('',(#61009,#61010,#61011,#61012));
#14652=EDGE_LOOP('',(#61013,#61014,#61015,#61016));
#14653=EDGE_LOOP('',(#61017,#61018,#61019,#61020));
#14654=EDGE_LOOP('',(#61021,#61022,#61023,#61024));
#14655=EDGE_LOOP('',(#61025,#61026,#61027,#61028));
#14656=EDGE_LOOP('',(#61029,#61030,#61031,#61032));
#14657=EDGE_LOOP('',(#61033,#61034,#61035,#61036));
#14658=EDGE_LOOP('',(#61037,#61038,#61039,#61040));
#14659=EDGE_LOOP('',(#61041,#61042,#61043,#61044));
#14660=EDGE_LOOP('',(#61045,#61046,#61047,#61048));
#14661=EDGE_LOOP('',(#61049,#61050,#61051,#61052));
#14662=EDGE_LOOP('',(#61053,#61054,#61055,#61056));
#14663=EDGE_LOOP('',(#61057,#61058,#61059,#61060));
#14664=EDGE_LOOP('',(#61061,#61062,#61063,#61064));
#14665=EDGE_LOOP('',(#61065,#61066,#61067,#61068));
#14666=EDGE_LOOP('',(#61069,#61070,#61071,#61072));
#14667=EDGE_LOOP('',(#61073,#61074,#61075,#61076));
#14668=EDGE_LOOP('',(#61077,#61078,#61079,#61080));
#14669=EDGE_LOOP('',(#61081,#61082,#61083,#61084));
#14670=EDGE_LOOP('',(#61085,#61086,#61087,#61088));
#14671=EDGE_LOOP('',(#61089,#61090,#61091,#61092));
#14672=EDGE_LOOP('',(#61093,#61094,#61095,#61096));
#14673=EDGE_LOOP('',(#61097,#61098,#61099,#61100));
#14674=EDGE_LOOP('',(#61101,#61102,#61103,#61104));
#14675=EDGE_LOOP('',(#61105,#61106,#61107,#61108));
#14676=EDGE_LOOP('',(#61109,#61110,#61111,#61112));
#14677=EDGE_LOOP('',(#61113,#61114,#61115,#61116));
#14678=EDGE_LOOP('',(#61117,#61118,#61119,#61120));
#14679=EDGE_LOOP('',(#61121,#61122,#61123,#61124));
#14680=EDGE_LOOP('',(#61125,#61126,#61127,#61128));
#14681=EDGE_LOOP('',(#61129,#61130,#61131,#61132));
#14682=EDGE_LOOP('',(#61133,#61134,#61135,#61136));
#14683=EDGE_LOOP('',(#61137,#61138,#61139,#61140));
#14684=EDGE_LOOP('',(#61141,#61142,#61143,#61144));
#14685=EDGE_LOOP('',(#61145,#61146,#61147,#61148));
#14686=EDGE_LOOP('',(#61149,#61150,#61151,#61152));
#14687=EDGE_LOOP('',(#61153,#61154,#61155,#61156));
#14688=EDGE_LOOP('',(#61157,#61158,#61159,#61160));
#14689=EDGE_LOOP('',(#61161,#61162,#61163,#61164));
#14690=EDGE_LOOP('',(#61165,#61166,#61167,#61168));
#14691=EDGE_LOOP('',(#61169,#61170,#61171,#61172));
#14692=EDGE_LOOP('',(#61173,#61174,#61175,#61176));
#14693=EDGE_LOOP('',(#61177,#61178,#61179,#61180,#61181));
#14694=EDGE_LOOP('',(#61182,#61183,#61184,#61185,#61186));
#14695=EDGE_LOOP('',(#61187,#61188,#61189,#61190,#61191));
#14696=EDGE_LOOP('',(#61192,#61193,#61194,#61195,#61196));
#14697=EDGE_LOOP('',(#61197,#61198,#61199,#61200,#61201));
#14698=EDGE_LOOP('',(#61202,#61203,#61204,#61205,#61206));
#14699=EDGE_LOOP('',(#61207,#61208,#61209,#61210,#61211));
#14700=EDGE_LOOP('',(#61212,#61213,#61214,#61215,#61216));
#14701=EDGE_LOOP('',(#61217,#61218,#61219,#61220,#61221));
#14702=EDGE_LOOP('',(#61222,#61223,#61224,#61225,#61226));
#14703=EDGE_LOOP('',(#61227,#61228,#61229,#61230,#61231));
#14704=EDGE_LOOP('',(#61232,#61233,#61234,#61235,#61236));
#14705=EDGE_LOOP('',(#61237,#61238,#61239,#61240,#61241));
#14706=EDGE_LOOP('',(#61242,#61243,#61244,#61245,#61246));
#14707=EDGE_LOOP('',(#61247,#61248,#61249,#61250,#61251));
#14708=EDGE_LOOP('',(#61252,#61253,#61254,#61255,#61256));
#14709=EDGE_LOOP('',(#61257,#61258,#61259,#61260,#61261));
#14710=EDGE_LOOP('',(#61262,#61263,#61264,#61265,#61266));
#14711=EDGE_LOOP('',(#61267,#61268,#61269,#61270,#61271));
#14712=EDGE_LOOP('',(#61272,#61273,#61274,#61275,#61276));
#14713=EDGE_LOOP('',(#61277,#61278,#61279,#61280,#61281));
#14714=EDGE_LOOP('',(#61282,#61283,#61284,#61285,#61286));
#14715=EDGE_LOOP('',(#61287,#61288,#61289,#61290,#61291));
#14716=EDGE_LOOP('',(#61292,#61293,#61294,#61295,#61296));
#14717=EDGE_LOOP('',(#61297,#61298,#61299,#61300,#61301));
#14718=EDGE_LOOP('',(#61302,#61303,#61304,#61305,#61306));
#14719=EDGE_LOOP('',(#61307,#61308,#61309,#61310,#61311));
#14720=EDGE_LOOP('',(#61312,#61313,#61314,#61315,#61316));
#14721=EDGE_LOOP('',(#61317,#61318,#61319,#61320,#61321));
#14722=EDGE_LOOP('',(#61322,#61323,#61324,#61325,#61326));
#14723=EDGE_LOOP('',(#61327,#61328,#61329,#61330,#61331));
#14724=EDGE_LOOP('',(#61332,#61333,#61334,#61335,#61336));
#14725=EDGE_LOOP('',(#61337,#61338,#61339,#61340,#61341));
#14726=EDGE_LOOP('',(#61342,#61343,#61344,#61345,#61346));
#14727=EDGE_LOOP('',(#61347,#61348,#61349,#61350,#61351));
#14728=EDGE_LOOP('',(#61352,#61353,#61354,#61355,#61356));
#14729=EDGE_LOOP('',(#61357,#61358,#61359,#61360,#61361));
#14730=EDGE_LOOP('',(#61362,#61363,#61364,#61365,#61366));
#14731=EDGE_LOOP('',(#61367,#61368,#61369,#61370,#61371));
#14732=EDGE_LOOP('',(#61372,#61373,#61374,#61375,#61376));
#14733=EDGE_LOOP('',(#61377,#61378,#61379,#61380,#61381));
#14734=EDGE_LOOP('',(#61382,#61383,#61384,#61385,#61386));
#14735=EDGE_LOOP('',(#61387,#61388,#61389,#61390,#61391));
#14736=EDGE_LOOP('',(#61392,#61393,#61394,#61395,#61396));
#14737=EDGE_LOOP('',(#61397,#61398,#61399,#61400,#61401));
#14738=EDGE_LOOP('',(#61402,#61403,#61404,#61405,#61406));
#14739=EDGE_LOOP('',(#61407,#61408,#61409,#61410,#61411));
#14740=EDGE_LOOP('',(#61412,#61413,#61414,#61415,#61416));
#14741=EDGE_LOOP('',(#61417,#61418,#61419,#61420,#61421));
#14742=EDGE_LOOP('',(#61422,#61423,#61424,#61425,#61426));
#14743=EDGE_LOOP('',(#61427,#61428,#61429,#61430,#61431));
#14744=EDGE_LOOP('',(#61432,#61433,#61434,#61435,#61436));
#14745=EDGE_LOOP('',(#61437,#61438,#61439,#61440,#61441));
#14746=EDGE_LOOP('',(#61442,#61443,#61444,#61445,#61446));
#14747=EDGE_LOOP('',(#61447,#61448,#61449,#61450,#61451));
#14748=EDGE_LOOP('',(#61452,#61453,#61454,#61455,#61456));
#14749=EDGE_LOOP('',(#61457,#61458,#61459,#61460,#61461));
#14750=EDGE_LOOP('',(#61462,#61463,#61464,#61465,#61466));
#14751=EDGE_LOOP('',(#61467,#61468,#61469,#61470));
#14752=EDGE_LOOP('',(#61471,#61472,#61473,#61474));
#14753=EDGE_LOOP('',(#61475,#61476,#61477,#61478));
#14754=EDGE_LOOP('',(#61479,#61480,#61481,#61482));
#14755=EDGE_LOOP('',(#61483,#61484,#61485,#61486));
#14756=EDGE_LOOP('',(#61487,#61488,#61489,#61490));
#14757=EDGE_LOOP('',(#61491,#61492,#61493,#61494));
#14758=EDGE_LOOP('',(#61495,#61496,#61497,#61498));
#14759=EDGE_LOOP('',(#61499,#61500,#61501,#61502));
#14760=EDGE_LOOP('',(#61503,#61504,#61505,#61506));
#14761=EDGE_LOOP('',(#61507,#61508,#61509,#61510));
#14762=EDGE_LOOP('',(#61511,#61512,#61513,#61514));
#14763=EDGE_LOOP('',(#61515,#61516,#61517,#61518));
#14764=EDGE_LOOP('',(#61519,#61520,#61521,#61522));
#14765=EDGE_LOOP('',(#61523,#61524,#61525,#61526));
#14766=EDGE_LOOP('',(#61527,#61528,#61529,#61530));
#14767=EDGE_LOOP('',(#61531,#61532,#61533,#61534));
#14768=EDGE_LOOP('',(#61535,#61536,#61537,#61538));
#14769=EDGE_LOOP('',(#61539,#61540,#61541,#61542));
#14770=EDGE_LOOP('',(#61543,#61544,#61545,#61546));
#14771=EDGE_LOOP('',(#61547,#61548,#61549,#61550));
#14772=EDGE_LOOP('',(#61551,#61552,#61553,#61554));
#14773=EDGE_LOOP('',(#61555,#61556,#61557,#61558));
#14774=EDGE_LOOP('',(#61559,#61560,#61561,#61562));
#14775=EDGE_LOOP('',(#61563,#61564,#61565,#61566));
#14776=EDGE_LOOP('',(#61567,#61568,#61569,#61570));
#14777=EDGE_LOOP('',(#61571,#61572,#61573,#61574));
#14778=EDGE_LOOP('',(#61575,#61576,#61577,#61578));
#14779=EDGE_LOOP('',(#61579,#61580,#61581,#61582));
#14780=EDGE_LOOP('',(#61583,#61584,#61585,#61586));
#14781=EDGE_LOOP('',(#61587,#61588,#61589,#61590));
#14782=EDGE_LOOP('',(#61591,#61592,#61593,#61594));
#14783=EDGE_LOOP('',(#61595,#61596,#61597,#61598));
#14784=EDGE_LOOP('',(#61599,#61600,#61601,#61602));
#14785=EDGE_LOOP('',(#61603,#61604,#61605,#61606));
#14786=EDGE_LOOP('',(#61607,#61608,#61609,#61610));
#14787=EDGE_LOOP('',(#61611,#61612,#61613,#61614));
#14788=EDGE_LOOP('',(#61615,#61616,#61617,#61618));
#14789=EDGE_LOOP('',(#61619,#61620,#61621,#61622));
#14790=EDGE_LOOP('',(#61623,#61624,#61625,#61626));
#14791=EDGE_LOOP('',(#61627,#61628,#61629,#61630));
#14792=EDGE_LOOP('',(#61631,#61632,#61633,#61634));
#14793=EDGE_LOOP('',(#61635,#61636,#61637,#61638));
#14794=EDGE_LOOP('',(#61639,#61640,#61641,#61642));
#14795=EDGE_LOOP('',(#61643,#61644,#61645,#61646));
#14796=EDGE_LOOP('',(#61647,#61648,#61649,#61650));
#14797=EDGE_LOOP('',(#61651,#61652,#61653,#61654));
#14798=EDGE_LOOP('',(#61655,#61656,#61657,#61658));
#14799=EDGE_LOOP('',(#61659,#61660,#61661,#61662));
#14800=EDGE_LOOP('',(#61663,#61664,#61665,#61666));
#14801=EDGE_LOOP('',(#61667,#61668,#61669,#61670));
#14802=EDGE_LOOP('',(#61671,#61672,#61673,#61674));
#14803=EDGE_LOOP('',(#61675,#61676,#61677,#61678));
#14804=EDGE_LOOP('',(#61679,#61680,#61681,#61682));
#14805=EDGE_LOOP('',(#61683,#61684,#61685,#61686));
#14806=EDGE_LOOP('',(#61687,#61688,#61689,#61690));
#14807=EDGE_LOOP('',(#61691,#61692,#61693,#61694));
#14808=EDGE_LOOP('',(#61695,#61696,#61697,#61698));
#14809=EDGE_LOOP('',(#61699,#61700,#61701,#61702));
#14810=EDGE_LOOP('',(#61703,#61704,#61705,#61706));
#14811=EDGE_LOOP('',(#61707,#61708,#61709,#61710));
#14812=EDGE_LOOP('',(#61711,#61712,#61713,#61714));
#14813=EDGE_LOOP('',(#61715,#61716,#61717,#61718));
#14814=EDGE_LOOP('',(#61719,#61720,#61721,#61722));
#14815=EDGE_LOOP('',(#61723,#61724,#61725,#61726));
#14816=EDGE_LOOP('',(#61727,#61728,#61729,#61730));
#14817=EDGE_LOOP('',(#61731,#61732,#61733,#61734));
#14818=EDGE_LOOP('',(#61735,#61736,#61737,#61738));
#14819=EDGE_LOOP('',(#61739,#61740,#61741,#61742));
#14820=EDGE_LOOP('',(#61743,#61744,#61745,#61746));
#14821=EDGE_LOOP('',(#61747,#61748,#61749,#61750));
#14822=EDGE_LOOP('',(#61751,#61752,#61753,#61754));
#14823=EDGE_LOOP('',(#61755,#61756,#61757,#61758));
#14824=EDGE_LOOP('',(#61759,#61760,#61761,#61762));
#14825=EDGE_LOOP('',(#61763,#61764,#61765,#61766));
#14826=EDGE_LOOP('',(#61767,#61768,#61769,#61770));
#14827=EDGE_LOOP('',(#61771,#61772,#61773,#61774));
#14828=EDGE_LOOP('',(#61775,#61776,#61777,#61778));
#14829=EDGE_LOOP('',(#61779,#61780,#61781,#61782));
#14830=EDGE_LOOP('',(#61783,#61784,#61785,#61786));
#14831=EDGE_LOOP('',(#61787,#61788,#61789,#61790));
#14832=EDGE_LOOP('',(#61791,#61792,#61793,#61794));
#14833=EDGE_LOOP('',(#61795,#61796,#61797,#61798));
#14834=EDGE_LOOP('',(#61799,#61800,#61801,#61802));
#14835=EDGE_LOOP('',(#61803,#61804,#61805,#61806));
#14836=EDGE_LOOP('',(#61807,#61808,#61809,#61810));
#14837=EDGE_LOOP('',(#61811,#61812,#61813,#61814));
#14838=EDGE_LOOP('',(#61815,#61816,#61817,#61818));
#14839=EDGE_LOOP('',(#61819,#61820,#61821,#61822));
#14840=EDGE_LOOP('',(#61823,#61824,#61825,#61826));
#14841=EDGE_LOOP('',(#61827,#61828,#61829,#61830));
#14842=EDGE_LOOP('',(#61831,#61832,#61833,#61834));
#14843=EDGE_LOOP('',(#61835,#61836,#61837,#61838));
#14844=EDGE_LOOP('',(#61839,#61840,#61841,#61842));
#14845=EDGE_LOOP('',(#61843,#61844,#61845,#61846));
#14846=EDGE_LOOP('',(#61847,#61848,#61849,#61850));
#14847=EDGE_LOOP('',(#61851,#61852,#61853,#61854));
#14848=EDGE_LOOP('',(#61855,#61856,#61857,#61858));
#14849=EDGE_LOOP('',(#61859,#61860,#61861,#61862));
#14850=EDGE_LOOP('',(#61863,#61864,#61865,#61866));
#14851=EDGE_LOOP('',(#61867,#61868,#61869,#61870));
#14852=EDGE_LOOP('',(#61871,#61872,#61873,#61874));
#14853=EDGE_LOOP('',(#61875,#61876,#61877,#61878));
#14854=EDGE_LOOP('',(#61879,#61880,#61881,#61882));
#14855=EDGE_LOOP('',(#61883,#61884,#61885,#61886));
#14856=EDGE_LOOP('',(#61887,#61888,#61889,#61890));
#14857=EDGE_LOOP('',(#61891,#61892,#61893,#61894));
#14858=EDGE_LOOP('',(#61895,#61896,#61897,#61898));
#14859=EDGE_LOOP('',(#61899,#61900,#61901,#61902));
#14860=EDGE_LOOP('',(#61903,#61904,#61905,#61906));
#14861=EDGE_LOOP('',(#61907,#61908,#61909,#61910));
#14862=EDGE_LOOP('',(#61911,#61912,#61913,#61914));
#14863=EDGE_LOOP('',(#61915,#61916,#61917,#61918));
#14864=EDGE_LOOP('',(#61919,#61920,#61921,#61922));
#14865=EDGE_LOOP('',(#61923,#61924,#61925,#61926));
#14866=EDGE_LOOP('',(#61927,#61928,#61929,#61930));
#14867=EDGE_LOOP('',(#61931,#61932,#61933,#61934));
#14868=EDGE_LOOP('',(#61935,#61936,#61937,#61938));
#14869=EDGE_LOOP('',(#61939,#61940,#61941,#61942));
#14870=EDGE_LOOP('',(#61943,#61944,#61945,#61946));
#14871=EDGE_LOOP('',(#61947,#61948,#61949,#61950));
#14872=EDGE_LOOP('',(#61951,#61952,#61953,#61954));
#14873=EDGE_LOOP('',(#61955,#61956,#61957,#61958));
#14874=EDGE_LOOP('',(#61959,#61960,#61961,#61962));
#14875=EDGE_LOOP('',(#61963,#61964,#61965,#61966));
#14876=EDGE_LOOP('',(#61967,#61968,#61969,#61970));
#14877=EDGE_LOOP('',(#61971,#61972,#61973,#61974));
#14878=EDGE_LOOP('',(#61975,#61976,#61977,#61978));
#14879=EDGE_LOOP('',(#61979,#61980,#61981,#61982));
#14880=EDGE_LOOP('',(#61983,#61984,#61985,#61986));
#14881=EDGE_LOOP('',(#61987,#61988,#61989,#61990));
#14882=EDGE_LOOP('',(#61991,#61992,#61993,#61994));
#14883=EDGE_LOOP('',(#61995,#61996,#61997,#61998));
#14884=EDGE_LOOP('',(#61999,#62000,#62001,#62002));
#14885=EDGE_LOOP('',(#62003,#62004,#62005,#62006));
#14886=EDGE_LOOP('',(#62007,#62008,#62009,#62010));
#14887=EDGE_LOOP('',(#62011,#62012,#62013,#62014));
#14888=EDGE_LOOP('',(#62015,#62016,#62017,#62018));
#14889=EDGE_LOOP('',(#62019,#62020,#62021,#62022));
#14890=EDGE_LOOP('',(#62023,#62024,#62025,#62026));
#14891=EDGE_LOOP('',(#62027,#62028,#62029,#62030));
#14892=EDGE_LOOP('',(#62031,#62032,#62033,#62034));
#14893=EDGE_LOOP('',(#62035,#62036,#62037,#62038));
#14894=EDGE_LOOP('',(#62039,#62040,#62041,#62042));
#14895=EDGE_LOOP('',(#62043,#62044,#62045,#62046));
#14896=EDGE_LOOP('',(#62047,#62048,#62049,#62050));
#14897=EDGE_LOOP('',(#62051,#62052,#62053,#62054));
#14898=EDGE_LOOP('',(#62055,#62056,#62057,#62058));
#14899=EDGE_LOOP('',(#62059,#62060,#62061,#62062));
#14900=EDGE_LOOP('',(#62063,#62064,#62065,#62066));
#14901=EDGE_LOOP('',(#62067,#62068,#62069,#62070));
#14902=EDGE_LOOP('',(#62071,#62072,#62073,#62074));
#14903=EDGE_LOOP('',(#62075,#62076,#62077,#62078));
#14904=EDGE_LOOP('',(#62079,#62080,#62081,#62082));
#14905=EDGE_LOOP('',(#62083,#62084,#62085,#62086));
#14906=EDGE_LOOP('',(#62087,#62088,#62089,#62090));
#14907=EDGE_LOOP('',(#62091,#62092,#62093,#62094));
#14908=EDGE_LOOP('',(#62095,#62096,#62097,#62098));
#14909=EDGE_LOOP('',(#62099,#62100,#62101,#62102));
#14910=EDGE_LOOP('',(#62103,#62104,#62105,#62106));
#14911=EDGE_LOOP('',(#62107,#62108,#62109,#62110));
#14912=EDGE_LOOP('',(#62111,#62112,#62113,#62114));
#14913=EDGE_LOOP('',(#62115,#62116,#62117,#62118));
#14914=EDGE_LOOP('',(#62119,#62120,#62121,#62122));
#14915=EDGE_LOOP('',(#62123,#62124,#62125,#62126));
#14916=EDGE_LOOP('',(#62127,#62128,#62129,#62130));
#14917=EDGE_LOOP('',(#62131,#62132,#62133,#62134));
#14918=EDGE_LOOP('',(#62135,#62136,#62137,#62138));
#14919=EDGE_LOOP('',(#62139,#62140,#62141,#62142));
#14920=EDGE_LOOP('',(#62143,#62144,#62145,#62146));
#14921=EDGE_LOOP('',(#62147,#62148,#62149,#62150));
#14922=EDGE_LOOP('',(#62151,#62152,#62153,#62154));
#14923=EDGE_LOOP('',(#62155,#62156,#62157,#62158));
#14924=EDGE_LOOP('',(#62159,#62160,#62161,#62162));
#14925=EDGE_LOOP('',(#62163,#62164,#62165,#62166));
#14926=EDGE_LOOP('',(#62167,#62168,#62169,#62170));
#14927=EDGE_LOOP('',(#62171,#62172,#62173,#62174));
#14928=EDGE_LOOP('',(#62175,#62176,#62177,#62178));
#14929=EDGE_LOOP('',(#62179,#62180,#62181,#62182));
#14930=EDGE_LOOP('',(#62183,#62184,#62185,#62186));
#14931=EDGE_LOOP('',(#62187,#62188,#62189,#62190));
#14932=EDGE_LOOP('',(#62191,#62192,#62193,#62194));
#14933=EDGE_LOOP('',(#62195,#62196,#62197,#62198));
#14934=EDGE_LOOP('',(#62199,#62200,#62201,#62202));
#14935=EDGE_LOOP('',(#62203,#62204,#62205,#62206));
#14936=EDGE_LOOP('',(#62207,#62208,#62209,#62210));
#14937=EDGE_LOOP('',(#62211,#62212,#62213,#62214));
#14938=EDGE_LOOP('',(#62215,#62216,#62217,#62218));
#14939=EDGE_LOOP('',(#62219,#62220,#62221,#62222));
#14940=EDGE_LOOP('',(#62223,#62224,#62225,#62226));
#14941=EDGE_LOOP('',(#62227,#62228,#62229,#62230));
#14942=EDGE_LOOP('',(#62231,#62232,#62233,#62234));
#14943=EDGE_LOOP('',(#62235,#62236,#62237,#62238));
#14944=EDGE_LOOP('',(#62239,#62240,#62241,#62242));
#14945=EDGE_LOOP('',(#62243,#62244,#62245,#62246));
#14946=EDGE_LOOP('',(#62247,#62248,#62249,#62250));
#14947=EDGE_LOOP('',(#62251,#62252,#62253,#62254));
#14948=EDGE_LOOP('',(#62255,#62256,#62257,#62258));
#14949=EDGE_LOOP('',(#62259,#62260,#62261,#62262));
#14950=EDGE_LOOP('',(#62263,#62264,#62265,#62266));
#14951=EDGE_LOOP('',(#62267,#62268,#62269,#62270));
#14952=EDGE_LOOP('',(#62271,#62272,#62273,#62274));
#14953=EDGE_LOOP('',(#62275,#62276,#62277,#62278));
#14954=EDGE_LOOP('',(#62279,#62280,#62281,#62282));
#14955=EDGE_LOOP('',(#62283,#62284,#62285,#62286));
#14956=EDGE_LOOP('',(#62287,#62288,#62289,#62290));
#14957=EDGE_LOOP('',(#62291,#62292,#62293,#62294));
#14958=EDGE_LOOP('',(#62295,#62296,#62297,#62298));
#14959=EDGE_LOOP('',(#62299,#62300,#62301,#62302));
#14960=EDGE_LOOP('',(#62303,#62304,#62305,#62306));
#14961=EDGE_LOOP('',(#62307,#62308,#62309,#62310));
#14962=EDGE_LOOP('',(#62311,#62312,#62313,#62314));
#14963=EDGE_LOOP('',(#62315,#62316,#62317,#62318));
#14964=EDGE_LOOP('',(#62319,#62320,#62321,#62322));
#14965=EDGE_LOOP('',(#62323,#62324,#62325,#62326));
#14966=EDGE_LOOP('',(#62327,#62328,#62329,#62330));
#14967=EDGE_LOOP('',(#62331,#62332,#62333,#62334));
#14968=EDGE_LOOP('',(#62335,#62336,#62337,#62338));
#14969=EDGE_LOOP('',(#62339,#62340,#62341,#62342));
#14970=EDGE_LOOP('',(#62343,#62344,#62345,#62346));
#14971=EDGE_LOOP('',(#62347,#62348,#62349,#62350));
#14972=EDGE_LOOP('',(#62351,#62352,#62353,#62354));
#14973=EDGE_LOOP('',(#62355,#62356,#62357,#62358));
#14974=EDGE_LOOP('',(#62359,#62360,#62361,#62362));
#14975=EDGE_LOOP('',(#62363,#62364,#62365,#62366));
#14976=EDGE_LOOP('',(#62367,#62368,#62369,#62370));
#14977=EDGE_LOOP('',(#62371,#62372,#62373,#62374));
#14978=EDGE_LOOP('',(#62375,#62376,#62377,#62378));
#14979=EDGE_LOOP('',(#62379,#62380,#62381,#62382));
#14980=EDGE_LOOP('',(#62383,#62384,#62385,#62386));
#14981=EDGE_LOOP('',(#62387,#62388,#62389,#62390));
#14982=EDGE_LOOP('',(#62391,#62392,#62393,#62394));
#14983=EDGE_LOOP('',(#62395,#62396,#62397,#62398));
#14984=EDGE_LOOP('',(#62399,#62400,#62401,#62402));
#14985=EDGE_LOOP('',(#62403,#62404,#62405,#62406));
#14986=EDGE_LOOP('',(#62407,#62408,#62409,#62410));
#14987=EDGE_LOOP('',(#62411,#62412,#62413,#62414));
#14988=EDGE_LOOP('',(#62415,#62416,#62417,#62418));
#14989=EDGE_LOOP('',(#62419,#62420,#62421,#62422));
#14990=EDGE_LOOP('',(#62423,#62424,#62425,#62426));
#14991=EDGE_LOOP('',(#62427,#62428,#62429,#62430));
#14992=EDGE_LOOP('',(#62431,#62432,#62433,#62434));
#14993=EDGE_LOOP('',(#62435,#62436,#62437,#62438));
#14994=EDGE_LOOP('',(#62439,#62440,#62441,#62442));
#14995=EDGE_LOOP('',(#62443,#62444,#62445,#62446));
#14996=EDGE_LOOP('',(#62447,#62448,#62449,#62450));
#14997=EDGE_LOOP('',(#62451,#62452,#62453,#62454));
#14998=EDGE_LOOP('',(#62455,#62456,#62457,#62458));
#14999=EDGE_LOOP('',(#62459,#62460,#62461,#62462));
#15000=EDGE_LOOP('',(#62463,#62464,#62465,#62466));
#15001=EDGE_LOOP('',(#62467,#62468,#62469,#62470));
#15002=EDGE_LOOP('',(#62471,#62472,#62473,#62474));
#15003=EDGE_LOOP('',(#62475,#62476,#62477,#62478));
#15004=EDGE_LOOP('',(#62479,#62480,#62481,#62482));
#15005=EDGE_LOOP('',(#62483,#62484,#62485,#62486));
#15006=EDGE_LOOP('',(#62487,#62488,#62489,#62490));
#15007=EDGE_LOOP('',(#62491,#62492,#62493,#62494));
#15008=EDGE_LOOP('',(#62495,#62496,#62497,#62498));
#15009=EDGE_LOOP('',(#62499,#62500,#62501,#62502));
#15010=EDGE_LOOP('',(#62503,#62504,#62505,#62506));
#15011=EDGE_LOOP('',(#62507,#62508,#62509,#62510));
#15012=EDGE_LOOP('',(#62511,#62512,#62513,#62514));
#15013=EDGE_LOOP('',(#62515,#62516,#62517,#62518));
#15014=EDGE_LOOP('',(#62519,#62520,#62521,#62522));
#15015=EDGE_LOOP('',(#62523,#62524,#62525,#62526));
#15016=EDGE_LOOP('',(#62527,#62528,#62529,#62530));
#15017=EDGE_LOOP('',(#62531,#62532,#62533,#62534));
#15018=EDGE_LOOP('',(#62535,#62536,#62537,#62538));
#15019=EDGE_LOOP('',(#62539,#62540,#62541,#62542));
#15020=EDGE_LOOP('',(#62543,#62544,#62545,#62546));
#15021=EDGE_LOOP('',(#62547,#62548,#62549,#62550));
#15022=EDGE_LOOP('',(#62551,#62552,#62553,#62554));
#15023=EDGE_LOOP('',(#62555,#62556,#62557,#62558));
#15024=EDGE_LOOP('',(#62559,#62560,#62561,#62562));
#15025=EDGE_LOOP('',(#62563,#62564,#62565,#62566));
#15026=EDGE_LOOP('',(#62567,#62568,#62569,#62570));
#15027=EDGE_LOOP('',(#62571,#62572,#62573,#62574));
#15028=EDGE_LOOP('',(#62575,#62576,#62577,#62578));
#15029=EDGE_LOOP('',(#62579,#62580,#62581,#62582));
#15030=EDGE_LOOP('',(#62583,#62584,#62585,#62586));
#15031=EDGE_LOOP('',(#62587,#62588,#62589,#62590));
#15032=EDGE_LOOP('',(#62591,#62592,#62593,#62594));
#15033=EDGE_LOOP('',(#62595,#62596,#62597,#62598));
#15034=EDGE_LOOP('',(#62599,#62600,#62601,#62602));
#15035=EDGE_LOOP('',(#62603,#62604,#62605,#62606));
#15036=EDGE_LOOP('',(#62607,#62608,#62609,#62610));
#15037=EDGE_LOOP('',(#62611,#62612,#62613,#62614));
#15038=EDGE_LOOP('',(#62615,#62616,#62617,#62618));
#15039=EDGE_LOOP('',(#62619,#62620,#62621,#62622));
#15040=EDGE_LOOP('',(#62623,#62624,#62625,#62626));
#15041=EDGE_LOOP('',(#62627,#62628,#62629,#62630));
#15042=EDGE_LOOP('',(#62631,#62632,#62633,#62634));
#15043=EDGE_LOOP('',(#62635,#62636,#62637,#62638));
#15044=EDGE_LOOP('',(#62639,#62640,#62641,#62642));
#15045=EDGE_LOOP('',(#62643,#62644,#62645,#62646));
#15046=EDGE_LOOP('',(#62647,#62648,#62649,#62650));
#15047=EDGE_LOOP('',(#62651,#62652,#62653,#62654));
#15048=EDGE_LOOP('',(#62655,#62656,#62657,#62658));
#15049=EDGE_LOOP('',(#62659,#62660,#62661,#62662));
#15050=EDGE_LOOP('',(#62663,#62664,#62665,#62666));
#15051=EDGE_LOOP('',(#62667,#62668,#62669,#62670));
#15052=EDGE_LOOP('',(#62671,#62672,#62673,#62674));
#15053=EDGE_LOOP('',(#62675,#62676,#62677,#62678));
#15054=EDGE_LOOP('',(#62679,#62680,#62681,#62682));
#15055=EDGE_LOOP('',(#62683,#62684,#62685,#62686));
#15056=EDGE_LOOP('',(#62687,#62688,#62689,#62690));
#15057=EDGE_LOOP('',(#62691,#62692,#62693,#62694));
#15058=EDGE_LOOP('',(#62695,#62696,#62697,#62698));
#15059=EDGE_LOOP('',(#62699,#62700,#62701,#62702));
#15060=EDGE_LOOP('',(#62703,#62704,#62705,#62706));
#15061=EDGE_LOOP('',(#62707,#62708,#62709,#62710));
#15062=EDGE_LOOP('',(#62711,#62712,#62713,#62714));
#15063=EDGE_LOOP('',(#62715,#62716,#62717,#62718));
#15064=EDGE_LOOP('',(#62719,#62720,#62721,#62722));
#15065=EDGE_LOOP('',(#62723,#62724,#62725,#62726));
#15066=EDGE_LOOP('',(#62727,#62728,#62729,#62730));
#15067=EDGE_LOOP('',(#62731,#62732,#62733,#62734));
#15068=EDGE_LOOP('',(#62735,#62736,#62737,#62738));
#15069=EDGE_LOOP('',(#62739,#62740,#62741,#62742));
#15070=EDGE_LOOP('',(#62743,#62744,#62745,#62746));
#15071=EDGE_LOOP('',(#62747,#62748,#62749,#62750));
#15072=EDGE_LOOP('',(#62751,#62752,#62753,#62754));
#15073=EDGE_LOOP('',(#62755,#62756,#62757,#62758));
#15074=EDGE_LOOP('',(#62759,#62760,#62761,#62762));
#15075=EDGE_LOOP('',(#62763,#62764,#62765,#62766));
#15076=EDGE_LOOP('',(#62767,#62768,#62769,#62770));
#15077=EDGE_LOOP('',(#62771,#62772,#62773,#62774));
#15078=EDGE_LOOP('',(#62775,#62776,#62777,#62778));
#15079=EDGE_LOOP('',(#62779,#62780,#62781,#62782));
#15080=EDGE_LOOP('',(#62783,#62784,#62785,#62786));
#15081=EDGE_LOOP('',(#62787,#62788,#62789,#62790));
#15082=EDGE_LOOP('',(#62791,#62792,#62793,#62794));
#15083=EDGE_LOOP('',(#62795,#62796,#62797,#62798));
#15084=EDGE_LOOP('',(#62799,#62800,#62801,#62802));
#15085=EDGE_LOOP('',(#62803,#62804,#62805,#62806));
#15086=EDGE_LOOP('',(#62807,#62808,#62809,#62810));
#15087=EDGE_LOOP('',(#62811,#62812,#62813,#62814));
#15088=EDGE_LOOP('',(#62815,#62816,#62817,#62818));
#15089=EDGE_LOOP('',(#62819,#62820,#62821,#62822));
#15090=EDGE_LOOP('',(#62823,#62824,#62825,#62826));
#15091=EDGE_LOOP('',(#62827,#62828,#62829,#62830));
#15092=EDGE_LOOP('',(#62831,#62832,#62833,#62834));
#15093=EDGE_LOOP('',(#62835,#62836,#62837,#62838));
#15094=EDGE_LOOP('',(#62839,#62840,#62841,#62842));
#15095=EDGE_LOOP('',(#62843,#62844,#62845,#62846));
#15096=EDGE_LOOP('',(#62847,#62848,#62849,#62850));
#15097=EDGE_LOOP('',(#62851,#62852,#62853,#62854));
#15098=EDGE_LOOP('',(#62855,#62856,#62857,#62858));
#15099=EDGE_LOOP('',(#62859,#62860,#62861,#62862));
#15100=EDGE_LOOP('',(#62863,#62864,#62865,#62866));
#15101=EDGE_LOOP('',(#62867,#62868,#62869,#62870));
#15102=EDGE_LOOP('',(#62871,#62872,#62873,#62874));
#15103=EDGE_LOOP('',(#62875,#62876,#62877,#62878));
#15104=EDGE_LOOP('',(#62879,#62880,#62881,#62882));
#15105=EDGE_LOOP('',(#62883,#62884,#62885,#62886));
#15106=EDGE_LOOP('',(#62887,#62888,#62889,#62890));
#15107=EDGE_LOOP('',(#62891,#62892,#62893,#62894));
#15108=EDGE_LOOP('',(#62895,#62896,#62897,#62898));
#15109=EDGE_LOOP('',(#62899,#62900,#62901,#62902));
#15110=EDGE_LOOP('',(#62903,#62904,#62905,#62906));
#15111=EDGE_LOOP('',(#62907,#62908,#62909,#62910));
#15112=EDGE_LOOP('',(#62911,#62912,#62913,#62914));
#15113=EDGE_LOOP('',(#62915,#62916,#62917,#62918));
#15114=EDGE_LOOP('',(#62919,#62920,#62921,#62922));
#15115=EDGE_LOOP('',(#62923,#62924,#62925,#62926));
#15116=EDGE_LOOP('',(#62927,#62928,#62929,#62930));
#15117=EDGE_LOOP('',(#62931,#62932,#62933,#62934));
#15118=EDGE_LOOP('',(#62935,#62936,#62937,#62938));
#15119=EDGE_LOOP('',(#62939,#62940,#62941,#62942));
#15120=EDGE_LOOP('',(#62943,#62944,#62945,#62946));
#15121=EDGE_LOOP('',(#62947,#62948,#62949,#62950));
#15122=EDGE_LOOP('',(#62951,#62952,#62953,#62954));
#15123=EDGE_LOOP('',(#62955,#62956,#62957,#62958));
#15124=EDGE_LOOP('',(#62959,#62960,#62961));
#15125=EDGE_LOOP('',(#62962,#62963,#62964));
#15126=EDGE_LOOP('',(#62965,#62966,#62967));
#15127=EDGE_LOOP('',(#62968,#62969,#62970));
#15128=EDGE_LOOP('',(#62971,#62972,#62973,#62974));
#15129=EDGE_LOOP('',(#62975,#62976,#62977,#62978));
#15130=EDGE_LOOP('',(#62979,#62980,#62981));
#15131=EDGE_LOOP('',(#62982,#62983,#62984));
#15132=EDGE_LOOP('',(#62985,#62986,#62987));
#15133=EDGE_LOOP('',(#62988,#62989,#62990));
#15134=EDGE_LOOP('',(#62991,#62992,#62993,#62994));
#15135=EDGE_LOOP('',(#62995,#62996,#62997,#62998));
#15136=EDGE_LOOP('',(#62999,#63000,#63001));
#15137=EDGE_LOOP('',(#63002,#63003,#63004));
#15138=EDGE_LOOP('',(#63005,#63006,#63007));
#15139=EDGE_LOOP('',(#63008,#63009,#63010));
#15140=EDGE_LOOP('',(#63011,#63012,#63013,#63014));
#15141=EDGE_LOOP('',(#63015,#63016,#63017,#63018));
#15142=EDGE_LOOP('',(#63019,#63020,#63021));
#15143=EDGE_LOOP('',(#63022,#63023,#63024));
#15144=EDGE_LOOP('',(#63025,#63026,#63027));
#15145=EDGE_LOOP('',(#63028,#63029,#63030));
#15146=EDGE_LOOP('',(#63031,#63032,#63033,#63034));
#15147=EDGE_LOOP('',(#63035,#63036,#63037,#63038));
#15148=EDGE_LOOP('',(#63039,#63040,#63041));
#15149=EDGE_LOOP('',(#63042,#63043,#63044));
#15150=EDGE_LOOP('',(#63045,#63046,#63047));
#15151=EDGE_LOOP('',(#63048,#63049,#63050));
#15152=EDGE_LOOP('',(#63051,#63052,#63053,#63054));
#15153=EDGE_LOOP('',(#63055,#63056,#63057,#63058));
#15154=EDGE_LOOP('',(#63059,#63060,#63061));
#15155=EDGE_LOOP('',(#63062,#63063,#63064));
#15156=EDGE_LOOP('',(#63065,#63066,#63067));
#15157=EDGE_LOOP('',(#63068,#63069,#63070));
#15158=EDGE_LOOP('',(#63071,#63072,#63073,#63074));
#15159=EDGE_LOOP('',(#63075,#63076,#63077,#63078));
#15160=EDGE_LOOP('',(#63079,#63080,#63081));
#15161=EDGE_LOOP('',(#63082,#63083,#63084));
#15162=EDGE_LOOP('',(#63085,#63086,#63087));
#15163=EDGE_LOOP('',(#63088,#63089,#63090));
#15164=EDGE_LOOP('',(#63091,#63092,#63093,#63094));
#15165=EDGE_LOOP('',(#63095,#63096,#63097,#63098));
#15166=EDGE_LOOP('',(#63099,#63100,#63101));
#15167=EDGE_LOOP('',(#63102,#63103,#63104));
#15168=EDGE_LOOP('',(#63105,#63106,#63107));
#15169=EDGE_LOOP('',(#63108,#63109,#63110));
#15170=EDGE_LOOP('',(#63111,#63112,#63113,#63114));
#15171=EDGE_LOOP('',(#63115,#63116,#63117,#63118));
#15172=EDGE_LOOP('',(#63119,#63120,#63121));
#15173=EDGE_LOOP('',(#63122,#63123,#63124));
#15174=EDGE_LOOP('',(#63125,#63126,#63127));
#15175=EDGE_LOOP('',(#63128,#63129,#63130));
#15176=EDGE_LOOP('',(#63131,#63132,#63133,#63134));
#15177=EDGE_LOOP('',(#63135,#63136,#63137,#63138));
#15178=EDGE_LOOP('',(#63139,#63140,#63141));
#15179=EDGE_LOOP('',(#63142,#63143,#63144));
#15180=EDGE_LOOP('',(#63145,#63146,#63147));
#15181=EDGE_LOOP('',(#63148,#63149,#63150));
#15182=EDGE_LOOP('',(#63151,#63152,#63153,#63154));
#15183=EDGE_LOOP('',(#63155,#63156,#63157,#63158));
#15184=EDGE_LOOP('',(#63159,#63160,#63161));
#15185=EDGE_LOOP('',(#63162,#63163,#63164));
#15186=EDGE_LOOP('',(#63165,#63166,#63167));
#15187=EDGE_LOOP('',(#63168,#63169,#63170));
#15188=EDGE_LOOP('',(#63171,#63172,#63173,#63174));
#15189=EDGE_LOOP('',(#63175,#63176,#63177,#63178));
#15190=EDGE_LOOP('',(#63179,#63180,#63181));
#15191=EDGE_LOOP('',(#63182,#63183,#63184));
#15192=EDGE_LOOP('',(#63185,#63186,#63187));
#15193=EDGE_LOOP('',(#63188,#63189,#63190));
#15194=EDGE_LOOP('',(#63191,#63192,#63193,#63194));
#15195=EDGE_LOOP('',(#63195,#63196,#63197,#63198));
#15196=EDGE_LOOP('',(#63199,#63200,#63201));
#15197=EDGE_LOOP('',(#63202,#63203,#63204));
#15198=EDGE_LOOP('',(#63205,#63206,#63207));
#15199=EDGE_LOOP('',(#63208,#63209,#63210));
#15200=EDGE_LOOP('',(#63211,#63212,#63213,#63214));
#15201=EDGE_LOOP('',(#63215,#63216,#63217,#63218));
#15202=EDGE_LOOP('',(#63219,#63220,#63221));
#15203=EDGE_LOOP('',(#63222,#63223,#63224));
#15204=EDGE_LOOP('',(#63225,#63226,#63227));
#15205=EDGE_LOOP('',(#63228,#63229,#63230));
#15206=EDGE_LOOP('',(#63231,#63232,#63233,#63234));
#15207=EDGE_LOOP('',(#63235,#63236,#63237,#63238));
#15208=EDGE_LOOP('',(#63239,#63240,#63241));
#15209=EDGE_LOOP('',(#63242,#63243,#63244));
#15210=EDGE_LOOP('',(#63245,#63246,#63247));
#15211=EDGE_LOOP('',(#63248,#63249,#63250));
#15212=EDGE_LOOP('',(#63251,#63252,#63253,#63254));
#15213=EDGE_LOOP('',(#63255,#63256,#63257,#63258));
#15214=EDGE_LOOP('',(#63259,#63260,#63261));
#15215=EDGE_LOOP('',(#63262,#63263,#63264));
#15216=EDGE_LOOP('',(#63265,#63266,#63267));
#15217=EDGE_LOOP('',(#63268,#63269,#63270));
#15218=EDGE_LOOP('',(#63271,#63272,#63273,#63274));
#15219=EDGE_LOOP('',(#63275,#63276,#63277,#63278));
#15220=EDGE_LOOP('',(#63279,#63280,#63281));
#15221=EDGE_LOOP('',(#63282,#63283,#63284));
#15222=EDGE_LOOP('',(#63285,#63286,#63287));
#15223=EDGE_LOOP('',(#63288,#63289,#63290));
#15224=EDGE_LOOP('',(#63291,#63292,#63293,#63294));
#15225=EDGE_LOOP('',(#63295,#63296,#63297,#63298));
#15226=EDGE_LOOP('',(#63299,#63300,#63301));
#15227=EDGE_LOOP('',(#63302,#63303,#63304));
#15228=EDGE_LOOP('',(#63305,#63306,#63307));
#15229=EDGE_LOOP('',(#63308,#63309,#63310));
#15230=EDGE_LOOP('',(#63311,#63312,#63313,#63314));
#15231=EDGE_LOOP('',(#63315,#63316,#63317,#63318));
#15232=EDGE_LOOP('',(#63319,#63320,#63321));
#15233=EDGE_LOOP('',(#63322,#63323,#63324));
#15234=EDGE_LOOP('',(#63325,#63326,#63327));
#15235=EDGE_LOOP('',(#63328,#63329,#63330));
#15236=EDGE_LOOP('',(#63331,#63332,#63333,#63334));
#15237=EDGE_LOOP('',(#63335,#63336,#63337,#63338));
#15238=EDGE_LOOP('',(#63339,#63340,#63341));
#15239=EDGE_LOOP('',(#63342,#63343,#63344));
#15240=EDGE_LOOP('',(#63345,#63346,#63347));
#15241=EDGE_LOOP('',(#63348,#63349,#63350));
#15242=EDGE_LOOP('',(#63351,#63352,#63353,#63354));
#15243=EDGE_LOOP('',(#63355,#63356,#63357,#63358));
#15244=EDGE_LOOP('',(#63359,#63360,#63361));
#15245=EDGE_LOOP('',(#63362,#63363,#63364));
#15246=EDGE_LOOP('',(#63365,#63366,#63367));
#15247=EDGE_LOOP('',(#63368,#63369,#63370));
#15248=EDGE_LOOP('',(#63371,#63372,#63373,#63374));
#15249=EDGE_LOOP('',(#63375,#63376,#63377,#63378));
#15250=EDGE_LOOP('',(#63379,#63380,#63381));
#15251=EDGE_LOOP('',(#63382,#63383,#63384));
#15252=EDGE_LOOP('',(#63385,#63386,#63387));
#15253=EDGE_LOOP('',(#63388,#63389,#63390));
#15254=EDGE_LOOP('',(#63391,#63392,#63393,#63394));
#15255=EDGE_LOOP('',(#63395,#63396,#63397,#63398));
#15256=EDGE_LOOP('',(#63399,#63400,#63401));
#15257=EDGE_LOOP('',(#63402,#63403,#63404));
#15258=EDGE_LOOP('',(#63405,#63406,#63407));
#15259=EDGE_LOOP('',(#63408,#63409,#63410));
#15260=EDGE_LOOP('',(#63411,#63412,#63413,#63414));
#15261=EDGE_LOOP('',(#63415,#63416,#63417,#63418));
#15262=EDGE_LOOP('',(#63419,#63420,#63421));
#15263=EDGE_LOOP('',(#63422,#63423,#63424));
#15264=EDGE_LOOP('',(#63425,#63426,#63427));
#15265=EDGE_LOOP('',(#63428,#63429,#63430));
#15266=EDGE_LOOP('',(#63431,#63432,#63433,#63434));
#15267=EDGE_LOOP('',(#63435,#63436,#63437,#63438));
#15268=EDGE_LOOP('',(#63439,#63440,#63441));
#15269=EDGE_LOOP('',(#63442,#63443,#63444));
#15270=EDGE_LOOP('',(#63445,#63446,#63447));
#15271=EDGE_LOOP('',(#63448,#63449,#63450));
#15272=EDGE_LOOP('',(#63451,#63452,#63453,#63454));
#15273=EDGE_LOOP('',(#63455,#63456,#63457,#63458));
#15274=EDGE_LOOP('',(#63459,#63460,#63461));
#15275=EDGE_LOOP('',(#63462,#63463,#63464));
#15276=EDGE_LOOP('',(#63465,#63466,#63467));
#15277=EDGE_LOOP('',(#63468,#63469,#63470));
#15278=EDGE_LOOP('',(#63471,#63472,#63473,#63474));
#15279=EDGE_LOOP('',(#63475,#63476,#63477,#63478));
#15280=EDGE_LOOP('',(#63479,#63480,#63481));
#15281=EDGE_LOOP('',(#63482,#63483,#63484));
#15282=EDGE_LOOP('',(#63485,#63486,#63487));
#15283=EDGE_LOOP('',(#63488,#63489,#63490));
#15284=EDGE_LOOP('',(#63491,#63492,#63493,#63494));
#15285=EDGE_LOOP('',(#63495,#63496,#63497,#63498));
#15286=EDGE_LOOP('',(#63499,#63500,#63501));
#15287=EDGE_LOOP('',(#63502,#63503,#63504));
#15288=EDGE_LOOP('',(#63505,#63506,#63507));
#15289=EDGE_LOOP('',(#63508,#63509,#63510));
#15290=EDGE_LOOP('',(#63511,#63512,#63513,#63514));
#15291=EDGE_LOOP('',(#63515,#63516,#63517,#63518));
#15292=EDGE_LOOP('',(#63519,#63520,#63521));
#15293=EDGE_LOOP('',(#63522,#63523,#63524));
#15294=EDGE_LOOP('',(#63525,#63526,#63527));
#15295=EDGE_LOOP('',(#63528,#63529,#63530));
#15296=EDGE_LOOP('',(#63531,#63532,#63533,#63534));
#15297=EDGE_LOOP('',(#63535,#63536,#63537,#63538,#63539));
#15298=EDGE_LOOP('',(#63540,#63541,#63542,#63543));
#15299=EDGE_LOOP('',(#63544,#63545,#63546,#63547));
#15300=EDGE_LOOP('',(#63548,#63549,#63550,#63551));
#15301=EDGE_LOOP('',(#63552,#63553,#63554,#63555));
#15302=EDGE_LOOP('',(#63556,#63557,#63558,#63559));
#15303=EDGE_LOOP('',(#63560,#63561,#63562,#63563));
#15304=EDGE_LOOP('',(#63564,#63565,#63566,#63567));
#15305=EDGE_LOOP('',(#63568,#63569,#63570,#63571));
#15306=EDGE_LOOP('',(#63572,#63573,#63574,#63575));
#15307=EDGE_LOOP('',(#63576,#63577,#63578,#63579));
#15308=EDGE_LOOP('',(#63580,#63581,#63582,#63583));
#15309=EDGE_LOOP('',(#63584,#63585,#63586,#63587));
#15310=EDGE_LOOP('',(#63588,#63589,#63590,#63591));
#15311=EDGE_LOOP('',(#63592,#63593,#63594,#63595));
#15312=EDGE_LOOP('',(#63596,#63597,#63598,#63599));
#15313=EDGE_LOOP('',(#63600,#63601,#63602,#63603));
#15314=EDGE_LOOP('',(#63604,#63605,#63606,#63607));
#15315=EDGE_LOOP('',(#63608,#63609,#63610,#63611));
#15316=EDGE_LOOP('',(#63612,#63613,#63614,#63615));
#15317=EDGE_LOOP('',(#63616,#63617,#63618,#63619));
#15318=EDGE_LOOP('',(#63620,#63621,#63622,#63623));
#15319=EDGE_LOOP('',(#63624,#63625,#63626,#63627));
#15320=EDGE_LOOP('',(#63628,#63629,#63630,#63631));
#15321=EDGE_LOOP('',(#63632,#63633,#63634,#63635));
#15322=EDGE_LOOP('',(#63636,#63637,#63638,#63639));
#15323=EDGE_LOOP('',(#63640,#63641,#63642,#63643));
#15324=EDGE_LOOP('',(#63644,#63645,#63646,#63647));
#15325=EDGE_LOOP('',(#63648,#63649,#63650,#63651));
#15326=EDGE_LOOP('',(#63652,#63653,#63654,#63655));
#15327=EDGE_LOOP('',(#63656,#63657,#63658,#63659));
#15328=EDGE_LOOP('',(#63660,#63661,#63662,#63663));
#15329=EDGE_LOOP('',(#63664,#63665,#63666,#63667));
#15330=EDGE_LOOP('',(#63668,#63669,#63670,#63671));
#15331=EDGE_LOOP('',(#63672,#63673,#63674,#63675));
#15332=EDGE_LOOP('',(#63676,#63677,#63678,#63679));
#15333=EDGE_LOOP('',(#63680,#63681,#63682,#63683));
#15334=EDGE_LOOP('',(#63684,#63685,#63686,#63687));
#15335=EDGE_LOOP('',(#63688,#63689,#63690,#63691));
#15336=EDGE_LOOP('',(#63692,#63693,#63694,#63695));
#15337=EDGE_LOOP('',(#63696,#63697,#63698,#63699));
#15338=EDGE_LOOP('',(#63700,#63701,#63702,#63703));
#15339=EDGE_LOOP('',(#63704,#63705,#63706,#63707));
#15340=EDGE_LOOP('',(#63708,#63709,#63710,#63711));
#15341=EDGE_LOOP('',(#63712,#63713,#63714,#63715));
#15342=EDGE_LOOP('',(#63716,#63717,#63718,#63719));
#15343=EDGE_LOOP('',(#63720,#63721,#63722,#63723));
#15344=EDGE_LOOP('',(#63724,#63725,#63726,#63727));
#15345=EDGE_LOOP('',(#63728,#63729,#63730,#63731));
#15346=EDGE_LOOP('',(#63732,#63733,#63734,#63735));
#15347=EDGE_LOOP('',(#63736,#63737,#63738,#63739));
#15348=EDGE_LOOP('',(#63740,#63741,#63742,#63743));
#15349=EDGE_LOOP('',(#63744,#63745,#63746,#63747));
#15350=EDGE_LOOP('',(#63748,#63749,#63750,#63751));
#15351=EDGE_LOOP('',(#63752,#63753,#63754,#63755));
#15352=EDGE_LOOP('',(#63756,#63757,#63758,#63759));
#15353=EDGE_LOOP('',(#63760,#63761,#63762,#63763));
#15354=EDGE_LOOP('',(#63764,#63765,#63766,#63767));
#15355=EDGE_LOOP('',(#63768,#63769,#63770,#63771));
#15356=EDGE_LOOP('',(#63772,#63773,#63774,#63775));
#15357=EDGE_LOOP('',(#63776,#63777,#63778,#63779));
#15358=EDGE_LOOP('',(#63780,#63781,#63782));
#15359=EDGE_LOOP('',(#63783,#63784,#63785,#63786));
#15360=EDGE_LOOP('',(#63787,#63788,#63789,#63790,#63791));
#15361=EDGE_LOOP('',(#63792,#63793,#63794,#63795));
#15362=EDGE_LOOP('',(#63796,#63797,#63798));
#15363=EDGE_LOOP('',(#63799,#63800,#63801,#63802));
#15364=EDGE_LOOP('',(#63803,#63804,#63805,#63806,#63807));
#15365=EDGE_LOOP('',(#63808,#63809,#63810,#63811));
#15366=EDGE_LOOP('',(#63812,#63813,#63814));
#15367=EDGE_LOOP('',(#63815,#63816,#63817,#63818));
#15368=EDGE_LOOP('',(#63819,#63820,#63821,#63822,#63823));
#15369=EDGE_LOOP('',(#63824,#63825,#63826,#63827));
#15370=EDGE_LOOP('',(#63828,#63829,#63830));
#15371=EDGE_LOOP('',(#63831,#63832,#63833,#63834));
#15372=EDGE_LOOP('',(#63835,#63836,#63837,#63838,#63839));
#15373=EDGE_LOOP('',(#63840,#63841,#63842,#63843));
#15374=EDGE_LOOP('',(#63844,#63845,#63846));
#15375=EDGE_LOOP('',(#63847,#63848,#63849,#63850));
#15376=EDGE_LOOP('',(#63851,#63852,#63853,#63854,#63855));
#15377=EDGE_LOOP('',(#63856,#63857,#63858,#63859));
#15378=EDGE_LOOP('',(#63860,#63861,#63862));
#15379=EDGE_LOOP('',(#63863,#63864,#63865,#63866));
#15380=EDGE_LOOP('',(#63867,#63868,#63869,#63870,#63871));
#15381=EDGE_LOOP('',(#63872,#63873,#63874,#63875));
#15382=EDGE_LOOP('',(#63876,#63877,#63878));
#15383=EDGE_LOOP('',(#63879,#63880,#63881,#63882));
#15384=EDGE_LOOP('',(#63883,#63884,#63885,#63886));
#15385=EDGE_LOOP('',(#63887,#63888,#63889));
#15386=EDGE_LOOP('',(#63890,#63891,#63892,#63893));
#15387=EDGE_LOOP('',(#63894,#63895,#63896,#63897,#63898));
#15388=EDGE_LOOP('',(#63899,#63900,#63901,#63902));
#15389=EDGE_LOOP('',(#63903,#63904,#63905));
#15390=EDGE_LOOP('',(#63906,#63907,#63908,#63909));
#15391=EDGE_LOOP('',(#63910,#63911,#63912,#63913,#63914));
#15392=EDGE_LOOP('',(#63915,#63916,#63917,#63918));
#15393=EDGE_LOOP('',(#63919,#63920,#63921));
#15394=EDGE_LOOP('',(#63922,#63923,#63924,#63925));
#15395=EDGE_LOOP('',(#63926,#63927,#63928,#63929,#63930));
#15396=EDGE_LOOP('',(#63931,#63932,#63933,#63934));
#15397=EDGE_LOOP('',(#63935,#63936,#63937));
#15398=EDGE_LOOP('',(#63938,#63939,#63940,#63941));
#15399=EDGE_LOOP('',(#63942,#63943,#63944,#63945,#63946));
#15400=EDGE_LOOP('',(#63947,#63948,#63949,#63950));
#15401=EDGE_LOOP('',(#63951,#63952,#63953));
#15402=EDGE_LOOP('',(#63954,#63955,#63956,#63957));
#15403=EDGE_LOOP('',(#63958,#63959,#63960,#63961,#63962));
#15404=EDGE_LOOP('',(#63963,#63964,#63965,#63966));
#15405=EDGE_LOOP('',(#63967,#63968,#63969));
#15406=EDGE_LOOP('',(#63970,#63971,#63972,#63973));
#15407=EDGE_LOOP('',(#63974,#63975,#63976,#63977,#63978));
#15408=EDGE_LOOP('',(#63979,#63980,#63981,#63982));
#15409=EDGE_LOOP('',(#63983,#63984,#63985));
#15410=EDGE_LOOP('',(#63986,#63987,#63988,#63989));
#15411=EDGE_LOOP('',(#63990,#63991,#63992,#63993,#63994));
#15412=EDGE_LOOP('',(#63995,#63996,#63997,#63998));
#15413=EDGE_LOOP('',(#63999,#64000,#64001));
#15414=EDGE_LOOP('',(#64002,#64003,#64004,#64005));
#15415=EDGE_LOOP('',(#64006,#64007,#64008,#64009,#64010));
#15416=EDGE_LOOP('',(#64011,#64012,#64013,#64014));
#15417=EDGE_LOOP('',(#64015,#64016,#64017));
#15418=EDGE_LOOP('',(#64018,#64019,#64020,#64021));
#15419=EDGE_LOOP('',(#64022,#64023,#64024,#64025,#64026));
#15420=EDGE_LOOP('',(#64027,#64028,#64029,#64030));
#15421=EDGE_LOOP('',(#64031,#64032,#64033));
#15422=EDGE_LOOP('',(#64034,#64035,#64036,#64037));
#15423=EDGE_LOOP('',(#64038,#64039,#64040,#64041,#64042));
#15424=EDGE_LOOP('',(#64043,#64044,#64045,#64046));
#15425=EDGE_LOOP('',(#64047,#64048,#64049));
#15426=EDGE_LOOP('',(#64050,#64051,#64052,#64053));
#15427=EDGE_LOOP('',(#64054,#64055,#64056,#64057,#64058));
#15428=EDGE_LOOP('',(#64059,#64060,#64061,#64062));
#15429=EDGE_LOOP('',(#64063,#64064,#64065));
#15430=EDGE_LOOP('',(#64066,#64067,#64068,#64069));
#15431=EDGE_LOOP('',(#64070,#64071,#64072,#64073,#64074));
#15432=EDGE_LOOP('',(#64075,#64076,#64077,#64078));
#15433=EDGE_LOOP('',(#64079,#64080,#64081));
#15434=EDGE_LOOP('',(#64082,#64083,#64084,#64085));
#15435=EDGE_LOOP('',(#64086,#64087,#64088,#64089,#64090));
#15436=EDGE_LOOP('',(#64091,#64092,#64093,#64094));
#15437=EDGE_LOOP('',(#64095,#64096,#64097));
#15438=EDGE_LOOP('',(#64098,#64099,#64100,#64101));
#15439=EDGE_LOOP('',(#64102,#64103,#64104,#64105,#64106));
#15440=EDGE_LOOP('',(#64107,#64108,#64109,#64110));
#15441=EDGE_LOOP('',(#64111,#64112,#64113));
#15442=EDGE_LOOP('',(#64114,#64115,#64116,#64117));
#15443=EDGE_LOOP('',(#64118,#64119,#64120,#64121,#64122));
#15444=EDGE_LOOP('',(#64123,#64124,#64125,#64126));
#15445=EDGE_LOOP('',(#64127,#64128,#64129));
#15446=EDGE_LOOP('',(#64130,#64131,#64132,#64133));
#15447=EDGE_LOOP('',(#64134,#64135,#64136,#64137,#64138));
#15448=EDGE_LOOP('',(#64139,#64140,#64141,#64142));
#15449=EDGE_LOOP('',(#64143,#64144,#64145));
#15450=EDGE_LOOP('',(#64146,#64147,#64148,#64149));
#15451=EDGE_LOOP('',(#64150,#64151,#64152,#64153,#64154));
#15452=EDGE_LOOP('',(#64155,#64156,#64157,#64158));
#15453=EDGE_LOOP('',(#64159,#64160,#64161));
#15454=EDGE_LOOP('',(#64162,#64163,#64164,#64165));
#15455=EDGE_LOOP('',(#64166,#64167,#64168,#64169,#64170));
#15456=EDGE_LOOP('',(#64171,#64172,#64173,#64174));
#15457=EDGE_LOOP('',(#64175,#64176,#64177));
#15458=EDGE_LOOP('',(#64178,#64179,#64180,#64181));
#15459=EDGE_LOOP('',(#64182,#64183,#64184,#64185,#64186));
#15460=EDGE_LOOP('',(#64187,#64188,#64189,#64190));
#15461=EDGE_LOOP('',(#64191,#64192,#64193));
#15462=EDGE_LOOP('',(#64194,#64195,#64196,#64197));
#15463=EDGE_LOOP('',(#64198,#64199,#64200,#64201,#64202));
#15464=EDGE_LOOP('',(#64203,#64204,#64205,#64206));
#15465=EDGE_LOOP('',(#64207,#64208,#64209));
#15466=EDGE_LOOP('',(#64210,#64211,#64212,#64213));
#15467=EDGE_LOOP('',(#64214,#64215,#64216,#64217,#64218));
#15468=EDGE_LOOP('',(#64219,#64220,#64221));
#15469=EDGE_LOOP('',(#64222,#64223,#64224,#64225,#64226));
#15470=EDGE_LOOP('',(#64227,#64228,#64229,#64230));
#15471=EDGE_LOOP('',(#64231));
#15472=EDGE_LOOP('',(#64232));
#15473=EDGE_LOOP('',(#64233,#64234,#64235,#64236,#64237));
#15474=EDGE_LOOP('',(#64238,#64239,#64240,#64241,#64242));
#15475=EDGE_LOOP('',(#64243,#64244,#64245,#64246,#64247));
#15476=EDGE_LOOP('',(#64248,#64249,#64250,#64251,#64252));
#15477=EDGE_LOOP('',(#64253,#64254,#64255,#64256,#64257));
#15478=EDGE_LOOP('',(#64258,#64259,#64260,#64261,#64262));
#15479=EDGE_LOOP('',(#64263,#64264,#64265,#64266,#64267));
#15480=EDGE_LOOP('',(#64268,#64269,#64270,#64271,#64272));
#15481=EDGE_LOOP('',(#64273,#64274,#64275,#64276,#64277));
#15482=EDGE_LOOP('',(#64278,#64279,#64280,#64281,#64282));
#15483=EDGE_LOOP('',(#64283,#64284,#64285,#64286,#64287));
#15484=EDGE_LOOP('',(#64288,#64289,#64290,#64291,#64292));
#15485=EDGE_LOOP('',(#64293,#64294,#64295,#64296,#64297));
#15486=EDGE_LOOP('',(#64298,#64299,#64300,#64301,#64302));
#15487=EDGE_LOOP('',(#64303,#64304,#64305,#64306,#64307));
#15488=EDGE_LOOP('',(#64308,#64309,#64310,#64311,#64312));
#15489=EDGE_LOOP('',(#64313,#64314,#64315,#64316,#64317));
#15490=EDGE_LOOP('',(#64318,#64319,#64320,#64321,#64322));
#15491=EDGE_LOOP('',(#64323,#64324,#64325,#64326,#64327));
#15492=EDGE_LOOP('',(#64328,#64329,#64330,#64331,#64332));
#15493=EDGE_LOOP('',(#64333,#64334,#64335,#64336,#64337));
#15494=EDGE_LOOP('',(#64338,#64339,#64340,#64341,#64342));
#15495=EDGE_LOOP('',(#64343,#64344,#64345,#64346,#64347));
#15496=EDGE_LOOP('',(#64348,#64349,#64350,#64351,#64352));
#15497=EDGE_LOOP('',(#64353,#64354,#64355,#64356,#64357));
#15498=EDGE_LOOP('',(#64358,#64359,#64360,#64361,#64362));
#15499=EDGE_LOOP('',(#64363,#64364,#64365,#64366,#64367));
#15500=EDGE_LOOP('',(#64368,#64369,#64370,#64371,#64372));
#15501=EDGE_LOOP('',(#64373,#64374,#64375,#64376,#64377));
#15502=EDGE_LOOP('',(#64378,#64379,#64380,#64381,#64382));
#15503=EDGE_LOOP('',(#64383,#64384,#64385,#64386,#64387));
#15504=EDGE_LOOP('',(#64388,#64389,#64390,#64391,#64392));
#15505=EDGE_LOOP('',(#64393,#64394,#64395,#64396,#64397));
#15506=EDGE_LOOP('',(#64398,#64399,#64400,#64401,#64402));
#15507=EDGE_LOOP('',(#64403,#64404,#64405,#64406,#64407));
#15508=EDGE_LOOP('',(#64408,#64409,#64410,#64411,#64412));
#15509=EDGE_LOOP('',(#64413,#64414,#64415,#64416,#64417));
#15510=EDGE_LOOP('',(#64418,#64419,#64420,#64421,#64422));
#15511=EDGE_LOOP('',(#64423,#64424,#64425,#64426,#64427));
#15512=EDGE_LOOP('',(#64428,#64429,#64430,#64431,#64432));
#15513=EDGE_LOOP('',(#64433,#64434,#64435,#64436,#64437));
#15514=EDGE_LOOP('',(#64438,#64439,#64440,#64441,#64442));
#15515=EDGE_LOOP('',(#64443,#64444,#64445,#64446,#64447));
#15516=EDGE_LOOP('',(#64448,#64449,#64450,#64451,#64452));
#15517=EDGE_LOOP('',(#64453,#64454,#64455,#64456,#64457));
#15518=EDGE_LOOP('',(#64458,#64459,#64460,#64461,#64462));
#15519=EDGE_LOOP('',(#64463,#64464,#64465,#64466,#64467));
#15520=EDGE_LOOP('',(#64468,#64469,#64470,#64471,#64472));
#15521=EDGE_LOOP('',(#64473,#64474,#64475,#64476,#64477));
#15522=EDGE_LOOP('',(#64478,#64479,#64480,#64481,#64482));
#15523=EDGE_LOOP('',(#64483,#64484,#64485,#64486,#64487));
#15524=EDGE_LOOP('',(#64488,#64489,#64490,#64491,#64492));
#15525=EDGE_LOOP('',(#64493,#64494,#64495,#64496,#64497));
#15526=EDGE_LOOP('',(#64498,#64499,#64500,#64501,#64502));
#15527=EDGE_LOOP('',(#64503,#64504,#64505,#64506,#64507));
#15528=EDGE_LOOP('',(#64508,#64509,#64510,#64511,#64512));
#15529=EDGE_LOOP('',(#64513,#64514,#64515,#64516,#64517));
#15530=EDGE_LOOP('',(#64518,#64519,#64520,#64521,#64522));
#15531=EDGE_LOOP('',(#64523,#64524,#64525,#64526));
#15532=EDGE_LOOP('',(#64527,#64528,#64529,#64530));
#15533=EDGE_LOOP('',(#64531,#64532,#64533,#64534));
#15534=EDGE_LOOP('',(#64535,#64536,#64537,#64538));
#15535=EDGE_LOOP('',(#64539,#64540,#64541,#64542));
#15536=EDGE_LOOP('',(#64543,#64544,#64545,#64546));
#15537=EDGE_LOOP('',(#64547,#64548,#64549,#64550));
#15538=EDGE_LOOP('',(#64551,#64552,#64553,#64554));
#15539=EDGE_LOOP('',(#64555,#64556,#64557,#64558));
#15540=EDGE_LOOP('',(#64559,#64560,#64561,#64562));
#15541=EDGE_LOOP('',(#64563,#64564,#64565,#64566));
#15542=EDGE_LOOP('',(#64567,#64568,#64569,#64570));
#15543=EDGE_LOOP('',(#64571,#64572,#64573,#64574));
#15544=EDGE_LOOP('',(#64575,#64576,#64577,#64578));
#15545=EDGE_LOOP('',(#64579,#64580,#64581,#64582));
#15546=EDGE_LOOP('',(#64583,#64584,#64585,#64586));
#15547=EDGE_LOOP('',(#64587,#64588,#64589,#64590));
#15548=EDGE_LOOP('',(#64591,#64592,#64593,#64594));
#15549=EDGE_LOOP('',(#64595,#64596,#64597,#64598));
#15550=EDGE_LOOP('',(#64599,#64600,#64601,#64602));
#15551=EDGE_LOOP('',(#64603,#64604,#64605,#64606));
#15552=EDGE_LOOP('',(#64607,#64608,#64609,#64610));
#15553=EDGE_LOOP('',(#64611,#64612,#64613,#64614));
#15554=EDGE_LOOP('',(#64615,#64616,#64617,#64618));
#15555=EDGE_LOOP('',(#64619,#64620,#64621,#64622));
#15556=EDGE_LOOP('',(#64623,#64624,#64625,#64626));
#15557=EDGE_LOOP('',(#64627,#64628,#64629,#64630));
#15558=EDGE_LOOP('',(#64631,#64632,#64633,#64634));
#15559=EDGE_LOOP('',(#64635,#64636,#64637,#64638));
#15560=EDGE_LOOP('',(#64639,#64640,#64641,#64642));
#15561=EDGE_LOOP('',(#64643,#64644,#64645,#64646));
#15562=EDGE_LOOP('',(#64647,#64648,#64649,#64650));
#15563=EDGE_LOOP('',(#64651,#64652,#64653,#64654));
#15564=EDGE_LOOP('',(#64655,#64656,#64657,#64658));
#15565=EDGE_LOOP('',(#64659,#64660,#64661,#64662));
#15566=EDGE_LOOP('',(#64663,#64664,#64665,#64666));
#15567=EDGE_LOOP('',(#64667,#64668,#64669,#64670));
#15568=EDGE_LOOP('',(#64671,#64672,#64673,#64674));
#15569=EDGE_LOOP('',(#64675,#64676,#64677,#64678));
#15570=EDGE_LOOP('',(#64679,#64680,#64681,#64682));
#15571=EDGE_LOOP('',(#64683,#64684,#64685,#64686));
#15572=EDGE_LOOP('',(#64687,#64688,#64689,#64690));
#15573=EDGE_LOOP('',(#64691,#64692,#64693,#64694));
#15574=EDGE_LOOP('',(#64695,#64696,#64697,#64698));
#15575=EDGE_LOOP('',(#64699,#64700,#64701,#64702));
#15576=EDGE_LOOP('',(#64703,#64704,#64705,#64706));
#15577=EDGE_LOOP('',(#64707,#64708,#64709,#64710));
#15578=EDGE_LOOP('',(#64711,#64712,#64713,#64714));
#15579=EDGE_LOOP('',(#64715,#64716,#64717,#64718));
#15580=EDGE_LOOP('',(#64719,#64720,#64721,#64722));
#15581=EDGE_LOOP('',(#64723,#64724,#64725,#64726));
#15582=EDGE_LOOP('',(#64727,#64728,#64729,#64730));
#15583=EDGE_LOOP('',(#64731,#64732,#64733,#64734));
#15584=EDGE_LOOP('',(#64735,#64736,#64737,#64738));
#15585=EDGE_LOOP('',(#64739,#64740,#64741,#64742));
#15586=EDGE_LOOP('',(#64743,#64744,#64745,#64746));
#15587=EDGE_LOOP('',(#64747,#64748,#64749,#64750));
#15588=EDGE_LOOP('',(#64751,#64752,#64753,#64754));
#15589=EDGE_LOOP('',(#64755,#64756,#64757,#64758));
#15590=EDGE_LOOP('',(#64759,#64760,#64761,#64762));
#15591=EDGE_LOOP('',(#64763,#64764,#64765,#64766));
#15592=EDGE_LOOP('',(#64767,#64768,#64769,#64770));
#15593=EDGE_LOOP('',(#64771,#64772,#64773,#64774));
#15594=EDGE_LOOP('',(#64775,#64776,#64777,#64778));
#15595=EDGE_LOOP('',(#64779,#64780,#64781,#64782));
#15596=EDGE_LOOP('',(#64783,#64784,#64785,#64786));
#15597=EDGE_LOOP('',(#64787,#64788,#64789,#64790));
#15598=EDGE_LOOP('',(#64791,#64792,#64793,#64794));
#15599=EDGE_LOOP('',(#64795,#64796,#64797,#64798));
#15600=EDGE_LOOP('',(#64799,#64800,#64801,#64802));
#15601=EDGE_LOOP('',(#64803,#64804,#64805,#64806));
#15602=EDGE_LOOP('',(#64807,#64808,#64809,#64810));
#15603=EDGE_LOOP('',(#64811,#64812,#64813,#64814));
#15604=EDGE_LOOP('',(#64815,#64816,#64817,#64818));
#15605=EDGE_LOOP('',(#64819,#64820,#64821,#64822));
#15606=EDGE_LOOP('',(#64823,#64824,#64825,#64826));
#15607=EDGE_LOOP('',(#64827,#64828,#64829,#64830));
#15608=EDGE_LOOP('',(#64831,#64832,#64833,#64834));
#15609=EDGE_LOOP('',(#64835,#64836,#64837,#64838));
#15610=EDGE_LOOP('',(#64839,#64840,#64841,#64842));
#15611=EDGE_LOOP('',(#64843,#64844,#64845,#64846));
#15612=EDGE_LOOP('',(#64847,#64848,#64849,#64850));
#15613=EDGE_LOOP('',(#64851,#64852,#64853,#64854));
#15614=EDGE_LOOP('',(#64855,#64856,#64857,#64858));
#15615=EDGE_LOOP('',(#64859,#64860,#64861,#64862));
#15616=EDGE_LOOP('',(#64863,#64864,#64865,#64866));
#15617=EDGE_LOOP('',(#64867,#64868,#64869,#64870));
#15618=EDGE_LOOP('',(#64871,#64872,#64873,#64874));
#15619=EDGE_LOOP('',(#64875,#64876,#64877,#64878));
#15620=EDGE_LOOP('',(#64879,#64880,#64881,#64882));
#15621=EDGE_LOOP('',(#64883,#64884,#64885,#64886));
#15622=EDGE_LOOP('',(#64887,#64888,#64889,#64890));
#15623=EDGE_LOOP('',(#64891,#64892,#64893,#64894));
#15624=EDGE_LOOP('',(#64895,#64896,#64897,#64898));
#15625=EDGE_LOOP('',(#64899,#64900,#64901,#64902));
#15626=EDGE_LOOP('',(#64903,#64904,#64905,#64906));
#15627=EDGE_LOOP('',(#64907,#64908,#64909,#64910));
#15628=EDGE_LOOP('',(#64911,#64912,#64913,#64914));
#15629=EDGE_LOOP('',(#64915,#64916,#64917,#64918));
#15630=EDGE_LOOP('',(#64919,#64920,#64921,#64922));
#15631=EDGE_LOOP('',(#64923,#64924,#64925,#64926));
#15632=EDGE_LOOP('',(#64927,#64928,#64929,#64930));
#15633=EDGE_LOOP('',(#64931,#64932,#64933,#64934));
#15634=EDGE_LOOP('',(#64935,#64936,#64937,#64938));
#15635=EDGE_LOOP('',(#64939,#64940,#64941,#64942));
#15636=EDGE_LOOP('',(#64943,#64944,#64945,#64946));
#15637=EDGE_LOOP('',(#64947,#64948,#64949,#64950));
#15638=EDGE_LOOP('',(#64951,#64952,#64953,#64954));
#15639=EDGE_LOOP('',(#64955,#64956,#64957,#64958));
#15640=EDGE_LOOP('',(#64959,#64960,#64961,#64962));
#15641=EDGE_LOOP('',(#64963,#64964,#64965,#64966));
#15642=EDGE_LOOP('',(#64967,#64968,#64969,#64970));
#15643=EDGE_LOOP('',(#64971,#64972,#64973,#64974));
#15644=EDGE_LOOP('',(#64975,#64976,#64977,#64978));
#15645=EDGE_LOOP('',(#64979,#64980,#64981,#64982));
#15646=EDGE_LOOP('',(#64983,#64984,#64985,#64986));
#15647=EDGE_LOOP('',(#64987,#64988,#64989,#64990));
#15648=EDGE_LOOP('',(#64991,#64992,#64993,#64994));
#15649=EDGE_LOOP('',(#64995,#64996,#64997,#64998));
#15650=EDGE_LOOP('',(#64999,#65000,#65001,#65002));
#15651=EDGE_LOOP('',(#65003,#65004,#65005,#65006));
#15652=EDGE_LOOP('',(#65007,#65008,#65009,#65010));
#15653=EDGE_LOOP('',(#65011,#65012,#65013,#65014));
#15654=EDGE_LOOP('',(#65015,#65016,#65017,#65018));
#15655=EDGE_LOOP('',(#65019,#65020,#65021,#65022));
#15656=EDGE_LOOP('',(#65023,#65024,#65025,#65026));
#15657=EDGE_LOOP('',(#65027,#65028,#65029,#65030));
#15658=EDGE_LOOP('',(#65031,#65032,#65033,#65034));
#15659=EDGE_LOOP('',(#65035,#65036,#65037,#65038));
#15660=EDGE_LOOP('',(#65039,#65040,#65041,#65042));
#15661=EDGE_LOOP('',(#65043,#65044,#65045,#65046));
#15662=EDGE_LOOP('',(#65047,#65048,#65049,#65050));
#15663=EDGE_LOOP('',(#65051,#65052,#65053,#65054));
#15664=EDGE_LOOP('',(#65055,#65056,#65057,#65058));
#15665=EDGE_LOOP('',(#65059,#65060,#65061,#65062));
#15666=EDGE_LOOP('',(#65063,#65064,#65065,#65066));
#15667=EDGE_LOOP('',(#65067,#65068,#65069,#65070));
#15668=EDGE_LOOP('',(#65071,#65072,#65073,#65074));
#15669=EDGE_LOOP('',(#65075,#65076,#65077,#65078));
#15670=EDGE_LOOP('',(#65079,#65080,#65081,#65082));
#15671=EDGE_LOOP('',(#65083,#65084,#65085,#65086));
#15672=EDGE_LOOP('',(#65087,#65088,#65089,#65090));
#15673=EDGE_LOOP('',(#65091,#65092,#65093,#65094));
#15674=EDGE_LOOP('',(#65095));
#15675=EDGE_LOOP('',(#65096));
#15676=EDGE_LOOP('',(#65097,#65098,#65099,#65100));
#15677=EDGE_LOOP('',(#65101,#65102,#65103));
#15678=EDGE_LOOP('',(#65104,#65105,#65106));
#15679=EDGE_LOOP('',(#65107,#65108,#65109));
#15680=EDGE_LOOP('',(#65110,#65111,#65112));
#15681=EDGE_LOOP('',(#65113,#65114,#65115,#65116));
#15682=EDGE_LOOP('',(#65117,#65118,#65119,#65120));
#15683=EDGE_LOOP('',(#65121,#65122,#65123));
#15684=EDGE_LOOP('',(#65124,#65125,#65126));
#15685=EDGE_LOOP('',(#65127,#65128,#65129));
#15686=EDGE_LOOP('',(#65130,#65131,#65132));
#15687=EDGE_LOOP('',(#65133,#65134,#65135,#65136));
#15688=EDGE_LOOP('',(#65137,#65138,#65139,#65140));
#15689=EDGE_LOOP('',(#65141,#65142,#65143));
#15690=EDGE_LOOP('',(#65144,#65145,#65146));
#15691=EDGE_LOOP('',(#65147,#65148,#65149));
#15692=EDGE_LOOP('',(#65150,#65151,#65152));
#15693=EDGE_LOOP('',(#65153,#65154,#65155,#65156));
#15694=EDGE_LOOP('',(#65157,#65158,#65159,#65160));
#15695=EDGE_LOOP('',(#65161,#65162,#65163));
#15696=EDGE_LOOP('',(#65164,#65165,#65166));
#15697=EDGE_LOOP('',(#65167,#65168,#65169));
#15698=EDGE_LOOP('',(#65170,#65171,#65172));
#15699=EDGE_LOOP('',(#65173,#65174,#65175,#65176));
#15700=EDGE_LOOP('',(#65177,#65178,#65179,#65180));
#15701=EDGE_LOOP('',(#65181,#65182,#65183));
#15702=EDGE_LOOP('',(#65184,#65185,#65186));
#15703=EDGE_LOOP('',(#65187,#65188,#65189));
#15704=EDGE_LOOP('',(#65190,#65191,#65192));
#15705=EDGE_LOOP('',(#65193,#65194,#65195,#65196));
#15706=EDGE_LOOP('',(#65197,#65198,#65199,#65200));
#15707=EDGE_LOOP('',(#65201,#65202,#65203));
#15708=EDGE_LOOP('',(#65204,#65205,#65206));
#15709=EDGE_LOOP('',(#65207,#65208,#65209));
#15710=EDGE_LOOP('',(#65210,#65211,#65212));
#15711=EDGE_LOOP('',(#65213,#65214,#65215,#65216));
#15712=EDGE_LOOP('',(#65217,#65218,#65219,#65220));
#15713=EDGE_LOOP('',(#65221,#65222,#65223));
#15714=EDGE_LOOP('',(#65224,#65225,#65226));
#15715=EDGE_LOOP('',(#65227,#65228,#65229));
#15716=EDGE_LOOP('',(#65230,#65231,#65232));
#15717=EDGE_LOOP('',(#65233,#65234,#65235,#65236));
#15718=EDGE_LOOP('',(#65237,#65238,#65239,#65240));
#15719=EDGE_LOOP('',(#65241,#65242,#65243));
#15720=EDGE_LOOP('',(#65244,#65245,#65246));
#15721=EDGE_LOOP('',(#65247,#65248,#65249));
#15722=EDGE_LOOP('',(#65250,#65251,#65252));
#15723=EDGE_LOOP('',(#65253,#65254,#65255,#65256));
#15724=EDGE_LOOP('',(#65257,#65258,#65259,#65260));
#15725=EDGE_LOOP('',(#65261,#65262,#65263));
#15726=EDGE_LOOP('',(#65264,#65265,#65266));
#15727=EDGE_LOOP('',(#65267,#65268,#65269));
#15728=EDGE_LOOP('',(#65270,#65271,#65272));
#15729=EDGE_LOOP('',(#65273,#65274,#65275,#65276));
#15730=EDGE_LOOP('',(#65277,#65278,#65279,#65280));
#15731=EDGE_LOOP('',(#65281,#65282,#65283));
#15732=EDGE_LOOP('',(#65284,#65285,#65286));
#15733=EDGE_LOOP('',(#65287,#65288,#65289));
#15734=EDGE_LOOP('',(#65290,#65291,#65292));
#15735=EDGE_LOOP('',(#65293,#65294,#65295,#65296));
#15736=EDGE_LOOP('',(#65297,#65298,#65299,#65300));
#15737=EDGE_LOOP('',(#65301,#65302,#65303));
#15738=EDGE_LOOP('',(#65304,#65305,#65306));
#15739=EDGE_LOOP('',(#65307,#65308,#65309));
#15740=EDGE_LOOP('',(#65310,#65311,#65312));
#15741=EDGE_LOOP('',(#65313,#65314,#65315,#65316));
#15742=EDGE_LOOP('',(#65317,#65318,#65319,#65320));
#15743=EDGE_LOOP('',(#65321,#65322,#65323));
#15744=EDGE_LOOP('',(#65324,#65325,#65326));
#15745=EDGE_LOOP('',(#65327,#65328,#65329));
#15746=EDGE_LOOP('',(#65330,#65331,#65332));
#15747=EDGE_LOOP('',(#65333,#65334,#65335,#65336));
#15748=EDGE_LOOP('',(#65337,#65338,#65339,#65340));
#15749=EDGE_LOOP('',(#65341,#65342,#65343));
#15750=EDGE_LOOP('',(#65344,#65345,#65346));
#15751=EDGE_LOOP('',(#65347,#65348,#65349));
#15752=EDGE_LOOP('',(#65350,#65351,#65352));
#15753=EDGE_LOOP('',(#65353,#65354,#65355,#65356));
#15754=EDGE_LOOP('',(#65357,#65358,#65359,#65360));
#15755=EDGE_LOOP('',(#65361,#65362,#65363));
#15756=EDGE_LOOP('',(#65364,#65365,#65366));
#15757=EDGE_LOOP('',(#65367,#65368,#65369));
#15758=EDGE_LOOP('',(#65370,#65371,#65372));
#15759=EDGE_LOOP('',(#65373,#65374,#65375,#65376));
#15760=EDGE_LOOP('',(#65377,#65378,#65379,#65380,#65381));
#15761=EDGE_LOOP('',(#65382,#65383,#65384,#65385));
#15762=EDGE_LOOP('',(#65386,#65387,#65388,#65389));
#15763=EDGE_LOOP('',(#65390,#65391,#65392));
#15764=EDGE_LOOP('',(#65393,#65394,#65395));
#15765=EDGE_LOOP('',(#65396,#65397,#65398,#65399));
#15766=EDGE_LOOP('',(#65400,#65401,#65402,#65403));
#15767=EDGE_LOOP('',(#65404,#65405,#65406));
#15768=EDGE_LOOP('',(#65407,#65408,#65409));
#15769=EDGE_LOOP('',(#65410,#65411,#65412));
#15770=EDGE_LOOP('',(#65413,#65414,#65415));
#15771=EDGE_LOOP('',(#65416,#65417,#65418,#65419));
#15772=EDGE_LOOP('',(#65420,#65421,#65422,#65423));
#15773=EDGE_LOOP('',(#65424,#65425,#65426));
#15774=EDGE_LOOP('',(#65427,#65428,#65429));
#15775=EDGE_LOOP('',(#65430,#65431,#65432));
#15776=EDGE_LOOP('',(#65433,#65434,#65435));
#15777=EDGE_LOOP('',(#65436,#65437,#65438,#65439));
#15778=EDGE_LOOP('',(#65440,#65441,#65442,#65443));
#15779=EDGE_LOOP('',(#65444,#65445,#65446));
#15780=EDGE_LOOP('',(#65447,#65448,#65449));
#15781=EDGE_LOOP('',(#65450,#65451,#65452));
#15782=EDGE_LOOP('',(#65453,#65454,#65455));
#15783=EDGE_LOOP('',(#65456,#65457,#65458,#65459));
#15784=EDGE_LOOP('',(#65460,#65461,#65462,#65463));
#15785=EDGE_LOOP('',(#65464,#65465,#65466));
#15786=EDGE_LOOP('',(#65467,#65468,#65469));
#15787=EDGE_LOOP('',(#65470,#65471,#65472));
#15788=EDGE_LOOP('',(#65473,#65474,#65475));
#15789=EDGE_LOOP('',(#65476,#65477,#65478,#65479));
#15790=EDGE_LOOP('',(#65480,#65481,#65482,#65483));
#15791=EDGE_LOOP('',(#65484,#65485,#65486));
#15792=EDGE_LOOP('',(#65487,#65488,#65489));
#15793=EDGE_LOOP('',(#65490,#65491,#65492));
#15794=EDGE_LOOP('',(#65493,#65494,#65495));
#15795=EDGE_LOOP('',(#65496,#65497,#65498,#65499));
#15796=EDGE_LOOP('',(#65500,#65501,#65502,#65503));
#15797=EDGE_LOOP('',(#65504,#65505,#65506));
#15798=EDGE_LOOP('',(#65507,#65508,#65509));
#15799=EDGE_LOOP('',(#65510,#65511,#65512));
#15800=EDGE_LOOP('',(#65513,#65514,#65515));
#15801=EDGE_LOOP('',(#65516,#65517,#65518,#65519));
#15802=EDGE_LOOP('',(#65520,#65521,#65522,#65523));
#15803=EDGE_LOOP('',(#65524,#65525,#65526));
#15804=EDGE_LOOP('',(#65527,#65528,#65529));
#15805=EDGE_LOOP('',(#65530,#65531,#65532));
#15806=EDGE_LOOP('',(#65533,#65534,#65535));
#15807=EDGE_LOOP('',(#65536,#65537,#65538,#65539));
#15808=EDGE_LOOP('',(#65540,#65541,#65542,#65543));
#15809=EDGE_LOOP('',(#65544,#65545,#65546));
#15810=EDGE_LOOP('',(#65547,#65548,#65549));
#15811=EDGE_LOOP('',(#65550,#65551,#65552));
#15812=EDGE_LOOP('',(#65553,#65554,#65555));
#15813=EDGE_LOOP('',(#65556,#65557,#65558,#65559));
#15814=EDGE_LOOP('',(#65560,#65561,#65562,#65563));
#15815=EDGE_LOOP('',(#65564,#65565,#65566));
#15816=EDGE_LOOP('',(#65567,#65568,#65569));
#15817=EDGE_LOOP('',(#65570,#65571,#65572));
#15818=EDGE_LOOP('',(#65573,#65574,#65575));
#15819=EDGE_LOOP('',(#65576,#65577,#65578,#65579));
#15820=EDGE_LOOP('',(#65580,#65581,#65582,#65583));
#15821=EDGE_LOOP('',(#65584,#65585,#65586));
#15822=EDGE_LOOP('',(#65587,#65588,#65589));
#15823=EDGE_LOOP('',(#65590,#65591,#65592));
#15824=EDGE_LOOP('',(#65593,#65594,#65595));
#15825=EDGE_LOOP('',(#65596,#65597,#65598,#65599));
#15826=EDGE_LOOP('',(#65600,#65601,#65602,#65603));
#15827=EDGE_LOOP('',(#65604,#65605,#65606));
#15828=EDGE_LOOP('',(#65607,#65608,#65609));
#15829=EDGE_LOOP('',(#65610,#65611,#65612));
#15830=EDGE_LOOP('',(#65613,#65614,#65615));
#15831=EDGE_LOOP('',(#65616,#65617,#65618,#65619));
#15832=EDGE_LOOP('',(#65620,#65621,#65622,#65623));
#15833=EDGE_LOOP('',(#65624,#65625,#65626));
#15834=EDGE_LOOP('',(#65627,#65628,#65629));
#15835=EDGE_LOOP('',(#65630,#65631,#65632));
#15836=EDGE_LOOP('',(#65633,#65634,#65635));
#15837=EDGE_LOOP('',(#65636,#65637,#65638,#65639));
#15838=EDGE_LOOP('',(#65640,#65641,#65642,#65643));
#15839=EDGE_LOOP('',(#65644,#65645,#65646));
#15840=EDGE_LOOP('',(#65647,#65648,#65649));
#15841=EDGE_LOOP('',(#65650,#65651,#65652));
#15842=EDGE_LOOP('',(#65653,#65654,#65655));
#15843=EDGE_LOOP('',(#65656,#65657,#65658,#65659));
#15844=EDGE_LOOP('',(#65660,#65661,#65662,#65663));
#15845=EDGE_LOOP('',(#65664,#65665,#65666));
#15846=EDGE_LOOP('',(#65667,#65668,#65669));
#15847=EDGE_LOOP('',(#65670,#65671,#65672));
#15848=EDGE_LOOP('',(#65673,#65674,#65675));
#15849=EDGE_LOOP('',(#65676,#65677,#65678,#65679));
#15850=EDGE_LOOP('',(#65680));
#15851=EDGE_LOOP('',(#65681));
#15852=EDGE_LOOP('',(#65682));
#15853=EDGE_LOOP('',(#65683));
#15929=CIRCLE('',#71474,7.06860568617886);
#15930=CIRCLE('',#71475,7.33422742101415);
#15931=CIRCLE('',#71476,7.06860448235925);
#15932=CIRCLE('',#71477,7.33422663168221);
#15933=CIRCLE('',#71478,7.06860281197277);
#15934=CIRCLE('',#71479,7.3342250351839);
#15935=CIRCLE('',#71480,7.06860459613159);
#15936=CIRCLE('',#71481,7.33422732999641);
#15937=CIRCLE('',#71482,7.06860394071194);
#15938=CIRCLE('',#71483,7.33422671536983);
#15939=CIRCLE('',#71484,7.0686060491576);
#15940=CIRCLE('',#71485,7.33422717282189);
#15941=CIRCLE('',#71486,7.06860489976384);
#15942=CIRCLE('',#71487,7.33422669740432);
#15943=CIRCLE('',#71488,7.06860638429797);
#15944=CIRCLE('',#71489,7.33422795178459);
#15945=CIRCLE('',#71490,7.06860552820924);
#15946=CIRCLE('',#71491,7.33422734233105);
#15947=CIRCLE('',#71492,7.06860556698004);
#15948=CIRCLE('',#71493,7.3342273785942);
#15949=CIRCLE('',#71494,7.06860632435079);
#15950=CIRCLE('',#71495,7.33422770117462);
#15951=CIRCLE('',#71496,7.06860456983854);
#15952=CIRCLE('',#71497,7.33422661758376);
#15953=CIRCLE('',#71498,7.06860572631863);
#15954=CIRCLE('',#71499,7.33422765525036);
#15955=CIRCLE('',#71500,7.06860502971023);
#15956=CIRCLE('',#71501,7.33422693890404);
#15957=CIRCLE('',#71502,7.06860404038351);
#15958=CIRCLE('',#71503,7.33422645405152);
#15959=CIRCLE('',#71504,7.06860678325798);
#15960=CIRCLE('',#71505,7.33422776502736);
#15961=CIRCLE('',#71506,7.0686056226588);
#15962=CIRCLE('',#71507,7.33422778643665);
#15963=CIRCLE('',#71508,7.0686072750088);
#15964=CIRCLE('',#71509,7.33422787644434);
#15965=CIRCLE('',#71510,7.06860627067123);
#15966=CIRCLE('',#71511,7.3342277579675);
#15967=CIRCLE('',#71512,7.06860326789228);
#15968=CIRCLE('',#71513,7.33422642819733);
#15969=CIRCLE('',#71514,7.0686053869475);
#15970=CIRCLE('',#71515,7.33422736323035);
#15971=CIRCLE('',#71516,7.06860674407459);
#15972=CIRCLE('',#71517,7.33422795034231);
#15973=CIRCLE('',#71518,7.06860600194252);
#15974=CIRCLE('',#71519,7.33422781452826);
#15975=CIRCLE('',#71520,7.06860366903633);
#15976=CIRCLE('',#71521,7.33422629778949);
#15977=CIRCLE('',#71522,7.06860610926342);
#15978=CIRCLE('',#71523,7.33422735913368);
#15979=CIRCLE('',#71524,7.06860368230427);
#15980=CIRCLE('',#71525,7.33422671614766);
#15981=CIRCLE('',#71526,7.06860444583504);
#15982=CIRCLE('',#71527,7.33422706459965);
#15983=CIRCLE('',#71528,7.06860456725667);
#15984=CIRCLE('',#71529,7.33422708330648);
#15985=CIRCLE('',#71530,7.06860367611818);
#15986=CIRCLE('',#71531,7.33422714254166);
#15987=CIRCLE('',#71532,6.75);
#15988=CIRCLE('',#71534,3.25);
#15989=CIRCLE('',#71535,3.25);
#15990=CIRCLE('',#71538,7.);
#15991=CIRCLE('',#71539,7.);
#15992=CIRCLE('',#71541,6.125);
#15993=CIRCLE('',#71542,6.125);
#15994=CIRCLE('',#71543,6.125);
#15995=CIRCLE('',#71545,6.425);
#15996=CIRCLE('',#71547,7.33422710637909);
#15997=CIRCLE('',#71548,7.06860836336948);
#15998=CIRCLE('',#71549,7.33422732564574);
#15999=CIRCLE('',#71550,7.06860903695343);
#16000=CIRCLE('',#71551,7.33422702882346);
#16001=CIRCLE('',#71552,7.06860901744208);
#16002=CIRCLE('',#71553,7.3342266652849);
#16003=CIRCLE('',#71554,7.06860850262219);
#16004=CIRCLE('',#71555,7.33422732891954);
#16005=CIRCLE('',#71556,7.06860961375978);
#16006=CIRCLE('',#71557,7.33422624237877);
#16007=CIRCLE('',#71558,7.06860708111272);
#16008=CIRCLE('',#71559,7.33422780073948);
#16009=CIRCLE('',#71560,7.06861064290494);
#16010=CIRCLE('',#71561,7.33422793495388);
#16011=CIRCLE('',#71562,7.0686098556057);
#16012=CIRCLE('',#71563,7.33422761064981);
#16013=CIRCLE('',#71564,7.06861003408136);
#16014=CIRCLE('',#71565,7.33422637344204);
#16015=CIRCLE('',#71566,7.06860802586876);
#16016=CIRCLE('',#71567,7.33422773665016);
#16017=CIRCLE('',#71568,7.06861056875248);
#16018=CIRCLE('',#71569,7.3342281502456);
#16019=CIRCLE('',#71570,7.06861172275373);
#16020=CIRCLE('',#71571,7.33422777311646);
#16021=CIRCLE('',#71572,7.06861072746278);
#16022=CIRCLE('',#71573,7.33422774759614);
#16023=CIRCLE('',#71574,7.06861069549746);
#16024=CIRCLE('',#71575,7.33422668479825);
#16025=CIRCLE('',#71576,7.06860648295125);
#16026=CIRCLE('',#71577,6.75);
#16027=CIRCLE('',#71578,7.33422546202569);
#16028=CIRCLE('',#71579,7.06860901630615);
#16029=CIRCLE('',#71580,7.33422758661738);
#16030=CIRCLE('',#71581,7.06860917719902);
#16031=CIRCLE('',#71582,7.33422552125982);
#16032=CIRCLE('',#71583,7.06860817918064);
#16033=CIRCLE('',#71584,7.33422791354406);
#16034=CIRCLE('',#71585,7.06861114651049);
#16035=CIRCLE('',#71586,7.33422729522531);
#16036=CIRCLE('',#71587,7.06860906896761);
#16037=CIRCLE('',#71588,7.33422754578351);
#16038=CIRCLE('',#71589,7.06860992934319);
#16039=CIRCLE('',#71590,7.33422816391154);
#16040=CIRCLE('',#71591,7.06861129437419);
#16041=CIRCLE('',#71592,7.33422524915925);
#16042=CIRCLE('',#71593,7.06860889389819);
#16043=CIRCLE('',#71594,7.33422708826522);
#16044=CIRCLE('',#71595,7.06860930316695);
#16045=CIRCLE('',#71596,7.33422690268295);
#16046=CIRCLE('',#71597,7.06860890902957);
#16047=CIRCLE('',#71598,7.33422725159127);
#16048=CIRCLE('',#71599,7.06860891185296);
#16049=CIRCLE('',#71600,7.33422516944886);
#16050=CIRCLE('',#71601,7.06860779698365);
#16051=CIRCLE('',#71602,7.33422681347524);
#16052=CIRCLE('',#71603,7.06860860032496);
#16053=CIRCLE('',#71604,7.33422734754571);
#16054=CIRCLE('',#71605,7.06861007792251);
#16055=CIRCLE('',#71607,7.65641797830405);
#16056=CIRCLE('',#71608,7.74391301990334);
#16057=CIRCLE('',#71610,7.74376760109424);
#16058=CIRCLE('',#71612,7.69259377819036);
#16059=CIRCLE('',#71613,7.68762408392115);
#16060=CIRCLE('',#71614,7.50000000109902);
#16061=CIRCLE('',#71615,7.69302971312151);
#16062=CIRCLE('',#71617,7.69146686117127);
#16063=CIRCLE('',#71618,7.69282866600189);
#16064=CIRCLE('',#71620,7.65227963154115);
#16065=CIRCLE('',#71622,7.65227968597654);
#16066=CIRCLE('',#71624,7.68301219447606);
#16067=CIRCLE('',#71625,7.69191399109765);
#16068=CIRCLE('',#71627,7.4999999993286);
#16069=CIRCLE('',#71628,7.6876252604557);
#16070=CIRCLE('',#71629,7.6925870430687);
#16071=CIRCLE('',#71630,7.6930268168054);
#16072=CIRCLE('',#71632,7.82251869020954);
#16073=CIRCLE('',#71634,7.68619221526501);
#16074=CIRCLE('',#71636,7.69282870015808);
#16075=CIRCLE('',#71637,7.69146686065975);
#16076=CIRCLE('',#71639,7.6929092573408);
#16077=CIRCLE('',#71640,7.6851083393197);
#16078=CIRCLE('',#71642,7.69191399110767);
#16079=CIRCLE('',#71643,7.68301221228793);
#16080=CIRCLE('',#71645,7.69207568232512);
#16081=CIRCLE('',#71646,7.69297980315297);
#16082=CIRCLE('',#71648,7.68619221509267);
#16083=CIRCLE('',#71650,7.69242170452788);
#16084=CIRCLE('',#71652,7.68475592667959);
#16085=CIRCLE('',#71654,7.69297983680142);
#16086=CIRCLE('',#71655,7.6920756821004);
#16087=CIRCLE('',#71657,7.69301888945012);
#16088=CIRCLE('',#71658,7.68356129670636);
#16089=CIRCLE('',#71660,7.69242170506121);
#16090=CIRCLE('',#71662,7.69254650683266);
#16091=CIRCLE('',#71663,7.69306084204855);
#16092=CIRCLE('',#71665,7.68475592668143);
#16093=CIRCLE('',#71667,7.69279341210589);
#16094=CIRCLE('',#71669,7.68355912148237);
#16095=CIRCLE('',#71670,7.69301686910343);
#16096=CIRCLE('',#71672,7.68318440412029);
#16097=CIRCLE('',#71674,7.69306086163512);
#16098=CIRCLE('',#71675,7.69254650650468);
#16099=CIRCLE('',#71677,7.6930586350727);
#16100=CIRCLE('',#71679,7.69287888052477);
#16101=CIRCLE('',#71680,7.69291157795238);
#16102=CIRCLE('',#71682,7.68318440411841);
#16103=CIRCLE('',#71684,7.69302871560608);
#16104=CIRCLE('',#71686,7.69305436245181);
#16105=CIRCLE('',#71689,7.69291157795224);
#16106=CIRCLE('',#71690,7.69287888052691);
#16107=CIRCLE('',#71692,7.69302871457533);
#16108=CIRCLE('',#71693,7.6876542201912);
#16109=CIRCLE('',#71694,7.44531753045275);
#16110=CIRCLE('',#71695,7.69302855940779);
#16111=CIRCLE('',#71696,7.44956381440377);
#16112=CIRCLE('',#71698,7.69059190152309);
#16113=CIRCLE('',#71699,7.68765459393669);
#16114=CIRCLE('',#71700,7.44531744983399);
#16115=CIRCLE('',#71701,7.69302885642449);
#16116=CIRCLE('',#71702,7.44956398909122);
#16117=CIRCLE('',#71704,7.69059185498203);
#16118=CIRCLE('',#71705,7.68765421571228);
#16119=CIRCLE('',#71706,7.44531728606217);
#16120=CIRCLE('',#71707,7.69302869881902);
#16121=CIRCLE('',#71708,7.44956390637391);
#16122=CIRCLE('',#71710,7.69059194313262);
#16123=CIRCLE('',#71711,7.68765427778048);
#16124=CIRCLE('',#71712,7.44531736610272);
#16125=CIRCLE('',#71713,7.69302857882909);
#16126=CIRCLE('',#71714,7.44956382734777);
#16127=CIRCLE('',#71716,7.69059182512427);
#16128=CIRCLE('',#71717,7.68765420156565);
#16129=CIRCLE('',#71718,7.44531757419449);
#16130=CIRCLE('',#71719,7.69302854010545);
#16131=CIRCLE('',#71720,7.449564220458);
#16132=CIRCLE('',#71722,7.69059201621511);
#16133=CIRCLE('',#71723,7.68765429038083);
#16134=CIRCLE('',#71724,7.44531728849294);
#16135=CIRCLE('',#71725,7.69302868404055);
#16136=CIRCLE('',#71726,7.44956402238821);
#16137=CIRCLE('',#71728,7.69059208059763);
#16138=CIRCLE('',#71729,7.68765413677979);
#16139=CIRCLE('',#71730,7.44531741562678);
#16140=CIRCLE('',#71731,7.44956416165948);
#16141=CIRCLE('',#71732,7.4453174835798);
#16142=CIRCLE('',#71733,7.69302857388115);
#16143=CIRCLE('',#71734,7.44956389304265);
#16144=CIRCLE('',#71736,7.69059204207201);
#16145=CIRCLE('',#71737,7.6876544760258);
#16146=CIRCLE('',#71738,7.44531737564562);
#16147=CIRCLE('',#71739,7.69302857633999);
#16148=CIRCLE('',#71740,7.44956413304808);
#16149=CIRCLE('',#71742,7.69059201870121);
#16150=CIRCLE('',#71743,7.68765433896887);
#16151=CIRCLE('',#71744,7.4453173960003);
#16152=CIRCLE('',#71745,7.6930287505808);
#16153=CIRCLE('',#71746,7.44956385182571);
#16154=CIRCLE('',#71748,7.690591959103);
#16155=CIRCLE('',#71749,7.68765455691847);
#16156=CIRCLE('',#71750,7.44531750464958);
#16157=CIRCLE('',#71751,7.69302872583272);
#16158=CIRCLE('',#71752,7.44956399165334);
#16159=CIRCLE('',#71754,7.69059185749854);
#16160=CIRCLE('',#71755,7.68765412355323);
#16161=CIRCLE('',#71756,7.44531742994769);
#16162=CIRCLE('',#71757,7.69302859365467);
#16163=CIRCLE('',#71758,7.4495641794038);
#16164=CIRCLE('',#71760,7.69059223800863);
#16165=CIRCLE('',#71761,7.68765432051477);
#16166=CIRCLE('',#71762,7.44531749413859);
#16167=CIRCLE('',#71763,7.69302870979168);
#16168=CIRCLE('',#71764,7.44956417574996);
#16169=CIRCLE('',#71766,7.69059211381182);
#16170=CIRCLE('',#71767,7.68765415326971);
#16171=CIRCLE('',#71768,7.4453174810649);
#16172=CIRCLE('',#71769,7.69302883594045);
#16173=CIRCLE('',#71770,7.44956398258887);
#16174=CIRCLE('',#71772,7.69059215577665);
#16175=CIRCLE('',#71773,7.68765415092922);
#16176=CIRCLE('',#71774,7.44531730976456);
#16177=CIRCLE('',#71775,7.69302855372752);
#16178=CIRCLE('',#71776,7.44956411333289);
#16179=CIRCLE('',#71778,7.69059175946082);
#16180=CIRCLE('',#71779,7.68765427356153);
#16181=CIRCLE('',#71780,7.44531745154568);
#16182=CIRCLE('',#71781,7.6930287837275);
#16183=CIRCLE('',#71782,7.44956391452336);
#16184=CIRCLE('',#71784,7.69059176728946);
#16185=CIRCLE('',#71785,7.68765435654041);
#16186=CIRCLE('',#71786,7.44531756343616);
#16187=CIRCLE('',#71787,7.69302889099309);
#16188=CIRCLE('',#71788,7.44956401906168);
#16189=CIRCLE('',#71790,7.69059179330732);
#16190=CIRCLE('',#71791,7.68765408720567);
#16191=CIRCLE('',#71792,7.44531755818733);
#16192=CIRCLE('',#71793,7.69302850275609);
#16193=CIRCLE('',#71794,7.44956393089751);
#16194=CIRCLE('',#71796,7.69059188019343);
#16195=CIRCLE('',#71797,7.68765433601994);
#16196=CIRCLE('',#71798,7.44531736902152);
#16197=CIRCLE('',#71799,7.69302878495204);
#16198=CIRCLE('',#71800,7.4495640374712);
#16199=CIRCLE('',#71802,7.69059212825047);
#16200=CIRCLE('',#71803,7.68765443964002);
#16201=CIRCLE('',#71804,7.44531739629565);
#16202=CIRCLE('',#71805,7.69302875141739);
#16203=CIRCLE('',#71806,7.44956382538056);
#16204=CIRCLE('',#71808,7.69059171696194);
#16205=CIRCLE('',#71809,7.68765428236649);
#16206=CIRCLE('',#71810,7.44531717926382);
#16207=CIRCLE('',#71811,7.69302889308604);
#16208=CIRCLE('',#71812,7.44956403577385);
#16209=CIRCLE('',#71814,7.69059180814142);
#16210=CIRCLE('',#71815,7.68765408817977);
#16211=CIRCLE('',#71816,7.44531754817613);
#16212=CIRCLE('',#71817,7.69302862085918);
#16213=CIRCLE('',#71818,7.44956414197099);
#16214=CIRCLE('',#71820,7.69059184122841);
#16215=CIRCLE('',#71821,7.68765444403783);
#16216=CIRCLE('',#71822,7.44531741523388);
#16217=CIRCLE('',#71823,7.6930286242407);
#16218=CIRCLE('',#71824,7.4495640397283);
#16219=CIRCLE('',#71826,7.69059178463958);
#16220=CIRCLE('',#71827,7.68765415898238);
#16221=CIRCLE('',#71828,7.44531739985699);
#16222=CIRCLE('',#71829,7.6930286520143);
#16223=CIRCLE('',#71830,7.44956409048606);
#16224=CIRCLE('',#71832,7.69059177271397);
#16225=CIRCLE('',#71833,7.68765414461077);
#16226=CIRCLE('',#71834,7.44531743415826);
#16227=CIRCLE('',#71835,7.69302855341372);
#16228=CIRCLE('',#71836,7.44956396224489);
#16229=CIRCLE('',#71837,7.68765176778231);
#16230=CIRCLE('',#71838,7.44531744815501);
#16231=CIRCLE('',#71840,7.69058939824306);
#16232=CIRCLE('',#71841,7.69302853509787);
#16233=CIRCLE('',#71842,7.44956392538232);
#16234=CIRCLE('',#71844,7.68765433956961);
#16235=CIRCLE('',#71845,7.69059203749584);
#16236=CIRCLE('',#71846,7.44531750825384);
#16237=CIRCLE('',#71847,7.69302869291321);
#16238=CIRCLE('',#71848,7.44956384698696);
#16239=CIRCLE('',#71850,7.69059210187196);
#16240=CIRCLE('',#71851,7.68765420261813);
#16241=CIRCLE('',#71852,7.44531758073562);
#16242=CIRCLE('',#71853,7.69302875800088);
#16243=CIRCLE('',#71854,7.44956383396013);
#16244=CIRCLE('',#71856,7.69059192649959);
#16245=CIRCLE('',#71857,7.68765418531522);
#16246=CIRCLE('',#71858,7.44531752816521);
#16247=CIRCLE('',#71860,7.69059202624217);
#16248=CIRCLE('',#71861,7.69302857898078);
#16249=CIRCLE('',#71862,7.44956388529172);
#16250=CIRCLE('',#71863,7.68994784729622);
#16251=CIRCLE('',#71864,7.69291176352318);
#16252=CIRCLE('',#71865,7.68994816169627);
#16253=CIRCLE('',#71867,7.69287916191551);
#16254=CIRCLE('',#71868,7.6908160876836);
#16255=CIRCLE('',#71869,7.69291193954018);
#16256=CIRCLE('',#71870,7.68994804701675);
#16257=CIRCLE('',#71872,7.6928791090222);
#16258=CIRCLE('',#71873,7.69081611331132);
#16259=CIRCLE('',#71874,7.69291178900954);
#16260=CIRCLE('',#71875,7.68994811657411);
#16261=CIRCLE('',#71877,7.69287932800169);
#16262=CIRCLE('',#71878,7.69081621527755);
#16263=CIRCLE('',#71879,7.6929116428541);
#16264=CIRCLE('',#71880,7.68994801473022);
#16265=CIRCLE('',#71882,7.6928789811809);
#16266=CIRCLE('',#71883,7.69081626752787);
#16267=CIRCLE('',#71884,7.69291192595448);
#16268=CIRCLE('',#71885,7.68994801135637);
#16269=CIRCLE('',#71887,7.69287905800627);
#16270=CIRCLE('',#71888,7.69081623259295);
#16271=CIRCLE('',#71889,7.69291165110062);
#16272=CIRCLE('',#71890,7.68994773730798);
#16273=CIRCLE('',#71892,7.6928792873396);
#16274=CIRCLE('',#71893,7.69081618096169);
#16275=CIRCLE('',#71894,7.69291179086277);
#16276=CIRCLE('',#71895,7.68994794565019);
#16277=CIRCLE('',#71897,7.69287917492001);
#16278=CIRCLE('',#71898,7.69081634191757);
#16279=CIRCLE('',#71899,7.69291211427012);
#16280=CIRCLE('',#71900,7.68994805258136);
#16281=CIRCLE('',#71902,7.69287935101192);
#16282=CIRCLE('',#71903,7.69081651118216);
#16283=CIRCLE('',#71904,7.69291165495763);
#16284=CIRCLE('',#71905,7.68994777136307);
#16285=CIRCLE('',#71907,7.69287897129759);
#16286=CIRCLE('',#71908,7.69081622705858);
#16287=CIRCLE('',#71909,7.69291174915485);
#16288=CIRCLE('',#71910,7.68994804232604);
#16289=CIRCLE('',#71912,7.692879343557);
#16290=CIRCLE('',#71913,7.69081608567409);
#16291=CIRCLE('',#71914,7.69291185563374);
#16292=CIRCLE('',#71915,7.6899479663059);
#16293=CIRCLE('',#71917,7.69287915934469);
#16294=CIRCLE('',#71918,7.69081633928341);
#16295=CIRCLE('',#71919,7.69291176261412);
#16296=CIRCLE('',#71920,7.68994794141999);
#16297=CIRCLE('',#71922,7.69287899177592);
#16298=CIRCLE('',#71923,7.6908164149815);
#16299=CIRCLE('',#71924,7.69291196007127);
#16300=CIRCLE('',#71925,7.68994808931707);
#16301=CIRCLE('',#71927,7.69287910182314);
#16302=CIRCLE('',#71928,7.69081639280079);
#16303=CIRCLE('',#71929,7.69291189125349);
#16304=CIRCLE('',#71930,7.68994771203019);
#16305=CIRCLE('',#71932,7.6928791573007);
#16306=CIRCLE('',#71933,7.69081611679542);
#16307=CIRCLE('',#71934,7.69291202082821);
#16308=CIRCLE('',#71935,7.68994808377934);
#16309=CIRCLE('',#71937,7.69287910535088);
#16310=CIRCLE('',#71938,7.69081634517804);
#16311=CIRCLE('',#71939,7.69291175642132);
#16312=CIRCLE('',#71940,7.68994812033888);
#16313=CIRCLE('',#71942,7.69287902700107);
#16314=CIRCLE('',#71943,7.69081646367517);
#16315=CIRCLE('',#71944,7.69291180726244);
#16316=CIRCLE('',#71945,7.68994797217316);
#16317=CIRCLE('',#71947,7.69287923229888);
#16318=CIRCLE('',#71948,7.69081620173846);
#16319=CIRCLE('',#71949,7.69291195486759);
#16320=CIRCLE('',#71950,7.68994791200507);
#16321=CIRCLE('',#71952,7.69287901866562);
#16322=CIRCLE('',#71953,7.6908162110816);
#16323=CIRCLE('',#71954,7.69291190742198);
#16324=CIRCLE('',#71955,7.68994789696625);
#16325=CIRCLE('',#71957,7.69287911479319);
#16326=CIRCLE('',#71958,7.69081629142424);
#16327=CIRCLE('',#71959,7.69291178333012);
#16328=CIRCLE('',#71960,7.68994811317839);
#16329=CIRCLE('',#71962,7.69287918394);
#16330=CIRCLE('',#71963,7.69081642538975);
#16331=CIRCLE('',#71964,7.69291204322326);
#16332=CIRCLE('',#71965,7.68994813733287);
#16333=CIRCLE('',#71967,7.69287899878939);
#16334=CIRCLE('',#71968,7.69081618466236);
#16335=CIRCLE('',#71969,7.69291183628174);
#16336=CIRCLE('',#71970,7.68994796202815);
#16337=CIRCLE('',#71972,7.69287933504919);
#16338=CIRCLE('',#71973,7.69081628474869);
#16339=CIRCLE('',#71974,7.69291197483368);
#16340=CIRCLE('',#71975,7.68994786758217);
#16341=CIRCLE('',#71977,7.69287921910946);
#16342=CIRCLE('',#71978,7.69081621348498);
#16343=CIRCLE('',#71979,7.69291174121852);
#16344=CIRCLE('',#71980,7.68994793911777);
#16345=CIRCLE('',#71982,7.69287914100389);
#16346=CIRCLE('',#71983,7.69081625308633);
#16347=CIRCLE('',#71984,7.69291162670279);
#16348=CIRCLE('',#71985,7.68994817762516);
#16349=CIRCLE('',#71987,7.69287912011789);
#16350=CIRCLE('',#71988,7.69081627762047);
#16351=CIRCLE('',#71989,7.69291180931249);
#16352=CIRCLE('',#71990,7.68994787650908);
#16353=CIRCLE('',#71992,7.69287925074076);
#16354=CIRCLE('',#71993,7.69081632400146);
#16355=CIRCLE('',#71994,7.69291183764281);
#16356=CIRCLE('',#71995,7.68994780337762);
#16357=CIRCLE('',#71997,7.69287902948873);
#16358=CIRCLE('',#71998,7.690816416425);
#16359=CIRCLE('',#72000,7.69291178964756);
#16360=CIRCLE('',#72001,7.69287934994747);
#16361=CIRCLE('',#72002,7.69081607066127);
#16362=CIRCLE('',#72003,7.44610039872259);
#16363=CIRCLE('',#72004,7.44610202947899);
#16364=CIRCLE('',#72005,7.44610171256494);
#16365=CIRCLE('',#72006,7.44610190544556);
#16366=CIRCLE('',#72007,7.44610194146778);
#16367=CIRCLE('',#72008,7.44610192630802);
#16368=CIRCLE('',#72009,7.44610186558304);
#16369=CIRCLE('',#72010,7.44610174233441);
#16370=CIRCLE('',#72011,7.446101890378);
#16371=CIRCLE('',#72012,7.4461017456576);
#16372=CIRCLE('',#72013,7.44610210531308);
#16373=CIRCLE('',#72014,7.4461020734202);
#16374=CIRCLE('',#72015,7.4461016563064);
#16375=CIRCLE('',#72016,7.44610189129619);
#16376=CIRCLE('',#72017,7.44610194481567);
#16377=CIRCLE('',#72018,7.44610180901079);
#16378=CIRCLE('',#72019,7.44610197957406);
#16379=CIRCLE('',#72020,7.44610171930393);
#16380=CIRCLE('',#72021,7.446101819203);
#16381=CIRCLE('',#72022,7.44610201214073);
#16382=CIRCLE('',#72023,7.44610203318976);
#16383=CIRCLE('',#72024,7.446102073294);
#16384=CIRCLE('',#72025,7.44610208015893);
#16385=CIRCLE('',#72026,7.44610205614831);
#16386=CIRCLE('',#72027,7.44610194233016);
#16387=CIRCLE('',#72028,7.44610181860739);
#16388=CIRCLE('',#72029,7.44610173753958);
#16389=CIRCLE('',#72030,7.44610226722038);
#16390=CIRCLE('',#72031,7.44610178954819);
#16391=CIRCLE('',#72032,7.44636428442216);
#16392=CIRCLE('',#72033,7.44966336559066);
#16393=CIRCLE('',#72034,7.4463619325723);
#16394=CIRCLE('',#72035,7.4496658498726);
#16395=CIRCLE('',#72036,7.4463620247186);
#16396=CIRCLE('',#72037,7.44966320020384);
#16397=CIRCLE('',#72038,7.44636200075496);
#16398=CIRCLE('',#72039,7.44966333026173);
#16399=CIRCLE('',#72040,7.44636191238419);
#16400=CIRCLE('',#72041,7.44966333924492);
#16401=CIRCLE('',#72042,7.44636196252416);
#16402=CIRCLE('',#72043,7.4496632872419);
#16403=CIRCLE('',#72044,7.44636196485215);
#16404=CIRCLE('',#72045,7.44966313666938);
#16405=CIRCLE('',#72046,7.44636197685158);
#16406=CIRCLE('',#72047,7.44966574562592);
#16407=CIRCLE('',#72048,7.44636166648237);
#16408=CIRCLE('',#72049,7.44966570381846);
#16409=CIRCLE('',#72050,7.44636196987988);
#16410=CIRCLE('',#72051,7.44966318966342);
#16411=CIRCLE('',#72052,7.44636215724432);
#16412=CIRCLE('',#72053,7.44966321197049);
#16413=CIRCLE('',#72054,7.44636200455026);
#16414=CIRCLE('',#72055,7.44966307490526);
#16415=CIRCLE('',#72056,7.44636191277395);
#16416=CIRCLE('',#72057,7.44966334625715);
#16417=CIRCLE('',#72058,7.44636197765117);
#16418=CIRCLE('',#72059,7.44966578539828);
#16419=CIRCLE('',#72060,7.44636171142628);
#16420=CIRCLE('',#72061,7.44966318204415);
#16421=CIRCLE('',#72062,7.4463619250286);
#16422=CIRCLE('',#72063,7.44966329395594);
#16423=CIRCLE('',#72064,7.44636184648991);
#16424=CIRCLE('',#72065,7.44966299354813);
#16425=CIRCLE('',#72066,7.44636186285757);
#16426=CIRCLE('',#72067,7.44966326944477);
#16427=CIRCLE('',#72068,7.44636419296111);
#16428=CIRCLE('',#72069,7.44966326236774);
#16429=CIRCLE('',#72070,7.44636197667011);
#16430=CIRCLE('',#72071,7.44966331460107);
#16431=CIRCLE('',#72072,7.44636210971674);
#16432=CIRCLE('',#72073,7.44966336557813);
#16433=CIRCLE('',#72074,7.44636219915216);
#16434=CIRCLE('',#72075,7.44966325286483);
#16435=CIRCLE('',#72076,7.4463620609399);
#16436=CIRCLE('',#72077,7.44966341877736);
#16437=CIRCLE('',#72078,7.44636193742211);
#16438=CIRCLE('',#72079,7.44966321797681);
#16439=CIRCLE('',#72080,7.44636182606499);
#16440=CIRCLE('',#72081,7.44966335654635);
#16441=CIRCLE('',#72082,7.44636204558943);
#16442=CIRCLE('',#72083,7.44966309407696);
#16443=CIRCLE('',#72084,7.44636178384992);
#16444=CIRCLE('',#72085,7.44966347089608);
#16445=CIRCLE('',#72086,7.446361748607);
#16446=CIRCLE('',#72087,7.44966325127484);
#16447=CIRCLE('',#72088,7.44636423009231);
#16448=CIRCLE('',#72089,7.44966580117451);
#16449=CIRCLE('',#72090,7.68852788878312);
#16450=CIRCLE('',#72092,7.68852788871217);
#16451=CIRCLE('',#72093,7.68852808094441);
#16452=CIRCLE('',#72095,7.68852808077644);
#16453=CIRCLE('',#72096,7.68852810841195);
#16454=CIRCLE('',#72098,7.68852810831765);
#16455=CIRCLE('',#72099,7.68852802787468);
#16456=CIRCLE('',#72101,7.68852802770763);
#16457=CIRCLE('',#72102,7.68852784840945);
#16458=CIRCLE('',#72104,7.68852784822142);
#16459=CIRCLE('',#72105,7.68852798010456);
#16460=CIRCLE('',#72107,7.68852798008635);
#16461=CIRCLE('',#72108,7.68852791683948);
#16462=CIRCLE('',#72110,7.6885279167122);
#16463=CIRCLE('',#72111,7.68852821066941);
#16464=CIRCLE('',#72113,7.68852821049969);
#16465=CIRCLE('',#72114,7.68852792917552);
#16466=CIRCLE('',#72116,7.68852792897721);
#16467=CIRCLE('',#72117,7.6885281434879);
#16468=CIRCLE('',#72119,7.68852814345323);
#16469=CIRCLE('',#72120,7.6885279546106);
#16470=CIRCLE('',#72122,7.68852795458423);
#16471=CIRCLE('',#72123,7.68852820378617);
#16472=CIRCLE('',#72125,7.68852820377537);
#16473=CIRCLE('',#72126,7.68852816718055);
#16474=CIRCLE('',#72128,7.68852816717759);
#16475=CIRCLE('',#72129,7.68852828726958);
#16476=CIRCLE('',#72131,7.68852828726758);
#16477=CIRCLE('',#72132,7.68852819473631);
#16478=CIRCLE('',#72134,7.68852819473974);
#16479=CIRCLE('',#72135,7.68852826003133);
#16480=CIRCLE('',#72137,7.68852826001605);
#16481=CIRCLE('',#72138,7.68852802375798);
#16482=CIRCLE('',#72140,7.68852802354785);
#16483=CIRCLE('',#72141,7.68852798333981);
#16484=CIRCLE('',#72143,7.6885279833);
#16485=CIRCLE('',#72144,7.68852790420368);
#16486=CIRCLE('',#72146,7.68852790420423);
#16487=CIRCLE('',#72147,7.68852797344957);
#16488=CIRCLE('',#72149,7.68852797345006);
#16489=CIRCLE('',#72150,7.68852812311045);
#16490=CIRCLE('',#72152,7.68852812311494);
#16491=CIRCLE('',#72153,7.6885280418327);
#16492=CIRCLE('',#72155,7.68852804183216);
#16493=CIRCLE('',#72156,7.68852794146179);
#16494=CIRCLE('',#72158,7.6885279414636);
#16495=CIRCLE('',#72159,7.68852772382627);
#16496=CIRCLE('',#72161,7.68852798822317);
#16497=CIRCLE('',#72162,7.68852794982855);
#16498=CIRCLE('',#72164,7.68852794991581);
#16499=CIRCLE('',#72165,7.68852776699871);
#16500=CIRCLE('',#72167,7.68852776692866);
#16501=CIRCLE('',#72168,7.68852774428418);
#16502=CIRCLE('',#72170,7.68852774423606);
#16503=CIRCLE('',#72171,7.68852783383721);
#16504=CIRCLE('',#72173,7.68852783378586);
#16505=CIRCLE('',#72174,7.68881294990728);
#16506=CIRCLE('',#72175,7.69305416871896);
#16507=CIRCLE('',#72177,7.6913546432824);
#16508=CIRCLE('',#72178,7.68881279059509);
#16509=CIRCLE('',#72179,7.69305425122366);
#16510=CIRCLE('',#72181,7.6913547410763);
#16511=CIRCLE('',#72182,7.68881286886724);
#16512=CIRCLE('',#72183,7.69305407050621);
#16513=CIRCLE('',#72185,7.6913548164225);
#16514=CIRCLE('',#72186,7.68881281359015);
#16515=CIRCLE('',#72187,7.69305419630861);
#16516=CIRCLE('',#72189,7.69135444944937);
#16517=CIRCLE('',#72190,7.68881291627626);
#16518=CIRCLE('',#72191,7.69305434953605);
#16519=CIRCLE('',#72193,7.69135469952928);
#16520=CIRCLE('',#72194,7.68881295725583);
#16521=CIRCLE('',#72195,7.6930541867945);
#16522=CIRCLE('',#72197,7.69135471403681);
#16523=CIRCLE('',#72198,7.68881304041654);
#16524=CIRCLE('',#72199,7.69305427557526);
#16525=CIRCLE('',#72201,7.6913545848261);
#16526=CIRCLE('',#72202,7.68881310970619);
#16527=CIRCLE('',#72203,7.69305424819788);
#16528=CIRCLE('',#72205,7.69135474309964);
#16529=CIRCLE('',#72206,7.6888131572352);
#16530=CIRCLE('',#72207,7.69305440873283);
#16531=CIRCLE('',#72209,7.6913547760876);
#16532=CIRCLE('',#72210,7.68881286389501);
#16533=CIRCLE('',#72211,7.6930543592403);
#16534=CIRCLE('',#72213,7.69135446595711);
#16535=CIRCLE('',#72214,7.68881294817899);
#16536=CIRCLE('',#72215,7.69305419837545);
#16537=CIRCLE('',#72217,7.69135491750166);
#16538=CIRCLE('',#72218,7.68881291089276);
#16539=CIRCLE('',#72219,7.69305429863986);
#16540=CIRCLE('',#72221,7.69135473804577);
#16541=CIRCLE('',#72222,7.6888130380488);
#16542=CIRCLE('',#72223,7.69305440505359);
#16543=CIRCLE('',#72225,7.69135457467);
#16544=CIRCLE('',#72226,7.68881275452481);
#16545=CIRCLE('',#72227,7.69305399990696);
#16546=CIRCLE('',#72229,7.69135445363969);
#16547=CIRCLE('',#72230,7.68881300384858);
#16548=CIRCLE('',#72231,7.69305432864807);
#16549=CIRCLE('',#72233,7.6913547228451);
#16550=CIRCLE('',#72234,7.68881285338845);
#16551=CIRCLE('',#72235,7.69305403777903);
#16552=CIRCLE('',#72237,7.69135477789989);
#16553=CIRCLE('',#72238,7.68881325214323);
#16554=CIRCLE('',#72239,7.69305437016307);
#16555=CIRCLE('',#72241,7.69135463961681);
#16556=CIRCLE('',#72242,7.68881274595675);
#16557=CIRCLE('',#72243,7.69305424024155);
#16558=CIRCLE('',#72245,7.691354591453);
#16559=CIRCLE('',#72246,7.68881313601843);
#16560=CIRCLE('',#72247,7.69305423658223);
#16561=CIRCLE('',#72249,7.69135483048538);
#16562=CIRCLE('',#72250,7.68881313175157);
#16563=CIRCLE('',#72251,7.69305421496098);
#16564=CIRCLE('',#72253,7.69135483246873);
#16565=CIRCLE('',#72254,7.68881287351973);
#16566=CIRCLE('',#72255,7.69305415299332);
#16567=CIRCLE('',#72257,7.69135468194924);
#16568=CIRCLE('',#72258,7.68881305745295);
#16569=CIRCLE('',#72259,7.69305441708648);
#16570=CIRCLE('',#72261,7.69135467139016);
#16571=CIRCLE('',#72262,7.6888130343247);
#16572=CIRCLE('',#72263,7.69305425088512);
#16573=CIRCLE('',#72265,7.69135479635185);
#16574=CIRCLE('',#72266,7.68881329210462);
#16575=CIRCLE('',#72267,7.69305436804117);
#16576=CIRCLE('',#72269,7.6913544468307);
#16577=CIRCLE('',#72270,7.68881306344792);
#16578=CIRCLE('',#72271,7.69305414738288);
#16579=CIRCLE('',#72273,7.69135456385503);
#16580=CIRCLE('',#72274,7.68881318269362);
#16581=CIRCLE('',#72275,7.69305422279801);
#16582=CIRCLE('',#72277,7.69135469458882);
#16583=CIRCLE('',#72278,7.68881305420038);
#16584=CIRCLE('',#72279,7.6930542709141);
#16585=CIRCLE('',#72281,7.69135459595344);
#16586=CIRCLE('',#72282,7.68881312219884);
#16587=CIRCLE('',#72283,7.69305435220014);
#16588=CIRCLE('',#72285,7.69135478455061);
#16589=CIRCLE('',#72286,7.44609831292764);
#16590=CIRCLE('',#72287,7.44609962301868);
#16591=CIRCLE('',#72288,7.44609935175357);
#16592=CIRCLE('',#72289,7.44609956374778);
#16593=CIRCLE('',#72290,7.44609960110811);
#16594=CIRCLE('',#72291,7.44609976907078);
#16595=CIRCLE('',#72292,7.44609970176048);
#16596=CIRCLE('',#72293,7.4460998316161);
#16597=CIRCLE('',#72294,7.44609995608563);
#16598=CIRCLE('',#72295,7.44609954146893);
#16599=CIRCLE('',#72296,7.44610000859957);
#16600=CIRCLE('',#72297,7.44609964341751);
#16601=CIRCLE('',#72298,7.44609943228571);
#16602=CIRCLE('',#72299,7.44609967299467);
#16603=CIRCLE('',#72300,7.4460995580868);
#16604=CIRCLE('',#72301,7.44609952767346);
#16605=CIRCLE('',#72302,7.44609942719343);
#16606=CIRCLE('',#72303,7.44609953709856);
#16607=CIRCLE('',#72304,7.44609964556177);
#16608=CIRCLE('',#72305,7.4460996868155);
#16609=CIRCLE('',#72306,7.44609954955322);
#16610=CIRCLE('',#72307,7.44609968798886);
#16611=CIRCLE('',#72308,7.44609966377836);
#16612=CIRCLE('',#72309,7.44609989884677);
#16613=CIRCLE('',#72310,7.44609968307516);
#16614=CIRCLE('',#72311,7.44609972796809);
#16615=CIRCLE('',#72312,7.44609940228724);
#16616=CIRCLE('',#72313,7.44609997449684);
#16617=CIRCLE('',#72314,7.44609986988839);
#16618=CIRCLE('',#72315,7.44703765958231);
#16619=CIRCLE('',#72316,7.44703740592205);
#16620=CIRCLE('',#72317,7.44703728970287);
#16621=CIRCLE('',#72318,7.44703734046266);
#16622=CIRCLE('',#72319,7.44703750753235);
#16623=CIRCLE('',#72320,7.44703765689882);
#16624=CIRCLE('',#72321,7.44703757846929);
#16625=CIRCLE('',#72322,7.4470374290604);
#16626=CIRCLE('',#72323,7.44703734393595);
#16627=CIRCLE('',#72324,7.44703746303222);
#16628=CIRCLE('',#72325,7.44703758748381);
#16629=CIRCLE('',#72326,7.44703737549802);
#16630=CIRCLE('',#72327,7.44703743508742);
#16631=CIRCLE('',#72328,7.44703765138706);
#16632=CIRCLE('',#72329,7.44703743978475);
#16633=CIRCLE('',#72330,7.44703751052387);
#16634=CIRCLE('',#72331,7.44703748822274);
#16635=CIRCLE('',#72332,7.44703753018844);
#16636=CIRCLE('',#72333,7.447037332229);
#16637=CIRCLE('',#72334,7.44703755755212);
#16638=CIRCLE('',#72335,7.44703741504868);
#16639=CIRCLE('',#72336,7.44703762292078);
#16640=CIRCLE('',#72337,7.44703724464123);
#16641=CIRCLE('',#72338,7.44703743114767);
#16642=CIRCLE('',#72339,7.44703751909643);
#16643=CIRCLE('',#72340,7.44703753083635);
#16644=CIRCLE('',#72341,7.44703745309058);
#16645=CIRCLE('',#72342,7.44703746637215);
#16646=CIRCLE('',#72343,7.44703740586822);
#16647=CIRCLE('',#72344,7.69059202594198);
#16648=CIRCLE('',#72346,7.69302856000655);
#16649=CIRCLE('',#72347,7.68765459426427);
#16650=CIRCLE('',#72348,7.690591902328);
#16651=CIRCLE('',#72350,7.69302885754567);
#16652=CIRCLE('',#72351,7.68765421623993);
#16653=CIRCLE('',#72352,7.69059185365515);
#16654=CIRCLE('',#72354,7.69302869987157);
#16655=CIRCLE('',#72355,7.68765427825275);
#16656=CIRCLE('',#72356,7.69059194180294);
#16657=CIRCLE('',#72358,7.69302857976961);
#16658=CIRCLE('',#72359,7.68765420205096);
#16659=CIRCLE('',#72360,7.6905918237196);
#16660=CIRCLE('',#72362,7.69302854134258);
#16661=CIRCLE('',#72363,7.6876542908369);
#16662=CIRCLE('',#72364,7.69059201504414);
#16663=CIRCLE('',#72366,7.69302868508283);
#16664=CIRCLE('',#72367,7.68765413714181);
#16665=CIRCLE('',#72368,7.69059207938841);
#16666=CIRCLE('',#72370,7.69302857487276);
#16667=CIRCLE('',#72371,7.68765447657531);
#16668=CIRCLE('',#72372,7.6905920405608);
#16669=CIRCLE('',#72374,7.69302857789015);
#16670=CIRCLE('',#72375,7.68765433942058);
#16671=CIRCLE('',#72376,7.69059201956098);
#16672=CIRCLE('',#72378,7.6930287518199);
#16673=CIRCLE('',#72379,7.68765455699274);
#16674=CIRCLE('',#72380,7.69059196034469);
#16675=CIRCLE('',#72382,7.69302872710911);
#16676=CIRCLE('',#72383,7.68765412359293);
#16677=CIRCLE('',#72384,7.69059185681044);
#16678=CIRCLE('',#72386,7.6930285949259);
#16679=CIRCLE('',#72387,7.68765432051234);
#16680=CIRCLE('',#72388,7.69059223732896);
#16681=CIRCLE('',#72390,7.69302871106017);
#16682=CIRCLE('',#72391,7.6876541532703);
#16683=CIRCLE('',#72392,7.69059211516317);
#16684=CIRCLE('',#72394,7.69302883712055);
#16685=CIRCLE('',#72395,7.68765415096754);
#16686=CIRCLE('',#72396,7.69059215704542);
#16687=CIRCLE('',#72398,7.69302855499968);
#16688=CIRCLE('',#72399,7.68765427356152);
#16689=CIRCLE('',#72400,7.69059175878684);
#16690=CIRCLE('',#72402,7.69302878492282);
#16691=CIRCLE('',#72403,7.68765435655919);
#16692=CIRCLE('',#72404,7.69059176654608);
#16693=CIRCLE('',#72406,7.69302889183546);
#16694=CIRCLE('',#72407,7.68765408745106);
#16695=CIRCLE('',#72408,7.69059179184688);
#16696=CIRCLE('',#72410,7.69302850426747);
#16697=CIRCLE('',#72411,7.68765433650955);
#16698=CIRCLE('',#72412,7.69059187920957);
#16699=CIRCLE('',#72414,7.693028786307);
#16700=CIRCLE('',#72415,7.6876544397187);
#16701=CIRCLE('',#72416,7.6905921275555);
#16702=CIRCLE('',#72418,7.69302875264593);
#16703=CIRCLE('',#72419,7.68765428237974);
#16704=CIRCLE('',#72420,7.69059171827927);
#16705=CIRCLE('',#72422,7.69302889434345);
#16706=CIRCLE('',#72423,7.6876540881813);
#16707=CIRCLE('',#72424,7.69059180948577);
#16708=CIRCLE('',#72426,7.69302862207645);
#16709=CIRCLE('',#72427,7.68765444403721);
#16710=CIRCLE('',#72428,7.69059184049164);
#16711=CIRCLE('',#72430,7.69302862547662);
#16712=CIRCLE('',#72431,7.68765415899986);
#16713=CIRCLE('',#72432,7.69059178595574);
#16714=CIRCLE('',#72433,7.69058741691256);
#16715=CIRCLE('',#72435,7.69302865324643);
#16716=CIRCLE('',#72436,7.68764993425013);
#16717=CIRCLE('',#72438,7.69059194581034);
#16718=CIRCLE('',#72439,7.69302855474821);
#16719=CIRCLE('',#72440,7.68765409297156);
#16720=CIRCLE('',#72442,7.69302853646235);
#16721=CIRCLE('',#72443,7.68765433980124);
#16722=CIRCLE('',#72444,7.6905920362682);
#16723=CIRCLE('',#72446,7.69302869406925);
#16724=CIRCLE('',#72447,7.6876542028167);
#16725=CIRCLE('',#72448,7.69059210092743);
#16726=CIRCLE('',#72450,7.69302875921919);
#16727=CIRCLE('',#72451,7.68765418549446);
#16728=CIRCLE('',#72452,7.69059192762103);
#16729=CIRCLE('',#72454,7.69302857768801);
#16730=CIRCLE('',#72455,7.68765422035337);
#16731=CIRCLE('',#72456,7.6895705373055);
#16732=CIRCLE('',#72457,7.68957071702817);
#16733=CIRCLE('',#72459,7.68318431078712);
#16734=CIRCLE('',#72460,7.68733814977416);
#16735=CIRCLE('',#72461,7.68957062858146);
#16736=CIRCLE('',#72463,7.68318471226888);
#16737=CIRCLE('',#72464,7.68733847129689);
#16738=CIRCLE('',#72465,7.68957064027973);
#16739=CIRCLE('',#72467,7.68318447973371);
#16740=CIRCLE('',#72468,7.68733822094465);
#16741=CIRCLE('',#72469,7.68957077150367);
#16742=CIRCLE('',#72471,7.68318420940126);
#16743=CIRCLE('',#72472,7.68733824007977);
#16744=CIRCLE('',#72473,7.6895707292031);
#16745=CIRCLE('',#72475,7.68318447990023);
#16746=CIRCLE('',#72476,7.68733833121305);
#16747=CIRCLE('',#72477,7.68957051214316);
#16748=CIRCLE('',#72479,7.68318398809391);
#16749=CIRCLE('',#72480,7.68733834665324);
#16750=CIRCLE('',#72481,7.68957088611825);
#16751=CIRCLE('',#72483,7.68318408620415);
#16752=CIRCLE('',#72484,7.68733822732077);
#16753=CIRCLE('',#72485,7.68957065040893);
#16754=CIRCLE('',#72487,7.68318452630675);
#16755=CIRCLE('',#72488,7.68733802736002);
#16756=CIRCLE('',#72489,7.68957094261063);
#16757=CIRCLE('',#72491,7.68318482090721);
#16758=CIRCLE('',#72492,7.68733816294838);
#16759=CIRCLE('',#72493,7.68957064665883);
#16760=CIRCLE('',#72495,7.68318426666719);
#16761=CIRCLE('',#72496,7.68733828478715);
#16762=CIRCLE('',#72497,7.68957074083717);
#16763=CIRCLE('',#72499,7.6831839731994);
#16764=CIRCLE('',#72500,7.68733823353924);
#16765=CIRCLE('',#72501,7.68957060360401);
#16766=CIRCLE('',#72503,7.68318443244907);
#16767=CIRCLE('',#72504,7.68733826168596);
#16768=CIRCLE('',#72505,7.68957074524144);
#16769=CIRCLE('',#72507,7.68318434353364);
#16770=CIRCLE('',#72508,7.68733841485494);
#16771=CIRCLE('',#72509,7.68957093395326);
#16772=CIRCLE('',#72511,7.68318462758714);
#16773=CIRCLE('',#72512,7.68733828523044);
#16774=CIRCLE('',#72513,7.68957078939204);
#16775=CIRCLE('',#72515,7.6831848112711);
#16776=CIRCLE('',#72516,7.68733844594019);
#16777=CIRCLE('',#72517,7.68957087822363);
#16778=CIRCLE('',#72519,7.68318425943269);
#16779=CIRCLE('',#72520,7.68733803337296);
#16780=CIRCLE('',#72521,7.68957040880922);
#16781=CIRCLE('',#72523,7.68318448193786);
#16782=CIRCLE('',#72524,7.68733838938515);
#16783=CIRCLE('',#72525,7.68957082558246);
#16784=CIRCLE('',#72527,7.68318409703543);
#16785=CIRCLE('',#72528,7.68733811369692);
#16786=CIRCLE('',#72529,7.68957078793141);
#16787=CIRCLE('',#72531,7.68318432153085);
#16788=CIRCLE('',#72532,7.6873382577664);
#16789=CIRCLE('',#72533,7.68957090366153);
#16790=CIRCLE('',#72535,7.68318447137218);
#16791=CIRCLE('',#72536,7.68733847367282);
#16792=CIRCLE('',#72537,7.68957060775697);
#16793=CIRCLE('',#72539,7.68318416167432);
#16794=CIRCLE('',#72540,7.68733827550981);
#16795=CIRCLE('',#72541,7.68957085438422);
#16796=CIRCLE('',#72543,7.68318476711715);
#16797=CIRCLE('',#72544,7.68733832707878);
#16798=CIRCLE('',#72545,7.68957080161283);
#16799=CIRCLE('',#72547,7.6831845569757);
#16800=CIRCLE('',#72548,7.68733833084729);
#16801=CIRCLE('',#72549,7.68957079004739);
#16802=CIRCLE('',#72551,7.68318419339156);
#16803=CIRCLE('',#72552,7.68733810715353);
#16804=CIRCLE('',#72553,7.68957079118119);
#16805=CIRCLE('',#72555,7.6831845910336);
#16806=CIRCLE('',#72556,7.68733835573841);
#16807=CIRCLE('',#72557,7.68957083928288);
#16808=CIRCLE('',#72559,7.68318437103514);
#16809=CIRCLE('',#72560,7.68733808432302);
#16810=CIRCLE('',#72561,7.68957083624163);
#16811=CIRCLE('',#72563,7.6831840524939);
#16812=CIRCLE('',#72564,7.68733811585128);
#16813=CIRCLE('',#72566,7.68318490909919);
#16814=CIRCLE('',#72567,7.68733853056307);
#16815=CIRCLE('',#72568,7.44531538645819);
#16816=CIRCLE('',#72569,7.44956381440597);
#16817=CIRCLE('',#72570,7.44531525600097);
#16818=CIRCLE('',#72571,7.44956398909259);
#16819=CIRCLE('',#72572,7.44531519228589);
#16820=CIRCLE('',#72573,7.44956390637326);
#16821=CIRCLE('',#72574,7.44531530198313);
#16822=CIRCLE('',#72575,7.44956382734727);
#16823=CIRCLE('',#72576,7.44531538463241);
#16824=CIRCLE('',#72577,7.44956422045783);
#16825=CIRCLE('',#72578,7.44531524460531);
#16826=CIRCLE('',#72579,7.44956402238707);
#16827=CIRCLE('',#72580,7.44531535871156);
#16828=CIRCLE('',#72581,7.44956416166019);
#16829=CIRCLE('',#72582,7.44531527750566);
#16830=CIRCLE('',#72583,7.44956389304393);
#16831=CIRCLE('',#72584,7.44531529542168);
#16832=CIRCLE('',#72585,7.44956413304856);
#16833=CIRCLE('',#72586,7.4453153154805);
#16834=CIRCLE('',#72587,7.44956385182501);
#16835=CIRCLE('',#72588,7.44531529811139);
#16836=CIRCLE('',#72589,7.44956399165328);
#16837=CIRCLE('',#72590,7.44531535591968);
#16838=CIRCLE('',#72591,7.44956417940239);
#16839=CIRCLE('',#72592,7.44531536039092);
#16840=CIRCLE('',#72593,7.44956417574995);
#16841=CIRCLE('',#72594,7.44531533180438);
#16842=CIRCLE('',#72595,7.44956398258933);
#16843=CIRCLE('',#72596,7.44531507760606);
#16844=CIRCLE('',#72597,7.44956411333289);
#16845=CIRCLE('',#72598,7.44531530812124);
#16846=CIRCLE('',#72599,7.44956391452336);
#16847=CIRCLE('',#72600,7.44531533056805);
#16848=CIRCLE('',#72601,7.44956401906169);
#16849=CIRCLE('',#72602,7.44531538142944);
#16850=CIRCLE('',#72603,7.44956393089749);
#16851=CIRCLE('',#72604,7.44531515711117);
#16852=CIRCLE('',#72605,7.4495640374712);
#16853=CIRCLE('',#72606,7.44531526111994);
#16854=CIRCLE('',#72607,7.4495638253791);
#16855=CIRCLE('',#72608,7.44531512832504);
#16856=CIRCLE('',#72609,7.4495640357743);
#16857=CIRCLE('',#72610,7.44531536062869);
#16858=CIRCLE('',#72611,7.44956414197099);
#16859=CIRCLE('',#72612,7.44531540976715);
#16860=CIRCLE('',#72613,7.4495640397269);
#16861=CIRCLE('',#72614,7.44531524242191);
#16862=CIRCLE('',#72615,7.44956409048664);
#16863=CIRCLE('',#72616,7.44531544260196);
#16864=CIRCLE('',#72617,7.44956396224621);
#16865=CIRCLE('',#72618,7.44531525344054);
#16866=CIRCLE('',#72619,7.4495639253832);
#16867=CIRCLE('',#72620,7.44531531942668);
#16868=CIRCLE('',#72621,7.44956384698854);
#16869=CIRCLE('',#72622,7.44531551160301);
#16870=CIRCLE('',#72623,7.4495640070332);
#16871=CIRCLE('',#72624,7.44531539934746);
#16872=CIRCLE('',#72625,7.44956388528947);
#16873=CIRCLE('',#72626,7.44501798128672);
#16874=CIRCLE('',#72627,7.44501863613543);
#16875=CIRCLE('',#72628,7.44501880349459);
#16876=CIRCLE('',#72629,7.44501892336087);
#16877=CIRCLE('',#72630,7.44501873113526);
#16878=CIRCLE('',#72631,7.44501877734031);
#16879=CIRCLE('',#72632,7.44501879135829);
#16880=CIRCLE('',#72633,7.44501889805359);
#16881=CIRCLE('',#72634,7.44501868281248);
#16882=CIRCLE('',#72635,7.44501877144378);
#16883=CIRCLE('',#72636,7.4450186464062);
#16884=CIRCLE('',#72637,7.44501897930043);
#16885=CIRCLE('',#72638,7.44501872350213);
#16886=CIRCLE('',#72639,7.44501872218195);
#16887=CIRCLE('',#72640,7.4450187414317);
#16888=CIRCLE('',#72641,7.44501896740992);
#16889=CIRCLE('',#72642,7.4450189666943);
#16890=CIRCLE('',#72643,7.44501886990939);
#16891=CIRCLE('',#72644,7.44501870710545);
#16892=CIRCLE('',#72645,7.44501889130117);
#16893=CIRCLE('',#72646,7.44501895300577);
#16894=CIRCLE('',#72647,7.44501885439827);
#16895=CIRCLE('',#72648,7.44501873231066);
#16896=CIRCLE('',#72649,7.44501863965835);
#16897=CIRCLE('',#72650,7.44501881787528);
#16898=CIRCLE('',#72651,7.44501870219928);
#16899=CIRCLE('',#72652,7.44501879756191);
#16900=CIRCLE('',#72653,7.44501886683483);
#16901=CIRCLE('',#72654,7.44501879564492);
#16902=CIRCLE('',#72655,7.68994768850121);
#16903=CIRCLE('',#72657,7.69081639039695);
#16904=CIRCLE('',#72658,7.69287902948567);
#16905=CIRCLE('',#72659,7.69291183764604);
#16906=CIRCLE('',#72660,7.68994776176434);
#16907=CIRCLE('',#72662,7.69081629816903);
#16908=CIRCLE('',#72663,7.69287925074);
#16909=CIRCLE('',#72664,7.69291180931347);
#16910=CIRCLE('',#72665,7.68994806307652);
#16911=CIRCLE('',#72667,7.69081625244724);
#16912=CIRCLE('',#72668,7.69287912011643);
#16913=CIRCLE('',#72669,7.69291162670421);
#16914=CIRCLE('',#72670,7.68994782425453);
#16915=CIRCLE('',#72672,7.69081622752238);
#16916=CIRCLE('',#72673,7.69287914100277);
#16917=CIRCLE('',#72674,7.69291174121858);
#16918=CIRCLE('',#72675,7.68994775281266);
#16919=CIRCLE('',#72677,7.69081618799205);
#16920=CIRCLE('',#72678,7.69287921910763);
#16921=CIRCLE('',#72679,7.69291197483402);
#16922=CIRCLE('',#72680,7.68994784764813);
#16923=CIRCLE('',#72682,7.69081625930234);
#16924=CIRCLE('',#72683,7.69287933505147);
#16925=CIRCLE('',#72684,7.69291183628208);
#16926=CIRCLE('',#72685,7.68994802235942);
#16927=CIRCLE('',#72687,7.69081615857865);
#16928=CIRCLE('',#72688,7.69287899879009);
#16929=CIRCLE('',#72689,7.6929120432216);
#16930=CIRCLE('',#72690,7.68994799837717);
#16931=CIRCLE('',#72692,7.69081639968424);
#16932=CIRCLE('',#72693,7.69287918394263);
#16933=CIRCLE('',#72694,7.6929117833322);
#16934=CIRCLE('',#72695,7.68994777527193);
#16935=CIRCLE('',#72697,7.69081626579946);
#16936=CIRCLE('',#72698,7.69287911479038);
#16937=CIRCLE('',#72699,7.69291190741967);
#16938=CIRCLE('',#72700,7.68994779714343);
#16939=CIRCLE('',#72702,7.69081618537138);
#16940=CIRCLE('',#72703,7.6928790186626);
#16941=CIRCLE('',#72704,7.69291195486959);
#16942=CIRCLE('',#72705,7.68994785743113);
#16943=CIRCLE('',#72707,7.69081617604151);
#16944=CIRCLE('',#72708,7.69287923229911);
#16945=CIRCLE('',#72709,7.69291180726217);
#16946=CIRCLE('',#72710,7.68994800537629);
#16947=CIRCLE('',#72712,7.69081643790944);
#16948=CIRCLE('',#72713,7.69287902700114);
#16949=CIRCLE('',#72714,7.69291175642132);
#16950=CIRCLE('',#72715,7.68994796871448);
#16951=CIRCLE('',#72717,7.6908163194903);
#16952=CIRCLE('',#72718,7.69287910534962);
#16953=CIRCLE('',#72719,7.69291202082806);
#16954=CIRCLE('',#72720,7.6899475970862);
#16955=CIRCLE('',#72722,7.6908162053019);
#16956=CIRCLE('',#72723,7.69287915730047);
#16957=CIRCLE('',#72724,7.6929118912537);
#16958=CIRCLE('',#72725,7.68994797437207);
#16959=CIRCLE('',#72727,7.69081636705849);
#16960=CIRCLE('',#72728,7.69287910182044);
#16961=CIRCLE('',#72729,7.69291196007138);
#16962=CIRCLE('',#72730,7.68994782657826);
#16963=CIRCLE('',#72732,7.69081638893993);
#16964=CIRCLE('',#72733,7.69287899177703);
#16965=CIRCLE('',#72734,7.69291176261553);
#16966=CIRCLE('',#72735,7.68994785039263);
#16967=CIRCLE('',#72737,7.69081631363439);
#16968=CIRCLE('',#72738,7.69287915934317);
#16969=CIRCLE('',#72739,7.69291185563463);
#16970=CIRCLE('',#72740,7.68994792779107);
#16971=CIRCLE('',#72742,7.69081611198666);
#16972=CIRCLE('',#72743,7.69287945730006);
#16973=CIRCLE('',#72744,7.69291174915492);
#16974=CIRCLE('',#72745,7.68994765651948);
#16975=CIRCLE('',#72747,7.69081620155709);
#16976=CIRCLE('',#72748,7.6928789712968);
#16977=CIRCLE('',#72749,7.69291165495841);
#16978=CIRCLE('',#72750,7.68994793766104);
#16979=CIRCLE('',#72752,7.69081648538269);
#16980=CIRCLE('',#72753,7.69287935101016);
#16981=CIRCLE('',#72754,7.69291211427012);
#16982=CIRCLE('',#72755,7.68994783081566);
#16983=CIRCLE('',#72757,7.69081631618511);
#16984=CIRCLE('',#72758,7.69287917491714);
#16985=CIRCLE('',#72759,7.69291179086216);
#16986=CIRCLE('',#72760,7.68994762249597);
#16987=CIRCLE('',#72762,7.69081615538454);
#16988=CIRCLE('',#72763,7.69287928734082);
#16989=CIRCLE('',#72764,7.69291165110122);
#16990=CIRCLE('',#72765,7.68994789648978);
#16991=CIRCLE('',#72766,7.69291192595375);
#16992=CIRCLE('',#72768,7.69081620706134);
#16993=CIRCLE('',#72769,7.69287911855576);
#16994=CIRCLE('',#72770,7.68994789980955);
#16995=CIRCLE('',#72772,7.69291164285274);
#16996=CIRCLE('',#72773,7.69081624184935);
#16997=CIRCLE('',#72774,7.69287898118367);
#16998=CIRCLE('',#72775,7.68994800192127);
#16999=CIRCLE('',#72777,7.69081618985827);
#17000=CIRCLE('',#72778,7.69287932799914);
#17001=CIRCLE('',#72779,7.69291178900987);
#17002=CIRCLE('',#72780,7.68994793193109);
#17003=CIRCLE('',#72782,7.69081608773444);
#17004=CIRCLE('',#72783,7.69287910901963);
#17005=CIRCLE('',#72784,7.69291193953742);
#17006=CIRCLE('',#72785,7.68994804678886);
#17007=CIRCLE('',#72787,7.69081606230325);
#17008=CIRCLE('',#72788,7.69287916191094);
#17009=CIRCLE('',#72789,7.69291176352222);
#17010=CIRCLE('',#72790,7.6899477324061);
#17011=CIRCLE('',#72792,7.6908160448308);
#17012=CIRCLE('',#72793,7.69287928896208);
#17013=CIRCLE('',#72794,7.69291178964863);
#17014=CIRCLE('',#72795,7.68969379605931);
#17015=CIRCLE('',#72797,7.68635993537705);
#17016=CIRCLE('',#72798,7.69279340224594);
#17017=CIRCLE('',#72799,7.68969366433993);
#17018=CIRCLE('',#72801,7.68635964596802);
#17019=CIRCLE('',#72802,7.69279317570462);
#17020=CIRCLE('',#72803,7.68969389957442);
#17021=CIRCLE('',#72805,7.68636012101837);
#17022=CIRCLE('',#72806,7.69279321981756);
#17023=CIRCLE('',#72807,7.68969357082102);
#17024=CIRCLE('',#72809,7.68635971152984);
#17025=CIRCLE('',#72810,7.69279330277333);
#17026=CIRCLE('',#72811,7.68969356005781);
#17027=CIRCLE('',#72813,7.68635984569196);
#17028=CIRCLE('',#72814,7.69279339299752);
#17029=CIRCLE('',#72815,7.68969378432535);
#17030=CIRCLE('',#72817,7.68636009876598);
#17031=CIRCLE('',#72818,7.69279319574932);
#17032=CIRCLE('',#72819,7.68969354635827);
#17033=CIRCLE('',#72821,7.68635984983445);
#17034=CIRCLE('',#72822,7.69279329838833);
#17035=CIRCLE('',#72823,7.68969384772044);
#17036=CIRCLE('',#72825,7.68635987722991);
#17037=CIRCLE('',#72826,7.69279306777004);
#17038=CIRCLE('',#72827,7.68969379587333);
#17039=CIRCLE('',#72829,7.68636009200399);
#17040=CIRCLE('',#72830,7.69279307273185);
#17041=CIRCLE('',#72831,7.68969360005298);
#17042=CIRCLE('',#72833,7.68636010647129);
#17043=CIRCLE('',#72834,7.69279313806582);
#17044=CIRCLE('',#72835,7.68969367951995);
#17045=CIRCLE('',#72837,7.6863598904456);
#17046=CIRCLE('',#72838,7.69279352359976);
#17047=CIRCLE('',#72839,7.68969372147397);
#17048=CIRCLE('',#72841,7.68635974611356);
#17049=CIRCLE('',#72842,7.69279344881826);
#17050=CIRCLE('',#72843,7.68969343633667);
#17051=CIRCLE('',#72845,7.68635971737299);
#17052=CIRCLE('',#72846,7.69279338068447);
#17053=CIRCLE('',#72847,7.68969375791827);
#17054=CIRCLE('',#72849,7.68635998328794);
#17055=CIRCLE('',#72850,7.69279332422182);
#17056=CIRCLE('',#72851,7.68969363714325);
#17057=CIRCLE('',#72853,7.68635991849997);
#17058=CIRCLE('',#72854,7.69279311575017);
#17059=CIRCLE('',#72855,7.68969369394559);
#17060=CIRCLE('',#72857,7.68635983689677);
#17061=CIRCLE('',#72858,7.69279334009542);
#17062=CIRCLE('',#72859,7.68969364964678);
#17063=CIRCLE('',#72861,7.68636005130882);
#17064=CIRCLE('',#72862,7.69279299577899);
#17065=CIRCLE('',#72863,7.68969389920012);
#17066=CIRCLE('',#72865,7.68635990825161);
#17067=CIRCLE('',#72866,7.69279308680408);
#17068=CIRCLE('',#72867,7.68969379341059);
#17069=CIRCLE('',#72869,7.6863602299655);
#17070=CIRCLE('',#72870,7.69279310613291);
#17071=CIRCLE('',#72871,7.68969380669233);
#17072=CIRCLE('',#72873,7.68635982548127);
#17073=CIRCLE('',#72874,7.69279340053383);
#17074=CIRCLE('',#72875,7.68969366719949);
#17075=CIRCLE('',#72877,7.68636003695748);
#17076=CIRCLE('',#72878,7.69279333592378);
#17077=CIRCLE('',#72879,7.68969377855696);
#17078=CIRCLE('',#72881,7.68635979155829);
#17079=CIRCLE('',#72882,7.69279341300475);
#17080=CIRCLE('',#72883,7.6896937574551);
#17081=CIRCLE('',#72885,7.68635978467662);
#17082=CIRCLE('',#72886,7.69279336051956);
#17083=CIRCLE('',#72887,7.68969364519625);
#17084=CIRCLE('',#72889,7.68636002417854);
#17085=CIRCLE('',#72890,7.69279335544202);
#17086=CIRCLE('',#72891,7.68969359825938);
#17087=CIRCLE('',#72893,7.68635983159926);
#17088=CIRCLE('',#72894,7.6927933468798);
#17089=CIRCLE('',#72895,7.6896938024155);
#17090=CIRCLE('',#72897,7.68635976539525);
#17091=CIRCLE('',#72898,7.69279326968129);
#17092=CIRCLE('',#72899,7.68969370355732);
#17093=CIRCLE('',#72901,7.68635995743284);
#17094=CIRCLE('',#72902,7.69279303053349);
#17095=CIRCLE('',#72903,7.68969378343039);
#17096=CIRCLE('',#72905,7.68635996847948);
#17097=CIRCLE('',#72906,7.69279317991971);
#17098=CIRCLE('',#72907,7.68969357197823);
#17099=CIRCLE('',#72909,7.68635979354931);
#17100=CIRCLE('',#72910,7.69279316452614);
#17101=CIRCLE('',#72911,7.44636423010508);
#17102=CIRCLE('',#72912,7.44966325127302);
#17103=CIRCLE('',#72913,7.44636174860661);
#17104=CIRCLE('',#72914,7.44966347089591);
#17105=CIRCLE('',#72915,7.44636178384942);
#17106=CIRCLE('',#72916,7.44966309407636);
#17107=CIRCLE('',#72917,7.44636204559121);
#17108=CIRCLE('',#72918,7.44966335654733);
#17109=CIRCLE('',#72919,7.44636182606712);
#17110=CIRCLE('',#72920,7.44966321797586);
#17111=CIRCLE('',#72921,7.44636193742149);
#17112=CIRCLE('',#72922,7.44966341877709);
#17113=CIRCLE('',#72923,7.44636206094047);
#17114=CIRCLE('',#72924,7.44966325286485);
#17115=CIRCLE('',#72925,7.44636219915386);
#17116=CIRCLE('',#72926,7.44966336557642);
#17117=CIRCLE('',#72927,7.44636210971655);
#17118=CIRCLE('',#72928,7.44966331459993);
#17119=CIRCLE('',#72929,7.44636197667186);
#17120=CIRCLE('',#72930,7.44966326236817);
#17121=CIRCLE('',#72931,7.44636419295865);
#17122=CIRCLE('',#72932,7.44966326944475);
#17123=CIRCLE('',#72933,7.44636186285971);
#17124=CIRCLE('',#72934,7.44966299354956);
#17125=CIRCLE('',#72935,7.44636184648999);
#17126=CIRCLE('',#72936,7.44966329395538);
#17127=CIRCLE('',#72937,7.44636192502926);
#17128=CIRCLE('',#72938,7.44966318204452);
#17129=CIRCLE('',#72939,7.44636171142564);
#17130=CIRCLE('',#72940,7.44966578527346);
#17131=CIRCLE('',#72941,7.44636197765164);
#17132=CIRCLE('',#72942,7.44966334625654);
#17133=CIRCLE('',#72943,7.44636191277442);
#17134=CIRCLE('',#72944,7.44966307490312);
#17135=CIRCLE('',#72945,7.44636200455071);
#17136=CIRCLE('',#72946,7.44966321197009);
#17137=CIRCLE('',#72947,7.44636215724628);
#17138=CIRCLE('',#72948,7.44966318966319);
#17139=CIRCLE('',#72949,7.44636196988074);
#17140=CIRCLE('',#72950,7.44966570382605);
#17141=CIRCLE('',#72951,7.44636166648058);
#17142=CIRCLE('',#72952,7.44966574550693);
#17143=CIRCLE('',#72953,7.44636197685232);
#17144=CIRCLE('',#72954,7.4496631366682);
#17145=CIRCLE('',#72955,7.44636196485188);
#17146=CIRCLE('',#72956,7.44966328724103);
#17147=CIRCLE('',#72957,7.44636196252542);
#17148=CIRCLE('',#72958,7.44966333924468);
#17149=CIRCLE('',#72959,7.44636191238592);
#17150=CIRCLE('',#72960,7.44966333026025);
#17151=CIRCLE('',#72961,7.44636200075493);
#17152=CIRCLE('',#72962,7.44966320020436);
#17153=CIRCLE('',#72963,7.44636202472126);
#17154=CIRCLE('',#72964,7.44966584986547);
#17155=CIRCLE('',#72965,7.44636193257106);
#17156=CIRCLE('',#72966,7.44966353760313);
#17157=CIRCLE('',#72967,7.44636196148033);
#17158=CIRCLE('',#72968,7.44966316450105);
#17159=CIRCLE('',#72969,7.44412064297541);
#17160=CIRCLE('',#72970,7.44962090241967);
#17161=CIRCLE('',#72971,7.4441215350551);
#17162=CIRCLE('',#72972,7.44962092331308);
#17163=CIRCLE('',#72973,7.44412171359309);
#17164=CIRCLE('',#72974,7.44962088978136);
#17165=CIRCLE('',#72975,7.44412165693904);
#17166=CIRCLE('',#72976,7.44962101012671);
#17167=CIRCLE('',#72977,7.4441216951693);
#17168=CIRCLE('',#72978,7.44962106412852);
#17169=CIRCLE('',#72979,7.44412170714691);
#17170=CIRCLE('',#72980,7.44962091777948);
#17171=CIRCLE('',#72981,7.44412154598296);
#17172=CIRCLE('',#72982,7.44962075048608);
#17173=CIRCLE('',#72983,7.44412169947591);
#17174=CIRCLE('',#72984,7.44962100045847);
#17175=CIRCLE('',#72985,7.44412167599847);
#17176=CIRCLE('',#72986,7.44962064288898);
#17177=CIRCLE('',#72987,7.44412165364346);
#17178=CIRCLE('',#72988,7.44962107754941);
#17179=CIRCLE('',#72989,7.44412166787335);
#17180=CIRCLE('',#72990,7.44962103513019);
#17181=CIRCLE('',#72991,7.44412183980246);
#17182=CIRCLE('',#72992,7.44962107444732);
#17183=CIRCLE('',#72993,7.44412153534108);
#17184=CIRCLE('',#72994,7.44962093878989);
#17185=CIRCLE('',#72995,7.44412162026275);
#17186=CIRCLE('',#72996,7.44962091020999);
#17187=CIRCLE('',#72997,7.44412164711026);
#17188=CIRCLE('',#72998,7.44962099065294);
#17189=CIRCLE('',#72999,7.44412173822533);
#17190=CIRCLE('',#73000,7.44962082298734);
#17191=CIRCLE('',#73001,7.44412191483093);
#17192=CIRCLE('',#73002,7.44962083948565);
#17193=CIRCLE('',#73003,7.44412154563418);
#17194=CIRCLE('',#73004,7.44962079753425);
#17195=CIRCLE('',#73005,7.44412180227944);
#17196=CIRCLE('',#73006,7.44962074392226);
#17197=CIRCLE('',#73007,7.4441217413041);
#17198=CIRCLE('',#73008,7.44962098648014);
#17199=CIRCLE('',#73009,7.4441217944993);
#17200=CIRCLE('',#73010,7.44962123096037);
#17201=CIRCLE('',#73011,7.44412161325592);
#17202=CIRCLE('',#73012,7.44962082725039);
#17203=CIRCLE('',#73013,7.44412158112357);
#17204=CIRCLE('',#73014,7.44962082581323);
#17205=CIRCLE('',#73015,7.44412158351607);
#17206=CIRCLE('',#73016,7.44962097025443);
#17207=CIRCLE('',#73017,7.44412174516809);
#17208=CIRCLE('',#73018,7.449620984779);
#17209=CIRCLE('',#73019,7.44412175042324);
#17210=CIRCLE('',#73020,7.44962076526355);
#17211=CIRCLE('',#73021,7.44412154988149);
#17212=CIRCLE('',#73022,7.44962082790196);
#17213=CIRCLE('',#73023,7.44412180935468);
#17214=CIRCLE('',#73024,7.44962098873196);
#17215=CIRCLE('',#73025,7.44412180009209);
#17216=CIRCLE('',#73026,7.44962076564967);
#17217=CIRCLE('',#73027,7.68881312209984);
#17218=CIRCLE('',#73028,7.69305842670495);
#17219=CIRCLE('',#73030,7.69135459595439);
#17220=CIRCLE('',#73031,7.68881305425059);
#17221=CIRCLE('',#73032,7.69305851563742);
#17222=CIRCLE('',#73034,7.69135469458866);
#17223=CIRCLE('',#73035,7.68881318241118);
#17224=CIRCLE('',#73036,7.69305837521999);
#17225=CIRCLE('',#73038,7.6913545638551);
#17226=CIRCLE('',#73039,7.68881306332511);
#17227=CIRCLE('',#73040,7.69305860510658);
#17228=CIRCLE('',#73042,7.69135444682733);
#17229=CIRCLE('',#73043,7.6888132919626);
#17230=CIRCLE('',#73044,7.69305837123098);
#17231=CIRCLE('',#73046,7.6913547963529);
#17232=CIRCLE('',#73047,7.68881303446479);
#17233=CIRCLE('',#73048,7.69305857205603);
#17234=CIRCLE('',#73050,7.69135467139072);
#17235=CIRCLE('',#73051,7.68881305751141);
#17236=CIRCLE('',#73052,7.6930583711798);
#17237=CIRCLE('',#73054,7.6913546819479);
#17238=CIRCLE('',#73055,7.68881287342277);
#17239=CIRCLE('',#73056,7.69305844639685);
#17240=CIRCLE('',#73058,7.691354832468);
#17241=CIRCLE('',#73059,7.68881313161581);
#17242=CIRCLE('',#73060,7.69305848534483);
#17243=CIRCLE('',#73062,7.69135483048795);
#17244=CIRCLE('',#73063,7.68881313584477);
#17245=CIRCLE('',#73064,7.69305850720062);
#17246=CIRCLE('',#73066,7.69135459145652);
#17247=CIRCLE('',#73067,7.68881274573051);
#17248=CIRCLE('',#73068,7.69305864966813);
#17249=CIRCLE('',#73070,7.69135463961226);
#17250=CIRCLE('',#73071,7.68881325189327);
#17251=CIRCLE('',#73072,7.69305821213215);
#17252=CIRCLE('',#73074,7.69135477789806);
#17253=CIRCLE('',#73075,7.68881285340086);
#17254=CIRCLE('',#73076,7.69305846026459);
#17255=CIRCLE('',#73078,7.69135472284591);
#17256=CIRCLE('',#73079,7.68881300396549);
#17257=CIRCLE('',#73080,7.69305817498246);
#17258=CIRCLE('',#73082,7.69135445363307);
#17259=CIRCLE('',#73083,7.68881275452915);
#17260=CIRCLE('',#73084,7.69305861452194);
#17261=CIRCLE('',#73086,7.69135457467286);
#17262=CIRCLE('',#73087,7.68881303796674);
#17263=CIRCLE('',#73088,7.69305858517097);
#17264=CIRCLE('',#73090,7.69135473804609);
#17265=CIRCLE('',#73091,7.68881291061956);
#17266=CIRCLE('',#73092,7.69305851660632);
#17267=CIRCLE('',#73094,7.69135491750274);
#17268=CIRCLE('',#73095,7.68881294783481);
#17269=CIRCLE('',#73096,7.69305865774133);
#17270=CIRCLE('',#73098,7.69135446595735);
#17271=CIRCLE('',#73099,7.68881286359618);
#17272=CIRCLE('',#73100,7.69305865167506);
#17273=CIRCLE('',#73102,7.69135477608768);
#17274=CIRCLE('',#73103,7.6888131570718);
#17275=CIRCLE('',#73104,7.69305841221193);
#17276=CIRCLE('',#73106,7.69135474309799);
#17277=CIRCLE('',#73107,7.68881310973368);
#17278=CIRCLE('',#73108,7.693058486018);
#17279=CIRCLE('',#73110,7.69135458482537);
#17280=CIRCLE('',#73111,7.68881304034411);
#17281=CIRCLE('',#73112,7.69305845743024);
#17282=CIRCLE('',#73113,7.68880897371152);
#17283=CIRCLE('',#73115,7.69135060068296);
#17284=CIRCLE('',#73116,7.69305863217014);
#17285=CIRCLE('',#73118,7.68881291601433);
#17286=CIRCLE('',#73119,7.69135469952759);
#17287=CIRCLE('',#73120,7.6930583361325);
#17288=CIRCLE('',#73122,7.69135444944665);
#17289=CIRCLE('',#73123,7.68881281368828);
#17290=CIRCLE('',#73124,7.69305827499903);
#17291=CIRCLE('',#73126,7.69135481642152);
#17292=CIRCLE('',#73127,7.68881286880164);
#17293=CIRCLE('',#73128,7.69305845317125);
#17294=CIRCLE('',#73130,7.69135474107584);
#17295=CIRCLE('',#73131,7.68881279052987);
#17296=CIRCLE('',#73132,7.69305840144874);
#17297=CIRCLE('',#73134,7.69135464328283);
#17298=CIRCLE('',#73135,7.68881294976904);
#17299=CIRCLE('',#73137,7.69135478455158);
#17300=CIRCLE('',#73138,7.6930585711826);
#17301=CIRCLE('',#73139,7.68894221452859);
#17302=CIRCLE('',#73140,7.69306082816528);
#17303=CIRCLE('',#73141,7.68894221816495);
#17304=CIRCLE('',#73143,7.69254652221787);
#17305=CIRCLE('',#73144,7.69154668134093);
#17306=CIRCLE('',#73145,7.69306103162729);
#17307=CIRCLE('',#73146,7.6889420578582);
#17308=CIRCLE('',#73148,7.69254632751691);
#17309=CIRCLE('',#73149,7.69154676522241);
#17310=CIRCLE('',#73150,7.69306084786072);
#17311=CIRCLE('',#73151,7.68894212344255);
#17312=CIRCLE('',#73153,7.69254629177713);
#17313=CIRCLE('',#73154,7.69154659721445);
#17314=CIRCLE('',#73155,7.69306125634641);
#17315=CIRCLE('',#73156,7.68894230414718);
#17316=CIRCLE('',#73158,7.69254630396056);
#17317=CIRCLE('',#73159,7.69154657372904);
#17318=CIRCLE('',#73160,7.6930610465379);
#17319=CIRCLE('',#73161,7.68894215940438);
#17320=CIRCLE('',#73163,7.69254651455718);
#17321=CIRCLE('',#73164,7.69154664597915);
#17322=CIRCLE('',#73165,7.6930611839578);
#17323=CIRCLE('',#73166,7.68894243281189);
#17324=CIRCLE('',#73168,7.69254635990402);
#17325=CIRCLE('',#73169,7.69154701073923);
#17326=CIRCLE('',#73170,7.69306102466985);
#17327=CIRCLE('',#73171,7.68894235114808);
#17328=CIRCLE('',#73173,7.69254624235975);
#17329=CIRCLE('',#73174,7.69154685393794);
#17330=CIRCLE('',#73175,7.69306122370397);
#17331=CIRCLE('',#73176,7.68894225719054);
#17332=CIRCLE('',#73178,7.69254660064401);
#17333=CIRCLE('',#73179,7.69154666639614);
#17334=CIRCLE('',#73180,7.69306112112687);
#17335=CIRCLE('',#73181,7.68894206668824);
#17336=CIRCLE('',#73183,7.69254659939187);
#17337=CIRCLE('',#73184,7.69154686958469);
#17338=CIRCLE('',#73185,7.69306098589994);
#17339=CIRCLE('',#73186,7.68894212480211);
#17340=CIRCLE('',#73188,7.69254664269419);
#17341=CIRCLE('',#73189,7.6915468406462);
#17342=CIRCLE('',#73190,7.69306087910567);
#17343=CIRCLE('',#73191,7.68894223701859);
#17344=CIRCLE('',#73193,7.6925462252469);
#17345=CIRCLE('',#73194,7.69154650914596);
#17346=CIRCLE('',#73195,7.6930609492561);
#17347=CIRCLE('',#73196,7.68894231759131);
#17348=CIRCLE('',#73198,7.69254645363533);
#17349=CIRCLE('',#73199,7.69154672029993);
#17350=CIRCLE('',#73200,7.69306078197452);
#17351=CIRCLE('',#73201,7.68894223814822);
#17352=CIRCLE('',#73203,7.69254661875416);
#17353=CIRCLE('',#73204,7.69154666835679);
#17354=CIRCLE('',#73205,7.69306108280045);
#17355=CIRCLE('',#73206,7.68894225175114);
#17356=CIRCLE('',#73208,7.69254659523722);
#17357=CIRCLE('',#73209,7.69154671923709);
#17358=CIRCLE('',#73210,7.69306124540043);
#17359=CIRCLE('',#73211,7.68894227989443);
#17360=CIRCLE('',#73213,7.69254654866584);
#17361=CIRCLE('',#73214,7.69154673015789);
#17362=CIRCLE('',#73215,7.69306085198288);
#17363=CIRCLE('',#73216,7.68894237178344);
#17364=CIRCLE('',#73218,7.69254635163619);
#17365=CIRCLE('',#73219,7.69154667037883);
#17366=CIRCLE('',#73220,7.6930607036298);
#17367=CIRCLE('',#73221,7.68894226104312);
#17368=CIRCLE('',#73223,7.6925464256185);
#17369=CIRCLE('',#73224,7.69154653529051);
#17370=CIRCLE('',#73225,7.69306131397639);
#17371=CIRCLE('',#73226,7.68894236076532);
#17372=CIRCLE('',#73228,7.69254629704884);
#17373=CIRCLE('',#73229,7.69154704329205);
#17374=CIRCLE('',#73230,7.69306084621818);
#17375=CIRCLE('',#73231,7.68894221484235);
#17376=CIRCLE('',#73233,7.69254616738453);
#17377=CIRCLE('',#73234,7.69154684700041);
#17378=CIRCLE('',#73235,7.69306089555524);
#17379=CIRCLE('',#73236,7.68894233735332);
#17380=CIRCLE('',#73238,7.69254632399395);
#17381=CIRCLE('',#73239,7.69154679094549);
#17382=CIRCLE('',#73240,7.69306100859483);
#17383=CIRCLE('',#73241,7.688942330024);
#17384=CIRCLE('',#73243,7.69254642332663);
#17385=CIRCLE('',#73244,7.69154660688702);
#17386=CIRCLE('',#73245,7.69306118917124);
#17387=CIRCLE('',#73246,7.68894225546997);
#17388=CIRCLE('',#73248,7.69254635523657);
#17389=CIRCLE('',#73249,7.69154694744465);
#17390=CIRCLE('',#73250,7.69306111921035);
#17391=CIRCLE('',#73251,7.68894236019955);
#17392=CIRCLE('',#73253,7.69254652854155);
#17393=CIRCLE('',#73254,7.69154674961277);
#17394=CIRCLE('',#73255,7.69306115184591);
#17395=CIRCLE('',#73256,7.68894222237977);
#17396=CIRCLE('',#73258,7.69254640727368);
#17397=CIRCLE('',#73259,7.69154705511724);
#17398=CIRCLE('',#73260,7.69306111025);
#17399=CIRCLE('',#73261,7.68894239205181);
#17400=CIRCLE('',#73263,7.69254643702591);
#17401=CIRCLE('',#73264,7.69154660575477);
#17402=CIRCLE('',#73265,7.6930610882171);
#17403=CIRCLE('',#73266,7.68894240872928);
#17404=CIRCLE('',#73268,7.69254646618558);
#17405=CIRCLE('',#73269,7.69154672452396);
#17406=CIRCLE('',#73270,7.69306091823566);
#17407=CIRCLE('',#73271,7.68894250390556);
#17408=CIRCLE('',#73273,7.69254667871653);
#17409=CIRCLE('',#73274,7.69154653598979);
#17410=CIRCLE('',#73276,7.69254664694874);
#17411=CIRCLE('',#73277,7.69154682436781);
#17412=CIRCLE('',#73278,7.69306105800644);
#17413=CIRCLE('',#73279,7.44703740601364);
#17414=CIRCLE('',#73280,7.4470374662542);
#17415=CIRCLE('',#73281,7.44703745308987);
#17416=CIRCLE('',#73282,7.44703753082965);
#17417=CIRCLE('',#73283,7.4470375186082);
#17418=CIRCLE('',#73284,7.44703758994448);
#17419=CIRCLE('',#73285,7.4470372444609);
#17420=CIRCLE('',#73286,7.44703762283394);
#17421=CIRCLE('',#73287,7.44703741449571);
#17422=CIRCLE('',#73288,7.44703755754407);
#17423=CIRCLE('',#73289,7.447037331955);
#17424=CIRCLE('',#73290,7.44703753013713);
#17425=CIRCLE('',#73291,7.44703748809038);
#17426=CIRCLE('',#73292,7.44703751023184);
#17427=CIRCLE('',#73293,7.44703743975908);
#17428=CIRCLE('',#73294,7.44703768317363);
#17429=CIRCLE('',#73295,7.44703743497953);
#17430=CIRCLE('',#73296,7.44703737548807);
#17431=CIRCLE('',#73297,7.44703772608559);
#17432=CIRCLE('',#73298,7.44703746302606);
#17433=CIRCLE('',#73299,7.44703734354391);
#17434=CIRCLE('',#73300,7.44703742894028);
#17435=CIRCLE('',#73301,7.44703756648655);
#17436=CIRCLE('',#73302,7.44703765672143);
#17437=CIRCLE('',#73303,7.44703750735441);
#17438=CIRCLE('',#73304,7.44703734033849);
#17439=CIRCLE('',#73305,7.44703728947688);
#17440=CIRCLE('',#73306,7.4470374059196);
#17441=CIRCLE('',#73307,7.44703765920018);
#17442=CIRCLE('',#73308,7.44726855569365);
#17443=CIRCLE('',#73309,7.44947025413789);
#17444=CIRCLE('',#73310,7.44726912411424);
#17445=CIRCLE('',#73311,7.44947031904609);
#17446=CIRCLE('',#73312,7.44726886787919);
#17447=CIRCLE('',#73313,7.4494704190352);
#17448=CIRCLE('',#73314,7.44726899435415);
#17449=CIRCLE('',#73315,7.44947048644738);
#17450=CIRCLE('',#73316,7.44726892731604);
#17451=CIRCLE('',#73317,7.44947035672239);
#17452=CIRCLE('',#73318,7.44726884235559);
#17453=CIRCLE('',#73319,7.44947051052393);
#17454=CIRCLE('',#73320,7.4472689609866);
#17455=CIRCLE('',#73321,7.44947032882476);
#17456=CIRCLE('',#73322,7.44726899765268);
#17457=CIRCLE('',#73323,7.44947053089078);
#17458=CIRCLE('',#73324,7.44726900882362);
#17459=CIRCLE('',#73325,7.44947043308556);
#17460=CIRCLE('',#73326,7.447269063795);
#17461=CIRCLE('',#73327,7.44947037014586);
#17462=CIRCLE('',#73328,7.44726913176407);
#17463=CIRCLE('',#73329,7.44947038677827);
#17464=CIRCLE('',#73330,7.44726899307883);
#17465=CIRCLE('',#73331,7.44947034090865);
#17466=CIRCLE('',#73332,7.44726925582051);
#17467=CIRCLE('',#73333,7.4494704560085);
#17468=CIRCLE('',#73334,7.44726916809589);
#17469=CIRCLE('',#73335,7.44947023321686);
#17470=CIRCLE('',#73336,7.44726899142159);
#17471=CIRCLE('',#73337,7.44947051639951);
#17472=CIRCLE('',#73338,7.44726916275001);
#17473=CIRCLE('',#73339,7.44947054644409);
#17474=CIRCLE('',#73340,7.44726926857587);
#17475=CIRCLE('',#73341,7.44947038945824);
#17476=CIRCLE('',#73342,7.44726894258526);
#17477=CIRCLE('',#73343,7.44947028478043);
#17478=CIRCLE('',#73344,7.44726903924242);
#17479=CIRCLE('',#73345,7.44947057242217);
#17480=CIRCLE('',#73346,7.44726901770602);
#17481=CIRCLE('',#73347,7.44947031239464);
#17482=CIRCLE('',#73348,7.4472693195082);
#17483=CIRCLE('',#73349,7.44947052977426);
#17484=CIRCLE('',#73350,7.44726918026073);
#17485=CIRCLE('',#73351,7.44947047782821);
#17486=CIRCLE('',#73352,7.44726905731159);
#17487=CIRCLE('',#73353,7.44947040140385);
#17488=CIRCLE('',#73354,7.44726922475979);
#17489=CIRCLE('',#73355,7.44947025629113);
#17490=CIRCLE('',#73356,7.44726901139042);
#17491=CIRCLE('',#73357,7.4494704667677);
#17492=CIRCLE('',#73358,7.44726890407121);
#17493=CIRCLE('',#73359,7.44947024139069);
#17494=CIRCLE('',#73360,7.44726911447529);
#17495=CIRCLE('',#73361,7.44947035700436);
#17496=CIRCLE('',#73362,7.44726922435685);
#17497=CIRCLE('',#73363,7.44947055337701);
#17498=CIRCLE('',#73364,7.44726892731434);
#17499=CIRCLE('',#73365,7.44947046068327);
#17500=CIRCLE('',#73366,7.68957748773136);
#17501=CIRCLE('',#73368,7.68734493565065);
#17502=CIRCLE('',#73369,7.68318405249157);
#17503=CIRCLE('',#73370,7.68957748458392);
#17504=CIRCLE('',#73372,7.68734489624771);
#17505=CIRCLE('',#73373,7.68318437103348);
#17506=CIRCLE('',#73374,7.68957744086419);
#17507=CIRCLE('',#73376,7.68734517552602);
#17508=CIRCLE('',#73377,7.68318459103349);
#17509=CIRCLE('',#73378,7.68957743242436);
#17510=CIRCLE('',#73380,7.68734491438801);
#17511=CIRCLE('',#73381,7.68318419339124);
#17512=CIRCLE('',#73382,7.68957745052179);
#17513=CIRCLE('',#73384,7.68734521661807);
#17514=CIRCLE('',#73385,7.68318455697533);
#17515=CIRCLE('',#73386,7.68957749671537);
#17516=CIRCLE('',#73388,7.68734510049166);
#17517=CIRCLE('',#73389,7.68318476711861);
#17518=CIRCLE('',#73390,7.68957725009669);
#17519=CIRCLE('',#73392,7.68734508539297);
#17520=CIRCLE('',#73393,7.68318416167277);
#17521=CIRCLE('',#73394,7.68957754605477);
#17522=CIRCLE('',#73396,7.68734531279094);
#17523=CIRCLE('',#73397,7.68318447137342);
#17524=CIRCLE('',#73398,7.68957743776089);
#17525=CIRCLE('',#73400,7.68734503598025);
#17526=CIRCLE('',#73401,7.68318432152863);
#17527=CIRCLE('',#73402,7.68957747820737);
#17528=CIRCLE('',#73404,7.68734493513009);
#17529=CIRCLE('',#73405,7.68318409703447);
#17530=CIRCLE('',#73406,7.68957705118966);
#17531=CIRCLE('',#73408,7.68734522406006);
#17532=CIRCLE('',#73409,7.6831844819381);
#17533=CIRCLE('',#73410,7.68957752053836);
#17534=CIRCLE('',#73412,7.68734483074303);
#17535=CIRCLE('',#73413,7.68318425943268);
#17536=CIRCLE('',#73414,7.6895774318264);
#17537=CIRCLE('',#73416,7.68734525206946);
#17538=CIRCLE('',#73417,7.68318481127215);
#17539=CIRCLE('',#73418,7.6895775763399);
#17540=CIRCLE('',#73420,7.68734508461849);
#17541=CIRCLE('',#73421,7.68318462759078);
#17542=CIRCLE('',#73422,7.68957738759692);
#17543=CIRCLE('',#73424,7.68734522525487);
#17544=CIRCLE('',#73425,7.68318434353235);
#17545=CIRCLE('',#73426,7.68957724595044);
#17546=CIRCLE('',#73428,7.68734506964628);
#17547=CIRCLE('',#73429,7.68318443245175);
#17548=CIRCLE('',#73430,7.68957738309765);
#17549=CIRCLE('',#73432,7.68734504312503);
#17550=CIRCLE('',#73433,7.68318397319927);
#17551=CIRCLE('',#73434,7.68957728912674);
#17552=CIRCLE('',#73436,7.68734509419147);
#17553=CIRCLE('',#73437,7.68318426666675);
#17554=CIRCLE('',#73438,7.68957758500744);
#17555=CIRCLE('',#73440,7.68734497218318);
#17556=CIRCLE('',#73441,7.68318482091028);
#17557=CIRCLE('',#73442,7.68957729276197);
#17558=CIRCLE('',#73444,7.6873448380935);
#17559=CIRCLE('',#73445,7.68318452630792);
#17560=CIRCLE('',#73446,7.68957752851105);
#17561=CIRCLE('',#73448,7.68734510837944);
#17562=CIRCLE('',#73449,7.68318408620418);
#17563=CIRCLE('',#73450,7.68957715464276);
#17564=CIRCLE('',#73452,7.68734514858287);
#17565=CIRCLE('',#73453,7.68318398809372);
#17566=CIRCLE('',#73454,7.68957737159601);
#17567=CIRCLE('',#73456,7.68734517557214);
#17568=CIRCLE('',#73457,7.68318447990036);
#17569=CIRCLE('',#73458,7.68957741388642);
#17570=CIRCLE('',#73460,7.68734505044421);
#17571=CIRCLE('',#73461,7.68318420939938);
#17572=CIRCLE('',#73462,7.68957728276303);
#17573=CIRCLE('',#73464,7.68734508066004);
#17574=CIRCLE('',#73465,7.68318447973266);
#17575=CIRCLE('',#73466,7.68957727092898);
#17576=CIRCLE('',#73468,7.6873452387982);
#17577=CIRCLE('',#73469,7.68318471227011);
#17578=CIRCLE('',#73470,7.68957735899398);
#17579=CIRCLE('',#73472,7.68734495766267);
#17580=CIRCLE('',#73473,7.68318431078746);
#17581=CIRCLE('',#73474,7.68957718057119);
#17582=CIRCLE('',#73476,7.68734532714596);
#17583=CIRCLE('',#73477,7.68318490909885);
#17584=CIRCLE('',#73478,7.68983489396897);
#17585=CIRCLE('',#73479,7.69301696143299);
#17586=CIRCLE('',#73481,7.69198148285114);
#17587=CIRCLE('',#73482,7.6835593980278);
#17588=CIRCLE('',#73483,7.68983488140878);
#17589=CIRCLE('',#73484,7.6930165800384);
#17590=CIRCLE('',#73486,7.69198186433056);
#17591=CIRCLE('',#73487,7.68355933601086);
#17592=CIRCLE('',#73488,7.6898349856185);
#17593=CIRCLE('',#73489,7.69301671090392);
#17594=CIRCLE('',#73491,7.69198175834686);
#17595=CIRCLE('',#73492,7.6835588366298);
#17596=CIRCLE('',#73493,7.68983478878477);
#17597=CIRCLE('',#73494,7.69301677755821);
#17598=CIRCLE('',#73496,7.6919818100264);
#17599=CIRCLE('',#73497,7.68355962336939);
#17600=CIRCLE('',#73498,7.68983500365314);
#17601=CIRCLE('',#73499,7.69301670443458);
#17602=CIRCLE('',#73501,7.69198173167657);
#17603=CIRCLE('',#73502,7.68355934414267);
#17604=CIRCLE('',#73503,7.68983492418413);
#17605=CIRCLE('',#73504,7.69301683580422);
#17606=CIRCLE('',#73506,7.69198163514051);
#17607=CIRCLE('',#73507,7.6835589110352);
#17608=CIRCLE('',#73508,7.68983487983782);
#17609=CIRCLE('',#73509,7.69301657714507);
#17610=CIRCLE('',#73511,7.69198183398963);
#17611=CIRCLE('',#73512,7.68355883494166);
#17612=CIRCLE('',#73513,7.68983489291763);
#17613=CIRCLE('',#73514,7.6930169715151);
#17614=CIRCLE('',#73516,7.69198147194979);
#17615=CIRCLE('',#73517,7.68355917426551);
#17616=CIRCLE('',#73518,7.68983510882082);
#17617=CIRCLE('',#73519,7.69301663246352);
#17618=CIRCLE('',#73521,7.69198163455624);
#17619=CIRCLE('',#73522,7.68355943924273);
#17620=CIRCLE('',#73523,7.68983479825435);
#17621=CIRCLE('',#73524,7.69301681989919);
#17622=CIRCLE('',#73526,7.6919815043616);
#17623=CIRCLE('',#73527,7.68355894458752);
#17624=CIRCLE('',#73528,7.6898351140751);
#17625=CIRCLE('',#73529,7.69301671501356);
#17626=CIRCLE('',#73531,7.69198167371706);
#17627=CIRCLE('',#73532,7.68355932858418);
#17628=CIRCLE('',#73533,7.68983517939378);
#17629=CIRCLE('',#73534,7.69301664922328);
#17630=CIRCLE('',#73536,7.69198155170029);
#17631=CIRCLE('',#73537,7.68355932581089);
#17632=CIRCLE('',#73538,7.68983489071601);
#17633=CIRCLE('',#73539,7.69301679907012);
#17634=CIRCLE('',#73541,7.69198165345984);
#17635=CIRCLE('',#73542,7.68355935171591);
#17636=CIRCLE('',#73543,7.68983486491984);
#17637=CIRCLE('',#73544,7.6930167136401);
#17638=CIRCLE('',#73546,7.69198156882893);
#17639=CIRCLE('',#73547,7.68355931944083);
#17640=CIRCLE('',#73548,7.6898350257074);
#17641=CIRCLE('',#73549,7.69301667356443);
#17642=CIRCLE('',#73551,7.69198166635035);
#17643=CIRCLE('',#73552,7.68355902854595);
#17644=CIRCLE('',#73553,7.68983514730196);
#17645=CIRCLE('',#73554,7.69301661826608);
#17646=CIRCLE('',#73556,7.69198176951274);
#17647=CIRCLE('',#73557,7.68355940594295);
#17648=CIRCLE('',#73558,7.6898350638292);
#17649=CIRCLE('',#73559,7.69301659660404);
#17650=CIRCLE('',#73561,7.69198160962702);
#17651=CIRCLE('',#73562,7.68355913972534);
#17652=CIRCLE('',#73563,7.68983478759058);
#17653=CIRCLE('',#73564,7.69301692248647);
#17654=CIRCLE('',#73566,7.6919815430316);
#17655=CIRCLE('',#73567,7.68355907541356);
#17656=CIRCLE('',#73568,7.68983480591283);
#17657=CIRCLE('',#73569,7.6930166833839);
#17658=CIRCLE('',#73571,7.69198180730898);
#17659=CIRCLE('',#73572,7.68355879276394);
#17660=CIRCLE('',#73573,7.68983495333692);
#17661=CIRCLE('',#73574,7.69301663935876);
#17662=CIRCLE('',#73576,7.69198160697219);
#17663=CIRCLE('',#73577,7.68355894623691);
#17664=CIRCLE('',#73578,7.68983489183394);
#17665=CIRCLE('',#73579,7.69301656700983);
#17666=CIRCLE('',#73581,7.69198148895534);
#17667=CIRCLE('',#73582,7.68355875344865);
#17668=CIRCLE('',#73583,7.68983508864516);
#17669=CIRCLE('',#73584,7.69301691731102);
#17670=CIRCLE('',#73586,7.69198162591986);
#17671=CIRCLE('',#73587,7.68355909405863);
#17672=CIRCLE('',#73588,7.68983508237929);
#17673=CIRCLE('',#73589,7.69301673454273);
#17674=CIRCLE('',#73591,7.69198177259239);
#17675=CIRCLE('',#73592,7.68355939897891);
#17676=CIRCLE('',#73593,7.68983525272473);
#17677=CIRCLE('',#73594,7.69301685764793);
#17678=CIRCLE('',#73596,7.69198163217241);
#17679=CIRCLE('',#73597,7.68355943041218);
#17680=CIRCLE('',#73598,7.68983498373113);
#17681=CIRCLE('',#73599,7.69301670508415);
#17682=CIRCLE('',#73601,7.69198185871811);
#17683=CIRCLE('',#73602,7.68355915919088);
#17684=CIRCLE('',#73603,7.6898348611317);
#17685=CIRCLE('',#73604,7.69301693833565);
#17686=CIRCLE('',#73606,7.69198149127824);
#17687=CIRCLE('',#73607,7.68355944766628);
#17688=CIRCLE('',#73608,7.68983495953567);
#17689=CIRCLE('',#73609,7.69301672696527);
#17690=CIRCLE('',#73611,7.69198153689078);
#17691=CIRCLE('',#73612,7.68355905642999);
#17692=CIRCLE('',#73613,7.68983511208836);
#17693=CIRCLE('',#73614,7.69301685417526);
#17694=CIRCLE('',#73616,7.69198149366435);
#17695=CIRCLE('',#73617,7.68355961099684);
#17696=CIRCLE('',#73618,7.4450188933114);
#17697=CIRCLE('',#73619,7.44501890449599);
#17698=CIRCLE('',#73620,7.44501879756203);
#17699=CIRCLE('',#73621,7.44501861859603);
#17700=CIRCLE('',#73622,7.44501870669753);
#17701=CIRCLE('',#73623,7.44501871524855);
#17702=CIRCLE('',#73624,7.44501858121209);
#17703=CIRCLE('',#73625,7.44501866536265);
#17704=CIRCLE('',#73626,7.44501872599696);
#17705=CIRCLE('',#73627,7.44501856118857);
#17706=CIRCLE('',#73628,7.44501846236666);
#17707=CIRCLE('',#73629,7.445018651669);
#17708=CIRCLE('',#73630,7.44501885804999);
#17709=CIRCLE('',#73631,7.44501884348547);
#17710=CIRCLE('',#73632,7.44501853237831);
#17711=CIRCLE('',#73633,7.44501869383856);
#17712=CIRCLE('',#73634,7.44501879936885);
#17713=CIRCLE('',#73635,7.44501890514634);
#17714=CIRCLE('',#73636,7.44501858495637);
#17715=CIRCLE('',#73637,7.4450186247389);
#17716=CIRCLE('',#73638,7.44501880900192);
#17717=CIRCLE('',#73639,7.44501880897738);
#17718=CIRCLE('',#73640,7.44501868801496);
#17719=CIRCLE('',#73641,7.44501845999727);
#17720=CIRCLE('',#73642,7.44501866742756);
#17721=CIRCLE('',#73643,7.44501869596626);
#17722=CIRCLE('',#73644,7.44501881893982);
#17723=CIRCLE('',#73645,7.44501863612009);
#17724=CIRCLE('',#73646,7.44501877643286);
#17725=CIRCLE('',#73647,7.44783687688711);
#17726=CIRCLE('',#73648,7.44783621953896);
#17727=CIRCLE('',#73649,7.44783669832343);
#17728=CIRCLE('',#73650,7.44783643383807);
#17729=CIRCLE('',#73651,7.44783642389326);
#17730=CIRCLE('',#73652,7.44783654872719);
#17731=CIRCLE('',#73653,7.44783637644797);
#17732=CIRCLE('',#73654,7.44783635948184);
#17733=CIRCLE('',#73655,7.4478365441613);
#17734=CIRCLE('',#73656,7.44783669119075);
#17735=CIRCLE('',#73657,7.44783686377082);
#17736=CIRCLE('',#73658,7.44783656581571);
#17737=CIRCLE('',#73659,7.44783643994268);
#17738=CIRCLE('',#73660,7.44783624491067);
#17739=CIRCLE('',#73661,7.44783654854467);
#17740=CIRCLE('',#73662,7.44783673428636);
#17741=CIRCLE('',#73663,7.44783662736838);
#17742=CIRCLE('',#73664,7.44783654086163);
#17743=CIRCLE('',#73665,7.44783627414982);
#17744=CIRCLE('',#73666,7.44783632320642);
#17745=CIRCLE('',#73667,7.4478366598755);
#17746=CIRCLE('',#73668,7.4478368763373);
#17747=CIRCLE('',#73669,7.44783643817806);
#17748=CIRCLE('',#73670,7.44783634404276);
#17749=CIRCLE('',#73671,7.44783650547921);
#17750=CIRCLE('',#73672,7.44783628390043);
#17751=CIRCLE('',#73673,7.44783629608604);
#17752=CIRCLE('',#73674,7.44783649178178);
#17753=CIRCLE('',#73675,7.44783649132846);
#17754=CIRCLE('',#73676,7.68969363660472);
#17755=CIRCLE('',#73678,7.69279317840802);
#17756=CIRCLE('',#73679,7.68635996865851);
#17757=CIRCLE('',#73680,7.68969386660789);
#17758=CIRCLE('',#73682,7.69279302868398);
#17759=CIRCLE('',#73683,7.68635995762749);
#17760=CIRCLE('',#73684,7.6896936900641);
#17761=CIRCLE('',#73686,7.69279326824012);
#17762=CIRCLE('',#73687,7.68635976553776);
#17763=CIRCLE('',#73688,7.68969386253329);
#17764=CIRCLE('',#73690,7.69279334574968);
#17765=CIRCLE('',#73691,7.68635983205112);
#17766=CIRCLE('',#73692,7.68969375114687);
#17767=CIRCLE('',#73694,7.69279335413577);
#17768=CIRCLE('',#73695,7.68636002466187);
#17769=CIRCLE('',#73696,7.68969359649545);
#17770=CIRCLE('',#73698,7.69279335917638);
#17771=CIRCLE('',#73699,7.68635978519035);
#17772=CIRCLE('',#73700,7.68969373989023);
#17773=CIRCLE('',#73702,7.69279333421998);
#17774=CIRCLE('',#73703,7.68636003724103);
#17775=CIRCLE('',#73704,7.68969374098561);
#17776=CIRCLE('',#73706,7.69279339904735);
#17777=CIRCLE('',#73707,7.68635982561929);
#17778=CIRCLE('',#73708,7.68969385681376);
#17779=CIRCLE('',#73710,7.69279310456421);
#17780=CIRCLE('',#73711,7.68636023014239);
#17781=CIRCLE('',#73712,7.68969387721714);
#17782=CIRCLE('',#73714,7.69279308553252);
#17783=CIRCLE('',#73715,7.68635990825226);
#17784=CIRCLE('',#73716,7.68969389757644);
#17785=CIRCLE('',#73718,7.69279299440528);
#17786=CIRCLE('',#73719,7.68636005141107);
#17787=CIRCLE('',#73720,7.68969366115901);
#17788=CIRCLE('',#73722,7.69279333913911);
#17789=CIRCLE('',#73723,7.68635983689438);
#17790=CIRCLE('',#73724,7.6896937696048);
#17791=CIRCLE('',#73726,7.69279311454176);
#17792=CIRCLE('',#73727,7.68635991851817);
#17793=CIRCLE('',#73728,7.68969363397531);
#17794=CIRCLE('',#73730,7.69279332251533);
#17795=CIRCLE('',#73731,7.68635998349788);
#17796=CIRCLE('',#73732,7.68969374897493);
#17797=CIRCLE('',#73734,7.69279337928139);
#17798=CIRCLE('',#73735,7.68635971742891);
#17799=CIRCLE('',#73736,7.6896937771446);
#17800=CIRCLE('',#73738,7.69279344747408);
#17801=CIRCLE('',#73739,7.68635974620921);
#17802=CIRCLE('',#73740,7.68969377094987);
#17803=CIRCLE('',#73742,7.692793522416);
#17804=CIRCLE('',#73743,7.6863598904576);
#17805=CIRCLE('',#73744,7.68969376075281);
#17806=CIRCLE('',#73746,7.6927931364953);
#17807=CIRCLE('',#73747,7.68636010655716);
#17808=CIRCLE('',#73748,7.68969359457469);
#17809=CIRCLE('',#73750,7.69279307209504);
#17810=CIRCLE('',#73751,7.6863600924503);
#17811=CIRCLE('',#73752,7.68969379778712);
#17812=CIRCLE('',#73754,7.6927930664211);
#17813=CIRCLE('',#73755,7.68635987732735);
#17814=CIRCLE('',#73756,7.68969392003808);
#17815=CIRCLE('',#73757,7.6896908311552);
#17816=CIRCLE('',#73759,7.69279329720953);
#17817=CIRCLE('',#73760,7.68635720976654);
#17818=CIRCLE('',#73762,7.68969386605261);
#17819=CIRCLE('',#73763,7.69279319432287);
#17820=CIRCLE('',#73764,7.68636009881248);
#17821=CIRCLE('',#73766,7.6927933916593);
#17822=CIRCLE('',#73767,7.68635984579723);
#17823=CIRCLE('',#73768,7.68969363382393);
#17824=CIRCLE('',#73770,7.69279330196327);
#17825=CIRCLE('',#73771,7.68635971171485);
#17826=CIRCLE('',#73772,7.68969361013494);
#17827=CIRCLE('',#73774,7.69279321901403);
#17828=CIRCLE('',#73775,7.68636012112819);
#17829=CIRCLE('',#73776,7.68969391216473);
#17830=CIRCLE('',#73778,7.69279317458319);
#17831=CIRCLE('',#73779,7.68635964597867);
#17832=CIRCLE('',#73780,7.68969355089801);
#17833=CIRCLE('',#73782,7.69279340184492);
#17834=CIRCLE('',#73783,7.68635993568266);
#17835=CIRCLE('',#73784,7.68969386466671);
#17836=CIRCLE('',#73786,7.6927931617596);
#17837=CIRCLE('',#73787,7.68635979372616);
#17838=CIRCLE('',#73788,7.69049143301784);
#17839=CIRCLE('',#73789,7.69049161415286);
#17840=CIRCLE('',#73791,7.68475569860886);
#17841=CIRCLE('',#73792,7.68602741023802);
#17842=CIRCLE('',#73793,7.69049152140508);
#17843=CIRCLE('',#73795,7.68475572981308);
#17844=CIRCLE('',#73796,7.68602772638459);
#17845=CIRCLE('',#73797,7.69049160139286);
#17846=CIRCLE('',#73799,7.6847557150075);
#17847=CIRCLE('',#73800,7.68602747013878);
#17848=CIRCLE('',#73801,7.69049165362067);
#17849=CIRCLE('',#73803,7.68475539161247);
#17850=CIRCLE('',#73804,7.68602763473392);
#17851=CIRCLE('',#73805,7.69049185324544);
#17852=CIRCLE('',#73807,7.68475566956591);
#17853=CIRCLE('',#73808,7.68602761290782);
#17854=CIRCLE('',#73809,7.69049145761145);
#17855=CIRCLE('',#73811,7.68475571189761);
#17856=CIRCLE('',#73812,7.68602760007439);
#17857=CIRCLE('',#73813,7.6904916485909);
#17858=CIRCLE('',#73815,7.68475573508915);
#17859=CIRCLE('',#73816,7.68602771007527);
#17860=CIRCLE('',#73817,7.69049150126655);
#17861=CIRCLE('',#73819,7.68475566164297);
#17862=CIRCLE('',#73820,7.68602755871313);
#17863=CIRCLE('',#73821,7.69049174527211);
#17864=CIRCLE('',#73823,7.68475596896526);
#17865=CIRCLE('',#73824,7.6860273611231);
#17866=CIRCLE('',#73825,7.69049164220205);
#17867=CIRCLE('',#73827,7.68475546250515);
#17868=CIRCLE('',#73828,7.68602787972657);
#17869=CIRCLE('',#73829,7.69049163629909);
#17870=CIRCLE('',#73831,7.68475572461334);
#17871=CIRCLE('',#73832,7.68602754757312);
#17872=CIRCLE('',#73833,7.69049166028763);
#17873=CIRCLE('',#73835,7.68475597486026);
#17874=CIRCLE('',#73836,7.68602729094763);
#17875=CIRCLE('',#73837,7.69049160408503);
#17876=CIRCLE('',#73839,7.68475528721708);
#17877=CIRCLE('',#73840,7.68602767517274);
#17878=CIRCLE('',#73841,7.69049163940496);
#17879=CIRCLE('',#73843,7.68475561008966);
#17880=CIRCLE('',#73844,7.68602753984931);
#17881=CIRCLE('',#73845,7.69049167756843);
#17882=CIRCLE('',#73847,7.68475597255132);
#17883=CIRCLE('',#73848,7.68602762271067);
#17884=CIRCLE('',#73849,7.69049159845339);
#17885=CIRCLE('',#73851,7.68475551206392);
#17886=CIRCLE('',#73852,7.68602756172998);
#17887=CIRCLE('',#73853,7.69049166255934);
#17888=CIRCLE('',#73855,7.68475579404613);
#17889=CIRCLE('',#73856,7.68602756269892);
#17890=CIRCLE('',#73857,7.69049166895877);
#17891=CIRCLE('',#73859,7.68475564415784);
#17892=CIRCLE('',#73860,7.6860273428279);
#17893=CIRCLE('',#73861,7.69049150448244);
#17894=CIRCLE('',#73863,7.68475576796664);
#17895=CIRCLE('',#73864,7.68602744803473);
#17896=CIRCLE('',#73865,7.69049144400215);
#17897=CIRCLE('',#73867,7.68475559032282);
#17898=CIRCLE('',#73868,7.68602747872486);
#17899=CIRCLE('',#73869,7.69049170918301);
#17900=CIRCLE('',#73871,7.68475579599015);
#17901=CIRCLE('',#73872,7.6860277113899);
#17902=CIRCLE('',#73873,7.69049155823195);
#17903=CIRCLE('',#73875,7.68475544644147);
#17904=CIRCLE('',#73876,7.68602747845228);
#17905=CIRCLE('',#73877,7.69049157336687);
#17906=CIRCLE('',#73879,7.68475573644825);
#17907=CIRCLE('',#73880,7.68602731299916);
#17908=CIRCLE('',#73881,7.69049175407852);
#17909=CIRCLE('',#73883,7.68475567017514);
#17910=CIRCLE('',#73884,7.68602748502965);
#17911=CIRCLE('',#73885,7.69049145574597);
#17912=CIRCLE('',#73887,7.6847555902511);
#17913=CIRCLE('',#73888,7.68602772472989);
#17914=CIRCLE('',#73889,7.69049164589603);
#17915=CIRCLE('',#73891,7.68475556041525);
#17916=CIRCLE('',#73892,7.68602739672098);
#17917=CIRCLE('',#73893,7.69049151223703);
#17918=CIRCLE('',#73895,7.68475595845802);
#17919=CIRCLE('',#73896,7.68602760723119);
#17920=CIRCLE('',#73898,7.68475569621939);
#17921=CIRCLE('',#73899,7.6860274156871);
#17922=CIRCLE('',#73900,7.4441241331261);
#17923=CIRCLE('',#73901,7.44962098873202);
#17924=CIRCLE('',#73902,7.44412180952238);
#17925=CIRCLE('',#73903,7.44962082790162);
#17926=CIRCLE('',#73904,7.44412154997683);
#17927=CIRCLE('',#73905,7.4496207652638);
#17928=CIRCLE('',#73906,7.44412175052952);
#17929=CIRCLE('',#73907,7.44962098477913);
#17930=CIRCLE('',#73908,7.44412174529551);
#17931=CIRCLE('',#73909,7.44962097025448);
#17932=CIRCLE('',#73910,7.44412158364088);
#17933=CIRCLE('',#73911,7.44962082581289);
#17934=CIRCLE('',#73912,7.44412158122055);
#17935=CIRCLE('',#73913,7.44962082724999);
#17936=CIRCLE('',#73914,7.44412161528393);
#17937=CIRCLE('',#73915,7.44962123096025);
#17938=CIRCLE('',#73916,7.44412179534068);
#17939=CIRCLE('',#73917,7.44962098648082);
#17940=CIRCLE('',#73918,7.44412174137443);
#17941=CIRCLE('',#73919,7.44962074392395);
#17942=CIRCLE('',#73920,7.44412180128965);
#17943=CIRCLE('',#73921,7.4496207975329);
#17944=CIRCLE('',#73922,7.44412154466149);
#17945=CIRCLE('',#73923,7.44962083948352);
#17946=CIRCLE('',#73924,7.44412191376129);
#17947=CIRCLE('',#73925,7.44962082298598);
#17948=CIRCLE('',#73926,7.44412173712964);
#17949=CIRCLE('',#73927,7.44962099064716);
#17950=CIRCLE('',#73928,7.44412164601454);
#17951=CIRCLE('',#73929,7.44962091021146);
#17952=CIRCLE('',#73930,7.44412161917552);
#17953=CIRCLE('',#73931,7.44962093879096);
#17954=CIRCLE('',#73932,7.44412153423081);
#17955=CIRCLE('',#73933,7.44962107444784);
#17956=CIRCLE('',#73934,7.44412183990525);
#17957=CIRCLE('',#73935,7.44962103513103);
#17958=CIRCLE('',#73936,7.44412166798311);
#17959=CIRCLE('',#73937,7.44962107754971);
#17960=CIRCLE('',#73938,7.4441216537555);
#17961=CIRCLE('',#73939,7.4496206428889);
#17962=CIRCLE('',#73940,7.44412167613138);
#17963=CIRCLE('',#73941,7.44962100045877);
#17964=CIRCLE('',#73942,7.44412169957312);
#17965=CIRCLE('',#73943,7.44962075048619);
#17966=CIRCLE('',#73944,7.44412154619005);
#17967=CIRCLE('',#73945,7.44962091788761);
#17968=CIRCLE('',#73946,7.44412170737385);
#17969=CIRCLE('',#73947,7.44962106412872);
#17970=CIRCLE('',#73948,7.44412169520957);
#17971=CIRCLE('',#73949,7.44962101012624);
#17972=CIRCLE('',#73950,7.44412165636468);
#17973=CIRCLE('',#73951,7.44962088978097);
#17974=CIRCLE('',#73952,7.44412171376414);
#17975=CIRCLE('',#73953,7.44962092331337);
#17976=CIRCLE('',#73954,7.44412153513632);
#17977=CIRCLE('',#73955,7.44962090241827);
#17978=CIRCLE('',#73956,7.44412157163877);
#17979=CIRCLE('',#73957,7.44962220320026);
#17980=CIRCLE('',#73958,7.44380150548939);
#17981=CIRCLE('',#73959,7.44380000680351);
#17982=CIRCLE('',#73960,7.4438001907365);
#17983=CIRCLE('',#73961,7.44379998723725);
#17984=CIRCLE('',#73962,7.44380000199902);
#17985=CIRCLE('',#73963,7.44379993030849);
#17986=CIRCLE('',#73964,7.44379976545896);
#17987=CIRCLE('',#73965,7.4437999487249);
#17988=CIRCLE('',#73966,7.44380009861783);
#17989=CIRCLE('',#73967,7.4437998982179);
#17990=CIRCLE('',#73968,7.44380017020166);
#17991=CIRCLE('',#73969,7.44379940853564);
#17992=CIRCLE('',#73970,7.44380004651171);
#17993=CIRCLE('',#73971,7.44379989072602);
#17994=CIRCLE('',#73972,7.44379996753508);
#17995=CIRCLE('',#73973,7.44380026452087);
#17996=CIRCLE('',#73974,7.44380001448714);
#17997=CIRCLE('',#73975,7.44379978702513);
#17998=CIRCLE('',#73976,7.44379988901668);
#17999=CIRCLE('',#73977,7.44379976723227);
#18000=CIRCLE('',#73978,7.44380009914586);
#18001=CIRCLE('',#73979,7.44380008131669);
#18002=CIRCLE('',#73980,7.4437999315236);
#18003=CIRCLE('',#73981,7.44379996658801);
#18004=CIRCLE('',#73982,7.44380005441912);
#18005=CIRCLE('',#73983,7.44380010128159);
#18006=CIRCLE('',#73984,7.44379996239169);
#18007=CIRCLE('',#73985,7.44380004600786);
#18008=CIRCLE('',#73986,7.44380002572478);
#18009=CIRCLE('',#73987,7.68894244416909);
#18010=CIRCLE('',#73989,7.69154643806877);
#18011=CIRCLE('',#73990,7.69254667889009);
#18012=CIRCLE('',#73991,7.69306086011482);
#18013=CIRCLE('',#73992,7.68894234890342);
#18014=CIRCLE('',#73994,7.69154662654791);
#18015=CIRCLE('',#73995,7.69254646639703);
#18016=CIRCLE('',#73996,7.69306109538576);
#18017=CIRCLE('',#73997,7.68894231004885);
#18018=CIRCLE('',#73999,7.69154650794579);
#18019=CIRCLE('',#74000,7.69254643716538);
#18020=CIRCLE('',#74001,7.69306098564575);
#18021=CIRCLE('',#74002,7.68894214032325);
#18022=CIRCLE('',#74004,7.69154695753898);
#18023=CIRCLE('',#74005,7.69254640742847);
#18024=CIRCLE('',#74006,7.69306102978304);
#18025=CIRCLE('',#74007,7.68894230068754);
#18026=CIRCLE('',#74009,7.6915466516697);
#18027=CIRCLE('',#74010,7.69254652874586);
#18028=CIRCLE('',#74011,7.69306103950312);
#18029=CIRCLE('',#74012,7.68894217261782);
#18030=CIRCLE('',#74014,7.6915468492434);
#18031=CIRCLE('',#74015,7.69254635550889);
#18032=CIRCLE('',#74016,7.69306106289197);
#18033=CIRCLE('',#74017,7.68894227017874);
#18034=CIRCLE('',#74019,7.69154650939399);
#18035=CIRCLE('',#74020,7.69254642329256);
#18036=CIRCLE('',#74021,7.69306091598276);
#18037=CIRCLE('',#74022,7.68894227758912);
#18038=CIRCLE('',#74024,7.69154669278215);
#18039=CIRCLE('',#74025,7.69254632430852);
#18040=CIRCLE('',#74026,7.69306090803412);
#18041=CIRCLE('',#74027,7.68894208372619);
#18042=CIRCLE('',#74029,7.69154674898312);
#18043=CIRCLE('',#74030,7.69254616753055);
#18044=CIRCLE('',#74031,7.69306114235764);
#18045=CIRCLE('',#74032,7.68894230100823);
#18046=CIRCLE('',#74034,7.69154694513176);
#18047=CIRCLE('',#74035,7.69254629731355);
#18048=CIRCLE('',#74036,7.69306123255489);
#18049=CIRCLE('',#74037,7.68894220126532);
#18050=CIRCLE('',#74039,7.69154643777242);
#18051=CIRCLE('',#74040,7.69254642561957);
#18052=CIRCLE('',#74041,7.69306066636817);
#18053=CIRCLE('',#74042,7.68894231213788);
#18054=CIRCLE('',#74044,7.6915465723561);
#18055=CIRCLE('',#74045,7.69254635178032);
#18056=CIRCLE('',#74046,7.69306080893017);
#18057=CIRCLE('',#74047,7.68894221503211);
#18058=CIRCLE('',#74049,7.6915466326821);
#18059=CIRCLE('',#74050,7.69254654865938);
#18060=CIRCLE('',#74051,7.69306113942179);
#18061=CIRCLE('',#74052,7.6889421698178);
#18062=CIRCLE('',#74054,7.69154662159575);
#18063=CIRCLE('',#74055,7.69254659525327);
#18064=CIRCLE('',#74056,7.6930609598333);
#18065=CIRCLE('',#74057,7.68894217840434);
#18066=CIRCLE('',#74059,7.69154657054028);
#18067=CIRCLE('',#74060,7.69254661883229);
#18068=CIRCLE('',#74061,7.69306076749964);
#18069=CIRCLE('',#74062,7.6889422576405);
#18070=CIRCLE('',#74064,7.69154662261387);
#18071=CIRCLE('',#74065,7.69254645368903);
#18072=CIRCLE('',#74066,7.69306084906152);
#18073=CIRCLE('',#74067,7.68894217718232);
#18074=CIRCLE('',#74069,7.6915464115028);
#18075=CIRCLE('',#74070,7.69254622518674);
#18076=CIRCLE('',#74071,7.69306080188211);
#18077=CIRCLE('',#74072,7.68894206501938);
#18078=CIRCLE('',#74074,7.69154674301802);
#18079=CIRCLE('',#74075,7.69254664274991);
#18080=CIRCLE('',#74076,7.69306095020453);
#18081=CIRCLE('',#74077,7.68894200646331);
#18082=CIRCLE('',#74079,7.69154677190965);
#18083=CIRCLE('',#74080,7.69254659932621);
#18084=CIRCLE('',#74081,7.69306102148478);
#18085=CIRCLE('',#74082,7.68894217824212);
#18086=CIRCLE('',#74084,7.69154656930193);
#18087=CIRCLE('',#74085,7.69254660059922);
#18088=CIRCLE('',#74086,7.69306110352981);
#18089=CIRCLE('',#74087,7.68894229148283);
#18090=CIRCLE('',#74088,7.69305583026409);
#18091=CIRCLE('',#74090,7.69154675624609);
#18092=CIRCLE('',#74091,7.69254128953939);
#18093=CIRCLE('',#74092,7.68894235630222);
#18094=CIRCLE('',#74094,7.693061068196);
#18095=CIRCLE('',#74095,7.69154691308647);
#18096=CIRCLE('',#74096,7.69254635983995);
#18097=CIRCLE('',#74097,7.68894209982254);
#18098=CIRCLE('',#74099,7.69154654828669);
#18099=CIRCLE('',#74100,7.69254651461116);
#18100=CIRCLE('',#74101,7.69306097724112);
#18101=CIRCLE('',#74102,7.68894224453809);
#18102=CIRCLE('',#74104,7.69154647613157);
#18103=CIRCLE('',#74105,7.69254630388625);
#18104=CIRCLE('',#74106,7.69306121587964);
#18105=CIRCLE('',#74107,7.68894206378456);
#18106=CIRCLE('',#74109,7.69154649978663);
#18107=CIRCLE('',#74110,7.69254629177802);
#18108=CIRCLE('',#74111,7.69306081211227);
#18109=CIRCLE('',#74112,7.68894199816537);
#18110=CIRCLE('',#74114,7.69154666770906);
#18111=CIRCLE('',#74115,7.69254632743289);
#18112=CIRCLE('',#74116,7.69306094639951);
#18113=CIRCLE('',#74117,7.68894215868675);
#18114=CIRCLE('',#74119,7.69154658380995);
#18115=CIRCLE('',#74120,7.69254652211315);
#18116=CIRCLE('',#74121,7.69306080752694);
#18117=CIRCLE('',#74122,7.6889421547065);
#18118=CIRCLE('',#74124,7.69154672679512);
#18119=CIRCLE('',#74125,7.69254664713157);
#18120=CIRCLE('',#74126,7.69306105760353);
#18121=CIRCLE('',#74127,7.68866079157655);
#18122=CIRCLE('',#74129,7.68493063279481);
#18123=CIRCLE('',#74130,7.69242158874635);
#18124=CIRCLE('',#74131,7.68866085610895);
#18125=CIRCLE('',#74133,7.68493073427246);
#18126=CIRCLE('',#74134,7.69242153534071);
#18127=CIRCLE('',#74135,7.68866057768082);
#18128=CIRCLE('',#74137,7.68493065739063);
#18129=CIRCLE('',#74138,7.69242136477564);
#18130=CIRCLE('',#74139,7.68866046048346);
#18131=CIRCLE('',#74141,7.68493071227508);
#18132=CIRCLE('',#74142,7.69242129349027);
#18133=CIRCLE('',#74143,7.68866070478409);
#18134=CIRCLE('',#74145,7.68493080555999);
#18135=CIRCLE('',#74146,7.69242166647581);
#18136=CIRCLE('',#74147,7.68866102373785);
#18137=CIRCLE('',#74149,7.68493073465088);
#18138=CIRCLE('',#74150,7.69242161162231);
#18139=CIRCLE('',#74151,7.68866070214171);
#18140=CIRCLE('',#74153,7.68493083698717);
#18141=CIRCLE('',#74154,7.69242127471809);
#18142=CIRCLE('',#74155,7.68866070803868);
#18143=CIRCLE('',#74157,7.68493077752384);
#18144=CIRCLE('',#74158,7.69242159894978);
#18145=CIRCLE('',#74159,7.68866068058214);
#18146=CIRCLE('',#74161,7.68493077403634);
#18147=CIRCLE('',#74162,7.69242172204927);
#18148=CIRCLE('',#74163,7.68866061784442);
#18149=CIRCLE('',#74165,7.68493085519223);
#18150=CIRCLE('',#74166,7.69242164669672);
#18151=CIRCLE('',#74167,7.68866071969335);
#18152=CIRCLE('',#74169,7.68493083532197);
#18153=CIRCLE('',#74170,7.69242155382646);
#18154=CIRCLE('',#74171,7.68866097614275);
#18155=CIRCLE('',#74173,7.68493088965889);
#18156=CIRCLE('',#74174,7.69242155472373);
#18157=CIRCLE('',#74175,7.68866091405694);
#18158=CIRCLE('',#74177,7.68493087532503);
#18159=CIRCLE('',#74178,7.69242155958861);
#18160=CIRCLE('',#74179,7.6886605506081);
#18161=CIRCLE('',#74181,7.68493084729003);
#18162=CIRCLE('',#74182,7.69242157979543);
#18163=CIRCLE('',#74183,7.68866092479545);
#18164=CIRCLE('',#74185,7.68493081256949);
#18165=CIRCLE('',#74186,7.69242124981822);
#18166=CIRCLE('',#74187,7.68866062458902);
#18167=CIRCLE('',#74189,7.68493062347516);
#18168=CIRCLE('',#74190,7.69242159436639);
#18169=CIRCLE('',#74191,7.68866058647684);
#18170=CIRCLE('',#74193,7.68493051543894);
#18171=CIRCLE('',#74194,7.69242137066694);
#18172=CIRCLE('',#74195,7.68866068309314);
#18173=CIRCLE('',#74197,7.68493068209183);
#18174=CIRCLE('',#74198,7.69242157194857);
#18175=CIRCLE('',#74199,7.68866082607717);
#18176=CIRCLE('',#74201,7.68493060370205);
#18177=CIRCLE('',#74202,7.69242145062432);
#18178=CIRCLE('',#74203,7.68866071711247);
#18179=CIRCLE('',#74205,7.68493098747741);
#18180=CIRCLE('',#74206,7.69242140154801);
#18181=CIRCLE('',#74207,7.68866067715954);
#18182=CIRCLE('',#74209,7.68493081669674);
#18183=CIRCLE('',#74210,7.69242147628779);
#18184=CIRCLE('',#74211,7.68866088453931);
#18185=CIRCLE('',#74213,7.6849306078979);
#18186=CIRCLE('',#74214,7.69242158409723);
#18187=CIRCLE('',#74215,7.68866096259156);
#18188=CIRCLE('',#74217,7.68493074117565);
#18189=CIRCLE('',#74218,7.6924217292055);
#18190=CIRCLE('',#74219,7.68866054447294);
#18191=CIRCLE('',#74221,7.68493089689092);
#18192=CIRCLE('',#74222,7.69242137389086);
#18193=CIRCLE('',#74223,7.6886607771901);
#18194=CIRCLE('',#74225,7.68493065069607);
#18195=CIRCLE('',#74226,7.69242148743181);
#18196=CIRCLE('',#74227,7.68866048060024);
#18197=CIRCLE('',#74229,7.68493057949617);
#18198=CIRCLE('',#74230,7.69242134436988);
#18199=CIRCLE('',#74231,7.68866077886559);
#18200=CIRCLE('',#74233,7.68493056970141);
#18201=CIRCLE('',#74234,7.69242169940791);
#18202=CIRCLE('',#74235,7.68866069476782);
#18203=CIRCLE('',#74237,7.68493069136092);
#18204=CIRCLE('',#74238,7.69242165135084);
#18205=CIRCLE('',#74239,7.44726893187504);
#18206=CIRCLE('',#74240,7.44947055337963);
#18207=CIRCLE('',#74241,7.44726922435689);
#18208=CIRCLE('',#74242,7.44947035700538);
#18209=CIRCLE('',#74243,7.44726911447711);
#18210=CIRCLE('',#74244,7.44947024139007);
#18211=CIRCLE('',#74245,7.44726890407395);
#18212=CIRCLE('',#74246,7.44947046676801);
#18213=CIRCLE('',#74247,7.44726901139079);
#18214=CIRCLE('',#74248,7.44947025629349);
#18215=CIRCLE('',#74249,7.44726922475947);
#18216=CIRCLE('',#74250,7.44947040140503);
#18217=CIRCLE('',#74251,7.44726905730899);
#18218=CIRCLE('',#74252,7.44947047782816);
#18219=CIRCLE('',#74253,7.44726918025779);
#18220=CIRCLE('',#74254,7.4494705297753);
#18221=CIRCLE('',#74255,7.44726931950462);
#18222=CIRCLE('',#74256,7.44947031239334);
#18223=CIRCLE('',#74257,7.44726901770317);
#18224=CIRCLE('',#74258,7.44947057242369);
#18225=CIRCLE('',#74259,7.44726903924226);
#18226=CIRCLE('',#74260,7.44947028478251);
#18227=CIRCLE('',#74261,7.44726894258544);
#18228=CIRCLE('',#74262,7.44947038945979);
#18229=CIRCLE('',#74263,7.44726926857445);
#18230=CIRCLE('',#74264,7.44947054644512);
#18231=CIRCLE('',#74265,7.44726916275161);
#18232=CIRCLE('',#74266,7.44947051640123);
#18233=CIRCLE('',#74267,7.44726899142121);
#18234=CIRCLE('',#74268,7.44947023322216);
#18235=CIRCLE('',#74269,7.44726916809674);
#18236=CIRCLE('',#74270,7.4494704560091);
#18237=CIRCLE('',#74271,7.44726925582064);
#18238=CIRCLE('',#74272,7.4494703409082);
#18239=CIRCLE('',#74273,7.44726899307573);
#18240=CIRCLE('',#74274,7.44947038677876);
#18241=CIRCLE('',#74275,7.44726913176375);
#18242=CIRCLE('',#74276,7.44947037014665);
#18243=CIRCLE('',#74277,7.44726906379561);
#18244=CIRCLE('',#74278,7.44947043308436);
#18245=CIRCLE('',#74279,7.44726900882387);
#18246=CIRCLE('',#74280,7.44947053089161);
#18247=CIRCLE('',#74281,7.44726899765228);
#18248=CIRCLE('',#74282,7.44947032882606);
#18249=CIRCLE('',#74283,7.44726896098699);
#18250=CIRCLE('',#74284,7.44947051052289);
#18251=CIRCLE('',#74285,7.44726884235526);
#18252=CIRCLE('',#74286,7.44947035672427);
#18253=CIRCLE('',#74287,7.4472689273175);
#18254=CIRCLE('',#74288,7.44947048644835);
#18255=CIRCLE('',#74289,7.44726899435253);
#18256=CIRCLE('',#74290,7.44947041903508);
#18257=CIRCLE('',#74291,7.44726886787733);
#18258=CIRCLE('',#74292,7.44947031904415);
#18259=CIRCLE('',#74293,7.44726912411596);
#18260=CIRCLE('',#74294,7.44947025413867);
#18261=CIRCLE('',#74295,7.44726903781441);
#18262=CIRCLE('',#74296,7.44947046972415);
#18263=CIRCLE('',#74297,7.44279297622348);
#18264=CIRCLE('',#74298,7.44938663848418);
#18265=CIRCLE('',#74299,7.44279152433174);
#18266=CIRCLE('',#74300,7.44938647943049);
#18267=CIRCLE('',#74301,7.44279186948023);
#18268=CIRCLE('',#74302,7.44938649896905);
#18269=CIRCLE('',#74303,7.44279179346431);
#18270=CIRCLE('',#74304,7.4493867369477);
#18271=CIRCLE('',#74305,7.44279170217027);
#18272=CIRCLE('',#74306,7.44938643383611);
#18273=CIRCLE('',#74307,7.44279175403518);
#18274=CIRCLE('',#74308,7.44938669614748);
#18275=CIRCLE('',#74309,7.44279173998518);
#18276=CIRCLE('',#74310,7.44938644404911);
#18277=CIRCLE('',#74311,7.44279180610017);
#18278=CIRCLE('',#74312,7.44938660521199);
#18279=CIRCLE('',#74313,7.44279157690661);
#18280=CIRCLE('',#74314,7.4493865971617);
#18281=CIRCLE('',#74315,7.44279168044848);
#18282=CIRCLE('',#74316,7.44938664408774);
#18283=CIRCLE('',#74317,7.44279151478295);
#18284=CIRCLE('',#74318,7.44938641050267);
#18285=CIRCLE('',#74319,7.44279159211148);
#18286=CIRCLE('',#74320,7.44938674882838);
#18287=CIRCLE('',#74321,7.44279173978052);
#18288=CIRCLE('',#74322,7.44938664066163);
#18289=CIRCLE('',#74323,7.44279187426533);
#18290=CIRCLE('',#74324,7.44938674154436);
#18291=CIRCLE('',#74325,7.4427917186894);
#18292=CIRCLE('',#74326,7.44938644598291);
#18293=CIRCLE('',#74327,7.44279156987268);
#18294=CIRCLE('',#74328,7.44938669306736);
#18295=CIRCLE('',#74329,7.44279186354848);
#18296=CIRCLE('',#74330,7.44938658334004);
#18297=CIRCLE('',#74331,7.44279172011691);
#18298=CIRCLE('',#74332,7.44938654099507);
#18299=CIRCLE('',#74333,7.44279154487388);
#18300=CIRCLE('',#74334,7.44938643919626);
#18301=CIRCLE('',#74335,7.44279169235632);
#18302=CIRCLE('',#74336,7.44938661848526);
#18303=CIRCLE('',#74337,7.44279153983535);
#18304=CIRCLE('',#74338,7.44938660972236);
#18305=CIRCLE('',#74339,7.44279172819363);
#18306=CIRCLE('',#74340,7.44938649240783);
#18307=CIRCLE('',#74341,7.44279144437215);
#18308=CIRCLE('',#74342,7.44938664563379);
#18309=CIRCLE('',#74343,7.44279157057872);
#18310=CIRCLE('',#74344,7.44938664600317);
#18311=CIRCLE('',#74345,7.44279166161903);
#18312=CIRCLE('',#74346,7.44938664447462);
#18313=CIRCLE('',#74347,7.4427916397829);
#18314=CIRCLE('',#74348,7.44938658372445);
#18315=CIRCLE('',#74349,7.44279157245851);
#18316=CIRCLE('',#74350,7.44938641775037);
#18317=CIRCLE('',#74351,7.44279169699838);
#18318=CIRCLE('',#74352,7.4493867450934);
#18319=CIRCLE('',#74353,7.4427916925524);
#18320=CIRCLE('',#74354,7.44938776348471);
#18321=CIRCLE('',#74355,7.68983511182372);
#18322=CIRCLE('',#74356,7.69301883077793);
#18323=CIRCLE('',#74358,7.68356108711578);
#18324=CIRCLE('',#74359,7.69198153688764);
#18325=CIRCLE('',#74360,7.6898349590935);
#18326=CIRCLE('',#74361,7.69301892560717);
#18327=CIRCLE('',#74363,7.68356157880052);
#18328=CIRCLE('',#74364,7.69198149127838);
#18329=CIRCLE('',#74365,7.68983486095025);
#18330=CIRCLE('',#74366,7.69301873113243);
#18331=CIRCLE('',#74368,7.68356126410177);
#18332=CIRCLE('',#74369,7.69198185871291);
#18333=CIRCLE('',#74370,7.68983498346275);
#18334=CIRCLE('',#74371,7.69301884923081);
#18335=CIRCLE('',#74373,7.68356161321587);
#18336=CIRCLE('',#74374,7.69198163216993);
#18337=CIRCLE('',#74375,7.68983525253744);
#18338=CIRCLE('',#74376,7.69301874197828);
#18339=CIRCLE('',#74378,7.68356149577362);
#18340=CIRCLE('',#74379,7.69198177259241);
#18341=CIRCLE('',#74380,7.6898350821565);
#18342=CIRCLE('',#74381,7.69301890869412);
#18343=CIRCLE('',#74383,7.68356131636576);
#18344=CIRCLE('',#74384,7.69198162591331);
#18345=CIRCLE('',#74385,7.68983508845765);
#18346=CIRCLE('',#74386,7.69301856377739);
#18347=CIRCLE('',#74388,7.68356096635524);
#18348=CIRCLE('',#74389,7.69198148894895);
#18349=CIRCLE('',#74390,7.68983489163653);
#18350=CIRCLE('',#74391,7.69301860717921);
#18351=CIRCLE('',#74393,7.68356109745221);
#18352=CIRCLE('',#74394,7.69198160697471);
#18353=CIRCLE('',#74395,7.68983495320323);
#18354=CIRCLE('',#74396,7.69301872744581);
#18355=CIRCLE('',#74398,7.68356097839941);
#18356=CIRCLE('',#74399,7.69198180730794);
#18357=CIRCLE('',#74400,7.6898348056083);
#18358=CIRCLE('',#74401,7.69301894532186);
#18359=CIRCLE('',#74403,7.68356155537256);
#18360=CIRCLE('',#74404,7.69198154302483);
#18361=CIRCLE('',#74405,7.68983478733256);
#18362=CIRCLE('',#74406,7.69301861129838);
#18363=CIRCLE('',#74408,7.68356132050169);
#18364=CIRCLE('',#74409,7.69198160962373);
#18365=CIRCLE('',#74410,7.6898350635965);
#18366=CIRCLE('',#74411,7.69301869003358);
#18367=CIRCLE('',#74413,7.68356146760216);
#18368=CIRCLE('',#74414,7.69198176950467);
#18369=CIRCLE('',#74415,7.68983514693778);
#18370=CIRCLE('',#74416,7.69301860446202);
#18371=CIRCLE('',#74418,7.68356117230564);
#18372=CIRCLE('',#74419,7.69198166634701);
#18373=CIRCLE('',#74420,7.68983502565558);
#18374=CIRCLE('',#74421,7.69301871453826);
#18375=CIRCLE('',#74423,7.68356136461527);
#18376=CIRCLE('',#74424,7.69198156882603);
#18377=CIRCLE('',#74425,7.68983486471204);
#18378=CIRCLE('',#74426,7.69301880820276);
#18379=CIRCLE('',#74428,7.6835614892657);
#18380=CIRCLE('',#74429,7.69198165345857);
#18381=CIRCLE('',#74430,7.68983489049233);
#18382=CIRCLE('',#74431,7.69301869930148);
#18383=CIRCLE('',#74433,7.68356141591065);
#18384=CIRCLE('',#74434,7.69198155169492);
#18385=CIRCLE('',#74435,7.68983517907979);
#18386=CIRCLE('',#74436,7.69301869436094);
#18387=CIRCLE('',#74438,7.68356149750982);
#18388=CIRCLE('',#74439,7.69198167371507);
#18389=CIRCLE('',#74440,7.68983511391616);
#18390=CIRCLE('',#74441,7.69301879179767);
#18391=CIRCLE('',#74443,7.68356108644306);
#18392=CIRCLE('',#74444,7.69198150436164);
#18393=CIRCLE('',#74445,7.68983479811495);
#18394=CIRCLE('',#74446,7.69301864826701);
#18395=CIRCLE('',#74448,7.68356158149942);
#18396=CIRCLE('',#74449,7.69198163455412);
#18397=CIRCLE('',#74450,7.6898351085822);
#18398=CIRCLE('',#74451,7.69301906315715);
#18399=CIRCLE('',#74452,7.68983488463856);
#18400=CIRCLE('',#74454,7.68356129710826);
#18401=CIRCLE('',#74455,7.69197999153342);
#18402=CIRCLE('',#74456,7.6930185941024);
#18403=CIRCLE('',#74458,7.68983487958893);
#18404=CIRCLE('',#74459,7.68356097068493);
#18405=CIRCLE('',#74460,7.69198183398909);
#18406=CIRCLE('',#74461,7.69301893341851);
#18407=CIRCLE('',#74463,7.68356105584901);
#18408=CIRCLE('',#74464,7.691981635138);
#18409=CIRCLE('',#74465,7.68983492376419);
#18410=CIRCLE('',#74466,7.69301870860216);
#18411=CIRCLE('',#74468,7.68356148397883);
#18412=CIRCLE('',#74469,7.69198173167317);
#18413=CIRCLE('',#74470,7.68983500343551);
#18414=CIRCLE('',#74471,7.69301882102673);
#18415=CIRCLE('',#74473,7.6835618363572);
#18416=CIRCLE('',#74474,7.69198181002405);
#18417=CIRCLE('',#74475,7.68983478848117);
#18418=CIRCLE('',#74476,7.6930186974174);
#18419=CIRCLE('',#74478,7.68356093215567);
#18420=CIRCLE('',#74479,7.69198175834627);
#18421=CIRCLE('',#74480,7.68983498544143);
#18422=CIRCLE('',#74481,7.69301860697724);
#18423=CIRCLE('',#74483,7.68356149559124);
#18424=CIRCLE('',#74484,7.69198186433126);
#18425=CIRCLE('',#74485,7.68983488114589);
#18426=CIRCLE('',#74486,7.69301896558328);
#18427=CIRCLE('',#74488,7.6835614765364);
#18428=CIRCLE('',#74489,7.69198148285223);
#18429=CIRCLE('',#74490,7.68983489375441);
#18430=CIRCLE('',#74492,7.6835617812463);
#18431=CIRCLE('',#74493,7.69198149369972);
#18432=CIRCLE('',#74494,7.69301888026525);
#18433=CIRCLE('',#74495,7.68779224917023);
#18434=CIRCLE('',#74496,7.69298006574425);
#18435=CIRCLE('',#74497,7.68779273536459);
#18436=CIRCLE('',#74499,7.69207574501788);
#18437=CIRCLE('',#74500,7.69213146141502);
#18438=CIRCLE('',#74501,7.69297998710772);
#18439=CIRCLE('',#74502,7.68779251605245);
#18440=CIRCLE('',#74504,7.69207574680839);
#18441=CIRCLE('',#74505,7.69213138451493);
#18442=CIRCLE('',#74506,7.69297998713124);
#18443=CIRCLE('',#74507,7.68779249899382);
#18444=CIRCLE('',#74509,7.69207597534737);
#18445=CIRCLE('',#74510,7.69213128631069);
#18446=CIRCLE('',#74511,7.69297994261074);
#18447=CIRCLE('',#74512,7.68779239378566);
#18448=CIRCLE('',#74514,7.69207570721692);
#18449=CIRCLE('',#74515,7.69213126984507);
#18450=CIRCLE('',#74516,7.69298018311711);
#18451=CIRCLE('',#74517,7.68779224134649);
#18452=CIRCLE('',#74519,7.69207556007882);
#18453=CIRCLE('',#74520,7.69213113842492);
#18454=CIRCLE('',#74521,7.69297969649806);
#18455=CIRCLE('',#74522,7.68779272659023);
#18456=CIRCLE('',#74524,7.69207579966006);
#18457=CIRCLE('',#74525,7.69213110313893);
#18458=CIRCLE('',#74526,7.69297999256842);
#18459=CIRCLE('',#74527,7.68779254733851);
#18460=CIRCLE('',#74529,7.69207587499486);
#18461=CIRCLE('',#74530,7.69213147841857);
#18462=CIRCLE('',#74531,7.69298003584678);
#18463=CIRCLE('',#74532,7.68779243244237);
#18464=CIRCLE('',#74534,7.69207592300941);
#18465=CIRCLE('',#74535,7.69213135839676);
#18466=CIRCLE('',#74536,7.69297963916946);
#18467=CIRCLE('',#74537,7.68779251761288);
#18468=CIRCLE('',#74539,7.69207559530714);
#18469=CIRCLE('',#74540,7.6921311551946);
#18470=CIRCLE('',#74541,7.69297987944067);
#18471=CIRCLE('',#74542,7.68779249007612);
#18472=CIRCLE('',#74544,7.69207589105174);
#18473=CIRCLE('',#74545,7.69213126619558);
#18474=CIRCLE('',#74546,7.6929798488236);
#18475=CIRCLE('',#74547,7.6877924665024);
#18476=CIRCLE('',#74549,7.69207585096444);
#18477=CIRCLE('',#74550,7.69213117664494);
#18478=CIRCLE('',#74551,7.6929799084806);
#18479=CIRCLE('',#74552,7.68779254617694);
#18480=CIRCLE('',#74554,7.69207557938261);
#18481=CIRCLE('',#74555,7.69213141206415);
#18482=CIRCLE('',#74556,7.69298005187903);
#18483=CIRCLE('',#74557,7.68779234786784);
#18484=CIRCLE('',#74559,7.69207555411377);
#18485=CIRCLE('',#74560,7.69213122220794);
#18486=CIRCLE('',#74561,7.69297992931294);
#18487=CIRCLE('',#74562,7.68779235903073);
#18488=CIRCLE('',#74564,7.69207559882269);
#18489=CIRCLE('',#74565,7.69213134942084);
#18490=CIRCLE('',#74566,7.69297972485294);
#18491=CIRCLE('',#74567,7.68779240123187);
#18492=CIRCLE('',#74569,7.69207573005627);
#18493=CIRCLE('',#74570,7.6921314015989);
#18494=CIRCLE('',#74571,7.69297970104874);
#18495=CIRCLE('',#74572,7.68779265551721);
#18496=CIRCLE('',#74574,7.69207589268163);
#18497=CIRCLE('',#74575,7.69213129959809);
#18498=CIRCLE('',#74576,7.69297968668024);
#18499=CIRCLE('',#74577,7.68779250869095);
#18500=CIRCLE('',#74579,7.69207588950927);
#18501=CIRCLE('',#74580,7.69213118506032);
#18502=CIRCLE('',#74581,7.69297988881807);
#18503=CIRCLE('',#74582,7.68779254555987);
#18504=CIRCLE('',#74584,7.69207550114612);
#18505=CIRCLE('',#74585,7.69213140964143);
#18506=CIRCLE('',#74586,7.69297991283635);
#18507=CIRCLE('',#74587,7.68779256256697);
#18508=CIRCLE('',#74589,7.69207573432771);
#18509=CIRCLE('',#74590,7.69213108454268);
#18510=CIRCLE('',#74591,7.69297992164463);
#18511=CIRCLE('',#74592,7.68779246229219);
#18512=CIRCLE('',#74594,7.69207557758637);
#18513=CIRCLE('',#74595,7.69213122910806);
#18514=CIRCLE('',#74596,7.69297951678655);
#18515=CIRCLE('',#74597,7.68779259311327);
#18516=CIRCLE('',#74599,7.6920758095773);
#18517=CIRCLE('',#74600,7.69213132888472);
#18518=CIRCLE('',#74601,7.6929797349126);
#18519=CIRCLE('',#74602,7.68779229636856);
#18520=CIRCLE('',#74604,7.69207562800561);
#18521=CIRCLE('',#74605,7.69213129153528);
#18522=CIRCLE('',#74606,7.692979834602);
#18523=CIRCLE('',#74607,7.68779266377073);
#18524=CIRCLE('',#74609,7.69207580213767);
#18525=CIRCLE('',#74610,7.6921315768473);
#18526=CIRCLE('',#74611,7.6929798230198);
#18527=CIRCLE('',#74612,7.68779254437404);
#18528=CIRCLE('',#74614,7.69207579340574);
#18529=CIRCLE('',#74615,7.69213126647313);
#18530=CIRCLE('',#74616,7.69297986777709);
#18531=CIRCLE('',#74617,7.68779245760159);
#18532=CIRCLE('',#74619,7.69207587460581);
#18533=CIRCLE('',#74620,7.69213107713119);
#18534=CIRCLE('',#74621,7.69297962621885);
#18535=CIRCLE('',#74622,7.68779243327501);
#18536=CIRCLE('',#74624,7.69207575079905);
#18537=CIRCLE('',#74625,7.69213132479969);
#18538=CIRCLE('',#74626,7.69298016664327);
#18539=CIRCLE('',#74627,7.6877923130605);
#18540=CIRCLE('',#74629,7.69207563694128);
#18541=CIRCLE('',#74630,7.69213116149794);
#18542=CIRCLE('',#74632,7.69298010510988);
#18543=CIRCLE('',#74633,7.69207576876764);
#18544=CIRCLE('',#74634,7.69213137879866);
#18545=CIRCLE('',#74635,7.44783641328649);
#18546=CIRCLE('',#74636,7.44783619459759);
#18547=CIRCLE('',#74637,7.44783667431494);
#18548=CIRCLE('',#74638,7.44783648690676);
#18549=CIRCLE('',#74639,7.44783636287797);
#18550=CIRCLE('',#74640,7.44783640046195);
#18551=CIRCLE('',#74641,7.44783629700487);
#18552=CIRCLE('',#74642,7.44783663820312);
#18553=CIRCLE('',#74643,7.4478364715662);
#18554=CIRCLE('',#74644,7.44783642856168);
#18555=CIRCLE('',#74645,7.44783643761439);
#18556=CIRCLE('',#74646,7.44783628905208);
#18557=CIRCLE('',#74647,7.447836548411);
#18558=CIRCLE('',#74648,7.447836498267);
#18559=CIRCLE('',#74649,7.44783622055948);
#18560=CIRCLE('',#74650,7.44783648709306);
#18561=CIRCLE('',#74651,7.44783649023616);
#18562=CIRCLE('',#74652,7.44783617526261);
#18563=CIRCLE('',#74653,7.44783638695771);
#18564=CIRCLE('',#74654,7.44783631507359);
#18565=CIRCLE('',#74655,7.4478362653215);
#18566=CIRCLE('',#74656,7.44783645134482);
#18567=CIRCLE('',#74657,7.44783627824958);
#18568=CIRCLE('',#74658,7.44783626083019);
#18569=CIRCLE('',#74659,7.44783643327715);
#18570=CIRCLE('',#74660,7.44783624465886);
#18571=CIRCLE('',#74661,7.44783631919974);
#18572=CIRCLE('',#74662,7.44783653783281);
#18573=CIRCLE('',#74663,7.44783620529739);
#18574=CIRCLE('',#74664,7.44803384909972);
#18575=CIRCLE('',#74665,7.44913307740183);
#18576=CIRCLE('',#74666,7.44803378567223);
#18577=CIRCLE('',#74667,7.44913310329878);
#18578=CIRCLE('',#74668,7.44803395927175);
#18579=CIRCLE('',#74669,7.44913311974701);
#18580=CIRCLE('',#74670,7.44803383645474);
#18581=CIRCLE('',#74671,7.44913289345156);
#18582=CIRCLE('',#74672,7.44803362260767);
#18583=CIRCLE('',#74673,7.44913288056903);
#18584=CIRCLE('',#74674,7.4480340141458);
#18585=CIRCLE('',#74675,7.4491330132607);
#18586=CIRCLE('',#74676,7.44803385602116);
#18587=CIRCLE('',#74677,7.44913295277711);
#18588=CIRCLE('',#74678,7.44803381421713);
#18589=CIRCLE('',#74679,7.44913281398462);
#18590=CIRCLE('',#74680,7.44803357600266);
#18591=CIRCLE('',#74681,7.44913295928944);
#18592=CIRCLE('',#74682,7.44803372945488);
#18593=CIRCLE('',#74683,7.4491329086292);
#18594=CIRCLE('',#74684,7.44803385612153);
#18595=CIRCLE('',#74685,7.44913287591789);
#18596=CIRCLE('',#74686,7.44803366892573);
#18597=CIRCLE('',#74687,7.44913297852707);
#18598=CIRCLE('',#74688,7.44803375446823);
#18599=CIRCLE('',#74689,7.44913288728968);
#18600=CIRCLE('',#74690,7.44803393218021);
#18601=CIRCLE('',#74691,7.44913297522573);
#18602=CIRCLE('',#74692,7.44803396683527);
#18603=CIRCLE('',#74693,7.44913300336485);
#18604=CIRCLE('',#74694,7.44803398523721);
#18605=CIRCLE('',#74695,7.44913299643533);
#18606=CIRCLE('',#74696,7.44803363076045);
#18607=CIRCLE('',#74697,7.44913306325659);
#18608=CIRCLE('',#74698,7.44803379354534);
#18609=CIRCLE('',#74699,7.44913305942148);
#18610=CIRCLE('',#74700,7.44803356826013);
#18611=CIRCLE('',#74701,7.44913290424177);
#18612=CIRCLE('',#74702,7.44803365409408);
#18613=CIRCLE('',#74703,7.44913280824488);
#18614=CIRCLE('',#74704,7.44803384284203);
#18615=CIRCLE('',#74705,7.44913294744356);
#18616=CIRCLE('',#74706,7.44803374549019);
#18617=CIRCLE('',#74707,7.44913301853901);
#18618=CIRCLE('',#74708,7.448033631895);
#18619=CIRCLE('',#74709,7.44913287088553);
#18620=CIRCLE('',#74710,7.44803395331646);
#18621=CIRCLE('',#74711,7.44913293159264);
#18622=CIRCLE('',#74712,7.44803389776359);
#18623=CIRCLE('',#74713,7.44913287459541);
#18624=CIRCLE('',#74714,7.44803371713281);
#18625=CIRCLE('',#74715,7.44913302945975);
#18626=CIRCLE('',#74716,7.44803360602241);
#18627=CIRCLE('',#74717,7.44913294186345);
#18628=CIRCLE('',#74718,7.44803394375277);
#18629=CIRCLE('',#74719,7.44913289030108);
#18630=CIRCLE('',#74720,7.44803392778243);
#18631=CIRCLE('',#74721,7.44913457387208);
#18632=CIRCLE('',#74722,7.6904915120903);
#18633=CIRCLE('',#74724,7.68602767954961);
#18634=CIRCLE('',#74725,7.68475595845984);
#18635=CIRCLE('',#74726,7.69049164556693);
#18636=CIRCLE('',#74728,7.6860274549623);
#18637=CIRCLE('',#74729,7.68475556041045);
#18638=CIRCLE('',#74730,7.6904914556618);
#18639=CIRCLE('',#74732,7.68602772470303);
#18640=CIRCLE('',#74733,7.68475559025044);
#18641=CIRCLE('',#74734,7.69049175372012);
#18642=CIRCLE('',#74736,7.6860275414872);
#18643=CIRCLE('',#74737,7.68475567016952);
#18644=CIRCLE('',#74738,7.69049157315506);
#18645=CIRCLE('',#74740,7.68602741691704);
#18646=CIRCLE('',#74741,7.68475573644778);
#18647=CIRCLE('',#74742,7.69049155795063);
#18648=CIRCLE('',#74744,7.68602762817755);
#18649=CIRCLE('',#74745,7.68475544644014);
#18650=CIRCLE('',#74746,7.69049170913725);
#18651=CIRCLE('',#74748,7.68602777328572);
#18652=CIRCLE('',#74749,7.68475579598828);
#18653=CIRCLE('',#74750,7.69049144376189);
#18654=CIRCLE('',#74752,7.6860275519339);
#18655=CIRCLE('',#74753,7.6847555903237);
#18656=CIRCLE('',#74754,7.69049150439373);
#18657=CIRCLE('',#74756,7.686027572523);
#18658=CIRCLE('',#74757,7.68475576796661);
#18659=CIRCLE('',#74758,7.69049166867953);
#18660=CIRCLE('',#74760,7.68602749781699);
#18661=CIRCLE('',#74761,7.68475564415941);
#18662=CIRCLE('',#74762,7.69049175623011);
#18663=CIRCLE('',#74764,7.68602768679713);
#18664=CIRCLE('',#74765,7.68475579407389);
#18665=CIRCLE('',#74766,7.6904915982339);
#18666=CIRCLE('',#74768,7.68602761932373);
#18667=CIRCLE('',#74769,7.68475551206412);
#18668=CIRCLE('',#74770,7.69049167739998);
#18669=CIRCLE('',#74772,7.68602773560612);
#18670=CIRCLE('',#74773,7.68475597254698);
#18671=CIRCLE('',#74774,7.69049163908932);
#18672=CIRCLE('',#74776,7.68602763499796);
#18673=CIRCLE('',#74777,7.68475561008889);
#18674=CIRCLE('',#74778,7.6904916039111);
#18675=CIRCLE('',#74780,7.68602777697084);
#18676=CIRCLE('',#74781,7.6847552872152);
#18677=CIRCLE('',#74782,7.69049166011924);
#18678=CIRCLE('',#74784,7.68602740222055);
#18679=CIRCLE('',#74785,7.6847559748612);
#18680=CIRCLE('',#74786,7.69049163611726);
#18681=CIRCLE('',#74788,7.68602755640669);
#18682=CIRCLE('',#74789,7.68475572461281);
#18683=CIRCLE('',#74790,7.69049164231659);
#18684=CIRCLE('',#74792,7.68602794546063);
#18685=CIRCLE('',#74793,7.68475546250343);
#18686=CIRCLE('',#74794,7.69049174506469);
#18687=CIRCLE('',#74796,7.6860275018867);
#18688=CIRCLE('',#74797,7.68475596896432);
#18689=CIRCLE('',#74798,7.69049150169301);
#18690=CIRCLE('',#74800,7.68602755868742);
#18691=CIRCLE('',#74801,7.68475566164481);
#18692=CIRCLE('',#74802,7.69049164829637);
#18693=CIRCLE('',#74804,7.6860277100533);
#18694=CIRCLE('',#74805,7.6847557649482);
#18695=CIRCLE('',#74806,7.69049145756513);
#18696=CIRCLE('',#74808,7.68602763433344);
#18697=CIRCLE('',#74809,7.68475571189682);
#18698=CIRCLE('',#74810,7.69049185304065);
#18699=CIRCLE('',#74812,7.68602765932689);
#18700=CIRCLE('',#74813,7.68475566956354);
#18701=CIRCLE('',#74814,7.69049165343505);
#18702=CIRCLE('',#74816,7.68602771109147);
#18703=CIRCLE('',#74817,7.68475539161365);
#18704=CIRCLE('',#74818,7.69049160121944);
#18705=CIRCLE('',#74820,7.68602760824521);
#18706=CIRCLE('',#74821,7.68475571500764);
#18707=CIRCLE('',#74822,7.6904915211749);
#18708=CIRCLE('',#74824,7.68602780856199);
#18709=CIRCLE('',#74825,7.6847557298162);
#18710=CIRCLE('',#74826,7.69049161397159);
#18711=CIRCLE('',#74828,7.68602759104342);
#18712=CIRCLE('',#74829,7.68475569860617);
#18713=CIRCLE('',#74830,7.69049161093906);
#18714=CIRCLE('',#74832,7.68602750154123);
#18715=CIRCLE('',#74833,7.68475569620964);
#18716=CIRCLE('',#74834,7.69071964350128);
#18717=CIRCLE('',#74835,7.69290937402825);
#18718=CIRCLE('',#74837,7.69247305559261);
#18719=CIRCLE('',#74838,7.68510858657417);
#18720=CIRCLE('',#74839,7.69071931991587);
#18721=CIRCLE('',#74840,7.6929095092742);
#18722=CIRCLE('',#74842,7.69247312683449);
#18723=CIRCLE('',#74843,7.68510841365212);
#18724=CIRCLE('',#74844,7.69071947734155);
#18725=CIRCLE('',#74845,7.69290960887181);
#18726=CIRCLE('',#74847,7.6924732208011);
#18727=CIRCLE('',#74848,7.68510854536878);
#18728=CIRCLE('',#74849,7.69071956256004);
#18729=CIRCLE('',#74850,7.69290939950309);
#18730=CIRCLE('',#74852,7.69247301618986);
#18731=CIRCLE('',#74853,7.68510859125701);
#18732=CIRCLE('',#74854,7.69071941009078);
#18733=CIRCLE('',#74855,7.69290942451445);
#18734=CIRCLE('',#74857,7.69247338976127);
#18735=CIRCLE('',#74858,7.68510814883287);
#18736=CIRCLE('',#74859,7.69071972027508);
#18737=CIRCLE('',#74860,7.69290958457193);
#18738=CIRCLE('',#74862,7.6924731006824);
#18739=CIRCLE('',#74863,7.68510844570157);
#18740=CIRCLE('',#74864,7.69071937182503);
#18741=CIRCLE('',#74865,7.69290951045335);
#18742=CIRCLE('',#74867,7.69247329398241);
#18743=CIRCLE('',#74868,7.68510857658084);
#18744=CIRCLE('',#74869,7.69071926896768);
#18745=CIRCLE('',#74870,7.69290926400206);
#18746=CIRCLE('',#74872,7.692472965827);
#18747=CIRCLE('',#74873,7.68510829632141);
#18748=CIRCLE('',#74874,7.69071976525315);
#18749=CIRCLE('',#74875,7.69290953088483);
#18750=CIRCLE('',#74877,7.69247297613951);
#18751=CIRCLE('',#74878,7.68510844465906);
#18752=CIRCLE('',#74879,7.69071952736592);
#18753=CIRCLE('',#74880,7.69290961078093);
#18754=CIRCLE('',#74882,7.69247336192443);
#18755=CIRCLE('',#74883,7.68510823576118);
#18756=CIRCLE('',#74884,7.69071910488742);
#18757=CIRCLE('',#74885,7.69290954220584);
#18758=CIRCLE('',#74887,7.69247305116375);
#18759=CIRCLE('',#74888,7.68510837553656);
#18760=CIRCLE('',#74889,7.6907197818452);
#18761=CIRCLE('',#74890,7.69290927403745);
#18762=CIRCLE('',#74892,7.6924731485281);
#18763=CIRCLE('',#74893,7.68510832326911);
#18764=CIRCLE('',#74894,7.69071950406307);
#18765=CIRCLE('',#74895,7.69290936631444);
#18766=CIRCLE('',#74897,7.69247307464989);
#18767=CIRCLE('',#74898,7.68510828425941);
#18768=CIRCLE('',#74899,7.69071946216712);
#18769=CIRCLE('',#74900,7.69290941446719);
#18770=CIRCLE('',#74902,7.69247304873191);
#18771=CIRCLE('',#74903,7.6851083560009);
#18772=CIRCLE('',#74904,7.69071926915612);
#18773=CIRCLE('',#74905,7.6929095789677);
#18774=CIRCLE('',#74907,7.69247302612856);
#18775=CIRCLE('',#74908,7.68510835534118);
#18776=CIRCLE('',#74909,7.69071925895707);
#18777=CIRCLE('',#74910,7.69290940858428);
#18778=CIRCLE('',#74912,7.69247308969198);
#18779=CIRCLE('',#74913,7.68510875718082);
#18780=CIRCLE('',#74914,7.69071945745377);
#18781=CIRCLE('',#74915,7.69290954197672);
#18782=CIRCLE('',#74917,7.69247324003157);
#18783=CIRCLE('',#74918,7.68510829808067);
#18784=CIRCLE('',#74919,7.69071947369913);
#18785=CIRCLE('',#74920,7.69290944451111);
#18786=CIRCLE('',#74922,7.69247321275003);
#18787=CIRCLE('',#74923,7.68510855412572);
#18788=CIRCLE('',#74924,7.6907198263024);
#18789=CIRCLE('',#74925,7.69290958609505);
#18790=CIRCLE('',#74927,7.69247307307029);
#18791=CIRCLE('',#74928,7.68510848229127);
#18792=CIRCLE('',#74929,7.69071931272457);
#18793=CIRCLE('',#74930,7.69290934384014);
#18794=CIRCLE('',#74932,7.69247294135857);
#18795=CIRCLE('',#74933,7.68510825693569);
#18796=CIRCLE('',#74934,7.69071969279383);
#18797=CIRCLE('',#74935,7.69290930370595);
#18798=CIRCLE('',#74937,7.69247310846389);
#18799=CIRCLE('',#74938,7.68510846585307);
#18800=CIRCLE('',#74939,7.69071948749216);
#18801=CIRCLE('',#74940,7.69290949403575);
#18802=CIRCLE('',#74942,7.69247315728539);
#18803=CIRCLE('',#74943,7.68510834082781);
#18804=CIRCLE('',#74944,7.69071939997457);
#18805=CIRCLE('',#74945,7.69290952855682);
#18806=CIRCLE('',#74947,7.69247303776945);
#18807=CIRCLE('',#74948,7.68510842071755);
#18808=CIRCLE('',#74949,7.69071963796669);
#18809=CIRCLE('',#74950,7.69290955191827);
#18810=CIRCLE('',#74952,7.69247316177193);
#18811=CIRCLE('',#74953,7.68510871141278);
#18812=CIRCLE('',#74954,7.69071941194508);
#18813=CIRCLE('',#74955,7.69290933842463);
#18814=CIRCLE('',#74957,7.69247308417318);
#18815=CIRCLE('',#74958,7.68510847787708);
#18816=CIRCLE('',#74959,7.69071991530501);
#18817=CIRCLE('',#74960,7.69290952062919);
#18818=CIRCLE('',#74962,7.69247329581856);
#18819=CIRCLE('',#74963,7.68510876545971);
#18820=CIRCLE('',#74964,7.6907197867592);
#18821=CIRCLE('',#74965,7.69290935515063);
#18822=CIRCLE('',#74967,7.69247337609866);
#18823=CIRCLE('',#74968,7.68510850861234);
#18824=CIRCLE('',#74969,7.69071945403784);
#18825=CIRCLE('',#74970,7.69290948998167);
#18826=CIRCLE('',#74972,7.69247313314689);
#18827=CIRCLE('',#74973,7.68510869604205);
#18828=CIRCLE('',#74974,7.69071944059307);
#18829=CIRCLE('',#74975,7.69290947143365);
#18830=CIRCLE('',#74977,7.69247316514867);
#18831=CIRCLE('',#74978,7.68510842022998);
#18832=CIRCLE('',#74979,7.44380002391397);
#18833=CIRCLE('',#74980,7.44379988874145);
#18834=CIRCLE('',#74981,7.44379993329164);
#18835=CIRCLE('',#74982,7.44380010832843);
#18836=CIRCLE('',#74983,7.44379991927684);
#18837=CIRCLE('',#74984,7.44379996464395);
#18838=CIRCLE('',#74985,7.44379988209734);
#18839=CIRCLE('',#74986,7.44380007941013);
#18840=CIRCLE('',#74987,7.44380009743758);
#18841=CIRCLE('',#74988,7.44380000595013);
#18842=CIRCLE('',#74989,7.44380013326231);
#18843=CIRCLE('',#74990,7.44379982184739);
#18844=CIRCLE('',#74991,7.44380001233149);
#18845=CIRCLE('',#74992,7.44379999221544);
#18846=CIRCLE('',#74993,7.44380023882436);
#18847=CIRCLE('',#74994,7.44379986021619);
#18848=CIRCLE('',#74995,7.44380004659804);
#18849=CIRCLE('',#74996,7.443799928756);
#18850=CIRCLE('',#74997,7.44380004662724);
#18851=CIRCLE('',#74998,7.44380011330874);
#18852=CIRCLE('',#74999,7.44379977393382);
#18853=CIRCLE('',#75000,7.44379999983162);
#18854=CIRCLE('',#75001,7.4437998681116);
#18855=CIRCLE('',#75002,7.44379987082435);
#18856=CIRCLE('',#75003,7.44380008391067);
#18857=CIRCLE('',#75004,7.44379991228719);
#18858=CIRCLE('',#75005,7.44380010924942);
#18859=CIRCLE('',#75006,7.44379986338863);
#18860=CIRCLE('',#75007,7.44379982284248);
#18861=CIRCLE('',#75008,7.4484934050301);
#18862=CIRCLE('',#75009,7.44849353356002);
#18863=CIRCLE('',#75010,7.44849326907406);
#18864=CIRCLE('',#75011,7.44849352280214);
#18865=CIRCLE('',#75012,7.44849342827269);
#18866=CIRCLE('',#75013,7.44849355988569);
#18867=CIRCLE('',#75014,7.4484931655973);
#18868=CIRCLE('',#75015,7.44849349295533);
#18869=CIRCLE('',#75016,7.44849326543234);
#18870=CIRCLE('',#75017,7.44849328197373);
#18871=CIRCLE('',#75018,7.44849352929703);
#18872=CIRCLE('',#75019,7.44849369791231);
#18873=CIRCLE('',#75020,7.44849332823307);
#18874=CIRCLE('',#75021,7.44849313701309);
#18875=CIRCLE('',#75022,7.44849327087256);
#18876=CIRCLE('',#75023,7.44849366004089);
#18877=CIRCLE('',#75024,7.44849335581452);
#18878=CIRCLE('',#75025,7.44849343783287);
#18879=CIRCLE('',#75026,7.44849348296527);
#18880=CIRCLE('',#75027,7.44849352337264);
#18881=CIRCLE('',#75028,7.44849316873619);
#18882=CIRCLE('',#75029,7.4484930581785);
#18883=CIRCLE('',#75030,7.44849340237214);
#18884=CIRCLE('',#75031,7.4484933646783);
#18885=CIRCLE('',#75032,7.44849311306844);
#18886=CIRCLE('',#75033,7.44849351728013);
#18887=CIRCLE('',#75034,7.44849339086825);
#18888=CIRCLE('',#75035,7.44849329819119);
#18889=CIRCLE('',#75036,7.44849349744587);
#18890=CIRCLE('',#75037,7.68866066419057);
#18891=CIRCLE('',#75039,7.69242169940883);
#18892=CIRCLE('',#75040,7.68493056987366);
#18893=CIRCLE('',#75041,7.68866083559874);
#18894=CIRCLE('',#75043,7.69242134353274);
#18895=CIRCLE('',#75044,7.68493057966198);
#18896=CIRCLE('',#75045,7.68866052233263);
#18897=CIRCLE('',#75047,7.69242148555441);
#18898=CIRCLE('',#75048,7.6849306508943);
#18899=CIRCLE('',#75049,7.68866073227249);
#18900=CIRCLE('',#75051,7.69242137324144);
#18901=CIRCLE('',#75052,7.68493089713476);
#18902=CIRCLE('',#75053,7.68866055304563);
#18903=CIRCLE('',#75055,7.69242172920828);
#18904=CIRCLE('',#75056,7.68493074123893);
#18905=CIRCLE('',#75057,7.68866094033109);
#18906=CIRCLE('',#75059,7.69242158192493);
#18907=CIRCLE('',#75060,7.68493060823818);
#18908=CIRCLE('',#75061,7.68866085719634);
#18909=CIRCLE('',#75063,7.69242147569298);
#18910=CIRCLE('',#75064,7.68493081691442);
#18911=CIRCLE('',#75065,7.68866062157112);
#18912=CIRCLE('',#75067,7.69242140132481);
#18913=CIRCLE('',#75068,7.68493098751244);
#18914=CIRCLE('',#75069,7.6886606753037);
#18915=CIRCLE('',#75071,7.69242144995276);
#18916=CIRCLE('',#75072,7.68493060396243);
#18917=CIRCLE('',#75073,7.68866084384972);
#18918=CIRCLE('',#75075,7.69242157147528);
#18919=CIRCLE('',#75076,7.6849306822516);
#18920=CIRCLE('',#75077,7.68866063109866);
#18921=CIRCLE('',#75079,7.6924213701606);
#18922=CIRCLE('',#75080,7.68493051561203);
#18923=CIRCLE('',#75081,7.68866059173287);
#18924=CIRCLE('',#75083,7.69242159344046);
#18925=CIRCLE('',#75084,7.68493062385534);
#18926=CIRCLE('',#75085,7.68866063284343);
#18927=CIRCLE('',#75087,7.69242124923371);
#18928=CIRCLE('',#75088,7.68493081278867);
#18929=CIRCLE('',#75089,7.6886608720667);
#18930=CIRCLE('',#75091,7.69242157913419);
#18931=CIRCLE('',#75092,7.68493084754879);
#18932=CIRCLE('',#75093,7.68866055711081);
#18933=CIRCLE('',#75095,7.69242155909154);
#18934=CIRCLE('',#75096,7.68493087550972);
#18935=CIRCLE('',#75097,7.68866089124528);
#18936=CIRCLE('',#75099,7.69242155407184);
#18937=CIRCLE('',#75100,7.6849308899177);
#18938=CIRCLE('',#75101,7.68866092368706);
#18939=CIRCLE('',#75103,7.69242155333496);
#18940=CIRCLE('',#75104,7.68493083551118);
#18941=CIRCLE('',#75105,7.68866067406947);
#18942=CIRCLE('',#75107,7.69242164601768);
#18943=CIRCLE('',#75108,7.68493085548053);
#18944=CIRCLE('',#75109,7.6886606467417);
#18945=CIRCLE('',#75110,7.68866065581878);
#18946=CIRCLE('',#75112,7.69242172154919);
#18947=CIRCLE('',#75113,7.68493083314559);
#18948=CIRCLE('',#75115,7.68866068182422);
#18949=CIRCLE('',#75116,7.69242159733574);
#18950=CIRCLE('',#75117,7.68493077787954);
#18951=CIRCLE('',#75119,7.69242127445083);
#18952=CIRCLE('',#75120,7.68493083815641);
#18953=CIRCLE('',#75121,7.68866066847167);
#18954=CIRCLE('',#75123,7.6924216099892);
#18955=CIRCLE('',#75124,7.68493073504257);
#18956=CIRCLE('',#75125,7.68866096801022);
#18957=CIRCLE('',#75127,7.69242166583259);
#18958=CIRCLE('',#75128,7.68493080608032);
#18959=CIRCLE('',#75129,7.68866070474647);
#18960=CIRCLE('',#75131,7.69242129303047);
#18961=CIRCLE('',#75132,7.68493071252555);
#18962=CIRCLE('',#75133,7.68866043240635);
#18963=CIRCLE('',#75135,7.69242136302723);
#18964=CIRCLE('',#75136,7.68493065757089);
#18965=CIRCLE('',#75137,7.68866061806458);
#18966=CIRCLE('',#75139,7.69242153493746);
#18967=CIRCLE('',#75140,7.68493073461862);
#18968=CIRCLE('',#75141,7.68866080163369);
#18969=CIRCLE('',#75143,7.69242158727534);
#18970=CIRCLE('',#75144,7.68493063280848);
#18971=CIRCLE('',#75145,7.68866076262201);
#18972=CIRCLE('',#75147,7.69242165119922);
#18973=CIRCLE('',#75148,7.68493069139677);
#18974=CIRCLE('',#75149,7.69127081155463);
#18975=CIRCLE('',#75150,7.69127055626591);
#18976=CIRCLE('',#75152,7.6861924517877);
#18977=CIRCLE('',#75153,7.68457503867442);
#18978=CIRCLE('',#75154,7.6912705500939);
#18979=CIRCLE('',#75156,7.68619242340395);
#18980=CIRCLE('',#75157,7.68457492993712);
#18981=CIRCLE('',#75158,7.69127068455703);
#18982=CIRCLE('',#75160,7.68619244919569);
#18983=CIRCLE('',#75161,7.68457463844531);
#18984=CIRCLE('',#75162,7.69127057713307);
#18985=CIRCLE('',#75164,7.68619237618486);
#18986=CIRCLE('',#75165,7.68457487674192);
#18987=CIRCLE('',#75166,7.69127048812816);
#18988=CIRCLE('',#75168,7.68619233802125);
#18989=CIRCLE('',#75169,7.6845748287119);
#18990=CIRCLE('',#75170,7.69127075034649);
#18991=CIRCLE('',#75172,7.68619237967728);
#18992=CIRCLE('',#75173,7.68457479157528);
#18993=CIRCLE('',#75174,7.69127036571813);
#18994=CIRCLE('',#75176,7.68619238988181);
#18995=CIRCLE('',#75177,7.68457461725162);
#18996=CIRCLE('',#75178,7.69127045249863);
#18997=CIRCLE('',#75180,7.68619204829374);
#18998=CIRCLE('',#75181,7.68457453773685);
#18999=CIRCLE('',#75182,7.69127064638078);
#19000=CIRCLE('',#75184,7.68619237600206);
#19001=CIRCLE('',#75185,7.68457478724656);
#19002=CIRCLE('',#75186,7.69127052554701);
#19003=CIRCLE('',#75188,7.68619240585107);
#19004=CIRCLE('',#75189,7.68457487023324);
#19005=CIRCLE('',#75190,7.69127052911353);
#19006=CIRCLE('',#75192,7.68619238696948);
#19007=CIRCLE('',#75193,7.68457496082485);
#19008=CIRCLE('',#75194,7.69127058561488);
#19009=CIRCLE('',#75196,7.68619247930092);
#19010=CIRCLE('',#75197,7.68457506128994);
#19011=CIRCLE('',#75198,7.69127080923463);
#19012=CIRCLE('',#75200,7.68619233888281);
#19013=CIRCLE('',#75201,7.68457463519578);
#19014=CIRCLE('',#75202,7.69127078773471);
#19015=CIRCLE('',#75204,7.68619219935353);
#19016=CIRCLE('',#75205,7.68457470543677);
#19017=CIRCLE('',#75206,7.691270399181);
#19018=CIRCLE('',#75208,7.68619198962228);
#19019=CIRCLE('',#75209,7.68457489833632);
#19020=CIRCLE('',#75210,7.691270688111);
#19021=CIRCLE('',#75212,7.68619233399208);
#19022=CIRCLE('',#75213,7.68457465206514);
#19023=CIRCLE('',#75214,7.69127056208363);
#19024=CIRCLE('',#75216,7.68619215948943);
#19025=CIRCLE('',#75217,7.68457483692094);
#19026=CIRCLE('',#75218,7.6912704118498);
#19027=CIRCLE('',#75220,7.68619216603717);
#19028=CIRCLE('',#75221,7.68457486107603);
#19029=CIRCLE('',#75222,7.69127053799002);
#19030=CIRCLE('',#75224,7.68619226704931);
#19031=CIRCLE('',#75225,7.68457463070158);
#19032=CIRCLE('',#75226,7.69127082549637);
#19033=CIRCLE('',#75228,7.6861921483599);
#19034=CIRCLE('',#75229,7.68457475933392);
#19035=CIRCLE('',#75230,7.69127049467909);
#19036=CIRCLE('',#75232,7.68619245625766);
#19037=CIRCLE('',#75233,7.6845747401418);
#19038=CIRCLE('',#75234,7.69127062955969);
#19039=CIRCLE('',#75236,7.6861923379648);
#19040=CIRCLE('',#75237,7.68457443282951);
#19041=CIRCLE('',#75238,7.69127051810462);
#19042=CIRCLE('',#75240,7.6861922613237);
#19043=CIRCLE('',#75241,7.68457458319326);
#19044=CIRCLE('',#75242,7.6912706708803);
#19045=CIRCLE('',#75244,7.68619213256596);
#19046=CIRCLE('',#75245,7.68457492991314);
#19047=CIRCLE('',#75246,7.69127080600108);
#19048=CIRCLE('',#75248,7.68619218432956);
#19049=CIRCLE('',#75249,7.68457489251587);
#19050=CIRCLE('',#75250,7.69127055889231);
#19051=CIRCLE('',#75252,7.68619230107384);
#19052=CIRCLE('',#75253,7.68457493081918);
#19053=CIRCLE('',#75254,7.69127080456184);
#19054=CIRCLE('',#75256,7.68619211116728);
#19055=CIRCLE('',#75257,7.68457463883207);
#19056=CIRCLE('',#75259,7.68619251400998);
#19057=CIRCLE('',#75260,7.6845748205109);
#19058=CIRCLE('',#75261,7.4427916924565);
#19059=CIRCLE('',#75262,7.44938674509435);
#19060=CIRCLE('',#75263,7.4427916969997);
#19061=CIRCLE('',#75264,7.44938641775046);
#19062=CIRCLE('',#75265,7.44279157245494);
#19063=CIRCLE('',#75266,7.44938658372192);
#19064=CIRCLE('',#75267,7.44279163978452);
#19065=CIRCLE('',#75268,7.44938664447408);
#19066=CIRCLE('',#75269,7.44279166161825);
#19067=CIRCLE('',#75270,7.44938664600266);
#19068=CIRCLE('',#75271,7.4427915705808);
#19069=CIRCLE('',#75272,7.4493866456339);
#19070=CIRCLE('',#75273,7.44279144437261);
#19071=CIRCLE('',#75274,7.44938649240699);
#19072=CIRCLE('',#75275,7.44279172819205);
#19073=CIRCLE('',#75276,7.44938660972169);
#19074=CIRCLE('',#75277,7.44279153983529);
#19075=CIRCLE('',#75278,7.44938661848499);
#19076=CIRCLE('',#75279,7.44279169235746);
#19077=CIRCLE('',#75280,7.4493864391964);
#19078=CIRCLE('',#75281,7.44279154487525);
#19079=CIRCLE('',#75282,7.44938654099421);
#19080=CIRCLE('',#75283,7.44279172011711);
#19081=CIRCLE('',#75284,7.44938658333673);
#19082=CIRCLE('',#75285,7.4427918635513);
#19083=CIRCLE('',#75286,7.44938669306789);
#19084=CIRCLE('',#75287,7.44279156987455);
#19085=CIRCLE('',#75288,7.44938644598266);
#19086=CIRCLE('',#75289,7.44279171868799);
#19087=CIRCLE('',#75290,7.44938674154503);
#19088=CIRCLE('',#75291,7.44279187426517);
#19089=CIRCLE('',#75292,7.44938664065949);
#19090=CIRCLE('',#75293,7.4427917397805);
#19091=CIRCLE('',#75294,7.44938674882648);
#19092=CIRCLE('',#75295,7.44279159211471);
#19093=CIRCLE('',#75296,7.4493864104988);
#19094=CIRCLE('',#75297,7.4427915147825);
#19095=CIRCLE('',#75298,7.44938664409182);
#19096=CIRCLE('',#75299,7.4427916804493);
#19097=CIRCLE('',#75300,7.44938659716179);
#19098=CIRCLE('',#75301,7.44279157690395);
#19099=CIRCLE('',#75302,7.4493866052108);
#19100=CIRCLE('',#75303,7.4427918060999);
#19101=CIRCLE('',#75304,7.44938644404683);
#19102=CIRCLE('',#75305,7.44279173998652);
#19103=CIRCLE('',#75306,7.44938669614659);
#19104=CIRCLE('',#75307,7.44279175403481);
#19105=CIRCLE('',#75308,7.44938643383545);
#19106=CIRCLE('',#75309,7.4427917021702);
#19107=CIRCLE('',#75310,7.44938673694741);
#19108=CIRCLE('',#75311,7.44279179346418);
#19109=CIRCLE('',#75312,7.44938649896921);
#19110=CIRCLE('',#75313,7.44279186948);
#19111=CIRCLE('',#75314,7.44938647943056);
#19112=CIRCLE('',#75315,7.44279152433162);
#19113=CIRCLE('',#75316,7.44938663848424);
#19114=CIRCLE('',#75317,7.44279176344005);
#19115=CIRCLE('',#75318,7.44938662526195);
#19116=CIRCLE('',#75319,7.44244299886662);
#19117=CIRCLE('',#75320,7.44095548421823);
#19118=CIRCLE('',#75321,7.44244298946305);
#19119=CIRCLE('',#75322,7.440954223166);
#19120=CIRCLE('',#75323,7.4424427311987);
#19121=CIRCLE('',#75324,7.44095387434625);
#19122=CIRCLE('',#75325,7.44244277833805);
#19123=CIRCLE('',#75326,7.44095736009521);
#19124=CIRCLE('',#75327,7.44244288256841);
#19125=CIRCLE('',#75328,7.44095752755222);
#19126=CIRCLE('',#75329,7.44244270744006);
#19127=CIRCLE('',#75330,7.44095501712413);
#19128=CIRCLE('',#75331,7.44244304911953);
#19129=CIRCLE('',#75332,7.44095203379445);
#19130=CIRCLE('',#75333,7.44244280952999);
#19131=CIRCLE('',#75334,7.44095769834498);
#19132=CIRCLE('',#75335,7.44244289587029);
#19133=CIRCLE('',#75336,7.44095745023879);
#19134=CIRCLE('',#75337,7.44244302207017);
#19135=CIRCLE('',#75338,7.44095760338765);
#19136=CIRCLE('',#75339,7.44244281563661);
#19137=CIRCLE('',#75340,7.4409577473395);
#19138=CIRCLE('',#75341,7.44244321398108);
#19139=CIRCLE('',#75342,7.44095779132071);
#19140=CIRCLE('',#75343,7.44244315736397);
#19141=CIRCLE('',#75344,7.4409577080112);
#19142=CIRCLE('',#75345,7.44244295675951);
#19143=CIRCLE('',#75346,7.44095736424415);
#19144=CIRCLE('',#75347,7.44244298039767);
#19145=CIRCLE('',#75348,7.44095496920714);
#19146=CIRCLE('',#75349,7.44244271315192);
#19147=CIRCLE('',#75350,7.44095755998995);
#19148=CIRCLE('',#75351,7.44244297307453);
#19149=CIRCLE('',#75352,7.44095766223601);
#19150=CIRCLE('',#75353,7.4424429736192);
#19151=CIRCLE('',#75354,7.440957801943);
#19152=CIRCLE('',#75355,7.44244272416091);
#19153=CIRCLE('',#75356,7.44095740321613);
#19154=CIRCLE('',#75357,7.44244273072479);
#19155=CIRCLE('',#75358,7.44095491418459);
#19156=CIRCLE('',#75359,7.44244311098566);
#19157=CIRCLE('',#75360,7.44095786108218);
#19158=CIRCLE('',#75361,7.44244297361896);
#19159=CIRCLE('',#75362,7.44095570443945);
#19160=CIRCLE('',#75363,7.44244305661406);
#19161=CIRCLE('',#75364,7.44095759956823);
#19162=CIRCLE('',#75365,7.44244283248213);
#19163=CIRCLE('',#75366,7.44095776193031);
#19164=CIRCLE('',#75367,7.44244305468507);
#19165=CIRCLE('',#75368,7.44095754355548);
#19166=CIRCLE('',#75369,7.44244311316591);
#19167=CIRCLE('',#75370,7.4409575180813);
#19168=CIRCLE('',#75371,7.44244309319939);
#19169=CIRCLE('',#75372,7.44095757869953);
#19170=CIRCLE('',#75373,7.44244306799778);
#19171=CIRCLE('',#75374,7.44095769610902);
#19172=CIRCLE('',#75375,7.44244283771634);
#19173=CIRCLE('',#75376,7.44095775953863);
#19174=CIRCLE('',#75377,7.68779987598528);
#19175=CIRCLE('',#75379,7.69213911214462);
#19176=CIRCLE('',#75380,7.6920756369326);
#19177=CIRCLE('',#75381,7.69298007561764);
#19178=CIRCLE('',#75382,7.68780001961496);
#19179=CIRCLE('',#75384,7.69213927835789);
#19180=CIRCLE('',#75385,7.6920757509153);
#19181=CIRCLE('',#75386,7.69297964419018);
#19182=CIRCLE('',#75387,7.68780004212317);
#19183=CIRCLE('',#75389,7.69213902840961);
#19184=CIRCLE('',#75390,7.69207587461716);
#19185=CIRCLE('',#75391,7.69297980034034);
#19186=CIRCLE('',#75392,7.6878001308452);
#19187=CIRCLE('',#75394,7.69213921734648);
#19188=CIRCLE('',#75395,7.69207579361869);
#19189=CIRCLE('',#75396,7.69297983101562);
#19190=CIRCLE('',#75397,7.68780025023278);
#19191=CIRCLE('',#75399,7.69213952883728);
#19192=CIRCLE('',#75400,7.69207580197621);
#19193=CIRCLE('',#75401,7.69297982478878);
#19194=CIRCLE('',#75402,7.68779986441889);
#19195=CIRCLE('',#75404,7.6921392380946);
#19196=CIRCLE('',#75405,7.69207562806071);
#19197=CIRCLE('',#75406,7.69297964858726);
#19198=CIRCLE('',#75407,7.68780017958496);
#19199=CIRCLE('',#75409,7.69213927808702);
#19200=CIRCLE('',#75410,7.69207580973648);
#19201=CIRCLE('',#75411,7.69297955940116);
#19202=CIRCLE('',#75412,7.6878000487883);
#19203=CIRCLE('',#75414,7.69213918193528);
#19204=CIRCLE('',#75415,7.69207557777341);
#19205=CIRCLE('',#75416,7.69297987360811);
#19206=CIRCLE('',#75417,7.68780014906733);
#19207=CIRCLE('',#75419,7.69213903655958);
#19208=CIRCLE('',#75420,7.69207573433436);
#19209=CIRCLE('',#75421,7.69297987702054);
#19210=CIRCLE('',#75422,7.68780012097624);
#19211=CIRCLE('',#75424,7.69213935945283);
#19212=CIRCLE('',#75425,7.69207550113426);
#19213=CIRCLE('',#75426,7.69297981265693);
#19214=CIRCLE('',#75427,7.68780009515455);
#19215=CIRCLE('',#75429,7.69213913633929);
#19216=CIRCLE('',#75430,7.69207588964463);
#19217=CIRCLE('',#75431,7.69297974048077);
#19218=CIRCLE('',#75432,7.6878002419802);
#19219=CIRCLE('',#75434,7.69213925351272);
#19220=CIRCLE('',#75435,7.69207589283663);
#19221=CIRCLE('',#75436,7.69297965290336);
#19222=CIRCLE('',#75437,7.68779998772601);
#19223=CIRCLE('',#75439,7.6921393541975);
#19224=CIRCLE('',#75440,7.6920757304034);
#19225=CIRCLE('',#75441,7.69297967023091);
#19226=CIRCLE('',#75442,7.68779994551434);
#19227=CIRCLE('',#75444,7.69213930088781);
#19228=CIRCLE('',#75445,7.69207559901337);
#19229=CIRCLE('',#75446,7.69297989596743);
#19230=CIRCLE('',#75447,7.68779991185942);
#19231=CIRCLE('',#75449,7.69213917580588);
#19232=CIRCLE('',#75450,7.6920755545249);
#19233=CIRCLE('',#75451,7.69297996142688);
#19234=CIRCLE('',#75452,7.68780013268247);
#19235=CIRCLE('',#75454,7.69213936384868);
#19236=CIRCLE('',#75455,7.69207557960442);
#19237=CIRCLE('',#75456,7.69297986023381);
#19238=CIRCLE('',#75457,7.68780005293755);
#19239=CIRCLE('',#75459,7.69213913010854);
#19240=CIRCLE('',#75460,7.69207585108794);
#19241=CIRCLE('',#75461,7.69297978582869);
#19242=CIRCLE('',#75462,7.68780007656642);
#19243=CIRCLE('',#75464,7.69213921788967);
#19244=CIRCLE('',#75465,7.69207589128317);
#19245=CIRCLE('',#75466,7.69297984684176);
#19246=CIRCLE('',#75467,7.68780010408504);
#19247=CIRCLE('',#75468,7.69298334471343);
#19248=CIRCLE('',#75470,7.69213910727534);
#19249=CIRCLE('',#75471,7.6920757654561);
#19250=CIRCLE('',#75472,7.68779996873446);
#19251=CIRCLE('',#75474,7.69297991901627);
#19252=CIRCLE('',#75475,7.69213930969562);
#19253=CIRCLE('',#75476,7.69207592317019);
#19254=CIRCLE('',#75477,7.68780013382243);
#19255=CIRCLE('',#75479,7.69213942886634);
#19256=CIRCLE('',#75480,7.6920758753375);
#19257=CIRCLE('',#75481,7.69297992907677);
#19258=CIRCLE('',#75482,7.68780029888024);
#19259=CIRCLE('',#75484,7.69213905821546);
#19260=CIRCLE('',#75485,7.69207580074562);
#19261=CIRCLE('',#75486,7.69297961425628);
#19262=CIRCLE('',#75487,7.68779982784028);
#19263=CIRCLE('',#75489,7.69213908924868);
#19264=CIRCLE('',#75490,7.69207556045218);
#19265=CIRCLE('',#75491,7.69298013005251);
#19266=CIRCLE('',#75492,7.68779998030444);
#19267=CIRCLE('',#75494,7.69213921944148);
#19268=CIRCLE('',#75495,7.69207570737084);
#19269=CIRCLE('',#75496,7.69297990621452);
#19270=CIRCLE('',#75497,7.68780008546734);
#19271=CIRCLE('',#75499,7.69213923785092);
#19272=CIRCLE('',#75500,7.69207597549898);
#19273=CIRCLE('',#75501,7.69297993767572);
#19274=CIRCLE('',#75502,7.68780010256743);
#19275=CIRCLE('',#75504,7.69213933368374);
#19276=CIRCLE('',#75505,7.69207574696965);
#19277=CIRCLE('',#75506,7.69297995944248);
#19278=CIRCLE('',#75507,7.68780030910691);
#19279=CIRCLE('',#75509,7.69213941349967);
#19280=CIRCLE('',#75510,7.69207574512427);
#19281=CIRCLE('',#75511,7.69297998602037);
#19282=CIRCLE('',#75512,7.68779983566749);
#19283=CIRCLE('',#75514,7.69213933139663);
#19284=CIRCLE('',#75515,7.69207576875101);
#19285=CIRCLE('',#75516,7.69298010510637);
#19286=CIRCLE('',#75517,7.68749379848418);
#19287=CIRCLE('',#75518,7.68301220936602);
#19288=CIRCLE('',#75520,7.68336765832104);
#19289=CIRCLE('',#75521,7.6919138393445);
#19290=CIRCLE('',#75522,7.68749368284053);
#19291=CIRCLE('',#75523,7.68301221189442);
#19292=CIRCLE('',#75525,7.68336749358452);
#19293=CIRCLE('',#75526,7.69191387505139);
#19294=CIRCLE('',#75527,7.6874936500375);
#19295=CIRCLE('',#75528,7.68301221407298);
#19296=CIRCLE('',#75530,7.68336735652439);
#19297=CIRCLE('',#75531,7.6919140322907);
#19298=CIRCLE('',#75532,7.68749361405354);
#19299=CIRCLE('',#75533,7.68301221215543);
#19300=CIRCLE('',#75535,7.6833673735488);
#19301=CIRCLE('',#75536,7.69191393357619);
#19302=CIRCLE('',#75537,7.6874936404206);
#19303=CIRCLE('',#75538,7.68301221332253);
#19304=CIRCLE('',#75540,7.68336740565764);
#19305=CIRCLE('',#75541,7.69191406168244);
#19306=CIRCLE('',#75542,7.68749365696169);
#19307=CIRCLE('',#75543,7.68301221294907);
#19308=CIRCLE('',#75545,7.68336733055345);
#19309=CIRCLE('',#75546,7.69191418046433);
#19310=CIRCLE('',#75547,7.68749354363047);
#19311=CIRCLE('',#75548,7.68301221095471);
#19312=CIRCLE('',#75550,7.68336738565683);
#19313=CIRCLE('',#75551,7.69191372264169);
#19314=CIRCLE('',#75552,7.68749349224528);
#19315=CIRCLE('',#75553,7.68301221064353);
#19316=CIRCLE('',#75555,7.68336738932367);
#19317=CIRCLE('',#75556,7.69191396675306);
#19318=CIRCLE('',#75557,7.68749348186479);
#19319=CIRCLE('',#75558,7.68301221199004);
#19320=CIRCLE('',#75560,7.68336735043043);
#19321=CIRCLE('',#75561,7.69191399165648);
#19322=CIRCLE('',#75562,7.6874936906741);
#19323=CIRCLE('',#75563,7.6830122101649);
#19324=CIRCLE('',#75565,7.68336749295722);
#19325=CIRCLE('',#75566,7.69191368406498);
#19326=CIRCLE('',#75567,7.68749375958476);
#19327=CIRCLE('',#75568,7.68301221355929);
#19328=CIRCLE('',#75570,7.68336761356554);
#19329=CIRCLE('',#75571,7.69191369346876);
#19330=CIRCLE('',#75572,7.68749349900514);
#19331=CIRCLE('',#75573,7.68301221076865);
#19332=CIRCLE('',#75575,7.68336753179772);
#19333=CIRCLE('',#75576,7.69191383055458);
#19334=CIRCLE('',#75577,7.68749375089716);
#19335=CIRCLE('',#75578,7.68301221150777);
#19336=CIRCLE('',#75580,7.68336747881597);
#19337=CIRCLE('',#75581,7.69191397460675);
#19338=CIRCLE('',#75582,7.68749352075251);
#19339=CIRCLE('',#75583,7.68301221097374);
#19340=CIRCLE('',#75585,7.68336756935006);
#19341=CIRCLE('',#75586,7.69191398566389);
#19342=CIRCLE('',#75587,7.68749364370246);
#19343=CIRCLE('',#75588,7.68301221186137);
#19344=CIRCLE('',#75590,7.68336744364852);
#19345=CIRCLE('',#75591,7.69191378010229);
#19346=CIRCLE('',#75592,7.68749362324088);
#19347=CIRCLE('',#75593,7.68301221420808);
#19348=CIRCLE('',#75595,7.68336717811929);
#19349=CIRCLE('',#75596,7.69191369357022);
#19350=CIRCLE('',#75597,7.68749372241741);
#19351=CIRCLE('',#75598,7.68301221285528);
#19352=CIRCLE('',#75600,7.68336758509296);
#19353=CIRCLE('',#75601,7.69191402168073);
#19354=CIRCLE('',#75602,7.68749342450953);
#19355=CIRCLE('',#75603,7.68301221387731);
#19356=CIRCLE('',#75605,7.68336728225106);
#19357=CIRCLE('',#75606,7.69191373128225);
#19358=CIRCLE('',#75607,7.68749330062709);
#19359=CIRCLE('',#75608,7.68301221092703);
#19360=CIRCLE('',#75610,7.6833673135599);
#19361=CIRCLE('',#75611,7.69191383199074);
#19362=CIRCLE('',#75612,7.68749350532316);
#19363=CIRCLE('',#75613,7.68301220914882);
#19364=CIRCLE('',#75615,7.68336732981034);
#19365=CIRCLE('',#75616,7.69191374607332);
#19366=CIRCLE('',#75617,7.68749344497074);
#19367=CIRCLE('',#75618,7.68301221052208);
#19368=CIRCLE('',#75620,7.68336743835863);
#19369=CIRCLE('',#75621,7.6919136898869);
#19370=CIRCLE('',#75622,7.68749352925105);
#19371=CIRCLE('',#75623,7.6830122108982);
#19372=CIRCLE('',#75625,7.68336749193465);
#19373=CIRCLE('',#75626,7.69191374707215);
#19374=CIRCLE('',#75627,7.68749342834959);
#19375=CIRCLE('',#75628,7.68301221156059);
#19376=CIRCLE('',#75630,7.68336746141577);
#19377=CIRCLE('',#75631,7.69191379733266);
#19378=CIRCLE('',#75632,7.68749361435392);
#19379=CIRCLE('',#75633,7.68301221014136);
#19380=CIRCLE('',#75635,7.68336753222251);
#19381=CIRCLE('',#75636,7.69191372571);
#19382=CIRCLE('',#75637,7.68749381076509);
#19383=CIRCLE('',#75638,7.68301221123153);
#19384=CIRCLE('',#75640,7.68336754629794);
#19385=CIRCLE('',#75641,7.69191383423275);
#19386=CIRCLE('',#75642,7.68749342355177);
#19387=CIRCLE('',#75643,7.68301221354761);
#19388=CIRCLE('',#75645,7.68336748605867);
#19389=CIRCLE('',#75646,7.6919137494078);
#19390=CIRCLE('',#75647,7.68749358233999);
#19391=CIRCLE('',#75648,7.68301221002473);
#19392=CIRCLE('',#75650,7.68336726913135);
#19393=CIRCLE('',#75651,7.69191389093633);
#19394=CIRCLE('',#75652,7.68749376897362);
#19395=CIRCLE('',#75653,7.68301221192537);
#19396=CIRCLE('',#75655,7.68336744990501);
#19397=CIRCLE('',#75656,7.69191370262879);
#19398=CIRCLE('',#75657,7.44803384851454);
#19399=CIRCLE('',#75658,7.44913450462972);
#19400=CIRCLE('',#75659,7.44803398219469);
#19401=CIRCLE('',#75660,7.44913469696842);
#19402=CIRCLE('',#75661,7.44803387896228);
#19403=CIRCLE('',#75662,7.44913455497489);
#19404=CIRCLE('',#75663,7.44803375459079);
#19405=CIRCLE('',#75664,7.44913437189458);
#19406=CIRCLE('',#75665,7.44803357474873);
#19407=CIRCLE('',#75666,7.44913453499902);
#19408=CIRCLE('',#75667,7.44803385001612);
#19409=CIRCLE('',#75668,7.44913451718387);
#19410=CIRCLE('',#75669,7.44803391202732);
#19411=CIRCLE('',#75670,7.44913461578382);
#19412=CIRCLE('',#75671,7.44803360525087);
#19413=CIRCLE('',#75672,7.4491345971037);
#19414=CIRCLE('',#75673,7.44803378927701);
#19415=CIRCLE('',#75674,7.44913432274363);
#19416=CIRCLE('',#75675,7.44803368961488);
#19417=CIRCLE('',#75676,7.44913456568358);
#19418=CIRCLE('',#75677,7.44803365322234);
#19419=CIRCLE('',#75678,7.44913480209481);
#19420=CIRCLE('',#75679,7.44803390829095);
#19421=CIRCLE('',#75680,7.44913460310339);
#19422=CIRCLE('',#75681,7.44803389391838);
#19423=CIRCLE('',#75682,7.44913450509804);
#19424=CIRCLE('',#75683,7.44803392620582);
#19425=CIRCLE('',#75684,7.44913469047441);
#19426=CIRCLE('',#75685,7.44803382347946);
#19427=CIRCLE('',#75686,7.44913463784643);
#19428=CIRCLE('',#75687,7.44803355457882);
#19429=CIRCLE('',#75688,7.44913452161491);
#19430=CIRCLE('',#75689,7.4480337889387);
#19431=CIRCLE('',#75690,7.44913473774987);
#19432=CIRCLE('',#75691,7.448033913198);
#19433=CIRCLE('',#75692,7.44913445044758);
#19434=CIRCLE('',#75693,7.44803397228211);
#19435=CIRCLE('',#75694,7.44913447637274);
#19436=CIRCLE('',#75695,7.44803364060588);
#19437=CIRCLE('',#75696,7.44913448737058);
#19438=CIRCLE('',#75697,7.4480336731345);
#19439=CIRCLE('',#75698,7.44913441547656);
#19440=CIRCLE('',#75699,7.44803395858171);
#19441=CIRCLE('',#75700,7.44913447418484);
#19442=CIRCLE('',#75701,7.44803370781974);
#19443=CIRCLE('',#75702,7.44913452595731);
#19444=CIRCLE('',#75703,7.44803398418143);
#19445=CIRCLE('',#75704,7.44913433288211);
#19446=CIRCLE('',#75705,7.4480338757853);
#19447=CIRCLE('',#75706,7.44913460036394);
#19448=CIRCLE('',#75707,7.44803388492082);
#19449=CIRCLE('',#75708,7.44913465652709);
#19450=CIRCLE('',#75709,7.44803384571758);
#19451=CIRCLE('',#75710,7.44913454636581);
#19452=CIRCLE('',#75711,7.44803400343632);
#19453=CIRCLE('',#75712,7.44913456029597);
#19454=CIRCLE('',#75713,7.44803398483153);
#19455=CIRCLE('',#75714,7.44913457166606);
#19456=CIRCLE('',#75715,7.4413211943494);
#19457=CIRCLE('',#75716,7.44901103064392);
#19458=CIRCLE('',#75717,7.44132095495296);
#19459=CIRCLE('',#75718,7.4490108071008);
#19460=CIRCLE('',#75719,7.44132110146733);
#19461=CIRCLE('',#75720,7.44901084248561);
#19462=CIRCLE('',#75721,7.44132115396875);
#19463=CIRCLE('',#75722,7.4490108478241);
#19464=CIRCLE('',#75723,7.44132088248758);
#19465=CIRCLE('',#75724,7.44901098371057);
#19466=CIRCLE('',#75725,7.44132119244584);
#19467=CIRCLE('',#75726,7.44901084522929);
#19468=CIRCLE('',#75727,7.44132104374616);
#19469=CIRCLE('',#75728,7.4490108674322);
#19470=CIRCLE('',#75729,7.44132094601478);
#19471=CIRCLE('',#75730,7.44901095358382);
#19472=CIRCLE('',#75731,7.44132123695688);
#19473=CIRCLE('',#75732,7.44901100863758);
#19474=CIRCLE('',#75733,7.44132128324603);
#19475=CIRCLE('',#75734,7.44901122973375);
#19476=CIRCLE('',#75735,7.441321102259);
#19477=CIRCLE('',#75736,7.44901091613927);
#19478=CIRCLE('',#75737,7.44132135859951);
#19479=CIRCLE('',#75738,7.44901110309397);
#19480=CIRCLE('',#75739,7.44132112331111);
#19481=CIRCLE('',#75740,7.44901083347829);
#19482=CIRCLE('',#75741,7.44132113658644);
#19483=CIRCLE('',#75742,7.44901114277293);
#19484=CIRCLE('',#75743,7.44132111690915);
#19485=CIRCLE('',#75744,7.44901102648347);
#19486=CIRCLE('',#75745,7.44132120475744);
#19487=CIRCLE('',#75746,7.44901099402831);
#19488=CIRCLE('',#75747,7.44132096463125);
#19489=CIRCLE('',#75748,7.44901083584814);
#19490=CIRCLE('',#75749,7.4413210929216);
#19491=CIRCLE('',#75750,7.4490110982641);
#19492=CIRCLE('',#75751,7.44132132070251);
#19493=CIRCLE('',#75752,7.44901109082903);
#19494=CIRCLE('',#75753,7.44132120601386);
#19495=CIRCLE('',#75754,7.4490109760887);
#19496=CIRCLE('',#75755,7.44132094853748);
#19497=CIRCLE('',#75756,7.44901104573919);
#19498=CIRCLE('',#75757,7.44132133289946);
#19499=CIRCLE('',#75758,7.44901091837957);
#19500=CIRCLE('',#75759,7.44132104242884);
#19501=CIRCLE('',#75760,7.44901110784316);
#19502=CIRCLE('',#75761,7.44132131435686);
#19503=CIRCLE('',#75762,7.44901111063083);
#19504=CIRCLE('',#75763,7.44132116557491);
#19505=CIRCLE('',#75764,7.44901114766872);
#19506=CIRCLE('',#75765,7.44132105308794);
#19507=CIRCLE('',#75766,7.44901111040163);
#19508=CIRCLE('',#75767,7.44132115326213);
#19509=CIRCLE('',#75768,7.44901094168477);
#19510=CIRCLE('',#75769,7.44132132093481);
#19511=CIRCLE('',#75770,7.44901098494123);
#19512=CIRCLE('',#75771,7.44132106569402);
#19513=CIRCLE('',#75772,7.44901109317039);
#19514=CIRCLE('',#75773,7.69071959970527);
#19515=CIRCLE('',#75774,7.69290939170015);
#19516=CIRCLE('',#75776,7.68510869473579);
#19517=CIRCLE('',#75777,7.69247313181522);
#19518=CIRCLE('',#75778,7.69071955964098);
#19519=CIRCLE('',#75779,7.69290924111574);
#19520=CIRCLE('',#75781,7.68510850730758);
#19521=CIRCLE('',#75782,7.69247337495618);
#19522=CIRCLE('',#75783,7.69071987258783);
#19523=CIRCLE('',#75784,7.69290934854507);
#19524=CIRCLE('',#75786,7.68510876399039);
#19525=CIRCLE('',#75787,7.69247329496086);
#19526=CIRCLE('',#75788,7.69071994582592);
#19527=CIRCLE('',#75789,7.69290933421014);
#19528=CIRCLE('',#75791,7.68510847654784);
#19529=CIRCLE('',#75792,7.69247308294324);
#19530=CIRCLE('',#75793,7.69071960871418);
#19531=CIRCLE('',#75794,7.69290940799771);
#19532=CIRCLE('',#75796,7.68510870977505);
#19533=CIRCLE('',#75797,7.69247316111689);
#19534=CIRCLE('',#75798,7.69071969948865);
#19535=CIRCLE('',#75799,7.6929094723082);
#19536=CIRCLE('',#75801,7.68510841922913);
#19537=CIRCLE('',#75802,7.69247303678556);
#19538=CIRCLE('',#75803,7.69071954763419);
#19539=CIRCLE('',#75804,7.69290907104058);
#19540=CIRCLE('',#75806,7.68510846447336);
#19541=CIRCLE('',#75807,7.69247310718083);
#19542=CIRCLE('',#75808,7.69071966170006);
#19543=CIRCLE('',#75809,7.69290922853116);
#19544=CIRCLE('',#75811,7.68510825538929);
#19545=CIRCLE('',#75812,7.69247294051526);
#19546=CIRCLE('',#75813,7.69071939845317);
#19547=CIRCLE('',#75814,7.69290936931524);
#19548=CIRCLE('',#75816,7.68510848083308);
#19549=CIRCLE('',#75817,7.69247307202873);
#19550=CIRCLE('',#75818,7.69071981594158);
#19551=CIRCLE('',#75819,7.6929093391863);
#19552=CIRCLE('',#75821,7.68510855261831);
#19553=CIRCLE('',#75822,7.69247321174325);
#19554=CIRCLE('',#75823,7.69071957035312);
#19555=CIRCLE('',#75824,7.69290951603948);
#19556=CIRCLE('',#75826,7.68510829636783);
#19557=CIRCLE('',#75827,7.69247323943103);
#19558=CIRCLE('',#75828,7.69071963430168);
#19559=CIRCLE('',#75829,7.6929093702572);
#19560=CIRCLE('',#75831,7.68510875562769);
#19561=CIRCLE('',#75832,7.69247308876346);
#19562=CIRCLE('',#75833,7.69071942344645);
#19563=CIRCLE('',#75834,7.69290950832545);
#19564=CIRCLE('',#75836,7.68510835375617);
#19565=CIRCLE('',#75837,7.69247302527313);
#19566=CIRCLE('',#75838,7.69071939950264);
#19567=CIRCLE('',#75839,7.69290936749314);
#19568=CIRCLE('',#75841,7.68510836777632);
#19569=CIRCLE('',#75842,7.69247305611594);
#19570=CIRCLE('',#75843,7.69071961909296);
#19571=CIRCLE('',#75844,7.69290919018266);
#19572=CIRCLE('',#75846,7.68510828270712);
#19573=CIRCLE('',#75847,7.6924730737966);
#19574=CIRCLE('',#75848,7.69071953135699);
#19575=CIRCLE('',#75849,7.69290916339466);
#19576=CIRCLE('',#75851,7.6851083217593);
#19577=CIRCLE('',#75852,7.69247314750845);
#19578=CIRCLE('',#75853,7.69071986907438);
#19579=CIRCLE('',#75854,7.69290953902085);
#19580=CIRCLE('',#75856,7.68510837394138);
#19581=CIRCLE('',#75857,7.69247305034484);
#19582=CIRCLE('',#75858,7.69071930171358);
#19583=CIRCLE('',#75859,7.69290932887283);
#19584=CIRCLE('',#75860,7.69071977715674);
#19585=CIRCLE('',#75862,7.68510823425748);
#19586=CIRCLE('',#75863,7.69247335097436);
#19587=CIRCLE('',#75864,7.69290935866333);
#19588=CIRCLE('',#75866,7.69071979600336);
#19589=CIRCLE('',#75867,7.68510844318284);
#19590=CIRCLE('',#75868,7.69247297516043);
#19591=CIRCLE('',#75869,7.69290922621531);
#19592=CIRCLE('',#75871,7.68510829481802);
#19593=CIRCLE('',#75872,7.69247296501133);
#19594=CIRCLE('',#75873,7.690719430586);
#19595=CIRCLE('',#75874,7.69290943818744);
#19596=CIRCLE('',#75876,7.6851085752498);
#19597=CIRCLE('',#75877,7.69247329305699);
#19598=CIRCLE('',#75878,7.6907195047278);
#19599=CIRCLE('',#75879,7.69290943255748);
#19600=CIRCLE('',#75881,7.6851084444481);
#19601=CIRCLE('',#75882,7.69247310035162);
#19602=CIRCLE('',#75883,7.69071977042907);
#19603=CIRCLE('',#75884,7.6929094119709);
#19604=CIRCLE('',#75886,7.68510814741828);
#19605=CIRCLE('',#75887,7.69247338886281);
#19606=CIRCLE('',#75888,7.69071960333338);
#19607=CIRCLE('',#75889,7.69290924908488);
#19608=CIRCLE('',#75891,7.68510858977449);
#19609=CIRCLE('',#75892,7.69247301517223);
#19610=CIRCLE('',#75893,7.69071961584303);
#19611=CIRCLE('',#75894,7.69290943617607);
#19612=CIRCLE('',#75896,7.68510854394081);
#19613=CIRCLE('',#75897,7.69247321977988);
#19614=CIRCLE('',#75898,7.69071960742313);
#19615=CIRCLE('',#75899,7.69290947518489);
#19616=CIRCLE('',#75901,7.6851084124167);
#19617=CIRCLE('',#75902,7.692473125738);
#19618=CIRCLE('',#75903,7.69071948944326);
#19619=CIRCLE('',#75904,7.69290916341741);
#19620=CIRCLE('',#75906,7.68510858529319);
#19621=CIRCLE('',#75907,7.69247305436387);
#19622=CIRCLE('',#75908,7.69071973580169);
#19623=CIRCLE('',#75910,7.68510842030487);
#19624=CIRCLE('',#75911,7.69247333638098);
#19625=CIRCLE('',#75912,7.69290942736885);
#19626=CIRCLE('',#75913,7.68652125258421);
#19627=CIRCLE('',#75914,7.69282875740582);
#19628=CIRCLE('',#75915,7.68652100331372);
#19629=CIRCLE('',#75917,7.6914667428899);
#19630=CIRCLE('',#75918,7.69259295877942);
#19631=CIRCLE('',#75919,7.6928285833299);
#19632=CIRCLE('',#75920,7.68652127594459);
#19633=CIRCLE('',#75922,7.69146681080176);
#19634=CIRCLE('',#75923,7.69259297862081);
#19635=CIRCLE('',#75924,7.69282843296274);
#19636=CIRCLE('',#75925,7.68652090920759);
#19637=CIRCLE('',#75927,7.69146684910729);
#19638=CIRCLE('',#75928,7.69259297478972);
#19639=CIRCLE('',#75929,7.69282860552218);
#19640=CIRCLE('',#75930,7.68652108293123);
#19641=CIRCLE('',#75932,7.69146686813508);
#19642=CIRCLE('',#75933,7.69259330949854);
#19643=CIRCLE('',#75934,7.69282869815639);
#19644=CIRCLE('',#75935,7.68652074921531);
#19645=CIRCLE('',#75937,7.69146690596385);
#19646=CIRCLE('',#75938,7.69259299948719);
#19647=CIRCLE('',#75939,7.6928286906566);
#19648=CIRCLE('',#75940,7.68652109333483);
#19649=CIRCLE('',#75942,7.69146675750791);
#19650=CIRCLE('',#75943,7.6925931093011);
#19651=CIRCLE('',#75944,7.69282869693757);
#19652=CIRCLE('',#75945,7.68652104364437);
#19653=CIRCLE('',#75947,7.69146695632385);
#19654=CIRCLE('',#75948,7.69259310070212);
#19655=CIRCLE('',#75949,7.69282887352166);
#19656=CIRCLE('',#75950,7.68652108043192);
#19657=CIRCLE('',#75952,7.69146699472229);
#19658=CIRCLE('',#75953,7.69259277764863);
#19659=CIRCLE('',#75954,7.69282890930485);
#19660=CIRCLE('',#75955,7.68652092359468);
#19661=CIRCLE('',#75957,7.69146705541028);
#19662=CIRCLE('',#75958,7.69259296496278);
#19663=CIRCLE('',#75959,7.69282843664662);
#19664=CIRCLE('',#75960,7.68652115719435);
#19665=CIRCLE('',#75962,7.69146673705696);
#19666=CIRCLE('',#75963,7.69259321935627);
#19667=CIRCLE('',#75964,7.69282882471994);
#19668=CIRCLE('',#75965,7.68652064772346);
#19669=CIRCLE('',#75967,7.69146698196332);
#19670=CIRCLE('',#75968,7.69259287177747);
#19671=CIRCLE('',#75969,7.69282868899355);
#19672=CIRCLE('',#75970,7.68652103514881);
#19673=CIRCLE('',#75972,7.69146685569191);
#19674=CIRCLE('',#75973,7.69259309981762);
#19675=CIRCLE('',#75974,7.69282854518402);
#19676=CIRCLE('',#75975,7.68652103954227);
#19677=CIRCLE('',#75977,7.69146694444271);
#19678=CIRCLE('',#75978,7.69259317491516);
#19679=CIRCLE('',#75979,7.69282857118346);
#19680=CIRCLE('',#75980,7.68652091557019);
#19681=CIRCLE('',#75982,7.69146693442679);
#19682=CIRCLE('',#75983,7.69259322507444);
#19683=CIRCLE('',#75984,7.69282862399722);
#19684=CIRCLE('',#75985,7.6865210214333);
#19685=CIRCLE('',#75987,7.69146696851046);
#19686=CIRCLE('',#75988,7.69259302665222);
#19687=CIRCLE('',#75989,7.69282879735318);
#19688=CIRCLE('',#75990,7.68652119183878);
#19689=CIRCLE('',#75992,7.6914669639946);
#19690=CIRCLE('',#75993,7.69259292103988);
#19691=CIRCLE('',#75994,7.69282874450741);
#19692=CIRCLE('',#75995,7.68652105551807);
#19693=CIRCLE('',#75997,7.69146714762904);
#19694=CIRCLE('',#75998,7.69259288284633);
#19695=CIRCLE('',#75999,7.69282866315263);
#19696=CIRCLE('',#76000,7.68652089784828);
#19697=CIRCLE('',#76002,7.69146679082288);
#19698=CIRCLE('',#76003,7.69259284738132);
#19699=CIRCLE('',#76004,7.6928286055099);
#19700=CIRCLE('',#76005,7.68652117428447);
#19701=CIRCLE('',#76007,7.69146687423611);
#19702=CIRCLE('',#76008,7.69259312630066);
#19703=CIRCLE('',#76009,7.69282854762959);
#19704=CIRCLE('',#76010,7.68652091794378);
#19705=CIRCLE('',#76012,7.69146693235952);
#19706=CIRCLE('',#76013,7.69259296419184);
#19707=CIRCLE('',#76014,7.6928286411893);
#19708=CIRCLE('',#76015,7.68652109672698);
#19709=CIRCLE('',#76017,7.69146698605118);
#19710=CIRCLE('',#76018,7.69259315091713);
#19711=CIRCLE('',#76019,7.69282866039554);
#19712=CIRCLE('',#76020,7.68652107644955);
#19713=CIRCLE('',#76022,7.69146698903455);
#19714=CIRCLE('',#76023,7.69259283508703);
#19715=CIRCLE('',#76024,7.69282861894892);
#19716=CIRCLE('',#76025,7.68652105529621);
#19717=CIRCLE('',#76027,7.69146674605424);
#19718=CIRCLE('',#76028,7.69259335565016);
#19719=CIRCLE('',#76029,7.69282853049398);
#19720=CIRCLE('',#76030,7.68652116318974);
#19721=CIRCLE('',#76032,7.69146694427004);
#19722=CIRCLE('',#76033,7.69259292454759);
#19723=CIRCLE('',#76034,7.6928285859662);
#19724=CIRCLE('',#76035,7.68652097175582);
#19725=CIRCLE('',#76037,7.6914667707658);
#19726=CIRCLE('',#76038,7.69259272968989);
#19727=CIRCLE('',#76039,7.69282886046399);
#19728=CIRCLE('',#76040,7.68652116672586);
#19729=CIRCLE('',#76042,7.69146683433244);
#19730=CIRCLE('',#76043,7.69259301880423);
#19731=CIRCLE('',#76044,7.69282879163902);
#19732=CIRCLE('',#76045,7.68652116214323);
#19733=CIRCLE('',#76047,7.69146685349496);
#19734=CIRCLE('',#76048,7.69259288894782);
#19735=CIRCLE('',#76050,7.69282889360003);
#19736=CIRCLE('',#76051,7.69146687684282);
#19737=CIRCLE('',#76052,7.69259298503778);
#19738=CIRCLE('',#76053,7.44849410662996);
#19739=CIRCLE('',#76054,7.44849381909938);
#19740=CIRCLE('',#76055,7.44849352954868);
#19741=CIRCLE('',#76056,7.44849366767847);
#19742=CIRCLE('',#76057,7.44849372412611);
#19743=CIRCLE('',#76058,7.44849351536438);
#19744=CIRCLE('',#76059,7.44849386390378);
#19745=CIRCLE('',#76060,7.44849383559205);
#19746=CIRCLE('',#76061,7.44849362513138);
#19747=CIRCLE('',#76062,7.44849403562714);
#19748=CIRCLE('',#76063,7.44849380156);
#19749=CIRCLE('',#76064,7.44849359869955);
#19750=CIRCLE('',#76065,7.44849353315651);
#19751=CIRCLE('',#76066,7.44849367933962);
#19752=CIRCLE('',#76067,7.44849361815174);
#19753=CIRCLE('',#76068,7.44849354947402);
#19754=CIRCLE('',#76069,7.44849360859411);
#19755=CIRCLE('',#76070,7.44849387443723);
#19756=CIRCLE('',#76071,7.44849384303392);
#19757=CIRCLE('',#76072,7.44849367558001);
#19758=CIRCLE('',#76073,7.4484935470774);
#19759=CIRCLE('',#76074,7.44849384385892);
#19760=CIRCLE('',#76075,7.44849359872572);
#19761=CIRCLE('',#76076,7.44849408646692);
#19762=CIRCLE('',#76077,7.44849355781418);
#19763=CIRCLE('',#76078,7.4484936666066);
#19764=CIRCLE('',#76079,7.44849345259137);
#19765=CIRCLE('',#76080,7.44849356703623);
#19766=CIRCLE('',#76081,7.44849370149879);
#19767=CIRCLE('',#76082,7.44865568659265);
#19768=CIRCLE('',#76083,7.44865937960774);
#19769=CIRCLE('',#76084,7.44865913396485);
#19770=CIRCLE('',#76085,7.44865931568455);
#19771=CIRCLE('',#76086,7.44865925259037);
#19772=CIRCLE('',#76087,7.44865929525452);
#19773=CIRCLE('',#76088,7.44865921080257);
#19774=CIRCLE('',#76089,7.44865955529151);
#19775=CIRCLE('',#76090,7.44865928674846);
#19776=CIRCLE('',#76091,7.44865922499772);
#19777=CIRCLE('',#76092,7.44865931108114);
#19778=CIRCLE('',#76093,7.44865928116721);
#19779=CIRCLE('',#76094,7.44865918721158);
#19780=CIRCLE('',#76095,7.44865919870178);
#19781=CIRCLE('',#76096,7.44865899043498);
#19782=CIRCLE('',#76097,7.4486591905494);
#19783=CIRCLE('',#76098,7.44865927813933);
#19784=CIRCLE('',#76099,7.44865918139085);
#19785=CIRCLE('',#76100,7.44865899005308);
#19786=CIRCLE('',#76101,7.44865934134193);
#19787=CIRCLE('',#76102,7.44865927352978);
#19788=CIRCLE('',#76103,7.44865923002346);
#19789=CIRCLE('',#76104,7.44865948062892);
#19790=CIRCLE('',#76105,7.44865965464616);
#19791=CIRCLE('',#76106,7.44865928521786);
#19792=CIRCLE('',#76107,7.4486594721013);
#19793=CIRCLE('',#76108,7.44865959839951);
#19794=CIRCLE('',#76109,7.44865921433909);
#19795=CIRCLE('',#76110,7.44865908323347);
#19796=CIRCLE('',#76111,7.4486593118649);
#19797=CIRCLE('',#76112,7.44865908538773);
#19798=CIRCLE('',#76113,7.44865921583991);
#19799=CIRCLE('',#76114,7.44865905758467);
#19800=CIRCLE('',#76115,7.44865917327891);
#19801=CIRCLE('',#76116,7.44865915459675);
#19802=CIRCLE('',#76117,7.44865925173067);
#19803=CIRCLE('',#76118,7.44865941707331);
#19804=CIRCLE('',#76119,7.44865926585465);
#19805=CIRCLE('',#76120,7.44865916843667);
#19806=CIRCLE('',#76121,7.44865944335422);
#19807=CIRCLE('',#76122,7.448659413303);
#19808=CIRCLE('',#76123,7.44865942691477);
#19809=CIRCLE('',#76124,7.44865940352853);
#19810=CIRCLE('',#76125,7.44865923760662);
#19811=CIRCLE('',#76126,7.4486589261236);
#19812=CIRCLE('',#76127,7.44865921280821);
#19813=CIRCLE('',#76128,7.44865925297232);
#19814=CIRCLE('',#76129,7.44865925983128);
#19815=CIRCLE('',#76130,7.44865905615583);
#19816=CIRCLE('',#76131,7.44865931020424);
#19817=CIRCLE('',#76132,7.44865920703909);
#19818=CIRCLE('',#76133,7.44865931223064);
#19819=CIRCLE('',#76134,7.44865933486815);
#19820=CIRCLE('',#76135,7.44865945618035);
#19821=CIRCLE('',#76136,7.44865951918199);
#19822=CIRCLE('',#76137,7.44865939903092);
#19823=CIRCLE('',#76138,7.44865894316317);
#19824=CIRCLE('',#76139,7.44865840446174);
#19825=CIRCLE('',#76140,7.69127072586956);
#19826=CIRCLE('',#76142,7.68457460674455);
#19827=CIRCLE('',#76143,7.68619211118041);
#19828=CIRCLE('',#76144,7.69127048035928);
#19829=CIRCLE('',#76146,7.6845748989775);
#19830=CIRCLE('',#76147,7.68619230097393);
#19831=CIRCLE('',#76148,7.69127072734795);
#19832=CIRCLE('',#76150,7.68457486072764);
#19833=CIRCLE('',#76151,7.68619218421117);
#19834=CIRCLE('',#76152,7.69127059228028);
#19835=CIRCLE('',#76154,7.68457489788836);
#19836=CIRCLE('',#76155,7.68619213247947);
#19837=CIRCLE('',#76156,7.69127043945911);
#19838=CIRCLE('',#76158,7.68457455052392);
#19839=CIRCLE('',#76159,7.68619226163088);
#19840=CIRCLE('',#76160,7.69127055095902);
#19841=CIRCLE('',#76162,7.68457440060584);
#19842=CIRCLE('',#76163,7.68619233813979);
#19843=CIRCLE('',#76164,7.69127041614661);
#19844=CIRCLE('',#76166,7.68457470784324);
#19845=CIRCLE('',#76167,7.68619245636635);
#19846=CIRCLE('',#76168,7.69127074694672);
#19847=CIRCLE('',#76170,7.68457472723724);
#19848=CIRCLE('',#76171,7.68619214830769);
#19849=CIRCLE('',#76172,7.6912704594167);
#19850=CIRCLE('',#76174,7.68457459816734);
#19851=CIRCLE('',#76175,7.68619226715557);
#19852=CIRCLE('',#76176,7.69127033329633);
#19853=CIRCLE('',#76178,7.68457482854662);
#19854=CIRCLE('',#76179,7.68619216619574);
#19855=CIRCLE('',#76180,7.69127048343821);
#19856=CIRCLE('',#76182,7.68457480457462);
#19857=CIRCLE('',#76183,7.68619215958249);
#19858=CIRCLE('',#76184,7.69127060962555);
#19859=CIRCLE('',#76186,7.68457461941056);
#19860=CIRCLE('',#76187,7.68619233436519);
#19861=CIRCLE('',#76188,7.69127032053058);
#19862=CIRCLE('',#76190,7.68457486588462);
#19863=CIRCLE('',#76191,7.68619198984053);
#19864=CIRCLE('',#76192,7.6912707090811);
#19865=CIRCLE('',#76194,7.68457467311279);
#19866=CIRCLE('',#76195,7.68619219941248);
#19867=CIRCLE('',#76196,7.69127073069181);
#19868=CIRCLE('',#76198,7.68457460246984);
#19869=CIRCLE('',#76199,7.68619233913455);
#19870=CIRCLE('',#76200,7.69127050692399);
#19871=CIRCLE('',#76202,7.68457502878878);
#19872=CIRCLE('',#76203,7.68619247937977);
#19873=CIRCLE('',#76204,7.69127044695868);
#19874=CIRCLE('',#76206,7.68457492840789);
#19875=CIRCLE('',#76207,7.68619238711067);
#19876=CIRCLE('',#76208,7.69127044714542);
#19877=CIRCLE('',#76210,7.68457483781455);
#19878=CIRCLE('',#76211,7.68619239818768);
#19879=CIRCLE('',#76212,7.6912705679341);
#19880=CIRCLE('',#76214,7.68457475473604);
#19881=CIRCLE('',#76215,7.6861923761129);
#19882=CIRCLE('',#76216,7.69127037387414);
#19883=CIRCLE('',#76218,7.68457450488223);
#19884=CIRCLE('',#76219,7.68619204868803);
#19885=CIRCLE('',#76220,7.69127028712799);
#19886=CIRCLE('',#76222,7.68457458476216);
#19887=CIRCLE('',#76223,7.68619239048162);
#19888=CIRCLE('',#76224,7.6912706719256);
#19889=CIRCLE('',#76226,7.6845747590727);
#19890=CIRCLE('',#76227,7.68619238035232);
#19891=CIRCLE('',#76228,7.69127041025873);
#19892=CIRCLE('',#76230,7.68457479696758);
#19893=CIRCLE('',#76231,7.68619233870747);
#19894=CIRCLE('',#76232,7.69127049859815);
#19895=CIRCLE('',#76234,7.68457484445074);
#19896=CIRCLE('',#76235,7.68619237638544);
#19897=CIRCLE('',#76236,7.69127060614202);
#19898=CIRCLE('',#76238,7.68457460589843);
#19899=CIRCLE('',#76239,7.68619244940214);
#19900=CIRCLE('',#76240,7.69127047150333);
#19901=CIRCLE('',#76242,7.68457489791198);
#19902=CIRCLE('',#76243,7.68619242344552);
#19903=CIRCLE('',#76244,7.69127045407736);
#19904=CIRCLE('',#76246,7.68457500660473);
#19905=CIRCLE('',#76247,7.6861924517686);
#19906=CIRCLE('',#76248,7.6912707330029);
#19907=CIRCLE('',#76250,7.68457466228632);
#19908=CIRCLE('',#76251,7.68619251401022);
#19909=CIRCLE('',#76252,7.69146686787997);
#19910=CIRCLE('',#76254,7.82251840653599);
#19911=CIRCLE('',#76255,7.5);
#19912=CIRCLE('',#76256,7.59069481717915);
#19913=CIRCLE('',#76257,7.69258716744121);
#19914=CIRCLE('',#76259,7.68762526081301);
#19915=CIRCLE('',#76260,7.69302723584648);
#19916=CIRCLE('',#76261,7.6914669335521);
#19917=CIRCLE('',#76263,7.8225175300266);
#19918=CIRCLE('',#76264,7.5);
#19919=CIRCLE('',#76265,7.59069440111666);
#19920=CIRCLE('',#76266,7.69258698386699);
#19921=CIRCLE('',#76268,7.6876252599103);
#19922=CIRCLE('',#76269,7.69302682389199);
#19923=CIRCLE('',#76270,7.69146690421046);
#19924=CIRCLE('',#76272,7.82251875480618);
#19925=CIRCLE('',#76273,7.5);
#19926=CIRCLE('',#76274,7.59069338205172);
#19927=CIRCLE('',#76275,7.69258686333969);
#19928=CIRCLE('',#76277,7.68762525574649);
#19929=CIRCLE('',#76278,7.69302727554353);
#19930=CIRCLE('',#76279,7.69146709488188);
#19931=CIRCLE('',#76281,7.82251728176977);
#19932=CIRCLE('',#76282,7.5);
#19933=CIRCLE('',#76283,7.59069543016537);
#19934=CIRCLE('',#76284,7.69258682496256);
#19935=CIRCLE('',#76286,7.68762526082337);
#19936=CIRCLE('',#76287,7.69302713009884);
#19937=CIRCLE('',#76288,7.69146671807737);
#19938=CIRCLE('',#76290,7.82251832350922);
#19939=CIRCLE('',#76291,7.5);
#19940=CIRCLE('',#76292,7.59069396884935);
#19941=CIRCLE('',#76293,7.69258678977922);
#19942=CIRCLE('',#76295,7.68762526056082);
#19943=CIRCLE('',#76296,7.69302727988512);
#19944=CIRCLE('',#76297,7.69146679685476);
#19945=CIRCLE('',#76299,7.82251933308047);
#19946=CIRCLE('',#76300,7.5);
#19947=CIRCLE('',#76301,7.59069343155577);
#19948=CIRCLE('',#76302,7.69258706872097);
#19949=CIRCLE('',#76304,7.68762525718788);
#19950=CIRCLE('',#76305,7.69302681329328);
#19951=CIRCLE('',#76306,7.69146687729561);
#19952=CIRCLE('',#76308,7.82251862585163);
#19953=CIRCLE('',#76309,7.5);
#19954=CIRCLE('',#76310,7.59069479464637);
#19955=CIRCLE('',#76311,7.6925869064859);
#19956=CIRCLE('',#76313,7.68762525251179);
#19957=CIRCLE('',#76314,7.69302733400162);
#19958=CIRCLE('',#76315,7.69146691743636);
#19959=CIRCLE('',#76317,7.82250967679436);
#19960=CIRCLE('',#76318,7.50000000248332);
#19961=CIRCLE('',#76319,7.59068816853269);
#19962=CIRCLE('',#76320,7.69258709343339);
#19963=CIRCLE('',#76322,7.68762523296301);
#19964=CIRCLE('',#76323,7.6930279875728);
#19965=CIRCLE('',#76324,7.69146692446018);
#19966=CIRCLE('',#76326,7.8225175108103);
#19967=CIRCLE('',#76327,7.49999999940595);
#19968=CIRCLE('',#76328,7.59069378897348);
#19969=CIRCLE('',#76329,7.6925867774697);
#19970=CIRCLE('',#76331,7.68762526045872);
#19971=CIRCLE('',#76332,7.69302685790954);
#19972=CIRCLE('',#76333,7.69146666499951);
#19973=CIRCLE('',#76335,7.8225186365657);
#19974=CIRCLE('',#76336,7.5);
#19975=CIRCLE('',#76337,7.5906952985796);
#19976=CIRCLE('',#76338,7.69258729805551);
#19977=CIRCLE('',#76340,7.68762525347159);
#19978=CIRCLE('',#76341,7.69302718749449);
#19979=CIRCLE('',#76342,7.69146686263873);
#19980=CIRCLE('',#76344,7.82251721175383);
#19981=CIRCLE('',#76345,7.5);
#19982=CIRCLE('',#76346,7.59069451273781);
#19983=CIRCLE('',#76347,7.69258686754086);
#19984=CIRCLE('',#76349,7.68762526096746);
#19985=CIRCLE('',#76350,7.69302674459465);
#19986=CIRCLE('',#76351,7.69146671373895);
#19987=CIRCLE('',#76353,7.82251808428171);
#19988=CIRCLE('',#76354,7.5);
#19989=CIRCLE('',#76355,7.59069374492181);
#19990=CIRCLE('',#76356,7.69258667231221);
#19991=CIRCLE('',#76358,7.68762525764248);
#19992=CIRCLE('',#76359,7.69302694483297);
#19993=CIRCLE('',#76360,7.6914667777091);
#19994=CIRCLE('',#76362,7.82251948114017);
#19995=CIRCLE('',#76363,7.5);
#19996=CIRCLE('',#76364,7.59069550339663);
#19997=CIRCLE('',#76365,7.69258696142463);
#19998=CIRCLE('',#76367,7.68762525340374);
#19999=CIRCLE('',#76368,7.69302753262858);
#20000=CIRCLE('',#76369,7.69146682910809);
#20001=CIRCLE('',#76371,7.82251845684075);
#20002=CIRCLE('',#76372,7.4999999942942);
#20003=CIRCLE('',#76373,7.59069770697273);
#20004=CIRCLE('',#76374,7.69258687256424);
#20005=CIRCLE('',#76376,7.68762525883221);
#20006=CIRCLE('',#76377,7.69302540852278);
#20007=CIRCLE('',#76378,7.69146682537179);
#20008=CIRCLE('',#76380,7.82251740569397);
#20009=CIRCLE('',#76381,7.5);
#20010=CIRCLE('',#76382,7.5906938352263);
#20011=CIRCLE('',#76383,7.69258692758798);
#20012=CIRCLE('',#76385,7.68762526064097);
#20013=CIRCLE('',#76386,7.69302747298765);
#20014=CIRCLE('',#76387,7.69146668182604);
#20015=CIRCLE('',#76389,7.82249259703888);
#20016=CIRCLE('',#76390,7.50000000673024);
#20017=CIRCLE('',#76391,7.59066676519396);
#20018=CIRCLE('',#76392,7.69258690134813);
#20019=CIRCLE('',#76394,7.68762517911986);
#20020=CIRCLE('',#76395,7.69303027347115);
#20021=CIRCLE('',#76396,7.69146681677351);
#20022=CIRCLE('',#76398,7.82252001763851);
#20023=CIRCLE('',#76399,7.5);
#20024=CIRCLE('',#76400,7.5906957203843);
#20025=CIRCLE('',#76401,7.6925869212363);
#20026=CIRCLE('',#76403,7.68762525249949);
#20027=CIRCLE('',#76404,7.69302688449732);
#20028=CIRCLE('',#76405,7.6914667677436);
#20029=CIRCLE('',#76407,7.82251273949175);
#20030=CIRCLE('',#76408,7.50000000064172);
#20031=CIRCLE('',#76409,7.59069442908617);
#20032=CIRCLE('',#76410,7.69258691740677);
#20033=CIRCLE('',#76412,7.68762525458648);
#20034=CIRCLE('',#76413,7.69302693606317);
#20035=CIRCLE('',#76414,7.69146678671437);
#20036=CIRCLE('',#76416,7.8225191103349);
#20037=CIRCLE('',#76417,7.5);
#20038=CIRCLE('',#76418,7.59069367691366);
#20039=CIRCLE('',#76419,7.6925872519601);
#20040=CIRCLE('',#76421,7.68762525742582);
#20041=CIRCLE('',#76422,7.69302681144429);
#20042=CIRCLE('',#76423,7.69146690370976);
#20043=CIRCLE('',#76425,7.82252001537044);
#20044=CIRCLE('',#76426,7.5);
#20045=CIRCLE('',#76427,7.59069563834516);
#20046=CIRCLE('',#76428,7.69258694194281);
#20047=CIRCLE('',#76430,7.68762525324496);
#20048=CIRCLE('',#76431,7.69302701810835);
#20049=CIRCLE('',#76432,7.69146668394716);
#20050=CIRCLE('',#76434,7.8225179891651);
#20051=CIRCLE('',#76435,7.5);
#20052=CIRCLE('',#76436,7.59069461311006);
#20053=CIRCLE('',#76437,7.69258705176433);
#20054=CIRCLE('',#76439,7.68762526126733);
#20055=CIRCLE('',#76440,7.6930269002785);
#20056=CIRCLE('',#76441,7.69146695448782);
#20057=CIRCLE('',#76443,7.82251924419094);
#20058=CIRCLE('',#76444,7.5);
#20059=CIRCLE('',#76445,7.5906956283804);
#20060=CIRCLE('',#76446,7.69258672080425);
#20061=CIRCLE('',#76448,7.68762525373694);
#20062=CIRCLE('',#76449,7.69302738155323);
#20063=CIRCLE('',#76450,7.69146697187919);
#20064=CIRCLE('',#76452,7.82251727378208);
#20065=CIRCLE('',#76453,7.5);
#20066=CIRCLE('',#76454,7.59069479425888);
#20067=CIRCLE('',#76455,7.69258690733685);
#20068=CIRCLE('',#76457,7.68762526044002);
#20069=CIRCLE('',#76458,7.69302754569702);
#20070=CIRCLE('',#76459,7.69146666607425);
#20071=CIRCLE('',#76461,7.59069441948473);
#20072=CIRCLE('',#76462,7.82251798645301);
#20073=CIRCLE('',#76463,7.5);
#20074=CIRCLE('',#76464,7.6925871618964);
#20075=CIRCLE('',#76466,7.68762525885893);
#20076=CIRCLE('',#76467,7.69302665420329);
#20077=CIRCLE('',#76468,7.69146689979605);
#20078=CIRCLE('',#76470,7.82251978501935);
#20079=CIRCLE('',#76471,7.5);
#20080=CIRCLE('',#76472,7.59069590106119);
#20081=CIRCLE('',#76473,7.69258681409144);
#20082=CIRCLE('',#76475,7.6876252550984);
#20083=CIRCLE('',#76476,7.69302724211033);
#20084=CIRCLE('',#76477,7.69146681916298);
#20085=CIRCLE('',#76479,7.82249229350671);
#20086=CIRCLE('',#76480,7.50000000534226);
#20087=CIRCLE('',#76481,7.59067387639011);
#20088=CIRCLE('',#76482,7.69258704209278);
#20089=CIRCLE('',#76484,7.68762520350044);
#20090=CIRCLE('',#76485,7.69302958178729);
#20091=CIRCLE('',#76486,7.69146689253006);
#20092=CIRCLE('',#76488,7.82251865702507);
#20093=CIRCLE('',#76489,7.5);
#20094=CIRCLE('',#76490,7.5906939527085);
#20095=CIRCLE('',#76491,7.69258711727703);
#20096=CIRCLE('',#76493,7.68762525990507);
#20097=CIRCLE('',#76494,7.69302679994652);
#20098=CIRCLE('',#76495,7.69146679484481);
#20099=CIRCLE('',#76497,7.82251964766403);
#20100=CIRCLE('',#76498,7.5);
#20101=CIRCLE('',#76499,7.59069606874455);
#20102=CIRCLE('',#76500,7.6925871115328);
#20103=CIRCLE('',#76502,7.68762525495669);
#20104=CIRCLE('',#76503,7.693027073272);
#20105=CIRCLE('',#76504,7.44244283769794);
#20106=CIRCLE('',#76505,7.44095770943715);
#20107=CIRCLE('',#76506,7.44244306799496);
#20108=CIRCLE('',#76507,7.44095757010981);
#20109=CIRCLE('',#76508,7.44244309319976);
#20110=CIRCLE('',#76509,7.44095742817923);
#20111=CIRCLE('',#76510,7.44244311316663);
#20112=CIRCLE('',#76511,7.44095754355266);
#20113=CIRCLE('',#76512,7.44244305468164);
#20114=CIRCLE('',#76513,7.44095776188464);
#20115=CIRCLE('',#76514,7.44244283248188);
#20116=CIRCLE('',#76515,7.44095758755588);
#20117=CIRCLE('',#76516,7.44244305661218);
#20118=CIRCLE('',#76517,7.44095764658766);
#20119=CIRCLE('',#76518,7.44244297361853);
#20120=CIRCLE('',#76519,7.44095787039397);
#20121=CIRCLE('',#76520,7.44244311098298);
#20122=CIRCLE('',#76521,7.44095785023995);
#20123=CIRCLE('',#76522,7.44244273072371);
#20124=CIRCLE('',#76523,7.4409574148811);
#20125=CIRCLE('',#76524,7.44244272416301);
#20126=CIRCLE('',#76525,7.44095780193666);
#20127=CIRCLE('',#76526,7.44244297361728);
#20128=CIRCLE('',#76527,7.440957610396);
#20129=CIRCLE('',#76528,7.4424429730741);
#20130=CIRCLE('',#76529,7.44095755696898);
#20131=CIRCLE('',#76530,7.44244271315511);
#20132=CIRCLE('',#76531,7.44095776333132);
#20133=CIRCLE('',#76532,7.44244298039844);
#20134=CIRCLE('',#76533,7.44095780334038);
#20135=CIRCLE('',#76534,7.44244295675995);
#20136=CIRCLE('',#76535,7.44095761896929);
#20137=CIRCLE('',#76536,7.44244315736419);
#20138=CIRCLE('',#76537,7.44095780583516);
#20139=CIRCLE('',#76538,7.44244321398115);
#20140=CIRCLE('',#76539,7.44095772672058);
#20141=CIRCLE('',#76540,7.44244281563632);
#20142=CIRCLE('',#76541,7.44095770658529);
#20143=CIRCLE('',#76542,7.44244302207351);
#20144=CIRCLE('',#76543,7.44095746764818);
#20145=CIRCLE('',#76544,7.44244289586982);
#20146=CIRCLE('',#76545,7.44095768094371);
#20147=CIRCLE('',#76546,7.44244280952974);
#20148=CIRCLE('',#76547,7.44095773094304);
#20149=CIRCLE('',#76548,7.4424430491187);
#20150=CIRCLE('',#76549,7.44095767432048);
#20151=CIRCLE('',#76550,7.44244270743924);
#20152=CIRCLE('',#76551,7.44095752751371);
#20153=CIRCLE('',#76552,7.44244288256829);
#20154=CIRCLE('',#76553,7.44095736787357);
#20155=CIRCLE('',#76554,7.44244277833773);
#20156=CIRCLE('',#76555,7.44095751266216);
#20157=CIRCLE('',#76556,7.44244273120023);
#20158=CIRCLE('',#76557,7.44095773230911);
#20159=CIRCLE('',#76558,7.44244298946042);
#20160=CIRCLE('',#76559,7.44095782336618);
#20161=CIRCLE('',#76560,7.44244299886607);
#20162=CIRCLE('',#76561,7.44095775950143);
#20163=CIRCLE('',#76562,7.4490144514855);
#20164=CIRCLE('',#76564,7.44132516904529);
#20165=CIRCLE('',#76565,7.44901473192042);
#20166=CIRCLE('',#76567,7.44132484712343);
#20167=CIRCLE('',#76568,7.44901479614434);
#20168=CIRCLE('',#76570,7.44132482041918);
#20169=CIRCLE('',#76571,7.44901479564489);
#20170=CIRCLE('',#76573,7.44132496027544);
#20171=CIRCLE('',#76574,7.44901507868705);
#20172=CIRCLE('',#76576,7.44132520829404);
#20173=CIRCLE('',#76577,7.44901501492555);
#20174=CIRCLE('',#76579,7.44132488589972);
#20175=CIRCLE('',#76580,7.44901478829298);
#20176=CIRCLE('',#76582,7.44132486965578);
#20177=CIRCLE('',#76583,7.44901473111701);
#20178=CIRCLE('',#76585,7.44132485677684);
#20179=CIRCLE('',#76586,7.44901484613321);
#20180=CIRCLE('',#76588,7.44132500892796);
#20181=CIRCLE('',#76589,7.44901483116979);
#20182=CIRCLE('',#76591,7.44132496353816);
#20183=CIRCLE('',#76592,7.44901486184386);
#20184=CIRCLE('',#76594,7.44132491390273);
#20185=CIRCLE('',#76595,7.44901487890267);
#20186=CIRCLE('',#76597,7.44132504759939);
#20187=CIRCLE('',#76598,7.44901483114893);
#20188=CIRCLE('',#76600,7.44132499108792);
#20189=CIRCLE('',#76601,7.44901499426344);
#20190=CIRCLE('',#76603,7.4413246644582);
#20191=CIRCLE('',#76604,7.44901483808788);
#20192=CIRCLE('',#76606,7.44132492098853);
#20193=CIRCLE('',#76607,7.44901479349699);
#20194=CIRCLE('',#76609,7.44132509181846);
#20195=CIRCLE('',#76610,7.44901473074534);
#20196=CIRCLE('',#76612,7.44132489601627);
#20197=CIRCLE('',#76613,7.44901472236486);
#20198=CIRCLE('',#76615,7.44132507039419);
#20199=CIRCLE('',#76616,7.44901483480963);
#20200=CIRCLE('',#76618,7.44132469514174);
#20201=CIRCLE('',#76619,7.44901479709459);
#20202=CIRCLE('',#76621,7.44132504572367);
#20203=CIRCLE('',#76622,7.44901468721301);
#20204=CIRCLE('',#76624,7.44132502969007);
#20205=CIRCLE('',#76625,7.44901473934094);
#20206=CIRCLE('',#76627,7.44132472221971);
#20207=CIRCLE('',#76628,7.44901475240328);
#20208=CIRCLE('',#76630,7.44132510783735);
#20209=CIRCLE('',#76631,7.44901479470681);
#20210=CIRCLE('',#76633,7.4413250143831);
#20211=CIRCLE('',#76634,7.44901503648164);
#20212=CIRCLE('',#76636,7.44132470383829);
#20213=CIRCLE('',#76637,7.44901468881883);
#20214=CIRCLE('',#76639,7.44132501660734);
#20215=CIRCLE('',#76640,7.44901508212225);
#20216=CIRCLE('',#76642,7.44132490803545);
#20217=CIRCLE('',#76643,7.4490147610041);
#20218=CIRCLE('',#76645,7.44132506641251);
#20219=CIRCLE('',#76646,7.44901494283557);
#20220=CIRCLE('',#76648,7.44132440239759);
#20221=CIRCLE('',#76649,7.68749376892044);
#20222=CIRCLE('',#76650,7.68301219198009);
#20223=CIRCLE('',#76652,7.69191389092581);
#20224=CIRCLE('',#76653,7.68336726913004);
#20225=CIRCLE('',#76654,7.68749358218551);
#20226=CIRCLE('',#76655,7.68301219563752);
#20227=CIRCLE('',#76657,7.69191374939714);
#20228=CIRCLE('',#76658,7.68336748606017);
#20229=CIRCLE('',#76659,7.68749342341548);
#20230=CIRCLE('',#76660,7.6830121930893);
#20231=CIRCLE('',#76662,7.69191383422036);
#20232=CIRCLE('',#76663,7.6833675462965);
#20233=CIRCLE('',#76664,7.68749355836631);
#20234=CIRCLE('',#76665,7.68301219225916);
#20235=CIRCLE('',#76667,7.69191372570169);
#20236=CIRCLE('',#76668,7.68336753222351);
#20237=CIRCLE('',#76669,7.68749361423602);
#20238=CIRCLE('',#76670,7.68301219362676);
#20239=CIRCLE('',#76672,7.69191379732158);
#20240=CIRCLE('',#76673,7.68336746141775);
#20241=CIRCLE('',#76674,7.68749342824239);
#20242=CIRCLE('',#76675,7.68301219329349);
#20243=CIRCLE('',#76677,7.69191374706803);
#20244=CIRCLE('',#76678,7.68336749193853);
#20245=CIRCLE('',#76679,7.68749352909174);
#20246=CIRCLE('',#76680,7.68301219252271);
#20247=CIRCLE('',#76682,7.69191368987804);
#20248=CIRCLE('',#76683,7.68336743836054);
#20249=CIRCLE('',#76684,7.68749344500409);
#20250=CIRCLE('',#76685,7.68301219123024);
#20251=CIRCLE('',#76687,7.69191374606969);
#20252=CIRCLE('',#76688,7.68336732981191);
#20253=CIRCLE('',#76689,7.68749350523767);
#20254=CIRCLE('',#76690,7.68301219285518);
#20255=CIRCLE('',#76692,7.6919138319802);
#20256=CIRCLE('',#76693,7.68336731355951);
#20257=CIRCLE('',#76694,7.68749330057477);
#20258=CIRCLE('',#76695,7.68301219615952);
#20259=CIRCLE('',#76697,7.69191373127678);
#20260=CIRCLE('',#76698,7.68336728225312);
#20261=CIRCLE('',#76699,7.68749342441889);
#20262=CIRCLE('',#76700,7.68301219484171);
#20263=CIRCLE('',#76702,7.69191402167153);
#20264=CIRCLE('',#76703,7.68336758509357);
#20265=CIRCLE('',#76704,7.6874937223061);
#20266=CIRCLE('',#76705,7.68301219642771);
#20267=CIRCLE('',#76707,7.69191369356068);
#20268=CIRCLE('',#76708,7.68336717812141);
#20269=CIRCLE('',#76709,7.68749362319715);
#20270=CIRCLE('',#76710,7.68301219414976);
#20271=CIRCLE('',#76712,7.69191378009799);
#20272=CIRCLE('',#76713,7.68336744364646);
#20273=CIRCLE('',#76714,7.68749364365068);
#20274=CIRCLE('',#76715,7.68301219269508);
#20275=CIRCLE('',#76717,7.69191398565423);
#20276=CIRCLE('',#76718,7.6833675693493);
#20277=CIRCLE('',#76719,7.68749352067635);
#20278=CIRCLE('',#76720,7.68301219368827);
#20279=CIRCLE('',#76722,7.69191397459453);
#20280=CIRCLE('',#76723,7.68336747881971);
#20281=CIRCLE('',#76724,7.687493750851);
#20282=CIRCLE('',#76725,7.68301219327867);
#20283=CIRCLE('',#76727,7.6919138305455);
#20284=CIRCLE('',#76728,7.6833675318038);
#20285=CIRCLE('',#76729,7.6874934988961);
#20286=CIRCLE('',#76730,7.68301217777242);
#20287=CIRCLE('',#76731,7.68748726252765);
#20288=CIRCLE('',#76733,7.69191369346136);
#20289=CIRCLE('',#76734,7.68336107784681);
#20290=CIRCLE('',#76735,7.68301219232485);
#20291=CIRCLE('',#76737,7.68749369060519);
#20292=CIRCLE('',#76738,7.69191368405268);
#20293=CIRCLE('',#76739,7.68336749296103);
#20294=CIRCLE('',#76740,7.68301219423829);
#20295=CIRCLE('',#76742,7.69191399164696);
#20296=CIRCLE('',#76743,7.68336735042955);
#20297=CIRCLE('',#76744,7.68749348176495);
#20298=CIRCLE('',#76745,7.68301219268255);
#20299=CIRCLE('',#76747,7.69191396674004);
#20300=CIRCLE('',#76748,7.68336738932368);
#20301=CIRCLE('',#76749,7.6874934921015);
#20302=CIRCLE('',#76750,7.68301219326198);
#20303=CIRCLE('',#76752,7.69191372263682);
#20304=CIRCLE('',#76753,7.68336738565898);
#20305=CIRCLE('',#76754,7.68749354355261);
#20306=CIRCLE('',#76755,7.68301219519444);
#20307=CIRCLE('',#76757,7.69191418045274);
#20308=CIRCLE('',#76758,7.68336733055388);
#20309=CIRCLE('',#76759,7.68749365685344);
#20310=CIRCLE('',#76760,7.68301219552715);
#20311=CIRCLE('',#76762,7.69191406167057);
#20312=CIRCLE('',#76763,7.68336740565433);
#20313=CIRCLE('',#76764,7.68749364032046);
#20314=CIRCLE('',#76765,7.68301219454201);
#20315=CIRCLE('',#76767,7.69191393356503);
#20316=CIRCLE('',#76768,7.68336737355074);
#20317=CIRCLE('',#76769,7.68749361389151);
#20318=CIRCLE('',#76770,7.6830121964021);
#20319=CIRCLE('',#76772,7.6919140322792);
#20320=CIRCLE('',#76773,7.68336735652281);
#20321=CIRCLE('',#76774,7.68749364999818);
#20322=CIRCLE('',#76775,7.68301219423073);
#20323=CIRCLE('',#76777,7.6919138750408);
#20324=CIRCLE('',#76778,7.68336749358252);
#20325=CIRCLE('',#76779,7.687493682695);
#20326=CIRCLE('',#76780,7.6830121913286);
#20327=CIRCLE('',#76782,7.69191383933637);
#20328=CIRCLE('',#76783,7.68336765832302);
#20329=CIRCLE('',#76784,7.68749379841072);
#20330=CIRCLE('',#76786,7.6919137026217);
#20331=CIRCLE('',#76787,7.68336744990483);
#20332=CIRCLE('',#76788,7.68301219395284);
#20333=CIRCLE('',#76816,7.44132107797583);
#20334=CIRCLE('',#76817,7.44901098494131);
#20335=CIRCLE('',#76818,7.44132132093448);
#20336=CIRCLE('',#76819,7.44901094168559);
#20337=CIRCLE('',#76820,7.44132115326169);
#20338=CIRCLE('',#76821,7.44901111040069);
#20339=CIRCLE('',#76822,7.4413210530835);
#20340=CIRCLE('',#76823,7.44901114767026);
#20341=CIRCLE('',#76824,7.44132116557519);
#20342=CIRCLE('',#76825,7.44901111062852);
#20343=CIRCLE('',#76826,7.4413213143581);
#20344=CIRCLE('',#76827,7.44901110784486);
#20345=CIRCLE('',#76828,7.44132104242765);
#20346=CIRCLE('',#76829,7.44901091837715);
#20347=CIRCLE('',#76830,7.44132133289912);
#20348=CIRCLE('',#76831,7.44901104574036);
#20349=CIRCLE('',#76832,7.44132094853763);
#20350=CIRCLE('',#76833,7.44901097608923);
#20351=CIRCLE('',#76834,7.44132120601532);
#20352=CIRCLE('',#76835,7.44901109082872);
#20353=CIRCLE('',#76836,7.44132132070303);
#20354=CIRCLE('',#76837,7.44901109826273);
#20355=CIRCLE('',#76838,7.44132109292228);
#20356=CIRCLE('',#76839,7.44901083584621);
#20357=CIRCLE('',#76840,7.44132096463299);
#20358=CIRCLE('',#76841,7.44901099402833);
#20359=CIRCLE('',#76842,7.4413212047583);
#20360=CIRCLE('',#76843,7.44901102648147);
#20361=CIRCLE('',#76844,7.44132111690801);
#20362=CIRCLE('',#76845,7.44901114277106);
#20363=CIRCLE('',#76846,7.44132113658756);
#20364=CIRCLE('',#76847,7.44901083347679);
#20365=CIRCLE('',#76848,7.44132112331147);
#20366=CIRCLE('',#76849,7.44901110309528);
#20367=CIRCLE('',#76850,7.44132135859989);
#20368=CIRCLE('',#76851,7.44901091613842);
#20369=CIRCLE('',#76852,7.44132110226029);
#20370=CIRCLE('',#76853,7.44901122973458);
#20371=CIRCLE('',#76854,7.44132128324485);
#20372=CIRCLE('',#76855,7.44901100863801);
#20373=CIRCLE('',#76856,7.44132123695719);
#20374=CIRCLE('',#76857,7.44901095358546);
#20375=CIRCLE('',#76858,7.44132094601733);
#20376=CIRCLE('',#76859,7.44901086743548);
#20377=CIRCLE('',#76860,7.44132104374503);
#20378=CIRCLE('',#76861,7.44901084522942);
#20379=CIRCLE('',#76862,7.44132119244628);
#20380=CIRCLE('',#76863,7.4490109837086);
#20381=CIRCLE('',#76864,7.44132088248784);
#20382=CIRCLE('',#76865,7.44901084782327);
#20383=CIRCLE('',#76866,7.44132115396878);
#20384=CIRCLE('',#76867,7.4490108424845);
#20385=CIRCLE('',#76868,7.44132110146778);
#20386=CIRCLE('',#76869,7.44901080710049);
#20387=CIRCLE('',#76870,7.4413209549527);
#20388=CIRCLE('',#76871,7.4490110306471);
#20389=CIRCLE('',#76872,7.44132119434995);
#20390=CIRCLE('',#76873,7.4490110973393);
#20391=CIRCLE('',#76874,7.44096163290917);
#20392=CIRCLE('',#76875,7.44244523922687);
#20393=CIRCLE('',#76876,7.44096407826071);
#20394=CIRCLE('',#76877,7.44244536654789);
#20395=CIRCLE('',#76878,7.44096431502101);
#20396=CIRCLE('',#76879,7.44244539029637);
#20397=CIRCLE('',#76880,7.44096110369019);
#20398=CIRCLE('',#76881,7.44244518327569);
#20399=CIRCLE('',#76882,7.44096431779229);
#20400=CIRCLE('',#76883,7.44244519836295);
#20401=CIRCLE('',#76884,7.44096158135734);
#20402=CIRCLE('',#76885,7.44244549869616);
#20403=CIRCLE('',#76886,7.44096453896483);
#20404=CIRCLE('',#76887,7.44244541427963);
#20405=CIRCLE('',#76888,7.44096231054569);
#20406=CIRCLE('',#76889,7.44244541753372);
#20407=CIRCLE('',#76890,7.44096437264636);
#20408=CIRCLE('',#76891,7.4424453223831);
#20409=CIRCLE('',#76892,7.44096446338278);
#20410=CIRCLE('',#76893,7.44244557095827);
#20411=CIRCLE('',#76894,7.44096277132953);
#20412=CIRCLE('',#76895,7.44244557551138);
#20413=CIRCLE('',#76896,7.44096431516055);
#20414=CIRCLE('',#76897,7.44244547318913);
#20415=CIRCLE('',#76898,7.44096446933956);
#20416=CIRCLE('',#76899,7.44244540321972);
#20417=CIRCLE('',#76900,7.44096428290229);
#20418=CIRCLE('',#76901,7.44244515431675);
#20419=CIRCLE('',#76902,7.44096420555444);
#20420=CIRCLE('',#76903,7.44244556754339);
#20421=CIRCLE('',#76904,7.44096234565355);
#20422=CIRCLE('',#76905,7.44244540483046);
#20423=CIRCLE('',#76906,7.44096082293892);
#20424=CIRCLE('',#76907,7.44244512639587);
#20425=CIRCLE('',#76908,7.44096039470945);
#20426=CIRCLE('',#76909,7.4424450755022);
#20427=CIRCLE('',#76910,7.44096406266067);
#20428=CIRCLE('',#76911,7.44244522712707);
#20429=CIRCLE('',#76912,7.44096433481613);
#20430=CIRCLE('',#76913,7.4424452051413);
#20431=CIRCLE('',#76914,7.44096156994441);
#20432=CIRCLE('',#76915,7.44244537053809);
#20433=CIRCLE('',#76916,7.44095843279229);
#20434=CIRCLE('',#76917,7.44244517593898);
#20435=CIRCLE('',#76918,7.44096426134897);
#20436=CIRCLE('',#76919,7.44244529727346);
#20437=CIRCLE('',#76920,7.44096403234586);
#20438=CIRCLE('',#76921,7.44244532704227);
#20439=CIRCLE('',#76922,7.44096419576632);
#20440=CIRCLE('',#76923,7.44244508418218);
#20441=CIRCLE('',#76924,7.44096433950973);
#20442=CIRCLE('',#76925,7.44244551802685);
#20443=CIRCLE('',#76926,7.44096450056671);
#20444=CIRCLE('',#76927,7.44244556495398);
#20445=CIRCLE('',#76928,7.44096417004577);
#20446=CIRCLE('',#76929,7.44244524080392);
#20447=CIRCLE('',#76930,7.44096030726756);
#20448=CIRCLE('',#76931,7.44243697652006);
#20449=CIRCLE('',#76932,7.6865219858248);
#20450=CIRCLE('',#76934,7.69259356655966);
#20451=CIRCLE('',#76935,7.69146685349983);
#20452=CIRCLE('',#76936,7.69282882739483);
#20453=CIRCLE('',#76937,7.68652199057024);
#20454=CIRCLE('',#76939,7.69259369657614);
#20455=CIRCLE('',#76940,7.69146683430398);
#20456=CIRCLE('',#76941,7.69282880669103);
#20457=CIRCLE('',#76942,7.68652179559924);
#20458=CIRCLE('',#76944,7.69259340746021);
#20459=CIRCLE('',#76945,7.691466770726);
#20460=CIRCLE('',#76946,7.69282855100629);
#20461=CIRCLE('',#76947,7.68652198594906);
#20462=CIRCLE('',#76949,7.69259360268407);
#20463=CIRCLE('',#76950,7.69146694460064);
#20464=CIRCLE('',#76951,7.69282855102511);
#20465=CIRCLE('',#76952,7.6865218785945);
#20466=CIRCLE('',#76954,7.69259403322546);
#20467=CIRCLE('',#76955,7.691466746238);
#20468=CIRCLE('',#76956,7.69282867576847);
#20469=CIRCLE('',#76957,7.68652189966966);
#20470=CIRCLE('',#76959,7.69259351263286);
#20471=CIRCLE('',#76960,7.69146698897258);
#20472=CIRCLE('',#76961,7.69282864997746);
#20473=CIRCLE('',#76962,7.68652192033685);
#20474=CIRCLE('',#76964,7.69259382860018);
#20475=CIRCLE('',#76965,7.69146698613297);
#20476=CIRCLE('',#76966,7.6928286936219);
#20477=CIRCLE('',#76967,7.68652172845389);
#20478=CIRCLE('',#76969,7.69259364164714);
#20479=CIRCLE('',#76970,7.69146693267229);
#20480=CIRCLE('',#76971,7.69282862604479);
#20481=CIRCLE('',#76972,7.68652199760421);
#20482=CIRCLE('',#76974,7.69259380387986);
#20483=CIRCLE('',#76975,7.69146687436047);
#20484=CIRCLE('',#76976,7.69282864390347);
#20485=CIRCLE('',#76977,7.68652169413379);
#20486=CIRCLE('',#76979,7.69259352494882);
#20487=CIRCLE('',#76980,7.69146679101874);
#20488=CIRCLE('',#76981,7.6928287469085);
#20489=CIRCLE('',#76982,7.68652187802919);
#20490=CIRCLE('',#76984,7.69259356016282);
#20491=CIRCLE('',#76985,7.691467148089);
#20492=CIRCLE('',#76986,7.69282870572607);
#20493=CIRCLE('',#76987,7.68652201488452);
#20494=CIRCLE('',#76989,7.69259359852887);
#20495=CIRCLE('',#76990,7.69146696424068);
#20496=CIRCLE('',#76991,7.69282881299637);
#20497=CIRCLE('',#76992,7.68652184436031);
#20498=CIRCLE('',#76994,7.69259370349727);
#20499=CIRCLE('',#76995,7.69146696882247);
#20500=CIRCLE('',#76996,7.692828605017);
#20501=CIRCLE('',#76997,7.68652173871916);
#20502=CIRCLE('',#76999,7.69259390260136);
#20503=CIRCLE('',#77000,7.6914669348861);
#20504=CIRCLE('',#77001,7.69282861236544);
#20505=CIRCLE('',#77002,7.68652186283024);
#20506=CIRCLE('',#77004,7.69259385249028);
#20507=CIRCLE('',#77005,7.69146694463207);
#20508=CIRCLE('',#77006,7.69282860917482);
#20509=CIRCLE('',#77007,7.68652185817288);
#20510=CIRCLE('',#77009,7.69259377730403);
#20511=CIRCLE('',#77010,7.69146685597649);
#20512=CIRCLE('',#77011,7.69282867861488);
#20513=CIRCLE('',#77012,7.68652147082297);
#20514=CIRCLE('',#77013,7.69282887165906);
#20515=CIRCLE('',#77015,7.69259354930379);
#20516=CIRCLE('',#77016,7.69146699781378);
#20517=CIRCLE('',#77017,7.68652198036796);
#20518=CIRCLE('',#77019,7.6928284639639);
#20519=CIRCLE('',#77020,7.69259389688855);
#20520=CIRCLE('',#77021,7.69146673727659);
#20521=CIRCLE('',#77022,7.68652174668928);
#20522=CIRCLE('',#77024,7.69259364248133);
#20523=CIRCLE('',#77025,7.6914670556374);
#20524=CIRCLE('',#77026,7.69282887904053);
#20525=CIRCLE('',#77027,7.68652190379035);
#20526=CIRCLE('',#77029,7.69259345492421);
#20527=CIRCLE('',#77030,7.69146699481387);
#20528=CIRCLE('',#77031,7.69282881879384);
#20529=CIRCLE('',#77032,7.68652186672836);
#20530=CIRCLE('',#77034,7.69259377821932);
#20531=CIRCLE('',#77035,7.6914669565814);
#20532=CIRCLE('',#77036,7.69282865899933);
#20533=CIRCLE('',#77037,7.68652191668875);
#20534=CIRCLE('',#77039,7.69259378690776);
#20535=CIRCLE('',#77040,7.69146675768012);
#20536=CIRCLE('',#77041,7.69282872733812);
#20537=CIRCLE('',#77042,7.68652157256796);
#20538=CIRCLE('',#77044,7.69259367709038);
#20539=CIRCLE('',#77045,7.69146690611445);
#20540=CIRCLE('',#77046,7.69282864252631);
#20541=CIRCLE('',#77047,7.68652190628653);
#20542=CIRCLE('',#77049,7.69259398711421);
#20543=CIRCLE('',#77050,7.69146686903634);
#20544=CIRCLE('',#77051,7.69282859515984);
#20545=CIRCLE('',#77052,7.68652173300724);
#20546=CIRCLE('',#77054,7.69259365254763);
#20547=CIRCLE('',#77055,7.69146684927592);
#20548=CIRCLE('',#77056,7.69282842455778);
#20549=CIRCLE('',#77057,7.68652209975129);
#20550=CIRCLE('',#77059,7.69259365638295);
#20551=CIRCLE('',#77060,7.69146681076176);
#20552=CIRCLE('',#77061,7.69282857884792);
#20553=CIRCLE('',#77062,7.6865218269609);
#20554=CIRCLE('',#77064,7.69259363649161);
#20555=CIRCLE('',#77065,7.69146674289333);
#20556=CIRCLE('',#77066,7.69282882374801);
#20557=CIRCLE('',#77067,7.6865220526541);
#20558=CIRCLE('',#77069,7.69259366273547);
#20559=CIRCLE('',#77070,7.69146687686865);
#20560=CIRCLE('',#77071,7.69282889340358);
#20561=CIRCLE('',#77072,7.44708419294032);
#20562=CIRCLE('',#77073,7.44708561793515);
#20563=CIRCLE('',#77074,7.44708600142821);
#20564=CIRCLE('',#77075,7.44708641170203);
#20565=CIRCLE('',#77076,7.44708560826829);
#20566=CIRCLE('',#77077,7.44708515266404);
#20567=CIRCLE('',#77078,7.44708543844587);
#20568=CIRCLE('',#77079,7.44708521174704);
#20569=CIRCLE('',#77080,7.44708527016981);
#20570=CIRCLE('',#77081,7.44708459620124);
#20571=CIRCLE('',#77082,7.44708505445453);
#20572=CIRCLE('',#77083,7.44708454602176);
#20573=CIRCLE('',#77084,7.44708534479393);
#20574=CIRCLE('',#77085,7.44708562750459);
#20575=CIRCLE('',#77086,7.44708578392729);
#20576=CIRCLE('',#77087,7.44708545070702);
#20577=CIRCLE('',#77088,7.44708472173902);
#20578=CIRCLE('',#77089,7.44708366242392);
#20579=CIRCLE('',#77090,7.44708569711275);
#20580=CIRCLE('',#77091,7.4470842021165);
#20581=CIRCLE('',#77092,7.44708438198736);
#20582=CIRCLE('',#77093,7.44708479532805);
#20583=CIRCLE('',#77094,7.44708591037287);
#20584=CIRCLE('',#77095,7.44708525478703);
#20585=CIRCLE('',#77096,7.44708597637106);
#20586=CIRCLE('',#77097,7.44708599827779);
#20587=CIRCLE('',#77098,7.44708594245394);
#20588=CIRCLE('',#77099,7.44708653118089);
#20589=CIRCLE('',#77100,7.44708486685733);
#20590=CIRCLE('',#77101,7.44865545447364);
#20591=CIRCLE('',#77102,7.44865939903026);
#20592=CIRCLE('',#77103,7.44865951919544);
#20593=CIRCLE('',#77104,7.44865945619483);
#20594=CIRCLE('',#77105,7.44865934537791);
#20595=CIRCLE('',#77106,7.44865932466116);
#20596=CIRCLE('',#77107,7.44865920703867);
#20597=CIRCLE('',#77108,7.44865931020773);
#20598=CIRCLE('',#77109,7.44865905615679);
#20599=CIRCLE('',#77110,7.4486592598318);
#20600=CIRCLE('',#77111,7.44865928637504);
#20601=CIRCLE('',#77112,7.44865925240711);
#20602=CIRCLE('',#77113,7.44865896325401);
#20603=CIRCLE('',#77114,7.44865928152926);
#20604=CIRCLE('',#77115,7.44865939449395);
#20605=CIRCLE('',#77116,7.44865941621312);
#20606=CIRCLE('',#77117,7.44865941330856);
#20607=CIRCLE('',#77118,7.44865944336093);
#20608=CIRCLE('',#77119,7.44865922828271);
#20609=CIRCLE('',#77120,7.44865933672944);
#20610=CIRCLE('',#77121,7.44865941706835);
#20611=CIRCLE('',#77122,7.44865925172642);
#20612=CIRCLE('',#77123,7.44865915460453);
#20613=CIRCLE('',#77124,7.44865917328653);
#20614=CIRCLE('',#77125,7.4486590458652);
#20615=CIRCLE('',#77126,7.44865920197224);
#20616=CIRCLE('',#77127,7.4486590853991);
#20617=CIRCLE('',#77128,7.44865931187507);
#20618=CIRCLE('',#77129,7.44865912418389);
#20619=CIRCLE('',#77130,7.44865926283462);
#20620=CIRCLE('',#77131,7.44865959840247);
#20621=CIRCLE('',#77132,7.44865947209281);
#20622=CIRCLE('',#77133,7.448659285211);
#20623=CIRCLE('',#77134,7.44865965464314);
#20624=CIRCLE('',#77135,7.4486594992884);
#20625=CIRCLE('',#77136,7.44865925212478);
#20626=CIRCLE('',#77137,7.44865927353072);
#20627=CIRCLE('',#77138,7.44865934135186);
#20628=CIRCLE('',#77139,7.44865899006064);
#20629=CIRCLE('',#77140,7.4486591813801);
#20630=CIRCLE('',#77141,7.44865933458729);
#20631=CIRCLE('',#77142,7.44865925740424);
#20632=CIRCLE('',#77143,7.44865899043323);
#20633=CIRCLE('',#77144,7.4486591987037);
#20634=CIRCLE('',#77145,7.44865918721473);
#20635=CIRCLE('',#77146,7.44865928117158);
#20636=CIRCLE('',#77147,7.44865931234976);
#20637=CIRCLE('',#77148,7.44865922650077);
#20638=CIRCLE('',#77149,7.44865928675125);
#20639=CIRCLE('',#77150,7.44865955530131);
#20640=CIRCLE('',#77151,7.44865926751029);
#20641=CIRCLE('',#77152,7.4486593624084);
#20642=CIRCLE('',#77153,7.44865929684653);
#20643=CIRCLE('',#77154,7.44865936809075);
#20644=CIRCLE('',#77155,7.44865917887384);
#20645=CIRCLE('',#77156,7.44865943280146);
#20646=CIRCLE('',#77157,7.44865921044527);
#20647=CIRCLE('',#77158,7.44865545099262);
#20648=CIRCLE('',#77159,7.69146687677613);
#20649=CIRCLE('',#77160,7.69259385246013);
#20650=CIRCLE('',#77162,7.59069874782905);
#20651=CIRCLE('',#77163,7.5);
#20652=CIRCLE('',#77164,7.82252136132111);
#20653=CIRCLE('',#77165,7.69146690843554);
#20654=CIRCLE('',#77167,7.6930292059074);
#20655=CIRCLE('',#77168,7.68762402195699);
#20656=CIRCLE('',#77169,7.69259377727589);
#20657=CIRCLE('',#77171,7.59069211449223);
#20658=CIRCLE('',#77172,7.50000000166363);
#20659=CIRCLE('',#77173,7.82251325481052);
#20660=CIRCLE('',#77174,7.69146675991688);
#20661=CIRCLE('',#77176,7.69303011297896);
#20662=CIRCLE('',#77177,7.68762407921375);
#20663=CIRCLE('',#77178,7.69259354927485);
#20664=CIRCLE('',#77180,7.59069769736449);
#20665=CIRCLE('',#77181,7.5);
#20666=CIRCLE('',#77182,7.82251999913105);
#20667=CIRCLE('',#77183,7.69146691035308);
#20668=CIRCLE('',#77185,7.69302947585912);
#20669=CIRCLE('',#77186,7.68762361462464);
#20670=CIRCLE('',#77187,7.69259389685879);
#20671=CIRCLE('',#77189,7.59069939624143);
#20672=CIRCLE('',#77190,7.5);
#20673=CIRCLE('',#77191,7.82251960680243);
#20674=CIRCLE('',#77192,7.69146668179339);
#20675=CIRCLE('',#77194,7.69302912297621);
#20676=CIRCLE('',#77195,7.68762414399008);
#20677=CIRCLE('',#77196,7.69259364245232);
#20678=CIRCLE('',#77198,7.59069600435376);
#20679=CIRCLE('',#77199,7.49999999874647);
#20680=CIRCLE('',#77200,7.82252200020871);
#20681=CIRCLE('',#77201,7.69146698767325);
#20682=CIRCLE('',#77203,7.69302909653028);
#20683=CIRCLE('',#77204,7.68762361645412);
#20684=CIRCLE('',#77205,7.69259345652704);
#20685=CIRCLE('',#77207,7.59069728841729);
#20686=CIRCLE('',#77208,7.5);
#20687=CIRCLE('',#77209,7.82251866109699);
#20688=CIRCLE('',#77210,7.69146697030562);
#20689=CIRCLE('',#77212,7.69302954298555);
#20690=CIRCLE('',#77213,7.68762412063256);
#20691=CIRCLE('',#77215,7.59069979460845);
#20692=CIRCLE('',#77216,7.82251748897697);
#20693=CIRCLE('',#77217,7.69259378687915);
#20694=CIRCLE('',#77219,7.5906965376454);
#20695=CIRCLE('',#77220,7.5);
#20696=CIRCLE('',#77221,7.82252007915959);
#20697=CIRCLE('',#77222,7.69146669971079);
#20698=CIRCLE('',#77224,7.69302935579719);
#20699=CIRCLE('',#77225,7.68762414150259);
#20700=CIRCLE('',#77226,7.69259367706596);
#20701=CIRCLE('',#77228,7.59069776346958);
#20702=CIRCLE('',#77229,7.5);
#20703=CIRCLE('',#77230,7.82251960093144);
#20704=CIRCLE('',#77231,7.69146682697528);
#20705=CIRCLE('',#77233,7.69302926405833);
#20706=CIRCLE('',#77234,7.68762375277491);
#20707=CIRCLE('',#77235,7.69259398708472);
#20708=CIRCLE('',#77237,7.59069794350898);
#20709=CIRCLE('',#77238,7.5);
#20710=CIRCLE('',#77239,7.82251987647052);
#20711=CIRCLE('',#77240,7.69146679719617);
#20712=CIRCLE('',#77242,7.69302918497997);
#20713=CIRCLE('',#77243,7.68762412023477);
#20714=CIRCLE('',#77244,7.69259365251753);
#20715=CIRCLE('',#77246,7.59069258889142);
#20716=CIRCLE('',#77247,7.50000000205533);
#20717=CIRCLE('',#77248,7.82251175100706);
#20718=CIRCLE('',#77249,7.69146677708364);
#20719=CIRCLE('',#77251,7.6930299715105);
#20720=CIRCLE('',#77252,7.68762395064371);
#20721=CIRCLE('',#77253,7.69259365635744);
#20722=CIRCLE('',#77255,7.59069822792092);
#20723=CIRCLE('',#77256,7.5);
#20724=CIRCLE('',#77257,7.82251954047492);
#20725=CIRCLE('',#77258,7.69146673573611);
#20726=CIRCLE('',#77260,7.69302919174222);
#20727=CIRCLE('',#77261,7.68762427055975);
#20728=CIRCLE('',#77262,7.69259363646344);
#20729=CIRCLE('',#77264,7.59069647196464);
#20730=CIRCLE('',#77265,7.5);
#20731=CIRCLE('',#77266,7.82252147084837);
#20732=CIRCLE('',#77267,7.69146669772047);
#20733=CIRCLE('',#77269,7.69302957755455);
#20734=CIRCLE('',#77270,7.68762378726061);
#20735=CIRCLE('',#77271,7.6925936627046);
#20736=CIRCLE('',#77273,7.59069961187685);
#20737=CIRCLE('',#77274,7.5);
#20738=CIRCLE('',#77275,7.82251898575182);
#20739=CIRCLE('',#77276,7.69146684104373);
#20740=CIRCLE('',#77278,7.69302968603334);
#20741=CIRCLE('',#77279,7.68762426893667);
#20742=CIRCLE('',#77280,7.69259352803836);
#20743=CIRCLE('',#77282,7.59067639984585);
#20744=CIRCLE('',#77283,7.49999999294556);
#20745=CIRCLE('',#77284,7.82252591612768);
#20746=CIRCLE('',#77285,7.69146684492744);
#20747=CIRCLE('',#77287,7.69302416594306);
#20748=CIRCLE('',#77288,7.68762143965011);
#20749=CIRCLE('',#77289,7.69259369654752);
#20750=CIRCLE('',#77291,7.59067895629939);
#20751=CIRCLE('',#77292,7.50000000515093);
#20752=CIRCLE('',#77293,7.82249887507338);
#20753=CIRCLE('',#77294,7.69146673782841);
#20754=CIRCLE('',#77296,7.69303172916898);
#20755=CIRCLE('',#77297,7.68762421120419);
#20756=CIRCLE('',#77298,7.69259340743115);
#20757=CIRCLE('',#77300,7.59069883361731);
#20758=CIRCLE('',#77301,7.5);
#20759=CIRCLE('',#77302,7.82251900978043);
#20760=CIRCLE('',#77303,7.69146672944481);
#20761=CIRCLE('',#77305,7.69302925783024);
#20762=CIRCLE('',#77306,7.68762403548546);
#20763=CIRCLE('',#77307,7.69259360265325);
#20764=CIRCLE('',#77309,7.59069234582906);
#20765=CIRCLE('',#77310,7.50000000204315);
#20766=CIRCLE('',#77311,7.82251190864904);
#20767=CIRCLE('',#77312,7.69146687267438);
#20768=CIRCLE('',#77314,7.6930300327545);
#20769=CIRCLE('',#77315,7.68762420011832);
#20770=CIRCLE('',#77316,7.69259403319664);
#20771=CIRCLE('',#77318,7.59069832506839);
#20772=CIRCLE('',#77319,7.5);
#20773=CIRCLE('',#77320,7.82252133604163);
#20774=CIRCLE('',#77321,7.69146668069641);
#20775=CIRCLE('',#77323,7.69302933000856);
#20776=CIRCLE('',#77324,7.68762385993089);
#20777=CIRCLE('',#77325,7.69259351260242);
#20778=CIRCLE('',#77327,7.59069953203992);
#20779=CIRCLE('',#77328,7.49999999916126);
#20780=CIRCLE('',#77329,7.82252167476504);
#20781=CIRCLE('',#77330,7.69146689993987);
#20782=CIRCLE('',#77332,7.69302894205857);
#20783=CIRCLE('',#77333,7.68762386124297);
#20784=CIRCLE('',#77334,7.69259382856953);
#20785=CIRCLE('',#77336,7.59069658460535);
#20786=CIRCLE('',#77337,7.5);
#20787=CIRCLE('',#77338,7.82251979523547);
#20788=CIRCLE('',#77339,7.69146690128489);
#20789=CIRCLE('',#77341,7.69302933458611);
#20790=CIRCLE('',#77342,7.68762413533275);
#20791=CIRCLE('',#77343,7.69259364161605);
#20792=CIRCLE('',#77345,7.59067929887621);
#20793=CIRCLE('',#77346,7.49999999332733);
#20794=CIRCLE('',#77347,7.82252591988282);
#20795=CIRCLE('',#77348,7.69146689318844);
#20796=CIRCLE('',#77350,7.69302410711918);
#20797=CIRCLE('',#77351,7.68762099378799);
#20798=CIRCLE('',#77352,7.69259380384968);
#20799=CIRCLE('',#77354,7.59069962299981);
#20800=CIRCLE('',#77355,7.49999999937961);
#20801=CIRCLE('',#77356,7.82252173215583);
#20802=CIRCLE('',#77357,7.69146681270038);
#20803=CIRCLE('',#77359,7.69302893927606);
#20804=CIRCLE('',#77360,7.68762367868796);
#20805=CIRCLE('',#77361,7.69259352492098);
#20806=CIRCLE('',#77363,7.59069572709328);
#20807=CIRCLE('',#77364,7.5);
#20808=CIRCLE('',#77365,7.82252094087956);
#20809=CIRCLE('',#77366,7.69146671041594);
#20810=CIRCLE('',#77368,7.69302952805748);
#20811=CIRCLE('',#77369,7.68762376227097);
#20812=CIRCLE('',#77370,7.69259356013278);
#20813=CIRCLE('',#77372,7.59069385159072);
#20814=CIRCLE('',#77373,7.50000000212692);
#20815=CIRCLE('',#77374,7.8225116641969);
#20816=CIRCLE('',#77375,7.69146704737195);
#20817=CIRCLE('',#77377,7.6930302213243);
#20818=CIRCLE('',#77378,7.68762409347789);
#20819=CIRCLE('',#77379,7.69259359850366);
#20820=CIRCLE('',#77381,7.59068937344032);
#20821=CIRCLE('',#77382,7.49999999790811);
#20822=CIRCLE('',#77383,7.82252249489037);
#20823=CIRCLE('',#77384,7.69146692025778);
#20824=CIRCLE('',#77386,7.69302791572941);
#20825=CIRCLE('',#77387,7.68762336613701);
#20826=CIRCLE('',#77388,7.69259369059137);
#20827=CIRCLE('',#77390,7.59068004933096);
#20828=CIRCLE('',#77391,7.50000000528208);
#20829=CIRCLE('',#77392,7.82249852360222);
#20830=CIRCLE('',#77393,7.69146694937379);
#20831=CIRCLE('',#77395,7.69303144785881);
#20832=CIRCLE('',#77396,7.68762406157333);
#20833=CIRCLE('',#77397,7.6925939025748);
#20834=CIRCLE('',#77399,7.59069691634231);
#20835=CIRCLE('',#77400,7.5);
#20836=CIRCLE('',#77401,7.82252063468176);
#20837=CIRCLE('',#77402,7.69146688362149);
#20838=CIRCLE('',#77404,7.69302929330036);
#20839=CIRCLE('',#77405,7.68762381313008);
#20840=CIRCLE('',#77407,7.59070352038018);
#20841=CIRCLE('',#77408,7.5);
#20842=CIRCLE('',#77409,7.82251782820925);
#20843=CIRCLE('',#77411,7.69302934908707);
#20844=CIRCLE('',#77412,7.69259384669478);
#20845=CIRCLE('',#77413,7.68762391142974);
#20846=CIRCLE('',#77416,7.44901494297204);
#20847=CIRCLE('',#77417,7.44132506654215);
#20848=CIRCLE('',#77419,7.44901476114322);
#20849=CIRCLE('',#77420,7.44132490818521);
#20850=CIRCLE('',#77422,7.44901509298134);
#20851=CIRCLE('',#77423,7.44132503659772);
#20852=CIRCLE('',#77425,7.44901469632941);
#20853=CIRCLE('',#77426,7.44132470988597);
#20854=CIRCLE('',#77428,7.44901504095824);
#20855=CIRCLE('',#77429,7.44132501451318);
#20856=CIRCLE('',#77431,7.44901483010211);
#20857=CIRCLE('',#77432,7.44132514658019);
#20858=CIRCLE('',#77434,7.44901479188647);
#20859=CIRCLE('',#77435,7.44132476474595);
#20860=CIRCLE('',#77437,7.44901472892966);
#20861=CIRCLE('',#77438,7.44132502466893);
#20862=CIRCLE('',#77440,7.44901468919714);
#20863=CIRCLE('',#77441,7.44132504613859);
#20864=CIRCLE('',#77443,7.44901486108914);
#20865=CIRCLE('',#77444,7.44132476292834);
#20866=CIRCLE('',#77446,7.44901483491887);
#20867=CIRCLE('',#77447,7.44132507072986);
#20868=CIRCLE('',#77449,7.44901472271123);
#20869=CIRCLE('',#77450,7.4413248964315);
#20870=CIRCLE('',#77452,7.44901471799794);
#20871=CIRCLE('',#77453,7.44132508046603);
#20872=CIRCLE('',#77455,7.44901479385614);
#20873=CIRCLE('',#77456,7.44132492111921);
#20874=CIRCLE('',#77458,7.44901488147878);
#20875=CIRCLE('',#77459,7.44132470821559);
#20876=CIRCLE('',#77461,7.44901498855247);
#20877=CIRCLE('',#77462,7.44132499121307);
#20878=CIRCLE('',#77464,7.44901483127117);
#20879=CIRCLE('',#77465,7.44132504797884);
#20880=CIRCLE('',#77467,7.44901489864582);
#20881=CIRCLE('',#77468,7.44132493649476);
#20882=CIRCLE('',#77470,7.44901486221692);
#20883=CIRCLE('',#77471,7.44132496814157);
#20884=CIRCLE('',#77473,7.44901483539481);
#20885=CIRCLE('',#77474,7.44132500908834);
#20886=CIRCLE('',#77476,7.44901490637958);
#20887=CIRCLE('',#77477,7.44132492102672);
#20888=CIRCLE('',#77479,7.44901473158954);
#20889=CIRCLE('',#77480,7.44132485247813);
#20890=CIRCLE('',#77482,7.4490147691237);
#20891=CIRCLE('',#77483,7.4413249053069);
#20892=CIRCLE('',#77485,7.44901503522182);
#20893=CIRCLE('',#77486,7.44132521103752);
#20894=CIRCLE('',#77488,7.44901507867795);
#20895=CIRCLE('',#77489,7.44132496020567);
#20896=CIRCLE('',#77491,7.44901485555681);
#20897=CIRCLE('',#77492,7.44132488477906);
#20898=CIRCLE('',#77494,7.44901484283174);
#20899=CIRCLE('',#77495,7.44132489754185);
#20900=CIRCLE('',#77497,7.44901477941788);
#20901=CIRCLE('',#77498,7.44132522014264);
#20902=CIRCLE('',#77500,7.44901488052498);
#20903=CIRCLE('',#77501,7.44132492046871);
#20904=CIRCLE('',#77529,7.44096471604082);
#20905=CIRCLE('',#77531,7.44244280479572);
#20906=CIRCLE('',#77532,7.44096416773314);
#20907=CIRCLE('',#77533,7.44244635429767);
#20908=CIRCLE('',#77534,7.44096478167989);
#20909=CIRCLE('',#77536,7.44244637802895);
#20910=CIRCLE('',#77537,7.44096485769064);
#20911=CIRCLE('',#77539,7.44244602496989);
#20912=CIRCLE('',#77540,7.44096452100884);
#20913=CIRCLE('',#77542,7.44244619382863);
#20914=CIRCLE('',#77543,7.44096449640376);
#20915=CIRCLE('',#77545,7.44244617677346);
#20916=CIRCLE('',#77546,7.44096457251793);
#20917=CIRCLE('',#77548,7.44244606805147);
#20918=CIRCLE('',#77549,7.44096415252455);
#20919=CIRCLE('',#77550,7.4424462802272);
#20920=CIRCLE('',#77551,7.4409643905002);
#20921=CIRCLE('',#77553,7.44244297309812);
#20922=CIRCLE('',#77554,7.440964522414);
#20923=CIRCLE('',#77556,7.44244281349285);
#20924=CIRCLE('',#77557,7.44096444919983);
#20925=CIRCLE('',#77559,7.44244591738352);
#20926=CIRCLE('',#77560,7.44096472203706);
#20927=CIRCLE('',#77562,7.44244303675119);
#20928=CIRCLE('',#77563,7.44096433176278);
#20929=CIRCLE('',#77564,7.44244641043208);
#20930=CIRCLE('',#77565,7.44096493845626);
#20931=CIRCLE('',#77567,7.44244635687994);
#20932=CIRCLE('',#77568,7.44096466855212);
#20933=CIRCLE('',#77570,7.44244606261698);
#20934=CIRCLE('',#77571,7.44096415428745);
#20935=CIRCLE('',#77572,7.44244639328344);
#20936=CIRCLE('',#77573,7.44096469441773);
#20937=CIRCLE('',#77575,7.44244630739266);
#20938=CIRCLE('',#77576,7.44096419562405);
#20939=CIRCLE('',#77577,7.44244624249257);
#20940=CIRCLE('',#77578,7.4409645724652);
#20941=CIRCLE('',#77580,7.44244637955912);
#20942=CIRCLE('',#77581,7.440964794856);
#20943=CIRCLE('',#77583,7.44244316277483);
#20944=CIRCLE('',#77584,7.44096432388314);
#20945=CIRCLE('',#77585,7.44244637094867);
#20946=CIRCLE('',#77586,7.44096418647052);
#20947=CIRCLE('',#77587,7.44244622685979);
#20948=CIRCLE('',#77588,7.44096487306209);
#20949=CIRCLE('',#77590,7.44244622980629);
#20950=CIRCLE('',#77591,7.44096479527389);
#20951=CIRCLE('',#77593,7.4424460518505);
#20952=CIRCLE('',#77594,7.44096474402759);
#20953=CIRCLE('',#77596,7.44244294054158);
#20954=CIRCLE('',#77597,7.4409647417251);
#20955=CIRCLE('',#77599,7.44244620220576);
#20956=CIRCLE('',#77600,7.4409646578587);
#20957=CIRCLE('',#77602,7.44244618615641);
#20958=CIRCLE('',#77603,7.44096450421653);
#20959=CIRCLE('',#77605,7.44244303871399);
#20960=CIRCLE('',#77606,7.44096475675713);
#20961=CIRCLE('',#77608,7.44244301437565);
#20962=CIRCLE('',#77610,7.4470849954363);
#20963=CIRCLE('',#77611,7.44708566575379);
#20964=CIRCLE('',#77612,7.4470854060469);
#20965=CIRCLE('',#77613,7.4470852658502);
#20966=CIRCLE('',#77614,7.44708613132106);
#20967=CIRCLE('',#77615,7.44708473838514);
#20968=CIRCLE('',#77616,7.44708613257339);
#20969=CIRCLE('',#77617,7.44708536736408);
#20970=CIRCLE('',#77618,7.44708498295746);
#20971=CIRCLE('',#77619,7.44708484853103);
#20972=CIRCLE('',#77620,7.44708634291999);
#20973=CIRCLE('',#77621,7.44708473348576);
#20974=CIRCLE('',#77622,7.4470839111118);
#20975=CIRCLE('',#77623,7.44708556794052);
#20976=CIRCLE('',#77624,7.44708535112535);
#20977=CIRCLE('',#77625,7.44708660484889);
#20978=CIRCLE('',#77626,7.44708634387299);
#20979=CIRCLE('',#77627,7.44708553329505);
#20980=CIRCLE('',#77628,7.44708613245776);
#20981=CIRCLE('',#77629,7.4470848224883);
#20982=CIRCLE('',#77630,7.44708488318781);
#20983=CIRCLE('',#77631,7.44708557450435);
#20984=CIRCLE('',#77632,7.44708512104896);
#20985=CIRCLE('',#77633,7.44708624028346);
#20986=CIRCLE('',#77634,7.44708479120748);
#20987=CIRCLE('',#77635,7.44708627845845);
#20988=CIRCLE('',#77636,7.44708548323966);
#20989=CIRCLE('',#77637,7.44708601562468);
#20990=CIRCLE('',#77638,7.44708424622066);
#21046=B_SPLINE_CURVE_WITH_KNOTS('',3,(#92442,#92443,#92444,#92445,#92446,
#92447),.UNSPECIFIED.,.F.,.F.,(4,2,4),(-0.0592625039988469,-0.0381784708554363,
-1.00000000442108E-6),.UNSPECIFIED.);
#21047=B_SPLINE_CURVE_WITH_KNOTS('',3,(#92449,#92450,#92451,#92452,#92453,
#92454,#92455,#92456,#92457,#92458),.UNSPECIFIED.,.F.,.F.,(4,2,2,2,4),(9.99985499371358E-7,
0.00990798547874647,0.0199209917052848,0.0400020007437245,0.0800923349447478),
 .UNSPECIFIED.);
#21048=B_SPLINE_CURVE_WITH_KNOTS('',3,(#92464,#92465,#92466,#92467,#92468,
#92469),.UNSPECIFIED.,.F.,.F.,(4,2,4),(0.,0.016366392747835,0.032834133837728),
 .UNSPECIFIED.);
#21049=B_SPLINE_CURVE_WITH_KNOTS('',3,(#92471,#92472,#92473,#92474,#92475,
#92476,#92477,#92478,#92479,#92480),.UNSPECIFIED.,.F.,.F.,(4,3,3,4),(3.12055520624018E-12,
7.37661517073135E-5,0.000147532580837493,0.00027986750847265),
 .UNSPECIFIED.);
#21050=B_SPLINE_CURVE_WITH_KNOTS('',3,(#92482,#92483,#92484,#92485,#92486,
#92487),.UNSPECIFIED.,.F.,.F.,(4,2,4),(1.000000003925E-6,0.0379299703047647,
0.0758579941174657),.UNSPECIFIED.);
#21051=B_SPLINE_CURVE_WITH_KNOTS('',3,(#92489,#92490,#92491,#92492,#92493,
#92494,#92495,#92496,#92497,#92498),.UNSPECIFIED.,.F.,.F.,(4,2,2,2,4),(1.00013078331987E-6,
0.00990710921000036,0.0199202404646063,0.0400015002295186,0.0800923350090046),
 .UNSPECIFIED.);
#21052=B_SPLINE_CURVE_WITH_KNOTS('',3,(#92504,#92505,#92506,#92507,#92508,
#92509),.UNSPECIFIED.,.F.,.F.,(4,2,4),(0.,0.016366874952083,0.0328340574266459),
 .UNSPECIFIED.);
#21053=B_SPLINE_CURVE_WITH_KNOTS('',3,(#92511,#92512,#92513,#92514,#92515,
#92516,#92517,#92518,#92519,#92520),.UNSPECIFIED.,.F.,.F.,(4,3,3,4),(2.15830403525905E-12,
7.37661523423699E-5,0.000147532582109008,0.000279867507510834),
 .UNSPECIFIED.);
#21054=B_SPLINE_CURVE_WITH_KNOTS('',3,(#92522,#92523,#92524,#92525,#92526,
#92527),.UNSPECIFIED.,.F.,.F.,(4,2,4),(1.00000000432393E-6,0.0379299702663971,
0.0758579940911893),.UNSPECIFIED.);
#21055=B_SPLINE_CURVE_WITH_KNOTS('',3,(#92529,#92530,#92531,#92532,#92533,
#92534,#92535,#92536,#92537,#92538),.UNSPECIFIED.,.F.,.F.,(4,2,2,2,4),(1.00017476251821E-6,
0.0099071092209813,0.0199202404680647,0.0400015001924167,0.0800923349270695),
 .UNSPECIFIED.);
#21056=B_SPLINE_CURVE_WITH_KNOTS('',3,(#92544,#92545,#92546,#92547,#92548,
#92549),.UNSPECIFIED.,.F.,.F.,(4,2,4),(0.,0.0163668763525077,0.0328340636938574),
 .UNSPECIFIED.);
#21057=B_SPLINE_CURVE_WITH_KNOTS('',3,(#92551,#92552,#92553,#92554,#92555,
#92556,#92557,#92558,#92559,#92560),.UNSPECIFIED.,.F.,.F.,(4,3,3,4),(2.52904142129497E-12,
7.37661520584279E-5,0.000147532581535914,0.00027986750749572),
 .UNSPECIFIED.);
#21058=B_SPLINE_CURVE_WITH_KNOTS('',3,(#92562,#92563,#92564,#92565,#92566,
#92567),.UNSPECIFIED.,.F.,.F.,(4,2,4),(1.00000000433087E-6,0.0379299703178269,
0.0758579941192071),.UNSPECIFIED.);
#21059=B_SPLINE_CURVE_WITH_KNOTS('',3,(#92569,#92570,#92571,#92572,#92573,
#92574,#92575,#92576,#92577,#92578),.UNSPECIFIED.,.F.,.F.,(4,2,2,2,4),(1.00014526185026E-6,
0.00990710922096496,0.0199202404714764,0.0400015002087619,0.0800923349616018),
 .UNSPECIFIED.);
#21060=B_SPLINE_CURVE_WITH_KNOTS('',3,(#92584,#92585,#92586,#92587,#92588,
#92589),.UNSPECIFIED.,.F.,.F.,(4,2,4),(0.,0.0163668761217582,0.0328340625366268),
 .UNSPECIFIED.);
#21061=B_SPLINE_CURVE_WITH_KNOTS('',3,(#92591,#92592,#92593,#92594,#92595,
#92596,#92597,#92598,#92599,#92600),.UNSPECIFIED.,.F.,.F.,(4,3,3,4),(2.88097431277638E-12,
7.37661520465302E-5,0.000147532581515671,0.000279867510177933),
 .UNSPECIFIED.);
#21062=B_SPLINE_CURVE_WITH_KNOTS('',3,(#92602,#92603,#92604,#92605,#92606,
#92607),.UNSPECIFIED.,.F.,.F.,(4,2,4),(1.00000000441414E-6,0.0379299703846838,
0.0758579942063754),.UNSPECIFIED.);
#21063=B_SPLINE_CURVE_WITH_KNOTS('',3,(#92609,#92610,#92611,#92612,#92613,
#92614,#92615,#92616,#92617,#92618),.UNSPECIFIED.,.F.,.F.,(4,2,2,2,4),(1.00010992915299E-6,
0.0099071091906864,0.019920240414248,0.040001500107306,0.080092334757455),
 .UNSPECIFIED.);
#21064=B_SPLINE_CURVE_WITH_KNOTS('',3,(#92624,#92625,#92626,#92627,#92628,
#92629),.UNSPECIFIED.,.F.,.F.,(4,2,4),(0.,0.0163668780737397,0.0328340708943008),
 .UNSPECIFIED.);
#21065=B_SPLINE_CURVE_WITH_KNOTS('',3,(#92631,#92632,#92633,#92634,#92635,
#92636,#92637,#92638,#92639,#92640),.UNSPECIFIED.,.F.,.F.,(4,3,3,4),(2.17438718025666E-12,
7.37661519451421E-5,0.000147532581312125,0.000279867506786178),
 .UNSPECIFIED.);
#21066=B_SPLINE_CURVE_WITH_KNOTS('',3,(#92642,#92643,#92644,#92645,#92646,
#92647),.UNSPECIFIED.,.F.,.F.,(4,2,4),(1.00000000362519E-6,0.0379299702686182,
0.07585799407784),.UNSPECIFIED.);
#21067=B_SPLINE_CURVE_WITH_KNOTS('',3,(#92649,#92650,#92651,#92652,#92653,
#92654,#92655,#92656,#92657,#92658),.UNSPECIFIED.,.F.,.F.,(4,2,2,2,4),(1.00008837944867E-6,
0.00990710923003866,0.0199202405024881,0.0400015002946333,0.080092335142938),
 .UNSPECIFIED.);
#21068=B_SPLINE_CURVE_WITH_KNOTS('',3,(#92664,#92665,#92666,#92667,#92668,
#92669),.UNSPECIFIED.,.F.,.F.,(4,2,4),(0.,0.0163663928143568,0.0328341344900907),
 .UNSPECIFIED.);
#21069=B_SPLINE_CURVE_WITH_KNOTS('',3,(#92671,#92672,#92673,#92674,#92675,
#92676,#92677,#92678,#92679,#92680),.UNSPECIFIED.,.F.,.F.,(4,3,3,4),(2.64934922214782E-12,
7.37661518159472E-5,0.000147532581049749,0.000279867507628596),
 .UNSPECIFIED.);
#21070=B_SPLINE_CURVE_WITH_KNOTS('',3,(#92682,#92683,#92684,#92685,#92686,
#92687),.UNSPECIFIED.,.F.,.F.,(4,2,4),(1.00000000451822E-6,0.0379299702450166,
0.0758579940565196),.UNSPECIFIED.);
#21071=B_SPLINE_CURVE_WITH_KNOTS('',3,(#92689,#92690,#92691,#92692,#92693,
#92694,#92695,#92696,#92697,#92698),.UNSPECIFIED.,.F.,.F.,(4,2,2,2,4),(1.00014647044652E-6,
0.00990710920230482,0.0199202404453444,0.0400015001848174,0.0800923349138297),
 .UNSPECIFIED.);
#21072=B_SPLINE_CURVE_WITH_KNOTS('',3,(#92704,#92705,#92706,#92707,#92708,
#92709),.UNSPECIFIED.,.F.,.F.,(4,2,4),(0.,0.0163663706141495,0.0328340656287997),
 .UNSPECIFIED.);
#21073=B_SPLINE_CURVE_WITH_KNOTS('',3,(#92711,#92712,#92713,#92714,#92715,
#92716,#92717,#92718,#92719,#92720),.UNSPECIFIED.,.F.,.F.,(4,3,3,4),(2.78736780820764E-12,
7.3766151409991E-5,0.00014753258024197,0.000279867509359074),
 .UNSPECIFIED.);
#21074=B_SPLINE_CURVE_WITH_KNOTS('',3,(#92722,#92723,#92724,#92725,#92726,
#92727),.UNSPECIFIED.,.F.,.F.,(4,2,4),(1.00000000405091E-6,0.0379299703316601,
0.0758579941712396),.UNSPECIFIED.);
#21075=B_SPLINE_CURVE_WITH_KNOTS('',3,(#92729,#92730,#92731,#92732,#92733,
#92734,#92735,#92736,#92737,#92738),.UNSPECIFIED.,.F.,.F.,(4,2,2,2,4),(1.0001287590813E-6,
0.00990710922500387,0.0199202404932373,0.040001500277097,0.0800923351051997),
 .UNSPECIFIED.);
#21076=B_SPLINE_CURVE_WITH_KNOTS('',3,(#92744,#92745,#92746,#92747,#92748,
#92749),.UNSPECIFIED.,.F.,.F.,(4,2,4),(0.,0.0163663733575533,0.0328340772555867),
 .UNSPECIFIED.);
#21077=B_SPLINE_CURVE_WITH_KNOTS('',3,(#92751,#92752,#92753,#92754,#92755,
#92756,#92757,#92758,#92759,#92760),.UNSPECIFIED.,.F.,.F.,(4,3,3,4),(3.46919833266426E-12,
7.37661524662696E-5,0.0001475325823551,0.000279867508005713),
 .UNSPECIFIED.);
#21078=B_SPLINE_CURVE_WITH_KNOTS('',3,(#92762,#92763,#92764,#92765,#92766,
#92767),.UNSPECIFIED.,.F.,.F.,(4,2,4),(1.00000000386265E-6,0.0379299702966132,
0.07585799410702),.UNSPECIFIED.);
#21079=B_SPLINE_CURVE_WITH_KNOTS('',3,(#92769,#92770,#92771,#92772,#92773,
#92774,#92775,#92776,#92777,#92778),.UNSPECIFIED.,.F.,.F.,(4,2,2,2,4),(1.00009055644546E-6,
0.00990710921856916,0.0199202404809799,0.0400015002530257,0.0800923350565718),
 .UNSPECIFIED.);
#21080=B_SPLINE_CURVE_WITH_KNOTS('',3,(#92784,#92785,#92786,#92787,#92788,
#92789),.UNSPECIFIED.,.F.,.F.,(4,2,4),(0.,0.0163663707641851,0.0328340662430508),
 .UNSPECIFIED.);
#21081=B_SPLINE_CURVE_WITH_KNOTS('',3,(#92791,#92792,#92793,#92794,#92795,
#92796,#92797,#92798,#92799,#92800),.UNSPECIFIED.,.F.,.F.,(4,3,3,4),(2.50094752839556E-12,
7.37661519728823E-5,0.000147532581366429,0.000279867507647884),
 .UNSPECIFIED.);
#21082=B_SPLINE_CURVE_WITH_KNOTS('',3,(#92802,#92803,#92804,#92805,#92806,
#92807),.UNSPECIFIED.,.F.,.F.,(4,2,4),(1.00000000426148E-6,0.0379299702609412,
0.0758579940783564),.UNSPECIFIED.);
#21083=B_SPLINE_CURVE_WITH_KNOTS('',3,(#92809,#92810,#92811,#92812,#92813,
#92814,#92815,#92816,#92817,#92818),.UNSPECIFIED.,.F.,.F.,(4,2,2,2,4),(1.00016604854426E-6,
0.00990710920452595,0.0199202404482969,0.0400015001930305,0.0800923349310915),
 .UNSPECIFIED.);
#21084=B_SPLINE_CURVE_WITH_KNOTS('',3,(#92824,#92825,#92826,#92827,#92828,
#92829),.UNSPECIFIED.,.F.,.F.,(4,2,4),(0.,0.01636639315645,0.0328341357805788),
 .UNSPECIFIED.);
#21085=B_SPLINE_CURVE_WITH_KNOTS('',3,(#92831,#92832,#92833,#92834,#92835,
#92836,#92837,#92838,#92839,#92840),.UNSPECIFIED.,.F.,.F.,(4,3,3,4),(2.94307093505262E-12,
7.37661527913104E-5,0.000147532583003831,0.000279867507750485),
 .UNSPECIFIED.);
#21086=B_SPLINE_CURVE_WITH_KNOTS('',3,(#92842,#92843,#92844,#92845,#92846,
#92847),.UNSPECIFIED.,.F.,.F.,(4,2,4),(1.00000000359874E-6,0.0379299703013,
0.075857994144482),.UNSPECIFIED.);
#21087=B_SPLINE_CURVE_WITH_KNOTS('',3,(#92849,#92850,#92851,#92852,#92853,
#92854,#92855,#92856,#92857,#92858),.UNSPECIFIED.,.F.,.F.,(4,2,2,2,4),(1.00013394837672E-6,
0.00990710922800834,0.0199202404912242,0.0400015002501556,0.0800923350518471),
 .UNSPECIFIED.);
#21088=B_SPLINE_CURVE_WITH_KNOTS('',3,(#92864,#92865,#92866,#92867,#92868,
#92869),.UNSPECIFIED.,.F.,.F.,(4,2,4),(0.,0.0163663710780007,0.032834067324964),
 .UNSPECIFIED.);
#21089=B_SPLINE_CURVE_WITH_KNOTS('',3,(#92871,#92872,#92873,#92874,#92875,
#92876,#92877,#92878,#92879,#92880),.UNSPECIFIED.,.F.,.F.,(4,3,3,4),(3.2213193587114E-12,
7.3766151590614E-5,0.000147532580599784,0.000279867509316411),
 .UNSPECIFIED.);
#21090=B_SPLINE_CURVE_WITH_KNOTS('',3,(#92882,#92883,#92884,#92885,#92886,
#92887),.UNSPECIFIED.,.F.,.F.,(4,2,4),(1.00000000392768E-6,0.037929970348679,
0.075857994134376),.UNSPECIFIED.);
#21091=B_SPLINE_CURVE_WITH_KNOTS('',3,(#92889,#92890,#92891,#92892,#92893,
#92894,#92895,#92896,#92897,#92898),.UNSPECIFIED.,.F.,.F.,(4,2,2,2,4),(9.9997700206558E-7,
0.00990798545880012,0.0199209916821671,0.0400020007165947,0.0800923349030195),
 .UNSPECIFIED.);
#21092=B_SPLINE_CURVE_WITH_KNOTS('',3,(#92904,#92905,#92906,#92907,#92908,
#92909),.UNSPECIFIED.,.F.,.F.,(4,2,4),(0.,0.0163663718390811,0.0328340706570268),
 .UNSPECIFIED.);
#21093=B_SPLINE_CURVE_WITH_KNOTS('',3,(#92911,#92912,#92913,#92914,#92915,
#92916,#92917,#92918,#92919,#92920),.UNSPECIFIED.,.F.,.F.,(4,3,3,4),(2.5445448407392E-12,
7.37661519646406E-5,0.000147532581351944,0.000279867507127543),
 .UNSPECIFIED.);
#21094=B_SPLINE_CURVE_WITH_KNOTS('',3,(#92922,#92923,#92924,#92925,#92926,
#92927),.UNSPECIFIED.,.F.,.F.,(4,2,4),(1.0000000036189E-6,0.0379299702266974,
0.0758579940621541),.UNSPECIFIED.);
#21095=B_SPLINE_CURVE_WITH_KNOTS('',3,(#92929,#92930,#92931,#92932,#92933,
#92934,#92935,#92936,#92937,#92938),.UNSPECIFIED.,.F.,.F.,(4,2,2,2,4),(9.99988358708106E-7,
0.00990798546912516,0.0199209916873161,0.0400020007141071,0.0800923348808819),
 .UNSPECIFIED.);
#21096=B_SPLINE_CURVE_WITH_KNOTS('',3,(#92944,#92945,#92946,#92947,#92948,
#92949),.UNSPECIFIED.,.F.,.F.,(4,2,4),(0.,0.0163668779555029,0.0328340697895225),
 .UNSPECIFIED.);
#21097=B_SPLINE_CURVE_WITH_KNOTS('',3,(#92951,#92952,#92953,#92954,#92955,
#92956,#92957,#92958,#92959,#92960),.UNSPECIFIED.,.F.,.F.,(4,3,3,4),(2.81817145205986E-12,
7.37661516072452E-5,0.000147532580637628,0.000279867508117206),
 .UNSPECIFIED.);
#21098=B_SPLINE_CURVE_WITH_KNOTS('',3,(#92962,#92963,#92964,#92965,#92966,
#92967),.UNSPECIFIED.,.F.,.F.,(4,2,4),(1.00000000417821E-6,0.0379299702638397,
0.0758579940710071),.UNSPECIFIED.);
#21099=B_SPLINE_CURVE_WITH_KNOTS('',3,(#92969,#92970,#92971,#92972,#92973,
#92974,#92975,#92976,#92977,#92978),.UNSPECIFIED.,.F.,.F.,(4,2,2,2,4),(1.00014734702119E-6,
0.00990710921590618,0.0199202404703475,0.0400015002220982,0.0800923349919604),
 .UNSPECIFIED.);
#21100=B_SPLINE_CURVE_WITH_KNOTS('',3,(#92984,#92985,#92986,#92987,#92988,
#92989),.UNSPECIFIED.,.F.,.F.,(4,2,4),(0.,0.0163668780647285,0.032834070559676),
 .UNSPECIFIED.);
#21101=B_SPLINE_CURVE_WITH_KNOTS('',3,(#92991,#92992,#92993,#92994,#92995,
#92996,#92997,#92998,#92999,#93000),.UNSPECIFIED.,.F.,.F.,(4,3,3,4),(3.17358619411357E-12,
7.37661526734922E-5,0.000147532582768413,0.000279867509043945),
 .UNSPECIFIED.);
#21102=B_SPLINE_CURVE_WITH_KNOTS('',3,(#93002,#93003,#93004,#93005,#93006,
#93007),.UNSPECIFIED.,.F.,.F.,(4,2,4),(1.00000000444189E-6,0.0379299703416276,
0.0758579941445551),.UNSPECIFIED.);
#21103=B_SPLINE_CURVE_WITH_KNOTS('',3,(#93009,#93010,#93011,#93012,#93013,
#93014,#93015,#93016,#93017,#93018),.UNSPECIFIED.,.F.,.F.,(4,2,2,2,4),(1.00000822225027E-6,
0.00990092359092381,0.0199067792115138,0.0399734104969956,0.0800924093120953),
 .UNSPECIFIED.);
#21104=B_SPLINE_CURVE_WITH_KNOTS('',3,(#93024,#93025,#93026,#93027,#93028,
#93029),.UNSPECIFIED.,.F.,.F.,(4,2,4),(0.,0.0163668790308347,0.0328340750476689),
 .UNSPECIFIED.);
#21105=B_SPLINE_CURVE_WITH_KNOTS('',3,(#93031,#93032,#93033,#93034,#93035,
#93036,#93037,#93038,#93039,#93040),.UNSPECIFIED.,.F.,.F.,(4,3,3,4),(2.10757257581087E-12,
7.37661524777434E-5,0.000147532582380299,0.000279867505938687),
 .UNSPECIFIED.);
#21106=B_SPLINE_CURVE_WITH_KNOTS('',3,(#93042,#93043,#93044,#93045,#93046,
#93047),.UNSPECIFIED.,.F.,.F.,(4,2,4),(1.00000000390311E-6,0.0379299702530284,
0.0758579940725049),.UNSPECIFIED.);
#21107=B_SPLINE_CURVE_WITH_KNOTS('',3,(#93049,#93050,#93051,#93052,#93053,
#93054,#93055,#93056,#93057,#93058),.UNSPECIFIED.,.F.,.F.,(4,2,2,2,4),(9.99973126498073E-7,
0.00990798551049127,0.0199209917726281,0.0400020008332237,0.0800923351454191),
 .UNSPECIFIED.);
#21108=B_SPLINE_CURVE_WITH_KNOTS('',3,(#93064,#93065,#93066,#93067,#93068,
#93069),.UNSPECIFIED.,.F.,.F.,(4,2,4),(0.,0.0163668787190169,0.0328340732796807),
 .UNSPECIFIED.);
#21109=B_SPLINE_CURVE_WITH_KNOTS('',3,(#93071,#93072,#93073,#93074,#93075,
#93076,#93077,#93078,#93079,#93080),.UNSPECIFIED.,.F.,.F.,(4,3,3,4),(2.49687519012765E-12,
7.37661519882218E-5,0.000147532581397849,0.000279867507261817),
 .UNSPECIFIED.);
#21110=B_SPLINE_CURVE_WITH_KNOTS('',3,(#93082,#93083,#93084,#93085,#93086,
#93087),.UNSPECIFIED.,.F.,.F.,(4,2,4),(1.00000000414424E-6,0.0379299702789192,
0.0758579940530802),.UNSPECIFIED.);
#21111=B_SPLINE_CURVE_WITH_KNOTS('',3,(#93089,#93090,#93091,#93092,#93093,
#93094,#93095,#93096,#93097,#93098),.UNSPECIFIED.,.F.,.F.,(4,2,2,2,4),(1.00014742275135E-6,
0.00990710919278961,0.0199202404213151,0.0400015001384411,0.0800923348165605),
 .UNSPECIFIED.);
#21112=B_SPLINE_CURVE_WITH_KNOTS('',3,(#93104,#93105,#93106,#93107,#93108,
#93109),.UNSPECIFIED.,.F.,.F.,(4,2,4),(0.,0.0163663713767149,0.0328340684866575),
 .UNSPECIFIED.);
#21113=B_SPLINE_CURVE_WITH_KNOTS('',3,(#93111,#93112,#93113,#93114,#93115,
#93116,#93117,#93118,#93119,#93120),.UNSPECIFIED.,.F.,.F.,(4,3,3,4),(3.0256058344888E-12,
7.37661519876092E-5,0.000147532581400851,0.000279867509036399),
 .UNSPECIFIED.);
#21114=B_SPLINE_CURVE_WITH_KNOTS('',3,(#93122,#93123,#93124,#93125,#93126,
#93127),.UNSPECIFIED.,.F.,.F.,(4,2,4),(1.00000000404653E-6,0.0379299702945319,
0.0758579941263343),.UNSPECIFIED.);
#21115=B_SPLINE_CURVE_WITH_KNOTS('',3,(#93129,#93130,#93131,#93132,#93133,
#93134,#93135,#93136,#93137,#93138),.UNSPECIFIED.,.F.,.F.,(4,2,2,2,4),(9.99980262838728E-7,
0.00990798549176339,0.0199209917417096,0.040002000814808,0.0800923350984535),
 .UNSPECIFIED.);
#21116=B_SPLINE_CURVE_WITH_KNOTS('',3,(#93144,#93145,#93146,#93147,#93148,
#93149),.UNSPECIFIED.,.F.,.F.,(4,2,4),(0.,0.0163668992924121,0.0328341351884076),
 .UNSPECIFIED.);
#21117=B_SPLINE_CURVE_WITH_KNOTS('',3,(#93151,#93152,#93153,#93154,#93155,
#93156,#93157,#93158,#93159,#93160),.UNSPECIFIED.,.F.,.F.,(4,3,3,4),(3.40751591842374E-12,
7.37661512684975E-5,0.000147532579958051,0.000279867508816005),
 .UNSPECIFIED.);
#21118=B_SPLINE_CURVE_WITH_KNOTS('',3,(#93162,#93163,#93164,#93165,#93166,
#93167),.UNSPECIFIED.,.F.,.F.,(4,2,4),(1.00000000455291E-6,0.0379299703035672,
0.0758579941397041),.UNSPECIFIED.);
#21119=B_SPLINE_CURVE_WITH_KNOTS('',3,(#93169,#93170,#93171,#93172,#93173,
#93174,#93175,#93176,#93177,#93178),.UNSPECIFIED.,.F.,.F.,(4,2,2,2,4),(1.00011613515136E-6,
0.0099071092388292,0.0199202405152284,0.0400015002954983,0.0800923351443803),
 .UNSPECIFIED.);
#21120=B_SPLINE_CURVE_WITH_KNOTS('',3,(#93184,#93185,#93186,#93187,#93188,
#93189),.UNSPECIFIED.,.F.,.F.,(4,2,4),(0.,0.0163669013159866,0.0328341564473171),
 .UNSPECIFIED.);
#21121=B_SPLINE_CURVE_WITH_KNOTS('',3,(#93191,#93192,#93193,#93194,#93195,
#93196,#93197,#93198,#93199,#93200),.UNSPECIFIED.,.F.,.F.,(4,3,3,4),(2.38430817117071E-12,
7.37661520320999E-5,0.000147532581486473,0.000279867506432603),
 .UNSPECIFIED.);
#21122=B_SPLINE_CURVE_WITH_KNOTS('',3,(#93202,#93203,#93204,#93205,#93206,
#93207),.UNSPECIFIED.,.F.,.F.,(4,2,4),(1.00000000416434E-6,0.0379299702998902,
0.0758579941108125),.UNSPECIFIED.);
#21123=B_SPLINE_CURVE_WITH_KNOTS('',3,(#93209,#93210,#93211,#93212,#93213,
#93214,#93215,#93216,#93217,#93218),.UNSPECIFIED.,.F.,.F.,(4,2,2,2,4),(1.0001326989014E-6,
0.00990710921300061,0.0199202404553874,0.0400015001785639,0.0800923349002753),
 .UNSPECIFIED.);
#21124=B_SPLINE_CURVE_WITH_KNOTS('',3,(#93224,#93225,#93226,#93227,#93228,
#93229),.UNSPECIFIED.,.F.,.F.,(4,2,4),(0.,0.0163663722316209,0.0328340721658131),
 .UNSPECIFIED.);
#21125=B_SPLINE_CURVE_WITH_KNOTS('',3,(#93231,#93232,#93233,#93234,#93235,
#93236,#93237,#93238,#93239,#93240),.UNSPECIFIED.,.F.,.F.,(4,3,3,4),(2.73095436148419E-12,
7.37661519688125E-5,0.000147532581358385,0.000279867507995266),
 .UNSPECIFIED.);
#21126=B_SPLINE_CURVE_WITH_KNOTS('',3,(#93242,#93243,#93244,#93245,#93246,
#93247),.UNSPECIFIED.,.F.,.F.,(4,2,4),(1.00000000457373E-6,0.0379299703677344,
0.0758579942099292),.UNSPECIFIED.);
#21127=B_SPLINE_CURVE_WITH_KNOTS('',3,(#93249,#93250,#93251,#93252,#93253,
#93254,#93255,#93256,#93257,#93258),.UNSPECIFIED.,.F.,.F.,(4,2,2,2,4),(1.00012017720786E-6,
0.00990710919520347,0.0199202404356974,0.0400015001784051,0.0800923349040917),
 .UNSPECIFIED.);
#21128=B_SPLINE_CURVE_WITH_KNOTS('',3,(#93264,#93265,#93266,#93267,#93268,
#93269),.UNSPECIFIED.,.F.,.F.,(4,2,4),(3.83630396277799E-12,0.0163668745938823,
0.0328340565233965),.UNSPECIFIED.);
#21129=B_SPLINE_CURVE_WITH_KNOTS('',3,(#93271,#93272,#93273,#93274,#93275,
#93276,#93277,#93278,#93279,#93280),.UNSPECIFIED.,.F.,.F.,(4,3,3,4),(3.25946590633978E-12,
7.37661521820108E-5,0.000147532581786437,0.00027986750976964),
 .UNSPECIFIED.);
#21130=B_SPLINE_CURVE_WITH_KNOTS('',3,(#93282,#93283,#93284,#93285,#93286,
#93287),.UNSPECIFIED.,.F.,.F.,(4,2,4),(1.00000000415046E-6,0.0379299703148109,
0.0758579941369265),.UNSPECIFIED.);
#21131=B_SPLINE_CURVE_WITH_KNOTS('',3,(#93289,#93290,#93291,#93292,#93293,
#93294,#93295,#93296,#93297,#93298),.UNSPECIFIED.,.F.,.F.,(4,2,2,2,4),(1.00012063412176E-6,
0.00990710919855529,0.0199202404331729,0.0400015001406257,0.0800923348263209),
 .UNSPECIFIED.);
#21132=B_SPLINE_CURVE_WITH_KNOTS('',3,(#93304,#93305,#93306,#93307,#93308,
#93309),.UNSPECIFIED.,.F.,.F.,(4,2,4),(0.,0.0163668752628176,0.0328340592043943),
 .UNSPECIFIED.);
#21133=B_SPLINE_CURVE_WITH_KNOTS('',3,(#93311,#93312,#93313,#93314,#93315,
#93316,#93317,#93318,#93319,#93320),.UNSPECIFIED.,.F.,.F.,(4,3,3,4),(2.29487801882904E-12,
7.37661521139689E-5,0.000147532581650881,0.000279867507355526),
 .UNSPECIFIED.);
#21134=B_SPLINE_CURVE_WITH_KNOTS('',3,(#93322,#93323,#93324,#93325,#93326,
#93327),.UNSPECIFIED.,.F.,.F.,(4,2,4),(1.00000000393238E-6,0.0379299702930691,
0.075857994094199),.UNSPECIFIED.);
#21135=B_SPLINE_CURVE_WITH_KNOTS('',3,(#93329,#93330,#93331,#93332,#93333,
#93334,#93335,#93336,#93337,#93338),.UNSPECIFIED.,.F.,.F.,(4,2,2,2,4),(9.99989189735644E-7,
0.00990798549187738,0.0199209917267273,0.0400020007675218,0.0800923349869818),
 .UNSPECIFIED.);
#21136=B_SPLINE_CURVE_WITH_KNOTS('',3,(#93344,#93345,#93346,#93347,#93348,
#93349),.UNSPECIFIED.,.F.,.F.,(4,2,4),(0.,0.0163663702233432,0.0328340634422152),
 .UNSPECIFIED.);
#21137=B_SPLINE_CURVE_WITH_KNOTS('',3,(#93351,#93352,#93353,#93354,#93355,
#93356,#93357,#93358,#93359,#93360),.UNSPECIFIED.,.F.,.F.,(4,3,3,4),(2.84831854509737E-12,
7.37661522492544E-5,0.000147532581921937,0.000279867509387217),
 .UNSPECIFIED.);
#21138=B_SPLINE_CURVE_WITH_KNOTS('',3,(#93362,#93363,#93364,#93365,#93366,
#93367),.UNSPECIFIED.,.F.,.F.,(4,2,4),(1.00000000471945E-6,0.0379299702451825,
0.0758579940332816),.UNSPECIFIED.);
#21139=B_SPLINE_CURVE_WITH_KNOTS('',3,(#93369,#93370,#93371,#93372,#93373,
#93374,#93375,#93376,#93377,#93378),.UNSPECIFIED.,.F.,.F.,(4,2,2,2,4),(9.99982675614226E-7,
0.0099079855147948,0.0199209917696819,0.0400020008257346,0.080092335117848),
 .UNSPECIFIED.);
#21140=B_SPLINE_CURVE_WITH_KNOTS('',3,(#93384,#93385,#93386,#93387,#93388,
#93389),.UNSPECIFIED.,.F.,.F.,(4,2,4),(0.,0.0163668783924265,0.032834071637775),
 .UNSPECIFIED.);
#21141=B_SPLINE_CURVE_WITH_KNOTS('',3,(#93391,#93392,#93393,#93394,#93395,
#93396,#93397,#93398,#93399,#93400),.UNSPECIFIED.,.F.,.F.,(4,3,3,4),(3.02052600740393E-12,
7.37661515665198E-5,0.000147532580553431,0.000279867508957916),
 .UNSPECIFIED.);
#21142=B_SPLINE_CURVE_WITH_KNOTS('',3,(#93402,#93403,#93404,#93405,#93406,
#93407),.UNSPECIFIED.,.F.,.F.,(4,2,4),(1.00000000469169E-6,0.0379299703573031,
0.0758579941482047),.UNSPECIFIED.);
#21143=B_SPLINE_CURVE_WITH_KNOTS('',3,(#93409,#93410,#93411,#93412,#93413,
#93414,#93415,#93416,#93417,#93418),.UNSPECIFIED.,.F.,.F.,(4,2,2,2,4),(1.00011190317721E-6,
0.00990710920835209,0.019920240458195,0.0400015002087949,0.0800923349658839),
 .UNSPECIFIED.);
#21144=B_SPLINE_CURVE_WITH_KNOTS('',3,(#93424,#93425,#93426,#93427,#93428,
#93429),.UNSPECIFIED.,.F.,.F.,(4,2,4),(0.,0.0163663732731319,0.032834076643976),
 .UNSPECIFIED.);
#21145=B_SPLINE_CURVE_WITH_KNOTS('',3,(#93431,#93432,#93433,#93434,#93435,
#93436,#93437,#93438,#93439,#93440),.UNSPECIFIED.,.F.,.F.,(4,3,3,4),(2.40629713607431E-12,
7.3766152893624E-5,0.000147532583211465,0.000279867506089791),
 .UNSPECIFIED.);
#21146=B_SPLINE_CURVE_WITH_KNOTS('',3,(#93442,#93443,#93444,#93445,#93446,
#93447),.UNSPECIFIED.,.F.,.F.,(4,2,4),(1.00000000385909E-6,0.0379299702449765,
0.0758579940418474),.UNSPECIFIED.);
#21147=B_SPLINE_CURVE_WITH_KNOTS('',3,(#93449,#93450,#93451,#93452,#93453,
#93454,#93455,#93456,#93457,#93458),.UNSPECIFIED.,.F.,.F.,(4,2,2,2,4),(1.00016638365941E-6,
0.00990710918754969,0.0199202404186389,0.0400015001540122,0.0800923348470809),
 .UNSPECIFIED.);
#21148=B_SPLINE_CURVE_WITH_KNOTS('',3,(#93464,#93465,#93466,#93467,#93468,
#93469),.UNSPECIFIED.,.F.,.F.,(4,2,4),(0.,0.0163668772734967,0.0328340674544946),
 .UNSPECIFIED.);
#21149=B_SPLINE_CURVE_WITH_KNOTS('',3,(#93471,#93472,#93473,#93474,#93475,
#93476,#93477,#93478,#93479,#93480),.UNSPECIFIED.,.F.,.F.,(4,3,3,4),(2.7020001199329E-12,
7.37661511205436E-5,0.000147532579662811,0.000279867506975402),
 .UNSPECIFIED.);
#21150=B_SPLINE_CURVE_WITH_KNOTS('',3,(#93482,#93483,#93484,#93485,#93486,
#93487),.UNSPECIFIED.,.F.,.F.,(4,2,4),(1.00000000378671E-6,0.0379299702724514,
0.0758579940657682),.UNSPECIFIED.);
#21151=B_SPLINE_CURVE_WITH_KNOTS('',3,(#93489,#93490,#93491,#93492,#93493,
#93494,#93495,#93496,#93497,#93498),.UNSPECIFIED.,.F.,.F.,(4,2,2,2,4),(1.00012567259566E-6,
0.00990710919527812,0.0199202404298848,0.0400015001616016,0.0800923348642403),
 .UNSPECIFIED.);
#21152=B_SPLINE_CURVE_WITH_KNOTS('',3,(#93504,#93505,#93506,#93507,#93508,
#93509),.UNSPECIFIED.,.F.,.F.,(4,2,4),(0.,0.0163668767440042,0.0328340647550787),
 .UNSPECIFIED.);
#21153=B_SPLINE_CURVE_WITH_KNOTS('',3,(#93511,#93512,#93513,#93514,#93515,
#93516,#93517,#93518,#93519,#93520),.UNSPECIFIED.,.F.,.F.,(4,3,3,4),(3.05699471743467E-12,
7.37661510434139E-5,0.000147532579507185,0.000279867509435222),
 .UNSPECIFIED.);
#21154=B_SPLINE_CURVE_WITH_KNOTS('',3,(#93522,#93523,#93524,#93525,#93526,
#93527),.UNSPECIFIED.,.F.,.F.,(4,2,4),(1.00000000405056E-6,0.0379299703561028,
0.075857994162927),.UNSPECIFIED.);
#21155=B_SPLINE_CURVE_WITH_KNOTS('',3,(#93529,#93530,#93531,#93532,#93533,
#93534,#93535,#93536,#93537,#93538),.UNSPECIFIED.,.F.,.F.,(4,2,2,2,4),(1.00011518016948E-6,
0.00990710920032543,0.0199202404477273,0.0400015002058067,0.0800923349587456),
 .UNSPECIFIED.);
#21156=B_SPLINE_CURVE_WITH_KNOTS('',3,(#93544,#93545,#93546,#93547,#93548,
#93549),.UNSPECIFIED.,.F.,.F.,(4,2,4),(0.,0.016366369401344,0.0328340610916559),
 .UNSPECIFIED.);
#21157=B_SPLINE_CURVE_WITH_KNOTS('',3,(#93551,#93552,#93553,#93554,#93555,
#93556,#93557,#93558,#93559,#93560),.UNSPECIFIED.,.F.,.F.,(4,3,3,4),(2.30225153103726E-12,
7.37661521669142E-5,0.000147532581753493,0.000279867507571026),
 .UNSPECIFIED.);
#21158=B_SPLINE_CURVE_WITH_KNOTS('',3,(#93562,#93563,#93564,#93565,#93566,
#93567),.UNSPECIFIED.,.F.,.F.,(4,2,4),(1.00000000436556E-6,0.0379299702578409,
0.0758579940974071),.UNSPECIFIED.);
#21159=B_SPLINE_CURVE_WITH_KNOTS('',3,(#93569,#93570,#93571,#93572,#93573,
#93574,#93575,#93576,#93577,#93578),.UNSPECIFIED.,.F.,.F.,(4,2,2,2,4),(1.00016793091942E-6,
0.0099071092151007,0.0199202404525576,0.0400015001511786,0.0800923348409666),
 .UNSPECIFIED.);
#21160=B_SPLINE_CURVE_WITH_KNOTS('',3,(#93584,#93585,#93586,#93587,#93588,
#93589),.UNSPECIFIED.,.F.,.F.,(4,2,4),(-0.0328438284890723,-0.0141443269679191,
-0.0109909790759362),.UNSPECIFIED.);
#21161=B_SPLINE_CURVE_WITH_KNOTS('',3,(#93594,#93595,#93596,#93597),
 .UNSPECIFIED.,.F.,.F.,(4,4),(-0.0109909790759362,0.),.UNSPECIFIED.);
#21162=B_SPLINE_CURVE_WITH_KNOTS('',3,(#93598,#93599,#93600,#93601,#93602,
#93603),.UNSPECIFIED.,.F.,.F.,(4,2,4),(-0.0270230498387851,-0.0216021935132955,
-0.016285344354504),.UNSPECIFIED.);
#21163=B_SPLINE_CURVE_WITH_KNOTS('',3,(#93612,#93613,#93614,#93615,#93616,
#93617),.UNSPECIFIED.,.F.,.F.,(4,2,4),(-0.016285344354504,-0.0148457764538674,
0.),.UNSPECIFIED.);
#21164=B_SPLINE_CURVE_WITH_KNOTS('',3,(#93618,#93619,#93620,#93621),
 .UNSPECIFIED.,.F.,.F.,(4,4),(-0.0758581196727035,-0.0592625039988469),
 .UNSPECIFIED.);
#21165=B_SPLINE_CURVE_WITH_KNOTS('',3,(#93643,#93644,#93645,#93646,#93647,
#93648),.UNSPECIFIED.,.F.,.F.,(4,2,4),(9.99999999955596E-7,0.0185727541481888,
0.0324222158011904),.UNSPECIFIED.);
#21166=B_SPLINE_CURVE_WITH_KNOTS('',3,(#93654,#93655,#93656,#93657,#93658,
#93659,#93660,#93661,#93662,#93663),.UNSPECIFIED.,.F.,.F.,(4,2,2,2,4),(1.00000000424299E-6,
0.0379563433916625,0.0569679482505531,0.0664477168182853,0.0758271106987986),
 .UNSPECIFIED.);
#21167=B_SPLINE_CURVE_WITH_KNOTS('',3,(#93665,#93666,#93667,#93668,#93669,
#93670),.UNSPECIFIED.,.F.,.F.,(4,2,4),(4.06438238585956E-10,0.0379279704158864,
0.0758568871894573),.UNSPECIFIED.);
#21168=B_SPLINE_CURVE_WITH_KNOTS('',3,(#93672,#93673,#93674,#93675,#93676,
#93677),.UNSPECIFIED.,.F.,.F.,(4,2,4),(4.33743085104919E-12,0.0139935348994338,
0.0280841169043245),.UNSPECIFIED.);
#21169=B_SPLINE_CURVE_WITH_KNOTS('',3,(#93679,#93680,#93681,#93682,#93683,
#93684),.UNSPECIFIED.,.F.,.F.,(4,2,4),(9.99999224806747E-7,0.0162155345072075,
0.0323312975240217),.UNSPECIFIED.);
#21170=B_SPLINE_CURVE_WITH_KNOTS('',3,(#93690,#93691,#93692,#93693,#93694,
#93695,#93696,#93697,#93698,#93699),.UNSPECIFIED.,.F.,.F.,(4,2,2,2,4),(1.00000000407308E-6,
0.0379563433696533,0.0569679482437729,0.0664477168002803,0.0758271106578579),
 .UNSPECIFIED.);
#21171=B_SPLINE_CURVE_WITH_KNOTS('',3,(#93701,#93702,#93703,#93704,#93705,
#93706),.UNSPECIFIED.,.F.,.F.,(4,2,4),(4.06757014420253E-10,0.0379279703868986,
0.0758568871285899),.UNSPECIFIED.);
#21172=B_SPLINE_CURVE_WITH_KNOTS('',3,(#93708,#93709,#93710,#93711,#93712,
#93713),.UNSPECIFIED.,.F.,.F.,(4,2,4),(6.99834882007157E-12,0.013993537777293,
0.0280841250980986),.UNSPECIFIED.);
#21173=B_SPLINE_CURVE_WITH_KNOTS('',3,(#93715,#93716,#93717,#93718,#93719,
#93720),.UNSPECIFIED.,.F.,.F.,(4,2,4),(9.99999224629494E-7,0.0162155364639106,
0.0323313007103116),.UNSPECIFIED.);
#21174=B_SPLINE_CURVE_WITH_KNOTS('',3,(#93726,#93727,#93728,#93729,#93730,
#93731,#93732,#93733,#93734,#93735),.UNSPECIFIED.,.F.,.F.,(4,2,2,2,4),(1.00000000378622E-6,
0.037956817286507,0.0569686595417362,0.0664485464642953,0.0758271106620216),
 .UNSPECIFIED.);
#21175=B_SPLINE_CURVE_WITH_KNOTS('',3,(#93737,#93738,#93739,#93740,#93741,
#93742),.UNSPECIFIED.,.F.,.F.,(4,2,4),(4.63120919050251E-10,0.0379279704591495,
0.0758568871468356),.UNSPECIFIED.);
#21176=B_SPLINE_CURVE_WITH_KNOTS('',3,(#93744,#93745,#93746,#93747,#93748,
#93749),.UNSPECIFIED.,.F.,.F.,(4,2,4),(8.63811169450238E-12,0.0139935396137458,
0.0280841305290667),.UNSPECIFIED.);
#21177=B_SPLINE_CURVE_WITH_KNOTS('',3,(#93751,#93752,#93753,#93754,#93755,
#93756),.UNSPECIFIED.,.F.,.F.,(4,2,4),(9.99999224316896E-7,0.0162160349179906,
0.0323312991030676),.UNSPECIFIED.);
#21178=B_SPLINE_CURVE_WITH_KNOTS('',3,(#93762,#93763,#93764,#93765,#93766,
#93767,#93768,#93769,#93770,#93771),.UNSPECIFIED.,.F.,.F.,(4,2,2,2,4),(1.00000000406093E-6,
0.037956343374081,0.0569679482574388,0.0664477168139411,0.0758271106626968),
 .UNSPECIFIED.);
#21179=B_SPLINE_CURVE_WITH_KNOTS('',3,(#93773,#93774,#93775,#93776,#93777,
#93778),.UNSPECIFIED.,.F.,.F.,(4,2,4),(3.92675587073167E-10,0.037927970360737,
0.0758568871110415),.UNSPECIFIED.);
#21180=B_SPLINE_CURVE_WITH_KNOTS('',3,(#93780,#93781,#93782,#93783,#93784,
#93785),.UNSPECIFIED.,.F.,.F.,(4,2,4),(1.58913783375628E-11,0.0139935478892337,
0.0280841525392221),.UNSPECIFIED.);
#21181=B_SPLINE_CURVE_WITH_KNOTS('',3,(#93787,#93788,#93789,#93790,#93791,
#93792),.UNSPECIFIED.,.F.,.F.,(4,2,4),(9.99999224520166E-7,0.0162155358781851,
0.0323312933119785),.UNSPECIFIED.);
#21182=B_SPLINE_CURVE_WITH_KNOTS('',3,(#93798,#93799,#93800,#93801,#93802,
#93803,#93804,#93805,#93806,#93807),.UNSPECIFIED.,.F.,.F.,(4,2,2,2,4),(1.00000000369756E-6,
0.0379563434110503,0.0569679482969297,0.0664477168651638,0.0758271107410538),
 .UNSPECIFIED.);
#21183=B_SPLINE_CURVE_WITH_KNOTS('',3,(#93809,#93810,#93811,#93812,#93813,
#93814),.UNSPECIFIED.,.F.,.F.,(4,2,4),(3.99842486074308E-10,0.0379279703576063,
0.0758568870804365),.UNSPECIFIED.);
#21184=B_SPLINE_CURVE_WITH_KNOTS('',3,(#93816,#93817,#93818,#93819,#93820,
#93821),.UNSPECIFIED.,.F.,.F.,(4,2,4),(1.22693307893903E-11,0.0139935437268641,
0.0280841401722759),.UNSPECIFIED.);
#21185=B_SPLINE_CURVE_WITH_KNOTS('',3,(#93823,#93824,#93825,#93826,#93827,
#93828),.UNSPECIFIED.,.F.,.F.,(4,2,4),(9.99999224684185E-7,0.0162155357538767,
0.0323312957951966),.UNSPECIFIED.);
#21186=B_SPLINE_CURVE_WITH_KNOTS('',3,(#93834,#93835,#93836,#93837,#93838,
#93839,#93840,#93841,#93842,#93843),.UNSPECIFIED.,.F.,.F.,(4,2,2,2,4),(1.00000000379667E-6,
0.0379563433696758,0.0569679482212681,0.0664477167812651,0.0758271106479268),
 .UNSPECIFIED.);
#21187=B_SPLINE_CURVE_WITH_KNOTS('',3,(#93845,#93846,#93847,#93848,#93849,
#93850),.UNSPECIFIED.,.F.,.F.,(4,2,4),(4.67025503490487E-10,0.037927970471215,
0.0758568871651145),.UNSPECIFIED.);
#21188=B_SPLINE_CURVE_WITH_KNOTS('',3,(#93852,#93853,#93854,#93855,#93856,
#93857),.UNSPECIFIED.,.F.,.F.,(4,2,4),(3.51810538021842E-12,0.0139935355162212,
0.0280841208099387),.UNSPECIFIED.);
#21189=B_SPLINE_CURVE_WITH_KNOTS('',3,(#93859,#93860,#93861,#93862,#93863,
#93864),.UNSPECIFIED.,.F.,.F.,(4,2,4),(9.999992243271E-7,0.016216036316379,
0.0323313046569059),.UNSPECIFIED.);
#21190=B_SPLINE_CURVE_WITH_KNOTS('',3,(#93870,#93871,#93872,#93873,#93874,
#93875,#93876,#93877,#93878,#93879),.UNSPECIFIED.,.F.,.F.,(4,2,2,2,4),(1.00000000425964E-6,
0.037956817259286,0.0569686594990577,0.0664485464162528,0.0758271106124966),
 .UNSPECIFIED.);
#21191=B_SPLINE_CURVE_WITH_KNOTS('',3,(#93881,#93882,#93883,#93884,#93885,
#93886),.UNSPECIFIED.,.F.,.F.,(4,2,4),(3.68350940632322E-10,0.0379279703483229,
0.0758568871354953),.UNSPECIFIED.);
#21192=B_SPLINE_CURVE_WITH_KNOTS('',3,(#93888,#93889,#93890,#93891,#93892,
#93893),.UNSPECIFIED.,.F.,.F.,(4,2,4),(2.49236911550552E-12,0.0139935338696049,
0.0280841166260514),.UNSPECIFIED.);
#21193=B_SPLINE_CURVE_WITH_KNOTS('',3,(#93895,#93896,#93897,#93898,#93899,
#93900),.UNSPECIFIED.,.F.,.F.,(4,2,4),(9.99999224696981E-7,0.0162155368944896,
0.0323313032520044),.UNSPECIFIED.);
#21194=B_SPLINE_CURVE_WITH_KNOTS('',3,(#93906,#93907,#93908,#93909,#93910,
#93911,#93912,#93913,#93914,#93915),.UNSPECIFIED.,.F.,.F.,(4,2,2,2,4),(1.00000000432823E-6,
0.0379563433944539,0.0569679482649521,0.0664477168316037,0.0758271107060209),
 .UNSPECIFIED.);
#21195=B_SPLINE_CURVE_WITH_KNOTS('',3,(#93917,#93918,#93919,#93920,#93921,
#93922),.UNSPECIFIED.,.F.,.F.,(4,2,4),(4.41129519225011E-10,0.0379279704414067,
0.0758568871645413),.UNSPECIFIED.);
#21196=B_SPLINE_CURVE_WITH_KNOTS('',3,(#93924,#93925,#93926,#93927,#93928,
#93929),.UNSPECIFIED.,.F.,.F.,(4,2,4),(0.,0.013993531306137,0.0280841099083931),
 .UNSPECIFIED.);
#21197=B_SPLINE_CURVE_WITH_KNOTS('',3,(#93931,#93932,#93933,#93934,#93935,
#93936),.UNSPECIFIED.,.F.,.F.,(4,2,4),(9.99999224281765E-7,0.0162160348181736,
0.032331303545734),.UNSPECIFIED.);
#21198=B_SPLINE_CURVE_WITH_KNOTS('',3,(#93942,#93943,#93944,#93945,#93946,
#93947,#93948,#93949,#93950,#93951),.UNSPECIFIED.,.F.,.F.,(4,2,2,2,4),(1.00000000356021E-6,
0.0379563433798304,0.0569679482573238,0.0664477168162998,0.0758271106759946),
 .UNSPECIFIED.);
#21199=B_SPLINE_CURVE_WITH_KNOTS('',3,(#93953,#93954,#93955,#93956,#93957,
#93958),.UNSPECIFIED.,.F.,.F.,(4,2,4),(4.1900957551012E-10,0.0379279704210826,
0.0758568871645112),.UNSPECIFIED.);
#21200=B_SPLINE_CURVE_WITH_KNOTS('',3,(#93960,#93961,#93962,#93963,#93964,
#93965),.UNSPECIFIED.,.F.,.F.,(4,2,4),(1.24119165113354E-11,0.0139935438438368,
0.0280841407058771),.UNSPECIFIED.);
#21201=B_SPLINE_CURVE_WITH_KNOTS('',3,(#93967,#93968,#93969,#93970,#93971,
#93972),.UNSPECIFIED.,.F.,.F.,(4,2,4),(9.99999224431024E-7,0.0162160333729869,
0.0323312937322819),.UNSPECIFIED.);
#21202=B_SPLINE_CURVE_WITH_KNOTS('',3,(#93978,#93979,#93980,#93981,#93982,
#93983,#93984,#93985,#93986,#93987),.UNSPECIFIED.,.F.,.F.,(4,2,2,2,4),(1.00000000436287E-6,
0.0379563433599197,0.056967948210949,0.0664477167676862,0.0758271106367201),
 .UNSPECIFIED.);
#21203=B_SPLINE_CURVE_WITH_KNOTS('',3,(#93989,#93990,#93991,#93992,#93993,
#93994),.UNSPECIFIED.,.F.,.F.,(4,2,4),(4.52709987453159E-10,0.0379279704650473,
0.0758568871764037),.UNSPECIFIED.);
#21204=B_SPLINE_CURVE_WITH_KNOTS('',3,(#93996,#93997,#93998,#93999,#94000,
#94001),.UNSPECIFIED.,.F.,.F.,(4,2,4),(1.71019733157448E-11,0.0139935490883922,
0.0280841550414123),.UNSPECIFIED.);
#21205=B_SPLINE_CURVE_WITH_KNOTS('',3,(#94003,#94004,#94005,#94006,#94007,
#94008),.UNSPECIFIED.,.F.,.F.,(4,2,4),(0.,0.0162146158527736,0.0323304210442275),
 .UNSPECIFIED.);
#21206=B_SPLINE_CURVE_WITH_KNOTS('',3,(#94014,#94015,#94016,#94017,#94018,
#94019,#94020,#94021,#94022,#94023),.UNSPECIFIED.,.F.,.F.,(4,2,2,2,4),(1.00000000413671E-6,
0.037956343355812,0.0569679481985058,0.0664477167564262,0.0758271106214051),
 .UNSPECIFIED.);
#21207=B_SPLINE_CURVE_WITH_KNOTS('',3,(#94025,#94026,#94027,#94028,#94029,
#94030),.UNSPECIFIED.,.F.,.F.,(4,2,4),(4.50704316609119E-10,0.0379279704742771,
0.0758568872115808),.UNSPECIFIED.);
#21208=B_SPLINE_CURVE_WITH_KNOTS('',3,(#94032,#94033,#94034,#94035,#94036,
#94037),.UNSPECIFIED.,.F.,.F.,(4,2,4),(1.1315969324254E-11,0.0139935427060249,
0.0280841376217774),.UNSPECIFIED.);
#21209=B_SPLINE_CURVE_WITH_KNOTS('',3,(#94039,#94040,#94041,#94042,#94043,
#94044),.UNSPECIFIED.,.F.,.F.,(4,2,4),(9.99999224704977E-7,0.0162160818110645,
0.0323313688967677),.UNSPECIFIED.);
#21210=B_SPLINE_CURVE_WITH_KNOTS('',3,(#94050,#94051,#94052,#94053,#94054,
#94055,#94056,#94057,#94058,#94059),.UNSPECIFIED.,.F.,.F.,(4,2,2,2,4),(1.00000000408188E-6,
0.0379568172594891,0.0569686594994689,0.06644854641549,0.07582711061623),
 .UNSPECIFIED.);
#21211=B_SPLINE_CURVE_WITH_KNOTS('',3,(#94061,#94062,#94063,#94064,#94065,
#94066),.UNSPECIFIED.,.F.,.F.,(4,2,4),(4.53942780162584E-10,0.0379279704428565,
0.0758568871390405),.UNSPECIFIED.);
#21212=B_SPLINE_CURVE_WITH_KNOTS('',3,(#94068,#94069,#94070,#94071,#94072,
#94073),.UNSPECIFIED.,.F.,.F.,(4,2,4),(9.54664759693469E-12,0.0139935407727207,
0.0280841357480742),.UNSPECIFIED.);
#21213=B_SPLINE_CURVE_WITH_KNOTS('',3,(#94075,#94076,#94077,#94078,#94079,
#94080),.UNSPECIFIED.,.F.,.F.,(4,2,4),(9.99999224540365E-7,0.0162155366783889,
0.0323312991674447),.UNSPECIFIED.);
#21214=B_SPLINE_CURVE_WITH_KNOTS('',3,(#94086,#94087,#94088,#94089,#94090,
#94091,#94092,#94093,#94094,#94095),.UNSPECIFIED.,.F.,.F.,(4,2,2,2,4),(1.00000000364162E-6,
0.0379568172549171,0.0569686594920516,0.0664485464067164,0.0758271105977281),
 .UNSPECIFIED.);
#21215=B_SPLINE_CURVE_WITH_KNOTS('',3,(#94097,#94098,#94099,#94100,#94101,
#94102),.UNSPECIFIED.,.F.,.F.,(4,2,4),(4.45560040758764E-10,0.0379279704071412,
0.0758568870806577),.UNSPECIFIED.);
#21216=B_SPLINE_CURVE_WITH_KNOTS('',3,(#94104,#94105,#94106,#94107,#94108,
#94109),.UNSPECIFIED.,.F.,.F.,(4,2,4),(1.32865392961759E-11,0.0139935448170323,
0.028084143171579),.UNSPECIFIED.);
#21217=B_SPLINE_CURVE_WITH_KNOTS('',3,(#94111,#94112,#94113,#94114,#94115,
#94116),.UNSPECIFIED.,.F.,.F.,(4,2,4),(9.99999224337034E-7,0.0162160343091742,
0.0323312950264872),.UNSPECIFIED.);
#21218=B_SPLINE_CURVE_WITH_KNOTS('',3,(#94122,#94123,#94124,#94125,#94126,
#94127,#94128,#94129,#94130,#94131),.UNSPECIFIED.,.F.,.F.,(4,2,2,2,4),(1.00000000399103E-6,
0.0379568172873199,0.0569686595159996,0.0664485464437832,0.0758271106644221),
 .UNSPECIFIED.);
#21219=B_SPLINE_CURVE_WITH_KNOTS('',3,(#94133,#94134,#94135,#94136,#94137,
#94138),.UNSPECIFIED.,.F.,.F.,(4,2,4),(4.07805439493781E-10,0.0379279703896745,
0.0758568871301433),.UNSPECIFIED.);
#21220=B_SPLINE_CURVE_WITH_KNOTS('',3,(#94140,#94141,#94142,#94143,#94144,
#94145),.UNSPECIFIED.,.F.,.F.,(4,2,4),(1.43882151926213E-11,0.0139935461168279,
0.0280841488166543),.UNSPECIFIED.);
#21221=B_SPLINE_CURVE_WITH_KNOTS('',3,(#94147,#94148,#94149,#94150,#94151,
#94152),.UNSPECIFIED.,.F.,.F.,(4,2,4),(9.99999224565596E-7,0.0162155350301745,
0.0323312922684458),.UNSPECIFIED.);
#21222=B_SPLINE_CURVE_WITH_KNOTS('',3,(#94158,#94159,#94160,#94161,#94162,
#94163,#94164,#94165,#94166,#94167),.UNSPECIFIED.,.F.,.F.,(4,2,2,2,4),(-0.0758271700234285,
-0.0664543880836614,-0.0569813146737242,-0.0379831721396834,-0.0221455761492257),
 .UNSPECIFIED.);
#21223=B_SPLINE_CURVE_WITH_KNOTS('',3,(#94172,#94173,#94174,#94175),
 .UNSPECIFIED.,.F.,.F.,(4,4),(-0.0221455761492257,-9.99999999980183E-7),
 .UNSPECIFIED.);
#21224=B_SPLINE_CURVE_WITH_KNOTS('',3,(#94177,#94178,#94179,#94180,#94181,
#94182),.UNSPECIFIED.,.F.,.F.,(4,2,4),(4.30157251214004E-10,0.0379279704161376,
0.0758568871359327),.UNSPECIFIED.);
#21225=B_SPLINE_CURVE_WITH_KNOTS('',3,(#94184,#94185,#94186,#94187,#94188,
#94189),.UNSPECIFIED.,.F.,.F.,(4,2,4),(1.12023496069153E-11,0.0139935425843184,
0.0280841373842571),.UNSPECIFIED.);
#21226=B_SPLINE_CURVE_WITH_KNOTS('',3,(#94191,#94192,#94193,#94194,#94195,
#94196),.UNSPECIFIED.,.F.,.F.,(4,2,4),(9.99999224499498E-7,0.0162160340438454,
0.0323312958745362),.UNSPECIFIED.);
#21227=B_SPLINE_CURVE_WITH_KNOTS('',3,(#94202,#94203,#94204,#94205,#94206,
#94207,#94208,#94209,#94210,#94211),.UNSPECIFIED.,.F.,.F.,(4,2,2,2,4),(1.00000000386564E-6,
0.0379563433383663,0.0569679481833149,0.0664477167348935,0.075827110588995),
 .UNSPECIFIED.);
#21228=B_SPLINE_CURVE_WITH_KNOTS('',3,(#94213,#94214,#94215,#94216,#94217,
#94218),.UNSPECIFIED.,.F.,.F.,(4,2,4),(5.00598833072905E-10,0.0379279705397505,
0.0758568872272186),.UNSPECIFIED.);
#21229=B_SPLINE_CURVE_WITH_KNOTS('',3,(#94220,#94221,#94222,#94223,#94224,
#94225),.UNSPECIFIED.,.F.,.F.,(4,2,4),(1.07902976010742E-11,0.0139935419946153,
0.0280841374988874),.UNSPECIFIED.);
#21230=B_SPLINE_CURVE_WITH_KNOTS('',3,(#94227,#94228,#94229,#94230,#94231,
#94232),.UNSPECIFIED.,.F.,.F.,(4,2,4),(9.99999224512423E-7,0.0162155368357054,
0.0323312989032803),.UNSPECIFIED.);
#21231=B_SPLINE_CURVE_WITH_KNOTS('',3,(#94238,#94239,#94240,#94241,#94242,
#94243,#94244,#94245,#94246,#94247),.UNSPECIFIED.,.F.,.F.,(4,2,2,2,4),(1.00000000413658E-6,
0.0379568172452287,0.0569686594899139,0.0664485464004263,0.075827110594861),
 .UNSPECIFIED.);
#21232=B_SPLINE_CURVE_WITH_KNOTS('',3,(#94249,#94250,#94251,#94252,#94253,
#94254),.UNSPECIFIED.,.F.,.F.,(4,2,4),(4.41601881795433E-10,0.0379279704780061,
0.0758568872380842),.UNSPECIFIED.);
#21233=B_SPLINE_CURVE_WITH_KNOTS('',3,(#94256,#94257,#94258,#94259,#94260,
#94261),.UNSPECIFIED.,.F.,.F.,(4,2,4),(1.11945846996415E-11,0.0139935425581397,
0.0280841384616102),.UNSPECIFIED.);
#21234=B_SPLINE_CURVE_WITH_KNOTS('',3,(#94263,#94264,#94265,#94266,#94267,
#94268),.UNSPECIFIED.,.F.,.F.,(4,2,4),(9.99999224334761E-7,0.0162160341154941,
0.0323312959179037),.UNSPECIFIED.);
#21235=B_SPLINE_CURVE_WITH_KNOTS('',3,(#94274,#94275,#94276,#94277,#94278,
#94279,#94280,#94281,#94282,#94283),.UNSPECIFIED.,.F.,.F.,(4,2,2,2,4),(1.00000000363513E-6,
0.0379563433668786,0.056967948246606,0.0664477168006794,0.075827110651616),
 .UNSPECIFIED.);
#21236=B_SPLINE_CURVE_WITH_KNOTS('',3,(#94285,#94286,#94287,#94288,#94289,
#94290),.UNSPECIFIED.,.F.,.F.,(4,2,4),(4.12300237846166E-10,0.0379279703799779,
0.0758568871008718),.UNSPECIFIED.);
#21237=B_SPLINE_CURVE_WITH_KNOTS('',3,(#94292,#94293,#94294,#94295,#94296,
#94297),.UNSPECIFIED.,.F.,.F.,(4,2,4),(8.75187855439104E-12,0.0139935398483156,
0.0280841287853482),.UNSPECIFIED.);
#21238=B_SPLINE_CURVE_WITH_KNOTS('',3,(#94299,#94300,#94301,#94302,#94303,
#94304),.UNSPECIFIED.,.F.,.F.,(4,2,4),(9.99999224518061E-7,0.0162155367220943,
0.0323312998042448),.UNSPECIFIED.);
#21239=B_SPLINE_CURVE_WITH_KNOTS('',3,(#94310,#94311,#94312,#94313,#94314,
#94315,#94316,#94317,#94318,#94319),.UNSPECIFIED.,.F.,.F.,(4,2,2,2,4),(1.00000000375627E-6,
0.0379568172655732,0.0569686594889428,0.0664485464097976,0.0758271106265263),
 .UNSPECIFIED.);
#21240=B_SPLINE_CURVE_WITH_KNOTS('',3,(#94321,#94322,#94323,#94324,#94325,
#94326),.UNSPECIFIED.,.F.,.F.,(4,2,4),(4.8792649542259E-10,0.0379279704959347,
0.075856887169228),.UNSPECIFIED.);
#21241=B_SPLINE_CURVE_WITH_KNOTS('',3,(#94328,#94329,#94330,#94331,#94332,
#94333),.UNSPECIFIED.,.F.,.F.,(4,2,4),(1.15848085350532E-11,0.0139935428846778,
0.0280841380768979),.UNSPECIFIED.);
#21242=B_SPLINE_CURVE_WITH_KNOTS('',3,(#94335,#94336,#94337,#94338,#94339,
#94340),.UNSPECIFIED.,.F.,.F.,(4,2,4),(9.99999224886843E-7,0.0162155815394017,
0.0323313648688343),.UNSPECIFIED.);
#21243=B_SPLINE_CURVE_WITH_KNOTS('',3,(#94346,#94347,#94348,#94349,#94350,
#94351,#94352,#94353,#94354,#94355),.UNSPECIFIED.,.F.,.F.,(4,2,2,2,4),(1.00000000377922E-6,
0.0379568172709777,0.0569686595142048,0.0664485464331935,0.0758271106440092),
 .UNSPECIFIED.);
#21244=B_SPLINE_CURVE_WITH_KNOTS('',3,(#94357,#94358,#94359,#94360,#94361,
#94362),.UNSPECIFIED.,.F.,.F.,(4,2,4),(4.02285801780176E-10,0.0379279703983211,
0.0758568871633483),.UNSPECIFIED.);
#21245=B_SPLINE_CURVE_WITH_KNOTS('',3,(#94364,#94365,#94366,#94367,#94368,
#94369),.UNSPECIFIED.,.F.,.F.,(4,2,4),(7.63640398019089E-12,0.0139935385798663,
0.0280841271630634),.UNSPECIFIED.);
#21246=B_SPLINE_CURVE_WITH_KNOTS('',3,(#94371,#94372,#94373,#94374,#94375,
#94376),.UNSPECIFIED.,.F.,.F.,(4,2,4),(9.99999224383416E-7,0.0162160350398016,
0.0323312999701239),.UNSPECIFIED.);
#21247=B_SPLINE_CURVE_WITH_KNOTS('',3,(#94382,#94383,#94384,#94385,#94386,
#94387,#94388,#94389,#94390,#94391),.UNSPECIFIED.,.F.,.F.,(4,2,2,2,4),(1.00000000414352E-6,
0.0379568172834359,0.0569686595273031,0.0664485464513015,0.075827110649782),
 .UNSPECIFIED.);
#21248=B_SPLINE_CURVE_WITH_KNOTS('',3,(#94393,#94394,#94395,#94396,#94397,
#94398),.UNSPECIFIED.,.F.,.F.,(4,2,4),(4.50592995525949E-10,0.037927970445616,
0.0758568871542498),.UNSPECIFIED.);
#21249=B_SPLINE_CURVE_WITH_KNOTS('',3,(#94400,#94401,#94402,#94403,#94404,
#94405),.UNSPECIFIED.,.F.,.F.,(4,2,4),(1.61499532360511E-11,0.0139935481505983,
0.0280841523577774),.UNSPECIFIED.);
#21250=B_SPLINE_CURVE_WITH_KNOTS('',3,(#94407,#94408,#94409,#94410,#94411,
#94412),.UNSPECIFIED.,.F.,.F.,(4,2,4),(9.99999224621297E-7,0.0162155344678765,
0.0323312900667826),.UNSPECIFIED.);
#21251=B_SPLINE_CURVE_WITH_KNOTS('',3,(#94418,#94419,#94420,#94421,#94422,
#94423,#94424,#94425,#94426,#94427),.UNSPECIFIED.,.F.,.F.,(4,2,2,2,4),(1.00000000406719E-6,
0.0379563433891528,0.0569679482616479,0.0664477168250839,0.0758271106891875),
 .UNSPECIFIED.);
#21252=B_SPLINE_CURVE_WITH_KNOTS('',3,(#94429,#94430,#94431,#94432,#94433,
#94434),.UNSPECIFIED.,.F.,.F.,(4,2,4),(4.85813906449347E-10,0.0379279704877334,
0.0758568871526431),.UNSPECIFIED.);
#21253=B_SPLINE_CURVE_WITH_KNOTS('',3,(#94436,#94437,#94438,#94439,#94440,
#94441),.UNSPECIFIED.,.F.,.F.,(4,2,4),(7.09238533573901E-12,0.0139935379133358,
0.0280841263197077),.UNSPECIFIED.);
#21254=B_SPLINE_CURVE_WITH_KNOTS('',3,(#94443,#94444,#94445,#94446,#94447,
#94448),.UNSPECIFIED.,.F.,.F.,(4,2,4),(9.99999224719861E-7,0.0162155351467326,
0.0323312974128403),.UNSPECIFIED.);
#21255=B_SPLINE_CURVE_WITH_KNOTS('',3,(#94454,#94455,#94456,#94457,#94458,
#94459,#94460,#94461,#94462,#94463),.UNSPECIFIED.,.F.,.F.,(4,2,2,2,4),(1.00000000397735E-6,
0.0379563433805459,0.0569679482540589,0.0664477168149957,0.0758271106758986),
 .UNSPECIFIED.);
#21256=B_SPLINE_CURVE_WITH_KNOTS('',3,(#94465,#94466,#94467,#94468,#94469,
#94470),.UNSPECIFIED.,.F.,.F.,(4,2,4),(4.00195118598817E-10,0.0379279703924894,
0.075856887158006),.UNSPECIFIED.);
#21257=B_SPLINE_CURVE_WITH_KNOTS('',3,(#94472,#94473,#94474,#94475,#94476,
#94477),.UNSPECIFIED.,.F.,.F.,(4,2,4),(1.06230877155031E-11,0.0139935419498799,
0.0280841336437773),.UNSPECIFIED.);
#21258=B_SPLINE_CURVE_WITH_KNOTS('',3,(#94479,#94480,#94481,#94482,#94483,
#94484),.UNSPECIFIED.,.F.,.F.,(4,2,4),(9.99999224736563E-7,0.016216079244363,
0.0323313639624725),.UNSPECIFIED.);
#21259=B_SPLINE_CURVE_WITH_KNOTS('',3,(#94490,#94491,#94492,#94493,#94494,
#94495,#94496,#94497,#94498,#94499),.UNSPECIFIED.,.F.,.F.,(4,2,2,2,4),(1.00000000417821E-6,
0.0379563433979393,0.0569679482732456,0.0664477168381609,0.0758271107099495),
 .UNSPECIFIED.);
#21260=B_SPLINE_CURVE_WITH_KNOTS('',3,(#94501,#94502,#94503,#94504,#94505,
#94506),.UNSPECIFIED.,.F.,.F.,(4,2,4),(4.0532723640096E-10,0.0379279703802278,
0.0758568871197231),.UNSPECIFIED.);
#21261=B_SPLINE_CURVE_WITH_KNOTS('',3,(#94508,#94509,#94510,#94511,#94512,
#94513),.UNSPECIFIED.,.F.,.F.,(4,2,4),(1.12206825926819E-11,0.0139935425716113,
0.028084137770905),.UNSPECIFIED.);
#21262=B_SPLINE_CURVE_WITH_KNOTS('',3,(#94515,#94516,#94517,#94518,#94519,
#94520),.UNSPECIFIED.,.F.,.F.,(4,2,4),(9.9999922448182E-7,0.0162160353978402,
0.0323312982641253),.UNSPECIFIED.);
#21263=B_SPLINE_CURVE_WITH_KNOTS('',3,(#94526,#94527,#94528,#94529,#94530,
#94531,#94532,#94533,#94534,#94535),.UNSPECIFIED.,.F.,.F.,(4,2,2,2,4),(1.00000000387064E-6,
0.0379568172584223,0.0569686594876483,0.0664485464050056,0.075827110600589),
 .UNSPECIFIED.);
#21264=B_SPLINE_CURVE_WITH_KNOTS('',3,(#94537,#94538,#94539,#94540,#94541,
#94542),.UNSPECIFIED.,.F.,.F.,(4,2,4),(4.12888251482128E-10,0.0379279704138806,
0.0758568871648448),.UNSPECIFIED.);
#21265=B_SPLINE_CURVE_WITH_KNOTS('',3,(#94544,#94545,#94546,#94547,#94548,
#94549),.UNSPECIFIED.,.F.,.F.,(4,2,4),(0.,0.0139935332973863,0.0280841151669687),
 .UNSPECIFIED.);
#21266=B_SPLINE_CURVE_WITH_KNOTS('',3,(#94551,#94552,#94553,#94554,#94555,
#94556),.UNSPECIFIED.,.F.,.F.,(4,2,4),(9.99999224551354E-7,0.0162155349792288,
0.0323312997435385),.UNSPECIFIED.);
#21267=B_SPLINE_CURVE_WITH_KNOTS('',3,(#94562,#94563,#94564,#94565,#94566,
#94567,#94568,#94569,#94570,#94571),.UNSPECIFIED.,.F.,.F.,(4,2,2,2,4),(1.00000000356798E-6,
0.0379568172412224,0.0569686594552851,0.0664485463696981,0.0758271105702251),
 .UNSPECIFIED.);
#21268=B_SPLINE_CURVE_WITH_KNOTS('',3,(#94573,#94574,#94575,#94576,#94577,
#94578),.UNSPECIFIED.,.F.,.F.,(4,2,4),(3.64868537171598E-10,0.0379279703614429,
0.0758568871712085),.UNSPECIFIED.);
#21269=B_SPLINE_CURVE_WITH_KNOTS('',3,(#94580,#94581,#94582,#94583,#94584,
#94585),.UNSPECIFIED.,.F.,.F.,(4,2,4),(6.44180871999126E-12,0.0139935372731912,
0.0280841226769515),.UNSPECIFIED.);
#21270=B_SPLINE_CURVE_WITH_KNOTS('',3,(#94587,#94588,#94589,#94590,#94591,
#94592),.UNSPECIFIED.,.F.,.F.,(4,2,4),(9.99999224526279E-7,0.0162155344780205,
0.032331296485654),.UNSPECIFIED.);
#21271=B_SPLINE_CURVE_WITH_KNOTS('',3,(#94598,#94599,#94600,#94601,#94602,
#94603,#94604,#94605,#94606,#94607),.UNSPECIFIED.,.F.,.F.,(4,2,2,2,4),(1.00000000349721E-6,
0.0379563433579657,0.0569679482030397,0.0664477167607536,0.0758271106218004),
 .UNSPECIFIED.);
#21272=B_SPLINE_CURVE_WITH_KNOTS('',3,(#94609,#94610,#94611,#94612,#94613,
#94614),.UNSPECIFIED.,.F.,.F.,(4,2,4),(4.26548368142854E-10,0.0379279704250161,
0.0758568871602098),.UNSPECIFIED.);
#21273=B_SPLINE_CURVE_WITH_KNOTS('',3,(#94616,#94617,#94618,#94619,#94620,
#94621),.UNSPECIFIED.,.F.,.F.,(4,2,4),(3.13376810563237E-12,0.0139935334468091,
0.0280841165406132),.UNSPECIFIED.);
#21274=B_SPLINE_CURVE_WITH_KNOTS('',3,(#94623,#94624,#94625,#94626,#94627,
#94628),.UNSPECIFIED.,.F.,.F.,(4,2,4),(9.99999224127026E-7,0.0162160349129812,
0.0323313031017378),.UNSPECIFIED.);
#21275=B_SPLINE_CURVE_WITH_KNOTS('',3,(#94634,#94635,#94636,#94637,#94638,
#94639,#94640,#94641,#94642,#94643),.UNSPECIFIED.,.F.,.F.,(4,2,2,2,4),(1.00000000397699E-6,
0.0379563433877628,0.0569679482648382,0.0664477168267006,0.0758271106864307),
 .UNSPECIFIED.);
#21276=B_SPLINE_CURVE_WITH_KNOTS('',3,(#94645,#94646,#94647,#94648,#94649,
#94650),.UNSPECIFIED.,.F.,.F.,(4,2,4),(4.51041142554055E-10,0.0379279704343085,
0.0758568871257714),.UNSPECIFIED.);
#21277=B_SPLINE_CURVE_WITH_KNOTS('',3,(#94652,#94653,#94654,#94655,#94656,
#94657),.UNSPECIFIED.,.F.,.F.,(4,2,4),(1.03812220056963E-11,0.0139935416117796,
0.0280841359913486),.UNSPECIFIED.);
#21278=B_SPLINE_CURVE_WITH_KNOTS('',3,(#94659,#94660,#94661,#94662,#94663,
#94664),.UNSPECIFIED.,.F.,.F.,(4,2,4),(9.99999224857224E-7,0.0162155810644067,
0.0323313650204243),.UNSPECIFIED.);
#21279=B_SPLINE_CURVE_WITH_KNOTS('',3,(#94670,#94671,#94672,#94673,#94674,
#94675,#94676,#94677,#94678,#94679),.UNSPECIFIED.,.F.,.F.,(4,2,2,2,4),(1.0000000038219E-6,
0.0379568172482033,0.0569686594889151,0.0664485463999001,0.0758271105862111),
 .UNSPECIFIED.);
#21280=B_SPLINE_CURVE_WITH_KNOTS('',3,(#94681,#94682,#94683,#94684,#94685,
#94686),.UNSPECIFIED.,.F.,.F.,(4,2,4),(-0.0758570191918898,-0.0376794341351815,
0.),.UNSPECIFIED.);
#21281=B_SPLINE_CURVE_WITH_KNOTS('',3,(#94687,#94688,#94689,#94690,#94691,
#94692),.UNSPECIFIED.,.F.,.F.,(4,2,4),(-0.0282156346918979,-0.0107712544614244,
0.),.UNSPECIFIED.);
#21282=B_SPLINE_CURVE_WITH_KNOTS('',3,(#94700,#94701,#94702,#94703,#94704,
#94705),.UNSPECIFIED.,.F.,.F.,(4,2,4),(0.,0.0318022370756533,0.0638030678347898),
 .UNSPECIFIED.);
#21283=B_SPLINE_CURVE_WITH_KNOTS('',3,(#94706,#94707,#94708,#94709,#94710,
#94711,#94712,#94713),.UNSPECIFIED.,.F.,.F.,(4,2,2,4),(1.00002351979535E-6,
0.0322596484045106,0.048328981783262,0.0657704479132027),.UNSPECIFIED.);
#21284=B_SPLINE_CURVE_WITH_KNOTS('',3,(#94717,#94718,#94719,#94720,#94721,
#94722,#94723,#94724),.UNSPECIFIED.,.F.,.F.,(4,2,2,4),(-0.0546200763337987,
-0.0278707187231514,-0.0145797848975232,-9.99992618986541E-7),
 .UNSPECIFIED.);
#21285=B_SPLINE_CURVE_WITH_KNOTS('',3,(#94728,#94729,#94730,#94731,#94732,
#94733),.UNSPECIFIED.,.F.,.F.,(4,2,4),(0.,0.0318022364823239,0.0638030654864799),
 .UNSPECIFIED.);
#21286=B_SPLINE_CURVE_WITH_KNOTS('',3,(#94734,#94735,#94736,#94737,#94738,
#94739,#94740,#94741),.UNSPECIFIED.,.F.,.F.,(4,2,2,4),(1.00001841571144E-6,
0.032259648553329,0.0483293807870212,0.065770447844771),.UNSPECIFIED.);
#21287=B_SPLINE_CURVE_WITH_KNOTS('',3,(#94745,#94746,#94747,#94748,#94749,
#94750,#94751,#94752,#94753,#94754,#94755,#94756),.UNSPECIFIED.,.F.,.F.,
(4,2,2,2,2,4),(-0.0574506082503417,-0.0538408015157791,-0.0502541378176846,
-0.0430780609089014,-0.0287160413013061,-1.00000000285982E-6),
 .UNSPECIFIED.);
#21288=B_SPLINE_CURVE_WITH_KNOTS('',3,(#94767,#94768,#94769,#94770,#94771,
#94772),.UNSPECIFIED.,.F.,.F.,(4,2,4),(-0.0576729188689788,-0.0288412634208716,
-1.67970789167565E-9),.UNSPECIFIED.);
#21289=B_SPLINE_CURVE_WITH_KNOTS('',3,(#94774,#94775,#94776,#94777,#94778,
#94779),.UNSPECIFIED.,.F.,.F.,(4,2,4),(-0.0573169284412124,-0.0286580503374737,
-1.00000000297085E-6),.UNSPECIFIED.);
#21290=B_SPLINE_CURVE_WITH_KNOTS('',3,(#94786,#94787,#94788,#94789,#94790,
#94791,#94792,#94793),.UNSPECIFIED.,.F.,.F.,(4,2,2,4),(-0.0565385909428617,
-0.0289781083737342,-0.0150821709628815,-9.99995018437222E-7),
 .UNSPECIFIED.);
#21291=B_SPLINE_CURVE_WITH_KNOTS('',3,(#94797,#94798,#94799,#94800,#94801,
#94802),.UNSPECIFIED.,.F.,.F.,(4,2,4),(0.,0.0322203319290619,0.0646290674001349),
 .UNSPECIFIED.);
#21292=B_SPLINE_CURVE_WITH_KNOTS('',3,(#94803,#94804,#94805,#94806,#94807,
#94808,#94809,#94810),.UNSPECIFIED.,.F.,.F.,(4,2,2,4),(1.00000000422679E-6,
0.0321173160094374,0.0481218021664386,0.0656773384695804),.UNSPECIFIED.);
#21293=B_SPLINE_CURVE_WITH_KNOTS('',3,(#94814,#94815,#94816,#94817,#94818,
#94819,#94820,#94821),.UNSPECIFIED.,.F.,.F.,(4,2,2,4),(-0.0565222177897274,
-0.0287750557807116,-0.0149768293136968,-9.9999999243635E-7),
 .UNSPECIFIED.);
#21294=B_SPLINE_CURVE_WITH_KNOTS('',3,(#94825,#94826,#94827,#94828,#94829,
#94830),.UNSPECIFIED.,.F.,.F.,(4,2,4),(0.,0.0322203317627138,0.0646290667350684),
 .UNSPECIFIED.);
#21295=B_SPLINE_CURVE_WITH_KNOTS('',3,(#94831,#94832,#94833,#94834,#94835,
#94836,#94837,#94838),.UNSPECIFIED.,.F.,.F.,(4,2,2,4),(9.99991096423042E-7,
0.0321173160104707,0.0481218021604403,0.0656773383081977),.UNSPECIFIED.);
#21296=B_SPLINE_CURVE_WITH_KNOTS('',3,(#94842,#94843,#94844,#94845,#94846,
#94847),.UNSPECIFIED.,.F.,.F.,(4,2,4),(-0.0571302337105162,-0.0285614237412303,
-1.08116577482442E-7),.UNSPECIFIED.);
#21297=B_SPLINE_CURVE_WITH_KNOTS('',3,(#94852,#94853,#94854,#94855,#94856,
#94857),.UNSPECIFIED.,.F.,.F.,(4,2,4),(-0.057780362676554,-0.0288853032294261,
0.),.UNSPECIFIED.);
#21298=B_SPLINE_CURVE_WITH_KNOTS('',3,(#94867,#94868,#94869,#94870,#94871,
#94872,#94873,#94874,#94875,#94876,#94877,#94878),.UNSPECIFIED.,.F.,.F.,
(4,2,2,2,2,4),(-0.0566496423577783,-0.0283349494939652,-0.014173165215246,
-0.00709713719677714,-0.00356047877726275,-9.99998007325086E-7),
 .UNSPECIFIED.);
#21299=B_SPLINE_CURVE_WITH_KNOTS('',3,(#94882,#94883,#94884,#94885,#94886,
#94887),.UNSPECIFIED.,.F.,.F.,(4,2,4),(-0.0195678427684003,-0.0097789163088001,
-1.00000000131592E-6),.UNSPECIFIED.);
#21300=B_SPLINE_CURVE_WITH_KNOTS('',3,(#94892,#94893,#94894,#94895,#94896,
#94897,#94898,#94899,#94900,#94901,#94902,#94903),.UNSPECIFIED.,.F.,.F.,
(4,2,2,2,2,4),(-0.0561346680975214,-0.0280769187502913,-0.0140437952091259,
-0.00703222858058154,-0.00352782999598223,-9.99998002995885E-7),
 .UNSPECIFIED.);
#21301=B_SPLINE_CURVE_WITH_KNOTS('',3,(#94905,#94906,#94907,#94908,#94909,
#94910,#94911,#94912,#94913,#94914,#94915,#94916),.UNSPECIFIED.,.F.,.F.,
(4,2,2,2,2,4),(-0.0574560295636826,-0.0538528231387187,-0.0502681692185173,
-0.0430935180878714,-0.0287239461347426,-1.00000000320677E-6),
 .UNSPECIFIED.);
#21302=B_SPLINE_CURVE_WITH_KNOTS('',3,(#94919,#94920,#94921,#94922,#94923,
#94924,#94925),.UNSPECIFIED.,.F.,.F.,(4,3,4),(0.561466076970076,0.571428571428571,
0.573654350219912),.UNSPECIFIED.);
#21303=B_SPLINE_CURVE_WITH_KNOTS('',3,(#94929,#94930,#94931,#94932,#94933,
#94934),.UNSPECIFIED.,.F.,.F.,(4,2,4),(-0.0573159301739154,-0.028658877119166,
-1.49350296713147E-9),.UNSPECIFIED.);
#21304=B_SPLINE_CURVE_WITH_KNOTS('',3,(#94936,#94937,#94938,#94939,#94940,
#94941),.UNSPECIFIED.,.F.,.F.,(4,2,4),(-0.057672909991192,-0.0288316538962247,
0.),.UNSPECIFIED.);
#21305=B_SPLINE_CURVE_WITH_KNOTS('',3,(#94948,#94949,#94950,#94951,#94952,
#94953),.UNSPECIFIED.,.F.,.F.,(4,2,4),(-0.0574770388054117,-0.0287417250918333,
-8.17334270396264E-7),.UNSPECIFIED.);
#21306=B_SPLINE_CURVE_WITH_KNOTS('',3,(#94958,#94959,#94960,#94961,#94962,
#94963,#94964,#94965,#94966,#94967,#94968,#94969),.UNSPECIFIED.,.F.,.F.,
(4,2,2,2,2,4),(-0.0561043953618418,-0.0280676019824481,-0.0140500801416394,
-0.00703969588014835,-0.00353423521231409,-9.99997658238257E-7),
 .UNSPECIFIED.);
#21307=B_SPLINE_CURVE_WITH_KNOTS('',3,(#94973,#94974,#94975,#94976,#94977,
#94978),.UNSPECIFIED.,.F.,.F.,(4,2,4),(-0.057780356336134,-0.0288950562791449,
0.),.UNSPECIFIED.);
#21308=B_SPLINE_CURVE_WITH_KNOTS('',3,(#94983,#94984,#94985,#94986,#94987,
#94988),.UNSPECIFIED.,.F.,.F.,(4,2,4),(-0.0571301202613454,-0.0285688614738928,
0.),.UNSPECIFIED.);
#21309=B_SPLINE_CURVE_WITH_KNOTS('',3,(#94992,#94993,#94994,#94995,#94996,
#94997),.UNSPECIFIED.,.F.,.F.,(4,2,4),(-0.0576223282239704,-0.0288154818312603,
-4.30884426246665E-9),.UNSPECIFIED.);
#21310=B_SPLINE_CURVE_WITH_KNOTS('',3,(#94999,#95000,#95001,#95002,#95003,
#95004),.UNSPECIFIED.,.F.,.F.,(4,2,4),(-0.0573676464321654,-0.0286819361988204,
0.),.UNSPECIFIED.);
#21311=B_SPLINE_CURVE_WITH_KNOTS('',3,(#95011,#95012,#95013,#95014,#95015,
#95016),.UNSPECIFIED.,.F.,.F.,(4,2,4),(-0.0574342915312409,-0.0287114331456016,
0.),.UNSPECIFIED.);
#21312=B_SPLINE_CURVE_WITH_KNOTS('',3,(#95018,#95019,#95020,#95021,#95022,
#95023),.UNSPECIFIED.,.F.,.F.,(4,2,4),(-0.0568985403506689,-0.0284516023352449,
0.),.UNSPECIFIED.);
#21313=B_SPLINE_CURVE_WITH_KNOTS('',3,(#95025,#95026,#95027,#95028,#95029,
#95030,#95031),.UNSPECIFIED.,.F.,.F.,(4,3,4),(0.556108173865715,0.558333952657055,
0.56829644714547),.UNSPECIFIED.);
#21314=B_SPLINE_CURVE_WITH_KNOTS('',3,(#95036,#95037,#95038,#95039,#95040,
#95041,#95042,#95043,#95044,#95045,#95046,#95047),.UNSPECIFIED.,.F.,.F.,
(4,2,2,2,2,4),(-0.0570428819745678,-0.053445882283523,-0.0498799833985174,
-0.0427507600747344,-0.0285037200159628,-1.0000000026239E-6),
 .UNSPECIFIED.);
#21315=B_SPLINE_CURVE_WITH_KNOTS('',3,(#95049,#95050,#95051,#95052,#95053,
#95054,#95055),.UNSPECIFIED.,.F.,.F.,(4,3,4),(0.211502584834035,0.214285714285714,
0.223668160738941),.UNSPECIFIED.);
#21316=B_SPLINE_CURVE_WITH_KNOTS('',3,(#95058,#95059,#95060,#95061,#95062,
#95063,#95064,#95065,#95066,#95067,#95068,#95069),.UNSPECIFIED.,.F.,.F.,
(4,2,2,2,2,4),(-0.0570603956094416,-0.0285361344066156,-0.0142653177533523,
-0.00713983414874365,-0.00357971212702635,-9.99998303868496E-7),
 .UNSPECIFIED.);
#21317=B_SPLINE_CURVE_WITH_KNOTS('',3,(#95073,#95074,#95075,#95076,#95077,
#95078),.UNSPECIFIED.,.F.,.F.,(4,2,4),(-0.0568990633806027,-0.0284467206821982,
0.),.UNSPECIFIED.);
#21318=B_SPLINE_CURVE_WITH_KNOTS('',3,(#95080,#95081,#95082,#95083,#95084,
#95085),.UNSPECIFIED.,.F.,.F.,(4,2,4),(-0.0572914498457208,-0.0286510536431491,
-5.32725437971115E-7),.UNSPECIFIED.);
#21319=B_SPLINE_CURVE_WITH_KNOTS('',3,(#95088,#95089,#95090,#95091,#95092,
#95093,#95094),.UNSPECIFIED.,.F.,.F.,(4,3,4),(0.492524364188642,0.5,0.504719756176228),
 .UNSPECIFIED.);
#21320=B_SPLINE_CURVE_WITH_KNOTS('',3,(#95098,#95099,#95100,#95101,#95102,
#95103),.UNSPECIFIED.,.F.,.F.,(4,2,4),(-0.0573676595233862,-0.0286856897691478,
-3.24605807949115E-9),.UNSPECIFIED.);
#21321=B_SPLINE_CURVE_WITH_KNOTS('',3,(#95105,#95106,#95107,#95108,#95109,
#95110),.UNSPECIFIED.,.F.,.F.,(4,2,4),(-0.0576233201986482,-0.0288078428910178,
-9.99999995414337E-7),.UNSPECIFIED.);
#21322=B_SPLINE_CURVE_WITH_KNOTS('',3,(#95117,#95118,#95119,#95120,#95121,
#95122,#95123,#95124,#95125,#95126,#95127,#95128),.UNSPECIFIED.,.F.,.F.,
(4,2,2,2,2,4),(-0.0575510646040713,-0.0539361302807107,-0.0503439519248105,
-0.0431560029091156,-0.0287668658360023,-6.83499958589739E-7),
 .UNSPECIFIED.);
#21323=B_SPLINE_CURVE_WITH_KNOTS('',3,(#95133,#95134,#95135,#95136,#95137,
#95138),.UNSPECIFIED.,.F.,.F.,(4,2,4),(-0.0569454872676998,-0.0284745632844492,
0.),.UNSPECIFIED.);
#21324=B_SPLINE_CURVE_WITH_KNOTS('',3,(#95142,#95143,#95144,#95145,#95146,
#95147,#95148,#95149,#95150,#95151,#95152,#95153),.UNSPECIFIED.,.F.,.F.,
(4,2,2,2,2,4),(-0.0577515660945151,-0.0541295044023544,-0.0505262579966018,
-0.0433144621568262,-0.028870780592887,-1.00000000295003E-6),
 .UNSPECIFIED.);
#21325=B_SPLINE_CURVE_WITH_KNOTS('',3,(#95157,#95158,#95159,#95160,#95161,
#95162,#95163),.UNSPECIFIED.,.F.,.F.,(4,3,4),(0.216822083469361,0.226204530183523,
0.228987659635173),.UNSPECIFIED.);
#21326=B_SPLINE_CURVE_WITH_KNOTS('',3,(#95164,#95165,#95166,#95167,#95168,
#95169,#95170,#95171,#95172,#95173,#95174,#95175),.UNSPECIFIED.,.F.,.F.,
(4,2,2,2,2,4),(-0.0560479076491692,-0.0280423569795766,-0.014043826238136,
-0.00703895705498456,-0.0035352576931815,-9.9999747336922E-7),
 .UNSPECIFIED.);
#21327=B_SPLINE_CURVE_WITH_KNOTS('',3,(#95179,#95180,#95181,#95182,#95183,
#95184,#95185,#95186,#95187,#95188,#95189,#95190),.UNSPECIFIED.,.F.,.F.,
(4,2,2,2,2,4),(-0.0566023976945684,-0.0283201143529454,-0.0141826474504683,
-0.00710842036500782,-0.00357007369472462,-9.9999751700883E-7),
 .UNSPECIFIED.);
#21328=B_SPLINE_CURVE_WITH_KNOTS('',3,(#95192,#95193,#95194,#95195,#95196,
#95197,#95198,#95199,#95200,#95201,#95202,#95203),.UNSPECIFIED.,.F.,.F.,
(4,2,2,2,2,4),(-0.057449477443241,-0.0538288949054542,-0.0502387956155639,
-0.0430598494232536,-0.0287081071699643,-1.00000000289452E-6),
 .UNSPECIFIED.);
#21329=B_SPLINE_CURVE_WITH_KNOTS('',3,(#95210,#95211,#95212,#95213,#95214,
#95215),.UNSPECIFIED.,.F.,.F.,(4,2,4),(-0.0572909149330641,-0.0286403950999783,
0.),.UNSPECIFIED.);
#21330=B_SPLINE_CURVE_WITH_KNOTS('',3,(#95217,#95218,#95219,#95220,#95221,
#95222),.UNSPECIFIED.,.F.,.F.,(4,2,4),(-0.0568990693197607,-0.0284523472314896,
0.),.UNSPECIFIED.);
#21331=B_SPLINE_CURVE_WITH_KNOTS('',3,(#95224,#95225,#95226,#95227,#95228,
#95229,#95230),.UNSPECIFIED.,.F.,.F.,(4,3,4),(0.48715514075043,0.491874896926658,
0.499350532549397),.UNSPECIFIED.);
#21332=B_SPLINE_CURVE_WITH_KNOTS('',3,(#95235,#95236,#95237,#95238,#95239,
#95240),.UNSPECIFIED.,.F.,.F.,(4,2,4),(-0.0569334986336709,-0.028463750652435,
0.),.UNSPECIFIED.);
#21333=B_SPLINE_CURVE_WITH_KNOTS('',3,(#95242,#95243,#95244,#95245,#95246,
#95247,#95248),.UNSPECIFIED.,.F.,.F.,(4,3,4),(0.280433082999174,0.285714285714286,
0.292621536178163),.UNSPECIFIED.);
#21334=B_SPLINE_CURVE_WITH_KNOTS('',3,(#95251,#95252,#95253,#95254,#95255,
#95256),.UNSPECIFIED.,.F.,.F.,(4,2,4),(-0.0576789591924046,-0.0288354074676834,
0.),.UNSPECIFIED.);
#21335=B_SPLINE_CURVE_WITH_KNOTS('',3,(#95260,#95261,#95262,#95263,#95264,
#95265),.UNSPECIFIED.,.F.,.F.,(4,2,4),(-0.0569460402994186,-0.0284714798019895,
-5.58604225278371E-7),.UNSPECIFIED.);
#21336=B_SPLINE_CURVE_WITH_KNOTS('',3,(#95270,#95271,#95272,#95273,#95274,
#95275,#95276,#95277,#95278,#95279,#95280,#95281),.UNSPECIFIED.,.F.,.F.,
(4,2,2,2,2,4),(-0.0567857357688743,-0.0284022147232368,-0.0142045302570797,
-0.00711221946963176,-0.00356783632949885,-9.99998100444099E-7),
 .UNSPECIFIED.);
#21337=B_SPLINE_CURVE_WITH_KNOTS('',3,(#95285,#95286,#95287,#95288,#95289,
#95290,#95291,#95292,#95293,#95294,#95295,#95296),.UNSPECIFIED.,.F.,.F.,
(4,2,2,2,2,4),(-0.0562112132080888,-0.0281141846482453,-0.014059733108161,
-0.00703911312658264,-0.00353058973831441,-9.99998096606457E-7),
 .UNSPECIFIED.);
#21338=B_SPLINE_CURVE_WITH_KNOTS('',3,(#95298,#95299,#95300,#95301,#95302,
#95303),.UNSPECIFIED.,.F.,.F.,(4,2,4),(-0.0571470876313668,-0.0285778247753777,
0.),.UNSPECIFIED.);
#21339=B_SPLINE_CURVE_WITH_KNOTS('',3,(#95306,#95307,#95308,#95309,#95310,
#95311,#95312),.UNSPECIFIED.,.F.,.F.,(4,3,4),(0.42358846369814,0.428571428571429,
0.435775021750423),.UNSPECIFIED.);
#21340=B_SPLINE_CURVE_WITH_KNOTS('',3,(#95316,#95317,#95318,#95319,#95320,
#95321,#95322,#95323,#95324,#95325,#95326,#95327),.UNSPECIFIED.,.F.,.F.,
(4,2,2,2,2,4),(-0.056491689856467,-0.0282631794095709,-0.0141502161320577,
-0.00709071219975629,-0.00356034429513153,-9.99997614407541E-7),
 .UNSPECIFIED.);
#21341=B_SPLINE_CURVE_WITH_KNOTS('',3,(#95329,#95330,#95331,#95332,#95333,
#95334,#95335,#95336,#95337,#95338,#95339,#95340),.UNSPECIFIED.,.F.,.F.,
(4,2,2,2,2,4),(-0.0576025270320224,-0.0539702627479672,-0.0503692695304019,
-0.0431697930140531,-0.0287820217781061,0.),.UNSPECIFIED.);
#21342=B_SPLINE_CURVE_WITH_KNOTS('',3,(#95347,#95348,#95349,#95350,#95351,
#95352,#95353,#95354,#95355,#95356,#95357,#95358),.UNSPECIFIED.,.F.,.F.,
(4,2,2,2,2,4),(-0.0576015134966977,-0.0539845538225833,-0.0503896326973789,
-0.0431957729790647,-0.0287931162727432,-1.00000000270717E-6),
 .UNSPECIFIED.);
#21343=B_SPLINE_CURVE_WITH_KNOTS('',3,(#95362,#95363,#95364,#95365,#95366,
#95367,#95368,#95369,#95370,#95371),.UNSPECIFIED.,.F.,.F.,(4,3,3,4),(0.423693445108574,
0.425620451530082,0.435349091794206,0.435879799328077),.UNSPECIFIED.);
#21344=B_SPLINE_CURVE_WITH_KNOTS('',3,(#95372,#95373,#95374,#95375,#95376,
#95377),.UNSPECIFIED.,.F.,.F.,(4,2,4),(-0.0569012107371194,-0.0284528191557688,
0.),.UNSPECIFIED.);
#21345=B_SPLINE_CURVE_WITH_KNOTS('',3,(#95381,#95382,#95383,#95384,#95385,
#95386,#95387,#95388,#95389,#95390,#95391,#95392),.UNSPECIFIED.,.F.,.F.,
(4,2,2,2,2,4),(-0.0565652487692742,-0.0283008643122265,-0.0141717032683938,
-0.00710245601855418,-0.00356680599387045,-9.99997547592113E-7),
 .UNSPECIFIED.);
#21346=B_SPLINE_CURVE_WITH_KNOTS('',3,(#95394,#95395,#95396,#95397,#95398,
#95399,#95400,#95401,#95402,#95403,#95404,#95405),.UNSPECIFIED.,.F.,.F.,
(4,2,2,2,2,4),(-0.057501043497419,-0.0538762460046872,-0.0502825459294232,
-0.0430968152660369,-0.0287331731616107,-1.00000000260309E-6),
 .UNSPECIFIED.);
#21347=B_SPLINE_CURVE_WITH_KNOTS('',3,(#95412,#95413,#95414,#95415,#95416,
#95417),.UNSPECIFIED.,.F.,.F.,(4,2,4),(-0.0571470909339385,-0.028569266384501,
0.),.UNSPECIFIED.);
#21348=B_SPLINE_CURVE_WITH_KNOTS('',3,(#95419,#95420,#95421,#95422,#95423,
#95424,#95425,#95426,#95427,#95428,#95429,#95430),.UNSPECIFIED.,.F.,.F.,
(4,2,2,2,2,4),(-0.056963594349972,-0.0533866976743353,-0.0498311496816505,
-0.042716432598767,-0.0284736097788437,0.),.UNSPECIFIED.);
#21349=B_SPLINE_CURVE_WITH_KNOTS('',3,(#95432,#95433,#95434,#95435,#95436,
#95437,#95438),.UNSPECIFIED.,.F.,.F.,(4,3,4),(0.418382980245726,0.425586573424719,
0.430569538466614),.UNSPECIFIED.);
#21350=B_SPLINE_CURVE_WITH_KNOTS('',3,(#95443,#95444,#95445,#95446,#95447,
#95448),.UNSPECIFIED.,.F.,.F.,(4,2,4),(-0.0568968449092943,-0.02844581624333,
0.),.UNSPECIFIED.);
#21351=B_SPLINE_CURVE_WITH_KNOTS('',3,(#95450,#95451,#95452,#95453,#95454,
#95455,#95456),.UNSPECIFIED.,.F.,.F.,(4,3,4),(0.349369696074498,0.357142857142857,
0.361565077307018),.UNSPECIFIED.);
#21352=B_SPLINE_CURVE_WITH_KNOTS('',3,(#95459,#95460,#95461,#95462,#95463,
#95464),.UNSPECIFIED.,.F.,.F.,(4,2,4),(-0.0576283753952648,-0.0288101399450005,
0.),.UNSPECIFIED.);
#21353=B_SPLINE_CURVE_WITH_KNOTS('',3,(#95468,#95469,#95470,#95471,#95472,
#95473),.UNSPECIFIED.,.F.,.F.,(4,2,4),(-0.0569022074868186,-0.0284493899561334,
-1.0000000028286E-6),.UNSPECIFIED.);
#21354=B_SPLINE_CURVE_WITH_KNOTS('',3,(#95482,#95483,#95484,#95485,#95486,
#95487,#95488,#95489,#95490,#95491,#95492,#95493),.UNSPECIFIED.,.F.,.F.,
(4,2,2,2,2,4),(-0.056854015708012,-0.0284350428379476,-0.0142190433503679,
-0.00711841544860163,-0.0035700841982292,-9.99999247833419E-7),
 .UNSPECIFIED.);
#21355=B_SPLINE_CURVE_WITH_KNOTS('',3,(#95497,#95498,#95499,#95500,#95501,
#95502),.UNSPECIFIED.,.F.,.F.,(4,2,4),(-0.0570232805196483,-0.0285078556311891,
-1.09020267119453E-9),.UNSPECIFIED.);
#21356=B_SPLINE_CURVE_WITH_KNOTS('',3,(#95504,#95505,#95506,#95507,#95508,
#95509),.UNSPECIFIED.,.F.,.F.,(4,2,4),(-0.057023271731261,-0.0285154214692224,
0.),.UNSPECIFIED.);
#21357=B_SPLINE_CURVE_WITH_KNOTS('',3,(#95511,#95512,#95513,#95514,#95515,
#95516,#95517),.UNSPECIFIED.,.F.,.F.,(4,3,4),(0.349440546254527,0.359118183105585,
0.36160232099164),.UNSPECIFIED.);
#21358=B_SPLINE_CURVE_WITH_KNOTS('',3,(#95518,#95519,#95520,#95521,#95522,
#95523,#95524),.UNSPECIFIED.,.F.,.F.,(4,3,4),(0.354658719256804,0.357142857142857,
0.366820493993916),.UNSPECIFIED.);
#21359=B_SPLINE_CURVE_WITH_KNOTS('',3,(#95528,#95529,#95530,#95531,#95532,
#95533,#95534,#95535,#95536,#95537,#95538,#95539),.UNSPECIFIED.,.F.,.F.,
(4,2,2,2,2,4),(-0.0565283690570396,-0.0282817312463688,-0.0141608157756246,
-0.00709651449638661,-0.0035635432192549,-9.9999757965272E-7),
 .UNSPECIFIED.);
#21360=B_SPLINE_CURVE_WITH_KNOTS('',3,(#95541,#95542,#95543,#95544,#95545,
#95546,#95547,#95548,#95549,#95550,#95551,#95552),.UNSPECIFIED.,.F.,.F.,
(4,2,2,2,2,4),(-0.0575523718254953,-0.0539243377199946,-0.0503269858744379,
-0.0431343708071144,-0.0287586370093804,-1.00000000284595E-6),
 .UNSPECIFIED.);
#21361=B_SPLINE_CURVE_WITH_KNOTS('',3,(#95559,#95560,#95561,#95562,#95563,
#95564),.UNSPECIFIED.,.F.,.F.,(4,2,4),(-0.0576291512983601,-0.0288190103098961,
-7.73829620326349E-7),.UNSPECIFIED.);
#21362=B_SPLINE_CURVE_WITH_KNOTS('',3,(#95568,#95569,#95570,#95571,#95572,
#95573,#95574),.UNSPECIFIED.,.F.,.F.,(4,3,4),(0.354554262465766,0.35897648262994,
0.366749643698295),.UNSPECIFIED.);
#21363=B_SPLINE_CURVE_WITH_KNOTS('',3,(#95575,#95576,#95577,#95578,#95579,
#95580),.UNSPECIFIED.,.F.,.F.,(4,2,4),(-0.0568968542642774,-0.0284510332534586,
0.),.UNSPECIFIED.);
#21364=B_SPLINE_CURVE_WITH_KNOTS('',3,(#95594,#95595,#95596,#95597,#95598,
#95599),.UNSPECIFIED.,.F.,.F.,(4,2,4),(-0.0253041165894682,-0.0126519422562814,
-1.27103497865599E-9),.UNSPECIFIED.);
#21365=B_SPLINE_CURVE_WITH_KNOTS('',3,(#95619,#95620,#95621,#95622,#95623,
#95624),.UNSPECIFIED.,.F.,.F.,(4,2,4),(1.22797086782227E-9,0.0126519421698446,
0.0253041165830267),.UNSPECIFIED.);
#21366=B_SPLINE_CURVE_WITH_KNOTS('',3,(#95629,#95630,#95631,#95632,#95633,
#95634,#95635),.UNSPECIFIED.,.F.,.F.,(4,3,4),(0.354554262464466,0.35897648262994,
0.366749643698293),.UNSPECIFIED.);
#21367=B_SPLINE_CURVE_WITH_KNOTS('',3,(#95667,#95668,#95669,#95670,#95671,
#95672),.UNSPECIFIED.,.F.,.F.,(4,2,4),(1.22886243997288E-9,0.0126519421847456,
0.0253041066747003),.UNSPECIFIED.);
#21368=B_SPLINE_CURVE_WITH_KNOTS('',3,(#95677,#95678,#95679,#95680,#95681,
#95682,#95683),.UNSPECIFIED.,.F.,.F.,(4,3,4),(0.354554262465908,0.35897648262994,
0.366749643698296),.UNSPECIFIED.);
#21369=B_SPLINE_CURVE_WITH_KNOTS('',3,(#95715,#95716,#95717,#95718,#95719,
#95720),.UNSPECIFIED.,.F.,.F.,(4,2,4),(1.13389382337564E-9,0.0126519420571103,
0.0253041165505429),.UNSPECIFIED.);
#21370=B_SPLINE_CURVE_WITH_KNOTS('',3,(#95725,#95726,#95727,#95728,#95729,
#95730,#95731),.UNSPECIFIED.,.F.,.F.,(4,3,4),(0.354554262471115,0.35897648262994,
0.366749643698296),.UNSPECIFIED.);
#21371=B_SPLINE_CURVE_WITH_KNOTS('',3,(#95763,#95764,#95765,#95766,#95767,
#95768),.UNSPECIFIED.,.F.,.F.,(4,2,4),(1.25614526516976E-9,0.0126519421969114,
0.0253041165716633),.UNSPECIFIED.);
#21372=B_SPLINE_CURVE_WITH_KNOTS('',3,(#95773,#95774,#95775,#95776,#95777,
#95778,#95779),.UNSPECIFIED.,.F.,.F.,(4,3,4),(0.354554262465665,0.35897648262994,
0.366749643597688),.UNSPECIFIED.);
#21373=B_SPLINE_CURVE_WITH_KNOTS('',3,(#95811,#95812,#95813,#95814,#95815,
#95816),.UNSPECIFIED.,.F.,.F.,(4,2,4),(1.23585522307083E-9,0.0126519421620591,
0.0253041165217407),.UNSPECIFIED.);
#21374=B_SPLINE_CURVE_WITH_KNOTS('',3,(#95821,#95822,#95823,#95824,#95825,
#95826,#95827),.UNSPECIFIED.,.F.,.F.,(4,3,4),(0.354554262462879,0.35897648262994,
0.366749643698301),.UNSPECIFIED.);
#21375=B_SPLINE_CURVE_WITH_KNOTS('',3,(#95859,#95860,#95861,#95862,#95863,
#95864),.UNSPECIFIED.,.F.,.F.,(4,2,4),(1.25375314193379E-9,0.0126519422133957,
0.0253041068088959),.UNSPECIFIED.);
#21376=B_SPLINE_CURVE_WITH_KNOTS('',3,(#95869,#95870,#95871,#95872,#95873,
#95874,#95875),.UNSPECIFIED.,.F.,.F.,(4,3,4),(0.354554262465713,0.35897648262993,
0.366749643698289),.UNSPECIFIED.);
#21377=B_SPLINE_CURVE_WITH_KNOTS('',3,(#95904,#95905,#95906,#95907,#95908,
#95909),.UNSPECIFIED.,.F.,.F.,(4,2,4),(1.21054583768177E-9,0.0126519421279297,
0.0253041165445498),.UNSPECIFIED.);
#21378=B_SPLINE_CURVE_WITH_KNOTS('',3,(#95940,#95941,#95942,#95943,#95944,
#95945),.UNSPECIFIED.,.F.,.F.,(4,2,4),(1.24500010488438E-9,0.0126519422047664,
0.0253041166155102),.UNSPECIFIED.);
#21379=B_SPLINE_CURVE_WITH_KNOTS('',3,(#95950,#95951,#95952,#95953,#95954,
#95955,#95956),.UNSPECIFIED.,.F.,.F.,(4,3,4),(0.354554262464056,0.35897648262994,
0.366749643698291),.UNSPECIFIED.);
#21380=B_SPLINE_CURVE_WITH_KNOTS('',3,(#95988,#95989,#95990,#95991,#95992,
#95993),.UNSPECIFIED.,.F.,.F.,(4,2,4),(1.2271250292988E-9,0.0126519421558845,
0.0253041165535596),.UNSPECIFIED.);
#21381=B_SPLINE_CURVE_WITH_KNOTS('',3,(#95998,#95999,#96000,#96001,#96002,
#96003,#96004),.UNSPECIFIED.,.F.,.F.,(4,3,4),(0.354554262463436,0.35897648262994,
0.366749643698311),.UNSPECIFIED.);
#21382=B_SPLINE_CURVE_WITH_KNOTS('',3,(#96036,#96037,#96038,#96039,#96040,
#96041),.UNSPECIFIED.,.F.,.F.,(4,2,4),(1.14384665945145E-9,0.0126519420645045,
0.0253041165155239),.UNSPECIFIED.);
#21383=B_SPLINE_CURVE_WITH_KNOTS('',3,(#96046,#96047,#96048,#96049,#96050,
#96051,#96052),.UNSPECIFIED.,.F.,.F.,(4,3,4),(0.354554262467878,0.35897648262994,
0.366749643698312),.UNSPECIFIED.);
#21384=B_SPLINE_CURVE_WITH_KNOTS('',3,(#96084,#96085,#96086,#96087,#96088,
#96089),.UNSPECIFIED.,.F.,.F.,(4,2,4),(1.27010831980957E-9,0.0126519422191132,
0.0253041067971292),.UNSPECIFIED.);
#21385=B_SPLINE_CURVE_WITH_KNOTS('',3,(#96094,#96095,#96096,#96097,#96098,
#96099,#96100),.UNSPECIFIED.,.F.,.F.,(4,3,4),(0.354554262465897,0.35897648262994,
0.366749643698316),.UNSPECIFIED.);
#21386=B_SPLINE_CURVE_WITH_KNOTS('',3,(#96132,#96133,#96134,#96135,#96136,
#96137),.UNSPECIFIED.,.F.,.F.,(4,2,4),(1.27669895031569E-9,0.0126519422171678,
0.0253041165713666),.UNSPECIFIED.);
#21387=B_SPLINE_CURVE_WITH_KNOTS('',3,(#96142,#96143,#96144,#96145,#96146,
#96147,#96148),.UNSPECIFIED.,.F.,.F.,(4,3,4),(0.35455426246392,0.35897648262994,
0.366749643698315),.UNSPECIFIED.);
#21388=B_SPLINE_CURVE_WITH_KNOTS('',3,(#96180,#96181,#96182,#96183,#96184,
#96185),.UNSPECIFIED.,.F.,.F.,(4,2,4),(1.24828610089926E-9,0.0126519421970288,
0.025304116576285),.UNSPECIFIED.);
#21389=B_SPLINE_CURVE_WITH_KNOTS('',3,(#96190,#96191,#96192,#96193,#96194,
#96195,#96196),.UNSPECIFIED.,.F.,.F.,(4,3,4),(0.354554262462922,0.35897648262994,
0.366749643698316),.UNSPECIFIED.);
#21390=B_SPLINE_CURVE_WITH_KNOTS('',3,(#96228,#96229,#96230,#96231,#96232,
#96233),.UNSPECIFIED.,.F.,.F.,(4,2,4),(1.17451322090098E-9,0.0126519421270214,
0.0253041066457466),.UNSPECIFIED.);
#21391=B_SPLINE_CURVE_WITH_KNOTS('',3,(#96238,#96239,#96240,#96241,#96242,
#96243,#96244),.UNSPECIFIED.,.F.,.F.,(4,3,4),(0.354554262469628,0.35897648262994,
0.366749643698311),.UNSPECIFIED.);
#21392=B_SPLINE_CURVE_WITH_KNOTS('',3,(#96276,#96277,#96278,#96279,#96280,
#96281),.UNSPECIFIED.,.F.,.F.,(4,2,4),(1.25626333734773E-9,0.0126519421841047,
0.0253041165416163),.UNSPECIFIED.);
#21393=B_SPLINE_CURVE_WITH_KNOTS('',3,(#96286,#96287,#96288,#96289,#96290,
#96291,#96292),.UNSPECIFIED.,.F.,.F.,(4,3,4),(0.354554262467893,0.35897648262994,
0.366749643698315),.UNSPECIFIED.);
#21394=B_SPLINE_CURVE_WITH_KNOTS('',3,(#96324,#96325,#96326,#96327,#96328,
#96329),.UNSPECIFIED.,.F.,.F.,(4,2,4),(1.28286378602738E-9,0.0126519422213083,
0.025304116568378),.UNSPECIFIED.);
#21395=B_SPLINE_CURVE_WITH_KNOTS('',3,(#96334,#96335,#96336,#96337,#96338,
#96339,#96340),.UNSPECIFIED.,.F.,.F.,(4,3,4),(0.354554262466374,0.35897648262994,
0.366749643698312),.UNSPECIFIED.);
#21396=B_SPLINE_CURVE_WITH_KNOTS('',3,(#96372,#96373,#96374,#96375,#96376,
#96377),.UNSPECIFIED.,.F.,.F.,(4,2,4),(1.22233787626692E-9,0.0126519421803246,
0.025304106896539),.UNSPECIFIED.);
#21397=B_SPLINE_CURVE_WITH_KNOTS('',3,(#96382,#96383,#96384,#96385,#96386,
#96387,#96388),.UNSPECIFIED.,.F.,.F.,(4,3,4),(0.354554262464919,0.35897648262994,
0.366749643698291),.UNSPECIFIED.);
#21398=B_SPLINE_CURVE_WITH_KNOTS('',3,(#96420,#96421,#96422,#96423,#96424,
#96425),.UNSPECIFIED.,.F.,.F.,(4,2,4),(1.1695959771263E-9,0.0126519420867781,
0.0253041165465765),.UNSPECIFIED.);
#21399=B_SPLINE_CURVE_WITH_KNOTS('',3,(#96430,#96431,#96432,#96433,#96434,
#96435,#96436),.UNSPECIFIED.,.F.,.F.,(4,3,4),(0.354554262461511,0.35897648262994,
0.366749643698308),.UNSPECIFIED.);
#21400=B_SPLINE_CURVE_WITH_KNOTS('',3,(#96468,#96469,#96470,#96471,#96472,
#96473),.UNSPECIFIED.,.F.,.F.,(4,2,4),(1.14093229735712E-9,0.0126519420364998,
0.0253041164963297),.UNSPECIFIED.);
#21401=B_SPLINE_CURVE_WITH_KNOTS('',3,(#96478,#96479,#96480,#96481,#96482,
#96483,#96484),.UNSPECIFIED.,.F.,.F.,(4,3,4),(0.354554262463035,0.35897648262994,
0.366749643698315),.UNSPECIFIED.);
#21402=B_SPLINE_CURVE_WITH_KNOTS('',3,(#96516,#96517,#96518,#96519,#96520,
#96521),.UNSPECIFIED.,.F.,.F.,(4,2,4),(1.20804074884595E-9,0.0126519421458698,
0.0253041067969118),.UNSPECIFIED.);
#21403=B_SPLINE_CURVE_WITH_KNOTS('',3,(#96526,#96527,#96528,#96529,#96530,
#96531,#96532),.UNSPECIFIED.,.F.,.F.,(4,3,4),(0.354554262464831,0.35897648262994,
0.366749643698314),.UNSPECIFIED.);
#21404=B_SPLINE_CURVE_WITH_KNOTS('',3,(#96564,#96565,#96566,#96567,#96568,
#96569),.UNSPECIFIED.,.F.,.F.,(4,2,4),(1.27795252779781E-9,0.0126519422530381,
0.0253041068907193),.UNSPECIFIED.);
#21405=B_SPLINE_CURVE_WITH_KNOTS('',3,(#96574,#96575,#96576,#96577,#96578,
#96579,#96580),.UNSPECIFIED.,.F.,.F.,(4,3,4),(0.354554262463694,0.35897648262994,
0.366749643698315),.UNSPECIFIED.);
#21406=B_SPLINE_CURVE_WITH_KNOTS('',3,(#96612,#96613,#96614,#96615,#96616,
#96617),.UNSPECIFIED.,.F.,.F.,(4,2,4),(1.24746944309948E-9,0.0126519422080134,
0.0253041165805001),.UNSPECIFIED.);
#21407=B_SPLINE_CURVE_WITH_KNOTS('',3,(#96622,#96623,#96624,#96625,#96626,
#96627,#96628),.UNSPECIFIED.,.F.,.F.,(4,3,4),(0.354554262464067,0.35897648262994,
0.366749643698313),.UNSPECIFIED.);
#21408=B_SPLINE_CURVE_WITH_KNOTS('',3,(#96660,#96661,#96662,#96663,#96664,
#96665),.UNSPECIFIED.,.F.,.F.,(4,2,4),(1.20027758822408E-9,0.0126519421518311,
0.0253041067937676),.UNSPECIFIED.);
#21409=B_SPLINE_CURVE_WITH_KNOTS('',3,(#96670,#96671,#96672,#96673,#96674,
#96675,#96676),.UNSPECIFIED.,.F.,.F.,(4,3,4),(0.354554262466755,0.35897648262994,
0.366749643698314),.UNSPECIFIED.);
#21410=B_SPLINE_CURVE_WITH_KNOTS('',3,(#96708,#96709,#96710,#96711,#96712,
#96713),.UNSPECIFIED.,.F.,.F.,(4,2,4),(1.27554372607159E-9,0.0126519422389094,
0.0253041066678855),.UNSPECIFIED.);
#21411=B_SPLINE_CURVE_WITH_KNOTS('',3,(#96718,#96719,#96720,#96721,#96722,
#96723,#96724),.UNSPECIFIED.,.F.,.F.,(4,3,4),(0.35455426245947,0.35897648262994,
0.366749643698315),.UNSPECIFIED.);
#21412=B_SPLINE_CURVE_WITH_KNOTS('',3,(#96756,#96757,#96758,#96759,#96760,
#96761),.UNSPECIFIED.,.F.,.F.,(4,2,4),(1.1855147445423E-9,0.0126519421080607,
0.0253041145041627),.UNSPECIFIED.);
#21413=B_SPLINE_CURVE_WITH_KNOTS('',3,(#96777,#96778,#96779,#96780,#96781,
#96782,#96783),.UNSPECIFIED.,.F.,.F.,(4,3,4),(0.354554262463581,0.35897648262994,
0.366749643698313),.UNSPECIFIED.);
#21414=B_SPLINE_CURVE_WITH_KNOTS('',3,(#96804,#96805,#96806,#96807,#96808,
#96809),.UNSPECIFIED.,.F.,.F.,(4,2,4),(1.18324628300808E-9,0.0126519421085243,
0.0253041165600097),.UNSPECIFIED.);
#21415=B_SPLINE_CURVE_WITH_KNOTS('',3,(#96816,#96817,#96818,#96819,#96820,
#96821,#96822),.UNSPECIFIED.,.F.,.F.,(4,3,4),(0.354554262466107,0.358976482629941,
0.366749643597822),.UNSPECIFIED.);
#21416=B_SPLINE_CURVE_WITH_KNOTS('',3,(#96852,#96853,#96854,#96855,#96856,
#96857),.UNSPECIFIED.,.F.,.F.,(4,2,4),(1.25428146867077E-9,0.0126519422262571,
0.025304116573377),.UNSPECIFIED.);
#21417=B_SPLINE_CURVE_WITH_KNOTS('',3,(#96862,#96863,#96864,#96865,#96866,
#96867,#96868),.UNSPECIFIED.,.F.,.F.,(4,3,4),(0.354554262464714,0.35897648262994,
0.366749643698308),.UNSPECIFIED.);
#21418=B_SPLINE_CURVE_WITH_KNOTS('',3,(#96900,#96901,#96902,#96903,#96904,
#96905),.UNSPECIFIED.,.F.,.F.,(4,2,4),(1.20977334660385E-9,0.0126519421769555,
0.0253041067646983),.UNSPECIFIED.);
#21419=B_SPLINE_CURVE_WITH_KNOTS('',3,(#96910,#96911,#96912,#96913,#96914,
#96915,#96916),.UNSPECIFIED.,.F.,.F.,(4,3,4),(0.354554262461012,0.35897648262994,
0.366749643698309),.UNSPECIFIED.);
#21420=B_SPLINE_CURVE_WITH_KNOTS('',3,(#96932,#96933,#96934,#96935,#96936,
#96937,#96938),.UNSPECIFIED.,.F.,.F.,(4,3,4),(0.354554262463031,0.358976482629941,
0.366749643698308),.UNSPECIFIED.);
#21421=B_SPLINE_CURVE_WITH_KNOTS('',3,(#96969,#96970,#96971,#96972,#96973,
#96974),.UNSPECIFIED.,.F.,.F.,(4,2,4),(-0.025301896117623,-0.0126507931980699,
0.),.UNSPECIFIED.);
#21422=B_SPLINE_CURVE_WITH_KNOTS('',3,(#96991,#96992,#96993,#96994,#96995,
#96996),.UNSPECIFIED.,.F.,.F.,(4,2,4),(0.,0.0126507931358136,0.0253018398292252),
 .UNSPECIFIED.);
#21423=B_SPLINE_CURVE_WITH_KNOTS('',3,(#97027,#97028,#97029,#97030,#97031,
#97032),.UNSPECIFIED.,.F.,.F.,(4,2,4),(0.,0.0126507931414294,0.0253018407176949),
 .UNSPECIFIED.);
#21424=B_SPLINE_CURVE_WITH_KNOTS('',3,(#97063,#97064,#97065,#97066,#97067,
#97068),.UNSPECIFIED.,.F.,.F.,(4,2,4),(0.,0.0126507932051544,0.0253018397046649),
 .UNSPECIFIED.);
#21425=B_SPLINE_CURVE_WITH_KNOTS('',3,(#97099,#97100,#97101,#97102,#97103,
#97104),.UNSPECIFIED.,.F.,.F.,(4,2,4),(0.,0.0126507931990055,0.0253018403750161),
 .UNSPECIFIED.);
#21426=B_SPLINE_CURVE_WITH_KNOTS('',3,(#97135,#97136,#97137,#97138,#97139,
#97140),.UNSPECIFIED.,.F.,.F.,(4,2,4),(0.,0.0126507931801839,0.0253018454104523),
 .UNSPECIFIED.);
#21427=B_SPLINE_CURVE_WITH_KNOTS('',3,(#97171,#97172,#97173,#97174,#97175,
#97176),.UNSPECIFIED.,.F.,.F.,(4,2,4),(0.,0.0126507932159568,0.0253018398833246),
 .UNSPECIFIED.);
#21428=B_SPLINE_CURVE_WITH_KNOTS('',3,(#97207,#97208,#97209,#97210,#97211,
#97212),.UNSPECIFIED.,.F.,.F.,(4,2,4),(0.,0.0126507931255922,0.0253018388190776),
 .UNSPECIFIED.);
#21429=B_SPLINE_CURVE_WITH_KNOTS('',3,(#97243,#97244,#97245,#97246,#97247,
#97248),.UNSPECIFIED.,.F.,.F.,(4,2,4),(0.,0.0126507931615463,0.0253018378775686),
 .UNSPECIFIED.);
#21430=B_SPLINE_CURVE_WITH_KNOTS('',3,(#97279,#97280,#97281,#97282,#97283,
#97284),.UNSPECIFIED.,.F.,.F.,(4,2,4),(0.,0.0126507931939829,0.0253018409739029),
 .UNSPECIFIED.);
#21431=B_SPLINE_CURVE_WITH_KNOTS('',3,(#97315,#97316,#97317,#97318,#97319,
#97320),.UNSPECIFIED.,.F.,.F.,(4,2,4),(0.,0.0126507931551591,0.0253018408201183),
 .UNSPECIFIED.);
#21432=B_SPLINE_CURVE_WITH_KNOTS('',3,(#97351,#97352,#97353,#97354,#97355,
#97356),.UNSPECIFIED.,.F.,.F.,(4,2,4),(0.,0.0126507931660361,0.0253018422985339),
 .UNSPECIFIED.);
#21433=B_SPLINE_CURVE_WITH_KNOTS('',3,(#97387,#97388,#97389,#97390,#97391,
#97392),.UNSPECIFIED.,.F.,.F.,(4,2,4),(0.,0.0126507931795489,0.025301839656477),
 .UNSPECIFIED.);
#21434=B_SPLINE_CURVE_WITH_KNOTS('',3,(#97423,#97424,#97425,#97426,#97427,
#97428),.UNSPECIFIED.,.F.,.F.,(4,2,4),(0.,0.01265079313631,0.0253018368638526),
 .UNSPECIFIED.);
#21435=B_SPLINE_CURVE_WITH_KNOTS('',3,(#97456,#97457,#97458,#97459,#97460,
#97461),.UNSPECIFIED.,.F.,.F.,(4,2,4),(0.,0.012650792312641,0.0253018368495781),
 .UNSPECIFIED.);
#21436=B_SPLINE_CURVE_WITH_KNOTS('',3,(#97486,#97487,#97488,#97489,#97490,
#97491),.UNSPECIFIED.,.F.,.F.,(4,2,4),(0.,0.0126507931787782,0.0253018436051588),
 .UNSPECIFIED.);
#21437=B_SPLINE_CURVE_WITH_KNOTS('',3,(#97522,#97523,#97524,#97525,#97526,
#97527),.UNSPECIFIED.,.F.,.F.,(4,2,4),(0.,0.0126507932173269,0.025301841499238),
 .UNSPECIFIED.);
#21438=B_SPLINE_CURVE_WITH_KNOTS('',3,(#97558,#97559,#97560,#97561,#97562,
#97563),.UNSPECIFIED.,.F.,.F.,(4,2,4),(0.,0.0126507931648626,0.0253018400005243),
 .UNSPECIFIED.);
#21439=B_SPLINE_CURVE_WITH_KNOTS('',3,(#97594,#97595,#97596,#97597,#97598,
#97599),.UNSPECIFIED.,.F.,.F.,(4,2,4),(0.,0.0126507931986836,0.0253018399228487),
 .UNSPECIFIED.);
#21440=B_SPLINE_CURVE_WITH_KNOTS('',3,(#97630,#97631,#97632,#97633,#97634,
#97635),.UNSPECIFIED.,.F.,.F.,(4,2,4),(0.,0.0126507931659456,0.0253018397804687),
 .UNSPECIFIED.);
#21441=B_SPLINE_CURVE_WITH_KNOTS('',3,(#97666,#97667,#97668,#97669,#97670,
#97671),.UNSPECIFIED.,.F.,.F.,(4,2,4),(0.,0.0126507931509,0.0253018442887582),
 .UNSPECIFIED.);
#21442=B_SPLINE_CURVE_WITH_KNOTS('',3,(#97702,#97703,#97704,#97705,#97706,
#97707),.UNSPECIFIED.,.F.,.F.,(4,2,4),(0.,0.0126507932004658,0.0253018400813751),
 .UNSPECIFIED.);
#21443=B_SPLINE_CURVE_WITH_KNOTS('',3,(#97738,#97739,#97740,#97741,#97742,
#97743),.UNSPECIFIED.,.F.,.F.,(4,2,4),(0.,0.0126507931937709,0.0253018404936856),
 .UNSPECIFIED.);
#21444=B_SPLINE_CURVE_WITH_KNOTS('',3,(#97774,#97775,#97776,#97777,#97778,
#97779),.UNSPECIFIED.,.F.,.F.,(4,2,4),(0.,0.012650793170194,0.0253018416319173),
 .UNSPECIFIED.);
#21445=B_SPLINE_CURVE_WITH_KNOTS('',3,(#97810,#97811,#97812,#97813,#97814,
#97815),.UNSPECIFIED.,.F.,.F.,(4,2,4),(0.,0.012650793154378,0.0253018399998241),
 .UNSPECIFIED.);
#21446=B_SPLINE_CURVE_WITH_KNOTS('',3,(#97846,#97847,#97848,#97849,#97850,
#97851),.UNSPECIFIED.,.F.,.F.,(4,2,4),(0.,0.0126507931692436,0.0253018366163615),
 .UNSPECIFIED.);
#21447=B_SPLINE_CURVE_WITH_KNOTS('',3,(#97882,#97883,#97884,#97885,#97886,
#97887),.UNSPECIFIED.,.F.,.F.,(4,2,4),(0.,0.0126507931424441,0.0253018434987612),
 .UNSPECIFIED.);
#21448=B_SPLINE_CURVE_WITH_KNOTS('',3,(#97918,#97919,#97920,#97921,#97922,
#97923),.UNSPECIFIED.,.F.,.F.,(4,2,4),(0.,0.012650793177975,0.0253018389948225),
 .UNSPECIFIED.);
#21449=B_SPLINE_CURVE_WITH_KNOTS('',3,(#97954,#97955,#97956,#97957,#97958,
#97959),.UNSPECIFIED.,.F.,.F.,(4,2,4),(0.,0.0126507931974926,0.0253018394441971),
 .UNSPECIFIED.);
#21450=B_SPLINE_CURVE_WITH_KNOTS('',3,(#98001,#98002,#98003,#98004,#98005,
#98006),.UNSPECIFIED.,.F.,.F.,(4,2,4),(-0.0252968222747317,-0.0126485340355752,
-3.97891684877916E-11),.UNSPECIFIED.);
#21451=B_SPLINE_CURVE_WITH_KNOTS('',3,(#98027,#98028,#98029,#98030,#98031,
#98032),.UNSPECIFIED.,.F.,.F.,(4,2,4),(2.4930055133702E-11,0.0126487642954686,
0.0252973918365075),.UNSPECIFIED.);
#21452=B_SPLINE_CURVE_WITH_KNOTS('',3,(#98060,#98061,#98062,#98063,#98064,
#98065),.UNSPECIFIED.,.F.,.F.,(4,2,4),(1.06299847981298E-12,0.0126487806109542,
0.0252974322648405),.UNSPECIFIED.);
#21453=B_SPLINE_CURVE_WITH_KNOTS('',3,(#98093,#98094,#98095,#98096,#98097,
#98098),.UNSPECIFIED.,.F.,.F.,(4,2,4),(0.,0.0126487819673612,0.0252974355355889),
 .UNSPECIFIED.);
#21454=B_SPLINE_CURVE_WITH_KNOTS('',3,(#98126,#98127,#98128,#98129,#98130,
#98131),.UNSPECIFIED.,.F.,.F.,(4,2,4),(2.02216262117331E-11,0.0126485332971288,
0.0252968216372051),.UNSPECIFIED.);
#21455=B_SPLINE_CURVE_WITH_KNOTS('',3,(#98159,#98160,#98161,#98162,#98163,
#98164),.UNSPECIFIED.,.F.,.F.,(4,2,4),(7.79977517694186E-12,0.0126487761627237,
0.0252974213259377),.UNSPECIFIED.);
#21456=B_SPLINE_CURVE_WITH_KNOTS('',3,(#98192,#98193,#98194,#98195,#98196,
#98197),.UNSPECIFIED.,.F.,.F.,(4,2,4),(2.34210737441738E-11,0.0126485332359888,
0.0252968215446288),.UNSPECIFIED.);
#21457=B_SPLINE_CURVE_WITH_KNOTS('',3,(#98225,#98226,#98227,#98228,#98229,
#98230),.UNSPECIFIED.,.F.,.F.,(4,2,4),(1.19327002275374E-11,0.0126487730325725,
0.0252974135839664),.UNSPECIFIED.);
#21458=B_SPLINE_CURVE_WITH_KNOTS('',3,(#98253,#98254,#98255,#98256,#98257,
#98258,#98259),.UNSPECIFIED.,.F.,.F.,(4,3,4),(0.349440546428683,0.359118183105575,
0.366891343983517),.UNSPECIFIED.);
#21459=B_SPLINE_CURVE_WITH_KNOTS('',3,(#98260,#98261,#98262,#98263,#98264,
#98265),.UNSPECIFIED.,.F.,.F.,(4,2,4),(7.32486372522864E-12,0.012648776417134,
0.0252974219410064),.UNSPECIFIED.);
#21460=B_SPLINE_CURVE_WITH_KNOTS('',3,(#98293,#98294,#98295,#98296,#98297,
#98298),.UNSPECIFIED.,.F.,.F.,(4,2,4),(2.09439513833029E-11,0.0126487669063908,
0.0252973984035197),.UNSPECIFIED.);
#21461=B_SPLINE_CURVE_WITH_KNOTS('',3,(#98326,#98327,#98328,#98329,#98330,
#98331),.UNSPECIFIED.,.F.,.F.,(4,2,4),(1.75967404397773E-11,0.0126487691768794,
0.0252974041382715),.UNSPECIFIED.);
#21462=B_SPLINE_CURVE_WITH_KNOTS('',3,(#98359,#98360,#98361,#98362,#98363,
#98364),.UNSPECIFIED.,.F.,.F.,(4,2,4),(1.83356697675752E-11,0.0126485331736315,
0.0252968214947279),.UNSPECIFIED.);
#21463=B_SPLINE_CURVE_WITH_KNOTS('',3,(#98392,#98393,#98394,#98395,#98396,
#98397),.UNSPECIFIED.,.F.,.F.,(4,2,4),(0.,0.0126487818894144,0.0252974352300546),
 .UNSPECIFIED.);
#21464=B_SPLINE_CURVE_WITH_KNOTS('',3,(#98420,#98421,#98422,#98423,#98424,
#98425,#98426),.UNSPECIFIED.,.F.,.F.,(4,3,4),(0.34944054642042,0.359118183105584,
0.366891343966254),.UNSPECIFIED.);
#21465=B_SPLINE_CURVE_WITH_KNOTS('',3,(#98427,#98428,#98429,#98430,#98431,
#98432),.UNSPECIFIED.,.F.,.F.,(4,2,4),(2.2110290768274E-11,0.0126487661437097,
0.0252973965918914),.UNSPECIFIED.);
#21466=B_SPLINE_CURVE_WITH_KNOTS('',3,(#98455,#98456,#98457,#98458,#98459,
#98460,#98461),.UNSPECIFIED.,.F.,.F.,(4,3,4),(0.34944054643076,0.359118183105584,
0.366891343982794),.UNSPECIFIED.);
#21467=B_SPLINE_CURVE_WITH_KNOTS('',3,(#98462,#98463,#98464,#98465,#98466,
#98467),.UNSPECIFIED.,.F.,.F.,(4,2,4),(1.85027300324741E-11,0.0126487683840182,
0.0252974020813789),.UNSPECIFIED.);
#21468=B_SPLINE_CURVE_WITH_KNOTS('',3,(#98495,#98496,#98497,#98498,#98499,
#98500),.UNSPECIFIED.,.F.,.F.,(4,2,4),(6.19813334009103E-12,0.0126487769390593,
0.0252974231853191),.UNSPECIFIED.);
#21469=B_SPLINE_CURVE_WITH_KNOTS('',3,(#98528,#98529,#98530,#98531,#98532,
#98533),.UNSPECIFIED.,.F.,.F.,(4,2,4),(2.73609851843378E-11,0.0126485332881475,
0.0252968216301982),.UNSPECIFIED.);
#21470=B_SPLINE_CURVE_WITH_KNOTS('',3,(#98556,#98557,#98558,#98559,#98560,
#98561,#98562),.UNSPECIFIED.,.F.,.F.,(4,3,4),(0.349440546443715,0.359118183105584,
0.366891343968371),.UNSPECIFIED.);
#21471=B_SPLINE_CURVE_WITH_KNOTS('',3,(#98563,#98564,#98565,#98566,#98567,
#98568),.UNSPECIFIED.,.F.,.F.,(4,2,4),(2.1438238389322E-11,0.0126485333091484,
0.0252968216454632),.UNSPECIFIED.);
#21472=B_SPLINE_CURVE_WITH_KNOTS('',3,(#98596,#98597,#98598,#98599,#98600,
#98601),.UNSPECIFIED.,.F.,.F.,(4,2,4),(0.,0.0126487830481352,0.0252974383448801),
 .UNSPECIFIED.);
#21473=B_SPLINE_CURVE_WITH_KNOTS('',3,(#98629,#98630,#98631,#98632,#98633,
#98634),.UNSPECIFIED.,.F.,.F.,(4,2,4),(1.81243554678628E-11,0.0126485332044211,
0.0252968215077904),.UNSPECIFIED.);
#21474=B_SPLINE_CURVE_WITH_KNOTS('',3,(#98662,#98663,#98664,#98665,#98666,
#98667),.UNSPECIFIED.,.F.,.F.,(4,2,4),(2.03986063368461E-11,0.0126487673816439,
0.0252973996335729),.UNSPECIFIED.);
#21475=B_SPLINE_CURVE_WITH_KNOTS('',3,(#98695,#98696,#98697,#98698,#98699,
#98700),.UNSPECIFIED.,.F.,.F.,(4,2,4),(2.09995354766813E-11,0.0126487669715886,
0.025297398571651),.UNSPECIFIED.);
#21476=B_SPLINE_CURVE_WITH_KNOTS('',3,(#98728,#98729,#98730,#98731,#98732,
#98733),.UNSPECIFIED.,.F.,.F.,(4,2,4),(1.41098486060602E-11,0.0126487722024124,
0.0252974114970913),.UNSPECIFIED.);
#21477=B_SPLINE_CURVE_WITH_KNOTS('',3,(#98756,#98757,#98758,#98759,#98760,
#98761,#98762),.UNSPECIFIED.,.F.,.F.,(4,3,4),(0.349440546421231,0.359118183105583,
0.366891343969192),.UNSPECIFIED.);
#21478=B_SPLINE_CURVE_WITH_KNOTS('',3,(#98763,#98764,#98765,#98766,#98767,
#98768),.UNSPECIFIED.,.F.,.F.,(4,2,4),(2.14692335976709E-11,0.0126487665330256,
0.0252973975434842),.UNSPECIFIED.);
#21479=B_SPLINE_CURVE_WITH_KNOTS('',3,(#98791,#98792,#98793,#98794,#98795,
#98796,#98797),.UNSPECIFIED.,.F.,.F.,(4,3,4),(0.349440546426762,0.359118183105585,
0.36689134398469),.UNSPECIFIED.);
#21480=B_SPLINE_CURVE_WITH_KNOTS('',3,(#98798,#98799,#98800,#98801,#98802,
#98803),.UNSPECIFIED.,.F.,.F.,(4,2,4),(1.42644977650254E-11,0.0126487720073413,
0.0252974110349891),.UNSPECIFIED.);
#21481=B_SPLINE_CURVE_WITH_KNOTS('',3,(#98826,#98827,#98828,#98829,#98830,
#98831,#98832),.UNSPECIFIED.,.F.,.F.,(4,3,4),(0.349440546444724,0.359118183105575,
0.366891343976162),.UNSPECIFIED.);
#21482=B_SPLINE_CURVE_WITH_KNOTS('',3,(#98833,#98834,#98835,#98836,#98837,
#98838),.UNSPECIFIED.,.F.,.F.,(4,2,4),(2.30917275227515E-11,0.0126487657781454,
0.0252973956021664),.UNSPECIFIED.);
#21483=B_SPLINE_CURVE_WITH_KNOTS('',3,(#98866,#98867,#98868,#98869,#98870,
#98871),.UNSPECIFIED.,.F.,.F.,(4,2,4),(3.48171027160651E-12,0.0126487789656072,
0.0252974281398367),.UNSPECIFIED.);
#21484=B_SPLINE_CURVE_WITH_KNOTS('',3,(#98899,#98900,#98901,#98902,#98903,
#98904),.UNSPECIFIED.,.F.,.F.,(4,2,4),(2.39852113345501E-11,0.0126485332174892,
0.0252968215388629),.UNSPECIFIED.);
#21485=B_SPLINE_CURVE_WITH_KNOTS('',3,(#98932,#98933,#98934,#98935,#98936,
#98937),.UNSPECIFIED.,.F.,.F.,(4,2,4),(2.27914024165646E-11,0.0126487660730579,
0.025297396383094),.UNSPECIFIED.);
#21486=B_SPLINE_CURVE_WITH_KNOTS('',3,(#98959,#98960,#98961,#98962,#98963,
#98964,#98965),.UNSPECIFIED.,.F.,.F.,(4,3,4),(0.34944054635293,0.359118183105576,
0.366891343960253),.UNSPECIFIED.);
#21487=B_SPLINE_CURVE_WITH_KNOTS('',3,(#98977,#98978,#98979,#98980,#98981,
#98982),.UNSPECIFIED.,.F.,.F.,(4,2,4),(-0.0253024024802803,-0.0126513104386297,
-3.22408107156225E-11),.UNSPECIFIED.);
#21488=B_SPLINE_CURVE_WITH_KNOTS('',3,(#98992,#98993,#98994,#98995,#98996,
#98997),.UNSPECIFIED.,.F.,.F.,(4,2,4),(0.,0.0126514186993098,0.0253028391623086),
 .UNSPECIFIED.);
#21489=B_SPLINE_CURVE_WITH_KNOTS('',3,(#99017,#99018,#99019,#99020,#99021,
#99022),.UNSPECIFIED.,.F.,.F.,(4,2,4),(0.,0.0126513104266705,0.0253026028382203),
 .UNSPECIFIED.);
#21490=B_SPLINE_CURVE_WITH_KNOTS('',3,(#99042,#99043,#99044,#99045,#99046,
#99047),.UNSPECIFIED.,.F.,.F.,(4,2,4),(0.,0.0126513104352019,0.0253026054726913),
 .UNSPECIFIED.);
#21491=B_SPLINE_CURVE_WITH_KNOTS('',3,(#99067,#99068,#99069,#99070,#99071,
#99072),.UNSPECIFIED.,.F.,.F.,(4,2,4),(0.,0.0126514192705249,0.0253028843562621),
 .UNSPECIFIED.);
#21492=B_SPLINE_CURVE_WITH_KNOTS('',3,(#99092,#99093,#99094,#99095,#99096,
#99097),.UNSPECIFIED.,.F.,.F.,(4,2,4),(3.07303747784289E-11,0.0126513104659004,
0.0253025998666621),.UNSPECIFIED.);
#21493=B_SPLINE_CURVE_WITH_KNOTS('',3,(#99117,#99118,#99119,#99120,#99121,
#99122),.UNSPECIFIED.,.F.,.F.,(4,2,4),(0.,0.012651415837005,0.025302853406244),
 .UNSPECIFIED.);
#21494=B_SPLINE_CURVE_WITH_KNOTS('',3,(#99142,#99143,#99144,#99145,#99146,
#99147),.UNSPECIFIED.,.F.,.F.,(4,2,4),(3.17187722703119E-11,0.0126513104750006,
0.025302575716232),.UNSPECIFIED.);
#21495=B_SPLINE_CURVE_WITH_KNOTS('',3,(#99167,#99168,#99169,#99170,#99171,
#99172),.UNSPECIFIED.,.F.,.F.,(4,2,4),(0.,0.0126513104444747,0.0253025668836647),
 .UNSPECIFIED.);
#21496=B_SPLINE_CURVE_WITH_KNOTS('',3,(#99192,#99193,#99194,#99195,#99196,
#99197),.UNSPECIFIED.,.F.,.F.,(4,2,4),(0.,0.0126514173543735,0.0253028567149204),
 .UNSPECIFIED.);
#21497=B_SPLINE_CURVE_WITH_KNOTS('',3,(#99217,#99218,#99219,#99220,#99221,
#99222),.UNSPECIFIED.,.F.,.F.,(4,2,4),(1.21088415704605E-11,0.0126513104312721,
0.025302596907673),.UNSPECIFIED.);
#21498=B_SPLINE_CURVE_WITH_KNOTS('',3,(#99242,#99243,#99244,#99245,#99246,
#99247),.UNSPECIFIED.,.F.,.F.,(4,2,4),(0.,0.0126514160175796,0.0253028651351513),
 .UNSPECIFIED.);
#21499=B_SPLINE_CURVE_WITH_KNOTS('',3,(#99267,#99268,#99269,#99270,#99271,
#99272),.UNSPECIFIED.,.F.,.F.,(4,2,4),(0.,0.0126513104367901,0.0253025876817578),
 .UNSPECIFIED.);
#21500=B_SPLINE_CURVE_WITH_KNOTS('',3,(#99292,#99293,#99294,#99295,#99296,
#99297),.UNSPECIFIED.,.F.,.F.,(4,2,4),(1.85760836726596E-11,0.012651310426484,
0.0253026171941702),.UNSPECIFIED.);
#21501=B_SPLINE_CURVE_WITH_KNOTS('',3,(#99317,#99318,#99319,#99320,#99321,
#99322),.UNSPECIFIED.,.F.,.F.,(4,2,4),(3.0195017719144E-9,0.0126513119669391,
0.0253025600041394),.UNSPECIFIED.);
#21502=B_SPLINE_CURVE_WITH_KNOTS('',3,(#99342,#99343,#99344,#99345,#99346,
#99347),.UNSPECIFIED.,.F.,.F.,(4,2,4),(0.,0.0126514153988426,0.0253028618808356),
 .UNSPECIFIED.);
#21503=B_SPLINE_CURVE_WITH_KNOTS('',3,(#99367,#99368,#99369,#99370,#99371,
#99372),.UNSPECIFIED.,.F.,.F.,(4,2,4),(0.,0.0126514155647745,0.0253028678646022),
 .UNSPECIFIED.);
#21504=B_SPLINE_CURVE_WITH_KNOTS('',3,(#99392,#99393,#99394,#99395,#99396,
#99397),.UNSPECIFIED.,.F.,.F.,(4,2,4),(0.,0.01265141535393,0.0253028708923844),
 .UNSPECIFIED.);
#21505=B_SPLINE_CURVE_WITH_KNOTS('',3,(#99417,#99418,#99419,#99420,#99421,
#99422),.UNSPECIFIED.,.F.,.F.,(4,2,4),(0.,0.0126513104241505,0.0253026011176279),
 .UNSPECIFIED.);
#21506=B_SPLINE_CURVE_WITH_KNOTS('',3,(#99442,#99443,#99444,#99445,#99446,
#99447),.UNSPECIFIED.,.F.,.F.,(4,2,4),(0.,0.0126513104450393,0.0253025900704875),
 .UNSPECIFIED.);
#21507=B_SPLINE_CURVE_WITH_KNOTS('',3,(#99467,#99468,#99469,#99470,#99471,
#99472),.UNSPECIFIED.,.F.,.F.,(4,2,4),(0.,0.0126514181045253,0.0253028758811497),
 .UNSPECIFIED.);
#21508=B_SPLINE_CURVE_WITH_KNOTS('',3,(#99492,#99493,#99494,#99495,#99496,
#99497),.UNSPECIFIED.,.F.,.F.,(4,2,4),(0.,0.0126514168979517,0.0253028479507141),
 .UNSPECIFIED.);
#21509=B_SPLINE_CURVE_WITH_KNOTS('',3,(#99517,#99518,#99519,#99520,#99521,
#99522),.UNSPECIFIED.,.F.,.F.,(4,2,4),(1.03319412963558E-11,0.0126513104477166,
0.0253025953666836),.UNSPECIFIED.);
#21510=B_SPLINE_CURVE_WITH_KNOTS('',3,(#99542,#99543,#99544,#99545,#99546,
#99547),.UNSPECIFIED.,.F.,.F.,(4,2,4),(0.,0.0126513104317339,0.0253026134134014),
 .UNSPECIFIED.);
#21511=B_SPLINE_CURVE_WITH_KNOTS('',3,(#99567,#99568,#99569,#99570,#99571,
#99572),.UNSPECIFIED.,.F.,.F.,(4,2,4),(1.4734659535817E-11,0.0126513104749262,
0.0253025667468672),.UNSPECIFIED.);
#21512=B_SPLINE_CURVE_WITH_KNOTS('',3,(#99592,#99593,#99594,#99595,#99596,
#99597),.UNSPECIFIED.,.F.,.F.,(4,2,4),(0.,0.0126513104535364,0.025302578952868),
 .UNSPECIFIED.);
#21513=B_SPLINE_CURVE_WITH_KNOTS('',3,(#99617,#99618,#99619,#99620,#99621,
#99622),.UNSPECIFIED.,.F.,.F.,(4,2,4),(0.,0.0126514183264595,0.0253028634934918),
 .UNSPECIFIED.);
#21514=B_SPLINE_CURVE_WITH_KNOTS('',3,(#99642,#99643,#99644,#99645,#99646,
#99647),.UNSPECIFIED.,.F.,.F.,(4,2,4),(0.,0.0126513104631919,0.0253025656851542),
 .UNSPECIFIED.);
#21515=B_SPLINE_CURVE_WITH_KNOTS('',3,(#99667,#99668,#99669,#99670,#99671,
#99672),.UNSPECIFIED.,.F.,.F.,(4,2,4),(1.83621424804334E-11,0.0126513104370361,
0.0253026040775267),.UNSPECIFIED.);
#21516=B_SPLINE_CURVE_WITH_KNOTS('',3,(#99700,#99701,#99702,#99703,#99704,
#99705),.UNSPECIFIED.,.F.,.F.,(4,2,4),(-0.0252992074861097,-0.0126497276181275,
-4.51872914086771E-11),.UNSPECIFIED.);
#21517=B_SPLINE_CURVE_WITH_KNOTS('',3,(#99711,#99712,#99713,#99714,#99715,
#99716,#99717),.UNSPECIFIED.,.F.,.F.,(4,3,4),(0.34944054625452,0.359118183105574,
0.361602320900268),.UNSPECIFIED.);
#21518=B_SPLINE_CURVE_WITH_KNOTS('',3,(#99718,#99719,#99720,#99721,#99722,
#99723,#99724),.UNSPECIFIED.,.F.,.F.,(4,3,4),(0.354658719348169,0.357142857142857,
0.36682049399392),.UNSPECIFIED.);
#21519=B_SPLINE_CURVE_WITH_KNOTS('',3,(#99749,#99750,#99751,#99752,#99753,
#99754),.UNSPECIFIED.,.F.,.F.,(4,2,4),(-0.025299207529245,-0.0126497275618106,
-4.79960515775701E-11),.UNSPECIFIED.);
#21520=B_SPLINE_CURVE_WITH_KNOTS('',3,(#99760,#99761,#99762,#99763,#99764,
#99765,#99766),.UNSPECIFIED.,.F.,.F.,(4,3,4),(0.34944054625453,0.359118183105579,
0.361602320908138),.UNSPECIFIED.);
#21521=B_SPLINE_CURVE_WITH_KNOTS('',3,(#99767,#99768,#99769,#99770,#99771,
#99772,#99773),.UNSPECIFIED.,.F.,.F.,(4,3,4),(0.354658719340306,0.357142857142857,
0.366820493993925),.UNSPECIFIED.);
#21522=B_SPLINE_CURVE_WITH_KNOTS('',3,(#99798,#99799,#99800,#99801,#99802,
#99803),.UNSPECIFIED.,.F.,.F.,(4,2,4),(-0.0252992074685758,-0.0126497275506734,
0.),.UNSPECIFIED.);
#21523=B_SPLINE_CURVE_WITH_KNOTS('',3,(#99809,#99810,#99811,#99812,#99813,
#99814,#99815),.UNSPECIFIED.,.F.,.F.,(4,3,4),(0.349440546254528,0.359118183105579,
0.361602320895715),.UNSPECIFIED.);
#21524=B_SPLINE_CURVE_WITH_KNOTS('',3,(#99816,#99817,#99818,#99819,#99820,
#99821,#99822),.UNSPECIFIED.,.F.,.F.,(4,3,4),(0.354658719352732,0.357142857142857,
0.366820493993922),.UNSPECIFIED.);
#21525=B_SPLINE_CURVE_WITH_KNOTS('',3,(#99847,#99848,#99849,#99850,#99851,
#99852),.UNSPECIFIED.,.F.,.F.,(4,2,4),(-0.0252992075308213,-0.0126497276054392,
-6.4287731388335E-11),.UNSPECIFIED.);
#21526=B_SPLINE_CURVE_WITH_KNOTS('',3,(#99858,#99859,#99860,#99861,#99862,
#99863,#99864),.UNSPECIFIED.,.F.,.F.,(4,3,4),(0.349440546254525,0.359118183105574,
0.361602320910271),.UNSPECIFIED.);
#21527=B_SPLINE_CURVE_WITH_KNOTS('',3,(#99865,#99866,#99867,#99868,#99869,
#99870,#99871),.UNSPECIFIED.,.F.,.F.,(4,3,4),(0.35465871933817,0.357142857142857,
0.366820493993925),.UNSPECIFIED.);
#21528=B_SPLINE_CURVE_WITH_KNOTS('',3,(#99896,#99897,#99898,#99899,#99900,
#99901),.UNSPECIFIED.,.F.,.F.,(4,2,4),(-0.0252992075674429,-0.0126497276439361,
-7.94698716555242E-11),.UNSPECIFIED.);
#21529=B_SPLINE_CURVE_WITH_KNOTS('',3,(#99907,#99908,#99909,#99910,#99911,
#99912,#99913),.UNSPECIFIED.,.F.,.F.,(4,3,4),(0.349440546254528,0.359118183105575,
0.361602320917548),.UNSPECIFIED.);
#21530=B_SPLINE_CURVE_WITH_KNOTS('',3,(#99914,#99915,#99916,#99917,#99918,
#99919,#99920),.UNSPECIFIED.,.F.,.F.,(4,3,4),(0.354658719330895,0.357142857142857,
0.366820493993926),.UNSPECIFIED.);
#21531=B_SPLINE_CURVE_WITH_KNOTS('',3,(#99945,#99946,#99947,#99948,#99949,
#99950),.UNSPECIFIED.,.F.,.F.,(4,2,4),(-0.0252992075443036,-0.0126497275685402,
0.),.UNSPECIFIED.);
#21532=B_SPLINE_CURVE_WITH_KNOTS('',3,(#99956,#99957,#99958,#99959,#99960,
#99961,#99962),.UNSPECIFIED.,.F.,.F.,(4,3,4),(0.349440546254499,0.359118183105556,
0.361602320891685),.UNSPECIFIED.);
#21533=B_SPLINE_CURVE_WITH_KNOTS('',3,(#99963,#99964,#99965,#99966,#99967,
#99968,#99969),.UNSPECIFIED.,.F.,.F.,(4,3,4),(0.354658719356734,0.357142857142857,
0.366820493993918),.UNSPECIFIED.);
#21534=B_SPLINE_CURVE_WITH_KNOTS('',3,(#99994,#99995,#99996,#99997,#99998,
#99999),.UNSPECIFIED.,.F.,.F.,(4,2,4),(-0.0252992075564514,-0.0126497275878325,
-3.48532661065271E-11),.UNSPECIFIED.);
#21535=B_SPLINE_CURVE_WITH_KNOTS('',3,(#100005,#100006,#100007,#100008,
#100009,#100010,#100011),.UNSPECIFIED.,.F.,.F.,(4,3,4),(0.349440546254505,
0.359118183105556,0.361602320899659),.UNSPECIFIED.);
#21536=B_SPLINE_CURVE_WITH_KNOTS('',3,(#100012,#100013,#100014,#100015,
#100016,#100017,#100018),.UNSPECIFIED.,.F.,.F.,(4,3,4),(0.354658719348767,
0.357142857142857,0.366820493993923),.UNSPECIFIED.);
#21537=B_SPLINE_CURVE_WITH_KNOTS('',3,(#100043,#100044,#100045,#100046,
#100047,#100048),.UNSPECIFIED.,.F.,.F.,(4,2,4),(-0.0252992075025414,-0.0126497275798582,
-1.42233204381004E-11),.UNSPECIFIED.);
#21538=B_SPLINE_CURVE_WITH_KNOTS('',3,(#100054,#100055,#100056,#100057,
#100058,#100059,#100060),.UNSPECIFIED.,.F.,.F.,(4,3,4),(0.349440546254509,
0.359118183105557,0.361602320896234),.UNSPECIFIED.);
#21539=B_SPLINE_CURVE_WITH_KNOTS('',3,(#100061,#100062,#100063,#100064,
#100065,#100066,#100067),.UNSPECIFIED.,.F.,.F.,(4,3,4),(0.354658719352205,
0.357142857142857,0.366820493993925),.UNSPECIFIED.);
#21540=B_SPLINE_CURVE_WITH_KNOTS('',3,(#100092,#100093,#100094,#100095,
#100096,#100097),.UNSPECIFIED.,.F.,.F.,(4,2,4),(-0.0252992074674949,-0.0126497275846532,
-3.89155270508201E-11),.UNSPECIFIED.);
#21541=B_SPLINE_CURVE_WITH_KNOTS('',3,(#100103,#100104,#100105,#100106,
#100107,#100108,#100109),.UNSPECIFIED.,.F.,.F.,(4,3,4),(0.349440546254512,
0.359118183105557,0.361602320897654),.UNSPECIFIED.);
#21542=B_SPLINE_CURVE_WITH_KNOTS('',3,(#100110,#100111,#100112,#100113,
#100114,#100115,#100116),.UNSPECIFIED.,.F.,.F.,(4,3,4),(0.354658719350777,
0.357142857142857,0.366820493993927),.UNSPECIFIED.);
#21543=B_SPLINE_CURVE_WITH_KNOTS('',3,(#100141,#100142,#100143,#100144,
#100145,#100146),.UNSPECIFIED.,.F.,.F.,(4,2,4),(-0.0252992074820837,-0.012649727615419,
-2.83656396982135E-11),.UNSPECIFIED.);
#21544=B_SPLINE_CURVE_WITH_KNOTS('',3,(#100152,#100153,#100154,#100155,
#100156,#100157,#100158),.UNSPECIFIED.,.F.,.F.,(4,3,4),(0.349440546254527,
0.359118183105584,0.361602320896335),.UNSPECIFIED.);
#21545=B_SPLINE_CURVE_WITH_KNOTS('',3,(#100159,#100160,#100161,#100162,
#100163,#100164,#100165),.UNSPECIFIED.,.F.,.F.,(4,3,4),(0.354658719352108,
0.357142857142857,0.366820493993918),.UNSPECIFIED.);
#21546=B_SPLINE_CURVE_WITH_KNOTS('',3,(#100190,#100191,#100192,#100193,
#100194,#100195),.UNSPECIFIED.,.F.,.F.,(4,2,4),(-0.0252992074819737,-0.012649727562162,
-2.75737106758545E-11),.UNSPECIFIED.);
#21547=B_SPLINE_CURVE_WITH_KNOTS('',3,(#100201,#100202,#100203,#100204,
#100205,#100206,#100207),.UNSPECIFIED.,.F.,.F.,(4,3,4),(0.349440546254526,
0.359118183105584,0.361602320903358),.UNSPECIFIED.);
#21548=B_SPLINE_CURVE_WITH_KNOTS('',3,(#100208,#100209,#100210,#100211,
#100212,#100213,#100214),.UNSPECIFIED.,.F.,.F.,(4,3,4),(0.354658719345086,
0.357142857142857,0.366820493993917),.UNSPECIFIED.);
#21549=B_SPLINE_CURVE_WITH_KNOTS('',3,(#100239,#100240,#100241,#100242,
#100243,#100244),.UNSPECIFIED.,.F.,.F.,(4,2,4),(-0.0252992074565818,-0.0126497275867138,
-2.09927422667455E-11),.UNSPECIFIED.);
#21550=B_SPLINE_CURVE_WITH_KNOTS('',3,(#100250,#100251,#100252,#100253,
#100254,#100255,#100256),.UNSPECIFIED.,.F.,.F.,(4,3,4),(0.349440546254526,
0.359118183105584,0.361602320894819),.UNSPECIFIED.);
#21551=B_SPLINE_CURVE_WITH_KNOTS('',3,(#100257,#100258,#100259,#100260,
#100261,#100262,#100263),.UNSPECIFIED.,.F.,.F.,(4,3,4),(0.354658719353623,
0.357142857142857,0.366820493993916),.UNSPECIFIED.);
#21552=B_SPLINE_CURVE_WITH_KNOTS('',3,(#100288,#100289,#100290,#100291,
#100292,#100293),.UNSPECIFIED.,.F.,.F.,(4,2,4),(-0.0252992075329033,-0.0126497275798029,
-2.34377101060446E-11),.UNSPECIFIED.);
#21553=B_SPLINE_CURVE_WITH_KNOTS('',3,(#100299,#100300,#100301,#100302,
#100303,#100304,#100305),.UNSPECIFIED.,.F.,.F.,(4,3,4),(0.349440546254526,
0.359118183105585,0.361602320898788),.UNSPECIFIED.);
#21554=B_SPLINE_CURVE_WITH_KNOTS('',3,(#100306,#100307,#100308,#100309,
#100310,#100311,#100312),.UNSPECIFIED.,.F.,.F.,(4,3,4),(0.354658719349655,
0.357142857142857,0.366820493993916),.UNSPECIFIED.);
#21555=B_SPLINE_CURVE_WITH_KNOTS('',3,(#100337,#100338,#100339,#100340,
#100341,#100342),.UNSPECIFIED.,.F.,.F.,(4,2,4),(-0.0252992075070475,-0.0126497275566533,
-2.2880430189387E-11),.UNSPECIFIED.);
#21556=B_SPLINE_CURVE_WITH_KNOTS('',3,(#100348,#100349,#100350,#100351,
#100352,#100353,#100354),.UNSPECIFIED.,.F.,.F.,(4,3,4),(0.349440546254526,
0.359118183105584,0.361602320894655),.UNSPECIFIED.);
#21557=B_SPLINE_CURVE_WITH_KNOTS('',3,(#100355,#100356,#100357,#100358,
#100359,#100360,#100361),.UNSPECIFIED.,.F.,.F.,(4,3,4),(0.354658719353787,
0.357142857142857,0.366820493993916),.UNSPECIFIED.);
#21558=B_SPLINE_CURVE_WITH_KNOTS('',3,(#100383,#100384,#100385,#100386,
#100387,#100388),.UNSPECIFIED.,.F.,.F.,(4,2,4),(-0.025299207444391,-0.0126497275600756,
0.),.UNSPECIFIED.);
#21559=B_SPLINE_CURVE_WITH_KNOTS('',3,(#100414,#100415,#100416,#100417,
#100418,#100419),.UNSPECIFIED.,.F.,.F.,(4,2,4),(-0.0252992075196953,-0.0126497275585676,
0.),.UNSPECIFIED.);
#21560=B_SPLINE_CURVE_WITH_KNOTS('',3,(#100425,#100426,#100427,#100428,
#100429,#100430,#100431),.UNSPECIFIED.,.F.,.F.,(4,3,4),(0.349440546254527,
0.359118183105584,0.361602320894789),.UNSPECIFIED.);
#21561=B_SPLINE_CURVE_WITH_KNOTS('',3,(#100432,#100433,#100434,#100435,
#100436,#100437,#100438),.UNSPECIFIED.,.F.,.F.,(4,3,4),(0.354658719353653,
0.357142857142857,0.366820493993915),.UNSPECIFIED.);
#21562=B_SPLINE_CURVE_WITH_KNOTS('',3,(#100463,#100464,#100465,#100466,
#100467,#100468),.UNSPECIFIED.,.F.,.F.,(4,2,4),(-0.0252992074993662,-0.0126497275569599,
0.),.UNSPECIFIED.);
#21563=B_SPLINE_CURVE_WITH_KNOTS('',3,(#100474,#100475,#100476,#100477,
#100478,#100479,#100480),.UNSPECIFIED.,.F.,.F.,(4,3,4),(0.349440546254526,
0.359118183105584,0.361602320897223),.UNSPECIFIED.);
#21564=B_SPLINE_CURVE_WITH_KNOTS('',3,(#100481,#100482,#100483,#100484,
#100485,#100486,#100487),.UNSPECIFIED.,.F.,.F.,(4,3,4),(0.35465871935122,
0.357142857142857,0.366820493993917),.UNSPECIFIED.);
#21565=B_SPLINE_CURVE_WITH_KNOTS('',3,(#100512,#100513,#100514,#100515,
#100516,#100517),.UNSPECIFIED.,.F.,.F.,(4,2,4),(-0.0252992075499003,-0.0126497275861227,
-2.70313389727495E-11),.UNSPECIFIED.);
#21566=B_SPLINE_CURVE_WITH_KNOTS('',3,(#100523,#100524,#100525,#100526,
#100527,#100528,#100529),.UNSPECIFIED.,.F.,.F.,(4,3,4),(0.349440546254538,
0.359118183105585,0.361602320901477),.UNSPECIFIED.);
#21567=B_SPLINE_CURVE_WITH_KNOTS('',3,(#100530,#100531,#100532,#100533,
#100534,#100535,#100536),.UNSPECIFIED.,.F.,.F.,(4,3,4),(0.354658719346978,
0.357142857142857,0.366820493993928),.UNSPECIFIED.);
#21568=B_SPLINE_CURVE_WITH_KNOTS('',3,(#100561,#100562,#100563,#100564,
#100565,#100566),.UNSPECIFIED.,.F.,.F.,(4,2,4),(-0.0252992074665769,-0.0126497276102527,
-3.18740624172253E-11),.UNSPECIFIED.);
#21569=B_SPLINE_CURVE_WITH_KNOTS('',3,(#100572,#100573,#100574,#100575,
#100576,#100577,#100578),.UNSPECIFIED.,.F.,.F.,(4,3,4),(0.349440546254528,
0.359118183105584,0.361602320899168),.UNSPECIFIED.);
#21570=B_SPLINE_CURVE_WITH_KNOTS('',3,(#100579,#100580,#100581,#100582,
#100583,#100584,#100585),.UNSPECIFIED.,.F.,.F.,(4,3,4),(0.354658719349277,
0.357142857142857,0.366820493993918),.UNSPECIFIED.);
#21571=B_SPLINE_CURVE_WITH_KNOTS('',3,(#100610,#100611,#100612,#100613,
#100614,#100615),.UNSPECIFIED.,.F.,.F.,(4,2,4),(-0.0252992075104434,-0.0126497276265894,
-5.31206086062941E-11),.UNSPECIFIED.);
#21572=B_SPLINE_CURVE_WITH_KNOTS('',3,(#100621,#100622,#100623,#100624,
#100625,#100626,#100627),.UNSPECIFIED.,.F.,.F.,(4,3,4),(0.349440546254525,
0.359118183105584,0.361602320908414),.UNSPECIFIED.);
#21573=B_SPLINE_CURVE_WITH_KNOTS('',3,(#100628,#100629,#100630,#100631,
#100632,#100633,#100634),.UNSPECIFIED.,.F.,.F.,(4,3,4),(0.354658719340028,
0.357142857142857,0.366820493993916),.UNSPECIFIED.);
#21574=B_SPLINE_CURVE_WITH_KNOTS('',3,(#100659,#100660,#100661,#100662,
#100663,#100664),.UNSPECIFIED.,.F.,.F.,(4,2,4),(-0.0252992075512971,-0.0126497276191108,
-3.96639145139321E-11),.UNSPECIFIED.);
#21575=B_SPLINE_CURVE_WITH_KNOTS('',3,(#100670,#100671,#100672,#100673,
#100674,#100675,#100676),.UNSPECIFIED.,.F.,.F.,(4,3,4),(0.349440546254525,
0.359118183105584,0.361602320899554),.UNSPECIFIED.);
#21576=B_SPLINE_CURVE_WITH_KNOTS('',3,(#100677,#100678,#100679,#100680,
#100681,#100682,#100683),.UNSPECIFIED.,.F.,.F.,(4,3,4),(0.354658719348888,
0.357142857142857,0.366820493993916),.UNSPECIFIED.);
#21577=B_SPLINE_CURVE_WITH_KNOTS('',3,(#100708,#100709,#100710,#100711,
#100712,#100713),.UNSPECIFIED.,.F.,.F.,(4,2,4),(-0.0252992075592725,-0.0126497275811909,
-1.37217980034077E-11),.UNSPECIFIED.);
#21578=B_SPLINE_CURVE_WITH_KNOTS('',3,(#100719,#100720,#100721,#100722,
#100723,#100724,#100725),.UNSPECIFIED.,.F.,.F.,(4,3,4),(0.349440546254526,
0.359118183105584,0.361602320896881),.UNSPECIFIED.);
#21579=B_SPLINE_CURVE_WITH_KNOTS('',3,(#100726,#100727,#100728,#100729,
#100730,#100731,#100732),.UNSPECIFIED.,.F.,.F.,(4,3,4),(0.354658719351561,
0.357142857142857,0.366820493993916),.UNSPECIFIED.);
#21580=B_SPLINE_CURVE_WITH_KNOTS('',3,(#100757,#100758,#100759,#100760,
#100761,#100762),.UNSPECIFIED.,.F.,.F.,(4,2,4),(-0.0252992074877316,-0.0126497275715462,
-3.83596869546476E-11),.UNSPECIFIED.);
#21581=B_SPLINE_CURVE_WITH_KNOTS('',3,(#100768,#100769,#100770,#100771,
#100772,#100773,#100774),.UNSPECIFIED.,.F.,.F.,(4,3,4),(0.349440546254526,
0.359118183105585,0.361602320902751),.UNSPECIFIED.);
#21582=B_SPLINE_CURVE_WITH_KNOTS('',3,(#100775,#100776,#100777,#100778,
#100779,#100780,#100781),.UNSPECIFIED.,.F.,.F.,(4,3,4),(0.354658719345692,
0.357142857142857,0.366820493993916),.UNSPECIFIED.);
#21583=B_SPLINE_CURVE_WITH_KNOTS('',3,(#100806,#100807,#100808,#100809,
#100810,#100811),.UNSPECIFIED.,.F.,.F.,(4,2,4),(-0.0252992075355198,-0.0126497275638241,
-1.5956104493231E-11),.UNSPECIFIED.);
#21584=B_SPLINE_CURVE_WITH_KNOTS('',3,(#100817,#100818,#100819,#100820,
#100821,#100822,#100823),.UNSPECIFIED.,.F.,.F.,(4,3,4),(0.349440546254526,
0.359118183105584,0.361602320894257),.UNSPECIFIED.);
#21585=B_SPLINE_CURVE_WITH_KNOTS('',3,(#100824,#100825,#100826,#100827,
#100828,#100829,#100830),.UNSPECIFIED.,.F.,.F.,(4,3,4),(0.354658719354185,
0.357142857142857,0.366820493993915),.UNSPECIFIED.);
#21586=B_SPLINE_CURVE_WITH_KNOTS('',3,(#100855,#100856,#100857,#100858,
#100859,#100860),.UNSPECIFIED.,.F.,.F.,(4,2,4),(-0.0252992075880614,-0.0126497276978079,
-1.04693153452073E-10),.UNSPECIFIED.);
#21587=B_SPLINE_CURVE_WITH_KNOTS('',3,(#100877,#100878,#100879,#100880,
#100881,#100882,#100883),.UNSPECIFIED.,.F.,.F.,(4,3,4),(0.354658719352825,
0.357142857142857,0.366820493993845),.UNSPECIFIED.);
#21588=B_SPLINE_CURVE_WITH_KNOTS('',3,(#100888,#100889,#100890,#100891,
#100892,#100893,#100894),.UNSPECIFIED.,.F.,.F.,(4,3,4),(0.349440546254584,
0.359118183105571,0.361602320905615),.UNSPECIFIED.);
#21589=B_SPLINE_CURVE_WITH_KNOTS('',3,(#100905,#100906,#100907,#100908,
#100909,#100910),.UNSPECIFIED.,.F.,.F.,(4,2,4),(-0.0252992075859009,-0.0126497275934163,
-3.14907752652083E-11),.UNSPECIFIED.);
#21590=B_SPLINE_CURVE_WITH_KNOTS('',3,(#100913,#100914,#100915,#100916,
#100917,#100918,#100919),.UNSPECIFIED.,.F.,.F.,(4,3,4),(0.354658719349017,
0.357142857142857,0.366820493993916),.UNSPECIFIED.);
#21591=B_SPLINE_CURVE_WITH_KNOTS('',3,(#100922,#100923,#100924,#100925,
#100926,#100927,#100928),.UNSPECIFIED.,.F.,.F.,(4,3,4),(0.349440546254519,
0.359118183105576,0.361602320899417),.UNSPECIFIED.);
#21592=B_SPLINE_CURVE_WITH_KNOTS('',3,(#100953,#100954,#100955,#100956,
#100957,#100958),.UNSPECIFIED.,.F.,.F.,(4,2,4),(-0.02529920751647,-0.0126497276304353,
-7.15628598046969E-11),.UNSPECIFIED.);
#21593=B_SPLINE_CURVE_WITH_KNOTS('',3,(#100964,#100965,#100966,#100967,
#100968,#100969,#100970),.UNSPECIFIED.,.F.,.F.,(4,3,4),(0.349440546254522,
0.359118183105575,0.361602320915514),.UNSPECIFIED.);
#21594=B_SPLINE_CURVE_WITH_KNOTS('',3,(#100971,#100972,#100973,#100974,
#100975,#100976,#100977),.UNSPECIFIED.,.F.,.F.,(4,3,4),(0.354658719332922,
0.357142857142857,0.366820493993919),.UNSPECIFIED.);
#21595=B_SPLINE_CURVE_WITH_KNOTS('',3,(#101002,#101003,#101004,#101005,
#101006,#101007),.UNSPECIFIED.,.F.,.F.,(4,2,4),(-0.0252992075126512,-0.012649727600527,
-5.9683594871851E-11),.UNSPECIFIED.);
#21596=B_SPLINE_CURVE_WITH_KNOTS('',3,(#101013,#101014,#101015,#101016,
#101017,#101018,#101019),.UNSPECIFIED.,.F.,.F.,(4,3,4),(0.34944054625452,
0.359118183105575,0.361602320910578),.UNSPECIFIED.);
#21597=B_SPLINE_CURVE_WITH_KNOTS('',3,(#101020,#101021,#101022,#101023,
#101024,#101025,#101026),.UNSPECIFIED.,.F.,.F.,(4,3,4),(0.354658719337858,
0.357142857142857,0.366820493993919),.UNSPECIFIED.);
#21598=B_SPLINE_CURVE_WITH_KNOTS('',3,(#101051,#101052,#101053,#101054,
#101055,#101056),.UNSPECIFIED.,.F.,.F.,(4,2,4),(-0.0252992074769014,-0.0126497275766772,
-2.69583487477743E-11),.UNSPECIFIED.);
#21599=B_SPLINE_CURVE_WITH_KNOTS('',3,(#101062,#101063,#101064,#101065,
#101066,#101067,#101068),.UNSPECIFIED.,.F.,.F.,(4,3,4),(0.349440546254521,
0.359118183105576,0.361602320899696),.UNSPECIFIED.);
#21600=B_SPLINE_CURVE_WITH_KNOTS('',3,(#101069,#101070,#101071,#101072,
#101073,#101074,#101075),.UNSPECIFIED.,.F.,.F.,(4,3,4),(0.35465871934874,
0.357142857142857,0.366820493993919),.UNSPECIFIED.);
#21601=B_SPLINE_CURVE_WITH_KNOTS('',3,(#101105,#101106,#101107,#101108,
#101109,#101110),.UNSPECIFIED.,.F.,.F.,(4,2,4),(-0.0253041039872367,-0.0126521677792654,
0.),.UNSPECIFIED.);
#21602=B_SPLINE_CURVE_WITH_KNOTS('',3,(#101146,#101147,#101148,#101149,
#101150,#101151),.UNSPECIFIED.,.F.,.F.,(4,2,4),(-0.0253041039005391,-0.0126521677027421,
0.),.UNSPECIFIED.);
#21603=B_SPLINE_CURVE_WITH_KNOTS('',3,(#101187,#101188,#101189,#101190,
#101191,#101192),.UNSPECIFIED.,.F.,.F.,(4,2,4),(-0.0253041039632652,-0.012652167781081,
0.),.UNSPECIFIED.);
#21604=B_SPLINE_CURVE_WITH_KNOTS('',3,(#101228,#101229,#101230,#101231,
#101232,#101233),.UNSPECIFIED.,.F.,.F.,(4,2,4),(-0.0253041039571526,-0.0126521677600083,
0.),.UNSPECIFIED.);
#21605=B_SPLINE_CURVE_WITH_KNOTS('',3,(#101269,#101270,#101271,#101272,
#101273,#101274),.UNSPECIFIED.,.F.,.F.,(4,2,4),(-0.0253041038880339,-0.0126521676975068,
0.),.UNSPECIFIED.);
#21606=B_SPLINE_CURVE_WITH_KNOTS('',3,(#101310,#101311,#101312,#101313,
#101314,#101315),.UNSPECIFIED.,.F.,.F.,(4,2,4),(-0.0253041039499959,-0.0126521677582051,
0.),.UNSPECIFIED.);
#21607=B_SPLINE_CURVE_WITH_KNOTS('',3,(#101351,#101352,#101353,#101354,
#101355,#101356),.UNSPECIFIED.,.F.,.F.,(4,2,4),(-0.0253041038968693,-0.0126521677390511,
0.),.UNSPECIFIED.);
#21608=B_SPLINE_CURVE_WITH_KNOTS('',3,(#101392,#101393,#101394,#101395,
#101396,#101397),.UNSPECIFIED.,.F.,.F.,(4,2,4),(-0.025304103953758,-0.0126521677536738,
0.),.UNSPECIFIED.);
#21609=B_SPLINE_CURVE_WITH_KNOTS('',3,(#101433,#101434,#101435,#101436,
#101437,#101438),.UNSPECIFIED.,.F.,.F.,(4,2,4),(-0.0253041039231198,-0.0126521677416848,
0.),.UNSPECIFIED.);
#21610=B_SPLINE_CURVE_WITH_KNOTS('',3,(#101474,#101475,#101476,#101477,
#101478,#101479),.UNSPECIFIED.,.F.,.F.,(4,2,4),(-0.0253041039323966,-0.0126521677644877,
0.),.UNSPECIFIED.);
#21611=B_SPLINE_CURVE_WITH_KNOTS('',3,(#101515,#101516,#101517,#101518,
#101519,#101520),.UNSPECIFIED.,.F.,.F.,(4,2,4),(-0.0253041039471639,-0.0126521677898284,
0.),.UNSPECIFIED.);
#21612=B_SPLINE_CURVE_WITH_KNOTS('',3,(#101556,#101557,#101558,#101559,
#101560,#101561),.UNSPECIFIED.,.F.,.F.,(4,2,4),(-0.0253041039397315,-0.0126521677657765,
0.),.UNSPECIFIED.);
#21613=B_SPLINE_CURVE_WITH_KNOTS('',3,(#101597,#101598,#101599,#101600,
#101601,#101602),.UNSPECIFIED.,.F.,.F.,(4,2,4),(-0.0253041038956333,-0.0126521677148479,
0.),.UNSPECIFIED.);
#21614=B_SPLINE_CURVE_WITH_KNOTS('',3,(#101638,#101639,#101640,#101641,
#101642,#101643),.UNSPECIFIED.,.F.,.F.,(4,2,4),(-0.0253041039012348,-0.0126521676969631,
0.),.UNSPECIFIED.);
#21615=B_SPLINE_CURVE_WITH_KNOTS('',3,(#101679,#101680,#101681,#101682,
#101683,#101684),.UNSPECIFIED.,.F.,.F.,(4,2,4),(-0.0253041040308761,-0.0126521678473633,
0.),.UNSPECIFIED.);
#21616=B_SPLINE_CURVE_WITH_KNOTS('',3,(#101720,#101721,#101722,#101723,
#101724,#101725),.UNSPECIFIED.,.F.,.F.,(4,2,4),(-0.0253041039070892,-0.012652167715741,
0.),.UNSPECIFIED.);
#21617=B_SPLINE_CURVE_WITH_KNOTS('',3,(#101761,#101762,#101763,#101764,
#101765,#101766),.UNSPECIFIED.,.F.,.F.,(4,2,4),(-0.0253041038669996,-0.0126521677219567,
0.),.UNSPECIFIED.);
#21618=B_SPLINE_CURVE_WITH_KNOTS('',3,(#101802,#101803,#101804,#101805,
#101806,#101807),.UNSPECIFIED.,.F.,.F.,(4,2,4),(-0.0253041038574588,-0.0126521676654783,
0.),.UNSPECIFIED.);
#21619=B_SPLINE_CURVE_WITH_KNOTS('',3,(#101843,#101844,#101845,#101846,
#101847,#101848),.UNSPECIFIED.,.F.,.F.,(4,2,4),(-0.0253041039409774,-0.0126521677661099,
0.),.UNSPECIFIED.);
#21620=B_SPLINE_CURVE_WITH_KNOTS('',3,(#101884,#101885,#101886,#101887,
#101888,#101889),.UNSPECIFIED.,.F.,.F.,(4,2,4),(-0.0253041039068838,-0.0126521677169225,
0.),.UNSPECIFIED.);
#21621=B_SPLINE_CURVE_WITH_KNOTS('',3,(#101925,#101926,#101927,#101928,
#101929,#101930),.UNSPECIFIED.,.F.,.F.,(4,2,4),(-0.0253041039770956,-0.0126521677689033,
0.),.UNSPECIFIED.);
#21622=B_SPLINE_CURVE_WITH_KNOTS('',3,(#101963,#101964,#101965,#101966,
#101967,#101968),.UNSPECIFIED.,.F.,.F.,(4,2,4),(-0.0253041039055625,-0.0126521677474333,
0.),.UNSPECIFIED.);
#21623=B_SPLINE_CURVE_WITH_KNOTS('',3,(#101994,#101995,#101996,#101997,
#101998,#101999),.UNSPECIFIED.,.F.,.F.,(4,2,4),(-0.0253041039293055,-0.0126521677635233,
0.),.UNSPECIFIED.);
#21624=B_SPLINE_CURVE_WITH_KNOTS('',3,(#102035,#102036,#102037,#102038,
#102039,#102040),.UNSPECIFIED.,.F.,.F.,(4,2,4),(-0.0253041039232594,-0.0126521677538064,
0.),.UNSPECIFIED.);
#21625=B_SPLINE_CURVE_WITH_KNOTS('',3,(#102076,#102077,#102078,#102079,
#102080,#102081),.UNSPECIFIED.,.F.,.F.,(4,2,4),(-0.02530410389646,-0.0126521677360228,
0.),.UNSPECIFIED.);
#21626=B_SPLINE_CURVE_WITH_KNOTS('',3,(#102117,#102118,#102119,#102120,
#102121,#102122),.UNSPECIFIED.,.F.,.F.,(4,2,4),(-0.0253041039850785,-0.0126521678235967,
0.),.UNSPECIFIED.);
#21627=B_SPLINE_CURVE_WITH_KNOTS('',3,(#102158,#102159,#102160,#102161,
#102162,#102163),.UNSPECIFIED.,.F.,.F.,(4,2,4),(-0.0253041038917768,-0.0126521677471262,
0.),.UNSPECIFIED.);
#21628=B_SPLINE_CURVE_WITH_KNOTS('',3,(#102199,#102200,#102201,#102202,
#102203,#102204),.UNSPECIFIED.,.F.,.F.,(4,2,4),(-0.0253041039399128,-0.01265216776193,
0.),.UNSPECIFIED.);
#21629=B_SPLINE_CURVE_WITH_KNOTS('',3,(#102240,#102241,#102242,#102243,
#102244,#102245),.UNSPECIFIED.,.F.,.F.,(4,2,4),(-0.0253041038279282,-0.0126521676565885,
0.),.UNSPECIFIED.);
#21630=B_SPLINE_CURVE_WITH_KNOTS('',3,(#102275,#102276,#102277,#102278,
#102279,#102280),.UNSPECIFIED.,.F.,.F.,(4,2,4),(-0.0252994184233411,-0.0126495849026555,
0.),.UNSPECIFIED.);
#21631=B_SPLINE_CURVE_WITH_KNOTS('',3,(#102295,#102296,#102297,#102298,
#102299,#102300,#102301),.UNSPECIFIED.,.F.,.F.,(4,3,4),(0.349298845963836,
0.35897648262994,0.366749642030242),.UNSPECIFIED.);
#21632=B_SPLINE_CURVE_WITH_KNOTS('',3,(#102310,#102311,#102312,#102313,
#102314,#102315),.UNSPECIFIED.,.F.,.F.,(4,2,4),(-0.025299364436483,-0.0126495718869962,
0.),.UNSPECIFIED.);
#21633=B_SPLINE_CURVE_WITH_KNOTS('',3,(#102330,#102331,#102332,#102333,
#102334,#102335,#102336),.UNSPECIFIED.,.F.,.F.,(4,3,4),(0.349298845971303,
0.358976482629938,0.366749642018671),.UNSPECIFIED.);
#21634=B_SPLINE_CURVE_WITH_KNOTS('',3,(#102345,#102346,#102347,#102348,
#102349,#102350),.UNSPECIFIED.,.F.,.F.,(4,2,4),(-0.0252994181275643,-0.0126495848436817,
0.),.UNSPECIFIED.);
#21635=B_SPLINE_CURVE_WITH_KNOTS('',3,(#102365,#102366,#102367,#102368,
#102369,#102370,#102371),.UNSPECIFIED.,.F.,.F.,(4,3,4),(0.3492988459672,
0.358976482629936,0.366749642025355),.UNSPECIFIED.);
#21636=B_SPLINE_CURVE_WITH_KNOTS('',3,(#102380,#102381,#102382,#102383,
#102384,#102385),.UNSPECIFIED.,.F.,.F.,(4,2,4),(-0.0252994180828767,-0.0126495848091462,
0.),.UNSPECIFIED.);
#21637=B_SPLINE_CURVE_WITH_KNOTS('',3,(#102400,#102401,#102402,#102403,
#102404,#102405,#102406),.UNSPECIFIED.,.F.,.F.,(4,3,4),(0.34929884596835,
0.358976482629936,0.366749642036658),.UNSPECIFIED.);
#21638=B_SPLINE_CURVE_WITH_KNOTS('',3,(#102415,#102416,#102417,#102418,
#102419,#102420),.UNSPECIFIED.,.F.,.F.,(4,2,4),(-0.0252994182000983,-0.0126495848420178,
0.),.UNSPECIFIED.);
#21639=B_SPLINE_CURVE_WITH_KNOTS('',3,(#102435,#102436,#102437,#102438,
#102439,#102440,#102441),.UNSPECIFIED.,.F.,.F.,(4,3,4),(0.349298845930643,
0.358976482629938,0.366749642035256),.UNSPECIFIED.);
#21640=B_SPLINE_CURVE_WITH_KNOTS('',3,(#102450,#102451,#102452,#102453,
#102454,#102455),.UNSPECIFIED.,.F.,.F.,(4,2,4),(-0.0252994179754861,-0.0126495848168498,
0.),.UNSPECIFIED.);
#21641=B_SPLINE_CURVE_WITH_KNOTS('',3,(#102470,#102471,#102472,#102473,
#102474,#102475,#102476),.UNSPECIFIED.,.F.,.F.,(4,3,4),(0.349298845948969,
0.358976482629922,0.366749642024373),.UNSPECIFIED.);
#21642=B_SPLINE_CURVE_WITH_KNOTS('',3,(#102485,#102486,#102487,#102488,
#102489,#102490),.UNSPECIFIED.,.F.,.F.,(4,2,4),(-0.0252994179869716,-0.0126495848061804,
0.),.UNSPECIFIED.);
#21643=B_SPLINE_CURVE_WITH_KNOTS('',3,(#102505,#102506,#102507,#102508,
#102509,#102510,#102511),.UNSPECIFIED.,.F.,.F.,(4,3,4),(0.349298845956751,
0.358976482629922,0.366749642032673),.UNSPECIFIED.);
#21644=B_SPLINE_CURVE_WITH_KNOTS('',3,(#102520,#102521,#102522,#102523,
#102524,#102525),.UNSPECIFIED.,.F.,.F.,(4,2,4),(-0.0252994179954849,-0.0126495848078521,
0.),.UNSPECIFIED.);
#21645=B_SPLINE_CURVE_WITH_KNOTS('',3,(#102540,#102541,#102542,#102543,
#102544,#102545,#102546),.UNSPECIFIED.,.F.,.F.,(4,3,4),(0.349298845945899,
0.358976482629922,0.366749642023676),.UNSPECIFIED.);
#21646=B_SPLINE_CURVE_WITH_KNOTS('',3,(#102555,#102556,#102557,#102558,
#102559,#102560),.UNSPECIFIED.,.F.,.F.,(4,2,4),(-0.0252993639960928,-0.0126495717892771,
0.),.UNSPECIFIED.);
#21647=B_SPLINE_CURVE_WITH_KNOTS('',3,(#102575,#102576,#102577,#102578,
#102579,#102580,#102581),.UNSPECIFIED.,.F.,.F.,(4,3,4),(0.349298845963625,
0.358976482629922,0.36674964202969),.UNSPECIFIED.);
#21648=B_SPLINE_CURVE_WITH_KNOTS('',3,(#102590,#102591,#102592,#102593,
#102594,#102595),.UNSPECIFIED.,.F.,.F.,(4,2,4),(-0.0252994181967913,-0.0126495848488086,
0.),.UNSPECIFIED.);
#21649=B_SPLINE_CURVE_WITH_KNOTS('',3,(#102610,#102611,#102612,#102613,
#102614,#102615,#102616),.UNSPECIFIED.,.F.,.F.,(4,3,4),(0.349298845932533,
0.35897648262994,0.36674964202247),.UNSPECIFIED.);
#21650=B_SPLINE_CURVE_WITH_KNOTS('',3,(#102625,#102626,#102627,#102628,
#102629,#102630),.UNSPECIFIED.,.F.,.F.,(4,2,4),(-0.0252993643205837,-0.0126495718771281,
0.),.UNSPECIFIED.);
#21651=B_SPLINE_CURVE_WITH_KNOTS('',3,(#102645,#102646,#102647,#102648,
#102649,#102650,#102651),.UNSPECIFIED.,.F.,.F.,(4,3,4),(0.349298845921702,
0.35897648262994,0.366749642024241),.UNSPECIFIED.);
#21652=B_SPLINE_CURVE_WITH_KNOTS('',3,(#102660,#102661,#102662,#102663,
#102664,#102665),.UNSPECIFIED.,.F.,.F.,(4,2,4),(-0.0252993635718202,-0.0126495716991594,
0.),.UNSPECIFIED.);
#21653=B_SPLINE_CURVE_WITH_KNOTS('',3,(#102680,#102681,#102682,#102683,
#102684,#102685,#102686),.UNSPECIFIED.,.F.,.F.,(4,3,4),(0.349298845969534,
0.35897648262994,0.366749642035329),.UNSPECIFIED.);
#21654=B_SPLINE_CURVE_WITH_KNOTS('',3,(#102695,#102696,#102697,#102698,
#102699,#102700),.UNSPECIFIED.,.F.,.F.,(4,2,4),(-0.0252994179273683,-0.0126495847910784,
0.),.UNSPECIFIED.);
#21655=B_SPLINE_CURVE_WITH_KNOTS('',3,(#102715,#102716,#102717,#102718,
#102719,#102720,#102721),.UNSPECIFIED.,.F.,.F.,(4,3,4),(0.34929884595549,
0.35897648262994,0.366749642022583),.UNSPECIFIED.);
#21656=B_SPLINE_CURVE_WITH_KNOTS('',3,(#102730,#102731,#102732,#102733,
#102734,#102735),.UNSPECIFIED.,.F.,.F.,(4,2,4),(-0.0252993644889527,-0.0126495719101191,
0.),.UNSPECIFIED.);
#21657=B_SPLINE_CURVE_WITH_KNOTS('',3,(#102750,#102751,#102752,#102753,
#102754,#102755,#102756),.UNSPECIFIED.,.F.,.F.,(4,3,4),(0.349298845947852,
0.35897648262994,0.366749642016953),.UNSPECIFIED.);
#21658=B_SPLINE_CURVE_WITH_KNOTS('',3,(#102765,#102766,#102767,#102768,
#102769,#102770),.UNSPECIFIED.,.F.,.F.,(4,2,4),(-0.0252994181077383,-0.0126495848252762,
0.),.UNSPECIFIED.);
#21659=B_SPLINE_CURVE_WITH_KNOTS('',3,(#102785,#102786,#102787,#102788,
#102789,#102790,#102791),.UNSPECIFIED.,.F.,.F.,(4,3,4),(0.349298845953694,
0.35897648262994,0.366749642014227),.UNSPECIFIED.);
#21660=B_SPLINE_CURVE_WITH_KNOTS('',3,(#102800,#102801,#102802,#102803,
#102804,#102805),.UNSPECIFIED.,.F.,.F.,(4,2,4),(-0.0252994180307134,-0.0126495848285684,
0.),.UNSPECIFIED.);
#21661=B_SPLINE_CURVE_WITH_KNOTS('',3,(#102820,#102821,#102822,#102823,
#102824,#102825,#102826),.UNSPECIFIED.,.F.,.F.,(4,3,4),(0.349298845961314,
0.35897648262994,0.366749642024527),.UNSPECIFIED.);
#21662=B_SPLINE_CURVE_WITH_KNOTS('',3,(#102835,#102836,#102837,#102838,
#102839,#102840),.UNSPECIFIED.,.F.,.F.,(4,2,4),(-0.0252993640217252,-0.0126495718156864,
0.),.UNSPECIFIED.);
#21663=B_SPLINE_CURVE_WITH_KNOTS('',3,(#102855,#102856,#102857,#102858,
#102859,#102860,#102861),.UNSPECIFIED.,.F.,.F.,(4,3,4),(0.349298845962747,
0.35897648262994,0.366749642025728),.UNSPECIFIED.);
#21664=B_SPLINE_CURVE_WITH_KNOTS('',3,(#102870,#102871,#102872,#102873,
#102874,#102875),.UNSPECIFIED.,.F.,.F.,(4,2,4),(-0.0252993637637311,-0.0126495717496519,
0.),.UNSPECIFIED.);
#21665=B_SPLINE_CURVE_WITH_KNOTS('',3,(#102890,#102891,#102892,#102893,
#102894,#102895,#102896),.UNSPECIFIED.,.F.,.F.,(4,3,4),(0.34929884594429,
0.35897648262994,0.366749642019548),.UNSPECIFIED.);
#21666=B_SPLINE_CURVE_WITH_KNOTS('',3,(#102905,#102906,#102907,#102908,
#102909,#102910),.UNSPECIFIED.,.F.,.F.,(4,2,4),(-0.0252993637208719,-0.0126495717243885,
0.),.UNSPECIFIED.);
#21667=B_SPLINE_CURVE_WITH_KNOTS('',3,(#102925,#102926,#102927,#102928,
#102929,#102930,#102931),.UNSPECIFIED.,.F.,.F.,(4,3,4),(0.349298845943498,
0.35897648262994,0.366749642024082),.UNSPECIFIED.);
#21668=B_SPLINE_CURVE_WITH_KNOTS('',3,(#102940,#102941,#102942,#102943,
#102944,#102945),.UNSPECIFIED.,.F.,.F.,(4,2,4),(-0.0252994182535981,-0.0126495848574988,
0.),.UNSPECIFIED.);
#21669=B_SPLINE_CURVE_WITH_KNOTS('',3,(#102960,#102961,#102962,#102963,
#102964,#102965,#102966),.UNSPECIFIED.,.F.,.F.,(4,3,4),(0.349298845939575,
0.35897648262994,0.366749642029799),.UNSPECIFIED.);
#21670=B_SPLINE_CURVE_WITH_KNOTS('',3,(#102975,#102976,#102977,#102978,
#102979,#102980),.UNSPECIFIED.,.F.,.F.,(4,2,4),(-0.0252994180810671,-0.0126495848269979,
0.),.UNSPECIFIED.);
#21671=B_SPLINE_CURVE_WITH_KNOTS('',3,(#102995,#102996,#102997,#102998,
#102999,#103000,#103001),.UNSPECIFIED.,.F.,.F.,(4,3,4),(0.349298845945691,
0.35897648262994,0.366749642035111),.UNSPECIFIED.);
#21672=B_SPLINE_CURVE_WITH_KNOTS('',3,(#103010,#103011,#103012,#103013,
#103014,#103015),.UNSPECIFIED.,.F.,.F.,(4,2,4),(-0.0252994181543156,-0.012649584865264,
0.),.UNSPECIFIED.);
#21673=B_SPLINE_CURVE_WITH_KNOTS('',3,(#103030,#103031,#103032,#103033,
#103034,#103035,#103036),.UNSPECIFIED.,.F.,.F.,(4,3,4),(0.349298845951285,
0.35897648262994,0.366749642035188),.UNSPECIFIED.);
#21674=B_SPLINE_CURVE_WITH_KNOTS('',3,(#103045,#103046,#103047,#103048,
#103049,#103050),.UNSPECIFIED.,.F.,.F.,(4,2,4),(-0.0252994183497646,-0.0126495848853004,
0.),.UNSPECIFIED.);
#21675=B_SPLINE_CURVE_WITH_KNOTS('',3,(#103065,#103066,#103067,#103068,
#103069,#103070,#103071),.UNSPECIFIED.,.F.,.F.,(4,3,4),(0.349298845943866,
0.35897648262994,0.366749642036405),.UNSPECIFIED.);
#21676=B_SPLINE_CURVE_WITH_KNOTS('',3,(#103080,#103081,#103082,#103083,
#103084,#103085),.UNSPECIFIED.,.F.,.F.,(4,2,4),(-0.0252993644655463,-0.0126495719273563,
0.),.UNSPECIFIED.);
#21677=B_SPLINE_CURVE_WITH_KNOTS('',3,(#103100,#103101,#103102,#103103,
#103104,#103105,#103106),.UNSPECIFIED.,.F.,.F.,(4,3,4),(0.349298845958209,
0.35897648262994,0.366749642025503),.UNSPECIFIED.);
#21678=B_SPLINE_CURVE_WITH_KNOTS('',3,(#103115,#103116,#103117,#103118,
#103119,#103120),.UNSPECIFIED.,.F.,.F.,(4,2,4),(-0.0252993642339217,-0.0126495718654069,
0.),.UNSPECIFIED.);
#21679=B_SPLINE_CURVE_WITH_KNOTS('',3,(#103135,#103136,#103137,#103138,
#103139,#103140,#103141),.UNSPECIFIED.,.F.,.F.,(4,3,4),(0.34929884594229,
0.358976482629936,0.366749642031194),.UNSPECIFIED.);
#21680=B_SPLINE_CURVE_WITH_KNOTS('',3,(#103150,#103151,#103152,#103153,
#103154,#103155),.UNSPECIFIED.,.F.,.F.,(4,2,4),(-0.0252993643902813,-0.0126495719066374,
0.),.UNSPECIFIED.);
#21681=B_SPLINE_CURVE_WITH_KNOTS('',3,(#103170,#103171,#103172,#103173,
#103174,#103175,#103176),.UNSPECIFIED.,.F.,.F.,(4,3,4),(0.349298845965109,
0.358976482629922,0.366749642028045),.UNSPECIFIED.);
#21682=B_SPLINE_CURVE_WITH_KNOTS('',3,(#103185,#103186,#103187,#103188,
#103189,#103190),.UNSPECIFIED.,.F.,.F.,(4,2,4),(-0.0252993639302304,-0.0126495717682941,
0.),.UNSPECIFIED.);
#21683=B_SPLINE_CURVE_WITH_KNOTS('',3,(#103205,#103206,#103207,#103208,
#103209,#103210,#103211),.UNSPECIFIED.,.F.,.F.,(4,3,4),(0.349298845937363,
0.35897648262994,0.366749642034294),.UNSPECIFIED.);
#21684=B_SPLINE_CURVE_WITH_KNOTS('',3,(#103220,#103221,#103222,#103223,
#103224,#103225),.UNSPECIFIED.,.F.,.F.,(4,2,4),(-0.0252993641752915,-0.0126495718180406,
0.),.UNSPECIFIED.);
#21685=B_SPLINE_CURVE_WITH_KNOTS('',3,(#103240,#103241,#103242,#103243,
#103244,#103245,#103246),.UNSPECIFIED.,.F.,.F.,(4,3,4),(0.349298845962219,
0.35897648262994,0.366749642022716),.UNSPECIFIED.);
#21686=B_SPLINE_CURVE_WITH_KNOTS('',3,(#103255,#103256,#103257,#103258,
#103259,#103260),.UNSPECIFIED.,.F.,.F.,(4,2,4),(-0.0252994180664517,-0.0126495848125946,
0.),.UNSPECIFIED.);
#21687=B_SPLINE_CURVE_WITH_KNOTS('',3,(#103275,#103276,#103277,#103278,
#103279,#103280,#103281),.UNSPECIFIED.,.F.,.F.,(4,3,4),(0.349298845879221,
0.358976482629941,0.36674964202409),.UNSPECIFIED.);
#21688=B_SPLINE_CURVE_WITH_KNOTS('',3,(#103290,#103291,#103292,#103293,
#103294,#103295),.UNSPECIFIED.,.F.,.F.,(4,2,4),(-0.025296958792191,-0.012648355834516,
0.),.UNSPECIFIED.);
#21689=B_SPLINE_CURVE_WITH_KNOTS('',3,(#103306,#103307,#103308,#103309,
#103310,#103311,#103312),.UNSPECIFIED.,.F.,.F.,(4,3,4),(0.418312080788897,
0.428571428571429,0.435775021767613),.UNSPECIFIED.);
#21690=B_SPLINE_CURVE_WITH_KNOTS('',3,(#103321,#103322,#103323,#103324,
#103325,#103326),.UNSPECIFIED.,.F.,.F.,(4,2,4),(-0.0252969554483052,-0.0126483549025546,
0.),.UNSPECIFIED.);
#21691=B_SPLINE_CURVE_WITH_KNOTS('',3,(#103337,#103338,#103339,#103340,
#103341,#103342,#103343),.UNSPECIFIED.,.F.,.F.,(4,3,4),(0.418312080810239,
0.428571428568827,0.435775021479951),.UNSPECIFIED.);
#21692=B_SPLINE_CURVE_WITH_KNOTS('',3,(#103352,#103353,#103354,#103355,
#103356,#103357),.UNSPECIFIED.,.F.,.F.,(4,2,4),(-0.025297157865339,-0.0126484038625859,
0.),.UNSPECIFIED.);
#21693=B_SPLINE_CURVE_WITH_KNOTS('',3,(#103368,#103369,#103370,#103371,
#103372,#103373,#103374),.UNSPECIFIED.,.F.,.F.,(4,3,4),(0.41831208080354,
0.428571428571429,0.4357750217547),.UNSPECIFIED.);
#21694=B_SPLINE_CURVE_WITH_KNOTS('',3,(#103383,#103384,#103385,#103386,
#103387,#103388),.UNSPECIFIED.,.F.,.F.,(4,2,4),(-0.0252969589615879,-0.0126483559234329,
0.),.UNSPECIFIED.);
#21695=B_SPLINE_CURVE_WITH_KNOTS('',3,(#103399,#103400,#103401,#103402,
#103403,#103404,#103405),.UNSPECIFIED.,.F.,.F.,(4,3,4),(0.418312080798011,
0.428571428571429,0.435775021762071),.UNSPECIFIED.);
#21696=B_SPLINE_CURVE_WITH_KNOTS('',3,(#103414,#103415,#103416,#103417,
#103418,#103419),.UNSPECIFIED.,.F.,.F.,(4,2,4),(-0.0252969587987205,-0.0126483557936413,
0.),.UNSPECIFIED.);
#21697=B_SPLINE_CURVE_WITH_KNOTS('',3,(#103430,#103431,#103432,#103433,
#103434,#103435,#103436),.UNSPECIFIED.,.F.,.F.,(4,3,4),(0.418312080798033,
0.428571428571429,0.43577502176659),.UNSPECIFIED.);
#21698=B_SPLINE_CURVE_WITH_KNOTS('',3,(#103445,#103446,#103447,#103448,
#103449,#103450),.UNSPECIFIED.,.F.,.F.,(4,2,4),(-0.0252969587895803,-0.0126483557947713,
0.),.UNSPECIFIED.);
#21699=B_SPLINE_CURVE_WITH_KNOTS('',3,(#103461,#103462,#103463,#103464,
#103465,#103466,#103467),.UNSPECIFIED.,.F.,.F.,(4,3,4),(0.418312080811542,
0.428571428571429,0.435775021766799),.UNSPECIFIED.);
#21700=B_SPLINE_CURVE_WITH_KNOTS('',3,(#103476,#103477,#103478,#103479,
#103480,#103481),.UNSPECIFIED.,.F.,.F.,(4,2,4),(-0.0252969588307827,-0.0126483558513836,
0.),.UNSPECIFIED.);
#21701=B_SPLINE_CURVE_WITH_KNOTS('',3,(#103492,#103493,#103494,#103495,
#103496,#103497,#103498),.UNSPECIFIED.,.F.,.F.,(4,3,4),(0.418312080793796,
0.428571428571429,0.435775021765992),.UNSPECIFIED.);
#21702=B_SPLINE_CURVE_WITH_KNOTS('',3,(#103507,#103508,#103509,#103510,
#103511,#103512),.UNSPECIFIED.,.F.,.F.,(4,2,4),(-0.0252969588840719,-0.0126483558613075,
0.),.UNSPECIFIED.);
#21703=B_SPLINE_CURVE_WITH_KNOTS('',3,(#103523,#103524,#103525,#103526,
#103527,#103528,#103529),.UNSPECIFIED.,.F.,.F.,(4,3,4),(0.418312080801105,
0.428571428571429,0.43577502176165),.UNSPECIFIED.);
#21704=B_SPLINE_CURVE_WITH_KNOTS('',3,(#103538,#103539,#103540,#103541,
#103542,#103543),.UNSPECIFIED.,.F.,.F.,(4,2,4),(-0.0252969587965309,-0.0126483558081197,
0.),.UNSPECIFIED.);
#21705=B_SPLINE_CURVE_WITH_KNOTS('',3,(#103554,#103555,#103556,#103557,
#103558,#103559,#103560),.UNSPECIFIED.,.F.,.F.,(4,3,4),(0.41831208081577,
0.428571428571429,0.435775021758859),.UNSPECIFIED.);
#21706=B_SPLINE_CURVE_WITH_KNOTS('',3,(#103569,#103570,#103571,#103572,
#103573,#103574),.UNSPECIFIED.,.F.,.F.,(4,2,4),(-0.0252969587879319,-0.0126483558043734,
0.),.UNSPECIFIED.);
#21707=B_SPLINE_CURVE_WITH_KNOTS('',3,(#103585,#103586,#103587,#103588,
#103589,#103590,#103591),.UNSPECIFIED.,.F.,.F.,(4,3,4),(0.418312080803554,
0.428571428571429,0.435775021758034),.UNSPECIFIED.);
#21708=B_SPLINE_CURVE_WITH_KNOTS('',3,(#103600,#103601,#103602,#103603,
#103604,#103605),.UNSPECIFIED.,.F.,.F.,(4,2,4),(-0.0252969588289607,-0.0126483558674192,
0.),.UNSPECIFIED.);
#21709=B_SPLINE_CURVE_WITH_KNOTS('',3,(#103616,#103617,#103618,#103619,
#103620,#103621,#103622),.UNSPECIFIED.,.F.,.F.,(4,3,4),(0.41831208080598,
0.428571428571429,0.435775021762065),.UNSPECIFIED.);
#21710=B_SPLINE_CURVE_WITH_KNOTS('',3,(#103631,#103632,#103633,#103634,
#103635,#103636),.UNSPECIFIED.,.F.,.F.,(4,2,4),(-0.0252969588379448,-0.0126483558443588,
0.),.UNSPECIFIED.);
#21711=B_SPLINE_CURVE_WITH_KNOTS('',3,(#103647,#103648,#103649,#103650,
#103651,#103652,#103653),.UNSPECIFIED.,.F.,.F.,(4,3,4),(0.418312080802205,
0.428571428571429,0.435775021765829),.UNSPECIFIED.);
#21712=B_SPLINE_CURVE_WITH_KNOTS('',3,(#103662,#103663,#103664,#103665,
#103666,#103667),.UNSPECIFIED.,.F.,.F.,(4,2,4),(-0.0252969588740578,-0.0126483558687873,
0.),.UNSPECIFIED.);
#21713=B_SPLINE_CURVE_WITH_KNOTS('',3,(#103678,#103679,#103680,#103681,
#103682,#103683,#103684),.UNSPECIFIED.,.F.,.F.,(4,3,4),(0.41831208081761,
0.428571428571429,0.435775021762013),.UNSPECIFIED.);
#21714=B_SPLINE_CURVE_WITH_KNOTS('',3,(#103693,#103694,#103695,#103696,
#103697,#103698),.UNSPECIFIED.,.F.,.F.,(4,2,4),(-0.0252969588665305,-0.0126483558558781,
0.),.UNSPECIFIED.);
#21715=B_SPLINE_CURVE_WITH_KNOTS('',3,(#103709,#103710,#103711,#103712,
#103713,#103714,#103715),.UNSPECIFIED.,.F.,.F.,(4,3,4),(0.418312080799316,
0.428571428571429,0.435775021764603),.UNSPECIFIED.);
#21716=B_SPLINE_CURVE_WITH_KNOTS('',3,(#103724,#103725,#103726,#103727,
#103728,#103729),.UNSPECIFIED.,.F.,.F.,(4,2,4),(-0.0252969588070961,-0.0126483558109704,
0.),.UNSPECIFIED.);
#21717=B_SPLINE_CURVE_WITH_KNOTS('',3,(#103740,#103741,#103742,#103743,
#103744,#103745,#103746),.UNSPECIFIED.,.F.,.F.,(4,3,4),(0.418312080790721,
0.428571428571429,0.435775021760828),.UNSPECIFIED.);
#21718=B_SPLINE_CURVE_WITH_KNOTS('',3,(#103755,#103756,#103757,#103758,
#103759,#103760),.UNSPECIFIED.,.F.,.F.,(4,2,4),(-0.0252969587698119,-0.0126483558105197,
0.),.UNSPECIFIED.);
#21719=B_SPLINE_CURVE_WITH_KNOTS('',3,(#103771,#103772,#103773,#103774,
#103775,#103776,#103777),.UNSPECIFIED.,.F.,.F.,(4,3,4),(0.418312080813446,
0.428571428571429,0.43577502176075),.UNSPECIFIED.);
#21720=B_SPLINE_CURVE_WITH_KNOTS('',3,(#103786,#103787,#103788,#103789,
#103790,#103791),.UNSPECIFIED.,.F.,.F.,(4,2,4),(-0.0252969588634707,-0.0126483558476927,
0.),.UNSPECIFIED.);
#21721=B_SPLINE_CURVE_WITH_KNOTS('',3,(#103802,#103803,#103804,#103805,
#103806,#103807,#103808),.UNSPECIFIED.,.F.,.F.,(4,3,4),(0.418312080804051,
0.428571428571429,0.435775021758984),.UNSPECIFIED.);
#21722=B_SPLINE_CURVE_WITH_KNOTS('',3,(#103817,#103818,#103819,#103820,
#103821,#103822),.UNSPECIFIED.,.F.,.F.,(4,2,4),(-0.0252969588415939,-0.0126483558254068,
0.),.UNSPECIFIED.);
#21723=B_SPLINE_CURVE_WITH_KNOTS('',3,(#103833,#103834,#103835,#103836,
#103837,#103838,#103839),.UNSPECIFIED.,.F.,.F.,(4,3,4),(0.418312080799403,
0.428571428571429,0.435775021765068),.UNSPECIFIED.);
#21724=B_SPLINE_CURVE_WITH_KNOTS('',3,(#103848,#103849,#103850,#103851,
#103852,#103853),.UNSPECIFIED.,.F.,.F.,(4,2,4),(-0.0252969588213482,-0.012648355813714,
0.),.UNSPECIFIED.);
#21725=B_SPLINE_CURVE_WITH_KNOTS('',3,(#103864,#103865,#103866,#103867,
#103868,#103869,#103870),.UNSPECIFIED.,.F.,.F.,(4,3,4),(0.418312080807609,
0.428571428571429,0.435775021753525),.UNSPECIFIED.);
#21726=B_SPLINE_CURVE_WITH_KNOTS('',3,(#103879,#103880,#103881,#103882,
#103883,#103884),.UNSPECIFIED.,.F.,.F.,(4,2,4),(-0.0252969587836844,-0.0126483558118128,
0.),.UNSPECIFIED.);
#21727=B_SPLINE_CURVE_WITH_KNOTS('',3,(#103895,#103896,#103897,#103898,
#103899,#103900,#103901),.UNSPECIFIED.,.F.,.F.,(4,3,4),(0.418312080808486,
0.428571428571429,0.435775021760694),.UNSPECIFIED.);
#21728=B_SPLINE_CURVE_WITH_KNOTS('',3,(#103910,#103911,#103912,#103913,
#103914,#103915),.UNSPECIFIED.,.F.,.F.,(4,2,4),(-0.025296958843695,-0.0126483558867024,
0.),.UNSPECIFIED.);
#21729=B_SPLINE_CURVE_WITH_KNOTS('',3,(#103926,#103927,#103928,#103929,
#103930,#103931,#103932),.UNSPECIFIED.,.F.,.F.,(4,3,4),(0.418312080808666,
0.428571428571429,0.435775021775203),.UNSPECIFIED.);
#21730=B_SPLINE_CURVE_WITH_KNOTS('',3,(#103941,#103942,#103943,#103944,
#103945,#103946),.UNSPECIFIED.,.F.,.F.,(4,2,4),(-0.0252969589066171,-0.0126483559109774,
0.),.UNSPECIFIED.);
#21731=B_SPLINE_CURVE_WITH_KNOTS('',3,(#103957,#103958,#103959,#103960,
#103961,#103962,#103963),.UNSPECIFIED.,.F.,.F.,(4,3,4),(0.418312080805564,
0.428571428571429,0.435775021766875),.UNSPECIFIED.);
#21732=B_SPLINE_CURVE_WITH_KNOTS('',3,(#103972,#103973,#103974,#103975,
#103976,#103977),.UNSPECIFIED.,.F.,.F.,(4,2,4),(-0.025296958834738,-0.0126483558248854,
0.),.UNSPECIFIED.);
#21733=B_SPLINE_CURVE_WITH_KNOTS('',3,(#103988,#103989,#103990,#103991,
#103992,#103993,#103994),.UNSPECIFIED.,.F.,.F.,(4,3,4),(0.418312080801487,
0.428571428571429,0.435775021756058),.UNSPECIFIED.);
#21734=B_SPLINE_CURVE_WITH_KNOTS('',3,(#104003,#104004,#104005,#104006,
#104007,#104008),.UNSPECIFIED.,.F.,.F.,(4,2,4),(-0.0252969588750053,-0.0126483558821439,
0.),.UNSPECIFIED.);
#21735=B_SPLINE_CURVE_WITH_KNOTS('',3,(#104019,#104020,#104021,#104022,
#104023,#104024,#104025),.UNSPECIFIED.,.F.,.F.,(4,3,4),(0.418312080794997,
0.428571428571429,0.435775021752916),.UNSPECIFIED.);
#21736=B_SPLINE_CURVE_WITH_KNOTS('',3,(#104034,#104035,#104036,#104037,
#104038,#104039),.UNSPECIFIED.,.F.,.F.,(4,2,4),(-0.0252969588282311,-0.0126483558783853,
0.),.UNSPECIFIED.);
#21737=B_SPLINE_CURVE_WITH_KNOTS('',3,(#104050,#104051,#104052,#104053,
#104054,#104055,#104056),.UNSPECIFIED.,.F.,.F.,(4,3,4),(0.418312080810649,
0.428571428571429,0.435775021752433),.UNSPECIFIED.);
#21738=B_SPLINE_CURVE_WITH_KNOTS('',3,(#104065,#104066,#104067,#104068,
#104069,#104070),.UNSPECIFIED.,.F.,.F.,(4,2,4),(-0.0252969588845412,-0.0126483558846912,
0.),.UNSPECIFIED.);
#21739=B_SPLINE_CURVE_WITH_KNOTS('',3,(#104081,#104082,#104083,#104084,
#104085,#104086,#104087),.UNSPECIFIED.,.F.,.F.,(4,3,4),(0.418312080811903,
0.428571428571429,0.435775021768874),.UNSPECIFIED.);
#21740=B_SPLINE_CURVE_WITH_KNOTS('',3,(#104096,#104097,#104098,#104099,
#104100,#104101),.UNSPECIFIED.,.F.,.F.,(4,2,4),(-0.0252963500157696,-0.0126482087099505,
0.),.UNSPECIFIED.);
#21741=B_SPLINE_CURVE_WITH_KNOTS('',3,(#104112,#104113,#104114,#104115,
#104116,#104117,#104118),.UNSPECIFIED.,.F.,.F.,(4,3,4),(0.418312080811404,
0.428571428568158,0.435775021492859),.UNSPECIFIED.);
#21742=B_SPLINE_CURVE_WITH_KNOTS('',3,(#104127,#104128,#104129,#104130,
#104131,#104132),.UNSPECIFIED.,.F.,.F.,(4,2,4),(-0.0252969588787896,-0.0126483558460195,
0.),.UNSPECIFIED.);
#21743=B_SPLINE_CURVE_WITH_KNOTS('',3,(#104143,#104144,#104145,#104146,
#104147,#104148,#104149),.UNSPECIFIED.,.F.,.F.,(4,3,4),(0.418312080803512,
0.428571428571429,0.435775021758132),.UNSPECIFIED.);
#21744=B_SPLINE_CURVE_WITH_KNOTS('',3,(#104158,#104159,#104160,#104161,
#104162,#104163),.UNSPECIFIED.,.F.,.F.,(4,2,4),(-0.0252969588807337,-0.01264835587897,
0.),.UNSPECIFIED.);
#21745=B_SPLINE_CURVE_WITH_KNOTS('',3,(#104174,#104175,#104176,#104177,
#104178,#104179,#104180),.UNSPECIFIED.,.F.,.F.,(4,3,4),(0.41831208078803,
0.428571428571429,0.435775021765591),.UNSPECIFIED.);
#21746=B_SPLINE_CURVE_WITH_KNOTS('',3,(#104191,#104192,#104193,#104194,
#104195,#104196),.UNSPECIFIED.,.F.,.F.,(4,2,4),(-0.0252969686694848,-0.0126483614906356,
-6.97684167383361E-11),.UNSPECIFIED.);
#21747=B_SPLINE_CURVE_WITH_KNOTS('',3,(#104213,#104214,#104215,#104216,
#104217,#104218,#104219),.UNSPECIFIED.,.F.,.F.,(4,3,4),(0.34936969607449,
0.357142857142857,0.361565077308306),.UNSPECIFIED.);
#21748=B_SPLINE_CURVE_WITH_KNOTS('',3,(#104220,#104221,#104222,#104223,
#104224,#104225),.UNSPECIFIED.,.F.,.F.,(4,2,4),(7.00580731665936E-10,0.012648362193168,
0.0252968604256022),.UNSPECIFIED.);
#21749=B_SPLINE_CURVE_WITH_KNOTS('',3,(#104256,#104257,#104258,#104259,
#104260,#104261,#104262),.UNSPECIFIED.,.F.,.F.,(4,3,4),(0.349369696074507,
0.357142857142857,0.361565077306898),.UNSPECIFIED.);
#21750=B_SPLINE_CURVE_WITH_KNOTS('',3,(#104263,#104264,#104265,#104266,
#104267,#104268),.UNSPECIFIED.,.F.,.F.,(4,2,4),(7.69823548708584E-10,0.0126483622614854,
0.0252968526961796),.UNSPECIFIED.);
#21751=B_SPLINE_CURVE_WITH_KNOTS('',3,(#104299,#104300,#104301,#104302,
#104303,#104304,#104305),.UNSPECIFIED.,.F.,.F.,(4,3,4),(0.349369696074506,
0.357142857142857,0.361565077301677),.UNSPECIFIED.);
#21752=B_SPLINE_CURVE_WITH_KNOTS('',3,(#104306,#104307,#104308,#104309,
#104310,#104311),.UNSPECIFIED.,.F.,.F.,(4,2,4),(7.50211286994472E-10,0.0126483622730504,
0.0252968521458539),.UNSPECIFIED.);
#21753=B_SPLINE_CURVE_WITH_KNOTS('',3,(#104342,#104343,#104344,#104345,
#104346,#104347,#104348),.UNSPECIFIED.,.F.,.F.,(4,3,4),(0.349369696074504,
0.357142857142857,0.361565077307123),.UNSPECIFIED.);
#21754=B_SPLINE_CURVE_WITH_KNOTS('',3,(#104349,#104350,#104351,#104352,
#104353,#104354),.UNSPECIFIED.,.F.,.F.,(4,2,4),(7.32488769304241E-10,0.0126483622343914,
0.0252969687268146),.UNSPECIFIED.);
#21755=B_SPLINE_CURVE_WITH_KNOTS('',3,(#104385,#104386,#104387,#104388,
#104389,#104390,#104391),.UNSPECIFIED.,.F.,.F.,(4,3,4),(0.349369696074505,
0.357142857142857,0.361565077309921),.UNSPECIFIED.);
#21756=B_SPLINE_CURVE_WITH_KNOTS('',3,(#104392,#104393,#104394,#104395,
#104396,#104397),.UNSPECIFIED.,.F.,.F.,(4,2,4),(8.14431072066256E-10,0.0126483623470854,
0.0252968548170038),.UNSPECIFIED.);
#21757=B_SPLINE_CURVE_WITH_KNOTS('',3,(#104428,#104429,#104430,#104431,
#104432,#104433,#104434),.UNSPECIFIED.,.F.,.F.,(4,3,4),(0.349369696074496,
0.357142857142857,0.361565077307065),.UNSPECIFIED.);
#21758=B_SPLINE_CURVE_WITH_KNOTS('',3,(#104435,#104436,#104437,#104438,
#104439,#104440),.UNSPECIFIED.,.F.,.F.,(4,2,4),(7.81136850193204E-10,0.0126483622731924,
0.0252969686706485),.UNSPECIFIED.);
#21759=B_SPLINE_CURVE_WITH_KNOTS('',3,(#104469,#104470,#104471,#104472,
#104473,#104474),.UNSPECIFIED.,.F.,.F.,(4,2,4),(8.10397729245745E-10,0.0126483623554498,
0.025296856312765),.UNSPECIFIED.);
#21760=B_SPLINE_CURVE_WITH_KNOTS('',3,(#104499,#104500,#104501,#104502,
#104503,#104504,#104505),.UNSPECIFIED.,.F.,.F.,(4,3,4),(0.349369696074502,
0.357142857142857,0.361565077308727),.UNSPECIFIED.);
#21761=B_SPLINE_CURVE_WITH_KNOTS('',3,(#104506,#104507,#104508,#104509,
#104510,#104511),.UNSPECIFIED.,.F.,.F.,(4,2,4),(8.04641163913392E-10,0.0126483623562947,
0.0252968547386476),.UNSPECIFIED.);
#21762=B_SPLINE_CURVE_WITH_KNOTS('',3,(#104542,#104543,#104544,#104545,
#104546,#104547,#104548),.UNSPECIFIED.,.F.,.F.,(4,3,4),(0.349369696074505,
0.357142857142857,0.361565077309479),.UNSPECIFIED.);
#21763=B_SPLINE_CURVE_WITH_KNOTS('',3,(#104549,#104550,#104551,#104552,
#104553,#104554),.UNSPECIFIED.,.F.,.F.,(4,2,4),(7.62322842763532E-10,0.0126483622669495,
0.0252968591342625),.UNSPECIFIED.);
#21764=B_SPLINE_CURVE_WITH_KNOTS('',3,(#104585,#104586,#104587,#104588,
#104589,#104590,#104591),.UNSPECIFIED.,.F.,.F.,(4,3,4),(0.349369696074486,
0.357142857142857,0.361565077304992),.UNSPECIFIED.);
#21765=B_SPLINE_CURVE_WITH_KNOTS('',3,(#104592,#104593,#104594,#104595,
#104596,#104597),.UNSPECIFIED.,.F.,.F.,(4,2,4),(8.65804712474563E-10,0.0126483624251677,
0.0252968581181851),.UNSPECIFIED.);
#21766=B_SPLINE_CURVE_WITH_KNOTS('',3,(#104628,#104629,#104630,#104631,
#104632,#104633,#104634),.UNSPECIFIED.,.F.,.F.,(4,3,4),(0.349369696074485,
0.357142857142857,0.361565077306903),.UNSPECIFIED.);
#21767=B_SPLINE_CURVE_WITH_KNOTS('',3,(#104635,#104636,#104637,#104638,
#104639,#104640),.UNSPECIFIED.,.F.,.F.,(4,2,4),(8.39204876451129E-10,0.0126483623445493,
0.0252969686854641),.UNSPECIFIED.);
#21768=B_SPLINE_CURVE_WITH_KNOTS('',3,(#104671,#104672,#104673,#104674,
#104675,#104676,#104677),.UNSPECIFIED.,.F.,.F.,(4,3,4),(0.349369696074483,
0.357142857142857,0.361565077308867),.UNSPECIFIED.);
#21769=B_SPLINE_CURVE_WITH_KNOTS('',3,(#104678,#104679,#104680,#104681,
#104682,#104683),.UNSPECIFIED.,.F.,.F.,(4,2,4),(6.69232072890605E-10,0.0126483621759807,
0.0252968521824175),.UNSPECIFIED.);
#21770=B_SPLINE_CURVE_WITH_KNOTS('',3,(#104714,#104715,#104716,#104717,
#104718,#104719,#104720),.UNSPECIFIED.,.F.,.F.,(4,3,4),(0.349369696074482,
0.357142857142857,0.361565077309969),.UNSPECIFIED.);
#21771=B_SPLINE_CURVE_WITH_KNOTS('',3,(#104721,#104722,#104723,#104724,
#104725,#104726),.UNSPECIFIED.,.F.,.F.,(4,2,4),(8.06443979909319E-10,0.0126483623181598,
0.0252968594199354),.UNSPECIFIED.);
#21772=B_SPLINE_CURVE_WITH_KNOTS('',3,(#104757,#104758,#104759,#104760,
#104761,#104762,#104763),.UNSPECIFIED.,.F.,.F.,(4,3,4),(0.349369696074483,
0.357142857142857,0.361565077303164),.UNSPECIFIED.);
#21773=B_SPLINE_CURVE_WITH_KNOTS('',3,(#104764,#104765,#104766,#104767,
#104768,#104769),.UNSPECIFIED.,.F.,.F.,(4,2,4),(7.81820570877324E-10,0.012648362295298,
0.0252968584739717),.UNSPECIFIED.);
#21774=B_SPLINE_CURVE_WITH_KNOTS('',3,(#104800,#104801,#104802,#104803,
#104804,#104805,#104806),.UNSPECIFIED.,.F.,.F.,(4,3,4),(0.349369696074483,
0.357142857142857,0.361565077304905),.UNSPECIFIED.);
#21775=B_SPLINE_CURVE_WITH_KNOTS('',3,(#104807,#104808,#104809,#104810,
#104811,#104812),.UNSPECIFIED.,.F.,.F.,(4,2,4),(7.71314115196913E-10,0.0126483622892186,
0.0252968544306222),.UNSPECIFIED.);
#21776=B_SPLINE_CURVE_WITH_KNOTS('',3,(#104843,#104844,#104845,#104846,
#104847,#104848,#104849),.UNSPECIFIED.,.F.,.F.,(4,3,4),(0.349369696074483,
0.357142857142857,0.361565077306421),.UNSPECIFIED.);
#21777=B_SPLINE_CURVE_WITH_KNOTS('',3,(#104850,#104851,#104852,#104853,
#104854,#104855),.UNSPECIFIED.,.F.,.F.,(4,2,4),(7.63409067584006E-10,0.0126483622648431,
0.0252969687459862),.UNSPECIFIED.);
#21778=B_SPLINE_CURVE_WITH_KNOTS('',3,(#104886,#104887,#104888,#104889,
#104890,#104891,#104892),.UNSPECIFIED.,.F.,.F.,(4,3,4),(0.349369696074485,
0.357142857142857,0.361565077307845),.UNSPECIFIED.);
#21779=B_SPLINE_CURVE_WITH_KNOTS('',3,(#104893,#104894,#104895,#104896,
#104897,#104898),.UNSPECIFIED.,.F.,.F.,(4,2,4),(7.41711010567428E-10,0.0126483622632217,
0.0252969687427512),.UNSPECIFIED.);
#21780=B_SPLINE_CURVE_WITH_KNOTS('',3,(#104929,#104930,#104931,#104932,
#104933,#104934,#104935),.UNSPECIFIED.,.F.,.F.,(4,3,4),(0.349369696074508,
0.357142857142857,0.361565077311298),.UNSPECIFIED.);
#21781=B_SPLINE_CURVE_WITH_KNOTS('',3,(#104936,#104937,#104938,#104939,
#104940,#104941),.UNSPECIFIED.,.F.,.F.,(4,2,4),(8.26445337013183E-10,0.0126483623626397,
0.02529685160036),.UNSPECIFIED.);
#21782=B_SPLINE_CURVE_WITH_KNOTS('',3,(#104972,#104973,#104974,#104975,
#104976,#104977,#104978),.UNSPECIFIED.,.F.,.F.,(4,3,4),(0.349369696074486,
0.357142857142857,0.36156507730966),.UNSPECIFIED.);
#21783=B_SPLINE_CURVE_WITH_KNOTS('',3,(#104979,#104980,#104981,#104982,
#104983,#104984),.UNSPECIFIED.,.F.,.F.,(4,2,4),(7.94101837835612E-10,0.0126483622803908,
0.025296968651002),.UNSPECIFIED.);
#21784=B_SPLINE_CURVE_WITH_KNOTS('',3,(#105015,#105016,#105017,#105018,
#105019,#105020,#105021),.UNSPECIFIED.,.F.,.F.,(4,3,4),(0.349369696074483,
0.357142857142857,0.361565077307964),.UNSPECIFIED.);
#21785=B_SPLINE_CURVE_WITH_KNOTS('',3,(#105022,#105023,#105024,#105025,
#105026,#105027),.UNSPECIFIED.,.F.,.F.,(4,2,4),(8.07063340628222E-10,0.012648362327054,
0.0252968589528559),.UNSPECIFIED.);
#21786=B_SPLINE_CURVE_WITH_KNOTS('',3,(#105058,#105059,#105060,#105061,
#105062,#105063,#105064),.UNSPECIFIED.,.F.,.F.,(4,3,4),(0.349369696074483,
0.357142857142857,0.361565077309104),.UNSPECIFIED.);
#21787=B_SPLINE_CURVE_WITH_KNOTS('',3,(#105065,#105066,#105067,#105068,
#105069,#105070),.UNSPECIFIED.,.F.,.F.,(4,2,4),(7.65451655524924E-10,0.0126483622724694,
0.0252968591854015),.UNSPECIFIED.);
#21788=B_SPLINE_CURVE_WITH_KNOTS('',3,(#105101,#105102,#105103,#105104,
#105105,#105106,#105107),.UNSPECIFIED.,.F.,.F.,(4,3,4),(0.349369696218661,
0.357142857142857,0.361565077308603),.UNSPECIFIED.);
#21789=B_SPLINE_CURVE_WITH_KNOTS('',3,(#105108,#105109,#105110,#105111,
#105112,#105113),.UNSPECIFIED.,.F.,.F.,(4,2,4),(7.81105724995815E-10,0.0126483623097206,
0.0252968567736768),.UNSPECIFIED.);
#21790=B_SPLINE_CURVE_WITH_KNOTS('',3,(#105144,#105145,#105146,#105147,
#105148,#105149,#105150),.UNSPECIFIED.,.F.,.F.,(4,3,4),(0.349369696074482,
0.357142857142857,0.361565077306041),.UNSPECIFIED.);
#21791=B_SPLINE_CURVE_WITH_KNOTS('',3,(#105151,#105152,#105153,#105154,
#105155,#105156),.UNSPECIFIED.,.F.,.F.,(4,2,4),(8.00844415925551E-10,0.0126483623092148,
0.0252968593149661),.UNSPECIFIED.);
#21792=B_SPLINE_CURVE_WITH_KNOTS('',3,(#105187,#105188,#105189,#105190,
#105191,#105192,#105193),.UNSPECIFIED.,.F.,.F.,(4,3,4),(0.349369696074482,
0.357142857142857,0.361565077235015),.UNSPECIFIED.);
#21793=B_SPLINE_CURVE_WITH_KNOTS('',3,(#105194,#105195,#105196,#105197,
#105198,#105199),.UNSPECIFIED.,.F.,.F.,(4,2,4),(7.92615025759124E-10,0.0126483623291085,
0.0252969675663554),.UNSPECIFIED.);
#21794=B_SPLINE_CURVE_WITH_KNOTS('',3,(#105231,#105232,#105233,#105234,
#105235,#105236,#105237),.UNSPECIFIED.,.F.,.F.,(4,3,4),(0.349369696074483,
0.357142857142857,0.361565077309371),.UNSPECIFIED.);
#21795=B_SPLINE_CURVE_WITH_KNOTS('',3,(#105238,#105239,#105240,#105241,
#105242,#105243),.UNSPECIFIED.,.F.,.F.,(4,2,4),(7.5751650602434E-10,0.0126483622660331,
0.0252968596312452),.UNSPECIFIED.);
#21796=B_SPLINE_CURVE_WITH_KNOTS('',3,(#105273,#105274,#105275,#105276,
#105277,#105278,#105279),.UNSPECIFIED.,.F.,.F.,(4,3,4),(0.349369696074489,
0.357142857142857,0.361565077306682),.UNSPECIFIED.);
#21797=B_SPLINE_CURVE_WITH_KNOTS('',3,(#105280,#105281,#105282,#105283,
#105284,#105285),.UNSPECIFIED.,.F.,.F.,(4,2,4),(7.3826513221905E-10,0.0126483622505896,
0.0252968535266115),.UNSPECIFIED.);
#21798=B_SPLINE_CURVE_WITH_KNOTS('',3,(#105316,#105317,#105318,#105319,
#105320,#105321,#105322),.UNSPECIFIED.,.F.,.F.,(4,3,4),(0.349369696074491,
0.357142857142857,0.36156507730807),.UNSPECIFIED.);
#21799=B_SPLINE_CURVE_WITH_KNOTS('',3,(#105323,#105324,#105325,#105326,
#105327,#105328),.UNSPECIFIED.,.F.,.F.,(4,2,4),(8.11323775009062E-10,0.0126483623175429,
0.0252969686971379),.UNSPECIFIED.);
#21800=B_SPLINE_CURVE_WITH_KNOTS('',3,(#105359,#105360,#105361,#105362,
#105363,#105364,#105365),.UNSPECIFIED.,.F.,.F.,(4,3,4),(0.349369696074491,
0.357142857142857,0.361565077311784),.UNSPECIFIED.);
#21801=B_SPLINE_CURVE_WITH_KNOTS('',3,(#105366,#105367,#105368,#105369,
#105370,#105371),.UNSPECIFIED.,.F.,.F.,(4,2,4),(8.09533550101154E-10,0.0126483623456002,
0.0252968596199317),.UNSPECIFIED.);
#21802=B_SPLINE_CURVE_WITH_KNOTS('',3,(#105391,#105392,#105393,#105394,
#105395,#105396,#105397),.UNSPECIFIED.,.F.,.F.,(4,3,4),(0.349369696074489,
0.357142857142857,0.36156507730976),.UNSPECIFIED.);
#21803=B_SPLINE_CURVE_WITH_KNOTS('',3,(#105424,#105425,#105426,#105427,
#105428,#105429),.UNSPECIFIED.,.F.,.F.,(4,2,4),(-0.0253004834485108,-0.0126501091547225,
0.),.UNSPECIFIED.);
#21804=B_SPLINE_CURVE_WITH_KNOTS('',3,(#105450,#105451,#105452,#105453,
#105454,#105455,#105456),.UNSPECIFIED.,.F.,.F.,(4,3,4),(0.418382980245727,
0.425586573424719,0.43056953839039),.UNSPECIFIED.);
#21805=B_SPLINE_CURVE_WITH_KNOTS('',3,(#105457,#105458,#105459,#105460,
#105461,#105462),.UNSPECIFIED.,.F.,.F.,(4,2,4),(0.,0.0126500391806866,0.025300173152611),
 .UNSPECIFIED.);
#21806=B_SPLINE_CURVE_WITH_KNOTS('',3,(#105497,#105498,#105499,#105500,
#105501,#105502,#105503),.UNSPECIFIED.,.F.,.F.,(4,3,4),(0.418382980245723,
0.425586573424717,0.430569538378419),.UNSPECIFIED.);
#21807=B_SPLINE_CURVE_WITH_KNOTS('',3,(#105504,#105505,#105506,#105507,
#105508,#105509),.UNSPECIFIED.,.F.,.F.,(4,2,4),(0.,0.0126500373960896,0.0253001674275433),
 .UNSPECIFIED.);
#21808=B_SPLINE_CURVE_WITH_KNOTS('',3,(#105544,#105545,#105546,#105547,
#105548,#105549,#105550),.UNSPECIFIED.,.F.,.F.,(4,3,4),(0.418382980245722,
0.425586573424716,0.430569538399632),.UNSPECIFIED.);
#21809=B_SPLINE_CURVE_WITH_KNOTS('',3,(#105551,#105552,#105553,#105554,
#105555,#105556),.UNSPECIFIED.,.F.,.F.,(4,2,4),(0.,0.0126500411768972,0.0253001831563636),
 .UNSPECIFIED.);
#21810=B_SPLINE_CURVE_WITH_KNOTS('',3,(#105591,#105592,#105593,#105594,
#105595,#105596,#105597),.UNSPECIFIED.,.F.,.F.,(4,3,4),(0.418382980245724,
0.425586573424717,0.430569538392051),.UNSPECIFIED.);
#21811=B_SPLINE_CURVE_WITH_KNOTS('',3,(#105598,#105599,#105600,#105601,
#105602,#105603),.UNSPECIFIED.,.F.,.F.,(4,2,4),(0.,0.0126500418776801,0.0253001843093937),
 .UNSPECIFIED.);
#21812=B_SPLINE_CURVE_WITH_KNOTS('',3,(#105638,#105639,#105640,#105641,
#105642,#105643,#105644),.UNSPECIFIED.,.F.,.F.,(4,3,4),(0.418382980245725,
0.425586573424718,0.4305695383971),.UNSPECIFIED.);
#21813=B_SPLINE_CURVE_WITH_KNOTS('',3,(#105645,#105646,#105647,#105648,
#105649,#105650),.UNSPECIFIED.,.F.,.F.,(4,2,4),(0.,0.0126500363474391,0.025300163098201),
 .UNSPECIFIED.);
#21814=B_SPLINE_CURVE_WITH_KNOTS('',3,(#105685,#105686,#105687,#105688,
#105689,#105690,#105691),.UNSPECIFIED.,.F.,.F.,(4,3,4),(0.418382980245724,
0.425586573424719,0.430569538393884),.UNSPECIFIED.);
#21815=B_SPLINE_CURVE_WITH_KNOTS('',3,(#105692,#105693,#105694,#105695,
#105696,#105697),.UNSPECIFIED.,.F.,.F.,(4,2,4),(0.,0.0126500414911137,0.0253001827568244),
 .UNSPECIFIED.);
#21816=B_SPLINE_CURVE_WITH_KNOTS('',3,(#105732,#105733,#105734,#105735,
#105736,#105737,#105738),.UNSPECIFIED.,.F.,.F.,(4,3,4),(0.418382980245725,
0.425586573424719,0.430569538386616),.UNSPECIFIED.);
#21817=B_SPLINE_CURVE_WITH_KNOTS('',3,(#105739,#105740,#105741,#105742,
#105743,#105744),.UNSPECIFIED.,.F.,.F.,(4,2,4),(0.,0.0126500410508636,0.0253001825996073),
 .UNSPECIFIED.);
#21818=B_SPLINE_CURVE_WITH_KNOTS('',3,(#105779,#105780,#105781,#105782,
#105783,#105784,#105785),.UNSPECIFIED.,.F.,.F.,(4,3,4),(0.418382980245726,
0.425586573424719,0.430569538390433),.UNSPECIFIED.);
#21819=B_SPLINE_CURVE_WITH_KNOTS('',3,(#105786,#105787,#105788,#105789,
#105790,#105791),.UNSPECIFIED.,.F.,.F.,(4,2,4),(0.,0.0126500463105737,0.0253002044259655),
 .UNSPECIFIED.);
#21820=B_SPLINE_CURVE_WITH_KNOTS('',3,(#105826,#105827,#105828,#105829,
#105830,#105831,#105832),.UNSPECIFIED.,.F.,.F.,(4,3,4),(0.418382980245725,
0.425586573424719,0.430569538389505),.UNSPECIFIED.);
#21821=B_SPLINE_CURVE_WITH_KNOTS('',3,(#105833,#105834,#105835,#105836,
#105837,#105838),.UNSPECIFIED.,.F.,.F.,(4,2,4),(0.,0.0126500469432477,0.0253002069662176),
 .UNSPECIFIED.);
#21822=B_SPLINE_CURVE_WITH_KNOTS('',3,(#105873,#105874,#105875,#105876,
#105877,#105878,#105879),.UNSPECIFIED.,.F.,.F.,(4,3,4),(0.418382980245725,
0.425586573424719,0.430569538398029),.UNSPECIFIED.);
#21823=B_SPLINE_CURVE_WITH_KNOTS('',3,(#105880,#105881,#105882,#105883,
#105884,#105885),.UNSPECIFIED.,.F.,.F.,(4,2,4),(0.,0.0126500409124451,0.0253001820291273),
 .UNSPECIFIED.);
#21824=B_SPLINE_CURVE_WITH_KNOTS('',3,(#105920,#105921,#105922,#105923,
#105924,#105925,#105926),.UNSPECIFIED.,.F.,.F.,(4,3,4),(0.418382980245725,
0.425586573424719,0.430569538391061),.UNSPECIFIED.);
#21825=B_SPLINE_CURVE_WITH_KNOTS('',3,(#105927,#105928,#105929,#105930,
#105931,#105932),.UNSPECIFIED.,.F.,.F.,(4,2,4),(0.,0.0126500343052672,0.025300152987705),
 .UNSPECIFIED.);
#21826=B_SPLINE_CURVE_WITH_KNOTS('',3,(#105967,#105968,#105969,#105970,
#105971,#105972,#105973),.UNSPECIFIED.,.F.,.F.,(4,3,4),(0.418382980245725,
0.425586573424719,0.430569538390843),.UNSPECIFIED.);
#21827=B_SPLINE_CURVE_WITH_KNOTS('',3,(#105974,#105975,#105976,#105977,
#105978,#105979),.UNSPECIFIED.,.F.,.F.,(4,2,4),(0.,0.0126500451007784,0.0253001993831248),
 .UNSPECIFIED.);
#21828=B_SPLINE_CURVE_WITH_KNOTS('',3,(#106014,#106015,#106016,#106017,
#106018,#106019,#106020),.UNSPECIFIED.,.F.,.F.,(4,3,4),(0.418382980245737,
0.425586573424719,0.430569538385267),.UNSPECIFIED.);
#21829=B_SPLINE_CURVE_WITH_KNOTS('',3,(#106021,#106022,#106023,#106024,
#106025,#106026),.UNSPECIFIED.,.F.,.F.,(4,2,4),(0.,0.0126500265595761,0.0253001225025087),
 .UNSPECIFIED.);
#21830=B_SPLINE_CURVE_WITH_KNOTS('',3,(#106059,#106060,#106061,#106062,
#106063,#106064),.UNSPECIFIED.,.F.,.F.,(4,2,4),(0.,0.0126500408464834,0.0253001817619994),
 .UNSPECIFIED.);
#21831=B_SPLINE_CURVE_WITH_KNOTS('',3,(#106093,#106094,#106095,#106096,
#106097,#106098,#106099),.UNSPECIFIED.,.F.,.F.,(4,3,4),(0.418382980245723,
0.425586573424718,0.430569538398013),.UNSPECIFIED.);
#21832=B_SPLINE_CURVE_WITH_KNOTS('',3,(#106100,#106101,#106102,#106103,
#106104,#106105),.UNSPECIFIED.,.F.,.F.,(4,2,4),(0.,0.0126500337393545,0.0253001522465286),
 .UNSPECIFIED.);
#21833=B_SPLINE_CURVE_WITH_KNOTS('',3,(#106140,#106141,#106142,#106143,
#106144,#106145,#106146),.UNSPECIFIED.,.F.,.F.,(4,3,4),(0.418382980245725,
0.425586573424719,0.430569538387757),.UNSPECIFIED.);
#21834=B_SPLINE_CURVE_WITH_KNOTS('',3,(#106147,#106148,#106149,#106150,
#106151,#106152),.UNSPECIFIED.,.F.,.F.,(4,2,4),(0.,0.0126500416219824,0.0253001832968014),
 .UNSPECIFIED.);
#21835=B_SPLINE_CURVE_WITH_KNOTS('',3,(#106187,#106188,#106189,#106190,
#106191,#106192,#106193),.UNSPECIFIED.,.F.,.F.,(4,3,4),(0.418382980245725,
0.425586573424719,0.43056953838762),.UNSPECIFIED.);
#21836=B_SPLINE_CURVE_WITH_KNOTS('',3,(#106194,#106195,#106196,#106197,
#106198,#106199),.UNSPECIFIED.,.F.,.F.,(4,2,4),(0.,0.0126500323628606,0.0253001465573658),
 .UNSPECIFIED.);
#21837=B_SPLINE_CURVE_WITH_KNOTS('',3,(#106234,#106235,#106236,#106237,
#106238,#106239,#106240),.UNSPECIFIED.,.F.,.F.,(4,3,4),(0.418382980245734,
0.425586573424719,0.430569538393455),.UNSPECIFIED.);
#21838=B_SPLINE_CURVE_WITH_KNOTS('',3,(#106241,#106242,#106243,#106244,
#106245,#106246),.UNSPECIFIED.,.F.,.F.,(4,2,4),(0.,0.0126500346168763,0.0253001558984566),
 .UNSPECIFIED.);
#21839=B_SPLINE_CURVE_WITH_KNOTS('',3,(#106281,#106282,#106283,#106284,
#106285,#106286,#106287),.UNSPECIFIED.,.F.,.F.,(4,3,4),(0.418382980245729,
0.425586573424719,0.430569538392008),.UNSPECIFIED.);
#21840=B_SPLINE_CURVE_WITH_KNOTS('',3,(#106288,#106289,#106290,#106291,
#106292,#106293),.UNSPECIFIED.,.F.,.F.,(4,2,4),(0.,0.0126500414343824,0.025300184143714),
 .UNSPECIFIED.);
#21841=B_SPLINE_CURVE_WITH_KNOTS('',3,(#106328,#106329,#106330,#106331,
#106332,#106333,#106334),.UNSPECIFIED.,.F.,.F.,(4,3,4),(0.418382980245735,
0.425586573424719,0.430569538400022),.UNSPECIFIED.);
#21842=B_SPLINE_CURVE_WITH_KNOTS('',3,(#106335,#106336,#106337,#106338,
#106339,#106340),.UNSPECIFIED.,.F.,.F.,(4,2,4),(0.,0.0126500380777214,0.0253001702961879),
 .UNSPECIFIED.);
#21843=B_SPLINE_CURVE_WITH_KNOTS('',3,(#106375,#106376,#106377,#106378,
#106379,#106380,#106381),.UNSPECIFIED.,.F.,.F.,(4,3,4),(0.418382980245724,
0.425586573424719,0.430569538389702),.UNSPECIFIED.);
#21844=B_SPLINE_CURVE_WITH_KNOTS('',3,(#106382,#106383,#106384,#106385,
#106386,#106387),.UNSPECIFIED.,.F.,.F.,(4,2,4),(0.,0.0126500397057998,0.0253001753999798),
 .UNSPECIFIED.);
#21845=B_SPLINE_CURVE_WITH_KNOTS('',3,(#106422,#106423,#106424,#106425,
#106426,#106427,#106428),.UNSPECIFIED.,.F.,.F.,(4,3,4),(0.418382980245737,
0.425586573424719,0.430569538402528),.UNSPECIFIED.);
#21846=B_SPLINE_CURVE_WITH_KNOTS('',3,(#106429,#106430,#106431,#106432,
#106433,#106434),.UNSPECIFIED.,.F.,.F.,(4,2,4),(0.,0.0126500408866683,0.0253001802457082),
 .UNSPECIFIED.);
#21847=B_SPLINE_CURVE_WITH_KNOTS('',3,(#106469,#106470,#106471,#106472,
#106473,#106474,#106475),.UNSPECIFIED.,.F.,.F.,(4,3,4),(0.418382980245736,
0.425586573424719,0.430569538397518),.UNSPECIFIED.);
#21848=B_SPLINE_CURVE_WITH_KNOTS('',3,(#106476,#106477,#106478,#106479,
#106480,#106481),.UNSPECIFIED.,.F.,.F.,(4,2,4),(0.,0.0126500372775695,0.0253001652845494),
 .UNSPECIFIED.);
#21849=B_SPLINE_CURVE_WITH_KNOTS('',3,(#106516,#106517,#106518,#106519,
#106520,#106521,#106522),.UNSPECIFIED.,.F.,.F.,(4,3,4),(0.418382980245731,
0.425586573424719,0.430569538388258),.UNSPECIFIED.);
#21850=B_SPLINE_CURVE_WITH_KNOTS('',3,(#106523,#106524,#106525,#106526,
#106527,#106528),.UNSPECIFIED.,.F.,.F.,(4,2,4),(0.,0.0126500414738515,0.0253001843471962),
 .UNSPECIFIED.);
#21851=B_SPLINE_CURVE_WITH_KNOTS('',3,(#106563,#106564,#106565,#106566,
#106567,#106568,#106569),.UNSPECIFIED.,.F.,.F.,(4,3,4),(0.418382980245733,
0.425586573424719,0.430569538390303),.UNSPECIFIED.);
#21852=B_SPLINE_CURVE_WITH_KNOTS('',3,(#106570,#106571,#106572,#106573,
#106574,#106575),.UNSPECIFIED.,.F.,.F.,(4,2,4),(0.,0.0126500431760547,0.0253001897296639),
 .UNSPECIFIED.);
#21853=B_SPLINE_CURVE_WITH_KNOTS('',3,(#106610,#106611,#106612,#106613,
#106614,#106615,#106616),.UNSPECIFIED.,.F.,.F.,(4,3,4),(0.418382980245732,
0.425586573424719,0.430569538389363),.UNSPECIFIED.);
#21854=B_SPLINE_CURVE_WITH_KNOTS('',3,(#106617,#106618,#106619,#106620,
#106621,#106622),.UNSPECIFIED.,.F.,.F.,(4,2,4),(0.,0.0126500312589351,0.0253001419686268),
 .UNSPECIFIED.);
#21855=B_SPLINE_CURVE_WITH_KNOTS('',3,(#106657,#106658,#106659,#106660,
#106661,#106662,#106663),.UNSPECIFIED.,.F.,.F.,(4,3,4),(0.418382980245735,
0.425586573424719,0.430569538384267),.UNSPECIFIED.);
#21856=B_SPLINE_CURVE_WITH_KNOTS('',3,(#106664,#106665,#106666,#106667,
#106668,#106669),.UNSPECIFIED.,.F.,.F.,(4,2,4),(0.,0.0126500413506874,0.0253001821506214),
 .UNSPECIFIED.);
#21857=B_SPLINE_CURVE_WITH_KNOTS('',3,(#106704,#106705,#106706,#106707,
#106708,#106709,#106710),.UNSPECIFIED.,.F.,.F.,(4,3,4),(0.418382980245734,
0.425586573424719,0.430569538388081),.UNSPECIFIED.);
#21858=B_SPLINE_CURVE_WITH_KNOTS('',3,(#106711,#106712,#106713,#106714,
#106715,#106716),.UNSPECIFIED.,.F.,.F.,(4,2,4),(0.,0.0126500449936537,0.0253001972767284),
 .UNSPECIFIED.);
#21859=B_SPLINE_CURVE_WITH_KNOTS('',3,(#106736,#106737,#106738,#106739,
#106740,#106741,#106742),.UNSPECIFIED.,.F.,.F.,(4,3,4),(0.418382980245736,
0.425586573424719,0.430569538291038),.UNSPECIFIED.);
#21860=B_SPLINE_CURVE_WITH_KNOTS('',3,(#106769,#106770,#106771,#106772,
#106773,#106774),.UNSPECIFIED.,.F.,.F.,(4,2,4),(-0.0253039373669134,-0.0126520853650402,
-1.68311233006424E-11),.UNSPECIFIED.);
#21861=B_SPLINE_CURVE_WITH_KNOTS('',3,(#106792,#106793,#106794,#106795,
#106796,#106797),.UNSPECIFIED.,.F.,.F.,(4,2,4),(5.00322396733526E-11,0.0126520854893629,
0.0253039374589922),.UNSPECIFIED.);
#21862=B_SPLINE_CURVE_WITH_KNOTS('',3,(#106822,#106823,#106824,#106825,
#106826,#106827),.UNSPECIFIED.,.F.,.F.,(4,2,4),(0.,0.0126521070316687,0.0253039905324995),
 .UNSPECIFIED.);
#21863=B_SPLINE_CURVE_WITH_KNOTS('',3,(#106852,#106853,#106854,#106855,
#106856,#106857),.UNSPECIFIED.,.F.,.F.,(4,2,4),(3.2725810366945E-11,0.012652085552786,
0.0253039375042351),.UNSPECIFIED.);
#21864=B_SPLINE_CURVE_WITH_KNOTS('',3,(#106882,#106883,#106884,#106885,
#106886,#106887),.UNSPECIFIED.,.F.,.F.,(4,2,4),(3.62590749629602E-11,0.0126520854371781,
0.0253039374058216),.UNSPECIFIED.);
#21865=B_SPLINE_CURVE_WITH_KNOTS('',3,(#106912,#106913,#106914,#106915,
#106916,#106917),.UNSPECIFIED.,.F.,.F.,(4,2,4),(2.02885766718425E-11,0.0126520854063949,
0.0253039373604974),.UNSPECIFIED.);
#21866=B_SPLINE_CURVE_WITH_KNOTS('',3,(#106942,#106943,#106944,#106945,
#106946,#106947),.UNSPECIFIED.,.F.,.F.,(4,2,4),(0.,0.0126521067265982,0.0253039898193607),
 .UNSPECIFIED.);
#21867=B_SPLINE_CURVE_WITH_KNOTS('',3,(#106972,#106973,#106974,#106975,
#106976,#106977),.UNSPECIFIED.,.F.,.F.,(4,2,4),(3.68450136684406E-11,0.0126520854796589,
0.0253039374247473),.UNSPECIFIED.);
#21868=B_SPLINE_CURVE_WITH_KNOTS('',3,(#107002,#107003,#107004,#107005,
#107006,#107007),.UNSPECIFIED.,.F.,.F.,(4,2,4),(2.96031499286255E-11,0.0126520854663196,
0.0253039374535887),.UNSPECIFIED.);
#21869=B_SPLINE_CURVE_WITH_KNOTS('',3,(#107032,#107033,#107034,#107035,
#107036,#107037),.UNSPECIFIED.,.F.,.F.,(4,2,4),(4.94442604005428E-11,0.0126520854736033,
0.0253039374303011),.UNSPECIFIED.);
#21870=B_SPLINE_CURVE_WITH_KNOTS('',3,(#107062,#107063,#107064,#107065,
#107066,#107067),.UNSPECIFIED.,.F.,.F.,(4,2,4),(3.71849020065102E-11,0.0126520855144434,
0.0253039374629825),.UNSPECIFIED.);
#21871=B_SPLINE_CURVE_WITH_KNOTS('',3,(#107092,#107093,#107094,#107095,
#107096,#107097),.UNSPECIFIED.,.F.,.F.,(4,2,4),(0.,0.0126521066711647,0.0253039897145172),
 .UNSPECIFIED.);
#21872=B_SPLINE_CURVE_WITH_KNOTS('',3,(#107122,#107123,#107124,#107125,
#107126,#107127),.UNSPECIFIED.,.F.,.F.,(4,2,4),(3.91930707781718E-11,0.0126520854197006,
0.0253039373881218),.UNSPECIFIED.);
#21873=B_SPLINE_CURVE_WITH_KNOTS('',3,(#107152,#107153,#107154,#107155,
#107156,#107157),.UNSPECIFIED.,.F.,.F.,(4,2,4),(3.22351797597082E-11,0.0126520854379891,
0.0253039374147879),.UNSPECIFIED.);
#21874=B_SPLINE_CURVE_WITH_KNOTS('',3,(#107182,#107183,#107184,#107185,
#107186,#107187),.UNSPECIFIED.,.F.,.F.,(4,2,4),(0.,0.0126521071464492,0.0253039907276813),
 .UNSPECIFIED.);
#21875=B_SPLINE_CURVE_WITH_KNOTS('',3,(#107212,#107213,#107214,#107215,
#107216,#107217),.UNSPECIFIED.,.F.,.F.,(4,2,4),(2.49933480749287E-11,0.012652085408633,
0.0253039373642647),.UNSPECIFIED.);
#21876=B_SPLINE_CURVE_WITH_KNOTS('',3,(#107242,#107243,#107244,#107245,
#107246,#107247),.UNSPECIFIED.,.F.,.F.,(4,2,4),(2.40689927792338E-11,0.0126520853975297,
0.0253039373640824),.UNSPECIFIED.);
#21877=B_SPLINE_CURVE_WITH_KNOTS('',3,(#107272,#107273,#107274,#107275,
#107276,#107277),.UNSPECIFIED.,.F.,.F.,(4,2,4),(0.,0.0126521065211899,0.025303989285167),
 .UNSPECIFIED.);
#21878=B_SPLINE_CURVE_WITH_KNOTS('',3,(#107302,#107303,#107304,#107305,
#107306,#107307),.UNSPECIFIED.,.F.,.F.,(4,2,4),(4.20186388401848E-11,0.0126520855280583,
0.0253039374729705),.UNSPECIFIED.);
#21879=B_SPLINE_CURVE_WITH_KNOTS('',3,(#107332,#107333,#107334,#107335,
#107336,#107337),.UNSPECIFIED.,.F.,.F.,(4,2,4),(4.83695302925847E-11,0.0126520855344403,
0.0253039374579568),.UNSPECIFIED.);
#21880=B_SPLINE_CURVE_WITH_KNOTS('',3,(#107362,#107363,#107364,#107365,
#107366,#107367),.UNSPECIFIED.,.F.,.F.,(4,2,4),(0.,0.0126521066564263,0.025303989600833),
 .UNSPECIFIED.);
#21881=B_SPLINE_CURVE_WITH_KNOTS('',3,(#107392,#107393,#107394,#107395,
#107396,#107397),.UNSPECIFIED.,.F.,.F.,(4,2,4),(0.,0.0126521065478162,0.0253039894337947),
 .UNSPECIFIED.);
#21882=B_SPLINE_CURVE_WITH_KNOTS('',3,(#107422,#107423,#107424,#107425,
#107426,#107427),.UNSPECIFIED.,.F.,.F.,(4,2,4),(3.73971469161031E-11,0.0126520854361138,
0.0253039374245403),.UNSPECIFIED.);
#21883=B_SPLINE_CURVE_WITH_KNOTS('',3,(#107452,#107453,#107454,#107455,
#107456,#107457),.UNSPECIFIED.,.F.,.F.,(4,2,4),(0.,0.0126521067630497,0.0253039898367866),
 .UNSPECIFIED.);
#21884=B_SPLINE_CURVE_WITH_KNOTS('',3,(#107482,#107483,#107484,#107485,
#107486,#107487),.UNSPECIFIED.,.F.,.F.,(4,2,4),(0.,0.0126521069832498,0.0253039905019251),
 .UNSPECIFIED.);
#21885=B_SPLINE_CURVE_WITH_KNOTS('',3,(#107512,#107513,#107514,#107515,
#107516,#107517),.UNSPECIFIED.,.F.,.F.,(4,2,4),(0.,0.0126521057049491,0.0253039872136905),
 .UNSPECIFIED.);
#21886=B_SPLINE_CURVE_WITH_KNOTS('',3,(#107542,#107543,#107544,#107545,
#107546,#107547),.UNSPECIFIED.,.F.,.F.,(4,2,4),(3.70643827480995E-11,0.0126520855149235,
0.0253039374681902),.UNSPECIFIED.);
#21887=B_SPLINE_CURVE_WITH_KNOTS('',3,(#107572,#107573,#107574,#107575,
#107576,#107577),.UNSPECIFIED.,.F.,.F.,(4,2,4),(2.5219425645624E-11,0.0126520853989294,
0.0253039373990772),.UNSPECIFIED.);
#21888=B_SPLINE_CURVE_WITH_KNOTS('',3,(#107602,#107603,#107604,#107605,
#107606,#107607),.UNSPECIFIED.,.F.,.F.,(4,2,4),(0.,0.0126521068930367,0.0253039901669712),
 .UNSPECIFIED.);
#21889=B_SPLINE_CURVE_WITH_KNOTS('',3,(#107638,#107639,#107640,#107641,
#107642,#107643),.UNSPECIFIED.,.F.,.F.,(4,2,4),(-0.0239802018525615,-0.0121950471650718,
0.),.UNSPECIFIED.);
#21890=B_SPLINE_CURVE_WITH_KNOTS('',3,(#107656,#107657,#107658,#107659,
#107660,#107661,#107662,#107663,#107664,#107665),.UNSPECIFIED.,.F.,.F.,
(4,3,3,4),(0.280433083274049,0.285714285714286,0.295522983040218,0.297856505248244),
 .UNSPECIFIED.);
#21891=B_SPLINE_CURVE_WITH_KNOTS('',3,(#107666,#107667,#107668,#107669,
#107670,#107671),.UNSPECIFIED.,.F.,.F.,(4,2,4),(1.96584679017892E-11,0.0121950713546208,
0.0239801149705389),.UNSPECIFIED.);
#21892=B_SPLINE_CURVE_WITH_KNOTS('',3,(#107690,#107691,#107692,#107693,
#107694,#107695,#107696,#107697,#107698,#107699),.UNSPECIFIED.,.F.,.F.,
(4,3,3,4),(0.280433083285969,0.285714285714286,0.295522995362072,0.297856505172786),
 .UNSPECIFIED.);
#21893=B_SPLINE_CURVE_WITH_KNOTS('',3,(#107700,#107701,#107702,#107703,
#107704,#107705),.UNSPECIFIED.,.F.,.F.,(4,2,4),(0.,0.012195047336033,0.0239801017797112),
 .UNSPECIFIED.);
#21894=B_SPLINE_CURVE_WITH_KNOTS('',3,(#107724,#107725,#107726,#107727,
#107728,#107729,#107730,#107731,#107732,#107733),.UNSPECIFIED.,.F.,.F.,
(4,3,3,4),(0.280433083276854,0.285714285714286,0.295522991230299,0.297856505265968),
 .UNSPECIFIED.);
#21895=B_SPLINE_CURVE_WITH_KNOTS('',3,(#107734,#107735,#107736,#107737,
#107738,#107739),.UNSPECIFIED.,.F.,.F.,(4,2,4),(0.,0.0121950484646937,0.0239801019007123),
 .UNSPECIFIED.);
#21896=B_SPLINE_CURVE_WITH_KNOTS('',3,(#107758,#107759,#107760,#107761,
#107762,#107763,#107764,#107765,#107766,#107767),.UNSPECIFIED.,.F.,.F.,
(4,3,3,4),(0.280433083284697,0.285714285714286,0.295522993835511,0.297856505255382),
 .UNSPECIFIED.);
#21897=B_SPLINE_CURVE_WITH_KNOTS('',3,(#107768,#107769,#107770,#107771,
#107772,#107773),.UNSPECIFIED.,.F.,.F.,(4,2,4),(1.35452992190566E-11,0.0121950714296532,
0.0239801142217455),.UNSPECIFIED.);
#21898=B_SPLINE_CURVE_WITH_KNOTS('',3,(#107792,#107793,#107794,#107795,
#107796,#107797,#107798,#107799,#107800,#107801),.UNSPECIFIED.,.F.,.F.,
(4,3,3,4),(0.280433083290967,0.285714285714286,0.295522994762218,0.297856505265025),
 .UNSPECIFIED.);
#21899=B_SPLINE_CURVE_WITH_KNOTS('',3,(#107802,#107803,#107804,#107805,
#107806,#107807),.UNSPECIFIED.,.F.,.F.,(4,2,4),(0.,0.0121950482292334,0.0239801014592522),
 .UNSPECIFIED.);
#21900=B_SPLINE_CURVE_WITH_KNOTS('',3,(#107826,#107827,#107828,#107829,
#107830,#107831,#107832,#107833,#107834,#107835),.UNSPECIFIED.,.F.,.F.,
(4,3,3,4),(0.280433083288239,0.285714285714286,0.295522996978597,0.297856505254091),
 .UNSPECIFIED.);
#21901=B_SPLINE_CURVE_WITH_KNOTS('',3,(#107836,#107837,#107838,#107839,
#107840,#107841),.UNSPECIFIED.,.F.,.F.,(4,2,4),(1.58847548231737E-11,0.0121950487701971,
0.0239801006388348),.UNSPECIFIED.);
#21902=B_SPLINE_CURVE_WITH_KNOTS('',3,(#107860,#107861,#107862,#107863,
#107864,#107865,#107866,#107867,#107868,#107869),.UNSPECIFIED.,.F.,.F.,
(4,3,3,4),(0.280433083282487,0.285714285714286,0.295523001219465,0.297856505259234),
 .UNSPECIFIED.);
#21903=B_SPLINE_CURVE_WITH_KNOTS('',3,(#107870,#107871,#107872,#107873,
#107874,#107875),.UNSPECIFIED.,.F.,.F.,(4,2,4),(3.69147784996206E-12,0.0121950483221972,
0.0239800995344619),.UNSPECIFIED.);
#21904=B_SPLINE_CURVE_WITH_KNOTS('',3,(#107894,#107895,#107896,#107897,
#107898,#107899,#107900,#107901,#107902,#107903),.UNSPECIFIED.,.F.,.F.,
(4,3,3,4),(0.280433083270248,0.285714285714286,0.29552299698461,0.297856505261087),
 .UNSPECIFIED.);
#21905=B_SPLINE_CURVE_WITH_KNOTS('',3,(#107904,#107905,#107906,#107907,
#107908,#107909),.UNSPECIFIED.,.F.,.F.,(4,2,4),(3.16935510257326E-11,0.0121950711124471,
0.0239802523921913),.UNSPECIFIED.);
#21906=B_SPLINE_CURVE_WITH_KNOTS('',3,(#107928,#107929,#107930,#107931,
#107932,#107933,#107934,#107935,#107936,#107937),.UNSPECIFIED.,.F.,.F.,
(4,3,3,4),(0.280433083278328,0.285714285714286,0.295522993463896,0.297856505255155),
 .UNSPECIFIED.);
#21907=B_SPLINE_CURVE_WITH_KNOTS('',3,(#107938,#107939,#107940,#107941,
#107942,#107943),.UNSPECIFIED.,.F.,.F.,(4,2,4),(0.,0.0121950479326978,0.0239802446945865),
 .UNSPECIFIED.);
#21908=B_SPLINE_CURVE_WITH_KNOTS('',3,(#107962,#107963,#107964,#107965,
#107966,#107967,#107968,#107969,#107970,#107971),.UNSPECIFIED.,.F.,.F.,
(4,3,3,4),(0.280433083278448,0.285714285714286,0.295522984237966,0.297856505262794),
 .UNSPECIFIED.);
#21909=B_SPLINE_CURVE_WITH_KNOTS('',3,(#107972,#107973,#107974,#107975,
#107976,#107977),.UNSPECIFIED.,.F.,.F.,(4,2,4),(1.19422519947047E-11,0.0121950722182005,
0.0239801149202022),.UNSPECIFIED.);
#21910=B_SPLINE_CURVE_WITH_KNOTS('',3,(#107996,#107997,#107998,#107999,
#108000,#108001,#108002,#108003,#108004,#108005),.UNSPECIFIED.,.F.,.F.,
(4,3,3,4),(0.280433083272196,0.285714285714286,0.295522983838497,0.297856505268764),
 .UNSPECIFIED.);
#21911=B_SPLINE_CURVE_WITH_KNOTS('',3,(#108006,#108007,#108008,#108009,
#108010,#108011),.UNSPECIFIED.,.F.,.F.,(4,2,4),(2.37913079241714E-11,0.0121950715982599,
0.0239801154865616),.UNSPECIFIED.);
#21912=B_SPLINE_CURVE_WITH_KNOTS('',3,(#108030,#108031,#108032,#108033,
#108034,#108035,#108036,#108037,#108038,#108039),.UNSPECIFIED.,.F.,.F.,
(4,3,3,4),(0.280433083265126,0.285714285714286,0.295522972255689,0.297856505261105),
 .UNSPECIFIED.);
#21913=B_SPLINE_CURVE_WITH_KNOTS('',3,(#108040,#108041,#108042,#108043,
#108044,#108045),.UNSPECIFIED.,.F.,.F.,(4,2,4),(1.79830820846869E-11,0.0121950496409893,
0.0239801035787929),.UNSPECIFIED.);
#21914=B_SPLINE_CURVE_WITH_KNOTS('',3,(#108064,#108065,#108066,#108067,
#108068,#108069,#108070,#108071,#108072,#108073),.UNSPECIFIED.,.F.,.F.,
(4,3,3,4),(0.280433083271004,0.285714285714286,0.295523013441985,0.297856505260165),
 .UNSPECIFIED.);
#21915=B_SPLINE_CURVE_WITH_KNOTS('',3,(#108074,#108075,#108076,#108077,
#108078,#108079),.UNSPECIFIED.,.F.,.F.,(4,2,4),(1.86023239308098E-11,0.0121950714651211,
0.0239801130672781),.UNSPECIFIED.);
#21916=B_SPLINE_CURVE_WITH_KNOTS('',3,(#108098,#108099,#108100,#108101,
#108102,#108103,#108104,#108105,#108106,#108107),.UNSPECIFIED.,.F.,.F.,
(4,3,3,4),(0.280433083273177,0.285714285714286,0.295522970086385,0.297856505263728),
 .UNSPECIFIED.);
#21917=B_SPLINE_CURVE_WITH_KNOTS('',3,(#108108,#108109,#108110,#108111,
#108112,#108113),.UNSPECIFIED.,.F.,.F.,(4,2,4),(0.,0.01219507291151,0.0239801176553648),
 .UNSPECIFIED.);
#21918=B_SPLINE_CURVE_WITH_KNOTS('',3,(#108132,#108133,#108134,#108135,
#108136,#108137,#108138,#108139,#108140,#108141),.UNSPECIFIED.,.F.,.F.,
(4,3,3,4),(0.280433083276883,0.285714285714286,0.295522990479267,0.297856505260856),
 .UNSPECIFIED.);
#21919=B_SPLINE_CURVE_WITH_KNOTS('',3,(#108142,#108143,#108144,#108145,
#108146,#108147),.UNSPECIFIED.,.F.,.F.,(4,2,4),(1.53035637300338E-11,0.01219504982936,
0.0239802464558618),.UNSPECIFIED.);
#21920=B_SPLINE_CURVE_WITH_KNOTS('',3,(#108166,#108167,#108168,#108169,
#108170,#108171,#108172,#108173,#108174,#108175),.UNSPECIFIED.,.F.,.F.,
(4,3,3,4),(0.280433083287991,0.285714285714286,0.295522992480121,0.297856505269155),
 .UNSPECIFIED.);
#21921=B_SPLINE_CURVE_WITH_KNOTS('',3,(#108176,#108177,#108178,#108179,
#108180,#108181),.UNSPECIFIED.,.F.,.F.,(4,2,4),(0.,0.0121950472906913,0.0239801004075415),
 .UNSPECIFIED.);
#21922=B_SPLINE_CURVE_WITH_KNOTS('',3,(#108200,#108201,#108202,#108203,
#108204,#108205,#108206,#108207,#108208,#108209),.UNSPECIFIED.,.F.,.F.,
(4,3,3,4),(0.280433083278512,0.285714285714286,0.295522990639051,0.297856505260552),
 .UNSPECIFIED.);
#21923=B_SPLINE_CURVE_WITH_KNOTS('',3,(#108210,#108211,#108212,#108213,
#108214,#108215),.UNSPECIFIED.,.F.,.F.,(4,2,4),(1.43098409550063E-11,0.0121950484351843,
0.0239801006439196),.UNSPECIFIED.);
#21924=B_SPLINE_CURVE_WITH_KNOTS('',3,(#108234,#108235,#108236,#108237,
#108238,#108239,#108240,#108241,#108242,#108243),.UNSPECIFIED.,.F.,.F.,
(4,3,3,4),(0.280433083287628,0.285714285714286,0.29552299030318,0.297856505246354),
 .UNSPECIFIED.);
#21925=B_SPLINE_CURVE_WITH_KNOTS('',3,(#108244,#108245,#108246,#108247,
#108248,#108249),.UNSPECIFIED.,.F.,.F.,(4,2,4),(0.,0.0121950478615351,0.0239802452375475),
 .UNSPECIFIED.);
#21926=B_SPLINE_CURVE_WITH_KNOTS('',3,(#108268,#108269,#108270,#108271,
#108272,#108273,#108274,#108275,#108276,#108277),.UNSPECIFIED.,.F.,.F.,
(4,3,3,4),(0.280433083285338,0.285714285714286,0.295522998736992,0.297856505260913),
 .UNSPECIFIED.);
#21927=B_SPLINE_CURVE_WITH_KNOTS('',3,(#108278,#108279,#108280,#108281,
#108282,#108283),.UNSPECIFIED.,.F.,.F.,(4,2,4),(1.23192632431422E-11,0.0121950718427872,
0.0239801151610334),.UNSPECIFIED.);
#21928=B_SPLINE_CURVE_WITH_KNOTS('',3,(#108302,#108303,#108304,#108305,
#108306,#108307,#108308,#108309,#108310,#108311),.UNSPECIFIED.,.F.,.F.,
(4,3,3,4),(0.280433083281084,0.285714285714286,0.295523005586588,0.29785650526148),
 .UNSPECIFIED.);
#21929=B_SPLINE_CURVE_WITH_KNOTS('',3,(#108312,#108313,#108314,#108315,
#108316,#108317),.UNSPECIFIED.,.F.,.F.,(4,2,4),(0.,0.0121950485817599,0.0239802616992687),
 .UNSPECIFIED.);
#21930=B_SPLINE_CURVE_WITH_KNOTS('',3,(#108336,#108337,#108338,#108339,
#108340,#108341,#108342,#108343,#108344,#108345),.UNSPECIFIED.,.F.,.F.,
(4,3,3,4),(0.280433083273359,0.285714285714286,0.29552298438251,0.297856505254811),
 .UNSPECIFIED.);
#21931=B_SPLINE_CURVE_WITH_KNOTS('',3,(#108346,#108347,#108348,#108349,
#108350,#108351),.UNSPECIFIED.,.F.,.F.,(4,2,4),(0.,0.012195047999912,0.0239801007748419),
 .UNSPECIFIED.);
#21932=B_SPLINE_CURVE_WITH_KNOTS('',3,(#108370,#108371,#108372,#108373,
#108374,#108375,#108376,#108377,#108378,#108379),.UNSPECIFIED.,.F.,.F.,
(4,3,3,4),(0.28043308327774,0.285714285714286,0.295522991827137,0.297856505260904),
 .UNSPECIFIED.);
#21933=B_SPLINE_CURVE_WITH_KNOTS('',3,(#108380,#108381,#108382,#108383,
#108384,#108385),.UNSPECIFIED.,.F.,.F.,(4,2,4),(1.7066885657581E-11,0.0121950714643382,
0.0239802435135067),.UNSPECIFIED.);
#21934=B_SPLINE_CURVE_WITH_KNOTS('',3,(#108404,#108405,#108406,#108407,
#108408,#108409,#108410,#108411,#108412,#108413),.UNSPECIFIED.,.F.,.F.,
(4,3,3,4),(0.280433083267565,0.285714285714286,0.29552299565643,0.297856505250778),
 .UNSPECIFIED.);
#21935=B_SPLINE_CURVE_WITH_KNOTS('',3,(#108414,#108415,#108416,#108417,
#108418,#108419),.UNSPECIFIED.,.F.,.F.,(4,2,4),(0.,0.0121950489545227,0.0239802380202973),
 .UNSPECIFIED.);
#21936=B_SPLINE_CURVE_WITH_KNOTS('',3,(#108438,#108439,#108440,#108441,
#108442,#108443,#108444,#108445,#108446,#108447),.UNSPECIFIED.,.F.,.F.,
(4,3,3,4),(0.28043308327945,0.285714285714286,0.295523008074204,0.297856505255121),
 .UNSPECIFIED.);
#21937=B_SPLINE_CURVE_WITH_KNOTS('',3,(#108448,#108449,#108450,#108451,
#108452,#108453),.UNSPECIFIED.,.F.,.F.,(4,2,4),(3.70023008560456E-12,0.0121950487788839,
0.0239801006020893),.UNSPECIFIED.);
#21938=B_SPLINE_CURVE_WITH_KNOTS('',3,(#108472,#108473,#108474,#108475,
#108476,#108477,#108478,#108479,#108480,#108481),.UNSPECIFIED.,.F.,.F.,
(4,3,3,4),(0.280433083278303,0.285714285714286,0.295522997600256,0.297856505256509),
 .UNSPECIFIED.);
#21939=B_SPLINE_CURVE_WITH_KNOTS('',3,(#108482,#108483,#108484,#108485,
#108486,#108487),.UNSPECIFIED.,.F.,.F.,(4,2,4),(1.94609576978618E-11,0.0121950711287126,
0.0239801127297749),.UNSPECIFIED.);
#21940=B_SPLINE_CURVE_WITH_KNOTS('',3,(#108506,#108507,#108508,#108509,
#108510,#108511,#108512,#108513,#108514,#108515),.UNSPECIFIED.,.F.,.F.,
(4,3,3,4),(0.280433083281729,0.285714285714286,0.295522987820966,0.297856505269623),
 .UNSPECIFIED.);
#21941=B_SPLINE_CURVE_WITH_KNOTS('',3,(#108516,#108517,#108518,#108519,
#108520,#108521),.UNSPECIFIED.,.F.,.F.,(4,2,4),(0.,0.0121950465272298,0.0239800988628031),
 .UNSPECIFIED.);
#21942=B_SPLINE_CURVE_WITH_KNOTS('',3,(#108540,#108541,#108542,#108543,
#108544,#108545,#108546,#108547,#108548,#108549),.UNSPECIFIED.,.F.,.F.,
(4,3,3,4),(0.280433083277661,0.285714285714286,0.295523015653847,0.297856505175428),
 .UNSPECIFIED.);
#21943=B_SPLINE_CURVE_WITH_KNOTS('',3,(#108550,#108551,#108552,#108553,
#108554,#108555),.UNSPECIFIED.,.F.,.F.,(4,2,4),(3.87647476110657E-11,0.0121950705143623,
0.0239801118280503),.UNSPECIFIED.);
#21944=B_SPLINE_CURVE_WITH_KNOTS('',3,(#108574,#108575,#108576,#108577,
#108578,#108579,#108580,#108581,#108582,#108583),.UNSPECIFIED.,.F.,.F.,
(4,3,3,4),(0.280433083277927,0.285714285714286,0.295522982173905,0.297856505255156),
 .UNSPECIFIED.);
#21945=B_SPLINE_CURVE_WITH_KNOTS('',3,(#108584,#108585,#108586,#108587,
#108588,#108589),.UNSPECIFIED.,.F.,.F.,(4,2,4),(3.62025672719479E-11,0.0121950717827385,
0.0239802380575927),.UNSPECIFIED.);
#21946=B_SPLINE_CURVE_WITH_KNOTS('',3,(#108625,#108626,#108627,#108628,
#108629,#108630),.UNSPECIFIED.,.F.,.F.,(4,2,4),(-0.0253011686839678,-0.0126507408832311,
0.),.UNSPECIFIED.);
#21947=B_SPLINE_CURVE_WITH_KNOTS('',3,(#108661,#108662,#108663,#108664,
#108665,#108666),.UNSPECIFIED.,.F.,.F.,(4,2,4),(-0.0253011842158085,-0.0126507472101198,
0.),.UNSPECIFIED.);
#21948=B_SPLINE_CURVE_WITH_KNOTS('',3,(#108697,#108698,#108699,#108700,
#108701,#108702),.UNSPECIFIED.,.F.,.F.,(4,2,4),(-0.0253011598820241,-0.0126507373294872,
0.),.UNSPECIFIED.);
#21949=B_SPLINE_CURVE_WITH_KNOTS('',3,(#108733,#108734,#108735,#108736,
#108737,#108738),.UNSPECIFIED.,.F.,.F.,(4,2,4),(-0.0253011788463282,-0.0126507450350469,
0.),.UNSPECIFIED.);
#21950=B_SPLINE_CURVE_WITH_KNOTS('',3,(#108769,#108770,#108771,#108772,
#108773,#108774),.UNSPECIFIED.,.F.,.F.,(4,2,4),(-0.0253011577904646,-0.0126507365079484,
0.),.UNSPECIFIED.);
#21951=B_SPLINE_CURVE_WITH_KNOTS('',3,(#108805,#108806,#108807,#108808,
#108809,#108810),.UNSPECIFIED.,.F.,.F.,(4,2,4),(-0.0253012250062976,-0.0126507412061137,
0.),.UNSPECIFIED.);
#21952=B_SPLINE_CURVE_WITH_KNOTS('',3,(#108841,#108842,#108843,#108844,
#108845,#108846),.UNSPECIFIED.,.F.,.F.,(4,2,4),(-0.0253011816847251,-0.0126507461326866,
0.),.UNSPECIFIED.);
#21953=B_SPLINE_CURVE_WITH_KNOTS('',3,(#108877,#108878,#108879,#108880,
#108881,#108882),.UNSPECIFIED.,.F.,.F.,(4,2,4),(-0.0253012223511792,-0.0126507403440478,
0.),.UNSPECIFIED.);
#21954=B_SPLINE_CURVE_WITH_KNOTS('',3,(#108913,#108914,#108915,#108916,
#108917,#108918),.UNSPECIFIED.,.F.,.F.,(4,2,4),(-0.0253016719835357,-0.0126509447160589,
0.),.UNSPECIFIED.);
#21955=B_SPLINE_CURVE_WITH_KNOTS('',3,(#108949,#108950,#108951,#108952,
#108953,#108954),.UNSPECIFIED.,.F.,.F.,(4,2,4),(-0.025301225482847,-0.0126507413694676,
0.),.UNSPECIFIED.);
#21956=B_SPLINE_CURVE_WITH_KNOTS('',3,(#108985,#108986,#108987,#108988,
#108989,#108990),.UNSPECIFIED.,.F.,.F.,(4,2,4),(-0.0253012382215821,-0.0126507466593568,
0.),.UNSPECIFIED.);
#21957=B_SPLINE_CURVE_WITH_KNOTS('',3,(#109021,#109022,#109023,#109024,
#109025,#109026),.UNSPECIFIED.,.F.,.F.,(4,2,4),(-0.0253011573204577,-0.012650736311468,
0.),.UNSPECIFIED.);
#21958=B_SPLINE_CURVE_WITH_KNOTS('',3,(#109057,#109058,#109059,#109060,
#109061,#109062),.UNSPECIFIED.,.F.,.F.,(4,2,4),(-0.0253012336000751,-0.0126507450371835,
0.),.UNSPECIFIED.);
#21959=B_SPLINE_CURVE_WITH_KNOTS('',3,(#109093,#109094,#109095,#109096,
#109097,#109098),.UNSPECIFIED.,.F.,.F.,(4,2,4),(-0.0253011662532075,-0.0126507399598049,
0.),.UNSPECIFIED.);
#21960=B_SPLINE_CURVE_WITH_KNOTS('',3,(#109126,#109127,#109128,#109129,
#109130,#109131),.UNSPECIFIED.,.F.,.F.,(4,2,4),(-0.0253012343126556,-0.0126507458318833,
-1.68951004922424E-9),.UNSPECIFIED.);
#21961=B_SPLINE_CURVE_WITH_KNOTS('',3,(#109156,#109157,#109158,#109159,
#109160,#109161),.UNSPECIFIED.,.F.,.F.,(4,2,4),(-0.0253011892711839,-0.0126507493052928,
0.),.UNSPECIFIED.);
#21962=B_SPLINE_CURVE_WITH_KNOTS('',3,(#109192,#109193,#109194,#109195,
#109196,#109197),.UNSPECIFIED.,.F.,.F.,(4,2,4),(-0.0253012396201875,-0.0126507472829344,
0.),.UNSPECIFIED.);
#21963=B_SPLINE_CURVE_WITH_KNOTS('',3,(#109228,#109229,#109230,#109231,
#109232,#109233),.UNSPECIFIED.,.F.,.F.,(4,2,4),(-0.0253011545055926,-0.0126507352075945,
0.),.UNSPECIFIED.);
#21964=B_SPLINE_CURVE_WITH_KNOTS('',3,(#109264,#109265,#109266,#109267,
#109268,#109269),.UNSPECIFIED.,.F.,.F.,(4,2,4),(-0.0253012183482151,-0.0126507384139842,
0.),.UNSPECIFIED.);
#21965=B_SPLINE_CURVE_WITH_KNOTS('',3,(#109300,#109301,#109302,#109303,
#109304,#109305),.UNSPECIFIED.,.F.,.F.,(4,2,4),(-0.0253011924401833,-0.012650750468979,
0.),.UNSPECIFIED.);
#21966=B_SPLINE_CURVE_WITH_KNOTS('',3,(#109336,#109337,#109338,#109339,
#109340,#109341),.UNSPECIFIED.,.F.,.F.,(4,2,4),(-0.025301227630379,-0.0126507422531963,
0.),.UNSPECIFIED.);
#21967=B_SPLINE_CURVE_WITH_KNOTS('',3,(#109372,#109373,#109374,#109375,
#109376,#109377),.UNSPECIFIED.,.F.,.F.,(4,2,4),(-0.0253012454181613,-0.0126507494057004,
0.),.UNSPECIFIED.);
#21968=B_SPLINE_CURVE_WITH_KNOTS('',3,(#109408,#109409,#109410,#109411,
#109412,#109413),.UNSPECIFIED.,.F.,.F.,(4,2,4),(-0.0253011792550513,-0.0126507451606773,
0.),.UNSPECIFIED.);
#21969=B_SPLINE_CURVE_WITH_KNOTS('',3,(#109444,#109445,#109446,#109447,
#109448,#109449),.UNSPECIFIED.,.F.,.F.,(4,2,4),(-0.025302199809708,-0.0126511583700983,
0.),.UNSPECIFIED.);
#21970=B_SPLINE_CURVE_WITH_KNOTS('',3,(#109481,#109482,#109483,#109484,
#109485,#109486),.UNSPECIFIED.,.F.,.F.,(4,2,4),(-0.0253011840298263,-0.0126507471467937,
0.),.UNSPECIFIED.);
#21971=B_SPLINE_CURVE_WITH_KNOTS('',3,(#109516,#109517,#109518,#109519,
#109520,#109521),.UNSPECIFIED.,.F.,.F.,(4,2,4),(-0.0253011859268071,-0.0126507478575772,
0.),.UNSPECIFIED.);
#21972=B_SPLINE_CURVE_WITH_KNOTS('',3,(#109552,#109553,#109554,#109555,
#109556,#109557),.UNSPECIFIED.,.F.,.F.,(4,2,4),(-0.025301169220318,-0.0126507411821087,
0.),.UNSPECIFIED.);
#21973=B_SPLINE_CURVE_WITH_KNOTS('',3,(#109588,#109589,#109590,#109591,
#109592,#109593),.UNSPECIFIED.,.F.,.F.,(4,2,4),(-0.0253012393925589,-0.0126507468711187,
0.),.UNSPECIFIED.);
#21974=B_SPLINE_CURVE_WITH_KNOTS('',3,(#109624,#109625,#109626,#109627,
#109628,#109629),.UNSPECIFIED.,.F.,.F.,(4,2,4),(-0.0253012437221507,-0.0126507489284059,
0.),.UNSPECIFIED.);
#21975=B_SPLINE_CURVE_WITH_KNOTS('',3,(#109657,#109658,#109659,#109660,
#109661,#109662),.UNSPECIFIED.,.F.,.F.,(4,2,4),(-0.0252968356990071,-0.0126485400410685,
0.),.UNSPECIFIED.);
#21976=B_SPLINE_CURVE_WITH_KNOTS('',3,(#109678,#109679,#109680,#109681,
#109682,#109683,#109684),.UNSPECIFIED.,.F.,.F.,(4,3,4),(0.285597313263199,
0.292504563548801,0.29778576616136),.UNSPECIFIED.);
#21977=B_SPLINE_CURVE_WITH_KNOTS('',3,(#109700,#109701,#109702,#109703,
#109704,#109705),.UNSPECIFIED.,.F.,.F.,(4,2,4),(-0.0252965361700464,-0.0126482848477994,
0.),.UNSPECIFIED.);
#21978=B_SPLINE_CURVE_WITH_KNOTS('',3,(#109721,#109722,#109723,#109724,
#109725,#109726,#109727),.UNSPECIFIED.,.F.,.F.,(4,3,4),(0.285597313263249,
0.292504563548819,0.297785766263882),.UNSPECIFIED.);
#21979=B_SPLINE_CURVE_WITH_KNOTS('',3,(#109743,#109744,#109745,#109746,
#109747,#109748),.UNSPECIFIED.,.F.,.F.,(4,2,4),(-0.0252968357524213,-0.0126485400643503,
0.),.UNSPECIFIED.);
#21980=B_SPLINE_CURVE_WITH_KNOTS('',3,(#109764,#109765,#109766,#109767,
#109768,#109769,#109770),.UNSPECIFIED.,.F.,.F.,(4,3,4),(0.285597313263242,
0.292504563548821,0.297785766263882),.UNSPECIFIED.);
#21981=B_SPLINE_CURVE_WITH_KNOTS('',3,(#109786,#109787,#109788,#109789,
#109790,#109791),.UNSPECIFIED.,.F.,.F.,(4,2,4),(-0.0252968357378529,-0.012648540059275,
0.),.UNSPECIFIED.);
#21982=B_SPLINE_CURVE_WITH_KNOTS('',3,(#109807,#109808,#109809,#109810,
#109811,#109812,#109813),.UNSPECIFIED.,.F.,.F.,(4,3,4),(0.285597313263251,
0.292504563548821,0.297785766263885),.UNSPECIFIED.);
#21983=B_SPLINE_CURVE_WITH_KNOTS('',3,(#109829,#109830,#109831,#109832,
#109833,#109834),.UNSPECIFIED.,.F.,.F.,(4,2,4),(-0.0252968357985692,-0.0126485400760452,
0.),.UNSPECIFIED.);
#21984=B_SPLINE_CURVE_WITH_KNOTS('',3,(#109850,#109851,#109852,#109853,
#109854,#109855,#109856),.UNSPECIFIED.,.F.,.F.,(4,3,4),(0.285597313263242,
0.292504563548821,0.297785766263878),.UNSPECIFIED.);
#21985=B_SPLINE_CURVE_WITH_KNOTS('',3,(#109872,#109873,#109874,#109875,
#109876,#109877),.UNSPECIFIED.,.F.,.F.,(4,2,4),(-0.0252968357636569,-0.012648540092616,
-1.44209019725672E-11),.UNSPECIFIED.);
#21986=B_SPLINE_CURVE_WITH_KNOTS('',3,(#109893,#109894,#109895,#109896,
#109897,#109898,#109899),.UNSPECIFIED.,.F.,.F.,(4,3,4),(0.285597313263247,
0.292504563548818,0.297785766263879),.UNSPECIFIED.);
#21987=B_SPLINE_CURVE_WITH_KNOTS('',3,(#109915,#109916,#109917,#109918,
#109919,#109920),.UNSPECIFIED.,.F.,.F.,(4,2,4),(-0.0252962100658619,-0.0126482866101926,
0.),.UNSPECIFIED.);
#21988=B_SPLINE_CURVE_WITH_KNOTS('',3,(#109936,#109937,#109938,#109939,
#109940,#109941,#109942),.UNSPECIFIED.,.F.,.F.,(4,3,4),(0.285597313263248,
0.292504563548819,0.297785766161452),.UNSPECIFIED.);
#21989=B_SPLINE_CURVE_WITH_KNOTS('',3,(#109958,#109959,#109960,#109961,
#109962,#109963),.UNSPECIFIED.,.F.,.F.,(4,2,4),(-0.0252968357810003,-0.012648540091324,
0.),.UNSPECIFIED.);
#21990=B_SPLINE_CURVE_WITH_KNOTS('',3,(#109979,#109980,#109981,#109982,
#109983,#109984,#109985),.UNSPECIFIED.,.F.,.F.,(4,3,4),(0.285597313263238,
0.292504563548819,0.297785766263878),.UNSPECIFIED.);
#21991=B_SPLINE_CURVE_WITH_KNOTS('',3,(#110001,#110002,#110003,#110004,
#110005,#110006),.UNSPECIFIED.,.F.,.F.,(4,2,4),(-0.0252968357048677,-0.0126485400491316,
0.),.UNSPECIFIED.);
#21992=B_SPLINE_CURVE_WITH_KNOTS('',3,(#110022,#110023,#110024,#110025,
#110026,#110027,#110028),.UNSPECIFIED.,.F.,.F.,(4,3,4),(0.285597313263247,
0.292504563548818,0.297785766263879),.UNSPECIFIED.);
#21993=B_SPLINE_CURVE_WITH_KNOTS('',3,(#110044,#110045,#110046,#110047,
#110048,#110049),.UNSPECIFIED.,.F.,.F.,(4,2,4),(-0.0252968357538185,-0.0126485400631416,
0.),.UNSPECIFIED.);
#21994=B_SPLINE_CURVE_WITH_KNOTS('',3,(#110065,#110066,#110067,#110068,
#110069,#110070,#110071),.UNSPECIFIED.,.F.,.F.,(4,3,4),(0.28559731326324,
0.292504563548819,0.297785766263876),.UNSPECIFIED.);
#21995=B_SPLINE_CURVE_WITH_KNOTS('',3,(#110087,#110088,#110089,#110090,
#110091,#110092),.UNSPECIFIED.,.F.,.F.,(4,2,4),(-0.02529683573446,-0.0126485400816567,
-1.60400685789153E-11),.UNSPECIFIED.);
#21996=B_SPLINE_CURVE_WITH_KNOTS('',3,(#110108,#110109,#110110,#110111,
#110112,#110113,#110114),.UNSPECIFIED.,.F.,.F.,(4,3,4),(0.285597313263248,
0.292504563548819,0.297785766263886),.UNSPECIFIED.);
#21997=B_SPLINE_CURVE_WITH_KNOTS('',3,(#110130,#110131,#110132,#110133,
#110134,#110135),.UNSPECIFIED.,.F.,.F.,(4,2,4),(-0.0252968357641617,-0.012648540066526,
0.),.UNSPECIFIED.);
#21998=B_SPLINE_CURVE_WITH_KNOTS('',3,(#110151,#110152,#110153,#110154,
#110155,#110156,#110157),.UNSPECIFIED.,.F.,.F.,(4,3,4),(0.28559731326324,
0.292504563548819,0.297785766263877),.UNSPECIFIED.);
#21999=B_SPLINE_CURVE_WITH_KNOTS('',3,(#110173,#110174,#110175,#110176,
#110177,#110178),.UNSPECIFIED.,.F.,.F.,(4,2,4),(-0.0252968357896558,-0.0126485400701538,
0.),.UNSPECIFIED.);
#22000=B_SPLINE_CURVE_WITH_KNOTS('',3,(#110194,#110195,#110196,#110197,
#110198,#110199,#110200),.UNSPECIFIED.,.F.,.F.,(4,3,4),(0.285597313263243,
0.292504563548818,0.297785766263875),.UNSPECIFIED.);
#22001=B_SPLINE_CURVE_WITH_KNOTS('',3,(#110216,#110217,#110218,#110219,
#110220,#110221),.UNSPECIFIED.,.F.,.F.,(4,2,4),(-0.0252962100515733,-0.0126482866018716,
0.),.UNSPECIFIED.);
#22002=B_SPLINE_CURVE_WITH_KNOTS('',3,(#110237,#110238,#110239,#110240,
#110241,#110242,#110243),.UNSPECIFIED.,.F.,.F.,(4,3,4),(0.285597313263226,
0.292504563548819,0.297785766161952),.UNSPECIFIED.);
#22003=B_SPLINE_CURVE_WITH_KNOTS('',3,(#110259,#110260,#110261,#110262,
#110263,#110264),.UNSPECIFIED.,.F.,.F.,(4,2,4),(-0.0252968357284577,-0.0126485400553069,
0.),.UNSPECIFIED.);
#22004=B_SPLINE_CURVE_WITH_KNOTS('',3,(#110280,#110281,#110282,#110283,
#110284,#110285,#110286),.UNSPECIFIED.,.F.,.F.,(4,3,4),(0.285597313263246,
0.292504563548817,0.297785766263879),.UNSPECIFIED.);
#22005=B_SPLINE_CURVE_WITH_KNOTS('',3,(#110302,#110303,#110304,#110305,
#110306,#110307),.UNSPECIFIED.,.F.,.F.,(4,2,4),(-0.0252968356959624,-0.0126485400460954,
0.),.UNSPECIFIED.);
#22006=B_SPLINE_CURVE_WITH_KNOTS('',3,(#110323,#110324,#110325,#110326,
#110327,#110328,#110329),.UNSPECIFIED.,.F.,.F.,(4,3,4),(0.285597313263248,
0.292504563548818,0.297785766162127),.UNSPECIFIED.);
#22007=B_SPLINE_CURVE_WITH_KNOTS('',3,(#110345,#110346,#110347,#110348,
#110349,#110350),.UNSPECIFIED.,.F.,.F.,(4,2,4),(-0.0252968357533458,-0.0126485400629371,
0.),.UNSPECIFIED.);
#22008=B_SPLINE_CURVE_WITH_KNOTS('',3,(#110366,#110367,#110368,#110369,
#110370,#110371,#110372),.UNSPECIFIED.,.F.,.F.,(4,3,4),(0.285597313263239,
0.292504563548819,0.297785766263876),.UNSPECIFIED.);
#22009=B_SPLINE_CURVE_WITH_KNOTS('',3,(#110388,#110389,#110390,#110391,
#110392,#110393),.UNSPECIFIED.,.F.,.F.,(4,2,4),(-0.0252968357468296,-0.0126485400548369,
0.),.UNSPECIFIED.);
#22010=B_SPLINE_CURVE_WITH_KNOTS('',3,(#110409,#110410,#110411,#110412,
#110413,#110414,#110415),.UNSPECIFIED.,.F.,.F.,(4,3,4),(0.28559731326325,
0.29250456354882,0.297785766263875),.UNSPECIFIED.);
#22011=B_SPLINE_CURVE_WITH_KNOTS('',3,(#110431,#110432,#110433,#110434,
#110435,#110436),.UNSPECIFIED.,.F.,.F.,(4,2,4),(-0.0252968357312852,-0.0126485401030248,
-1.36424656294043E-11),.UNSPECIFIED.);
#22012=B_SPLINE_CURVE_WITH_KNOTS('',3,(#110452,#110453,#110454,#110455,
#110456,#110457,#110458),.UNSPECIFIED.,.F.,.F.,(4,3,4),(0.285597313263231,
0.29250456354882,0.297785766263871),.UNSPECIFIED.);
#22013=B_SPLINE_CURVE_WITH_KNOTS('',3,(#110474,#110475,#110476,#110477,
#110478,#110479),.UNSPECIFIED.,.F.,.F.,(4,2,4),(-0.0252968357450572,-0.0126485400721381,
0.),.UNSPECIFIED.);
#22014=B_SPLINE_CURVE_WITH_KNOTS('',3,(#110495,#110496,#110497,#110498,
#110499,#110500,#110501),.UNSPECIFIED.,.F.,.F.,(4,3,4),(0.285597313263232,
0.292504563548818,0.297785766263874),.UNSPECIFIED.);
#22015=B_SPLINE_CURVE_WITH_KNOTS('',3,(#110517,#110518,#110519,#110520,
#110521,#110522),.UNSPECIFIED.,.F.,.F.,(4,2,4),(-0.0252968357143134,-0.0126485400567964,
-1.93689682348452E-11),.UNSPECIFIED.);
#22016=B_SPLINE_CURVE_WITH_KNOTS('',3,(#110538,#110539,#110540,#110541,
#110542,#110543,#110544),.UNSPECIFIED.,.F.,.F.,(4,3,4),(0.28559731326322,
0.292504563548818,0.297785766263867),.UNSPECIFIED.);
#22017=B_SPLINE_CURVE_WITH_KNOTS('',3,(#110560,#110561,#110562,#110563,
#110564,#110565),.UNSPECIFIED.,.F.,.F.,(4,2,4),(-0.0252968357957303,-0.0126485400617688,
0.),.UNSPECIFIED.);
#22018=B_SPLINE_CURVE_WITH_KNOTS('',3,(#110581,#110582,#110583,#110584,
#110585,#110586,#110587),.UNSPECIFIED.,.F.,.F.,(4,3,4),(0.285597313263247,
0.29250456354882,0.297785766162087),.UNSPECIFIED.);
#22019=B_SPLINE_CURVE_WITH_KNOTS('',3,(#110603,#110604,#110605,#110606,
#110607,#110608),.UNSPECIFIED.,.F.,.F.,(4,2,4),(-0.02529683571073,-0.0126485400556655,
0.),.UNSPECIFIED.);
#22020=B_SPLINE_CURVE_WITH_KNOTS('',3,(#110624,#110625,#110626,#110627,
#110628,#110629,#110630),.UNSPECIFIED.,.F.,.F.,(4,3,4),(0.285597313263225,
0.29250456354882,0.297785766161269),.UNSPECIFIED.);
#22021=B_SPLINE_CURVE_WITH_KNOTS('',3,(#110646,#110647,#110648,#110649,
#110650,#110651),.UNSPECIFIED.,.F.,.F.,(4,2,4),(-0.0252962192621954,-0.0126482903584362,
0.),.UNSPECIFIED.);
#22022=B_SPLINE_CURVE_WITH_KNOTS('',3,(#110667,#110668,#110669,#110670,
#110671,#110672,#110673),.UNSPECIFIED.,.F.,.F.,(4,3,4),(0.28559731326323,
0.29250456354882,0.297785766161143),.UNSPECIFIED.);
#22023=B_SPLINE_CURVE_WITH_KNOTS('',3,(#110689,#110690,#110691,#110692,
#110693,#110694),.UNSPECIFIED.,.F.,.F.,(4,2,4),(-0.0252968357981397,-0.0126485400435585,
0.),.UNSPECIFIED.);
#22024=B_SPLINE_CURVE_WITH_KNOTS('',3,(#110710,#110711,#110712,#110713,
#110714,#110715,#110716),.UNSPECIFIED.,.F.,.F.,(4,3,4),(0.285597313263077,
0.292504563548664,0.29778576626372),.UNSPECIFIED.);
#22025=B_SPLINE_CURVE_WITH_KNOTS('',3,(#110732,#110733,#110734,#110735,
#110736,#110737),.UNSPECIFIED.,.F.,.F.,(4,2,4),(-0.0252968358008816,-0.0126485400633527,
0.),.UNSPECIFIED.);
#22026=B_SPLINE_CURVE_WITH_KNOTS('',3,(#110753,#110754,#110755,#110756,
#110757,#110758,#110759),.UNSPECIFIED.,.F.,.F.,(4,3,4),(0.285597313263235,
0.29250456354882,0.297785766263876),.UNSPECIFIED.);
#22027=B_SPLINE_CURVE_WITH_KNOTS('',3,(#110775,#110776,#110777,#110778,
#110779,#110780),.UNSPECIFIED.,.F.,.F.,(4,2,4),(-0.0252965522558592,-0.0126482890945447,
0.),.UNSPECIFIED.);
#22028=B_SPLINE_CURVE_WITH_KNOTS('',3,(#110796,#110797,#110798,#110799,
#110800,#110801,#110802),.UNSPECIFIED.,.F.,.F.,(4,3,4),(0.285597313263115,
0.292504563548722,0.297785766263765),.UNSPECIFIED.);
#22029=B_SPLINE_CURVE_WITH_KNOTS('',3,(#110818,#110819,#110820,#110821,
#110822,#110823),.UNSPECIFIED.,.F.,.F.,(4,2,4),(-0.0252968358006324,-0.0126485401203243,
-1.55508869670307E-11),.UNSPECIFIED.);
#22030=B_SPLINE_CURVE_WITH_KNOTS('',3,(#110839,#110840,#110841,#110842,
#110843,#110844,#110845),.UNSPECIFIED.,.F.,.F.,(4,3,4),(0.28559731326323,
0.292504563548818,0.297785766263871),.UNSPECIFIED.);
#22031=B_SPLINE_CURVE_WITH_KNOTS('',3,(#110861,#110862,#110863,#110864,
#110865,#110866),.UNSPECIFIED.,.F.,.F.,(4,2,4),(-0.0252968357955371,-0.0126485400856769,
0.),.UNSPECIFIED.);
#22032=B_SPLINE_CURVE_WITH_KNOTS('',3,(#110882,#110883,#110884,#110885,
#110886,#110887,#110888),.UNSPECIFIED.,.F.,.F.,(4,3,4),(0.285597313263132,
0.292504563548721,0.297785766161844),.UNSPECIFIED.);
#22033=B_SPLINE_CURVE_WITH_KNOTS('',3,(#110906,#110907,#110908,#110909,
#110910,#110911),.UNSPECIFIED.,.F.,.F.,(4,2,4),(-0.0253021439456766,-0.0126510635839076,
0.),.UNSPECIFIED.);
#22034=B_SPLINE_CURVE_WITH_KNOTS('',3,(#110931,#110932,#110933,#110934,
#110935,#110936),.UNSPECIFIED.,.F.,.F.,(4,2,4),(-0.0253021899398336,-0.0126510747308192,
0.),.UNSPECIFIED.);
#22035=B_SPLINE_CURVE_WITH_KNOTS('',3,(#110956,#110957,#110958,#110959,
#110960,#110961),.UNSPECIFIED.,.F.,.F.,(4,2,4),(-0.0253021070217382,-0.0126510669277047,
0.),.UNSPECIFIED.);
#22036=B_SPLINE_CURVE_WITH_KNOTS('',3,(#110981,#110982,#110983,#110984,
#110985,#110986),.UNSPECIFIED.,.F.,.F.,(4,2,4),(-0.0253021927970414,-0.0126510754230541,
0.),.UNSPECIFIED.);
#22037=B_SPLINE_CURVE_WITH_KNOTS('',3,(#111006,#111007,#111008,#111009,
#111010,#111011),.UNSPECIFIED.,.F.,.F.,(4,2,4),(-0.0253022032712972,-0.0126510779593872,
0.),.UNSPECIFIED.);
#22038=B_SPLINE_CURVE_WITH_KNOTS('',3,(#111031,#111032,#111033,#111034,
#111035,#111036),.UNSPECIFIED.,.F.,.F.,(4,2,4),(-0.025302125896764,-0.0126510592235906,
0.),.UNSPECIFIED.);
#22039=B_SPLINE_CURVE_WITH_KNOTS('',3,(#111056,#111057,#111058,#111059,
#111060,#111061),.UNSPECIFIED.,.F.,.F.,(4,2,4),(-0.0253021609281757,-0.0126510677054464,
0.),.UNSPECIFIED.);
#22040=B_SPLINE_CURVE_WITH_KNOTS('',3,(#111081,#111082,#111083,#111084,
#111085,#111086),.UNSPECIFIED.,.F.,.F.,(4,2,4),(-0.025302142839597,-0.0126510754321364,
0.),.UNSPECIFIED.);
#22041=B_SPLINE_CURVE_WITH_KNOTS('',3,(#111106,#111107,#111108,#111109,
#111110,#111111),.UNSPECIFIED.,.F.,.F.,(4,2,4),(-0.0253020820197401,-0.0126510608438811,
0.),.UNSPECIFIED.);
#22042=B_SPLINE_CURVE_WITH_KNOTS('',3,(#111131,#111132,#111133,#111134,
#111135,#111136),.UNSPECIFIED.,.F.,.F.,(4,2,4),(-0.0253021871069684,-0.0126510740451975,
0.),.UNSPECIFIED.);
#22043=B_SPLINE_CURVE_WITH_KNOTS('',3,(#111156,#111157,#111158,#111159,
#111160,#111161),.UNSPECIFIED.,.F.,.F.,(4,2,4),(-0.025302149705,-0.0126510649876481,
0.),.UNSPECIFIED.);
#22044=B_SPLINE_CURVE_WITH_KNOTS('',3,(#111181,#111182,#111183,#111184,
#111185,#111186),.UNSPECIFIED.,.F.,.F.,(4,2,4),(-0.0253020798756929,-0.0126510600294986,
0.),.UNSPECIFIED.);
#22045=B_SPLINE_CURVE_WITH_KNOTS('',3,(#111206,#111207,#111208,#111209,
#111210,#111211),.UNSPECIFIED.,.F.,.F.,(4,2,4),(-0.0253020866229389,-0.0126510616784989,
0.),.UNSPECIFIED.);
#22046=B_SPLINE_CURVE_WITH_KNOTS('',3,(#111231,#111232,#111233,#111234,
#111235,#111236),.UNSPECIFIED.,.F.,.F.,(4,2,4),(-0.0253020878185704,-0.0126510619506973,
0.),.UNSPECIFIED.);
#22047=B_SPLINE_CURVE_WITH_KNOTS('',3,(#111256,#111257,#111258,#111259,
#111260,#111261),.UNSPECIFIED.,.F.,.F.,(4,2,4),(-0.0253022023503169,-0.0126510769560669,
0.),.UNSPECIFIED.);
#22048=B_SPLINE_CURVE_WITH_KNOTS('',3,(#111281,#111282,#111283,#111284,
#111285,#111286),.UNSPECIFIED.,.F.,.F.,(4,2,4),(-0.0253021184453625,-0.0126510574029242,
0.),.UNSPECIFIED.);
#22049=B_SPLINE_CURVE_WITH_KNOTS('',3,(#111306,#111307,#111308,#111309,
#111310,#111311),.UNSPECIFIED.,.F.,.F.,(4,2,4),(-0.0253021758358634,-0.012651071322494,
0.),.UNSPECIFIED.);
#22050=B_SPLINE_CURVE_WITH_KNOTS('',3,(#111331,#111332,#111333,#111334,
#111335,#111336),.UNSPECIFIED.,.F.,.F.,(4,2,4),(-0.0253020938917967,-0.0126510634950911,
0.),.UNSPECIFIED.);
#22051=B_SPLINE_CURVE_WITH_KNOTS('',3,(#111356,#111357,#111358,#111359,
#111360,#111361),.UNSPECIFIED.,.F.,.F.,(4,2,4),(-0.0253021022560184,-0.0126510654632121,
0.),.UNSPECIFIED.);
#22052=B_SPLINE_CURVE_WITH_KNOTS('',3,(#111381,#111382,#111383,#111384,
#111385,#111386),.UNSPECIFIED.,.F.,.F.,(4,2,4),(-0.0253021159724824,-0.0126510689880673,
0.),.UNSPECIFIED.);
#22053=B_SPLINE_CURVE_WITH_KNOTS('',3,(#111406,#111407,#111408,#111409,
#111410,#111411),.UNSPECIFIED.,.F.,.F.,(4,2,4),(-0.0253021883308794,-0.0126510743448658,
0.),.UNSPECIFIED.);
#22054=B_SPLINE_CURVE_WITH_KNOTS('',3,(#111431,#111432,#111433,#111434,
#111435,#111436),.UNSPECIFIED.,.F.,.F.,(4,2,4),(-0.0253021990250197,-0.0126510769120973,
0.),.UNSPECIFIED.);
#22055=B_SPLINE_CURVE_WITH_KNOTS('',3,(#111456,#111457,#111458,#111459,
#111460,#111461),.UNSPECIFIED.,.F.,.F.,(4,2,4),(-0.0253021158044732,-0.0126510687683093,
0.),.UNSPECIFIED.);
#22056=B_SPLINE_CURVE_WITH_KNOTS('',3,(#111481,#111482,#111483,#111484,
#111485,#111486),.UNSPECIFIED.,.F.,.F.,(4,2,4),(-0.0253021521740526,-0.0126510655702641,
0.),.UNSPECIFIED.);
#22057=B_SPLINE_CURVE_WITH_KNOTS('',3,(#111506,#111507,#111508,#111509,
#111510,#111511),.UNSPECIFIED.,.F.,.F.,(4,2,4),(-0.0253020706818732,-0.0126510582491332,
0.),.UNSPECIFIED.);
#22058=B_SPLINE_CURVE_WITH_KNOTS('',3,(#111531,#111532,#111533,#111534,
#111535,#111536),.UNSPECIFIED.,.F.,.F.,(4,2,4),(-0.0253021317551461,-0.0126510606484672,
0.),.UNSPECIFIED.);
#22059=B_SPLINE_CURVE_WITH_KNOTS('',3,(#111556,#111557,#111558,#111559,
#111560,#111561),.UNSPECIFIED.,.F.,.F.,(4,2,4),(-0.0253021549968402,-0.0126510662743969,
0.),.UNSPECIFIED.);
#22060=B_SPLINE_CURVE_WITH_KNOTS('',3,(#111581,#111582,#111583,#111584,
#111585,#111586),.UNSPECIFIED.,.F.,.F.,(4,2,4),(-0.025302121984863,-0.012651070596378,
0.),.UNSPECIFIED.);
#22061=B_SPLINE_CURVE_WITH_KNOTS('',3,(#111606,#111607,#111608,#111609,
#111610,#111611),.UNSPECIFIED.,.F.,.F.,(4,2,4),(-0.0253021247416108,-0.0126510589319846,
0.),.UNSPECIFIED.);
#22062=B_SPLINE_CURVE_WITH_KNOTS('',3,(#111627,#111628,#111629,#111630,
#111631,#111632),.UNSPECIFIED.,.F.,.F.,(4,2,4),(-0.0253038261819231,-0.0126517946770251,
0.),.UNSPECIFIED.);
#22063=B_SPLINE_CURVE_WITH_KNOTS('',3,(#111652,#111653,#111654,#111655,
#111656,#111657),.UNSPECIFIED.,.F.,.F.,(4,2,4),(-0.0253038261618308,-0.0126517946582728,
0.),.UNSPECIFIED.);
#22064=B_SPLINE_CURVE_WITH_KNOTS('',3,(#111677,#111678,#111679,#111680,
#111681,#111682),.UNSPECIFIED.,.F.,.F.,(4,2,4),(-0.0253038261636585,-0.0126517946628466,
0.),.UNSPECIFIED.);
#22065=B_SPLINE_CURVE_WITH_KNOTS('',3,(#111702,#111703,#111704,#111705,
#111706,#111707),.UNSPECIFIED.,.F.,.F.,(4,2,4),(-0.0253038261705201,-0.0126517946637361,
0.),.UNSPECIFIED.);
#22066=B_SPLINE_CURVE_WITH_KNOTS('',3,(#111727,#111728,#111729,#111730,
#111731,#111732),.UNSPECIFIED.,.F.,.F.,(4,2,4),(-0.0253038261771642,-0.0126517946734875,
0.),.UNSPECIFIED.);
#22067=B_SPLINE_CURVE_WITH_KNOTS('',3,(#111752,#111753,#111754,#111755,
#111756,#111757),.UNSPECIFIED.,.F.,.F.,(4,2,4),(-0.0253038261793075,-0.0126517946600724,
0.),.UNSPECIFIED.);
#22068=B_SPLINE_CURVE_WITH_KNOTS('',3,(#111777,#111778,#111779,#111780,
#111781,#111782),.UNSPECIFIED.,.F.,.F.,(4,2,4),(-0.0253038260537912,-0.0126517945966899,
0.),.UNSPECIFIED.);
#22069=B_SPLINE_CURVE_WITH_KNOTS('',3,(#111802,#111803,#111804,#111805,
#111806,#111807),.UNSPECIFIED.,.F.,.F.,(4,2,4),(-0.0253038260654538,-0.0126517945962593,
0.),.UNSPECIFIED.);
#22070=B_SPLINE_CURVE_WITH_KNOTS('',3,(#111827,#111828,#111829,#111830,
#111831,#111832),.UNSPECIFIED.,.F.,.F.,(4,2,4),(-0.0253038261582367,-0.0126517946456034,
0.),.UNSPECIFIED.);
#22071=B_SPLINE_CURVE_WITH_KNOTS('',3,(#111852,#111853,#111854,#111855,
#111856,#111857),.UNSPECIFIED.,.F.,.F.,(4,2,4),(-0.0253038261809024,-0.0126517946637246,
0.),.UNSPECIFIED.);
#22072=B_SPLINE_CURVE_WITH_KNOTS('',3,(#111877,#111878,#111879,#111880,
#111881,#111882),.UNSPECIFIED.,.F.,.F.,(4,2,4),(-0.0253038262366878,-0.012651794713052,
0.),.UNSPECIFIED.);
#22073=B_SPLINE_CURVE_WITH_KNOTS('',3,(#111902,#111903,#111904,#111905,
#111906,#111907),.UNSPECIFIED.,.F.,.F.,(4,2,4),(-0.0253038261934627,-0.0126517946811558,
0.),.UNSPECIFIED.);
#22074=B_SPLINE_CURVE_WITH_KNOTS('',3,(#111927,#111928,#111929,#111930,
#111931,#111932),.UNSPECIFIED.,.F.,.F.,(4,2,4),(-0.0253038261820815,-0.0126517946816107,
0.),.UNSPECIFIED.);
#22075=B_SPLINE_CURVE_WITH_KNOTS('',3,(#111952,#111953,#111954,#111955,
#111956,#111957),.UNSPECIFIED.,.F.,.F.,(4,2,4),(-0.0253038261910213,-0.0126517946722807,
0.),.UNSPECIFIED.);
#22076=B_SPLINE_CURVE_WITH_KNOTS('',3,(#111977,#111978,#111979,#111980,
#111981,#111982),.UNSPECIFIED.,.F.,.F.,(4,2,4),(-0.0253038261161507,-0.0126517946202027,
0.),.UNSPECIFIED.);
#22077=B_SPLINE_CURVE_WITH_KNOTS('',3,(#112002,#112003,#112004,#112005,
#112006,#112007),.UNSPECIFIED.,.F.,.F.,(4,2,4),(-0.0253038261824897,-0.0126517946767165,
0.),.UNSPECIFIED.);
#22078=B_SPLINE_CURVE_WITH_KNOTS('',3,(#112027,#112028,#112029,#112030,
#112031,#112032),.UNSPECIFIED.,.F.,.F.,(4,2,4),(-0.0253038261177518,-0.0126517946220728,
0.),.UNSPECIFIED.);
#22079=B_SPLINE_CURVE_WITH_KNOTS('',3,(#112052,#112053,#112054,#112055,
#112056,#112057),.UNSPECIFIED.,.F.,.F.,(4,2,4),(-0.0253038260398844,-0.012651794577381,
0.),.UNSPECIFIED.);
#22080=B_SPLINE_CURVE_WITH_KNOTS('',3,(#112077,#112078,#112079,#112080,
#112081,#112082),.UNSPECIFIED.,.F.,.F.,(4,2,4),(-0.0253038262042702,-0.0126517946823898,
0.),.UNSPECIFIED.);
#22081=B_SPLINE_CURVE_WITH_KNOTS('',3,(#112102,#112103,#112104,#112105,
#112106,#112107),.UNSPECIFIED.,.F.,.F.,(4,2,4),(-0.0253038261656433,-0.0126517946704612,
0.),.UNSPECIFIED.);
#22082=B_SPLINE_CURVE_WITH_KNOTS('',3,(#112127,#112128,#112129,#112130,
#112131,#112132),.UNSPECIFIED.,.F.,.F.,(4,2,4),(-0.0253038262116252,-0.0126517946724291,
0.),.UNSPECIFIED.);
#22083=B_SPLINE_CURVE_WITH_KNOTS('',3,(#112152,#112153,#112154,#112155,
#112156,#112157),.UNSPECIFIED.,.F.,.F.,(4,2,4),(-0.0253038260383867,-0.0126517945850157,
0.),.UNSPECIFIED.);
#22084=B_SPLINE_CURVE_WITH_KNOTS('',3,(#112177,#112178,#112179,#112180,
#112181,#112182),.UNSPECIFIED.,.F.,.F.,(4,2,4),(-0.0253038260350243,-0.0126517945880563,
0.),.UNSPECIFIED.);
#22085=B_SPLINE_CURVE_WITH_KNOTS('',3,(#112202,#112203,#112204,#112205,
#112206,#112207),.UNSPECIFIED.,.F.,.F.,(4,2,4),(-0.0253038261822948,-0.0126517946782481,
0.),.UNSPECIFIED.);
#22086=B_SPLINE_CURVE_WITH_KNOTS('',3,(#112227,#112228,#112229,#112230,
#112231,#112232),.UNSPECIFIED.,.F.,.F.,(4,2,4),(-0.0253038260539314,-0.0126517945868141,
0.),.UNSPECIFIED.);
#22087=B_SPLINE_CURVE_WITH_KNOTS('',3,(#112252,#112253,#112254,#112255,
#112256,#112257),.UNSPECIFIED.,.F.,.F.,(4,2,4),(-0.025303826121645,-0.0126517946312714,
0.),.UNSPECIFIED.);
#22088=B_SPLINE_CURVE_WITH_KNOTS('',3,(#112277,#112278,#112279,#112280,
#112281,#112282),.UNSPECIFIED.,.F.,.F.,(4,2,4),(-0.0253038261942185,-0.0126517946844356,
0.),.UNSPECIFIED.);
#22089=B_SPLINE_CURVE_WITH_KNOTS('',3,(#112302,#112303,#112304,#112305,
#112306,#112307),.UNSPECIFIED.,.F.,.F.,(4,2,4),(-0.025303826173704,-0.0126517946618426,
0.),.UNSPECIFIED.);
#22090=B_SPLINE_CURVE_WITH_KNOTS('',3,(#112327,#112328,#112329,#112330,
#112331,#112332),.UNSPECIFIED.,.F.,.F.,(4,2,4),(-0.0253038261369524,-0.0126517946406959,
0.),.UNSPECIFIED.);
#22091=B_SPLINE_CURVE_WITH_KNOTS('',3,(#112358,#112359,#112360,#112361,
#112362,#112363),.UNSPECIFIED.,.F.,.F.,(4,2,4),(-0.0253042779522863,-0.012652023863074,
-1.26281767681702E-9),.UNSPECIFIED.);
#22092=B_SPLINE_CURVE_WITH_KNOTS('',3,(#112377,#112378,#112379,#112380,
#112381,#112382),.UNSPECIFIED.,.F.,.F.,(4,2,4),(1.1700669172451E-9,0.0126520237688829,
0.0253042779723858),.UNSPECIFIED.);
#22093=B_SPLINE_CURVE_WITH_KNOTS('',3,(#112386,#112387,#112388,#112389,
#112390,#112391,#112392,#112393,#112394,#112395),.UNSPECIFIED.,.F.,.F.,
(4,3,3,4),(0.423693445112789,0.425620451530082,0.435349112748823,0.435879799328077),
 .UNSPECIFIED.);
#22094=B_SPLINE_CURVE_WITH_KNOTS('',3,(#112423,#112424,#112425,#112426,
#112427,#112428),.UNSPECIFIED.,.F.,.F.,(4,2,4),(1.15992411025749E-9,0.0126520237432614,
0.0253042712906343),.UNSPECIFIED.);
#22095=B_SPLINE_CURVE_WITH_KNOTS('',3,(#112432,#112433,#112434,#112435,
#112436,#112437,#112438,#112439,#112440,#112441),.UNSPECIFIED.,.F.,.F.,
(4,3,3,4),(0.423693445112179,0.425620451529627,0.435349127020628,0.435879799327622),
 .UNSPECIFIED.);
#22096=B_SPLINE_CURVE_WITH_KNOTS('',3,(#112469,#112470,#112471,#112472,
#112473,#112474),.UNSPECIFIED.,.F.,.F.,(4,2,4),(1.11407146647048E-9,0.0126520237062802,
0.0253042779618027),.UNSPECIFIED.);
#22097=B_SPLINE_CURVE_WITH_KNOTS('',3,(#112478,#112479,#112480,#112481,
#112482,#112483,#112484,#112485,#112486,#112487),.UNSPECIFIED.,.F.,.F.,
(4,3,3,4),(0.423693445112109,0.425620451530078,0.435349107778184,0.435879799328077),
 .UNSPECIFIED.);
#22098=B_SPLINE_CURVE_WITH_KNOTS('',3,(#112515,#112516,#112517,#112518,
#112519,#112520),.UNSPECIFIED.,.F.,.F.,(4,2,4),(1.18075426500004E-9,0.0126520237729946,
0.0253042779397471),.UNSPECIFIED.);
#22099=B_SPLINE_CURVE_WITH_KNOTS('',3,(#112524,#112525,#112526,#112527,
#112528,#112529,#112530,#112531,#112532,#112533),.UNSPECIFIED.,.F.,.F.,
(4,3,3,4),(0.423693445111464,0.42562045153008,0.43534911319926,0.435879799328077),
 .UNSPECIFIED.);
#22100=B_SPLINE_CURVE_WITH_KNOTS('',3,(#112561,#112562,#112563,#112564,
#112565,#112566),.UNSPECIFIED.,.F.,.F.,(4,2,4),(1.16849614942433E-9,0.0126520237539986,
0.0253042779543373),.UNSPECIFIED.);
#22101=B_SPLINE_CURVE_WITH_KNOTS('',3,(#112570,#112571,#112572,#112573,
#112574,#112575,#112576,#112577,#112578,#112579),.UNSPECIFIED.,.F.,.F.,
(4,3,3,4),(0.423693445106931,0.425620451530083,0.435349096540701,0.435879799328077),
 .UNSPECIFIED.);
#22102=B_SPLINE_CURVE_WITH_KNOTS('',3,(#112607,#112608,#112609,#112610,
#112611,#112612),.UNSPECIFIED.,.F.,.F.,(4,2,4),(1.16282290389696E-9,0.0126520237489755,
0.0253042779541902),.UNSPECIFIED.);
#22103=B_SPLINE_CURVE_WITH_KNOTS('',3,(#112616,#112617,#112618,#112619,
#112620,#112621,#112622,#112623,#112624,#112625),.UNSPECIFIED.,.F.,.F.,
(4,3,3,4),(0.423693445111984,0.425620451530082,0.43534912265206,0.435879799328077),
 .UNSPECIFIED.);
#22104=B_SPLINE_CURVE_WITH_KNOTS('',3,(#112650,#112651,#112652,#112653,
#112654,#112655),.UNSPECIFIED.,.F.,.F.,(4,2,4),(1.18800802144311E-9,0.0126520237832224,
0.025304277956622),.UNSPECIFIED.);
#22105=B_SPLINE_CURVE_WITH_KNOTS('',3,(#112681,#112682,#112683,#112684,
#112685,#112686),.UNSPECIFIED.,.F.,.F.,(4,2,4),(1.2101211537022E-9,0.0126520238473612,
0.0253042780494095),.UNSPECIFIED.);
#22106=B_SPLINE_CURVE_WITH_KNOTS('',3,(#112690,#112691,#112692,#112693,
#112694,#112695,#112696,#112697,#112698,#112699),.UNSPECIFIED.,.F.,.F.,
(4,3,3,4),(0.423693445109638,0.425620451530082,0.435349112840729,0.435879799328077),
 .UNSPECIFIED.);
#22107=B_SPLINE_CURVE_WITH_KNOTS('',3,(#112727,#112728,#112729,#112730,
#112731,#112732),.UNSPECIFIED.,.F.,.F.,(4,2,4),(1.22235445067349E-9,0.0126520238432788,
0.0253042779912354),.UNSPECIFIED.);
#22108=B_SPLINE_CURVE_WITH_KNOTS('',3,(#112736,#112737,#112738,#112739,
#112740,#112741,#112742,#112743,#112744,#112745),.UNSPECIFIED.,.F.,.F.,
(4,3,3,4),(0.423693445113625,0.425620451530082,0.435349157516574,0.435879799328077),
 .UNSPECIFIED.);
#22109=B_SPLINE_CURVE_WITH_KNOTS('',3,(#112773,#112774,#112775,#112776,
#112777,#112778),.UNSPECIFIED.,.F.,.F.,(4,2,4),(1.17023127225093E-9,0.0126520237785776,
0.0253042779737898),.UNSPECIFIED.);
#22110=B_SPLINE_CURVE_WITH_KNOTS('',3,(#112782,#112783,#112784,#112785,
#112786,#112787,#112788,#112789,#112790,#112791),.UNSPECIFIED.,.F.,.F.,
(4,3,3,4),(0.423693445113355,0.425620451530082,0.435349129767105,0.435879799328077),
 .UNSPECIFIED.);
#22111=B_SPLINE_CURVE_WITH_KNOTS('',3,(#112819,#112820,#112821,#112822,
#112823,#112824),.UNSPECIFIED.,.F.,.F.,(4,2,4),(1.28536851121112E-9,0.0126520239134261,
0.0253042780053408),.UNSPECIFIED.);
#22112=B_SPLINE_CURVE_WITH_KNOTS('',3,(#112828,#112829,#112830,#112831,
#112832,#112833,#112834,#112835,#112836,#112837),.UNSPECIFIED.,.F.,.F.,
(4,3,3,4),(0.423693445111432,0.425620451530082,0.435349117131884,0.435879799328077),
 .UNSPECIFIED.);
#22113=B_SPLINE_CURVE_WITH_KNOTS('',3,(#112865,#112866,#112867,#112868,
#112869,#112870),.UNSPECIFIED.,.F.,.F.,(4,2,4),(1.17556302170415E-9,0.0126520237584382,
0.0253042779055835),.UNSPECIFIED.);
#22114=B_SPLINE_CURVE_WITH_KNOTS('',3,(#112874,#112875,#112876,#112877,
#112878,#112879,#112880,#112881,#112882,#112883),.UNSPECIFIED.,.F.,.F.,
(4,3,3,4),(0.423693445111161,0.425620451530082,0.435349124551651,0.435879799328077),
 .UNSPECIFIED.);
#22115=B_SPLINE_CURVE_WITH_KNOTS('',3,(#112911,#112912,#112913,#112914,
#112915,#112916),.UNSPECIFIED.,.F.,.F.,(4,2,4),(1.22626055802122E-9,0.0126520238411188,
0.0253042779960663),.UNSPECIFIED.);
#22116=B_SPLINE_CURVE_WITH_KNOTS('',3,(#112920,#112921,#112922,#112923,
#112924,#112925,#112926,#112927,#112928,#112929),.UNSPECIFIED.,.F.,.F.,
(4,3,3,4),(0.423693445108059,0.425620451530082,0.435349094660655,0.435879799328077),
 .UNSPECIFIED.);
#22117=B_SPLINE_CURVE_WITH_KNOTS('',3,(#112957,#112958,#112959,#112960,
#112961,#112962),.UNSPECIFIED.,.F.,.F.,(4,2,4),(1.106444852458E-9,0.0126520237073674,
0.0253042779997113),.UNSPECIFIED.);
#22118=B_SPLINE_CURVE_WITH_KNOTS('',3,(#112966,#112967,#112968,#112969,
#112970,#112971,#112972,#112973,#112974,#112975),.UNSPECIFIED.,.F.,.F.,
(4,3,3,4),(0.42369344511326,0.425620451530082,0.43534910544585,0.435879799328077),
 .UNSPECIFIED.);
#22119=B_SPLINE_CURVE_WITH_KNOTS('',3,(#113003,#113004,#113005,#113006,
#113007,#113008),.UNSPECIFIED.,.F.,.F.,(4,2,4),(1.27267692598761E-9,0.012652023900116,
0.025304278035874),.UNSPECIFIED.);
#22120=B_SPLINE_CURVE_WITH_KNOTS('',3,(#113012,#113013,#113014,#113015,
#113016,#113017,#113018,#113019,#113020,#113021),.UNSPECIFIED.,.F.,.F.,
(4,3,3,4),(0.423693445114586,0.425620451530082,0.435349109594699,0.435879799328077),
 .UNSPECIFIED.);
#22121=B_SPLINE_CURVE_WITH_KNOTS('',3,(#113049,#113050,#113051,#113052,
#113053,#113054),.UNSPECIFIED.,.F.,.F.,(4,2,4),(1.23842331568108E-9,0.0126520238471676,
0.0253042779962425),.UNSPECIFIED.);
#22122=B_SPLINE_CURVE_WITH_KNOTS('',3,(#113058,#113059,#113060,#113061,
#113062,#113063,#113064,#113065,#113066,#113067),.UNSPECIFIED.,.F.,.F.,
(4,3,3,4),(0.423693445111866,0.425620451530082,0.435349102000603,0.435879799328077),
 .UNSPECIFIED.);
#22123=B_SPLINE_CURVE_WITH_KNOTS('',3,(#113095,#113096,#113097,#113098,
#113099,#113100),.UNSPECIFIED.,.F.,.F.,(4,2,4),(1.15725186408572E-9,0.0126520237695305,
0.0253042712996014),.UNSPECIFIED.);
#22124=B_SPLINE_CURVE_WITH_KNOTS('',3,(#113104,#113105,#113106,#113107,
#113108,#113109,#113110,#113111,#113112,#113113),.UNSPECIFIED.,.F.,.F.,
(4,3,3,4),(0.423693445111451,0.425620451530082,0.435349090690307,0.435879799328077),
 .UNSPECIFIED.);
#22125=B_SPLINE_CURVE_WITH_KNOTS('',3,(#113141,#113142,#113143,#113144,
#113145,#113146),.UNSPECIFIED.,.F.,.F.,(4,2,4),(1.14185159363066E-9,0.0126520237378726,
0.0253042715112374),.UNSPECIFIED.);
#22126=B_SPLINE_CURVE_WITH_KNOTS('',3,(#113150,#113151,#113152,#113153,
#113154,#113155,#113156,#113157,#113158,#113159),.UNSPECIFIED.,.F.,.F.,
(4,3,3,4),(0.423693445113878,0.425620451530082,0.435349119213872,0.435879799328077),
 .UNSPECIFIED.);
#22127=B_SPLINE_CURVE_WITH_KNOTS('',3,(#113187,#113188,#113189,#113190,
#113191,#113192),.UNSPECIFIED.,.F.,.F.,(4,2,4),(1.16461691057117E-9,0.0126520237709924,
0.0253042713679864),.UNSPECIFIED.);
#22128=B_SPLINE_CURVE_WITH_KNOTS('',3,(#113196,#113197,#113198,#113199,
#113200,#113201,#113202,#113203,#113204,#113205),.UNSPECIFIED.,.F.,.F.,
(4,3,3,4),(0.423693445112217,0.425620451530082,0.435349133653143,0.435879799328077),
 .UNSPECIFIED.);
#22129=B_SPLINE_CURVE_WITH_KNOTS('',3,(#113233,#113234,#113235,#113236,
#113237,#113238),.UNSPECIFIED.,.F.,.F.,(4,2,4),(1.19393976681407E-9,0.012652023807887,
0.025304277979508),.UNSPECIFIED.);
#22130=B_SPLINE_CURVE_WITH_KNOTS('',3,(#113242,#113243,#113244,#113245,
#113246,#113247,#113248,#113249,#113250,#113251),.UNSPECIFIED.,.F.,.F.,
(4,3,3,4),(0.423693445114459,0.425620451530082,0.435349141726896,0.435879799328077),
 .UNSPECIFIED.);
#22131=B_SPLINE_CURVE_WITH_KNOTS('',3,(#113279,#113280,#113281,#113282,
#113283,#113284),.UNSPECIFIED.,.F.,.F.,(4,2,4),(1.18834254830485E-9,0.0126520238105013,
0.0253042780047543),.UNSPECIFIED.);
#22132=B_SPLINE_CURVE_WITH_KNOTS('',3,(#113288,#113289,#113290,#113291,
#113292,#113293,#113294,#113295,#113296,#113297),.UNSPECIFIED.,.F.,.F.,
(4,3,3,4),(0.42369344511739,0.425620451530082,0.435349104601121,0.435879799328077),
 .UNSPECIFIED.);
#22133=B_SPLINE_CURVE_WITH_KNOTS('',3,(#113325,#113326,#113327,#113328,
#113329,#113330),.UNSPECIFIED.,.F.,.F.,(4,2,4),(1.16347538958191E-9,0.0126520237493745,
0.0253042779226141),.UNSPECIFIED.);
#22134=B_SPLINE_CURVE_WITH_KNOTS('',3,(#113334,#113335,#113336,#113337,
#113338,#113339,#113340,#113341,#113342,#113343),.UNSPECIFIED.,.F.,.F.,
(4,3,3,4),(0.42369344511639,0.425620451530082,0.435349124373817,0.435879799328077),
 .UNSPECIFIED.);
#22135=B_SPLINE_CURVE_WITH_KNOTS('',3,(#113371,#113372,#113373,#113374,
#113375,#113376),.UNSPECIFIED.,.F.,.F.,(4,2,4),(1.19336501661349E-9,0.0126520238269788,
0.0253042780057151),.UNSPECIFIED.);
#22136=B_SPLINE_CURVE_WITH_KNOTS('',3,(#113393,#113394,#113395,#113396,
#113397,#113398,#113399,#113400,#113401,#113402),.UNSPECIFIED.,.F.,.F.,
(4,3,3,4),(0.423693445110999,0.425620451530082,0.435349097348392,0.435879799328077),
 .UNSPECIFIED.);
#22137=B_SPLINE_CURVE_WITH_KNOTS('',3,(#113418,#113419,#113420,#113421,
#113422,#113423),.UNSPECIFIED.,.F.,.F.,(4,2,4),(1.2375369201656E-9,0.0126520238657896,
0.0253042779874803),.UNSPECIFIED.);
#22138=B_SPLINE_CURVE_WITH_KNOTS('',3,(#113428,#113429,#113430,#113431,
#113432,#113433,#113434,#113435,#113436,#113437),.UNSPECIFIED.,.F.,.F.,
(4,3,3,4),(0.423693445114954,0.425620451530081,0.435349115952807,0.435879799328076),
 .UNSPECIFIED.);
#22139=B_SPLINE_CURVE_WITH_KNOTS('',3,(#113463,#113464,#113465,#113466,
#113467,#113468),.UNSPECIFIED.,.F.,.F.,(4,2,4),(1.20901278985797E-9,0.012652023824525,
0.0253042780280582),.UNSPECIFIED.);
#22140=B_SPLINE_CURVE_WITH_KNOTS('',3,(#113472,#113473,#113474,#113475,
#113476,#113477,#113478,#113479,#113480,#113481),.UNSPECIFIED.,.F.,.F.,
(4,3,3,4),(0.423693445116275,0.42562045153008,0.435349117168475,0.435879799328076),
 .UNSPECIFIED.);
#22141=B_SPLINE_CURVE_WITH_KNOTS('',3,(#113509,#113510,#113511,#113512,
#113513,#113514),.UNSPECIFIED.,.F.,.F.,(4,2,4),(1.17875583662026E-9,0.0126520237881625,
0.0253042780043191),.UNSPECIFIED.);
#22142=B_SPLINE_CURVE_WITH_KNOTS('',3,(#113518,#113519,#113520,#113521,
#113522,#113523,#113524,#113525,#113526,#113527),.UNSPECIFIED.,.F.,.F.,
(4,3,3,4),(0.423693445111073,0.425620451530046,0.43534911295555,0.435879799328042),
 .UNSPECIFIED.);
#22143=B_SPLINE_CURVE_WITH_KNOTS('',3,(#113555,#113556,#113557,#113558,
#113559,#113560),.UNSPECIFIED.,.F.,.F.,(4,2,4),(1.20261278446102E-9,0.0126520238272278,
0.0253042779650853),.UNSPECIFIED.);
#22144=B_SPLINE_CURVE_WITH_KNOTS('',3,(#113564,#113565,#113566,#113567,
#113568,#113569,#113570,#113571,#113572,#113573),.UNSPECIFIED.,.F.,.F.,
(4,3,3,4),(0.423693445111824,0.425620451530081,0.43534910285596,0.435879799328077),
 .UNSPECIFIED.);
#22145=B_SPLINE_CURVE_WITH_KNOTS('',3,(#113601,#113602,#113603,#113604,
#113605,#113606),.UNSPECIFIED.,.F.,.F.,(4,2,4),(1.20880002326826E-9,0.0126520238377698,
0.0253042780378564),.UNSPECIFIED.);
#22146=B_SPLINE_CURVE_WITH_KNOTS('',3,(#113610,#113611,#113612,#113613,
#113614,#113615,#113616,#113617,#113618,#113619),.UNSPECIFIED.,.F.,.F.,
(4,3,3,4),(0.42369344511094,0.425620451530084,0.435349107308875,0.435879799328079),
 .UNSPECIFIED.);
#22147=B_SPLINE_CURVE_WITH_KNOTS('',3,(#113637,#113638,#113639,#113640,
#113641,#113642,#113643,#113644,#113645,#113646),.UNSPECIFIED.,.F.,.F.,
(4,3,3,4),(0.423693445114842,0.425620451530082,0.43534908570091,0.435879799328077),
 .UNSPECIFIED.);
#22148=B_SPLINE_CURVE_WITH_KNOTS('',3,(#113674,#113675,#113676,#113677,
#113678,#113679),.UNSPECIFIED.,.F.,.F.,(4,2,4),(-0.0253007225797769,-0.0126503093936141,
0.),.UNSPECIFIED.);
#22149=B_SPLINE_CURVE_WITH_KNOTS('',3,(#113690,#113691,#113692,#113693,
#113694,#113695),.UNSPECIFIED.,.F.,.F.,(4,2,4),(5.88572981754996E-11,0.012650362637997,
0.0253009421921536),.UNSPECIFIED.);
#22150=B_SPLINE_CURVE_WITH_KNOTS('',3,(#113723,#113724,#113725,#113726,
#113727,#113728),.UNSPECIFIED.,.F.,.F.,(4,2,4),(6.4603455012057E-13,0.012650362567377,
0.0253009421633366),.UNSPECIFIED.);
#22151=B_SPLINE_CURVE_WITH_KNOTS('',3,(#113756,#113757,#113758,#113759,
#113760,#113761),.UNSPECIFIED.,.F.,.F.,(4,2,4),(2.71656584680603E-11,0.0126503625947692,
0.0253009421778162),.UNSPECIFIED.);
#22152=B_SPLINE_CURVE_WITH_KNOTS('',3,(#113789,#113790,#113791,#113792,
#113793,#113794),.UNSPECIFIED.,.F.,.F.,(4,2,4),(1.56002353552081E-11,0.012650362595027,
0.0253009422056366),.UNSPECIFIED.);
#22153=B_SPLINE_CURVE_WITH_KNOTS('',3,(#113822,#113823,#113824,#113825,
#113826,#113827),.UNSPECIFIED.,.F.,.F.,(4,2,4),(1.07002170564841E-11,0.012650362575683,
0.0253009421765229),.UNSPECIFIED.);
#22154=B_SPLINE_CURVE_WITH_KNOTS('',3,(#113855,#113856,#113857,#113858,
#113859,#113860),.UNSPECIFIED.,.F.,.F.,(4,2,4),(2.95270400716744E-11,0.0126503626042908,
0.0253009421738308),.UNSPECIFIED.);
#22155=B_SPLINE_CURVE_WITH_KNOTS('',3,(#113888,#113889,#113890,#113891,
#113892,#113893),.UNSPECIFIED.,.F.,.F.,(4,2,4),(5.34197508784737E-11,0.0126503626330273,
0.0253009421896363),.UNSPECIFIED.);
#22156=B_SPLINE_CURVE_WITH_KNOTS('',3,(#113921,#113922,#113923,#113924,
#113925,#113926),.UNSPECIFIED.,.F.,.F.,(4,2,4),(0.,0.0126503625628352,0.025300942169246),
 .UNSPECIFIED.);
#22157=B_SPLINE_CURVE_WITH_KNOTS('',3,(#113954,#113955,#113956,#113957,
#113958,#113959),.UNSPECIFIED.,.F.,.F.,(4,2,4),(0.,0.0126502910580625,0.0253006468831475),
 .UNSPECIFIED.);
#22158=B_SPLINE_CURVE_WITH_KNOTS('',3,(#113987,#113988,#113989,#113990,
#113991,#113992),.UNSPECIFIED.,.F.,.F.,(4,2,4),(1.51033193667582E-11,0.0126502983372392,
0.0253006769133421),.UNSPECIFIED.);
#22159=B_SPLINE_CURVE_WITH_KNOTS('',3,(#114020,#114021,#114022,#114023,
#114024,#114025),.UNSPECIFIED.,.F.,.F.,(4,2,4),(5.56132844431405E-11,0.0126503626325985,
0.0253009421779566),.UNSPECIFIED.);
#22160=B_SPLINE_CURVE_WITH_KNOTS('',3,(#114053,#114054,#114055,#114056,
#114057,#114058),.UNSPECIFIED.,.F.,.F.,(4,2,4),(6.25195221049412E-12,0.0126503625909652,
0.0253009421864759),.UNSPECIFIED.);
#22161=B_SPLINE_CURVE_WITH_KNOTS('',3,(#114086,#114087,#114088,#114089,
#114090,#114091),.UNSPECIFIED.,.F.,.F.,(4,2,4),(0.,0.0126503625566611,0.0253009421443978),
 .UNSPECIFIED.);
#22162=B_SPLINE_CURVE_WITH_KNOTS('',3,(#114116,#114117,#114118,#114119,
#114120,#114121),.UNSPECIFIED.,.F.,.F.,(4,2,4),(0.,0.0126503625643437,0.0253009421646361),
 .UNSPECIFIED.);
#22163=B_SPLINE_CURVE_WITH_KNOTS('',3,(#114143,#114144,#114145,#114146,
#114147,#114148),.UNSPECIFIED.,.F.,.F.,(4,2,4),(0.,0.0126502899166928,0.0253006421576979),
 .UNSPECIFIED.);
#22164=B_SPLINE_CURVE_WITH_KNOTS('',3,(#114176,#114177,#114178,#114179,
#114180,#114181),.UNSPECIFIED.,.F.,.F.,(4,2,4),(0.,0.0126503625623808,0.0253009421582833),
 .UNSPECIFIED.);
#22165=B_SPLINE_CURVE_WITH_KNOTS('',3,(#114209,#114210,#114211,#114212,
#114213,#114214),.UNSPECIFIED.,.F.,.F.,(4,2,4),(0.,0.0126502911500827,0.0253006472795662),
 .UNSPECIFIED.);
#22166=B_SPLINE_CURVE_WITH_KNOTS('',3,(#114242,#114243,#114244,#114245,
#114246,#114247),.UNSPECIFIED.,.F.,.F.,(4,2,4),(0.,0.0126502936779606,0.0253006577235599),
 .UNSPECIFIED.);
#22167=B_SPLINE_CURVE_WITH_KNOTS('',3,(#114275,#114276,#114277,#114278,
#114279,#114280),.UNSPECIFIED.,.F.,.F.,(4,2,4),(0.,0.012650287926731,0.0253006339425118),
 .UNSPECIFIED.);
#22168=B_SPLINE_CURVE_WITH_KNOTS('',3,(#114308,#114309,#114310,#114311,
#114312,#114313),.UNSPECIFIED.,.F.,.F.,(4,2,4),(0.,0.0126502886773374,0.025300637020662),
 .UNSPECIFIED.);
#22169=B_SPLINE_CURVE_WITH_KNOTS('',3,(#114341,#114342,#114343,#114344,
#114345,#114346),.UNSPECIFIED.,.F.,.F.,(4,2,4),(1.44578481018274E-11,0.01265029636312,
0.0253006688299366),.UNSPECIFIED.);
#22170=B_SPLINE_CURVE_WITH_KNOTS('',3,(#114374,#114375,#114376,#114377,
#114378,#114379),.UNSPECIFIED.,.F.,.F.,(4,2,4),(5.41752395831836E-11,0.0126503626593091,
0.0253009422415678),.UNSPECIFIED.);
#22171=B_SPLINE_CURVE_WITH_KNOTS('',3,(#114407,#114408,#114409,#114410,
#114411,#114412),.UNSPECIFIED.,.F.,.F.,(4,2,4),(3.09190381982686E-11,0.0126503626247606,
0.0253009422203617),.UNSPECIFIED.);
#22172=B_SPLINE_CURVE_WITH_KNOTS('',3,(#114440,#114441,#114442,#114443,
#114444,#114445),.UNSPECIFIED.,.F.,.F.,(4,2,4),(9.36296347676373E-11,0.0126503626925452,
0.0253009422282069),.UNSPECIFIED.);
#22173=B_SPLINE_CURVE_WITH_KNOTS('',3,(#114473,#114474,#114475,#114476,
#114477,#114478),.UNSPECIFIED.,.F.,.F.,(4,2,4),(7.07874032726965E-11,0.0126503626643126,
0.0253009422144023),.UNSPECIFIED.);
#22174=B_SPLINE_CURVE_WITH_KNOTS('',3,(#114506,#114507,#114508,#114509,
#114510,#114511),.UNSPECIFIED.,.F.,.F.,(4,2,4),(2.09563593890109E-11,0.0126503626199398,
0.025300942218264),.UNSPECIFIED.);
#22175=B_SPLINE_CURVE_WITH_KNOTS('',3,(#114539,#114540,#114541,#114542,
#114543,#114544),.UNSPECIFIED.,.F.,.F.,(4,2,4),(5.43237340880536E-11,0.0126503626330034,
0.0253009421773611),.UNSPECIFIED.);
#22176=B_SPLINE_CURVE_WITH_KNOTS('',3,(#114572,#114573,#114574,#114575,
#114576,#114577),.UNSPECIFIED.,.F.,.F.,(4,2,4),(0.,0.0126502912747948,0.0253006477804102),
 .UNSPECIFIED.);
#22177=B_SPLINE_CURVE_WITH_KNOTS('',3,(#114616,#114617,#114618,#114619,
#114620,#114621),.UNSPECIFIED.,.F.,.F.,(4,2,4),(-0.0252968045231955,-0.0126485258141896,
-2.22512321068624E-11),.UNSPECIFIED.);
#22178=B_SPLINE_CURVE_WITH_KNOTS('',3,(#114633,#114634,#114635,#114636,
#114637,#114638,#114639),.UNSPECIFIED.,.F.,.F.,(4,3,4),(0.41838298048767,
0.425586573424719,0.435845921192635),.UNSPECIFIED.);
#22179=B_SPLINE_CURVE_WITH_KNOTS('',3,(#114640,#114641,#114642,#114643,
#114644,#114645),.UNSPECIFIED.,.F.,.F.,(4,2,4),(4.66294882059351E-11,0.0126485259138885,
0.0252970983760051),.UNSPECIFIED.);
#22180=B_SPLINE_CURVE_WITH_KNOTS('',3,(#114664,#114665,#114666,#114667,
#114668,#114669,#114670),.UNSPECIFIED.,.F.,.F.,(4,3,4),(0.418382980503281,
0.425586573427989,0.435845921181019),.UNSPECIFIED.);
#22181=B_SPLINE_CURVE_WITH_KNOTS('',3,(#114671,#114672,#114673,#114674,
#114675,#114676),.UNSPECIFIED.,.F.,.F.,(4,2,4),(7.11845429795811E-11,0.0126485259324948,
0.0252971191976161),.UNSPECIFIED.);
#22182=B_SPLINE_CURVE_WITH_KNOTS('',3,(#114695,#114696,#114697,#114698,
#114699,#114700,#114701),.UNSPECIFIED.,.F.,.F.,(4,3,4),(0.418382980491422,
0.425586573424719,0.435845921184262),.UNSPECIFIED.);
#22183=B_SPLINE_CURVE_WITH_KNOTS('',3,(#114702,#114703,#114704,#114705,
#114706,#114707),.UNSPECIFIED.,.F.,.F.,(4,2,4),(2.24980277352272E-11,0.0126485258472688,
0.0252968045308311),.UNSPECIFIED.);
#22184=B_SPLINE_CURVE_WITH_KNOTS('',3,(#114726,#114727,#114728,#114729,
#114730,#114731,#114732),.UNSPECIFIED.,.F.,.F.,(4,3,4),(0.418382980513766,
0.425586573424719,0.435845921185484),.UNSPECIFIED.);
#22185=B_SPLINE_CURVE_WITH_KNOTS('',3,(#114733,#114734,#114735,#114736,
#114737,#114738),.UNSPECIFIED.,.F.,.F.,(4,2,4),(0.,0.0126485258164944,0.0252971009464653),
 .UNSPECIFIED.);
#22186=B_SPLINE_CURVE_WITH_KNOTS('',3,(#114757,#114758,#114759,#114760,
#114761,#114762,#114763),.UNSPECIFIED.,.F.,.F.,(4,3,4),(0.41838298049633,
0.42558657342472,0.435845921201898),.UNSPECIFIED.);
#22187=B_SPLINE_CURVE_WITH_KNOTS('',3,(#114764,#114765,#114766,#114767,
#114768,#114769),.UNSPECIFIED.,.F.,.F.,(4,2,4),(0.,0.0126485258144204,0.0252971006606839),
 .UNSPECIFIED.);
#22188=B_SPLINE_CURVE_WITH_KNOTS('',3,(#114788,#114789,#114790,#114791,
#114792,#114793,#114794),.UNSPECIFIED.,.F.,.F.,(4,3,4),(0.418382980505268,
0.425586573424719,0.435845921194646),.UNSPECIFIED.);
#22189=B_SPLINE_CURVE_WITH_KNOTS('',3,(#114795,#114796,#114797,#114798,
#114799,#114800),.UNSPECIFIED.,.F.,.F.,(4,2,4),(4.26339680314858E-11,0.0126485258971309,
0.0252971049135187),.UNSPECIFIED.);
#22190=B_SPLINE_CURVE_WITH_KNOTS('',3,(#114819,#114820,#114821,#114822,
#114823,#114824,#114825),.UNSPECIFIED.,.F.,.F.,(4,3,4),(0.418382980489403,
0.425586573424719,0.435845921190568),.UNSPECIFIED.);
#22191=B_SPLINE_CURVE_WITH_KNOTS('',3,(#114826,#114827,#114828,#114829,
#114830,#114831),.UNSPECIFIED.,.F.,.F.,(4,2,4),(0.,0.0126485258278667,0.0252968045262884),
 .UNSPECIFIED.);
#22192=B_SPLINE_CURVE_WITH_KNOTS('',3,(#114850,#114851,#114852,#114853,
#114854,#114855,#114856),.UNSPECIFIED.,.F.,.F.,(4,3,4),(0.418382980479098,
0.425586573428812,0.435845921190934),.UNSPECIFIED.);
#22193=B_SPLINE_CURVE_WITH_KNOTS('',3,(#114857,#114858,#114859,#114860,
#114861,#114862),.UNSPECIFIED.,.F.,.F.,(4,2,4),(3.90943730181204E-11,0.0126485258853341,
0.0252971112237266),.UNSPECIFIED.);
#22194=B_SPLINE_CURVE_WITH_KNOTS('',3,(#114881,#114882,#114883,#114884,
#114885,#114886,#114887),.UNSPECIFIED.,.F.,.F.,(4,3,4),(0.418382980500125,
0.425586573424719,0.435845921187664),.UNSPECIFIED.);
#22195=B_SPLINE_CURVE_WITH_KNOTS('',3,(#114888,#114889,#114890,#114891,
#114892,#114893),.UNSPECIFIED.,.F.,.F.,(4,2,4),(0.,0.0126485257976926,0.0252971245771656),
 .UNSPECIFIED.);
#22196=B_SPLINE_CURVE_WITH_KNOTS('',3,(#114912,#114913,#114914,#114915,
#114916,#114917,#114918),.UNSPECIFIED.,.F.,.F.,(4,3,4),(0.418382980499946,
0.425586573424719,0.43584592119258),.UNSPECIFIED.);
#22197=B_SPLINE_CURVE_WITH_KNOTS('',3,(#114919,#114920,#114921,#114922,
#114923,#114924),.UNSPECIFIED.,.F.,.F.,(4,2,4),(3.15449347118237E-11,0.0126485258940253,
0.0252970679240388),.UNSPECIFIED.);
#22198=B_SPLINE_CURVE_WITH_KNOTS('',3,(#114943,#114944,#114945,#114946,
#114947,#114948,#114949),.UNSPECIFIED.,.F.,.F.,(4,3,4),(0.41838298051113,
0.425586573424719,0.43584592119673),.UNSPECIFIED.);
#22199=B_SPLINE_CURVE_WITH_KNOTS('',3,(#114950,#114951,#114952,#114953,
#114954,#114955),.UNSPECIFIED.,.F.,.F.,(4,2,4),(2.73994050346722E-11,0.0126485258720225,
0.0252971368971687),.UNSPECIFIED.);
#22200=B_SPLINE_CURVE_WITH_KNOTS('',3,(#114974,#114975,#114976,#114977,
#114978,#114979,#114980),.UNSPECIFIED.,.F.,.F.,(4,3,4),(0.418382980509798,
0.425586573424719,0.435845921192082),.UNSPECIFIED.);
#22201=B_SPLINE_CURVE_WITH_KNOTS('',3,(#114981,#114982,#114983,#114984,
#114985,#114986),.UNSPECIFIED.,.F.,.F.,(4,2,4),(0.,0.012648525759877,0.0252971056115158),
 .UNSPECIFIED.);
#22202=B_SPLINE_CURVE_WITH_KNOTS('',3,(#115005,#115006,#115007,#115008,
#115009,#115010,#115011),.UNSPECIFIED.,.F.,.F.,(4,3,4),(0.418382980515049,
0.425586573424719,0.435845921182687),.UNSPECIFIED.);
#22203=B_SPLINE_CURVE_WITH_KNOTS('',3,(#115012,#115013,#115014,#115015,
#115016,#115017),.UNSPECIFIED.,.F.,.F.,(4,2,4),(1.57213468215666E-11,0.0126485258342171,
0.0252970836244904),.UNSPECIFIED.);
#22204=B_SPLINE_CURVE_WITH_KNOTS('',3,(#115036,#115037,#115038,#115039,
#115040,#115041,#115042),.UNSPECIFIED.,.F.,.F.,(4,3,4),(0.418382980513029,
0.425586573424719,0.435845921203653),.UNSPECIFIED.);
#22205=B_SPLINE_CURVE_WITH_KNOTS('',3,(#115043,#115044,#115045,#115046,
#115047,#115048),.UNSPECIFIED.,.F.,.F.,(4,2,4),(2.05864342097627E-11,0.0126485258407764,
0.0252971103490747),.UNSPECIFIED.);
#22206=B_SPLINE_CURVE_WITH_KNOTS('',3,(#115067,#115068,#115069,#115070,
#115071,#115072,#115073),.UNSPECIFIED.,.F.,.F.,(4,3,4),(0.418382980485447,
0.425586573430397,0.435845921197401),.UNSPECIFIED.);
#22207=B_SPLINE_CURVE_WITH_KNOTS('',3,(#115074,#115075,#115076,#115077,
#115078,#115079),.UNSPECIFIED.,.F.,.F.,(4,2,4),(3.23008789845055E-11,0.0126485258643573,
0.0252968045171681),.UNSPECIFIED.);
#22208=B_SPLINE_CURVE_WITH_KNOTS('',3,(#115098,#115099,#115100,#115101,
#115102,#115103,#115104),.UNSPECIFIED.,.F.,.F.,(4,3,4),(0.418382980476632,
0.425586573424719,0.435845921178522),.UNSPECIFIED.);
#22209=B_SPLINE_CURVE_WITH_KNOTS('',3,(#115105,#115106,#115107,#115108,
#115109,#115110),.UNSPECIFIED.,.F.,.F.,(4,2,4),(1.63062190473775E-11,0.0126485258563253,
0.0252970933324197),.UNSPECIFIED.);
#22210=B_SPLINE_CURVE_WITH_KNOTS('',3,(#115129,#115130,#115131,#115132,
#115133,#115134,#115135),.UNSPECIFIED.,.F.,.F.,(4,3,4),(0.418382980482894,
0.425586573424719,0.435845921193928),.UNSPECIFIED.);
#22211=B_SPLINE_CURVE_WITH_KNOTS('',3,(#115136,#115137,#115138,#115139,
#115140,#115141),.UNSPECIFIED.,.F.,.F.,(4,2,4),(3.7095862061997E-11,0.0126485258540792,
0.0252968044964005),.UNSPECIFIED.);
#22212=B_SPLINE_CURVE_WITH_KNOTS('',3,(#115160,#115161,#115162,#115163,
#115164,#115165,#115166),.UNSPECIFIED.,.F.,.F.,(4,3,4),(0.418382980504012,
0.425586573424719,0.435845921190153),.UNSPECIFIED.);
#22213=B_SPLINE_CURVE_WITH_KNOTS('',3,(#115167,#115168,#115169,#115170,
#115171,#115172),.UNSPECIFIED.,.F.,.F.,(4,2,4),(0.,0.0126485258021332,0.0252971237755114),
 .UNSPECIFIED.);
#22214=B_SPLINE_CURVE_WITH_KNOTS('',3,(#115191,#115192,#115193,#115194,
#115195,#115196,#115197),.UNSPECIFIED.,.F.,.F.,(4,3,4),(0.418382980512901,
0.425586573424719,0.435845921194506),.UNSPECIFIED.);
#22215=B_SPLINE_CURVE_WITH_KNOTS('',3,(#115198,#115199,#115200,#115201,
#115202,#115203),.UNSPECIFIED.,.F.,.F.,(4,2,4),(0.,0.0126485258091614,0.0252971262357942),
 .UNSPECIFIED.);
#22216=B_SPLINE_CURVE_WITH_KNOTS('',3,(#115222,#115223,#115224,#115225,
#115226,#115227,#115228),.UNSPECIFIED.,.F.,.F.,(4,3,4),(0.418382980499795,
0.425586573424719,0.435845921180363),.UNSPECIFIED.);
#22217=B_SPLINE_CURVE_WITH_KNOTS('',3,(#115229,#115230,#115231,#115232,
#115233,#115234),.UNSPECIFIED.,.F.,.F.,(4,2,4),(4.64361638924081E-11,0.0126485259046725,
0.0252970696604553),.UNSPECIFIED.);
#22218=B_SPLINE_CURVE_WITH_KNOTS('',3,(#115253,#115254,#115255,#115256,
#115257,#115258,#115259),.UNSPECIFIED.,.F.,.F.,(4,3,4),(0.418382980506079,
0.425586573424719,0.435845921191126),.UNSPECIFIED.);
#22219=B_SPLINE_CURVE_WITH_KNOTS('',3,(#115260,#115261,#115262,#115263,
#115264,#115265),.UNSPECIFIED.,.F.,.F.,(4,2,4),(3.43470368829114E-11,0.0126485258935371,
0.025297100751394),.UNSPECIFIED.);
#22220=B_SPLINE_CURVE_WITH_KNOTS('',3,(#115284,#115285,#115286,#115287,
#115288,#115289,#115290),.UNSPECIFIED.,.F.,.F.,(4,3,4),(0.418382980491293,
0.425586573424719,0.435845921202337),.UNSPECIFIED.);
#22221=B_SPLINE_CURVE_WITH_KNOTS('',3,(#115291,#115292,#115293,#115294,
#115295,#115296),.UNSPECIFIED.,.F.,.F.,(4,2,4),(0.,0.0126485258178913,0.0252971044575565),
 .UNSPECIFIED.);
#22222=B_SPLINE_CURVE_WITH_KNOTS('',3,(#115315,#115316,#115317,#115318,
#115319,#115320,#115321),.UNSPECIFIED.,.F.,.F.,(4,3,4),(0.418382980502393,
0.425586573424719,0.435845921184591),.UNSPECIFIED.);
#22223=B_SPLINE_CURVE_WITH_KNOTS('',3,(#115322,#115323,#115324,#115325,
#115326,#115327),.UNSPECIFIED.,.F.,.F.,(4,2,4),(1.51903425992353E-11,0.0126485258653875,
0.0252971164487305),.UNSPECIFIED.);
#22224=B_SPLINE_CURVE_WITH_KNOTS('',3,(#115346,#115347,#115348,#115349,
#115350,#115351,#115352),.UNSPECIFIED.,.F.,.F.,(4,3,4),(0.418382980495824,
0.425586573424718,0.435845921198099),.UNSPECIFIED.);
#22225=B_SPLINE_CURVE_WITH_KNOTS('',3,(#115353,#115354,#115355,#115356,
#115357,#115358),.UNSPECIFIED.,.F.,.F.,(4,2,4),(2.98048045712891E-11,0.0126485258797525,
0.0252970894690396),.UNSPECIFIED.);
#22226=B_SPLINE_CURVE_WITH_KNOTS('',3,(#115377,#115378,#115379,#115380,
#115381,#115382,#115383),.UNSPECIFIED.,.F.,.F.,(4,3,4),(0.418382980492499,
0.425586573424717,0.435845921198154),.UNSPECIFIED.);
#22227=B_SPLINE_CURVE_WITH_KNOTS('',3,(#115384,#115385,#115386,#115387,
#115388,#115389),.UNSPECIFIED.,.F.,.F.,(4,2,4),(0.,0.0126485257710713,0.0252971071417041),
 .UNSPECIFIED.);
#22228=B_SPLINE_CURVE_WITH_KNOTS('',3,(#115408,#115409,#115410,#115411,
#115412,#115413,#115414),.UNSPECIFIED.,.F.,.F.,(4,3,4),(0.418382980519489,
0.425586573424717,0.43584592119026),.UNSPECIFIED.);
#22229=B_SPLINE_CURVE_WITH_KNOTS('',3,(#115415,#115416,#115417,#115418,
#115419,#115420),.UNSPECIFIED.,.F.,.F.,(4,2,4),(4.64859468063662E-11,0.0126485259129894,
0.0252970884641446),.UNSPECIFIED.);
#22230=B_SPLINE_CURVE_WITH_KNOTS('',3,(#115439,#115440,#115441,#115442,
#115443,#115444,#115445),.UNSPECIFIED.,.F.,.F.,(4,3,4),(0.418382980516194,
0.425586573427319,0.435845921190088),.UNSPECIFIED.);
#22231=B_SPLINE_CURVE_WITH_KNOTS('',3,(#115446,#115447,#115448,#115449,
#115450,#115451),.UNSPECIFIED.,.F.,.F.,(4,2,4),(0.,0.0126485257202768,0.0252968057988102),
 .UNSPECIFIED.);
#22232=B_SPLINE_CURVE_WITH_KNOTS('',3,(#115470,#115471,#115472,#115473,
#115474,#115475,#115476),.UNSPECIFIED.,.F.,.F.,(4,3,4),(0.4183829805162,
0.425586573424721,0.435845921204263),.UNSPECIFIED.);
#22233=B_SPLINE_CURVE_WITH_KNOTS('',3,(#115477,#115478,#115479,#115480,
#115481,#115482),.UNSPECIFIED.,.F.,.F.,(4,2,4),(0.,0.0126485257808135,0.0252971162212155),
 .UNSPECIFIED.);
#22234=B_SPLINE_CURVE_WITH_KNOTS('',3,(#115500,#115501,#115502,#115503,
#115504,#115505,#115506),.UNSPECIFIED.,.F.,.F.,(4,3,4),(0.418382980217902,
0.425586573424719,0.43584592120451),.UNSPECIFIED.);
#22235=B_SPLINE_CURVE_WITH_KNOTS('',3,(#115518,#115519,#115520,#115521,
#115522,#115523),.UNSPECIFIED.,.F.,.F.,(4,2,4),(-0.0253030036884475,-0.012651613278566,
-6.34804847576831E-11),.UNSPECIFIED.);
#22236=B_SPLINE_CURVE_WITH_KNOTS('',3,(#115533,#115534,#115535,#115536,
#115537,#115538),.UNSPECIFIED.,.F.,.F.,(4,2,4),(3.87453103820511E-11,0.0126516133862915,
0.0253031602499559),.UNSPECIFIED.);
#22237=B_SPLINE_CURVE_WITH_KNOTS('',3,(#115558,#115559,#115560,#115561,
#115562,#115563),.UNSPECIFIED.,.F.,.F.,(4,2,4),(4.58383947136018E-11,0.012651613414177,
0.0253031740182665),.UNSPECIFIED.);
#22238=B_SPLINE_CURVE_WITH_KNOTS('',3,(#115583,#115584,#115585,#115586,
#115587,#115588),.UNSPECIFIED.,.F.,.F.,(4,2,4),(4.18194213214573E-11,0.0126516134067451,
0.0253031663402117),.UNSPECIFIED.);
#22239=B_SPLINE_CURVE_WITH_KNOTS('',3,(#115608,#115609,#115610,#115611,
#115612,#115613),.UNSPECIFIED.,.F.,.F.,(4,2,4),(3.68892339334775E-11,0.0126516134027975,
0.0253031428857036),.UNSPECIFIED.);
#22240=B_SPLINE_CURVE_WITH_KNOTS('',3,(#115633,#115634,#115635,#115636,
#115637,#115638),.UNSPECIFIED.,.F.,.F.,(4,2,4),(2.71107081691789E-11,0.0126516134121481,
0.025303136374457),.UNSPECIFIED.);
#22241=B_SPLINE_CURVE_WITH_KNOTS('',3,(#115658,#115659,#115660,#115661,
#115662,#115663),.UNSPECIFIED.,.F.,.F.,(4,2,4),(3.26941782094869E-11,0.0126516134056775,
0.0253031680303436),.UNSPECIFIED.);
#22242=B_SPLINE_CURVE_WITH_KNOTS('',3,(#115683,#115684,#115685,#115686,
#115687,#115688),.UNSPECIFIED.,.F.,.F.,(4,2,4),(4.29248539613176E-11,0.0126516134308501,
0.0253031435702894),.UNSPECIFIED.);
#22243=B_SPLINE_CURVE_WITH_KNOTS('',3,(#115708,#115709,#115710,#115711,
#115712,#115713),.UNSPECIFIED.,.F.,.F.,(4,2,4),(4.08007483957115E-11,0.0126516133998519,
0.0253031686506958),.UNSPECIFIED.);
#22244=B_SPLINE_CURVE_WITH_KNOTS('',3,(#115733,#115734,#115735,#115736,
#115737,#115738),.UNSPECIFIED.,.F.,.F.,(4,2,4),(3.58839648859037E-11,0.0126516133978681,
0.0253031555621786),.UNSPECIFIED.);
#22245=B_SPLINE_CURVE_WITH_KNOTS('',3,(#115758,#115759,#115760,#115761,
#115762,#115763),.UNSPECIFIED.,.F.,.F.,(4,2,4),(3.84531833298233E-11,0.0126516133967504,
0.0253031484415909),.UNSPECIFIED.);
#22246=B_SPLINE_CURVE_WITH_KNOTS('',3,(#115783,#115784,#115785,#115786,
#115787,#115788),.UNSPECIFIED.,.F.,.F.,(4,2,4),(2.3523365575452E-11,0.0126516133974983,
0.0253031368632556),.UNSPECIFIED.);
#22247=B_SPLINE_CURVE_WITH_KNOTS('',3,(#115808,#115809,#115810,#115811,
#115812,#115813),.UNSPECIFIED.,.F.,.F.,(4,2,4),(3.54867886648582E-11,0.0126516133853951,
0.0253031853795223),.UNSPECIFIED.);
#22248=B_SPLINE_CURVE_WITH_KNOTS('',3,(#115833,#115834,#115835,#115836,
#115837,#115838),.UNSPECIFIED.,.F.,.F.,(4,2,4),(5.96584564652658E-11,0.0126516134216209,
0.0253031646523377),.UNSPECIFIED.);
#22249=B_SPLINE_CURVE_WITH_KNOTS('',3,(#115858,#115859,#115860,#115861,
#115862,#115863),.UNSPECIFIED.,.F.,.F.,(4,2,4),(2.61156380054951E-9,0.0126516146787517,
0.025303174973131),.UNSPECIFIED.);
#22250=B_SPLINE_CURVE_WITH_KNOTS('',3,(#115883,#115884,#115885,#115886,
#115887,#115888),.UNSPECIFIED.,.F.,.F.,(4,2,4),(5.71527271307145E-11,0.0126516134042058,
0.0253031689996759),.UNSPECIFIED.);
#22251=B_SPLINE_CURVE_WITH_KNOTS('',3,(#115908,#115909,#115910,#115911,
#115912,#115913),.UNSPECIFIED.,.F.,.F.,(4,2,4),(6.59575722847113E-11,0.0126516134261569,
0.0253031712577939),.UNSPECIFIED.);
#22252=B_SPLINE_CURVE_WITH_KNOTS('',3,(#115933,#115934,#115935,#115936,
#115937,#115938),.UNSPECIFIED.,.F.,.F.,(4,2,4),(4.89391602995011E-11,0.0126516134447811,
0.0253031474960944),.UNSPECIFIED.);
#22253=B_SPLINE_CURVE_WITH_KNOTS('',3,(#115958,#115959,#115960,#115961,
#115962,#115963),.UNSPECIFIED.,.F.,.F.,(4,2,4),(4.80211333153906E-11,0.0126516134311367,
0.0253031660088819),.UNSPECIFIED.);
#22254=B_SPLINE_CURVE_WITH_KNOTS('',3,(#115983,#115984,#115985,#115986,
#115987,#115988),.UNSPECIFIED.,.F.,.F.,(4,2,4),(3.50832677987883E-11,0.0126516134091697,
0.0253031507487546),.UNSPECIFIED.);
#22255=B_SPLINE_CURVE_WITH_KNOTS('',3,(#116008,#116009,#116010,#116011,
#116012,#116013),.UNSPECIFIED.,.F.,.F.,(4,2,4),(2.28582008011667E-11,0.0126516133708363,
0.0253031658492592),.UNSPECIFIED.);
#22256=B_SPLINE_CURVE_WITH_KNOTS('',3,(#116033,#116034,#116035,#116036,
#116037,#116038),.UNSPECIFIED.,.F.,.F.,(4,2,4),(4.89625279206728E-11,0.0126516134300723,
0.0253031516310349),.UNSPECIFIED.);
#22257=B_SPLINE_CURVE_WITH_KNOTS('',3,(#116058,#116059,#116060,#116061,
#116062,#116063),.UNSPECIFIED.,.F.,.F.,(4,2,4),(5.84024084571817E-11,0.0126516134275552,
0.0253031615539805),.UNSPECIFIED.);
#22258=B_SPLINE_CURVE_WITH_KNOTS('',3,(#116083,#116084,#116085,#116086,
#116087,#116088),.UNSPECIFIED.,.F.,.F.,(4,2,4),(4.19633384918058E-11,0.01265161340334,
0.0253031729642154),.UNSPECIFIED.);
#22259=B_SPLINE_CURVE_WITH_KNOTS('',3,(#116108,#116109,#116110,#116111,
#116112,#116113),.UNSPECIFIED.,.F.,.F.,(4,2,4),(6.65337760895935E-11,0.0126516134575257,
0.0253031412759839),.UNSPECIFIED.);
#22260=B_SPLINE_CURVE_WITH_KNOTS('',3,(#116133,#116134,#116135,#116136,
#116137,#116138),.UNSPECIFIED.,.F.,.F.,(4,2,4),(0.,0.01265144724142,0.0253027587103005),
 .UNSPECIFIED.);
#22261=B_SPLINE_CURVE_WITH_KNOTS('',3,(#116158,#116159,#116160,#116161,
#116162,#116163),.UNSPECIFIED.,.F.,.F.,(4,2,4),(4.59033859231186E-11,0.0126516134106719,
0.0253031557895132),.UNSPECIFIED.);
#22262=B_SPLINE_CURVE_WITH_KNOTS('',3,(#116183,#116184,#116185,#116186,
#116187,#116188),.UNSPECIFIED.,.F.,.F.,(4,2,4),(3.2887239724366E-11,0.0126516134042047,
0.0253031298135651),.UNSPECIFIED.);
#22263=B_SPLINE_CURVE_WITH_KNOTS('',3,(#116208,#116209,#116210,#116211,
#116212,#116213),.UNSPECIFIED.,.F.,.F.,(4,2,4),(4.46558329558303E-11,0.0126516134319913,
0.0253031460002336),.UNSPECIFIED.);
#22264=B_SPLINE_CURVE_WITH_KNOTS('',3,(#116245,#116246,#116247,#116248,
#116249,#116250),.UNSPECIFIED.,.F.,.F.,(4,2,4),(-0.0253003002535201,-0.0126502136751869,
0.),.UNSPECIFIED.);
#22265=B_SPLINE_CURVE_WITH_KNOTS('',3,(#116257,#116258,#116259,#116260,
#116261,#116262,#116263),.UNSPECIFIED.,.F.,.F.,(4,3,4),(0.423588463701997,
0.428571428571429,0.435775021750426),.UNSPECIFIED.);
#22266=B_SPLINE_CURVE_WITH_KNOTS('',3,(#116292,#116293,#116294,#116295,
#116296,#116297),.UNSPECIFIED.,.F.,.F.,(4,2,4),(-0.0253003344256375,-0.0126502201925933,
0.),.UNSPECIFIED.);
#22267=B_SPLINE_CURVE_WITH_KNOTS('',3,(#116304,#116305,#116306,#116307,
#116308,#116309,#116310),.UNSPECIFIED.,.F.,.F.,(4,3,4),(0.423588463698078,
0.428571428571429,0.435775021750426),.UNSPECIFIED.);
#22268=B_SPLINE_CURVE_WITH_KNOTS('',3,(#116339,#116340,#116341,#116342,
#116343,#116344),.UNSPECIFIED.,.F.,.F.,(4,2,4),(-0.0253003283210845,-0.0126502130868413,
0.),.UNSPECIFIED.);
#22269=B_SPLINE_CURVE_WITH_KNOTS('',3,(#116351,#116352,#116353,#116354,
#116355,#116356,#116357),.UNSPECIFIED.,.F.,.F.,(4,3,4),(0.423588463701574,
0.428571428571429,0.435775021750427),.UNSPECIFIED.);
#22270=B_SPLINE_CURVE_WITH_KNOTS('',3,(#116386,#116387,#116388,#116389,
#116390,#116391),.UNSPECIFIED.,.F.,.F.,(4,2,4),(-0.0253002993995992,-0.0126502117370564,
0.),.UNSPECIFIED.);
#22271=B_SPLINE_CURVE_WITH_KNOTS('',3,(#116398,#116399,#116400,#116401,
#116402,#116403,#116404),.UNSPECIFIED.,.F.,.F.,(4,3,4),(0.423588463702291,
0.428571428571429,0.435775021750427),.UNSPECIFIED.);
#22272=B_SPLINE_CURVE_WITH_KNOTS('',3,(#116433,#116434,#116435,#116436,
#116437,#116438),.UNSPECIFIED.,.F.,.F.,(4,2,4),(-0.0253002995693567,-0.0126502089156248,
0.),.UNSPECIFIED.);
#22273=B_SPLINE_CURVE_WITH_KNOTS('',3,(#116445,#116446,#116447,#116448,
#116449,#116450,#116451),.UNSPECIFIED.,.F.,.F.,(4,3,4),(0.423588463706974,
0.428571428571429,0.435775021750427),.UNSPECIFIED.);
#22274=B_SPLINE_CURVE_WITH_KNOTS('',3,(#116480,#116481,#116482,#116483,
#116484,#116485),.UNSPECIFIED.,.F.,.F.,(4,2,4),(-0.02530030063837,-0.0126502070972325,
0.),.UNSPECIFIED.);
#22275=B_SPLINE_CURVE_WITH_KNOTS('',3,(#116492,#116493,#116494,#116495,
#116496,#116497,#116498),.UNSPECIFIED.,.F.,.F.,(4,3,4),(0.423588463701487,
0.428571428571429,0.435775021750431),.UNSPECIFIED.);
#22276=B_SPLINE_CURVE_WITH_KNOTS('',3,(#116527,#116528,#116529,#116530,
#116531,#116532),.UNSPECIFIED.,.F.,.F.,(4,2,4),(-0.0253002888255266,-0.012650205446942,
0.),.UNSPECIFIED.);
#22277=B_SPLINE_CURVE_WITH_KNOTS('',3,(#116539,#116540,#116541,#116542,
#116543,#116544,#116545),.UNSPECIFIED.,.F.,.F.,(4,3,4),(0.423588463699211,
0.428571428571429,0.435775021750432),.UNSPECIFIED.);
#22278=B_SPLINE_CURVE_WITH_KNOTS('',3,(#116574,#116575,#116576,#116577,
#116578,#116579),.UNSPECIFIED.,.F.,.F.,(4,2,4),(-0.0253002899033947,-0.0126502073537179,
0.),.UNSPECIFIED.);
#22279=B_SPLINE_CURVE_WITH_KNOTS('',3,(#116586,#116587,#116588,#116589,
#116590,#116591,#116592),.UNSPECIFIED.,.F.,.F.,(4,3,4),(0.423588463707525,
0.428571428571429,0.435775021750425),.UNSPECIFIED.);
#22280=B_SPLINE_CURVE_WITH_KNOTS('',3,(#116621,#116622,#116623,#116624,
#116625,#116626),.UNSPECIFIED.,.F.,.F.,(4,2,4),(-0.0253002950377611,-0.0126502055337274,
0.),.UNSPECIFIED.);
#22281=B_SPLINE_CURVE_WITH_KNOTS('',3,(#116633,#116634,#116635,#116636,
#116637,#116638,#116639),.UNSPECIFIED.,.F.,.F.,(4,3,4),(0.423588463701111,
0.428571428571429,0.435775021750424),.UNSPECIFIED.);
#22282=B_SPLINE_CURVE_WITH_KNOTS('',3,(#116668,#116669,#116670,#116671,
#116672,#116673),.UNSPECIFIED.,.F.,.F.,(4,2,4),(-0.0253002956570495,-0.012650211905278,
0.),.UNSPECIFIED.);
#22283=B_SPLINE_CURVE_WITH_KNOTS('',3,(#116680,#116681,#116682,#116683,
#116684,#116685,#116686),.UNSPECIFIED.,.F.,.F.,(4,3,4),(0.423588463700703,
0.428571428571429,0.435775021750423),.UNSPECIFIED.);
#22284=B_SPLINE_CURVE_WITH_KNOTS('',3,(#116715,#116716,#116717,#116718,
#116719,#116720),.UNSPECIFIED.,.F.,.F.,(4,2,4),(-0.0253003154846229,-0.0126502108025514,
0.),.UNSPECIFIED.);
#22285=B_SPLINE_CURVE_WITH_KNOTS('',3,(#116727,#116728,#116729,#116730,
#116731,#116732,#116733),.UNSPECIFIED.,.F.,.F.,(4,3,4),(0.423588463700741,
0.428571428571429,0.435775021750425),.UNSPECIFIED.);
#22286=B_SPLINE_CURVE_WITH_KNOTS('',3,(#116762,#116763,#116764,#116765,
#116766,#116767),.UNSPECIFIED.,.F.,.F.,(4,2,4),(-0.0253003226012023,-0.0126502117300696,
0.),.UNSPECIFIED.);
#22287=B_SPLINE_CURVE_WITH_KNOTS('',3,(#116774,#116775,#116776,#116777,
#116778,#116779,#116780),.UNSPECIFIED.,.F.,.F.,(4,3,4),(0.423588463704446,
0.428571428571429,0.435775021750425),.UNSPECIFIED.);
#22288=B_SPLINE_CURVE_WITH_KNOTS('',3,(#116809,#116810,#116811,#116812,
#116813,#116814),.UNSPECIFIED.,.F.,.F.,(4,2,4),(-0.0253003011424229,-0.0126502110863886,
0.),.UNSPECIFIED.);
#22289=B_SPLINE_CURVE_WITH_KNOTS('',3,(#116821,#116822,#116823,#116824,
#116825,#116826,#116827),.UNSPECIFIED.,.F.,.F.,(4,3,4),(0.42358846370506,
0.428571428571429,0.435775021750424),.UNSPECIFIED.);
#22290=B_SPLINE_CURVE_WITH_KNOTS('',3,(#116856,#116857,#116858,#116859,
#116860,#116861),.UNSPECIFIED.,.F.,.F.,(4,2,4),(-0.0253003126779101,-0.012650207513558,
0.),.UNSPECIFIED.);
#22291=B_SPLINE_CURVE_WITH_KNOTS('',3,(#116868,#116869,#116870,#116871,
#116872,#116873,#116874),.UNSPECIFIED.,.F.,.F.,(4,3,4),(0.423588463700609,
0.428571428571429,0.435775021750423),.UNSPECIFIED.);
#22292=B_SPLINE_CURVE_WITH_KNOTS('',3,(#116900,#116901,#116902,#116903,
#116904,#116905),.UNSPECIFIED.,.F.,.F.,(4,2,4),(-0.0253003114676457,-0.012650210849963,
0.),.UNSPECIFIED.);
#22293=B_SPLINE_CURVE_WITH_KNOTS('',3,(#116935,#116936,#116937,#116938,
#116939,#116940),.UNSPECIFIED.,.F.,.F.,(4,2,4),(-0.0253003381099669,-0.0126502129708172,
0.),.UNSPECIFIED.);
#22294=B_SPLINE_CURVE_WITH_KNOTS('',3,(#116947,#116948,#116949,#116950,
#116951,#116952,#116953),.UNSPECIFIED.,.F.,.F.,(4,3,4),(0.423588463705018,
0.428571428571429,0.435775021750423),.UNSPECIFIED.);
#22295=B_SPLINE_CURVE_WITH_KNOTS('',3,(#116982,#116983,#116984,#116985,
#116986,#116987),.UNSPECIFIED.,.F.,.F.,(4,2,4),(-0.0253002919638189,-0.0126502103961476,
0.),.UNSPECIFIED.);
#22296=B_SPLINE_CURVE_WITH_KNOTS('',3,(#116994,#116995,#116996,#116997,
#116998,#116999,#117000),.UNSPECIFIED.,.F.,.F.,(4,3,4),(0.423588463703294,
0.428571428571429,0.435775021750423),.UNSPECIFIED.);
#22297=B_SPLINE_CURVE_WITH_KNOTS('',3,(#117029,#117030,#117031,#117032,
#117033,#117034),.UNSPECIFIED.,.F.,.F.,(4,2,4),(-0.0253003060377706,-0.0126502066926115,
0.),.UNSPECIFIED.);
#22298=B_SPLINE_CURVE_WITH_KNOTS('',3,(#117041,#117042,#117043,#117044,
#117045,#117046,#117047),.UNSPECIFIED.,.F.,.F.,(4,3,4),(0.423588463707126,
0.428571428571429,0.435775021750423),.UNSPECIFIED.);
#22299=B_SPLINE_CURVE_WITH_KNOTS('',3,(#117076,#117077,#117078,#117079,
#117080,#117081),.UNSPECIFIED.,.F.,.F.,(4,2,4),(-0.0253002904690498,-0.0126502049689941,
0.),.UNSPECIFIED.);
#22300=B_SPLINE_CURVE_WITH_KNOTS('',3,(#117088,#117089,#117090,#117091,
#117092,#117093,#117094),.UNSPECIFIED.,.F.,.F.,(4,3,4),(0.423588463703339,
0.428571428571429,0.435775021750424),.UNSPECIFIED.);
#22301=B_SPLINE_CURVE_WITH_KNOTS('',3,(#117123,#117124,#117125,#117126,
#117127,#117128),.UNSPECIFIED.,.F.,.F.,(4,2,4),(-0.0253002929170949,-0.0126502123732119,
0.),.UNSPECIFIED.);
#22302=B_SPLINE_CURVE_WITH_KNOTS('',3,(#117135,#117136,#117137,#117138,
#117139,#117140,#117141),.UNSPECIFIED.,.F.,.F.,(4,3,4),(0.423588463702277,
0.428571428571429,0.435775021750435),.UNSPECIFIED.);
#22303=B_SPLINE_CURVE_WITH_KNOTS('',3,(#117170,#117171,#117172,#117173,
#117174,#117175),.UNSPECIFIED.,.F.,.F.,(4,2,4),(-0.0253003074016301,-0.0126502132546601,
0.),.UNSPECIFIED.);
#22304=B_SPLINE_CURVE_WITH_KNOTS('',3,(#117182,#117183,#117184,#117185,
#117186,#117187,#117188),.UNSPECIFIED.,.F.,.F.,(4,3,4),(0.423588463700518,
0.428571428571429,0.435775021750425),.UNSPECIFIED.);
#22305=B_SPLINE_CURVE_WITH_KNOTS('',3,(#117217,#117218,#117219,#117220,
#117221,#117222),.UNSPECIFIED.,.F.,.F.,(4,2,4),(-0.0253003088399219,-0.0126502137216067,
0.),.UNSPECIFIED.);
#22306=B_SPLINE_CURVE_WITH_KNOTS('',3,(#117229,#117230,#117231,#117232,
#117233,#117234,#117235),.UNSPECIFIED.,.F.,.F.,(4,3,4),(0.423588463703113,
0.428571428571429,0.435775021750423),.UNSPECIFIED.);
#22307=B_SPLINE_CURVE_WITH_KNOTS('',3,(#117264,#117265,#117266,#117267,
#117268,#117269),.UNSPECIFIED.,.F.,.F.,(4,2,4),(-0.0253004034332267,-0.0126502524469241,
0.),.UNSPECIFIED.);
#22308=B_SPLINE_CURVE_WITH_KNOTS('',3,(#117286,#117287,#117288,#117289,
#117290,#117291,#117292),.UNSPECIFIED.,.F.,.F.,(4,3,4),(0.423588464,0.428571428571429,
0.435775021750423),.UNSPECIFIED.);
#22309=B_SPLINE_CURVE_WITH_KNOTS('',3,(#117312,#117313,#117314,#117315,
#117316,#117317),.UNSPECIFIED.,.F.,.F.,(4,2,4),(-0.0253002982362509,-0.0126502053143726,
0.),.UNSPECIFIED.);
#22310=B_SPLINE_CURVE_WITH_KNOTS('',3,(#117320,#117321,#117322,#117323,
#117324,#117325,#117326),.UNSPECIFIED.,.F.,.F.,(4,3,4),(0.423588463703712,
0.428571428571429,0.435775021750422),.UNSPECIFIED.);
#22311=B_SPLINE_CURVE_WITH_KNOTS('',3,(#117358,#117359,#117360,#117361,
#117362,#117363),.UNSPECIFIED.,.F.,.F.,(4,2,4),(-0.0253003050044024,-0.0126502128753276,
0.),.UNSPECIFIED.);
#22312=B_SPLINE_CURVE_WITH_KNOTS('',3,(#117370,#117371,#117372,#117373,
#117374,#117375,#117376),.UNSPECIFIED.,.F.,.F.,(4,3,4),(0.423588463699629,
0.428571428571429,0.435775021750427),.UNSPECIFIED.);
#22313=B_SPLINE_CURVE_WITH_KNOTS('',3,(#117405,#117406,#117407,#117408,
#117409,#117410),.UNSPECIFIED.,.F.,.F.,(4,2,4),(-0.0253004073418385,-0.0126502524207922,
-2.2591730569621E-11),.UNSPECIFIED.);
#22314=B_SPLINE_CURVE_WITH_KNOTS('',3,(#117417,#117418,#117419,#117420,
#117421,#117422,#117423),.UNSPECIFIED.,.F.,.F.,(4,3,4),(0.423588463703243,
0.428571428571429,0.435775021750423),.UNSPECIFIED.);
#22315=B_SPLINE_CURVE_WITH_KNOTS('',3,(#117452,#117453,#117454,#117455,
#117456,#117457),.UNSPECIFIED.,.F.,.F.,(4,2,4),(-0.0253003262789758,-0.0126502195059414,
0.),.UNSPECIFIED.);
#22316=B_SPLINE_CURVE_WITH_KNOTS('',3,(#117464,#117465,#117466,#117467,
#117468,#117469,#117470),.UNSPECIFIED.,.F.,.F.,(4,3,4),(0.4235884637035,
0.428571428571429,0.435775021750422),.UNSPECIFIED.);
#22317=B_SPLINE_CURVE_WITH_KNOTS('',3,(#117499,#117500,#117501,#117502,
#117503,#117504),.UNSPECIFIED.,.F.,.F.,(4,2,4),(-0.0253003219384624,-0.0126502122908252,
0.),.UNSPECIFIED.);
#22318=B_SPLINE_CURVE_WITH_KNOTS('',3,(#117511,#117512,#117513,#117514,
#117515,#117516,#117517),.UNSPECIFIED.,.F.,.F.,(4,3,4),(0.423588463701606,
0.428571428571429,0.435775021750424),.UNSPECIFIED.);
#22319=B_SPLINE_CURVE_WITH_KNOTS('',3,(#117546,#117547,#117548,#117549,
#117550,#117551),.UNSPECIFIED.,.F.,.F.,(4,2,4),(-0.0253003053942314,-0.012650212995059,
0.),.UNSPECIFIED.);
#22320=B_SPLINE_CURVE_WITH_KNOTS('',3,(#117558,#117559,#117560,#117561,
#117562,#117563,#117564),.UNSPECIFIED.,.F.,.F.,(4,3,4),(0.423588463705113,
0.428571428571429,0.435775021750427),.UNSPECIFIED.);
#22321=B_SPLINE_CURVE_WITH_KNOTS('',3,(#117594,#117595,#117596,#117597,
#117598,#117599),.UNSPECIFIED.,.F.,.F.,(4,2,4),(-0.0253041425103788,-0.0126521901452956,
-6.82617870562119E-9),.UNSPECIFIED.);
#22322=B_SPLINE_CURVE_WITH_KNOTS('',3,(#117631,#117632,#117633,#117634,
#117635,#117636),.UNSPECIFIED.,.F.,.F.,(4,2,4),(-0.0253041425255257,-0.0126521901587595,
-6.82582376385077E-9),.UNSPECIFIED.);
#22323=B_SPLINE_CURVE_WITH_KNOTS('',3,(#117668,#117669,#117670,#117671,
#117672,#117673),.UNSPECIFIED.,.F.,.F.,(4,2,4),(-0.025304142490585,-0.0126521901211421,
-6.82654235223401E-9),.UNSPECIFIED.);
#22324=B_SPLINE_CURVE_WITH_KNOTS('',3,(#117705,#117706,#117707,#117708,
#117709,#117710),.UNSPECIFIED.,.F.,.F.,(4,2,4),(-0.0253041424713178,-0.0126521901284008,
-6.82603369661638E-9),.UNSPECIFIED.);
#22325=B_SPLINE_CURVE_WITH_KNOTS('',3,(#117742,#117743,#117744,#117745,
#117746,#117747),.UNSPECIFIED.,.F.,.F.,(4,2,4),(-0.0253041424469162,-0.0126521900930259,
-6.8265111168031E-9),.UNSPECIFIED.);
#22326=B_SPLINE_CURVE_WITH_KNOTS('',3,(#117779,#117780,#117781,#117782,
#117783,#117784),.UNSPECIFIED.,.F.,.F.,(4,2,4),(-0.0253041424488234,-0.0126521901167656,
-6.82550236816293E-9),.UNSPECIFIED.);
#22327=B_SPLINE_CURVE_WITH_KNOTS('',3,(#117816,#117817,#117818,#117819,
#117820,#117821),.UNSPECIFIED.,.F.,.F.,(4,2,4),(-0.025304142540414,-0.0126521901499399,
-6.82589951228607E-9),.UNSPECIFIED.);
#22328=B_SPLINE_CURVE_WITH_KNOTS('',3,(#117853,#117854,#117855,#117856,
#117857,#117858),.UNSPECIFIED.,.F.,.F.,(4,2,4),(-0.025304142479695,-0.0126521901100803,
-6.82574482005482E-9),.UNSPECIFIED.);
#22329=B_SPLINE_CURVE_WITH_KNOTS('',3,(#117890,#117891,#117892,#117893,
#117894,#117895),.UNSPECIFIED.,.F.,.F.,(4,2,4),(-0.0253041424980153,-0.0126521901257506,
-6.82570476875921E-9),.UNSPECIFIED.);
#22330=B_SPLINE_CURVE_WITH_KNOTS('',3,(#117927,#117928,#117929,#117930,
#117931,#117932),.UNSPECIFIED.,.F.,.F.,(4,2,4),(-0.025304142491032,-0.0126521901125237,
-6.82627537135216E-9),.UNSPECIFIED.);
#22331=B_SPLINE_CURVE_WITH_KNOTS('',3,(#117964,#117965,#117966,#117967,
#117968,#117969),.UNSPECIFIED.,.F.,.F.,(4,2,4),(-0.0253041425312974,-0.0126521901352363,
-6.82676192659271E-9),.UNSPECIFIED.);
#22332=B_SPLINE_CURVE_WITH_KNOTS('',3,(#118001,#118002,#118003,#118004,
#118005,#118006),.UNSPECIFIED.,.F.,.F.,(4,2,4),(-0.0253041424787179,-0.012652190106218,
-6.82538371654662E-9),.UNSPECIFIED.);
#22333=B_SPLINE_CURVE_WITH_KNOTS('',3,(#118038,#118039,#118040,#118041,
#118042,#118043),.UNSPECIFIED.,.F.,.F.,(4,2,4),(-0.0253041424998502,-0.0126521901348214,
-6.82580466801475E-9),.UNSPECIFIED.);
#22334=B_SPLINE_CURVE_WITH_KNOTS('',3,(#118075,#118076,#118077,#118078,
#118079,#118080),.UNSPECIFIED.,.F.,.F.,(4,2,4),(-0.025304142498564,-0.0126521901183685,
-6.82583610814302E-9),.UNSPECIFIED.);
#22335=B_SPLINE_CURVE_WITH_KNOTS('',3,(#118112,#118113,#118114,#118115,
#118116,#118117),.UNSPECIFIED.,.F.,.F.,(4,2,4),(-0.0253041424916259,-0.0126521901166737,
-6.82764770762456E-9),.UNSPECIFIED.);
#22336=B_SPLINE_CURVE_WITH_KNOTS('',3,(#118149,#118150,#118151,#118152,
#118153,#118154),.UNSPECIFIED.,.F.,.F.,(4,2,4),(-0.0253041424690007,-0.0126521901065946,
-6.8259175742269E-9),.UNSPECIFIED.);
#22337=B_SPLINE_CURVE_WITH_KNOTS('',3,(#118186,#118187,#118188,#118189,
#118190,#118191),.UNSPECIFIED.,.F.,.F.,(4,2,4),(-0.0253041425161077,-0.0126521901267836,
-6.8255786092597E-9),.UNSPECIFIED.);
#22338=B_SPLINE_CURVE_WITH_KNOTS('',3,(#118223,#118224,#118225,#118226,
#118227,#118228),.UNSPECIFIED.,.F.,.F.,(4,2,4),(-0.0253041424674938,-0.0126521901252898,
-6.8265300703918E-9),.UNSPECIFIED.);
#22339=B_SPLINE_CURVE_WITH_KNOTS('',3,(#118260,#118261,#118262,#118263,
#118264,#118265),.UNSPECIFIED.,.F.,.F.,(4,2,4),(-0.0253041424683401,-0.0126521901028931,
-6.82533373569383E-9),.UNSPECIFIED.);
#22340=B_SPLINE_CURVE_WITH_KNOTS('',3,(#118297,#118298,#118299,#118300,
#118301,#118302),.UNSPECIFIED.,.F.,.F.,(4,2,4),(-0.0253041425372917,-0.0126521901365104,
-6.82659049427992E-9),.UNSPECIFIED.);
#22341=B_SPLINE_CURVE_WITH_KNOTS('',3,(#118334,#118335,#118336,#118337,
#118338,#118339),.UNSPECIFIED.,.F.,.F.,(4,2,4),(-0.0253041425207301,-0.0126521901506318,
-6.82613092786721E-9),.UNSPECIFIED.);
#22342=B_SPLINE_CURVE_WITH_KNOTS('',3,(#118368,#118369,#118370,#118371,
#118372,#118373),.UNSPECIFIED.,.F.,.F.,(4,2,4),(-0.0253041424491209,-0.0126521901251303,
-6.82641140836715E-9),.UNSPECIFIED.);
#22343=B_SPLINE_CURVE_WITH_KNOTS('',3,(#118399,#118400,#118401,#118402,
#118403,#118404),.UNSPECIFIED.,.F.,.F.,(4,2,4),(-0.0253041424633494,-0.0126521901007878,
-6.82618439551419E-9),.UNSPECIFIED.);
#22344=B_SPLINE_CURVE_WITH_KNOTS('',3,(#118436,#118437,#118438,#118439,
#118440,#118441),.UNSPECIFIED.,.F.,.F.,(4,2,4),(-0.0253041424547078,-0.0126521901059465,
-6.82610486538171E-9),.UNSPECIFIED.);
#22345=B_SPLINE_CURVE_WITH_KNOTS('',3,(#118473,#118474,#118475,#118476,
#118477,#118478),.UNSPECIFIED.,.F.,.F.,(4,2,4),(-0.0253041425072535,-0.0126521901327817,
-6.82570005031136E-9),.UNSPECIFIED.);
#22346=B_SPLINE_CURVE_WITH_KNOTS('',3,(#118510,#118511,#118512,#118513,
#118514,#118515),.UNSPECIFIED.,.F.,.F.,(4,2,4),(-0.0253041425403756,-0.0126521901449272,
-6.82594121156899E-9),.UNSPECIFIED.);
#22347=B_SPLINE_CURVE_WITH_KNOTS('',3,(#118547,#118548,#118549,#118550,
#118551,#118552),.UNSPECIFIED.,.F.,.F.,(4,2,4),(-0.0253041425154124,-0.0126521901361906,
-6.82690581496614E-9),.UNSPECIFIED.);
#22348=B_SPLINE_CURVE_WITH_KNOTS('',3,(#118584,#118585,#118586,#118587,
#118588,#118589),.UNSPECIFIED.,.F.,.F.,(4,2,4),(-0.0253041424813593,-0.0126521901081155,
-6.82638875981745E-9),.UNSPECIFIED.);
#22349=B_SPLINE_CURVE_WITH_KNOTS('',3,(#118621,#118622,#118623,#118624,
#118625,#118626),.UNSPECIFIED.,.F.,.F.,(4,2,4),(-0.0253041424562475,-0.0126521901130813,
-6.82592604661636E-9),.UNSPECIFIED.);
#22350=B_SPLINE_CURVE_WITH_KNOTS('',3,(#118652,#118653,#118654,#118655,
#118656,#118657),.UNSPECIFIED.,.F.,.F.,(4,2,4),(-0.0257378279794269,-0.0126489395998484,
-2.53007684247741E-12),.UNSPECIFIED.);
#22351=B_SPLINE_CURVE_WITH_KNOTS('',3,(#118668,#118669,#118670,#118671,
#118672,#118673,#118674,#118675,#118676,#118677),.UNSPECIFIED.,.F.,.F.,
(4,3,3,4),(0.280362344104003,0.290171079270419,0.29250456354882,0.297785765985179),
 .UNSPECIFIED.);
#22352=B_SPLINE_CURVE_WITH_KNOTS('',3,(#118686,#118687,#118688,#118689,
#118690,#118691),.UNSPECIFIED.,.F.,.F.,(4,2,4),(-0.0257380902616007,-0.0126490009764804,
-3.02954050734883E-11),.UNSPECIFIED.);
#22353=B_SPLINE_CURVE_WITH_KNOTS('',3,(#118702,#118703,#118704,#118705,
#118706,#118707,#118708,#118709,#118710,#118711),.UNSPECIFIED.,.F.,.F.,
(4,3,3,4),(0.28036234408759,0.290171081638759,0.292504563548819,0.29778576598543),
 .UNSPECIFIED.);
#22354=B_SPLINE_CURVE_WITH_KNOTS('',3,(#118720,#118721,#118722,#118723,
#118724,#118725),.UNSPECIFIED.,.F.,.F.,(4,2,4),(-0.0257380523508611,-0.0126490009951788,
-3.81559714379698E-11),.UNSPECIFIED.);
#22355=B_SPLINE_CURVE_WITH_KNOTS('',3,(#118736,#118737,#118738,#118739,
#118740,#118741,#118742,#118743,#118744,#118745),.UNSPECIFIED.,.F.,.F.,
(4,3,3,4),(0.28036234408821,0.290171081007977,0.29250456354882,0.297785765981378),
 .UNSPECIFIED.);
#22356=B_SPLINE_CURVE_WITH_KNOTS('',3,(#118754,#118755,#118756,#118757,
#118758,#118759),.UNSPECIFIED.,.F.,.F.,(4,2,4),(-0.0257380907249933,-0.0126490010455048,
-6.705476104929E-11),.UNSPECIFIED.);
#22357=B_SPLINE_CURVE_WITH_KNOTS('',3,(#118770,#118771,#118772,#118773,
#118774,#118775,#118776,#118777,#118778,#118779),.UNSPECIFIED.,.F.,.F.,
(4,3,3,4),(0.280362344098491,0.290171080844525,0.29250456354882,0.297785765984799),
 .UNSPECIFIED.);
#22358=B_SPLINE_CURVE_WITH_KNOTS('',3,(#118788,#118789,#118790,#118791,
#118792,#118793),.UNSPECIFIED.,.F.,.F.,(4,2,4),(-0.0257380554680191,-0.0126490010287918,
-5.39744776650863E-11),.UNSPECIFIED.);
#22359=B_SPLINE_CURVE_WITH_KNOTS('',3,(#118804,#118805,#118806,#118807,
#118808,#118809,#118810,#118811,#118812,#118813),.UNSPECIFIED.,.F.,.F.,
(4,3,3,4),(0.280362344097552,0.290171073932283,0.29250456354882,0.297785765983655),
 .UNSPECIFIED.);
#22360=B_SPLINE_CURVE_WITH_KNOTS('',3,(#118822,#118823,#118824,#118825,
#118826,#118827),.UNSPECIFIED.,.F.,.F.,(4,2,4),(-0.0257377635808991,-0.0126489324097131,
0.),.UNSPECIFIED.);
#22361=B_SPLINE_CURVE_WITH_KNOTS('',3,(#118838,#118839,#118840,#118841,
#118842,#118843,#118844,#118845,#118846,#118847),.UNSPECIFIED.,.F.,.F.,
(4,3,3,4),(0.280362344104031,0.290171080688324,0.29250456354882,0.297785765995541),
 .UNSPECIFIED.);
#22362=B_SPLINE_CURVE_WITH_KNOTS('',3,(#118856,#118857,#118858,#118859,
#118860,#118861),.UNSPECIFIED.,.F.,.F.,(4,2,4),(-0.025737814464929,-0.0126489362667142,
-7.08981484631721E-13),.UNSPECIFIED.);
#22363=B_SPLINE_CURVE_WITH_KNOTS('',3,(#118872,#118873,#118874,#118875,
#118876,#118877,#118878,#118879,#118880,#118881),.UNSPECIFIED.,.F.,.F.,
(4,3,3,4),(0.280362344094927,0.290171080286353,0.29250456354882,0.297785765985366),
 .UNSPECIFIED.);
#22364=B_SPLINE_CURVE_WITH_KNOTS('',3,(#118890,#118891,#118892,#118893,
#118894,#118895),.UNSPECIFIED.,.F.,.F.,(4,2,4),(-0.0257380533657887,-0.0126490009459565,
-1.05018493901099E-11),.UNSPECIFIED.);
#22365=B_SPLINE_CURVE_WITH_KNOTS('',3,(#118906,#118907,#118908,#118909,
#118910,#118911,#118912,#118913,#118914,#118915),.UNSPECIFIED.,.F.,.F.,
(4,3,3,4),(0.280362344104297,0.290171083310114,0.29250456354882,0.297785765989853),
 .UNSPECIFIED.);
#22366=B_SPLINE_CURVE_WITH_KNOTS('',3,(#118924,#118925,#118926,#118927,
#118928,#118929),.UNSPECIFIED.,.F.,.F.,(4,2,4),(-0.0257377135008693,-0.012648921070624,
0.),.UNSPECIFIED.);
#22367=B_SPLINE_CURVE_WITH_KNOTS('',3,(#118940,#118941,#118942,#118943,
#118944,#118945,#118946,#118947,#118948,#118949),.UNSPECIFIED.,.F.,.F.,
(4,3,3,4),(0.28036234409434,0.290171079087173,0.29250456354882,0.297785765982063),
 .UNSPECIFIED.);
#22368=B_SPLINE_CURVE_WITH_KNOTS('',3,(#118958,#118959,#118960,#118961,
#118962,#118963),.UNSPECIFIED.,.F.,.F.,(4,2,4),(-0.0257380894295356,-0.0126490009412378,
-1.8889799446864E-11),.UNSPECIFIED.);
#22369=B_SPLINE_CURVE_WITH_KNOTS('',3,(#118974,#118975,#118976,#118977,
#118978,#118979,#118980,#118981,#118982,#118983),.UNSPECIFIED.,.F.,.F.,
(4,3,3,4),(0.280362344092742,0.290171082917341,0.29250456354882,0.297785765977771),
 .UNSPECIFIED.);
#22370=B_SPLINE_CURVE_WITH_KNOTS('',3,(#118992,#118993,#118994,#118995,
#118996,#118997),.UNSPECIFIED.,.F.,.F.,(4,2,4),(-0.02573774657654,-0.0126489291735479,
-1.30898243633215E-11),.UNSPECIFIED.);
#22371=B_SPLINE_CURVE_WITH_KNOTS('',3,(#119008,#119009,#119010,#119011,
#119012,#119013,#119014,#119015,#119016,#119017),.UNSPECIFIED.,.F.,.F.,
(4,3,3,4),(0.280362344109662,0.290171080351025,0.29250456354882,0.297785765975465),
 .UNSPECIFIED.);
#22372=B_SPLINE_CURVE_WITH_KNOTS('',3,(#119026,#119027,#119028,#119029,
#119030,#119031),.UNSPECIFIED.,.F.,.F.,(4,2,4),(-0.025738054439123,-0.0126490009490752,
-2.59499158272725E-11),.UNSPECIFIED.);
#22373=B_SPLINE_CURVE_WITH_KNOTS('',3,(#119042,#119043,#119044,#119045,
#119046,#119047,#119048,#119049,#119050,#119051),.UNSPECIFIED.,.F.,.F.,
(4,3,3,4),(0.280362344093884,0.290171081351687,0.29250456354882,0.29778576598458),
 .UNSPECIFIED.);
#22374=B_SPLINE_CURVE_WITH_KNOTS('',3,(#119060,#119061,#119062,#119063,
#119064,#119065),.UNSPECIFIED.,.F.,.F.,(4,2,4),(-0.0257380522579974,-0.0126490009637378,
-1.46792578092914E-11),.UNSPECIFIED.);
#22375=B_SPLINE_CURVE_WITH_KNOTS('',3,(#119076,#119077,#119078,#119079,
#119080,#119081,#119082,#119083,#119084,#119085),.UNSPECIFIED.,.F.,.F.,
(4,3,3,4),(0.280362344086871,0.29017107886419,0.29250456354882,0.297785765975111),
 .UNSPECIFIED.);
#22376=B_SPLINE_CURVE_WITH_KNOTS('',3,(#119094,#119095,#119096,#119097,
#119098,#119099),.UNSPECIFIED.,.F.,.F.,(4,2,4),(-0.0257377497019341,-0.0126489292638499,
0.),.UNSPECIFIED.);
#22377=B_SPLINE_CURVE_WITH_KNOTS('',3,(#119110,#119111,#119112,#119113,
#119114,#119115,#119116,#119117,#119118,#119119),.UNSPECIFIED.,.F.,.F.,
(4,3,3,4),(0.280362344097843,0.290171077351318,0.29250456354882,0.297785765986222),
 .UNSPECIFIED.);
#22378=B_SPLINE_CURVE_WITH_KNOTS('',3,(#119128,#119129,#119130,#119131,
#119132,#119133),.UNSPECIFIED.,.F.,.F.,(4,2,4),(-0.0257380889613719,-0.0126490009095234,
0.),.UNSPECIFIED.);
#22379=B_SPLINE_CURVE_WITH_KNOTS('',3,(#119144,#119145,#119146,#119147,
#119148,#119149,#119150,#119151,#119152,#119153),.UNSPECIFIED.,.F.,.F.,
(4,3,3,4),(0.280362344087793,0.290171079520635,0.29250456354882,0.297785765989929),
 .UNSPECIFIED.);
#22380=B_SPLINE_CURVE_WITH_KNOTS('',3,(#119162,#119163,#119164,#119165,
#119166,#119167),.UNSPECIFIED.,.F.,.F.,(4,2,4),(-0.0257380910289757,-0.0126490010077677,
-4.76177708375047E-11),.UNSPECIFIED.);
#22381=B_SPLINE_CURVE_WITH_KNOTS('',3,(#119178,#119179,#119180,#119181,
#119182,#119183,#119184,#119185,#119186,#119187),.UNSPECIFIED.,.F.,.F.,
(4,3,3,4),(0.280362344092674,0.290171082508215,0.29250456354882,0.2977857659921),
 .UNSPECIFIED.);
#22382=B_SPLINE_CURVE_WITH_KNOTS('',3,(#119196,#119197,#119198,#119199,
#119200,#119201),.UNSPECIFIED.,.F.,.F.,(4,2,4),(-0.0257380538364327,-0.0126490009720209,
-4.27359085619639E-11),.UNSPECIFIED.);
#22383=B_SPLINE_CURVE_WITH_KNOTS('',3,(#119212,#119213,#119214,#119215,
#119216,#119217,#119218,#119219,#119220,#119221),.UNSPECIFIED.,.F.,.F.,
(4,3,3,4),(0.280362344096328,0.290171079866836,0.29250456354882,0.29778576599798),
 .UNSPECIFIED.);
#22384=B_SPLINE_CURVE_WITH_KNOTS('',3,(#119230,#119231,#119232,#119233,
#119234,#119235),.UNSPECIFIED.,.F.,.F.,(4,2,4),(-0.0257380885351855,-0.0126490009655906,
-5.36579392029779E-11),.UNSPECIFIED.);
#22385=B_SPLINE_CURVE_WITH_KNOTS('',3,(#119246,#119247,#119248,#119249,
#119250,#119251,#119252,#119253,#119254,#119255),.UNSPECIFIED.,.F.,.F.,
(4,3,3,4),(0.280362344087404,0.290171079583168,0.29250456354882,0.29778576599091),
 .UNSPECIFIED.);
#22386=B_SPLINE_CURVE_WITH_KNOTS('',3,(#119264,#119265,#119266,#119267,
#119268,#119269),.UNSPECIFIED.,.F.,.F.,(4,2,4),(-0.0257380906026673,-0.0126490009878925,
-2.80112807948818E-11),.UNSPECIFIED.);
#22387=B_SPLINE_CURVE_WITH_KNOTS('',3,(#119280,#119281,#119282,#119283,
#119284,#119285,#119286,#119287,#119288,#119289),.UNSPECIFIED.,.F.,.F.,
(4,3,3,4),(0.28036234409184,0.290171081060908,0.29250456354882,0.297785765984655),
 .UNSPECIFIED.);
#22388=B_SPLINE_CURVE_WITH_KNOTS('',3,(#119298,#119299,#119300,#119301,
#119302,#119303),.UNSPECIFIED.,.F.,.F.,(4,2,4),(-0.0257377476829762,-0.0126489293355879,
0.),.UNSPECIFIED.);
#22389=B_SPLINE_CURVE_WITH_KNOTS('',3,(#119314,#119315,#119316,#119317,
#119318,#119319,#119320,#119321,#119322,#119323),.UNSPECIFIED.,.F.,.F.,
(4,3,3,4),(0.280362344098895,0.290171085510633,0.29250456354882,0.297785765984775),
 .UNSPECIFIED.);
#22390=B_SPLINE_CURVE_WITH_KNOTS('',3,(#119332,#119333,#119334,#119335,
#119336,#119337),.UNSPECIFIED.,.F.,.F.,(4,2,4),(-0.0257377936615723,-0.012648931273962,
0.),.UNSPECIFIED.);
#22391=B_SPLINE_CURVE_WITH_KNOTS('',3,(#119348,#119349,#119350,#119351,
#119352,#119353,#119354,#119355,#119356,#119357),.UNSPECIFIED.,.F.,.F.,
(4,3,3,4),(0.280362344096488,0.290171081541738,0.29250456354882,0.297785765992854),
 .UNSPECIFIED.);
#22392=B_SPLINE_CURVE_WITH_KNOTS('',3,(#119366,#119367,#119368,#119369,
#119370,#119371),.UNSPECIFIED.,.F.,.F.,(4,2,4),(-0.0257380555399184,-0.0126490010070952,
-3.87272332258437E-11),.UNSPECIFIED.);
#22393=B_SPLINE_CURVE_WITH_KNOTS('',3,(#119382,#119383,#119384,#119385,
#119386,#119387,#119388,#119389,#119390,#119391),.UNSPECIFIED.,.F.,.F.,
(4,3,3,4),(0.280362344096632,0.290171080874968,0.29250456354882,0.297785765980618),
 .UNSPECIFIED.);
#22394=B_SPLINE_CURVE_WITH_KNOTS('',3,(#119400,#119401,#119402,#119403,
#119404,#119405),.UNSPECIFIED.,.F.,.F.,(4,2,4),(-0.0257380552031559,-0.0126490009621647,
-2.14355651284581E-11),.UNSPECIFIED.);
#22395=B_SPLINE_CURVE_WITH_KNOTS('',3,(#119416,#119417,#119418,#119419,
#119420,#119421,#119422,#119423,#119424,#119425),.UNSPECIFIED.,.F.,.F.,
(4,3,3,4),(0.280362344102986,0.290171073386061,0.292504563548819,0.297785765974851),
 .UNSPECIFIED.);
#22396=B_SPLINE_CURVE_WITH_KNOTS('',3,(#119434,#119435,#119436,#119437,
#119438,#119439),.UNSPECIFIED.,.F.,.F.,(4,2,4),(-0.0257380531289192,-0.0126490009645852,
-2.70962662030083E-11),.UNSPECIFIED.);
#22397=B_SPLINE_CURVE_WITH_KNOTS('',3,(#119450,#119451,#119452,#119453,
#119454,#119455,#119456,#119457,#119458,#119459),.UNSPECIFIED.,.F.,.F.,
(4,3,3,4),(0.280362344089115,0.290171084276077,0.292504563548822,0.297785765972127),
 .UNSPECIFIED.);
#22398=B_SPLINE_CURVE_WITH_KNOTS('',3,(#119468,#119469,#119470,#119471,
#119472,#119473),.UNSPECIFIED.,.F.,.F.,(4,2,4),(-0.0257380896009897,-0.012649000953846,
-1.29762312006676E-11),.UNSPECIFIED.);
#22399=B_SPLINE_CURVE_WITH_KNOTS('',3,(#119484,#119485,#119486,#119487,
#119488,#119489,#119490,#119491,#119492,#119493),.UNSPECIFIED.,.F.,.F.,
(4,3,3,4),(0.280362344103357,0.290171079085373,0.292504563548816,0.297785765978392),
 .UNSPECIFIED.);
#22400=B_SPLINE_CURVE_WITH_KNOTS('',3,(#119502,#119503,#119504,#119505,
#119506,#119507),.UNSPECIFIED.,.F.,.F.,(4,2,4),(-0.025738053166032,-0.0126490009774138,
-3.8124906009962E-11),.UNSPECIFIED.);
#22401=B_SPLINE_CURVE_WITH_KNOTS('',3,(#119518,#119519,#119520,#119521,
#119522,#119523,#119524,#119525,#119526,#119527),.UNSPECIFIED.,.F.,.F.,
(4,3,3,4),(0.280362344088634,0.290171076593144,0.292504563548811,0.29778576598622),
 .UNSPECIFIED.);
#22402=B_SPLINE_CURVE_WITH_KNOTS('',3,(#119536,#119537,#119538,#119539,
#119540,#119541),.UNSPECIFIED.,.F.,.F.,(4,2,4),(-0.0257380507764179,-0.0126490009275113,
0.),.UNSPECIFIED.);
#22403=B_SPLINE_CURVE_WITH_KNOTS('',3,(#119552,#119553,#119554,#119555,
#119556,#119557,#119558,#119559,#119560,#119561),.UNSPECIFIED.,.F.,.F.,
(4,3,3,4),(0.280362344090312,0.290171084260232,0.292504563548813,0.297785765977126),
 .UNSPECIFIED.);
#22404=B_SPLINE_CURVE_WITH_KNOTS('',3,(#119570,#119571,#119572,#119573,
#119574,#119575),.UNSPECIFIED.,.F.,.F.,(4,2,4),(-0.0257380885569789,-0.0126490009347652,
-1.58122993865195E-11),.UNSPECIFIED.);
#22405=B_SPLINE_CURVE_WITH_KNOTS('',3,(#119586,#119587,#119588,#119589,
#119590,#119591,#119592,#119593,#119594,#119595),.UNSPECIFIED.,.F.,.F.,
(4,3,3,4),(0.280362344110013,0.290171077184626,0.292504563548815,0.297785765989047),
 .UNSPECIFIED.);
#22406=B_SPLINE_CURVE_WITH_KNOTS('',3,(#119604,#119605,#119606,#119607,
#119608,#119609),.UNSPECIFIED.,.F.,.F.,(4,2,4),(-0.0257380525083116,-0.0126490009941628,
-2.24978022322908E-11),.UNSPECIFIED.);
#22407=B_SPLINE_CURVE_WITH_KNOTS('',3,(#119620,#119621,#119622,#119623,
#119624,#119625,#119626,#119627,#119628,#119629),.UNSPECIFIED.,.F.,.F.,
(4,3,3,4),(0.280362344001298,0.290171046132489,0.29250456354882,0.297785765999036),
 .UNSPECIFIED.);
#22408=B_SPLINE_CURVE_WITH_KNOTS('',3,(#119638,#119639,#119640,#119641,
#119642,#119643,#119644,#119645,#119646,#119647),.UNSPECIFIED.,.F.,.F.,
(4,3,3,4),(1.78416752250298E-15,8.70313175311398E-5,0.000170023930203073,
0.000253018981535489),.UNSPECIFIED.);
#22409=B_SPLINE_CURVE_WITH_KNOTS('',3,(#119658,#119659,#119660,#119661,
#119662,#119663,#119664,#119665,#119666,#119667),.UNSPECIFIED.,.F.,.F.,
(4,3,3,4),(0.487259899834934,0.497067956779899,0.5,0.504719756176226),
 .UNSPECIFIED.);
#22410=B_SPLINE_CURVE_WITH_KNOTS('',3,(#119676,#119677,#119678,#119679,
#119680,#119681,#119682,#119683,#119684,#119685),.UNSPECIFIED.,.F.,.F.,
(4,3,3,4),(3.41332323048545E-14,8.70313175545581E-5,0.000170023930246138,
0.000253018981134818),.UNSPECIFIED.);
#22411=B_SPLINE_CURVE_WITH_KNOTS('',3,(#119696,#119697,#119698,#119699,
#119700,#119701,#119702,#119703,#119704,#119705),.UNSPECIFIED.,.F.,.F.,
(4,3,3,4),(0.487259899830027,0.497067953928199,0.5,0.504719756176227),
 .UNSPECIFIED.);
#22412=B_SPLINE_CURVE_WITH_KNOTS('',3,(#119714,#119715,#119716,#119717,
#119718,#119719,#119720,#119721,#119722,#119723),.UNSPECIFIED.,.F.,.F.,
(4,3,3,4),(2.45274570368324E-14,8.70313177460311E-5,0.000170023930143113,
0.000253018980672992),.UNSPECIFIED.);
#22413=B_SPLINE_CURVE_WITH_KNOTS('',3,(#119734,#119735,#119736,#119737,
#119738,#119739,#119740,#119741,#119742,#119743),.UNSPECIFIED.,.F.,.F.,
(4,3,3,4),(0.487259899841302,0.497067955279116,0.5,0.504719756176227),
 .UNSPECIFIED.);
#22414=B_SPLINE_CURVE_WITH_KNOTS('',3,(#119752,#119753,#119754,#119755,
#119756,#119757,#119758,#119759,#119760,#119761),.UNSPECIFIED.,.F.,.F.,
(4,3,3,4),(1.70470283076348E-14,8.70313174616613E-5,0.000170023930255742,
0.000253018981768342),.UNSPECIFIED.);
#22415=B_SPLINE_CURVE_WITH_KNOTS('',3,(#119772,#119773,#119774,#119775,
#119776,#119777,#119778,#119779,#119780,#119781),.UNSPECIFIED.,.F.,.F.,
(4,3,3,4),(0.487259899828108,0.497067956582658,0.5,0.504719756176227),
 .UNSPECIFIED.);
#22416=B_SPLINE_CURVE_WITH_KNOTS('',3,(#119790,#119791,#119792,#119793,
#119794,#119795,#119796,#119797,#119798,#119799),.UNSPECIFIED.,.F.,.F.,
(4,3,3,4),(8.61735280637014E-14,8.70313175901959E-5,0.000170023930245986,
0.000253018981322021),.UNSPECIFIED.);
#22417=B_SPLINE_CURVE_WITH_KNOTS('',3,(#119810,#119811,#119812,#119813,
#119814,#119815,#119816,#119817,#119818,#119819),.UNSPECIFIED.,.F.,.F.,
(4,3,3,4),(0.487259899824588,0.497067952915038,0.5,0.504719756176227),
 .UNSPECIFIED.);
#22418=B_SPLINE_CURVE_WITH_KNOTS('',3,(#119828,#119829,#119830,#119831,
#119832,#119833,#119834,#119835,#119836,#119837),.UNSPECIFIED.,.F.,.F.,
(4,3,3,4),(6.4801676788079E-14,8.70313176737056E-5,0.000170023930339139,
0.000253018981507554),.UNSPECIFIED.);
#22419=B_SPLINE_CURVE_WITH_KNOTS('',3,(#119848,#119849,#119850,#119851,
#119852,#119853,#119854,#119855,#119856,#119857),.UNSPECIFIED.,.F.,.F.,
(4,3,3,4),(0.487259899837411,0.497067955332477,0.5,0.504719756176226),
 .UNSPECIFIED.);
#22420=B_SPLINE_CURVE_WITH_KNOTS('',3,(#119866,#119867,#119868,#119869,
#119870,#119871,#119872,#119873,#119874,#119875),.UNSPECIFIED.,.F.,.F.,
(4,3,3,4),(4.46624994070207E-14,8.703131763642E-5,0.0001700239303354,0.000253018981642442),
 .UNSPECIFIED.);
#22421=B_SPLINE_CURVE_WITH_KNOTS('',3,(#119886,#119887,#119888,#119889,
#119890,#119891,#119892,#119893,#119894,#119895),.UNSPECIFIED.,.F.,.F.,
(4,3,3,4),(0.487259899847783,0.497067955749335,0.5,0.504719756176227),
 .UNSPECIFIED.);
#22422=B_SPLINE_CURVE_WITH_KNOTS('',3,(#119904,#119905,#119906,#119907,
#119908,#119909,#119910,#119911,#119912,#119913),.UNSPECIFIED.,.F.,.F.,
(4,3,3,4),(1.90268839248483E-14,8.70313177274394E-5,0.000170023930133409,
0.000253018980982867),.UNSPECIFIED.);
#22423=B_SPLINE_CURVE_WITH_KNOTS('',3,(#119924,#119925,#119926,#119927,
#119928,#119929,#119930,#119931,#119932,#119933),.UNSPECIFIED.,.F.,.F.,
(4,3,3,4),(0.487259899837452,0.497067951424618,0.5,0.504719756176228),
 .UNSPECIFIED.);
#22424=B_SPLINE_CURVE_WITH_KNOTS('',3,(#119942,#119943,#119944,#119945,
#119946,#119947,#119948,#119949,#119950,#119951),.UNSPECIFIED.,.F.,.F.,
(4,3,3,4),(1.63355867732691E-14,8.70313177195555E-5,0.000170023930283018,
0.000253018981197976),.UNSPECIFIED.);
#22425=B_SPLINE_CURVE_WITH_KNOTS('',3,(#119962,#119963,#119964,#119965,
#119966,#119967,#119968,#119969,#119970,#119971),.UNSPECIFIED.,.F.,.F.,
(4,3,3,4),(0.487259899844168,0.497067950844091,0.5,0.504719756176228),
 .UNSPECIFIED.);
#22426=B_SPLINE_CURVE_WITH_KNOTS('',3,(#119980,#119981,#119982,#119983,
#119984,#119985,#119986,#119987,#119988,#119989),.UNSPECIFIED.,.F.,.F.,
(4,3,3,4),(4.32089986161599E-14,8.70313176778163E-5,0.000170023930202668,
0.000253018981062845),.UNSPECIFIED.);
#22427=B_SPLINE_CURVE_WITH_KNOTS('',3,(#120000,#120001,#120002,#120003,
#120004,#120005,#120006,#120007,#120008,#120009),.UNSPECIFIED.,.F.,.F.,
(4,3,3,4),(0.487259899833474,0.497067957211732,0.5,0.504719756176228),
 .UNSPECIFIED.);
#22428=B_SPLINE_CURVE_WITH_KNOTS('',3,(#120018,#120019,#120020,#120021,
#120022,#120023,#120024,#120025,#120026,#120027),.UNSPECIFIED.,.F.,.F.,
(4,3,3,4),(5.85668130751604E-14,8.70313175937449E-5,0.000170023930273888,
0.000253018981217468),.UNSPECIFIED.);
#22429=B_SPLINE_CURVE_WITH_KNOTS('',3,(#120038,#120039,#120040,#120041,
#120042,#120043,#120044,#120045,#120046,#120047),.UNSPECIFIED.,.F.,.F.,
(4,3,3,4),(0.487259899836209,0.497067955102255,0.5,0.504719756176228),
 .UNSPECIFIED.);
#22430=B_SPLINE_CURVE_WITH_KNOTS('',3,(#120056,#120057,#120058,#120059,
#120060,#120061,#120062,#120063,#120064,#120065),.UNSPECIFIED.,.F.,.F.,
(4,3,3,4),(7.01370277151711E-14,8.70313175559056E-5,0.000170023930128497,
0.00025301898233016),.UNSPECIFIED.);
#22431=B_SPLINE_CURVE_WITH_KNOTS('',3,(#120076,#120077,#120078,#120079,
#120080,#120081,#120082,#120083,#120084,#120085),.UNSPECIFIED.,.F.,.F.,
(4,3,3,4),(0.487259899821166,0.497067952690467,0.5,0.504719756176228),
 .UNSPECIFIED.);
#22432=B_SPLINE_CURVE_WITH_KNOTS('',3,(#120094,#120095,#120096,#120097,
#120098,#120099,#120100,#120101,#120102,#120103),.UNSPECIFIED.,.F.,.F.,
(4,3,3,4),(3.4379490863589E-14,8.70313176981463E-5,0.000170023930243521,
0.000253018982813477),.UNSPECIFIED.);
#22433=B_SPLINE_CURVE_WITH_KNOTS('',3,(#120114,#120115,#120116,#120117,
#120118,#120119,#120120,#120121,#120122,#120123),.UNSPECIFIED.,.F.,.F.,
(4,3,3,4),(0.487259899831263,0.497067954216751,0.5,0.504719756173849),
 .UNSPECIFIED.);
#22434=B_SPLINE_CURVE_WITH_KNOTS('',3,(#120132,#120133,#120134,#120135,
#120136,#120137,#120138,#120139,#120140,#120141),.UNSPECIFIED.,.F.,.F.,
(4,3,3,4),(5.43013114251202E-14,8.70313176102924E-5,0.000170023930127259,
0.000253018981186722),.UNSPECIFIED.);
#22435=B_SPLINE_CURVE_WITH_KNOTS('',3,(#120152,#120153,#120154,#120155,
#120156,#120157,#120158,#120159,#120160,#120161),.UNSPECIFIED.,.F.,.F.,
(4,3,3,4),(0.48725989983763,0.497067952795034,0.5,0.504719756176228),
 .UNSPECIFIED.);
#22436=B_SPLINE_CURVE_WITH_KNOTS('',3,(#120170,#120171,#120172,#120173,
#120174,#120175,#120176,#120177,#120178,#120179),.UNSPECIFIED.,.F.,.F.,
(4,3,3,4),(2.41375655958049E-14,8.70313176307348E-5,0.000170023930272469,
0.00025301898123237),.UNSPECIFIED.);
#22437=B_SPLINE_CURVE_WITH_KNOTS('',3,(#120190,#120191,#120192,#120193,
#120194,#120195,#120196,#120197,#120198,#120199),.UNSPECIFIED.,.F.,.F.,
(4,3,3,4),(0.487259899839516,0.497067955878832,0.5,0.504719756176228),
 .UNSPECIFIED.);
#22438=B_SPLINE_CURVE_WITH_KNOTS('',3,(#120208,#120209,#120210,#120211,
#120212,#120213,#120214,#120215,#120216,#120217),.UNSPECIFIED.,.F.,.F.,
(4,3,3,4),(5.85991331726249E-14,8.70313175998023E-5,0.000170023930181731,
0.000253018980908884),.UNSPECIFIED.);
#22439=B_SPLINE_CURVE_WITH_KNOTS('',3,(#120228,#120229,#120230,#120231,
#120232,#120233,#120234,#120235,#120236,#120237),.UNSPECIFIED.,.F.,.F.,
(4,3,3,4),(0.487259899833153,0.497067954345318,0.5,0.50471975617623),
 .UNSPECIFIED.);
#22440=B_SPLINE_CURVE_WITH_KNOTS('',3,(#120246,#120247,#120248,#120249,
#120250,#120251,#120252,#120253,#120254,#120255),.UNSPECIFIED.,.F.,.F.,
(4,3,3,4),(2.95380358239764E-15,8.70313176641763E-5,0.000170023930380612,
0.000253018981633287),.UNSPECIFIED.);
#22441=B_SPLINE_CURVE_WITH_KNOTS('',3,(#120266,#120267,#120268,#120269,
#120270,#120271,#120272,#120273,#120274,#120275),.UNSPECIFIED.,.F.,.F.,
(4,3,3,4),(0.487259899831205,0.497067957272829,0.5,0.504719756176228),
 .UNSPECIFIED.);
#22442=B_SPLINE_CURVE_WITH_KNOTS('',3,(#120284,#120285,#120286,#120287,
#120288,#120289,#120290,#120291,#120292,#120293),.UNSPECIFIED.,.F.,.F.,
(4,3,3,4),(6.94791745557739E-14,8.70313178044004E-5,0.00017002393033166,
0.000253018982522185),.UNSPECIFIED.);
#22443=B_SPLINE_CURVE_WITH_KNOTS('',3,(#120304,#120305,#120306,#120307,
#120308,#120309,#120310,#120311,#120312,#120313),.UNSPECIFIED.,.F.,.F.,
(4,3,3,4),(0.487259899845777,0.497067954429802,0.5,0.504719756176228),
 .UNSPECIFIED.);
#22444=B_SPLINE_CURVE_WITH_KNOTS('',3,(#120322,#120323,#120324,#120325,
#120326,#120327,#120328,#120329,#120330,#120331),.UNSPECIFIED.,.F.,.F.,
(4,3,3,4),(1.05931133367487E-14,8.70313177939862E-5,0.000170023930133989,
0.000253018980682019),.UNSPECIFIED.);
#22445=B_SPLINE_CURVE_WITH_KNOTS('',3,(#120342,#120343,#120344,#120345,
#120346,#120347,#120348,#120349,#120350,#120351),.UNSPECIFIED.,.F.,.F.,
(4,3,3,4),(0.487259899839067,0.497067957978687,0.5,0.504719756176227),
 .UNSPECIFIED.);
#22446=B_SPLINE_CURVE_WITH_KNOTS('',3,(#120360,#120361,#120362,#120363,
#120364,#120365,#120366,#120367,#120368,#120369),.UNSPECIFIED.,.F.,.F.,
(4,3,3,4),(5.08094850759228E-14,8.70313176670443E-5,0.000170023930229356,
0.000253018982807892),.UNSPECIFIED.);
#22447=B_SPLINE_CURVE_WITH_KNOTS('',3,(#120380,#120381,#120382,#120383,
#120384,#120385,#120386,#120387,#120388,#120389),.UNSPECIFIED.,.F.,.F.,
(4,3,3,4),(0.487259899830092,0.497067957473563,0.5,0.504719756176228),
 .UNSPECIFIED.);
#22448=B_SPLINE_CURVE_WITH_KNOTS('',3,(#120398,#120399,#120400,#120401,
#120402,#120403,#120404,#120405,#120406,#120407),.UNSPECIFIED.,.F.,.F.,
(4,3,3,4),(2.04923360970009E-14,8.70313176284759E-5,0.000170023930120259,
0.000253018980880619),.UNSPECIFIED.);
#22449=B_SPLINE_CURVE_WITH_KNOTS('',3,(#120418,#120419,#120420,#120421,
#120422,#120423,#120424,#120425,#120426,#120427),.UNSPECIFIED.,.F.,.F.,
(4,3,3,4),(0.487259899843493,0.497067955675083,0.5,0.504719756176228),
 .UNSPECIFIED.);
#22450=B_SPLINE_CURVE_WITH_KNOTS('',3,(#120436,#120437,#120438,#120439,
#120440,#120441,#120442,#120443,#120444,#120445),.UNSPECIFIED.,.F.,.F.,
(4,3,3,4),(1.46986958788117E-14,8.7031317872638E-5,0.000170023930227489,
0.000253018980856544),.UNSPECIFIED.);
#22451=B_SPLINE_CURVE_WITH_KNOTS('',3,(#120456,#120457,#120458,#120459,
#120460,#120461,#120462,#120463,#120464,#120465),.UNSPECIFIED.,.F.,.F.,
(4,3,3,4),(0.487259899836764,0.497067953025495,0.5,0.504719756176228),
 .UNSPECIFIED.);
#22452=B_SPLINE_CURVE_WITH_KNOTS('',3,(#120474,#120475,#120476,#120477,
#120478,#120479,#120480,#120481,#120482,#120483),.UNSPECIFIED.,.F.,.F.,
(4,3,3,4),(2.60369811470792E-14,8.70313175752751E-5,0.000170023930220742,
0.000253018981334628),.UNSPECIFIED.);
#22453=B_SPLINE_CURVE_WITH_KNOTS('',3,(#120494,#120495,#120496,#120497,
#120498,#120499,#120500,#120501,#120502,#120503),.UNSPECIFIED.,.F.,.F.,
(4,3,3,4),(0.487259899825349,0.497067954507092,0.5,0.504719756176228),
 .UNSPECIFIED.);
#22454=B_SPLINE_CURVE_WITH_KNOTS('',3,(#120512,#120513,#120514,#120515,
#120516,#120517,#120518,#120519,#120520,#120521),.UNSPECIFIED.,.F.,.F.,
(4,3,3,4),(4.69113067077989E-15,8.7031317644139E-5,0.000170023930301228,
0.000253018981429277),.UNSPECIFIED.);
#22455=B_SPLINE_CURVE_WITH_KNOTS('',3,(#120532,#120533,#120534,#120535,
#120536,#120537,#120538,#120539,#120540,#120541),.UNSPECIFIED.,.F.,.F.,
(4,3,3,4),(0.487259899844095,0.497067955819474,0.5,0.50471975617627),
 .UNSPECIFIED.);
#22456=B_SPLINE_CURVE_WITH_KNOTS('',3,(#120550,#120551,#120552,#120553,
#120554,#120555,#120556,#120557,#120558,#120559),.UNSPECIFIED.,.F.,.F.,
(4,3,3,4),(3.4930305600279E-14,8.70313175915354E-5,0.000170023930262545,
0.000253018983021755),.UNSPECIFIED.);
#22457=B_SPLINE_CURVE_WITH_KNOTS('',3,(#120570,#120571,#120572,#120573,
#120574,#120575,#120576,#120577,#120578,#120579),.UNSPECIFIED.,.F.,.F.,
(4,3,3,4),(0.487259899834473,0.497067957474287,0.5,0.504719756169005),
 .UNSPECIFIED.);
#22458=B_SPLINE_CURVE_WITH_KNOTS('',3,(#120588,#120589,#120590,#120591,
#120592,#120593,#120594,#120595,#120596,#120597),.UNSPECIFIED.,.F.,.F.,
(4,3,3,4),(4.37878311359043E-14,8.70313175424253E-5,0.000170023930052117,
0.00025301898111264),.UNSPECIFIED.);
#22459=B_SPLINE_CURVE_WITH_KNOTS('',3,(#120608,#120609,#120610,#120611,
#120612,#120613,#120614,#120615,#120616,#120617),.UNSPECIFIED.,.F.,.F.,
(4,3,3,4),(0.48725989983526,0.497067953412607,0.5,0.504719756176228),
 .UNSPECIFIED.);
#22460=B_SPLINE_CURVE_WITH_KNOTS('',3,(#120626,#120627,#120628,#120629,
#120630,#120631,#120632,#120633,#120634,#120635),.UNSPECIFIED.,.F.,.F.,
(4,3,3,4),(4.39618627902034E-14,8.70313175297401E-5,0.00017002392999475,
0.000253018980685548),.UNSPECIFIED.);
#22461=B_SPLINE_CURVE_WITH_KNOTS('',3,(#120646,#120647,#120648,#120649,
#120650,#120651,#120652,#120653,#120654,#120655),.UNSPECIFIED.,.F.,.F.,
(4,3,3,4),(0.487259899838253,0.497067957395083,0.5,0.504719756176302),
 .UNSPECIFIED.);
#22462=B_SPLINE_CURVE_WITH_KNOTS('',3,(#120664,#120665,#120666,#120667,
#120668,#120669,#120670,#120671,#120672,#120673),.UNSPECIFIED.,.F.,.F.,
(4,3,3,4),(3.42316589032284E-14,8.70313175711171E-5,0.000170023930344364,
0.00025301898162994),.UNSPECIFIED.);
#22463=B_SPLINE_CURVE_WITH_KNOTS('',3,(#120684,#120685,#120686,#120687,
#120688,#120689,#120690,#120691,#120692,#120693),.UNSPECIFIED.,.F.,.F.,
(4,3,3,4),(0.487259899828096,0.497067950830241,0.5,0.504719756176228),
 .UNSPECIFIED.);
#22464=B_SPLINE_CURVE_WITH_KNOTS('',3,(#120702,#120703,#120704,#120705,
#120706,#120707,#120708,#120709,#120710,#120711),.UNSPECIFIED.,.F.,.F.,
(4,3,3,4),(2.21213965425014E-14,8.7031317560607E-5,0.000170023930173682,
0.000253018981224706),.UNSPECIFIED.);
#22465=B_SPLINE_CURVE_WITH_KNOTS('',3,(#120722,#120723,#120724,#120725,
#120726,#120727,#120728,#120729,#120730,#120731),.UNSPECIFIED.,.F.,.F.,
(4,3,3,4),(0.48725989985259,0.49706793422622,0.5,0.504719756176227),
 .UNSPECIFIED.);
#22466=B_SPLINE_CURVE_WITH_KNOTS('',3,(#120742,#120743,#120744,#120745,
#120746,#120747),.UNSPECIFIED.,.F.,.F.,(4,2,4),(-0.025296973443844,-0.0126483645724683,
0.),.UNSPECIFIED.);
#22467=B_SPLINE_CURVE_WITH_KNOTS('',3,(#120764,#120765,#120766,#120767,
#120768,#120769,#120770),.UNSPECIFIED.,.F.,.F.,(4,3,4),(0.280433082999158,
0.285714285714286,0.292621536168419),.UNSPECIFIED.);
#22468=B_SPLINE_CURVE_WITH_KNOTS('',3,(#120771,#120772,#120773,#120774,
#120775,#120776),.UNSPECIFIED.,.F.,.F.,(4,2,4),(0.,0.0126482240284275,0.0252963923636814),
 .UNSPECIFIED.);
#22469=B_SPLINE_CURVE_WITH_KNOTS('',3,(#120807,#120808,#120809,#120810,
#120811,#120812,#120813),.UNSPECIFIED.,.F.,.F.,(4,3,4),(0.280433082999159,
0.285714285714286,0.292621536173129),.UNSPECIFIED.);
#22470=B_SPLINE_CURVE_WITH_KNOTS('',3,(#120814,#120815,#120816,#120817,
#120818,#120819),.UNSPECIFIED.,.F.,.F.,(4,2,4),(0.,0.0126482072034737,0.0252962990115169),
 .UNSPECIFIED.);
#22471=B_SPLINE_CURVE_WITH_KNOTS('',3,(#120850,#120851,#120852,#120853,
#120854,#120855,#120856),.UNSPECIFIED.,.F.,.F.,(4,3,4),(0.280433082999158,
0.285714285714286,0.292621536172136),.UNSPECIFIED.);
#22472=B_SPLINE_CURVE_WITH_KNOTS('',3,(#120857,#120858,#120859,#120860,
#120861,#120862),.UNSPECIFIED.,.F.,.F.,(4,2,4),(0.,0.0126483645169886,0.025296944392472),
 .UNSPECIFIED.);
#22473=B_SPLINE_CURVE_WITH_KNOTS('',3,(#120893,#120894,#120895,#120896,
#120897,#120898,#120899),.UNSPECIFIED.,.F.,.F.,(4,3,4),(0.280433083101589,
0.285714285714286,0.292621536174457),.UNSPECIFIED.);
#22474=B_SPLINE_CURVE_WITH_KNOTS('',3,(#120900,#120901,#120902,#120903,
#120904,#120905),.UNSPECIFIED.,.F.,.F.,(4,2,4),(0.,0.0126483645307332,0.0252969476147786),
 .UNSPECIFIED.);
#22475=B_SPLINE_CURVE_WITH_KNOTS('',3,(#120936,#120937,#120938,#120939,
#120940,#120941,#120942),.UNSPECIFIED.,.F.,.F.,(4,3,4),(0.280433082999175,
0.285714285714286,0.292621536174032),.UNSPECIFIED.);
#22476=B_SPLINE_CURVE_WITH_KNOTS('',3,(#120943,#120944,#120945,#120946,
#120947,#120948),.UNSPECIFIED.,.F.,.F.,(4,2,4),(0.,0.0126482419654942,0.0252964414925125),
 .UNSPECIFIED.);
#22477=B_SPLINE_CURVE_WITH_KNOTS('',3,(#120979,#120980,#120981,#120982,
#120983,#120984,#120985),.UNSPECIFIED.,.F.,.F.,(4,3,4),(0.280433082999174,
0.285714285714286,0.292621536173361),.UNSPECIFIED.);
#22478=B_SPLINE_CURVE_WITH_KNOTS('',3,(#120986,#120987,#120988,#120989,
#120990,#120991),.UNSPECIFIED.,.F.,.F.,(4,2,4),(0.,0.0126482228971245,0.0252963611714074),
 .UNSPECIFIED.);
#22479=B_SPLINE_CURVE_WITH_KNOTS('',3,(#121020,#121021,#121022,#121023,
#121024,#121025),.UNSPECIFIED.,.F.,.F.,(4,2,4),(0.,0.0126483645137511,0.02529697344602),
 .UNSPECIFIED.);
#22480=B_SPLINE_CURVE_WITH_KNOTS('',3,(#121050,#121051,#121052,#121053,
#121054,#121055,#121056),.UNSPECIFIED.,.F.,.F.,(4,3,4),(0.280433082999157,
0.285714285714286,0.29262153617651),.UNSPECIFIED.);
#22481=B_SPLINE_CURVE_WITH_KNOTS('',3,(#121057,#121058,#121059,#121060,
#121061,#121062),.UNSPECIFIED.,.F.,.F.,(4,2,4),(0.,0.0126482295569889,0.025296415324654),
 .UNSPECIFIED.);
#22482=B_SPLINE_CURVE_WITH_KNOTS('',3,(#121093,#121094,#121095,#121096,
#121097,#121098,#121099),.UNSPECIFIED.,.F.,.F.,(4,3,4),(0.280433082999157,
0.285714285714286,0.292621536168029),.UNSPECIFIED.);
#22483=B_SPLINE_CURVE_WITH_KNOTS('',3,(#121100,#121101,#121102,#121103,
#121104,#121105),.UNSPECIFIED.,.F.,.F.,(4,2,4),(0.,0.0126482304749268,0.0252963910036341),
 .UNSPECIFIED.);
#22484=B_SPLINE_CURVE_WITH_KNOTS('',3,(#121136,#121137,#121138,#121139,
#121140,#121141,#121142),.UNSPECIFIED.,.F.,.F.,(4,3,4),(0.280433082999158,
0.285714285714286,0.292621536177272),.UNSPECIFIED.);
#22485=B_SPLINE_CURVE_WITH_KNOTS('',3,(#121143,#121144,#121145,#121146,
#121147,#121148),.UNSPECIFIED.,.F.,.F.,(4,2,4),(0.,0.0126482262354878,0.0252964015583787),
 .UNSPECIFIED.);
#22486=B_SPLINE_CURVE_WITH_KNOTS('',3,(#121179,#121180,#121181,#121182,
#121183,#121184,#121185),.UNSPECIFIED.,.F.,.F.,(4,3,4),(0.280433082999159,
0.285714285714286,0.292621536173701),.UNSPECIFIED.);
#22487=B_SPLINE_CURVE_WITH_KNOTS('',3,(#121186,#121187,#121188,#121189,
#121190,#121191),.UNSPECIFIED.,.F.,.F.,(4,2,4),(0.,0.0126482164487877,0.0252963341335591),
 .UNSPECIFIED.);
#22488=B_SPLINE_CURVE_WITH_KNOTS('',3,(#121222,#121223,#121224,#121225,
#121226,#121227,#121228),.UNSPECIFIED.,.F.,.F.,(4,3,4),(0.280433082999158,
0.285714285714286,0.292621536174503),.UNSPECIFIED.);
#22489=B_SPLINE_CURVE_WITH_KNOTS('',3,(#121229,#121230,#121231,#121232,
#121233,#121234),.UNSPECIFIED.,.F.,.F.,(4,2,4),(0.,0.0126482283807774,0.0252963831989578),
 .UNSPECIFIED.);
#22490=B_SPLINE_CURVE_WITH_KNOTS('',3,(#121265,#121266,#121267,#121268,
#121269,#121270,#121271),.UNSPECIFIED.,.F.,.F.,(4,3,4),(0.280433083100916,
0.285714285714286,0.292621536173779),.UNSPECIFIED.);
#22491=B_SPLINE_CURVE_WITH_KNOTS('',3,(#121272,#121273,#121274,#121275,
#121276,#121277),.UNSPECIFIED.,.F.,.F.,(4,2,4),(0.,0.0126482384135485,0.025296451907903),
 .UNSPECIFIED.);
#22492=B_SPLINE_CURVE_WITH_KNOTS('',3,(#121308,#121309,#121310,#121311,
#121312,#121313,#121314),.UNSPECIFIED.,.F.,.F.,(4,3,4),(0.280433082999158,
0.285714285714286,0.292621536171013),.UNSPECIFIED.);
#22493=B_SPLINE_CURVE_WITH_KNOTS('',3,(#121315,#121316,#121317,#121318,
#121319,#121320),.UNSPECIFIED.,.F.,.F.,(4,2,4),(0.,0.0126482186825741,0.0252963434366669),
 .UNSPECIFIED.);
#22494=B_SPLINE_CURVE_WITH_KNOTS('',3,(#121351,#121352,#121353,#121354,
#121355,#121356,#121357),.UNSPECIFIED.,.F.,.F.,(4,3,4),(0.280433082999157,
0.285714285714286,0.292621536174076),.UNSPECIFIED.);
#22495=B_SPLINE_CURVE_WITH_KNOTS('',3,(#121358,#121359,#121360,#121361,
#121362,#121363),.UNSPECIFIED.,.F.,.F.,(4,2,4),(0.,0.012648236612633,0.0252964210419331),
 .UNSPECIFIED.);
#22496=B_SPLINE_CURVE_WITH_KNOTS('',3,(#121394,#121395,#121396,#121397,
#121398,#121399,#121400),.UNSPECIFIED.,.F.,.F.,(4,3,4),(0.280433082999157,
0.285714285714286,0.292621536176529),.UNSPECIFIED.);
#22497=B_SPLINE_CURVE_WITH_KNOTS('',3,(#121401,#121402,#121403,#121404,
#121405,#121406),.UNSPECIFIED.,.F.,.F.,(4,2,4),(0.,0.0126482376119629,0.0252964485949374),
 .UNSPECIFIED.);
#22498=B_SPLINE_CURVE_WITH_KNOTS('',3,(#121437,#121438,#121439,#121440,
#121441,#121442,#121443),.UNSPECIFIED.,.F.,.F.,(4,3,4),(0.280433082999158,
0.285714285714286,0.292621536169643),.UNSPECIFIED.);
#22499=B_SPLINE_CURVE_WITH_KNOTS('',3,(#121444,#121445,#121446,#121447,
#121448,#121449),.UNSPECIFIED.,.F.,.F.,(4,2,4),(0.,0.0126482392731302,0.025296427401708),
 .UNSPECIFIED.);
#22500=B_SPLINE_CURVE_WITH_KNOTS('',3,(#121480,#121481,#121482,#121483,
#121484,#121485,#121486),.UNSPECIFIED.,.F.,.F.,(4,3,4),(0.280433082999157,
0.285714285714286,0.292621536170285),.UNSPECIFIED.);
#22501=B_SPLINE_CURVE_WITH_KNOTS('',3,(#121487,#121488,#121489,#121490,
#121491,#121492),.UNSPECIFIED.,.F.,.F.,(4,2,4),(0.,0.0126482325288649,0.0252964275932703),
 .UNSPECIFIED.);
#22502=B_SPLINE_CURVE_WITH_KNOTS('',3,(#121523,#121524,#121525,#121526,
#121527,#121528,#121529),.UNSPECIFIED.,.F.,.F.,(4,3,4),(0.280433082999157,
0.285714285714286,0.292621536172335),.UNSPECIFIED.);
#22503=B_SPLINE_CURVE_WITH_KNOTS('',3,(#121530,#121531,#121532,#121533,
#121534,#121535),.UNSPECIFIED.,.F.,.F.,(4,2,4),(0.,0.0126482279436222,0.0252963817618714),
 .UNSPECIFIED.);
#22504=B_SPLINE_CURVE_WITH_KNOTS('',3,(#121566,#121567,#121568,#121569,
#121570,#121571,#121572),.UNSPECIFIED.,.F.,.F.,(4,3,4),(0.280433082999181,
0.285714285714286,0.292621536171598),.UNSPECIFIED.);
#22505=B_SPLINE_CURVE_WITH_KNOTS('',3,(#121573,#121574,#121575,#121576,
#121577,#121578),.UNSPECIFIED.,.F.,.F.,(4,2,4),(0.,0.0126482391688131,0.0252964280773304),
 .UNSPECIFIED.);
#22506=B_SPLINE_CURVE_WITH_KNOTS('',3,(#121609,#121610,#121611,#121612,
#121613,#121614,#121615),.UNSPECIFIED.,.F.,.F.,(4,3,4),(0.280433082999157,
0.285714285714286,0.29262153616907),.UNSPECIFIED.);
#22507=B_SPLINE_CURVE_WITH_KNOTS('',3,(#121616,#121617,#121618,#121619,
#121620,#121621),.UNSPECIFIED.,.F.,.F.,(4,2,4),(0.,0.0126482300329072,0.0252964171687196),
 .UNSPECIFIED.);
#22508=B_SPLINE_CURVE_WITH_KNOTS('',3,(#121652,#121653,#121654,#121655,
#121656,#121657,#121658),.UNSPECIFIED.,.F.,.F.,(4,3,4),(0.280433082999157,
0.285714285714286,0.292621536200935),.UNSPECIFIED.);
#22509=B_SPLINE_CURVE_WITH_KNOTS('',3,(#121659,#121660,#121661,#121662,
#121663,#121664),.UNSPECIFIED.,.F.,.F.,(4,2,4),(0.,0.012648227663072,0.0252962420019202),
 .UNSPECIFIED.);
#22510=B_SPLINE_CURVE_WITH_KNOTS('',3,(#121696,#121697,#121698,#121699,
#121700,#121701,#121702),.UNSPECIFIED.,.F.,.F.,(4,3,4),(0.280433082999157,
0.285714285714286,0.292621536180055),.UNSPECIFIED.);
#22511=B_SPLINE_CURVE_WITH_KNOTS('',3,(#121703,#121704,#121705,#121706,
#121707,#121708),.UNSPECIFIED.,.F.,.F.,(4,2,4),(0.,0.0126482209953414,0.0252963798315834),
 .UNSPECIFIED.);
#22512=B_SPLINE_CURVE_WITH_KNOTS('',3,(#121738,#121739,#121740,#121741,
#121742,#121743,#121744),.UNSPECIFIED.,.F.,.F.,(4,3,4),(0.280433082999159,
0.285714285714286,0.292621536173583),.UNSPECIFIED.);
#22513=B_SPLINE_CURVE_WITH_KNOTS('',3,(#121745,#121746,#121747,#121748,
#121749,#121750),.UNSPECIFIED.,.F.,.F.,(4,2,4),(0.,0.0126483644971886,0.025296973432917),
 .UNSPECIFIED.);
#22514=B_SPLINE_CURVE_WITH_KNOTS('',3,(#121781,#121782,#121783,#121784,
#121785,#121786,#121787),.UNSPECIFIED.,.F.,.F.,(4,3,4),(0.28043308299918,
0.285714285714286,0.292621536175091),.UNSPECIFIED.);
#22515=B_SPLINE_CURVE_WITH_KNOTS('',3,(#121788,#121789,#121790,#121791,
#121792,#121793),.UNSPECIFIED.,.F.,.F.,(4,2,4),(0.,0.0126482219417105,0.0252963558424426),
 .UNSPECIFIED.);
#22516=B_SPLINE_CURVE_WITH_KNOTS('',3,(#121824,#121825,#121826,#121827,
#121828,#121829,#121830),.UNSPECIFIED.,.F.,.F.,(4,3,4),(0.280433082999174,
0.285714285714286,0.292621536175529),.UNSPECIFIED.);
#22517=B_SPLINE_CURVE_WITH_KNOTS('',3,(#121831,#121832,#121833,#121834,
#121835,#121836),.UNSPECIFIED.,.F.,.F.,(4,2,4),(0.,0.0126482161227793,0.025296332460369),
 .UNSPECIFIED.);
#22518=B_SPLINE_CURVE_WITH_KNOTS('',3,(#121867,#121868,#121869,#121870,
#121871,#121872,#121873),.UNSPECIFIED.,.F.,.F.,(4,3,4),(0.28043308310138,
0.285714285714286,0.29262153617452),.UNSPECIFIED.);
#22519=B_SPLINE_CURVE_WITH_KNOTS('',3,(#121874,#121875,#121876,#121877,
#121878,#121879),.UNSPECIFIED.,.F.,.F.,(4,2,4),(0.,0.0126482098067578,0.0252963055994983),
 .UNSPECIFIED.);
#22520=B_SPLINE_CURVE_WITH_KNOTS('',3,(#121910,#121911,#121912,#121913,
#121914,#121915,#121916),.UNSPECIFIED.,.F.,.F.,(4,3,4),(0.280433082999171,
0.285714285714286,0.292621536166647),.UNSPECIFIED.);
#22521=B_SPLINE_CURVE_WITH_KNOTS('',3,(#121917,#121918,#121919,#121920,
#121921,#121922),.UNSPECIFIED.,.F.,.F.,(4,2,4),(0.,0.0126482038455709,0.0252963088950863),
 .UNSPECIFIED.);
#22522=B_SPLINE_CURVE_WITH_KNOTS('',3,(#121942,#121943,#121944,#121945,
#121946,#121947,#121948),.UNSPECIFIED.,.F.,.F.,(4,3,4),(0.280433082999158,
0.285714285714286,0.292621536174994),.UNSPECIFIED.);
#22523=B_SPLINE_CURVE_WITH_KNOTS('',3,(#121971,#121972,#121973,#121974,
#121975,#121976),.UNSPECIFIED.,.F.,.F.,(4,2,4),(5.6486889799842E-11,0.0126507152822395,
0.0253011859160019),.UNSPECIFIED.);
#22524=B_SPLINE_CURVE_WITH_KNOTS('',3,(#121993,#121994,#121995,#121996,
#121997,#121998,#121999),.UNSPECIFIED.,.F.,.F.,(4,3,4),(0.487155140750429,
0.491874896926655,0.499350532547867),.UNSPECIFIED.);
#22525=B_SPLINE_CURVE_WITH_KNOTS('',3,(#122000,#122001,#122002,#122003,
#122004,#122005),.UNSPECIFIED.,.F.,.F.,(4,2,4),(-0.0253011697080569,-0.0126507154103212,
-1.97071942098503E-11),.UNSPECIFIED.);
#22526=B_SPLINE_CURVE_WITH_KNOTS('',3,(#122032,#122033,#122034,#122035,
#122036,#122037,#122038),.UNSPECIFIED.,.F.,.F.,(4,3,4),(0.487155140750429,
0.491874896926656,0.499350532544037),.UNSPECIFIED.);
#22527=B_SPLINE_CURVE_WITH_KNOTS('',3,(#122039,#122040,#122041,#122042,
#122043,#122044),.UNSPECIFIED.,.F.,.F.,(4,2,4),(-0.0253011722932434,-0.0126507154307367,
-1.9720863830841E-11),.UNSPECIFIED.);
#22528=B_SPLINE_CURVE_WITH_KNOTS('',3,(#122071,#122072,#122073,#122074,
#122075,#122076,#122077),.UNSPECIFIED.,.F.,.F.,(4,3,4),(0.487155140750429,
0.491874896926656,0.49935053256116),.UNSPECIFIED.);
#22529=B_SPLINE_CURVE_WITH_KNOTS('',3,(#122078,#122079,#122080,#122081,
#122082,#122083),.UNSPECIFIED.,.F.,.F.,(4,2,4),(-0.0253011660901163,-0.0126507154029974,
-1.91734475518679E-11),.UNSPECIFIED.);
#22530=B_SPLINE_CURVE_WITH_KNOTS('',3,(#122110,#122111,#122112,#122113,
#122114,#122115,#122116),.UNSPECIFIED.,.F.,.F.,(4,3,4),(0.487155140750429,
0.491874896926656,0.499350532539288),.UNSPECIFIED.);
#22531=B_SPLINE_CURVE_WITH_KNOTS('',3,(#122117,#122118,#122119,#122120,
#122121,#122122),.UNSPECIFIED.,.F.,.F.,(4,2,4),(-0.0253011685668152,-0.0126507154315906,
-2.02164084084355E-11),.UNSPECIFIED.);
#22532=B_SPLINE_CURVE_WITH_KNOTS('',3,(#122149,#122150,#122151,#122152,
#122153,#122154,#122155),.UNSPECIFIED.,.F.,.F.,(4,3,4),(0.487155140750429,
0.491874896926656,0.499350532553138),.UNSPECIFIED.);
#22533=B_SPLINE_CURVE_WITH_KNOTS('',3,(#122156,#122157,#122158,#122159,
#122160,#122161),.UNSPECIFIED.,.F.,.F.,(4,2,4),(-0.0253011700469523,-0.0126507154194713,
-1.94551180721092E-11),.UNSPECIFIED.);
#22534=B_SPLINE_CURVE_WITH_KNOTS('',3,(#122188,#122189,#122190,#122191,
#122192,#122193,#122194),.UNSPECIFIED.,.F.,.F.,(4,3,4),(0.487155140750429,
0.491874896926655,0.499350532552386),.UNSPECIFIED.);
#22535=B_SPLINE_CURVE_WITH_KNOTS('',3,(#122195,#122196,#122197,#122198,
#122199,#122200),.UNSPECIFIED.,.F.,.F.,(4,2,4),(-0.0253011664286715,-0.0126507154206639,
-1.996768375645E-11),.UNSPECIFIED.);
#22536=B_SPLINE_CURVE_WITH_KNOTS('',3,(#122227,#122228,#122229,#122230,
#122231,#122232,#122233),.UNSPECIFIED.,.F.,.F.,(4,3,4),(0.48715514075043,
0.491874896926657,0.499350532549246),.UNSPECIFIED.);
#22537=B_SPLINE_CURVE_WITH_KNOTS('',3,(#122234,#122235,#122236,#122237,
#122238,#122239),.UNSPECIFIED.,.F.,.F.,(4,2,4),(-0.0253011651441201,-0.0126507153978601,
-1.92457993986039E-11),.UNSPECIFIED.);
#22538=B_SPLINE_CURVE_WITH_KNOTS('',3,(#122266,#122267,#122268,#122269,
#122270,#122271,#122272),.UNSPECIFIED.,.F.,.F.,(4,3,4),(0.48715514075043,
0.491874896926658,0.499350532543253),.UNSPECIFIED.);
#22539=B_SPLINE_CURVE_WITH_KNOTS('',3,(#122273,#122274,#122275,#122276,
#122277,#122278),.UNSPECIFIED.,.F.,.F.,(4,2,4),(-0.0253011651017512,-0.0126507154393088,
-2.06919863188215E-11),.UNSPECIFIED.);
#22540=B_SPLINE_CURVE_WITH_KNOTS('',3,(#122305,#122306,#122307,#122308,
#122309,#122310,#122311),.UNSPECIFIED.,.F.,.F.,(4,3,4),(0.48715514075043,
0.491874896926658,0.499350532556912),.UNSPECIFIED.);
#22541=B_SPLINE_CURVE_WITH_KNOTS('',3,(#122312,#122313,#122314,#122315,
#122316,#122317),.UNSPECIFIED.,.F.,.F.,(4,2,4),(-0.0253011716954516,-0.0126507154317354,
-1.93546428883806E-11),.UNSPECIFIED.);
#22542=B_SPLINE_CURVE_WITH_KNOTS('',3,(#122344,#122345,#122346,#122347,
#122348,#122349,#122350),.UNSPECIFIED.,.F.,.F.,(4,3,4),(0.48715514075043,
0.491874896926658,0.499350532547458),.UNSPECIFIED.);
#22543=B_SPLINE_CURVE_WITH_KNOTS('',3,(#122351,#122352,#122353,#122354,
#122355,#122356),.UNSPECIFIED.,.F.,.F.,(4,2,4),(-0.0253011677574891,-0.0126507153846773,
-1.91839218122158E-11),.UNSPECIFIED.);
#22544=B_SPLINE_CURVE_WITH_KNOTS('',3,(#122383,#122384,#122385,#122386,
#122387,#122388,#122389),.UNSPECIFIED.,.F.,.F.,(4,3,4),(0.48715514075043,
0.491874896926658,0.499350532553758),.UNSPECIFIED.);
#22545=B_SPLINE_CURVE_WITH_KNOTS('',3,(#122390,#122391,#122392,#122393,
#122394,#122395),.UNSPECIFIED.,.F.,.F.,(4,2,4),(-0.0253011737432215,-0.0126507154147995,
-1.93375662704831E-11),.UNSPECIFIED.);
#22546=B_SPLINE_CURVE_WITH_KNOTS('',3,(#122422,#122423,#122424,#122425,
#122426,#122427,#122428),.UNSPECIFIED.,.F.,.F.,(4,3,4),(0.48715514075043,
0.491874896926658,0.499350532548837),.UNSPECIFIED.);
#22547=B_SPLINE_CURVE_WITH_KNOTS('',3,(#122429,#122430,#122431,#122432,
#122433,#122434),.UNSPECIFIED.,.F.,.F.,(4,2,4),(-0.0253011673355543,-0.0126507154295212,
-1.97535911239388E-11),.UNSPECIFIED.);
#22548=B_SPLINE_CURVE_WITH_KNOTS('',3,(#122461,#122462,#122463,#122464,
#122465,#122466,#122467),.UNSPECIFIED.,.F.,.F.,(4,3,4),(0.48715514075043,
0.491874896926658,0.499350532552698),.UNSPECIFIED.);
#22549=B_SPLINE_CURVE_WITH_KNOTS('',3,(#122468,#122469,#122470,#122471,
#122472,#122473),.UNSPECIFIED.,.F.,.F.,(4,2,4),(-0.0253011661288702,-0.0126507154045511,
-1.98644260762659E-11),.UNSPECIFIED.);
#22550=B_SPLINE_CURVE_WITH_KNOTS('',3,(#122498,#122499,#122500,#122501,
#122502,#122503),.UNSPECIFIED.,.F.,.F.,(4,2,4),(-0.0253011704521776,-0.0126507154221742,
0.),.UNSPECIFIED.);
#22551=B_SPLINE_CURVE_WITH_KNOTS('',3,(#122524,#122525,#122526,#122527,
#122528,#122529,#122530),.UNSPECIFIED.,.F.,.F.,(4,3,4),(0.48715514075043,
0.491874896926658,0.499350532549079),.UNSPECIFIED.);
#22552=B_SPLINE_CURVE_WITH_KNOTS('',3,(#122531,#122532,#122533,#122534,
#122535,#122536),.UNSPECIFIED.,.F.,.F.,(4,2,4),(-0.0253011669290482,-0.0126507153766242,
-1.8918901167897E-11),.UNSPECIFIED.);
#22553=B_SPLINE_CURVE_WITH_KNOTS('',3,(#122563,#122564,#122565,#122566,
#122567,#122568,#122569),.UNSPECIFIED.,.F.,.F.,(4,3,4),(0.48715514075043,
0.49187489692666,0.499350532564458),.UNSPECIFIED.);
#22554=B_SPLINE_CURVE_WITH_KNOTS('',3,(#122570,#122571,#122572,#122573,
#122574,#122575),.UNSPECIFIED.,.F.,.F.,(4,2,4),(-0.0253011658638423,-0.0126507154016559,
-1.91625708356735E-11),.UNSPECIFIED.);
#22555=B_SPLINE_CURVE_WITH_KNOTS('',3,(#122602,#122603,#122604,#122605,
#122606,#122607,#122608),.UNSPECIFIED.,.F.,.F.,(4,3,4),(0.48715514075043,
0.491874896926658,0.499350532549946),.UNSPECIFIED.);
#22556=B_SPLINE_CURVE_WITH_KNOTS('',3,(#122609,#122610,#122611,#122612,
#122613,#122614),.UNSPECIFIED.,.F.,.F.,(4,2,4),(-0.0253011702441171,-0.0126507154203099,
-1.94096856642734E-11),.UNSPECIFIED.);
#22557=B_SPLINE_CURVE_WITH_KNOTS('',3,(#122641,#122642,#122643,#122644,
#122645,#122646,#122647),.UNSPECIFIED.,.F.,.F.,(4,3,4),(0.48715514075043,
0.491874896926658,0.499350532550294),.UNSPECIFIED.);
#22558=B_SPLINE_CURVE_WITH_KNOTS('',3,(#122648,#122649,#122650,#122651,
#122652,#122653),.UNSPECIFIED.,.F.,.F.,(4,2,4),(-0.0253011727064749,-0.0126507154429837,
-1.9765349079659E-11),.UNSPECIFIED.);
#22559=B_SPLINE_CURVE_WITH_KNOTS('',3,(#122680,#122681,#122682,#122683,
#122684,#122685,#122686),.UNSPECIFIED.,.F.,.F.,(4,3,4),(0.48715514075043,
0.491874896926657,0.499350532550754),.UNSPECIFIED.);
#22560=B_SPLINE_CURVE_WITH_KNOTS('',3,(#122687,#122688,#122689,#122690,
#122691,#122692),.UNSPECIFIED.,.F.,.F.,(4,2,4),(-0.0253011673119558,-0.0126507154173595,
-1.93358315470071E-11),.UNSPECIFIED.);
#22561=B_SPLINE_CURVE_WITH_KNOTS('',3,(#122719,#122720,#122721,#122722,
#122723,#122724,#122725),.UNSPECIFIED.,.F.,.F.,(4,3,4),(0.48715514075043,
0.491874896926658,0.499350532545838),.UNSPECIFIED.);
#22562=B_SPLINE_CURVE_WITH_KNOTS('',3,(#122726,#122727,#122728,#122729,
#122730,#122731),.UNSPECIFIED.,.F.,.F.,(4,2,4),(-0.0253011657593956,-0.0126507154253452,
-2.02232536272717E-11),.UNSPECIFIED.);
#22563=B_SPLINE_CURVE_WITH_KNOTS('',3,(#122758,#122759,#122760,#122761,
#122762,#122763,#122764),.UNSPECIFIED.,.F.,.F.,(4,3,4),(0.48715514075043,
0.491874896926658,0.49935053255401),.UNSPECIFIED.);
#22564=B_SPLINE_CURVE_WITH_KNOTS('',3,(#122765,#122766,#122767,#122768,
#122769,#122770),.UNSPECIFIED.,.F.,.F.,(4,2,4),(-0.0253011655833842,-0.0126507154013209,
-1.94681874787772E-11),.UNSPECIFIED.);
#22565=B_SPLINE_CURVE_WITH_KNOTS('',3,(#122797,#122798,#122799,#122800,
#122801,#122802,#122803),.UNSPECIFIED.,.F.,.F.,(4,3,4),(0.48715514075043,
0.491874896926658,0.499350532553005),.UNSPECIFIED.);
#22566=B_SPLINE_CURVE_WITH_KNOTS('',3,(#122804,#122805,#122806,#122807,
#122808,#122809),.UNSPECIFIED.,.F.,.F.,(4,2,4),(-0.0253011660469114,-0.0126507153993854,
-1.99408337064888E-11),.UNSPECIFIED.);
#22567=B_SPLINE_CURVE_WITH_KNOTS('',3,(#122836,#122837,#122838,#122839,
#122840,#122841,#122842),.UNSPECIFIED.,.F.,.F.,(4,3,4),(0.48715514075043,
0.491874896926658,0.499350532550904),.UNSPECIFIED.);
#22568=B_SPLINE_CURVE_WITH_KNOTS('',3,(#122843,#122844,#122845,#122846,
#122847,#122848),.UNSPECIFIED.,.F.,.F.,(4,2,4),(-0.0253011738441044,-0.0126507154351814,
-1.93815970217504E-11),.UNSPECIFIED.);
#22569=B_SPLINE_CURVE_WITH_KNOTS('',3,(#122875,#122876,#122877,#122878,
#122879,#122880,#122881),.UNSPECIFIED.,.F.,.F.,(4,3,4),(0.48715514075043,
0.4918748969267,0.499350532551012),.UNSPECIFIED.);
#22570=B_SPLINE_CURVE_WITH_KNOTS('',3,(#122882,#122883,#122884,#122885,
#122886,#122887),.UNSPECIFIED.,.F.,.F.,(4,2,4),(-0.0253011672758786,-0.0126507154040944,
-1.97396612944267E-11),.UNSPECIFIED.);
#22571=B_SPLINE_CURVE_WITH_KNOTS('',3,(#122914,#122915,#122916,#122917,
#122918,#122919,#122920),.UNSPECIFIED.,.F.,.F.,(4,3,4),(0.48715514075043,
0.491874896926665,0.499350532557549),.UNSPECIFIED.);
#22572=B_SPLINE_CURVE_WITH_KNOTS('',3,(#122921,#122922,#122923,#122924,
#122925,#122926),.UNSPECIFIED.,.F.,.F.,(4,2,4),(-0.0253011654071048,-0.0126507153906956,
-1.85380495676402E-11),.UNSPECIFIED.);
#22573=B_SPLINE_CURVE_WITH_KNOTS('',3,(#122953,#122954,#122955,#122956,
#122957,#122958,#122959),.UNSPECIFIED.,.F.,.F.,(4,3,4),(0.48715514075043,
0.491874896926658,0.499350532557718),.UNSPECIFIED.);
#22574=B_SPLINE_CURVE_WITH_KNOTS('',3,(#122960,#122961,#122962,#122963,
#122964,#122965),.UNSPECIFIED.,.F.,.F.,(4,2,4),(-0.0253011666204797,-0.0126507154156547,
-1.98272821771983E-11),.UNSPECIFIED.);
#22575=B_SPLINE_CURVE_WITH_KNOTS('',3,(#122992,#122993,#122994,#122995,
#122996,#122997,#122998),.UNSPECIFIED.,.F.,.F.,(4,3,4),(0.48715514075043,
0.491874896926732,0.499350532545763),.UNSPECIFIED.);
#22576=B_SPLINE_CURVE_WITH_KNOTS('',3,(#122999,#123000,#123001,#123002,
#123003,#123004),.UNSPECIFIED.,.F.,.F.,(4,2,4),(-0.025301170657439,-0.0126507154100243,
-1.93889730659702E-11),.UNSPECIFIED.);
#22577=B_SPLINE_CURVE_WITH_KNOTS('',3,(#123031,#123032,#123033,#123034,
#123035,#123036,#123037),.UNSPECIFIED.,.F.,.F.,(4,3,4),(0.487155140750422,
0.49187489692665,0.49935053255025),.UNSPECIFIED.);
#22578=B_SPLINE_CURVE_WITH_KNOTS('',3,(#123038,#123039,#123040,#123041,
#123042,#123043),.UNSPECIFIED.,.F.,.F.,(4,2,4),(-0.0253011644296503,-0.0126507153998242,
-1.97393976164584E-11),.UNSPECIFIED.);
#22579=B_SPLINE_CURVE_WITH_KNOTS('',3,(#123059,#123060,#123061,#123062,
#123063,#123064,#123065),.UNSPECIFIED.,.F.,.F.,(4,3,4),(0.487155140750429,
0.491874896926656,0.499350532736371),.UNSPECIFIED.);
#22580=B_SPLINE_CURVE_WITH_KNOTS('',3,(#123088,#123089,#123090,#123091,
#123092,#123093),.UNSPECIFIED.,.F.,.F.,(4,2,4),(-0.025303642668681,-0.0126519393733511,
-4.93077419172483E-11),.UNSPECIFIED.);
#22581=B_SPLINE_CURVE_WITH_KNOTS('',3,(#123106,#123107,#123108,#123109,
#123110,#123111),.UNSPECIFIED.,.F.,.F.,(4,2,4),(5.52409649967746E-11,0.0126519401309947,
0.0253036433584956),.UNSPECIFIED.);
#22582=B_SPLINE_CURVE_WITH_KNOTS('',3,(#123131,#123132,#123133,#123134,
#123135,#123136),.UNSPECIFIED.,.F.,.F.,(4,2,4),(4.64000489761306E-11,0.0126519401026762,
0.0253036433353798),.UNSPECIFIED.);
#22583=B_SPLINE_CURVE_WITH_KNOTS('',3,(#123156,#123157,#123158,#123159,
#123160,#123161),.UNSPECIFIED.,.F.,.F.,(4,2,4),(3.79562095965757E-11,0.0126519401116534,
0.0253036433278902),.UNSPECIFIED.);
#22584=B_SPLINE_CURVE_WITH_KNOTS('',3,(#123181,#123182,#123183,#123184,
#123185,#123186),.UNSPECIFIED.,.F.,.F.,(4,2,4),(4.376061431345E-11,0.0126519401323004,
0.0253036433382299),.UNSPECIFIED.);
#22585=B_SPLINE_CURVE_WITH_KNOTS('',3,(#123206,#123207,#123208,#123209,
#123210,#123211),.UNSPECIFIED.,.F.,.F.,(4,2,4),(3.26183525282446E-11,0.0126519400760263,
0.0253036432997477),.UNSPECIFIED.);
#22586=B_SPLINE_CURVE_WITH_KNOTS('',3,(#123231,#123232,#123233,#123234,
#123235,#123236),.UNSPECIFIED.,.F.,.F.,(4,2,4),(1.78618766070422E-11,0.0126519400801105,
0.0253036432850591),.UNSPECIFIED.);
#22587=B_SPLINE_CURVE_WITH_KNOTS('',3,(#123256,#123257,#123258,#123259,
#123260,#123261),.UNSPECIFIED.,.F.,.F.,(4,2,4),(3.39279843673074E-11,0.012651940111472,
0.0253036433222914),.UNSPECIFIED.);
#22588=B_SPLINE_CURVE_WITH_KNOTS('',3,(#123281,#123282,#123283,#123284,
#123285,#123286),.UNSPECIFIED.,.F.,.F.,(4,2,4),(6.98571819218591E-11,0.0126519401540513,
0.0253036433771993),.UNSPECIFIED.);
#22589=B_SPLINE_CURVE_WITH_KNOTS('',3,(#123306,#123307,#123308,#123309,
#123310,#123311),.UNSPECIFIED.,.F.,.F.,(4,2,4),(3.01248371585428E-11,0.0126519400709428,
0.0253036432886881),.UNSPECIFIED.);
#22590=B_SPLINE_CURVE_WITH_KNOTS('',3,(#123331,#123332,#123333,#123334,
#123335,#123336),.UNSPECIFIED.,.F.,.F.,(4,2,4),(4.97562181263154E-11,0.0126519401134231,
0.0253036433393194),.UNSPECIFIED.);
#22591=B_SPLINE_CURVE_WITH_KNOTS('',3,(#123356,#123357,#123358,#123359,
#123360,#123361),.UNSPECIFIED.,.F.,.F.,(4,2,4),(5.67425406489046E-11,0.0126519401208395,
0.025303643305537),.UNSPECIFIED.);
#22592=B_SPLINE_CURVE_WITH_KNOTS('',3,(#123381,#123382,#123383,#123384,
#123385,#123386),.UNSPECIFIED.,.F.,.F.,(4,2,4),(5.49109704738617E-11,0.01265194014448,
0.0253036433621979),.UNSPECIFIED.);
#22593=B_SPLINE_CURVE_WITH_KNOTS('',3,(#123406,#123407,#123408,#123409,
#123410,#123411),.UNSPECIFIED.,.F.,.F.,(4,2,4),(4.33377220651269E-11,0.0126519400952753,
0.0253036433155586),.UNSPECIFIED.);
#22594=B_SPLINE_CURVE_WITH_KNOTS('',3,(#123431,#123432,#123433,#123434,
#123435,#123436),.UNSPECIFIED.,.F.,.F.,(4,2,4),(7.15206814981132E-11,0.0126519401294615,
0.0253036433132997),.UNSPECIFIED.);
#22595=B_SPLINE_CURVE_WITH_KNOTS('',3,(#123456,#123457,#123458,#123459,
#123460,#123461),.UNSPECIFIED.,.F.,.F.,(4,2,4),(4.56809817642753E-11,0.0126519401030549,
0.0253036433198694),.UNSPECIFIED.);
#22596=B_SPLINE_CURVE_WITH_KNOTS('',3,(#123481,#123482,#123483,#123484,
#123485,#123486),.UNSPECIFIED.,.F.,.F.,(4,2,4),(3.72911203642004E-11,0.0126519400850595,
0.0253036433156901),.UNSPECIFIED.);
#22597=B_SPLINE_CURVE_WITH_KNOTS('',3,(#123506,#123507,#123508,#123509,
#123510,#123511),.UNSPECIFIED.,.F.,.F.,(4,2,4),(3.15364244988512E-11,0.0126519400951044,
0.025303643329179),.UNSPECIFIED.);
#22598=B_SPLINE_CURVE_WITH_KNOTS('',3,(#123531,#123532,#123533,#123534,
#123535,#123536),.UNSPECIFIED.,.F.,.F.,(4,2,4),(2.15246642150142E-11,0.0126519400837596,
0.0253036433411845),.UNSPECIFIED.);
#22599=B_SPLINE_CURVE_WITH_KNOTS('',3,(#123556,#123557,#123558,#123559,
#123560,#123561),.UNSPECIFIED.,.F.,.F.,(4,2,4),(5.25951651961309E-11,0.0126519401235544,
0.0253036433427751),.UNSPECIFIED.);
#22600=B_SPLINE_CURVE_WITH_KNOTS('',3,(#123581,#123582,#123583,#123584,
#123585,#123586),.UNSPECIFIED.,.F.,.F.,(4,2,4),(8.04217133295527E-11,0.012651940139658,
0.0253036433290908),.UNSPECIFIED.);
#22601=B_SPLINE_CURVE_WITH_KNOTS('',3,(#123606,#123607,#123608,#123609,
#123610,#123611),.UNSPECIFIED.,.F.,.F.,(4,2,4),(5.19886781513755E-11,0.0126519401226947,
0.0253036433221645),.UNSPECIFIED.);
#22602=B_SPLINE_CURVE_WITH_KNOTS('',3,(#123631,#123632,#123633,#123634,
#123635,#123636),.UNSPECIFIED.,.F.,.F.,(4,2,4),(2.66805634994813E-11,0.0126519401007409,
0.0253036433160408),.UNSPECIFIED.);
#22603=B_SPLINE_CURVE_WITH_KNOTS('',3,(#123656,#123657,#123658,#123659,
#123660,#123661),.UNSPECIFIED.,.F.,.F.,(4,2,4),(5.55682401312492E-11,0.0126519401226915,
0.0253036433365694),.UNSPECIFIED.);
#22604=B_SPLINE_CURVE_WITH_KNOTS('',3,(#123681,#123682,#123683,#123684,
#123685,#123686),.UNSPECIFIED.,.F.,.F.,(4,2,4),(3.32378535415398E-11,0.012651940098632,
0.0253036433355196),.UNSPECIFIED.);
#22605=B_SPLINE_CURVE_WITH_KNOTS('',3,(#123706,#123707,#123708,#123709,
#123710,#123711),.UNSPECIFIED.,.F.,.F.,(4,2,4),(2.94105947720898E-11,0.012651940101243,
0.0253036433317081),.UNSPECIFIED.);
#22606=B_SPLINE_CURVE_WITH_KNOTS('',3,(#123731,#123732,#123733,#123734,
#123735,#123736),.UNSPECIFIED.,.F.,.F.,(4,2,4),(5.23976660158685E-11,0.0126519400966257,
0.025303643309186),.UNSPECIFIED.);
#22607=B_SPLINE_CURVE_WITH_KNOTS('',3,(#123756,#123757,#123758,#123759,
#123760,#123761),.UNSPECIFIED.,.F.,.F.,(4,2,4),(3.15595498847292E-11,0.0126519401075625,
0.0253036433442606),.UNSPECIFIED.);
#22608=B_SPLINE_CURVE_WITH_KNOTS('',3,(#123781,#123782,#123783,#123784,
#123785,#123786),.UNSPECIFIED.,.F.,.F.,(4,2,4),(3.08817990073898E-11,0.0126519400829584,
0.0253036433089566),.UNSPECIFIED.);
#22609=B_SPLINE_CURVE_WITH_KNOTS('',3,(#123816,#123817,#123818,#123819,
#123820,#123821,#123822,#123823,#123824,#123825),.UNSPECIFIED.,.F.,.F.,
(4,3,3,4),(6.6640610766212E-12,8.705316532067E-5,0.000170036750316901,0.000253022379909538),
 .UNSPECIFIED.);
#22610=B_SPLINE_CURVE_WITH_KNOTS('',3,(#123842,#123843,#123844,#123845,
#123846,#123847,#123848,#123849,#123850,#123851),.UNSPECIFIED.,.F.,.F.,
(4,3,3,4),(0.21150258497194,0.214285714285714,0.224091821226272,0.228883374862199),
 .UNSPECIFIED.);
#22611=B_SPLINE_CURVE_WITH_KNOTS('',3,(#123852,#123853,#123854,#123855,
#123856,#123857,#123858,#123859,#123860,#123861),.UNSPECIFIED.,.F.,.F.,
(4,3,3,4),(9.87472387492481E-14,8.70530730923297E-5,0.000170036649017195,
0.000253022524284304),.UNSPECIFIED.);
#22612=B_SPLINE_CURVE_WITH_KNOTS('',3,(#123893,#123894,#123895,#123896,
#123897,#123898,#123899,#123900,#123901,#123902),.UNSPECIFIED.,.F.,.F.,
(4,3,3,4),(9.66095229123471E-14,8.70530734827142E-5,0.000170036649712784,
0.000253022525284264),.UNSPECIFIED.);
#22613=B_SPLINE_CURVE_WITH_KNOTS('',3,(#123934,#123935,#123936,#123937,
#123938,#123939,#123940,#123941,#123942,#123943),.UNSPECIFIED.,.F.,.F.,
(4,3,3,4),(8.51722419461328E-14,8.70530733731967E-5,0.00017003664969144,
0.00025302252535137),.UNSPECIFIED.);
#22614=B_SPLINE_CURVE_WITH_KNOTS('',3,(#123970,#123971,#123972,#123973,
#123974,#123975,#123976,#123977,#123978,#123979),.UNSPECIFIED.,.F.,.F.,
(4,3,3,4),(0.21150258497204,0.214285714285714,0.224091815977165,0.228883374852172),
 .UNSPECIFIED.);
#22615=B_SPLINE_CURVE_WITH_KNOTS('',3,(#123980,#123981,#123982,#123983,
#123984,#123985,#123986,#123987,#123988,#123989),.UNSPECIFIED.,.F.,.F.,
(4,3,3,4),(1.01626207911617E-13,8.70530731189993E-5,0.000170036648882768,
0.000253022523989131),.UNSPECIFIED.);
#22616=B_SPLINE_CURVE_WITH_KNOTS('',3,(#124016,#124017,#124018,#124019,
#124020,#124021,#124022,#124023,#124024,#124025),.UNSPECIFIED.,.F.,.F.,
(4,3,3,4),(0.211502584960139,0.214285714285714,0.224091816970476,0.228883374861854),
 .UNSPECIFIED.);
#22617=B_SPLINE_CURVE_WITH_KNOTS('',3,(#124026,#124027,#124028,#124029,
#124030,#124031,#124032,#124033,#124034,#124035),.UNSPECIFIED.,.F.,.F.,
(4,3,3,4),(8.80036232291946E-15,8.70530734436068E-5,0.000170036649788735,
0.000253022525475915),.UNSPECIFIED.);
#22618=B_SPLINE_CURVE_WITH_KNOTS('',3,(#124067,#124068,#124069,#124070,
#124071,#124072,#124073,#124074,#124075,#124076),.UNSPECIFIED.,.F.,.F.,
(4,3,3,4),(1.25935783266693E-13,8.70530732380594E-5,0.000170036649043835,
0.000253022524191688),.UNSPECIFIED.);
#22619=B_SPLINE_CURVE_WITH_KNOTS('',3,(#124108,#124109,#124110,#124111,
#124112,#124113,#124114,#124115,#124116,#124117),.UNSPECIFIED.,.F.,.F.,
(4,3,3,4),(6.3468392922729E-14,8.70530730437247E-5,0.000170036649085858,
0.00025302252447051),.UNSPECIFIED.);
#22620=B_SPLINE_CURVE_WITH_KNOTS('',3,(#124149,#124150,#124151,#124152,
#124153,#124154,#124155,#124156,#124157,#124158),.UNSPECIFIED.,.F.,.F.,
(4,3,3,4),(5.57032184678306E-14,8.70530736151203E-5,0.000170036649919078,
0.000253022525565306),.UNSPECIFIED.);
#22621=B_SPLINE_CURVE_WITH_KNOTS('',3,(#124190,#124191,#124192,#124193,
#124194,#124195,#124196,#124197,#124198,#124199),.UNSPECIFIED.,.F.,.F.,
(4,3,3,4),(2.08112962572377E-14,8.70530731469877E-5,0.000170036648983745,
0.000253022524162933),.UNSPECIFIED.);
#22622=B_SPLINE_CURVE_WITH_KNOTS('',3,(#124226,#124227,#124228,#124229,
#124230,#124231,#124232,#124233,#124234,#124235),.UNSPECIFIED.,.F.,.F.,
(4,3,3,4),(0.211502584948017,0.214285714285714,0.224091813954176,0.228883374857004),
 .UNSPECIFIED.);
#22623=B_SPLINE_CURVE_WITH_KNOTS('',3,(#124236,#124237,#124238,#124239,
#124240,#124241,#124242,#124243,#124244,#124245),.UNSPECIFIED.,.F.,.F.,
(4,3,3,4),(1.0312806272257E-13,8.70530736274529E-5,0.000170036649568835,
0.000253022524852173),.UNSPECIFIED.);
#22624=B_SPLINE_CURVE_WITH_KNOTS('',3,(#124277,#124278,#124279,#124280,
#124281,#124282,#124283,#124284,#124285,#124286),.UNSPECIFIED.,.F.,.F.,
(4,3,3,4),(6.10883102621712E-14,8.70530732758973E-5,0.000170036649311073,
0.000253022524688439),.UNSPECIFIED.);
#22625=B_SPLINE_CURVE_WITH_KNOTS('',3,(#124318,#124319,#124320,#124321,
#124322,#124323,#124324,#124325,#124326,#124327),.UNSPECIFIED.,.F.,.F.,
(4,3,3,4),(9.87598498237521E-14,8.70530733707688E-5,0.000170036649518818,
0.000253022525009334),.UNSPECIFIED.);
#22626=B_SPLINE_CURVE_WITH_KNOTS('',3,(#124359,#124360,#124361,#124362,
#124363,#124364,#124365,#124366,#124367,#124368),.UNSPECIFIED.,.F.,.F.,
(4,3,3,4),(1.22916473070759E-13,8.70530733797046E-5,0.000170036649362786,
0.0002530225246876),.UNSPECIFIED.);
#22627=B_SPLINE_CURVE_WITH_KNOTS('',3,(#124395,#124396,#124397,#124398,
#124399,#124400,#124401,#124402,#124403,#124404,#124405,#124406,#124407,
#124408),.UNSPECIFIED.,.F.,.F.,(4,2,2,2,2,2,4),(6.1819644215993E-10,0.0398355571596381,
0.0598130476820354,0.0698194557541455,0.0748266666676206,0.0773312228469091,
0.0797213973169973),.UNSPECIFIED.);
#22628=B_SPLINE_CURVE_WITH_KNOTS('',3,(#124409,#124410,#124411,#124412,
#124413,#124414,#124415,#124416,#124417,#124418),.UNSPECIFIED.,.F.,.F.,
(4,3,3,4),(1.57386796031694E-13,8.70530729486484E-5,0.000170036648862666,
0.000253022524119131),.UNSPECIFIED.);
#22629=B_SPLINE_CURVE_WITH_KNOTS('',3,(#124445,#124446,#124447,#124448,
#124449,#124450,#124451,#124452,#124453,#124454,#124455,#124456,#124457,
#124458),.UNSPECIFIED.,.F.,.F.,(4,2,2,2,2,2,4),(5.57021547245071E-10,0.0398355724600839,
0.0598130687824846,0.0698194724814338,0.0748266812070732,0.0773312362921125,
0.0797214096953586),.UNSPECIFIED.);
#22630=B_SPLINE_CURVE_WITH_KNOTS('',3,(#124459,#124460,#124461,#124462,
#124463,#124464,#124465,#124466,#124467,#124468),.UNSPECIFIED.,.F.,.F.,
(4,3,3,4),(3.67379430042663E-14,8.70530734906078E-5,0.000170036649570195,
0.000253022524992311),.UNSPECIFIED.);
#22631=B_SPLINE_CURVE_WITH_KNOTS('',3,(#124495,#124496,#124497,#124498,
#124499,#124500,#124501,#124502,#124503,#124504,#124505,#124506,#124507,
#124508),.UNSPECIFIED.,.F.,.F.,(4,2,2,2,2,2,4),(5.85094002627536E-10,0.0398355551775198,
0.0598130479271771,0.0698194623582696,0.0748266764456829,0.0773312342105983,
0.079721410169492),.UNSPECIFIED.);
#22632=B_SPLINE_CURVE_WITH_KNOTS('',3,(#124509,#124510,#124511,#124512,
#124513,#124514,#124515,#124516,#124517,#124518),.UNSPECIFIED.,.F.,.F.,
(4,3,3,4),(6.03864091016704E-14,8.70530729984532E-5,0.000170036648893081,
0.000253022524129855),.UNSPECIFIED.);
#22633=B_SPLINE_CURVE_WITH_KNOTS('',3,(#124550,#124551,#124552,#124553,
#124554,#124555,#124556,#124557,#124558,#124559),.UNSPECIFIED.,.F.,.F.,
(4,3,3,4),(1.09033936088854E-13,8.70530732165782E-5,0.000170036649139827,
0.000253022524404992),.UNSPECIFIED.);
#22634=B_SPLINE_CURVE_WITH_KNOTS('',3,(#124591,#124592,#124593,#124594,
#124595,#124596,#124597,#124598,#124599,#124600),.UNSPECIFIED.,.F.,.F.,
(4,3,3,4),(1.18163273935885E-13,8.70530734410755E-5,0.000170036649704182,
0.000253022525309384),.UNSPECIFIED.);
#22635=B_SPLINE_CURVE_WITH_KNOTS('',3,(#124627,#124628,#124629,#124630,
#124631,#124632,#124633,#124634,#124635,#124636),.UNSPECIFIED.,.F.,.F.,
(4,3,3,4),(0.211502584965516,0.214285714285714,0.224091827574402,0.228883374872321),
 .UNSPECIFIED.);
#22636=B_SPLINE_CURVE_WITH_KNOTS('',3,(#124637,#124638,#124639,#124640,
#124641,#124642,#124643,#124644,#124645,#124646),.UNSPECIFIED.,.F.,.F.,
(4,3,3,4),(9.02433971457501E-14,8.70530732466902E-5,0.000170036649065817,
0.000253022524226767),.UNSPECIFIED.);
#22637=B_SPLINE_CURVE_WITH_KNOTS('',3,(#124678,#124679,#124680,#124681,
#124682,#124683,#124684,#124685,#124686,#124687),.UNSPECIFIED.,.F.,.F.,
(4,3,3,4),(7.51514809846539E-14,8.70530731548467E-5,0.000170036649085044,
0.000253022524357496),.UNSPECIFIED.);
#22638=B_SPLINE_CURVE_WITH_KNOTS('',3,(#124719,#124720,#124721,#124722,
#124723,#124724,#124725,#124726,#124727,#124728),.UNSPECIFIED.,.F.,.F.,
(4,3,3,4),(2.53717776951365E-14,8.70530732794565E-5,0.000170036649550751,
0.000253022525164439),.UNSPECIFIED.);
#22639=B_SPLINE_CURVE_WITH_KNOTS('',3,(#124755,#124756,#124757,#124758,
#124759,#124760,#124761,#124762,#124763,#124764),.UNSPECIFIED.,.F.,.F.,
(4,3,3,4),(0.211502584969517,0.214285714285714,0.224091819257381,0.228883374862328),
 .UNSPECIFIED.);
#22640=B_SPLINE_CURVE_WITH_KNOTS('',3,(#124765,#124766,#124767,#124768,
#124769,#124770,#124771,#124772,#124773,#124774),.UNSPECIFIED.,.F.,.F.,
(4,3,3,4),(7.89431934074236E-14,8.70530731075781E-5,0.000170036648965765,
0.000253022524166181),.UNSPECIFIED.);
#22641=B_SPLINE_CURVE_WITH_KNOTS('',3,(#124801,#124802,#124803,#124804,
#124805,#124806,#124807,#124808,#124809,#124810,#124811,#124812,#124813,
#124814),.UNSPECIFIED.,.F.,.F.,(4,2,2,2,2,2,4),(6.34474575368533E-10,0.0398355712933957,
0.059813071467123,0.0698194778032689,0.0748266878437471,0.077331243585381,
0.0797214176266301),.UNSPECIFIED.);
#22642=B_SPLINE_CURVE_WITH_KNOTS('',3,(#124815,#124816,#124817,#124818,
#124819,#124820,#124821,#124822,#124823,#124824),.UNSPECIFIED.,.F.,.F.,
(4,3,3,4),(1.31867107742812E-13,8.70530735910056E-5,0.000170036649834359,
0.000253022525420013),.UNSPECIFIED.);
#22643=B_SPLINE_CURVE_WITH_KNOTS('',3,(#124856,#124857,#124858,#124859,
#124860,#124861,#124862,#124863,#124864,#124865),.UNSPECIFIED.,.F.,.F.,
(4,3,3,4),(5.36960810667672E-14,8.70530735283642E-5,0.000170036649708884,
0.000253022525231527),.UNSPECIFIED.);
#22644=B_SPLINE_CURVE_WITH_KNOTS('',3,(#124897,#124898,#124899,#124900,
#124901,#124902,#124903,#124904,#124905,#124906),.UNSPECIFIED.,.F.,.F.,
(4,3,3,4),(7.80228131461319E-14,8.70530734703482E-5,0.000170036649594559,
0.000253022525060402),.UNSPECIFIED.);
#22645=B_SPLINE_CURVE_WITH_KNOTS('',3,(#124938,#124939,#124940,#124941,
#124942,#124943,#124944,#124945,#124946,#124947),.UNSPECIFIED.,.F.,.F.,
(4,3,3,4),(8.01062290819287E-15,8.7053073630607E-5,0.000170036649876423,
0.000253022525464228),.UNSPECIFIED.);
#22646=B_SPLINE_CURVE_WITH_KNOTS('',3,(#124974,#124975,#124976,#124977,
#124978,#124979,#124980,#124981,#124982,#124983),.UNSPECIFIED.,.F.,.F.,
(4,3,3,4),(0.211502584963299,0.214285714285714,0.224091802941358,0.228883374862355),
 .UNSPECIFIED.);
#22647=B_SPLINE_CURVE_WITH_KNOTS('',3,(#124984,#124985,#124986,#124987,
#124988,#124989,#124990,#124991,#124992,#124993),.UNSPECIFIED.,.F.,.F.,
(4,3,3,4),(8.73844952612567E-14,8.70530734589333E-5,0.000170036649623771,
0.000253022525131072),.UNSPECIFIED.);
#22648=B_SPLINE_CURVE_WITH_KNOTS('',3,(#125020,#125021,#125022,#125023,
#125024,#125025,#125026,#125027,#125028,#125029),.UNSPECIFIED.,.F.,.F.,
(4,3,3,4),(0.211502584978396,0.214285714285714,0.224091828316984,0.228883374866789),
 .UNSPECIFIED.);
#22649=B_SPLINE_CURVE_WITH_KNOTS('',3,(#125030,#125031,#125032,#125033,
#125034,#125035,#125036,#125037,#125038,#125039),.UNSPECIFIED.,.F.,.F.,
(4,3,3,4),(4.13945888189021E-14,8.70530734855099E-5,0.000170036649813318,
0.000253022525483275),.UNSPECIFIED.);
#22650=B_SPLINE_CURVE_WITH_KNOTS('',3,(#125065,#125066,#125067,#125068,
#125069,#125070,#125071,#125072,#125073,#125074,#125075,#125076,#125077,
#125078),.UNSPECIFIED.,.F.,.F.,(4,2,2,2,2,2,4),(9.84438766148368E-11,0.0398356066089345,
0.0598131576187708,0.0698195873416727,0.0748268090853319,0.077331370681033,
0.0797215503067857),.UNSPECIFIED.);
#22651=B_SPLINE_CURVE_WITH_KNOTS('',3,(#125092,#125093,#125094,#125095,
#125096,#125097),.UNSPECIFIED.,.F.,.F.,(4,2,4),(-0.0253009680193219,-0.0126505173686473,
-1.50651325789286E-9),.UNSPECIFIED.);
#22652=B_SPLINE_CURVE_WITH_KNOTS('',3,(#125125,#125126,#125127,#125128,
#125129,#125130),.UNSPECIFIED.,.F.,.F.,(4,2,4),(-0.0253008161710598,-0.0126505173063933,
-1.49706886817813E-9),.UNSPECIFIED.);
#22653=B_SPLINE_CURVE_WITH_KNOTS('',3,(#125158,#125159,#125160,#125161,
#125162,#125163),.UNSPECIFIED.,.F.,.F.,(4,2,4),(-0.0253008162502549,-0.012650517377553,
-1.51926837083094E-9),.UNSPECIFIED.);
#22654=B_SPLINE_CURVE_WITH_KNOTS('',3,(#125191,#125192,#125193,#125194,
#125195,#125196),.UNSPECIFIED.,.F.,.F.,(4,2,4),(-0.0253008161942039,-0.0126505173276397,
-1.51911317899933E-9),.UNSPECIFIED.);
#22655=B_SPLINE_CURVE_WITH_KNOTS('',3,(#125224,#125225,#125226,#125227,
#125228,#125229),.UNSPECIFIED.,.F.,.F.,(4,2,4),(-0.025300816184677,-0.0126505173051501,
-1.51005885226652E-9),.UNSPECIFIED.);
#22656=B_SPLINE_CURVE_WITH_KNOTS('',3,(#125257,#125258,#125259,#125260,
#125261,#125262),.UNSPECIFIED.,.F.,.F.,(4,2,4),(-0.0253008162356417,-0.012650517371839,
-1.5194880978453E-9),.UNSPECIFIED.);
#22657=B_SPLINE_CURVE_WITH_KNOTS('',3,(#125290,#125291,#125292,#125293,
#125294,#125295),.UNSPECIFIED.,.F.,.F.,(4,2,4),(-0.0253008162373823,-0.012650517352546,
-1.5117902658901E-9),.UNSPECIFIED.);
#22658=B_SPLINE_CURVE_WITH_KNOTS('',3,(#125323,#125324,#125325,#125326,
#125327,#125328),.UNSPECIFIED.,.F.,.F.,(4,2,4),(-0.0253009567060839,-0.012650517332386,
-1.49595632756294E-9),.UNSPECIFIED.);
#22659=B_SPLINE_CURVE_WITH_KNOTS('',3,(#125356,#125357,#125358,#125359,
#125360,#125361),.UNSPECIFIED.,.F.,.F.,(4,2,4),(-0.0253009734745182,-0.0126505174081292,
-1.53339678454767E-9),.UNSPECIFIED.);
#22660=B_SPLINE_CURVE_WITH_KNOTS('',3,(#125389,#125390,#125391,#125392,
#125393,#125394),.UNSPECIFIED.,.F.,.F.,(4,2,4),(-0.0253009751682653,-0.0126505173744186,
-1.50967184586737E-9),.UNSPECIFIED.);
#22661=B_SPLINE_CURVE_WITH_KNOTS('',3,(#125422,#125423,#125424,#125425,
#125426,#125427),.UNSPECIFIED.,.F.,.F.,(4,2,4),(-0.0253009628824026,-0.012650517367083,
-1.50349348596035E-9),.UNSPECIFIED.);
#22662=B_SPLINE_CURVE_WITH_KNOTS('',3,(#125455,#125456,#125457,#125458,
#125459,#125460),.UNSPECIFIED.,.F.,.F.,(4,2,4),(-0.0253009682533948,-0.0126505173592761,
-1.50435279511196E-9),.UNSPECIFIED.);
#22663=B_SPLINE_CURVE_WITH_KNOTS('',3,(#125488,#125489,#125490,#125491,
#125492,#125493),.UNSPECIFIED.,.F.,.F.,(4,2,4),(-0.0253008162097125,-0.0126505173692927,
-1.51393972705471E-9),.UNSPECIFIED.);
#22664=B_SPLINE_CURVE_WITH_KNOTS('',3,(#125521,#125522,#125523,#125524,
#125525,#125526),.UNSPECIFIED.,.F.,.F.,(4,2,4),(-0.0253009709382149,-0.0126505173850716,
-1.51950293320047E-9),.UNSPECIFIED.);
#22665=B_SPLINE_CURVE_WITH_KNOTS('',3,(#125551,#125552,#125553,#125554,
#125555,#125556),.UNSPECIFIED.,.F.,.F.,(4,2,4),(-0.0253008162162922,-0.0126505173663554,
-1.50183707484097E-9),.UNSPECIFIED.);
#22666=B_SPLINE_CURVE_WITH_KNOTS('',3,(#125578,#125579,#125580,#125581,
#125582,#125583),.UNSPECIFIED.,.F.,.F.,(4,2,4),(-0.0253008161965179,-0.0126505173531787,
-1.50008382798772E-9),.UNSPECIFIED.);
#22667=B_SPLINE_CURVE_WITH_KNOTS('',3,(#125611,#125612,#125613,#125614,
#125615,#125616),.UNSPECIFIED.,.F.,.F.,(4,2,4),(-0.0253008162312706,-0.0126505173673404,
-1.51304643467021E-9),.UNSPECIFIED.);
#22668=B_SPLINE_CURVE_WITH_KNOTS('',3,(#125644,#125645,#125646,#125647,
#125648,#125649),.UNSPECIFIED.,.F.,.F.,(4,2,4),(-0.0253008161733499,-0.0126505173152187,
-1.50923519515178E-9),.UNSPECIFIED.);
#22669=B_SPLINE_CURVE_WITH_KNOTS('',3,(#125677,#125678,#125679,#125680,
#125681,#125682),.UNSPECIFIED.,.F.,.F.,(4,2,4),(-0.0253009530091239,-0.0126505173737225,
-1.5033947455001E-9),.UNSPECIFIED.);
#22670=B_SPLINE_CURVE_WITH_KNOTS('',3,(#125710,#125711,#125712,#125713,
#125714,#125715),.UNSPECIFIED.,.F.,.F.,(4,2,4),(-0.0253009684925171,-0.0126505173770235,
-1.5125917671166E-9),.UNSPECIFIED.);
#22671=B_SPLINE_CURVE_WITH_KNOTS('',3,(#125743,#125744,#125745,#125746,
#125747,#125748),.UNSPECIFIED.,.F.,.F.,(4,2,4),(-0.0253008162223907,-0.0126505173844459,
-1.51811038739957E-9),.UNSPECIFIED.);
#22672=B_SPLINE_CURVE_WITH_KNOTS('',3,(#125776,#125777,#125778,#125779,
#125780,#125781),.UNSPECIFIED.,.F.,.F.,(4,2,4),(-0.0253008161851833,-0.0126505173103185,
-1.49799530765882E-9),.UNSPECIFIED.);
#22673=B_SPLINE_CURVE_WITH_KNOTS('',3,(#125810,#125811,#125812,#125813,
#125814,#125815),.UNSPECIFIED.,.F.,.F.,(4,2,4),(-0.025300816194907,-0.0126505173454016,
-1.51742879719863E-9),.UNSPECIFIED.);
#22674=B_SPLINE_CURVE_WITH_KNOTS('',3,(#125842,#125843,#125844,#125845,
#125846,#125847),.UNSPECIFIED.,.F.,.F.,(4,2,4),(-0.0253008162162837,-0.0126505173700267,
-1.50907499690822E-9),.UNSPECIFIED.);
#22675=B_SPLINE_CURVE_WITH_KNOTS('',3,(#125875,#125876,#125877,#125878,
#125879,#125880),.UNSPECIFIED.,.F.,.F.,(4,2,4),(-0.0253008162384224,-0.0126505173764547,
-1.50414914204533E-9),.UNSPECIFIED.);
#22676=B_SPLINE_CURVE_WITH_KNOTS('',3,(#125908,#125909,#125910,#125911,
#125912,#125913),.UNSPECIFIED.,.F.,.F.,(4,2,4),(-0.0253008162004374,-0.0126505173491142,
-1.50324420272741E-9),.UNSPECIFIED.);
#22677=B_SPLINE_CURVE_WITH_KNOTS('',3,(#125941,#125942,#125943,#125944,
#125945,#125946),.UNSPECIFIED.,.F.,.F.,(4,2,4),(-0.0253008162124498,-0.012650517365658,
-1.51088165242785E-9),.UNSPECIFIED.);
#22678=B_SPLINE_CURVE_WITH_KNOTS('',3,(#125974,#125975,#125976,#125977,
#125978,#125979),.UNSPECIFIED.,.F.,.F.,(4,2,4),(-0.0253008161865096,-0.01265051732059,
-1.5011254600461E-9),.UNSPECIFIED.);
#22679=B_SPLINE_CURVE_WITH_KNOTS('',3,(#126007,#126008,#126009,#126010,
#126011,#126012),.UNSPECIFIED.,.F.,.F.,(4,2,4),(-0.0253009718038439,-0.0126505173976087,
-1.53092769364371E-9),.UNSPECIFIED.);
#22680=B_SPLINE_CURVE_WITH_KNOTS('',3,(#126041,#126042,#126043,#126044,
#126045,#126046),.UNSPECIFIED.,.F.,.F.,(4,2,4),(-0.0252971444835285,-0.0126486652117214,
0.),.UNSPECIFIED.);
#22681=B_SPLINE_CURVE_WITH_KNOTS('',3,(#126058,#126059,#126060,#126061,
#126062,#126063,#126064),.UNSPECIFIED.,.F.,.F.,(4,3,4),(0.216822083469384,
0.226204530183526,0.228987659635175),.UNSPECIFIED.);
#22682=B_SPLINE_CURVE_WITH_KNOTS('',3,(#126084,#126085,#126086,#126087,
#126088,#126089),.UNSPECIFIED.,.F.,.F.,(4,2,4),(-0.0252971543978597,-0.0126486691839802,
0.),.UNSPECIFIED.);
#22683=B_SPLINE_CURVE_WITH_KNOTS('',3,(#126101,#126102,#126103,#126104,
#126105,#126106,#126107),.UNSPECIFIED.,.F.,.F.,(4,3,4),(0.216822083469368,
0.226204530183526,0.228987659635175),.UNSPECIFIED.);
#22684=B_SPLINE_CURVE_WITH_KNOTS('',3,(#126127,#126128,#126129,#126130,
#126131,#126132),.UNSPECIFIED.,.F.,.F.,(4,2,4),(-0.0252971379173837,-0.0126486624600064,
0.),.UNSPECIFIED.);
#22685=B_SPLINE_CURVE_WITH_KNOTS('',3,(#126144,#126145,#126146,#126147,
#126148,#126149,#126150),.UNSPECIFIED.,.F.,.F.,(4,3,4),(0.216822083469368,
0.226204530183526,0.228987659635175),.UNSPECIFIED.);
#22686=B_SPLINE_CURVE_WITH_KNOTS('',3,(#126170,#126171,#126172,#126173,
#126174,#126175),.UNSPECIFIED.,.F.,.F.,(4,2,4),(-0.025296843893326,-0.0126485434765334,
-1.79759367113785E-11),.UNSPECIFIED.);
#22687=B_SPLINE_CURVE_WITH_KNOTS('',3,(#126187,#126188,#126189,#126190,
#126191,#126192,#126193),.UNSPECIFIED.,.F.,.F.,(4,3,4),(0.216822083469368,
0.226204530183526,0.228987659635175),.UNSPECIFIED.);
#22688=B_SPLINE_CURVE_WITH_KNOTS('',3,(#126213,#126214,#126215,#126216,
#126217,#126218),.UNSPECIFIED.,.F.,.F.,(4,2,4),(-0.0252971503797783,-0.0126486675839431,
0.),.UNSPECIFIED.);
#22689=B_SPLINE_CURVE_WITH_KNOTS('',3,(#126230,#126231,#126232,#126233,
#126234,#126235,#126236),.UNSPECIFIED.,.F.,.F.,(4,3,4),(0.216822083469358,
0.226204530183526,0.228987659635175),.UNSPECIFIED.);
#22690=B_SPLINE_CURVE_WITH_KNOTS('',3,(#126256,#126257,#126258,#126259,
#126260,#126261),.UNSPECIFIED.,.F.,.F.,(4,2,4),(-0.0252971492907873,-0.0126486671489296,
0.),.UNSPECIFIED.);
#22691=B_SPLINE_CURVE_WITH_KNOTS('',3,(#126273,#126274,#126275,#126276,
#126277,#126278,#126279),.UNSPECIFIED.,.F.,.F.,(4,3,4),(0.216822083469368,
0.226204530183526,0.228987659635175),.UNSPECIFIED.);
#22692=B_SPLINE_CURVE_WITH_KNOTS('',3,(#126299,#126300,#126301,#126302,
#126303,#126304),.UNSPECIFIED.,.F.,.F.,(4,2,4),(-0.025296843880375,-0.0126485434460251,
-1.24961256620093E-11),.UNSPECIFIED.);
#22693=B_SPLINE_CURVE_WITH_KNOTS('',3,(#126316,#126317,#126318,#126319,
#126320,#126321,#126322),.UNSPECIFIED.,.F.,.F.,(4,3,4),(0.216822083469358,
0.226204530183526,0.228987659635175),.UNSPECIFIED.);
#22694=B_SPLINE_CURVE_WITH_KNOTS('',3,(#126342,#126343,#126344,#126345,
#126346,#126347),.UNSPECIFIED.,.F.,.F.,(4,2,4),(-0.0252971646096114,-0.0126486733003775,
0.),.UNSPECIFIED.);
#22695=B_SPLINE_CURVE_WITH_KNOTS('',3,(#126359,#126360,#126361,#126362,
#126363,#126364,#126365),.UNSPECIFIED.,.F.,.F.,(4,3,4),(0.216822083469364,
0.226204530183524,0.228987659635174),.UNSPECIFIED.);
#22696=B_SPLINE_CURVE_WITH_KNOTS('',3,(#126385,#126386,#126387,#126388,
#126389,#126390),.UNSPECIFIED.,.F.,.F.,(4,2,4),(-0.0252971681999182,-0.0126486747882726,
0.),.UNSPECIFIED.);
#22697=B_SPLINE_CURVE_WITH_KNOTS('',3,(#126402,#126403,#126404,#126405,
#126406,#126407,#126408),.UNSPECIFIED.,.F.,.F.,(4,3,4),(0.216822083469364,
0.226204530183524,0.228987659635174),.UNSPECIFIED.);
#22698=B_SPLINE_CURVE_WITH_KNOTS('',3,(#126428,#126429,#126430,#126431,
#126432,#126433),.UNSPECIFIED.,.F.,.F.,(4,2,4),(-0.0252971380209954,-0.0126486625735294,
0.),.UNSPECIFIED.);
#22699=B_SPLINE_CURVE_WITH_KNOTS('',3,(#126445,#126446,#126447,#126448,
#126449,#126450,#126451),.UNSPECIFIED.,.F.,.F.,(4,3,4),(0.216822083469354,
0.226204530183524,0.228987659635174),.UNSPECIFIED.);
#22700=B_SPLINE_CURVE_WITH_KNOTS('',3,(#126471,#126472,#126473,#126474,
#126475,#126476),.UNSPECIFIED.,.F.,.F.,(4,2,4),(-0.025297157550282,-0.0126486704428088,
0.),.UNSPECIFIED.);
#22701=B_SPLINE_CURVE_WITH_KNOTS('',3,(#126488,#126489,#126490,#126491,
#126492,#126493,#126494),.UNSPECIFIED.,.F.,.F.,(4,3,4),(0.216822083469364,
0.226204530183524,0.228987659635174),.UNSPECIFIED.);
#22702=B_SPLINE_CURVE_WITH_KNOTS('',3,(#126514,#126515,#126516,#126517,
#126518,#126519),.UNSPECIFIED.,.F.,.F.,(4,2,4),(-0.0252972106396085,-0.0126486717985792,
0.),.UNSPECIFIED.);
#22703=B_SPLINE_CURVE_WITH_KNOTS('',3,(#126531,#126532,#126533,#126534,
#126535,#126536,#126537),.UNSPECIFIED.,.F.,.F.,(4,3,4),(0.216822083469356,
0.226204530183524,0.228987659635174),.UNSPECIFIED.);
#22704=B_SPLINE_CURVE_WITH_KNOTS('',3,(#126557,#126558,#126559,#126560,
#126561,#126562),.UNSPECIFIED.,.F.,.F.,(4,2,4),(-0.0252971534510284,-0.0126486688573293,
0.),.UNSPECIFIED.);
#22705=B_SPLINE_CURVE_WITH_KNOTS('',3,(#126574,#126575,#126576,#126577,
#126578,#126579,#126580),.UNSPECIFIED.,.F.,.F.,(4,3,4),(0.216822083469364,
0.226204530183524,0.228987659635174),.UNSPECIFIED.);
#22706=B_SPLINE_CURVE_WITH_KNOTS('',3,(#126600,#126601,#126602,#126603,
#126604,#126605),.UNSPECIFIED.,.F.,.F.,(4,2,4),(-0.0252971604072883,-0.0126486716236138,
-8.09109723665102E-14),.UNSPECIFIED.);
#22707=B_SPLINE_CURVE_WITH_KNOTS('',3,(#126617,#126618,#126619,#126620,
#126621,#126622,#126623),.UNSPECIFIED.,.F.,.F.,(4,3,4),(0.216822083469356,
0.226204530183524,0.228987659635174),.UNSPECIFIED.);
#22708=B_SPLINE_CURVE_WITH_KNOTS('',3,(#126643,#126644,#126645,#126646,
#126647,#126648),.UNSPECIFIED.,.F.,.F.,(4,2,4),(-0.0252971585311309,-0.0126486708489145,
-4.90309182143989E-13),.UNSPECIFIED.);
#22709=B_SPLINE_CURVE_WITH_KNOTS('',3,(#126660,#126661,#126662,#126663,
#126664,#126665,#126666),.UNSPECIFIED.,.F.,.F.,(4,3,4),(0.216822083469359,
0.226204530183524,0.228987659635174),.UNSPECIFIED.);
#22710=B_SPLINE_CURVE_WITH_KNOTS('',3,(#126686,#126687,#126688,#126689,
#126690,#126691),.UNSPECIFIED.,.F.,.F.,(4,2,4),(-0.0252971600971946,-0.0126486714719039,
0.),.UNSPECIFIED.);
#22711=B_SPLINE_CURVE_WITH_KNOTS('',3,(#126703,#126704,#126705,#126706,
#126707,#126708,#126709),.UNSPECIFIED.,.F.,.F.,(4,3,4),(0.216822083469342,
0.226204530183524,0.228987659635174),.UNSPECIFIED.);
#22712=B_SPLINE_CURVE_WITH_KNOTS('',3,(#126729,#126730,#126731,#126732,
#126733,#126734),.UNSPECIFIED.,.F.,.F.,(4,2,4),(-0.0252971483010817,-0.0126486667440166,
0.),.UNSPECIFIED.);
#22713=B_SPLINE_CURVE_WITH_KNOTS('',3,(#126746,#126747,#126748,#126749,
#126750,#126751,#126752),.UNSPECIFIED.,.F.,.F.,(4,3,4),(0.216822083469362,
0.226204530183522,0.228987659635174),.UNSPECIFIED.);
#22714=B_SPLINE_CURVE_WITH_KNOTS('',3,(#126772,#126773,#126774,#126775,
#126776,#126777),.UNSPECIFIED.,.F.,.F.,(4,2,4),(-0.0252972379215595,-0.0126486787224415,
-4.86898715790218E-13),.UNSPECIFIED.);
#22715=B_SPLINE_CURVE_WITH_KNOTS('',3,(#126789,#126790,#126791,#126792,
#126793,#126794,#126795),.UNSPECIFIED.,.F.,.F.,(4,3,4),(0.216822083469365,
0.226204530183524,0.228987659635174),.UNSPECIFIED.);
#22716=B_SPLINE_CURVE_WITH_KNOTS('',3,(#126815,#126816,#126817,#126818,
#126819,#126820),.UNSPECIFIED.,.F.,.F.,(4,2,4),(-0.0252968437699015,-0.0126485433866258,
-1.85603164781778E-11),.UNSPECIFIED.);
#22717=B_SPLINE_CURVE_WITH_KNOTS('',3,(#126832,#126833,#126834,#126835,
#126836,#126837,#126838),.UNSPECIFIED.,.F.,.F.,(4,3,4),(0.216822083469354,
0.226204530183523,0.228987659635173),.UNSPECIFIED.);
#22718=B_SPLINE_CURVE_WITH_KNOTS('',3,(#126858,#126859,#126860,#126861,
#126862,#126863),.UNSPECIFIED.,.F.,.F.,(4,2,4),(-0.0252971672468309,-0.0126486744551382,
-5.57002360901393E-13),.UNSPECIFIED.);
#22719=B_SPLINE_CURVE_WITH_KNOTS('',3,(#126875,#126876,#126877,#126878,
#126879,#126880,#126881),.UNSPECIFIED.,.F.,.F.,(4,3,4),(0.216822083469377,
0.226204530183522,0.228987659635173),.UNSPECIFIED.);
#22720=B_SPLINE_CURVE_WITH_KNOTS('',3,(#126901,#126902,#126903,#126904,
#126905,#126906),.UNSPECIFIED.,.F.,.F.,(4,2,4),(-0.0252971463408049,-0.0126486659271449,
0.),.UNSPECIFIED.);
#22721=B_SPLINE_CURVE_WITH_KNOTS('',3,(#126918,#126919,#126920,#126921,
#126922,#126923,#126924),.UNSPECIFIED.,.F.,.F.,(4,3,4),(0.216822083469355,
0.22620453018352,0.228987659635174),.UNSPECIFIED.);
#22722=B_SPLINE_CURVE_WITH_KNOTS('',3,(#126941,#126942,#126943,#126944,
#126945,#126946),.UNSPECIFIED.,.F.,.F.,(4,2,4),(-0.0252971476460511,-0.0126486664505831,
0.),.UNSPECIFIED.);
#22723=B_SPLINE_CURVE_WITH_KNOTS('',3,(#126972,#126973,#126974,#126975,
#126976,#126977),.UNSPECIFIED.,.F.,.F.,(4,2,4),(-0.0252968438354448,-0.0126485434423394,
-1.27871359334453E-11),.UNSPECIFIED.);
#22724=B_SPLINE_CURVE_WITH_KNOTS('',3,(#126989,#126990,#126991,#126992,
#126993,#126994,#126995),.UNSPECIFIED.,.F.,.F.,(4,3,4),(0.216822083469191,
0.226204530183371,0.228987659635021),.UNSPECIFIED.);
#22725=B_SPLINE_CURVE_WITH_KNOTS('',3,(#127015,#127016,#127017,#127018,
#127019,#127020),.UNSPECIFIED.,.F.,.F.,(4,2,4),(-0.0252968438482744,-0.0126485434180359,
-2.16074103054353E-11),.UNSPECIFIED.);
#22726=B_SPLINE_CURVE_WITH_KNOTS('',3,(#127032,#127033,#127034,#127035,
#127036,#127037,#127038),.UNSPECIFIED.,.F.,.F.,(4,3,4),(0.216822083469273,
0.226204530183421,0.228987659635071),.UNSPECIFIED.);
#22727=B_SPLINE_CURVE_WITH_KNOTS('',3,(#127058,#127059,#127060,#127061,
#127062,#127063),.UNSPECIFIED.,.F.,.F.,(4,2,4),(-0.0252971457496129,-0.0126486657472849,
-9.65116875306649E-13),.UNSPECIFIED.);
#22728=B_SPLINE_CURVE_WITH_KNOTS('',3,(#127075,#127076,#127077,#127078,
#127079,#127080,#127081),.UNSPECIFIED.,.F.,.F.,(4,3,4),(0.216822083469326,
0.226204530183494,0.228987659635144),.UNSPECIFIED.);
#22729=B_SPLINE_CURVE_WITH_KNOTS('',3,(#127101,#127102,#127103,#127104,
#127105,#127106),.UNSPECIFIED.,.F.,.F.,(4,2,4),(-0.0252968438084748,-0.0126485434315949,
-8.85128428884663E-12),.UNSPECIFIED.);
#22730=B_SPLINE_CURVE_WITH_KNOTS('',3,(#127118,#127119,#127120,#127121,
#127122,#127123,#127124),.UNSPECIFIED.,.F.,.F.,(4,3,4),(0.216822083469354,
0.226204530183518,0.228987659635168),.UNSPECIFIED.);
#22731=B_SPLINE_CURVE_WITH_KNOTS('',3,(#127144,#127145,#127146,#127147,
#127148,#127149),.UNSPECIFIED.,.F.,.F.,(4,2,4),(-0.0252971314486642,-0.0126486598629424,
0.),.UNSPECIFIED.);
#22732=B_SPLINE_CURVE_WITH_KNOTS('',3,(#127161,#127162,#127163,#127164,
#127165,#127166,#127167),.UNSPECIFIED.,.F.,.F.,(4,3,4),(0.216822083469335,
0.226204530183512,0.228987659635174),.UNSPECIFIED.);
#22733=B_SPLINE_CURVE_WITH_KNOTS('',3,(#127187,#127188,#127189,#127190,
#127191,#127192),.UNSPECIFIED.,.F.,.F.,(4,2,4),(-0.0252968438717575,-0.0126485434602566,
-2.32165085767289E-11),.UNSPECIFIED.);
#22734=B_SPLINE_CURVE_WITH_KNOTS('',3,(#127204,#127205,#127206,#127207,
#127208,#127209,#127210),.UNSPECIFIED.,.F.,.F.,(4,3,4),(0.216822083469366,
0.226204530183524,0.228987659635173),.UNSPECIFIED.);
#22735=B_SPLINE_CURVE_WITH_KNOTS('',3,(#127230,#127231,#127232,#127233,
#127234,#127235),.UNSPECIFIED.,.F.,.F.,(4,2,4),(-0.0252971568839752,-0.0126486702042465,
-9.46274655855284E-12),.UNSPECIFIED.);
#22736=B_SPLINE_CURVE_WITH_KNOTS('',3,(#127247,#127248,#127249,#127250,
#127251,#127252,#127253),.UNSPECIFIED.,.F.,.F.,(4,3,4),(0.216822083514415,
0.226204530183526,0.228987659612923),.UNSPECIFIED.);
#22737=B_SPLINE_CURVE_WITH_KNOTS('',3,(#127271,#127272,#127273,#127274,
#127275,#127276),.UNSPECIFIED.,.F.,.F.,(4,2,4),(-0.0253028739767319,-0.012651396576206,
-3.6883829324097E-12),.UNSPECIFIED.);
#22738=B_SPLINE_CURVE_WITH_KNOTS('',3,(#127296,#127297,#127298,#127299,
#127300,#127301),.UNSPECIFIED.,.F.,.F.,(4,2,4),(-0.0253029052518879,-0.0126514041453768,
0.),.UNSPECIFIED.);
#22739=B_SPLINE_CURVE_WITH_KNOTS('',3,(#127321,#127322,#127323,#127324,
#127325,#127326),.UNSPECIFIED.,.F.,.F.,(4,2,4),(-0.0253028728360198,-0.0126513962951784,
0.),.UNSPECIFIED.);
#22740=B_SPLINE_CURVE_WITH_KNOTS('',3,(#127346,#127347,#127348,#127349,
#127350,#127351),.UNSPECIFIED.,.F.,.F.,(4,2,4),(-0.025302907356259,-0.0126513857913042,
0.),.UNSPECIFIED.);
#22741=B_SPLINE_CURVE_WITH_KNOTS('',3,(#127371,#127372,#127373,#127374,
#127375,#127376),.UNSPECIFIED.,.F.,.F.,(4,2,4),(-0.0253028831545656,-0.0126513987913224,
0.),.UNSPECIFIED.);
#22742=B_SPLINE_CURVE_WITH_KNOTS('',3,(#127396,#127397,#127398,#127399,
#127400,#127401),.UNSPECIFIED.,.F.,.F.,(4,2,4),(-0.0253028122000533,-0.0126513816288453,
0.),.UNSPECIFIED.);
#22743=B_SPLINE_CURVE_WITH_KNOTS('',3,(#127421,#127422,#127423,#127424,
#127425,#127426),.UNSPECIFIED.,.F.,.F.,(4,2,4),(-0.0253028437353472,-0.0126513892466307,
0.),.UNSPECIFIED.);
#22744=B_SPLINE_CURVE_WITH_KNOTS('',3,(#127446,#127447,#127448,#127449,
#127450,#127451),.UNSPECIFIED.,.F.,.F.,(4,2,4),(-0.0253028630135161,-0.0126513939175451,
-9.95696580741168E-13),.UNSPECIFIED.);
#22745=B_SPLINE_CURVE_WITH_KNOTS('',3,(#127471,#127472,#127473,#127474,
#127475,#127476),.UNSPECIFIED.,.F.,.F.,(4,2,4),(-0.0253028130466917,-0.0126513818408809,
0.),.UNSPECIFIED.);
#22746=B_SPLINE_CURVE_WITH_KNOTS('',3,(#127496,#127497,#127498,#127499,
#127500,#127501),.UNSPECIFIED.,.F.,.F.,(4,2,4),(-0.0253028790850444,-0.0126513978144101,
0.),.UNSPECIFIED.);
#22747=B_SPLINE_CURVE_WITH_KNOTS('',3,(#127521,#127522,#127523,#127524,
#127525,#127526),.UNSPECIFIED.,.F.,.F.,(4,2,4),(-0.0253028351982294,-0.0126513871967198,
0.),.UNSPECIFIED.);
#22748=B_SPLINE_CURVE_WITH_KNOTS('',3,(#127546,#127547,#127548,#127549,
#127550,#127551),.UNSPECIFIED.,.F.,.F.,(4,2,4),(-0.0253028711195569,-0.0126513958878269,
0.),.UNSPECIFIED.);
#22749=B_SPLINE_CURVE_WITH_KNOTS('',3,(#127571,#127572,#127573,#127574,
#127575,#127576),.UNSPECIFIED.,.F.,.F.,(4,2,4),(-0.0253028106499282,-0.0126513812345954,
0.),.UNSPECIFIED.);
#22750=B_SPLINE_CURVE_WITH_KNOTS('',3,(#127596,#127597,#127598,#127599,
#127600,#127601),.UNSPECIFIED.,.F.,.F.,(4,2,4),(-0.0253028259256569,-0.012651384927295,
0.),.UNSPECIFIED.);
#22751=B_SPLINE_CURVE_WITH_KNOTS('',3,(#127621,#127622,#127623,#127624,
#127625,#127626),.UNSPECIFIED.,.F.,.F.,(4,2,4),(-0.0253028151460171,-0.0126513816870844,
0.),.UNSPECIFIED.);
#22752=B_SPLINE_CURVE_WITH_KNOTS('',3,(#127646,#127647,#127648,#127649,
#127650,#127651),.UNSPECIFIED.,.F.,.F.,(4,2,4),(-0.0253028241929751,-0.0126513845149919,
0.),.UNSPECIFIED.);
#22753=B_SPLINE_CURVE_WITH_KNOTS('',3,(#127671,#127672,#127673,#127674,
#127675,#127676),.UNSPECIFIED.,.F.,.F.,(4,2,4),(-0.0253027974941012,-0.0126513780688482,
0.),.UNSPECIFIED.);
#22754=B_SPLINE_CURVE_WITH_KNOTS('',3,(#127696,#127697,#127698,#127699,
#127700,#127701),.UNSPECIFIED.,.F.,.F.,(4,2,4),(-0.0253028916207358,-0.012651400860891,
-8.60581397810201E-12),.UNSPECIFIED.);
#22755=B_SPLINE_CURVE_WITH_KNOTS('',3,(#127721,#127722,#127723,#127724,
#127725,#127726),.UNSPECIFIED.,.F.,.F.,(4,2,4),(-0.0253028691100921,-0.0126513953986287,
0.),.UNSPECIFIED.);
#22756=B_SPLINE_CURVE_WITH_KNOTS('',3,(#127746,#127747,#127748,#127749,
#127750,#127751),.UNSPECIFIED.,.F.,.F.,(4,2,4),(-0.0253028553317749,-0.0126513920673582,
0.),.UNSPECIFIED.);
#22757=B_SPLINE_CURVE_WITH_KNOTS('',3,(#127771,#127772,#127773,#127774,
#127775,#127776),.UNSPECIFIED.,.F.,.F.,(4,2,4),(-0.0253028299266163,-0.0126513859094088,
0.),.UNSPECIFIED.);
#22758=B_SPLINE_CURVE_WITH_KNOTS('',3,(#127796,#127797,#127798,#127799,
#127800,#127801),.UNSPECIFIED.,.F.,.F.,(4,2,4),(-0.0253028786820699,-0.012651397717359,
0.),.UNSPECIFIED.);
#22759=B_SPLINE_CURVE_WITH_KNOTS('',3,(#127821,#127822,#127823,#127824,
#127825,#127826),.UNSPECIFIED.,.F.,.F.,(4,2,4),(-0.0253028312099245,-0.0126513862313255,
0.),.UNSPECIFIED.);
#22760=B_SPLINE_CURVE_WITH_KNOTS('',3,(#127846,#127847,#127848,#127849,
#127850,#127851),.UNSPECIFIED.,.F.,.F.,(4,2,4),(-0.0253028926284109,-0.0126514011093113,
-1.22269798452646E-11),.UNSPECIFIED.);
#22761=B_SPLINE_CURVE_WITH_KNOTS('',3,(#127871,#127872,#127873,#127874,
#127875,#127876),.UNSPECIFIED.,.F.,.F.,(4,2,4),(-0.0253028799039149,-0.0126513980109877,
0.),.UNSPECIFIED.);
#22762=B_SPLINE_CURVE_WITH_KNOTS('',3,(#127896,#127897,#127898,#127899,
#127900,#127901),.UNSPECIFIED.,.F.,.F.,(4,2,4),(-0.0253028344455026,-0.0126513870067865,
0.),.UNSPECIFIED.);
#22763=B_SPLINE_CURVE_WITH_KNOTS('',3,(#127921,#127922,#127923,#127924,
#127925,#127926),.UNSPECIFIED.,.F.,.F.,(4,2,4),(-0.0253028196011567,-0.0126513834190112,
0.),.UNSPECIFIED.);
#22764=B_SPLINE_CURVE_WITH_KNOTS('',3,(#127946,#127947,#127948,#127949,
#127950,#127951),.UNSPECIFIED.,.F.,.F.,(4,2,4),(-0.0253028454527611,-0.0126513896648064,
0.),.UNSPECIFIED.);
#22765=B_SPLINE_CURVE_WITH_KNOTS('',3,(#127971,#127972,#127973,#127974,
#127975,#127976),.UNSPECIFIED.,.F.,.F.,(4,2,4),(-0.025302850388932,-0.0126513908575762,
0.),.UNSPECIFIED.);
#22766=B_SPLINE_CURVE_WITH_KNOTS('',3,(#127996,#127997,#127998,#127999,
#128000,#128001),.UNSPECIFIED.,.F.,.F.,(4,2,4),(-0.0253033843897737,-0.0126515788041554,
0.),.UNSPECIFIED.);
#22767=B_SPLINE_CURVE_WITH_KNOTS('',3,(#128021,#128022,#128023,#128024,
#128025,#128026),.UNSPECIFIED.,.F.,.F.,(4,2,4),(-0.0253033832420356,-0.0126515785261838,
0.),.UNSPECIFIED.);
#22768=B_SPLINE_CURVE_WITH_KNOTS('',3,(#128046,#128047,#128048,#128049,
#128050,#128051),.UNSPECIFIED.,.F.,.F.,(4,2,4),(-0.0253033740386864,-0.0126515763143982,
0.),.UNSPECIFIED.);
#22769=B_SPLINE_CURVE_WITH_KNOTS('',3,(#128071,#128072,#128073,#128074,
#128075,#128076),.UNSPECIFIED.,.F.,.F.,(4,2,4),(-0.0253033861264452,-0.0126515792102181,
0.),.UNSPECIFIED.);
#22770=B_SPLINE_CURVE_WITH_KNOTS('',3,(#128096,#128097,#128098,#128099,
#128100,#128101),.UNSPECIFIED.,.F.,.F.,(4,2,4),(-0.0253033810482984,-0.0126515780031574,
0.),.UNSPECIFIED.);
#22771=B_SPLINE_CURVE_WITH_KNOTS('',3,(#128121,#128122,#128123,#128124,
#128125,#128126),.UNSPECIFIED.,.F.,.F.,(4,2,4),(-0.0253033777369397,-0.0126515772095753,
0.),.UNSPECIFIED.);
#22772=B_SPLINE_CURVE_WITH_KNOTS('',3,(#128146,#128147,#128148,#128149,
#128150,#128151),.UNSPECIFIED.,.F.,.F.,(4,2,4),(-0.0253033817433229,-0.0126515781718898,
0.),.UNSPECIFIED.);
#22773=B_SPLINE_CURVE_WITH_KNOTS('',3,(#128171,#128172,#128173,#128174,
#128175,#128176),.UNSPECIFIED.,.F.,.F.,(4,2,4),(-0.0253033806303322,-0.0126515778996289,
0.),.UNSPECIFIED.);
#22774=B_SPLINE_CURVE_WITH_KNOTS('',3,(#128196,#128197,#128198,#128199,
#128200,#128201),.UNSPECIFIED.,.F.,.F.,(4,2,4),(-0.0253033856248397,-0.0126515790956557,
0.),.UNSPECIFIED.);
#22775=B_SPLINE_CURVE_WITH_KNOTS('',3,(#128221,#128222,#128223,#128224,
#128225,#128226),.UNSPECIFIED.,.F.,.F.,(4,2,4),(-0.0253033748819442,-0.0126515765228282,
0.),.UNSPECIFIED.);
#22776=B_SPLINE_CURVE_WITH_KNOTS('',3,(#128246,#128247,#128248,#128249,
#128250,#128251),.UNSPECIFIED.,.F.,.F.,(4,2,4),(-0.0253033797315389,-0.0126515776842218,
0.),.UNSPECIFIED.);
#22777=B_SPLINE_CURVE_WITH_KNOTS('',3,(#128271,#128272,#128273,#128274,
#128275,#128276),.UNSPECIFIED.,.F.,.F.,(4,2,4),(-0.0253033826888565,-0.0126515783920459,
0.),.UNSPECIFIED.);
#22778=B_SPLINE_CURVE_WITH_KNOTS('',3,(#128296,#128297,#128298,#128299,
#128300,#128301),.UNSPECIFIED.,.F.,.F.,(4,2,4),(-0.0253033840777337,-0.0126515787360371,
0.),.UNSPECIFIED.);
#22779=B_SPLINE_CURVE_WITH_KNOTS('',3,(#128321,#128322,#128323,#128324,
#128325,#128326),.UNSPECIFIED.,.F.,.F.,(4,2,4),(-0.0253033822757597,-0.0126515782887475,
0.),.UNSPECIFIED.);
#22780=B_SPLINE_CURVE_WITH_KNOTS('',3,(#128346,#128347,#128348,#128349,
#128350,#128351),.UNSPECIFIED.,.F.,.F.,(4,2,4),(-0.0253033742799991,-0.0126515763728792,
0.),.UNSPECIFIED.);
#22781=B_SPLINE_CURVE_WITH_KNOTS('',3,(#128371,#128372,#128373,#128374,
#128375,#128376),.UNSPECIFIED.,.F.,.F.,(4,2,4),(-0.0253033801552282,-0.0126515778085634,
0.),.UNSPECIFIED.);
#22782=B_SPLINE_CURVE_WITH_KNOTS('',3,(#128396,#128397,#128398,#128399,
#128400,#128401),.UNSPECIFIED.,.F.,.F.,(4,2,4),(-0.0253033803562783,-0.0126515778479792,
0.),.UNSPECIFIED.);
#22783=B_SPLINE_CURVE_WITH_KNOTS('',3,(#128421,#128422,#128423,#128424,
#128425,#128426),.UNSPECIFIED.,.F.,.F.,(4,2,4),(-0.0253033694534652,-0.012651575195471,
0.),.UNSPECIFIED.);
#22784=B_SPLINE_CURVE_WITH_KNOTS('',3,(#128446,#128447,#128448,#128449,
#128450,#128451),.UNSPECIFIED.,.F.,.F.,(4,2,4),(-0.0253033830525098,-0.0126515784811636,
0.),.UNSPECIFIED.);
#22785=B_SPLINE_CURVE_WITH_KNOTS('',3,(#128471,#128472,#128473,#128474,
#128475,#128476),.UNSPECIFIED.,.F.,.F.,(4,2,4),(-0.0253033843082028,-0.0126515787848035,
0.),.UNSPECIFIED.);
#22786=B_SPLINE_CURVE_WITH_KNOTS('',3,(#128496,#128497,#128498,#128499,
#128500,#128501),.UNSPECIFIED.,.F.,.F.,(4,2,4),(-0.0253033812413081,-0.0126515780528382,
0.),.UNSPECIFIED.);
#22787=B_SPLINE_CURVE_WITH_KNOTS('',3,(#128521,#128522,#128523,#128524,
#128525,#128526),.UNSPECIFIED.,.F.,.F.,(4,2,4),(-0.0253033830476991,-0.0126515784832709,
0.),.UNSPECIFIED.);
#22788=B_SPLINE_CURVE_WITH_KNOTS('',3,(#128546,#128547,#128548,#128549,
#128550,#128551),.UNSPECIFIED.,.F.,.F.,(4,2,4),(-0.0253033836750068,-0.0126515786334012,
0.),.UNSPECIFIED.);
#22789=B_SPLINE_CURVE_WITH_KNOTS('',3,(#128571,#128572,#128573,#128574,
#128575,#128576),.UNSPECIFIED.,.F.,.F.,(4,2,4),(-0.0253033825810839,-0.0126515756532059,
0.),.UNSPECIFIED.);
#22790=B_SPLINE_CURVE_WITH_KNOTS('',3,(#128596,#128597,#128598,#128599,
#128600,#128601),.UNSPECIFIED.,.F.,.F.,(4,2,4),(-0.0253033895259107,-0.0126515800295567,
0.),.UNSPECIFIED.);
#22791=B_SPLINE_CURVE_WITH_KNOTS('',3,(#128621,#128622,#128623,#128624,
#128625,#128626),.UNSPECIFIED.,.F.,.F.,(4,2,4),(-0.0253033761450526,-0.0126515768170734,
0.),.UNSPECIFIED.);
#22792=B_SPLINE_CURVE_WITH_KNOTS('',3,(#128646,#128647,#128648,#128649,
#128650,#128651),.UNSPECIFIED.,.F.,.F.,(4,2,4),(-0.025303373204294,-0.0126515760996267,
0.),.UNSPECIFIED.);
#22793=B_SPLINE_CURVE_WITH_KNOTS('',3,(#128671,#128672,#128673,#128674,
#128675,#128676),.UNSPECIFIED.,.F.,.F.,(4,2,4),(-0.0253033948806666,-0.0126515786313182,
0.),.UNSPECIFIED.);
#22794=B_SPLINE_CURVE_WITH_KNOTS('',3,(#128696,#128697,#128698,#128699,
#128700,#128701),.UNSPECIFIED.,.F.,.F.,(4,2,4),(-0.0253033736777205,-0.0126515762376764,
0.),.UNSPECIFIED.);
#22795=B_SPLINE_CURVE_WITH_KNOTS('',3,(#128723,#128724,#128725,#128726,
#128727,#128728),.UNSPECIFIED.,.F.,.F.,(4,2,4),(-0.0253043033132767,-0.0126520369393918,
-6.38408319264538E-10),.UNSPECIFIED.);
#22796=B_SPLINE_CURVE_WITH_KNOTS('',3,(#128742,#128743,#128744,#128745,
#128746,#128747),.UNSPECIFIED.,.F.,.F.,(4,2,4),(0.,0.0126520362387386,0.0253042905785001),
 .UNSPECIFIED.);
#22797=B_SPLINE_CURVE_WITH_KNOTS('',3,(#128779,#128780,#128781,#128782,
#128783,#128784),.UNSPECIFIED.,.F.,.F.,(4,2,4),(0.,0.0126520361926197,0.0253043033152966),
 .UNSPECIFIED.);
#22798=B_SPLINE_CURVE_WITH_KNOTS('',3,(#128816,#128817,#128818,#128819,
#128820,#128821),.UNSPECIFIED.,.F.,.F.,(4,2,4),(0.,0.0126520362195973,0.0253043033558742),
 .UNSPECIFIED.);
#22799=B_SPLINE_CURVE_WITH_KNOTS('',3,(#128853,#128854,#128855,#128856,
#128857,#128858),.UNSPECIFIED.,.F.,.F.,(4,2,4),(0.,0.0126520361797729,0.025304303294787),
 .UNSPECIFIED.);
#22800=B_SPLINE_CURVE_WITH_KNOTS('',3,(#128890,#128891,#128892,#128893,
#128894,#128895),.UNSPECIFIED.,.F.,.F.,(4,2,4),(0.,0.0126520361573668,0.0253043032401671),
 .UNSPECIFIED.);
#22801=B_SPLINE_CURVE_WITH_KNOTS('',3,(#128927,#128928,#128929,#128930,
#128931,#128932),.UNSPECIFIED.,.F.,.F.,(4,2,4),(0.,0.0126520361926624,0.0253043032962206),
 .UNSPECIFIED.);
#22802=B_SPLINE_CURVE_WITH_KNOTS('',3,(#128961,#128962,#128963,#128964,
#128965,#128966),.UNSPECIFIED.,.F.,.F.,(4,2,4),(0.,0.0126520361036732,0.0253043031691565),
 .UNSPECIFIED.);
#22803=B_SPLINE_CURVE_WITH_KNOTS('',3,(#128992,#128993,#128994,#128995,
#128996,#128997),.UNSPECIFIED.,.F.,.F.,(4,2,4),(0.,0.0126520361585796,0.0253043032725374),
 .UNSPECIFIED.);
#22804=B_SPLINE_CURVE_WITH_KNOTS('',3,(#129029,#129030,#129031,#129032,
#129033,#129034),.UNSPECIFIED.,.F.,.F.,(4,2,4),(0.,0.0126520362195468,0.0253043033535025),
 .UNSPECIFIED.);
#22805=B_SPLINE_CURVE_WITH_KNOTS('',3,(#129066,#129067,#129068,#129069,
#129070,#129071),.UNSPECIFIED.,.F.,.F.,(4,2,4),(0.,0.0126520362088481,0.0253043033103538),
 .UNSPECIFIED.);
#22806=B_SPLINE_CURVE_WITH_KNOTS('',3,(#129103,#129104,#129105,#129106,
#129107,#129108),.UNSPECIFIED.,.F.,.F.,(4,2,4),(0.,0.0126520361410593,0.0253043032289179),
 .UNSPECIFIED.);
#22807=B_SPLINE_CURVE_WITH_KNOTS('',3,(#129140,#129141,#129142,#129143,
#129144,#129145),.UNSPECIFIED.,.F.,.F.,(4,2,4),(0.,0.0126520362269873,0.0253043033582737),
 .UNSPECIFIED.);
#22808=B_SPLINE_CURVE_WITH_KNOTS('',3,(#129177,#129178,#129179,#129180,
#129181,#129182),.UNSPECIFIED.,.F.,.F.,(4,2,4),(0.,0.012652036199835,0.0253043032947752),
 .UNSPECIFIED.);
#22809=B_SPLINE_CURVE_WITH_KNOTS('',3,(#129214,#129215,#129216,#129217,
#129218,#129219),.UNSPECIFIED.,.F.,.F.,(4,2,4),(0.,0.0126520361816904,0.0253043032966714),
 .UNSPECIFIED.);
#22810=B_SPLINE_CURVE_WITH_KNOTS('',3,(#129251,#129252,#129253,#129254,
#129255,#129256),.UNSPECIFIED.,.F.,.F.,(4,2,4),(0.,0.0126520362137016,0.0253043033359496),
 .UNSPECIFIED.);
#22811=B_SPLINE_CURVE_WITH_KNOTS('',3,(#129288,#129289,#129290,#129291,
#129292,#129293),.UNSPECIFIED.,.F.,.F.,(4,2,4),(0.,0.0126520361685449,0.025304303271054),
 .UNSPECIFIED.);
#22812=B_SPLINE_CURVE_WITH_KNOTS('',3,(#129325,#129326,#129327,#129328,
#129329,#129330),.UNSPECIFIED.,.F.,.F.,(4,2,4),(0.,0.0126520362138179,0.0253043033188563),
 .UNSPECIFIED.);
#22813=B_SPLINE_CURVE_WITH_KNOTS('',3,(#129362,#129363,#129364,#129365,
#129366,#129367),.UNSPECIFIED.,.F.,.F.,(4,2,4),(0.,0.0126520362234447,0.0253043033614193),
 .UNSPECIFIED.);
#22814=B_SPLINE_CURVE_WITH_KNOTS('',3,(#129399,#129400,#129401,#129402,
#129403,#129404),.UNSPECIFIED.,.F.,.F.,(4,2,4),(0.,0.012652036196369,0.0253043033046761),
 .UNSPECIFIED.);
#22815=B_SPLINE_CURVE_WITH_KNOTS('',3,(#129436,#129437,#129438,#129439,
#129440,#129441),.UNSPECIFIED.,.F.,.F.,(4,2,4),(0.,0.0126520361957964,0.0253043033114854),
 .UNSPECIFIED.);
#22816=B_SPLINE_CURVE_WITH_KNOTS('',3,(#129473,#129474,#129475,#129476,
#129477,#129478),.UNSPECIFIED.,.F.,.F.,(4,2,4),(0.,0.0126520362475334,0.025304303358282),
 .UNSPECIFIED.);
#22817=B_SPLINE_CURVE_WITH_KNOTS('',3,(#129511,#129512,#129513,#129514,
#129515,#129516),.UNSPECIFIED.,.F.,.F.,(4,2,4),(0.,0.0126520362011008,0.0253043033315781),
 .UNSPECIFIED.);
#22818=B_SPLINE_CURVE_WITH_KNOTS('',3,(#129547,#129548,#129549,#129550,
#129551,#129552),.UNSPECIFIED.,.F.,.F.,(4,2,4),(0.,0.0126520361475817,0.0253042904271869),
 .UNSPECIFIED.);
#22819=B_SPLINE_CURVE_WITH_KNOTS('',3,(#129584,#129585,#129586,#129587,
#129588,#129589),.UNSPECIFIED.,.F.,.F.,(4,2,4),(0.,0.0126520361853694,0.0253043032746957),
 .UNSPECIFIED.);
#22820=B_SPLINE_CURVE_WITH_KNOTS('',3,(#129621,#129622,#129623,#129624,
#129625,#129626),.UNSPECIFIED.,.F.,.F.,(4,2,4),(0.,0.0126520361360175,0.0253043032161038),
 .UNSPECIFIED.);
#22821=B_SPLINE_CURVE_WITH_KNOTS('',3,(#129658,#129659,#129660,#129661,
#129662,#129663),.UNSPECIFIED.,.F.,.F.,(4,2,4),(0.,0.0126520361850182,0.0253043032915964),
 .UNSPECIFIED.);
#22822=B_SPLINE_CURVE_WITH_KNOTS('',3,(#129695,#129696,#129697,#129698,
#129699,#129700),.UNSPECIFIED.,.F.,.F.,(4,2,4),(0.,0.0126520361578346,0.0253043032710374),
 .UNSPECIFIED.);
#22823=B_SPLINE_CURVE_WITH_KNOTS('',3,(#129732,#129733,#129734,#129735,
#129736,#129737),.UNSPECIFIED.,.F.,.F.,(4,2,4),(0.,0.0126520361522041,0.025304303253814),
 .UNSPECIFIED.);
#22824=B_SPLINE_CURVE_WITH_KNOTS('',3,(#129780,#129781,#129782,#129783,
#129784,#129785),.UNSPECIFIED.,.F.,.F.,(4,2,4),(-0.0253000309094781,-0.0126498687848718,
-4.91224203674756E-10),.UNSPECIFIED.);
#22825=B_SPLINE_CURVE_WITH_KNOTS('',3,(#129803,#129804,#129805,#129806,
#129807,#129808),.UNSPECIFIED.,.F.,.F.,(4,2,4),(1.78041757562141E-11,0.0126499269416387,
0.0253002644237282),.UNSPECIFIED.);
#22826=B_SPLINE_CURVE_WITH_KNOTS('',3,(#129836,#129837,#129838,#129839,
#129840,#129841),.UNSPECIFIED.,.F.,.F.,(4,2,4),(0.,0.0126499190882602,0.025300232813381),
 .UNSPECIFIED.);
#22827=B_SPLINE_CURVE_WITH_KNOTS('',3,(#129869,#129870,#129871,#129872,
#129873,#129874),.UNSPECIFIED.,.F.,.F.,(4,2,4),(0.,0.0126499179894866,0.0253002280646286),
 .UNSPECIFIED.);
#22828=B_SPLINE_CURVE_WITH_KNOTS('',3,(#129902,#129903,#129904,#129905,
#129906,#129907),.UNSPECIFIED.,.F.,.F.,(4,2,4),(0.,0.0126499160711492,0.0253002173995517),
 .UNSPECIFIED.);
#22829=B_SPLINE_CURVE_WITH_KNOTS('',3,(#129935,#129936,#129937,#129938,
#129939,#129940),.UNSPECIFIED.,.F.,.F.,(4,2,4),(0.,0.0126499241869609,0.0253002547372993),
 .UNSPECIFIED.);
#22830=B_SPLINE_CURVE_WITH_KNOTS('',3,(#129968,#129969,#129970,#129971,
#129972,#129973),.UNSPECIFIED.,.F.,.F.,(4,2,4),(0.,0.012649920952608,0.0253002398139683),
 .UNSPECIFIED.);
#22831=B_SPLINE_CURVE_WITH_KNOTS('',3,(#130001,#130002,#130003,#130004,
#130005,#130006),.UNSPECIFIED.,.F.,.F.,(4,2,4),(0.,0.0126499122637278,0.0253002035574413),
 .UNSPECIFIED.);
#22832=B_SPLINE_CURVE_WITH_KNOTS('',3,(#130034,#130035,#130036,#130037,
#130038,#130039),.UNSPECIFIED.,.F.,.F.,(4,2,4),(0.,0.0126499201850027,0.0253002413629696),
 .UNSPECIFIED.);
#22833=B_SPLINE_CURVE_WITH_KNOTS('',3,(#130067,#130068,#130069,#130070,
#130071,#130072),.UNSPECIFIED.,.F.,.F.,(4,2,4),(0.,0.0126499197289081,0.0253002334179211),
 .UNSPECIFIED.);
#22834=B_SPLINE_CURVE_WITH_KNOTS('',3,(#130100,#130101,#130102,#130103,
#130104,#130105),.UNSPECIFIED.,.F.,.F.,(4,2,4),(3.40689536786532E-11,0.0126499313200275,
0.025300279930029),.UNSPECIFIED.);
#22835=B_SPLINE_CURVE_WITH_KNOTS('',3,(#130133,#130134,#130135,#130136,
#130137,#130138),.UNSPECIFIED.,.F.,.F.,(4,2,4),(0.,0.0126499129678583,0.0253002083264279),
 .UNSPECIFIED.);
#22836=B_SPLINE_CURVE_WITH_KNOTS('',3,(#130166,#130167,#130168,#130169,
#130170,#130171),.UNSPECIFIED.,.F.,.F.,(4,2,4),(0.,0.0126499173031919,0.0253002270982126),
 .UNSPECIFIED.);
#22837=B_SPLINE_CURVE_WITH_KNOTS('',3,(#130199,#130200,#130201,#130202,
#130203,#130204),.UNSPECIFIED.,.F.,.F.,(4,2,4),(0.,0.0126499174786902,0.0253002255234055),
 .UNSPECIFIED.);
#22838=B_SPLINE_CURVE_WITH_KNOTS('',3,(#130229,#130230,#130231,#130232,
#130233,#130234),.UNSPECIFIED.,.F.,.F.,(4,2,4),(0.,0.0126499218690464,0.0253002426716667),
 .UNSPECIFIED.);
#22839=B_SPLINE_CURVE_WITH_KNOTS('',3,(#130256,#130257,#130258,#130259,
#130260,#130261),.UNSPECIFIED.,.F.,.F.,(4,2,4),(3.66601265270061E-13,0.0126499208786554,
0.0253002406126026),.UNSPECIFIED.);
#22840=B_SPLINE_CURVE_WITH_KNOTS('',3,(#130289,#130290,#130291,#130292,
#130293,#130294),.UNSPECIFIED.,.F.,.F.,(4,2,4),(0.,0.0126499118483472,0.025300203303257),
 .UNSPECIFIED.);
#22841=B_SPLINE_CURVE_WITH_KNOTS('',3,(#130322,#130323,#130324,#130325,
#130326,#130327),.UNSPECIFIED.,.F.,.F.,(4,2,4),(0.,0.0126499224943342,0.0253002451178913),
 .UNSPECIFIED.);
#22842=B_SPLINE_CURVE_WITH_KNOTS('',3,(#130355,#130356,#130357,#130358,
#130359,#130360),.UNSPECIFIED.,.F.,.F.,(4,2,4),(0.,0.0126499208891092,0.0253002369915565),
 .UNSPECIFIED.);
#22843=B_SPLINE_CURVE_WITH_KNOTS('',3,(#130388,#130389,#130390,#130391,
#130392,#130393),.UNSPECIFIED.,.F.,.F.,(4,2,4),(0.,0.0126499173509548,0.02530022847158),
 .UNSPECIFIED.);
#22844=B_SPLINE_CURVE_WITH_KNOTS('',3,(#130421,#130422,#130423,#130424,
#130425,#130426),.UNSPECIFIED.,.F.,.F.,(4,2,4),(0.,0.0126499220452902,0.0253002430940821),
 .UNSPECIFIED.);
#22845=B_SPLINE_CURVE_WITH_KNOTS('',3,(#130454,#130455,#130456,#130457,
#130458,#130459),.UNSPECIFIED.,.F.,.F.,(4,2,4),(0.,0.0126499180091474,0.0253002282305368),
 .UNSPECIFIED.);
#22846=B_SPLINE_CURVE_WITH_KNOTS('',3,(#130487,#130488,#130489,#130490,
#130491,#130492),.UNSPECIFIED.,.F.,.F.,(4,2,4),(0.,0.012649918574299,0.0253002280488269),
 .UNSPECIFIED.);
#22847=B_SPLINE_CURVE_WITH_KNOTS('',3,(#130520,#130521,#130522,#130523,
#130524,#130525),.UNSPECIFIED.,.F.,.F.,(4,2,4),(1.8513899150215E-12,0.0126499209523983,
0.0253002401365578),.UNSPECIFIED.);
#22848=B_SPLINE_CURVE_WITH_KNOTS('',3,(#130553,#130554,#130555,#130556,
#130557,#130558),.UNSPECIFIED.,.F.,.F.,(4,2,4),(0.,0.0126499148037353,0.0253002131144609),
 .UNSPECIFIED.);
#22849=B_SPLINE_CURVE_WITH_KNOTS('',3,(#130586,#130587,#130588,#130589,
#130590,#130591),.UNSPECIFIED.,.F.,.F.,(4,2,4),(0.,0.0126499223276825,0.025300244583305),
 .UNSPECIFIED.);
#22850=B_SPLINE_CURVE_WITH_KNOTS('',3,(#130619,#130620,#130621,#130622,
#130623,#130624),.UNSPECIFIED.,.F.,.F.,(4,2,4),(0.,0.0126499138887409,0.0253002122279321),
 .UNSPECIFIED.);
#22851=B_SPLINE_CURVE_WITH_KNOTS('',3,(#130652,#130653,#130654,#130655,
#130656,#130657),.UNSPECIFIED.,.F.,.F.,(4,2,4),(0.,0.0126499283749239,0.025300265794938),
 .UNSPECIFIED.);
#22852=B_SPLINE_CURVE_WITH_KNOTS('',3,(#130685,#130686,#130687,#130688,
#130689,#130690),.UNSPECIFIED.,.F.,.F.,(4,2,4),(5.49015481529974E-12,0.0126499266970771,
0.0253002635542269),.UNSPECIFIED.);
#22853=B_SPLINE_CURVE_WITH_KNOTS('',3,(#130729,#130730,#130731,#130732,
#130733,#130734,#130735,#130736,#130737,#130738),.UNSPECIFIED.,.F.,.F.,
(4,3,3,4),(2.21153070827588E-11,8.70314493453333E-5,0.00017002405947175,
0.000253018845956519),.UNSPECIFIED.);
#22854=B_SPLINE_CURVE_WITH_KNOTS('',3,(#130750,#130751,#130752,#130753,
#130754,#130755,#130756,#130757,#130758,#130759),.UNSPECIFIED.,.F.,.F.,
(4,3,3,4),(0.487155140750431,0.491874896926658,0.501682966399308,0.504614996906574),
 .UNSPECIFIED.);
#22855=B_SPLINE_CURVE_WITH_KNOTS('',3,(#130760,#130761,#130762,#130763,
#130764,#130765,#130766,#130767,#130768,#130769),.UNSPECIFIED.,.F.,.F.,
(4,3,3,4),(3.45096454849108E-14,8.70313175711171E-5,0.000170023946878408,
0.000253018998164665),.UNSPECIFIED.);
#22856=B_SPLINE_CURVE_WITH_KNOTS('',3,(#130788,#130789,#130790,#130791,
#130792,#130793,#130794,#130795,#130796,#130797),.UNSPECIFIED.,.F.,.F.,
(4,3,3,4),(0.487155140750431,0.491874896926659,0.501682934290902,0.504614996906058),
 .UNSPECIFIED.);
#22857=B_SPLINE_CURVE_WITH_KNOTS('',3,(#130798,#130799,#130800,#130801,
#130802,#130803,#130804,#130805,#130806,#130807),.UNSPECIFIED.,.F.,.F.,
(4,3,3,4),(4.42529392960305E-14,8.70313175297394E-5,0.000170023946584964,
0.000253018997273752),.UNSPECIFIED.);
#22858=B_SPLINE_CURVE_WITH_KNOTS('',3,(#130826,#130827,#130828,#130829,
#130830,#130831,#130832,#130833,#130834,#130835),.UNSPECIFIED.,.F.,.F.,
(4,3,3,4),(0.487155141219239,0.491874896926658,0.5016829678529,0.504614997100588),
 .UNSPECIFIED.);
#22859=B_SPLINE_CURVE_WITH_KNOTS('',3,(#130836,#130837,#130838,#130839,
#130840,#130841,#130842,#130843,#130844,#130845),.UNSPECIFIED.,.F.,.F.,
(4,3,3,4),(4.40863300248104E-14,8.70313175424259E-5,0.000170023946631832,
0.000253018997693025),.UNSPECIFIED.);
#22860=B_SPLINE_CURVE_WITH_KNOTS('',3,(#130864,#130865,#130866,#130867,
#130868,#130869,#130870,#130871,#130872,#130873),.UNSPECIFIED.,.F.,.F.,
(4,3,3,4),(0.48715514075043,0.491874896926658,0.501682951102274,0.504614996907853),
 .UNSPECIFIED.);
#22861=B_SPLINE_CURVE_WITH_KNOTS('',3,(#130874,#130875,#130876,#130877,
#130878,#130879,#130880,#130881,#130882,#130883),.UNSPECIFIED.,.F.,.F.,
(4,3,3,4),(3.46722191321165E-14,8.70313175915362E-5,0.000170023946671659,
0.00025301899802548),.UNSPECIFIED.);
#22862=B_SPLINE_CURVE_WITH_KNOTS('',3,(#130902,#130903,#130904,#130905,
#130906,#130907,#130908,#130909,#130910,#130911),.UNSPECIFIED.,.F.,.F.,
(4,3,3,4),(0.487155140750431,0.491874896926659,0.501682951028305,0.50461499691759),
 .UNSPECIFIED.);
#22863=B_SPLINE_CURVE_WITH_KNOTS('',3,(#130912,#130913,#130914,#130915,
#130916,#130917,#130918,#130919,#130920,#130921),.UNSPECIFIED.,.F.,.F.,
(4,3,3,4),(4.40712627940313E-15,8.70313176441398E-5,0.000170023946915369,
0.000253018998042543),.UNSPECIFIED.);
#22864=B_SPLINE_CURVE_WITH_KNOTS('',3,(#130940,#130941,#130942,#130943,
#130944,#130945,#130946,#130947,#130948,#130949),.UNSPECIFIED.,.F.,.F.,
(4,3,3,4),(0.48715514075043,0.491874896926657,0.501682983217295,0.504614996910036),
 .UNSPECIFIED.);
#22865=B_SPLINE_CURVE_WITH_KNOTS('',3,(#130950,#130951,#130952,#130953,
#130954,#130955,#130956,#130957,#130958,#130959),.UNSPECIFIED.,.F.,.F.,
(4,3,3,4),(2.20993341838628E-14,8.7031317575276E-5,0.000170023946675526,
0.000253018997790063),.UNSPECIFIED.);
#22866=B_SPLINE_CURVE_WITH_KNOTS('',3,(#130978,#130979,#130980,#130981,
#130982,#130983,#130984,#130985,#130986,#130987),.UNSPECIFIED.,.F.,.F.,
(4,3,3,4),(0.487155140750431,0.491874896926659,0.501682969053896,0.504614996915088),
 .UNSPECIFIED.);
#22867=B_SPLINE_CURVE_WITH_KNOTS('',3,(#130988,#130989,#130990,#130991,
#130992,#130993,#130994,#130995,#130996,#130997),.UNSPECIFIED.,.F.,.F.,
(4,3,3,4),(1.50225347390965E-14,8.70313178726407E-5,0.000170023946784008,
0.000253018997413668),.UNSPECIFIED.);
#22868=B_SPLINE_CURVE_WITH_KNOTS('',3,(#131016,#131017,#131018,#131019,
#131020,#131021,#131022,#131023,#131024,#131025),.UNSPECIFIED.,.F.,.F.,
(4,3,3,4),(0.487155140750431,0.491874896926659,0.501682955711557,0.5046149968907),
 .UNSPECIFIED.);
#22869=B_SPLINE_CURVE_WITH_KNOTS('',3,(#131026,#131027,#131028,#131029,
#131030,#131031,#131032,#131033,#131034,#131035),.UNSPECIFIED.,.F.,.F.,
(4,3,3,4),(2.40986300177914E-14,8.70313176284771E-5,0.000170023946621484,
0.000253018997382508),.UNSPECIFIED.);
#22870=B_SPLINE_CURVE_WITH_KNOTS('',3,(#131054,#131055,#131056,#131057,
#131058,#131059,#131060,#131061,#131062,#131063),.UNSPECIFIED.,.F.,.F.,
(4,3,3,4),(0.487155140750431,0.491874896926659,0.501682948684918,0.504614996896031),
 .UNSPECIFIED.);
#22871=B_SPLINE_CURVE_WITH_KNOTS('',3,(#131064,#131065,#131066,#131067,
#131068,#131069,#131070,#131071,#131072,#131073),.UNSPECIFIED.,.F.,.F.,
(4,3,3,4),(5.11111839094562E-14,8.70313176670455E-5,0.000170023946742311,
0.000253018998036814),.UNSPECIFIED.);
#22872=B_SPLINE_CURVE_WITH_KNOTS('',3,(#131092,#131093,#131094,#131095,
#131096,#131097,#131098,#131099,#131100,#131101),.UNSPECIFIED.,.F.,.F.,
(4,3,3,4),(0.487155140750431,0.491874896926659,0.501682945300711,0.504614996917612),
 .UNSPECIFIED.);
#22873=B_SPLINE_CURVE_WITH_KNOTS('',3,(#131102,#131103,#131104,#131105,
#131106,#131107,#131108,#131109,#131110,#131111),.UNSPECIFIED.,.F.,.F.,
(4,3,3,4),(1.09252828245397E-14,8.70313177939855E-5,0.000170023946750202,
0.000253018997298873),.UNSPECIFIED.);
#22874=B_SPLINE_CURVE_WITH_KNOTS('',3,(#131130,#131131,#131132,#131133,
#131134,#131135,#131136,#131137,#131138,#131139),.UNSPECIFIED.,.F.,.F.,
(4,3,3,4),(0.487155140750431,0.491874896926659,0.501682936956871,0.504614996892545),
 .UNSPECIFIED.);
#22875=B_SPLINE_CURVE_WITH_KNOTS('',3,(#131140,#131141,#131142,#131143,
#131144,#131145,#131146,#131147,#131148,#131149),.UNSPECIFIED.,.F.,.F.,
(4,3,3,4),(8.03179267346919E-14,8.70313175544202E-5,0.00017002394659626,
0.000253018998009225),.UNSPECIFIED.);
#22876=B_SPLINE_CURVE_WITH_KNOTS('',3,(#131168,#131169,#131170,#131171,
#131172,#131173,#131174,#131175,#131176,#131177),.UNSPECIFIED.,.F.,.F.,
(4,3,3,4),(0.487155140750431,0.491874896926659,0.50168294484991,0.504614996903372),
 .UNSPECIFIED.);
#22877=B_SPLINE_CURVE_WITH_KNOTS('',3,(#131178,#131179,#131180,#131181,
#131182,#131183,#131184,#131185,#131186,#131187),.UNSPECIFIED.,.F.,.F.,
(4,3,3,4),(2.68559350286825E-15,8.70313176641771E-5,0.000170023946805897,
0.000253018998059253),.UNSPECIFIED.);
#22878=B_SPLINE_CURVE_WITH_KNOTS('',3,(#131206,#131207,#131208,#131209,
#131210,#131211,#131212,#131213,#131214,#131215),.UNSPECIFIED.,.F.,.F.,
(4,3,3,4),(0.487155140750431,0.491874896926659,0.501682963492984,0.504614996928294),
 .UNSPECIFIED.);
#22879=B_SPLINE_CURVE_WITH_KNOTS('',3,(#131216,#131217,#131218,#131219,
#131220,#131221,#131222,#131223,#131224,#131225),.UNSPECIFIED.,.F.,.F.,
(4,3,3,4),(5.89210988424711E-14,8.70313175998042E-5,0.000170023946622594,
0.000253018997350292),.UNSPECIFIED.);
#22880=B_SPLINE_CURVE_WITH_KNOTS('',3,(#131244,#131245,#131246,#131247,
#131248,#131249,#131250,#131251,#131252,#131253),.UNSPECIFIED.,.F.,.F.,
(4,3,3,4),(0.487155140750431,0.491874896926659,0.501682946832188,0.504614996917156),
 .UNSPECIFIED.);
#22881=B_SPLINE_CURVE_WITH_KNOTS('',3,(#131254,#131255,#131256,#131257,
#131258,#131259,#131260,#131261,#131262,#131263),.UNSPECIFIED.,.F.,.F.,
(4,3,3,4),(2.38020884134642E-14,8.70313176307367E-5,0.000170023946762134,
0.000253018997722667),.UNSPECIFIED.);
#22882=B_SPLINE_CURVE_WITH_KNOTS('',3,(#131282,#131283,#131284,#131285,
#131286,#131287,#131288,#131289,#131290,#131291),.UNSPECIFIED.,.F.,.F.,
(4,3,3,4),(0.487155140750431,0.491874896926659,0.501682964139925,0.504614996914888),
 .UNSPECIFIED.);
#22883=B_SPLINE_CURVE_WITH_KNOTS('',3,(#131292,#131293,#131294,#131295,
#131296,#131297,#131298,#131299,#131300,#131301),.UNSPECIFIED.,.F.,.F.,
(4,3,3,4),(5.46374512450486E-14,8.70313176102908E-5,0.000170023946589689,
0.000253018997649783),.UNSPECIFIED.);
#22884=B_SPLINE_CURVE_WITH_KNOTS('',3,(#131320,#131321,#131322,#131323,
#131324,#131325,#131326,#131327,#131328,#131329),.UNSPECIFIED.,.F.,.F.,
(4,3,3,4),(0.487155140750431,0.491874896926659,0.501682932609467,0.504614996903104),
 .UNSPECIFIED.);
#22885=B_SPLINE_CURVE_WITH_KNOTS('',3,(#131330,#131331,#131332,#131333,
#131334,#131335,#131336,#131337,#131338,#131339),.UNSPECIFIED.,.F.,.F.,
(4,3,3,4),(3.40449100493074E-14,8.70313176981428E-5,0.000170023946803936,
0.000253018997932282),.UNSPECIFIED.);
#22886=B_SPLINE_CURVE_WITH_KNOTS('',3,(#131358,#131359,#131360,#131361,
#131362,#131363,#131364,#131365,#131366,#131367),.UNSPECIFIED.,.F.,.F.,
(4,3,3,4),(0.487155140750431,0.491874896926659,0.501682979942645,0.504614996909924),
 .UNSPECIFIED.);
#22887=B_SPLINE_CURVE_WITH_KNOTS('',3,(#131368,#131369,#131370,#131371,
#131372,#131373,#131374,#131375,#131376,#131377),.UNSPECIFIED.,.F.,.F.,
(4,3,3,4),(7.04341793940837E-14,8.70313175559068E-5,0.000170023946529521,
0.000253018997753187),.UNSPECIFIED.);
#22888=B_SPLINE_CURVE_WITH_KNOTS('',3,(#131396,#131397,#131398,#131399,
#131400,#131401,#131402,#131403,#131404,#131405),.UNSPECIFIED.,.F.,.F.,
(4,3,3,4),(0.487155140750431,0.491874896926659,0.501682957929202,0.504614996911627),
 .UNSPECIFIED.);
#22889=B_SPLINE_CURVE_WITH_KNOTS('',3,(#131406,#131407,#131408,#131409,
#131410,#131411,#131412,#131413,#131414,#131415),.UNSPECIFIED.,.F.,.F.,
(4,3,3,4),(5.8236891808638E-14,8.70313175937467E-5,0.00017002394674638,
0.000253018997690592),.UNSPECIFIED.);
#22890=B_SPLINE_CURVE_WITH_KNOTS('',3,(#131434,#131435,#131436,#131437,
#131438,#131439,#131440,#131441,#131442,#131443),.UNSPECIFIED.,.F.,.F.,
(4,3,3,4),(0.487155140750431,0.491874896926659,0.501682960207111,0.504614996926001),
 .UNSPECIFIED.);
#22891=B_SPLINE_CURVE_WITH_KNOTS('',3,(#131444,#131445,#131446,#131447,
#131448,#131449,#131450,#131451,#131452,#131453),.UNSPECIFIED.,.F.,.F.,
(4,3,3,4),(4.35401475432296E-14,8.70313176778195E-5,0.000170023946767764,
0.000253018997628577),.UNSPECIFIED.);
#22892=B_SPLINE_CURVE_WITH_KNOTS('',3,(#131472,#131473,#131474,#131475,
#131476,#131477,#131478,#131479,#131480,#131481),.UNSPECIFIED.,.F.,.F.,
(4,3,3,4),(0.487155140750431,0.491874896926659,0.50168295550842,0.504614996916598),
 .UNSPECIFIED.);
#22893=B_SPLINE_CURVE_WITH_KNOTS('',3,(#131482,#131483,#131484,#131485,
#131486,#131487,#131488,#131489,#131490,#131491),.UNSPECIFIED.,.F.,.F.,
(4,3,3,4),(1.62990603401336E-14,8.70313177195538E-5,0.000170023946752221,
0.000253018997668107),.UNSPECIFIED.);
#22894=B_SPLINE_CURVE_WITH_KNOTS('',3,(#131510,#131511,#131512,#131513,
#131514,#131515,#131516,#131517,#131518,#131519),.UNSPECIFIED.,.F.,.F.,
(4,3,3,4),(0.487155140750431,0.491874896926659,0.501682952896135,0.504614996920383),
 .UNSPECIFIED.);
#22895=B_SPLINE_CURVE_WITH_KNOTS('',3,(#131520,#131521,#131522,#131523,
#131524,#131525,#131526,#131527,#131528,#131529),.UNSPECIFIED.,.F.,.F.,
(4,3,3,4),(1.90242114645572E-14,8.70313177274409E-5,0.000170023946650131,
0.000253018997500558),.UNSPECIFIED.);
#22896=B_SPLINE_CURVE_WITH_KNOTS('',3,(#131548,#131549,#131550,#131551,
#131552,#131553,#131554,#131555,#131556,#131557),.UNSPECIFIED.,.F.,.F.,
(4,3,3,4),(0.487155140750322,0.491874896944685,0.501682945346985,0.5046149969228),
 .UNSPECIFIED.);
#22897=B_SPLINE_CURVE_WITH_KNOTS('',3,(#131558,#131559,#131560,#131561,
#131562,#131563,#131564,#131565,#131566,#131567),.UNSPECIFIED.,.F.,.F.,
(4,3,3,4),(4.49589306676502E-14,8.70313176364226E-5,0.000170023946820726,
0.000253018998381774),.UNSPECIFIED.);
#22898=B_SPLINE_CURVE_WITH_KNOTS('',3,(#131586,#131587,#131588,#131589,
#131590,#131591,#131592,#131593,#131594,#131595),.UNSPECIFIED.,.F.,.F.,
(4,3,3,4),(0.48715514075043,0.491874896926657,0.501682938066946,0.504614996890883),
 .UNSPECIFIED.);
#22899=B_SPLINE_CURVE_WITH_KNOTS('',3,(#131596,#131597,#131598,#131599,
#131600,#131601,#131602,#131603,#131604,#131605),.UNSPECIFIED.,.F.,.F.,
(4,3,3,4),(6.45004693156233E-14,8.70313176737041E-5,0.000170023946903362,
0.000253018998072501),.UNSPECIFIED.);
#22900=B_SPLINE_CURVE_WITH_KNOTS('',3,(#131624,#131625,#131626,#131627,
#131628,#131629,#131630,#131631,#131632,#131633),.UNSPECIFIED.,.F.,.F.,
(4,3,3,4),(0.487155140750429,0.491874896926656,0.501682960511284,0.504614996906757),
 .UNSPECIFIED.);
#22901=B_SPLINE_CURVE_WITH_KNOTS('',3,(#131634,#131635,#131636,#131637,
#131638,#131639,#131640,#131641,#131642,#131643),.UNSPECIFIED.,.F.,.F.,
(4,3,3,4),(8.58872897030667E-14,8.70313175901969E-5,0.000170023946786314,
0.000253018997863018),.UNSPECIFIED.);
#22902=B_SPLINE_CURVE_WITH_KNOTS('',3,(#131662,#131663,#131664,#131665,
#131666,#131667,#131668,#131669,#131670,#131671),.UNSPECIFIED.,.F.,.F.,
(4,3,3,4),(0.487155140750429,0.491874896926656,0.501682948681635,0.504614996927245),
 .UNSPECIFIED.);
#22903=B_SPLINE_CURVE_WITH_KNOTS('',3,(#131672,#131673,#131674,#131675,
#131676,#131677,#131678,#131679,#131680,#131681),.UNSPECIFIED.,.F.,.F.,
(4,3,3,4),(2.08206417731207E-14,8.70313174616608E-5,0.000170023946642585,
0.000253018998155892),.UNSPECIFIED.);
#22904=B_SPLINE_CURVE_WITH_KNOTS('',3,(#131700,#131701,#131702,#131703,
#131704,#131705,#131706,#131707,#131708,#131709),.UNSPECIFIED.,.F.,.F.,
(4,3,3,4),(0.487155140750429,0.491874896926656,0.501682945866074,0.504614996901574),
 .UNSPECIFIED.);
#22905=B_SPLINE_CURVE_WITH_KNOTS('',3,(#131710,#131711,#131712,#131713,
#131714,#131715,#131716,#131717,#131718,#131719),.UNSPECIFIED.,.F.,.F.,
(4,3,3,4),(2.48137664125078E-14,8.70313177460333E-5,0.000170023946742254,
0.000253018997272817),.UNSPECIFIED.);
#22906=B_SPLINE_CURVE_WITH_KNOTS('',3,(#131738,#131739,#131740,#131741,
#131742,#131743,#131744,#131745,#131746,#131747),.UNSPECIFIED.,.F.,.F.,
(4,3,3,4),(0.48715514075043,0.491874896926657,0.50168298795909,0.504614996907841),
 .UNSPECIFIED.);
#22907=B_SPLINE_CURVE_WITH_KNOTS('',3,(#131748,#131749,#131750,#131751,
#131752,#131753,#131754,#131755,#131756,#131757),.UNSPECIFIED.,.F.,.F.,
(4,3,3,4),(3.3796818005368E-14,8.70313175545553E-5,0.000170023946800974,
0.000253018997690298),.UNSPECIFIED.);
#22908=B_SPLINE_CURVE_WITH_KNOTS('',3,(#131776,#131777,#131778,#131779,
#131780,#131781,#131782,#131783,#131784,#131785),.UNSPECIFIED.,.F.,.F.,
(4,3,3,4),(0.487155140750429,0.491874896926655,0.501682932157906,0.504614996931886),
 .UNSPECIFIED.);
#22909=B_SPLINE_CURVE_WITH_KNOTS('',3,(#131786,#131787,#131788,#131789,
#131790,#131791,#131792,#131793,#131794,#131795),.UNSPECIFIED.,.F.,.F.,
(4,3,3,4),(2.07661001644807E-15,8.70313175311407E-5,0.000170023946662789,
0.000253018997995876),.UNSPECIFIED.);
#22910=B_SPLINE_CURVE_WITH_KNOTS('',3,(#131813,#131814,#131815,#131816,
#131817,#131818,#131819,#131820,#131821,#131822),.UNSPECIFIED.,.F.,.F.,
(4,3,3,4),(0.487155140750429,0.491874896926655,0.501682941477529,0.504614996918119),
 .UNSPECIFIED.);
#22911=B_SPLINE_CURVE_WITH_KNOTS('',3,(#131830,#131831,#131832,#131833,
#131834,#131835),.UNSPECIFIED.,.F.,.F.,(4,2,4),(1.57854982172886E-9,0.0126517047617616,
0.0253036326772259),.UNSPECIFIED.);
#22912=B_SPLINE_CURVE_WITH_KNOTS('',3,(#131849,#131850,#131851,#131852,
#131853,#131854),.UNSPECIFIED.,.F.,.F.,(4,2,4),(2.36098174900286E-11,0.012651852400468,
0.0253034805000543),.UNSPECIFIED.);
#22913=B_SPLINE_CURVE_WITH_KNOTS('',3,(#131877,#131878,#131879,#131880,
#131881,#131882),.UNSPECIFIED.,.F.,.F.,(4,2,4),(3.720761616377E-11,0.0126518524995529,
0.0253034806719167),.UNSPECIFIED.);
#22914=B_SPLINE_CURVE_WITH_KNOTS('',3,(#131905,#131906,#131907,#131908,
#131909,#131910),.UNSPECIFIED.,.F.,.F.,(4,2,4),(3.31366397850511E-11,0.0126518524135823,
0.0253034805076842),.UNSPECIFIED.);
#22915=B_SPLINE_CURVE_WITH_KNOTS('',3,(#131933,#131934,#131935,#131936,
#131937,#131938),.UNSPECIFIED.,.F.,.F.,(4,2,4),(1.35863014051303E-11,0.0126518524614331,
0.0253034806458099),.UNSPECIFIED.);
#22916=B_SPLINE_CURVE_WITH_KNOTS('',3,(#131961,#131962,#131963,#131964,
#131965,#131966),.UNSPECIFIED.,.F.,.F.,(4,2,4),(4.31669193783089E-11,0.0126518524382602,
0.0253034805401726),.UNSPECIFIED.);
#22917=B_SPLINE_CURVE_WITH_KNOTS('',3,(#131989,#131990,#131991,#131992,
#131993,#131994),.UNSPECIFIED.,.F.,.F.,(4,2,4),(6.96683009010555E-11,0.0126518525612664,
0.0253034807264326),.UNSPECIFIED.);
#22918=B_SPLINE_CURVE_WITH_KNOTS('',3,(#132017,#132018,#132019,#132020,
#132021,#132022),.UNSPECIFIED.,.F.,.F.,(4,2,4),(4.19890970197388E-11,0.0126518524349447,
0.0253034805319675),.UNSPECIFIED.);
#22919=B_SPLINE_CURVE_WITH_KNOTS('',3,(#132045,#132046,#132047,#132048,
#132049,#132050),.UNSPECIFIED.,.F.,.F.,(4,2,4),(4.79039532650115E-11,0.0126518525289848,
0.025303480711971),.UNSPECIFIED.);
#22920=B_SPLINE_CURVE_WITH_KNOTS('',3,(#132073,#132074,#132075,#132076,
#132077,#132078),.UNSPECIFIED.,.F.,.F.,(4,2,4),(4.44665067478317E-11,0.0126518525087782,
0.0253034806759089),.UNSPECIFIED.);
#22921=B_SPLINE_CURVE_WITH_KNOTS('',3,(#132101,#132102,#132103,#132104,
#132105,#132106),.UNSPECIFIED.,.F.,.F.,(4,2,4),(3.72079750079819E-11,0.0126518524179389,
0.0253034805068538),.UNSPECIFIED.);
#22922=B_SPLINE_CURVE_WITH_KNOTS('',3,(#132129,#132130,#132131,#132132,
#132133,#132134),.UNSPECIFIED.,.F.,.F.,(4,2,4),(3.82846828684018E-11,0.0126518524409263,
0.0253034805527796),.UNSPECIFIED.);
#22923=B_SPLINE_CURVE_WITH_KNOTS('',3,(#132157,#132158,#132159,#132160,
#132161,#132162),.UNSPECIFIED.,.F.,.F.,(4,2,4),(1.79986607487896E-11,0.0126518524642799,
0.0253034806422095),.UNSPECIFIED.);
#22924=B_SPLINE_CURVE_WITH_KNOTS('',3,(#132185,#132186,#132187,#132188,
#132189,#132190),.UNSPECIFIED.,.F.,.F.,(4,2,4),(4.07151250871006E-11,0.012651852533892,
0.0253034807373435),.UNSPECIFIED.);
#22925=B_SPLINE_CURVE_WITH_KNOTS('',3,(#132213,#132214,#132215,#132216,
#132217,#132218),.UNSPECIFIED.,.F.,.F.,(4,2,4),(2.20594989622044E-9,0.0126518535108752,
0.025303480534335),.UNSPECIFIED.);
#22926=B_SPLINE_CURVE_WITH_KNOTS('',3,(#132241,#132242,#132243,#132244,
#132245,#132246),.UNSPECIFIED.,.F.,.F.,(4,2,4),(1.399374402428E-11,0.0126518524586418,
0.0253034806364679),.UNSPECIFIED.);
#22927=B_SPLINE_CURVE_WITH_KNOTS('',3,(#132269,#132270,#132271,#132272,
#132273,#132274),.UNSPECIFIED.,.F.,.F.,(4,2,4),(3.74743840632193E-11,0.0126518525084182,
0.025303480686356),.UNSPECIFIED.);
#22928=B_SPLINE_CURVE_WITH_KNOTS('',3,(#132297,#132298,#132299,#132300,
#132301,#132302),.UNSPECIFIED.,.F.,.F.,(4,2,4),(4.5835016463154E-11,0.0126518524280129,
0.0253034805099347),.UNSPECIFIED.);
#22929=B_SPLINE_CURVE_WITH_KNOTS('',3,(#132325,#132326,#132327,#132328,
#132329,#132330),.UNSPECIFIED.,.F.,.F.,(4,2,4),(3.4966361747514E-11,0.0126518524971628,
0.0253034806732593),.UNSPECIFIED.);
#22930=B_SPLINE_CURVE_WITH_KNOTS('',3,(#132353,#132354,#132355,#132356,
#132357,#132358),.UNSPECIFIED.,.F.,.F.,(4,2,4),(3.97303333440308E-11,0.012651852433962,
0.0253034805347979),.UNSPECIFIED.);
#22931=B_SPLINE_CURVE_WITH_KNOTS('',3,(#132381,#132382,#132383,#132384,
#132385,#132386),.UNSPECIFIED.,.F.,.F.,(4,2,4),(3.27648748939136E-11,0.0126518525041262,
0.0253034806924794),.UNSPECIFIED.);
#22932=B_SPLINE_CURVE_WITH_KNOTS('',3,(#132409,#132410,#132411,#132412,
#132413,#132414),.UNSPECIFIED.,.F.,.F.,(4,2,4),(3.36371781765561E-11,0.0126518524974542,
0.0253034806785961),.UNSPECIFIED.);
#22933=B_SPLINE_CURVE_WITH_KNOTS('',3,(#132437,#132438,#132439,#132440,
#132441,#132442),.UNSPECIFIED.,.F.,.F.,(4,2,4),(2.79900002971549E-11,0.0126518524054462,
0.0253034805046033),.UNSPECIFIED.);
#22934=B_SPLINE_CURVE_WITH_KNOTS('',3,(#132465,#132466,#132467,#132468,
#132469,#132470),.UNSPECIFIED.,.F.,.F.,(4,2,4),(1.61552872164343E-11,0.0126518523983396,
0.0253034805129489),.UNSPECIFIED.);
#22935=B_SPLINE_CURVE_WITH_KNOTS('',3,(#132493,#132494,#132495,#132496,
#132497,#132498),.UNSPECIFIED.,.F.,.F.,(4,2,4),(3.59283638053901E-11,0.0126518525083403,
0.0253034806945798),.UNSPECIFIED.);
#22936=B_SPLINE_CURVE_WITH_KNOTS('',3,(#132521,#132522,#132523,#132524,
#132525,#132526),.UNSPECIFIED.,.F.,.F.,(4,2,4),(3.19092675899861E-11,0.0126518524958068,
0.0253034806753266),.UNSPECIFIED.);
#22937=B_SPLINE_CURVE_WITH_KNOTS('',3,(#132549,#132550,#132551,#132552,
#132553,#132554),.UNSPECIFIED.,.F.,.F.,(4,2,4),(5.01111450311739E-11,0.0126518524534616,
0.0253034805513483),.UNSPECIFIED.);
#22938=B_SPLINE_CURVE_WITH_KNOTS('',3,(#132577,#132578,#132579,#132580,
#132581,#132582),.UNSPECIFIED.,.F.,.F.,(4,2,4),(3.86162407489939E-11,0.0126518525018019,
0.0253034806727814),.UNSPECIFIED.);
#22939=B_SPLINE_CURVE_WITH_KNOTS('',3,(#132605,#132606,#132607,#132608,
#132609,#132610),.UNSPECIFIED.,.F.,.F.,(4,2,4),(2.26099460019981E-11,0.0126518524785923,
0.0253034806615711),.UNSPECIFIED.);
#22940=B_SPLINE_CURVE_WITH_KNOTS('',3,(#132646,#132647,#132648,#132649,
#132650,#132651),.UNSPECIFIED.,.F.,.F.,(4,2,4),(0.,0.012650581650196,0.025301429662558),
 .UNSPECIFIED.);
#22941=B_SPLINE_CURVE_WITH_KNOTS('',3,(#132658,#132659,#132660,#132661,
#132662,#132663,#132664),.UNSPECIFIED.,.F.,.F.,(4,3,4),(0.492524364188282,
0.5,0.504719756176227),.UNSPECIFIED.);
#22942=B_SPLINE_CURVE_WITH_KNOTS('',3,(#132685,#132686,#132687,#132688,
#132689,#132690),.UNSPECIFIED.,.F.,.F.,(4,2,4),(0.,0.0126505787819665,0.0253014176959488),
 .UNSPECIFIED.);
#22943=B_SPLINE_CURVE_WITH_KNOTS('',3,(#132697,#132698,#132699,#132700,
#132701,#132702,#132703),.UNSPECIFIED.,.F.,.F.,(4,3,4),(0.492524364190509,
0.5,0.504719756176228),.UNSPECIFIED.);
#22944=B_SPLINE_CURVE_WITH_KNOTS('',3,(#132724,#132725,#132726,#132727,
#132728,#132729),.UNSPECIFIED.,.F.,.F.,(4,2,4),(0.,0.0126505799555268,0.0253014225909201),
 .UNSPECIFIED.);
#22945=B_SPLINE_CURVE_WITH_KNOTS('',3,(#132736,#132737,#132738,#132739,
#132740,#132741,#132742),.UNSPECIFIED.,.F.,.F.,(4,3,4),(0.492524364184477,
0.5,0.504719756176228),.UNSPECIFIED.);
#22946=B_SPLINE_CURVE_WITH_KNOTS('',3,(#132763,#132764,#132765,#132766,
#132767,#132768),.UNSPECIFIED.,.F.,.F.,(4,2,4),(0.,0.0126505812154814,0.0253014191594166),
 .UNSPECIFIED.);
#22947=B_SPLINE_CURVE_WITH_KNOTS('',3,(#132775,#132776,#132777,#132778,
#132779,#132780,#132781),.UNSPECIFIED.,.F.,.F.,(4,3,4),(0.492524364184568,
0.5,0.504719756176228),.UNSPECIFIED.);
#22948=B_SPLINE_CURVE_WITH_KNOTS('',3,(#132802,#132803,#132804,#132805,
#132806,#132807),.UNSPECIFIED.,.F.,.F.,(4,2,4),(0.,0.0126505803545275,0.025301424226586),
 .UNSPECIFIED.);
#22949=B_SPLINE_CURVE_WITH_KNOTS('',3,(#132814,#132815,#132816,#132817,
#132818,#132819,#132820),.UNSPECIFIED.,.F.,.F.,(4,3,4),(0.492524364187926,
0.5,0.504719756176228),.UNSPECIFIED.);
#22950=B_SPLINE_CURVE_WITH_KNOTS('',3,(#132841,#132842,#132843,#132844,
#132845,#132846),.UNSPECIFIED.,.F.,.F.,(4,2,4),(0.,0.0126505775499235,0.0253014126906162),
 .UNSPECIFIED.);
#22951=B_SPLINE_CURVE_WITH_KNOTS('',3,(#132853,#132854,#132855,#132856,
#132857,#132858,#132859),.UNSPECIFIED.,.F.,.F.,(4,3,4),(0.492524364187916,
0.5,0.504719756176227),.UNSPECIFIED.);
#22952=B_SPLINE_CURVE_WITH_KNOTS('',3,(#132880,#132881,#132882,#132883,
#132884,#132885),.UNSPECIFIED.,.F.,.F.,(4,2,4),(0.,0.0126505808589483,0.0253014264769213),
 .UNSPECIFIED.);
#22953=B_SPLINE_CURVE_WITH_KNOTS('',3,(#132892,#132893,#132894,#132895,
#132896,#132897,#132898),.UNSPECIFIED.,.F.,.F.,(4,3,4),(0.492524364186843,
0.5,0.504719756176228),.UNSPECIFIED.);
#22954=B_SPLINE_CURVE_WITH_KNOTS('',3,(#132919,#132920,#132921,#132922,
#132923,#132924),.UNSPECIFIED.,.F.,.F.,(4,2,4),(0.,0.0126505811248473,0.02530142745166),
 .UNSPECIFIED.);
#22955=B_SPLINE_CURVE_WITH_KNOTS('',3,(#132931,#132932,#132933,#132934,
#132935,#132936,#132937),.UNSPECIFIED.,.F.,.F.,(4,3,4),(0.492524364186291,
0.5,0.504719756176228),.UNSPECIFIED.);
#22956=B_SPLINE_CURVE_WITH_KNOTS('',3,(#132958,#132959,#132960,#132961,
#132962,#132963),.UNSPECIFIED.,.F.,.F.,(4,2,4),(0.,0.0126505818313986,0.0253014303880561),
 .UNSPECIFIED.);
#22957=B_SPLINE_CURVE_WITH_KNOTS('',3,(#132995,#132996,#132997,#132998,
#132999,#133000),.UNSPECIFIED.,.F.,.F.,(4,2,4),(0.,0.0126505798191397,0.0253014219508626),
 .UNSPECIFIED.);
#22958=B_SPLINE_CURVE_WITH_KNOTS('',3,(#133007,#133008,#133009,#133010,
#133011,#133012,#133013),.UNSPECIFIED.,.F.,.F.,(4,3,4),(0.492524364187932,
0.5,0.504719756176228),.UNSPECIFIED.);
#22959=B_SPLINE_CURVE_WITH_KNOTS('',3,(#133034,#133035,#133036,#133037,
#133038,#133039),.UNSPECIFIED.,.F.,.F.,(4,2,4),(0.,0.0126505777803537,0.0253014137319526),
 .UNSPECIFIED.);
#22960=B_SPLINE_CURVE_WITH_KNOTS('',3,(#133046,#133047,#133048,#133049,
#133050,#133051,#133052),.UNSPECIFIED.,.F.,.F.,(4,3,4),(0.492524364188889,
0.5,0.504719756176228),.UNSPECIFIED.);
#22961=B_SPLINE_CURVE_WITH_KNOTS('',3,(#133073,#133074,#133075,#133076,
#133077,#133078),.UNSPECIFIED.,.F.,.F.,(4,2,4),(0.,0.0126505789353812,0.0253014184523535),
 .UNSPECIFIED.);
#22962=B_SPLINE_CURVE_WITH_KNOTS('',3,(#133085,#133086,#133087,#133088,
#133089,#133090,#133091),.UNSPECIFIED.,.F.,.F.,(4,3,4),(0.492524364188364,
0.5,0.504719756176228),.UNSPECIFIED.);
#22963=B_SPLINE_CURVE_WITH_KNOTS('',3,(#133112,#133113,#133114,#133115,
#133116,#133117),.UNSPECIFIED.,.F.,.F.,(4,2,4),(0.,0.0126505814576675,0.0253014288471314),
 .UNSPECIFIED.);
#22964=B_SPLINE_CURVE_WITH_KNOTS('',3,(#133124,#133125,#133126,#133127,
#133128,#133129,#133130),.UNSPECIFIED.,.F.,.F.,(4,3,4),(0.49252436418111,
0.5,0.504719756176228),.UNSPECIFIED.);
#22965=B_SPLINE_CURVE_WITH_KNOTS('',3,(#133151,#133152,#133153,#133154,
#133155,#133156),.UNSPECIFIED.,.F.,.F.,(4,2,4),(0.,0.0126505805067179,0.0253014249386929),
 .UNSPECIFIED.);
#22966=B_SPLINE_CURVE_WITH_KNOTS('',3,(#133163,#133164,#133165,#133166,
#133167,#133168,#133169),.UNSPECIFIED.,.F.,.F.,(4,3,4),(0.49252436418881,
0.5,0.504719756176228),.UNSPECIFIED.);
#22967=B_SPLINE_CURVE_WITH_KNOTS('',3,(#133187,#133188,#133189,#133190,
#133191,#133192),.UNSPECIFIED.,.F.,.F.,(4,2,4),(0.,0.0126505788899671,0.0253014181768197),
 .UNSPECIFIED.);
#22968=B_SPLINE_CURVE_WITH_KNOTS('',3,(#133214,#133215,#133216,#133217,
#133218,#133219),.UNSPECIFIED.,.F.,.F.,(4,2,4),(0.,0.0126505816109507,0.0253014294816165),
 .UNSPECIFIED.);
#22969=B_SPLINE_CURVE_WITH_KNOTS('',3,(#133226,#133227,#133228,#133229,
#133230,#133231,#133232),.UNSPECIFIED.,.F.,.F.,(4,3,4),(0.492524364186993,
0.5,0.504719756176228),.UNSPECIFIED.);
#22970=B_SPLINE_CURVE_WITH_KNOTS('',3,(#133253,#133254,#133255,#133256,
#133257,#133258),.UNSPECIFIED.,.F.,.F.,(4,2,4),(0.,0.0126505803329357,0.0253014241800918),
 .UNSPECIFIED.);
#22971=B_SPLINE_CURVE_WITH_KNOTS('',3,(#133265,#133266,#133267,#133268,
#133269,#133270,#133271),.UNSPECIFIED.,.F.,.F.,(4,3,4),(0.49252436418892,
0.5,0.504719756176228),.UNSPECIFIED.);
#22972=B_SPLINE_CURVE_WITH_KNOTS('',3,(#133292,#133293,#133294,#133295,
#133296,#133297),.UNSPECIFIED.,.F.,.F.,(4,2,4),(0.,0.0126505772916147,0.025301411659512),
 .UNSPECIFIED.);
#22973=B_SPLINE_CURVE_WITH_KNOTS('',3,(#133304,#133305,#133306,#133307,
#133308,#133309,#133310),.UNSPECIFIED.,.F.,.F.,(4,3,4),(0.492524364186463,
0.5,0.504719756176228),.UNSPECIFIED.);
#22974=B_SPLINE_CURVE_WITH_KNOTS('',3,(#133331,#133332,#133333,#133334,
#133335,#133336),.UNSPECIFIED.,.F.,.F.,(4,2,4),(0.,0.0126505800967122,0.0253014231919566),
 .UNSPECIFIED.);
#22975=B_SPLINE_CURVE_WITH_KNOTS('',3,(#133343,#133344,#133345,#133346,
#133347,#133348,#133349),.UNSPECIFIED.,.F.,.F.,(4,3,4),(0.492524364189609,
0.5,0.504719756176228),.UNSPECIFIED.);
#22976=B_SPLINE_CURVE_WITH_KNOTS('',3,(#133370,#133371,#133372,#133373,
#133374,#133375),.UNSPECIFIED.,.F.,.F.,(4,2,4),(0.,0.0126505783151481,0.0253014157848534),
 .UNSPECIFIED.);
#22977=B_SPLINE_CURVE_WITH_KNOTS('',3,(#133382,#133383,#133384,#133385,
#133386,#133387,#133388),.UNSPECIFIED.,.F.,.F.,(4,3,4),(0.492524364184887,
0.5,0.504719756176228),.UNSPECIFIED.);
#22978=B_SPLINE_CURVE_WITH_KNOTS('',3,(#133409,#133410,#133411,#133412,
#133413,#133414),.UNSPECIFIED.,.F.,.F.,(4,2,4),(0.,0.0126505813529116,0.0253014285382464),
 .UNSPECIFIED.);
#22979=B_SPLINE_CURVE_WITH_KNOTS('',3,(#133427,#133428,#133429,#133430,
#133431,#133432,#133433),.UNSPECIFIED.,.F.,.F.,(4,3,4),(0.492524364,0.5,
0.504719756176228),.UNSPECIFIED.);
#22980=B_SPLINE_CURVE_WITH_KNOTS('',3,(#133449,#133450,#133451,#133452,
#133453,#133454),.UNSPECIFIED.,.F.,.F.,(4,2,4),(0.,0.0126505813382396,0.0253014283032559),
 .UNSPECIFIED.);
#22981=B_SPLINE_CURVE_WITH_KNOTS('',3,(#133457,#133458,#133459,#133460,
#133461,#133462,#133463),.UNSPECIFIED.,.F.,.F.,(4,3,4),(0.492524364188681,
0.5,0.504719756194363),.UNSPECIFIED.);
#22982=B_SPLINE_CURVE_WITH_KNOTS('',3,(#133487,#133488,#133489,#133490,
#133491,#133492),.UNSPECIFIED.,.F.,.F.,(4,2,4),(0.,0.0126505807185899,0.0253014258572568),
 .UNSPECIFIED.);
#22983=B_SPLINE_CURVE_WITH_KNOTS('',3,(#133499,#133500,#133501,#133502,
#133503,#133504,#133505),.UNSPECIFIED.,.F.,.F.,(4,3,4),(0.492524364187148,
0.5,0.504719756176227),.UNSPECIFIED.);
#22984=B_SPLINE_CURVE_WITH_KNOTS('',3,(#133526,#133527,#133528,#133529,
#133530,#133531),.UNSPECIFIED.,.F.,.F.,(4,2,4),(0.,0.01265057904704,0.0253014188722932),
 .UNSPECIFIED.);
#22985=B_SPLINE_CURVE_WITH_KNOTS('',3,(#133538,#133539,#133540,#133541,
#133542,#133543,#133544),.UNSPECIFIED.,.F.,.F.,(4,3,4),(0.492524364186767,
0.5,0.504719756176227),.UNSPECIFIED.);
#22986=B_SPLINE_CURVE_WITH_KNOTS('',3,(#133565,#133566,#133567,#133568,
#133569,#133570),.UNSPECIFIED.,.F.,.F.,(4,2,4),(0.,0.0126505798077898,0.0253014219006744),
 .UNSPECIFIED.);
#22987=B_SPLINE_CURVE_WITH_KNOTS('',3,(#133577,#133578,#133579,#133580,
#133581,#133582,#133583),.UNSPECIFIED.,.F.,.F.,(4,3,4),(0.492524364193697,
0.5,0.504719756176227),.UNSPECIFIED.);
#22988=B_SPLINE_CURVE_WITH_KNOTS('',3,(#133604,#133605,#133606,#133607,
#133608,#133609),.UNSPECIFIED.,.F.,.F.,(4,2,4),(0.,0.0126505808801605,0.0253014264674703),
 .UNSPECIFIED.);
#22989=B_SPLINE_CURVE_WITH_KNOTS('',3,(#133616,#133617,#133618,#133619,
#133620,#133621,#133622),.UNSPECIFIED.,.F.,.F.,(4,3,4),(0.492524364182756,
0.5,0.504719756176227),.UNSPECIFIED.);
#22990=B_SPLINE_CURVE_WITH_KNOTS('',3,(#133643,#133644,#133645,#133646,
#133647,#133648),.UNSPECIFIED.,.F.,.F.,(4,2,4),(0.,0.0126505779800128,0.0253014145110505),
 .UNSPECIFIED.);
#22991=B_SPLINE_CURVE_WITH_KNOTS('',3,(#133655,#133656,#133657,#133658,
#133659,#133660,#133661),.UNSPECIFIED.,.F.,.F.,(4,3,4),(0.49252436419132,
0.5,0.504719756176227),.UNSPECIFIED.);
#22992=B_SPLINE_CURVE_WITH_KNOTS('',3,(#133682,#133683,#133684,#133685,
#133686,#133687),.UNSPECIFIED.,.F.,.F.,(4,2,4),(0.,0.0126505794608813,0.0253014205743486),
 .UNSPECIFIED.);
#22993=B_SPLINE_CURVE_WITH_KNOTS('',3,(#133694,#133695,#133696,#133697,
#133698,#133699,#133700),.UNSPECIFIED.,.F.,.F.,(4,3,4),(0.492524364189435,
0.5,0.504719756176226),.UNSPECIFIED.);
#22994=B_SPLINE_CURVE_WITH_KNOTS('',3,(#133721,#133722,#133723,#133724,
#133725,#133726),.UNSPECIFIED.,.F.,.F.,(4,2,4),(0.,0.0126505804869144,0.0253014248256905),
 .UNSPECIFIED.);
#22995=B_SPLINE_CURVE_WITH_KNOTS('',3,(#133733,#133734,#133735,#133736,
#133737,#133738,#133739),.UNSPECIFIED.,.F.,.F.,(4,3,4),(0.492524364190348,
0.5,0.504719756176226),.UNSPECIFIED.);
#22996=B_SPLINE_CURVE_WITH_KNOTS('',3,(#133761,#133762,#133763,#133764,
#133765,#133766),.UNSPECIFIED.,.F.,.F.,(4,2,4),(-0.025304064498856,-0.0126521398388827,
-4.2125573862517E-11),.UNSPECIFIED.);
#22997=B_SPLINE_CURVE_WITH_KNOTS('',3,(#133790,#133791,#133792,#133793,
#133794,#133795),.UNSPECIFIED.,.F.,.F.,(4,2,4),(-0.0253040630374336,-0.0126521397986007,
-4.20119217192649E-11),.UNSPECIFIED.);
#22998=B_SPLINE_CURVE_WITH_KNOTS('',3,(#133819,#133820,#133821,#133822,
#133823,#133824),.UNSPECIFIED.,.F.,.F.,(4,2,4),(-0.0253040694676751,-0.0126521398389519,
-4.19704826448708E-11),.UNSPECIFIED.);
#22999=B_SPLINE_CURVE_WITH_KNOTS('',3,(#133848,#133849,#133850,#133851,
#133852,#133853),.UNSPECIFIED.,.F.,.F.,(4,2,4),(-0.0253040643721042,-0.0126521398535919,
-4.26806090469967E-11),.UNSPECIFIED.);
#23000=B_SPLINE_CURVE_WITH_KNOTS('',3,(#133877,#133878,#133879,#133880,
#133881,#133882),.UNSPECIFIED.,.F.,.F.,(4,2,4),(-0.0253040634165168,-0.0126521398236705,
-4.2208906508856E-11),.UNSPECIFIED.);
#23001=B_SPLINE_CURVE_WITH_KNOTS('',3,(#133906,#133907,#133908,#133909,
#133910,#133911),.UNSPECIFIED.,.F.,.F.,(4,2,4),(-0.0253040638021277,-0.0126521398274489,
-4.2573208847152E-11),.UNSPECIFIED.);
#23002=B_SPLINE_CURVE_WITH_KNOTS('',3,(#133935,#133936,#133937,#133938,
#133939,#133940),.UNSPECIFIED.,.F.,.F.,(4,2,4),(-0.0253040643923574,-0.0126521398266015,
-4.24393506448517E-11),.UNSPECIFIED.);
#23003=B_SPLINE_CURVE_WITH_KNOTS('',3,(#133964,#133965,#133966,#133967,
#133968,#133969),.UNSPECIFIED.,.F.,.F.,(4,2,4),(-0.0253040634154255,-0.0126521398084239,
-4.14864566311568E-11),.UNSPECIFIED.);
#23004=B_SPLINE_CURVE_WITH_KNOTS('',3,(#133993,#133994,#133995,#133996,
#133997,#133998),.UNSPECIFIED.,.F.,.F.,(4,2,4),(-0.0253040606038705,-0.0126521398219097,
-4.27034241301527E-11),.UNSPECIFIED.);
#23005=B_SPLINE_CURVE_WITH_KNOTS('',3,(#134022,#134023,#134024,#134025,
#134026,#134027),.UNSPECIFIED.,.F.,.F.,(4,2,4),(-0.0253040613299487,-0.0126521397910629,
-4.1742501816211E-11),.UNSPECIFIED.);
#23006=B_SPLINE_CURVE_WITH_KNOTS('',3,(#134051,#134052,#134053,#134054,
#134055,#134056),.UNSPECIFIED.,.F.,.F.,(4,2,4),(-0.025304066853621,-0.0126521398258534,
-4.13601410065301E-11),.UNSPECIFIED.);
#23007=B_SPLINE_CURVE_WITH_KNOTS('',3,(#134080,#134081,#134082,#134083,
#134084,#134085),.UNSPECIFIED.,.F.,.F.,(4,2,4),(-0.0253040666533286,-0.0126521398324811,
-4.16749482146095E-11),.UNSPECIFIED.);
#23008=B_SPLINE_CURVE_WITH_KNOTS('',3,(#134109,#134110,#134111,#134112,
#134113,#134114),.UNSPECIFIED.,.F.,.F.,(4,2,4),(-0.0253040634792013,-0.0126521398329723,
-4.27786313317302E-11),.UNSPECIFIED.);
#23009=B_SPLINE_CURVE_WITH_KNOTS('',3,(#134138,#134139,#134140,#134141,
#134142,#134143),.UNSPECIFIED.,.F.,.F.,(4,2,4),(-0.0253040635443814,-0.012652139804696,
-4.21150510299118E-11),.UNSPECIFIED.);
#23010=B_SPLINE_CURVE_WITH_KNOTS('',3,(#134167,#134168,#134169,#134170,
#134171,#134172),.UNSPECIFIED.,.F.,.F.,(4,2,4),(-0.0253040652094674,-0.0126521398118821,
-4.18545927083347E-11),.UNSPECIFIED.);
#23011=B_SPLINE_CURVE_WITH_KNOTS('',3,(#134196,#134197,#134198,#134199,
#134200,#134201),.UNSPECIFIED.,.F.,.F.,(4,2,4),(-0.0253040622867192,-0.0126521398070244,
-4.19272325191677E-11),.UNSPECIFIED.);
#23012=B_SPLINE_CURVE_WITH_KNOTS('',3,(#134225,#134226,#134227,#134228,
#134229,#134230),.UNSPECIFIED.,.F.,.F.,(4,2,4),(-0.0253040666146288,-0.0126521398295065,
-4.18443925342959E-11),.UNSPECIFIED.);
#23013=B_SPLINE_CURVE_WITH_KNOTS('',3,(#134254,#134255,#134256,#134257,
#134258,#134259),.UNSPECIFIED.,.F.,.F.,(4,2,4),(-0.02530406558539,-0.0126521398311914,
-4.21956844465221E-11),.UNSPECIFIED.);
#23014=B_SPLINE_CURVE_WITH_KNOTS('',3,(#134283,#134284,#134285,#134286,
#134287,#134288),.UNSPECIFIED.,.F.,.F.,(4,2,4),(-0.0253040616874405,-0.0126521398383703,
-4.3402618304933E-11),.UNSPECIFIED.);
#23015=B_SPLINE_CURVE_WITH_KNOTS('',3,(#134312,#134313,#134314,#134315,
#134316,#134317),.UNSPECIFIED.,.F.,.F.,(4,2,4),(-0.0253040610757602,-0.0126521398054598,
-4.21142877515823E-11),.UNSPECIFIED.);
#23016=B_SPLINE_CURVE_WITH_KNOTS('',3,(#134341,#134342,#134343,#134344,
#134345,#134346),.UNSPECIFIED.,.F.,.F.,(4,2,4),(-0.0253040624336241,-0.0126521398363262,
-4.2850282350182E-11),.UNSPECIFIED.);
#23017=B_SPLINE_CURVE_WITH_KNOTS('',3,(#134370,#134371,#134372,#134373,
#134374,#134375),.UNSPECIFIED.,.F.,.F.,(4,2,4),(-0.0253040617305736,-0.0126521398066379,
-4.31877381079637E-11),.UNSPECIFIED.);
#23018=B_SPLINE_CURVE_WITH_KNOTS('',3,(#134399,#134400,#134401,#134402,
#134403,#134404),.UNSPECIFIED.,.F.,.F.,(4,2,4),(-0.025304059734234,-0.0126521397823564,
-4.21624471447224E-11),.UNSPECIFIED.);
#23019=B_SPLINE_CURVE_WITH_KNOTS('',3,(#134428,#134429,#134430,#134431,
#134432,#134433),.UNSPECIFIED.,.F.,.F.,(4,2,4),(-0.0253040664569554,-0.0126521398563623,
-4.28707382094107E-11),.UNSPECIFIED.);
#23020=B_SPLINE_CURVE_WITH_KNOTS('',3,(#134457,#134458,#134459,#134460,
#134461,#134462),.UNSPECIFIED.,.F.,.F.,(4,2,4),(-0.025304062021989,-0.0126521398169023,
-4.14917475377585E-11),.UNSPECIFIED.);
#23021=B_SPLINE_CURVE_WITH_KNOTS('',3,(#134486,#134487,#134488,#134489,
#134490,#134491),.UNSPECIFIED.,.F.,.F.,(4,2,4),(-0.0253040667762494,-0.0126521398634984,
-4.26520728458168E-11),.UNSPECIFIED.);
#23022=B_SPLINE_CURVE_WITH_KNOTS('',3,(#134515,#134516,#134517,#134518,
#134519,#134520),.UNSPECIFIED.,.F.,.F.,(4,2,4),(-0.025304062706261,-0.0126521398103911,
-4.19324540368304E-11),.UNSPECIFIED.);
#23023=B_SPLINE_CURVE_WITH_KNOTS('',3,(#134544,#134545,#134546,#134547,
#134548,#134549),.UNSPECIFIED.,.F.,.F.,(4,2,4),(-0.0253040678335757,-0.0126521398507726,
-4.24169657731177E-11),.UNSPECIFIED.);
#23024=B_SPLINE_CURVE_WITH_KNOTS('',3,(#134573,#134574,#134575,#134576,
#134577,#134578),.UNSPECIFIED.,.F.,.F.,(4,2,4),(-0.0253040639899681,-0.0126521397979972,
-4.20035950465802E-11),.UNSPECIFIED.);
#23025=B_SPLINE_CURVE_WITH_KNOTS('',3,(#134604,#134605,#134606,#134607,
#134608,#134609,#134610,#134611,#134612,#134613),.UNSPECIFIED.,.F.,.F.,
(4,3,3,4),(4.14193967595349E-14,8.70530734855011E-5,0.000170036649813278,
0.000253022525483205),.UNSPECIFIED.);
#23026=B_SPLINE_CURVE_WITH_KNOTS('',3,(#134628,#134629,#134630,#134631,
#134632,#134633,#134634,#134635,#134636,#134637),.UNSPECIFIED.,.F.,.F.,
(4,3,3,4),(0.211606869610061,0.221412979786492,0.226204530183524,0.228987659497871),
 .UNSPECIFIED.);
#23027=B_SPLINE_CURVE_WITH_KNOTS('',3,(#134650,#134651,#134652,#134653,
#134654,#134655,#134656,#134657,#134658,#134659),.UNSPECIFIED.,.F.,.F.,
(4,3,3,4),(8.73864678274336E-14,8.70530734589771E-5,0.000170036649623857,
0.000253022525131198),.UNSPECIFIED.);
#23028=B_SPLINE_CURVE_WITH_KNOTS('',3,(#134674,#134675,#134676,#134677,
#134678,#134679,#134680,#134681,#134682,#134683),.UNSPECIFIED.,.F.,.F.,
(4,3,3,4),(0.211606869614525,0.221412980312189,0.226204530183508,0.228987659512711),
 .UNSPECIFIED.);
#23029=B_SPLINE_CURVE_WITH_KNOTS('',3,(#134696,#134697,#134698,#134699,
#134700,#134701,#134702,#134703,#134704,#134705),.UNSPECIFIED.,.F.,.F.,
(4,3,3,4),(8.03981756062997E-15,8.70530736309221E-5,0.000170036649877014,
0.000253022525465094),.UNSPECIFIED.);
#23030=B_SPLINE_CURVE_WITH_KNOTS('',3,(#134720,#134721,#134722,#134723,
#134724,#134725,#134726,#134727,#134728,#134729),.UNSPECIFIED.,.F.,.F.,
(4,3,3,4),(0.211606869609531,0.221412979024587,0.2262045301835,0.228987659519257),
 .UNSPECIFIED.);
#23031=B_SPLINE_CURVE_WITH_KNOTS('',3,(#134742,#134743,#134744,#134745,
#134746,#134747,#134748,#134749,#134750,#134751),.UNSPECIFIED.,.F.,.F.,
(4,3,3,4),(7.79800256787147E-14,8.70530734703506E-5,0.000170036649594596,
0.000253022525060469),.UNSPECIFIED.);
#23032=B_SPLINE_CURVE_WITH_KNOTS('',3,(#134766,#134767,#134768,#134769,
#134770,#134771,#134772,#134773,#134774,#134775),.UNSPECIFIED.,.F.,.F.,
(4,3,3,4),(0.211606869610436,0.221412979506795,0.226204530183523,0.228987659511922),
 .UNSPECIFIED.);
#23033=B_SPLINE_CURVE_WITH_KNOTS('',3,(#134788,#134789,#134790,#134791,
#134792,#134793,#134794,#134795,#134796,#134797),.UNSPECIFIED.,.F.,.F.,
(4,3,3,4),(5.37189951081576E-14,8.70530735283743E-5,0.000170036649708885,
0.000253022525231511),.UNSPECIFIED.);
#23034=B_SPLINE_CURVE_WITH_KNOTS('',3,(#134812,#134813,#134814,#134815,
#134816,#134817,#134818,#134819,#134820,#134821),.UNSPECIFIED.,.F.,.F.,
(4,3,3,4),(0.211606869618575,0.221412979552959,0.226204530183407,0.228987659520732),
 .UNSPECIFIED.);
#23035=B_SPLINE_CURVE_WITH_KNOTS('',3,(#134834,#134835,#134836,#134837,
#134838,#134839,#134840,#134841,#134842,#134843),.UNSPECIFIED.,.F.,.F.,
(4,3,3,4),(1.31873644434942E-13,8.7053073591002E-5,0.000170036649834339,
0.000253022525419973),.UNSPECIFIED.);
#23036=B_SPLINE_CURVE_WITH_KNOTS('',3,(#134858,#134859,#134860,#134861,
#134862,#134863,#134864,#134865,#134866,#134867,#134868,#134869,#134870,
#134871),.UNSPECIFIED.,.F.,.F.,(4,2,2,2,2,2,4),(9.99263316600448E-7,0.00392100953657802,
0.00802861323508025,0.0162407021656379,0.0326517370626527,0.0654159013494179,
0.13074836471509),.UNSPECIFIED.);
#23037=B_SPLINE_CURVE_WITH_KNOTS('',3,(#134884,#134885,#134886,#134887,
#134888,#134889,#134890,#134891,#134892,#134893),.UNSPECIFIED.,.F.,.F.,
(4,3,3,4),(7.89927548210784E-14,8.70530731075762E-5,0.000170036648965722,
0.0002530225241661),.UNSPECIFIED.);
#23038=B_SPLINE_CURVE_WITH_KNOTS('',3,(#134908,#134909,#134910,#134911,
#134912,#134913,#134914,#134915,#134916,#134917),.UNSPECIFIED.,.F.,.F.,
(4,3,3,4),(0.211606869614502,0.221412981431605,0.226204530183495,0.228987659498062),
 .UNSPECIFIED.);
#23039=B_SPLINE_CURVE_WITH_KNOTS('',3,(#134930,#134931,#134932,#134933,
#134934,#134935,#134936,#134937,#134938,#134939),.UNSPECIFIED.,.F.,.F.,
(4,3,3,4),(2.52334893766153E-14,8.70530732793856E-5,0.000170036649550745,
0.000253022525164497),.UNSPECIFIED.);
#23040=B_SPLINE_CURVE_WITH_KNOTS('',3,(#134954,#134955,#134956,#134957,
#134958,#134959,#134960,#134961,#134962,#134963),.UNSPECIFIED.,.F.,.F.,
(4,3,3,4),(0.211606869621102,0.221412977824722,0.226204530183524,0.228987659510322),
 .UNSPECIFIED.);
#23041=B_SPLINE_CURVE_WITH_KNOTS('',3,(#134976,#134977,#134978,#134979,
#134980,#134981,#134982,#134983,#134984,#134985),.UNSPECIFIED.,.F.,.F.,
(4,3,3,4),(7.50943469913966E-14,8.70530731548489E-5,0.00017003664908509,
0.000253022524357588),.UNSPECIFIED.);
#23042=B_SPLINE_CURVE_WITH_KNOTS('',3,(#135000,#135001,#135002,#135003,
#135004,#135005,#135006,#135007,#135008,#135009),.UNSPECIFIED.,.F.,.F.,
(4,3,3,4),(0.211606870032462,0.22141297801983,0.226204530183524,0.228987659635174),
 .UNSPECIFIED.);
#23043=B_SPLINE_CURVE_WITH_KNOTS('',3,(#135022,#135023,#135024,#135025,
#135026,#135027,#135028,#135029,#135030,#135031),.UNSPECIFIED.,.F.,.F.,
(4,3,3,4),(9.02311911813612E-14,8.70530732466921E-5,0.000170036649065836,
0.000253022524226805),.UNSPECIFIED.);
#23044=B_SPLINE_CURVE_WITH_KNOTS('',3,(#135046,#135047,#135048,#135049,
#135050,#135051,#135052,#135053,#135054,#135055),.UNSPECIFIED.,.F.,.F.,
(4,3,3,4),(0.211606869604561,0.221412978253218,0.22620453018352,0.228987659509309),
 .UNSPECIFIED.);
#23045=B_SPLINE_CURVE_WITH_KNOTS('',3,(#135068,#135069,#135070,#135071,
#135072,#135073,#135074,#135075,#135076,#135077),.UNSPECIFIED.,.F.,.F.,
(4,3,3,4),(1.07741326354794E-13,8.70530734410574E-5,0.000170036649714572,
0.000253022525330184),.UNSPECIFIED.);
#23046=B_SPLINE_CURVE_WITH_KNOTS('',3,(#135092,#135093,#135094,#135095,
#135096,#135097,#135098,#135099,#135100,#135101),.UNSPECIFIED.,.F.,.F.,
(4,3,3,4),(0.211606869612044,0.221412977691357,0.226204530183524,0.228987659517864),
 .UNSPECIFIED.);
#23047=B_SPLINE_CURVE_WITH_KNOTS('',3,(#135114,#135115,#135116,#135117,
#135118,#135119,#135120,#135121,#135122,#135123),.UNSPECIFIED.,.F.,.F.,
(4,3,3,4),(1.09031513920967E-13,8.70530732165772E-5,0.000170036649139832,
0.000253022524405007),.UNSPECIFIED.);
#23048=B_SPLINE_CURVE_WITH_KNOTS('',3,(#135138,#135139,#135140,#135141,
#135142,#135143,#135144,#135145,#135146,#135147),.UNSPECIFIED.,.F.,.F.,
(4,3,3,4),(0.211606870045396,0.221412978124601,0.226204530183484,0.228987659635174),
 .UNSPECIFIED.);
#23049=B_SPLINE_CURVE_WITH_KNOTS('',3,(#135160,#135161,#135162,#135163,
#135164,#135165,#135166,#135167,#135168,#135169),.UNSPECIFIED.,.F.,.F.,
(4,3,3,4),(6.03891784362884E-14,8.70530729984545E-5,0.000170036648893098,
0.00025302252412988),.UNSPECIFIED.);
#23050=B_SPLINE_CURVE_WITH_KNOTS('',3,(#135184,#135185,#135186,#135187,
#135188,#135189,#135190,#135191,#135192,#135193,#135194,#135195,#135196,
#135197),.UNSPECIFIED.,.F.,.F.,(4,2,2,2,2,2,4),(9.99274182381302E-7,0.00392100953236448,
0.00802861321169121,0.0162407021070139,0.0326517369455817,0.0654158886697625,
0.130748337459387),.UNSPECIFIED.);
#23051=B_SPLINE_CURVE_WITH_KNOTS('',3,(#135210,#135211,#135212,#135213,
#135214,#135215,#135216,#135217,#135218,#135219),.UNSPECIFIED.,.F.,.F.,
(4,3,3,4),(3.67379430042663E-14,8.70530734914654E-5,0.000170036649570622,
0.000253022524992313),.UNSPECIFIED.);
#23052=B_SPLINE_CURVE_WITH_KNOTS('',3,(#135234,#135235,#135236,#135237,
#135238,#135239,#135240,#135241,#135242,#135243,#135244,#135245,#135246,
#135247),.UNSPECIFIED.,.F.,.F.,(4,2,2,2,2,2,4),(9.99256961840177E-7,0.00392100965143877,
0.00802861351822096,0.0162407027811937,0.0326517383265419,0.0654159021312143,
0.130748376681168),.UNSPECIFIED.);
#23053=B_SPLINE_CURVE_WITH_KNOTS('',3,(#135260,#135261,#135262,#135263,
#135264,#135265,#135266,#135267,#135268,#135269),.UNSPECIFIED.,.F.,.F.,
(4,3,3,4),(1.57387654128723E-13,8.70530729486441E-5,0.000170036648862656,
0.000253022524119109),.UNSPECIFIED.);
#23054=B_SPLINE_CURVE_WITH_KNOTS('',3,(#135284,#135285,#135286,#135287,
#135288,#135289,#135290,#135291,#135292,#135293,#135294,#135295,#135296,
#135297),.UNSPECIFIED.,.F.,.F.,(4,2,2,2,2,2,4),(9.99262507793807E-7,0.00392100954195238,
0.00802861324845085,0.016240702191923,0.0326517371002704,0.0654158952120646,
0.130748362235185),.UNSPECIFIED.);
#23055=B_SPLINE_CURVE_WITH_KNOTS('',3,(#135310,#135311,#135312,#135313,
#135314,#135315,#135316,#135317,#135318,#135319),.UNSPECIFIED.,.F.,.F.,
(4,3,3,4),(1.22918305753956E-13,8.70530733818197E-5,0.000170036649366911,
0.000253022524693734),.UNSPECIFIED.);
#23056=B_SPLINE_CURVE_WITH_KNOTS('',3,(#135334,#135335,#135336,#135337,
#135338,#135339,#135340,#135341,#135342,#135343),.UNSPECIFIED.,.F.,.F.,
(4,3,3,4),(0.211606869609805,0.221412978520094,0.226204530183364,0.228987659522938),
 .UNSPECIFIED.);
#23057=B_SPLINE_CURVE_WITH_KNOTS('',3,(#135356,#135357,#135358,#135359,
#135360,#135361,#135362,#135363,#135364,#135365),.UNSPECIFIED.,.F.,.F.,
(4,3,3,4),(9.87657324158844E-14,8.70530733720858E-5,0.000170036649521387,
0.000253022525013159),.UNSPECIFIED.);
#23058=B_SPLINE_CURVE_WITH_KNOTS('',3,(#135380,#135381,#135382,#135383,
#135384,#135385,#135386,#135387,#135388,#135389),.UNSPECIFIED.,.F.,.F.,
(4,3,3,4),(0.211606870036805,0.221412975969717,0.226204530183423,0.228987659635174),
 .UNSPECIFIED.);
#23059=B_SPLINE_CURVE_WITH_KNOTS('',3,(#135402,#135403,#135404,#135405,
#135406,#135407,#135408,#135409,#135410,#135411),.UNSPECIFIED.,.F.,.F.,
(4,3,3,4),(6.10802431102158E-14,8.7053073275896E-5,0.000170036649311064,
0.00025302252468842),.UNSPECIFIED.);
#23060=B_SPLINE_CURVE_WITH_KNOTS('',3,(#135426,#135427,#135428,#135429,
#135430,#135431,#135432,#135433,#135434,#135435),.UNSPECIFIED.,.F.,.F.,
(4,3,3,4),(0.211606869622254,0.221412979041746,0.226204530183396,0.22898765948021),
 .UNSPECIFIED.);
#23061=B_SPLINE_CURVE_WITH_KNOTS('',3,(#135448,#135449,#135450,#135451,
#135452,#135453,#135454,#135455,#135456,#135457),.UNSPECIFIED.,.F.,.F.,
(4,3,3,4),(1.03129267188451E-13,8.7053073632608E-5,0.00017003664957889,
0.000253022524867124),.UNSPECIFIED.);
#23062=B_SPLINE_CURVE_WITH_KNOTS('',3,(#135472,#135473,#135474,#135475,
#135476,#135477,#135478,#135479,#135480,#135481),.UNSPECIFIED.,.F.,.F.,
(4,3,3,4),(0.211606869619466,0.221412978868105,0.226204530183133,0.228987659519068),
 .UNSPECIFIED.);
#23063=B_SPLINE_CURVE_WITH_KNOTS('',3,(#135494,#135495,#135496,#135497,
#135498,#135499,#135500,#135501,#135502,#135503),.UNSPECIFIED.,.F.,.F.,
(4,3,3,4),(2.08121007347066E-14,8.7053073146988E-5,0.000170036648983739,
0.000253022524162919),.UNSPECIFIED.);
#23064=B_SPLINE_CURVE_WITH_KNOTS('',3,(#135518,#135519,#135520,#135521,
#135522,#135523,#135524,#135525,#135526,#135527),.UNSPECIFIED.,.F.,.F.,
(4,3,3,4),(0.211606870038675,0.221412976851843,0.226204530183384,0.228987659635175),
 .UNSPECIFIED.);
#23065=B_SPLINE_CURVE_WITH_KNOTS('',3,(#135540,#135541,#135542,#135543,
#135544,#135545,#135546,#135547,#135548,#135549),.UNSPECIFIED.,.F.,.F.,
(4,3,3,4),(5.5757338411683E-14,8.70530736151624E-5,0.00017003664991911,
0.000253022525565324),.UNSPECIFIED.);
#23066=B_SPLINE_CURVE_WITH_KNOTS('',3,(#135564,#135565,#135566,#135567,
#135568,#135569,#135570,#135571,#135572,#135573),.UNSPECIFIED.,.F.,.F.,
(4,3,3,4),(0.211606869613814,0.221412976950775,0.22620453018352,0.228987659505786),
 .UNSPECIFIED.);
#23067=B_SPLINE_CURVE_WITH_KNOTS('',3,(#135586,#135587,#135588,#135589,
#135590,#135591,#135592,#135593,#135594,#135595),.UNSPECIFIED.,.F.,.F.,
(4,3,3,4),(6.46825384166277E-14,8.7053073213682E-5,0.000170036649169692,
0.000253022524468235),.UNSPECIFIED.);
#23068=B_SPLINE_CURVE_WITH_KNOTS('',3,(#135610,#135611,#135612,#135613,
#135614,#135615,#135616,#135617,#135618,#135619),.UNSPECIFIED.,.F.,.F.,
(4,3,3,4),(0.211606869605571,0.221412978487561,0.226204530183522,0.228987659505563),
 .UNSPECIFIED.);
#23069=B_SPLINE_CURVE_WITH_KNOTS('',3,(#135632,#135633,#135634,#135635,
#135636,#135637,#135638,#135639,#135640,#135641),.UNSPECIFIED.,.F.,.F.,
(4,3,3,4),(1.25934867797587E-13,8.70530732380585E-5,0.00017003664904369,
0.000253022524191407),.UNSPECIFIED.);
#23070=B_SPLINE_CURVE_WITH_KNOTS('',3,(#135656,#135657,#135658,#135659,
#135660,#135661,#135662,#135663,#135664,#135665),.UNSPECIFIED.,.F.,.F.,
(4,3,3,4),(0.211606870056587,0.221412979815329,0.226204530183526,0.228987659635175),
 .UNSPECIFIED.);
#23071=B_SPLINE_CURVE_WITH_KNOTS('',3,(#135678,#135679,#135680,#135681,
#135682,#135683,#135684,#135685,#135686,#135687),.UNSPECIFIED.,.F.,.F.,
(4,3,3,4),(8.80606518148291E-15,8.70530734448549E-5,0.000170036649791158,
0.000253022525475898),.UNSPECIFIED.);
#23072=B_SPLINE_CURVE_WITH_KNOTS('',3,(#135702,#135703,#135704,#135705,
#135706,#135707,#135708,#135709,#135710,#135711),.UNSPECIFIED.,.F.,.F.,
(4,3,3,4),(0.211606869615,0.221412981214008,0.226204530183526,0.228987659511592),
 .UNSPECIFIED.);
#23073=B_SPLINE_CURVE_WITH_KNOTS('',3,(#135724,#135725,#135726,#135727,
#135728,#135729,#135730,#135731,#135732,#135733),.UNSPECIFIED.,.F.,.F.,
(4,3,3,4),(1.01634978089741E-13,8.70530731190007E-5,0.000170036648882755,
0.000253022523989102),.UNSPECIFIED.);
#23074=B_SPLINE_CURVE_WITH_KNOTS('',3,(#135748,#135749,#135750,#135751,
#135752,#135753,#135754,#135755,#135756,#135757),.UNSPECIFIED.,.F.,.F.,
(4,3,3,4),(0.21160686962461,0.221412977210515,0.226204530183525,0.228987659495652),
 .UNSPECIFIED.);
#23075=B_SPLINE_CURVE_WITH_KNOTS('',3,(#135770,#135771,#135772,#135773,
#135774,#135775,#135776,#135777,#135778,#135779),.UNSPECIFIED.,.F.,.F.,
(4,3,3,4),(8.51741288654366E-14,8.70530733732294E-5,0.000170036649691492,
0.000253022525351441),.UNSPECIFIED.);
#23076=B_SPLINE_CURVE_WITH_KNOTS('',3,(#135794,#135795,#135796,#135797,
#135798,#135799,#135800,#135801,#135802,#135803),.UNSPECIFIED.,.F.,.F.,
(4,3,3,4),(0.211606870017552,0.221412978920659,0.226204530183525,0.228987659635174),
 .UNSPECIFIED.);
#23077=B_SPLINE_CURVE_WITH_KNOTS('',3,(#135816,#135817,#135818,#135819,
#135820,#135821,#135822,#135823,#135824,#135825),.UNSPECIFIED.,.F.,.F.,
(4,3,3,4),(9.67597096038106E-14,8.70530734827708E-5,0.000170036649712742,
0.000253022525284123),.UNSPECIFIED.);
#23078=B_SPLINE_CURVE_WITH_KNOTS('',3,(#135840,#135841,#135842,#135843,
#135844,#135845,#135846,#135847,#135848,#135849),.UNSPECIFIED.,.F.,.F.,
(4,3,3,4),(0.211606869611342,0.221412977795872,0.226204530183296,0.228987659507632),
 .UNSPECIFIED.);
#23079=B_SPLINE_CURVE_WITH_KNOTS('',3,(#135862,#135863,#135864,#135865,
#135866,#135867,#135868,#135869,#135870,#135871),.UNSPECIFIED.,.F.,.F.,
(4,3,3,4),(9.87701739216603E-14,8.70530730923315E-5,0.000170036649017183,
0.000253022524284285),.UNSPECIFIED.);
#23080=B_SPLINE_CURVE_WITH_KNOTS('',3,(#135886,#135887,#135888,#135889,
#135890,#135891,#135892,#135893,#135894,#135895),.UNSPECIFIED.,.F.,.F.,
(4,3,3,4),(0.211606869614618,0.221412977874128,0.226204530183525,0.228987659495887),
 .UNSPECIFIED.);
#23081=B_SPLINE_CURVE_WITH_KNOTS('',3,(#135908,#135909,#135910,#135911,
#135912,#135913,#135914,#135915,#135916,#135917),.UNSPECIFIED.,.F.,.F.,
(4,3,3,4),(1.02970012907908E-13,8.70530731785482E-5,0.000170036649084164,
0.000253022524331985),.UNSPECIFIED.);
#23082=B_SPLINE_CURVE_WITH_KNOTS('',3,(#135932,#135933,#135934,#135935,
#135936,#135937,#135938,#135939,#135940,#135941,#135942,#135943,#135944,
#135945),.UNSPECIFIED.,.F.,.F.,(4,2,2,2,2,2,4),(9.99231836108335E-7,0.00392100953658189,
0.00802861330453663,0.0162407023730482,0.032651737543804,0.0654159064689534,
0.130748385933526),.UNSPECIFIED.);
#23083=B_SPLINE_CURVE_WITH_KNOTS('',3,(#135958,#135959,#135960,#135961,
#135962,#135963,#135964,#135965,#135966,#135967),.UNSPECIFIED.,.F.,.F.,
(4,3,3,4),(2.23301994145838E-13,8.70609203873829E-5,0.00017004098563854,
0.000253023205833107),.UNSPECIFIED.);
#23084=B_SPLINE_CURVE_WITH_KNOTS('',3,(#135982,#135983,#135984,#135985,
#135986,#135987,#135988,#135989,#135990,#135991,#135992,#135993,#135994,
#135995),.UNSPECIFIED.,.F.,.F.,(4,2,2,2,2,2,4),(9.66170382949012E-7,0.00392697974081771,
0.00804085973309614,0.0162655707091348,0.0327021207330737,0.065518343067229,
0.130949505770759),.UNSPECIFIED.);
#23085=B_SPLINE_CURVE_WITH_KNOTS('',3,(#136008,#136009,#136010,#136011,
#136012,#136013,#136014,#136015,#136016,#136017),.UNSPECIFIED.,.F.,.F.,
(4,3,3,4),(1.54112774829538E-13,8.70609205573687E-5,0.000170040985736614,
0.000253023205859177),.UNSPECIFIED.);
#23086=B_SPLINE_CURVE_WITH_KNOTS('',3,(#136032,#136033,#136034,#136035,
#136036,#136037,#136038,#136039,#136040,#136041),.UNSPECIFIED.,.F.,.F.,
(4,3,3,4),(0.556212830500469,0.566018334268703,0.571428571428571,0.573654350170116),
 .UNSPECIFIED.);
#23087=B_SPLINE_CURVE_WITH_KNOTS('',3,(#136054,#136055,#136056,#136057,
#136058,#136059,#136060,#136061,#136062,#136063),.UNSPECIFIED.,.F.,.F.,
(4,3,3,4),(2.31230172025941E-13,8.70609204481204E-5,0.00017004098573502,
0.00025302320596535),.UNSPECIFIED.);
#23088=B_SPLINE_CURVE_WITH_KNOTS('',3,(#136078,#136079,#136080,#136081,
#136082,#136083,#136084,#136085,#136086,#136087,#136088,#136089,#136090,
#136091),.UNSPECIFIED.,.F.,.F.,(4,2,2,2,2,2,4),(9.66208308196074E-7,0.00392697967644637,
0.00804085952878198,0.0162655702222953,0.0327021196697788,0.0655183472628571,
0.130949503112459),.UNSPECIFIED.);
#23089=B_SPLINE_CURVE_WITH_KNOTS('',3,(#136104,#136105,#136106,#136107,
#136108,#136109,#136110,#136111,#136112,#136113,#136114,#136115,#136116),
 .UNSPECIFIED.,.F.,.F.,(4,3,3,3,4),(9.22977705889797E-14,8.70609205457749E-5,
0.000149888113578299,0.00017004098589941,0.000253023206195647),
 .UNSPECIFIED.);
#23090=B_SPLINE_CURVE_WITH_KNOTS('',3,(#136131,#136132,#136133,#136134,
#136135,#136136,#136137,#136138,#136139,#136140),.UNSPECIFIED.,.F.,.F.,
(4,3,3,4),(0.556212830497425,0.566018335391702,0.571428571428571,0.573654350184794),
 .UNSPECIFIED.);
#23091=B_SPLINE_CURVE_WITH_KNOTS('',3,(#136153,#136154,#136155,#136156,
#136157,#136158,#136159,#136160,#136161,#136162),.UNSPECIFIED.,.F.,.F.,
(4,3,3,4),(1.21696510425184E-13,8.70609206928594E-5,0.000170040985934045,
0.000253023206118154),.UNSPECIFIED.);
#23092=B_SPLINE_CURVE_WITH_KNOTS('',3,(#136177,#136178,#136179,#136180,
#136181,#136182,#136183,#136184,#136185,#136186,#136187,#136188,#136189,
#136190),.UNSPECIFIED.,.F.,.F.,(4,2,2,2,2,2,4),(9.66228217625918E-7,0.00392697956919349,
0.00804085924933738,0.0162655695995458,0.0327021183655822,0.065518345398006,
0.130949516846548),.UNSPECIFIED.);
#23093=B_SPLINE_CURVE_WITH_KNOTS('',3,(#136203,#136204,#136205,#136206,
#136207,#136208,#136209,#136210,#136211,#136212),.UNSPECIFIED.,.F.,.F.,
(4,3,3,4),(1.83368163365468E-13,8.70609205947636E-5,0.000170040985795044,
0.000253023205937427),.UNSPECIFIED.);
#23094=B_SPLINE_CURVE_WITH_KNOTS('',3,(#136227,#136228,#136229,#136230,
#136231,#136232,#136233,#136234,#136235,#136236),.UNSPECIFIED.,.F.,.F.,
(4,3,3,4),(0.556212830502335,0.566018335768767,0.571428571428571,0.57365435021991),
 .UNSPECIFIED.);
#23095=B_SPLINE_CURVE_WITH_KNOTS('',3,(#136249,#136250,#136251,#136252,
#136253,#136254,#136255,#136256,#136257,#136258),.UNSPECIFIED.,.F.,.F.,
(4,3,3,4),(2.19221044078209E-13,8.70609204363992E-5,0.000170040985578205,
0.000253023205662227),.UNSPECIFIED.);
#23096=B_SPLINE_CURVE_WITH_KNOTS('',3,(#136273,#136274,#136275,#136276,
#136277,#136278,#136279,#136280,#136281,#136282,#136283,#136284,#136285,
#136286),.UNSPECIFIED.,.F.,.F.,(4,2,2,2,2,2,4),(9.66236086782783E-7,0.00392697943596319,
0.00804085891948424,0.0162655688791268,0.0327021168735546,0.0655183394151674,
0.130949508120157),.UNSPECIFIED.);
#23097=B_SPLINE_CURVE_WITH_KNOTS('',3,(#136299,#136300,#136301,#136302,
#136303,#136304,#136305,#136306,#136307,#136308),.UNSPECIFIED.,.F.,.F.,
(4,3,3,4),(1.68080143162128E-13,8.70609204517327E-5,0.000170040985610495,
0.000253023205711627),.UNSPECIFIED.);
#23098=B_SPLINE_CURVE_WITH_KNOTS('',3,(#136323,#136324,#136325,#136326,
#136327,#136328,#136329,#136330,#136331,#136332),.UNSPECIFIED.,.F.,.F.,
(4,3,3,4),(0.556212830495103,0.566018336597087,0.571428571428571,0.573654350166826),
 .UNSPECIFIED.);
#23099=B_SPLINE_CURVE_WITH_KNOTS('',3,(#136345,#136346,#136347,#136348,
#136349,#136350,#136351,#136352,#136353,#136354),.UNSPECIFIED.,.F.,.F.,
(4,3,3,4),(1.34197132127504E-13,8.7060920586027E-5,0.00017004098587252,
0.000253023206102087),.UNSPECIFIED.);
#23100=B_SPLINE_CURVE_WITH_KNOTS('',3,(#136369,#136370,#136371,#136372,
#136373,#136374,#136375,#136376,#136377,#136378),.UNSPECIFIED.,.F.,.F.,
(4,3,3,4),(0.556212830497077,0.566018336499488,0.571428571428571,0.573654350165251),
 .UNSPECIFIED.);
#23101=B_SPLINE_CURVE_WITH_KNOTS('',3,(#136391,#136392,#136393,#136394,
#136395,#136396,#136397,#136398,#136399,#136400),.UNSPECIFIED.,.F.,.F.,
(4,3,3,4),(2.08605666433404E-13,8.70609206450327E-5,0.000170040985681761,
0.000253023205661205),.UNSPECIFIED.);
#23102=B_SPLINE_CURVE_WITH_KNOTS('',3,(#136415,#136416,#136417,#136418,
#136419,#136420,#136421,#136422,#136423,#136424,#136425,#136426,#136427,
#136428),.UNSPECIFIED.,.F.,.F.,(4,2,2,2,2,2,4),(9.66229434957699E-7,0.00392697962088967,
0.00804085935796308,0.0162655698264246,0.0327021188437879,0.065518347343508,
0.130949526287197),.UNSPECIFIED.);
#23103=B_SPLINE_CURVE_WITH_KNOTS('',3,(#136441,#136442,#136443,#136444,
#136445,#136446,#136447,#136448,#136449,#136450),.UNSPECIFIED.,.F.,.F.,
(4,3,3,4),(8.45001259843959E-14,8.70609204120089E-5,0.000170040985741675,
0.000253023206012994),.UNSPECIFIED.);
#23104=B_SPLINE_CURVE_WITH_KNOTS('',3,(#136482,#136483,#136484,#136485,
#136486,#136487,#136488,#136489,#136490,#136491),.UNSPECIFIED.,.F.,.F.,
(4,3,3,4),(1.51987334395212E-13,8.70609206640265E-5,0.000170040985730083,
0.000253023205738738),.UNSPECIFIED.);
#23105=B_SPLINE_CURVE_WITH_KNOTS('',3,(#136523,#136524,#136525,#136526,
#136527,#136528,#136529,#136530,#136531,#136532),.UNSPECIFIED.,.F.,.F.,
(4,3,3,4),(2.21373845505911E-13,8.7060920434661E-5,0.000170040985496251,
0.000253023205500094),.UNSPECIFIED.);
#23106=B_SPLINE_CURVE_WITH_KNOTS('',3,(#136547,#136548,#136549,#136550,
#136551,#136552,#136553,#136554,#136555,#136556),.UNSPECIFIED.,.F.,.F.,
(4,3,3,4),(0.556212830498472,0.566018335338913,0.571428571428571,0.573654350176112),
 .UNSPECIFIED.);
#23107=B_SPLINE_CURVE_WITH_KNOTS('',3,(#136569,#136570,#136571,#136572,
#136573,#136574,#136575,#136576,#136577,#136578),.UNSPECIFIED.,.F.,.F.,
(4,3,3,4),(1.17323887739643E-13,8.70609205778466E-5,0.000170040985778564,
0.000253023205922772),.UNSPECIFIED.);
#23108=B_SPLINE_CURVE_WITH_KNOTS('',3,(#136593,#136594,#136595,#136596,
#136597,#136598,#136599,#136600,#136601,#136602,#136603,#136604,#136605,
#136606),.UNSPECIFIED.,.F.,.F.,(4,2,2,2,2,2,4),(9.66258725593663E-7,0.00392697940720579,
0.00804085883290391,0.0162655686774062,0.0327021164455095,0.0655183366867418,
0.130949485166268),.UNSPECIFIED.);
#23109=B_SPLINE_CURVE_WITH_KNOTS('',3,(#136619,#136620,#136621,#136622,
#136623,#136624,#136625,#136626,#136627,#136628),.UNSPECIFIED.,.F.,.F.,
(4,3,3,4),(9.6474942780677E-14,8.70609207631378E-5,0.000170040985962259,
0.000253023206105505),.UNSPECIFIED.);
#23110=B_SPLINE_CURVE_WITH_KNOTS('',3,(#136643,#136644,#136645,#136646,
#136647,#136648,#136649,#136650,#136651,#136652),.UNSPECIFIED.,.F.,.F.,
(4,3,3,4),(0.556212830494827,0.566018337704693,0.571428571428571,0.573654350156748),
 .UNSPECIFIED.);
#23111=B_SPLINE_CURVE_WITH_KNOTS('',3,(#136665,#136666,#136667,#136668,
#136669,#136670,#136671,#136672,#136673,#136674,#136675,#136676,#136677),
 .UNSPECIFIED.,.F.,.F.,(4,3,3,3,4),(1.69396119959038E-13,8.70609205411585E-5,
0.00014988811322635,0.000170040985712469,0.000253023205827122),
 .UNSPECIFIED.);
#23112=B_SPLINE_CURVE_WITH_KNOTS('',3,(#136709,#136710,#136711,#136712,
#136713,#136714,#136715,#136716,#136717,#136718),.UNSPECIFIED.,.F.,.F.,
(4,3,3,4),(2.53759373651446E-13,8.70609204134188E-5,0.00017004098566721,
0.000253023205863598),.UNSPECIFIED.);
#23113=B_SPLINE_CURVE_WITH_KNOTS('',3,(#136733,#136734,#136735,#136736,
#136737,#136738,#136739,#136740,#136741,#136742,#136743,#136744,#136745,
#136746),.UNSPECIFIED.,.F.,.F.,(4,2,2,2,2,2,4),(9.66185494312226E-7,0.00392697955586284,
0.00804085929090517,0.0162655697528746,0.0327021187492143,0.0655183447212016,
0.130949516658934),.UNSPECIFIED.);
#23114=B_SPLINE_CURVE_WITH_KNOTS('',3,(#136759,#136760,#136761,#136762,
#136763,#136764,#136765,#136766,#136767,#136768),.UNSPECIFIED.,.F.,.F.,
(4,3,3,4),(1.35512089641325E-13,8.70609204684551E-5,0.00017004098566191,
0.000253023205798563),.UNSPECIFIED.);
#23115=B_SPLINE_CURVE_WITH_KNOTS('',3,(#136800,#136801,#136802,#136803,
#136804,#136805,#136806,#136807,#136808,#136809),.UNSPECIFIED.,.F.,.F.,
(4,3,3,4),(1.92969421757801E-13,8.7060920517829E-5,0.000170040985827322,
0.00025302320608008),.UNSPECIFIED.);
#23116=B_SPLINE_CURVE_WITH_KNOTS('',3,(#136824,#136825,#136826,#136827,
#136828,#136829,#136830,#136831,#136832,#136833,#136834,#136835,#136836,
#136837),.UNSPECIFIED.,.F.,.F.,(4,2,2,2,2,2,4),(9.66178287892415E-7,0.00392697957748608,
0.0080408593582245,0.0162655699127301,0.0327021190987407,0.0655183508972541,
0.130949528205721),.UNSPECIFIED.);
#23117=B_SPLINE_CURVE_WITH_KNOTS('',3,(#136850,#136851,#136852,#136853,
#136854,#136855,#136856,#136857,#136858,#136859,#136860,#136861,#136862),
 .UNSPECIFIED.,.F.,.F.,(4,3,3,3,4),(8.40873567267271E-14,8.70609204912656E-5,
0.000149888113153304,0.000170040985908062,0.000253023206266478),
 .UNSPECIFIED.);
#23118=B_SPLINE_CURVE_WITH_KNOTS('',3,(#136877,#136878,#136879,#136880,
#136881,#136882,#136883,#136884,#136885,#136886),.UNSPECIFIED.,.F.,.F.,
(4,3,3,4),(0.556212830496238,0.566018336002845,0.571428571428571,0.573654350219912),
 .UNSPECIFIED.);
#23119=B_SPLINE_CURVE_WITH_KNOTS('',3,(#136899,#136900,#136901,#136902,
#136903,#136904,#136905,#136906,#136907,#136908,#136909,#136910,#136911),
 .UNSPECIFIED.,.F.,.F.,(4,3,3,3,4),(2.14110068371842E-13,8.70609204644119E-5,
0.00014988811341431,0.000170040985596898,0.00025302320567211),
 .UNSPECIFIED.);
#23120=B_SPLINE_CURVE_WITH_KNOTS('',3,(#136926,#136927,#136928,#136929,
#136930,#136931,#136932,#136933,#136934,#136935),.UNSPECIFIED.,.F.,.F.,
(4,3,3,4),(0.556212830493125,0.566018337095459,0.571428571428571,0.573654350190219),
 .UNSPECIFIED.);
#23121=B_SPLINE_CURVE_WITH_KNOTS('',3,(#136948,#136949,#136950,#136951,
#136952,#136953,#136954,#136955,#136956,#136957),.UNSPECIFIED.,.F.,.F.,
(4,3,3,4),(9.00758862279578E-14,8.70609204372189E-5,0.00017004098588756,
0.000253023206279836),.UNSPECIFIED.);
#23122=B_SPLINE_CURVE_WITH_KNOTS('',3,(#136972,#136973,#136974,#136975,
#136976,#136977,#136978,#136979,#136980,#136981,#136982,#136983,#136984,
#136985),.UNSPECIFIED.,.F.,.F.,(4,2,2,2,2,2,4),(9.66205425621697E-7,0.00392697955933081,
0.0080408592506326,0.0162655696235016,0.0327021184357382,0.0655183462173166,
0.130949515010481),.UNSPECIFIED.);
#23123=B_SPLINE_CURVE_WITH_KNOTS('',3,(#136998,#136999,#137000,#137001,
#137002,#137003,#137004,#137005,#137006,#137007),.UNSPECIFIED.,.F.,.F.,
(4,3,3,4),(9.05841708095265E-14,8.70609207349165E-5,0.000170040985889652,
0.000253023205987879),.UNSPECIFIED.);
#23124=B_SPLINE_CURVE_WITH_KNOTS('',3,(#137022,#137023,#137024,#137025,
#137026,#137027,#137028,#137029,#137030,#137031,#137032,#137033,#137034,
#137035),.UNSPECIFIED.,.F.,.F.,(4,2,2,2,2,2,4),(9.66222234121705E-7,0.0039269794756902,
0.00804085902143472,0.0162655691092118,0.0327021173752005,0.0655183417329978,
0.13094951369088),.UNSPECIFIED.);
#23125=B_SPLINE_CURVE_WITH_KNOTS('',3,(#137048,#137049,#137050,#137051,
#137052,#137053,#137054,#137055,#137056,#137057),.UNSPECIFIED.,.F.,.F.,
(4,3,3,4),(1.80010415397423E-13,8.70609205854221E-5,0.000170040985761325,
0.000253023205880155),.UNSPECIFIED.);
#23126=B_SPLINE_CURVE_WITH_KNOTS('',3,(#137089,#137090,#137091,#137092,
#137093,#137094,#137095,#137096,#137097,#137098),.UNSPECIFIED.,.F.,.F.,
(4,3,3,4),(1.78220905471141E-13,8.70609204854381E-5,0.000170040985755445,
0.00025302320596902),.UNSPECIFIED.);
#23127=B_SPLINE_CURVE_WITH_KNOTS('',3,(#137130,#137131,#137132,#137133,
#137134,#137135,#137136,#137137,#137138,#137139),.UNSPECIFIED.,.F.,.F.,
(4,3,3,4),(1.58771823130732E-13,8.706092047505E-5,0.000170040985667919,
0.000253023205802976),.UNSPECIFIED.);
#23128=B_SPLINE_CURVE_WITH_KNOTS('',3,(#137154,#137155,#137156,#137157,
#137158,#137159,#137160,#137161,#137162,#137163,#137164,#137165,#137166,
#137167),.UNSPECIFIED.,.F.,.F.,(4,2,2,2,2,2,4),(9.66239005217944E-7,0.00392697936493239,
0.00804085874914389,0.0162655685121116,0.0327021161219164,0.0655183394313766,
0.13094949754352),.UNSPECIFIED.);
#23129=B_SPLINE_CURVE_WITH_KNOTS('',3,(#137180,#137181,#137182,#137183,
#137184,#137185,#137186,#137187,#137188,#137189),.UNSPECIFIED.,.F.,.F.,
(4,3,3,4),(1.50946766794193E-13,8.70609205558374E-5,0.000170040985841153,
0.000253023206069007),.UNSPECIFIED.);
#23130=B_SPLINE_CURVE_WITH_KNOTS('',3,(#137221,#137222,#137223,#137224,
#137225,#137226,#137227,#137228,#137229,#137230),.UNSPECIFIED.,.F.,.F.,
(4,3,3,4),(1.65491426438259E-13,8.70609204190512E-5,0.000170040985661301,
0.000253023205846518),.UNSPECIFIED.);
#23131=B_SPLINE_CURVE_WITH_KNOTS('',3,(#137245,#137246,#137247,#137248,
#137249,#137250,#137251,#137252,#137253,#137254),.UNSPECIFIED.,.F.,.F.,
(4,3,3,4),(0.556212830497802,0.566018335697945,0.571428571428571,0.573654350193131),
 .UNSPECIFIED.);
#23132=B_SPLINE_CURVE_WITH_KNOTS('',3,(#137267,#137268,#137269,#137270,
#137271,#137272,#137273,#137274,#137275,#137276,#137277,#137278,#137279),
 .UNSPECIFIED.,.F.,.F.,(4,3,3,3,4),(1.70398673709338E-13,8.70609205616646E-5,
0.000149888113059747,0.000170040985758334,0.000253023205898846),
 .UNSPECIFIED.);
#23133=B_SPLINE_CURVE_WITH_KNOTS('',3,(#137294,#137295,#137296,#137297,
#137298,#137299,#137300,#137301,#137302,#137303,#137304,#137305,#137306,
#137307),.UNSPECIFIED.,.F.,.F.,(4,2,2,2,2,2,4),(9.66463546611146E-7,0.0039269796958211,
0.00804085923376171,0.0162655693016797,0.03270211751058,0.0655183395302705,
0.130949485085588),.UNSPECIFIED.);
#23134=B_SPLINE_CURVE_WITH_KNOTS('',3,(#137322,#137323,#137324,#137325,
#137326,#137327),.UNSPECIFIED.,.F.,.F.,(4,2,4),(-0.0252969421656862,-0.0126483573154483,
-1.73911152839823E-10),.UNSPECIFIED.);
#23135=B_SPLINE_CURVE_WITH_KNOTS('',3,(#137340,#137341,#137342,#137343,
#137344,#137345,#137346),.UNSPECIFIED.,.F.,.F.,(4,3,4),(0.211502584834065,
0.214285714285714,0.223668160746706),.UNSPECIFIED.);
#23136=B_SPLINE_CURVE_WITH_KNOTS('',3,(#137347,#137348,#137349,#137350,
#137351,#137352),.UNSPECIFIED.,.F.,.F.,(4,2,4),(9.42251804061677E-11,0.0126483643388585,
0.0252969714247671),.UNSPECIFIED.);
#23137=B_SPLINE_CURVE_WITH_KNOTS('',3,(#137383,#137384,#137385,#137386,
#137387,#137388,#137389),.UNSPECIFIED.,.F.,.F.,(4,3,4),(0.211502584834048,
0.214285714285714,0.22366816074129),.UNSPECIFIED.);
#23138=B_SPLINE_CURVE_WITH_KNOTS('',3,(#137390,#137391,#137392,#137393,
#137394,#137395),.UNSPECIFIED.,.F.,.F.,(4,2,4),(1.25234643137483E-10,0.0126483644130537,
0.0252969715703692),.UNSPECIFIED.);
#23139=B_SPLINE_CURVE_WITH_KNOTS('',3,(#137426,#137427,#137428,#137429,
#137430,#137431,#137432),.UNSPECIFIED.,.F.,.F.,(4,3,4),(0.21150258483404,
0.214285714285714,0.223668160746203),.UNSPECIFIED.);
#23140=B_SPLINE_CURVE_WITH_KNOTS('',3,(#137433,#137434,#137435,#137436,
#137437,#137438),.UNSPECIFIED.,.F.,.F.,(4,2,4),(1.42901220958907E-10,0.0126483641798076,
0.0252969707431301),.UNSPECIFIED.);
#23141=B_SPLINE_CURVE_WITH_KNOTS('',3,(#137469,#137470,#137471,#137472,
#137473,#137474,#137475),.UNSPECIFIED.,.F.,.F.,(4,3,4),(0.211502584834064,
0.214285714285714,0.223668160739962),.UNSPECIFIED.);
#23142=B_SPLINE_CURVE_WITH_KNOTS('',3,(#137476,#137477,#137478,#137479,
#137480,#137481),.UNSPECIFIED.,.F.,.F.,(4,2,4),(1.57040128483674E-10,0.0126483646230286,
0.0252969722387553),.UNSPECIFIED.);
#23143=B_SPLINE_CURVE_WITH_KNOTS('',3,(#137512,#137513,#137514,#137515,
#137516,#137517,#137518),.UNSPECIFIED.,.F.,.F.,(4,3,4),(0.211502584834063,
0.214285714285714,0.223668160743146),.UNSPECIFIED.);
#23144=B_SPLINE_CURVE_WITH_KNOTS('',3,(#137519,#137520,#137521,#137522,
#137523,#137524),.UNSPECIFIED.,.F.,.F.,(4,2,4),(1.52830003479099E-10,0.0126483646010041,
0.0252969722035216),.UNSPECIFIED.);
#23145=B_SPLINE_CURVE_WITH_KNOTS('',3,(#137555,#137556,#137557,#137558,
#137559,#137560,#137561),.UNSPECIFIED.,.F.,.F.,(4,3,4),(0.211502584834064,
0.214285714285714,0.223668160739557),.UNSPECIFIED.);
#23146=B_SPLINE_CURVE_WITH_KNOTS('',3,(#137562,#137563,#137564,#137565,
#137566,#137567),.UNSPECIFIED.,.F.,.F.,(4,2,4),(1.48807329848891E-10,0.0126483641904826,
0.0252969707513306),.UNSPECIFIED.);
#23147=B_SPLINE_CURVE_WITH_KNOTS('',3,(#137596,#137597,#137598,#137599,
#137600,#137601),.UNSPECIFIED.,.F.,.F.,(4,2,4),(1.81998596448827E-10,0.0126483575178079,
0.0252969430018216),.UNSPECIFIED.);
#23148=B_SPLINE_CURVE_WITH_KNOTS('',3,(#137626,#137627,#137628,#137629,
#137630,#137631,#137632),.UNSPECIFIED.,.F.,.F.,(4,3,4),(0.211502584834064,
0.214285714285714,0.223668160743121),.UNSPECIFIED.);
#23149=B_SPLINE_CURVE_WITH_KNOTS('',3,(#137633,#137634,#137635,#137636,
#137637,#137638),.UNSPECIFIED.,.F.,.F.,(4,2,4),(9.7444894850297E-11,0.0126483571249872,
0.0252969416070819),.UNSPECIFIED.);
#23150=B_SPLINE_CURVE_WITH_KNOTS('',3,(#137669,#137670,#137671,#137672,
#137673,#137674,#137675),.UNSPECIFIED.,.F.,.F.,(4,3,4),(0.211502584834064,
0.214285714285714,0.223668160737537),.UNSPECIFIED.);
#23151=B_SPLINE_CURVE_WITH_KNOTS('',3,(#137676,#137677,#137678,#137679,
#137680,#137681),.UNSPECIFIED.,.F.,.F.,(4,2,4),(1.68360222936878E-10,0.0126483646033732,
0.0252969722045489),.UNSPECIFIED.);
#23152=B_SPLINE_CURVE_WITH_KNOTS('',3,(#137712,#137713,#137714,#137715,
#137716,#137717,#137718),.UNSPECIFIED.,.F.,.F.,(4,3,4),(0.21150258483406,
0.214285714285714,0.223668160740989),.UNSPECIFIED.);
#23153=B_SPLINE_CURVE_WITH_KNOTS('',3,(#137719,#137720,#137721,#137722,
#137723,#137724),.UNSPECIFIED.,.F.,.F.,(4,2,4),(1.3435638487885E-10,0.0126483643087339,
0.0252969712788357),.UNSPECIFIED.);
#23154=B_SPLINE_CURVE_WITH_KNOTS('',3,(#137755,#137756,#137757,#137758,
#137759,#137760,#137761),.UNSPECIFIED.,.F.,.F.,(4,3,4),(0.211502584834064,
0.214285714285714,0.223668160735638),.UNSPECIFIED.);
#23155=B_SPLINE_CURVE_WITH_KNOTS('',3,(#137762,#137763,#137764,#137765,
#137766,#137767),.UNSPECIFIED.,.F.,.F.,(4,2,4),(1.03868961680616E-10,0.0126483570659925,
0.0252969412940665),.UNSPECIFIED.);
#23156=B_SPLINE_CURVE_WITH_KNOTS('',3,(#137798,#137799,#137800,#137801,
#137802,#137803,#137804),.UNSPECIFIED.,.F.,.F.,(4,3,4),(0.211502584834024,
0.214285714285714,0.223668160739353),.UNSPECIFIED.);
#23157=B_SPLINE_CURVE_WITH_KNOTS('',3,(#137805,#137806,#137807,#137808,
#137809,#137810),.UNSPECIFIED.,.F.,.F.,(4,2,4),(9.76223213263302E-11,0.0126483642710012,
0.0252969711027679),.UNSPECIFIED.);
#23158=B_SPLINE_CURVE_WITH_KNOTS('',3,(#137841,#137842,#137843,#137844,
#137845,#137846,#137847),.UNSPECIFIED.,.F.,.F.,(4,3,4),(0.211502584834064,
0.214285714285714,0.223668160736429),.UNSPECIFIED.);
#23159=B_SPLINE_CURVE_WITH_KNOTS('',3,(#137848,#137849,#137850,#137851,
#137852,#137853),.UNSPECIFIED.,.F.,.F.,(4,2,4),(1.53232547903038E-10,0.0126483575945804,
0.0252969433218694),.UNSPECIFIED.);
#23160=B_SPLINE_CURVE_WITH_KNOTS('',3,(#137884,#137885,#137886,#137887,
#137888,#137889,#137890),.UNSPECIFIED.,.F.,.F.,(4,3,4),(0.211502584834064,
0.214285714285714,0.223668160740088),.UNSPECIFIED.);
#23161=B_SPLINE_CURVE_WITH_KNOTS('',3,(#137891,#137892,#137893,#137894,
#137895,#137896),.UNSPECIFIED.,.F.,.F.,(4,2,4),(1.70742253820634E-10,0.0126483643594943,
0.0252969713224395),.UNSPECIFIED.);
#23162=B_SPLINE_CURVE_WITH_KNOTS('',3,(#137927,#137928,#137929,#137930,
#137931,#137932,#137933),.UNSPECIFIED.,.F.,.F.,(4,3,4),(0.211502584833965,
0.214285714285714,0.22366816073647),.UNSPECIFIED.);
#23163=B_SPLINE_CURVE_WITH_KNOTS('',3,(#137934,#137935,#137936,#137937,
#137938,#137939),.UNSPECIFIED.,.F.,.F.,(4,2,4),(1.17570601323076E-10,0.0126483643814668,
0.0252969715083944),.UNSPECIFIED.);
#23164=B_SPLINE_CURVE_WITH_KNOTS('',3,(#137970,#137971,#137972,#137973,
#137974,#137975,#137976),.UNSPECIFIED.,.F.,.F.,(4,3,4),(0.211502584833903,
0.214285714285714,0.223668160739684),.UNSPECIFIED.);
#23165=B_SPLINE_CURVE_WITH_KNOTS('',3,(#137977,#137978,#137979,#137980,
#137981,#137982),.UNSPECIFIED.,.F.,.F.,(4,2,4),(1.58595950739882E-10,0.0126483645926137,
0.0252969721769568),.UNSPECIFIED.);
#23166=B_SPLINE_CURVE_WITH_KNOTS('',3,(#138013,#138014,#138015,#138016,
#138017,#138018,#138019),.UNSPECIFIED.,.F.,.F.,(4,3,4),(0.211502584833963,
0.214285714285714,0.223668160739601),.UNSPECIFIED.);
#23167=B_SPLINE_CURVE_WITH_KNOTS('',3,(#138020,#138021,#138022,#138023,
#138024,#138025),.UNSPECIFIED.,.F.,.F.,(4,2,4),(1.37481879759042E-10,0.0126483642605855,
0.0252969710301908),.UNSPECIFIED.);
#23168=B_SPLINE_CURVE_WITH_KNOTS('',3,(#138056,#138057,#138058,#138059,
#138060,#138061,#138062),.UNSPECIFIED.,.F.,.F.,(4,3,4),(0.211502584833935,
0.214285714285714,0.223668160739935),.UNSPECIFIED.);
#23169=B_SPLINE_CURVE_WITH_KNOTS('',3,(#138063,#138064,#138065,#138066,
#138067,#138068),.UNSPECIFIED.,.F.,.F.,(4,2,4),(1.15062703877832E-10,0.0126483572960972,
0.0252969421882394),.UNSPECIFIED.);
#23170=B_SPLINE_CURVE_WITH_KNOTS('',3,(#138099,#138100,#138101,#138102,
#138103,#138104,#138105),.UNSPECIFIED.,.F.,.F.,(4,3,4),(0.211502584833671,
0.214285714285714,0.223668160740443),.UNSPECIFIED.);
#23171=B_SPLINE_CURVE_WITH_KNOTS('',3,(#138106,#138107,#138108,#138109,
#138110,#138111),.UNSPECIFIED.,.F.,.F.,(4,2,4),(1.65806997188092E-10,0.0126483573808185,
0.0252969424808111),.UNSPECIFIED.);
#23172=B_SPLINE_CURVE_WITH_KNOTS('',3,(#138142,#138143,#138144,#138145,
#138146,#138147,#138148),.UNSPECIFIED.,.F.,.F.,(4,3,4),(0.211502584833923,
0.214285714285714,0.223668160474533),.UNSPECIFIED.);
#23173=B_SPLINE_CURVE_WITH_KNOTS('',3,(#138149,#138150,#138151,#138152,
#138153,#138154),.UNSPECIFIED.,.F.,.F.,(4,2,4),(1.3364996508922E-10,0.0126483641814018,
0.0252969708486838),.UNSPECIFIED.);
#23174=B_SPLINE_CURVE_WITH_KNOTS('',3,(#138186,#138187,#138188,#138189,
#138190,#138191,#138192),.UNSPECIFIED.,.F.,.F.,(4,3,4),(0.21150258483406,
0.214285714285714,0.223668160737251),.UNSPECIFIED.);
#23175=B_SPLINE_CURVE_WITH_KNOTS('',3,(#138193,#138194,#138195,#138196,
#138197,#138198),.UNSPECIFIED.,.F.,.F.,(4,2,4),(1.65464212098833E-10,0.012648364586302,
0.0252969721645957),.UNSPECIFIED.);
#23176=B_SPLINE_CURVE_WITH_KNOTS('',3,(#138228,#138229,#138230,#138231,
#138232,#138233,#138234),.UNSPECIFIED.,.F.,.F.,(4,3,4),(0.211502584834061,
0.214285714285714,0.223668160736262),.UNSPECIFIED.);
#23177=B_SPLINE_CURVE_WITH_KNOTS('',3,(#138235,#138236,#138237,#138238,
#138239,#138240),.UNSPECIFIED.,.F.,.F.,(4,2,4),(7.5709302282454E-11,0.0126483643841512,
0.0252969716087726),.UNSPECIFIED.);
#23178=B_SPLINE_CURVE_WITH_KNOTS('',3,(#138271,#138272,#138273,#138274,
#138275,#138276,#138277),.UNSPECIFIED.,.F.,.F.,(4,3,4),(0.211502584834065,
0.214285714285714,0.223668160742396),.UNSPECIFIED.);
#23179=B_SPLINE_CURVE_WITH_KNOTS('',3,(#138278,#138279,#138280,#138281,
#138282,#138283),.UNSPECIFIED.,.F.,.F.,(4,2,4),(1.28302262445121E-10,0.0126483641874972,
0.0252969707835284),.UNSPECIFIED.);
#23180=B_SPLINE_CURVE_WITH_KNOTS('',3,(#138314,#138315,#138316,#138317,
#138318,#138319,#138320),.UNSPECIFIED.,.F.,.F.,(4,3,4),(0.211502584834065,
0.214285714285714,0.223668160739137),.UNSPECIFIED.);
#23181=B_SPLINE_CURVE_WITH_KNOTS('',3,(#138321,#138322,#138323,#138324,
#138325,#138326),.UNSPECIFIED.,.F.,.F.,(4,2,4),(1.21129596779304E-10,0.0126483571382297,
0.0252969415887335),.UNSPECIFIED.);
#23182=B_SPLINE_CURVE_WITH_KNOTS('',3,(#138357,#138358,#138359,#138360,
#138361,#138362,#138363),.UNSPECIFIED.,.F.,.F.,(4,3,4),(0.211502584834064,
0.214285714285714,0.223668160739874),.UNSPECIFIED.);
#23183=B_SPLINE_CURVE_WITH_KNOTS('',3,(#138364,#138365,#138366,#138367,
#138368,#138369),.UNSPECIFIED.,.F.,.F.,(4,2,4),(8.64124104036477E-11,0.0126483569711156,
0.0252969409241859),.UNSPECIFIED.);
#23184=B_SPLINE_CURVE_WITH_KNOTS('',3,(#138400,#138401,#138402,#138403,
#138404,#138405,#138406),.UNSPECIFIED.,.F.,.F.,(4,3,4),(0.211502584834065,
0.214285714285714,0.223668160739885),.UNSPECIFIED.);
#23185=B_SPLINE_CURVE_WITH_KNOTS('',3,(#138407,#138408,#138409,#138410,
#138411,#138412),.UNSPECIFIED.,.F.,.F.,(4,2,4),(2.07944688460402E-10,0.012648364645067,
0.02529697221805),.UNSPECIFIED.);
#23186=B_SPLINE_CURVE_WITH_KNOTS('',3,(#138443,#138444,#138445,#138446,
#138447,#138448,#138449),.UNSPECIFIED.,.F.,.F.,(4,3,4),(0.211502584834065,
0.214285714285714,0.223668160741145),.UNSPECIFIED.);
#23187=B_SPLINE_CURVE_WITH_KNOTS('',3,(#138450,#138451,#138452,#138453,
#138454,#138455),.UNSPECIFIED.,.F.,.F.,(4,2,4),(1.69193695001643E-10,0.0126483642077223,
0.0252969707648244),.UNSPECIFIED.);
#23188=B_SPLINE_CURVE_WITH_KNOTS('',3,(#138486,#138487,#138488,#138489,
#138490,#138491,#138492),.UNSPECIFIED.,.F.,.F.,(4,3,4),(0.211502584834065,
0.214285714285714,0.223668160742228),.UNSPECIFIED.);
#23189=B_SPLINE_CURVE_WITH_KNOTS('',3,(#138493,#138494,#138495,#138496,
#138497,#138498),.UNSPECIFIED.,.F.,.F.,(4,2,4),(4.48927338603257E-11,0.0126483642352892,
0.0252969711325811),.UNSPECIFIED.);
#23190=B_SPLINE_CURVE_WITH_KNOTS('',3,(#138522,#138523,#138524,#138525,
#138526,#138527,#138528),.UNSPECIFIED.,.F.,.F.,(4,3,4),(0.211502584834063,
0.214285714285714,0.223668160734462),.UNSPECIFIED.);
#23191=B_SPLINE_CURVE_WITH_KNOTS('',3,(#138551,#138552,#138553,#138554,
#138555,#138556),.UNSPECIFIED.,.F.,.F.,(4,2,4),(1.55326272845714E-12,0.0126511155057583,
0.0253019892655775),.UNSPECIFIED.);
#23192=B_SPLINE_CURVE_WITH_KNOTS('',3,(#138573,#138574,#138575,#138576,
#138577,#138578,#138579),.UNSPECIFIED.,.F.,.F.,(4,3,4),(0.556108173865714,
0.558333952657053,0.568296447146679),.UNSPECIFIED.);
#23193=B_SPLINE_CURVE_WITH_KNOTS('',3,(#138580,#138581,#138582,#138583,
#138584,#138585),.UNSPECIFIED.,.F.,.F.,(4,2,4),(-0.0253019896340801,-0.012651115732023,
-4.08147370067891E-11),.UNSPECIFIED.);
#23194=B_SPLINE_CURVE_WITH_KNOTS('',3,(#138616,#138617,#138618,#138619,
#138620,#138621,#138622),.UNSPECIFIED.,.F.,.F.,(4,3,4),(0.556108173865714,
0.558333952657053,0.568296447141869),.UNSPECIFIED.);
#23195=B_SPLINE_CURVE_WITH_KNOTS('',3,(#138623,#138624,#138625,#138626,
#138627,#138628),.UNSPECIFIED.,.F.,.F.,(4,2,4),(-0.0253019894957092,-0.0126511156236248,
-2.40536167372962E-11),.UNSPECIFIED.);
#23196=B_SPLINE_CURVE_WITH_KNOTS('',3,(#138659,#138660,#138661,#138662,
#138663,#138664,#138665),.UNSPECIFIED.,.F.,.F.,(4,3,4),(0.556108173865714,
0.558333952657053,0.568296447138677),.UNSPECIFIED.);
#23197=B_SPLINE_CURVE_WITH_KNOTS('',3,(#138666,#138667,#138668,#138669,
#138670,#138671),.UNSPECIFIED.,.F.,.F.,(4,2,4),(-0.0253019896232341,-0.0126511156790116,
-3.02607001956279E-11),.UNSPECIFIED.);
#23198=B_SPLINE_CURVE_WITH_KNOTS('',3,(#138702,#138703,#138704,#138705,
#138706,#138707,#138708),.UNSPECIFIED.,.F.,.F.,(4,3,4),(0.556108173865714,
0.558333952657053,0.568296447137058),.UNSPECIFIED.);
#23199=B_SPLINE_CURVE_WITH_KNOTS('',3,(#138709,#138710,#138711,#138712,
#138713,#138714),.UNSPECIFIED.,.F.,.F.,(4,2,4),(-0.0253019894885685,-0.0126511156165778,
-1.93016713723182E-11),.UNSPECIFIED.);
#23200=B_SPLINE_CURVE_WITH_KNOTS('',3,(#138745,#138746,#138747,#138748,
#138749,#138750,#138751),.UNSPECIFIED.,.F.,.F.,(4,3,4),(0.556108173865714,
0.558333952657053,0.568296447144668),.UNSPECIFIED.);
#23201=B_SPLINE_CURVE_WITH_KNOTS('',3,(#138752,#138753,#138754,#138755,
#138756,#138757),.UNSPECIFIED.,.F.,.F.,(4,2,4),(-0.02530198959003,-0.0126511156559188,
-1.74384499895819E-11),.UNSPECIFIED.);
#23202=B_SPLINE_CURVE_WITH_KNOTS('',3,(#138788,#138789,#138790,#138791,
#138792,#138793,#138794),.UNSPECIFIED.,.F.,.F.,(4,3,4),(0.556108173865714,
0.558333952657053,0.568296447144199),.UNSPECIFIED.);
#23203=B_SPLINE_CURVE_WITH_KNOTS('',3,(#138795,#138796,#138797,#138798,
#138799,#138800),.UNSPECIFIED.,.F.,.F.,(4,2,4),(-0.0253019895178097,-0.0126511156113887,
-1.91482177336333E-11),.UNSPECIFIED.);
#23204=B_SPLINE_CURVE_WITH_KNOTS('',3,(#138831,#138832,#138833,#138834,
#138835,#138836,#138837),.UNSPECIFIED.,.F.,.F.,(4,3,4),(0.556108173865714,
0.558333952657053,0.568296447147839),.UNSPECIFIED.);
#23205=B_SPLINE_CURVE_WITH_KNOTS('',3,(#138838,#138839,#138840,#138841,
#138842,#138843),.UNSPECIFIED.,.F.,.F.,(4,2,4),(-0.0253019896252546,-0.012651115666266,
-1.96323547696498E-11),.UNSPECIFIED.);
#23206=B_SPLINE_CURVE_WITH_KNOTS('',3,(#138874,#138875,#138876,#138877,
#138878,#138879,#138880),.UNSPECIFIED.,.F.,.F.,(4,3,4),(0.556108173865714,
0.558333952657053,0.568296447147786),.UNSPECIFIED.);
#23207=B_SPLINE_CURVE_WITH_KNOTS('',3,(#138881,#138882,#138883,#138884,
#138885,#138886),.UNSPECIFIED.,.F.,.F.,(4,2,4),(-0.0253019895396078,-0.0126511156269564,
-2.44738500299047E-11),.UNSPECIFIED.);
#23208=B_SPLINE_CURVE_WITH_KNOTS('',3,(#138917,#138918,#138919,#138920,
#138921,#138922,#138923),.UNSPECIFIED.,.F.,.F.,(4,3,4),(0.556108173865715,
0.558333952657054,0.568296447135626),.UNSPECIFIED.);
#23209=B_SPLINE_CURVE_WITH_KNOTS('',3,(#138924,#138925,#138926,#138927,
#138928,#138929),.UNSPECIFIED.,.F.,.F.,(4,2,4),(-0.0253019895314073,-0.012651115614323,
-3.54363170751437E-11),.UNSPECIFIED.);
#23210=B_SPLINE_CURVE_WITH_KNOTS('',3,(#138960,#138961,#138962,#138963,
#138964,#138965,#138966),.UNSPECIFIED.,.F.,.F.,(4,3,4),(0.556108173865715,
0.558333952657055,0.568296447138926),.UNSPECIFIED.);
#23211=B_SPLINE_CURVE_WITH_KNOTS('',3,(#138967,#138968,#138969,#138970,
#138971,#138972),.UNSPECIFIED.,.F.,.F.,(4,2,4),(-0.025301989606925,-0.0126511156406089,
-2.78329234659758E-11),.UNSPECIFIED.);
#23212=B_SPLINE_CURVE_WITH_KNOTS('',3,(#139003,#139004,#139005,#139006,
#139007,#139008,#139009),.UNSPECIFIED.,.F.,.F.,(4,3,4),(0.556108173865715,
0.558333952657055,0.568296447147264),.UNSPECIFIED.);
#23213=B_SPLINE_CURVE_WITH_KNOTS('',3,(#139010,#139011,#139012,#139013,
#139014,#139015),.UNSPECIFIED.,.F.,.F.,(4,2,4),(-0.0253019896476435,-0.0126511157227825,
-2.66785100955236E-11),.UNSPECIFIED.);
#23214=B_SPLINE_CURVE_WITH_KNOTS('',3,(#139046,#139047,#139048,#139049,
#139050,#139051,#139052),.UNSPECIFIED.,.F.,.F.,(4,3,4),(0.556108173865715,
0.558333952657055,0.56829644715269),.UNSPECIFIED.);
#23215=B_SPLINE_CURVE_WITH_KNOTS('',3,(#139053,#139054,#139055,#139056,
#139057,#139058),.UNSPECIFIED.,.F.,.F.,(4,2,4),(-0.0253019895519308,-0.0126511156492357,
-3.55825612030625E-11),.UNSPECIFIED.);
#23216=B_SPLINE_CURVE_WITH_KNOTS('',3,(#139089,#139090,#139091,#139092,
#139093,#139094,#139095),.UNSPECIFIED.,.F.,.F.,(4,3,4),(0.556108173865715,
0.558333952657055,0.568296447144007),.UNSPECIFIED.);
#23217=B_SPLINE_CURVE_WITH_KNOTS('',3,(#139096,#139097,#139098,#139099,
#139100,#139101),.UNSPECIFIED.,.F.,.F.,(4,2,4),(-0.025301989516701,-0.01265111561885,
-5.85913262352022E-12),.UNSPECIFIED.);
#23218=B_SPLINE_CURVE_WITH_KNOTS('',3,(#139130,#139131,#139132,#139133,
#139134,#139135),.UNSPECIFIED.,.F.,.F.,(4,2,4),(-0.0253019896278924,-0.0126511156474334,
0.),.UNSPECIFIED.);
#23219=B_SPLINE_CURVE_WITH_KNOTS('',3,(#139160,#139161,#139162,#139163,
#139164,#139165,#139166),.UNSPECIFIED.,.F.,.F.,(4,3,4),(0.556108173865715,
0.558333952657055,0.568296447138361),.UNSPECIFIED.);
#23220=B_SPLINE_CURVE_WITH_KNOTS('',3,(#139167,#139168,#139169,#139170,
#139171,#139172),.UNSPECIFIED.,.F.,.F.,(4,2,4),(-0.025301989496816,-0.0126511156321275,
-2.29995258949067E-11),.UNSPECIFIED.);
#23221=B_SPLINE_CURVE_WITH_KNOTS('',3,(#139203,#139204,#139205,#139206,
#139207,#139208,#139209),.UNSPECIFIED.,.F.,.F.,(4,3,4),(0.556108173865715,
0.558333952657055,0.56829644715017),.UNSPECIFIED.);
#23222=B_SPLINE_CURVE_WITH_KNOTS('',3,(#139210,#139211,#139212,#139213,
#139214,#139215),.UNSPECIFIED.,.F.,.F.,(4,2,4),(-0.0253019895418659,-0.0126511156530789,
-2.9359289305253E-11),.UNSPECIFIED.);
#23223=B_SPLINE_CURVE_WITH_KNOTS('',3,(#139246,#139247,#139248,#139249,
#139250,#139251,#139252),.UNSPECIFIED.,.F.,.F.,(4,3,4),(0.556108173865715,
0.558333952657055,0.568296447135577),.UNSPECIFIED.);
#23224=B_SPLINE_CURVE_WITH_KNOTS('',3,(#139253,#139254,#139255,#139256,
#139257,#139258),.UNSPECIFIED.,.F.,.F.,(4,2,4),(-0.0253019895837948,-0.0126511156586353,
-1.96183694289864E-11),.UNSPECIFIED.);
#23225=B_SPLINE_CURVE_WITH_KNOTS('',3,(#139289,#139290,#139291,#139292,
#139293,#139294,#139295),.UNSPECIFIED.,.F.,.F.,(4,3,4),(0.556108173865715,
0.558333952657055,0.568296447140135),.UNSPECIFIED.);
#23226=B_SPLINE_CURVE_WITH_KNOTS('',3,(#139296,#139297,#139298,#139299,
#139300,#139301),.UNSPECIFIED.,.F.,.F.,(4,2,4),(-0.0253019895221298,-0.0126511156124946,
-2.86418840034219E-11),.UNSPECIFIED.);
#23227=B_SPLINE_CURVE_WITH_KNOTS('',3,(#139332,#139333,#139334,#139335,
#139336,#139337,#139338),.UNSPECIFIED.,.F.,.F.,(4,3,4),(0.556108173865715,
0.558333952657055,0.568296447141357),.UNSPECIFIED.);
#23228=B_SPLINE_CURVE_WITH_KNOTS('',3,(#139339,#139340,#139341,#139342,
#139343,#139344),.UNSPECIFIED.,.F.,.F.,(4,2,4),(-0.0253019896253231,-0.0126511157,
-2.89356767713134E-11),.UNSPECIFIED.);
#23229=B_SPLINE_CURVE_WITH_KNOTS('',3,(#139375,#139376,#139377,#139378,
#139379,#139380,#139381),.UNSPECIFIED.,.F.,.F.,(4,3,4),(0.556108173865716,
0.558333952657057,0.568296447129919),.UNSPECIFIED.);
#23230=B_SPLINE_CURVE_WITH_KNOTS('',3,(#139382,#139383,#139384,#139385,
#139386,#139387),.UNSPECIFIED.,.F.,.F.,(4,2,4),(-0.0253019895356154,-0.0126511156254898,
-2.51503019799149E-11),.UNSPECIFIED.);
#23231=B_SPLINE_CURVE_WITH_KNOTS('',3,(#139418,#139419,#139420,#139421,
#139422,#139423,#139424),.UNSPECIFIED.,.F.,.F.,(4,3,4),(0.556108173865715,
0.558333952657055,0.568296447143907),.UNSPECIFIED.);
#23232=B_SPLINE_CURVE_WITH_KNOTS('',3,(#139425,#139426,#139427,#139428,
#139429,#139430),.UNSPECIFIED.,.F.,.F.,(4,2,4),(-0.0253019895393503,-0.0126511156383291,
-2.10483228069158E-11),.UNSPECIFIED.);
#23233=B_SPLINE_CURVE_WITH_KNOTS('',3,(#139461,#139462,#139463,#139464,
#139465,#139466,#139467),.UNSPECIFIED.,.F.,.F.,(4,3,4),(0.556108173865715,
0.558333952657055,0.568296447145893),.UNSPECIFIED.);
#23234=B_SPLINE_CURVE_WITH_KNOTS('',3,(#139468,#139469,#139470,#139471,
#139472,#139473),.UNSPECIFIED.,.F.,.F.,(4,2,4),(-0.025301989566972,-0.0126511156375726,
-1.20351853483136E-11),.UNSPECIFIED.);
#23235=B_SPLINE_CURVE_WITH_KNOTS('',3,(#139504,#139505,#139506,#139507,
#139508,#139509,#139510),.UNSPECIFIED.,.F.,.F.,(4,3,4),(0.556108173865715,
0.558333952657055,0.568296447143574),.UNSPECIFIED.);
#23236=B_SPLINE_CURVE_WITH_KNOTS('',3,(#139511,#139512,#139513,#139514,
#139515,#139516),.UNSPECIFIED.,.F.,.F.,(4,2,4),(-0.0253019895694301,-0.0126511156503794,
-6.77978506669064E-12),.UNSPECIFIED.);
#23237=B_SPLINE_CURVE_WITH_KNOTS('',3,(#139547,#139548,#139549,#139550,
#139551,#139552,#139553),.UNSPECIFIED.,.F.,.F.,(4,3,4),(0.556108173865716,
0.558333952657056,0.56829644714022),.UNSPECIFIED.);
#23238=B_SPLINE_CURVE_WITH_KNOTS('',3,(#139554,#139555,#139556,#139557,
#139558,#139559),.UNSPECIFIED.,.F.,.F.,(4,2,4),(-0.0253019895254194,-0.0126511155865999,
-2.44209027999709E-11),.UNSPECIFIED.);
#23239=B_SPLINE_CURVE_WITH_KNOTS('',3,(#139590,#139591,#139592,#139593,
#139594,#139595,#139596),.UNSPECIFIED.,.F.,.F.,(4,3,4),(0.556108173865715,
0.558333952657055,0.568296447128213),.UNSPECIFIED.);
#23240=B_SPLINE_CURVE_WITH_KNOTS('',3,(#139597,#139598,#139599,#139600,
#139601,#139602),.UNSPECIFIED.,.F.,.F.,(4,2,4),(-0.0253019895140171,-0.0126511156345661,
-1.57640844822282E-11),.UNSPECIFIED.);
#23241=B_SPLINE_CURVE_WITH_KNOTS('',3,(#139633,#139634,#139635,#139636,
#139637,#139638,#139639),.UNSPECIFIED.,.F.,.F.,(4,3,4),(0.556108173865715,
0.558333952657071,0.56829644714659),.UNSPECIFIED.);
#23242=B_SPLINE_CURVE_WITH_KNOTS('',3,(#139640,#139641,#139642,#139643,
#139644,#139645),.UNSPECIFIED.,.F.,.F.,(4,2,4),(-0.0253019896200955,-0.0126511156782531,
-1.58387990223385E-11),.UNSPECIFIED.);
#23243=B_SPLINE_CURVE_WITH_KNOTS('',3,(#139676,#139677,#139678,#139679,
#139680,#139681,#139682),.UNSPECIFIED.,.F.,.F.,(4,3,4),(0.556108173865714,
0.558333952657053,0.568296447152951),.UNSPECIFIED.);
#23244=B_SPLINE_CURVE_WITH_KNOTS('',3,(#139683,#139684,#139685,#139686,
#139687,#139688),.UNSPECIFIED.,.F.,.F.,(4,2,4),(-0.0253019895367723,-0.0126511156270699,
-2.72321817873511E-11),.UNSPECIFIED.);
#23245=B_SPLINE_CURVE_WITH_KNOTS('',3,(#139719,#139720,#139721,#139722,
#139723,#139724,#139725),.UNSPECIFIED.,.F.,.F.,(4,3,4),(0.556108173865714,
0.558333952657053,0.568296447150853),.UNSPECIFIED.);
#23246=B_SPLINE_CURVE_WITH_KNOTS('',3,(#139726,#139727,#139728,#139729,
#139730,#139731),.UNSPECIFIED.,.F.,.F.,(4,2,4),(-0.0253019894899887,-0.012651115619704,
-1.88235260711878E-11),.UNSPECIFIED.);
#23247=B_SPLINE_CURVE_WITH_KNOTS('',3,(#139751,#139752,#139753,#139754,
#139755,#139756,#139757),.UNSPECIFIED.,.F.,.F.,(4,3,4),(0.556108173865714,
0.558333952657053,0.568296447114548),.UNSPECIFIED.);
#23248=B_SPLINE_CURVE_WITH_KNOTS('',3,(#139784,#139785,#139786,#139787,
#139788,#139789),.UNSPECIFIED.,.F.,.F.,(4,2,4),(-0.0253032195848505,-0.0126517291919461,
0.),.UNSPECIFIED.);
#23249=B_SPLINE_CURVE_WITH_KNOTS('',3,(#139798,#139799,#139800,#139801,
#139802,#139803),.UNSPECIFIED.,.F.,.F.,(4,2,4),(0.,0.0126517048550591,0.0253031720944598),
 .UNSPECIFIED.);
#23250=B_SPLINE_CURVE_WITH_KNOTS('',3,(#139823,#139824,#139825,#139826,
#139827,#139828),.UNSPECIFIED.,.F.,.F.,(4,2,4),(4.38171128399974E-11,0.0126517292144799,
0.0253032373814633),.UNSPECIFIED.);
#23251=B_SPLINE_CURVE_WITH_KNOTS('',3,(#139848,#139849,#139850,#139851,
#139852,#139853),.UNSPECIFIED.,.F.,.F.,(4,2,4),(3.57814230103522E-11,0.0126517292120754,
0.0253032358787696),.UNSPECIFIED.);
#23252=B_SPLINE_CURVE_WITH_KNOTS('',3,(#139873,#139874,#139875,#139876,
#139877,#139878),.UNSPECIFIED.,.F.,.F.,(4,2,4),(1.2439987344094E-11,0.0126517291603593,
0.0253032288431388),.UNSPECIFIED.);
#23253=B_SPLINE_CURVE_WITH_KNOTS('',3,(#139898,#139899,#139900,#139901,
#139902,#139903),.UNSPECIFIED.,.F.,.F.,(4,2,4),(0.,0.0126517046604698,0.0253031780482239),
 .UNSPECIFIED.);
#23254=B_SPLINE_CURVE_WITH_KNOTS('',3,(#139923,#139924,#139925,#139926,
#139927,#139928),.UNSPECIFIED.,.F.,.F.,(4,2,4),(0.,0.0126517291322339,0.025303231857666),
 .UNSPECIFIED.);
#23255=B_SPLINE_CURVE_WITH_KNOTS('',3,(#139948,#139949,#139950,#139951,
#139952,#139953),.UNSPECIFIED.,.F.,.F.,(4,2,4),(0.,0.0126517291489857,0.0253032322180855),
 .UNSPECIFIED.);
#23256=B_SPLINE_CURVE_WITH_KNOTS('',3,(#139973,#139974,#139975,#139976,
#139977,#139978),.UNSPECIFIED.,.F.,.F.,(4,2,4),(3.64720174388672E-11,0.0126517292140638,
0.0253032332575142),.UNSPECIFIED.);
#23257=B_SPLINE_CURVE_WITH_KNOTS('',3,(#139998,#139999,#140000,#140001,
#140002,#140003),.UNSPECIFIED.,.F.,.F.,(4,2,4),(0.,0.0126517291501688,0.0253032315632285),
 .UNSPECIFIED.);
#23258=B_SPLINE_CURVE_WITH_KNOTS('',3,(#140023,#140024,#140025,#140026,
#140027,#140028),.UNSPECIFIED.,.F.,.F.,(4,2,4),(4.98468781855941E-11,0.0126517292310175,
0.0253032323234676),.UNSPECIFIED.);
#23259=B_SPLINE_CURVE_WITH_KNOTS('',3,(#140048,#140049,#140050,#140051,
#140052,#140053),.UNSPECIFIED.,.F.,.F.,(4,2,4),(1.78170881484123E-11,0.0126517291939891,
0.0253032393088991),.UNSPECIFIED.);
#23260=B_SPLINE_CURVE_WITH_KNOTS('',3,(#140073,#140074,#140075,#140076,
#140077,#140078),.UNSPECIFIED.,.F.,.F.,(4,2,4),(0.,0.012651729151704,0.0253032336443197),
 .UNSPECIFIED.);
#23261=B_SPLINE_CURVE_WITH_KNOTS('',3,(#140098,#140099,#140100,#140101,
#140102,#140103),.UNSPECIFIED.,.F.,.F.,(4,2,4),(1.29662877955301E-11,0.0126517291972145,
0.0253032338446115),.UNSPECIFIED.);
#23262=B_SPLINE_CURVE_WITH_KNOTS('',3,(#140123,#140124,#140125,#140126,
#140127,#140128),.UNSPECIFIED.,.F.,.F.,(4,2,4),(1.06872879746175E-11,0.0126517291668657,
0.0253032367900497),.UNSPECIFIED.);
#23263=B_SPLINE_CURVE_WITH_KNOTS('',3,(#140148,#140149,#140150,#140151,
#140152,#140153),.UNSPECIFIED.,.F.,.F.,(4,2,4),(0.,0.0126517291525847,0.0253032326082015),
 .UNSPECIFIED.);
#23264=B_SPLINE_CURVE_WITH_KNOTS('',3,(#140173,#140174,#140175,#140176,
#140177,#140178),.UNSPECIFIED.,.F.,.F.,(4,2,4),(0.,0.0126517291593631,0.0253032317143608),
 .UNSPECIFIED.);
#23265=B_SPLINE_CURVE_WITH_KNOTS('',3,(#140198,#140199,#140200,#140201,
#140202,#140203),.UNSPECIFIED.,.F.,.F.,(4,2,4),(0.,0.0126517291345216,0.025303232365844),
 .UNSPECIFIED.);
#23266=B_SPLINE_CURVE_WITH_KNOTS('',3,(#140223,#140224,#140225,#140226,
#140227,#140228),.UNSPECIFIED.,.F.,.F.,(4,2,4),(2.76890456237896E-11,0.0126517291812319,
0.0253032339729562),.UNSPECIFIED.);
#23267=B_SPLINE_CURVE_WITH_KNOTS('',3,(#140248,#140249,#140250,#140251,
#140252,#140253),.UNSPECIFIED.,.F.,.F.,(4,2,4),(0.,0.012651729178449,0.0253032365218916),
 .UNSPECIFIED.);
#23268=B_SPLINE_CURVE_WITH_KNOTS('',3,(#140273,#140274,#140275,#140276,
#140277,#140278),.UNSPECIFIED.,.F.,.F.,(4,2,4),(0.,0.0126517291320085,0.025303230810267),
 .UNSPECIFIED.);
#23269=B_SPLINE_CURVE_WITH_KNOTS('',3,(#140298,#140299,#140300,#140301,
#140302,#140303),.UNSPECIFIED.,.F.,.F.,(4,2,4),(1.74085481906006E-11,0.0126517291619092,
0.0253032334768344),.UNSPECIFIED.);
#23270=B_SPLINE_CURVE_WITH_KNOTS('',3,(#140323,#140324,#140325,#140326,
#140327,#140328),.UNSPECIFIED.,.F.,.F.,(4,2,4),(0.,0.0126517291613853,0.0253032329245391),
 .UNSPECIFIED.);
#23271=B_SPLINE_CURVE_WITH_KNOTS('',3,(#140348,#140349,#140350,#140351,
#140352,#140353),.UNSPECIFIED.,.F.,.F.,(4,2,4),(1.10512950735125E-11,0.0126517291598583,
0.0253032349922658),.UNSPECIFIED.);
#23272=B_SPLINE_CURVE_WITH_KNOTS('',3,(#140373,#140374,#140375,#140376,
#140377,#140378),.UNSPECIFIED.,.F.,.F.,(4,2,4),(0.,0.0126517291624426,0.025303233284192),
 .UNSPECIFIED.);
#23273=B_SPLINE_CURVE_WITH_KNOTS('',3,(#140398,#140399,#140400,#140401,
#140402,#140403),.UNSPECIFIED.,.F.,.F.,(4,2,4),(3.26902022083678E-11,0.0126517291872101,
0.0253032306372425),.UNSPECIFIED.);
#23274=B_SPLINE_CURVE_WITH_KNOTS('',3,(#140423,#140424,#140425,#140426,
#140427,#140428),.UNSPECIFIED.,.F.,.F.,(4,2,4),(5.06203466173173E-11,0.0126517292236369,
0.0253032369878863),.UNSPECIFIED.);
#23275=B_SPLINE_CURVE_WITH_KNOTS('',3,(#140448,#140449,#140450,#140451,
#140452,#140453),.UNSPECIFIED.,.F.,.F.,(4,2,4),(1.01410125554829E-11,0.0126517291529624,
0.0253032321074454),.UNSPECIFIED.);
#23276=B_SPLINE_CURVE_WITH_KNOTS('',3,(#140473,#140474,#140475,#140476,
#140477,#140478),.UNSPECIFIED.,.F.,.F.,(4,2,4),(0.,0.0126517291283134,0.0253032314766247),
 .UNSPECIFIED.);
#23277=B_SPLINE_CURVE_WITH_KNOTS('',3,(#140508,#140509,#140510,#140511,
#140512,#140513),.UNSPECIFIED.,.F.,.F.,(4,2,4),(-0.0257915092833096,-0.0126485466669513,
-2.19810107615626E-11),.UNSPECIFIED.);
#23278=B_SPLINE_CURVE_WITH_KNOTS('',3,(#140527,#140528,#140529,#140530,
#140531,#140532),.UNSPECIFIED.,.F.,.F.,(4,2,4),(2.70362522355475E-11,0.0126485466623622,
0.0257911586180436),.UNSPECIFIED.);
#23279=B_SPLINE_CURVE_WITH_KNOTS('',3,(#140556,#140557,#140558,#140559,
#140560,#140561),.UNSPECIFIED.,.F.,.F.,(4,2,4),(1.43542774964306E-11,0.0126485466751825,
0.025791424513763),.UNSPECIFIED.);
#23280=B_SPLINE_CURVE_WITH_KNOTS('',3,(#140585,#140586,#140587,#140588,
#140589,#140590),.UNSPECIFIED.,.F.,.F.,(4,2,4),(6.79797826907082E-11,0.0126485467551672,
0.0257912698313032),.UNSPECIFIED.);
#23281=B_SPLINE_CURVE_WITH_KNOTS('',3,(#140614,#140615,#140616,#140617,
#140618,#140619),.UNSPECIFIED.,.F.,.F.,(4,2,4),(3.16048530260618E-11,0.0126485466866181,
0.0257913915485856),.UNSPECIFIED.);
#23282=B_SPLINE_CURVE_WITH_KNOTS('',3,(#140648,#140649,#140650,#140651,
#140652,#140653),.UNSPECIFIED.,.F.,.F.,(4,2,4),(2.60113353670021E-11,0.0126485466803885,
0.025791354907496),.UNSPECIFIED.);
#23283=B_SPLINE_CURVE_WITH_KNOTS('',3,(#140677,#140678,#140679,#140680,
#140681,#140682),.UNSPECIFIED.,.F.,.F.,(4,2,4),(5.48323673168424E-11,0.0126485466970084,
0.0257912960282793),.UNSPECIFIED.);
#23284=B_SPLINE_CURVE_WITH_KNOTS('',3,(#140706,#140707,#140708,#140709,
#140710,#140711),.UNSPECIFIED.,.F.,.F.,(4,2,4),(5.26304401860954E-11,0.0126485467607656,
0.0257913064734023),.UNSPECIFIED.);
#23285=B_SPLINE_CURVE_WITH_KNOTS('',3,(#140735,#140736,#140737,#140738,
#140739,#140740),.UNSPECIFIED.,.F.,.F.,(4,2,4),(3.13430767661628E-11,0.0126485466847367,
0.0257914462712551),.UNSPECIFIED.);
#23286=B_SPLINE_CURVE_WITH_KNOTS('',3,(#140764,#140765,#140766,#140767,
#140768,#140769),.UNSPECIFIED.,.F.,.F.,(4,2,4),(3.72919687755852E-11,0.0126485466486127,
0.0257915212993866),.UNSPECIFIED.);
#23287=B_SPLINE_CURVE_WITH_KNOTS('',3,(#140793,#140794,#140795,#140796,
#140797,#140798),.UNSPECIFIED.,.F.,.F.,(4,2,4),(3.33686758784895E-11,0.0126485466185285,
0.0257914200237712),.UNSPECIFIED.);
#23288=B_SPLINE_CURVE_WITH_KNOTS('',3,(#140822,#140823,#140824,#140825,
#140826,#140827),.UNSPECIFIED.,.F.,.F.,(4,2,4),(1.92687878762538E-11,0.0126485466368729,
0.0257914335980706),.UNSPECIFIED.);
#23289=B_SPLINE_CURVE_WITH_KNOTS('',3,(#140851,#140852,#140853,#140854,
#140855,#140856),.UNSPECIFIED.,.F.,.F.,(4,2,4),(2.44340999839289E-11,0.0126485466797976,
0.025791423235164),.UNSPECIFIED.);
#23290=B_SPLINE_CURVE_WITH_KNOTS('',3,(#140880,#140881,#140882,#140883,
#140884,#140885),.UNSPECIFIED.,.F.,.F.,(4,2,4),(5.66736717316295E-11,0.0126485467389853,
0.0257913878277949),.UNSPECIFIED.);
#23291=B_SPLINE_CURVE_WITH_KNOTS('',3,(#140914,#140915,#140916,#140917,
#140918,#140919),.UNSPECIFIED.,.F.,.F.,(4,2,4),(0.,0.012648546623643,0.0257912485305581),
 .UNSPECIFIED.);
#23292=B_SPLINE_CURVE_WITH_KNOTS('',3,(#140943,#140944,#140945,#140946,
#140947,#140948),.UNSPECIFIED.,.F.,.F.,(4,2,4),(5.37728797176222E-11,0.0126485467320549,
0.0257913769744669),.UNSPECIFIED.);
#23293=B_SPLINE_CURVE_WITH_KNOTS('',3,(#140972,#140973,#140974,#140975,
#140976,#140977),.UNSPECIFIED.,.F.,.F.,(4,2,4),(0.,0.0126485466447246,0.0257914432668697),
 .UNSPECIFIED.);
#23294=B_SPLINE_CURVE_WITH_KNOTS('',3,(#141001,#141002,#141003,#141004,
#141005,#141006),.UNSPECIFIED.,.F.,.F.,(4,2,4),(4.69338058508619E-11,0.0126485467018863,
0.0257913835745087),.UNSPECIFIED.);
#23295=B_SPLINE_CURVE_WITH_KNOTS('',3,(#141035,#141036,#141037,#141038,
#141039,#141040),.UNSPECIFIED.,.F.,.F.,(4,2,4),(2.38219565115975E-11,0.012648546654904,
0.0257914732516701),.UNSPECIFIED.);
#23296=B_SPLINE_CURVE_WITH_KNOTS('',3,(#141064,#141065,#141066,#141067,
#141068,#141069),.UNSPECIFIED.,.F.,.F.,(4,2,4),(2.97326209195323E-11,0.0126485466848618,
0.0257915677794139),.UNSPECIFIED.);
#23297=B_SPLINE_CURVE_WITH_KNOTS('',3,(#141093,#141094,#141095,#141096,
#141097,#141098),.UNSPECIFIED.,.F.,.F.,(4,2,4),(2.79225229640744E-11,0.0126485466708951,
0.0257914238548662),.UNSPECIFIED.);
#23298=B_SPLINE_CURVE_WITH_KNOTS('',3,(#141122,#141123,#141124,#141125,
#141126,#141127),.UNSPECIFIED.,.F.,.F.,(4,2,4),(1.32799613034488E-11,0.0126485465903112,
0.0257914139200059),.UNSPECIFIED.);
#23299=B_SPLINE_CURVE_WITH_KNOTS('',3,(#141151,#141152,#141153,#141154,
#141155,#141156),.UNSPECIFIED.,.F.,.F.,(4,2,4),(3.26716219031941E-11,0.0126485466900674,
0.025791388788007),.UNSPECIFIED.);
#23300=B_SPLINE_CURVE_WITH_KNOTS('',3,(#141180,#141181,#141182,#141183,
#141184,#141185),.UNSPECIFIED.,.F.,.F.,(4,2,4),(6.80582916254403E-11,0.0126485467142699,
0.0257914144991197),.UNSPECIFIED.);
#23301=B_SPLINE_CURVE_WITH_KNOTS('',3,(#141214,#141215,#141216,#141217,
#141218,#141219),.UNSPECIFIED.,.F.,.F.,(4,2,4),(4.44473432394692E-11,0.0126485466600686,
0.0257912643856431),.UNSPECIFIED.);
#23302=B_SPLINE_CURVE_WITH_KNOTS('',3,(#141248,#141249,#141250,#141251,
#141252,#141253),.UNSPECIFIED.,.F.,.F.,(4,2,4),(3.6215316177288E-11,0.0126485466901811,
0.0257914329539347),.UNSPECIFIED.);
#23303=B_SPLINE_CURVE_WITH_KNOTS('',3,(#141277,#141278,#141279,#141280,
#141281,#141282),.UNSPECIFIED.,.F.,.F.,(4,2,4),(2.63012159668852E-11,0.0126485466618793,
0.0257914669865645),.UNSPECIFIED.);
#23304=B_SPLINE_CURVE_WITH_KNOTS('',3,(#141306,#141307,#141308,#141309,
#141310,#141311),.UNSPECIFIED.,.F.,.F.,(4,2,4),(4.52322623488674E-11,0.0126485467153518,
0.0257913545346247),.UNSPECIFIED.);
#23305=B_SPLINE_CURVE_WITH_KNOTS('',3,(#141335,#141336,#141337,#141338,
#141339,#141340),.UNSPECIFIED.,.F.,.F.,(4,2,4),(4.14734752956722E-11,0.0126485466677345,
0.0257914043426878),.UNSPECIFIED.);
#23306=B_SPLINE_CURVE_WITH_KNOTS('',3,(#141377,#141378,#141379,#141380,
#141381,#141382),.UNSPECIFIED.,.F.,.F.,(4,2,4),(-0.0252997150098972,-0.0126500317843385,
-9.10712679921821E-9),.UNSPECIFIED.);
#23307=B_SPLINE_CURVE_WITH_KNOTS('',3,(#141410,#141411,#141412,#141413,
#141414,#141415),.UNSPECIFIED.,.F.,.F.,(4,2,4),(-0.0252993192639046,-0.0126498730539567,
-9.07035945657553E-9),.UNSPECIFIED.);
#23308=B_SPLINE_CURVE_WITH_KNOTS('',3,(#141443,#141444,#141445,#141446,
#141447,#141448),.UNSPECIFIED.,.F.,.F.,(4,2,4),(-0.0252993221176286,-0.0126498617303957,
-9.08144366998376E-9),.UNSPECIFIED.);
#23309=B_SPLINE_CURVE_WITH_KNOTS('',3,(#141476,#141477,#141478,#141479,
#141480,#141481),.UNSPECIFIED.,.F.,.F.,(4,2,4),(-0.025299328104327,-0.0126498714243405,
-9.07123582152836E-9),.UNSPECIFIED.);
#23310=B_SPLINE_CURVE_WITH_KNOTS('',3,(#141509,#141510,#141511,#141512,
#141513,#141514),.UNSPECIFIED.,.F.,.F.,(4,2,4),(-0.025299338488532,-0.0126498691500846,
-9.07425860494082E-9),.UNSPECIFIED.);
#23311=B_SPLINE_CURVE_WITH_KNOTS('',3,(#141542,#141543,#141544,#141545,
#141546,#141547),.UNSPECIFIED.,.F.,.F.,(4,2,4),(-0.0252997272114458,-0.0126500317748764,
-9.10567698325648E-9),.UNSPECIFIED.);
#23312=B_SPLINE_CURVE_WITH_KNOTS('',3,(#141575,#141576,#141577,#141578,
#141579,#141580),.UNSPECIFIED.,.F.,.F.,(4,2,4),(-0.0252993471269051,-0.01264987588227,
-9.06701983285907E-9),.UNSPECIFIED.);
#23313=B_SPLINE_CURVE_WITH_KNOTS('',3,(#141608,#141609,#141610,#141611,
#141612,#141613),.UNSPECIFIED.,.F.,.F.,(4,2,4),(-0.0252993194291543,-0.0126498641945722,
-9.07929462515278E-9),.UNSPECIFIED.);
#23314=B_SPLINE_CURVE_WITH_KNOTS('',3,(#141641,#141642,#141643,#141644,
#141645,#141646),.UNSPECIFIED.,.F.,.F.,(4,2,4),(-0.0252993149765833,-0.0126498658638244,
-9.07693491550288E-9),.UNSPECIFIED.);
#23315=B_SPLINE_CURVE_WITH_KNOTS('',3,(#141674,#141675,#141676,#141677,
#141678,#141679),.UNSPECIFIED.,.F.,.F.,(4,2,4),(-0.0252997346785984,-0.0126500317266587,
-9.10414309565621E-9),.UNSPECIFIED.);
#23316=B_SPLINE_CURVE_WITH_KNOTS('',3,(#141707,#141708,#141709,#141710,
#141711,#141712),.UNSPECIFIED.,.F.,.F.,(4,2,4),(-0.0252993458238753,-0.0126498773505181,
-9.0656312422277E-9),.UNSPECIFIED.);
#23317=B_SPLINE_CURVE_WITH_KNOTS('',3,(#141740,#141741,#141742,#141743,
#141744,#141745),.UNSPECIFIED.,.F.,.F.,(4,2,4),(-0.0252993101823874,-0.0126498642958816,
-9.07914507464191E-9),.UNSPECIFIED.);
#23318=B_SPLINE_CURVE_WITH_KNOTS('',3,(#141773,#141774,#141775,#141776,
#141777,#141778),.UNSPECIFIED.,.F.,.F.,(4,2,4),(-0.0252993301983058,-0.0126498632692199,
-9.07977696154583E-9),.UNSPECIFIED.);
#23319=B_SPLINE_CURVE_WITH_KNOTS('',3,(#141806,#141807,#141808,#141809,
#141810,#141811),.UNSPECIFIED.,.F.,.F.,(4,2,4),(-0.0252993173610177,-0.012649865812899,
-9.07689320581162E-9),.UNSPECIFIED.);
#23320=B_SPLINE_CURVE_WITH_KNOTS('',3,(#141836,#141837,#141838,#141839,
#141840,#141841),.UNSPECIFIED.,.F.,.F.,(4,2,4),(-0.0252993161138789,-0.0126498661496497,
-9.07674461980701E-9),.UNSPECIFIED.);
#23321=B_SPLINE_CURVE_WITH_KNOTS('',3,(#141863,#141864,#141865,#141866,
#141867,#141868),.UNSPECIFIED.,.F.,.F.,(4,2,4),(-0.0252997344586295,-0.0126500317232582,
-9.10763827896566E-9),.UNSPECIFIED.);
#23322=B_SPLINE_CURVE_WITH_KNOTS('',3,(#141896,#141897,#141898,#141899,
#141900,#141901),.UNSPECIFIED.,.F.,.F.,(4,2,4),(-0.0252993204603601,-0.0126498639881955,
-9.07887972440014E-9),.UNSPECIFIED.);
#23323=B_SPLINE_CURVE_WITH_KNOTS('',3,(#141929,#141930,#141931,#141932,
#141933,#141934),.UNSPECIFIED.,.F.,.F.,(4,2,4),(-0.0252993253610345,-0.012649862213264,
-9.08052791293024E-9),.UNSPECIFIED.);
#23324=B_SPLINE_CURVE_WITH_KNOTS('',3,(#141962,#141963,#141964,#141965,
#141966,#141967),.UNSPECIFIED.,.F.,.F.,(4,2,4),(-0.0252992970947547,-0.0126498664943603,
-9.07626198851097E-9),.UNSPECIFIED.);
#23325=B_SPLINE_CURVE_WITH_KNOTS('',3,(#141995,#141996,#141997,#141998,
#141999,#142000),.UNSPECIFIED.,.F.,.F.,(4,2,4),(-0.0252992902045865,-0.0126498538085401,
-9.05754709082385E-9),.UNSPECIFIED.);
#23326=B_SPLINE_CURVE_WITH_KNOTS('',3,(#142029,#142030,#142031,#142032,
#142033,#142034),.UNSPECIFIED.,.F.,.F.,(4,2,4),(-0.025299728807157,-0.0126500317762664,
-9.11489488747419E-9),.UNSPECIFIED.);
#23327=B_SPLINE_CURVE_WITH_KNOTS('',3,(#142061,#142062,#142063,#142064,
#142065,#142066),.UNSPECIFIED.,.F.,.F.,(4,2,4),(-0.0252993271765603,-0.0126498623727777,
-9.0807460960407E-9),.UNSPECIFIED.);
#23328=B_SPLINE_CURVE_WITH_KNOTS('',3,(#142094,#142095,#142096,#142097,
#142098,#142099),.UNSPECIFIED.,.F.,.F.,(4,2,4),(-0.0252997271572641,-0.0126500317584131,
-9.10477810159294E-9),.UNSPECIFIED.);
#23329=B_SPLINE_CURVE_WITH_KNOTS('',3,(#142127,#142128,#142129,#142130,
#142131,#142132),.UNSPECIFIED.,.F.,.F.,(4,2,4),(-0.0252993045945163,-0.0126498634942832,
-9.07959531518121E-9),.UNSPECIFIED.);
#23330=B_SPLINE_CURVE_WITH_KNOTS('',3,(#142160,#142161,#142162,#142163,
#142164,#142165),.UNSPECIFIED.,.F.,.F.,(4,2,4),(-0.0252993278041195,-0.0126498659235352,
-9.07719203621649E-9),.UNSPECIFIED.);
#23331=B_SPLINE_CURVE_WITH_KNOTS('',3,(#142193,#142194,#142195,#142196,
#142197,#142198),.UNSPECIFIED.,.F.,.F.,(4,2,4),(-0.0252993190119561,-0.0126498640052631,
-9.0793093460162E-9),.UNSPECIFIED.);
#23332=B_SPLINE_CURVE_WITH_KNOTS('',3,(#142226,#142227,#142228,#142229,
#142230,#142231),.UNSPECIFIED.,.F.,.F.,(4,2,4),(-0.0252993234646114,-0.0126498667429259,
-9.07600854194168E-9),.UNSPECIFIED.);
#23333=B_SPLINE_CURVE_WITH_KNOTS('',3,(#142259,#142260,#142261,#142262,
#142263,#142264),.UNSPECIFIED.,.F.,.F.,(4,2,4),(-0.0252997144599162,-0.012650031762626,
-9.10456312425145E-9),.UNSPECIFIED.);
#23334=B_SPLINE_CURVE_WITH_KNOTS('',3,(#142292,#142293,#142294,#142295,
#142296,#142297),.UNSPECIFIED.,.F.,.F.,(4,2,4),(-0.0252993049756229,-0.0126498626584025,
-9.0801991724232E-9),.UNSPECIFIED.);
#23335=B_SPLINE_CURVE_WITH_KNOTS('',3,(#142330,#142331,#142332,#142333,
#142334,#142335),.UNSPECIFIED.,.F.,.F.,(4,2,4),(0.,0.0126483033528629,0.0252967254469703),
 .UNSPECIFIED.);
#23336=B_SPLINE_CURVE_WITH_KNOTS('',3,(#142371,#142372,#142373,#142374,
#142375,#142376),.UNSPECIFIED.,.F.,.F.,(4,2,4),(0.,0.0126483617678804,0.0252969654295701),
 .UNSPECIFIED.);
#23337=B_SPLINE_CURVE_WITH_KNOTS('',3,(#142412,#142413,#142414,#142415,
#142416,#142417),.UNSPECIFIED.,.F.,.F.,(4,2,4),(0.,0.0126482976272339,0.0252967020886337),
 .UNSPECIFIED.);
#23338=B_SPLINE_CURVE_WITH_KNOTS('',3,(#142453,#142454,#142455,#142456,
#142457,#142458),.UNSPECIFIED.,.F.,.F.,(4,2,4),(0.,0.0126483617612936,0.0252969765449637),
 .UNSPECIFIED.);
#23339=B_SPLINE_CURVE_WITH_KNOTS('',3,(#142494,#142495,#142496,#142497,
#142498,#142499),.UNSPECIFIED.,.F.,.F.,(4,2,4),(0.,0.0126483617791059,0.0252969761281077),
 .UNSPECIFIED.);
#23340=B_SPLINE_CURVE_WITH_KNOTS('',3,(#142535,#142536,#142537,#142538,
#142539,#142540),.UNSPECIFIED.,.F.,.F.,(4,2,4),(0.,0.0126483617559022,0.0252969652965633),
 .UNSPECIFIED.);
#23341=B_SPLINE_CURVE_WITH_KNOTS('',3,(#142576,#142577,#142578,#142579,
#142580,#142581),.UNSPECIFIED.,.F.,.F.,(4,2,4),(0.,0.0126483052677277,0.0252967333732343),
 .UNSPECIFIED.);
#23342=B_SPLINE_CURVE_WITH_KNOTS('',3,(#142617,#142618,#142619,#142620,
#142621,#142622),.UNSPECIFIED.,.F.,.F.,(4,2,4),(0.,0.0126482994530337,0.0252967093118385),
 .UNSPECIFIED.);
#23343=B_SPLINE_CURVE_WITH_KNOTS('',3,(#142658,#142659,#142660,#142661,
#142662,#142663),.UNSPECIFIED.,.F.,.F.,(4,2,4),(0.,0.0126483617643872,0.0252969765390469),
 .UNSPECIFIED.);
#23344=B_SPLINE_CURVE_WITH_KNOTS('',3,(#142699,#142700,#142701,#142702,
#142703,#142704),.UNSPECIFIED.,.F.,.F.,(4,2,4),(0.,0.0126482983272483,0.0252967047813038),
 .UNSPECIFIED.);
#23345=B_SPLINE_CURVE_WITH_KNOTS('',3,(#142740,#142741,#142742,#142743,
#142744,#142745),.UNSPECIFIED.,.F.,.F.,(4,2,4),(0.,0.0126483000717647,0.0252967121149593),
 .UNSPECIFIED.);
#23346=B_SPLINE_CURVE_WITH_KNOTS('',3,(#142781,#142782,#142783,#142784,
#142785,#142786),.UNSPECIFIED.,.F.,.F.,(4,2,4),(0.,0.0126483617690835,0.0252969653140276),
 .UNSPECIFIED.);
#23347=B_SPLINE_CURVE_WITH_KNOTS('',3,(#142822,#142823,#142824,#142825,
#142826,#142827),.UNSPECIFIED.,.F.,.F.,(4,2,4),(2.42740058061956E-11,0.0126483617583391,
0.0252969653213079),.UNSPECIFIED.);
#23348=B_SPLINE_CURVE_WITH_KNOTS('',3,(#142863,#142864,#142865,#142866,
#142867,#142868),.UNSPECIFIED.,.F.,.F.,(4,2,4),(0.,0.0126483617625851,0.0252969737117307),
 .UNSPECIFIED.);
#23349=B_SPLINE_CURVE_WITH_KNOTS('',3,(#142904,#142905,#142906,#142907,
#142908,#142909),.UNSPECIFIED.,.F.,.F.,(4,2,4),(0.,0.0126483617752743,0.0252969768202461),
 .UNSPECIFIED.);
#23350=B_SPLINE_CURVE_WITH_KNOTS('',3,(#142945,#142946,#142947,#142948,
#142949,#142950),.UNSPECIFIED.,.F.,.F.,(4,2,4),(0.,0.0126483617401393,0.025296965465005),
 .UNSPECIFIED.);
#23351=B_SPLINE_CURVE_WITH_KNOTS('',3,(#142986,#142987,#142988,#142989,
#142990,#142991),.UNSPECIFIED.,.F.,.F.,(4,2,4),(0.,0.012648298093685,0.0252967038543137),
 .UNSPECIFIED.);
#23352=B_SPLINE_CURVE_WITH_KNOTS('',3,(#143027,#143028,#143029,#143030,
#143031,#143032),.UNSPECIFIED.,.F.,.F.,(4,2,4),(0.,0.0126483024110683,0.0252967329236766),
 .UNSPECIFIED.);
#23353=B_SPLINE_CURVE_WITH_KNOTS('',3,(#143068,#143069,#143070,#143071,
#143072,#143073),.UNSPECIFIED.,.F.,.F.,(4,2,4),(1.9407486965572E-11,0.0126483617769253,
0.0252969745847458),.UNSPECIFIED.);
#23354=B_SPLINE_CURVE_WITH_KNOTS('',3,(#143109,#143110,#143111,#143112,
#143113,#143114),.UNSPECIFIED.,.F.,.F.,(4,2,4),(3.3601607052622E-11,0.012648308385465,
0.0252967460828744),.UNSPECIFIED.);
#23355=B_SPLINE_CURVE_WITH_KNOTS('',3,(#143150,#143151,#143152,#143153,
#143154,#143155),.UNSPECIFIED.,.F.,.F.,(4,2,4),(0.,0.0126483007561831,0.0252967254663462),
 .UNSPECIFIED.);
#23356=B_SPLINE_CURVE_WITH_KNOTS('',3,(#143188,#143189,#143190,#143191,
#143192,#143193),.UNSPECIFIED.,.F.,.F.,(4,2,4),(0.,0.0126482990716502,0.0252967077163187),
 .UNSPECIFIED.);
#23357=B_SPLINE_CURVE_WITH_KNOTS('',3,(#143223,#143224,#143225,#143226,
#143227,#143228),.UNSPECIFIED.,.F.,.F.,(4,2,4),(4.24920173066688E-11,0.0126483000002919,
0.025296722178295),.UNSPECIFIED.);
#23358=B_SPLINE_CURVE_WITH_KNOTS('',3,(#143264,#143265,#143266,#143267,
#143268,#143269),.UNSPECIFIED.,.F.,.F.,(4,2,4),(0.,0.0126482982349249,0.0252967043333024),
 .UNSPECIFIED.);
#23359=B_SPLINE_CURVE_WITH_KNOTS('',3,(#143305,#143306,#143307,#143308,
#143309,#143310),.UNSPECIFIED.,.F.,.F.,(4,2,4),(0.,0.0126483617896171,0.025296965364044),
 .UNSPECIFIED.);
#23360=B_SPLINE_CURVE_WITH_KNOTS('',3,(#143346,#143347,#143348,#143349,
#143350,#143351),.UNSPECIFIED.,.F.,.F.,(4,2,4),(0.,0.0126483617446494,0.0252969654514837),
 .UNSPECIFIED.);
#23361=B_SPLINE_CURVE_WITH_KNOTS('',3,(#143387,#143388,#143389,#143390,
#143391,#143392),.UNSPECIFIED.,.F.,.F.,(4,2,4),(0.,0.01264836176774,0.0252969653009797),
 .UNSPECIFIED.);
#23362=B_SPLINE_CURVE_WITH_KNOTS('',3,(#143428,#143429,#143430,#143431,
#143432,#143433),.UNSPECIFIED.,.F.,.F.,(4,2,4),(0.,0.012648361762527,0.0252969743405282),
 .UNSPECIFIED.);
#23363=B_SPLINE_CURVE_WITH_KNOTS('',3,(#143469,#143470,#143471,#143472,
#143473,#143474),.UNSPECIFIED.,.F.,.F.,(4,2,4),(3.26919061841809E-11,0.0126483617530401,
0.025296965503827),.UNSPECIFIED.);
#23364=B_SPLINE_CURVE_WITH_KNOTS('',3,(#143504,#143505,#143506,#143507,
#143508,#143509),.UNSPECIFIED.,.F.,.F.,(4,2,4),(-0.0253036322111694,-0.0126517037466635,
-1.82800663495186E-10),.UNSPECIFIED.);
#23365=B_SPLINE_CURVE_WITH_KNOTS('',3,(#143529,#143530,#143531,#143532,
#143533,#143534),.UNSPECIFIED.,.F.,.F.,(4,2,4),(-0.0253032917436892,-0.0126516212476504,
-6.7092234545818E-12),.UNSPECIFIED.);
#23366=B_SPLINE_CURVE_WITH_KNOTS('',3,(#143554,#143555,#143556,#143557,
#143558,#143559),.UNSPECIFIED.,.F.,.F.,(4,2,4),(-0.0253036321774632,-0.0126517036083302,
-2.09170042397844E-11),.UNSPECIFIED.);
#23367=B_SPLINE_CURVE_WITH_KNOTS('',3,(#143579,#143580,#143581,#143582,
#143583,#143584),.UNSPECIFIED.,.F.,.F.,(4,2,4),(-0.0253036321684814,-0.0126517036417179,
-1.15808182488131E-10),.UNSPECIFIED.);
#23368=B_SPLINE_CURVE_WITH_KNOTS('',3,(#143604,#143605,#143606,#143607,
#143608,#143609),.UNSPECIFIED.,.F.,.F.,(4,2,4),(-0.0253036321869942,-0.0126517036462115,
-1.10797839653065E-10),.UNSPECIFIED.);
#23369=B_SPLINE_CURVE_WITH_KNOTS('',3,(#143629,#143630,#143631,#143632,
#143633,#143634),.UNSPECIFIED.,.F.,.F.,(4,2,4),(-0.0253036322201411,-0.0126517037535042,
-1.90251512460771E-10),.UNSPECIFIED.);
#23370=B_SPLINE_CURVE_WITH_KNOTS('',3,(#143654,#143655,#143656,#143657,
#143658,#143659),.UNSPECIFIED.,.F.,.F.,(4,2,4),(-0.0253036322061587,-0.0126517037427219,
-1.93522909502919E-10),.UNSPECIFIED.);
#23371=B_SPLINE_CURVE_WITH_KNOTS('',3,(#143679,#143680,#143681,#143682,
#143683,#143684),.UNSPECIFIED.,.F.,.F.,(4,2,4),(-0.0253036321241486,-0.0126517036041792,
-9.10544729892937E-11),.UNSPECIFIED.);
#23372=B_SPLINE_CURVE_WITH_KNOTS('',3,(#143704,#143705,#143706,#143707,
#143708,#143709),.UNSPECIFIED.,.F.,.F.,(4,2,4),(-0.0253032837977553,-0.0126516193848244,
-1.11454907802955E-10),.UNSPECIFIED.);
#23373=B_SPLINE_CURVE_WITH_KNOTS('',3,(#143729,#143730,#143731,#143732,
#143733,#143734),.UNSPECIFIED.,.F.,.F.,(4,2,4),(-0.0253032936362909,-0.0126516217100339,
-6.41719316574196E-12),.UNSPECIFIED.);
#23374=B_SPLINE_CURVE_WITH_KNOTS('',3,(#143754,#143755,#143756,#143757,
#143758,#143759),.UNSPECIFIED.,.F.,.F.,(4,2,4),(-0.0253036321434187,-0.0126517035746939,
0.),.UNSPECIFIED.);
#23375=B_SPLINE_CURVE_WITH_KNOTS('',3,(#143779,#143780,#143781,#143782,
#143783,#143784),.UNSPECIFIED.,.F.,.F.,(4,2,4),(-0.0253032880541102,-0.0126516204139794,
-1.41031603062558E-10),.UNSPECIFIED.);
#23376=B_SPLINE_CURVE_WITH_KNOTS('',3,(#143804,#143805,#143806,#143807,
#143808,#143809),.UNSPECIFIED.,.F.,.F.,(4,2,4),(-0.0253036322200184,-0.0126517036652856,
-4.99830593581052E-11),.UNSPECIFIED.);
#23377=B_SPLINE_CURVE_WITH_KNOTS('',3,(#143829,#143830,#143831,#143832,
#143833,#143834),.UNSPECIFIED.,.F.,.F.,(4,2,4),(-0.0253036322039681,-0.012651703705871,
-1.54916319355936E-10),.UNSPECIFIED.);
#23378=B_SPLINE_CURVE_WITH_KNOTS('',3,(#143854,#143855,#143856,#143857,
#143858,#143859),.UNSPECIFIED.,.F.,.F.,(4,2,4),(-0.0253036299712287,-0.0126517025076815,
-2.78628856098528E-12),.UNSPECIFIED.);
#23379=B_SPLINE_CURVE_WITH_KNOTS('',3,(#143879,#143880,#143881,#143882,
#143883,#143884),.UNSPECIFIED.,.F.,.F.,(4,2,4),(-0.0253032960389127,-0.0126516223592375,
-1.19824782041089E-10),.UNSPECIFIED.);
#23380=B_SPLINE_CURVE_WITH_KNOTS('',3,(#143904,#143905,#143906,#143907,
#143908,#143909),.UNSPECIFIED.,.F.,.F.,(4,2,4),(-0.0253032498580712,-0.0126516111196444,
0.),.UNSPECIFIED.);
#23381=B_SPLINE_CURVE_WITH_KNOTS('',3,(#143929,#143930,#143931,#143932,
#143933,#143934),.UNSPECIFIED.,.F.,.F.,(4,2,4),(-0.0253032543198873,-0.012651612194739,
0.),.UNSPECIFIED.);
#23382=B_SPLINE_CURVE_WITH_KNOTS('',3,(#143954,#143955,#143956,#143957,
#143958,#143959),.UNSPECIFIED.,.F.,.F.,(4,2,4),(-0.0253036321462399,-0.0126517035856047,
-7.17744960687661E-12),.UNSPECIFIED.);
#23383=B_SPLINE_CURVE_WITH_KNOTS('',3,(#143979,#143980,#143981,#143982,
#143983,#143984),.UNSPECIFIED.,.F.,.F.,(4,2,4),(-0.0253032981944482,-0.0126516228680173,
-1.27145845935095E-10),.UNSPECIFIED.);
#23384=B_SPLINE_CURVE_WITH_KNOTS('',3,(#144004,#144005,#144006,#144007,
#144008,#144009),.UNSPECIFIED.,.F.,.F.,(4,2,4),(-0.0253032720073819,-0.0126516164724433,
0.),.UNSPECIFIED.);
#23385=B_SPLINE_CURVE_WITH_KNOTS('',3,(#144029,#144030,#144031,#144032,
#144033,#144034),.UNSPECIFIED.,.F.,.F.,(4,2,4),(-0.025303632136923,-0.012651703583944,
-8.44966457913543E-12),.UNSPECIFIED.);
#23386=B_SPLINE_CURVE_WITH_KNOTS('',3,(#144054,#144055,#144056,#144057,
#144058,#144059),.UNSPECIFIED.,.F.,.F.,(4,2,4),(-0.0253036321454915,-0.0126517036104632,
-1.04495596203735E-10),.UNSPECIFIED.);
#23387=B_SPLINE_CURVE_WITH_KNOTS('',3,(#144079,#144080,#144081,#144082,
#144083,#144084),.UNSPECIFIED.,.F.,.F.,(4,2,4),(-0.0253036321600805,-0.0126517035775229,
0.),.UNSPECIFIED.);
#23388=B_SPLINE_CURVE_WITH_KNOTS('',3,(#144104,#144105,#144106,#144107,
#144108,#144109),.UNSPECIFIED.,.F.,.F.,(4,2,4),(-0.0253036321591695,-0.0126517036265382,
-2.34760544337576E-11),.UNSPECIFIED.);
#23389=B_SPLINE_CURVE_WITH_KNOTS('',3,(#144129,#144130,#144131,#144132,
#144133,#144134),.UNSPECIFIED.,.F.,.F.,(4,2,4),(-0.0253036322011602,-0.0126517037454701,
-1.96367942739695E-10),.UNSPECIFIED.);
#23390=B_SPLINE_CURVE_WITH_KNOTS('',3,(#144154,#144155,#144156,#144157,
#144158,#144159),.UNSPECIFIED.,.F.,.F.,(4,2,4),(-0.0253036321964258,-0.0126517036155337,
-2.2322820675269E-11),.UNSPECIFIED.);
#23391=B_SPLINE_CURVE_WITH_KNOTS('',3,(#144179,#144180,#144181,#144182,
#144183,#144184),.UNSPECIFIED.,.F.,.F.,(4,2,4),(-0.0253032929844905,-0.0126516215735631,
-3.93026722278478E-11),.UNSPECIFIED.);
#23392=B_SPLINE_CURVE_WITH_KNOTS('',3,(#144204,#144205,#144206,#144207,
#144208,#144209),.UNSPECIFIED.,.F.,.F.,(4,2,4),(-0.0253036321980525,-0.0126517036572632,
-4.59963178656153E-11),.UNSPECIFIED.);
#23393=B_SPLINE_CURVE_WITH_KNOTS('',3,(#144229,#144230,#144231,#144232,
#144233,#144234),.UNSPECIFIED.,.F.,.F.,(4,2,4),(-0.0253028607889791,-0.0126513115894774,
-1.43257597451374E-9),.UNSPECIFIED.);
#23394=B_SPLINE_CURVE_WITH_KNOTS('',3,(#144250,#144251,#144252,#144253,
#144254,#144255),.UNSPECIFIED.,.F.,.F.,(4,2,4),(-0.0253028678808171,-0.0126513117178962,
-1.53780291972661E-9),.UNSPECIFIED.);
#23395=B_SPLINE_CURVE_WITH_KNOTS('',3,(#144271,#144272,#144273,#144274,
#144275,#144276),.UNSPECIFIED.,.F.,.F.,(4,2,4),(-0.0253028686448891,-0.012651311734525,
-1.57900790706544E-9),.UNSPECIFIED.);
#23396=B_SPLINE_CURVE_WITH_KNOTS('',3,(#144292,#144293,#144294,#144295,
#144296,#144297),.UNSPECIFIED.,.F.,.F.,(4,2,4),(-0.0253028608314155,-0.0126513117590326,
-1.57566134445508E-9),.UNSPECIFIED.);
#23397=B_SPLINE_CURVE_WITH_KNOTS('',3,(#144313,#144314,#144315,#144316,
#144317,#144318),.UNSPECIFIED.,.F.,.F.,(4,2,4),(-0.0253028679915641,-0.0126513116532287,
-1.47354626417462E-9),.UNSPECIFIED.);
#23398=B_SPLINE_CURVE_WITH_KNOTS('',3,(#144334,#144335,#144336,#144337,
#144338,#144339),.UNSPECIFIED.,.F.,.F.,(4,2,4),(-0.0253028685599515,-0.0126513116039704,
-1.43719535231068E-9),.UNSPECIFIED.);
#23399=B_SPLINE_CURVE_WITH_KNOTS('',3,(#144355,#144356,#144357,#144358,
#144359,#144360),.UNSPECIFIED.,.F.,.F.,(4,2,4),(-0.0253028676392111,-0.0126513116536948,
-1.4995063558898E-9),.UNSPECIFIED.);
#23400=B_SPLINE_CURVE_WITH_KNOTS('',3,(#144376,#144377,#144378,#144379,
#144380,#144381),.UNSPECIFIED.,.F.,.F.,(4,2,4),(-0.0253028684857489,-0.0126513116569664,
-1.46742496279217E-9),.UNSPECIFIED.);
#23401=B_SPLINE_CURVE_WITH_KNOTS('',3,(#144397,#144398,#144399,#144400,
#144401,#144402),.UNSPECIFIED.,.F.,.F.,(4,2,4),(-0.0253028680664795,-0.0126513116285446,
-1.47392072158414E-9),.UNSPECIFIED.);
#23402=B_SPLINE_CURVE_WITH_KNOTS('',3,(#144418,#144419,#144420,#144421,
#144422,#144423),.UNSPECIFIED.,.F.,.F.,(4,2,4),(-0.0253028674744424,-0.0126513116179339,
-1.4976289791635E-9),.UNSPECIFIED.);
#23403=B_SPLINE_CURVE_WITH_KNOTS('',3,(#144439,#144440,#144441,#144442,
#144443,#144444),.UNSPECIFIED.,.F.,.F.,(4,2,4),(-0.0253028608153995,-0.012651311643751,
-1.49117444087077E-9),.UNSPECIFIED.);
#23404=B_SPLINE_CURVE_WITH_KNOTS('',3,(#144460,#144461,#144462,#144463,
#144464,#144465),.UNSPECIFIED.,.F.,.F.,(4,2,4),(-0.0253028688025471,-0.012651311694285,
-1.5592264354658E-9),.UNSPECIFIED.);
#23405=B_SPLINE_CURVE_WITH_KNOTS('',3,(#144481,#144482,#144483,#144484,
#144485,#144486),.UNSPECIFIED.,.F.,.F.,(4,2,4),(-0.0253028685614985,-0.0126513116925499,
-1.51033512779675E-9),.UNSPECIFIED.);
#23406=B_SPLINE_CURVE_WITH_KNOTS('',3,(#144502,#144503,#144504,#144505,
#144506,#144507),.UNSPECIFIED.,.F.,.F.,(4,2,4),(-0.0253028684579291,-0.0126513116076864,
-1.46460564856565E-9),.UNSPECIFIED.);
#23407=B_SPLINE_CURVE_WITH_KNOTS('',3,(#144523,#144524,#144525,#144526,
#144527,#144528),.UNSPECIFIED.,.F.,.F.,(4,2,4),(-0.0253028607761515,-0.0126513116250043,
-1.47685470450187E-9),.UNSPECIFIED.);
#23408=B_SPLINE_CURVE_WITH_KNOTS('',3,(#144544,#144545,#144546,#144547,
#144548,#144549),.UNSPECIFIED.,.F.,.F.,(4,2,4),(-0.0253028685031401,-0.0126513115444502,
-1.40921434937935E-9),.UNSPECIFIED.);
#23409=B_SPLINE_CURVE_WITH_KNOTS('',3,(#144565,#144566,#144567,#144568,
#144569,#144570),.UNSPECIFIED.,.F.,.F.,(4,2,4),(-0.0253028690751082,-0.0126513117151343,
-1.54119479678361E-9),.UNSPECIFIED.);
#23410=B_SPLINE_CURVE_WITH_KNOTS('',3,(#144586,#144587,#144588,#144589,
#144590,#144591),.UNSPECIFIED.,.F.,.F.,(4,2,4),(-0.0253028693983055,-0.0126513115448918,
-1.40235656073684E-9),.UNSPECIFIED.);
#23411=B_SPLINE_CURVE_WITH_KNOTS('',3,(#144607,#144608,#144609,#144610,
#144611,#144612),.UNSPECIFIED.,.F.,.F.,(4,2,4),(-0.0253028676030852,-0.0126513117658921,
-1.59613115432999E-9),.UNSPECIFIED.);
#23412=B_SPLINE_CURVE_WITH_KNOTS('',3,(#144628,#144629,#144630,#144631,
#144632,#144633),.UNSPECIFIED.,.F.,.F.,(4,2,4),(-0.0253028678921412,-0.0126513117315833,
-1.53634311175765E-9),.UNSPECIFIED.);
#23413=B_SPLINE_CURVE_WITH_KNOTS('',3,(#144649,#144650,#144651,#144652,
#144653,#144654),.UNSPECIFIED.,.F.,.F.,(4,2,4),(-0.0253028607407018,-0.0126513115927762,
-1.45961178560361E-9),.UNSPECIFIED.);
#23414=B_SPLINE_CURVE_WITH_KNOTS('',3,(#144670,#144671,#144672,#144673,
#144674,#144675),.UNSPECIFIED.,.F.,.F.,(4,2,4),(-0.0253028677288099,-0.0126513116203026,
-1.49586819667147E-9),.UNSPECIFIED.);
#23415=B_SPLINE_CURVE_WITH_KNOTS('',3,(#144691,#144692,#144693,#144694,
#144695,#144696),.UNSPECIFIED.,.F.,.F.,(4,2,4),(-0.0253028677262056,-0.0126513116265939,
-1.50229979151151E-9),.UNSPECIFIED.);
#23416=B_SPLINE_CURVE_WITH_KNOTS('',3,(#144712,#144713,#144714,#144715,
#144716,#144717),.UNSPECIFIED.,.F.,.F.,(4,2,4),(-0.0253028607760877,-0.0126513115295272,
-1.38452104295195E-9),.UNSPECIFIED.);
#23417=B_SPLINE_CURVE_WITH_KNOTS('',3,(#144733,#144734,#144735,#144736,
#144737,#144738),.UNSPECIFIED.,.F.,.F.,(4,2,4),(-0.0253028684626624,-0.012651311551332,
-1.42760715055035E-9),.UNSPECIFIED.);
#23418=B_SPLINE_CURVE_WITH_KNOTS('',3,(#144754,#144755,#144756,#144757,
#144758,#144759),.UNSPECIFIED.,.F.,.F.,(4,2,4),(-0.0253028607935486,-0.0126513115878577,
-1.42838934777401E-9),.UNSPECIFIED.);
#23419=B_SPLINE_CURVE_WITH_KNOTS('',3,(#144775,#144776,#144777,#144778,
#144779,#144780),.UNSPECIFIED.,.F.,.F.,(4,2,4),(-0.0253028607669744,-0.0126513116157709,
-1.47254117580098E-9),.UNSPECIFIED.);
#23420=B_SPLINE_CURVE_WITH_KNOTS('',3,(#144796,#144797,#144798,#144799,
#144800,#144801),.UNSPECIFIED.,.F.,.F.,(4,2,4),(-0.0253028683470321,-0.0126513117988463,
-1.62334940975728E-9),.UNSPECIFIED.);
#23421=B_SPLINE_CURVE_WITH_KNOTS('',3,(#144817,#144818,#144819,#144820,
#144821,#144822),.UNSPECIFIED.,.F.,.F.,(4,2,4),(-0.0253028608496447,-0.0126513116279292,
-1.4460164489416E-9),.UNSPECIFIED.);
#23422=B_SPLINE_CURVE_WITH_KNOTS('',3,(#144840,#144841,#144842,#144843,
#144844,#144845),.UNSPECIFIED.,.F.,.F.,(4,2,4),(-0.0253042129381971,-0.0126519919856879,
0.),.UNSPECIFIED.);
#23423=B_SPLINE_CURVE_WITH_KNOTS('',3,(#144855,#144856,#144857,#144858,
#144859,#144860),.UNSPECIFIED.,.F.,.F.,(4,2,4),(0.,0.0126519843067729,0.0253041804503512),
 .UNSPECIFIED.);
#23424=B_SPLINE_CURVE_WITH_KNOTS('',3,(#144884,#144885,#144886,#144887,
#144888,#144889),.UNSPECIFIED.,.F.,.F.,(4,2,4),(0.,0.0126519865865287,0.0253041900617945),
 .UNSPECIFIED.);
#23425=B_SPLINE_CURVE_WITH_KNOTS('',3,(#144913,#144914,#144915,#144916,
#144917,#144918),.UNSPECIFIED.,.F.,.F.,(4,2,4),(0.,0.0126519847777877,0.0253041824957834),
 .UNSPECIFIED.);
#23426=B_SPLINE_CURVE_WITH_KNOTS('',3,(#144942,#144943,#144944,#144945,
#144946,#144947),.UNSPECIFIED.,.F.,.F.,(4,2,4),(0.,0.0126519869389596,0.025304191433575),
 .UNSPECIFIED.);
#23427=B_SPLINE_CURVE_WITH_KNOTS('',3,(#144971,#144972,#144973,#144974,
#144975,#144976),.UNSPECIFIED.,.F.,.F.,(4,2,4),(0.,0.0126519849592999,0.025304183155069),
 .UNSPECIFIED.);
#23428=B_SPLINE_CURVE_WITH_KNOTS('',3,(#145000,#145001,#145002,#145003,
#145004,#145005),.UNSPECIFIED.,.F.,.F.,(4,2,4),(0.,0.0126519878879565,0.0253041955637346),
 .UNSPECIFIED.);
#23429=B_SPLINE_CURVE_WITH_KNOTS('',3,(#145026,#145027,#145028,#145029,
#145030,#145031),.UNSPECIFIED.,.F.,.F.,(4,2,4),(0.,0.0126519870093447,0.025304191879591),
 .UNSPECIFIED.);
#23430=B_SPLINE_CURVE_WITH_KNOTS('',3,(#145049,#145050,#145051,#145052,
#145053,#145054),.UNSPECIFIED.,.F.,.F.,(4,2,4),(0.,0.012651986717139,0.0253041906799449),
 .UNSPECIFIED.);
#23431=B_SPLINE_CURVE_WITH_KNOTS('',3,(#145078,#145079,#145080,#145081,
#145082,#145083),.UNSPECIFIED.,.F.,.F.,(4,2,4),(0.,0.0126519873096693,0.0253041931288259),
 .UNSPECIFIED.);
#23432=B_SPLINE_CURVE_WITH_KNOTS('',3,(#145107,#145108,#145109,#145110,
#145111,#145112),.UNSPECIFIED.,.F.,.F.,(4,2,4),(0.,0.0126519870612146,0.0253041921126481),
 .UNSPECIFIED.);
#23433=B_SPLINE_CURVE_WITH_KNOTS('',3,(#145136,#145137,#145138,#145139,
#145140,#145141),.UNSPECIFIED.,.F.,.F.,(4,2,4),(0.,0.0126519852924514,0.0253041846331273),
 .UNSPECIFIED.);
#23434=B_SPLINE_CURVE_WITH_KNOTS('',3,(#145165,#145166,#145167,#145168,
#145169,#145170),.UNSPECIFIED.,.F.,.F.,(4,2,4),(0.,0.0126519848460903,0.0253041826856367),
 .UNSPECIFIED.);
#23435=B_SPLINE_CURVE_WITH_KNOTS('',3,(#145194,#145195,#145196,#145197,
#145198,#145199),.UNSPECIFIED.,.F.,.F.,(4,2,4),(0.,0.0126519867876667,0.0253041908553758),
 .UNSPECIFIED.);
#23436=B_SPLINE_CURVE_WITH_KNOTS('',3,(#145223,#145224,#145225,#145226,
#145227,#145228),.UNSPECIFIED.,.F.,.F.,(4,2,4),(0.,0.0126519854542322,0.0253041852847222),
 .UNSPECIFIED.);
#23437=B_SPLINE_CURVE_WITH_KNOTS('',3,(#145252,#145253,#145254,#145255,
#145256,#145257),.UNSPECIFIED.,.F.,.F.,(4,2,4),(0.,0.0126519862176949,0.0253041884552269),
 .UNSPECIFIED.);
#23438=B_SPLINE_CURVE_WITH_KNOTS('',3,(#145281,#145282,#145283,#145284,
#145285,#145286),.UNSPECIFIED.,.F.,.F.,(4,2,4),(0.,0.0126519862606805,0.0253041886986062),
 .UNSPECIFIED.);
#23439=B_SPLINE_CURVE_WITH_KNOTS('',3,(#145310,#145311,#145312,#145313,
#145314,#145315),.UNSPECIFIED.,.F.,.F.,(4,2,4),(0.,0.0126519848133697,0.0253041826121683),
 .UNSPECIFIED.);
#23440=B_SPLINE_CURVE_WITH_KNOTS('',3,(#145339,#145340,#145341,#145342,
#145343,#145344),.UNSPECIFIED.,.F.,.F.,(4,2,4),(0.,0.0126519847288218,0.0253041821993781),
 .UNSPECIFIED.);
#23441=B_SPLINE_CURVE_WITH_KNOTS('',3,(#145368,#145369,#145370,#145371,
#145372,#145373),.UNSPECIFIED.,.F.,.F.,(4,2,4),(0.,0.0126519871577642,0.0253041925457795),
 .UNSPECIFIED.);
#23442=B_SPLINE_CURVE_WITH_KNOTS('',3,(#145398,#145399,#145400,#145401,
#145402,#145403),.UNSPECIFIED.,.F.,.F.,(4,2,4),(0.,0.0126519875408859,0.0253041941268785),
 .UNSPECIFIED.);
#23443=B_SPLINE_CURVE_WITH_KNOTS('',3,(#145426,#145427,#145428,#145429,
#145430,#145431),.UNSPECIFIED.,.F.,.F.,(4,2,4),(0.,0.0126519862827976,0.0253041887203517),
 .UNSPECIFIED.);
#23444=B_SPLINE_CURVE_WITH_KNOTS('',3,(#145455,#145456,#145457,#145458,
#145459,#145460),.UNSPECIFIED.,.F.,.F.,(4,2,4),(0.,0.012651985852953,0.0253041869280763),
 .UNSPECIFIED.);
#23445=B_SPLINE_CURVE_WITH_KNOTS('',3,(#145484,#145485,#145486,#145487,
#145488,#145489),.UNSPECIFIED.,.F.,.F.,(4,2,4),(0.,0.0126519861145527,0.0253041880659203),
 .UNSPECIFIED.);
#23446=B_SPLINE_CURVE_WITH_KNOTS('',3,(#145513,#145514,#145515,#145516,
#145517,#145518),.UNSPECIFIED.,.F.,.F.,(4,2,4),(0.,0.0126519863202011,0.0253041888160825),
 .UNSPECIFIED.);
#23447=B_SPLINE_CURVE_WITH_KNOTS('',3,(#145542,#145543,#145544,#145545,
#145546,#145547),.UNSPECIFIED.,.F.,.F.,(4,2,4),(0.,0.0126519859054325,0.0253041871291788),
 .UNSPECIFIED.);
#23448=B_SPLINE_CURVE_WITH_KNOTS('',3,(#145571,#145572,#145573,#145574,
#145575,#145576),.UNSPECIFIED.,.F.,.F.,(4,2,4),(0.,0.0126519835229689,0.0253041772181617),
 .UNSPECIFIED.);
#23449=B_SPLINE_CURVE_WITH_KNOTS('',3,(#145600,#145601,#145602,#145603,
#145604,#145605),.UNSPECIFIED.,.F.,.F.,(4,2,4),(0.,0.0126519864390143,0.0253041893892579),
 .UNSPECIFIED.);
#23450=B_SPLINE_CURVE_WITH_KNOTS('',3,(#145629,#145630,#145631,#145632,
#145633,#145634),.UNSPECIFIED.,.F.,.F.,(4,2,4),(0.,0.0126519858357069,0.025304186822954),
 .UNSPECIFIED.);
#23451=B_SPLINE_CURVE_WITH_KNOTS('',3,(#145669,#145670,#145671,#145672,
#145673,#145674),.UNSPECIFIED.,.F.,.F.,(4,2,4),(-0.0252989398056719,-0.0126493213074638,
0.),.UNSPECIFIED.);
#23452=B_SPLINE_CURVE_WITH_KNOTS('',3,(#145692,#145693,#145694,#145695,
#145696,#145697),.UNSPECIFIED.,.F.,.F.,(4,2,4),(0.,0.012649316395125,0.0252988129119735),
 .UNSPECIFIED.);
#23453=B_SPLINE_CURVE_WITH_KNOTS('',3,(#145725,#145726,#145727,#145728,
#145729,#145730),.UNSPECIFIED.,.F.,.F.,(4,2,4),(0.,0.0126493159533226,0.0252988074100563),
 .UNSPECIFIED.);
#23454=B_SPLINE_CURVE_WITH_KNOTS('',3,(#145758,#145759,#145760,#145761,
#145762,#145763),.UNSPECIFIED.,.F.,.F.,(4,2,4),(0.,0.012649321310377,0.0252988283293789),
 .UNSPECIFIED.);
#23455=B_SPLINE_CURVE_WITH_KNOTS('',3,(#145791,#145792,#145793,#145794,
#145795,#145796),.UNSPECIFIED.,.F.,.F.,(4,2,4),(0.,0.0126493158064216,0.0252988080156246),
 .UNSPECIFIED.);
#23456=B_SPLINE_CURVE_WITH_KNOTS('',3,(#145824,#145825,#145826,#145827,
#145828,#145829),.UNSPECIFIED.,.F.,.F.,(4,2,4),(0.,0.0126493154719441,0.0252988076384874),
 .UNSPECIFIED.);
#23457=B_SPLINE_CURVE_WITH_KNOTS('',3,(#145857,#145858,#145859,#145860,
#145861,#145862),.UNSPECIFIED.,.F.,.F.,(4,2,4),(0.,0.0126493163036998,0.0252988096871266),
 .UNSPECIFIED.);
#23458=B_SPLINE_CURVE_WITH_KNOTS('',3,(#145890,#145891,#145892,#145893,
#145894,#145895),.UNSPECIFIED.,.F.,.F.,(4,2,4),(0.,0.0126493213088601,0.0252988339968301),
 .UNSPECIFIED.);
#23459=B_SPLINE_CURVE_WITH_KNOTS('',3,(#145923,#145924,#145925,#145926,
#145927,#145928),.UNSPECIFIED.,.F.,.F.,(4,2,4),(0.,0.0126493212450843,0.0252988321670426),
 .UNSPECIFIED.);
#23460=B_SPLINE_CURVE_WITH_KNOTS('',3,(#145956,#145957,#145958,#145959,
#145960,#145961),.UNSPECIFIED.,.F.,.F.,(4,2,4),(0.,0.0126493164888677,0.0252988100939839),
 .UNSPECIFIED.);
#23461=B_SPLINE_CURVE_WITH_KNOTS('',3,(#145989,#145990,#145991,#145992,
#145993,#145994),.UNSPECIFIED.,.F.,.F.,(4,2,4),(0.,0.0126493167066686,0.0252988109105679),
 .UNSPECIFIED.);
#23462=B_SPLINE_CURVE_WITH_KNOTS('',3,(#146022,#146023,#146024,#146025,
#146026,#146027),.UNSPECIFIED.,.F.,.F.,(4,2,4),(0.,0.0126493212346032,0.025298829133827),
 .UNSPECIFIED.);
#23463=B_SPLINE_CURVE_WITH_KNOTS('',3,(#146055,#146056,#146057,#146058,
#146059,#146060),.UNSPECIFIED.,.F.,.F.,(4,2,4),(0.,0.0126493159995195,0.0252988104878458),
 .UNSPECIFIED.);
#23464=B_SPLINE_CURVE_WITH_KNOTS('',3,(#146088,#146089,#146090,#146091,
#146092,#146093),.UNSPECIFIED.,.F.,.F.,(4,2,4),(0.,0.0126493213102731,0.0252988320787696),
 .UNSPECIFIED.);
#23465=B_SPLINE_CURVE_WITH_KNOTS('',3,(#146118,#146119,#146120,#146121,
#146122,#146123),.UNSPECIFIED.,.F.,.F.,(4,2,4),(0.,0.0126493213088555,0.0252988287166666),
 .UNSPECIFIED.);
#23466=B_SPLINE_CURVE_WITH_KNOTS('',3,(#146145,#146146,#146147,#146148,
#146149,#146150),.UNSPECIFIED.,.F.,.F.,(4,2,4),(0.,0.0126493211988361,0.0252988317094231),
 .UNSPECIFIED.);
#23467=B_SPLINE_CURVE_WITH_KNOTS('',3,(#146178,#146179,#146180,#146181,
#146182,#146183),.UNSPECIFIED.,.F.,.F.,(4,2,4),(0.,0.012649321215418,0.0252988292224408),
 .UNSPECIFIED.);
#23468=B_SPLINE_CURVE_WITH_KNOTS('',3,(#146211,#146212,#146213,#146214,
#146215,#146216),.UNSPECIFIED.,.F.,.F.,(4,2,4),(0.,0.0126493160353129,0.0252988086035777),
 .UNSPECIFIED.);
#23469=B_SPLINE_CURVE_WITH_KNOTS('',3,(#146244,#146245,#146246,#146247,
#146248,#146249),.UNSPECIFIED.,.F.,.F.,(4,2,4),(0.,0.0126493212877845,0.0252988315664183),
 .UNSPECIFIED.);
#23470=B_SPLINE_CURVE_WITH_KNOTS('',3,(#146277,#146278,#146279,#146280,
#146281,#146282),.UNSPECIFIED.,.F.,.F.,(4,2,4),(0.,0.0126493212849581,0.0252988352832389),
 .UNSPECIFIED.);
#23471=B_SPLINE_CURVE_WITH_KNOTS('',3,(#146310,#146311,#146312,#146313,
#146314,#146315),.UNSPECIFIED.,.F.,.F.,(4,2,4),(0.,0.012649316194881,0.0252988129351232),
 .UNSPECIFIED.);
#23472=B_SPLINE_CURVE_WITH_KNOTS('',3,(#146343,#146344,#146345,#146346,
#146347,#146348),.UNSPECIFIED.,.F.,.F.,(4,2,4),(0.,0.0126493167128799,0.025298817624995),
 .UNSPECIFIED.);
#23473=B_SPLINE_CURVE_WITH_KNOTS('',3,(#146376,#146377,#146378,#146379,
#146380,#146381),.UNSPECIFIED.,.F.,.F.,(4,2,4),(0.,0.0126493213076427,0.0252988335485302),
 .UNSPECIFIED.);
#23474=B_SPLINE_CURVE_WITH_KNOTS('',3,(#146409,#146410,#146411,#146412,
#146413,#146414),.UNSPECIFIED.,.F.,.F.,(4,2,4),(0.,0.0126493213070669,0.025298828284289),
 .UNSPECIFIED.);
#23475=B_SPLINE_CURVE_WITH_KNOTS('',3,(#146442,#146443,#146444,#146445,
#146446,#146447),.UNSPECIFIED.,.F.,.F.,(4,2,4),(0.,0.0126493165134168,0.0252988152984364),
 .UNSPECIFIED.);
#23476=B_SPLINE_CURVE_WITH_KNOTS('',3,(#146475,#146476,#146477,#146478,
#146479,#146480),.UNSPECIFIED.,.F.,.F.,(4,2,4),(0.,0.0126493159700643,0.025298809661145),
 .UNSPECIFIED.);
#23477=B_SPLINE_CURVE_WITH_KNOTS('',3,(#146508,#146509,#146510,#146511,
#146512,#146513),.UNSPECIFIED.,.F.,.F.,(4,2,4),(0.,0.0126493213142762,0.0252988279997388),
 .UNSPECIFIED.);
#23478=B_SPLINE_CURVE_WITH_KNOTS('',3,(#146541,#146542,#146543,#146544,
#146545,#146546),.UNSPECIFIED.,.F.,.F.,(4,2,4),(0.,0.0126493162481951,0.0252988083212156),
 .UNSPECIFIED.);
#23479=B_SPLINE_CURVE_WITH_KNOTS('',3,(#146574,#146575,#146576,#146577,
#146578,#146579),.UNSPECIFIED.,.F.,.F.,(4,2,4),(0.,0.0126493163255192,0.0252988106377532),
 .UNSPECIFIED.);
#23480=B_SPLINE_CURVE_WITH_KNOTS('',3,(#146622,#146623,#146624,#146625,
#146626,#146627,#146628,#146629,#146630,#146631,#146632,#146633,#146634),
 .UNSPECIFIED.,.F.,.F.,(4,3,3,3,4),(0.,8.70610642392342E-5,0.00010313475499915,
0.000170041092769086,0.000253022912732791),.UNSPECIFIED.);
#23481=B_SPLINE_CURVE_WITH_KNOTS('',3,(#146650,#146651,#146652,#146653,
#146654,#146655,#146656,#146657,#146658,#146659),.UNSPECIFIED.,.F.,.F.,
(4,3,3,4),(0.556108173894251,0.558333952657053,0.568139465476172,0.573549700889344),
 .UNSPECIFIED.);
#23482=B_SPLINE_CURVE_WITH_KNOTS('',3,(#146660,#146661,#146662,#146663,
#146664,#146665,#146666,#146667,#146668,#146669),.UNSPECIFIED.,.F.,.F.,
(4,3,3,4),(1.69231154865856E-13,8.70609204190528E-5,0.000170040985661312,
0.000253023205846536),.UNSPECIFIED.);
#23483=B_SPLINE_CURVE_WITH_KNOTS('',3,(#146701,#146702,#146703,#146704,
#146705,#146706,#146707,#146708,#146709,#146710),.UNSPECIFIED.,.F.,.F.,
(4,3,3,4),(1.54680663374548E-13,8.70609205558343E-5,0.000170040985841156,
0.000253023206069013),.UNSPECIFIED.);
#23484=B_SPLINE_CURVE_WITH_KNOTS('',3,(#146737,#146738,#146739,#146740,
#146741,#146742,#146743,#146744,#146745,#146746,#146747,#146748,#146749,
#146750),.UNSPECIFIED.,.F.,.F.,(4,2,2,2,2,2,4),(3.17115822501972E-10,0.0399756457172238,
0.0600249637123924,0.0700670077817768,0.0750919619185494,0.0776053703943144,
0.080004019688016),.UNSPECIFIED.);
#23485=B_SPLINE_CURVE_WITH_KNOTS('',3,(#146751,#146752,#146753,#146754,
#146755,#146756,#146757,#146758,#146759,#146760),.UNSPECIFIED.,.F.,.F.,
(4,3,3,4),(1.61821296805164E-13,8.70609204750516E-5,0.000170040985668408,
0.000253023205803955),.UNSPECIFIED.);
#23486=B_SPLINE_CURVE_WITH_KNOTS('',3,(#146792,#146793,#146794,#146795,
#146796,#146797,#146798,#146799,#146800,#146801),.UNSPECIFIED.,.F.,.F.,
(4,3,3,4),(1.8179717827368E-13,8.70609204854375E-5,0.000170040985755457,
0.000253023205969049),.UNSPECIFIED.);
#23487=B_SPLINE_CURVE_WITH_KNOTS('',3,(#146833,#146834,#146835,#146836,
#146837,#146838,#146839,#146840,#146841,#146842),.UNSPECIFIED.,.F.,.F.,
(4,3,3,4),(1.82791368656842E-13,8.70609205854241E-5,0.000170040985761326,
0.000253023205880162),.UNSPECIFIED.);
#23488=B_SPLINE_CURVE_WITH_KNOTS('',3,(#146869,#146870,#146871,#146872,
#146873,#146874,#146875,#146876,#146877,#146878,#146879,#146880,#146881,
#146882),.UNSPECIFIED.,.F.,.F.,(4,2,2,2,2,2,4),(3.25736694958069E-10,0.0399756350505435,
0.060024947723225,0.070066996420522,0.0750919528708576,0.0776053625034702,
0.0800040128963778),.UNSPECIFIED.);
#23489=B_SPLINE_CURVE_WITH_KNOTS('',3,(#146883,#146884,#146885,#146886,
#146887,#146888,#146889,#146890,#146891,#146892),.UNSPECIFIED.,.F.,.F.,
(4,3,3,4),(9.38154535606092E-14,8.70609207349159E-5,0.00017004098588965,
0.000253023205987876),.UNSPECIFIED.);
#23490=B_SPLINE_CURVE_WITH_KNOTS('',3,(#146919,#146920,#146921,#146922,
#146923,#146924,#146925,#146926,#146927,#146928,#146929,#146930,#146931,
#146932),.UNSPECIFIED.,.F.,.F.,(4,2,2,2,2,2,4),(3.42543828201874E-10,0.0399756356949133,
0.0600249478091022,0.0700669878091456,0.0750919399147613,0.077605347375955,
0.0800039956845119),.UNSPECIFIED.);
#23491=B_SPLINE_CURVE_WITH_KNOTS('',3,(#146933,#146934,#146935,#146936,
#146937,#146938,#146939,#146940,#146941,#146942),.UNSPECIFIED.,.F.,.F.,
(4,3,3,4),(9.32267848327091E-14,8.70609204372164E-5,0.000170040985887543,
0.000253023206279809),.UNSPECIFIED.);
#23492=B_SPLINE_CURVE_WITH_KNOTS('',3,(#146969,#146970,#146971,#146972,
#146973,#146974,#146975,#146976,#146977,#146978),.UNSPECIFIED.,.F.,.F.,
(4,3,3,4),(0.556108173897008,0.558333952657056,0.568139434940753,0.57354970089104),
 .UNSPECIFIED.);
#23493=B_SPLINE_CURVE_WITH_KNOTS('',3,(#146979,#146980,#146981,#146982,
#146983,#146984,#146985,#146986,#146987,#146988,#146989,#146990,#146991),
 .UNSPECIFIED.,.F.,.F.,(4,3,3,3,4),(2.17783596318746E-13,8.70609204643982E-5,
0.000149888113335004,0.000170040985596686,0.000253023205671698),
 .UNSPECIFIED.);
#23494=B_SPLINE_CURVE_WITH_KNOTS('',3,(#147018,#147019,#147020,#147021,
#147022,#147023,#147024,#147025,#147026,#147027),.UNSPECIFIED.,.F.,.F.,
(4,3,3,4),(0.556108173865716,0.558333952657056,0.568139432990237,0.573549700892214),
 .UNSPECIFIED.);
#23495=B_SPLINE_CURVE_WITH_KNOTS('',3,(#147028,#147029,#147030,#147031,
#147032,#147033,#147034,#147035,#147036,#147037,#147038,#147039,#147040),
 .UNSPECIFIED.,.F.,.F.,(4,3,3,3,4),(8.71190282254634E-14,8.70609204912651E-5,
0.000149888113153294,0.000170040985908022,0.000253023206266396),
 .UNSPECIFIED.);
#23496=B_SPLINE_CURVE_WITH_KNOTS('',3,(#147067,#147068,#147069,#147070,
#147071,#147072,#147073,#147074,#147075,#147076,#147077,#147078,#147079,
#147080),.UNSPECIFIED.,.F.,.F.,(4,2,2,2,2,2,4),(2.72062316739559E-10,0.0399756540412885,
0.0600249697811288,0.0700669995408656,0.075091946519025,0.0776053514146817,
0.080003997248157),.UNSPECIFIED.);
#23497=B_SPLINE_CURVE_WITH_KNOTS('',3,(#147081,#147082,#147083,#147084,
#147085,#147086,#147087,#147088,#147089,#147090),.UNSPECIFIED.,.F.,.F.,
(4,3,3,4),(1.96283630672745E-13,8.7060920517827E-5,0.000170040985827293,
0.000253023206080021),.UNSPECIFIED.);
#23498=B_SPLINE_CURVE_WITH_KNOTS('',3,(#147122,#147123,#147124,#147125,
#147126,#147127,#147128,#147129,#147130,#147131),.UNSPECIFIED.,.F.,.F.,
(4,3,3,4),(1.38795067579082E-13,8.7060920468453E-5,0.000170040985661875,
0.000253023205798495),.UNSPECIFIED.);
#23499=B_SPLINE_CURVE_WITH_KNOTS('',3,(#147158,#147159,#147160,#147161,
#147162,#147163,#147164,#147165,#147166,#147167,#147168,#147169,#147170,
#147171),.UNSPECIFIED.,.F.,.F.,(4,2,2,2,2,2,4),(2.7352003332601E-10,0.0399756335387596,
0.0600249433548185,0.0700669840178637,0.0750919364533658,0.0776053440791422,
0.0800039925289707),.UNSPECIFIED.);
#23500=B_SPLINE_CURVE_WITH_KNOTS('',3,(#147172,#147173,#147174,#147175,
#147176,#147177,#147178,#147179,#147180,#147181),.UNSPECIFIED.,.F.,.F.,
(4,3,3,4),(2.56474145581824E-13,8.70609204134192E-5,0.000170040985667171,
0.000253023205863517),.UNSPECIFIED.);
#23501=B_SPLINE_CURVE_WITH_KNOTS('',3,(#147213,#147214,#147215,#147216,
#147217,#147218,#147219,#147220,#147221,#147222,#147223,#147224,#147225),
 .UNSPECIFIED.,.F.,.F.,(4,3,3,3,4),(1.72563598568684E-13,8.70609205411575E-5,
0.00014988811322632,0.000170040985712443,0.00025302320582707),
 .UNSPECIFIED.);
#23502=B_SPLINE_CURVE_WITH_KNOTS('',3,(#147252,#147253,#147254,#147255,
#147256,#147257,#147258,#147259,#147260,#147261),.UNSPECIFIED.,.F.,.F.,
(4,3,3,4),(0.556108173930173,0.558333952657056,0.568139440253929,0.573549700889268),
 .UNSPECIFIED.);
#23503=B_SPLINE_CURVE_WITH_KNOTS('',3,(#147262,#147263,#147264,#147265,
#147266,#147267,#147268,#147269,#147270,#147271),.UNSPECIFIED.,.F.,.F.,
(4,3,3,4),(9.95524747780889E-14,8.70609207631359E-5,0.000170040985962216,
0.000253023206105423),.UNSPECIFIED.);
#23504=B_SPLINE_CURVE_WITH_KNOTS('',3,(#147298,#147299,#147300,#147301,
#147302,#147303,#147304,#147305,#147306,#147307,#147308,#147309,#147310,
#147311),.UNSPECIFIED.,.F.,.F.,(4,2,2,2,2,2,4),(2.08407129104266E-10,0.0399756526762724,
0.0600249688922645,0.0700670003688512,0.0750919482058424,0.0776053535310304,
0.0800039998029628),.UNSPECIFIED.);
#23505=B_SPLINE_CURVE_WITH_KNOTS('',3,(#147312,#147313,#147314,#147315,
#147316,#147317,#147318,#147319,#147320,#147321),.UNSPECIFIED.,.F.,.F.,
(4,3,3,4),(1.10306306544097E-13,8.70609205778296E-5,0.00017004098578854,
0.000253023205942734),.UNSPECIFIED.);
#23506=B_SPLINE_CURVE_WITH_KNOTS('',3,(#147348,#147349,#147350,#147351,
#147352,#147353,#147354,#147355,#147356,#147357),.UNSPECIFIED.,.F.,.F.,
(4,3,3,4),(0.556108173910857,0.558333952657056,0.568139440135517,0.573549700893365),
 .UNSPECIFIED.);
#23507=B_SPLINE_CURVE_WITH_KNOTS('',3,(#147358,#147359,#147360,#147361,
#147362,#147363,#147364,#147365,#147366,#147367),.UNSPECIFIED.,.F.,.F.,
(4,3,3,4),(2.24448260341437E-13,8.70609204346609E-5,0.000170040985496222,
0.000253023205500031),.UNSPECIFIED.);
#23508=B_SPLINE_CURVE_WITH_KNOTS('',3,(#147399,#147400,#147401,#147402,
#147403,#147404,#147405,#147406,#147407,#147408),.UNSPECIFIED.,.F.,.F.,
(4,3,3,4),(1.55289471312465E-13,8.70609206640267E-5,0.000170040985730055,
0.00025302320573868),.UNSPECIFIED.);
#23509=B_SPLINE_CURVE_WITH_KNOTS('',3,(#147435,#147436,#147437,#147438,
#147439,#147440,#147441,#147442,#147443,#147444),.UNSPECIFIED.,.F.,.F.,
(4,3,3,4),(0.556108173913933,0.558333952657056,0.568139463253051,0.573549700879883),
 .UNSPECIFIED.);
#23510=B_SPLINE_CURVE_WITH_KNOTS('',3,(#147445,#147446,#147447,#147448,
#147449,#147450,#147451,#147452,#147453,#147454),.UNSPECIFIED.,.F.,.F.,
(4,3,3,4),(8.75431270138763E-14,8.70609204120076E-5,0.000170040985741647,
0.000253023206012933),.UNSPECIFIED.);
#23511=B_SPLINE_CURVE_WITH_KNOTS('',3,(#147481,#147482,#147483,#147484,
#147485,#147486,#147487,#147488,#147489,#147490,#147491,#147492,#147493,
#147494),.UNSPECIFIED.,.F.,.F.,(4,2,2,2,2,2,4),(2.99556102725697E-10,0.0399756352567531,
0.0600249465583133,0.070066989855618,0.0750919436067488,0.0776053518899977,
0.0800040009606207),.UNSPECIFIED.);
#23512=B_SPLINE_CURVE_WITH_KNOTS('',3,(#147495,#147496,#147497,#147498,
#147499,#147500,#147501,#147502,#147503,#147504),.UNSPECIFIED.,.F.,.F.,
(4,3,3,4),(2.11907265441818E-13,8.70609206450316E-5,0.000170040985681721,
0.000253023205661128),.UNSPECIFIED.);
#23513=B_SPLINE_CURVE_WITH_KNOTS('',3,(#147531,#147532,#147533,#147534,
#147535,#147536,#147537,#147538,#147539,#147540),.UNSPECIFIED.,.F.,.F.,
(4,3,3,4),(0.556108173921688,0.558333952657057,0.568139461882756,0.573549700889244),
 .UNSPECIFIED.);
#23514=B_SPLINE_CURVE_WITH_KNOTS('',3,(#147541,#147542,#147543,#147544,
#147545,#147546,#147547,#147548,#147549,#147550),.UNSPECIFIED.,.F.,.F.,
(4,3,3,4),(1.37524544768384E-13,8.70609205860296E-5,0.000170040985872499,
0.000253023206102047),.UNSPECIFIED.);
#23515=B_SPLINE_CURVE_WITH_KNOTS('',3,(#147577,#147578,#147579,#147580,
#147581,#147582,#147583,#147584,#147585,#147586),.UNSPECIFIED.,.F.,.F.,
(4,3,3,4),(0.556108173920208,0.558333952657064,0.568139457501484,0.573549700896862),
 .UNSPECIFIED.);
#23516=B_SPLINE_CURVE_WITH_KNOTS('',3,(#147587,#147588,#147589,#147590,
#147591,#147592,#147593,#147594,#147595,#147596),.UNSPECIFIED.,.F.,.F.,
(4,3,3,4),(1.71159403601284E-13,8.70609204517324E-5,0.000170040985610444,
0.000253023205711528),.UNSPECIFIED.);
#23517=B_SPLINE_CURVE_WITH_KNOTS('',3,(#147623,#147624,#147625,#147626,
#147627,#147628,#147629,#147630,#147631,#147632,#147633,#147634,#147635,
#147636),.UNSPECIFIED.,.F.,.F.,(4,2,2,2,2,2,4),(3.15293603599107E-10,0.0399756318238306,
0.0600249397363027,0.0700669805933937,0.075091933125416,0.0776053407993536,
0.0800039893127443),.UNSPECIFIED.);
#23518=B_SPLINE_CURVE_WITH_KNOTS('',3,(#147637,#147638,#147639,#147640,
#147641,#147642,#147643,#147644,#147645,#147646),.UNSPECIFIED.,.F.,.F.,
(4,3,3,4),(2.22592601224058E-13,8.70609204363956E-5,0.000170040985578146,
0.000253023205662112),.UNSPECIFIED.);
#23519=B_SPLINE_CURVE_WITH_KNOTS('',3,(#147673,#147674,#147675,#147676,
#147677,#147678,#147679,#147680,#147681,#147682),.UNSPECIFIED.,.F.,.F.,
(4,3,3,4),(0.556108173873244,0.558333952657066,0.568139478039504,0.573549700885696),
 .UNSPECIFIED.);
#23520=B_SPLINE_CURVE_WITH_KNOTS('',3,(#147683,#147684,#147685,#147686,
#147687,#147688,#147689,#147690,#147691,#147692),.UNSPECIFIED.,.F.,.F.,
(4,3,3,4),(1.86698732542565E-13,8.70609205947636E-5,0.000170040985794769,
0.000253023205936877),.UNSPECIFIED.);
#23521=B_SPLINE_CURVE_WITH_KNOTS('',3,(#147719,#147720,#147721,#147722,
#147723,#147724,#147725,#147726,#147727,#147728,#147729,#147730,#147731,
#147732),.UNSPECIFIED.,.F.,.F.,(4,2,2,2,2,2,4),(2.73861150635604E-10,0.0399756418181266,
0.0600249547070785,0.0700669927695654,0.0750919439059226,0.0776053508825574,
0.0800039986914438),.UNSPECIFIED.);
#23522=B_SPLINE_CURVE_WITH_KNOTS('',3,(#147733,#147734,#147735,#147736,
#147737,#147738,#147739,#147740,#147741,#147742),.UNSPECIFIED.,.F.,.F.,
(4,3,3,4),(1.25089518386443E-13,8.70609206928586E-5,0.000170040985933957,
0.000253023206117974),.UNSPECIFIED.);
#23523=B_SPLINE_CURVE_WITH_KNOTS('',3,(#147769,#147770,#147771,#147772,
#147773,#147774,#147775,#147776,#147777,#147778),.UNSPECIFIED.,.F.,.F.,
(4,3,3,4),(0.556108173902585,0.558333952657053,0.568139480300036,0.573549700888651),
 .UNSPECIFIED.);
#23524=B_SPLINE_CURVE_WITH_KNOTS('',3,(#147779,#147780,#147781,#147782,
#147783,#147784,#147785,#147786,#147787,#147788,#147789,#147790,#147791),
 .UNSPECIFIED.,.F.,.F.,(4,3,3,3,4),(9.56422294869686E-14,8.70609205457756E-5,
0.000149888113578247,0.00017004098589937,0.000253023206195566),
 .UNSPECIFIED.);
#23525=B_SPLINE_CURVE_WITH_KNOTS('',3,(#147818,#147819,#147820,#147821,
#147822,#147823,#147824,#147825,#147826,#147827,#147828,#147829,#147830,
#147831),.UNSPECIFIED.,.F.,.F.,(4,2,2,2,2,2,4),(2.38543663118769E-10,0.03997565913649,
0.0600249813095576,0.0700670156573217,0.0750919649363173,0.077605370984128,
0.0800040179180761),.UNSPECIFIED.);
#23526=B_SPLINE_CURVE_WITH_KNOTS('',3,(#147832,#147833,#147834,#147835,
#147836,#147837,#147838,#147839,#147840,#147841),.UNSPECIFIED.,.F.,.F.,
(4,3,3,4),(2.3455914248856E-13,8.70609204481195E-5,0.000170040985735005,
0.000253023205965325),.UNSPECIFIED.);
#23527=B_SPLINE_CURVE_WITH_KNOTS('',3,(#147868,#147869,#147870,#147871,
#147872,#147873,#147874,#147875,#147876,#147877),.UNSPECIFIED.,.F.,.F.,
(4,3,3,4),(0.556108173916858,0.558333952657053,0.5681394446842,0.57354970088037),
 .UNSPECIFIED.);
#23528=B_SPLINE_CURVE_WITH_KNOTS('',3,(#147878,#147879,#147880,#147881,
#147882,#147883,#147884,#147885,#147886,#147887),.UNSPECIFIED.,.F.,.F.,
(4,3,3,4),(1.57842903223202E-13,8.70609205573698E-5,0.000170040985736597,
0.000253023205859146),.UNSPECIFIED.);
#23529=B_SPLINE_CURVE_WITH_KNOTS('',3,(#147914,#147915,#147916,#147917,
#147918,#147919,#147920,#147921,#147922,#147923,#147924,#147925,#147926,
#147927),.UNSPECIFIED.,.F.,.F.,(4,2,2,2,2,2,4),(2.49802435109874E-10,0.0399756361689207,
0.0600249451800575,0.0700669820430787,0.0750919325770055,0.0776053392515876,
0.0800039867512925),.UNSPECIFIED.);
#23530=B_SPLINE_CURVE_WITH_KNOTS('',3,(#147928,#147929,#147930,#147931,
#147932,#147933,#147934,#147935,#147936,#147937),.UNSPECIFIED.,.F.,.F.,
(4,3,3,4),(2.27093858578823E-13,8.7060920387382E-5,0.000170040985638493,
0.000253023205833007),.UNSPECIFIED.);
#23531=B_SPLINE_CURVE_WITH_KNOTS('',3,(#147963,#147964,#147965,#147966,
#147967,#147968,#147969,#147970,#147971,#147972,#147973,#147974,#147975,
#147976),.UNSPECIFIED.,.F.,.F.,(4,2,2,2,2,2,4),(1.87595803499913E-10,0.0399756516265179,
0.0600249695553755,0.0700670019266469,0.0750919502131022,0.0776053557636566,
0.0800040022491232),.UNSPECIFIED.);
#23532=B_SPLINE_CURVE_WITH_KNOTS('',3,(#147984,#147985,#147986,#147987,
#147988,#147989),.UNSPECIFIED.,.F.,.F.,(4,2,4),(0.,0.0126518799230764,0.0253039866726396),
 .UNSPECIFIED.);
#23533=B_SPLINE_CURVE_WITH_KNOTS('',3,(#148003,#148004,#148005,#148006,
#148007,#148008),.UNSPECIFIED.,.F.,.F.,(4,2,4),(-0.0253039870735502,-0.0126518801554942,
-4.4945748511882E-11),.UNSPECIFIED.);
#23534=B_SPLINE_CURVE_WITH_KNOTS('',3,(#148028,#148029,#148030,#148031,
#148032,#148033),.UNSPECIFIED.,.F.,.F.,(4,2,4),(-0.025303988212384,-0.0126518801493775,
-6.78167313972189E-11),.UNSPECIFIED.);
#23535=B_SPLINE_CURVE_WITH_KNOTS('',3,(#148053,#148054,#148055,#148056,
#148057,#148058),.UNSPECIFIED.,.F.,.F.,(4,2,4),(-0.0253039877294629,-0.0126518801101943,
0.),.UNSPECIFIED.);
#23536=B_SPLINE_CURVE_WITH_KNOTS('',3,(#148078,#148079,#148080,#148081,
#148082,#148083),.UNSPECIFIED.,.F.,.F.,(4,2,4),(-0.0253039877142318,-0.0126518802515817,
-1.27645775893637E-10),.UNSPECIFIED.);
#23537=B_SPLINE_CURVE_WITH_KNOTS('',3,(#148103,#148104,#148105,#148106,
#148107,#148108),.UNSPECIFIED.,.F.,.F.,(4,2,4),(-0.0253039881409112,-0.012651880135877,
-6.53908663328373E-11),.UNSPECIFIED.);
#23538=B_SPLINE_CURVE_WITH_KNOTS('',3,(#148128,#148129,#148130,#148131,
#148132,#148133),.UNSPECIFIED.,.F.,.F.,(4,2,4),(-0.0253039874124978,-0.0126518802797077,
-1.45539209156498E-10),.UNSPECIFIED.);
#23539=B_SPLINE_CURVE_WITH_KNOTS('',3,(#148153,#148154,#148155,#148156,
#148157,#148158),.UNSPECIFIED.,.F.,.F.,(4,2,4),(-0.025303987819935,-0.0126518802163937,
-9.41260888676076E-11),.UNSPECIFIED.);
#23540=B_SPLINE_CURVE_WITH_KNOTS('',3,(#148178,#148179,#148180,#148181,
#148182,#148183),.UNSPECIFIED.,.F.,.F.,(4,2,4),(-0.025303987005773,-0.0126518802269383,
-8.98671033422449E-11),.UNSPECIFIED.);
#23541=B_SPLINE_CURVE_WITH_KNOTS('',3,(#148203,#148204,#148205,#148206,
#148207,#148208),.UNSPECIFIED.,.F.,.F.,(4,2,4),(-0.0253039876388824,-0.0126518800737849,
0.),.UNSPECIFIED.);
#23542=B_SPLINE_CURVE_WITH_KNOTS('',3,(#148228,#148229,#148230,#148231,
#148232,#148233),.UNSPECIFIED.,.F.,.F.,(4,2,4),(-0.0253039873540886,-0.0126518801299279,
-2.55819705696769E-11),.UNSPECIFIED.);
#23543=B_SPLINE_CURVE_WITH_KNOTS('',3,(#148253,#148254,#148255,#148256,
#148257,#148258),.UNSPECIFIED.,.F.,.F.,(4,2,4),(-0.0253039877440053,-0.0126518801932579,
-6.41805636414361E-11),.UNSPECIFIED.);
#23544=B_SPLINE_CURVE_WITH_KNOTS('',3,(#148278,#148279,#148280,#148281,
#148282,#148283),.UNSPECIFIED.,.F.,.F.,(4,2,4),(-0.025303988161419,-0.0126518802705622,
-1.48159921831148E-10),.UNSPECIFIED.);
#23545=B_SPLINE_CURVE_WITH_KNOTS('',3,(#148303,#148304,#148305,#148306,
#148307,#148308),.UNSPECIFIED.,.F.,.F.,(4,2,4),(-0.0253039868057278,-0.0126518802510195,
-1.43891034504184E-10),.UNSPECIFIED.);
#23546=B_SPLINE_CURVE_WITH_KNOTS('',3,(#148328,#148329,#148330,#148331,
#148332,#148333),.UNSPECIFIED.,.F.,.F.,(4,2,4),(-0.0253039861773998,-0.0126518792406827,
-1.25047541765788E-12),.UNSPECIFIED.);
#23547=B_SPLINE_CURVE_WITH_KNOTS('',3,(#148353,#148354,#148355,#148356,
#148357,#148358),.UNSPECIFIED.,.F.,.F.,(4,2,4),(-0.0253039872355756,-0.012651880214651,
-8.66837955582067E-11),.UNSPECIFIED.);
#23548=B_SPLINE_CURVE_WITH_KNOTS('',3,(#148378,#148379,#148380,#148381,
#148382,#148383),.UNSPECIFIED.,.F.,.F.,(4,2,4),(-0.025303986926397,-0.0126518801426057,
-3.96025053028826E-11),.UNSPECIFIED.);
#23549=B_SPLINE_CURVE_WITH_KNOTS('',3,(#148403,#148404,#148405,#148406,
#148407,#148408),.UNSPECIFIED.,.F.,.F.,(4,2,4),(-0.0253039871076078,-0.0126518802996017,
-1.54504083138551E-10),.UNSPECIFIED.);
#23550=B_SPLINE_CURVE_WITH_KNOTS('',3,(#148428,#148429,#148430,#148431,
#148432,#148433),.UNSPECIFIED.,.F.,.F.,(4,2,4),(-0.0253039881080807,-0.012651880317787,
-1.8657949837908E-10),.UNSPECIFIED.);
#23551=B_SPLINE_CURVE_WITH_KNOTS('',3,(#148453,#148454,#148455,#148456,
#148457,#148458),.UNSPECIFIED.,.F.,.F.,(4,2,4),(-0.0253039878268396,-0.012651880171774,
-5.62077259735894E-11),.UNSPECIFIED.);
#23552=B_SPLINE_CURVE_WITH_KNOTS('',3,(#148478,#148479,#148480,#148481,
#148482,#148483),.UNSPECIFIED.,.F.,.F.,(4,2,4),(-0.0253039875227548,-0.012651880215428,
-9.63703908340996E-11),.UNSPECIFIED.);
#23553=B_SPLINE_CURVE_WITH_KNOTS('',3,(#148503,#148504,#148505,#148506,
#148507,#148508),.UNSPECIFIED.,.F.,.F.,(4,2,4),(-0.0253039869108518,-0.0126518801654752,
-5.19251655561881E-11),.UNSPECIFIED.);
#23554=B_SPLINE_CURVE_WITH_KNOTS('',3,(#148528,#148529,#148530,#148531,
#148532,#148533),.UNSPECIFIED.,.F.,.F.,(4,2,4),(-0.0253039878151877,-0.0126518800924445,
0.),.UNSPECIFIED.);
#23555=B_SPLINE_CURVE_WITH_KNOTS('',3,(#148553,#148554,#148555,#148556,
#148557,#148558),.UNSPECIFIED.,.F.,.F.,(4,2,4),(-0.0253039878504019,-0.0126518801601293,
-8.34110037983837E-11),.UNSPECIFIED.);
#23556=B_SPLINE_CURVE_WITH_KNOTS('',3,(#148578,#148579,#148580,#148581,
#148582,#148583),.UNSPECIFIED.,.F.,.F.,(4,2,4),(-0.0253039876310961,-0.0126518802884517,
-1.63184913498648E-10),.UNSPECIFIED.);
#23557=B_SPLINE_CURVE_WITH_KNOTS('',3,(#148603,#148604,#148605,#148606,
#148607,#148608),.UNSPECIFIED.,.F.,.F.,(4,2,4),(-0.0253039877773045,-0.012651880230267,
-8.69090979738196E-11),.UNSPECIFIED.);
#23558=B_SPLINE_CURVE_WITH_KNOTS('',3,(#148628,#148629,#148630,#148631,
#148632,#148633),.UNSPECIFIED.,.F.,.F.,(4,2,4),(-0.025303986895663,-0.0126518801777525,
-8.87840599650414E-11),.UNSPECIFIED.);
#23559=B_SPLINE_CURVE_WITH_KNOTS('',3,(#148653,#148654,#148655,#148656,
#148657,#148658),.UNSPECIFIED.,.F.,.F.,(4,2,4),(-0.0253039879972589,-0.0126518801718497,
-6.59172473549408E-11),.UNSPECIFIED.);
#23560=B_SPLINE_CURVE_WITH_KNOTS('',3,(#148678,#148679,#148680,#148681,
#148682,#148683),.UNSPECIFIED.,.F.,.F.,(4,2,4),(-0.0253039869494593,-0.0126518802187377,
-1.08653201019715E-10),.UNSPECIFIED.);
#23561=B_SPLINE_CURVE_WITH_KNOTS('',3,(#148715,#148716,#148717,#148718,
#148719,#148720),.UNSPECIFIED.,.F.,.F.,(4,2,4),(1.2316114164264E-10,0.012650972362086,
0.0253021873423967),.UNSPECIFIED.);
#23562=B_SPLINE_CURVE_WITH_KNOTS('',3,(#148727,#148728,#148729,#148730,
#148731,#148732,#148733),.UNSPECIFIED.,.F.,.F.,(4,3,4),(0.561466076967393,
0.571428571428571,0.57365435021991),.UNSPECIFIED.);
#23563=B_SPLINE_CURVE_WITH_KNOTS('',3,(#148758,#148759,#148760,#148761,
#148762,#148763),.UNSPECIFIED.,.F.,.F.,(4,2,4),(0.,0.012650972319385,0.0253021873649507),
 .UNSPECIFIED.);
#23564=B_SPLINE_CURVE_WITH_KNOTS('',3,(#148770,#148771,#148772,#148773,
#148774,#148775,#148776),.UNSPECIFIED.,.F.,.F.,(4,3,4),(0.561466076966358,
0.571428571428571,0.57365435021991),.UNSPECIFIED.);
#23565=B_SPLINE_CURVE_WITH_KNOTS('',3,(#148801,#148802,#148803,#148804,
#148805,#148806),.UNSPECIFIED.,.F.,.F.,(4,2,4),(0.,0.012650972315468,0.025302187363785),
 .UNSPECIFIED.);
#23566=B_SPLINE_CURVE_WITH_KNOTS('',3,(#148813,#148814,#148815,#148816,
#148817,#148818,#148819),.UNSPECIFIED.,.F.,.F.,(4,3,4),(0.561466076969539,
0.571428571428571,0.573654350219911),.UNSPECIFIED.);
#23567=B_SPLINE_CURVE_WITH_KNOTS('',3,(#148844,#148845,#148846,#148847,
#148848,#148849),.UNSPECIFIED.,.F.,.F.,(4,2,4),(9.04688586768257E-11,0.0126509723542132,
0.0253021873590814),.UNSPECIFIED.);
#23568=B_SPLINE_CURVE_WITH_KNOTS('',3,(#148856,#148857,#148858,#148859,
#148860,#148861,#148862),.UNSPECIFIED.,.F.,.F.,(4,3,4),(0.561466076978747,
0.571428571428571,0.573654350219911),.UNSPECIFIED.);
#23569=B_SPLINE_CURVE_WITH_KNOTS('',3,(#148887,#148888,#148889,#148890,
#148891,#148892),.UNSPECIFIED.,.F.,.F.,(4,2,4),(1.55063105361005E-10,0.0126509724789961,
0.0253021874395334),.UNSPECIFIED.);
#23570=B_SPLINE_CURVE_WITH_KNOTS('',3,(#148899,#148900,#148901,#148902,
#148903,#148904,#148905),.UNSPECIFIED.,.F.,.F.,(4,3,4),(0.561466076972735,
0.571428571428571,0.573654350219911),.UNSPECIFIED.);
#23571=B_SPLINE_CURVE_WITH_KNOTS('',3,(#148930,#148931,#148932,#148933,
#148934,#148935),.UNSPECIFIED.,.F.,.F.,(4,2,4),(1.18014507066057E-10,0.0126509723379533,
0.0253021873193351),.UNSPECIFIED.);
#23572=B_SPLINE_CURVE_WITH_KNOTS('',3,(#148942,#148943,#148944,#148945,
#148946,#148947,#148948),.UNSPECIFIED.,.F.,.F.,(4,3,4),(0.561466076971035,
0.571428571428571,0.573654350219911),.UNSPECIFIED.);
#23573=B_SPLINE_CURVE_WITH_KNOTS('',3,(#148973,#148974,#148975,#148976,
#148977,#148978),.UNSPECIFIED.,.F.,.F.,(4,2,4),(1.33608236322443E-10,0.0126509723640742,
0.0253021873406959),.UNSPECIFIED.);
#23574=B_SPLINE_CURVE_WITH_KNOTS('',3,(#148985,#148986,#148987,#148988,
#148989,#148990,#148991),.UNSPECIFIED.,.F.,.F.,(4,3,4),(0.561466076969876,
0.571428571428571,0.573654350219911),.UNSPECIFIED.);
#23575=B_SPLINE_CURVE_WITH_KNOTS('',3,(#149016,#149017,#149018,#149019,
#149020,#149021),.UNSPECIFIED.,.F.,.F.,(4,2,4),(8.75960167674949E-11,0.012650972335585,
0.025302187348281),.UNSPECIFIED.);
#23576=B_SPLINE_CURVE_WITH_KNOTS('',3,(#149028,#149029,#149030,#149031,
#149032,#149033,#149034),.UNSPECIFIED.,.F.,.F.,(4,3,4),(0.561466076970862,
0.571428571428571,0.573654350219911),.UNSPECIFIED.);
#23577=B_SPLINE_CURVE_WITH_KNOTS('',3,(#149059,#149060,#149061,#149062,
#149063,#149064),.UNSPECIFIED.,.F.,.F.,(4,2,4),(1.13250179511007E-10,0.0126509723673497,
0.0253021873796661),.UNSPECIFIED.);
#23578=B_SPLINE_CURVE_WITH_KNOTS('',3,(#149071,#149072,#149073,#149074,
#149075,#149076,#149077),.UNSPECIFIED.,.F.,.F.,(4,3,4),(0.561466076977858,
0.571428571428571,0.573654350219911),.UNSPECIFIED.);
#23579=B_SPLINE_CURVE_WITH_KNOTS('',3,(#149102,#149103,#149104,#149105,
#149106,#149107),.UNSPECIFIED.,.F.,.F.,(4,2,4),(3.19290848309924E-11,0.012650984626482,
0.0253022387208064),.UNSPECIFIED.);
#23580=B_SPLINE_CURVE_WITH_KNOTS('',3,(#149114,#149115,#149116,#149117,
#149118,#149119,#149120),.UNSPECIFIED.,.F.,.F.,(4,3,4),(0.561466076972143,
0.571428571428571,0.573654350219912),.UNSPECIFIED.);
#23581=B_SPLINE_CURVE_WITH_KNOTS('',3,(#149145,#149146,#149147,#149148,
#149149,#149150),.UNSPECIFIED.,.F.,.F.,(4,2,4),(3.90657541139824E-11,0.0126509723622263,
0.0253021873944465),.UNSPECIFIED.);
#23582=B_SPLINE_CURVE_WITH_KNOTS('',3,(#149157,#149158,#149159,#149160,
#149161,#149162,#149163),.UNSPECIFIED.,.F.,.F.,(4,3,4),(0.561466076972731,
0.571428571428571,0.573654350219911),.UNSPECIFIED.);
#23583=B_SPLINE_CURVE_WITH_KNOTS('',3,(#149188,#149189,#149190,#149191,
#149192,#149193),.UNSPECIFIED.,.F.,.F.,(4,2,4),(1.43287852277096E-10,0.0126509723742098,
0.0253021873653449),.UNSPECIFIED.);
#23584=B_SPLINE_CURVE_WITH_KNOTS('',3,(#149200,#149201,#149202,#149203,
#149204,#149205,#149206),.UNSPECIFIED.,.F.,.F.,(4,3,4),(0.561466076975045,
0.571428571428571,0.573654350219911),.UNSPECIFIED.);
#23585=B_SPLINE_CURVE_WITH_KNOTS('',3,(#149231,#149232,#149233,#149234,
#149235,#149236),.UNSPECIFIED.,.F.,.F.,(4,2,4),(6.13476290471813E-12,0.012650972297768,
0.0253021873857862),.UNSPECIFIED.);
#23586=B_SPLINE_CURVE_WITH_KNOTS('',3,(#149243,#149244,#149245,#149246,
#149247,#149248,#149249),.UNSPECIFIED.,.F.,.F.,(4,3,4),(0.561466076967729,
0.571428571428571,0.573654350219911),.UNSPECIFIED.);
#23587=B_SPLINE_CURVE_WITH_KNOTS('',3,(#149274,#149275,#149276,#149277,
#149278,#149279),.UNSPECIFIED.,.F.,.F.,(4,2,4),(1.30084725401937E-10,0.0126509853979978,
0.0253022417622605),.UNSPECIFIED.);
#23588=B_SPLINE_CURVE_WITH_KNOTS('',3,(#149286,#149287,#149288,#149289,
#149290,#149291,#149292),.UNSPECIFIED.,.F.,.F.,(4,3,4),(0.561466076973636,
0.571428571428571,0.573654350219912),.UNSPECIFIED.);
#23589=B_SPLINE_CURVE_WITH_KNOTS('',3,(#149314,#149315,#149316,#149317,
#149318,#149319),.UNSPECIFIED.,.F.,.F.,(4,2,4),(5.6077424021607E-11,0.0126509723730836,
0.0253021874161603),.UNSPECIFIED.);
#23590=B_SPLINE_CURVE_WITH_KNOTS('',3,(#149345,#149346,#149347,#149348,
#149349,#149350),.UNSPECIFIED.,.F.,.F.,(4,2,4),(9.5934436762368E-11,0.0126509723665809,
0.0253021873569743),.UNSPECIFIED.);
#23591=B_SPLINE_CURVE_WITH_KNOTS('',3,(#149357,#149358,#149359,#149360,
#149361,#149362,#149363),.UNSPECIFIED.,.F.,.F.,(4,3,4),(0.561466076970824,
0.571428571428571,0.573654350219912),.UNSPECIFIED.);
#23592=B_SPLINE_CURVE_WITH_KNOTS('',3,(#149388,#149389,#149390,#149391,
#149392,#149393),.UNSPECIFIED.,.F.,.F.,(4,2,4),(0.,0.012650972289366,0.025302187368722),
 .UNSPECIFIED.);
#23593=B_SPLINE_CURVE_WITH_KNOTS('',3,(#149400,#149401,#149402,#149403,
#149404,#149405,#149406),.UNSPECIFIED.,.F.,.F.,(4,3,4),(0.561466076966466,
0.571428571428571,0.573654350219911),.UNSPECIFIED.);
#23594=B_SPLINE_CURVE_WITH_KNOTS('',3,(#149431,#149432,#149433,#149434,
#149435,#149436),.UNSPECIFIED.,.F.,.F.,(4,2,4),(2.03238081656241E-11,0.0126509859875903,
0.025302244503775),.UNSPECIFIED.);
#23595=B_SPLINE_CURVE_WITH_KNOTS('',3,(#149443,#149444,#149445,#149446,
#149447,#149448,#149449),.UNSPECIFIED.,.F.,.F.,(4,3,4),(0.561466076969195,
0.571428571428571,0.573654350219911),.UNSPECIFIED.);
#23596=B_SPLINE_CURVE_WITH_KNOTS('',3,(#149474,#149475,#149476,#149477,
#149478,#149479),.UNSPECIFIED.,.F.,.F.,(4,2,4),(7.54818598705809E-11,0.0126509724217488,
0.0253021872329842),.UNSPECIFIED.);
#23597=B_SPLINE_CURVE_WITH_KNOTS('',3,(#149492,#149493,#149494,#149495,
#149496,#149497,#149498),.UNSPECIFIED.,.F.,.F.,(4,3,4),(0.561466077,0.571428571428571,
0.573654350219911),.UNSPECIFIED.);
#23598=B_SPLINE_CURVE_WITH_KNOTS('',3,(#149518,#149519,#149520,#149521,
#149522,#149523),.UNSPECIFIED.,.F.,.F.,(4,2,4),(1.59968285071419E-10,0.0126509724314883,
0.0253021874246143),.UNSPECIFIED.);
#23599=B_SPLINE_CURVE_WITH_KNOTS('',3,(#149526,#149527,#149528,#149529,
#149530,#149531,#149532),.UNSPECIFIED.,.F.,.F.,(4,3,4),(0.561466076974998,
0.571428571428571,0.573654350219913),.UNSPECIFIED.);
#23600=B_SPLINE_CURVE_WITH_KNOTS('',3,(#149560,#149561,#149562,#149563,
#149564,#149565),.UNSPECIFIED.,.F.,.F.,(4,2,4),(0.,0.0126509723220439,0.0253021873975209),
 .UNSPECIFIED.);
#23601=B_SPLINE_CURVE_WITH_KNOTS('',3,(#149572,#149573,#149574,#149575,
#149576,#149577,#149578),.UNSPECIFIED.,.F.,.F.,(4,3,4),(0.561466076968925,
0.571428571428571,0.573654350219921),.UNSPECIFIED.);
#23602=B_SPLINE_CURVE_WITH_KNOTS('',3,(#149603,#149604,#149605,#149606,
#149607,#149608),.UNSPECIFIED.,.F.,.F.,(4,2,4),(3.40001431064816E-11,0.0126509723440331,
0.0253021873749516),.UNSPECIFIED.);
#23603=B_SPLINE_CURVE_WITH_KNOTS('',3,(#149615,#149616,#149617,#149618,
#149619,#149620,#149621),.UNSPECIFIED.,.F.,.F.,(4,3,4),(0.561466076968893,
0.571428571428571,0.57365435021992),.UNSPECIFIED.);
#23604=B_SPLINE_CURVE_WITH_KNOTS('',3,(#149646,#149647,#149648,#149649,
#149650,#149651),.UNSPECIFIED.,.F.,.F.,(4,2,4),(1.61417479377113E-10,0.0126509724299645,
0.025302187398691),.UNSPECIFIED.);
#23605=B_SPLINE_CURVE_WITH_KNOTS('',3,(#149658,#149659,#149660,#149661,
#149662,#149663,#149664),.UNSPECIFIED.,.F.,.F.,(4,3,4),(0.561466076970706,
0.571428571428571,0.573654350219922),.UNSPECIFIED.);
#23606=B_SPLINE_CURVE_WITH_KNOTS('',3,(#149689,#149690,#149691,#149692,
#149693,#149694),.UNSPECIFIED.,.F.,.F.,(4,2,4),(1.72077501315142E-11,0.0126509723056168,
0.0253021873602548),.UNSPECIFIED.);
#23607=B_SPLINE_CURVE_WITH_KNOTS('',3,(#149701,#149702,#149703,#149704,
#149705,#149706,#149707),.UNSPECIFIED.,.F.,.F.,(4,3,4),(0.561466076970486,
0.571428571428571,0.57365435021991),.UNSPECIFIED.);
#23608=B_SPLINE_CURVE_WITH_KNOTS('',3,(#149732,#149733,#149734,#149735,
#149736,#149737),.UNSPECIFIED.,.F.,.F.,(4,2,4),(0.,0.0126509722816313,0.0253021873170131),
 .UNSPECIFIED.);
#23609=B_SPLINE_CURVE_WITH_KNOTS('',3,(#149744,#149745,#149746,#149747,
#149748,#149749,#149750),.UNSPECIFIED.,.F.,.F.,(4,3,4),(0.561466076974285,
0.571428571428571,0.57365435021991),.UNSPECIFIED.);
#23610=B_SPLINE_CURVE_WITH_KNOTS('',3,(#149775,#149776,#149777,#149778,
#149779,#149780),.UNSPECIFIED.,.F.,.F.,(4,2,4),(1.75845480016369E-10,0.0126509724250738,
0.0253021874139565),.UNSPECIFIED.);
#23611=B_SPLINE_CURVE_WITH_KNOTS('',3,(#149787,#149788,#149789,#149790,
#149791,#149792,#149793),.UNSPECIFIED.,.F.,.F.,(4,3,4),(0.561466076973471,
0.571428571428571,0.57365435021991),.UNSPECIFIED.);
#23612=B_SPLINE_CURVE_WITH_KNOTS('',3,(#149818,#149819,#149820,#149821,
#149822,#149823),.UNSPECIFIED.,.F.,.F.,(4,2,4),(2.3529783390845E-11,0.0126509723223139,
0.0253021873783273),.UNSPECIFIED.);
#23613=B_SPLINE_CURVE_WITH_KNOTS('',3,(#149830,#149831,#149832,#149833,
#149834,#149835,#149836),.UNSPECIFIED.,.F.,.F.,(4,3,4),(0.561466076971879,
0.571428571428571,0.57365435021991),.UNSPECIFIED.);
#23614=B_SPLINE_CURVE_WITH_KNOTS('',3,(#149861,#149862,#149863,#149864,
#149865,#149866),.UNSPECIFIED.,.F.,.F.,(4,2,4),(4.81522774177321E-11,0.0126509851968905,
0.0253022411313395),.UNSPECIFIED.);
#23615=B_SPLINE_CURVE_WITH_KNOTS('',3,(#149873,#149874,#149875,#149876,
#149877,#149878,#149879),.UNSPECIFIED.,.F.,.F.,(4,3,4),(0.561466076969465,
0.571428571428571,0.57365435021991),.UNSPECIFIED.);
#23616=B_SPLINE_CURVE_WITH_KNOTS('',3,(#149904,#149905,#149906,#149907,
#149908,#149909),.UNSPECIFIED.,.F.,.F.,(4,2,4),(0.,0.0126509722877906,0.0253021873372228),
 .UNSPECIFIED.);
#23617=B_SPLINE_CURVE_WITH_KNOTS('',3,(#149916,#149917,#149918,#149919,
#149920,#149921,#149922),.UNSPECIFIED.,.F.,.F.,(4,3,4),(0.561466076971086,
0.571428571428571,0.57365435021991),.UNSPECIFIED.);
#23618=B_SPLINE_CURVE_WITH_KNOTS('',3,(#149948,#149949,#149950,#149951,
#149952,#149953),.UNSPECIFIED.,.F.,.F.,(4,2,4),(-0.0253038285839127,-0.0126520268760324,
0.),.UNSPECIFIED.);
#23619=B_SPLINE_CURVE_WITH_KNOTS('',3,(#149987,#149988,#149989,#149990,
#149991,#149992),.UNSPECIFIED.,.F.,.F.,(4,2,4),(-0.0253038286551005,-0.012652026917456,
0.),.UNSPECIFIED.);
#23620=B_SPLINE_CURVE_WITH_KNOTS('',3,(#150026,#150027,#150028,#150029,
#150030,#150031),.UNSPECIFIED.,.F.,.F.,(4,2,4),(-0.0253038285468146,-0.0126520268079982,
0.),.UNSPECIFIED.);
#23621=B_SPLINE_CURVE_WITH_KNOTS('',3,(#150065,#150066,#150067,#150068,
#150069,#150070),.UNSPECIFIED.,.F.,.F.,(4,2,4),(-0.0253038284106424,-0.0126520267846328,
-1.9438166354302E-11),.UNSPECIFIED.);
#23622=B_SPLINE_CURVE_WITH_KNOTS('',3,(#150104,#150105,#150106,#150107,
#150108,#150109),.UNSPECIFIED.,.F.,.F.,(4,2,4),(-0.0253038285523641,-0.0126520269075616,
-8.06536434860838E-12),.UNSPECIFIED.);
#23623=B_SPLINE_CURVE_WITH_KNOTS('',3,(#150143,#150144,#150145,#150146,
#150147,#150148),.UNSPECIFIED.,.F.,.F.,(4,2,4),(-0.0253038285807823,-0.012652026911929,
0.),.UNSPECIFIED.);
#23624=B_SPLINE_CURVE_WITH_KNOTS('',3,(#150182,#150183,#150184,#150185,
#150186,#150187),.UNSPECIFIED.,.F.,.F.,(4,2,4),(-0.0253038286017608,-0.0126520268893115,
0.),.UNSPECIFIED.);
#23625=B_SPLINE_CURVE_WITH_KNOTS('',3,(#150221,#150222,#150223,#150224,
#150225,#150226),.UNSPECIFIED.,.F.,.F.,(4,2,4),(-0.0253038285628698,-0.0126520269487189,
-1.01505019667325E-11),.UNSPECIFIED.);
#23626=B_SPLINE_CURVE_WITH_KNOTS('',3,(#150260,#150261,#150262,#150263,
#150264,#150265),.UNSPECIFIED.,.F.,.F.,(4,2,4),(-0.0253038284600093,-0.0126520268733603,
-1.30362942662998E-11),.UNSPECIFIED.);
#23627=B_SPLINE_CURVE_WITH_KNOTS('',3,(#150299,#150300,#150301,#150302,
#150303,#150304),.UNSPECIFIED.,.F.,.F.,(4,2,4),(-0.0253038285157797,-0.0126520268380531,
0.),.UNSPECIFIED.);
#23628=B_SPLINE_CURVE_WITH_KNOTS('',3,(#150338,#150339,#150340,#150341,
#150342,#150343),.UNSPECIFIED.,.F.,.F.,(4,2,4),(-0.025303828580961,-0.0126520268888839,
-3.22808793584706E-12),.UNSPECIFIED.);
#23629=B_SPLINE_CURVE_WITH_KNOTS('',3,(#150377,#150378,#150379,#150380,
#150381,#150382),.UNSPECIFIED.,.F.,.F.,(4,2,4),(-0.0253038285191941,-0.0126520268349931,
0.),.UNSPECIFIED.);
#23630=B_SPLINE_CURVE_WITH_KNOTS('',3,(#150416,#150417,#150418,#150419,
#150420,#150421),.UNSPECIFIED.,.F.,.F.,(4,2,4),(-0.025303828506458,-0.0126520269004065,
-1.72773739759435E-11),.UNSPECIFIED.);
#23631=B_SPLINE_CURVE_WITH_KNOTS('',3,(#150455,#150456,#150457,#150458,
#150459,#150460),.UNSPECIFIED.,.F.,.F.,(4,2,4),(-0.0253038286343293,-0.0126520268567648,
0.),.UNSPECIFIED.);
#23632=B_SPLINE_CURVE_WITH_KNOTS('',3,(#150494,#150495,#150496,#150497,
#150498,#150499),.UNSPECIFIED.,.F.,.F.,(4,2,4),(-0.0253038285556593,-0.0126520268415039,
0.),.UNSPECIFIED.);
#23633=B_SPLINE_CURVE_WITH_KNOTS('',3,(#150533,#150534,#150535,#150536,
#150537,#150538),.UNSPECIFIED.,.F.,.F.,(4,2,4),(-0.025303828616761,-0.0126520269208739,
0.),.UNSPECIFIED.);
#23634=B_SPLINE_CURVE_WITH_KNOTS('',3,(#150572,#150573,#150574,#150575,
#150576,#150577),.UNSPECIFIED.,.F.,.F.,(4,2,4),(-0.0253038284604553,-0.0126520268848923,
-1.02886171804428E-11),.UNSPECIFIED.);
#23635=B_SPLINE_CURVE_WITH_KNOTS('',3,(#150611,#150612,#150613,#150614,
#150615,#150616),.UNSPECIFIED.,.F.,.F.,(4,2,4),(-0.0253038286149417,-0.0126520269606899,
-3.53035656264211E-12),.UNSPECIFIED.);
#23636=B_SPLINE_CURVE_WITH_KNOTS('',3,(#150650,#150651,#150652,#150653,
#150654,#150655),.UNSPECIFIED.,.F.,.F.,(4,2,4),(-0.0253038284892162,-0.0126520268129704,
-2.58471022362983E-12),.UNSPECIFIED.);
#23637=B_SPLINE_CURVE_WITH_KNOTS('',3,(#150689,#150690,#150691,#150692,
#150693,#150694),.UNSPECIFIED.,.F.,.F.,(4,2,4),(-0.0253038284441624,-0.0126520268794058,
-1.13759314468442E-11),.UNSPECIFIED.);
#23638=B_SPLINE_CURVE_WITH_KNOTS('',3,(#150728,#150729,#150730,#150731,
#150732,#150733),.UNSPECIFIED.,.F.,.F.,(4,2,4),(-0.0253038285376909,-0.0126520268358134,
0.),.UNSPECIFIED.);
#23639=B_SPLINE_CURVE_WITH_KNOTS('',3,(#150764,#150765,#150766,#150767,
#150768,#150769),.UNSPECIFIED.,.F.,.F.,(4,2,4),(-0.0253038285032559,-0.0126520268449107,
-7.70856642406947E-12),.UNSPECIFIED.);
#23640=B_SPLINE_CURVE_WITH_KNOTS('',3,(#150791,#150792,#150793,#150794,
#150795,#150796),.UNSPECIFIED.,.F.,.F.,(4,2,4),(-0.0253038286446529,-0.0126520268985584,
0.),.UNSPECIFIED.);
#23641=B_SPLINE_CURVE_WITH_KNOTS('',3,(#150830,#150831,#150832,#150833,
#150834,#150835),.UNSPECIFIED.,.F.,.F.,(4,2,4),(-0.0253038286142863,-0.012652026982915,
-1.52916915241441E-12),.UNSPECIFIED.);
#23642=B_SPLINE_CURVE_WITH_KNOTS('',3,(#150869,#150870,#150871,#150872,
#150873,#150874),.UNSPECIFIED.,.F.,.F.,(4,2,4),(-0.0253038286058837,-0.0126520269289845,
0.),.UNSPECIFIED.);
#23643=B_SPLINE_CURVE_WITH_KNOTS('',3,(#150908,#150909,#150910,#150911,
#150912,#150913),.UNSPECIFIED.,.F.,.F.,(4,2,4),(-0.0253038285954271,-0.0126520269217119,
-3.19100648682458E-12),.UNSPECIFIED.);
#23644=B_SPLINE_CURVE_WITH_KNOTS('',3,(#150947,#150948,#150949,#150950,
#150951,#150952),.UNSPECIFIED.,.F.,.F.,(4,2,4),(-0.025303828457649,-0.0126520268415871,
-1.61810773113835E-11),.UNSPECIFIED.);
#23645=B_SPLINE_CURVE_WITH_KNOTS('',3,(#150986,#150987,#150988,#150989,
#150990,#150991),.UNSPECIFIED.,.F.,.F.,(4,2,4),(-0.0253038285087455,-0.0126520267988281,
0.),.UNSPECIFIED.);
#23646=B_SPLINE_CURVE_WITH_KNOTS('',3,(#151025,#151026,#151027,#151028,
#151029,#151030),.UNSPECIFIED.,.F.,.F.,(4,2,4),(-0.0253038285970617,-0.0126520269741822,
-1.24514287769273E-11),.UNSPECIFIED.);
#23647=B_SPLINE_CURVE_WITH_KNOTS('',3,(#151062,#151063,#151064,#151065,
#151066,#151067),.UNSPECIFIED.,.F.,.F.,(4,2,4),(-0.0240533908522633,-0.0122571958022784,
0.),.UNSPECIFIED.);
#23648=B_SPLINE_CURVE_WITH_KNOTS('',3,(#151091,#151092,#151093,#151094,
#151095,#151096),.UNSPECIFIED.,.F.,.F.,(4,2,4),(-0.0240535314783445,-0.0122572446394088,
0.),.UNSPECIFIED.);
#23649=B_SPLINE_CURVE_WITH_KNOTS('',3,(#151120,#151121,#151122,#151123,
#151124,#151125),.UNSPECIFIED.,.F.,.F.,(4,2,4),(-0.0240532016237181,-0.0122571280238569,
0.),.UNSPECIFIED.);
#23650=B_SPLINE_CURVE_WITH_KNOTS('',3,(#151149,#151150,#151151,#151152,
#151153,#151154),.UNSPECIFIED.,.F.,.F.,(4,2,4),(-0.0240533156711824,-0.0122571705517197,
0.),.UNSPECIFIED.);
#23651=B_SPLINE_CURVE_WITH_KNOTS('',3,(#151183,#151184,#151185,#151186,
#151187,#151188),.UNSPECIFIED.,.F.,.F.,(4,2,4),(-0.0240537809878963,-0.0122573306077586,
0.),.UNSPECIFIED.);
#23652=B_SPLINE_CURVE_WITH_KNOTS('',3,(#151217,#151218,#151219,#151220,
#151221,#151222),.UNSPECIFIED.,.F.,.F.,(4,2,4),(-0.024053361759142,-0.0122571855913509,
0.),.UNSPECIFIED.);
#23653=B_SPLINE_CURVE_WITH_KNOTS('',3,(#151246,#151247,#151248,#151249,
#151250,#151251),.UNSPECIFIED.,.F.,.F.,(4,2,4),(-0.0240534328364565,-0.0122572100588516,
0.),.UNSPECIFIED.);
#23654=B_SPLINE_CURVE_WITH_KNOTS('',3,(#151275,#151276,#151277,#151278,
#151279,#151280),.UNSPECIFIED.,.F.,.F.,(4,2,4),(-0.0240533728250536,-0.0122571910559405,
0.),.UNSPECIFIED.);
#23655=B_SPLINE_CURVE_WITH_KNOTS('',3,(#151304,#151305,#151306,#151307,
#151308,#151309),.UNSPECIFIED.,.F.,.F.,(4,2,4),(-0.0240533442755893,-0.0122571809828921,
0.),.UNSPECIFIED.);
#23656=B_SPLINE_CURVE_WITH_KNOTS('',3,(#151333,#151334,#151335,#151336,
#151337,#151338),.UNSPECIFIED.,.F.,.F.,(4,2,4),(-0.0240529243109103,-0.012257032788197,
0.),.UNSPECIFIED.);
#23657=B_SPLINE_CURVE_WITH_KNOTS('',3,(#151362,#151363,#151364,#151365,
#151366,#151367),.UNSPECIFIED.,.F.,.F.,(4,2,4),(-0.0240532082872642,-0.0122571342903452,
0.),.UNSPECIFIED.);
#23658=B_SPLINE_CURVE_WITH_KNOTS('',3,(#151396,#151397,#151398,#151399,
#151400,#151401),.UNSPECIFIED.,.F.,.F.,(4,2,4),(-0.0240534422631641,-0.0122572124745634,
0.),.UNSPECIFIED.);
#23659=B_SPLINE_CURVE_WITH_KNOTS('',3,(#151425,#151426,#151427,#151428,
#151429,#151430),.UNSPECIFIED.,.F.,.F.,(4,2,4),(-0.0240532828403448,-0.0122571585650213,
0.),.UNSPECIFIED.);
#23660=B_SPLINE_CURVE_WITH_KNOTS('',3,(#151454,#151455,#151456,#151457,
#151458,#151459),.UNSPECIFIED.,.F.,.F.,(4,2,4),(-0.0240534794813553,-0.0122572283945417,
0.),.UNSPECIFIED.);
#23661=B_SPLINE_CURVE_WITH_KNOTS('',3,(#151483,#151484,#151485,#151486,
#151487,#151488),.UNSPECIFIED.,.F.,.F.,(4,2,4),(-0.02405383490832,-0.012257350841524,
0.),.UNSPECIFIED.);
#23662=B_SPLINE_CURVE_WITH_KNOTS('',3,(#151517,#151518,#151519,#151520,
#151521,#151522),.UNSPECIFIED.,.F.,.F.,(4,2,4),(-0.0240530169280848,-0.0122570654448755,
0.),.UNSPECIFIED.);
#23663=B_SPLINE_CURVE_WITH_KNOTS('',3,(#151546,#151547,#151548,#151549,
#151550,#151551),.UNSPECIFIED.,.F.,.F.,(4,2,4),(-0.0240533479705919,-0.0122571825715407,
0.),.UNSPECIFIED.);
#23664=B_SPLINE_CURVE_WITH_KNOTS('',3,(#151575,#151576,#151577,#151578,
#151579,#151580),.UNSPECIFIED.,.F.,.F.,(4,2,4),(-0.024053311848544,-0.0122571689410321,
0.),.UNSPECIFIED.);
#23665=B_SPLINE_CURVE_WITH_KNOTS('',3,(#151604,#151605,#151606,#151607,
#151608,#151609),.UNSPECIFIED.,.F.,.F.,(4,2,4),(-0.0240533439257344,-0.012257179103354,
0.),.UNSPECIFIED.);
#23666=B_SPLINE_CURVE_WITH_KNOTS('',3,(#151633,#151634,#151635,#151636,
#151637,#151638),.UNSPECIFIED.,.F.,.F.,(4,2,4),(-0.0240530635024099,-0.0122570824968178,
0.),.UNSPECIFIED.);
#23667=B_SPLINE_CURVE_WITH_KNOTS('',3,(#151662,#151663,#151664,#151665,
#151666,#151667),.UNSPECIFIED.,.F.,.F.,(4,2,4),(-0.024053273040655,-0.0122571549226549,
0.),.UNSPECIFIED.);
#23668=B_SPLINE_CURVE_WITH_KNOTS('',3,(#151691,#151692,#151693,#151694,
#151695,#151696),.UNSPECIFIED.,.F.,.F.,(4,2,4),(-0.0240536699122217,-0.0122572931629393,
0.),.UNSPECIFIED.);
#23669=B_SPLINE_CURVE_WITH_KNOTS('',3,(#151720,#151721,#151722,#151723,
#151724,#151725),.UNSPECIFIED.,.F.,.F.,(4,2,4),(-0.0240536981873685,-0.0122573028539489,
0.),.UNSPECIFIED.);
#23670=B_SPLINE_CURVE_WITH_KNOTS('',3,(#151749,#151750,#151751,#151752,
#151753,#151754),.UNSPECIFIED.,.F.,.F.,(4,2,4),(-0.024053529185018,-0.0122572436632474,
0.),.UNSPECIFIED.);
#23671=B_SPLINE_CURVE_WITH_KNOTS('',3,(#151783,#151784,#151785,#151786,
#151787,#151788),.UNSPECIFIED.,.F.,.F.,(4,2,4),(-0.0240534288870408,-0.0122572093109304,
0.),.UNSPECIFIED.);
#23672=B_SPLINE_CURVE_WITH_KNOTS('',3,(#151812,#151813,#151814,#151815,
#151816,#151817),.UNSPECIFIED.,.F.,.F.,(4,2,4),(-0.0240537713625275,-0.0122573281131518,
0.),.UNSPECIFIED.);
#23673=B_SPLINE_CURVE_WITH_KNOTS('',3,(#151841,#151842,#151843,#151844,
#151845,#151846),.UNSPECIFIED.,.F.,.F.,(4,2,4),(-0.0240533351661113,-0.0122571766305564,
0.),.UNSPECIFIED.);
#23674=B_SPLINE_CURVE_WITH_KNOTS('',3,(#151870,#151871,#151872,#151873,
#151874,#151875),.UNSPECIFIED.,.F.,.F.,(4,2,4),(-0.024054081148553,-0.0122574351715113,
0.),.UNSPECIFIED.);
#23675=B_SPLINE_CURVE_WITH_KNOTS('',3,(#151899,#151900,#151901,#151902,
#151903,#151904),.UNSPECIFIED.,.F.,.F.,(4,2,4),(-0.0240530980436435,-0.0122570945679079,
0.),.UNSPECIFIED.);
#23676=B_SPLINE_CURVE_WITH_KNOTS('',3,(#152515,#152516,#152517,#152518,
#152519,#152520),.UNSPECIFIED.,.F.,.F.,(4,2,4),(3.48126610442943E-11,0.0126485446413335,
0.025296968417101),.UNSPECIFIED.);
#23677=B_SPLINE_CURVE_WITH_KNOTS('',3,(#152538,#152539,#152540,#152541,
#152542,#152543),.UNSPECIFIED.,.F.,.F.,(4,2,4),(-0.0252968472729343,-0.0126485446090834,
-2.17366402655017E-11),.UNSPECIFIED.);
#23678=B_SPLINE_CURVE_WITH_KNOTS('',3,(#152579,#152580,#152581,#152582,
#152583,#152584),.UNSPECIFIED.,.F.,.F.,(4,2,4),(-0.0252968473826894,-0.0126485446000957,
-2.0234428715904E-11),.UNSPECIFIED.);
#23679=B_SPLINE_CURVE_WITH_KNOTS('',3,(#152620,#152621,#152622,#152623,
#152624,#152625),.UNSPECIFIED.,.F.,.F.,(4,2,4),(-0.0252968472290505,-0.0126485446178443,
-1.42757888843548E-11),.UNSPECIFIED.);
#23680=B_SPLINE_CURVE_WITH_KNOTS('',3,(#152661,#152662,#152663,#152664,
#152665,#152666),.UNSPECIFIED.,.F.,.F.,(4,2,4),(-0.0252968474456481,-0.0126485446475364,
-3.50366680113012E-11),.UNSPECIFIED.);
#23681=B_SPLINE_CURVE_WITH_KNOTS('',3,(#152702,#152703,#152704,#152705,
#152706,#152707),.UNSPECIFIED.,.F.,.F.,(4,2,4),(-0.0252969813766171,-0.0126485446434368,
-3.20461539249361E-11),.UNSPECIFIED.);
#23682=B_SPLINE_CURVE_WITH_KNOTS('',3,(#152743,#152744,#152745,#152746,
#152747,#152748),.UNSPECIFIED.,.F.,.F.,(4,2,4),(-0.0252969778573368,-0.0126485446281753,
-2.83896205155454E-11),.UNSPECIFIED.);
#23683=B_SPLINE_CURVE_WITH_KNOTS('',3,(#152781,#152782,#152783,#152784,
#152785,#152786),.UNSPECIFIED.,.F.,.F.,(4,2,4),(-0.0252969796412403,-0.0126485446363986,
-3.44679423891492E-11),.UNSPECIFIED.);
#23684=B_SPLINE_CURVE_WITH_KNOTS('',3,(#152816,#152817,#152818,#152819,
#152820,#152821),.UNSPECIFIED.,.F.,.F.,(4,2,4),(-0.0252969759465009,-0.0126485445986618,
0.),.UNSPECIFIED.);
#23685=B_SPLINE_CURVE_WITH_KNOTS('',3,(#152857,#152858,#152859,#152860,
#152861,#152862),.UNSPECIFIED.,.F.,.F.,(4,2,4),(-0.0252969599122676,-0.0126485446559965,
-2.64061897348178E-11),.UNSPECIFIED.);
#23686=B_SPLINE_CURVE_WITH_KNOTS('',3,(#152898,#152899,#152900,#152901,
#152902,#152903),.UNSPECIFIED.,.F.,.F.,(4,2,4),(-0.0252968474027855,-0.0126485446051056,
0.),.UNSPECIFIED.);
#23687=B_SPLINE_CURVE_WITH_KNOTS('',3,(#152939,#152940,#152941,#152942,
#152943,#152944),.UNSPECIFIED.,.F.,.F.,(4,2,4),(-0.0252969724871208,-0.0126485446152108,
0.),.UNSPECIFIED.);
#23688=B_SPLINE_CURVE_WITH_KNOTS('',3,(#152980,#152981,#152982,#152983,
#152984,#152985),.UNSPECIFIED.,.F.,.F.,(4,2,4),(-0.0252969815801744,-0.0126485446478389,
-3.94803981174086E-11),.UNSPECIFIED.);
#23689=B_SPLINE_CURVE_WITH_KNOTS('',3,(#153021,#153022,#153023,#153024,
#153025,#153026),.UNSPECIFIED.,.F.,.F.,(4,2,4),(-0.0252968472773642,-0.0126485446695086,
-5.66388602685208E-11),.UNSPECIFIED.);
#23690=B_SPLINE_CURVE_WITH_KNOTS('',3,(#153062,#153063,#153064,#153065,
#153066,#153067),.UNSPECIFIED.,.F.,.F.,(4,2,4),(-0.0252968473121451,-0.0126485446154412,
-1.1150868423071E-11),.UNSPECIFIED.);
#23691=B_SPLINE_CURVE_WITH_KNOTS('',3,(#153103,#153104,#153105,#153106,
#153107,#153108),.UNSPECIFIED.,.F.,.F.,(4,2,4),(-0.025296847243463,-0.0126485446122804,
-1.33509418798194E-11),.UNSPECIFIED.);
#23692=B_SPLINE_CURVE_WITH_KNOTS('',3,(#153144,#153145,#153146,#153147,
#153148,#153149),.UNSPECIFIED.,.F.,.F.,(4,2,4),(-0.0252968474367496,-0.0126485446764713,
-6.67833600920265E-11),.UNSPECIFIED.);
#23693=B_SPLINE_CURVE_WITH_KNOTS('',3,(#153185,#153186,#153187,#153188,
#153189,#153190),.UNSPECIFIED.,.F.,.F.,(4,2,4),(-0.0252968473967678,-0.0126485446111826,
-2.20091098124264E-11),.UNSPECIFIED.);
#23694=B_SPLINE_CURVE_WITH_KNOTS('',3,(#153226,#153227,#153228,#153229,
#153230,#153231),.UNSPECIFIED.,.F.,.F.,(4,2,4),(-0.025296977282385,-0.0126485447145659,
-8.45704270502345E-11),.UNSPECIFIED.);
#23695=B_SPLINE_CURVE_WITH_KNOTS('',3,(#153268,#153269,#153270,#153271,
#153272,#153273),.UNSPECIFIED.,.F.,.F.,(4,2,4),(-0.0252969810914952,-0.0126485446316171,
-2.47067262482137E-11),.UNSPECIFIED.);
#23696=B_SPLINE_CURVE_WITH_KNOTS('',3,(#153308,#153309,#153310,#153311,
#153312,#153313),.UNSPECIFIED.,.F.,.F.,(4,2,4),(-0.0252968472556989,-0.0126485446070453,
0.),.UNSPECIFIED.);
#23697=B_SPLINE_CURVE_WITH_KNOTS('',3,(#153349,#153350,#153351,#153352,
#153353,#153354),.UNSPECIFIED.,.F.,.F.,(4,2,4),(-0.0252969788338113,-0.0126485446612997,
-3.58097579367112E-11),.UNSPECIFIED.);
#23698=B_SPLINE_CURVE_WITH_KNOTS('',3,(#153390,#153391,#153392,#153393,
#153394,#153395),.UNSPECIFIED.,.F.,.F.,(4,2,4),(-0.0252969664419228,-0.012648544666138,
-3.73045691559604E-11),.UNSPECIFIED.);
#23699=B_SPLINE_CURVE_WITH_KNOTS('',3,(#153431,#153432,#153433,#153434,
#153435,#153436),.UNSPECIFIED.,.F.,.F.,(4,2,4),(-0.0252968473797348,-0.0126485446073801,
-2.24880981891662E-11),.UNSPECIFIED.);
#23700=B_SPLINE_CURVE_WITH_KNOTS('',3,(#153472,#153473,#153474,#153475,
#153476,#153477),.UNSPECIFIED.,.F.,.F.,(4,2,4),(-0.0252968473839868,-0.0126485445770089,
0.),.UNSPECIFIED.);
#23701=B_SPLINE_CURVE_WITH_KNOTS('',3,(#153513,#153514,#153515,#153516,
#153517,#153518),.UNSPECIFIED.,.F.,.F.,(4,2,4),(-0.0252968472873195,-0.0126485445945012,
-1.47688701546134E-11),.UNSPECIFIED.);
#23702=B_SPLINE_CURVE_WITH_KNOTS('',3,(#153554,#153555,#153556,#153557,
#153558,#153559),.UNSPECIFIED.,.F.,.F.,(4,2,4),(-0.0252969824708076,-0.0126485446988715,
-7.00456255497972E-11),.UNSPECIFIED.);
#23703=B_SPLINE_CURVE_WITH_KNOTS('',3,(#153595,#153596,#153597,#153598,
#153599,#153600),.UNSPECIFIED.,.F.,.F.,(4,2,4),(-0.0252968472865847,-0.0126485446264394,
-2.50634790699422E-11),.UNSPECIFIED.);
#23704=B_SPLINE_CURVE_WITH_KNOTS('',3,(#153636,#153637,#153638,#153639,
#153640,#153641),.UNSPECIFIED.,.F.,.F.,(4,2,4),(-0.0252969705196494,-0.012648544669824,
-3.72970924977789E-11),.UNSPECIFIED.);
#23705=B_SPLINE_CURVE_WITH_KNOTS('',3,(#153691,#153692,#153693,#153694,
#153695,#153696),.UNSPECIFIED.,.F.,.F.,(4,2,4),(0.,0.0141859771214826,0.0270902355424121),
 .UNSPECIFIED.);
#23706=B_SPLINE_CURVE_WITH_KNOTS('',3,(#153698,#153699,#153700,#153701,
#153702,#153703),.UNSPECIFIED.,.F.,.F.,(4,2,4),(0.000841213375608474,0.0328420548602157,
0.0646443104438985),.UNSPECIFIED.);
#23707=B_SPLINE_CURVE_WITH_KNOTS('',3,(#153717,#153718,#153719,#153720,
#153721,#153722),.UNSPECIFIED.,.F.,.F.,(4,2,4),(0.,0.0322203315702454,0.0646290661358398),
 .UNSPECIFIED.);
#23708=B_SPLINE_CURVE_WITH_KNOTS('',3,(#153723,#153724,#153725,#153726,
#153727,#153728),.UNSPECIFIED.,.F.,.F.,(4,2,4),(-0.0270903064616207,-0.014186058870529,
0.),.UNSPECIFIED.);
#23709=B_SPLINE_CURVE_WITH_KNOTS('',3,(#153731,#153732,#153733,#153734,
#153735,#153736,#153737,#153738),.UNSPECIFIED.,.F.,.F.,(4,2,2,4),(1.00000000424066E-6,
0.032117316005638,0.0481218021713528,0.0656773383786918),.UNSPECIFIED.);
#23710=B_SPLINE_CURVE_WITH_KNOTS('',3,(#153740,#153741,#153742,#153743,
#153744,#153745,#153746,#153747),.UNSPECIFIED.,.F.,.F.,(4,2,2,4),(1.00008813714387E-6,
0.0149899305188782,0.0288003387031098,0.056524442103007),.UNSPECIFIED.);
#23711=B_SPLINE_CURVE_WITH_KNOTS('',3,(#153748,#153749,#153750,#153751,
#153752,#153753),.UNSPECIFIED.,.F.,.F.,(4,2,4),(0.000841212496343715,0.0328420540155859,
0.0646443074565014),.UNSPECIFIED.);
#23712=B_SPLINE_CURVE_WITH_KNOTS('',3,(#153776,#153777,#153778,#153779,
#153780,#153781),.UNSPECIFIED.,.F.,.F.,(4,2,4),(0.,0.0322203314085649,0.0646290655094404),
 .UNSPECIFIED.);
#23713=B_SPLINE_CURVE_WITH_KNOTS('',3,(#153782,#153783,#153784,#153785,
#153786,#153787),.UNSPECIFIED.,.F.,.F.,(4,2,4),(-0.0270903064315289,-0.0141860587887412,
0.),.UNSPECIFIED.);
#23714=B_SPLINE_CURVE_WITH_KNOTS('',3,(#153790,#153791,#153792,#153793,
#153794,#153795,#153796,#153797),.UNSPECIFIED.,.F.,.F.,(4,2,2,4),(1.00000000422679E-6,
0.0321173159964771,0.0481218021303975,0.0656773382668063),.UNSPECIFIED.);
#23715=B_SPLINE_CURVE_WITH_KNOTS('',3,(#153799,#153800,#153801,#153802,
#153803,#153804,#153805,#153806),.UNSPECIFIED.,.F.,.F.,(4,2,2,4),(1.00015504287392E-6,
0.0149898933241323,0.028800226478695,0.0565241789207558),.UNSPECIFIED.);
#23716=B_SPLINE_CURVE_WITH_KNOTS('',3,(#153807,#153808,#153809,#153810,
#153811,#153812),.UNSPECIFIED.,.F.,.F.,(4,2,4),(0.000841212499847193,0.0328420540711237,
0.0646443098284148),.UNSPECIFIED.);
#23717=B_SPLINE_CURVE_WITH_KNOTS('',3,(#153835,#153836,#153837,#153838,
#153839,#153840),.UNSPECIFIED.,.F.,.F.,(4,2,4),(0.,0.0322203310170438,0.0646290639830013),
 .UNSPECIFIED.);
#23718=B_SPLINE_CURVE_WITH_KNOTS('',3,(#153841,#153842,#153843,#153844,
#153845,#153846),.UNSPECIFIED.,.F.,.F.,(4,2,4),(-0.0270903065350147,-0.0141860589225805,
0.),.UNSPECIFIED.);
#23719=B_SPLINE_CURVE_WITH_KNOTS('',3,(#153849,#153850,#153851,#153852,
#153853,#153854,#153855,#153856),.UNSPECIFIED.,.F.,.F.,(4,2,2,4),(1.00000000426148E-6,
0.0321173161023142,0.0481218022823433,0.0656773384116248),.UNSPECIFIED.);
#23720=B_SPLINE_CURVE_WITH_KNOTS('',3,(#153858,#153859,#153860,#153861,
#153862,#153863,#153864,#153865),.UNSPECIFIED.,.F.,.F.,(4,2,2,4),(1.00011528535774E-6,
0.014989896815884,0.0288002355221683,0.0565241993123861),.UNSPECIFIED.);
#23721=B_SPLINE_CURVE_WITH_KNOTS('',3,(#153866,#153867,#153868,#153869,
#153870,#153871),.UNSPECIFIED.,.F.,.F.,(4,2,4),(0.000841212480934865,0.032842054020484,
0.0646443080313221),.UNSPECIFIED.);
#23722=B_SPLINE_CURVE_WITH_KNOTS('',3,(#153894,#153895,#153896,#153897,
#153898,#153899),.UNSPECIFIED.,.F.,.F.,(4,2,4),(0.,0.0322203315669168,0.0646290661501098),
 .UNSPECIFIED.);
#23723=B_SPLINE_CURVE_WITH_KNOTS('',3,(#153900,#153901,#153902,#153903,
#153904,#153905),.UNSPECIFIED.,.F.,.F.,(4,2,4),(-0.0270903064252968,-0.0141860587916916,
0.),.UNSPECIFIED.);
#23724=B_SPLINE_CURVE_WITH_KNOTS('',3,(#153908,#153909,#153910,#153911,
#153912,#153913,#153914,#153915),.UNSPECIFIED.,.F.,.F.,(4,2,2,4),(1.00000000436556E-6,
0.0321173160280198,0.0481218021977914,0.0656773383565895),.UNSPECIFIED.);
#23725=B_SPLINE_CURVE_WITH_KNOTS('',3,(#153917,#153918,#153919,#153920,
#153921,#153922,#153923,#153924),.UNSPECIFIED.,.F.,.F.,(4,2,2,4),(1.00011613791014E-6,
0.0149899423335993,0.0288003757402801,0.0565245295965229),.UNSPECIFIED.);
#23726=B_SPLINE_CURVE_WITH_KNOTS('',3,(#153925,#153926,#153927,#153928,
#153929,#153930),.UNSPECIFIED.,.F.,.F.,(4,2,4),(0.00084121251482112,0.0328420540437307,
0.0646443075511192),.UNSPECIFIED.);
#23727=B_SPLINE_CURVE_WITH_KNOTS('',3,(#153953,#153954,#153955,#153956,
#153957,#153958),.UNSPECIFIED.,.F.,.F.,(4,2,4),(0.,0.0322203311065635,0.0646290643975586),
 .UNSPECIFIED.);
#23728=B_SPLINE_CURVE_WITH_KNOTS('',3,(#153959,#153960,#153961,#153962,
#153963,#153964),.UNSPECIFIED.,.F.,.F.,(4,2,4),(-0.0270903064149145,-0.0141860587690414,
0.),.UNSPECIFIED.);
#23729=B_SPLINE_CURVE_WITH_KNOTS('',3,(#153967,#153968,#153969,#153970,
#153971,#153972,#153973,#153974),.UNSPECIFIED.,.F.,.F.,(4,2,2,4),(1.00000000421291E-6,
0.0321173160083687,0.0481218021505993,0.0656773382163755),.UNSPECIFIED.);
#23730=B_SPLINE_CURVE_WITH_KNOTS('',3,(#153976,#153977,#153978,#153979,
#153980,#153981,#153982,#153983),.UNSPECIFIED.,.F.,.F.,(4,2,2,4),(1.0001428935229E-6,
0.0149898839800048,0.0288001961576573,0.0565241066066853),.UNSPECIFIED.);
#23731=B_SPLINE_CURVE_WITH_KNOTS('',3,(#153984,#153985,#153986,#153987,
#153988,#153989),.UNSPECIFIED.,.F.,.F.,(4,2,4),(0.000841212502526919,0.0328420540695526,
0.0646443094065842),.UNSPECIFIED.);
#23732=B_SPLINE_CURVE_WITH_KNOTS('',3,(#154012,#154013,#154014,#154015,
#154016,#154017),.UNSPECIFIED.,.F.,.F.,(4,2,4),(0.,0.0322203309313174,0.0646290637295966),
 .UNSPECIFIED.);
#23733=B_SPLINE_CURVE_WITH_KNOTS('',3,(#154018,#154019,#154020,#154021,
#154022,#154023),.UNSPECIFIED.,.F.,.F.,(4,2,4),(-0.0270903064312433,-0.0141860588372105,
0.),.UNSPECIFIED.);
#23734=B_SPLINE_CURVE_WITH_KNOTS('',3,(#154026,#154027,#154028,#154029,
#154030,#154031,#154032,#154033),.UNSPECIFIED.,.F.,.F.,(4,2,2,4),(1.00000000408107E-6,
0.0321173160914473,0.0481218022691526,0.06567733839924),.UNSPECIFIED.);
#23735=B_SPLINE_CURVE_WITH_KNOTS('',3,(#154035,#154036,#154037,#154038,
#154039,#154040,#154041,#154042),.UNSPECIFIED.,.F.,.F.,(4,2,2,4),(1.00014860399301E-6,
0.0149899446057504,0.0288003809775306,0.0565245409726297),.UNSPECIFIED.);
#23736=B_SPLINE_CURVE_WITH_KNOTS('',3,(#154043,#154044,#154045,#154046,
#154047,#154048),.UNSPECIFIED.,.F.,.F.,(4,2,4),(0.000841212512306117,0.0328420540410832,
0.0646443079873795),.UNSPECIFIED.);
#23737=B_SPLINE_CURVE_WITH_KNOTS('',3,(#154071,#154072,#154073,#154074,
#154075,#154076),.UNSPECIFIED.,.F.,.F.,(4,2,4),(0.,0.0322203316998426,0.0646290664672489),
 .UNSPECIFIED.);
#23738=B_SPLINE_CURVE_WITH_KNOTS('',3,(#154077,#154078,#154079,#154080,
#154081,#154082),.UNSPECIFIED.,.F.,.F.,(4,2,4),(-0.0270903064584401,-0.0141860588669718,
0.),.UNSPECIFIED.);
#23739=B_SPLINE_CURVE_WITH_KNOTS('',3,(#154085,#154086,#154087,#154088,
#154089,#154090,#154091,#154092),.UNSPECIFIED.,.F.,.F.,(4,2,2,4),(1.00000000417821E-6,
0.0321173160331573,0.0481218022107658,0.0656773383904979),.UNSPECIFIED.);
#23740=B_SPLINE_CURVE_WITH_KNOTS('',3,(#154094,#154095,#154096,#154097,
#154098,#154099,#154100,#154101),.UNSPECIFIED.,.F.,.F.,(4,2,2,4),(1.00017459187543E-6,
0.0149899208702244,0.0288003107957597,0.0565243773111484),.UNSPECIFIED.);
#23741=B_SPLINE_CURVE_WITH_KNOTS('',3,(#154102,#154103,#154104,#154105,
#154106,#154107),.UNSPECIFIED.,.F.,.F.,(4,2,4),(0.000841212498535907,0.0328420540394922,
0.0646443082333259),.UNSPECIFIED.);
#23742=B_SPLINE_CURVE_WITH_KNOTS('',3,(#154130,#154131,#154132,#154133,
#154134,#154135),.UNSPECIFIED.,.F.,.F.,(4,2,4),(0.,0.0322203315803248,0.0646290661264063),
 .UNSPECIFIED.);
#23743=B_SPLINE_CURVE_WITH_KNOTS('',3,(#154136,#154137,#154138,#154139,
#154140,#154141),.UNSPECIFIED.,.F.,.F.,(4,2,4),(-0.0270903065107537,-0.0141860588988156,
0.),.UNSPECIFIED.);
#23744=B_SPLINE_CURVE_WITH_KNOTS('',3,(#154144,#154145,#154146,#154147,
#154148,#154149,#154150,#154151),.UNSPECIFIED.,.F.,.F.,(4,2,2,4),(1.00000000423373E-6,
0.0321173160269704,0.048121802160199,0.0656773383201519),.UNSPECIFIED.);
#23745=B_SPLINE_CURVE_WITH_KNOTS('',3,(#154153,#154154,#154155,#154156,
#154157,#154158,#154159,#154160),.UNSPECIFIED.,.F.,.F.,(4,2,2,4),(1.00013892581745E-6,
0.0149899181546202,0.0288003020884492,0.0565243566919721),.UNSPECIFIED.);
#23746=B_SPLINE_CURVE_WITH_KNOTS('',3,(#154161,#154162,#154163,#154164,
#154165,#154166),.UNSPECIFIED.,.F.,.F.,(4,2,4),(0.000841212508110519,0.0328420540551423,
0.0646443085644263),.UNSPECIFIED.);
#23747=B_SPLINE_CURVE_WITH_KNOTS('',3,(#154189,#154190,#154191,#154192,
#154193,#154194),.UNSPECIFIED.,.F.,.F.,(4,2,4),(0.,0.0322203310983203,0.0646290643108364),
 .UNSPECIFIED.);
#23748=B_SPLINE_CURVE_WITH_KNOTS('',3,(#154195,#154196,#154197,#154198,
#154199,#154200),.UNSPECIFIED.,.F.,.F.,(4,2,4),(-0.0270903065126501,-0.0141860589068631,
0.),.UNSPECIFIED.);
#23749=B_SPLINE_CURVE_WITH_KNOTS('',3,(#154203,#154204,#154205,#154206,
#154207,#154208,#154209,#154210),.UNSPECIFIED.,.F.,.F.,(4,2,2,4),(1.00000000422679E-6,
0.0321173160957739,0.0481218023156141,0.0656773385260134),.UNSPECIFIED.);
#23750=B_SPLINE_CURVE_WITH_KNOTS('',3,(#154212,#154213,#154214,#154215,
#154216,#154217,#154218,#154219),.UNSPECIFIED.,.F.,.F.,(4,2,2,4),(1.00012353586113E-6,
0.0149899334156635,0.0288003481710984,0.0565244646056971),.UNSPECIFIED.);
#23751=B_SPLINE_CURVE_WITH_KNOTS('',3,(#154220,#154221,#154222,#154223,
#154224,#154225),.UNSPECIFIED.,.F.,.F.,(4,2,4),(0.000841212516248009,0.0328420540304007,
0.0646443083551271),.UNSPECIFIED.);
#23752=B_SPLINE_CURVE_WITH_KNOTS('',3,(#154248,#154249,#154250,#154251,
#154252,#154253),.UNSPECIFIED.,.F.,.F.,(4,2,4),(0.,0.0322203320530467,0.0646290679305432),
 .UNSPECIFIED.);
#23753=B_SPLINE_CURVE_WITH_KNOTS('',3,(#154254,#154255,#154256,#154257,
#154258,#154259),.UNSPECIFIED.,.F.,.F.,(4,2,4),(-0.0270903065054314,-0.0141860589103654,
0.),.UNSPECIFIED.);
#23754=B_SPLINE_CURVE_WITH_KNOTS('',3,(#154262,#154263,#154264,#154265,
#154266,#154267,#154268,#154269),.UNSPECIFIED.,.F.,.F.,(4,2,2,4),(1.00000000442801E-6,
0.032117316028803,0.0481218021765062,0.0656773384184277),.UNSPECIFIED.);
#23755=B_SPLINE_CURVE_WITH_KNOTS('',3,(#154271,#154272,#154273,#154274,
#154275,#154276,#154277,#154278),.UNSPECIFIED.,.F.,.F.,(4,2,2,4),(1.00016980558116E-6,
0.014989959175291,0.0288004270714822,0.0565246501588951),.UNSPECIFIED.);
#23756=B_SPLINE_CURVE_WITH_KNOTS('',3,(#154279,#154280,#154281,#154282,
#154283,#154284),.UNSPECIFIED.,.F.,.F.,(4,2,4),(0.000841212498799183,0.0328420540437319,
0.064644307927571),.UNSPECIFIED.);
#23757=B_SPLINE_CURVE_WITH_KNOTS('',3,(#154307,#154308,#154309,#154310,
#154311,#154312),.UNSPECIFIED.,.F.,.F.,(4,2,4),(0.,0.0322203314745356,0.0646290658004266),
 .UNSPECIFIED.);
#23758=B_SPLINE_CURVE_WITH_KNOTS('',3,(#154313,#154314,#154315,#154316,
#154317,#154318),.UNSPECIFIED.,.F.,.F.,(4,2,4),(-0.0270903064921837,-0.0141860588757323,
0.),.UNSPECIFIED.);
#23759=B_SPLINE_CURVE_WITH_KNOTS('',3,(#154321,#154322,#154323,#154324,
#154325,#154326,#154327,#154328),.UNSPECIFIED.,.F.,.F.,(4,2,2,4),(1.00000000403944E-6,
0.0321173159942312,0.0481218021528757,0.0656773383460366),.UNSPECIFIED.);
#23760=B_SPLINE_CURVE_WITH_KNOTS('',3,(#154330,#154331,#154332,#154333,
#154334,#154335,#154336,#154337),.UNSPECIFIED.,.F.,.F.,(4,2,2,4),(1.00021693869851E-6,
0.0149899233812258,0.0288003179063593,0.0565243937091347),.UNSPECIFIED.);
#23761=B_SPLINE_CURVE_WITH_KNOTS('',3,(#154338,#154339,#154340,#154341,
#154342,#154343),.UNSPECIFIED.,.F.,.F.,(4,2,4),(0.000841212519676827,0.0328420540777682,
0.0646443087952493),.UNSPECIFIED.);
#23762=B_SPLINE_CURVE_WITH_KNOTS('',3,(#154366,#154367,#154368,#154369,
#154370,#154371),.UNSPECIFIED.,.F.,.F.,(4,2,4),(0.,0.032220330961457,0.0646290638718947),
 .UNSPECIFIED.);
#23763=B_SPLINE_CURVE_WITH_KNOTS('',3,(#154372,#154373,#154374,#154375,
#154376,#154377),.UNSPECIFIED.,.F.,.F.,(4,2,4),(-0.0270903064237865,-0.0141860588161846,
0.),.UNSPECIFIED.);
#23764=B_SPLINE_CURVE_WITH_KNOTS('',3,(#154380,#154381,#154382,#154383,
#154384,#154385,#154386,#154387),.UNSPECIFIED.,.F.,.F.,(4,2,2,4),(1.00000000397005E-6,
0.0321173160729806,0.0481218022715349,0.0656773384478732),.UNSPECIFIED.);
#23765=B_SPLINE_CURVE_WITH_KNOTS('',3,(#154389,#154390,#154391,#154392,
#154393,#154394,#154395,#154396),.UNSPECIFIED.,.F.,.F.,(4,2,2,4),(1.00015850917621E-6,
0.0149899557945825,0.0288004171433498,0.0565246271762989),.UNSPECIFIED.);
#23766=B_SPLINE_CURVE_WITH_KNOTS('',3,(#154397,#154398,#154399,#154400,
#154401,#154402),.UNSPECIFIED.,.F.,.F.,(4,2,4),(0.000841212520024779,0.0328420540605427,
0.0646443083686256),.UNSPECIFIED.);
#23767=B_SPLINE_CURVE_WITH_KNOTS('',3,(#154425,#154426,#154427,#154428,
#154429,#154430),.UNSPECIFIED.,.F.,.F.,(4,2,4),(0.,0.0322203316707932,0.0646290665533952),
 .UNSPECIFIED.);
#23768=B_SPLINE_CURVE_WITH_KNOTS('',3,(#154431,#154432,#154433,#154434,
#154435,#154436),.UNSPECIFIED.,.F.,.F.,(4,2,4),(-0.0270903063691943,-0.0141860587297742,
0.),.UNSPECIFIED.);
#23769=B_SPLINE_CURVE_WITH_KNOTS('',3,(#154439,#154440,#154441,#154442,
#154443,#154444,#154445,#154446),.UNSPECIFIED.,.F.,.F.,(4,2,2,4),(1.00000000397699E-6,
0.0321173160397508,0.0481218022104113,0.0656773383873906),.UNSPECIFIED.);
#23770=B_SPLINE_CURVE_WITH_KNOTS('',3,(#154448,#154449,#154450,#154451,
#154452,#154453,#154454,#154455),.UNSPECIFIED.,.F.,.F.,(4,2,2,4),(1.00009241193544E-6,
0.0149899114490231,0.0288002806104871,0.0565243055933151),.UNSPECIFIED.);
#23771=B_SPLINE_CURVE_WITH_KNOTS('',3,(#154456,#154457,#154458,#154459,
#154460,#154461),.UNSPECIFIED.,.F.,.F.,(4,2,4),(0.000841212507969122,0.0328420540427537,
0.0646443075038919),.UNSPECIFIED.);
#23772=B_SPLINE_CURVE_WITH_KNOTS('',3,(#154482,#154483,#154484,#154485,
#154486,#154487),.UNSPECIFIED.,.F.,.F.,(4,2,4),(-0.027090306535355,-0.0141860588953685,
0.),.UNSPECIFIED.);
#23773=B_SPLINE_CURVE_WITH_KNOTS('',3,(#154510,#154511,#154512,#154513,
#154514,#154515),.UNSPECIFIED.,.F.,.F.,(4,2,4),(0.,0.0322203315533029,0.0646290660316353),
 .UNSPECIFIED.);
#23774=B_SPLINE_CURVE_WITH_KNOTS('',3,(#154516,#154517,#154518,#154519,
#154520,#154521),.UNSPECIFIED.,.F.,.F.,(4,2,4),(-0.0270903064994476,-0.0141860588902063,
0.),.UNSPECIFIED.);
#23775=B_SPLINE_CURVE_WITH_KNOTS('',3,(#154524,#154525,#154526,#154527,
#154528,#154529,#154530,#154531),.UNSPECIFIED.,.F.,.F.,(4,2,2,4),(1.00000000449046E-6,
0.0321173160115672,0.0481218021634407,0.0656773383366627),.UNSPECIFIED.);
#23776=B_SPLINE_CURVE_WITH_KNOTS('',3,(#154533,#154534,#154535,#154536,
#154537,#154538,#154539,#154540),.UNSPECIFIED.,.F.,.F.,(4,2,2,4),(1.00012267353931E-6,
0.0149899195388564,0.0288003053841497,0.0565243637255748),.UNSPECIFIED.);
#23777=B_SPLINE_CURVE_WITH_KNOTS('',3,(#154541,#154542,#154543,#154544,
#154545,#154546),.UNSPECIFIED.,.F.,.F.,(4,2,4),(0.000841212515697555,0.0328420540675755,
0.0646443081941838),.UNSPECIFIED.);
#23778=B_SPLINE_CURVE_WITH_KNOTS('',3,(#154569,#154570,#154571,#154572,
#154573,#154574),.UNSPECIFIED.,.F.,.F.,(4,2,4),(0.,0.0322203311701331,0.0646290645652637),
 .UNSPECIFIED.);
#23779=B_SPLINE_CURVE_WITH_KNOTS('',3,(#154575,#154576,#154577,#154578,
#154579,#154580),.UNSPECIFIED.,.F.,.F.,(4,2,4),(-0.0270903064750334,-0.0141860588293611,
0.),.UNSPECIFIED.);
#23780=B_SPLINE_CURVE_WITH_KNOTS('',3,(#154583,#154584,#154585,#154586,
#154587,#154588,#154589,#154590),.UNSPECIFIED.,.F.,.F.,(4,2,2,4),(1.00000000401862E-6,
0.0321173161163047,0.048121802319759,0.0656773384844766),.UNSPECIFIED.);
#23781=B_SPLINE_CURVE_WITH_KNOTS('',3,(#154592,#154593,#154594,#154595,
#154596,#154597,#154598,#154599),.UNSPECIFIED.,.F.,.F.,(4,2,2,4),(1.00012621567518E-6,
0.0149899307663365,0.028800340737718,0.0565244474880159),.UNSPECIFIED.);
#23782=B_SPLINE_CURVE_WITH_KNOTS('',3,(#154600,#154601,#154602,#154603,
#154604,#154605),.UNSPECIFIED.,.F.,.F.,(4,2,4),(0.000841212510412574,0.0328420540605121,
0.06464430886662),.UNSPECIFIED.);
#23783=B_SPLINE_CURVE_WITH_KNOTS('',3,(#154628,#154629,#154630,#154631,
#154632,#154633),.UNSPECIFIED.,.F.,.F.,(4,2,4),(0.,0.0322203316658832,0.0646290665311863),
 .UNSPECIFIED.);
#23784=B_SPLINE_CURVE_WITH_KNOTS('',3,(#154634,#154635,#154636,#154637,
#154638,#154639),.UNSPECIFIED.,.F.,.F.,(4,2,4),(-0.0270903064362176,-0.0141860588055876,
0.),.UNSPECIFIED.);
#23785=B_SPLINE_CURVE_WITH_KNOTS('',3,(#154642,#154643,#154644,#154645,
#154646,#154647,#154648,#154649),.UNSPECIFIED.,.F.,.F.,(4,2,2,4),(1.00000000410883E-6,
0.0321173160026744,0.0481218021569424,0.0656773383825617),.UNSPECIFIED.);
#23786=B_SPLINE_CURVE_WITH_KNOTS('',3,(#154651,#154652,#154653,#154654,
#154655,#154656,#154657,#154658),.UNSPECIFIED.,.F.,.F.,(4,2,2,4),(1.00011248478266E-6,
0.0149899105681496,0.028800278824881,0.056524301870037),.UNSPECIFIED.);
#23787=B_SPLINE_CURVE_WITH_KNOTS('',3,(#154659,#154660,#154661,#154662,
#154663,#154664),.UNSPECIFIED.,.F.,.F.,(4,2,4),(0.000841212512084421,0.0328420540328582,
0.0646443087371659),.UNSPECIFIED.);
#23788=B_SPLINE_CURVE_WITH_KNOTS('',3,(#154687,#154688,#154689,#154690,
#154691,#154692),.UNSPECIFIED.,.F.,.F.,(4,2,4),(0.,0.032220331299064,0.0646290651252309),
 .UNSPECIFIED.);
#23789=B_SPLINE_CURVE_WITH_KNOTS('',3,(#154693,#154694,#154695,#154696,
#154697,#154698),.UNSPECIFIED.,.F.,.F.,(4,2,4),(-0.0270903064032475,-0.0141860587633634,
0.),.UNSPECIFIED.);
#23790=B_SPLINE_CURVE_WITH_KNOTS('',3,(#154701,#154702,#154703,#154704,
#154705,#154706,#154707,#154708),.UNSPECIFIED.,.F.,.F.,(4,2,2,4),(1.00000000391454E-6,
0.0321173160046967,0.0481218021440837,0.0656773382680278),.UNSPECIFIED.);
#23791=B_SPLINE_CURVE_WITH_KNOTS('',3,(#154710,#154711,#154712,#154713,
#154714,#154715,#154716,#154717),.UNSPECIFIED.,.F.,.F.,(4,2,2,4),(1.00012376496616E-6,
0.0149899403925003,0.0288003683844058,0.0565245115545341),.UNSPECIFIED.);
#23792=B_SPLINE_CURVE_WITH_KNOTS('',3,(#154718,#154719,#154720,#154721,
#154722,#154723),.UNSPECIFIED.,.F.,.F.,(4,2,4),(0.00084121251706062,0.0328420540537706,
0.0646443079811129),.UNSPECIFIED.);
#23793=B_SPLINE_CURVE_WITH_KNOTS('',3,(#154746,#154747,#154748,#154749,
#154750,#154751),.UNSPECIFIED.,.F.,.F.,(4,2,4),(0.,0.0322203309785123,0.0646290639103093),
 .UNSPECIFIED.);
#23794=B_SPLINE_CURVE_WITH_KNOTS('',3,(#154752,#154753,#154754,#154755,
#154756,#154757),.UNSPECIFIED.,.F.,.F.,(4,2,4),(-0.0270903065056521,-0.0141860588741511,
0.),.UNSPECIFIED.);
#23795=B_SPLINE_CURVE_WITH_KNOTS('',3,(#154760,#154761,#154762,#154763,
#154764,#154765,#154766,#154767),.UNSPECIFIED.,.F.,.F.,(4,2,2,4),(1.00000000425454E-6,
0.0321173160975012,0.0481218022746217,0.065677338421128),.UNSPECIFIED.);
#23796=B_SPLINE_CURVE_WITH_KNOTS('',3,(#154769,#154770,#154771,#154772,
#154773,#154774,#154775,#154776),.UNSPECIFIED.,.F.,.F.,(4,2,2,4),(1.00015136715194E-6,
0.0149899861205894,0.02880050974179,0.0565248447377549),.UNSPECIFIED.);
#23797=B_SPLINE_CURVE_WITH_KNOTS('',3,(#154777,#154778,#154779,#154780,
#154781,#154782),.UNSPECIFIED.,.F.,.F.,(4,2,4),(0.000841212514893795,0.0328420540828173,
0.0646443082401466),.UNSPECIFIED.);
#23798=B_SPLINE_CURVE_WITH_KNOTS('',3,(#154805,#154806,#154807,#154808,
#154809,#154810),.UNSPECIFIED.,.F.,.F.,(4,2,4),(0.,0.0322203316164535,0.0646290663521486),
 .UNSPECIFIED.);
#23799=B_SPLINE_CURVE_WITH_KNOTS('',3,(#154811,#154812,#154813,#154814,
#154815,#154816),.UNSPECIFIED.,.F.,.F.,(4,2,4),(-0.027090306440936,-0.0141860588197551,
0.),.UNSPECIFIED.);
#23800=B_SPLINE_CURVE_WITH_KNOTS('',3,(#154819,#154820,#154821,#154822,
#154823,#154824,#154825,#154826),.UNSPECIFIED.,.F.,.F.,(4,2,2,4),(1.0000000041574E-6,
0.0321173160398495,0.0481218021954762,0.0656773384252558),.UNSPECIFIED.);
#23801=B_SPLINE_CURVE_WITH_KNOTS('',3,(#154828,#154829,#154830,#154831,
#154832,#154833,#154834,#154835),.UNSPECIFIED.,.F.,.F.,(4,2,2,4),(1.00008869019263E-6,
0.0149899304634008,0.0288003394410968,0.0565244443100335),.UNSPECIFIED.);
#23802=B_SPLINE_CURVE_WITH_KNOTS('',3,(#154836,#154837,#154838,#154839,
#154840,#154841),.UNSPECIFIED.,.F.,.F.,(4,2,4),(0.000841212512502353,0.0328420540374941,
0.0646443074408672),.UNSPECIFIED.);
#23803=B_SPLINE_CURVE_WITH_KNOTS('',3,(#154862,#154863,#154864,#154865,
#154866,#154867),.UNSPECIFIED.,.F.,.F.,(4,2,4),(-0.0270903064711485,-0.0141860588564947,
0.),.UNSPECIFIED.);
#23804=B_SPLINE_CURVE_WITH_KNOTS('',3,(#154890,#154891,#154892,#154893,
#154894,#154895),.UNSPECIFIED.,.F.,.F.,(4,2,4),(0.,0.032220331040302,0.0646290641347894),
 .UNSPECIFIED.);
#23805=B_SPLINE_CURVE_WITH_KNOTS('',3,(#154896,#154897,#154898,#154899,
#154900,#154901),.UNSPECIFIED.,.F.,.F.,(4,2,4),(-0.02709030651203,-0.0141860588716743,
0.),.UNSPECIFIED.);
#23806=B_SPLINE_CURVE_WITH_KNOTS('',3,(#154904,#154905,#154906,#154907,
#154908,#154909,#154910,#154911),.UNSPECIFIED.,.F.,.F.,(4,2,2,4),(9.9998998204146E-7,
0.0321173159898052,0.0481218021226243,0.0656773382297077),.UNSPECIFIED.);
#23807=B_SPLINE_CURVE_WITH_KNOTS('',3,(#154913,#154914,#154915,#154916,
#154917,#154918,#154919,#154920),.UNSPECIFIED.,.F.,.F.,(4,2,2,4),(1.00012131849139E-6,
0.0149901622886091,0.0288007887685852,0.0565244707711353),.UNSPECIFIED.);
#23808=B_SPLINE_CURVE_WITH_KNOTS('',3,(#154921,#154922,#154923,#154924,
#154925,#154926),.UNSPECIFIED.,.F.,.F.,(4,2,4),(0.00084121252107635,0.03284205406008,
0.0646443081956264),.UNSPECIFIED.);
#23809=B_SPLINE_CURVE_WITH_KNOTS('',3,(#154949,#154950,#154951,#154952,
#154953,#154954),.UNSPECIFIED.,.F.,.F.,(4,2,4),(0.,0.0322203319709312,0.0646290676419014),
 .UNSPECIFIED.);
#23810=B_SPLINE_CURVE_WITH_KNOTS('',3,(#154955,#154956,#154957,#154958,
#154959,#154960),.UNSPECIFIED.,.F.,.F.,(4,2,4),(-0.027090306419541,-0.0141860588100847,
0.),.UNSPECIFIED.);
#23811=B_SPLINE_CURVE_WITH_KNOTS('',3,(#154963,#154964,#154965,#154966,
#154967,#154968,#154969,#154970),.UNSPECIFIED.,.F.,.F.,(4,2,2,4),(1.00000000395617E-6,
0.0321173160087043,0.0481218021580067,0.0656773383989004),.UNSPECIFIED.);
#23812=B_SPLINE_CURVE_WITH_KNOTS('',3,(#154972,#154973,#154974,#154975,
#154976,#154977,#154978,#154979),.UNSPECIFIED.,.F.,.F.,(4,2,2,4),(1.00009951607972E-6,
0.0149899106455396,0.0288002790811247,0.0565243023502256),.UNSPECIFIED.);
#23813=B_SPLINE_CURVE_WITH_KNOTS('',3,(#154980,#154981,#154982,#154983,
#154984,#154985),.UNSPECIFIED.,.F.,.F.,(4,2,4),(0.000841212510310441,0.0328420540544761,
0.0646443082224731),.UNSPECIFIED.);
#23814=B_SPLINE_CURVE_WITH_KNOTS('',3,(#155008,#155009,#155010,#155011,
#155012,#155013),.UNSPECIFIED.,.F.,.F.,(4,2,4),(0.,0.0322203315633675,0.0646290661052855),
 .UNSPECIFIED.);
#23815=B_SPLINE_CURVE_WITH_KNOTS('',3,(#155014,#155015,#155016,#155017,
#155018,#155019),.UNSPECIFIED.,.F.,.F.,(4,2,4),(-0.0270903063858845,-0.0141860587941446,
0.),.UNSPECIFIED.);
#23816=B_SPLINE_CURVE_WITH_KNOTS('',3,(#155022,#155023,#155024,#155025,
#155026,#155027,#155028,#155029),.UNSPECIFIED.,.F.,.F.,(4,2,2,4),(1.00000000446965E-6,
0.0321173160234447,0.0481218021637841,0.0656773383422308),.UNSPECIFIED.);
#23817=B_SPLINE_CURVE_WITH_KNOTS('',3,(#155031,#155032,#155033,#155034,
#155035,#155036,#155037,#155038),.UNSPECIFIED.,.F.,.F.,(4,2,2,4),(1.00008421606349E-6,
0.0149899151239748,0.0288002930878146,0.0565243355189921),.UNSPECIFIED.);
#23818=B_SPLINE_CURVE_WITH_KNOTS('',3,(#155039,#155040,#155041,#155042,
#155043,#155044),.UNSPECIFIED.,.F.,.F.,(4,2,4),(0.000841212504543673,0.0328420540215709,
0.0646443077365915),.UNSPECIFIED.);
#23819=B_SPLINE_CURVE_WITH_KNOTS('',3,(#155067,#155068,#155069,#155070,
#155071,#155072),.UNSPECIFIED.,.F.,.F.,(4,2,4),(0.,0.0322203312992352,0.064629065097578),
 .UNSPECIFIED.);
#23820=B_SPLINE_CURVE_WITH_KNOTS('',3,(#155073,#155074,#155075,#155076,
#155077,#155078),.UNSPECIFIED.,.F.,.F.,(4,2,4),(-0.0270903065060037,-0.0141860588797379,
0.),.UNSPECIFIED.);
#23821=B_SPLINE_CURVE_WITH_KNOTS('',3,(#155081,#155082,#155083,#155084,
#155085,#155086,#155087,#155088),.UNSPECIFIED.,.F.,.F.,(4,2,2,4),(9.99989850218092E-7,
0.0321173160019981,0.0481218021363862,0.0656773382328053),.UNSPECIFIED.);
#23822=B_SPLINE_CURVE_WITH_KNOTS('',3,(#155090,#155091,#155092,#155093,
#155094,#155095,#155096,#155097),.UNSPECIFIED.,.F.,.F.,(4,2,2,4),(1.00014836394316E-6,
0.0149901114536482,0.0288006347456497,0.0565241094201872),.UNSPECIFIED.);
#23823=B_SPLINE_CURVE_WITH_KNOTS('',3,(#155098,#155099,#155100,#155101,
#155102,#155103),.UNSPECIFIED.,.F.,.F.,(4,2,4),(0.000841212522281091,0.0328420540517081,
0.0646443095449781),.UNSPECIFIED.);
#23824=B_SPLINE_CURVE_WITH_KNOTS('',3,(#155126,#155127,#155128,#155129,
#155130,#155131),.UNSPECIFIED.,.F.,.F.,(4,2,4),(0.,0.0322203308131721,0.064629063261788),
 .UNSPECIFIED.);
#23825=B_SPLINE_CURVE_WITH_KNOTS('',3,(#155132,#155133,#155134,#155135,
#155136,#155137),.UNSPECIFIED.,.F.,.F.,(4,2,4),(-0.0270903063886443,-0.0141860587785814,
0.),.UNSPECIFIED.);
#23826=B_SPLINE_CURVE_WITH_KNOTS('',3,(#155140,#155141,#155142,#155143,
#155144,#155145,#155146,#155147),.UNSPECIFIED.,.F.,.F.,(4,2,2,4),(1.00000000401168E-6,
0.0321173160581702,0.0481218022453477,0.0656773383503209),.UNSPECIFIED.);
#23827=B_SPLINE_CURVE_WITH_KNOTS('',3,(#155149,#155150,#155151,#155152,
#155153,#155154,#155155,#155156),.UNSPECIFIED.,.F.,.F.,(4,2,2,4),(1.00016934312906E-6,
0.0149899461668579,0.028800386619068,0.0565245547525933),.UNSPECIFIED.);
#23828=B_SPLINE_CURVE_WITH_KNOTS('',3,(#155157,#155158,#155159,#155160,
#155161,#155162),.UNSPECIFIED.,.F.,.F.,(4,2,4),(0.000841212503056033,0.0328420540648736,
0.0646443079179034),.UNSPECIFIED.);
#23829=B_SPLINE_CURVE_WITH_KNOTS('',3,(#155185,#155186,#155187,#155188,
#155189,#155190),.UNSPECIFIED.,.F.,.F.,(4,2,4),(0.,0.0322203317246494,0.0646290666940337),
 .UNSPECIFIED.);
#23830=B_SPLINE_CURVE_WITH_KNOTS('',3,(#155191,#155192,#155193,#155194,
#155195,#155196),.UNSPECIFIED.,.F.,.F.,(4,2,4),(-0.0270903064677105,-0.014186058827064,
0.),.UNSPECIFIED.);
#23831=B_SPLINE_CURVE_WITH_KNOTS('',3,(#155199,#155200,#155201,#155202,
#155203,#155204,#155205,#155206),.UNSPECIFIED.,.F.,.F.,(4,2,2,4),(1.00000000416434E-6,
0.032117316012009,0.048121802177314,0.0656773384064538),.UNSPECIFIED.);
#23832=B_SPLINE_CURVE_WITH_KNOTS('',3,(#155208,#155209,#155210,#155211,
#155212,#155213,#155214,#155215),.UNSPECIFIED.,.F.,.F.,(4,2,2,4),(1.00010778408823E-6,
0.0149898884705105,0.028800211788248,0.0565241445861282),.UNSPECIFIED.);
#23833=B_SPLINE_CURVE_WITH_KNOTS('',3,(#155216,#155217,#155218,#155219,
#155220,#155221),.UNSPECIFIED.,.F.,.F.,(4,2,4),(0.000841212508163703,0.0328420540409334,
0.0646443086155899),.UNSPECIFIED.);
#23834=B_SPLINE_CURVE_WITH_KNOTS('',3,(#155244,#155245,#155246,#155247,
#155248,#155249),.UNSPECIFIED.,.F.,.F.,(4,2,4),(0.,0.0322203309557638,0.0646290638560515),
 .UNSPECIFIED.);
#23835=B_SPLINE_CURVE_WITH_KNOTS('',3,(#155250,#155251,#155252,#155253,
#155254,#155255),.UNSPECIFIED.,.F.,.F.,(4,2,4),(-0.0270903064294424,-0.0141860588345496,
0.),.UNSPECIFIED.);
#23836=B_SPLINE_CURVE_WITH_KNOTS('',3,(#155258,#155259,#155260,#155261,
#155262,#155263,#155264,#155265),.UNSPECIFIED.,.F.,.F.,(4,2,2,4),(1.00000000420597E-6,
0.0321173159670649,0.048121802089453,0.0656773381295942),.UNSPECIFIED.);
#23837=B_SPLINE_CURVE_WITH_KNOTS('',3,(#155267,#155268,#155269,#155270,
#155271,#155272,#155273,#155274),.UNSPECIFIED.,.F.,.F.,(4,2,2,4),(1.00012040405606E-6,
0.0149899472299666,0.028800390838345,0.056524565189487),.UNSPECIFIED.);
#23838=B_SPLINE_CURVE_WITH_KNOTS('',3,(#155275,#155276,#155277,#155278,
#155279,#155280),.UNSPECIFIED.,.F.,.F.,(4,2,4),(0.000841212507813186,0.0328420540587639,
0.0646443079539742),.UNSPECIFIED.);
#23839=B_SPLINE_CURVE_WITH_KNOTS('',3,(#155293,#155294,#155295,#155296,
#155297,#155298),.UNSPECIFIED.,.F.,.F.,(4,2,4),(0.,0.0322203302008996,0.0646290631014971),
 .UNSPECIFIED.);
#23840=B_SPLINE_CURVE_WITH_KNOTS('',3,(#155300,#155301,#155302,#155303,
#155304,#155305,#155306,#155307),.UNSPECIFIED.,.F.,.F.,(4,2,2,4),(1.00000000396311E-6,
0.0321173162056066,0.0481218402735079,0.0656773352685673),.UNSPECIFIED.);
#23841=B_SPLINE_CURVE_WITH_KNOTS('',3,(#155308,#155309,#155310,#155311,
#155312,#155313,#155314,#155315),.UNSPECIFIED.,.F.,.F.,(4,2,2,4),(1.00019596529798E-6,
0.0149905409355991,0.0288008434416931,0.056524563022755),.UNSPECIFIED.);
#23842=B_SPLINE_CURVE_WITH_KNOTS('',3,(#155334,#155335,#155336,#155337,
#155338,#155339),.UNSPECIFIED.,.F.,.F.,(4,2,4),(-0.0253026342524986,-0.0126514544652314,
-1.88668421163829E-11),.UNSPECIFIED.);
#23843=B_SPLINE_CURVE_WITH_KNOTS('',3,(#155348,#155349,#155350,#155351,
#155352,#155353),.UNSPECIFIED.,.F.,.F.,(4,2,4),(0.,0.0126514363600221,0.0253026263497453),
 .UNSPECIFIED.);
#23844=B_SPLINE_CURVE_WITH_KNOTS('',3,(#155369,#155370,#155371,#155372,
#155373,#155374),.UNSPECIFIED.,.F.,.F.,(4,2,4),(3.32128913797922E-11,0.0126514528097758,
0.025302666580165),.UNSPECIFIED.);
#23845=B_SPLINE_CURVE_WITH_KNOTS('',3,(#155390,#155391,#155392,#155393,
#155394,#155395),.UNSPECIFIED.,.F.,.F.,(4,2,4),(2.48238510840293E-11,0.0126514528557191,
0.0253026666422664),.UNSPECIFIED.);
#23846=B_SPLINE_CURVE_WITH_KNOTS('',3,(#155411,#155412,#155413,#155414,
#155415,#155416),.UNSPECIFIED.,.F.,.F.,(4,2,4),(0.,0.0126514361044767,0.0253026254261494),
 .UNSPECIFIED.);
#23847=B_SPLINE_CURVE_WITH_KNOTS('',3,(#155432,#155433,#155434,#155435,
#155436,#155437),.UNSPECIFIED.,.F.,.F.,(4,2,4),(1.78381052840366E-11,0.012651452890063,
0.0253026666624878),.UNSPECIFIED.);
#23848=B_SPLINE_CURVE_WITH_KNOTS('',3,(#155453,#155454,#155455,#155456,
#155457,#155458),.UNSPECIFIED.,.F.,.F.,(4,2,4),(0.,0.0126514377629713,0.0253026295575941),
 .UNSPECIFIED.);
#23849=B_SPLINE_CURVE_WITH_KNOTS('',3,(#155474,#155475,#155476,#155477,
#155478,#155479),.UNSPECIFIED.,.F.,.F.,(4,2,4),(0.,0.0126514375141281,0.0253026290465384),
 .UNSPECIFIED.);
#23850=B_SPLINE_CURVE_WITH_KNOTS('',3,(#155495,#155496,#155497,#155498,
#155499,#155500),.UNSPECIFIED.,.F.,.F.,(4,2,4),(1.86039915567488E-11,0.0126514527918854,
0.0253026665522429),.UNSPECIFIED.);
#23851=B_SPLINE_CURVE_WITH_KNOTS('',3,(#155516,#155517,#155518,#155519,
#155520,#155521),.UNSPECIFIED.,.F.,.F.,(4,2,4),(0.,0.0126514374178867,0.0253026288727294),
 .UNSPECIFIED.);
#23852=B_SPLINE_CURVE_WITH_KNOTS('',3,(#155537,#155538,#155539,#155540,
#155541,#155542),.UNSPECIFIED.,.F.,.F.,(4,2,4),(0.,0.0126514379132605,0.0253026301647806),
 .UNSPECIFIED.);
#23853=B_SPLINE_CURVE_WITH_KNOTS('',3,(#155558,#155559,#155560,#155561,
#155562,#155563),.UNSPECIFIED.,.F.,.F.,(4,2,4),(0.,0.0126514341354231,0.02530262056224),
 .UNSPECIFIED.);
#23854=B_SPLINE_CURVE_WITH_KNOTS('',3,(#155579,#155580,#155581,#155582,
#155583,#155584),.UNSPECIFIED.,.F.,.F.,(4,2,4),(0.,0.0126514348780394,0.025302622573186),
 .UNSPECIFIED.);
#23855=B_SPLINE_CURVE_WITH_KNOTS('',3,(#155600,#155601,#155602,#155603,
#155604,#155605),.UNSPECIFIED.,.F.,.F.,(4,2,4),(0.,0.0126514359812692,0.0253026251414924),
 .UNSPECIFIED.);
#23856=B_SPLINE_CURVE_WITH_KNOTS('',3,(#155621,#155622,#155623,#155624,
#155625,#155626),.UNSPECIFIED.,.F.,.F.,(4,2,4),(2.48627244145729E-11,0.0126514528013674,
0.0253026665766467),.UNSPECIFIED.);
#23857=B_SPLINE_CURVE_WITH_KNOTS('',3,(#155642,#155643,#155644,#155645,
#155646,#155647),.UNSPECIFIED.,.F.,.F.,(4,2,4),(0.,0.0126514360446639,0.0253026253845719),
 .UNSPECIFIED.);
#23858=B_SPLINE_CURVE_WITH_KNOTS('',3,(#155663,#155664,#155665,#155666,
#155667,#155668),.UNSPECIFIED.,.F.,.F.,(4,2,4),(0.,0.0126514360075886,0.0253026253307672),
 .UNSPECIFIED.);
#23859=B_SPLINE_CURVE_WITH_KNOTS('',3,(#155684,#155685,#155686,#155687,
#155688,#155689),.UNSPECIFIED.,.F.,.F.,(4,2,4),(0.,0.0126514352765847,0.0253026235823062),
 .UNSPECIFIED.);
#23860=B_SPLINE_CURVE_WITH_KNOTS('',3,(#155705,#155706,#155707,#155708,
#155709,#155710),.UNSPECIFIED.,.F.,.F.,(4,2,4),(9.20122805263892E-12,0.0126514528186731,
0.025302666610893),.UNSPECIFIED.);
#23861=B_SPLINE_CURVE_WITH_KNOTS('',3,(#155726,#155727,#155728,#155729,
#155730,#155731),.UNSPECIFIED.,.F.,.F.,(4,2,4),(0.,0.0126514380585315,0.0253026303831182),
 .UNSPECIFIED.);
#23862=B_SPLINE_CURVE_WITH_KNOTS('',3,(#155747,#155748,#155749,#155750,
#155751,#155752),.UNSPECIFIED.,.F.,.F.,(4,2,4),(0.,0.0126514369475504,0.0253026276141575),
 .UNSPECIFIED.);
#23863=B_SPLINE_CURVE_WITH_KNOTS('',3,(#155768,#155769,#155770,#155771,
#155772,#155773),.UNSPECIFIED.,.F.,.F.,(4,2,4),(0.,0.0126514362674318,0.0253026258987748),
 .UNSPECIFIED.);
#23864=B_SPLINE_CURVE_WITH_KNOTS('',3,(#155789,#155790,#155791,#155792,
#155793,#155794),.UNSPECIFIED.,.F.,.F.,(4,2,4),(0.,0.0126514378601925,0.0253026298921727),
 .UNSPECIFIED.);
#23865=B_SPLINE_CURVE_WITH_KNOTS('',3,(#155810,#155811,#155812,#155813,
#155814,#155815),.UNSPECIFIED.,.F.,.F.,(4,2,4),(0.,0.0126514360091151,0.0253026252315581),
 .UNSPECIFIED.);
#23866=B_SPLINE_CURVE_WITH_KNOTS('',3,(#155831,#155832,#155833,#155834,
#155835,#155836),.UNSPECIFIED.,.F.,.F.,(4,2,4),(0.,0.012651437241266,0.025302628328002),
 .UNSPECIFIED.);
#23867=B_SPLINE_CURVE_WITH_KNOTS('',3,(#155852,#155853,#155854,#155855,
#155856,#155857),.UNSPECIFIED.,.F.,.F.,(4,2,4),(2.1570000216242E-11,0.012651452719397,
0.0253026665300329),.UNSPECIFIED.);
#23868=B_SPLINE_CURVE_WITH_KNOTS('',3,(#155873,#155874,#155875,#155876,
#155877,#155878),.UNSPECIFIED.,.F.,.F.,(4,2,4),(0.,0.0126514357414824,0.025302624730698),
 .UNSPECIFIED.);
#23869=B_SPLINE_CURVE_WITH_KNOTS('',3,(#155894,#155895,#155896,#155897,
#155898,#155899),.UNSPECIFIED.,.F.,.F.,(4,2,4),(0.,0.0126514374648161,0.0253026289492822),
 .UNSPECIFIED.);
#23870=B_SPLINE_CURVE_WITH_KNOTS('',3,(#155915,#155916,#155917,#155918,
#155919,#155920),.UNSPECIFIED.,.F.,.F.,(4,2,4),(2.26557866084254E-11,0.0126514528474184,
0.0253026666314633),.UNSPECIFIED.);
#23871=B_SPLINE_CURVE_WITH_KNOTS('',3,(#155951,#155952,#155953,#155954),
 .UNSPECIFIED.,.F.,.F.,(4,4),(9.26470581739597E-13,6.28597141856272E-5),
 .UNSPECIFIED.);
#23872=B_SPLINE_CURVE_WITH_KNOTS('',3,(#155972,#155973,#155974,#155975),
 .UNSPECIFIED.,.F.,.F.,(4,4),(1.04766320724494E-15,6.28597156104803E-5),
 .UNSPECIFIED.);
#23873=B_SPLINE_CURVE_WITH_KNOTS('',3,(#156015,#156016,#156017,#156018),
 .UNSPECIFIED.,.F.,.F.,(4,4),(8.08906446880292E-14,6.28597156343113E-5),
 .UNSPECIFIED.);
#23874=B_SPLINE_CURVE_WITH_KNOTS('',3,(#156058,#156059,#156060,#156061),
 .UNSPECIFIED.,.F.,.F.,(4,4),(2.37774944269479E-13,6.2859613216331E-5),
 .UNSPECIFIED.);
#23875=B_SPLINE_CURVE_WITH_KNOTS('',3,(#156101,#156102,#156103,#156104),
 .UNSPECIFIED.,.F.,.F.,(4,4),(2.29518468417639E-13,6.2859715533947E-5),
 .UNSPECIFIED.);
#23876=B_SPLINE_CURVE_WITH_KNOTS('',3,(#156144,#156145,#156146,#156147),
 .UNSPECIFIED.,.F.,.F.,(4,4),(2.70866639842599E-13,6.28596134458986E-5),
 .UNSPECIFIED.);
#23877=B_SPLINE_CURVE_WITH_KNOTS('',3,(#156187,#156188,#156189,#156190),
 .UNSPECIFIED.,.F.,.F.,(4,4),(2.23807374264663E-13,6.28597151266788E-5),
 .UNSPECIFIED.);
#23878=B_SPLINE_CURVE_WITH_KNOTS('',3,(#156230,#156231,#156232,#156233),
 .UNSPECIFIED.,.F.,.F.,(4,4),(1.87272302703493E-13,6.28596136423573E-5),
 .UNSPECIFIED.);
#23879=B_SPLINE_CURVE_WITH_KNOTS('',3,(#156273,#156274,#156275,#156276),
 .UNSPECIFIED.,.F.,.F.,(4,4),(2.8724223760636E-13,6.2859715332009E-5),
 .UNSPECIFIED.);
#23880=B_SPLINE_CURVE_WITH_KNOTS('',3,(#156316,#156317,#156318,#156319),
 .UNSPECIFIED.,.F.,.F.,(4,4),(1.70751514793651E-13,6.28596134861198E-5),
 .UNSPECIFIED.);
#23881=B_SPLINE_CURVE_WITH_KNOTS('',3,(#156359,#156360,#156361,#156362),
 .UNSPECIFIED.,.F.,.F.,(4,4),(3.03042579258976E-13,6.28597151227342E-5),
 .UNSPECIFIED.);
#23882=B_SPLINE_CURVE_WITH_KNOTS('',3,(#156402,#156403,#156404,#156405),
 .UNSPECIFIED.,.F.,.F.,(4,4),(5.08657612240452E-14,6.28596135406422E-5),
 .UNSPECIFIED.);
#23883=B_SPLINE_CURVE_WITH_KNOTS('',3,(#156445,#156446,#156447,#156448),
 .UNSPECIFIED.,.F.,.F.,(4,4),(5.28446618968616E-14,6.28597154269528E-5),
 .UNSPECIFIED.);
#23884=B_SPLINE_CURVE_WITH_KNOTS('',3,(#156488,#156489,#156490,#156491),
 .UNSPECIFIED.,.F.,.F.,(4,4),(2.55677946032555E-14,6.28597154812872E-5),
 .UNSPECIFIED.);
#23885=B_SPLINE_CURVE_WITH_KNOTS('',3,(#156531,#156532,#156533,#156534),
 .UNSPECIFIED.,.F.,.F.,(4,4),(3.0550090682991E-14,6.28596141204512E-5),
 .UNSPECIFIED.);
#23886=B_SPLINE_CURVE_WITH_KNOTS('',3,(#156574,#156575,#156576,#156577),
 .UNSPECIFIED.,.F.,.F.,(4,4),(2.44665260015811E-13,6.28596133307425E-5),
 .UNSPECIFIED.);
#23887=B_SPLINE_CURVE_WITH_KNOTS('',3,(#156617,#156618,#156619,#156620),
 .UNSPECIFIED.,.F.,.F.,(4,4),(1.31704635813045E-13,6.28597154645398E-5),
 .UNSPECIFIED.);
#23888=B_SPLINE_CURVE_WITH_KNOTS('',3,(#156660,#156661,#156662,#156663),
 .UNSPECIFIED.,.F.,.F.,(4,4),(1.60877020579121E-13,6.28597156681893E-5),
 .UNSPECIFIED.);
#23889=B_SPLINE_CURVE_WITH_KNOTS('',3,(#156703,#156704,#156705,#156706),
 .UNSPECIFIED.,.F.,.F.,(4,4),(7.17404455169434E-14,6.28596139390678E-5),
 .UNSPECIFIED.);
#23890=B_SPLINE_CURVE_WITH_KNOTS('',3,(#156746,#156747,#156748,#156749),
 .UNSPECIFIED.,.F.,.F.,(4,4),(6.75749921739619E-14,6.28597156566878E-5),
 .UNSPECIFIED.);
#23891=B_SPLINE_CURVE_WITH_KNOTS('',3,(#156789,#156790,#156791,#156792),
 .UNSPECIFIED.,.F.,.F.,(4,4),(1.12746347172328E-13,6.28596136474964E-5),
 .UNSPECIFIED.);
#23892=B_SPLINE_CURVE_WITH_KNOTS('',3,(#156832,#156833,#156834,#156835),
 .UNSPECIFIED.,.F.,.F.,(4,4),(2.88340174742551E-13,6.28596130517667E-5),
 .UNSPECIFIED.);
#23893=B_SPLINE_CURVE_WITH_KNOTS('',3,(#156875,#156876,#156877,#156878),
 .UNSPECIFIED.,.F.,.F.,(4,4),(1.38583212404894E-13,6.28596135251862E-5),
 .UNSPECIFIED.);
#23894=B_SPLINE_CURVE_WITH_KNOTS('',3,(#156918,#156919,#156920,#156921),
 .UNSPECIFIED.,.F.,.F.,(4,4),(3.44119806752207E-14,6.28596138372693E-5),
 .UNSPECIFIED.);
#23895=B_SPLINE_CURVE_WITH_KNOTS('',3,(#156961,#156962,#156963,#156964),
 .UNSPECIFIED.,.F.,.F.,(4,4),(5.94610859549734E-14,6.28597152568138E-5),
 .UNSPECIFIED.);
#23896=B_SPLINE_CURVE_WITH_KNOTS('',3,(#157004,#157005,#157006,#157007),
 .UNSPECIFIED.,.F.,.F.,(4,4),(1.8601570951842E-15,6.28596138115333E-5),
 .UNSPECIFIED.);
#23897=B_SPLINE_CURVE_WITH_KNOTS('',3,(#157047,#157048,#157049,#157050),
 .UNSPECIFIED.,.F.,.F.,(4,4),(1.99004818569542E-13,6.28596133094018E-5),
 .UNSPECIFIED.);
#23898=B_SPLINE_CURVE_WITH_KNOTS('',3,(#157090,#157091,#157092,#157093),
 .UNSPECIFIED.,.F.,.F.,(4,4),(1.38126555594922E-13,6.28596131963104E-5),
 .UNSPECIFIED.);
#23899=B_SPLINE_CURVE_WITH_KNOTS('',3,(#157133,#157134,#157135,#157136),
 .UNSPECIFIED.,.F.,.F.,(4,4),(6.20789635911566E-14,6.28596134471087E-5),
 .UNSPECIFIED.);
#23900=B_SPLINE_CURVE_WITH_KNOTS('',3,(#157179,#157180,#157181,#157182,
#157183,#157184),.UNSPECIFIED.,.F.,.F.,(4,2,4),(-0.0252983210333844,-0.012649302700262,
0.),.UNSPECIFIED.);
#23901=B_SPLINE_CURVE_WITH_KNOTS('',3,(#157212,#157213,#157214,#157215,
#157216,#157217),.UNSPECIFIED.,.F.,.F.,(4,2,4),(-0.0252983259187359,-0.012649308870704,
0.),.UNSPECIFIED.);
#23902=B_SPLINE_CURVE_WITH_KNOTS('',3,(#157245,#157246,#157247,#157248,
#157249,#157250),.UNSPECIFIED.,.F.,.F.,(4,2,4),(-0.0252983452113512,-0.0126493122835931,
0.),.UNSPECIFIED.);
#23903=B_SPLINE_CURVE_WITH_KNOTS('',3,(#157278,#157279,#157280,#157281,
#157282,#157283),.UNSPECIFIED.,.F.,.F.,(4,2,4),(-0.0252983126265095,-0.012649303527495,
0.),.UNSPECIFIED.);
#23904=B_SPLINE_CURVE_WITH_KNOTS('',3,(#157311,#157312,#157313,#157314,
#157315,#157316),.UNSPECIFIED.,.F.,.F.,(4,2,4),(-0.0252983051684543,-0.0126493005082459,
0.),.UNSPECIFIED.);
#23905=B_SPLINE_CURVE_WITH_KNOTS('',3,(#157344,#157345,#157346,#157347,
#157348,#157349),.UNSPECIFIED.,.F.,.F.,(4,2,4),(-0.0252983420341862,-0.0126493154664923,
0.),.UNSPECIFIED.);
#23906=B_SPLINE_CURVE_WITH_KNOTS('',3,(#157377,#157378,#157379,#157380,
#157381,#157382),.UNSPECIFIED.,.F.,.F.,(4,2,4),(-0.0252983184795831,-0.012649301187786,
0.),.UNSPECIFIED.);
#23907=B_SPLINE_CURVE_WITH_KNOTS('',3,(#157410,#157411,#157412,#157413,
#157414,#157415),.UNSPECIFIED.,.F.,.F.,(4,2,4),(-0.0252987422513607,-0.0126494774106738,
-2.8633935500455E-11),.UNSPECIFIED.);
#23908=B_SPLINE_CURVE_WITH_KNOTS('',3,(#157443,#157444,#157445,#157446,
#157447,#157448),.UNSPECIFIED.,.F.,.F.,(4,2,4),(-0.0252983196287654,-0.0126493019768695,
0.),.UNSPECIFIED.);
#23909=B_SPLINE_CURVE_WITH_KNOTS('',3,(#157476,#157477,#157478,#157479,
#157480,#157481),.UNSPECIFIED.,.F.,.F.,(4,2,4),(-0.0252987422906831,-0.0126494774423558,
-3.53359529137176E-11),.UNSPECIFIED.);
#23910=B_SPLINE_CURVE_WITH_KNOTS('',3,(#157509,#157510,#157511,#157512,
#157513,#157514),.UNSPECIFIED.,.F.,.F.,(4,2,4),(-0.0252983427352373,-0.0126493112443732,
0.),.UNSPECIFIED.);
#23911=B_SPLINE_CURVE_WITH_KNOTS('',3,(#157542,#157543,#157544,#157545,
#157546,#157547),.UNSPECIFIED.,.F.,.F.,(4,2,4),(-0.0252983604613678,-0.0126493184035386,
0.),.UNSPECIFIED.);
#23912=B_SPLINE_CURVE_WITH_KNOTS('',3,(#157575,#157576,#157577,#157578,
#157579,#157580),.UNSPECIFIED.,.F.,.F.,(4,2,4),(-0.0252983388699996,-0.0126493141276362,
0.),.UNSPECIFIED.);
#23913=B_SPLINE_CURVE_WITH_KNOTS('',3,(#157608,#157609,#157610,#157611,
#157612,#157613),.UNSPECIFIED.,.F.,.F.,(4,2,4),(-0.0252983093340518,-0.0126493021520564,
0.),.UNSPECIFIED.);
#23914=B_SPLINE_CURVE_WITH_KNOTS('',3,(#157638,#157639,#157640,#157641,
#157642,#157643),.UNSPECIFIED.,.F.,.F.,(4,2,4),(-0.0252983343649174,-0.0126493123664179,
0.),.UNSPECIFIED.);
#23915=B_SPLINE_CURVE_WITH_KNOTS('',3,(#157665,#157666,#157667,#157668,
#157669,#157670),.UNSPECIFIED.,.F.,.F.,(4,2,4),(-0.0252983139448652,-0.012649299232769,
0.),.UNSPECIFIED.);
#23916=B_SPLINE_CURVE_WITH_KNOTS('',3,(#157698,#157699,#157700,#157701,
#157702,#157703),.UNSPECIFIED.,.F.,.F.,(4,2,4),(-0.0252983284278702,-0.0126493053945732,
0.),.UNSPECIFIED.);
#23917=B_SPLINE_CURVE_WITH_KNOTS('',3,(#157731,#157732,#157733,#157734,
#157735,#157736),.UNSPECIFIED.,.F.,.F.,(4,2,4),(-0.025298752822132,-0.0126494774032927,
-2.07888706249548E-11),.UNSPECIFIED.);
#23918=B_SPLINE_CURVE_WITH_KNOTS('',3,(#157765,#157766,#157767,#157768,
#157769,#157770),.UNSPECIFIED.,.F.,.F.,(4,2,4),(-0.0252983533956398,-0.0126493200194815,
0.),.UNSPECIFIED.);
#23919=B_SPLINE_CURVE_WITH_KNOTS('',3,(#157797,#157798,#157799,#157800,
#157801,#157802),.UNSPECIFIED.,.F.,.F.,(4,2,4),(-0.0252983451914397,-0.0126493126064348,
0.),.UNSPECIFIED.);
#23920=B_SPLINE_CURVE_WITH_KNOTS('',3,(#157830,#157831,#157832,#157833,
#157834,#157835),.UNSPECIFIED.,.F.,.F.,(4,2,4),(-0.025298337408984,-0.0126493088979085,
0.),.UNSPECIFIED.);
#23921=B_SPLINE_CURVE_WITH_KNOTS('',3,(#157863,#157864,#157865,#157866,
#157867,#157868),.UNSPECIFIED.,.F.,.F.,(4,2,4),(-0.0252983425361315,-0.0126493108082732,
0.),.UNSPECIFIED.);
#23922=B_SPLINE_CURVE_WITH_KNOTS('',3,(#157896,#157897,#157898,#157899,
#157900,#157901),.UNSPECIFIED.,.F.,.F.,(4,2,4),(-0.0252983214371618,-0.0126493028038431,
0.),.UNSPECIFIED.);
#23923=B_SPLINE_CURVE_WITH_KNOTS('',3,(#157929,#157930,#157931,#157932,
#157933,#157934),.UNSPECIFIED.,.F.,.F.,(4,2,4),(-0.0252983382857441,-0.0126493089336017,
0.),.UNSPECIFIED.);
#23924=B_SPLINE_CURVE_WITH_KNOTS('',3,(#157962,#157963,#157964,#157965,
#157966,#157967),.UNSPECIFIED.,.F.,.F.,(4,2,4),(-0.0252983296574141,-0.0126493057311267,
0.),.UNSPECIFIED.);
#23925=B_SPLINE_CURVE_WITH_KNOTS('',3,(#157995,#157996,#157997,#157998,
#157999,#158000),.UNSPECIFIED.,.F.,.F.,(4,2,4),(-0.0252983425115197,-0.0126493156571284,
0.),.UNSPECIFIED.);
#23926=B_SPLINE_CURVE_WITH_KNOTS('',3,(#158028,#158029,#158030,#158031,
#158032,#158033),.UNSPECIFIED.,.F.,.F.,(4,2,4),(-0.0252983434321303,-0.0126493159559477,
0.),.UNSPECIFIED.);
#23927=B_SPLINE_CURVE_WITH_KNOTS('',3,(#158061,#158062,#158063,#158064,
#158065,#158066),.UNSPECIFIED.,.F.,.F.,(4,2,4),(-0.025298310545057,-0.0126492984757903,
0.),.UNSPECIFIED.);
#23928=B_SPLINE_CURVE_WITH_KNOTS('',3,(#158094,#158095,#158096,#158097,
#158098,#158099),.UNSPECIFIED.,.F.,.F.,(4,2,4),(-0.0252982986313331,-0.0126492979062713,
0.),.UNSPECIFIED.);
#23929=B_SPLINE_CURVE_WITH_KNOTS('',3,(#158136,#158137,#158138,#158139,
#158140,#158141,#158142,#158143,#158144,#158145),.UNSPECIFIED.,.F.,.F.,
(4,3,3,4),(4.25990453213117E-13,1.58768505726012E-5,3.06163004638053E-5,
4.5355765246366E-5),.UNSPECIFIED.);
#23930=B_SPLINE_CURVE_WITH_KNOTS('',3,(#158156,#158157,#158158,#158159,
#158160,#158161,#158162),.UNSPECIFIED.,.F.,.F.,(4,3,4),(0.0665257480074743,
0.0687515042649955,0.0736118336323568),.UNSPECIFIED.);
#23931=B_SPLINE_CURVE_WITH_KNOTS('',3,(#158184,#158185,#158186,#158187,
#158188,#158189,#158190,#158191,#158192,#158193),.UNSPECIFIED.,.F.,.F.,
(4,3,3,4),(1.99141659217819E-11,5.49564847615335E-5,0.000106404139403314,
0.000157852343447398),.UNSPECIFIED.);
#23932=B_SPLINE_CURVE_WITH_KNOTS('',3,(#158222,#158223,#158224,#158225,
#158226,#158227,#158228,#158229,#158230,#158231),.UNSPECIFIED.,.F.,.F.,
(4,3,3,4),(5.32676466607925E-13,1.58768508861865E-5,3.06163005726345E-5,
4.53557651504358E-5),.UNSPECIFIED.);
#23933=B_SPLINE_CURVE_WITH_KNOTS('',3,(#158242,#158243,#158244,#158245,
#158246,#158247,#158248),.UNSPECIFIED.,.F.,.F.,(4,3,4),(0.0665257254736559,
0.0687515042649955,0.0736118336370433),.UNSPECIFIED.);
#23934=B_SPLINE_CURVE_WITH_KNOTS('',3,(#158270,#158271,#158272,#158273,
#158274,#158275,#158276,#158277,#158278,#158279),.UNSPECIFIED.,.F.,.F.,
(4,3,3,4),(1.93863144415546E-11,5.49564848580405E-5,0.000106404139411967,
0.000157852343337258),.UNSPECIFIED.);
#23935=B_SPLINE_CURVE_WITH_KNOTS('',3,(#158308,#158309,#158310,#158311,
#158312,#158313,#158314,#158315,#158316,#158317),.UNSPECIFIED.,.F.,.F.,
(4,3,3,4),(5.5731114037476E-13,1.58768507104624E-5,3.06163004400154E-5,
4.53557650609786E-5),.UNSPECIFIED.);
#23936=B_SPLINE_CURVE_WITH_KNOTS('',3,(#158328,#158329,#158330,#158331,
#158332,#158333),.UNSPECIFIED.,.F.,.F.,(4,2,4),(-0.0324724419097549,-0.0162483431540196,
0.),.UNSPECIFIED.);
#23937=B_SPLINE_CURVE_WITH_KNOTS('',3,(#158355,#158356,#158357,#158358,
#158359,#158360,#158361,#158362,#158363,#158364),.UNSPECIFIED.,.F.,.F.,
(4,3,3,4),(1.94550864791645E-11,5.49564847847185E-5,0.000106404139445542,
0.000157852343508583),.UNSPECIFIED.);
#23938=B_SPLINE_CURVE_WITH_KNOTS('',3,(#158393,#158394,#158395,#158396,
#158397,#158398,#158399,#158400,#158401,#158402),.UNSPECIFIED.,.F.,.F.,
(4,3,3,4),(3.76772541217172E-13,1.58768505800345E-5,3.06163003300456E-5,
4.53557649715249E-5),.UNSPECIFIED.);
#23939=B_SPLINE_CURVE_WITH_KNOTS('',3,(#158413,#158414,#158415,#158416,
#158417,#158418,#158419),.UNSPECIFIED.,.F.,.F.,(4,3,4),(0.0665257474100939,
0.068751504264996,0.0736118336454257),.UNSPECIFIED.);
#23940=B_SPLINE_CURVE_WITH_KNOTS('',3,(#158441,#158442,#158443,#158444,
#158445,#158446,#158447,#158448,#158449,#158450),.UNSPECIFIED.,.F.,.F.,
(4,3,3,4),(1.96446060032063E-11,5.4956484838752E-5,0.000106404139406406,
0.000157852343376373),.UNSPECIFIED.);
#23941=B_SPLINE_CURVE_WITH_KNOTS('',3,(#158479,#158480,#158481,#158482,
#158483,#158484,#158485,#158486,#158487,#158488),.UNSPECIFIED.,.F.,.F.,
(4,3,3,4),(4.86755894837992E-13,1.58768505748808E-5,3.0616300507068E-5,
4.5355765330689E-5),.UNSPECIFIED.);
#23942=B_SPLINE_CURVE_WITH_KNOTS('',3,(#158525,#158526,#158527,#158528,
#158529,#158530,#158531,#158532,#158533,#158534),.UNSPECIFIED.,.F.,.F.,
(4,3,3,4),(1.99724871658589E-11,5.49564846709833E-5,0.000106404139381309,
0.000157852343435992),.UNSPECIFIED.);
#23943=B_SPLINE_CURVE_WITH_KNOTS('',3,(#158563,#158564,#158565,#158566,
#158567,#158568,#158569,#158570,#158571,#158572),.UNSPECIFIED.,.F.,.F.,
(4,3,3,4),(4.33749804775174E-13,1.58768504673084E-5,3.06163003327111E-5,
4.53557650894788E-5),.UNSPECIFIED.);
#23944=B_SPLINE_CURVE_WITH_KNOTS('',3,(#158583,#158584,#158585,#158586,
#158587,#158588,#158589),.UNSPECIFIED.,.F.,.F.,(4,3,4),(0.0665257474078056,
0.0687515042649963,0.0736118336407646),.UNSPECIFIED.);
#23945=B_SPLINE_CURVE_WITH_KNOTS('',3,(#158611,#158612,#158613,#158614,
#158615,#158616,#158617,#158618,#158619,#158620),.UNSPECIFIED.,.F.,.F.,
(4,3,3,4),(1.97606791947156E-11,5.49564847358755E-5,0.000106404139427357,
0.000157852343477407),.UNSPECIFIED.);
#23946=B_SPLINE_CURVE_WITH_KNOTS('',3,(#158649,#158650,#158651,#158652,
#158653,#158654,#158655,#158656,#158657,#158658),.UNSPECIFIED.,.F.,.F.,
(4,3,3,4),(3.72492554887973E-13,1.58768508262691E-5,3.06163004955292E-5,
4.5355765056191E-5),.UNSPECIFIED.);
#23947=B_SPLINE_CURVE_WITH_KNOTS('',3,(#158669,#158670,#158671,#158672,
#158673,#158674),.UNSPECIFIED.,.F.,.F.,(4,2,4),(-0.0324734603942446,-0.0162498515535043,
-9.9933629731791E-7),.UNSPECIFIED.);
#23948=B_SPLINE_CURVE_WITH_KNOTS('',3,(#158696,#158697,#158698,#158699,
#158700,#158701,#158702,#158703,#158704,#158705),.UNSPECIFIED.,.F.,.F.,
(4,3,3,4),(1.93519675222046E-11,5.49564847880802E-5,0.000106404139355769,
0.000157852343325931),.UNSPECIFIED.);
#23949=B_SPLINE_CURVE_WITH_KNOTS('',3,(#158734,#158735,#158736,#158737,
#158738,#158739,#158740,#158741,#158742,#158743),.UNSPECIFIED.,.F.,.F.,
(4,3,3,4),(4.97103074448361E-13,1.58768506527717E-5,3.06163004425891E-5,
4.53557651237911E-5),.UNSPECIFIED.);
#23950=B_SPLINE_CURVE_WITH_KNOTS('',3,(#158754,#158755,#158756,#158757,
#158758,#158759,#158760),.UNSPECIFIED.,.F.,.F.,(4,3,4),(0.0665257474071759,
0.0687515042649955,0.0736118336741103),.UNSPECIFIED.);
#23951=B_SPLINE_CURVE_WITH_KNOTS('',3,(#158782,#158783,#158784,#158785,
#158786,#158787,#158788,#158789,#158790,#158791),.UNSPECIFIED.,.F.,.F.,
(4,3,3,4),(1.96923621175035E-11,5.49564847036435E-5,0.000106404139397447,
0.000157852343493646),.UNSPECIFIED.);
#23952=B_SPLINE_CURVE_WITH_KNOTS('',3,(#158820,#158821,#158822,#158823,
#158824,#158825,#158826,#158827,#158828,#158829),.UNSPECIFIED.,.F.,.F.,
(4,3,3,4),(4.23342436434571E-13,1.58768506365923E-5,3.06163005047287E-5,
4.5355765264208E-5),.UNSPECIFIED.);
#23953=B_SPLINE_CURVE_WITH_KNOTS('',3,(#158840,#158841,#158842,#158843,
#158844,#158845),.UNSPECIFIED.,.F.,.F.,(4,2,4),(-0.0324734273212292,-0.0162498395840204,
-9.99919512960357E-7),.UNSPECIFIED.);
#23954=B_SPLINE_CURVE_WITH_KNOTS('',3,(#158867,#158868,#158869,#158870,
#158871,#158872,#158873,#158874,#158875,#158876),.UNSPECIFIED.,.F.,.F.,
(4,3,3,4),(1.97891657315654E-11,5.49564847358851E-5,0.000106404139393166,
0.000157852343452837),.UNSPECIFIED.);
#23955=B_SPLINE_CURVE_WITH_KNOTS('',3,(#158905,#158906,#158907,#158908,
#158909,#158910,#158911,#158912,#158913,#158914),.UNSPECIFIED.,.F.,.F.,
(4,3,3,4),(4.45427133556455E-13,1.58768506679322E-5,3.06163004489602E-5,
4.53557651213399E-5),.UNSPECIFIED.);
#23956=B_SPLINE_CURVE_WITH_KNOTS('',3,(#158925,#158926,#158927,#158928,
#158929,#158930,#158931),.UNSPECIFIED.,.F.,.F.,(4,3,4),(0.066525747412771,
0.0687515042650049,0.0736118336413792),.UNSPECIFIED.);
#23957=B_SPLINE_CURVE_WITH_KNOTS('',3,(#158953,#158954,#158955,#158956,
#158957,#158958,#158959,#158960,#158961,#158962),.UNSPECIFIED.,.F.,.F.,
(4,3,3,4),(1.99079370166527E-11,5.49564848485402E-5,0.000106404139310357,
0.000157852343174584),.UNSPECIFIED.);
#23958=B_SPLINE_CURVE_WITH_KNOTS('',3,(#158991,#158992,#158993,#158994,
#158995,#158996,#158997,#158998,#158999,#159000),.UNSPECIFIED.,.F.,.F.,
(4,3,3,4),(4.10262871629452E-13,1.5876850659983E-5,3.06163003713765E-5,
4.53557649741511E-5),.UNSPECIFIED.);
#23959=B_SPLINE_CURVE_WITH_KNOTS('',3,(#159011,#159012,#159013,#159014,
#159015,#159016,#159017),.UNSPECIFIED.,.F.,.F.,(4,3,4),(0.0665257254736557,
0.0687515042650046,0.0736118336259733),.UNSPECIFIED.);
#23960=B_SPLINE_CURVE_WITH_KNOTS('',3,(#159039,#159040,#159041,#159042,
#159043,#159044,#159045,#159046,#159047,#159048),.UNSPECIFIED.,.F.,.F.,
(4,3,3,4),(1.96994503283381E-11,5.49564846894993E-5,0.000106404139458188,
0.000157852343520435),.UNSPECIFIED.);
#23961=B_SPLINE_CURVE_WITH_KNOTS('',3,(#159077,#159078,#159079,#159080,
#159081,#159082,#159083,#159084,#159085,#159086),.UNSPECIFIED.,.F.,.F.,
(4,3,3,4),(4.3756932208846E-13,1.58768506118317E-5,3.06163003591576E-5,
4.5355764997848E-5),.UNSPECIFIED.);
#23962=B_SPLINE_CURVE_WITH_KNOTS('',3,(#159097,#159098,#159099,#159100,
#159101,#159102,#159103),.UNSPECIFIED.,.F.,.F.,(4,3,4),(0.0665257474083367,
0.0687515042650054,0.0736118336568276),.UNSPECIFIED.);
#23963=B_SPLINE_CURVE_WITH_KNOTS('',3,(#159125,#159126,#159127,#159128,
#159129,#159130,#159131,#159132,#159133,#159134),.UNSPECIFIED.,.F.,.F.,
(4,3,3,4),(1.95026631094892E-11,5.49564847805335E-5,0.000106404139539567,
0.000157852343624086),.UNSPECIFIED.);
#23964=B_SPLINE_CURVE_WITH_KNOTS('',3,(#159163,#159164,#159165,#159166,
#159167,#159168,#159169,#159170,#159171,#159172),.UNSPECIFIED.,.F.,.F.,
(4,3,3,4),(5.72598080427875E-13,1.58768505648184E-5,3.0616300343596E-5,
4.53557650137651E-5),.UNSPECIFIED.);
#23965=B_SPLINE_CURVE_WITH_KNOTS('',3,(#159183,#159184,#159185,#159186,
#159187,#159188),.UNSPECIFIED.,.F.,.F.,(4,2,4),(-0.0324734452498497,-0.0162498432494454,
-1.00000000166633E-6),.UNSPECIFIED.);
#23966=B_SPLINE_CURVE_WITH_KNOTS('',3,(#159210,#159211,#159212,#159213,
#159214,#159215,#159216,#159217,#159218,#159219),.UNSPECIFIED.,.F.,.F.,
(4,3,3,4),(1.96990710543907E-11,5.49564848806438E-5,0.000106404139562349,
0.000157852343603431),.UNSPECIFIED.);
#23967=B_SPLINE_CURVE_WITH_KNOTS('',3,(#159248,#159249,#159250,#159251,
#159252,#159253,#159254,#159255,#159256,#159257),.UNSPECIFIED.,.F.,.F.,
(4,3,3,4),(5.42714613550798E-13,1.58768507853872E-5,3.0616300474766E-5,
4.53557650554828E-5),.UNSPECIFIED.);
#23968=B_SPLINE_CURVE_WITH_KNOTS('',3,(#159268,#159269,#159270,#159271,
#159272,#159273),.UNSPECIFIED.,.F.,.F.,(4,2,4),(-0.0324724759362906,-0.0162483528856071,
0.),.UNSPECIFIED.);
#23969=B_SPLINE_CURVE_WITH_KNOTS('',3,(#159295,#159296,#159297,#159298,
#159299,#159300,#159301,#159302,#159303,#159304),.UNSPECIFIED.,.F.,.F.,
(4,3,3,4),(1.91843530344647E-11,5.49564848028284E-5,0.000106404139357679,
0.000157852343315008),.UNSPECIFIED.);
#23970=B_SPLINE_CURVE_WITH_KNOTS('',3,(#159333,#159334,#159335,#159336,
#159337,#159338,#159339,#159340,#159341,#159342),.UNSPECIFIED.,.F.,.F.,
(4,3,3,4),(5.72877897171871E-13,1.58768507696157E-5,3.06163006409456E-5,
4.53557654036395E-5),.UNSPECIFIED.);
#23971=B_SPLINE_CURVE_WITH_KNOTS('',3,(#159353,#159354,#159355,#159356,
#159357,#159358,#159359),.UNSPECIFIED.,.F.,.F.,(4,3,4),(0.0665257474130942,
0.0687515042650042,0.0736118336272697),.UNSPECIFIED.);
#23972=B_SPLINE_CURVE_WITH_KNOTS('',3,(#159381,#159382,#159383,#159384,
#159385,#159386,#159387,#159388,#159389,#159390),.UNSPECIFIED.,.F.,.F.,
(4,3,3,4),(1.96992446166412E-11,5.49564845849989E-5,0.000106404139248683,
0.000157852343250848),.UNSPECIFIED.);
#23973=B_SPLINE_CURVE_WITH_KNOTS('',3,(#159419,#159420,#159421,#159422,
#159423,#159424,#159425,#159426,#159427,#159428),.UNSPECIFIED.,.F.,.F.,
(4,3,3,4),(4.06608505957668E-13,1.58768507642259E-5,3.06163004292337E-5,
4.53557649856869E-5),.UNSPECIFIED.);
#23974=B_SPLINE_CURVE_WITH_KNOTS('',3,(#159439,#159440,#159441,#159442,
#159443,#159444,#159445),.UNSPECIFIED.,.F.,.F.,(4,3,4),(0.0665257474083745,
0.0687515042650048,0.0736118336494111),.UNSPECIFIED.);
#23975=B_SPLINE_CURVE_WITH_KNOTS('',3,(#159467,#159468,#159469,#159470,
#159471,#159472,#159473,#159474,#159475,#159476),.UNSPECIFIED.,.F.,.F.,
(4,3,3,4),(2.00282565627927E-11,5.4956484612054E-5,0.000106404139237452,
0.000157852343260917),.UNSPECIFIED.);
#23976=B_SPLINE_CURVE_WITH_KNOTS('',3,(#159505,#159506,#159507,#159508,
#159509,#159510,#159511,#159512,#159513,#159514),.UNSPECIFIED.,.F.,.F.,
(4,3,3,4),(4.24635773281619E-13,1.58768508533791E-5,3.06163006130592E-5,
4.53557652642364E-5),.UNSPECIFIED.);
#23977=B_SPLINE_CURVE_WITH_KNOTS('',3,(#159525,#159526,#159527,#159528,
#159529,#159530),.UNSPECIFIED.,.F.,.F.,(4,2,4),(-0.0324724492216348,-0.0162483449368564,
0.),.UNSPECIFIED.);
#23978=B_SPLINE_CURVE_WITH_KNOTS('',3,(#159552,#159553,#159554,#159555,
#159556,#159557,#159558,#159559,#159560,#159561),.UNSPECIFIED.,.F.,.F.,
(4,3,3,4),(1.95510594782417E-11,5.49564846343817E-5,0.00010640413941878,
0.000157852343605449),.UNSPECIFIED.);
#23979=B_SPLINE_CURVE_WITH_KNOTS('',3,(#159590,#159591,#159592,#159593,
#159594,#159595,#159596,#159597,#159598,#159599),.UNSPECIFIED.,.F.,.F.,
(4,3,3,4),(5.34422429970871E-13,1.58768507156534E-5,3.06163005847287E-5,
4.5355765345147E-5),.UNSPECIFIED.);
#23980=B_SPLINE_CURVE_WITH_KNOTS('',3,(#159610,#159611,#159612,#159613,
#159614,#159615),.UNSPECIFIED.,.F.,.F.,(4,2,4),(-0.0324724718076845,-0.0162483528768924,
0.),.UNSPECIFIED.);
#23981=B_SPLINE_CURVE_WITH_KNOTS('',3,(#159637,#159638,#159639,#159640,
#159641,#159642,#159643,#159644,#159645,#159646),.UNSPECIFIED.,.F.,.F.,
(4,3,3,4),(1.93183891144322E-11,5.49564847063177E-5,0.000106404139517368,
0.000157852343710412),.UNSPECIFIED.);
#23982=B_SPLINE_CURVE_WITH_KNOTS('',3,(#159675,#159676,#159677,#159678,
#159679,#159680,#159681,#159682,#159683,#159684),.UNSPECIFIED.,.F.,.F.,
(4,3,3,4),(6.12267080355569E-13,1.58768507909601E-5,3.06163004936341E-5,
4.53557650877082E-5),.UNSPECIFIED.);
#23983=B_SPLINE_CURVE_WITH_KNOTS('',3,(#159695,#159696,#159697,#159698,
#159699,#159700,#159701),.UNSPECIFIED.,.F.,.F.,(4,3,4),(0.0665257474091276,
0.0687515042650037,0.0736118336651023),.UNSPECIFIED.);
#23984=B_SPLINE_CURVE_WITH_KNOTS('',3,(#159723,#159724,#159725,#159726,
#159727,#159728,#159729,#159730,#159731,#159732),.UNSPECIFIED.,.F.,.F.,
(4,3,3,4),(1.92577364666127E-11,5.49564845527144E-5,0.000106404139360879,
0.000157852343571467),.UNSPECIFIED.);
#23985=B_SPLINE_CURVE_WITH_KNOTS('',3,(#159761,#159762,#159763,#159764,
#159765,#159766,#159767,#159768,#159769,#159770),.UNSPECIFIED.,.F.,.F.,
(4,3,3,4),(5.30241697382471E-13,1.58768505423667E-5,3.06163004809113E-5,
4.53557653108321E-5),.UNSPECIFIED.);
#23986=B_SPLINE_CURVE_WITH_KNOTS('',3,(#159781,#159782,#159783,#159784,
#159785,#159786),.UNSPECIFIED.,.F.,.F.,(4,2,4),(-0.0324724440917989,-0.0162483453836653,
0.),.UNSPECIFIED.);
#23987=B_SPLINE_CURVE_WITH_KNOTS('',3,(#159808,#159809,#159810,#159811,
#159812,#159813,#159814,#159815,#159816,#159817),.UNSPECIFIED.,.F.,.F.,
(4,3,3,4),(1.96520139212204E-11,5.49564848592545E-5,0.000106404139585418,
0.000157852343532562),.UNSPECIFIED.);
#23988=B_SPLINE_CURVE_WITH_KNOTS('',3,(#159846,#159847,#159848,#159849,
#159850,#159851,#159852,#159853,#159854,#159855),.UNSPECIFIED.,.F.,.F.,
(4,3,3,4),(4.53878480879253E-13,1.58768507388306E-5,3.06163005119187E-5,
4.53557651763179E-5),.UNSPECIFIED.);
#23989=B_SPLINE_CURVE_WITH_KNOTS('',3,(#159866,#159867,#159868,#159869,
#159870,#159871,#159872),.UNSPECIFIED.,.F.,.F.,(4,3,4),(0.0665257474082937,
0.0687515042650046,0.0736118336483852),.UNSPECIFIED.);
#23990=B_SPLINE_CURVE_WITH_KNOTS('',3,(#159894,#159895,#159896,#159897,
#159898,#159899,#159900,#159901,#159902,#159903),.UNSPECIFIED.,.F.,.F.,
(4,3,3,4),(1.92866355622382E-11,5.49564847070356E-5,0.000106404139504483,
0.000157852343704383),.UNSPECIFIED.);
#23991=B_SPLINE_CURVE_WITH_KNOTS('',3,(#159932,#159933,#159934,#159935,
#159936,#159937,#159938,#159939,#159940,#159941),.UNSPECIFIED.,.F.,.F.,
(4,3,3,4),(3.60097101546029E-13,1.58768506767972E-5,3.06163003015025E-5,
4.53557648175994E-5),.UNSPECIFIED.);
#23992=B_SPLINE_CURVE_WITH_KNOTS('',3,(#159952,#159953,#159954,#159955,
#159956,#159957,#159958),.UNSPECIFIED.,.F.,.F.,(4,3,4),(0.0665257474088453,
0.0687515042650069,0.0736118336634073),.UNSPECIFIED.);
#23993=B_SPLINE_CURVE_WITH_KNOTS('',3,(#159980,#159981,#159982,#159983,
#159984,#159985,#159986,#159987,#159988,#159989),.UNSPECIFIED.,.F.,.F.,
(4,3,3,4),(1.975508753699E-11,5.49564846646962E-5,0.000106404139476724,
0.000157852343691029),.UNSPECIFIED.);
#23994=B_SPLINE_CURVE_WITH_KNOTS('',3,(#160018,#160019,#160020,#160021,
#160022,#160023,#160024,#160025,#160026,#160027),.UNSPECIFIED.,.F.,.F.,
(4,3,3,4),(3.55815629379808E-13,1.58768504837401E-5,3.06163004587416E-5,
4.53557653250738E-5),.UNSPECIFIED.);
#23995=B_SPLINE_CURVE_WITH_KNOTS('',3,(#160038,#160039,#160040,#160041,
#160042,#160043,#160044),.UNSPECIFIED.,.F.,.F.,(4,3,4),(0.0665257474135242,
0.0687515042650059,0.0736118336248754),.UNSPECIFIED.);
#23996=B_SPLINE_CURVE_WITH_KNOTS('',3,(#160066,#160067,#160068,#160069,
#160070,#160071,#160072,#160073,#160074,#160075),.UNSPECIFIED.,.F.,.F.,
(4,3,3,4),(1.94487369940343E-11,5.49564848072225E-5,0.000106404139452461,
0.000157852343430733),.UNSPECIFIED.);
#23997=B_SPLINE_CURVE_WITH_KNOTS('',3,(#160104,#160105,#160106,#160107,
#160108,#160109,#160110,#160111,#160112,#160113),.UNSPECIFIED.,.F.,.F.,
(4,3,3,4),(4.88112751114793E-13,1.58768508220155E-5,3.06163006345242E-5,
4.53557653383791E-5),.UNSPECIFIED.);
#23998=B_SPLINE_CURVE_WITH_KNOTS('',3,(#160124,#160125,#160126,#160127,
#160128,#160129,#160130),.UNSPECIFIED.,.F.,.F.,(4,3,4),(0.0665257474068711,
0.0687515042649959,0.0736118336610845),.UNSPECIFIED.);
#23999=B_SPLINE_CURVE_WITH_KNOTS('',3,(#160152,#160153,#160154,#160155,
#160156,#160157,#160158,#160159,#160160,#160161),.UNSPECIFIED.,.F.,.F.,
(4,3,3,4),(1.91069259613115E-11,5.4956484720837E-5,0.000106404139379998,
0.000157852343441449),.UNSPECIFIED.);
#24000=B_SPLINE_CURVE_WITH_KNOTS('',3,(#160190,#160191,#160192,#160193,
#160194,#160195,#160196,#160197,#160198,#160199),.UNSPECIFIED.,.F.,.F.,
(4,3,3,4),(3.43528304253375E-13,1.58768508327752E-5,3.0616300487357E-5,
4.53557650332359E-5),.UNSPECIFIED.);
#24001=B_SPLINE_CURVE_WITH_KNOTS('',3,(#160210,#160211,#160212,#160213,
#160214,#160215),.UNSPECIFIED.,.F.,.F.,(4,2,4),(-0.0324734447985545,-0.0162498503876316,
-1.00000000177736E-6),.UNSPECIFIED.);
#24002=B_SPLINE_CURVE_WITH_KNOTS('',3,(#160237,#160238,#160239,#160240,
#160241,#160242,#160243,#160244,#160245,#160246),.UNSPECIFIED.,.F.,.F.,
(4,3,3,4),(1.91966606562681E-11,5.49564846408601E-5,0.000106404139400499,
0.000157852343415483),.UNSPECIFIED.);
#24003=B_SPLINE_CURVE_WITH_KNOTS('',3,(#160275,#160276,#160277,#160278,
#160279,#160280,#160281,#160282,#160283,#160284),.UNSPECIFIED.,.F.,.F.,
(4,3,3,4),(4.80195844454561E-13,1.58768506961566E-5,3.06163005244348E-5,
4.53557652441286E-5),.UNSPECIFIED.);
#24004=B_SPLINE_CURVE_WITH_KNOTS('',3,(#160295,#160296,#160297,#160298,
#160299,#160300,#160301),.UNSPECIFIED.,.F.,.F.,(4,3,4),(0.0665257474126737,
0.0687515042649959,0.0736118336563353),.UNSPECIFIED.);
#24005=B_SPLINE_CURVE_WITH_KNOTS('',3,(#160323,#160324,#160325,#160326,
#160327,#160328,#160329,#160330,#160331,#160332),.UNSPECIFIED.,.F.,.F.,
(4,3,3,4),(1.95587395262878E-11,5.49564849813836E-5,0.000106404139413079,
0.00015785234324718),.UNSPECIFIED.);
#24006=B_SPLINE_CURVE_WITH_KNOTS('',3,(#160361,#160362,#160363,#160364,
#160365,#160366,#160367,#160368,#160369,#160370),.UNSPECIFIED.,.F.,.F.,
(4,3,3,4),(3.33037896955563E-13,1.5876850567122E-5,3.06163004445858E-5,
4.53557652134316E-5),.UNSPECIFIED.);
#24007=B_SPLINE_CURVE_WITH_KNOTS('',3,(#160381,#160382,#160383,#160384,
#160385,#160386,#160387),.UNSPECIFIED.,.F.,.F.,(4,3,4),(0.0665257474066404,
0.0687515042649958,0.0736118336459457),.UNSPECIFIED.);
#24008=B_SPLINE_CURVE_WITH_KNOTS('',3,(#160409,#160410,#160411,#160412,
#160413,#160414,#160415,#160416,#160417,#160418),.UNSPECIFIED.,.F.,.F.,
(4,3,3,4),(1.99075229772508E-11,5.49564847828955E-5,0.000106404139424612,
0.000157852343348),.UNSPECIFIED.);
#24009=B_SPLINE_CURVE_WITH_KNOTS('',3,(#160447,#160448,#160449,#160450,
#160451,#160452,#160453,#160454,#160455,#160456),.UNSPECIFIED.,.F.,.F.,
(4,3,3,4),(3.41414203172804E-13,1.58768505874591E-5,3.06163003339983E-5,
4.53557649719169E-5),.UNSPECIFIED.);
#24010=B_SPLINE_CURVE_WITH_KNOTS('',3,(#160467,#160468,#160469,#160470,
#160471,#160472,#160473),.UNSPECIFIED.,.F.,.F.,(4,3,4),(0.06652574740877,
0.068751504264996,0.0736118336476656),.UNSPECIFIED.);
#24011=B_SPLINE_CURVE_WITH_KNOTS('',3,(#160495,#160496,#160497,#160498,
#160499,#160500,#160501,#160502,#160503,#160504),.UNSPECIFIED.,.F.,.F.,
(4,3,3,4),(1.94484427579567E-11,5.49564846028534E-5,0.00010640413945402,
0.000157852343648001),.UNSPECIFIED.);
#24012=B_SPLINE_CURVE_WITH_KNOTS('',3,(#160533,#160534,#160535,#160536,
#160537,#160538,#160539,#160540,#160541,#160542),.UNSPECIFIED.,.F.,.F.,
(4,3,3,4),(4.15431761292954E-13,1.58768508092275E-5,3.06163004475716E-5,
4.5355764977311E-5),.UNSPECIFIED.);
#24013=B_SPLINE_CURVE_WITH_KNOTS('',3,(#160553,#160554,#160555,#160556,
#160557,#160558,#160559),.UNSPECIFIED.,.F.,.F.,(4,3,4),(0.0665257474138115,
0.0687515042649961,0.0736118336459126),.UNSPECIFIED.);
#24014=B_SPLINE_CURVE_WITH_KNOTS('',3,(#160581,#160582,#160583,#160584,
#160585,#160586,#160587,#160588,#160589,#160590),.UNSPECIFIED.,.F.,.F.,
(4,3,3,4),(1.96216466760054E-11,5.4956484902517E-5,0.000106404139425267,
0.000157852343253078),.UNSPECIFIED.);
#24015=B_SPLINE_CURVE_WITH_KNOTS('',3,(#160609,#160610,#160611,#160612,
#160613,#160614),.UNSPECIFIED.,.F.,.F.,(4,2,4),(3.50146860978608E-11,0.0126520282634591,
0.025303829872637),.UNSPECIFIED.);
#24016=B_SPLINE_CURVE_WITH_KNOTS('',3,(#160634,#160635,#160636,#160637,
#160638,#160639),.UNSPECIFIED.,.F.,.F.,(4,2,4),(0.,0.0126520258962633,0.025303824074642),
 .UNSPECIFIED.);
#24017=B_SPLINE_CURVE_WITH_KNOTS('',3,(#160659,#160660,#160661,#160662,
#160663,#160664),.UNSPECIFIED.,.F.,.F.,(4,2,4),(0.,0.0126520281025744,0.0253038295843138),
 .UNSPECIFIED.);
#24018=B_SPLINE_CURVE_WITH_KNOTS('',3,(#160684,#160685,#160686,#160687,
#160688,#160689),.UNSPECIFIED.,.F.,.F.,(4,2,4),(0.,0.0126520265670996,0.0253038257319735),
 .UNSPECIFIED.);
#24019=B_SPLINE_CURVE_WITH_KNOTS('',3,(#160709,#160710,#160711,#160712,
#160713,#160714),.UNSPECIFIED.,.F.,.F.,(4,2,4),(0.,0.0126520266851299,0.0253038261543005),
 .UNSPECIFIED.);
#24020=B_SPLINE_CURVE_WITH_KNOTS('',3,(#160734,#160735,#160736,#160737,
#160738,#160739),.UNSPECIFIED.,.F.,.F.,(4,2,4),(0.,0.012652026020123,0.0253038244493337),
 .UNSPECIFIED.);
#24021=B_SPLINE_CURVE_WITH_KNOTS('',3,(#160759,#160760,#160761,#160762,
#160763,#160764),.UNSPECIFIED.,.F.,.F.,(4,2,4),(0.,0.0126520262984874,0.0253038249916903),
 .UNSPECIFIED.);
#24022=B_SPLINE_CURVE_WITH_KNOTS('',3,(#160784,#160785,#160786,#160787,
#160788,#160789),.UNSPECIFIED.,.F.,.F.,(4,2,4),(0.,0.0126520282590167,0.025303829881957),
 .UNSPECIFIED.);
#24023=B_SPLINE_CURVE_WITH_KNOTS('',3,(#160809,#160810,#160811,#160812,
#160813,#160814),.UNSPECIFIED.,.F.,.F.,(4,2,4),(0.,0.0126520269368647,0.0253038266869163),
 .UNSPECIFIED.);
#24024=B_SPLINE_CURVE_WITH_KNOTS('',3,(#160834,#160835,#160836,#160837,
#160838,#160839),.UNSPECIFIED.,.F.,.F.,(4,2,4),(0.,0.0126520263342759,0.0253038251684596),
 .UNSPECIFIED.);
#24025=B_SPLINE_CURVE_WITH_KNOTS('',3,(#160859,#160860,#160861,#160862,
#160863,#160864),.UNSPECIFIED.,.F.,.F.,(4,2,4),(0.,0.0126520256408363,0.0253038236240611),
 .UNSPECIFIED.);
#24026=B_SPLINE_CURVE_WITH_KNOTS('',3,(#160884,#160885,#160886,#160887,
#160888,#160889),.UNSPECIFIED.,.F.,.F.,(4,2,4),(0.,0.012652027883969,0.0253038291064795),
 .UNSPECIFIED.);
#24027=B_SPLINE_CURVE_WITH_KNOTS('',3,(#160909,#160910,#160911,#160912,
#160913,#160914),.UNSPECIFIED.,.F.,.F.,(4,2,4),(2.283603133213E-11,0.0126520283107723,
0.0253038299118963),.UNSPECIFIED.);
#24028=B_SPLINE_CURVE_WITH_KNOTS('',3,(#160934,#160935,#160936,#160937,
#160938,#160939),.UNSPECIFIED.,.F.,.F.,(4,2,4),(0.,0.0126520276386329,0.0253038283858036),
 .UNSPECIFIED.);
#24029=B_SPLINE_CURVE_WITH_KNOTS('',3,(#160959,#160960,#160961,#160962,
#160963,#160964),.UNSPECIFIED.,.F.,.F.,(4,2,4),(1.73862291501938E-9,0.0126520270262746,
0.0253038246440909),.UNSPECIFIED.);
#24030=B_SPLINE_CURVE_WITH_KNOTS('',3,(#160984,#160985,#160986,#160987,
#160988,#160989),.UNSPECIFIED.,.F.,.F.,(4,2,4),(0.,0.0126520283246941,0.0253038302032181),
 .UNSPECIFIED.);
#24031=B_SPLINE_CURVE_WITH_KNOTS('',3,(#161009,#161010,#161011,#161012,
#161013,#161014),.UNSPECIFIED.,.F.,.F.,(4,2,4),(0.,0.0126520255277967,0.0253038232885518),
 .UNSPECIFIED.);
#24032=B_SPLINE_CURVE_WITH_KNOTS('',3,(#161034,#161035,#161036,#161037,
#161038,#161039),.UNSPECIFIED.,.F.,.F.,(4,2,4),(6.06839707590124E-13,0.0126520265612889,
0.02530382571351),.UNSPECIFIED.);
#24033=B_SPLINE_CURVE_WITH_KNOTS('',3,(#161059,#161060,#161061,#161062,
#161063,#161064),.UNSPECIFIED.,.F.,.F.,(4,2,4),(0.,0.0126520273330737,0.025303827547897),
 .UNSPECIFIED.);
#24034=B_SPLINE_CURVE_WITH_KNOTS('',3,(#161084,#161085,#161086,#161087,
#161088,#161089),.UNSPECIFIED.,.F.,.F.,(4,2,4),(0.,0.0126520266653492,0.0253038258407741),
 .UNSPECIFIED.);
#24035=B_SPLINE_CURVE_WITH_KNOTS('',3,(#161109,#161110,#161111,#161112,
#161113,#161114),.UNSPECIFIED.,.F.,.F.,(4,2,4),(1.70116744281899E-11,0.012652028270309,
0.0253038299189388),.UNSPECIFIED.);
#24036=B_SPLINE_CURVE_WITH_KNOTS('',3,(#161134,#161135,#161136,#161137,
#161138,#161139),.UNSPECIFIED.,.F.,.F.,(4,2,4),(0.,0.012652026346306,0.0253038252129835),
 .UNSPECIFIED.);
#24037=B_SPLINE_CURVE_WITH_KNOTS('',3,(#161159,#161160,#161161,#161162,
#161163,#161164),.UNSPECIFIED.,.F.,.F.,(4,2,4),(0.,0.0126520272288475,0.0253038274605735),
 .UNSPECIFIED.);
#24038=B_SPLINE_CURVE_WITH_KNOTS('',3,(#161184,#161185,#161186,#161187,
#161188,#161189),.UNSPECIFIED.,.F.,.F.,(4,2,4),(0.,0.0126520253434002,0.0253038227547039),
 .UNSPECIFIED.);
#24039=B_SPLINE_CURVE_WITH_KNOTS('',3,(#161209,#161210,#161211,#161212,
#161213,#161214),.UNSPECIFIED.,.F.,.F.,(4,2,4),(0.,0.0126520265495153,0.025303825763251),
 .UNSPECIFIED.);
#24040=B_SPLINE_CURVE_WITH_KNOTS('',3,(#161234,#161235,#161236,#161237,
#161238,#161239),.UNSPECIFIED.,.F.,.F.,(4,2,4),(0.,0.0126520265638083,0.0253038256562407),
 .UNSPECIFIED.);
#24041=B_SPLINE_CURVE_WITH_KNOTS('',3,(#161259,#161260,#161261,#161262,
#161263,#161264),.UNSPECIFIED.,.F.,.F.,(4,2,4),(0.,0.0126520252611529,0.0253038225702637),
 .UNSPECIFIED.);
#24042=B_SPLINE_CURVE_WITH_KNOTS('',3,(#161284,#161285,#161286,#161287,
#161288,#161289),.UNSPECIFIED.,.F.,.F.,(4,2,4),(0.,0.0126520278786851,0.0253038289796549),
 .UNSPECIFIED.);
#24043=B_SPLINE_CURVE_WITH_KNOTS('',3,(#161309,#161310,#161311,#161312,
#161313,#161314),.UNSPECIFIED.,.F.,.F.,(4,2,4),(0.,0.0126520284756542,0.0253038304784128),
 .UNSPECIFIED.);
#24044=B_SPLINE_CURVE_WITH_KNOTS('',3,(#161340,#161341,#161342,#161343,
#161344,#161345),.UNSPECIFIED.,.F.,.F.,(4,2,4),(-0.0253039879324086,-0.0126518800290025,
-1.10254964880152E-11),.UNSPECIFIED.);
#24045=B_SPLINE_CURVE_WITH_KNOTS('',3,(#161355,#161356,#161357,#161358,
#161359,#161360),.UNSPECIFIED.,.F.,.F.,(4,2,4),(1.52206643631891E-9,0.0126518815909643,
0.0253039868896389),.UNSPECIFIED.);
#24046=B_SPLINE_CURVE_WITH_KNOTS('',3,(#161394,#161395,#161396,#161397,
#161398,#161399),.UNSPECIFIED.,.F.,.F.,(4,2,4),(1.51612725093129E-9,0.0126518816134216,
0.025303986957009),.UNSPECIFIED.);
#24047=B_SPLINE_CURVE_WITH_KNOTS('',3,(#161433,#161434,#161435,#161436,
#161437,#161438),.UNSPECIFIED.,.F.,.F.,(4,2,4),(1.43547212827194E-9,0.0126518815341548,
0.0253039869610686),.UNSPECIFIED.);
#24048=B_SPLINE_CURVE_WITH_KNOTS('',3,(#161472,#161473,#161474,#161475,
#161476,#161477),.UNSPECIFIED.,.F.,.F.,(4,2,4),(1.40821217994557E-9,0.0126518814793586,
0.0253039869121775),.UNSPECIFIED.);
#24049=B_SPLINE_CURVE_WITH_KNOTS('',3,(#161511,#161512,#161513,#161514,
#161515,#161516),.UNSPECIFIED.,.F.,.F.,(4,2,4),(1.34058371660886E-9,0.0126518813899474,
0.0253039868784617),.UNSPECIFIED.);
#24050=B_SPLINE_CURVE_WITH_KNOTS('',3,(#161550,#161551,#161552,#161553,
#161554,#161555),.UNSPECIFIED.,.F.,.F.,(4,2,4),(1.50113469982618E-9,0.01265188158503,
0.0253039869826423),.UNSPECIFIED.);
#24051=B_SPLINE_CURVE_WITH_KNOTS('',3,(#161586,#161587,#161588,#161589,
#161590,#161591),.UNSPECIFIED.,.F.,.F.,(4,2,4),(1.50445324217149E-9,0.0126518816050577,
0.025303986954268),.UNSPECIFIED.);
#24052=B_SPLINE_CURVE_WITH_KNOTS('',3,(#161617,#161618,#161619,#161620,
#161621,#161622),.UNSPECIFIED.,.F.,.F.,(4,2,4),(1.52727531068401E-9,0.0126518816268682,
0.0253039869661077),.UNSPECIFIED.);
#24053=B_SPLINE_CURVE_WITH_KNOTS('',3,(#161656,#161657,#161658,#161659,
#161660,#161661),.UNSPECIFIED.,.F.,.F.,(4,2,4),(1.41870323249377E-9,0.012651881462905,
0.0253039868467572),.UNSPECIFIED.);
#24054=B_SPLINE_CURVE_WITH_KNOTS('',3,(#161695,#161696,#161697,#161698,
#161699,#161700),.UNSPECIFIED.,.F.,.F.,(4,2,4),(1.53232704557586E-9,0.012651881631661,
0.0253039869495135),.UNSPECIFIED.);
#24055=B_SPLINE_CURVE_WITH_KNOTS('',3,(#161734,#161735,#161736,#161737,
#161738,#161739),.UNSPECIFIED.,.F.,.F.,(4,2,4),(1.38628499338917E-9,0.0126518814663333,
0.0253039869324201),.UNSPECIFIED.);
#24056=B_SPLINE_CURVE_WITH_KNOTS('',3,(#161773,#161774,#161775,#161776,
#161777,#161778),.UNSPECIFIED.,.F.,.F.,(4,2,4),(1.43816896721697E-9,0.0126518814925827,
0.0253039868824678),.UNSPECIFIED.);
#24057=B_SPLINE_CURVE_WITH_KNOTS('',3,(#161812,#161813,#161814,#161815,
#161816,#161817),.UNSPECIFIED.,.F.,.F.,(4,2,4),(1.41531481175481E-9,0.0126518814869672,
0.0253039869094249),.UNSPECIFIED.);
#24058=B_SPLINE_CURVE_WITH_KNOTS('',3,(#161851,#161852,#161853,#161854,
#161855,#161856),.UNSPECIFIED.,.F.,.F.,(4,2,4),(1.50211413795707E-9,0.012651881579894,
0.0253039869249388),.UNSPECIFIED.);
#24059=B_SPLINE_CURVE_WITH_KNOTS('',3,(#161890,#161891,#161892,#161893,
#161894,#161895),.UNSPECIFIED.,.F.,.F.,(4,2,4),(1.4974251600475E-9,0.0126518815659028,
0.0253039869225986),.UNSPECIFIED.);
#24060=B_SPLINE_CURVE_WITH_KNOTS('',3,(#161929,#161930,#161931,#161932,
#161933,#161934),.UNSPECIFIED.,.F.,.F.,(4,2,4),(1.44629883447371E-9,0.0126518815283366,
0.0253039869307436),.UNSPECIFIED.);
#24061=B_SPLINE_CURVE_WITH_KNOTS('',3,(#161968,#161969,#161970,#161971,
#161972,#161973),.UNSPECIFIED.,.F.,.F.,(4,2,4),(1.47110006734065E-9,0.0126518815235758,
0.0253039868593664),.UNSPECIFIED.);
#24062=B_SPLINE_CURVE_WITH_KNOTS('',3,(#162008,#162009,#162010,#162011,
#162012,#162013),.UNSPECIFIED.,.F.,.F.,(4,2,4),(1.4826859213418E-9,0.0126518815996713,
0.0253039869934791),.UNSPECIFIED.);
#24063=B_SPLINE_CURVE_WITH_KNOTS('',3,(#162046,#162047,#162048,#162049,
#162050,#162051),.UNSPECIFIED.,.F.,.F.,(4,2,4),(1.51322869999487E-9,0.0126518816030172,
0.0253039869465037),.UNSPECIFIED.);
#24064=B_SPLINE_CURVE_WITH_KNOTS('',3,(#162085,#162086,#162087,#162088,
#162089,#162090),.UNSPECIFIED.,.F.,.F.,(4,2,4),(1.44312089558744E-9,0.0126518814908936,
0.0253039868677599),.UNSPECIFIED.);
#24065=B_SPLINE_CURVE_WITH_KNOTS('',3,(#162124,#162125,#162126,#162127,
#162128,#162129),.UNSPECIFIED.,.F.,.F.,(4,2,4),(1.38491957805618E-9,0.0126518814509472,
0.0253039869037668),.UNSPECIFIED.);
#24066=B_SPLINE_CURVE_WITH_KNOTS('',3,(#162163,#162164,#162165,#162166,
#162167,#162168),.UNSPECIFIED.,.F.,.F.,(4,2,4),(1.4442356085963E-9,0.012651881521997,
0.0253039869119498),.UNSPECIFIED.);
#24067=B_SPLINE_CURVE_WITH_KNOTS('',3,(#162202,#162203,#162204,#162205,
#162206,#162207),.UNSPECIFIED.,.F.,.F.,(4,2,4),(1.4282679182595E-9,0.0126518815081054,
0.0253039869290959),.UNSPECIFIED.);
#24068=B_SPLINE_CURVE_WITH_KNOTS('',3,(#162241,#162242,#162243,#162244,
#162245,#162246),.UNSPECIFIED.,.F.,.F.,(4,2,4),(1.45021697356858E-9,0.012651881537926,
0.0253039869495223),.UNSPECIFIED.);
#24069=B_SPLINE_CURVE_WITH_KNOTS('',3,(#162280,#162281,#162282,#162283,
#162284,#162285),.UNSPECIFIED.,.F.,.F.,(4,2,4),(1.57796420795521E-9,0.0126518816874471,
0.0253039869733485),.UNSPECIFIED.);
#24070=B_SPLINE_CURVE_WITH_KNOTS('',3,(#162319,#162320,#162321,#162322,
#162323,#162324),.UNSPECIFIED.,.F.,.F.,(4,2,4),(1.54977618130921E-9,0.0126518816622565,
0.0253039869718755),.UNSPECIFIED.);
#24071=B_SPLINE_CURVE_WITH_KNOTS('',3,(#162358,#162359,#162360,#162361,
#162362,#162363),.UNSPECIFIED.,.F.,.F.,(4,2,4),(1.41539846907942E-9,0.0126518814803473,
0.0253039869013059),.UNSPECIFIED.);
#24072=B_SPLINE_CURVE_WITH_KNOTS('',3,(#162397,#162398,#162399,#162400,
#162401,#162402),.UNSPECIFIED.,.F.,.F.,(4,2,4),(1.48230471024643E-9,0.0126518815759344,
0.0253039869544491),.UNSPECIFIED.);
#24073=B_SPLINE_CURVE_WITH_KNOTS('',3,(#163039,#163040,#163041,#163042,
#163043,#163044),.UNSPECIFIED.,.F.,.F.,(4,2,4),(0.,0.0318022370486529,0.0638030677158179),
 .UNSPECIFIED.);
#24074=B_SPLINE_CURVE_WITH_KNOTS('',3,(#163045,#163046,#163047,#163048,
#163049,#163050),.UNSPECIFIED.,.F.,.F.,(4,2,4),(8.7491300728103E-11,0.0129043685365852,
0.0270905602892694),.UNSPECIFIED.);
#24075=B_SPLINE_CURVE_WITH_KNOTS('',3,(#163054,#163055,#163056,#163057,
#163058,#163059,#163060,#163061),.UNSPECIFIED.,.F.,.F.,(4,2,2,4),(1.00010025441208E-6,
0.0146013173462511,0.0279117437094298,0.0546218077071897),.UNSPECIFIED.);
#24076=B_SPLINE_CURVE_WITH_KNOTS('',3,(#163062,#163063,#163064,#163065,
#163066,#163067),.UNSPECIFIED.,.F.,.F.,(4,2,4),(0.000862177893008277,0.0332709227757339,
0.0654912697583216),.UNSPECIFIED.);
#24077=B_SPLINE_CURVE_WITH_KNOTS('',3,(#163068,#163069,#163070,#163071,
#163072,#163073,#163074,#163075),.UNSPECIFIED.,.F.,.F.,(4,2,2,4),(1.00002233420631E-6,
0.0322596484018977,0.048328981802378,0.0657704349945425),.UNSPECIFIED.);
#24078=B_SPLINE_CURVE_WITH_KNOTS('',3,(#163098,#163099,#163100,#163101,
#163102,#163103),.UNSPECIFIED.,.F.,.F.,(4,2,4),(0.,0.0318022366302916,0.0638030661107383),
 .UNSPECIFIED.);
#24079=B_SPLINE_CURVE_WITH_KNOTS('',3,(#163104,#163105,#163106,#163107,
#163108,#163109),.UNSPECIFIED.,.F.,.F.,(4,2,4),(1.37609960883432E-10,0.0129043686339332,
0.0270905603810427),.UNSPECIFIED.);
#24080=B_SPLINE_CURVE_WITH_KNOTS('',3,(#163113,#163114,#163115,#163116,
#163117,#163118,#163119,#163120),.UNSPECIFIED.,.F.,.F.,(4,2,2,4),(1.00011427568223E-6,
0.014601317221349,0.0279117434743883,0.0546218072225535),.UNSPECIFIED.);
#24081=B_SPLINE_CURVE_WITH_KNOTS('',3,(#163121,#163122,#163123,#163124,
#163125,#163126),.UNSPECIFIED.,.F.,.F.,(4,2,4),(0.000862177877279032,0.0332709227985011,
0.0654912694116861),.UNSPECIFIED.);
#24082=B_SPLINE_CURVE_WITH_KNOTS('',3,(#163127,#163128,#163129,#163130,
#163131,#163132,#163133,#163134),.UNSPECIFIED.,.F.,.F.,(4,2,2,4),(1.00001041491299E-6,
0.0322596485585965,0.0483293807968369,0.0657704943362129),.UNSPECIFIED.);
#24083=B_SPLINE_CURVE_WITH_KNOTS('',3,(#163157,#163158,#163159,#163160,
#163161,#163162),.UNSPECIFIED.,.F.,.F.,(4,2,4),(0.,0.0318022365401368,0.0638030657211654),
 .UNSPECIFIED.);
#24084=B_SPLINE_CURVE_WITH_KNOTS('',3,(#163163,#163164,#163165,#163166,
#163167,#163168),.UNSPECIFIED.,.F.,.F.,(4,2,4),(1.56778555886997E-10,0.0129043686228877,
0.0270905603149191),.UNSPECIFIED.);
#24085=B_SPLINE_CURVE_WITH_KNOTS('',3,(#163172,#163173,#163174,#163175,
#163176,#163177,#163178,#163179),.UNSPECIFIED.,.F.,.F.,(4,2,2,4),(1.00005385785841E-6,
0.0146013173333266,0.0279117437159111,0.0546218077264354),.UNSPECIFIED.);
#24086=B_SPLINE_CURVE_WITH_KNOTS('',3,(#163180,#163181,#163182,#163183,
#163184,#163185),.UNSPECIFIED.,.F.,.F.,(4,2,4),(0.00086217789495907,0.0332709228025803,
0.0654912700336115),.UNSPECIFIED.);
#24087=B_SPLINE_CURVE_WITH_KNOTS('',3,(#163186,#163187,#163188,#163189,
#163190,#163191,#163192,#163193),.UNSPECIFIED.,.F.,.F.,(4,2,2,4),(1.00002524481216E-6,
0.0322596484594912,0.0483289818203511,0.0657704376678658),.UNSPECIFIED.);
#24088=B_SPLINE_CURVE_WITH_KNOTS('',3,(#163216,#163217,#163218,#163219,
#163220,#163221),.UNSPECIFIED.,.F.,.F.,(4,2,4),(0.,0.0318022368851196,0.0638030671062939),
 .UNSPECIFIED.);
#24089=B_SPLINE_CURVE_WITH_KNOTS('',3,(#163222,#163223,#163224,#163225,
#163226,#163227),.UNSPECIFIED.,.F.,.F.,(4,2,4),(6.96464037490181E-11,0.0129043685514154,
0.0270905603507981),.UNSPECIFIED.);
#24090=B_SPLINE_CURVE_WITH_KNOTS('',3,(#163231,#163232,#163233,#163234,
#163235,#163236,#163237,#163238),.UNSPECIFIED.,.F.,.F.,(4,2,2,4),(1.00000561038452E-6,
0.0146013174108614,0.0279117438241032,0.0546218079462628),.UNSPECIFIED.);
#24091=B_SPLINE_CURVE_WITH_KNOTS('',3,(#163239,#163240,#163241,#163242,
#163243,#163244),.UNSPECIFIED.,.F.,.F.,(4,2,4),(0.000862177865670856,0.0332709227848291,
0.0654912681350928),.UNSPECIFIED.);
#24092=B_SPLINE_CURVE_WITH_KNOTS('',3,(#163245,#163246,#163247,#163248,
#163249,#163250,#163251,#163252),.UNSPECIFIED.,.F.,.F.,(4,2,2,4),(1.00002366431758E-6,
0.032259648361095,0.0483289818685821,0.0657705256693144),.UNSPECIFIED.);
#24093=B_SPLINE_CURVE_WITH_KNOTS('',3,(#163275,#163276,#163277,#163278,
#163279,#163280),.UNSPECIFIED.,.F.,.F.,(4,2,4),(0.,0.0318022368256888,0.0638030668561903),
 .UNSPECIFIED.);
#24094=B_SPLINE_CURVE_WITH_KNOTS('',3,(#163281,#163282,#163283,#163284,
#163285,#163286),.UNSPECIFIED.,.F.,.F.,(4,2,4),(1.2210755509226E-10,0.0129043685695377,
0.0270905602832235),.UNSPECIFIED.);
#24095=B_SPLINE_CURVE_WITH_KNOTS('',3,(#163290,#163291,#163292,#163293,
#163294,#163295,#163296,#163297),.UNSPECIFIED.,.F.,.F.,(4,2,2,4),(1.00004953502741E-6,
0.0146013174148623,0.0279117438317188,0.0546218079602826),.UNSPECIFIED.);
#24096=B_SPLINE_CURVE_WITH_KNOTS('',3,(#163298,#163299,#163300,#163301,
#163302,#163303),.UNSPECIFIED.,.F.,.F.,(4,2,4),(0.000862177878398796,0.0332709228090972,
0.0654912687885388),.UNSPECIFIED.);
#24097=B_SPLINE_CURVE_WITH_KNOTS('',3,(#163304,#163305,#163306,#163307,
#163308,#163309,#163310,#163311),.UNSPECIFIED.,.F.,.F.,(4,2,2,4),(1.00001979611187E-6,
0.0322596483810105,0.048328981853273,0.0657704806604372),.UNSPECIFIED.);
#24098=B_SPLINE_CURVE_WITH_KNOTS('',3,(#163334,#163335,#163336,#163337,
#163338,#163339),.UNSPECIFIED.,.F.,.F.,(4,2,4),(0.,0.0318022366459589,0.0638030661171089),
 .UNSPECIFIED.);
#24099=B_SPLINE_CURVE_WITH_KNOTS('',3,(#163340,#163341,#163342,#163343,
#163344,#163345),.UNSPECIFIED.,.F.,.F.,(4,2,4),(1.3871504433622E-10,0.0129043686056305,
0.027090560316242),.UNSPECIFIED.);
#24100=B_SPLINE_CURVE_WITH_KNOTS('',3,(#163349,#163350,#163351,#163352,
#163353,#163354,#163355,#163356),.UNSPECIFIED.,.F.,.F.,(4,2,2,4),(1.00010651614903E-6,
0.014601317341088,0.0279117437055757,0.0546218077017514),.UNSPECIFIED.);
#24101=B_SPLINE_CURVE_WITH_KNOTS('',3,(#163357,#163358,#163359,#163360,
#163361,#163362),.UNSPECIFIED.,.F.,.F.,(4,2,4),(0.000862177886856545,0.0332709227980972,
0.0654912694331754),.UNSPECIFIED.);
#24102=B_SPLINE_CURVE_WITH_KNOTS('',3,(#163363,#163364,#163365,#163366,
#163367,#163368,#163369,#163370),.UNSPECIFIED.,.F.,.F.,(4,2,2,4),(1.00002623835471E-6,
0.0322596484247313,0.0483289819388386,0.0657704876040361),.UNSPECIFIED.);
#24103=B_SPLINE_CURVE_WITH_KNOTS('',3,(#163393,#163394,#163395,#163396,
#163397,#163398),.UNSPECIFIED.,.F.,.F.,(4,2,4),(0.,0.031802237071236,0.063803067841117),
 .UNSPECIFIED.);
#24104=B_SPLINE_CURVE_WITH_KNOTS('',3,(#163399,#163400,#163401,#163402,
#163403,#163404),.UNSPECIFIED.,.F.,.F.,(4,2,4),(8.97238040975725E-11,0.0129043685964079,
0.0270905603759876),.UNSPECIFIED.);
#24105=B_SPLINE_CURVE_WITH_KNOTS('',3,(#163408,#163409,#163410,#163411,
#163412,#163413,#163414,#163415),.UNSPECIFIED.,.F.,.F.,(4,2,2,4),(1.00002862386086E-6,
0.0146013173707883,0.0279117437374226,0.0546218077585137),.UNSPECIFIED.);
#24106=B_SPLINE_CURVE_WITH_KNOTS('',3,(#163416,#163417,#163418,#163419,
#163420,#163421),.UNSPECIFIED.,.F.,.F.,(4,2,4),(0.000862177885270482,0.0332709227980682,
0.0654912690986148),.UNSPECIFIED.);
#24107=B_SPLINE_CURVE_WITH_KNOTS('',3,(#163422,#163423,#163424,#163425,
#163426,#163427,#163428,#163429),.UNSPECIFIED.,.F.,.F.,(4,2,2,4),(1.00002356029572E-6,
0.0322596484060167,0.048328981827194,0.0657704543396389),.UNSPECIFIED.);
#24108=B_SPLINE_CURVE_WITH_KNOTS('',3,(#163452,#163453,#163454,#163455,
#163456,#163457),.UNSPECIFIED.,.F.,.F.,(4,2,4),(0.,0.0318022368265858,0.0638030668440867),
 .UNSPECIFIED.);
#24109=B_SPLINE_CURVE_WITH_KNOTS('',3,(#163458,#163459,#163460,#163461,
#163462,#163463),.UNSPECIFIED.,.F.,.F.,(4,2,4),(7.73312172257338E-11,0.0129043685463946,
0.0270905603278464),.UNSPECIFIED.);
#24110=B_SPLINE_CURVE_WITH_KNOTS('',3,(#163467,#163468,#163469,#163470,
#163471,#163472,#163473,#163474),.UNSPECIFIED.,.F.,.F.,(4,2,2,4),(1.00003343547171E-6,
0.0146013172580736,0.0279117435229017,0.0546218073061002),.UNSPECIFIED.);
#24111=B_SPLINE_CURVE_WITH_KNOTS('',3,(#163475,#163476,#163477,#163478,
#163479,#163480),.UNSPECIFIED.,.F.,.F.,(4,2,4),(0.000862177869507918,0.0332709228067202,
0.0654912684970968),.UNSPECIFIED.);
#24112=B_SPLINE_CURVE_WITH_KNOTS('',3,(#163481,#163482,#163483,#163484,
#163485,#163486,#163487,#163488),.UNSPECIFIED.,.F.,.F.,(4,2,2,4),(1.00000000542028E-6,
0.0322601579816196,0.048329645776346,0.0657704668609788),.UNSPECIFIED.);
#24113=B_SPLINE_CURVE_WITH_KNOTS('',3,(#163511,#163512,#163513,#163514,
#163515,#163516),.UNSPECIFIED.,.F.,.F.,(4,2,4),(0.,0.0318022366541384,0.0638030661905318),
 .UNSPECIFIED.);
#24114=B_SPLINE_CURVE_WITH_KNOTS('',3,(#163517,#163518,#163519,#163520,
#163521,#163522),.UNSPECIFIED.,.F.,.F.,(4,2,4),(1.12505063382816E-10,0.0129043685892822,
0.0270905603283878),.UNSPECIFIED.);
#24115=B_SPLINE_CURVE_WITH_KNOTS('',3,(#163526,#163527,#163528,#163529,
#163530,#163531,#163532,#163533),.UNSPECIFIED.,.F.,.F.,(4,2,2,4),(1.00012890021697E-6,
0.0146013173418215,0.0279117436722552,0.0546218076156347),.UNSPECIFIED.);
#24116=B_SPLINE_CURVE_WITH_KNOTS('',3,(#163534,#163535,#163536,#163537,
#163538,#163539),.UNSPECIFIED.,.F.,.F.,(4,2,4),(0.000862177889171675,0.0332709228033765,
0.0654912698035889),.UNSPECIFIED.);
#24117=B_SPLINE_CURVE_WITH_KNOTS('',3,(#163540,#163541,#163542,#163543,
#163544,#163545,#163546,#163547),.UNSPECIFIED.,.F.,.F.,(4,2,2,4),(1.00002679077808E-6,
0.0322596484275461,0.048328981818852,0.0657704591728584),.UNSPECIFIED.);
#24118=B_SPLINE_CURVE_WITH_KNOTS('',3,(#163570,#163571,#163572,#163573,
#163574,#163575),.UNSPECIFIED.,.F.,.F.,(4,2,4),(0.,0.0318022371744154,0.0638030681800889),
 .UNSPECIFIED.);
#24119=B_SPLINE_CURVE_WITH_KNOTS('',3,(#163576,#163577,#163578,#163579,
#163580,#163581),.UNSPECIFIED.,.F.,.F.,(4,2,4),(9.91423357346709E-11,0.0129043685986688,
0.0270905603679262),.UNSPECIFIED.);
#24120=B_SPLINE_CURVE_WITH_KNOTS('',3,(#163585,#163586,#163587,#163588,
#163589,#163590,#163591,#163592),.UNSPECIFIED.,.F.,.F.,(4,2,2,4),(1.00003733888782E-6,
0.0146013174139753,0.0279117438449331,0.0546218080025472),.UNSPECIFIED.);
#24121=B_SPLINE_CURVE_WITH_KNOTS('',3,(#163593,#163594,#163595,#163596,
#163597,#163598),.UNSPECIFIED.,.F.,.F.,(4,2,4),(0.000862177880280482,0.0332709227870337,
0.0654912695286052),.UNSPECIFIED.);
#24122=B_SPLINE_CURVE_WITH_KNOTS('',3,(#163599,#163600,#163601,#163602,
#163603,#163604,#163605,#163606),.UNSPECIFIED.,.F.,.F.,(4,2,2,4),(1.00002302923444E-6,
0.0322596484271033,0.0483289818283658,0.0657703792188617),.UNSPECIFIED.);
#24123=B_SPLINE_CURVE_WITH_KNOTS('',3,(#163629,#163630,#163631,#163632,
#163633,#163634),.UNSPECIFIED.,.F.,.F.,(4,2,4),(0.,0.0318022370000935,0.0638030675232337),
 .UNSPECIFIED.);
#24124=B_SPLINE_CURVE_WITH_KNOTS('',3,(#163635,#163636,#163637,#163638,
#163639,#163640),.UNSPECIFIED.,.F.,.F.,(4,2,4),(1.9267454212823E-10,0.0129043686879843,
0.0270905603704255),.UNSPECIFIED.);
#24125=B_SPLINE_CURVE_WITH_KNOTS('',3,(#163644,#163645,#163646,#163647,
#163648,#163649,#163650,#163651),.UNSPECIFIED.,.F.,.F.,(4,2,2,4),(1.0000842295421E-6,
0.0146013174557693,0.027911743968052,0.054621808273341),.UNSPECIFIED.);
#24126=B_SPLINE_CURVE_WITH_KNOTS('',3,(#163652,#163653,#163654,#163655,
#163656,#163657),.UNSPECIFIED.,.F.,.F.,(4,2,4),(0.000862177868208357,0.0332709228138138,
0.0654912705713705),.UNSPECIFIED.);
#24127=B_SPLINE_CURVE_WITH_KNOTS('',3,(#163658,#163659,#163660,#163661,
#163662,#163663,#163664,#163665),.UNSPECIFIED.,.F.,.F.,(4,2,2,4),(1.00002005209412E-6,
0.0322596484007827,0.0483289817025159,0.0657704465338113),.UNSPECIFIED.);
#24128=B_SPLINE_CURVE_WITH_KNOTS('',3,(#163688,#163689,#163690,#163691,
#163692,#163693),.UNSPECIFIED.,.F.,.F.,(4,2,4),(0.,0.0318022365057461,0.0638030656639669),
 .UNSPECIFIED.);
#24129=B_SPLINE_CURVE_WITH_KNOTS('',3,(#163694,#163695,#163696,#163697,
#163698,#163699),.UNSPECIFIED.,.F.,.F.,(4,2,4),(1.33958587895767E-10,0.0129043686200364,
0.0270905603446428),.UNSPECIFIED.);
#24130=B_SPLINE_CURVE_WITH_KNOTS('',3,(#163703,#163704,#163705,#163706,
#163707,#163708,#163709,#163710),.UNSPECIFIED.,.F.,.F.,(4,2,2,4),(1.00011780482097E-6,
0.0146013173060188,0.0279117436337659,0.0546218075428107),.UNSPECIFIED.);
#24131=B_SPLINE_CURVE_WITH_KNOTS('',3,(#163711,#163712,#163713,#163714,
#163715,#163716),.UNSPECIFIED.,.F.,.F.,(4,2,4),(0.000862177886576435,0.0332709227901183,
0.065491269651234),.UNSPECIFIED.);
#24132=B_SPLINE_CURVE_WITH_KNOTS('',3,(#163717,#163718,#163719,#163720,
#163721,#163722,#163723,#163724),.UNSPECIFIED.,.F.,.F.,(4,2,2,4),(1.00003164852966E-6,
0.0322596484125287,0.0483289818412921,0.0657704875195388),.UNSPECIFIED.);
#24133=B_SPLINE_CURVE_WITH_KNOTS('',3,(#163747,#163748,#163749,#163750,
#163751,#163752),.UNSPECIFIED.,.F.,.F.,(4,2,4),(0.,0.0318022371619141,0.0638030681403605),
 .UNSPECIFIED.);
#24134=B_SPLINE_CURVE_WITH_KNOTS('',3,(#163753,#163754,#163755,#163756,
#163757,#163758),.UNSPECIFIED.,.F.,.F.,(4,2,4),(1.31137303927657E-10,0.0129043686309504,
0.0270905603876553),.UNSPECIFIED.);
#24135=B_SPLINE_CURVE_WITH_KNOTS('',3,(#163762,#163763,#163764,#163765,
#163766,#163767,#163768,#163769),.UNSPECIFIED.,.F.,.F.,(4,2,2,4),(1.0000066045744E-6,
0.0146013173014613,0.0279117436224652,0.0546218075309517),.UNSPECIFIED.);
#24136=B_SPLINE_CURVE_WITH_KNOTS('',3,(#163770,#163771,#163772,#163773,
#163774,#163775),.UNSPECIFIED.,.F.,.F.,(4,2,4),(0.000862177872504536,0.0332709228002364,
0.0654912680611743),.UNSPECIFIED.);
#24137=B_SPLINE_CURVE_WITH_KNOTS('',3,(#163776,#163777,#163778,#163779,
#163780,#163781,#163782,#163783),.UNSPECIFIED.,.F.,.F.,(4,2,2,4),(1.00000000502476E-6,
0.0322601580199571,0.0483296459045163,0.0657704340761967),.UNSPECIFIED.);
#24138=B_SPLINE_CURVE_WITH_KNOTS('',3,(#163806,#163807,#163808,#163809,
#163810,#163811),.UNSPECIFIED.,.F.,.F.,(4,2,4),(0.,0.0318022370629207,0.0638030677192703),
 .UNSPECIFIED.);
#24139=B_SPLINE_CURVE_WITH_KNOTS('',3,(#163812,#163813,#163814,#163815,
#163816,#163817),.UNSPECIFIED.,.F.,.F.,(4,2,4),(4.43721061285751E-11,0.0129043685092561,
0.0270905603194748),.UNSPECIFIED.);
#24140=B_SPLINE_CURVE_WITH_KNOTS('',3,(#163821,#163822,#163823,#163824,
#163825,#163826,#163827,#163828),.UNSPECIFIED.,.F.,.F.,(4,2,2,4),(1.00005818709817E-6,
0.0146013174074703,0.0279117438604932,0.0546218080317429),.UNSPECIFIED.);
#24141=B_SPLINE_CURVE_WITH_KNOTS('',3,(#163829,#163830,#163831,#163832,
#163833,#163834),.UNSPECIFIED.,.F.,.F.,(4,2,4),(0.000862177872220941,0.0332709228215002,
0.0654912694033259),.UNSPECIFIED.);
#24142=B_SPLINE_CURVE_WITH_KNOTS('',3,(#163835,#163836,#163837,#163838,
#163839,#163840,#163841,#163842),.UNSPECIFIED.,.F.,.F.,(4,2,2,4),(1.0000220664601E-6,
0.0322596483992001,0.0483289818283565,0.0657704757709717),.UNSPECIFIED.);
#24143=B_SPLINE_CURVE_WITH_KNOTS('',3,(#163865,#163866,#163867,#163868,
#163869,#163870),.UNSPECIFIED.,.F.,.F.,(4,2,4),(0.,0.031802236674665,0.0638030662404222),
 .UNSPECIFIED.);
#24144=B_SPLINE_CURVE_WITH_KNOTS('',3,(#163871,#163872,#163873,#163874,
#163875,#163876),.UNSPECIFIED.,.F.,.F.,(4,2,4),(9.38720859421175E-11,0.0129043685919122,
0.0270905603839031),.UNSPECIFIED.);
#24145=B_SPLINE_CURVE_WITH_KNOTS('',3,(#163880,#163881,#163882,#163883,
#163884,#163885,#163886,#163887),.UNSPECIFIED.,.F.,.F.,(4,2,2,4),(1.00004272345226E-6,
0.0146013174276833,0.0279117439161975,0.0546218081690105),.UNSPECIFIED.);
#24146=B_SPLINE_CURVE_WITH_KNOTS('',3,(#163888,#163889,#163890,#163891,
#163892,#163893),.UNSPECIFIED.,.F.,.F.,(4,2,4),(0.000862177861840343,0.0332709228033376,
0.065491269533001),.UNSPECIFIED.);
#24147=B_SPLINE_CURVE_WITH_KNOTS('',3,(#163894,#163895,#163896,#163897,
#163898,#163899,#163900,#163901),.UNSPECIFIED.,.F.,.F.,(4,2,2,4),(1.00003187443489E-6,
0.0322596484212709,0.0483289818280934,0.0657704966481162),.UNSPECIFIED.);
#24148=B_SPLINE_CURVE_WITH_KNOTS('',3,(#163924,#163925,#163926,#163927,
#163928,#163929),.UNSPECIFIED.,.F.,.F.,(4,2,4),(0.,0.0318022372878971,0.0638030686367771),
 .UNSPECIFIED.);
#24149=B_SPLINE_CURVE_WITH_KNOTS('',3,(#163930,#163931,#163932,#163933,
#163934,#163935),.UNSPECIFIED.,.F.,.F.,(4,2,4),(2.19837355546419E-10,0.0129043687148192,
0.0270905603643064),.UNSPECIFIED.);
#24150=B_SPLINE_CURVE_WITH_KNOTS('',3,(#163939,#163940,#163941,#163942,
#163943,#163944,#163945,#163946),.UNSPECIFIED.,.F.,.F.,(4,2,2,4),(1.00004875114485E-6,
0.0146013172814568,0.0279117435857797,0.0546218074509637),.UNSPECIFIED.);
#24151=B_SPLINE_CURVE_WITH_KNOTS('',3,(#163947,#163948,#163949,#163950,
#163951,#163952),.UNSPECIFIED.,.F.,.F.,(4,2,4),(0.000862177878349837,0.033270922788406,
0.065491269431635),.UNSPECIFIED.);
#24152=B_SPLINE_CURVE_WITH_KNOTS('',3,(#163953,#163954,#163955,#163956,
#163957,#163958,#163959,#163960),.UNSPECIFIED.,.F.,.F.,(4,2,2,4),(1.00000000494149E-6,
0.0322601580319804,0.0483296458311714,0.065770462953049),.UNSPECIFIED.);
#24153=B_SPLINE_CURVE_WITH_KNOTS('',3,(#163983,#163984,#163985,#163986,
#163987,#163988),.UNSPECIFIED.,.F.,.F.,(4,2,4),(0.,0.0318022369064364,0.0638030671624213),
 .UNSPECIFIED.);
#24154=B_SPLINE_CURVE_WITH_KNOTS('',3,(#163989,#163990,#163991,#163992,
#163993,#163994),.UNSPECIFIED.,.F.,.F.,(4,2,4),(9.32625206027885E-11,0.0129043685655828,
0.0270905603109179),.UNSPECIFIED.);
#24155=B_SPLINE_CURVE_WITH_KNOTS('',3,(#163998,#163999,#164000,#164001,
#164002,#164003,#164004,#164005),.UNSPECIFIED.,.F.,.F.,(4,2,2,4),(1.00008320850672E-6,
0.0146013173354036,0.0279117437282217,0.0546218077522595),.UNSPECIFIED.);
#24156=B_SPLINE_CURVE_WITH_KNOTS('',3,(#164006,#164007,#164008,#164009,
#164010,#164011),.UNSPECIFIED.,.F.,.F.,(4,2,4),(0.000862177875794326,0.0332709228033271,
0.0654912704313143),.UNSPECIFIED.);
#24157=B_SPLINE_CURVE_WITH_KNOTS('',3,(#164012,#164013,#164014,#164015,
#164016,#164017,#164018,#164019),.UNSPECIFIED.,.F.,.F.,(4,2,2,4),(1.00002037827966E-6,
0.0322596484166018,0.048328981784968,0.0657704224707429),.UNSPECIFIED.);
#24158=B_SPLINE_CURVE_WITH_KNOTS('',3,(#164042,#164043,#164044,#164045,
#164046,#164047),.UNSPECIFIED.,.F.,.F.,(4,2,4),(0.,0.0318022367084148,0.0638030663573333),
 .UNSPECIFIED.);
#24159=B_SPLINE_CURVE_WITH_KNOTS('',3,(#164048,#164049,#164050,#164051,
#164052,#164053),.UNSPECIFIED.,.F.,.F.,(4,2,4),(7.39165248157004E-11,0.0129043685471262,
0.0270905603326953),.UNSPECIFIED.);
#24160=B_SPLINE_CURVE_WITH_KNOTS('',3,(#164056,#164057,#164058,#164059,
#164060,#164061,#164062,#164063),.UNSPECIFIED.,.F.,.F.,(4,2,2,4),(1.00001038055159E-6,
0.0322596485761878,0.0483293807899552,0.065770445007709),.UNSPECIFIED.);
#24161=B_SPLINE_CURVE_WITH_KNOTS('',3,(#164065,#164066,#164067,#164068,
#164069,#164070,#164071,#164072),.UNSPECIFIED.,.F.,.F.,(4,2,2,4),(1.00011510446344E-6,
0.0146013172123083,0.0279117434572996,0.0546218071857167),.UNSPECIFIED.);
#24162=B_SPLINE_CURVE_WITH_KNOTS('',3,(#164073,#164074,#164075,#164076,
#164077,#164078),.UNSPECIFIED.,.F.,.F.,(4,2,4),(0.000862177870731658,0.033270922780569,
0.065491269410436),.UNSPECIFIED.);
#24163=B_SPLINE_CURVE_WITH_KNOTS('',3,(#164101,#164102,#164103,#164104,
#164105,#164106),.UNSPECIFIED.,.F.,.F.,(4,2,4),(0.,0.0318022372306193,0.063803068414536),
 .UNSPECIFIED.);
#24164=B_SPLINE_CURVE_WITH_KNOTS('',3,(#164107,#164108,#164109,#164110,
#164111,#164112),.UNSPECIFIED.,.F.,.F.,(4,2,4),(1.92328310124429E-11,0.0129043684699768,
0.027090560300435),.UNSPECIFIED.);
#24165=B_SPLINE_CURVE_WITH_KNOTS('',3,(#164116,#164117,#164118,#164119,
#164120,#164121,#164122,#164123),.UNSPECIFIED.,.F.,.F.,(4,2,2,4),(1.00002463706826E-6,
0.0146013173736547,0.0279117437525558,0.0546218077972195),.UNSPECIFIED.);
#24166=B_SPLINE_CURVE_WITH_KNOTS('',3,(#164124,#164125,#164126,#164127,
#164128,#164129),.UNSPECIFIED.,.F.,.F.,(4,2,4),(0.000862177875615986,0.0332709227871561,
0.0654912687910421),.UNSPECIFIED.);
#24167=B_SPLINE_CURVE_WITH_KNOTS('',3,(#164130,#164131,#164132,#164133,
#164134,#164135,#164136,#164137),.UNSPECIFIED.,.F.,.F.,(4,2,2,4),(1.00002578894445E-6,
0.0322596484058082,0.0483289818206998,0.0657704182650545),.UNSPECIFIED.);
#24168=B_SPLINE_CURVE_WITH_KNOTS('',3,(#164160,#164161,#164162,#164163,
#164164,#164165),.UNSPECIFIED.,.F.,.F.,(4,2,4),(0.,0.0318022368777994,0.0638030670912566),
 .UNSPECIFIED.);
#24169=B_SPLINE_CURVE_WITH_KNOTS('',3,(#164166,#164167,#164168,#164169,
#164170,#164171),.UNSPECIFIED.,.F.,.F.,(4,2,4),(2.9932138542956E-11,0.012904368491281,
0.0270905603178472),.UNSPECIFIED.);
#24170=B_SPLINE_CURVE_WITH_KNOTS('',3,(#164175,#164176,#164177,#164178,
#164179,#164180,#164181,#164182),.UNSPECIFIED.,.F.,.F.,(4,2,2,4),(1.00006907438983E-6,
0.0146013172290565,0.0279117434657564,0.0546218071603638),.UNSPECIFIED.);
#24171=B_SPLINE_CURVE_WITH_KNOTS('',3,(#164183,#164184,#164185,#164186,
#164187,#164188),.UNSPECIFIED.,.F.,.F.,(4,2,4),(0.000862177872540946,0.03327092279438,
0.0654912686680073),.UNSPECIFIED.);
#24172=B_SPLINE_CURVE_WITH_KNOTS('',3,(#164189,#164190,#164191,#164192,
#164193,#164194,#164195,#164196),.UNSPECIFIED.,.F.,.F.,(4,2,2,4),(1.00002232148558E-6,
0.0322596483697194,0.0483289817513477,0.0657704552935119),.UNSPECIFIED.);
#24173=B_SPLINE_CURVE_WITH_KNOTS('',3,(#164219,#164220,#164221,#164222,
#164223,#164224),.UNSPECIFIED.,.F.,.F.,(4,2,4),(0.,0.0318022367095504,0.0638030663978886),
 .UNSPECIFIED.);
#24174=B_SPLINE_CURVE_WITH_KNOTS('',3,(#164225,#164226,#164227,#164228,
#164229,#164230),.UNSPECIFIED.,.F.,.F.,(4,2,4),(5.38220907370343E-11,0.0129043685342898,
0.0270905603303698),.UNSPECIFIED.);
#24175=B_SPLINE_CURVE_WITH_KNOTS('',3,(#164234,#164235,#164236,#164237,
#164238,#164239,#164240,#164241),.UNSPECIFIED.,.F.,.F.,(4,2,2,4),(1.00004428863022E-6,
0.014601317347221,0.0279117437015493,0.0546218077194452),.UNSPECIFIED.);
#24176=B_SPLINE_CURVE_WITH_KNOTS('',3,(#164242,#164243,#164244,#164245,
#164246,#164247),.UNSPECIFIED.,.F.,.F.,(4,2,4),(0.00086217787073894,0.0332709228103609,
0.0654912690057304),.UNSPECIFIED.);
#24177=B_SPLINE_CURVE_WITH_KNOTS('',3,(#164248,#164249,#164250,#164251,
#164252,#164253,#164254,#164255),.UNSPECIFIED.,.F.,.F.,(4,2,2,4),(1.00001042848546E-6,
0.0322596485825745,0.0483293807633492,0.0657704522279636),.UNSPECIFIED.);
#24178=B_SPLINE_CURVE_WITH_KNOTS('',3,(#164276,#164277,#164278,#164279,
#164280,#164281),.UNSPECIFIED.,.F.,.F.,(4,2,4),(6.02571216718838E-11,0.0129043685074554,
0.0270905602953015),.UNSPECIFIED.);
#24179=B_SPLINE_CURVE_WITH_KNOTS('',3,(#164304,#164305,#164306,#164307,
#164308,#164309),.UNSPECIFIED.,.F.,.F.,(4,2,4),(0.,0.0318022370128911,0.0638030676050469),
 .UNSPECIFIED.);
#24180=B_SPLINE_CURVE_WITH_KNOTS('',3,(#164310,#164311,#164312,#164313,
#164314,#164315),.UNSPECIFIED.,.F.,.F.,(4,2,4),(8.5531026078725E-11,0.0129043685353172,
0.0270905602920881),.UNSPECIFIED.);
#24181=B_SPLINE_CURVE_WITH_KNOTS('',3,(#164319,#164320,#164321,#164322,
#164323,#164324,#164325,#164326),.UNSPECIFIED.,.F.,.F.,(4,2,2,4),(1.00002113419786E-6,
0.0146013173396389,0.0279117436545904,0.0546218075733236),.UNSPECIFIED.);
#24182=B_SPLINE_CURVE_WITH_KNOTS('',3,(#164327,#164328,#164329,#164330,
#164331,#164332),.UNSPECIFIED.,.F.,.F.,(4,2,4),(0.000862177868521618,0.0332709227807087,
0.0654912686615231),.UNSPECIFIED.);
#24183=B_SPLINE_CURVE_WITH_KNOTS('',3,(#164333,#164334,#164335,#164336,
#164337,#164338,#164339,#164340),.UNSPECIFIED.,.F.,.F.,(4,2,2,4),(1.00002253887209E-6,
0.0322596484176829,0.0483289817265474,0.0657704408776146),.UNSPECIFIED.);
#24184=B_SPLINE_CURVE_WITH_KNOTS('',3,(#164363,#164364,#164365,#164366,
#164367,#164368),.UNSPECIFIED.,.F.,.F.,(4,2,4),(0.,0.0318022368415226,0.0638030668558906),
 .UNSPECIFIED.);
#24185=B_SPLINE_CURVE_WITH_KNOTS('',3,(#164369,#164370,#164371,#164372,
#164373,#164374),.UNSPECIFIED.,.F.,.F.,(4,2,4),(1.91828848464759E-10,0.012904368692585,
0.0270905603822096),.UNSPECIFIED.);
#24186=B_SPLINE_CURVE_WITH_KNOTS('',3,(#164378,#164379,#164380,#164381,
#164382,#164383,#164384,#164385),.UNSPECIFIED.,.F.,.F.,(4,2,2,4),(1.00013954231101E-6,
0.0146013174437899,0.0279117439331808,0.0546218081909757),.UNSPECIFIED.);
#24187=B_SPLINE_CURVE_WITH_KNOTS('',3,(#164386,#164387,#164388,#164389,
#164390,#164391),.UNSPECIFIED.,.F.,.F.,(4,2,4),(0.000862177870883951,0.0332709228008459,
0.0654912703454599),.UNSPECIFIED.);
#24188=B_SPLINE_CURVE_WITH_KNOTS('',3,(#164392,#164393,#164394,#164395,
#164396,#164397,#164398,#164399),.UNSPECIFIED.,.F.,.F.,(4,2,2,4),(1.00001951865821E-6,
0.032259648377015,0.0483289817988393,0.0657705274395779),.UNSPECIFIED.);
#24189=B_SPLINE_CURVE_WITH_KNOTS('',3,(#164422,#164423,#164424,#164425,
#164426,#164427),.UNSPECIFIED.,.F.,.F.,(4,2,4),(0.,0.0318022366633233,0.0638030661847201),
 .UNSPECIFIED.);
#24190=B_SPLINE_CURVE_WITH_KNOTS('',3,(#164428,#164429,#164430,#164431,
#164432,#164433),.UNSPECIFIED.,.F.,.F.,(4,2,4),(1.65661467333103E-10,0.0129043686548563,
0.027090560365806),.UNSPECIFIED.);
#24191=B_SPLINE_CURVE_WITH_KNOTS('',3,(#164437,#164438,#164439,#164440,
#164441,#164442,#164443,#164444),.UNSPECIFIED.,.F.,.F.,(4,2,2,4),(1.00011334763741E-6,
0.0146013173318975,0.0279117436952686,0.0546218076709802),.UNSPECIFIED.);
#24192=B_SPLINE_CURVE_WITH_KNOTS('',3,(#164445,#164446,#164447,#164448,
#164449,#164450),.UNSPECIFIED.,.F.,.F.,(4,2,4),(0.000862177869665458,0.0332709228033468,
0.065491269792743),.UNSPECIFIED.);
#24193=B_SPLINE_CURVE_WITH_KNOTS('',3,(#164451,#164452,#164453,#164454,
#164455,#164456,#164457,#164458),.UNSPECIFIED.,.F.,.F.,(4,2,2,4),(1.00002568413595E-6,
0.0322596484404524,0.0483289818696783,0.0657704422348949),.UNSPECIFIED.);
#24194=B_SPLINE_CURVE_WITH_KNOTS('',3,(#164481,#164482,#164483,#164484,
#164485,#164486),.UNSPECIFIED.,.F.,.F.,(4,2,4),(0.,0.0318022370202324,0.0638030676475271),
 .UNSPECIFIED.);
#24195=B_SPLINE_CURVE_WITH_KNOTS('',3,(#164487,#164488,#164489,#164490,
#164491,#164492),.UNSPECIFIED.,.F.,.F.,(4,2,4),(5.2106907920701E-11,0.0129043685230414,
0.0270905603348801),.UNSPECIFIED.);
#24196=B_SPLINE_CURVE_WITH_KNOTS('',3,(#164496,#164497,#164498,#164499,
#164500,#164501,#164502,#164503),.UNSPECIFIED.,.F.,.F.,(4,2,2,4),(1.00000774691514E-6,
0.0146013173767995,0.0279117437417889,0.0546218077665882),.UNSPECIFIED.);
#24197=B_SPLINE_CURVE_WITH_KNOTS('',3,(#164504,#164505,#164506,#164507,
#164508,#164509),.UNSPECIFIED.,.F.,.F.,(4,2,4),(0.000862177887326279,0.0332709227781763,
0.0654912681008252),.UNSPECIFIED.);
#24198=B_SPLINE_CURVE_WITH_KNOTS('',3,(#164510,#164511,#164512,#164513,
#164514,#164515,#164516,#164517),.UNSPECIFIED.,.F.,.F.,(4,2,2,4),(1.00002353000188E-6,
0.0322596483765172,0.048328981748336,0.0657705087336826),.UNSPECIFIED.);
#24199=B_SPLINE_CURVE_WITH_KNOTS('',3,(#164540,#164541,#164542,#164543,
#164544,#164545),.UNSPECIFIED.,.F.,.F.,(4,2,4),(0.,0.0318022367256598,0.0638030664722531),
 .UNSPECIFIED.);
#24200=B_SPLINE_CURVE_WITH_KNOTS('',3,(#164546,#164547,#164548,#164549,
#164550,#164551),.UNSPECIFIED.,.F.,.F.,(4,2,4),(2.01278360991408E-10,0.012904368702619,
0.0270905603865655),.UNSPECIFIED.);
#24201=B_SPLINE_CURVE_WITH_KNOTS('',3,(#164555,#164556,#164557,#164558,
#164559,#164560,#164561,#164562),.UNSPECIFIED.,.F.,.F.,(4,2,2,4),(1.00005471192477E-6,
0.0146013174139742,0.0279117438576769,0.0546218080280394),.UNSPECIFIED.);
#24202=B_SPLINE_CURVE_WITH_KNOTS('',3,(#164563,#164564,#164565,#164566,
#164567,#164568),.UNSPECIFIED.,.F.,.F.,(4,2,4),(0.000862177891690164,0.033270922795287,
0.0654912693810284),.UNSPECIFIED.);
#24203=B_SPLINE_CURVE_WITH_KNOTS('',3,(#164569,#164570,#164571,#164572,
#164573,#164574,#164575,#164576),.UNSPECIFIED.,.F.,.F.,(4,2,2,4),(1.00002005877465E-6,
0.0322596483563003,0.0483289818364804,0.0657705118953467),.UNSPECIFIED.);
#24204=B_SPLINE_CURVE_WITH_KNOTS('',3,(#164599,#164600,#164601,#164602,
#164603,#164604),.UNSPECIFIED.,.F.,.F.,(4,2,4),(0.,0.0318022365359491,0.0638030657623883),
 .UNSPECIFIED.);
#24205=B_SPLINE_CURVE_WITH_KNOTS('',3,(#164605,#164606,#164607,#164608,
#164609,#164610),.UNSPECIFIED.,.F.,.F.,(4,2,4),(6.90463637186275E-11,0.012904368517414,
0.0270905602824478),.UNSPECIFIED.);
#24206=B_SPLINE_CURVE_WITH_KNOTS('',3,(#164614,#164615,#164616,#164617,
#164618,#164619,#164620,#164621),.UNSPECIFIED.,.F.,.F.,(4,2,2,4),(1.0000568146761E-6,
0.0146013172773308,0.0279117435819077,0.0546218074276922),.UNSPECIFIED.);
#24207=B_SPLINE_CURVE_WITH_KNOTS('',3,(#164622,#164623,#164624,#164625,
#164626,#164627),.UNSPECIFIED.,.F.,.F.,(4,2,4),(0.000862177887123505,0.0332709228044832,
0.0654912698592312),.UNSPECIFIED.);
#24208=B_SPLINE_CURVE_WITH_KNOTS('',3,(#164628,#164629,#164630,#164631,
#164632,#164633,#164634,#164635),.UNSPECIFIED.,.F.,.F.,(4,2,2,4),(1.00002664962971E-6,
0.0322596484345612,0.0483289817571778,0.0657704600907545),.UNSPECIFIED.);
#24209=B_SPLINE_CURVE_WITH_KNOTS('',3,(#164656,#164657,#164658,#164659,
#164660,#164661),.UNSPECIFIED.,.F.,.F.,(4,2,4),(8.0445768736485E-11,0.0129043685387808,
0.0270905603068917),.UNSPECIFIED.);
#24210=B_SPLINE_CURVE_WITH_KNOTS('',3,(#164723,#164724,#164725,#164726),
 .UNSPECIFIED.,.F.,.F.,(4,4),(1.36901751880817E-13,6.28596797410394E-5),
 .UNSPECIFIED.);
#24211=B_SPLINE_CURVE_WITH_KNOTS('',3,(#164901,#164902,#164903,#164904),
 .UNSPECIFIED.,.F.,.F.,(4,4),(2.8990353702476E-13,6.28596796479073E-5),
 .UNSPECIFIED.);
#24212=B_SPLINE_CURVE_WITH_KNOTS('',3,(#165051,#165052,#165053,#165054),
 .UNSPECIFIED.,.F.,.F.,(4,4),(1.3060029988537E-13,6.28596799494453E-5),
 .UNSPECIFIED.);
#24213=B_SPLINE_CURVE_WITH_KNOTS('',3,(#165145,#165146,#165147,#165148),
 .UNSPECIFIED.,.F.,.F.,(4,4),(2.49597551107631E-14,6.28596800970493E-5),
 .UNSPECIFIED.);
#24214=B_SPLINE_CURVE_WITH_KNOTS('',3,(#165211,#165212,#165213,#165214),
 .UNSPECIFIED.,.F.,.F.,(4,4),(5.02345579122992E-14,6.28596800978433E-5),
 .UNSPECIFIED.);
#24215=B_SPLINE_CURVE_WITH_KNOTS('',3,(#165305,#165306,#165307,#165308),
 .UNSPECIFIED.,.F.,.F.,(4,4),(2.86656754501717E-13,6.28596799612116E-5),
 .UNSPECIFIED.);
#24216=B_SPLINE_CURVE_WITH_KNOTS('',3,(#165343,#165344,#165345,#165346),
 .UNSPECIFIED.,.F.,.F.,(4,4),(1.86594799180136E-13,6.28596801443001E-5),
 .UNSPECIFIED.);
#24217=B_SPLINE_CURVE_WITH_KNOTS('',3,(#165570,#165571,#165572,#165573,
#165574,#165575,#165576,#165577,#165578,#165579),.UNSPECIFIED.,.F.,.F.,
(4,3,3,4),(1.17787866773368E-13,5.49564749796463E-5,0.000106404128884424,
0.000157852343070985),.UNSPECIFIED.);
#24218=B_SPLINE_CURVE_WITH_KNOTS('',3,(#165591,#165592,#165593,#165594,
#165595,#165596,#165597),.UNSPECIFIED.,.F.,.F.,(4,3,4),(0.0665682422880065,
0.0687940209133699,0.073654350294286),.UNSPECIFIED.);
#24219=B_SPLINE_CURVE_WITH_KNOTS('',3,(#165608,#165609,#165610,#165611,
#165612,#165613,#165614,#165615,#165616,#165617),.UNSPECIFIED.,.F.,.F.,
(4,3,3,4),(0.,1.58768507494459E-5,3.06163175981273E-5,4.53557993402422E-5),
 .UNSPECIFIED.);
#24220=B_SPLINE_CURVE_WITH_KNOTS('',3,(#165646,#165647,#165648,#165649,
#165650,#165651,#165652,#165653,#165654,#165655),.UNSPECIFIED.,.F.,.F.,
(4,3,3,4),(1.94492182330635E-11,5.49564846028493E-5,0.000106404139457275,
0.00015785234352159),.UNSPECIFIED.);
#24221=B_SPLINE_CURVE_WITH_KNOTS('',3,(#165677,#165678,#165679,#165680,
#165681,#165682,#165683),.UNSPECIFIED.,.F.,.F.,(4,3,4),(0.0665682423510953,
0.0687940209135822,0.073654350296252),.UNSPECIFIED.);
#24222=B_SPLINE_CURVE_WITH_KNOTS('',3,(#165694,#165695,#165696,#165697,
#165698,#165699,#165700,#165701,#165702,#165703),.UNSPECIFIED.,.F.,.F.,
(4,3,3,4),(0.,1.58768505414901E-5,3.06163174087771E-5,4.53557990557712E-5),
 .UNSPECIFIED.);
#24223=B_SPLINE_CURVE_WITH_KNOTS('',3,(#165732,#165733,#165734,#165735,
#165736,#165737,#165738,#165739,#165740,#165741),.UNSPECIFIED.,.F.,.F.,
(4,3,3,4),(1.99083318270911E-11,5.49564847828966E-5,0.000106404139427877,
0.00015785234326692),.UNSPECIFIED.);
#24224=B_SPLINE_CURVE_WITH_KNOTS('',3,(#165763,#165764,#165765,#165766,
#165767,#165768,#165769),.UNSPECIFIED.,.F.,.F.,(4,3,4),(0.0665682422773013,
0.068794020913582,0.0736543502945316),.UNSPECIFIED.);
#24225=B_SPLINE_CURVE_WITH_KNOTS('',3,(#165780,#165781,#165782,#165783,
#165784,#165785,#165786,#165787,#165788,#165789),.UNSPECIFIED.,.F.,.F.,
(4,3,3,4),(0.,1.58768505056132E-5,3.06163174471421E-5,4.53557992820988E-5),
 .UNSPECIFIED.);
#24226=B_SPLINE_CURVE_WITH_KNOTS('',3,(#165818,#165819,#165820,#165821,
#165822,#165823,#165824,#165825,#165826,#165827),.UNSPECIFIED.,.F.,.F.,
(4,3,3,4),(1.95992847885823E-11,5.49564849740209E-5,0.00010640413939413,
0.000157852343216646),.UNSPECIFIED.);
#24227=B_SPLINE_CURVE_WITH_KNOTS('',3,(#165849,#165850,#165851,#165852,
#165853,#165854,#165855),.UNSPECIFIED.,.F.,.F.,(4,3,4),(0.0665682422879086,
0.0687940209135822,0.0736543503049214),.UNSPECIFIED.);
#24228=B_SPLINE_CURVE_WITH_KNOTS('',3,(#165866,#165867,#165868,#165869,
#165870,#165871,#165872,#165873,#165874,#165875),.UNSPECIFIED.,.F.,.F.,
(4,3,3,4),(0.,1.58768506377367E-5,3.06163175608296E-5,4.53557993773814E-5),
 .UNSPECIFIED.);
#24229=B_SPLINE_CURVE_WITH_KNOTS('',3,(#165904,#165905,#165906,#165907,
#165908,#165909,#165910,#165911,#165912,#165913),.UNSPECIFIED.,.F.,.F.,
(4,3,3,4),(1.9227260917741E-11,5.49564846408612E-5,0.000106404139395807,
0.000157852343431087),.UNSPECIFIED.);
#24230=B_SPLINE_CURVE_WITH_KNOTS('',3,(#165935,#165936,#165937,#165938,
#165939,#165940),.UNSPECIFIED.,.F.,.F.,(4,2,4),(0.,0.0162313728147786,0.032488015400969),
 .UNSPECIFIED.);
#24231=B_SPLINE_CURVE_WITH_KNOTS('',3,(#165951,#165952,#165953,#165954,
#165955,#165956,#165957,#165958,#165959,#165960),.UNSPECIFIED.,.F.,.F.,
(4,3,3,4),(0.,1.58768507540077E-5,3.06163175287554E-5,4.53557991708055E-5),
 .UNSPECIFIED.);
#24232=B_SPLINE_CURVE_WITH_KNOTS('',3,(#165989,#165990,#165991,#165992,
#165993,#165994,#165995,#165996,#165997,#165998),.UNSPECIFIED.,.F.,.F.,
(4,3,3,4),(1.91076604433025E-11,5.49564847134886E-5,0.000106404139369031,
0.000157852343374027),.UNSPECIFIED.);
#24233=B_SPLINE_CURVE_WITH_KNOTS('',3,(#166020,#166021,#166022,#166023,
#166024,#166025,#166026),.UNSPECIFIED.,.F.,.F.,(4,3,4),(0.066568242293216,
0.0687940209135806,0.0736543503096691),.UNSPECIFIED.);
#24234=B_SPLINE_CURVE_WITH_KNOTS('',3,(#166037,#166038,#166039,#166040,
#166041,#166042,#166043,#166044,#166045,#166046),.UNSPECIFIED.,.F.,.F.,
(4,3,3,4),(0.,1.58768507491376E-5,3.06163176585412E-5,4.53557994613311E-5),
 .UNSPECIFIED.);
#24235=B_SPLINE_CURVE_WITH_KNOTS('',3,(#166075,#166076,#166077,#166078,
#166079,#166080,#166081,#166082,#166083,#166084),.UNSPECIFIED.,.F.,.F.,
(4,3,3,4),(1.94512450953462E-11,5.49564848072227E-5,0.000106404139447775,
0.000157852343402473),.UNSPECIFIED.);
#24236=B_SPLINE_CURVE_WITH_KNOTS('',3,(#166106,#166107,#166108,#166109,
#166110,#166111,#166112),.UNSPECIFIED.,.F.,.F.,(4,3,4),(0.0665682422965139,
0.0687940209135805,0.0736543502734499),.UNSPECIFIED.);
#24237=B_SPLINE_CURVE_WITH_KNOTS('',3,(#166123,#166124,#166125,#166126,
#166127,#166128,#166129,#166130,#166131,#166132),.UNSPECIFIED.,.F.,.F.,
(4,3,3,4),(0.,1.58768504200603E-5,3.06163174679481E-5,4.53557994092083E-5),
 .UNSPECIFIED.);
#24238=B_SPLINE_CURVE_WITH_KNOTS('',3,(#166161,#166162,#166163,#166164,
#166165,#166166,#166167,#166168,#166169,#166170),.UNSPECIFIED.,.F.,.F.,
(4,3,3,4),(1.97540479541651E-11,5.49564846745727E-5,0.000106404139491155,
0.00015785234371001),.UNSPECIFIED.);
#24239=B_SPLINE_CURVE_WITH_KNOTS('',3,(#166192,#166193,#166194,#166195,
#166196,#166197,#166198),.UNSPECIFIED.,.F.,.F.,(4,3,4),(0.0665682423719981,
0.0687940209135804,0.0736543503119808),.UNSPECIFIED.);
#24240=B_SPLINE_CURVE_WITH_KNOTS('',3,(#166209,#166210,#166211,#166212,
#166213,#166214,#166215,#166216,#166217,#166218),.UNSPECIFIED.,.F.,.F.,
(4,3,3,4),(0.,1.58768505877374E-5,3.06163173724542E-5,4.53557990505977E-5),
 .UNSPECIFIED.);
#24241=B_SPLINE_CURVE_WITH_KNOTS('',3,(#166247,#166248,#166249,#166250,
#166251,#166252,#166253,#166254,#166255,#166256),.UNSPECIFIED.,.F.,.F.,
(4,3,3,4),(1.93035758031966E-11,5.49564846983035E-5,0.000106404139490847,
0.000157852343630075),.UNSPECIFIED.);
#24242=B_SPLINE_CURVE_WITH_KNOTS('',3,(#166278,#166279,#166280,#166281,
#166282,#166283,#166284),.UNSPECIFIED.,.F.,.F.,(4,3,4),(0.0665682422788486,
0.0687940209135805,0.073654350296961),.UNSPECIFIED.);
#24243=B_SPLINE_CURVE_WITH_KNOTS('',3,(#166295,#166296,#166297,#166298,
#166299,#166300,#166301,#166302,#166303,#166304),.UNSPECIFIED.,.F.,.F.,
(4,3,3,4),(0.,1.58768506651977E-5,3.06163175950794E-5,4.53557994183095E-5),
 .UNSPECIFIED.);
#24244=B_SPLINE_CURVE_WITH_KNOTS('',3,(#166333,#166334,#166335,#166336,
#166337,#166338,#166339,#166340,#166341,#166342),.UNSPECIFIED.,.F.,.F.,
(4,3,3,4),(1.96543653144358E-11,5.49564848592507E-5,0.000106404139588688,
0.000157852343493213),.UNSPECIFIED.);
#24245=B_SPLINE_CURVE_WITH_KNOTS('',3,(#166364,#166365,#166366,#166367,
#166368,#166369),.UNSPECIFIED.,.F.,.F.,(4,2,4),(0.,0.0162318631985632,0.0324879936074455),
 .UNSPECIFIED.);
#24246=B_SPLINE_CURVE_WITH_KNOTS('',3,(#166380,#166381,#166382,#166383,
#166384,#166385,#166386,#166387,#166388,#166389),.UNSPECIFIED.,.F.,.F.,
(4,3,3,4),(0.,1.58768504813884E-5,3.06163176465143E-5,4.53557997050518E-5),
 .UNSPECIFIED.);
#24247=B_SPLINE_CURVE_WITH_KNOTS('',3,(#166418,#166419,#166420,#166421,
#166422,#166423,#166424,#166425,#166426,#166427),.UNSPECIFIED.,.F.,.F.,
(4,3,3,4),(1.92583943969339E-11,5.49564845470167E-5,0.000106404139345154,
0.000157852343544874),.UNSPECIFIED.);
#24248=B_SPLINE_CURVE_WITH_KNOTS('',3,(#166449,#166450,#166451,#166452,
#166453,#166454,#166455),.UNSPECIFIED.,.F.,.F.,(4,3,4),(0.066568242289363,
0.0687940209135806,0.0736543503213074),.UNSPECIFIED.);
#24249=B_SPLINE_CURVE_WITH_KNOTS('',3,(#166466,#166467,#166468,#166469,
#166470,#166471,#166472,#166473,#166474,#166475),.UNSPECIFIED.,.F.,.F.,
(4,3,3,4),(0.,1.58768507441245E-5,3.06163177021733E-5,4.53557995536538E-5),
 .UNSPECIFIED.);
#24250=B_SPLINE_CURVE_WITH_KNOTS('',3,(#166504,#166505,#166506,#166507,
#166508,#166509,#166510,#166511,#166512,#166513),.UNSPECIFIED.,.F.,.F.,
(4,3,3,4),(1.93203317729608E-11,5.4956484706313E-5,0.000106404139520639,
0.000157852343600362),.UNSPECIFIED.);
#24251=B_SPLINE_CURVE_WITH_KNOTS('',3,(#166535,#166536,#166537,#166538,
#166539,#166540),.UNSPECIFIED.,.F.,.F.,(4,2,4),(0.,0.0162313587612594,0.0324879705789074),
 .UNSPECIFIED.);
#24252=B_SPLINE_CURVE_WITH_KNOTS('',3,(#166551,#166552,#166553,#166554,
#166555,#166556,#166557,#166558,#166559,#166560),.UNSPECIFIED.,.F.,.F.,
(4,3,3,4),(0.,1.58768506403926E-5,3.06163176425318E-5,4.53557995380538E-5),
 .UNSPECIFIED.);
#24253=B_SPLINE_CURVE_WITH_KNOTS('',3,(#166589,#166590,#166591,#166592,
#166593,#166594,#166595,#166596,#166597,#166598),.UNSPECIFIED.,.F.,.F.,
(4,3,3,4),(1.95534039607494E-11,5.49564846228906E-5,0.000106404139399807,
0.000157852343557442),.UNSPECIFIED.);
#24254=B_SPLINE_CURVE_WITH_KNOTS('',3,(#166620,#166621,#166622,#166623,
#166624,#166625),.UNSPECIFIED.,.F.,.F.,(4,2,4),(3.14562329816648E-10,0.0162313566854201,
0.0324879763496492),.UNSPECIFIED.);
#24255=B_SPLINE_CURVE_WITH_KNOTS('',3,(#166636,#166637,#166638,#166639,
#166640,#166641,#166642,#166643,#166644,#166645),.UNSPECIFIED.,.F.,.F.,
(4,3,3,4),(0.,1.58768507855502E-5,3.06163176193626E-5,4.53557993467085E-5),
 .UNSPECIFIED.);
#24256=B_SPLINE_CURVE_WITH_KNOTS('',3,(#166674,#166675,#166676,#166677,
#166678,#166679,#166680,#166681,#166682,#166683),.UNSPECIFIED.,.F.,.F.,
(4,3,3,4),(2.00303227837484E-11,5.49564846133499E-5,0.000106404139235265,
0.000157852343259419),.UNSPECIFIED.);
#24257=B_SPLINE_CURVE_WITH_KNOTS('',3,(#166705,#166706,#166707,#166708,
#166709,#166710,#166711),.UNSPECIFIED.,.F.,.F.,(4,3,4),(0.0665682422875406,
0.0687940209135808,0.0736543502979871),.UNSPECIFIED.);
#24258=B_SPLINE_CURVE_WITH_KNOTS('',3,(#166722,#166723,#166724,#166725,
#166726,#166727,#166728,#166729,#166730,#166731),.UNSPECIFIED.,.F.,.F.,
(4,3,3,4),(0.,1.58768507135064E-5,3.06163176365131E-5,4.5355799453002E-5),
 .UNSPECIFIED.);
#24259=B_SPLINE_CURVE_WITH_KNOTS('',3,(#166760,#166761,#166762,#166763,
#166764,#166765,#166766,#166767,#166768,#166769),.UNSPECIFIED.,.F.,.F.,
(4,3,3,4),(1.96999729795625E-11,5.49564845850009E-5,0.000106404139251949,
0.000157852343152646),.UNSPECIFIED.);
#24260=B_SPLINE_CURVE_WITH_KNOTS('',3,(#166791,#166792,#166793,#166794,
#166795,#166796,#166797),.UNSPECIFIED.,.F.,.F.,(4,3,4),(0.0665682423196876,
0.0687940209135806,0.0736543502758461),.UNSPECIFIED.);
#24261=B_SPLINE_CURVE_WITH_KNOTS('',3,(#166808,#166809,#166810,#166811,
#166812,#166813,#166814,#166815,#166816,#166817),.UNSPECIFIED.,.F.,.F.,
(4,3,3,4),(0.,1.58768506886893E-5,3.06163176410586E-5,4.53557994868356E-5),
 .UNSPECIFIED.);
#24262=B_SPLINE_CURVE_WITH_KNOTS('',3,(#166846,#166847,#166848,#166849,
#166850,#166851,#166852,#166853,#166854,#166855),.UNSPECIFIED.,.F.,.F.,
(4,3,3,4),(1.91599846899834E-11,5.49564847847627E-5,0.00010640413932454,
0.000157852343266793),.UNSPECIFIED.);
#24263=B_SPLINE_CURVE_WITH_KNOTS('',3,(#166877,#166878,#166879,#166880,
#166881,#166882),.UNSPECIFIED.,.F.,.F.,(4,2,4),(1.23551874885213E-10,0.0162313622636938,
0.032487982563608),.UNSPECIFIED.);
#24264=B_SPLINE_CURVE_WITH_KNOTS('',3,(#166893,#166894,#166895,#166896,
#166897,#166898,#166899,#166900,#166901,#166902),.UNSPECIFIED.,.F.,.F.,
(4,3,3,4),(0.,1.58768507290829E-5,3.06163176207548E-5,4.5355799405801E-5),
 .UNSPECIFIED.);
#24265=B_SPLINE_CURVE_WITH_KNOTS('',3,(#166931,#166932,#166933,#166934,
#166935,#166936,#166937,#166938,#166939,#166940),.UNSPECIFIED.,.F.,.F.,
(4,3,3,4),(1.96998203546808E-11,5.49564848806434E-5,0.000106404139564187,
0.000157852343588196),.UNSPECIFIED.);
#24266=B_SPLINE_CURVE_WITH_KNOTS('',3,(#166962,#166963,#166964,#166965,
#166966,#166967),.UNSPECIFIED.,.F.,.F.,(4,2,4),(0.,0.0162318638811279,0.0324879967796798),
 .UNSPECIFIED.);
#24267=B_SPLINE_CURVE_WITH_KNOTS('',3,(#166978,#166979,#166980,#166981,
#166982,#166983,#166984,#166985,#166986,#166987),.UNSPECIFIED.,.F.,.F.,
(4,3,3,4),(0.,1.58768505079052E-5,3.06163175682341E-5,4.53557995219932E-5),
 .UNSPECIFIED.);
#24268=B_SPLINE_CURVE_WITH_KNOTS('',3,(#167016,#167017,#167018,#167019,
#167020,#167021,#167022,#167023,#167024,#167025),.UNSPECIFIED.,.F.,.F.,
(4,3,3,4),(1.95048878554873E-11,5.4956484780533E-5,0.0001064041395414,0.000157852343523395),
 .UNSPECIFIED.);
#24269=B_SPLINE_CURVE_WITH_KNOTS('',3,(#167047,#167048,#167049,#167050,
#167051,#167052,#167053),.UNSPECIFIED.,.F.,.F.,(4,3,4),(0.0665682423833946,
0.068794020913582,0.0736543503054048),.UNSPECIFIED.);
#24270=B_SPLINE_CURVE_WITH_KNOTS('',3,(#167064,#167065,#167066,#167067,
#167068,#167069,#167070,#167071,#167072,#167073),.UNSPECIFIED.,.F.,.F.,
(4,3,3,4),(0.,1.5876850585908E-5,3.06163176069253E-5,4.53557993666698E-5),
 .UNSPECIFIED.);
#24271=B_SPLINE_CURVE_WITH_KNOTS('',3,(#167102,#167103,#167104,#167105,
#167106,#167107,#167108,#167109,#167110,#167111),.UNSPECIFIED.,.F.,.F.,
(4,3,3,4),(1.97016435778415E-11,5.49564846894979E-5,0.000106404139460024,
0.000157852343464582),.UNSPECIFIED.);
#24272=B_SPLINE_CURVE_WITH_KNOTS('',3,(#167133,#167134,#167135,#167136,
#167137,#167138,#167139),.UNSPECIFIED.,.F.,.F.,(4,3,4),(0.0665682421563453,
0.0687940209135813,0.0736543502745496),.UNSPECIFIED.);
#24273=B_SPLINE_CURVE_WITH_KNOTS('',3,(#167150,#167151,#167152,#167153,
#167154,#167155,#167156,#167157,#167158,#167159),.UNSPECIFIED.,.F.,.F.,
(4,3,3,4),(0.,1.58768505916532E-5,3.06163175413448E-5,4.53557993844558E-5),
 .UNSPECIFIED.);
#24274=B_SPLINE_CURVE_WITH_KNOTS('',3,(#167188,#167189,#167190,#167191,
#167192,#167193,#167194,#167195,#167196,#167197),.UNSPECIFIED.,.F.,.F.,
(4,3,3,4),(1.99325371145902E-11,5.49564848457451E-5,0.000106404139306774,
0.000157852343170209),.UNSPECIFIED.);
#24275=B_SPLINE_CURVE_WITH_KNOTS('',3,(#167219,#167220,#167221,#167222,
#167223,#167224,#167225),.UNSPECIFIED.,.F.,.F.,(4,3,4),(0.0665682423052219,
0.0687940209135831,0.0736543502899574),.UNSPECIFIED.);
#24276=B_SPLINE_CURVE_WITH_KNOTS('',3,(#167236,#167237,#167238,#167239,
#167240,#167241,#167242,#167243,#167244,#167245),.UNSPECIFIED.,.F.,.F.,
(4,3,3,4),(0.,1.58768506225724E-5,3.06163176219113E-5,4.53557994801334E-5),
 .UNSPECIFIED.);
#24277=B_SPLINE_CURVE_WITH_KNOTS('',3,(#167274,#167275,#167276,#167277,
#167278,#167279,#167280,#167281,#167282,#167283),.UNSPECIFIED.,.F.,.F.,
(4,3,3,4),(1.97900793505604E-11,5.49564847299566E-5,0.00010640413938352,
0.000157852343353258),.UNSPECIFIED.);
#24278=B_SPLINE_CURVE_WITH_KNOTS('',3,(#167305,#167306,#167307,#167308,
#167309,#167310),.UNSPECIFIED.,.F.,.F.,(4,2,4),(3.3528454241449E-10,0.0162318622754898,
0.0324879964841344),.UNSPECIFIED.);
#24279=B_SPLINE_CURVE_WITH_KNOTS('',3,(#167321,#167322,#167323,#167324,
#167325,#167326,#167327,#167328,#167329,#167330),.UNSPECIFIED.,.F.,.F.,
(4,3,3,4),(0.,1.58768505730015E-5,3.06163175841791E-5,4.53557994200099E-5),
 .UNSPECIFIED.);
#24280=B_SPLINE_CURVE_WITH_KNOTS('',3,(#167359,#167360,#167361,#167362,
#167363,#167364,#167365,#167366,#167367,#167368),.UNSPECIFIED.,.F.,.F.,
(4,3,3,4),(1.96951086378155E-11,5.49564846772444E-5,0.000106404139348174,
0.000157852343421498),.UNSPECIFIED.);
#24281=B_SPLINE_CURVE_WITH_KNOTS('',3,(#167390,#167391,#167392,#167393,
#167394,#167395,#167396),.UNSPECIFIED.,.F.,.F.,(4,3,4),(0.0665682423954821,
0.0687940209135814,0.0736543503169011),.UNSPECIFIED.);
#24282=B_SPLINE_CURVE_WITH_KNOTS('',3,(#167407,#167408,#167409,#167410,
#167411,#167412,#167413,#167414,#167415,#167416),.UNSPECIFIED.,.F.,.F.,
(4,3,3,4),(0.,1.5876850579189E-5,3.06163176024993E-5,4.53557995192418E-5),
 .UNSPECIFIED.);
#24283=B_SPLINE_CURVE_WITH_KNOTS('',3,(#167445,#167446,#167447,#167448,
#167449,#167450,#167451,#167452,#167453,#167454),.UNSPECIFIED.,.F.,.F.,
(4,3,3,4),(1.92477551805011E-11,5.49564847799471E-5,0.000106404139341856,
0.000157852343306238),.UNSPECIFIED.);
#24284=B_SPLINE_CURVE_WITH_KNOTS('',3,(#167476,#167477,#167478,#167479,
#167480,#167481),.UNSPECIFIED.,.F.,.F.,(4,2,4),(0.,0.0162313684470647,0.0324879996631388),
 .UNSPECIFIED.);
#24285=B_SPLINE_CURVE_WITH_KNOTS('',3,(#167492,#167493,#167494,#167495,
#167496,#167497,#167498,#167499,#167500,#167501),.UNSPECIFIED.,.F.,.F.,
(4,3,3,4),(0.,1.5876850785568E-5,3.0616317651021E-5,4.53557993820318E-5),
 .UNSPECIFIED.);
#24286=B_SPLINE_CURVE_WITH_KNOTS('',3,(#167530,#167531,#167532,#167533,
#167534,#167535,#167536,#167537,#167538,#167539),.UNSPECIFIED.,.F.,.F.,
(4,3,3,4),(1.98724445707963E-11,5.49564847358756E-5,0.000106404139421232,
0.000157852343488376),.UNSPECIFIED.);
#24287=B_SPLINE_CURVE_WITH_KNOTS('',3,(#167561,#167562,#167563,#167564,
#167565,#167566,#167567),.UNSPECIFIED.,.F.,.F.,(4,3,4),(0.0665682422866777,
0.068794020913583,0.0736543502893516),.UNSPECIFIED.);
#24288=B_SPLINE_CURVE_WITH_KNOTS('',3,(#167578,#167579,#167580,#167581,
#167582,#167583,#167584,#167585,#167586,#167587),.UNSPECIFIED.,.F.,.F.,
(4,3,3,4),(0.,1.58768503791903E-5,3.06163174838833E-5,4.53557994819831E-5),
 .UNSPECIFIED.);
#24289=B_SPLINE_CURVE_WITH_KNOTS('',3,(#167616,#167617,#167618,#167619,
#167620,#167621,#167622,#167623,#167624,#167625),.UNSPECIFIED.,.F.,.F.,
(4,3,3,4),(1.99724342327927E-11,5.49564846709836E-5,0.00010640413938314,
0.000157852343341814),.UNSPECIFIED.);
#24290=B_SPLINE_CURVE_WITH_KNOTS('',3,(#167662,#167663,#167664,#167665,
#167666,#167667,#167668,#167669,#167670,#167671),.UNSPECIFIED.,.F.,.F.,
(4,3,3,4),(0.,1.58768505326137E-5,3.06163176813787E-5,4.53557996601019E-5),
 .UNSPECIFIED.);
#24291=B_SPLINE_CURVE_WITH_KNOTS('',3,(#167700,#167701,#167702,#167703,
#167704,#167705,#167706,#167707,#167708,#167709),.UNSPECIFIED.,.F.,.F.,
(4,3,3,4),(1.96441694070615E-11,5.49564848245943E-5,0.000106404139380829,
0.00015785234333938),.UNSPECIFIED.);
#24292=B_SPLINE_CURVE_WITH_KNOTS('',3,(#167731,#167732,#167733,#167734,
#167735,#167736,#167737),.UNSPECIFIED.,.F.,.F.,(4,3,4),(0.0665682422879882,
0.0687940209135823,0.0736543502940118),.UNSPECIFIED.);
#24293=B_SPLINE_CURVE_WITH_KNOTS('',3,(#167748,#167749,#167750,#167751,
#167752,#167753,#167754,#167755,#167756,#167757),.UNSPECIFIED.,.F.,.F.,
(4,3,3,4),(0.,1.58768505197501E-5,3.06163174240148E-5,4.53557992217912E-5),
 .UNSPECIFIED.);
#24294=B_SPLINE_CURVE_WITH_KNOTS('',3,(#167786,#167787,#167788,#167789,
#167790,#167791,#167792,#167793,#167794,#167795),.UNSPECIFIED.,.F.,.F.,
(4,3,3,4),(1.94539174373277E-11,5.4956484797753E-5,0.000106404139464652,
0.000157852343533767),.UNSPECIFIED.);
#24295=B_SPLINE_CURVE_WITH_KNOTS('',3,(#167817,#167818,#167819,#167820,
#167821,#167822),.UNSPECIFIED.,.F.,.F.,(4,2,4),(0.,0.0162313678326357,0.0324880090349668),
 .UNSPECIFIED.);
#24296=B_SPLINE_CURVE_WITH_KNOTS('',3,(#167833,#167834,#167835,#167836,
#167837,#167838,#167839,#167840,#167841,#167842),.UNSPECIFIED.,.F.,.F.,
(4,3,3,4),(0.,1.58768506195949E-5,3.0616317499383E-5,4.53557992726239E-5),
 .UNSPECIFIED.);
#24297=B_SPLINE_CURVE_WITH_KNOTS('',3,(#167871,#167872,#167873,#167874,
#167875,#167876,#167877,#167878,#167879,#167880),.UNSPECIFIED.,.F.,.F.,
(4,3,3,4),(1.93866854359336E-11,5.49564848580382E-5,0.000106404139413798,
0.000157852343265456),.UNSPECIFIED.);
#24298=B_SPLINE_CURVE_WITH_KNOTS('',3,(#167902,#167903,#167904,#167905,
#167906,#167907,#167908),.UNSPECIFIED.,.F.,.F.,(4,3,4),(0.0665682421712998,
0.0687940209135817,0.0736543502856294),.UNSPECIFIED.);
#24299=B_SPLINE_CURVE_WITH_KNOTS('',3,(#167919,#167920,#167921,#167922,
#167923,#167924,#167925,#167926,#167927,#167928),.UNSPECIFIED.,.F.,.F.,
(4,3,3,4),(0.,1.58768508095443E-5,3.06163176188101E-5,4.53557993214627E-5),
 .UNSPECIFIED.);
#24300=B_SPLINE_CURVE_WITH_KNOTS('',3,(#167957,#167958,#167959,#167960,
#167961,#167962,#167963,#167964,#167965,#167966),.UNSPECIFIED.,.F.,.F.,
(4,3,3,4),(1.99132794969912E-11,5.49564847506683E-5,0.000106404139384107,
0.000157852343419854),.UNSPECIFIED.);
#24301=B_SPLINE_CURVE_WITH_KNOTS('',3,(#167988,#167989,#167990,#167991,
#167992,#167993,#167994),.UNSPECIFIED.,.F.,.F.,(4,3,4),(0.0665682422923062,
0.0687940209135823,0.0736543502809432),.UNSPECIFIED.);
#24302=B_SPLINE_CURVE_WITH_KNOTS('',3,(#168005,#168006,#168007,#168008,
#168009,#168010,#168011,#168012,#168013,#168014),.UNSPECIFIED.,.F.,.F.,
(4,3,3,4),(0.,1.58768505171131E-5,3.0616317600087E-5,4.53557995764553E-5),
 .UNSPECIFIED.);
#24357=LINE('',#92440,#26445);
#24358=LINE('',#93591,#26446);
#24359=LINE('',#93608,#26447);
#24360=LINE('',#93626,#26448);
#24361=LINE('',#93633,#26449);
#24362=LINE('',#93638,#26450);
#24363=LINE('',#94169,#26451);
#24364=LINE('',#95591,#26452);
#24365=LINE('',#95626,#26453);
#24366=LINE('',#95646,#26454);
#24367=LINE('',#95674,#26455);
#24368=LINE('',#95694,#26456);
#24369=LINE('',#95722,#26457);
#24370=LINE('',#95742,#26458);
#24371=LINE('',#95770,#26459);
#24372=LINE('',#95790,#26460);
#24373=LINE('',#95818,#26461);
#24374=LINE('',#95838,#26462);
#24375=LINE('',#95866,#26463);
#24376=LINE('',#95886,#26464);
#24377=LINE('',#95911,#26465);
#24378=LINE('',#95919,#26466);
#24379=LINE('',#95947,#26467);
#24380=LINE('',#95967,#26468);
#24381=LINE('',#95995,#26469);
#24382=LINE('',#96015,#26470);
#24383=LINE('',#96043,#26471);
#24384=LINE('',#96063,#26472);
#24385=LINE('',#96091,#26473);
#24386=LINE('',#96111,#26474);
#24387=LINE('',#96139,#26475);
#24388=LINE('',#96159,#26476);
#24389=LINE('',#96187,#26477);
#24390=LINE('',#96207,#26478);
#24391=LINE('',#96235,#26479);
#24392=LINE('',#96255,#26480);
#24393=LINE('',#96283,#26481);
#24394=LINE('',#96303,#26482);
#24395=LINE('',#96331,#26483);
#24396=LINE('',#96351,#26484);
#24397=LINE('',#96379,#26485);
#24398=LINE('',#96399,#26486);
#24399=LINE('',#96427,#26487);
#24400=LINE('',#96447,#26488);
#24401=LINE('',#96475,#26489);
#24402=LINE('',#96495,#26490);
#24403=LINE('',#96523,#26491);
#24404=LINE('',#96543,#26492);
#24405=LINE('',#96571,#26493);
#24406=LINE('',#96591,#26494);
#24407=LINE('',#96619,#26495);
#24408=LINE('',#96639,#26496);
#24409=LINE('',#96667,#26497);
#24410=LINE('',#96687,#26498);
#24411=LINE('',#96715,#26499);
#24412=LINE('',#96735,#26500);
#24413=LINE('',#96763,#26501);
#24414=LINE('',#96773,#26502);
#24415=LINE('',#96811,#26503);
#24416=LINE('',#96832,#26504);
#24417=LINE('',#96859,#26505);
#24418=LINE('',#96879,#26506);
#24419=LINE('',#96907,#26507);
#24420=LINE('',#96927,#26508);
#24421=LINE('',#96957,#26509);
#24422=LINE('',#96977,#26510);
#24423=LINE('',#96988,#26511);
#24424=LINE('',#97009,#26512);
#24425=LINE('',#97024,#26513);
#24426=LINE('',#97045,#26514);
#24427=LINE('',#97060,#26515);
#24428=LINE('',#97081,#26516);
#24429=LINE('',#97096,#26517);
#24430=LINE('',#97117,#26518);
#24431=LINE('',#97132,#26519);
#24432=LINE('',#97153,#26520);
#24433=LINE('',#97168,#26521);
#24434=LINE('',#97189,#26522);
#24435=LINE('',#97204,#26523);
#24436=LINE('',#97225,#26524);
#24437=LINE('',#97240,#26525);
#24438=LINE('',#97261,#26526);
#24439=LINE('',#97276,#26527);
#24440=LINE('',#97297,#26528);
#24441=LINE('',#97312,#26529);
#24442=LINE('',#97333,#26530);
#24443=LINE('',#97348,#26531);
#24444=LINE('',#97369,#26532);
#24445=LINE('',#97384,#26533);
#24446=LINE('',#97405,#26534);
#24447=LINE('',#97420,#26535);
#24448=LINE('',#97441,#26536);
#24449=LINE('',#97455,#26537);
#24450=LINE('',#97472,#26538);
#24451=LINE('',#97483,#26539);
#24452=LINE('',#97504,#26540);
#24453=LINE('',#97519,#26541);
#24454=LINE('',#97540,#26542);
#24455=LINE('',#97555,#26543);
#24456=LINE('',#97576,#26544);
#24457=LINE('',#97591,#26545);
#24458=LINE('',#97612,#26546);
#24459=LINE('',#97627,#26547);
#24460=LINE('',#97648,#26548);
#24461=LINE('',#97663,#26549);
#24462=LINE('',#97684,#26550);
#24463=LINE('',#97699,#26551);
#24464=LINE('',#97720,#26552);
#24465=LINE('',#97735,#26553);
#24466=LINE('',#97756,#26554);
#24467=LINE('',#97771,#26555);
#24468=LINE('',#97792,#26556);
#24469=LINE('',#97807,#26557);
#24470=LINE('',#97828,#26558);
#24471=LINE('',#97843,#26559);
#24472=LINE('',#97864,#26560);
#24473=LINE('',#97879,#26561);
#24474=LINE('',#97900,#26562);
#24475=LINE('',#97915,#26563);
#24476=LINE('',#97936,#26564);
#24477=LINE('',#97951,#26565);
#24478=LINE('',#97972,#26566);
#24479=LINE('',#97992,#26567);
#24480=LINE('',#99706,#26568);
#24481=LINE('',#99739,#26569);
#24482=LINE('',#99755,#26570);
#24483=LINE('',#99788,#26571);
#24484=LINE('',#99804,#26572);
#24485=LINE('',#99837,#26573);
#24486=LINE('',#99853,#26574);
#24487=LINE('',#99886,#26575);
#24488=LINE('',#99902,#26576);
#24489=LINE('',#99935,#26577);
#24490=LINE('',#99951,#26578);
#24491=LINE('',#99984,#26579);
#24492=LINE('',#100000,#26580);
#24493=LINE('',#100033,#26581);
#24494=LINE('',#100049,#26582);
#24495=LINE('',#100082,#26583);
#24496=LINE('',#100098,#26584);
#24497=LINE('',#100131,#26585);
#24498=LINE('',#100147,#26586);
#24499=LINE('',#100180,#26587);
#24500=LINE('',#100196,#26588);
#24501=LINE('',#100229,#26589);
#24502=LINE('',#100245,#26590);
#24503=LINE('',#100278,#26591);
#24504=LINE('',#100294,#26592);
#24505=LINE('',#100327,#26593);
#24506=LINE('',#100343,#26594);
#24507=LINE('',#100376,#26595);
#24508=LINE('',#100389,#26596);
#24509=LINE('',#100404,#26597);
#24510=LINE('',#100420,#26598);
#24511=LINE('',#100453,#26599);
#24512=LINE('',#100469,#26600);
#24513=LINE('',#100502,#26601);
#24514=LINE('',#100518,#26602);
#24515=LINE('',#100551,#26603);
#24516=LINE('',#100567,#26604);
#24517=LINE('',#100600,#26605);
#24518=LINE('',#100616,#26606);
#24519=LINE('',#100649,#26607);
#24520=LINE('',#100665,#26608);
#24521=LINE('',#100698,#26609);
#24522=LINE('',#100714,#26610);
#24523=LINE('',#100747,#26611);
#24524=LINE('',#100763,#26612);
#24525=LINE('',#100796,#26613);
#24526=LINE('',#100812,#26614);
#24527=LINE('',#100845,#26615);
#24528=LINE('',#100861,#26616);
#24529=LINE('',#100884,#26617);
#24530=LINE('',#100902,#26618);
#24531=LINE('',#100943,#26619);
#24532=LINE('',#100959,#26620);
#24533=LINE('',#100992,#26621);
#24534=LINE('',#101008,#26622);
#24535=LINE('',#101041,#26623);
#24536=LINE('',#101057,#26624);
#24537=LINE('',#101090,#26625);
#24538=LINE('',#101102,#26626);
#24539=LINE('',#101123,#26627);
#24540=LINE('',#101143,#26628);
#24541=LINE('',#101164,#26629);
#24542=LINE('',#101184,#26630);
#24543=LINE('',#101205,#26631);
#24544=LINE('',#101225,#26632);
#24545=LINE('',#101246,#26633);
#24546=LINE('',#101266,#26634);
#24547=LINE('',#101287,#26635);
#24548=LINE('',#101307,#26636);
#24549=LINE('',#101328,#26637);
#24550=LINE('',#101348,#26638);
#24551=LINE('',#101369,#26639);
#24552=LINE('',#101389,#26640);
#24553=LINE('',#101410,#26641);
#24554=LINE('',#101430,#26642);
#24555=LINE('',#101451,#26643);
#24556=LINE('',#101471,#26644);
#24557=LINE('',#101492,#26645);
#24558=LINE('',#101512,#26646);
#24559=LINE('',#101533,#26647);
#24560=LINE('',#101553,#26648);
#24561=LINE('',#101574,#26649);
#24562=LINE('',#101594,#26650);
#24563=LINE('',#101615,#26651);
#24564=LINE('',#101635,#26652);
#24565=LINE('',#101656,#26653);
#24566=LINE('',#101676,#26654);
#24567=LINE('',#101697,#26655);
#24568=LINE('',#101717,#26656);
#24569=LINE('',#101738,#26657);
#24570=LINE('',#101758,#26658);
#24571=LINE('',#101779,#26659);
#24572=LINE('',#101799,#26660);
#24573=LINE('',#101820,#26661);
#24574=LINE('',#101840,#26662);
#24575=LINE('',#101861,#26663);
#24576=LINE('',#101881,#26664);
#24577=LINE('',#101902,#26665);
#24578=LINE('',#101922,#26666);
#24579=LINE('',#101943,#26667);
#24580=LINE('',#101962,#26668);
#24581=LINE('',#101979,#26669);
#24582=LINE('',#101991,#26670);
#24583=LINE('',#102012,#26671);
#24584=LINE('',#102032,#26672);
#24585=LINE('',#102053,#26673);
#24586=LINE('',#102073,#26674);
#24587=LINE('',#102094,#26675);
#24588=LINE('',#102114,#26676);
#24589=LINE('',#102135,#26677);
#24590=LINE('',#102155,#26678);
#24591=LINE('',#102176,#26679);
#24592=LINE('',#102196,#26680);
#24593=LINE('',#102217,#26681);
#24594=LINE('',#102237,#26682);
#24595=LINE('',#102258,#26683);
#24596=LINE('',#104190,#26684);
#24597=LINE('',#104226,#26685);
#24598=LINE('',#104239,#26686);
#24599=LINE('',#104269,#26687);
#24600=LINE('',#104282,#26688);
#24601=LINE('',#104312,#26689);
#24602=LINE('',#104325,#26690);
#24603=LINE('',#104355,#26691);
#24604=LINE('',#104368,#26692);
#24605=LINE('',#104398,#26693);
#24606=LINE('',#104411,#26694);
#24607=LINE('',#104441,#26695);
#24608=LINE('',#104454,#26696);
#24609=LINE('',#104475,#26697);
#24610=LINE('',#104482,#26698);
#24611=LINE('',#104512,#26699);
#24612=LINE('',#104525,#26700);
#24613=LINE('',#104555,#26701);
#24614=LINE('',#104568,#26702);
#24615=LINE('',#104598,#26703);
#24616=LINE('',#104611,#26704);
#24617=LINE('',#104641,#26705);
#24618=LINE('',#104654,#26706);
#24619=LINE('',#104684,#26707);
#24620=LINE('',#104697,#26708);
#24621=LINE('',#104727,#26709);
#24622=LINE('',#104740,#26710);
#24623=LINE('',#104770,#26711);
#24624=LINE('',#104783,#26712);
#24625=LINE('',#104813,#26713);
#24626=LINE('',#104826,#26714);
#24627=LINE('',#104856,#26715);
#24628=LINE('',#104869,#26716);
#24629=LINE('',#104899,#26717);
#24630=LINE('',#104912,#26718);
#24631=LINE('',#104942,#26719);
#24632=LINE('',#104955,#26720);
#24633=LINE('',#104985,#26721);
#24634=LINE('',#104998,#26722);
#24635=LINE('',#105028,#26723);
#24636=LINE('',#105041,#26724);
#24637=LINE('',#105071,#26725);
#24638=LINE('',#105084,#26726);
#24639=LINE('',#105114,#26727);
#24640=LINE('',#105127,#26728);
#24641=LINE('',#105157,#26729);
#24642=LINE('',#105170,#26730);
#24643=LINE('',#105200,#26731);
#24644=LINE('',#105209,#26732);
#24645=LINE('',#105229,#26733);
#24646=LINE('',#105256,#26734);
#24647=LINE('',#105286,#26735);
#24648=LINE('',#105299,#26736);
#24649=LINE('',#105329,#26737);
#24650=LINE('',#105342,#26738);
#24651=LINE('',#105372,#26739);
#24652=LINE('',#105385,#26740);
#24653=LINE('',#105412,#26741);
#24654=LINE('',#105432,#26742);
#24655=LINE('',#105448,#26743);
#24656=LINE('',#105475,#26744);
#24657=LINE('',#105495,#26745);
#24658=LINE('',#105522,#26746);
#24659=LINE('',#105542,#26747);
#24660=LINE('',#105569,#26748);
#24661=LINE('',#105589,#26749);
#24662=LINE('',#105616,#26750);
#24663=LINE('',#105636,#26751);
#24664=LINE('',#105663,#26752);
#24665=LINE('',#105683,#26753);
#24666=LINE('',#105710,#26754);
#24667=LINE('',#105730,#26755);
#24668=LINE('',#105757,#26756);
#24669=LINE('',#105777,#26757);
#24670=LINE('',#105804,#26758);
#24671=LINE('',#105824,#26759);
#24672=LINE('',#105851,#26760);
#24673=LINE('',#105871,#26761);
#24674=LINE('',#105898,#26762);
#24675=LINE('',#105918,#26763);
#24676=LINE('',#105945,#26764);
#24677=LINE('',#105965,#26765);
#24678=LINE('',#105992,#26766);
#24679=LINE('',#106012,#26767);
#24680=LINE('',#106039,#26768);
#24681=LINE('',#106058,#26769);
#24682=LINE('',#106075,#26770);
#24683=LINE('',#106091,#26771);
#24684=LINE('',#106118,#26772);
#24685=LINE('',#106138,#26773);
#24686=LINE('',#106165,#26774);
#24687=LINE('',#106185,#26775);
#24688=LINE('',#106212,#26776);
#24689=LINE('',#106232,#26777);
#24690=LINE('',#106259,#26778);
#24691=LINE('',#106279,#26779);
#24692=LINE('',#106306,#26780);
#24693=LINE('',#106326,#26781);
#24694=LINE('',#106353,#26782);
#24695=LINE('',#106373,#26783);
#24696=LINE('',#106400,#26784);
#24697=LINE('',#106420,#26785);
#24698=LINE('',#106447,#26786);
#24699=LINE('',#106467,#26787);
#24700=LINE('',#106494,#26788);
#24701=LINE('',#106514,#26789);
#24702=LINE('',#106541,#26790);
#24703=LINE('',#106561,#26791);
#24704=LINE('',#106588,#26792);
#24705=LINE('',#106608,#26793);
#24706=LINE('',#106635,#26794);
#24707=LINE('',#106655,#26795);
#24708=LINE('',#106682,#26796);
#24709=LINE('',#106702,#26797);
#24710=LINE('',#106729,#26798);
#24711=LINE('',#106760,#26799);
#24712=LINE('',#108631,#26800);
#24713=LINE('',#108647,#26801);
#24714=LINE('',#108667,#26802);
#24715=LINE('',#108683,#26803);
#24716=LINE('',#108703,#26804);
#24717=LINE('',#108719,#26805);
#24718=LINE('',#108739,#26806);
#24719=LINE('',#108755,#26807);
#24720=LINE('',#108775,#26808);
#24721=LINE('',#108791,#26809);
#24722=LINE('',#108811,#26810);
#24723=LINE('',#108827,#26811);
#24724=LINE('',#108847,#26812);
#24725=LINE('',#108863,#26813);
#24726=LINE('',#108883,#26814);
#24727=LINE('',#108899,#26815);
#24728=LINE('',#108919,#26816);
#24729=LINE('',#108935,#26817);
#24730=LINE('',#108955,#26818);
#24731=LINE('',#108971,#26819);
#24732=LINE('',#108991,#26820);
#24733=LINE('',#109007,#26821);
#24734=LINE('',#109027,#26822);
#24735=LINE('',#109043,#26823);
#24736=LINE('',#109063,#26824);
#24737=LINE('',#109079,#26825);
#24738=LINE('',#109099,#26826);
#24739=LINE('',#109115,#26827);
#24740=LINE('',#109132,#26828);
#24741=LINE('',#109142,#26829);
#24742=LINE('',#109162,#26830);
#24743=LINE('',#109178,#26831);
#24744=LINE('',#109198,#26832);
#24745=LINE('',#109214,#26833);
#24746=LINE('',#109234,#26834);
#24747=LINE('',#109250,#26835);
#24748=LINE('',#109270,#26836);
#24749=LINE('',#109286,#26837);
#24750=LINE('',#109306,#26838);
#24751=LINE('',#109322,#26839);
#24752=LINE('',#109342,#26840);
#24753=LINE('',#109358,#26841);
#24754=LINE('',#109378,#26842);
#24755=LINE('',#109394,#26843);
#24756=LINE('',#109414,#26844);
#24757=LINE('',#109430,#26845);
#24758=LINE('',#109450,#26846);
#24759=LINE('',#109462,#26847);
#24760=LINE('',#109478,#26848);
#24761=LINE('',#109502,#26849);
#24762=LINE('',#109522,#26850);
#24763=LINE('',#109538,#26851);
#24764=LINE('',#109558,#26852);
#24765=LINE('',#109574,#26853);
#24766=LINE('',#109594,#26854);
#24767=LINE('',#109610,#26855);
#24768=LINE('',#109630,#26856);
#24769=LINE('',#109646,#26857);
#24770=LINE('',#109654,#26858);
#24771=LINE('',#109685,#26859);
#24772=LINE('',#109697,#26860);
#24773=LINE('',#109728,#26861);
#24774=LINE('',#109740,#26862);
#24775=LINE('',#109771,#26863);
#24776=LINE('',#109783,#26864);
#24777=LINE('',#109814,#26865);
#24778=LINE('',#109826,#26866);
#24779=LINE('',#109857,#26867);
#24780=LINE('',#109869,#26868);
#24781=LINE('',#109900,#26869);
#24782=LINE('',#109912,#26870);
#24783=LINE('',#109943,#26871);
#24784=LINE('',#109955,#26872);
#24785=LINE('',#109986,#26873);
#24786=LINE('',#109998,#26874);
#24787=LINE('',#110029,#26875);
#24788=LINE('',#110041,#26876);
#24789=LINE('',#110072,#26877);
#24790=LINE('',#110084,#26878);
#24791=LINE('',#110115,#26879);
#24792=LINE('',#110127,#26880);
#24793=LINE('',#110158,#26881);
#24794=LINE('',#110170,#26882);
#24795=LINE('',#110201,#26883);
#24796=LINE('',#110213,#26884);
#24797=LINE('',#110244,#26885);
#24798=LINE('',#110256,#26886);
#24799=LINE('',#110287,#26887);
#24800=LINE('',#110299,#26888);
#24801=LINE('',#110330,#26889);
#24802=LINE('',#110342,#26890);
#24803=LINE('',#110373,#26891);
#24804=LINE('',#110385,#26892);
#24805=LINE('',#110416,#26893);
#24806=LINE('',#110428,#26894);
#24807=LINE('',#110459,#26895);
#24808=LINE('',#110471,#26896);
#24809=LINE('',#110502,#26897);
#24810=LINE('',#110514,#26898);
#24811=LINE('',#110545,#26899);
#24812=LINE('',#110557,#26900);
#24813=LINE('',#110588,#26901);
#24814=LINE('',#110600,#26902);
#24815=LINE('',#110631,#26903);
#24816=LINE('',#110643,#26904);
#24817=LINE('',#110674,#26905);
#24818=LINE('',#110686,#26906);
#24819=LINE('',#110717,#26907);
#24820=LINE('',#110729,#26908);
#24821=LINE('',#110760,#26909);
#24822=LINE('',#110772,#26910);
#24823=LINE('',#110803,#26911);
#24824=LINE('',#110815,#26912);
#24825=LINE('',#110846,#26913);
#24826=LINE('',#110858,#26914);
#24827=LINE('',#110889,#26915);
#24828=LINE('',#112357,#26916);
#24829=LINE('',#112383,#26917);
#24830=LINE('',#112409,#26918);
#24831=LINE('',#112429,#26919);
#24832=LINE('',#112455,#26920);
#24833=LINE('',#112475,#26921);
#24834=LINE('',#112501,#26922);
#24835=LINE('',#112521,#26923);
#24836=LINE('',#112547,#26924);
#24837=LINE('',#112567,#26925);
#24838=LINE('',#112593,#26926);
#24839=LINE('',#112613,#26927);
#24840=LINE('',#112639,#26928);
#24841=LINE('',#112656,#26929);
#24842=LINE('',#112667,#26930);
#24843=LINE('',#112687,#26931);
#24844=LINE('',#112713,#26932);
#24845=LINE('',#112733,#26933);
#24846=LINE('',#112759,#26934);
#24847=LINE('',#112779,#26935);
#24848=LINE('',#112805,#26936);
#24849=LINE('',#112825,#26937);
#24850=LINE('',#112851,#26938);
#24851=LINE('',#112871,#26939);
#24852=LINE('',#112897,#26940);
#24853=LINE('',#112917,#26941);
#24854=LINE('',#112943,#26942);
#24855=LINE('',#112963,#26943);
#24856=LINE('',#112989,#26944);
#24857=LINE('',#113009,#26945);
#24858=LINE('',#113035,#26946);
#24859=LINE('',#113055,#26947);
#24860=LINE('',#113081,#26948);
#24861=LINE('',#113101,#26949);
#24862=LINE('',#113127,#26950);
#24863=LINE('',#113147,#26951);
#24864=LINE('',#113173,#26952);
#24865=LINE('',#113193,#26953);
#24866=LINE('',#113219,#26954);
#24867=LINE('',#113239,#26955);
#24868=LINE('',#113265,#26956);
#24869=LINE('',#113285,#26957);
#24870=LINE('',#113311,#26958);
#24871=LINE('',#113331,#26959);
#24872=LINE('',#113357,#26960);
#24873=LINE('',#113377,#26961);
#24874=LINE('',#113390,#26962);
#24875=LINE('',#113415,#26963);
#24876=LINE('',#113449,#26964);
#24877=LINE('',#113469,#26965);
#24878=LINE('',#113495,#26966);
#24879=LINE('',#113515,#26967);
#24880=LINE('',#113541,#26968);
#24881=LINE('',#113561,#26969);
#24882=LINE('',#113587,#26970);
#24883=LINE('',#113607,#26971);
#24884=LINE('',#113633,#26972);
#24885=LINE('',#113659,#26973);
#24886=LINE('',#113673,#26974);
#24887=LINE('',#113687,#26975);
#24888=LINE('',#113708,#26976);
#24889=LINE('',#113720,#26977);
#24890=LINE('',#113741,#26978);
#24891=LINE('',#113753,#26979);
#24892=LINE('',#113774,#26980);
#24893=LINE('',#113786,#26981);
#24894=LINE('',#113807,#26982);
#24895=LINE('',#113819,#26983);
#24896=LINE('',#113840,#26984);
#24897=LINE('',#113852,#26985);
#24898=LINE('',#113873,#26986);
#24899=LINE('',#113885,#26987);
#24900=LINE('',#113906,#26988);
#24901=LINE('',#113918,#26989);
#24902=LINE('',#113939,#26990);
#24903=LINE('',#113951,#26991);
#24904=LINE('',#113972,#26992);
#24905=LINE('',#113984,#26993);
#24906=LINE('',#114005,#26994);
#24907=LINE('',#114017,#26995);
#24908=LINE('',#114038,#26996);
#24909=LINE('',#114050,#26997);
#24910=LINE('',#114071,#26998);
#24911=LINE('',#114083,#26999);
#24912=LINE('',#114104,#27000);
#24913=LINE('',#114115,#27001);
#24914=LINE('',#114132,#27002);
#24915=LINE('',#114140,#27003);
#24916=LINE('',#114161,#27004);
#24917=LINE('',#114173,#27005);
#24918=LINE('',#114194,#27006);
#24919=LINE('',#114206,#27007);
#24920=LINE('',#114227,#27008);
#24921=LINE('',#114239,#27009);
#24922=LINE('',#114260,#27010);
#24923=LINE('',#114272,#27011);
#24924=LINE('',#114293,#27012);
#24925=LINE('',#114305,#27013);
#24926=LINE('',#114326,#27014);
#24927=LINE('',#114338,#27015);
#24928=LINE('',#114359,#27016);
#24929=LINE('',#114371,#27017);
#24930=LINE('',#114392,#27018);
#24931=LINE('',#114404,#27019);
#24932=LINE('',#114425,#27020);
#24933=LINE('',#114437,#27021);
#24934=LINE('',#114458,#27022);
#24935=LINE('',#114470,#27023);
#24936=LINE('',#114491,#27024);
#24937=LINE('',#114503,#27025);
#24938=LINE('',#114524,#27026);
#24939=LINE('',#114536,#27027);
#24940=LINE('',#114557,#27028);
#24941=LINE('',#114569,#27029);
#24942=LINE('',#114590,#27030);
#24943=LINE('',#114607,#27031);
#24944=LINE('',#116251,#27032);
#24945=LINE('',#116278,#27033);
#24946=LINE('',#116298,#27034);
#24947=LINE('',#116325,#27035);
#24948=LINE('',#116345,#27036);
#24949=LINE('',#116372,#27037);
#24950=LINE('',#116392,#27038);
#24951=LINE('',#116419,#27039);
#24952=LINE('',#116439,#27040);
#24953=LINE('',#116466,#27041);
#24954=LINE('',#116486,#27042);
#24955=LINE('',#116513,#27043);
#24956=LINE('',#116533,#27044);
#24957=LINE('',#116560,#27045);
#24958=LINE('',#116580,#27046);
#24959=LINE('',#116607,#27047);
#24960=LINE('',#116627,#27048);
#24961=LINE('',#116654,#27049);
#24962=LINE('',#116674,#27050);
#24963=LINE('',#116701,#27051);
#24964=LINE('',#116721,#27052);
#24965=LINE('',#116748,#27053);
#24966=LINE('',#116768,#27054);
#24967=LINE('',#116795,#27055);
#24968=LINE('',#116815,#27056);
#24969=LINE('',#116842,#27057);
#24970=LINE('',#116862,#27058);
#24971=LINE('',#116889,#27059);
#24972=LINE('',#116906,#27060);
#24973=LINE('',#116921,#27061);
#24974=LINE('',#116941,#27062);
#24975=LINE('',#116968,#27063);
#24976=LINE('',#116988,#27064);
#24977=LINE('',#117015,#27065);
#24978=LINE('',#117035,#27066);
#24979=LINE('',#117062,#27067);
#24980=LINE('',#117082,#27068);
#24981=LINE('',#117109,#27069);
#24982=LINE('',#117129,#27070);
#24983=LINE('',#117156,#27071);
#24984=LINE('',#117176,#27072);
#24985=LINE('',#117203,#27073);
#24986=LINE('',#117223,#27074);
#24987=LINE('',#117250,#27075);
#24988=LINE('',#117270,#27076);
#24989=LINE('',#117293,#27077);
#24990=LINE('',#117309,#27078);
#24991=LINE('',#117344,#27079);
#24992=LINE('',#117364,#27080);
#24993=LINE('',#117391,#27081);
#24994=LINE('',#117411,#27082);
#24995=LINE('',#117438,#27083);
#24996=LINE('',#117458,#27084);
#24997=LINE('',#117485,#27085);
#24998=LINE('',#117505,#27086);
#24999=LINE('',#117532,#27087);
#25000=LINE('',#117552,#27088);
#25001=LINE('',#117579,#27089);
#25002=LINE('',#117591,#27090);
#25003=LINE('',#117612,#27091);
#25004=LINE('',#117628,#27092);
#25005=LINE('',#117649,#27093);
#25006=LINE('',#117665,#27094);
#25007=LINE('',#117686,#27095);
#25008=LINE('',#117702,#27096);
#25009=LINE('',#117723,#27097);
#25010=LINE('',#117739,#27098);
#25011=LINE('',#117760,#27099);
#25012=LINE('',#117776,#27100);
#25013=LINE('',#117797,#27101);
#25014=LINE('',#117813,#27102);
#25015=LINE('',#117834,#27103);
#25016=LINE('',#117850,#27104);
#25017=LINE('',#117871,#27105);
#25018=LINE('',#117887,#27106);
#25019=LINE('',#117908,#27107);
#25020=LINE('',#117924,#27108);
#25021=LINE('',#117945,#27109);
#25022=LINE('',#117961,#27110);
#25023=LINE('',#117982,#27111);
#25024=LINE('',#117998,#27112);
#25025=LINE('',#118019,#27113);
#25026=LINE('',#118035,#27114);
#25027=LINE('',#118056,#27115);
#25028=LINE('',#118072,#27116);
#25029=LINE('',#118093,#27117);
#25030=LINE('',#118109,#27118);
#25031=LINE('',#118130,#27119);
#25032=LINE('',#118146,#27120);
#25033=LINE('',#118167,#27121);
#25034=LINE('',#118183,#27122);
#25035=LINE('',#118204,#27123);
#25036=LINE('',#118220,#27124);
#25037=LINE('',#118241,#27125);
#25038=LINE('',#118257,#27126);
#25039=LINE('',#118278,#27127);
#25040=LINE('',#118294,#27128);
#25041=LINE('',#118315,#27129);
#25042=LINE('',#118331,#27130);
#25043=LINE('',#118352,#27131);
#25044=LINE('',#118367,#27132);
#25045=LINE('',#118384,#27133);
#25046=LINE('',#118396,#27134);
#25047=LINE('',#118417,#27135);
#25048=LINE('',#118433,#27136);
#25049=LINE('',#118454,#27137);
#25050=LINE('',#118470,#27138);
#25051=LINE('',#118491,#27139);
#25052=LINE('',#118507,#27140);
#25053=LINE('',#118528,#27141);
#25054=LINE('',#118544,#27142);
#25055=LINE('',#118565,#27143);
#25056=LINE('',#118581,#27144);
#25057=LINE('',#118602,#27145);
#25058=LINE('',#118618,#27146);
#25059=LINE('',#118639,#27147);
#25060=LINE('',#120741,#27148);
#25061=LINE('',#120777,#27149);
#25062=LINE('',#120790,#27150);
#25063=LINE('',#120820,#27151);
#25064=LINE('',#120833,#27152);
#25065=LINE('',#120863,#27153);
#25066=LINE('',#120876,#27154);
#25067=LINE('',#120906,#27155);
#25068=LINE('',#120919,#27156);
#25069=LINE('',#120949,#27157);
#25070=LINE('',#120962,#27158);
#25071=LINE('',#120992,#27159);
#25072=LINE('',#121005,#27160);
#25073=LINE('',#121026,#27161);
#25074=LINE('',#121033,#27162);
#25075=LINE('',#121063,#27163);
#25076=LINE('',#121076,#27164);
#25077=LINE('',#121106,#27165);
#25078=LINE('',#121119,#27166);
#25079=LINE('',#121149,#27167);
#25080=LINE('',#121162,#27168);
#25081=LINE('',#121192,#27169);
#25082=LINE('',#121205,#27170);
#25083=LINE('',#121235,#27171);
#25084=LINE('',#121248,#27172);
#25085=LINE('',#121278,#27173);
#25086=LINE('',#121291,#27174);
#25087=LINE('',#121321,#27175);
#25088=LINE('',#121334,#27176);
#25089=LINE('',#121364,#27177);
#25090=LINE('',#121377,#27178);
#25091=LINE('',#121407,#27179);
#25092=LINE('',#121420,#27180);
#25093=LINE('',#121450,#27181);
#25094=LINE('',#121463,#27182);
#25095=LINE('',#121493,#27183);
#25096=LINE('',#121506,#27184);
#25097=LINE('',#121536,#27185);
#25098=LINE('',#121549,#27186);
#25099=LINE('',#121579,#27187);
#25100=LINE('',#121592,#27188);
#25101=LINE('',#121622,#27189);
#25102=LINE('',#121635,#27190);
#25103=LINE('',#121665,#27191);
#25104=LINE('',#121674,#27192);
#25105=LINE('',#121694,#27193);
#25106=LINE('',#121721,#27194);
#25107=LINE('',#121751,#27195);
#25108=LINE('',#121764,#27196);
#25109=LINE('',#121794,#27197);
#25110=LINE('',#121807,#27198);
#25111=LINE('',#121837,#27199);
#25112=LINE('',#121850,#27200);
#25113=LINE('',#121880,#27201);
#25114=LINE('',#121893,#27202);
#25115=LINE('',#121923,#27203);
#25116=LINE('',#121936,#27204);
#25117=LINE('',#121963,#27205);
#25118=LINE('',#121979,#27206);
#25119=LINE('',#121991,#27207);
#25120=LINE('',#122014,#27208);
#25121=LINE('',#122030,#27209);
#25122=LINE('',#122053,#27210);
#25123=LINE('',#122069,#27211);
#25124=LINE('',#122092,#27212);
#25125=LINE('',#122108,#27213);
#25126=LINE('',#122131,#27214);
#25127=LINE('',#122147,#27215);
#25128=LINE('',#122170,#27216);
#25129=LINE('',#122186,#27217);
#25130=LINE('',#122209,#27218);
#25131=LINE('',#122225,#27219);
#25132=LINE('',#122248,#27220);
#25133=LINE('',#122264,#27221);
#25134=LINE('',#122287,#27222);
#25135=LINE('',#122303,#27223);
#25136=LINE('',#122326,#27224);
#25137=LINE('',#122342,#27225);
#25138=LINE('',#122365,#27226);
#25139=LINE('',#122381,#27227);
#25140=LINE('',#122404,#27228);
#25141=LINE('',#122420,#27229);
#25142=LINE('',#122443,#27230);
#25143=LINE('',#122459,#27231);
#25144=LINE('',#122482,#27232);
#25145=LINE('',#122497,#27233);
#25146=LINE('',#122510,#27234);
#25147=LINE('',#122522,#27235);
#25148=LINE('',#122545,#27236);
#25149=LINE('',#122561,#27237);
#25150=LINE('',#122584,#27238);
#25151=LINE('',#122600,#27239);
#25152=LINE('',#122623,#27240);
#25153=LINE('',#122639,#27241);
#25154=LINE('',#122662,#27242);
#25155=LINE('',#122678,#27243);
#25156=LINE('',#122701,#27244);
#25157=LINE('',#122717,#27245);
#25158=LINE('',#122740,#27246);
#25159=LINE('',#122756,#27247);
#25160=LINE('',#122779,#27248);
#25161=LINE('',#122795,#27249);
#25162=LINE('',#122818,#27250);
#25163=LINE('',#122834,#27251);
#25164=LINE('',#122857,#27252);
#25165=LINE('',#122873,#27253);
#25166=LINE('',#122896,#27254);
#25167=LINE('',#122912,#27255);
#25168=LINE('',#122935,#27256);
#25169=LINE('',#122951,#27257);
#25170=LINE('',#122974,#27258);
#25171=LINE('',#122990,#27259);
#25172=LINE('',#123013,#27260);
#25173=LINE('',#123029,#27261);
#25174=LINE('',#123052,#27262);
#25175=LINE('',#123079,#27263);
#25176=LINE('',#125098,#27264);
#25177=LINE('',#125111,#27265);
#25178=LINE('',#125131,#27266);
#25179=LINE('',#125144,#27267);
#25180=LINE('',#125164,#27268);
#25181=LINE('',#125177,#27269);
#25182=LINE('',#125197,#27270);
#25183=LINE('',#125210,#27271);
#25184=LINE('',#125230,#27272);
#25185=LINE('',#125243,#27273);
#25186=LINE('',#125263,#27274);
#25187=LINE('',#125276,#27275);
#25188=LINE('',#125296,#27276);
#25189=LINE('',#125309,#27277);
#25190=LINE('',#125329,#27278);
#25191=LINE('',#125342,#27279);
#25192=LINE('',#125362,#27280);
#25193=LINE('',#125375,#27281);
#25194=LINE('',#125395,#27282);
#25195=LINE('',#125408,#27283);
#25196=LINE('',#125428,#27284);
#25197=LINE('',#125441,#27285);
#25198=LINE('',#125461,#27286);
#25199=LINE('',#125474,#27287);
#25200=LINE('',#125494,#27288);
#25201=LINE('',#125507,#27289);
#25202=LINE('',#125527,#27290);
#25203=LINE('',#125540,#27291);
#25204=LINE('',#125557,#27292);
#25205=LINE('',#125564,#27293);
#25206=LINE('',#125584,#27294);
#25207=LINE('',#125597,#27295);
#25208=LINE('',#125617,#27296);
#25209=LINE('',#125630,#27297);
#25210=LINE('',#125650,#27298);
#25211=LINE('',#125663,#27299);
#25212=LINE('',#125683,#27300);
#25213=LINE('',#125696,#27301);
#25214=LINE('',#125716,#27302);
#25215=LINE('',#125729,#27303);
#25216=LINE('',#125749,#27304);
#25217=LINE('',#125762,#27305);
#25218=LINE('',#125782,#27306);
#25219=LINE('',#125791,#27307);
#25220=LINE('',#125807,#27308);
#25221=LINE('',#125828,#27309);
#25222=LINE('',#125848,#27310);
#25223=LINE('',#125861,#27311);
#25224=LINE('',#125881,#27312);
#25225=LINE('',#125894,#27313);
#25226=LINE('',#125914,#27314);
#25227=LINE('',#125927,#27315);
#25228=LINE('',#125947,#27316);
#25229=LINE('',#125960,#27317);
#25230=LINE('',#125980,#27318);
#25231=LINE('',#125993,#27319);
#25232=LINE('',#126013,#27320);
#25233=LINE('',#126026,#27321);
#25234=LINE('',#126038,#27322);
#25235=LINE('',#126065,#27323);
#25236=LINE('',#126081,#27324);
#25237=LINE('',#126108,#27325);
#25238=LINE('',#126124,#27326);
#25239=LINE('',#126151,#27327);
#25240=LINE('',#126167,#27328);
#25241=LINE('',#126194,#27329);
#25242=LINE('',#126210,#27330);
#25243=LINE('',#126237,#27331);
#25244=LINE('',#126253,#27332);
#25245=LINE('',#126280,#27333);
#25246=LINE('',#126296,#27334);
#25247=LINE('',#126323,#27335);
#25248=LINE('',#126339,#27336);
#25249=LINE('',#126366,#27337);
#25250=LINE('',#126382,#27338);
#25251=LINE('',#126409,#27339);
#25252=LINE('',#126425,#27340);
#25253=LINE('',#126452,#27341);
#25254=LINE('',#126468,#27342);
#25255=LINE('',#126495,#27343);
#25256=LINE('',#126511,#27344);
#25257=LINE('',#126538,#27345);
#25258=LINE('',#126554,#27346);
#25259=LINE('',#126581,#27347);
#25260=LINE('',#126597,#27348);
#25261=LINE('',#126624,#27349);
#25262=LINE('',#126640,#27350);
#25263=LINE('',#126667,#27351);
#25264=LINE('',#126683,#27352);
#25265=LINE('',#126710,#27353);
#25266=LINE('',#126726,#27354);
#25267=LINE('',#126753,#27355);
#25268=LINE('',#126769,#27356);
#25269=LINE('',#126796,#27357);
#25270=LINE('',#126812,#27358);
#25271=LINE('',#126839,#27359);
#25272=LINE('',#126855,#27360);
#25273=LINE('',#126882,#27361);
#25274=LINE('',#126898,#27362);
#25275=LINE('',#126925,#27363);
#25276=LINE('',#126940,#27364);
#25277=LINE('',#126957,#27365);
#25278=LINE('',#126969,#27366);
#25279=LINE('',#126996,#27367);
#25280=LINE('',#127012,#27368);
#25281=LINE('',#127039,#27369);
#25282=LINE('',#127055,#27370);
#25283=LINE('',#127082,#27371);
#25284=LINE('',#127098,#27372);
#25285=LINE('',#127125,#27373);
#25286=LINE('',#127141,#27374);
#25287=LINE('',#127168,#27375);
#25288=LINE('',#127184,#27376);
#25289=LINE('',#127211,#27377);
#25290=LINE('',#127227,#27378);
#25291=LINE('',#127254,#27379);
#25292=LINE('',#128722,#27380);
#25293=LINE('',#128748,#27381);
#25294=LINE('',#128765,#27382);
#25295=LINE('',#128785,#27383);
#25296=LINE('',#128802,#27384);
#25297=LINE('',#128822,#27385);
#25298=LINE('',#128839,#27386);
#25299=LINE('',#128859,#27387);
#25300=LINE('',#128876,#27388);
#25301=LINE('',#128896,#27389);
#25302=LINE('',#128913,#27390);
#25303=LINE('',#128933,#27391);
#25304=LINE('',#128950,#27392);
#25305=LINE('',#128967,#27393);
#25306=LINE('',#128978,#27394);
#25307=LINE('',#128998,#27395);
#25308=LINE('',#129015,#27396);
#25309=LINE('',#129035,#27397);
#25310=LINE('',#129052,#27398);
#25311=LINE('',#129072,#27399);
#25312=LINE('',#129089,#27400);
#25313=LINE('',#129109,#27401);
#25314=LINE('',#129126,#27402);
#25315=LINE('',#129146,#27403);
#25316=LINE('',#129163,#27404);
#25317=LINE('',#129183,#27405);
#25318=LINE('',#129200,#27406);
#25319=LINE('',#129220,#27407);
#25320=LINE('',#129237,#27408);
#25321=LINE('',#129257,#27409);
#25322=LINE('',#129274,#27410);
#25323=LINE('',#129294,#27411);
#25324=LINE('',#129311,#27412);
#25325=LINE('',#129331,#27413);
#25326=LINE('',#129348,#27414);
#25327=LINE('',#129368,#27415);
#25328=LINE('',#129385,#27416);
#25329=LINE('',#129405,#27417);
#25330=LINE('',#129422,#27418);
#25331=LINE('',#129442,#27419);
#25332=LINE('',#129459,#27420);
#25333=LINE('',#129479,#27421);
#25334=LINE('',#129492,#27422);
#25335=LINE('',#129508,#27423);
#25336=LINE('',#129533,#27424);
#25337=LINE('',#129553,#27425);
#25338=LINE('',#129570,#27426);
#25339=LINE('',#129590,#27427);
#25340=LINE('',#129607,#27428);
#25341=LINE('',#129627,#27429);
#25342=LINE('',#129644,#27430);
#25343=LINE('',#129664,#27431);
#25344=LINE('',#129681,#27432);
#25345=LINE('',#129701,#27433);
#25346=LINE('',#129718,#27434);
#25347=LINE('',#129738,#27435);
#25348=LINE('',#129755,#27436);
#25349=LINE('',#129772,#27437);
#25350=LINE('',#129788,#27438);
#25351=LINE('',#129800,#27439);
#25352=LINE('',#129817,#27440);
#25353=LINE('',#129833,#27441);
#25354=LINE('',#129850,#27442);
#25355=LINE('',#129866,#27443);
#25356=LINE('',#129883,#27444);
#25357=LINE('',#129899,#27445);
#25358=LINE('',#129916,#27446);
#25359=LINE('',#129932,#27447);
#25360=LINE('',#129949,#27448);
#25361=LINE('',#129965,#27449);
#25362=LINE('',#129982,#27450);
#25363=LINE('',#129998,#27451);
#25364=LINE('',#130015,#27452);
#25365=LINE('',#130031,#27453);
#25366=LINE('',#130048,#27454);
#25367=LINE('',#130064,#27455);
#25368=LINE('',#130081,#27456);
#25369=LINE('',#130097,#27457);
#25370=LINE('',#130114,#27458);
#25371=LINE('',#130130,#27459);
#25372=LINE('',#130147,#27460);
#25373=LINE('',#130163,#27461);
#25374=LINE('',#130180,#27462);
#25375=LINE('',#130196,#27463);
#25376=LINE('',#130213,#27464);
#25377=LINE('',#130228,#27465);
#25378=LINE('',#130241,#27466);
#25379=LINE('',#130253,#27467);
#25380=LINE('',#130270,#27468);
#25381=LINE('',#130286,#27469);
#25382=LINE('',#130303,#27470);
#25383=LINE('',#130319,#27471);
#25384=LINE('',#130336,#27472);
#25385=LINE('',#130352,#27473);
#25386=LINE('',#130369,#27474);
#25387=LINE('',#130385,#27475);
#25388=LINE('',#130402,#27476);
#25389=LINE('',#130418,#27477);
#25390=LINE('',#130435,#27478);
#25391=LINE('',#130451,#27479);
#25392=LINE('',#130468,#27480);
#25393=LINE('',#130484,#27481);
#25394=LINE('',#130501,#27482);
#25395=LINE('',#130517,#27483);
#25396=LINE('',#130534,#27484);
#25397=LINE('',#130550,#27485);
#25398=LINE('',#130567,#27486);
#25399=LINE('',#130583,#27487);
#25400=LINE('',#130600,#27488);
#25401=LINE('',#130616,#27489);
#25402=LINE('',#130633,#27490);
#25403=LINE('',#130649,#27491);
#25404=LINE('',#130666,#27492);
#25405=LINE('',#130682,#27493);
#25406=LINE('',#130699,#27494);
#25407=LINE('',#130720,#27495);
#25408=LINE('',#132652,#27496);
#25409=LINE('',#132675,#27497);
#25410=LINE('',#132691,#27498);
#25411=LINE('',#132714,#27499);
#25412=LINE('',#132730,#27500);
#25413=LINE('',#132753,#27501);
#25414=LINE('',#132769,#27502);
#25415=LINE('',#132792,#27503);
#25416=LINE('',#132808,#27504);
#25417=LINE('',#132831,#27505);
#25418=LINE('',#132847,#27506);
#25419=LINE('',#132870,#27507);
#25420=LINE('',#132886,#27508);
#25421=LINE('',#132909,#27509);
#25422=LINE('',#132925,#27510);
#25423=LINE('',#132948,#27511);
#25424=LINE('',#132964,#27512);
#25425=LINE('',#132985,#27513);
#25426=LINE('',#133001,#27514);
#25427=LINE('',#133024,#27515);
#25428=LINE('',#133040,#27516);
#25429=LINE('',#133063,#27517);
#25430=LINE('',#133079,#27518);
#25431=LINE('',#133102,#27519);
#25432=LINE('',#133118,#27520);
#25433=LINE('',#133141,#27521);
#25434=LINE('',#133157,#27522);
#25435=LINE('',#133180,#27523);
#25436=LINE('',#133193,#27524);
#25437=LINE('',#133204,#27525);
#25438=LINE('',#133220,#27526);
#25439=LINE('',#133243,#27527);
#25440=LINE('',#133259,#27528);
#25441=LINE('',#133282,#27529);
#25442=LINE('',#133298,#27530);
#25443=LINE('',#133321,#27531);
#25444=LINE('',#133337,#27532);
#25445=LINE('',#133360,#27533);
#25446=LINE('',#133376,#27534);
#25447=LINE('',#133399,#27535);
#25448=LINE('',#133415,#27536);
#25449=LINE('',#133434,#27537);
#25450=LINE('',#133446,#27538);
#25451=LINE('',#133477,#27539);
#25452=LINE('',#133493,#27540);
#25453=LINE('',#133516,#27541);
#25454=LINE('',#133532,#27542);
#25455=LINE('',#133555,#27543);
#25456=LINE('',#133571,#27544);
#25457=LINE('',#133594,#27545);
#25458=LINE('',#133610,#27546);
#25459=LINE('',#133633,#27547);
#25460=LINE('',#133649,#27548);
#25461=LINE('',#133672,#27549);
#25462=LINE('',#133688,#27550);
#25463=LINE('',#133711,#27551);
#25464=LINE('',#133727,#27552);
#25465=LINE('',#133750,#27553);
#25466=LINE('',#133758,#27554);
#25467=LINE('',#133775,#27555);
#25468=LINE('',#133787,#27556);
#25469=LINE('',#133804,#27557);
#25470=LINE('',#133816,#27558);
#25471=LINE('',#133833,#27559);
#25472=LINE('',#133845,#27560);
#25473=LINE('',#133862,#27561);
#25474=LINE('',#133874,#27562);
#25475=LINE('',#133891,#27563);
#25476=LINE('',#133903,#27564);
#25477=LINE('',#133920,#27565);
#25478=LINE('',#133932,#27566);
#25479=LINE('',#133949,#27567);
#25480=LINE('',#133961,#27568);
#25481=LINE('',#133978,#27569);
#25482=LINE('',#133990,#27570);
#25483=LINE('',#134007,#27571);
#25484=LINE('',#134019,#27572);
#25485=LINE('',#134036,#27573);
#25486=LINE('',#134048,#27574);
#25487=LINE('',#134065,#27575);
#25488=LINE('',#134077,#27576);
#25489=LINE('',#134094,#27577);
#25490=LINE('',#134106,#27578);
#25491=LINE('',#134123,#27579);
#25492=LINE('',#134135,#27580);
#25493=LINE('',#134152,#27581);
#25494=LINE('',#134164,#27582);
#25495=LINE('',#134181,#27583);
#25496=LINE('',#134193,#27584);
#25497=LINE('',#134210,#27585);
#25498=LINE('',#134222,#27586);
#25499=LINE('',#134239,#27587);
#25500=LINE('',#134251,#27588);
#25501=LINE('',#134268,#27589);
#25502=LINE('',#134280,#27590);
#25503=LINE('',#134297,#27591);
#25504=LINE('',#134309,#27592);
#25505=LINE('',#134326,#27593);
#25506=LINE('',#134338,#27594);
#25507=LINE('',#134355,#27595);
#25508=LINE('',#134367,#27596);
#25509=LINE('',#134384,#27597);
#25510=LINE('',#134396,#27598);
#25511=LINE('',#134413,#27599);
#25512=LINE('',#134425,#27600);
#25513=LINE('',#134442,#27601);
#25514=LINE('',#134454,#27602);
#25515=LINE('',#134471,#27603);
#25516=LINE('',#134483,#27604);
#25517=LINE('',#134500,#27605);
#25518=LINE('',#134512,#27606);
#25519=LINE('',#134529,#27607);
#25520=LINE('',#134541,#27608);
#25521=LINE('',#134558,#27609);
#25522=LINE('',#134570,#27610);
#25523=LINE('',#134587,#27611);
#25524=LINE('',#137321,#27612);
#25525=LINE('',#137353,#27613);
#25526=LINE('',#137370,#27614);
#25527=LINE('',#137396,#27615);
#25528=LINE('',#137413,#27616);
#25529=LINE('',#137439,#27617);
#25530=LINE('',#137456,#27618);
#25531=LINE('',#137482,#27619);
#25532=LINE('',#137499,#27620);
#25533=LINE('',#137525,#27621);
#25534=LINE('',#137542,#27622);
#25535=LINE('',#137568,#27623);
#25536=LINE('',#137585,#27624);
#25537=LINE('',#137602,#27625);
#25538=LINE('',#137613,#27626);
#25539=LINE('',#137639,#27627);
#25540=LINE('',#137656,#27628);
#25541=LINE('',#137682,#27629);
#25542=LINE('',#137699,#27630);
#25543=LINE('',#137725,#27631);
#25544=LINE('',#137742,#27632);
#25545=LINE('',#137768,#27633);
#25546=LINE('',#137785,#27634);
#25547=LINE('',#137811,#27635);
#25548=LINE('',#137828,#27636);
#25549=LINE('',#137854,#27637);
#25550=LINE('',#137871,#27638);
#25551=LINE('',#137897,#27639);
#25552=LINE('',#137914,#27640);
#25553=LINE('',#137940,#27641);
#25554=LINE('',#137957,#27642);
#25555=LINE('',#137983,#27643);
#25556=LINE('',#138000,#27644);
#25557=LINE('',#138026,#27645);
#25558=LINE('',#138043,#27646);
#25559=LINE('',#138069,#27647);
#25560=LINE('',#138086,#27648);
#25561=LINE('',#138112,#27649);
#25562=LINE('',#138129,#27650);
#25563=LINE('',#138155,#27651);
#25564=LINE('',#138168,#27652);
#25565=LINE('',#138184,#27653);
#25566=LINE('',#138215,#27654);
#25567=LINE('',#138241,#27655);
#25568=LINE('',#138258,#27656);
#25569=LINE('',#138284,#27657);
#25570=LINE('',#138301,#27658);
#25571=LINE('',#138327,#27659);
#25572=LINE('',#138344,#27660);
#25573=LINE('',#138370,#27661);
#25574=LINE('',#138387,#27662);
#25575=LINE('',#138413,#27663);
#25576=LINE('',#138430,#27664);
#25577=LINE('',#138456,#27665);
#25578=LINE('',#138473,#27666);
#25579=LINE('',#138499,#27667);
#25580=LINE('',#138516,#27668);
#25581=LINE('',#138539,#27669);
#25582=LINE('',#138559,#27670);
#25583=LINE('',#138571,#27671);
#25584=LINE('',#138598,#27672);
#25585=LINE('',#138614,#27673);
#25586=LINE('',#138641,#27674);
#25587=LINE('',#138657,#27675);
#25588=LINE('',#138684,#27676);
#25589=LINE('',#138700,#27677);
#25590=LINE('',#138727,#27678);
#25591=LINE('',#138743,#27679);
#25592=LINE('',#138770,#27680);
#25593=LINE('',#138786,#27681);
#25594=LINE('',#138813,#27682);
#25595=LINE('',#138829,#27683);
#25596=LINE('',#138856,#27684);
#25597=LINE('',#138872,#27685);
#25598=LINE('',#138899,#27686);
#25599=LINE('',#138915,#27687);
#25600=LINE('',#138942,#27688);
#25601=LINE('',#138958,#27689);
#25602=LINE('',#138985,#27690);
#25603=LINE('',#139001,#27691);
#25604=LINE('',#139028,#27692);
#25605=LINE('',#139044,#27693);
#25606=LINE('',#139071,#27694);
#25607=LINE('',#139087,#27695);
#25608=LINE('',#139114,#27696);
#25609=LINE('',#139129,#27697);
#25610=LINE('',#139146,#27698);
#25611=LINE('',#139158,#27699);
#25612=LINE('',#139185,#27700);
#25613=LINE('',#139201,#27701);
#25614=LINE('',#139228,#27702);
#25615=LINE('',#139244,#27703);
#25616=LINE('',#139271,#27704);
#25617=LINE('',#139287,#27705);
#25618=LINE('',#139314,#27706);
#25619=LINE('',#139330,#27707);
#25620=LINE('',#139357,#27708);
#25621=LINE('',#139373,#27709);
#25622=LINE('',#139400,#27710);
#25623=LINE('',#139416,#27711);
#25624=LINE('',#139443,#27712);
#25625=LINE('',#139459,#27713);
#25626=LINE('',#139486,#27714);
#25627=LINE('',#139502,#27715);
#25628=LINE('',#139529,#27716);
#25629=LINE('',#139545,#27717);
#25630=LINE('',#139572,#27718);
#25631=LINE('',#139588,#27719);
#25632=LINE('',#139615,#27720);
#25633=LINE('',#139631,#27721);
#25634=LINE('',#139658,#27722);
#25635=LINE('',#139674,#27723);
#25636=LINE('',#139701,#27724);
#25637=LINE('',#139717,#27725);
#25638=LINE('',#139744,#27726);
#25639=LINE('',#139771,#27727);
#25640=LINE('',#141383,#27728);
#25641=LINE('',#141400,#27729);
#25642=LINE('',#141416,#27730);
#25643=LINE('',#141433,#27731);
#25644=LINE('',#141449,#27732);
#25645=LINE('',#141466,#27733);
#25646=LINE('',#141482,#27734);
#25647=LINE('',#141499,#27735);
#25648=LINE('',#141515,#27736);
#25649=LINE('',#141532,#27737);
#25650=LINE('',#141548,#27738);
#25651=LINE('',#141565,#27739);
#25652=LINE('',#141581,#27740);
#25653=LINE('',#141598,#27741);
#25654=LINE('',#141614,#27742);
#25655=LINE('',#141631,#27743);
#25656=LINE('',#141647,#27744);
#25657=LINE('',#141664,#27745);
#25658=LINE('',#141680,#27746);
#25659=LINE('',#141697,#27747);
#25660=LINE('',#141713,#27748);
#25661=LINE('',#141730,#27749);
#25662=LINE('',#141746,#27750);
#25663=LINE('',#141763,#27751);
#25664=LINE('',#141779,#27752);
#25665=LINE('',#141796,#27753);
#25666=LINE('',#141812,#27754);
#25667=LINE('',#141829,#27755);
#25668=LINE('',#141842,#27756);
#25669=LINE('',#141853,#27757);
#25670=LINE('',#141869,#27758);
#25671=LINE('',#141886,#27759);
#25672=LINE('',#141902,#27760);
#25673=LINE('',#141919,#27761);
#25674=LINE('',#141935,#27762);
#25675=LINE('',#141952,#27763);
#25676=LINE('',#141968,#27764);
#25677=LINE('',#141985,#27765);
#25678=LINE('',#142001,#27766);
#25679=LINE('',#142014,#27767);
#25680=LINE('',#142026,#27768);
#25681=LINE('',#142051,#27769);
#25682=LINE('',#142067,#27770);
#25683=LINE('',#142084,#27771);
#25684=LINE('',#142100,#27772);
#25685=LINE('',#142117,#27773);
#25686=LINE('',#142133,#27774);
#25687=LINE('',#142150,#27775);
#25688=LINE('',#142166,#27776);
#25689=LINE('',#142183,#27777);
#25690=LINE('',#142199,#27778);
#25691=LINE('',#142216,#27779);
#25692=LINE('',#142232,#27780);
#25693=LINE('',#142249,#27781);
#25694=LINE('',#142265,#27782);
#25695=LINE('',#142282,#27783);
#25696=LINE('',#142298,#27784);
#25697=LINE('',#142315,#27785);
#25698=LINE('',#142327,#27786);
#25699=LINE('',#142352,#27787);
#25700=LINE('',#142368,#27788);
#25701=LINE('',#142393,#27789);
#25702=LINE('',#142409,#27790);
#25703=LINE('',#142434,#27791);
#25704=LINE('',#142450,#27792);
#25705=LINE('',#142475,#27793);
#25706=LINE('',#142491,#27794);
#25707=LINE('',#142516,#27795);
#25708=LINE('',#142532,#27796);
#25709=LINE('',#142557,#27797);
#25710=LINE('',#142573,#27798);
#25711=LINE('',#142598,#27799);
#25712=LINE('',#142614,#27800);
#25713=LINE('',#142639,#27801);
#25714=LINE('',#142655,#27802);
#25715=LINE('',#142680,#27803);
#25716=LINE('',#142696,#27804);
#25717=LINE('',#142721,#27805);
#25718=LINE('',#142737,#27806);
#25719=LINE('',#142762,#27807);
#25720=LINE('',#142778,#27808);
#25721=LINE('',#142803,#27809);
#25722=LINE('',#142819,#27810);
#25723=LINE('',#142844,#27811);
#25724=LINE('',#142860,#27812);
#25725=LINE('',#142885,#27813);
#25726=LINE('',#142901,#27814);
#25727=LINE('',#142926,#27815);
#25728=LINE('',#142942,#27816);
#25729=LINE('',#142967,#27817);
#25730=LINE('',#142983,#27818);
#25731=LINE('',#143008,#27819);
#25732=LINE('',#143024,#27820);
#25733=LINE('',#143049,#27821);
#25734=LINE('',#143065,#27822);
#25735=LINE('',#143090,#27823);
#25736=LINE('',#143106,#27824);
#25737=LINE('',#143131,#27825);
#25738=LINE('',#143147,#27826);
#25739=LINE('',#143172,#27827);
#25740=LINE('',#143187,#27828);
#25741=LINE('',#143208,#27829);
#25742=LINE('',#143220,#27830);
#25743=LINE('',#143245,#27831);
#25744=LINE('',#143261,#27832);
#25745=LINE('',#143286,#27833);
#25746=LINE('',#143302,#27834);
#25747=LINE('',#143327,#27835);
#25748=LINE('',#143343,#27836);
#25749=LINE('',#143368,#27837);
#25750=LINE('',#143384,#27838);
#25751=LINE('',#143409,#27839);
#25752=LINE('',#143425,#27840);
#25753=LINE('',#143450,#27841);
#25754=LINE('',#143466,#27842);
#25755=LINE('',#143491,#27843);
#25756=LINE('',#144839,#27844);
#25757=LINE('',#144861,#27845);
#25758=LINE('',#144874,#27846);
#25759=LINE('',#144890,#27847);
#25760=LINE('',#144903,#27848);
#25761=LINE('',#144919,#27849);
#25762=LINE('',#144932,#27850);
#25763=LINE('',#144948,#27851);
#25764=LINE('',#144961,#27852);
#25765=LINE('',#144977,#27853);
#25766=LINE('',#144990,#27854);
#25767=LINE('',#145006,#27855);
#25768=LINE('',#145019,#27856);
#25769=LINE('',#145032,#27857);
#25770=LINE('',#145039,#27858);
#25771=LINE('',#145055,#27859);
#25772=LINE('',#145068,#27860);
#25773=LINE('',#145084,#27861);
#25774=LINE('',#145097,#27862);
#25775=LINE('',#145113,#27863);
#25776=LINE('',#145126,#27864);
#25777=LINE('',#145142,#27865);
#25778=LINE('',#145155,#27866);
#25779=LINE('',#145171,#27867);
#25780=LINE('',#145184,#27868);
#25781=LINE('',#145200,#27869);
#25782=LINE('',#145213,#27870);
#25783=LINE('',#145229,#27871);
#25784=LINE('',#145242,#27872);
#25785=LINE('',#145258,#27873);
#25786=LINE('',#145271,#27874);
#25787=LINE('',#145287,#27875);
#25788=LINE('',#145300,#27876);
#25789=LINE('',#145316,#27877);
#25790=LINE('',#145329,#27878);
#25791=LINE('',#145345,#27879);
#25792=LINE('',#145358,#27880);
#25793=LINE('',#145374,#27881);
#25794=LINE('',#145383,#27882);
#25795=LINE('',#145395,#27883);
#25796=LINE('',#145416,#27884);
#25797=LINE('',#145432,#27885);
#25798=LINE('',#145445,#27886);
#25799=LINE('',#145461,#27887);
#25800=LINE('',#145474,#27888);
#25801=LINE('',#145490,#27889);
#25802=LINE('',#145503,#27890);
#25803=LINE('',#145519,#27891);
#25804=LINE('',#145532,#27892);
#25805=LINE('',#145548,#27893);
#25806=LINE('',#145561,#27894);
#25807=LINE('',#145577,#27895);
#25808=LINE('',#145590,#27896);
#25809=LINE('',#145606,#27897);
#25810=LINE('',#145619,#27898);
#25811=LINE('',#145635,#27899);
#25812=LINE('',#145648,#27900);
#25813=LINE('',#145661,#27901);
#25814=LINE('',#145677,#27902);
#25815=LINE('',#145689,#27903);
#25816=LINE('',#145706,#27904);
#25817=LINE('',#145722,#27905);
#25818=LINE('',#145739,#27906);
#25819=LINE('',#145755,#27907);
#25820=LINE('',#145772,#27908);
#25821=LINE('',#145788,#27909);
#25822=LINE('',#145805,#27910);
#25823=LINE('',#145821,#27911);
#25824=LINE('',#145838,#27912);
#25825=LINE('',#145854,#27913);
#25826=LINE('',#145871,#27914);
#25827=LINE('',#145887,#27915);
#25828=LINE('',#145904,#27916);
#25829=LINE('',#145920,#27917);
#25830=LINE('',#145937,#27918);
#25831=LINE('',#145953,#27919);
#25832=LINE('',#145970,#27920);
#25833=LINE('',#145986,#27921);
#25834=LINE('',#146003,#27922);
#25835=LINE('',#146019,#27923);
#25836=LINE('',#146036,#27924);
#25837=LINE('',#146052,#27925);
#25838=LINE('',#146069,#27926);
#25839=LINE('',#146085,#27927);
#25840=LINE('',#146102,#27928);
#25841=LINE('',#146117,#27929);
#25842=LINE('',#146130,#27930);
#25843=LINE('',#146142,#27931);
#25844=LINE('',#146159,#27932);
#25845=LINE('',#146175,#27933);
#25846=LINE('',#146192,#27934);
#25847=LINE('',#146208,#27935);
#25848=LINE('',#146225,#27936);
#25849=LINE('',#146241,#27937);
#25850=LINE('',#146258,#27938);
#25851=LINE('',#146274,#27939);
#25852=LINE('',#146291,#27940);
#25853=LINE('',#146307,#27941);
#25854=LINE('',#146324,#27942);
#25855=LINE('',#146340,#27943);
#25856=LINE('',#146357,#27944);
#25857=LINE('',#146373,#27945);
#25858=LINE('',#146390,#27946);
#25859=LINE('',#146406,#27947);
#25860=LINE('',#146423,#27948);
#25861=LINE('',#146439,#27949);
#25862=LINE('',#146456,#27950);
#25863=LINE('',#146472,#27951);
#25864=LINE('',#146489,#27952);
#25865=LINE('',#146505,#27953);
#25866=LINE('',#146522,#27954);
#25867=LINE('',#146538,#27955);
#25868=LINE('',#146555,#27956);
#25869=LINE('',#146571,#27957);
#25870=LINE('',#146588,#27958);
#25871=LINE('',#146609,#27959);
#25872=LINE('',#148721,#27960);
#25873=LINE('',#148744,#27961);
#25874=LINE('',#148764,#27962);
#25875=LINE('',#148787,#27963);
#25876=LINE('',#148807,#27964);
#25877=LINE('',#148830,#27965);
#25878=LINE('',#148850,#27966);
#25879=LINE('',#148873,#27967);
#25880=LINE('',#148893,#27968);
#25881=LINE('',#148916,#27969);
#25882=LINE('',#148936,#27970);
#25883=LINE('',#148959,#27971);
#25884=LINE('',#148979,#27972);
#25885=LINE('',#149002,#27973);
#25886=LINE('',#149022,#27974);
#25887=LINE('',#149045,#27975);
#25888=LINE('',#149065,#27976);
#25889=LINE('',#149088,#27977);
#25890=LINE('',#149108,#27978);
#25891=LINE('',#149131,#27979);
#25892=LINE('',#149151,#27980);
#25893=LINE('',#149174,#27981);
#25894=LINE('',#149194,#27982);
#25895=LINE('',#149217,#27983);
#25896=LINE('',#149237,#27984);
#25897=LINE('',#149260,#27985);
#25898=LINE('',#149280,#27986);
#25899=LINE('',#149303,#27987);
#25900=LINE('',#149320,#27988);
#25901=LINE('',#149331,#27989);
#25902=LINE('',#149351,#27990);
#25903=LINE('',#149374,#27991);
#25904=LINE('',#149394,#27992);
#25905=LINE('',#149417,#27993);
#25906=LINE('',#149437,#27994);
#25907=LINE('',#149460,#27995);
#25908=LINE('',#149480,#27996);
#25909=LINE('',#149499,#27997);
#25910=LINE('',#149515,#27998);
#25911=LINE('',#149546,#27999);
#25912=LINE('',#149566,#28000);
#25913=LINE('',#149589,#28001);
#25914=LINE('',#149609,#28002);
#25915=LINE('',#149632,#28003);
#25916=LINE('',#149652,#28004);
#25917=LINE('',#149675,#28005);
#25918=LINE('',#149695,#28006);
#25919=LINE('',#149718,#28007);
#25920=LINE('',#149738,#28008);
#25921=LINE('',#149761,#28009);
#25922=LINE('',#149781,#28010);
#25923=LINE('',#149804,#28011);
#25924=LINE('',#149824,#28012);
#25925=LINE('',#149847,#28013);
#25926=LINE('',#149867,#28014);
#25927=LINE('',#149890,#28015);
#25928=LINE('',#149910,#28016);
#25929=LINE('',#149933,#28017);
#25930=LINE('',#149945,#28018);
#25931=LINE('',#149969,#28019);
#25932=LINE('',#149984,#28020);
#25933=LINE('',#150008,#28021);
#25934=LINE('',#150023,#28022);
#25935=LINE('',#150047,#28023);
#25936=LINE('',#150062,#28024);
#25937=LINE('',#150086,#28025);
#25938=LINE('',#150101,#28026);
#25939=LINE('',#150125,#28027);
#25940=LINE('',#150140,#28028);
#25941=LINE('',#150164,#28029);
#25942=LINE('',#150179,#28030);
#25943=LINE('',#150203,#28031);
#25944=LINE('',#150218,#28032);
#25945=LINE('',#150242,#28033);
#25946=LINE('',#150257,#28034);
#25947=LINE('',#150281,#28035);
#25948=LINE('',#150296,#28036);
#25949=LINE('',#150320,#28037);
#25950=LINE('',#150335,#28038);
#25951=LINE('',#150359,#28039);
#25952=LINE('',#150374,#28040);
#25953=LINE('',#150398,#28041);
#25954=LINE('',#150413,#28042);
#25955=LINE('',#150437,#28043);
#25956=LINE('',#150452,#28044);
#25957=LINE('',#150476,#28045);
#25958=LINE('',#150491,#28046);
#25959=LINE('',#150515,#28047);
#25960=LINE('',#150530,#28048);
#25961=LINE('',#150554,#28049);
#25962=LINE('',#150569,#28050);
#25963=LINE('',#150593,#28051);
#25964=LINE('',#150608,#28052);
#25965=LINE('',#150632,#28053);
#25966=LINE('',#150647,#28054);
#25967=LINE('',#150671,#28055);
#25968=LINE('',#150686,#28056);
#25969=LINE('',#150710,#28057);
#25970=LINE('',#150725,#28058);
#25971=LINE('',#150749,#28059);
#25972=LINE('',#150763,#28060);
#25973=LINE('',#150776,#28061);
#25974=LINE('',#150788,#28062);
#25975=LINE('',#150812,#28063);
#25976=LINE('',#150827,#28064);
#25977=LINE('',#150851,#28065);
#25978=LINE('',#150866,#28066);
#25979=LINE('',#150890,#28067);
#25980=LINE('',#150905,#28068);
#25981=LINE('',#150929,#28069);
#25982=LINE('',#150944,#28070);
#25983=LINE('',#150968,#28071);
#25984=LINE('',#150983,#28072);
#25985=LINE('',#151007,#28073);
#25986=LINE('',#151022,#28074);
#25987=LINE('',#151046,#28075);
#25988=LINE('',#152514,#28076);
#25989=LINE('',#152544,#28077);
#25990=LINE('',#152561,#28078);
#25991=LINE('',#152585,#28079);
#25992=LINE('',#152602,#28080);
#25993=LINE('',#152626,#28081);
#25994=LINE('',#152643,#28082);
#25995=LINE('',#152667,#28083);
#25996=LINE('',#152684,#28084);
#25997=LINE('',#152708,#28085);
#25998=LINE('',#152725,#28086);
#25999=LINE('',#152749,#28087);
#26000=LINE('',#152766,#28088);
#26001=LINE('',#152787,#28089);
#26002=LINE('',#152798,#28090);
#26003=LINE('',#152822,#28091);
#26004=LINE('',#152839,#28092);
#26005=LINE('',#152863,#28093);
#26006=LINE('',#152880,#28094);
#26007=LINE('',#152904,#28095);
#26008=LINE('',#152921,#28096);
#26009=LINE('',#152945,#28097);
#26010=LINE('',#152962,#28098);
#26011=LINE('',#152986,#28099);
#26012=LINE('',#153003,#28100);
#26013=LINE('',#153027,#28101);
#26014=LINE('',#153044,#28102);
#26015=LINE('',#153068,#28103);
#26016=LINE('',#153085,#28104);
#26017=LINE('',#153109,#28105);
#26018=LINE('',#153126,#28106);
#26019=LINE('',#153150,#28107);
#26020=LINE('',#153167,#28108);
#26021=LINE('',#153191,#28109);
#26022=LINE('',#153208,#28110);
#26023=LINE('',#153232,#28111);
#26024=LINE('',#153245,#28112);
#26025=LINE('',#153265,#28113);
#26026=LINE('',#153290,#28114);
#26027=LINE('',#153314,#28115);
#26028=LINE('',#153331,#28116);
#26029=LINE('',#153355,#28117);
#26030=LINE('',#153372,#28118);
#26031=LINE('',#153396,#28119);
#26032=LINE('',#153413,#28120);
#26033=LINE('',#153437,#28121);
#26034=LINE('',#153454,#28122);
#26035=LINE('',#153478,#28123);
#26036=LINE('',#153495,#28124);
#26037=LINE('',#153519,#28125);
#26038=LINE('',#153536,#28126);
#26039=LINE('',#153560,#28127);
#26040=LINE('',#153577,#28128);
#26041=LINE('',#153601,#28129);
#26042=LINE('',#153618,#28130);
#26043=LINE('',#153642,#28131);
#26044=LINE('',#153659,#28132);
#26045=LINE('',#153680,#28133);
#26046=LINE('',#153704,#28134);
#26047=LINE('',#153715,#28135);
#26048=LINE('',#153763,#28136);
#26049=LINE('',#153774,#28137);
#26050=LINE('',#153822,#28138);
#26051=LINE('',#153833,#28139);
#26052=LINE('',#153881,#28140);
#26053=LINE('',#153892,#28141);
#26054=LINE('',#153940,#28142);
#26055=LINE('',#153951,#28143);
#26056=LINE('',#153999,#28144);
#26057=LINE('',#154010,#28145);
#26058=LINE('',#154058,#28146);
#26059=LINE('',#154069,#28147);
#26060=LINE('',#154117,#28148);
#26061=LINE('',#154128,#28149);
#26062=LINE('',#154176,#28150);
#26063=LINE('',#154187,#28151);
#26064=LINE('',#154235,#28152);
#26065=LINE('',#154246,#28153);
#26066=LINE('',#154294,#28154);
#26067=LINE('',#154305,#28155);
#26068=LINE('',#154353,#28156);
#26069=LINE('',#154364,#28157);
#26070=LINE('',#154412,#28158);
#26071=LINE('',#154423,#28159);
#26072=LINE('',#154471,#28160);
#26073=LINE('',#154481,#28161);
#26074=LINE('',#154497,#28162);
#26075=LINE('',#154508,#28163);
#26076=LINE('',#154556,#28164);
#26077=LINE('',#154567,#28165);
#26078=LINE('',#154615,#28166);
#26079=LINE('',#154626,#28167);
#26080=LINE('',#154674,#28168);
#26081=LINE('',#154685,#28169);
#26082=LINE('',#154733,#28170);
#26083=LINE('',#154744,#28171);
#26084=LINE('',#154792,#28172);
#26085=LINE('',#154803,#28173);
#26086=LINE('',#154851,#28174);
#26087=LINE('',#154861,#28175);
#26088=LINE('',#154877,#28176);
#26089=LINE('',#154888,#28177);
#26090=LINE('',#154936,#28178);
#26091=LINE('',#154947,#28179);
#26092=LINE('',#154995,#28180);
#26093=LINE('',#155006,#28181);
#26094=LINE('',#155054,#28182);
#26095=LINE('',#155065,#28183);
#26096=LINE('',#155113,#28184);
#26097=LINE('',#155124,#28185);
#26098=LINE('',#155172,#28186);
#26099=LINE('',#155183,#28187);
#26100=LINE('',#155231,#28188);
#26101=LINE('',#155242,#28189);
#26102=LINE('',#155290,#28190);
#26103=LINE('',#155325,#28191);
#26104=LINE('',#157185,#28192);
#26105=LINE('',#157202,#28193);
#26106=LINE('',#157218,#28194);
#26107=LINE('',#157235,#28195);
#26108=LINE('',#157251,#28196);
#26109=LINE('',#157268,#28197);
#26110=LINE('',#157284,#28198);
#26111=LINE('',#157301,#28199);
#26112=LINE('',#157317,#28200);
#26113=LINE('',#157334,#28201);
#26114=LINE('',#157350,#28202);
#26115=LINE('',#157367,#28203);
#26116=LINE('',#157383,#28204);
#26117=LINE('',#157400,#28205);
#26118=LINE('',#157416,#28206);
#26119=LINE('',#157433,#28207);
#26120=LINE('',#157449,#28208);
#26121=LINE('',#157466,#28209);
#26122=LINE('',#157482,#28210);
#26123=LINE('',#157499,#28211);
#26124=LINE('',#157515,#28212);
#26125=LINE('',#157532,#28213);
#26126=LINE('',#157548,#28214);
#26127=LINE('',#157565,#28215);
#26128=LINE('',#157581,#28216);
#26129=LINE('',#157598,#28217);
#26130=LINE('',#157614,#28218);
#26131=LINE('',#157631,#28219);
#26132=LINE('',#157644,#28220);
#26133=LINE('',#157655,#28221);
#26134=LINE('',#157671,#28222);
#26135=LINE('',#157688,#28223);
#26136=LINE('',#157704,#28224);
#26137=LINE('',#157721,#28225);
#26138=LINE('',#157737,#28226);
#26139=LINE('',#157750,#28227);
#26140=LINE('',#157762,#28228);
#26141=LINE('',#157787,#28229);
#26142=LINE('',#157803,#28230);
#26143=LINE('',#157820,#28231);
#26144=LINE('',#157836,#28232);
#26145=LINE('',#157853,#28233);
#26146=LINE('',#157869,#28234);
#26147=LINE('',#157886,#28235);
#26148=LINE('',#157902,#28236);
#26149=LINE('',#157919,#28237);
#26150=LINE('',#157935,#28238);
#26151=LINE('',#157952,#28239);
#26152=LINE('',#157968,#28240);
#26153=LINE('',#157985,#28241);
#26154=LINE('',#158001,#28242);
#26155=LINE('',#158018,#28243);
#26156=LINE('',#158034,#28244);
#26157=LINE('',#158051,#28245);
#26158=LINE('',#158067,#28246);
#26159=LINE('',#158084,#28247);
#26160=LINE('',#158100,#28248);
#26161=LINE('',#158117,#28249);
#26162=LINE('',#158129,#28250);
#26163=LINE('',#158173,#28251);
#26164=LINE('',#158204,#28252);
#26165=LINE('',#158259,#28253);
#26166=LINE('',#158290,#28254);
#26167=LINE('',#158344,#28255);
#26168=LINE('',#158375,#28256);
#26169=LINE('',#158430,#28257);
#26170=LINE('',#158461,#28258);
#26171=LINE('',#158514,#28259);
#26172=LINE('',#158545,#28260);
#26173=LINE('',#158600,#28261);
#26174=LINE('',#158631,#28262);
#26175=LINE('',#158685,#28263);
#26176=LINE('',#158716,#28264);
#26177=LINE('',#158771,#28265);
#26178=LINE('',#158802,#28266);
#26179=LINE('',#158856,#28267);
#26180=LINE('',#158887,#28268);
#26181=LINE('',#158942,#28269);
#26182=LINE('',#158973,#28270);
#26183=LINE('',#159028,#28271);
#26184=LINE('',#159059,#28272);
#26185=LINE('',#159114,#28273);
#26186=LINE('',#159145,#28274);
#26187=LINE('',#159199,#28275);
#26188=LINE('',#159230,#28276);
#26189=LINE('',#159284,#28277);
#26190=LINE('',#159315,#28278);
#26191=LINE('',#159370,#28279);
#26192=LINE('',#159401,#28280);
#26193=LINE('',#159456,#28281);
#26194=LINE('',#159487,#28282);
#26195=LINE('',#159541,#28283);
#26196=LINE('',#159572,#28284);
#26197=LINE('',#159626,#28285);
#26198=LINE('',#159657,#28286);
#26199=LINE('',#159712,#28287);
#26200=LINE('',#159743,#28288);
#26201=LINE('',#159797,#28289);
#26202=LINE('',#159828,#28290);
#26203=LINE('',#159883,#28291);
#26204=LINE('',#159914,#28292);
#26205=LINE('',#159969,#28293);
#26206=LINE('',#160000,#28294);
#26207=LINE('',#160055,#28295);
#26208=LINE('',#160086,#28296);
#26209=LINE('',#160141,#28297);
#26210=LINE('',#160172,#28298);
#26211=LINE('',#160226,#28299);
#26212=LINE('',#160257,#28300);
#26213=LINE('',#160312,#28301);
#26214=LINE('',#160343,#28302);
#26215=LINE('',#160398,#28303);
#26216=LINE('',#160429,#28304);
#26217=LINE('',#160484,#28305);
#26218=LINE('',#160515,#28306);
#26219=LINE('',#160570,#28307);
#26220=LINE('',#161339,#28308);
#26221=LINE('',#161361,#28309);
#26222=LINE('',#161381,#28310);
#26223=LINE('',#161400,#28311);
#26224=LINE('',#161420,#28312);
#26225=LINE('',#161439,#28313);
#26226=LINE('',#161459,#28314);
#26227=LINE('',#161478,#28315);
#26228=LINE('',#161498,#28316);
#26229=LINE('',#161517,#28317);
#26230=LINE('',#161537,#28318);
#26231=LINE('',#161556,#28319);
#26232=LINE('',#161576,#28320);
#26233=LINE('',#161592,#28321);
#26234=LINE('',#161607,#28322);
#26235=LINE('',#161623,#28323);
#26236=LINE('',#161643,#28324);
#26237=LINE('',#161662,#28325);
#26238=LINE('',#161682,#28326);
#26239=LINE('',#161701,#28327);
#26240=LINE('',#161721,#28328);
#26241=LINE('',#161740,#28329);
#26242=LINE('',#161760,#28330);
#26243=LINE('',#161779,#28331);
#26244=LINE('',#161799,#28332);
#26245=LINE('',#161818,#28333);
#26246=LINE('',#161838,#28334);
#26247=LINE('',#161857,#28335);
#26248=LINE('',#161877,#28336);
#26249=LINE('',#161896,#28337);
#26250=LINE('',#161916,#28338);
#26251=LINE('',#161935,#28339);
#26252=LINE('',#161955,#28340);
#26253=LINE('',#161974,#28341);
#26254=LINE('',#161994,#28342);
#26255=LINE('',#162005,#28343);
#26256=LINE('',#162033,#28344);
#26257=LINE('',#162052,#28345);
#26258=LINE('',#162072,#28346);
#26259=LINE('',#162091,#28347);
#26260=LINE('',#162111,#28348);
#26261=LINE('',#162130,#28349);
#26262=LINE('',#162150,#28350);
#26263=LINE('',#162169,#28351);
#26264=LINE('',#162189,#28352);
#26265=LINE('',#162208,#28353);
#26266=LINE('',#162228,#28354);
#26267=LINE('',#162247,#28355);
#26268=LINE('',#162267,#28356);
#26269=LINE('',#162286,#28357);
#26270=LINE('',#162306,#28358);
#26271=LINE('',#162325,#28359);
#26272=LINE('',#162345,#28360);
#26273=LINE('',#162364,#28361);
#26274=LINE('',#162384,#28362);
#26275=LINE('',#162403,#28363);
#26276=LINE('',#162423,#28364);
#26277=LINE('',#162445,#28365);
#26278=LINE('',#163037,#28366);
#26279=LINE('',#163085,#28367);
#26280=LINE('',#163096,#28368);
#26281=LINE('',#163144,#28369);
#26282=LINE('',#163155,#28370);
#26283=LINE('',#163203,#28371);
#26284=LINE('',#163214,#28372);
#26285=LINE('',#163262,#28373);
#26286=LINE('',#163273,#28374);
#26287=LINE('',#163321,#28375);
#26288=LINE('',#163332,#28376);
#26289=LINE('',#163380,#28377);
#26290=LINE('',#163391,#28378);
#26291=LINE('',#163439,#28379);
#26292=LINE('',#163450,#28380);
#26293=LINE('',#163498,#28381);
#26294=LINE('',#163509,#28382);
#26295=LINE('',#163557,#28383);
#26296=LINE('',#163568,#28384);
#26297=LINE('',#163616,#28385);
#26298=LINE('',#163627,#28386);
#26299=LINE('',#163675,#28387);
#26300=LINE('',#163686,#28388);
#26301=LINE('',#163734,#28389);
#26302=LINE('',#163745,#28390);
#26303=LINE('',#163793,#28391);
#26304=LINE('',#163804,#28392);
#26305=LINE('',#163852,#28393);
#26306=LINE('',#163863,#28394);
#26307=LINE('',#163911,#28395);
#26308=LINE('',#163922,#28396);
#26309=LINE('',#163970,#28397);
#26310=LINE('',#163981,#28398);
#26311=LINE('',#164029,#28399);
#26312=LINE('',#164040,#28400);
#26313=LINE('',#164088,#28401);
#26314=LINE('',#164099,#28402);
#26315=LINE('',#164147,#28403);
#26316=LINE('',#164158,#28404);
#26317=LINE('',#164206,#28405);
#26318=LINE('',#164217,#28406);
#26319=LINE('',#164265,#28407);
#26320=LINE('',#164275,#28408);
#26321=LINE('',#164291,#28409);
#26322=LINE('',#164302,#28410);
#26323=LINE('',#164350,#28411);
#26324=LINE('',#164361,#28412);
#26325=LINE('',#164409,#28413);
#26326=LINE('',#164420,#28414);
#26327=LINE('',#164468,#28415);
#26328=LINE('',#164479,#28416);
#26329=LINE('',#164527,#28417);
#26330=LINE('',#164538,#28418);
#26331=LINE('',#164586,#28419);
#26332=LINE('',#164597,#28420);
#26333=LINE('',#164645,#28421);
#26334=LINE('',#164655,#28422);
#26335=LINE('',#164671,#28423);
#26336=LINE('',#165580,#28424);
#26337=LINE('',#165635,#28425);
#26338=LINE('',#165666,#28426);
#26339=LINE('',#165721,#28427);
#26340=LINE('',#165752,#28428);
#26341=LINE('',#165807,#28429);
#26342=LINE('',#165838,#28430);
#26343=LINE('',#165893,#28431);
#26344=LINE('',#165924,#28432);
#26345=LINE('',#165978,#28433);
#26346=LINE('',#166009,#28434);
#26347=LINE('',#166064,#28435);
#26348=LINE('',#166095,#28436);
#26349=LINE('',#166150,#28437);
#26350=LINE('',#166181,#28438);
#26351=LINE('',#166236,#28439);
#26352=LINE('',#166267,#28440);
#26353=LINE('',#166322,#28441);
#26354=LINE('',#166353,#28442);
#26355=LINE('',#166407,#28443);
#26356=LINE('',#166438,#28444);
#26357=LINE('',#166493,#28445);
#26358=LINE('',#166524,#28446);
#26359=LINE('',#166578,#28447);
#26360=LINE('',#166609,#28448);
#26361=LINE('',#166663,#28449);
#26362=LINE('',#166694,#28450);
#26363=LINE('',#166749,#28451);
#26364=LINE('',#166780,#28452);
#26365=LINE('',#166835,#28453);
#26366=LINE('',#166866,#28454);
#26367=LINE('',#166920,#28455);
#26368=LINE('',#166951,#28456);
#26369=LINE('',#167005,#28457);
#26370=LINE('',#167036,#28458);
#26371=LINE('',#167091,#28459);
#26372=LINE('',#167122,#28460);
#26373=LINE('',#167177,#28461);
#26374=LINE('',#167208,#28462);
#26375=LINE('',#167263,#28463);
#26376=LINE('',#167294,#28464);
#26377=LINE('',#167348,#28465);
#26378=LINE('',#167379,#28466);
#26379=LINE('',#167434,#28467);
#26380=LINE('',#167465,#28468);
#26381=LINE('',#167519,#28469);
#26382=LINE('',#167550,#28470);
#26383=LINE('',#167605,#28471);
#26384=LINE('',#167636,#28472);
#26385=LINE('',#167689,#28473);
#26386=LINE('',#167720,#28474);
#26387=LINE('',#167775,#28475);
#26388=LINE('',#167806,#28476);
#26389=LINE('',#167860,#28477);
#26390=LINE('',#167891,#28478);
#26391=LINE('',#167946,#28479);
#26392=LINE('',#167977,#28480);
#26393=LINE('',#168032,#28481);
#26445=VECTOR('',#77769,6.75);
#26446=VECTOR('',#77886,6.75);
#26447=VECTOR('',#77893,3.25);
#26448=VECTOR('',#77902,7.);
#26449=VECTOR('',#77909,6.125);
#26450=VECTOR('',#77916,6.125);
#26451=VECTOR('',#77981,6.75);
#26452=VECTOR('',#78216,1000.);
#26453=VECTOR('',#78223,1000.);
#26454=VECTOR('',#78230,1000.);
#26455=VECTOR('',#78237,1000.);
#26456=VECTOR('',#78244,1000.);
#26457=VECTOR('',#78251,1000.);
#26458=VECTOR('',#78258,1000.);
#26459=VECTOR('',#78265,1000.);
#26460=VECTOR('',#78272,1000.);
#26461=VECTOR('',#78279,1000.);
#26462=VECTOR('',#78286,1000.);
#26463=VECTOR('',#78293,1000.);
#26464=VECTOR('',#78300,1000.);
#26465=VECTOR('',#78305,1000.);
#26466=VECTOR('',#78306,1000.);
#26467=VECTOR('',#78313,1000.);
#26468=VECTOR('',#78320,1000.);
#26469=VECTOR('',#78327,1000.);
#26470=VECTOR('',#78334,1000.);
#26471=VECTOR('',#78341,1000.);
#26472=VECTOR('',#78348,1000.);
#26473=VECTOR('',#78355,1000.);
#26474=VECTOR('',#78362,1000.);
#26475=VECTOR('',#78369,1000.);
#26476=VECTOR('',#78376,1000.);
#26477=VECTOR('',#78383,1000.);
#26478=VECTOR('',#78390,1000.);
#26479=VECTOR('',#78397,1000.);
#26480=VECTOR('',#78404,1000.);
#26481=VECTOR('',#78411,1000.);
#26482=VECTOR('',#78418,1000.);
#26483=VECTOR('',#78425,1000.);
#26484=VECTOR('',#78432,1000.);
#26485=VECTOR('',#78439,1000.);
#26486=VECTOR('',#78446,1000.);
#26487=VECTOR('',#78453,1000.);
#26488=VECTOR('',#78460,1000.);
#26489=VECTOR('',#78467,1000.);
#26490=VECTOR('',#78474,1000.);
#26491=VECTOR('',#78481,1000.);
#26492=VECTOR('',#78488,1000.);
#26493=VECTOR('',#78495,1000.);
#26494=VECTOR('',#78502,1000.);
#26495=VECTOR('',#78509,1000.);
#26496=VECTOR('',#78516,1000.);
#26497=VECTOR('',#78523,1000.);
#26498=VECTOR('',#78530,1000.);
#26499=VECTOR('',#78537,1000.);
#26500=VECTOR('',#78544,1000.);
#26501=VECTOR('',#78551,1000.);
#26502=VECTOR('',#78554,1000.);
#26503=VECTOR('',#78565,1000.);
#26504=VECTOR('',#78574,1000.);
#26505=VECTOR('',#78579,1000.);
#26506=VECTOR('',#78586,1000.);
#26507=VECTOR('',#78593,1000.);
#26508=VECTOR('',#78600,1000.);
#26509=VECTOR('',#78611,1000.);
#26510=VECTOR('',#78614,1000.);
#26511=VECTOR('',#78615,1000.);
#26512=VECTOR('',#78620,1000.);
#26513=VECTOR('',#78627,1000.);
#26514=VECTOR('',#78632,1000.);
#26515=VECTOR('',#78639,1000.);
#26516=VECTOR('',#78644,1000.);
#26517=VECTOR('',#78651,1000.);
#26518=VECTOR('',#78656,1000.);
#26519=VECTOR('',#78663,1000.);
#26520=VECTOR('',#78668,1000.);
#26521=VECTOR('',#78675,1000.);
#26522=VECTOR('',#78680,1000.);
#26523=VECTOR('',#78687,1000.);
#26524=VECTOR('',#78692,1000.);
#26525=VECTOR('',#78699,1000.);
#26526=VECTOR('',#78704,1000.);
#26527=VECTOR('',#78711,1000.);
#26528=VECTOR('',#78716,1000.);
#26529=VECTOR('',#78723,1000.);
#26530=VECTOR('',#78728,1000.);
#26531=VECTOR('',#78735,1000.);
#26532=VECTOR('',#78740,1000.);
#26533=VECTOR('',#78747,1000.);
#26534=VECTOR('',#78752,1000.);
#26535=VECTOR('',#78759,1000.);
#26536=VECTOR('',#78764,1000.);
#26537=VECTOR('',#78771,1000.);
#26538=VECTOR('',#78772,1000.);
#26539=VECTOR('',#78773,1000.);
#26540=VECTOR('',#78778,1000.);
#26541=VECTOR('',#78785,1000.);
#26542=VECTOR('',#78790,1000.);
#26543=VECTOR('',#78797,1000.);
#26544=VECTOR('',#78802,1000.);
#26545=VECTOR('',#78809,1000.);
#26546=VECTOR('',#78814,1000.);
#26547=VECTOR('',#78821,1000.);
#26548=VECTOR('',#78826,1000.);
#26549=VECTOR('',#78833,1000.);
#26550=VECTOR('',#78838,1000.);
#26551=VECTOR('',#78845,1000.);
#26552=VECTOR('',#78850,1000.);
#26553=VECTOR('',#78857,1000.);
#26554=VECTOR('',#78862,1000.);
#26555=VECTOR('',#78869,1000.);
#26556=VECTOR('',#78874,1000.);
#26557=VECTOR('',#78881,1000.);
#26558=VECTOR('',#78886,1000.);
#26559=VECTOR('',#78893,1000.);
#26560=VECTOR('',#78898,1000.);
#26561=VECTOR('',#78905,1000.);
#26562=VECTOR('',#78910,1000.);
#26563=VECTOR('',#78917,1000.);
#26564=VECTOR('',#78922,1000.);
#26565=VECTOR('',#78929,1000.);
#26566=VECTOR('',#78934,1000.);
#26567=VECTOR('',#78949,1000.);
#26568=VECTOR('',#79126,1000.);
#26569=VECTOR('',#79131,1000.);
#26570=VECTOR('',#79134,1000.);
#26571=VECTOR('',#79139,1000.);
#26572=VECTOR('',#79142,1000.);
#26573=VECTOR('',#79147,1000.);
#26574=VECTOR('',#79150,1000.);
#26575=VECTOR('',#79155,1000.);
#26576=VECTOR('',#79158,1000.);
#26577=VECTOR('',#79163,1000.);
#26578=VECTOR('',#79166,1000.);
#26579=VECTOR('',#79171,1000.);
#26580=VECTOR('',#79174,1000.);
#26581=VECTOR('',#79179,1000.);
#26582=VECTOR('',#79182,1000.);
#26583=VECTOR('',#79187,1000.);
#26584=VECTOR('',#79190,1000.);
#26585=VECTOR('',#79195,1000.);
#26586=VECTOR('',#79198,1000.);
#26587=VECTOR('',#79203,1000.);
#26588=VECTOR('',#79206,1000.);
#26589=VECTOR('',#79211,1000.);
#26590=VECTOR('',#79214,1000.);
#26591=VECTOR('',#79219,1000.);
#26592=VECTOR('',#79222,1000.);
#26593=VECTOR('',#79227,1000.);
#26594=VECTOR('',#79230,1000.);
#26595=VECTOR('',#79235,1000.);
#26596=VECTOR('',#79236,1000.);
#26597=VECTOR('',#79237,1000.);
#26598=VECTOR('',#79240,1000.);
#26599=VECTOR('',#79245,1000.);
#26600=VECTOR('',#79248,1000.);
#26601=VECTOR('',#79253,1000.);
#26602=VECTOR('',#79256,1000.);
#26603=VECTOR('',#79261,1000.);
#26604=VECTOR('',#79264,1000.);
#26605=VECTOR('',#79269,1000.);
#26606=VECTOR('',#79272,1000.);
#26607=VECTOR('',#79277,1000.);
#26608=VECTOR('',#79280,1000.);
#26609=VECTOR('',#79285,1000.);
#26610=VECTOR('',#79288,1000.);
#26611=VECTOR('',#79293,1000.);
#26612=VECTOR('',#79296,1000.);
#26613=VECTOR('',#79301,1000.);
#26614=VECTOR('',#79304,1000.);
#26615=VECTOR('',#79309,1000.);
#26616=VECTOR('',#79312,1000.);
#26617=VECTOR('',#79313,1000.);
#26618=VECTOR('',#79318,1000.);
#26619=VECTOR('',#79325,1000.);
#26620=VECTOR('',#79328,1000.);
#26621=VECTOR('',#79333,1000.);
#26622=VECTOR('',#79336,1000.);
#26623=VECTOR('',#79341,1000.);
#26624=VECTOR('',#79344,1000.);
#26625=VECTOR('',#79349,1000.);
#26626=VECTOR('',#79350,1000.);
#26627=VECTOR('',#79355,1000.);
#26628=VECTOR('',#79360,1000.);
#26629=VECTOR('',#79365,1000.);
#26630=VECTOR('',#79370,1000.);
#26631=VECTOR('',#79375,1000.);
#26632=VECTOR('',#79380,1000.);
#26633=VECTOR('',#79385,1000.);
#26634=VECTOR('',#79390,1000.);
#26635=VECTOR('',#79395,1000.);
#26636=VECTOR('',#79400,1000.);
#26637=VECTOR('',#79405,1000.);
#26638=VECTOR('',#79410,1000.);
#26639=VECTOR('',#79415,1000.);
#26640=VECTOR('',#79420,1000.);
#26641=VECTOR('',#79425,1000.);
#26642=VECTOR('',#79430,1000.);
#26643=VECTOR('',#79435,1000.);
#26644=VECTOR('',#79440,1000.);
#26645=VECTOR('',#79445,1000.);
#26646=VECTOR('',#79450,1000.);
#26647=VECTOR('',#79455,1000.);
#26648=VECTOR('',#79460,1000.);
#26649=VECTOR('',#79465,1000.);
#26650=VECTOR('',#79470,1000.);
#26651=VECTOR('',#79475,1000.);
#26652=VECTOR('',#79480,1000.);
#26653=VECTOR('',#79485,1000.);
#26654=VECTOR('',#79490,1000.);
#26655=VECTOR('',#79495,1000.);
#26656=VECTOR('',#79500,1000.);
#26657=VECTOR('',#79505,1000.);
#26658=VECTOR('',#79510,1000.);
#26659=VECTOR('',#79515,1000.);
#26660=VECTOR('',#79520,1000.);
#26661=VECTOR('',#79525,1000.);
#26662=VECTOR('',#79530,1000.);
#26663=VECTOR('',#79535,1000.);
#26664=VECTOR('',#79540,1000.);
#26665=VECTOR('',#79545,1000.);
#26666=VECTOR('',#79550,1000.);
#26667=VECTOR('',#79555,1000.);
#26668=VECTOR('',#79560,1000.);
#26669=VECTOR('',#79561,1000.);
#26670=VECTOR('',#79562,1000.);
#26671=VECTOR('',#79567,1000.);
#26672=VECTOR('',#79572,1000.);
#26673=VECTOR('',#79577,1000.);
#26674=VECTOR('',#79582,1000.);
#26675=VECTOR('',#79587,1000.);
#26676=VECTOR('',#79592,1000.);
#26677=VECTOR('',#79597,1000.);
#26678=VECTOR('',#79602,1000.);
#26679=VECTOR('',#79607,1000.);
#26680=VECTOR('',#79612,1000.);
#26681=VECTOR('',#79617,1000.);
#26682=VECTOR('',#79622,1000.);
#26683=VECTOR('',#79627,1000.);
#26684=VECTOR('',#79750,1000.);
#26685=VECTOR('',#79751,1000.);
#26686=VECTOR('',#79760,1000.);
#26687=VECTOR('',#79761,1000.);
#26688=VECTOR('',#79770,1000.);
#26689=VECTOR('',#79771,1000.);
#26690=VECTOR('',#79780,1000.);
#26691=VECTOR('',#79781,1000.);
#26692=VECTOR('',#79790,1000.);
#26693=VECTOR('',#79791,1000.);
#26694=VECTOR('',#79800,1000.);
#26695=VECTOR('',#79801,1000.);
#26696=VECTOR('',#79810,1000.);
#26697=VECTOR('',#79811,1000.);
#26698=VECTOR('',#79812,1000.);
#26699=VECTOR('',#79813,1000.);
#26700=VECTOR('',#79822,1000.);
#26701=VECTOR('',#79823,1000.);
#26702=VECTOR('',#79832,1000.);
#26703=VECTOR('',#79833,1000.);
#26704=VECTOR('',#79842,1000.);
#26705=VECTOR('',#79843,1000.);
#26706=VECTOR('',#79852,1000.);
#26707=VECTOR('',#79853,1000.);
#26708=VECTOR('',#79862,1000.);
#26709=VECTOR('',#79863,1000.);
#26710=VECTOR('',#79872,1000.);
#26711=VECTOR('',#79873,1000.);
#26712=VECTOR('',#79882,1000.);
#26713=VECTOR('',#79883,1000.);
#26714=VECTOR('',#79892,1000.);
#26715=VECTOR('',#79893,1000.);
#26716=VECTOR('',#79902,1000.);
#26717=VECTOR('',#79903,1000.);
#26718=VECTOR('',#79912,1000.);
#26719=VECTOR('',#79913,1000.);
#26720=VECTOR('',#79922,1000.);
#26721=VECTOR('',#79923,1000.);
#26722=VECTOR('',#79932,1000.);
#26723=VECTOR('',#79933,1000.);
#26724=VECTOR('',#79942,1000.);
#26725=VECTOR('',#79943,1000.);
#26726=VECTOR('',#79952,1000.);
#26727=VECTOR('',#79953,1000.);
#26728=VECTOR('',#79962,1000.);
#26729=VECTOR('',#79963,1000.);
#26730=VECTOR('',#79972,1000.);
#26731=VECTOR('',#79973,1000.);
#26732=VECTOR('',#79976,1000.);
#26733=VECTOR('',#79983,1000.);
#26734=VECTOR('',#79992,1000.);
#26735=VECTOR('',#79993,1000.);
#26736=VECTOR('',#80002,1000.);
#26737=VECTOR('',#80003,1000.);
#26738=VECTOR('',#80012,1000.);
#26739=VECTOR('',#80013,1000.);
#26740=VECTOR('',#80022,1000.);
#26741=VECTOR('',#80029,1000.);
#26742=VECTOR('',#80032,1000.);
#26743=VECTOR('',#80033,1000.);
#26744=VECTOR('',#80036,1000.);
#26745=VECTOR('',#80043,1000.);
#26746=VECTOR('',#80046,1000.);
#26747=VECTOR('',#80053,1000.);
#26748=VECTOR('',#80056,1000.);
#26749=VECTOR('',#80063,1000.);
#26750=VECTOR('',#80066,1000.);
#26751=VECTOR('',#80073,1000.);
#26752=VECTOR('',#80076,1000.);
#26753=VECTOR('',#80083,1000.);
#26754=VECTOR('',#80086,1000.);
#26755=VECTOR('',#80093,1000.);
#26756=VECTOR('',#80096,1000.);
#26757=VECTOR('',#80103,1000.);
#26758=VECTOR('',#80106,1000.);
#26759=VECTOR('',#80113,1000.);
#26760=VECTOR('',#80116,1000.);
#26761=VECTOR('',#80123,1000.);
#26762=VECTOR('',#80126,1000.);
#26763=VECTOR('',#80133,1000.);
#26764=VECTOR('',#80136,1000.);
#26765=VECTOR('',#80143,1000.);
#26766=VECTOR('',#80146,1000.);
#26767=VECTOR('',#80153,1000.);
#26768=VECTOR('',#80156,1000.);
#26769=VECTOR('',#80163,1000.);
#26770=VECTOR('',#80164,1000.);
#26771=VECTOR('',#80165,1000.);
#26772=VECTOR('',#80168,1000.);
#26773=VECTOR('',#80175,1000.);
#26774=VECTOR('',#80178,1000.);
#26775=VECTOR('',#80185,1000.);
#26776=VECTOR('',#80188,1000.);
#26777=VECTOR('',#80195,1000.);
#26778=VECTOR('',#80198,1000.);
#26779=VECTOR('',#80205,1000.);
#26780=VECTOR('',#80208,1000.);
#26781=VECTOR('',#80215,1000.);
#26782=VECTOR('',#80218,1000.);
#26783=VECTOR('',#80225,1000.);
#26784=VECTOR('',#80228,1000.);
#26785=VECTOR('',#80235,1000.);
#26786=VECTOR('',#80238,1000.);
#26787=VECTOR('',#80245,1000.);
#26788=VECTOR('',#80248,1000.);
#26789=VECTOR('',#80255,1000.);
#26790=VECTOR('',#80258,1000.);
#26791=VECTOR('',#80265,1000.);
#26792=VECTOR('',#80268,1000.);
#26793=VECTOR('',#80275,1000.);
#26794=VECTOR('',#80278,1000.);
#26795=VECTOR('',#80285,1000.);
#26796=VECTOR('',#80288,1000.);
#26797=VECTOR('',#80295,1000.);
#26798=VECTOR('',#80298,1000.);
#26799=VECTOR('',#80311,1000.);
#26800=VECTOR('',#80488,1000.);
#26801=VECTOR('',#80497,1000.);
#26802=VECTOR('',#80500,1000.);
#26803=VECTOR('',#80509,1000.);
#26804=VECTOR('',#80512,1000.);
#26805=VECTOR('',#80521,1000.);
#26806=VECTOR('',#80524,1000.);
#26807=VECTOR('',#80533,1000.);
#26808=VECTOR('',#80536,1000.);
#26809=VECTOR('',#80545,1000.);
#26810=VECTOR('',#80548,1000.);
#26811=VECTOR('',#80557,1000.);
#26812=VECTOR('',#80560,1000.);
#26813=VECTOR('',#80569,1000.);
#26814=VECTOR('',#80572,1000.);
#26815=VECTOR('',#80581,1000.);
#26816=VECTOR('',#80584,1000.);
#26817=VECTOR('',#80593,1000.);
#26818=VECTOR('',#80596,1000.);
#26819=VECTOR('',#80605,1000.);
#26820=VECTOR('',#80608,1000.);
#26821=VECTOR('',#80617,1000.);
#26822=VECTOR('',#80620,1000.);
#26823=VECTOR('',#80629,1000.);
#26824=VECTOR('',#80632,1000.);
#26825=VECTOR('',#80641,1000.);
#26826=VECTOR('',#80644,1000.);
#26827=VECTOR('',#80653,1000.);
#26828=VECTOR('',#80654,1000.);
#26829=VECTOR('',#80655,1000.);
#26830=VECTOR('',#80658,1000.);
#26831=VECTOR('',#80667,1000.);
#26832=VECTOR('',#80670,1000.);
#26833=VECTOR('',#80679,1000.);
#26834=VECTOR('',#80682,1000.);
#26835=VECTOR('',#80691,1000.);
#26836=VECTOR('',#80694,1000.);
#26837=VECTOR('',#80703,1000.);
#26838=VECTOR('',#80706,1000.);
#26839=VECTOR('',#80715,1000.);
#26840=VECTOR('',#80718,1000.);
#26841=VECTOR('',#80727,1000.);
#26842=VECTOR('',#80730,1000.);
#26843=VECTOR('',#80739,1000.);
#26844=VECTOR('',#80742,1000.);
#26845=VECTOR('',#80751,1000.);
#26846=VECTOR('',#80754,1000.);
#26847=VECTOR('',#80757,1000.);
#26848=VECTOR('',#80764,1000.);
#26849=VECTOR('',#80775,1000.);
#26850=VECTOR('',#80778,1000.);
#26851=VECTOR('',#80787,1000.);
#26852=VECTOR('',#80790,1000.);
#26853=VECTOR('',#80799,1000.);
#26854=VECTOR('',#80802,1000.);
#26855=VECTOR('',#80811,1000.);
#26856=VECTOR('',#80814,1000.);
#26857=VECTOR('',#80823,1000.);
#26858=VECTOR('',#80824,1000.);
#26859=VECTOR('',#80827,1000.);
#26860=VECTOR('',#80834,1000.);
#26861=VECTOR('',#80837,1000.);
#26862=VECTOR('',#80844,1000.);
#26863=VECTOR('',#80847,1000.);
#26864=VECTOR('',#80854,1000.);
#26865=VECTOR('',#80857,1000.);
#26866=VECTOR('',#80864,1000.);
#26867=VECTOR('',#80867,1000.);
#26868=VECTOR('',#80874,1000.);
#26869=VECTOR('',#80877,1000.);
#26870=VECTOR('',#80884,1000.);
#26871=VECTOR('',#80887,1000.);
#26872=VECTOR('',#80894,1000.);
#26873=VECTOR('',#80897,1000.);
#26874=VECTOR('',#80904,1000.);
#26875=VECTOR('',#80907,1000.);
#26876=VECTOR('',#80914,1000.);
#26877=VECTOR('',#80917,1000.);
#26878=VECTOR('',#80924,1000.);
#26879=VECTOR('',#80927,1000.);
#26880=VECTOR('',#80934,1000.);
#26881=VECTOR('',#80937,1000.);
#26882=VECTOR('',#80944,1000.);
#26883=VECTOR('',#80947,1000.);
#26884=VECTOR('',#80954,1000.);
#26885=VECTOR('',#80957,1000.);
#26886=VECTOR('',#80964,1000.);
#26887=VECTOR('',#80967,1000.);
#26888=VECTOR('',#80974,1000.);
#26889=VECTOR('',#80977,1000.);
#26890=VECTOR('',#80984,1000.);
#26891=VECTOR('',#80987,1000.);
#26892=VECTOR('',#80994,1000.);
#26893=VECTOR('',#80997,1000.);
#26894=VECTOR('',#81004,1000.);
#26895=VECTOR('',#81007,1000.);
#26896=VECTOR('',#81014,1000.);
#26897=VECTOR('',#81017,1000.);
#26898=VECTOR('',#81024,1000.);
#26899=VECTOR('',#81027,1000.);
#26900=VECTOR('',#81034,1000.);
#26901=VECTOR('',#81037,1000.);
#26902=VECTOR('',#81044,1000.);
#26903=VECTOR('',#81047,1000.);
#26904=VECTOR('',#81054,1000.);
#26905=VECTOR('',#81057,1000.);
#26906=VECTOR('',#81064,1000.);
#26907=VECTOR('',#81067,1000.);
#26908=VECTOR('',#81074,1000.);
#26909=VECTOR('',#81077,1000.);
#26910=VECTOR('',#81084,1000.);
#26911=VECTOR('',#81087,1000.);
#26912=VECTOR('',#81094,1000.);
#26913=VECTOR('',#81097,1000.);
#26914=VECTOR('',#81104,1000.);
#26915=VECTOR('',#81107,1000.);
#26916=VECTOR('',#81348,1000.);
#26917=VECTOR('',#81351,1000.);
#26918=VECTOR('',#81358,1000.);
#26919=VECTOR('',#81361,1000.);
#26920=VECTOR('',#81368,1000.);
#26921=VECTOR('',#81371,1000.);
#26922=VECTOR('',#81378,1000.);
#26923=VECTOR('',#81381,1000.);
#26924=VECTOR('',#81388,1000.);
#26925=VECTOR('',#81391,1000.);
#26926=VECTOR('',#81398,1000.);
#26927=VECTOR('',#81401,1000.);
#26928=VECTOR('',#81408,1000.);
#26929=VECTOR('',#81409,1000.);
#26930=VECTOR('',#81410,1000.);
#26931=VECTOR('',#81413,1000.);
#26932=VECTOR('',#81420,1000.);
#26933=VECTOR('',#81423,1000.);
#26934=VECTOR('',#81430,1000.);
#26935=VECTOR('',#81433,1000.);
#26936=VECTOR('',#81440,1000.);
#26937=VECTOR('',#81443,1000.);
#26938=VECTOR('',#81450,1000.);
#26939=VECTOR('',#81453,1000.);
#26940=VECTOR('',#81460,1000.);
#26941=VECTOR('',#81463,1000.);
#26942=VECTOR('',#81470,1000.);
#26943=VECTOR('',#81473,1000.);
#26944=VECTOR('',#81480,1000.);
#26945=VECTOR('',#81483,1000.);
#26946=VECTOR('',#81490,1000.);
#26947=VECTOR('',#81493,1000.);
#26948=VECTOR('',#81500,1000.);
#26949=VECTOR('',#81503,1000.);
#26950=VECTOR('',#81510,1000.);
#26951=VECTOR('',#81513,1000.);
#26952=VECTOR('',#81520,1000.);
#26953=VECTOR('',#81523,1000.);
#26954=VECTOR('',#81530,1000.);
#26955=VECTOR('',#81533,1000.);
#26956=VECTOR('',#81540,1000.);
#26957=VECTOR('',#81543,1000.);
#26958=VECTOR('',#81550,1000.);
#26959=VECTOR('',#81553,1000.);
#26960=VECTOR('',#81560,1000.);
#26961=VECTOR('',#81563,1000.);
#26962=VECTOR('',#81566,1000.);
#26963=VECTOR('',#81571,1000.);
#26964=VECTOR('',#81580,1000.);
#26965=VECTOR('',#81583,1000.);
#26966=VECTOR('',#81590,1000.);
#26967=VECTOR('',#81593,1000.);
#26968=VECTOR('',#81600,1000.);
#26969=VECTOR('',#81603,1000.);
#26970=VECTOR('',#81610,1000.);
#26971=VECTOR('',#81613,1000.);
#26972=VECTOR('',#81620,1000.);
#26973=VECTOR('',#81627,1000.);
#26974=VECTOR('',#81630,1000.);
#26975=VECTOR('',#81631,1000.);
#26976=VECTOR('',#81636,1000.);
#26977=VECTOR('',#81643,1000.);
#26978=VECTOR('',#81648,1000.);
#26979=VECTOR('',#81655,1000.);
#26980=VECTOR('',#81660,1000.);
#26981=VECTOR('',#81667,1000.);
#26982=VECTOR('',#81672,1000.);
#26983=VECTOR('',#81679,1000.);
#26984=VECTOR('',#81684,1000.);
#26985=VECTOR('',#81691,1000.);
#26986=VECTOR('',#81696,1000.);
#26987=VECTOR('',#81703,1000.);
#26988=VECTOR('',#81708,1000.);
#26989=VECTOR('',#81715,1000.);
#26990=VECTOR('',#81720,1000.);
#26991=VECTOR('',#81727,1000.);
#26992=VECTOR('',#81732,1000.);
#26993=VECTOR('',#81739,1000.);
#26994=VECTOR('',#81744,1000.);
#26995=VECTOR('',#81751,1000.);
#26996=VECTOR('',#81756,1000.);
#26997=VECTOR('',#81763,1000.);
#26998=VECTOR('',#81768,1000.);
#26999=VECTOR('',#81775,1000.);
#27000=VECTOR('',#81780,1000.);
#27001=VECTOR('',#81787,1000.);
#27002=VECTOR('',#81788,1000.);
#27003=VECTOR('',#81789,1000.);
#27004=VECTOR('',#81794,1000.);
#27005=VECTOR('',#81801,1000.);
#27006=VECTOR('',#81806,1000.);
#27007=VECTOR('',#81813,1000.);
#27008=VECTOR('',#81818,1000.);
#27009=VECTOR('',#81825,1000.);
#27010=VECTOR('',#81830,1000.);
#27011=VECTOR('',#81837,1000.);
#27012=VECTOR('',#81842,1000.);
#27013=VECTOR('',#81849,1000.);
#27014=VECTOR('',#81854,1000.);
#27015=VECTOR('',#81861,1000.);
#27016=VECTOR('',#81866,1000.);
#27017=VECTOR('',#81873,1000.);
#27018=VECTOR('',#81878,1000.);
#27019=VECTOR('',#81885,1000.);
#27020=VECTOR('',#81890,1000.);
#27021=VECTOR('',#81897,1000.);
#27022=VECTOR('',#81902,1000.);
#27023=VECTOR('',#81909,1000.);
#27024=VECTOR('',#81914,1000.);
#27025=VECTOR('',#81921,1000.);
#27026=VECTOR('',#81926,1000.);
#27027=VECTOR('',#81933,1000.);
#27028=VECTOR('',#81938,1000.);
#27029=VECTOR('',#81945,1000.);
#27030=VECTOR('',#81950,1000.);
#27031=VECTOR('',#81965,1000.);
#27032=VECTOR('',#82142,1000.);
#27033=VECTOR('',#82149,1000.);
#27034=VECTOR('',#82152,1000.);
#27035=VECTOR('',#82159,1000.);
#27036=VECTOR('',#82162,1000.);
#27037=VECTOR('',#82169,1000.);
#27038=VECTOR('',#82172,1000.);
#27039=VECTOR('',#82179,1000.);
#27040=VECTOR('',#82182,1000.);
#27041=VECTOR('',#82189,1000.);
#27042=VECTOR('',#82192,1000.);
#27043=VECTOR('',#82199,1000.);
#27044=VECTOR('',#82202,1000.);
#27045=VECTOR('',#82209,1000.);
#27046=VECTOR('',#82212,1000.);
#27047=VECTOR('',#82219,1000.);
#27048=VECTOR('',#82222,1000.);
#27049=VECTOR('',#82229,1000.);
#27050=VECTOR('',#82232,1000.);
#27051=VECTOR('',#82239,1000.);
#27052=VECTOR('',#82242,1000.);
#27053=VECTOR('',#82249,1000.);
#27054=VECTOR('',#82252,1000.);
#27055=VECTOR('',#82259,1000.);
#27056=VECTOR('',#82262,1000.);
#27057=VECTOR('',#82269,1000.);
#27058=VECTOR('',#82272,1000.);
#27059=VECTOR('',#82279,1000.);
#27060=VECTOR('',#82280,1000.);
#27061=VECTOR('',#82281,1000.);
#27062=VECTOR('',#82284,1000.);
#27063=VECTOR('',#82291,1000.);
#27064=VECTOR('',#82294,1000.);
#27065=VECTOR('',#82301,1000.);
#27066=VECTOR('',#82304,1000.);
#27067=VECTOR('',#82311,1000.);
#27068=VECTOR('',#82314,1000.);
#27069=VECTOR('',#82321,1000.);
#27070=VECTOR('',#82324,1000.);
#27071=VECTOR('',#82331,1000.);
#27072=VECTOR('',#82334,1000.);
#27073=VECTOR('',#82341,1000.);
#27074=VECTOR('',#82344,1000.);
#27075=VECTOR('',#82351,1000.);
#27076=VECTOR('',#82354,1000.);
#27077=VECTOR('',#82355,1000.);
#27078=VECTOR('',#82362,1000.);
#27079=VECTOR('',#82371,1000.);
#27080=VECTOR('',#82374,1000.);
#27081=VECTOR('',#82381,1000.);
#27082=VECTOR('',#82384,1000.);
#27083=VECTOR('',#82391,1000.);
#27084=VECTOR('',#82394,1000.);
#27085=VECTOR('',#82401,1000.);
#27086=VECTOR('',#82404,1000.);
#27087=VECTOR('',#82411,1000.);
#27088=VECTOR('',#82414,1000.);
#27089=VECTOR('',#82421,1000.);
#27090=VECTOR('',#82422,1000.);
#27091=VECTOR('',#82427,1000.);
#27092=VECTOR('',#82434,1000.);
#27093=VECTOR('',#82439,1000.);
#27094=VECTOR('',#82446,1000.);
#27095=VECTOR('',#82451,1000.);
#27096=VECTOR('',#82458,1000.);
#27097=VECTOR('',#82463,1000.);
#27098=VECTOR('',#82470,1000.);
#27099=VECTOR('',#82475,1000.);
#27100=VECTOR('',#82482,1000.);
#27101=VECTOR('',#82487,1000.);
#27102=VECTOR('',#82494,1000.);
#27103=VECTOR('',#82499,1000.);
#27104=VECTOR('',#82506,1000.);
#27105=VECTOR('',#82511,1000.);
#27106=VECTOR('',#82518,1000.);
#27107=VECTOR('',#82523,1000.);
#27108=VECTOR('',#82530,1000.);
#27109=VECTOR('',#82535,1000.);
#27110=VECTOR('',#82542,1000.);
#27111=VECTOR('',#82547,1000.);
#27112=VECTOR('',#82554,1000.);
#27113=VECTOR('',#82559,1000.);
#27114=VECTOR('',#82566,1000.);
#27115=VECTOR('',#82571,1000.);
#27116=VECTOR('',#82578,1000.);
#27117=VECTOR('',#82583,1000.);
#27118=VECTOR('',#82590,1000.);
#27119=VECTOR('',#82595,1000.);
#27120=VECTOR('',#82602,1000.);
#27121=VECTOR('',#82607,1000.);
#27122=VECTOR('',#82614,1000.);
#27123=VECTOR('',#82619,1000.);
#27124=VECTOR('',#82626,1000.);
#27125=VECTOR('',#82631,1000.);
#27126=VECTOR('',#82638,1000.);
#27127=VECTOR('',#82643,1000.);
#27128=VECTOR('',#82650,1000.);
#27129=VECTOR('',#82655,1000.);
#27130=VECTOR('',#82662,1000.);
#27131=VECTOR('',#82667,1000.);
#27132=VECTOR('',#82674,1000.);
#27133=VECTOR('',#82675,1000.);
#27134=VECTOR('',#82676,1000.);
#27135=VECTOR('',#82681,1000.);
#27136=VECTOR('',#82688,1000.);
#27137=VECTOR('',#82693,1000.);
#27138=VECTOR('',#82700,1000.);
#27139=VECTOR('',#82705,1000.);
#27140=VECTOR('',#82712,1000.);
#27141=VECTOR('',#82717,1000.);
#27142=VECTOR('',#82724,1000.);
#27143=VECTOR('',#82729,1000.);
#27144=VECTOR('',#82736,1000.);
#27145=VECTOR('',#82741,1000.);
#27146=VECTOR('',#82748,1000.);
#27147=VECTOR('',#82753,1000.);
#27148=VECTOR('',#82878,1000.);
#27149=VECTOR('',#82879,1000.);
#27150=VECTOR('',#82888,1000.);
#27151=VECTOR('',#82889,1000.);
#27152=VECTOR('',#82898,1000.);
#27153=VECTOR('',#82899,1000.);
#27154=VECTOR('',#82908,1000.);
#27155=VECTOR('',#82909,1000.);
#27156=VECTOR('',#82918,1000.);
#27157=VECTOR('',#82919,1000.);
#27158=VECTOR('',#82928,1000.);
#27159=VECTOR('',#82929,1000.);
#27160=VECTOR('',#82938,1000.);
#27161=VECTOR('',#82939,1000.);
#27162=VECTOR('',#82940,1000.);
#27163=VECTOR('',#82941,1000.);
#27164=VECTOR('',#82950,1000.);
#27165=VECTOR('',#82951,1000.);
#27166=VECTOR('',#82960,1000.);
#27167=VECTOR('',#82961,1000.);
#27168=VECTOR('',#82970,1000.);
#27169=VECTOR('',#82971,1000.);
#27170=VECTOR('',#82980,1000.);
#27171=VECTOR('',#82981,1000.);
#27172=VECTOR('',#82990,1000.);
#27173=VECTOR('',#82991,1000.);
#27174=VECTOR('',#83000,1000.);
#27175=VECTOR('',#83001,1000.);
#27176=VECTOR('',#83010,1000.);
#27177=VECTOR('',#83011,1000.);
#27178=VECTOR('',#83020,1000.);
#27179=VECTOR('',#83021,1000.);
#27180=VECTOR('',#83030,1000.);
#27181=VECTOR('',#83031,1000.);
#27182=VECTOR('',#83040,1000.);
#27183=VECTOR('',#83041,1000.);
#27184=VECTOR('',#83050,1000.);
#27185=VECTOR('',#83051,1000.);
#27186=VECTOR('',#83060,1000.);
#27187=VECTOR('',#83061,1000.);
#27188=VECTOR('',#83070,1000.);
#27189=VECTOR('',#83071,1000.);
#27190=VECTOR('',#83080,1000.);
#27191=VECTOR('',#83081,1000.);
#27192=VECTOR('',#83084,1000.);
#27193=VECTOR('',#83091,1000.);
#27194=VECTOR('',#83100,1000.);
#27195=VECTOR('',#83101,1000.);
#27196=VECTOR('',#83110,1000.);
#27197=VECTOR('',#83111,1000.);
#27198=VECTOR('',#83120,1000.);
#27199=VECTOR('',#83121,1000.);
#27200=VECTOR('',#83130,1000.);
#27201=VECTOR('',#83131,1000.);
#27202=VECTOR('',#83140,1000.);
#27203=VECTOR('',#83141,1000.);
#27204=VECTOR('',#83150,1000.);
#27205=VECTOR('',#83157,1000.);
#27206=VECTOR('',#83160,1000.);
#27207=VECTOR('',#83161,1000.);
#27208=VECTOR('',#83164,1000.);
#27209=VECTOR('',#83171,1000.);
#27210=VECTOR('',#83174,1000.);
#27211=VECTOR('',#83181,1000.);
#27212=VECTOR('',#83184,1000.);
#27213=VECTOR('',#83191,1000.);
#27214=VECTOR('',#83194,1000.);
#27215=VECTOR('',#83201,1000.);
#27216=VECTOR('',#83204,1000.);
#27217=VECTOR('',#83211,1000.);
#27218=VECTOR('',#83214,1000.);
#27219=VECTOR('',#83221,1000.);
#27220=VECTOR('',#83224,1000.);
#27221=VECTOR('',#83231,1000.);
#27222=VECTOR('',#83234,1000.);
#27223=VECTOR('',#83241,1000.);
#27224=VECTOR('',#83244,1000.);
#27225=VECTOR('',#83251,1000.);
#27226=VECTOR('',#83254,1000.);
#27227=VECTOR('',#83261,1000.);
#27228=VECTOR('',#83264,1000.);
#27229=VECTOR('',#83271,1000.);
#27230=VECTOR('',#83274,1000.);
#27231=VECTOR('',#83281,1000.);
#27232=VECTOR('',#83284,1000.);
#27233=VECTOR('',#83291,1000.);
#27234=VECTOR('',#83292,1000.);
#27235=VECTOR('',#83293,1000.);
#27236=VECTOR('',#83296,1000.);
#27237=VECTOR('',#83303,1000.);
#27238=VECTOR('',#83306,1000.);
#27239=VECTOR('',#83313,1000.);
#27240=VECTOR('',#83316,1000.);
#27241=VECTOR('',#83323,1000.);
#27242=VECTOR('',#83326,1000.);
#27243=VECTOR('',#83333,1000.);
#27244=VECTOR('',#83336,1000.);
#27245=VECTOR('',#83343,1000.);
#27246=VECTOR('',#83346,1000.);
#27247=VECTOR('',#83353,1000.);
#27248=VECTOR('',#83356,1000.);
#27249=VECTOR('',#83363,1000.);
#27250=VECTOR('',#83366,1000.);
#27251=VECTOR('',#83373,1000.);
#27252=VECTOR('',#83376,1000.);
#27253=VECTOR('',#83383,1000.);
#27254=VECTOR('',#83386,1000.);
#27255=VECTOR('',#83393,1000.);
#27256=VECTOR('',#83396,1000.);
#27257=VECTOR('',#83403,1000.);
#27258=VECTOR('',#83406,1000.);
#27259=VECTOR('',#83413,1000.);
#27260=VECTOR('',#83416,1000.);
#27261=VECTOR('',#83423,1000.);
#27262=VECTOR('',#83426,1000.);
#27263=VECTOR('',#83439,1000.);
#27264=VECTOR('',#83616,1000.);
#27265=VECTOR('',#83625,1000.);
#27266=VECTOR('',#83628,1000.);
#27267=VECTOR('',#83637,1000.);
#27268=VECTOR('',#83640,1000.);
#27269=VECTOR('',#83649,1000.);
#27270=VECTOR('',#83652,1000.);
#27271=VECTOR('',#83661,1000.);
#27272=VECTOR('',#83664,1000.);
#27273=VECTOR('',#83673,1000.);
#27274=VECTOR('',#83676,1000.);
#27275=VECTOR('',#83685,1000.);
#27276=VECTOR('',#83688,1000.);
#27277=VECTOR('',#83697,1000.);
#27278=VECTOR('',#83700,1000.);
#27279=VECTOR('',#83709,1000.);
#27280=VECTOR('',#83712,1000.);
#27281=VECTOR('',#83721,1000.);
#27282=VECTOR('',#83724,1000.);
#27283=VECTOR('',#83733,1000.);
#27284=VECTOR('',#83736,1000.);
#27285=VECTOR('',#83745,1000.);
#27286=VECTOR('',#83748,1000.);
#27287=VECTOR('',#83757,1000.);
#27288=VECTOR('',#83760,1000.);
#27289=VECTOR('',#83769,1000.);
#27290=VECTOR('',#83772,1000.);
#27291=VECTOR('',#83781,1000.);
#27292=VECTOR('',#83782,1000.);
#27293=VECTOR('',#83783,1000.);
#27294=VECTOR('',#83786,1000.);
#27295=VECTOR('',#83795,1000.);
#27296=VECTOR('',#83798,1000.);
#27297=VECTOR('',#83807,1000.);
#27298=VECTOR('',#83810,1000.);
#27299=VECTOR('',#83819,1000.);
#27300=VECTOR('',#83822,1000.);
#27301=VECTOR('',#83831,1000.);
#27302=VECTOR('',#83834,1000.);
#27303=VECTOR('',#83843,1000.);
#27304=VECTOR('',#83846,1000.);
#27305=VECTOR('',#83855,1000.);
#27306=VECTOR('',#83858,1000.);
#27307=VECTOR('',#83861,1000.);
#27308=VECTOR('',#83868,1000.);
#27309=VECTOR('',#83879,1000.);
#27310=VECTOR('',#83882,1000.);
#27311=VECTOR('',#83891,1000.);
#27312=VECTOR('',#83894,1000.);
#27313=VECTOR('',#83903,1000.);
#27314=VECTOR('',#83906,1000.);
#27315=VECTOR('',#83915,1000.);
#27316=VECTOR('',#83918,1000.);
#27317=VECTOR('',#83927,1000.);
#27318=VECTOR('',#83930,1000.);
#27319=VECTOR('',#83939,1000.);
#27320=VECTOR('',#83942,1000.);
#27321=VECTOR('',#83951,1000.);
#27322=VECTOR('',#83952,1000.);
#27323=VECTOR('',#83955,1000.);
#27324=VECTOR('',#83962,1000.);
#27325=VECTOR('',#83965,1000.);
#27326=VECTOR('',#83972,1000.);
#27327=VECTOR('',#83975,1000.);
#27328=VECTOR('',#83982,1000.);
#27329=VECTOR('',#83985,1000.);
#27330=VECTOR('',#83992,1000.);
#27331=VECTOR('',#83995,1000.);
#27332=VECTOR('',#84002,1000.);
#27333=VECTOR('',#84005,1000.);
#27334=VECTOR('',#84012,1000.);
#27335=VECTOR('',#84015,1000.);
#27336=VECTOR('',#84022,1000.);
#27337=VECTOR('',#84025,1000.);
#27338=VECTOR('',#84032,1000.);
#27339=VECTOR('',#84035,1000.);
#27340=VECTOR('',#84042,1000.);
#27341=VECTOR('',#84045,1000.);
#27342=VECTOR('',#84052,1000.);
#27343=VECTOR('',#84055,1000.);
#27344=VECTOR('',#84062,1000.);
#27345=VECTOR('',#84065,1000.);
#27346=VECTOR('',#84072,1000.);
#27347=VECTOR('',#84075,1000.);
#27348=VECTOR('',#84082,1000.);
#27349=VECTOR('',#84085,1000.);
#27350=VECTOR('',#84092,1000.);
#27351=VECTOR('',#84095,1000.);
#27352=VECTOR('',#84102,1000.);
#27353=VECTOR('',#84105,1000.);
#27354=VECTOR('',#84112,1000.);
#27355=VECTOR('',#84115,1000.);
#27356=VECTOR('',#84122,1000.);
#27357=VECTOR('',#84125,1000.);
#27358=VECTOR('',#84132,1000.);
#27359=VECTOR('',#84135,1000.);
#27360=VECTOR('',#84142,1000.);
#27361=VECTOR('',#84145,1000.);
#27362=VECTOR('',#84152,1000.);
#27363=VECTOR('',#84155,1000.);
#27364=VECTOR('',#84162,1000.);
#27365=VECTOR('',#84163,1000.);
#27366=VECTOR('',#84164,1000.);
#27367=VECTOR('',#84167,1000.);
#27368=VECTOR('',#84174,1000.);
#27369=VECTOR('',#84177,1000.);
#27370=VECTOR('',#84184,1000.);
#27371=VECTOR('',#84187,1000.);
#27372=VECTOR('',#84194,1000.);
#27373=VECTOR('',#84197,1000.);
#27374=VECTOR('',#84204,1000.);
#27375=VECTOR('',#84207,1000.);
#27376=VECTOR('',#84214,1000.);
#27377=VECTOR('',#84217,1000.);
#27378=VECTOR('',#84224,1000.);
#27379=VECTOR('',#84227,1000.);
#27380=VECTOR('',#84468,1000.);
#27381=VECTOR('',#84471,1000.);
#27382=VECTOR('',#84480,1000.);
#27383=VECTOR('',#84483,1000.);
#27384=VECTOR('',#84492,1000.);
#27385=VECTOR('',#84495,1000.);
#27386=VECTOR('',#84504,1000.);
#27387=VECTOR('',#84507,1000.);
#27388=VECTOR('',#84516,1000.);
#27389=VECTOR('',#84519,1000.);
#27390=VECTOR('',#84528,1000.);
#27391=VECTOR('',#84531,1000.);
#27392=VECTOR('',#84540,1000.);
#27393=VECTOR('',#84541,1000.);
#27394=VECTOR('',#84542,1000.);
#27395=VECTOR('',#84545,1000.);
#27396=VECTOR('',#84554,1000.);
#27397=VECTOR('',#84557,1000.);
#27398=VECTOR('',#84566,1000.);
#27399=VECTOR('',#84569,1000.);
#27400=VECTOR('',#84578,1000.);
#27401=VECTOR('',#84581,1000.);
#27402=VECTOR('',#84590,1000.);
#27403=VECTOR('',#84593,1000.);
#27404=VECTOR('',#84602,1000.);
#27405=VECTOR('',#84605,1000.);
#27406=VECTOR('',#84614,1000.);
#27407=VECTOR('',#84617,1000.);
#27408=VECTOR('',#84626,1000.);
#27409=VECTOR('',#84629,1000.);
#27410=VECTOR('',#84638,1000.);
#27411=VECTOR('',#84641,1000.);
#27412=VECTOR('',#84650,1000.);
#27413=VECTOR('',#84653,1000.);
#27414=VECTOR('',#84662,1000.);
#27415=VECTOR('',#84665,1000.);
#27416=VECTOR('',#84674,1000.);
#27417=VECTOR('',#84677,1000.);
#27418=VECTOR('',#84686,1000.);
#27419=VECTOR('',#84689,1000.);
#27420=VECTOR('',#84698,1000.);
#27421=VECTOR('',#84701,1000.);
#27422=VECTOR('',#84704,1000.);
#27423=VECTOR('',#84711,1000.);
#27424=VECTOR('',#84722,1000.);
#27425=VECTOR('',#84725,1000.);
#27426=VECTOR('',#84734,1000.);
#27427=VECTOR('',#84737,1000.);
#27428=VECTOR('',#84746,1000.);
#27429=VECTOR('',#84749,1000.);
#27430=VECTOR('',#84758,1000.);
#27431=VECTOR('',#84761,1000.);
#27432=VECTOR('',#84770,1000.);
#27433=VECTOR('',#84773,1000.);
#27434=VECTOR('',#84782,1000.);
#27435=VECTOR('',#84785,1000.);
#27436=VECTOR('',#84794,1000.);
#27437=VECTOR('',#84803,1000.);
#27438=VECTOR('',#84806,1000.);
#27439=VECTOR('',#84807,1000.);
#27440=VECTOR('',#84812,1000.);
#27441=VECTOR('',#84819,1000.);
#27442=VECTOR('',#84824,1000.);
#27443=VECTOR('',#84831,1000.);
#27444=VECTOR('',#84836,1000.);
#27445=VECTOR('',#84843,1000.);
#27446=VECTOR('',#84848,1000.);
#27447=VECTOR('',#84855,1000.);
#27448=VECTOR('',#84860,1000.);
#27449=VECTOR('',#84867,1000.);
#27450=VECTOR('',#84872,1000.);
#27451=VECTOR('',#84879,1000.);
#27452=VECTOR('',#84884,1000.);
#27453=VECTOR('',#84891,1000.);
#27454=VECTOR('',#84896,1000.);
#27455=VECTOR('',#84903,1000.);
#27456=VECTOR('',#84908,1000.);
#27457=VECTOR('',#84915,1000.);
#27458=VECTOR('',#84920,1000.);
#27459=VECTOR('',#84927,1000.);
#27460=VECTOR('',#84932,1000.);
#27461=VECTOR('',#84939,1000.);
#27462=VECTOR('',#84944,1000.);
#27463=VECTOR('',#84951,1000.);
#27464=VECTOR('',#84956,1000.);
#27465=VECTOR('',#84963,1000.);
#27466=VECTOR('',#84964,1000.);
#27467=VECTOR('',#84965,1000.);
#27468=VECTOR('',#84970,1000.);
#27469=VECTOR('',#84977,1000.);
#27470=VECTOR('',#84982,1000.);
#27471=VECTOR('',#84989,1000.);
#27472=VECTOR('',#84994,1000.);
#27473=VECTOR('',#85001,1000.);
#27474=VECTOR('',#85006,1000.);
#27475=VECTOR('',#85013,1000.);
#27476=VECTOR('',#85018,1000.);
#27477=VECTOR('',#85025,1000.);
#27478=VECTOR('',#85030,1000.);
#27479=VECTOR('',#85037,1000.);
#27480=VECTOR('',#85042,1000.);
#27481=VECTOR('',#85049,1000.);
#27482=VECTOR('',#85054,1000.);
#27483=VECTOR('',#85061,1000.);
#27484=VECTOR('',#85066,1000.);
#27485=VECTOR('',#85073,1000.);
#27486=VECTOR('',#85078,1000.);
#27487=VECTOR('',#85085,1000.);
#27488=VECTOR('',#85090,1000.);
#27489=VECTOR('',#85097,1000.);
#27490=VECTOR('',#85102,1000.);
#27491=VECTOR('',#85109,1000.);
#27492=VECTOR('',#85114,1000.);
#27493=VECTOR('',#85121,1000.);
#27494=VECTOR('',#85126,1000.);
#27495=VECTOR('',#85141,1000.);
#27496=VECTOR('',#85318,1000.);
#27497=VECTOR('',#85325,1000.);
#27498=VECTOR('',#85328,1000.);
#27499=VECTOR('',#85335,1000.);
#27500=VECTOR('',#85338,1000.);
#27501=VECTOR('',#85345,1000.);
#27502=VECTOR('',#85348,1000.);
#27503=VECTOR('',#85355,1000.);
#27504=VECTOR('',#85358,1000.);
#27505=VECTOR('',#85365,1000.);
#27506=VECTOR('',#85368,1000.);
#27507=VECTOR('',#85375,1000.);
#27508=VECTOR('',#85378,1000.);
#27509=VECTOR('',#85385,1000.);
#27510=VECTOR('',#85388,1000.);
#27511=VECTOR('',#85395,1000.);
#27512=VECTOR('',#85398,1000.);
#27513=VECTOR('',#85405,1000.);
#27514=VECTOR('',#85408,1000.);
#27515=VECTOR('',#85415,1000.);
#27516=VECTOR('',#85418,1000.);
#27517=VECTOR('',#85425,1000.);
#27518=VECTOR('',#85428,1000.);
#27519=VECTOR('',#85435,1000.);
#27520=VECTOR('',#85438,1000.);
#27521=VECTOR('',#85445,1000.);
#27522=VECTOR('',#85448,1000.);
#27523=VECTOR('',#85455,1000.);
#27524=VECTOR('',#85456,1000.);
#27525=VECTOR('',#85457,1000.);
#27526=VECTOR('',#85460,1000.);
#27527=VECTOR('',#85467,1000.);
#27528=VECTOR('',#85470,1000.);
#27529=VECTOR('',#85477,1000.);
#27530=VECTOR('',#85480,1000.);
#27531=VECTOR('',#85487,1000.);
#27532=VECTOR('',#85490,1000.);
#27533=VECTOR('',#85497,1000.);
#27534=VECTOR('',#85500,1000.);
#27535=VECTOR('',#85507,1000.);
#27536=VECTOR('',#85510,1000.);
#27537=VECTOR('',#85511,1000.);
#27538=VECTOR('',#85518,1000.);
#27539=VECTOR('',#85527,1000.);
#27540=VECTOR('',#85530,1000.);
#27541=VECTOR('',#85537,1000.);
#27542=VECTOR('',#85540,1000.);
#27543=VECTOR('',#85547,1000.);
#27544=VECTOR('',#85550,1000.);
#27545=VECTOR('',#85557,1000.);
#27546=VECTOR('',#85560,1000.);
#27547=VECTOR('',#85567,1000.);
#27548=VECTOR('',#85570,1000.);
#27549=VECTOR('',#85577,1000.);
#27550=VECTOR('',#85580,1000.);
#27551=VECTOR('',#85587,1000.);
#27552=VECTOR('',#85590,1000.);
#27553=VECTOR('',#85597,1000.);
#27554=VECTOR('',#85598,1000.);
#27555=VECTOR('',#85603,1000.);
#27556=VECTOR('',#85610,1000.);
#27557=VECTOR('',#85615,1000.);
#27558=VECTOR('',#85622,1000.);
#27559=VECTOR('',#85627,1000.);
#27560=VECTOR('',#85634,1000.);
#27561=VECTOR('',#85639,1000.);
#27562=VECTOR('',#85646,1000.);
#27563=VECTOR('',#85651,1000.);
#27564=VECTOR('',#85658,1000.);
#27565=VECTOR('',#85663,1000.);
#27566=VECTOR('',#85670,1000.);
#27567=VECTOR('',#85675,1000.);
#27568=VECTOR('',#85682,1000.);
#27569=VECTOR('',#85687,1000.);
#27570=VECTOR('',#85694,1000.);
#27571=VECTOR('',#85699,1000.);
#27572=VECTOR('',#85706,1000.);
#27573=VECTOR('',#85711,1000.);
#27574=VECTOR('',#85718,1000.);
#27575=VECTOR('',#85723,1000.);
#27576=VECTOR('',#85730,1000.);
#27577=VECTOR('',#85735,1000.);
#27578=VECTOR('',#85742,1000.);
#27579=VECTOR('',#85747,1000.);
#27580=VECTOR('',#85754,1000.);
#27581=VECTOR('',#85759,1000.);
#27582=VECTOR('',#85766,1000.);
#27583=VECTOR('',#85771,1000.);
#27584=VECTOR('',#85778,1000.);
#27585=VECTOR('',#85783,1000.);
#27586=VECTOR('',#85790,1000.);
#27587=VECTOR('',#85795,1000.);
#27588=VECTOR('',#85802,1000.);
#27589=VECTOR('',#85807,1000.);
#27590=VECTOR('',#85814,1000.);
#27591=VECTOR('',#85819,1000.);
#27592=VECTOR('',#85826,1000.);
#27593=VECTOR('',#85831,1000.);
#27594=VECTOR('',#85838,1000.);
#27595=VECTOR('',#85843,1000.);
#27596=VECTOR('',#85850,1000.);
#27597=VECTOR('',#85855,1000.);
#27598=VECTOR('',#85862,1000.);
#27599=VECTOR('',#85867,1000.);
#27600=VECTOR('',#85874,1000.);
#27601=VECTOR('',#85879,1000.);
#27602=VECTOR('',#85886,1000.);
#27603=VECTOR('',#85891,1000.);
#27604=VECTOR('',#85898,1000.);
#27605=VECTOR('',#85903,1000.);
#27606=VECTOR('',#85910,1000.);
#27607=VECTOR('',#85915,1000.);
#27608=VECTOR('',#85922,1000.);
#27609=VECTOR('',#85927,1000.);
#27610=VECTOR('',#85934,1000.);
#27611=VECTOR('',#85939,1000.);
#27612=VECTOR('',#86064,1000.);
#27613=VECTOR('',#86065,1000.);
#27614=VECTOR('',#86074,1000.);
#27615=VECTOR('',#86075,1000.);
#27616=VECTOR('',#86084,1000.);
#27617=VECTOR('',#86085,1000.);
#27618=VECTOR('',#86094,1000.);
#27619=VECTOR('',#86095,1000.);
#27620=VECTOR('',#86104,1000.);
#27621=VECTOR('',#86105,1000.);
#27622=VECTOR('',#86114,1000.);
#27623=VECTOR('',#86115,1000.);
#27624=VECTOR('',#86124,1000.);
#27625=VECTOR('',#86125,1000.);
#27626=VECTOR('',#86126,1000.);
#27627=VECTOR('',#86127,1000.);
#27628=VECTOR('',#86136,1000.);
#27629=VECTOR('',#86137,1000.);
#27630=VECTOR('',#86146,1000.);
#27631=VECTOR('',#86147,1000.);
#27632=VECTOR('',#86156,1000.);
#27633=VECTOR('',#86157,1000.);
#27634=VECTOR('',#86166,1000.);
#27635=VECTOR('',#86167,1000.);
#27636=VECTOR('',#86176,1000.);
#27637=VECTOR('',#86177,1000.);
#27638=VECTOR('',#86186,1000.);
#27639=VECTOR('',#86187,1000.);
#27640=VECTOR('',#86196,1000.);
#27641=VECTOR('',#86197,1000.);
#27642=VECTOR('',#86206,1000.);
#27643=VECTOR('',#86207,1000.);
#27644=VECTOR('',#86216,1000.);
#27645=VECTOR('',#86217,1000.);
#27646=VECTOR('',#86226,1000.);
#27647=VECTOR('',#86227,1000.);
#27648=VECTOR('',#86236,1000.);
#27649=VECTOR('',#86237,1000.);
#27650=VECTOR('',#86246,1000.);
#27651=VECTOR('',#86247,1000.);
#27652=VECTOR('',#86250,1000.);
#27653=VECTOR('',#86257,1000.);
#27654=VECTOR('',#86266,1000.);
#27655=VECTOR('',#86267,1000.);
#27656=VECTOR('',#86276,1000.);
#27657=VECTOR('',#86277,1000.);
#27658=VECTOR('',#86286,1000.);
#27659=VECTOR('',#86287,1000.);
#27660=VECTOR('',#86296,1000.);
#27661=VECTOR('',#86297,1000.);
#27662=VECTOR('',#86306,1000.);
#27663=VECTOR('',#86307,1000.);
#27664=VECTOR('',#86316,1000.);
#27665=VECTOR('',#86317,1000.);
#27666=VECTOR('',#86326,1000.);
#27667=VECTOR('',#86327,1000.);
#27668=VECTOR('',#86336,1000.);
#27669=VECTOR('',#86343,1000.);
#27670=VECTOR('',#86346,1000.);
#27671=VECTOR('',#86347,1000.);
#27672=VECTOR('',#86350,1000.);
#27673=VECTOR('',#86357,1000.);
#27674=VECTOR('',#86360,1000.);
#27675=VECTOR('',#86367,1000.);
#27676=VECTOR('',#86370,1000.);
#27677=VECTOR('',#86377,1000.);
#27678=VECTOR('',#86380,1000.);
#27679=VECTOR('',#86387,1000.);
#27680=VECTOR('',#86390,1000.);
#27681=VECTOR('',#86397,1000.);
#27682=VECTOR('',#86400,1000.);
#27683=VECTOR('',#86407,1000.);
#27684=VECTOR('',#86410,1000.);
#27685=VECTOR('',#86417,1000.);
#27686=VECTOR('',#86420,1000.);
#27687=VECTOR('',#86427,1000.);
#27688=VECTOR('',#86430,1000.);
#27689=VECTOR('',#86437,1000.);
#27690=VECTOR('',#86440,1000.);
#27691=VECTOR('',#86447,1000.);
#27692=VECTOR('',#86450,1000.);
#27693=VECTOR('',#86457,1000.);
#27694=VECTOR('',#86460,1000.);
#27695=VECTOR('',#86467,1000.);
#27696=VECTOR('',#86470,1000.);
#27697=VECTOR('',#86477,1000.);
#27698=VECTOR('',#86478,1000.);
#27699=VECTOR('',#86479,1000.);
#27700=VECTOR('',#86482,1000.);
#27701=VECTOR('',#86489,1000.);
#27702=VECTOR('',#86492,1000.);
#27703=VECTOR('',#86499,1000.);
#27704=VECTOR('',#86502,1000.);
#27705=VECTOR('',#86509,1000.);
#27706=VECTOR('',#86512,1000.);
#27707=VECTOR('',#86519,1000.);
#27708=VECTOR('',#86522,1000.);
#27709=VECTOR('',#86529,1000.);
#27710=VECTOR('',#86532,1000.);
#27711=VECTOR('',#86539,1000.);
#27712=VECTOR('',#86542,1000.);
#27713=VECTOR('',#86549,1000.);
#27714=VECTOR('',#86552,1000.);
#27715=VECTOR('',#86559,1000.);
#27716=VECTOR('',#86562,1000.);
#27717=VECTOR('',#86569,1000.);
#27718=VECTOR('',#86572,1000.);
#27719=VECTOR('',#86579,1000.);
#27720=VECTOR('',#86582,1000.);
#27721=VECTOR('',#86589,1000.);
#27722=VECTOR('',#86592,1000.);
#27723=VECTOR('',#86599,1000.);
#27724=VECTOR('',#86602,1000.);
#27725=VECTOR('',#86609,1000.);
#27726=VECTOR('',#86612,1000.);
#27727=VECTOR('',#86625,1000.);
#27728=VECTOR('',#86860,1000.);
#27729=VECTOR('',#86869,1000.);
#27730=VECTOR('',#86872,1000.);
#27731=VECTOR('',#86881,1000.);
#27732=VECTOR('',#86884,1000.);
#27733=VECTOR('',#86893,1000.);
#27734=VECTOR('',#86896,1000.);
#27735=VECTOR('',#86905,1000.);
#27736=VECTOR('',#86908,1000.);
#27737=VECTOR('',#86917,1000.);
#27738=VECTOR('',#86920,1000.);
#27739=VECTOR('',#86929,1000.);
#27740=VECTOR('',#86932,1000.);
#27741=VECTOR('',#86941,1000.);
#27742=VECTOR('',#86944,1000.);
#27743=VECTOR('',#86953,1000.);
#27744=VECTOR('',#86956,1000.);
#27745=VECTOR('',#86965,1000.);
#27746=VECTOR('',#86968,1000.);
#27747=VECTOR('',#86977,1000.);
#27748=VECTOR('',#86980,1000.);
#27749=VECTOR('',#86989,1000.);
#27750=VECTOR('',#86992,1000.);
#27751=VECTOR('',#87001,1000.);
#27752=VECTOR('',#87004,1000.);
#27753=VECTOR('',#87013,1000.);
#27754=VECTOR('',#87016,1000.);
#27755=VECTOR('',#87025,1000.);
#27756=VECTOR('',#87026,1000.);
#27757=VECTOR('',#87027,1000.);
#27758=VECTOR('',#87030,1000.);
#27759=VECTOR('',#87039,1000.);
#27760=VECTOR('',#87042,1000.);
#27761=VECTOR('',#87051,1000.);
#27762=VECTOR('',#87054,1000.);
#27763=VECTOR('',#87063,1000.);
#27764=VECTOR('',#87066,1000.);
#27765=VECTOR('',#87075,1000.);
#27766=VECTOR('',#87078,1000.);
#27767=VECTOR('',#87081,1000.);
#27768=VECTOR('',#87088,1000.);
#27769=VECTOR('',#87099,1000.);
#27770=VECTOR('',#87102,1000.);
#27771=VECTOR('',#87111,1000.);
#27772=VECTOR('',#87114,1000.);
#27773=VECTOR('',#87123,1000.);
#27774=VECTOR('',#87126,1000.);
#27775=VECTOR('',#87135,1000.);
#27776=VECTOR('',#87138,1000.);
#27777=VECTOR('',#87147,1000.);
#27778=VECTOR('',#87150,1000.);
#27779=VECTOR('',#87159,1000.);
#27780=VECTOR('',#87162,1000.);
#27781=VECTOR('',#87171,1000.);
#27782=VECTOR('',#87174,1000.);
#27783=VECTOR('',#87183,1000.);
#27784=VECTOR('',#87186,1000.);
#27785=VECTOR('',#87195,1000.);
#27786=VECTOR('',#87196,1000.);
#27787=VECTOR('',#87201,1000.);
#27788=VECTOR('',#87208,1000.);
#27789=VECTOR('',#87213,1000.);
#27790=VECTOR('',#87220,1000.);
#27791=VECTOR('',#87225,1000.);
#27792=VECTOR('',#87232,1000.);
#27793=VECTOR('',#87237,1000.);
#27794=VECTOR('',#87244,1000.);
#27795=VECTOR('',#87249,1000.);
#27796=VECTOR('',#87256,1000.);
#27797=VECTOR('',#87261,1000.);
#27798=VECTOR('',#87268,1000.);
#27799=VECTOR('',#87273,1000.);
#27800=VECTOR('',#87280,1000.);
#27801=VECTOR('',#87285,1000.);
#27802=VECTOR('',#87292,1000.);
#27803=VECTOR('',#87297,1000.);
#27804=VECTOR('',#87304,1000.);
#27805=VECTOR('',#87309,1000.);
#27806=VECTOR('',#87316,1000.);
#27807=VECTOR('',#87321,1000.);
#27808=VECTOR('',#87328,1000.);
#27809=VECTOR('',#87333,1000.);
#27810=VECTOR('',#87340,1000.);
#27811=VECTOR('',#87345,1000.);
#27812=VECTOR('',#87352,1000.);
#27813=VECTOR('',#87357,1000.);
#27814=VECTOR('',#87364,1000.);
#27815=VECTOR('',#87369,1000.);
#27816=VECTOR('',#87376,1000.);
#27817=VECTOR('',#87381,1000.);
#27818=VECTOR('',#87388,1000.);
#27819=VECTOR('',#87393,1000.);
#27820=VECTOR('',#87400,1000.);
#27821=VECTOR('',#87405,1000.);
#27822=VECTOR('',#87412,1000.);
#27823=VECTOR('',#87417,1000.);
#27824=VECTOR('',#87424,1000.);
#27825=VECTOR('',#87429,1000.);
#27826=VECTOR('',#87436,1000.);
#27827=VECTOR('',#87441,1000.);
#27828=VECTOR('',#87448,1000.);
#27829=VECTOR('',#87449,1000.);
#27830=VECTOR('',#87450,1000.);
#27831=VECTOR('',#87455,1000.);
#27832=VECTOR('',#87462,1000.);
#27833=VECTOR('',#87467,1000.);
#27834=VECTOR('',#87474,1000.);
#27835=VECTOR('',#87479,1000.);
#27836=VECTOR('',#87486,1000.);
#27837=VECTOR('',#87491,1000.);
#27838=VECTOR('',#87498,1000.);
#27839=VECTOR('',#87503,1000.);
#27840=VECTOR('',#87510,1000.);
#27841=VECTOR('',#87515,1000.);
#27842=VECTOR('',#87522,1000.);
#27843=VECTOR('',#87527,1000.);
#27844=VECTOR('',#87768,1000.);
#27845=VECTOR('',#87771,1000.);
#27846=VECTOR('',#87780,1000.);
#27847=VECTOR('',#87783,1000.);
#27848=VECTOR('',#87792,1000.);
#27849=VECTOR('',#87795,1000.);
#27850=VECTOR('',#87804,1000.);
#27851=VECTOR('',#87807,1000.);
#27852=VECTOR('',#87816,1000.);
#27853=VECTOR('',#87819,1000.);
#27854=VECTOR('',#87828,1000.);
#27855=VECTOR('',#87831,1000.);
#27856=VECTOR('',#87840,1000.);
#27857=VECTOR('',#87841,1000.);
#27858=VECTOR('',#87842,1000.);
#27859=VECTOR('',#87845,1000.);
#27860=VECTOR('',#87854,1000.);
#27861=VECTOR('',#87857,1000.);
#27862=VECTOR('',#87866,1000.);
#27863=VECTOR('',#87869,1000.);
#27864=VECTOR('',#87878,1000.);
#27865=VECTOR('',#87881,1000.);
#27866=VECTOR('',#87890,1000.);
#27867=VECTOR('',#87893,1000.);
#27868=VECTOR('',#87902,1000.);
#27869=VECTOR('',#87905,1000.);
#27870=VECTOR('',#87914,1000.);
#27871=VECTOR('',#87917,1000.);
#27872=VECTOR('',#87926,1000.);
#27873=VECTOR('',#87929,1000.);
#27874=VECTOR('',#87938,1000.);
#27875=VECTOR('',#87941,1000.);
#27876=VECTOR('',#87950,1000.);
#27877=VECTOR('',#87953,1000.);
#27878=VECTOR('',#87962,1000.);
#27879=VECTOR('',#87965,1000.);
#27880=VECTOR('',#87974,1000.);
#27881=VECTOR('',#87977,1000.);
#27882=VECTOR('',#87980,1000.);
#27883=VECTOR('',#87987,1000.);
#27884=VECTOR('',#87998,1000.);
#27885=VECTOR('',#88001,1000.);
#27886=VECTOR('',#88010,1000.);
#27887=VECTOR('',#88013,1000.);
#27888=VECTOR('',#88022,1000.);
#27889=VECTOR('',#88025,1000.);
#27890=VECTOR('',#88034,1000.);
#27891=VECTOR('',#88037,1000.);
#27892=VECTOR('',#88046,1000.);
#27893=VECTOR('',#88049,1000.);
#27894=VECTOR('',#88058,1000.);
#27895=VECTOR('',#88061,1000.);
#27896=VECTOR('',#88070,1000.);
#27897=VECTOR('',#88073,1000.);
#27898=VECTOR('',#88082,1000.);
#27899=VECTOR('',#88085,1000.);
#27900=VECTOR('',#88094,1000.);
#27901=VECTOR('',#88103,1000.);
#27902=VECTOR('',#88106,1000.);
#27903=VECTOR('',#88107,1000.);
#27904=VECTOR('',#88112,1000.);
#27905=VECTOR('',#88119,1000.);
#27906=VECTOR('',#88124,1000.);
#27907=VECTOR('',#88131,1000.);
#27908=VECTOR('',#88136,1000.);
#27909=VECTOR('',#88143,1000.);
#27910=VECTOR('',#88148,1000.);
#27911=VECTOR('',#88155,1000.);
#27912=VECTOR('',#88160,1000.);
#27913=VECTOR('',#88167,1000.);
#27914=VECTOR('',#88172,1000.);
#27915=VECTOR('',#88179,1000.);
#27916=VECTOR('',#88184,1000.);
#27917=VECTOR('',#88191,1000.);
#27918=VECTOR('',#88196,1000.);
#27919=VECTOR('',#88203,1000.);
#27920=VECTOR('',#88208,1000.);
#27921=VECTOR('',#88215,1000.);
#27922=VECTOR('',#88220,1000.);
#27923=VECTOR('',#88227,1000.);
#27924=VECTOR('',#88232,1000.);
#27925=VECTOR('',#88239,1000.);
#27926=VECTOR('',#88244,1000.);
#27927=VECTOR('',#88251,1000.);
#27928=VECTOR('',#88256,1000.);
#27929=VECTOR('',#88263,1000.);
#27930=VECTOR('',#88264,1000.);
#27931=VECTOR('',#88265,1000.);
#27932=VECTOR('',#88270,1000.);
#27933=VECTOR('',#88277,1000.);
#27934=VECTOR('',#88282,1000.);
#27935=VECTOR('',#88289,1000.);
#27936=VECTOR('',#88294,1000.);
#27937=VECTOR('',#88301,1000.);
#27938=VECTOR('',#88306,1000.);
#27939=VECTOR('',#88313,1000.);
#27940=VECTOR('',#88318,1000.);
#27941=VECTOR('',#88325,1000.);
#27942=VECTOR('',#88330,1000.);
#27943=VECTOR('',#88337,1000.);
#27944=VECTOR('',#88342,1000.);
#27945=VECTOR('',#88349,1000.);
#27946=VECTOR('',#88354,1000.);
#27947=VECTOR('',#88361,1000.);
#27948=VECTOR('',#88366,1000.);
#27949=VECTOR('',#88373,1000.);
#27950=VECTOR('',#88378,1000.);
#27951=VECTOR('',#88385,1000.);
#27952=VECTOR('',#88390,1000.);
#27953=VECTOR('',#88397,1000.);
#27954=VECTOR('',#88402,1000.);
#27955=VECTOR('',#88409,1000.);
#27956=VECTOR('',#88414,1000.);
#27957=VECTOR('',#88421,1000.);
#27958=VECTOR('',#88426,1000.);
#27959=VECTOR('',#88441,1000.);
#27960=VECTOR('',#88618,1000.);
#27961=VECTOR('',#88625,1000.);
#27962=VECTOR('',#88628,1000.);
#27963=VECTOR('',#88635,1000.);
#27964=VECTOR('',#88638,1000.);
#27965=VECTOR('',#88645,1000.);
#27966=VECTOR('',#88648,1000.);
#27967=VECTOR('',#88655,1000.);
#27968=VECTOR('',#88658,1000.);
#27969=VECTOR('',#88665,1000.);
#27970=VECTOR('',#88668,1000.);
#27971=VECTOR('',#88675,1000.);
#27972=VECTOR('',#88678,1000.);
#27973=VECTOR('',#88685,1000.);
#27974=VECTOR('',#88688,1000.);
#27975=VECTOR('',#88695,1000.);
#27976=VECTOR('',#88698,1000.);
#27977=VECTOR('',#88705,1000.);
#27978=VECTOR('',#88708,1000.);
#27979=VECTOR('',#88715,1000.);
#27980=VECTOR('',#88718,1000.);
#27981=VECTOR('',#88725,1000.);
#27982=VECTOR('',#88728,1000.);
#27983=VECTOR('',#88735,1000.);
#27984=VECTOR('',#88738,1000.);
#27985=VECTOR('',#88745,1000.);
#27986=VECTOR('',#88748,1000.);
#27987=VECTOR('',#88755,1000.);
#27988=VECTOR('',#88756,1000.);
#27989=VECTOR('',#88757,1000.);
#27990=VECTOR('',#88760,1000.);
#27991=VECTOR('',#88767,1000.);
#27992=VECTOR('',#88770,1000.);
#27993=VECTOR('',#88777,1000.);
#27994=VECTOR('',#88780,1000.);
#27995=VECTOR('',#88787,1000.);
#27996=VECTOR('',#88790,1000.);
#27997=VECTOR('',#88791,1000.);
#27998=VECTOR('',#88798,1000.);
#27999=VECTOR('',#88807,1000.);
#28000=VECTOR('',#88810,1000.);
#28001=VECTOR('',#88817,1000.);
#28002=VECTOR('',#88820,1000.);
#28003=VECTOR('',#88827,1000.);
#28004=VECTOR('',#88830,1000.);
#28005=VECTOR('',#88837,1000.);
#28006=VECTOR('',#88840,1000.);
#28007=VECTOR('',#88847,1000.);
#28008=VECTOR('',#88850,1000.);
#28009=VECTOR('',#88857,1000.);
#28010=VECTOR('',#88860,1000.);
#28011=VECTOR('',#88867,1000.);
#28012=VECTOR('',#88870,1000.);
#28013=VECTOR('',#88877,1000.);
#28014=VECTOR('',#88880,1000.);
#28015=VECTOR('',#88887,1000.);
#28016=VECTOR('',#88890,1000.);
#28017=VECTOR('',#88897,1000.);
#28018=VECTOR('',#88898,1000.);
#28019=VECTOR('',#88911,1000.);
#28020=VECTOR('',#88918,1000.);
#28021=VECTOR('',#88931,1000.);
#28022=VECTOR('',#88938,1000.);
#28023=VECTOR('',#88951,1000.);
#28024=VECTOR('',#88958,1000.);
#28025=VECTOR('',#88971,1000.);
#28026=VECTOR('',#88978,1000.);
#28027=VECTOR('',#88991,1000.);
#28028=VECTOR('',#88998,1000.);
#28029=VECTOR('',#89011,1000.);
#28030=VECTOR('',#89018,1000.);
#28031=VECTOR('',#89031,1000.);
#28032=VECTOR('',#89038,1000.);
#28033=VECTOR('',#89051,1000.);
#28034=VECTOR('',#89058,1000.);
#28035=VECTOR('',#89071,1000.);
#28036=VECTOR('',#89078,1000.);
#28037=VECTOR('',#89091,1000.);
#28038=VECTOR('',#89098,1000.);
#28039=VECTOR('',#89111,1000.);
#28040=VECTOR('',#89118,1000.);
#28041=VECTOR('',#89131,1000.);
#28042=VECTOR('',#89138,1000.);
#28043=VECTOR('',#89151,1000.);
#28044=VECTOR('',#89158,1000.);
#28045=VECTOR('',#89171,1000.);
#28046=VECTOR('',#89178,1000.);
#28047=VECTOR('',#89191,1000.);
#28048=VECTOR('',#89198,1000.);
#28049=VECTOR('',#89211,1000.);
#28050=VECTOR('',#89218,1000.);
#28051=VECTOR('',#89231,1000.);
#28052=VECTOR('',#89238,1000.);
#28053=VECTOR('',#89251,1000.);
#28054=VECTOR('',#89258,1000.);
#28055=VECTOR('',#89271,1000.);
#28056=VECTOR('',#89278,1000.);
#28057=VECTOR('',#89291,1000.);
#28058=VECTOR('',#89298,1000.);
#28059=VECTOR('',#89311,1000.);
#28060=VECTOR('',#89318,1000.);
#28061=VECTOR('',#89319,1000.);
#28062=VECTOR('',#89320,1000.);
#28063=VECTOR('',#89333,1000.);
#28064=VECTOR('',#89340,1000.);
#28065=VECTOR('',#89353,1000.);
#28066=VECTOR('',#89360,1000.);
#28067=VECTOR('',#89373,1000.);
#28068=VECTOR('',#89380,1000.);
#28069=VECTOR('',#89393,1000.);
#28070=VECTOR('',#89400,1000.);
#28071=VECTOR('',#89413,1000.);
#28072=VECTOR('',#89420,1000.);
#28073=VECTOR('',#89433,1000.);
#28074=VECTOR('',#89440,1000.);
#28075=VECTOR('',#89453,1000.);
#28076=VECTOR('',#89752,1000.);
#28077=VECTOR('',#89755,1000.);
#28078=VECTOR('',#89764,1000.);
#28079=VECTOR('',#89767,1000.);
#28080=VECTOR('',#89776,1000.);
#28081=VECTOR('',#89779,1000.);
#28082=VECTOR('',#89788,1000.);
#28083=VECTOR('',#89791,1000.);
#28084=VECTOR('',#89800,1000.);
#28085=VECTOR('',#89803,1000.);
#28086=VECTOR('',#89812,1000.);
#28087=VECTOR('',#89815,1000.);
#28088=VECTOR('',#89824,1000.);
#28089=VECTOR('',#89825,1000.);
#28090=VECTOR('',#89826,1000.);
#28091=VECTOR('',#89829,1000.);
#28092=VECTOR('',#89838,1000.);
#28093=VECTOR('',#89841,1000.);
#28094=VECTOR('',#89850,1000.);
#28095=VECTOR('',#89853,1000.);
#28096=VECTOR('',#89862,1000.);
#28097=VECTOR('',#89865,1000.);
#28098=VECTOR('',#89874,1000.);
#28099=VECTOR('',#89877,1000.);
#28100=VECTOR('',#89886,1000.);
#28101=VECTOR('',#89889,1000.);
#28102=VECTOR('',#89898,1000.);
#28103=VECTOR('',#89901,1000.);
#28104=VECTOR('',#89910,1000.);
#28105=VECTOR('',#89913,1000.);
#28106=VECTOR('',#89922,1000.);
#28107=VECTOR('',#89925,1000.);
#28108=VECTOR('',#89934,1000.);
#28109=VECTOR('',#89937,1000.);
#28110=VECTOR('',#89946,1000.);
#28111=VECTOR('',#89949,1000.);
#28112=VECTOR('',#89952,1000.);
#28113=VECTOR('',#89959,1000.);
#28114=VECTOR('',#89970,1000.);
#28115=VECTOR('',#89973,1000.);
#28116=VECTOR('',#89982,1000.);
#28117=VECTOR('',#89985,1000.);
#28118=VECTOR('',#89994,1000.);
#28119=VECTOR('',#89997,1000.);
#28120=VECTOR('',#90006,1000.);
#28121=VECTOR('',#90009,1000.);
#28122=VECTOR('',#90018,1000.);
#28123=VECTOR('',#90021,1000.);
#28124=VECTOR('',#90030,1000.);
#28125=VECTOR('',#90033,1000.);
#28126=VECTOR('',#90042,1000.);
#28127=VECTOR('',#90045,1000.);
#28128=VECTOR('',#90054,1000.);
#28129=VECTOR('',#90057,1000.);
#28130=VECTOR('',#90066,1000.);
#28131=VECTOR('',#90069,1000.);
#28132=VECTOR('',#90078,1000.);
#28133=VECTOR('',#90087,1000.);
#28134=VECTOR('',#90088,1000.);
#28135=VECTOR('',#90089,1000.);
#28136=VECTOR('',#90092,1000.);
#28137=VECTOR('',#90093,1000.);
#28138=VECTOR('',#90096,1000.);
#28139=VECTOR('',#90097,1000.);
#28140=VECTOR('',#90100,1000.);
#28141=VECTOR('',#90101,1000.);
#28142=VECTOR('',#90104,1000.);
#28143=VECTOR('',#90105,1000.);
#28144=VECTOR('',#90108,1000.);
#28145=VECTOR('',#90109,1000.);
#28146=VECTOR('',#90112,1000.);
#28147=VECTOR('',#90113,1000.);
#28148=VECTOR('',#90116,1000.);
#28149=VECTOR('',#90117,1000.);
#28150=VECTOR('',#90120,1000.);
#28151=VECTOR('',#90121,1000.);
#28152=VECTOR('',#90124,1000.);
#28153=VECTOR('',#90125,1000.);
#28154=VECTOR('',#90128,1000.);
#28155=VECTOR('',#90129,1000.);
#28156=VECTOR('',#90132,1000.);
#28157=VECTOR('',#90133,1000.);
#28158=VECTOR('',#90136,1000.);
#28159=VECTOR('',#90137,1000.);
#28160=VECTOR('',#90140,1000.);
#28161=VECTOR('',#90141,1000.);
#28162=VECTOR('',#90142,1000.);
#28163=VECTOR('',#90143,1000.);
#28164=VECTOR('',#90146,1000.);
#28165=VECTOR('',#90147,1000.);
#28166=VECTOR('',#90150,1000.);
#28167=VECTOR('',#90151,1000.);
#28168=VECTOR('',#90154,1000.);
#28169=VECTOR('',#90155,1000.);
#28170=VECTOR('',#90158,1000.);
#28171=VECTOR('',#90159,1000.);
#28172=VECTOR('',#90162,1000.);
#28173=VECTOR('',#90163,1000.);
#28174=VECTOR('',#90166,1000.);
#28175=VECTOR('',#90167,1000.);
#28176=VECTOR('',#90168,1000.);
#28177=VECTOR('',#90169,1000.);
#28178=VECTOR('',#90172,1000.);
#28179=VECTOR('',#90173,1000.);
#28180=VECTOR('',#90176,1000.);
#28181=VECTOR('',#90177,1000.);
#28182=VECTOR('',#90180,1000.);
#28183=VECTOR('',#90181,1000.);
#28184=VECTOR('',#90184,1000.);
#28185=VECTOR('',#90185,1000.);
#28186=VECTOR('',#90188,1000.);
#28187=VECTOR('',#90189,1000.);
#28188=VECTOR('',#90192,1000.);
#28189=VECTOR('',#90193,1000.);
#28190=VECTOR('',#90196,1000.);
#28191=VECTOR('',#90199,1000.);
#28192=VECTOR('',#90434,1000.);
#28193=VECTOR('',#90443,1000.);
#28194=VECTOR('',#90446,1000.);
#28195=VECTOR('',#90455,1000.);
#28196=VECTOR('',#90458,1000.);
#28197=VECTOR('',#90467,1000.);
#28198=VECTOR('',#90470,1000.);
#28199=VECTOR('',#90479,1000.);
#28200=VECTOR('',#90482,1000.);
#28201=VECTOR('',#90491,1000.);
#28202=VECTOR('',#90494,1000.);
#28203=VECTOR('',#90503,1000.);
#28204=VECTOR('',#90506,1000.);
#28205=VECTOR('',#90515,1000.);
#28206=VECTOR('',#90518,1000.);
#28207=VECTOR('',#90527,1000.);
#28208=VECTOR('',#90530,1000.);
#28209=VECTOR('',#90539,1000.);
#28210=VECTOR('',#90542,1000.);
#28211=VECTOR('',#90551,1000.);
#28212=VECTOR('',#90554,1000.);
#28213=VECTOR('',#90563,1000.);
#28214=VECTOR('',#90566,1000.);
#28215=VECTOR('',#90575,1000.);
#28216=VECTOR('',#90578,1000.);
#28217=VECTOR('',#90587,1000.);
#28218=VECTOR('',#90590,1000.);
#28219=VECTOR('',#90599,1000.);
#28220=VECTOR('',#90600,1000.);
#28221=VECTOR('',#90601,1000.);
#28222=VECTOR('',#90604,1000.);
#28223=VECTOR('',#90613,1000.);
#28224=VECTOR('',#90616,1000.);
#28225=VECTOR('',#90625,1000.);
#28226=VECTOR('',#90628,1000.);
#28227=VECTOR('',#90631,1000.);
#28228=VECTOR('',#90638,1000.);
#28229=VECTOR('',#90649,1000.);
#28230=VECTOR('',#90652,1000.);
#28231=VECTOR('',#90661,1000.);
#28232=VECTOR('',#90664,1000.);
#28233=VECTOR('',#90673,1000.);
#28234=VECTOR('',#90676,1000.);
#28235=VECTOR('',#90685,1000.);
#28236=VECTOR('',#90688,1000.);
#28237=VECTOR('',#90697,1000.);
#28238=VECTOR('',#90700,1000.);
#28239=VECTOR('',#90709,1000.);
#28240=VECTOR('',#90712,1000.);
#28241=VECTOR('',#90721,1000.);
#28242=VECTOR('',#90724,1000.);
#28243=VECTOR('',#90733,1000.);
#28244=VECTOR('',#90736,1000.);
#28245=VECTOR('',#90745,1000.);
#28246=VECTOR('',#90748,1000.);
#28247=VECTOR('',#90757,1000.);
#28248=VECTOR('',#90760,1000.);
#28249=VECTOR('',#90769,1000.);
#28250=VECTOR('',#90772,1000.);
#28251=VECTOR('',#90773,1000.);
#28252=VECTOR('',#90774,1000.);
#28253=VECTOR('',#90777,1000.);
#28254=VECTOR('',#90778,1000.);
#28255=VECTOR('',#90781,1000.);
#28256=VECTOR('',#90782,1000.);
#28257=VECTOR('',#90785,1000.);
#28258=VECTOR('',#90786,1000.);
#28259=VECTOR('',#90789,1000.);
#28260=VECTOR('',#90790,1000.);
#28261=VECTOR('',#90793,1000.);
#28262=VECTOR('',#90794,1000.);
#28263=VECTOR('',#90797,1000.);
#28264=VECTOR('',#90798,1000.);
#28265=VECTOR('',#90801,1000.);
#28266=VECTOR('',#90802,1000.);
#28267=VECTOR('',#90805,1000.);
#28268=VECTOR('',#90806,1000.);
#28269=VECTOR('',#90809,1000.);
#28270=VECTOR('',#90810,1000.);
#28271=VECTOR('',#90813,1000.);
#28272=VECTOR('',#90814,1000.);
#28273=VECTOR('',#90817,1000.);
#28274=VECTOR('',#90818,1000.);
#28275=VECTOR('',#90821,1000.);
#28276=VECTOR('',#90822,1000.);
#28277=VECTOR('',#90825,1000.);
#28278=VECTOR('',#90826,1000.);
#28279=VECTOR('',#90829,1000.);
#28280=VECTOR('',#90830,1000.);
#28281=VECTOR('',#90833,1000.);
#28282=VECTOR('',#90834,1000.);
#28283=VECTOR('',#90837,1000.);
#28284=VECTOR('',#90838,1000.);
#28285=VECTOR('',#90841,1000.);
#28286=VECTOR('',#90842,1000.);
#28287=VECTOR('',#90845,1000.);
#28288=VECTOR('',#90846,1000.);
#28289=VECTOR('',#90849,1000.);
#28290=VECTOR('',#90850,1000.);
#28291=VECTOR('',#90853,1000.);
#28292=VECTOR('',#90854,1000.);
#28293=VECTOR('',#90857,1000.);
#28294=VECTOR('',#90858,1000.);
#28295=VECTOR('',#90861,1000.);
#28296=VECTOR('',#90862,1000.);
#28297=VECTOR('',#90865,1000.);
#28298=VECTOR('',#90866,1000.);
#28299=VECTOR('',#90869,1000.);
#28300=VECTOR('',#90870,1000.);
#28301=VECTOR('',#90873,1000.);
#28302=VECTOR('',#90874,1000.);
#28303=VECTOR('',#90877,1000.);
#28304=VECTOR('',#90878,1000.);
#28305=VECTOR('',#90881,1000.);
#28306=VECTOR('',#90882,1000.);
#28307=VECTOR('',#90885,1000.);
#28308=VECTOR('',#91004,1000.);
#28309=VECTOR('',#91007,1000.);
#28310=VECTOR('',#91018,1000.);
#28311=VECTOR('',#91027,1000.);
#28312=VECTOR('',#91038,1000.);
#28313=VECTOR('',#91047,1000.);
#28314=VECTOR('',#91058,1000.);
#28315=VECTOR('',#91067,1000.);
#28316=VECTOR('',#91078,1000.);
#28317=VECTOR('',#91087,1000.);
#28318=VECTOR('',#91098,1000.);
#28319=VECTOR('',#91107,1000.);
#28320=VECTOR('',#91118,1000.);
#28321=VECTOR('',#91125,1000.);
#28322=VECTOR('',#91132,1000.);
#28323=VECTOR('',#91135,1000.);
#28324=VECTOR('',#91146,1000.);
#28325=VECTOR('',#91155,1000.);
#28326=VECTOR('',#91166,1000.);
#28327=VECTOR('',#91175,1000.);
#28328=VECTOR('',#91186,1000.);
#28329=VECTOR('',#91195,1000.);
#28330=VECTOR('',#91206,1000.);
#28331=VECTOR('',#91215,1000.);
#28332=VECTOR('',#91226,1000.);
#28333=VECTOR('',#91235,1000.);
#28334=VECTOR('',#91246,1000.);
#28335=VECTOR('',#91255,1000.);
#28336=VECTOR('',#91266,1000.);
#28337=VECTOR('',#91275,1000.);
#28338=VECTOR('',#91286,1000.);
#28339=VECTOR('',#91295,1000.);
#28340=VECTOR('',#91306,1000.);
#28341=VECTOR('',#91315,1000.);
#28342=VECTOR('',#91326,1000.);
#28343=VECTOR('',#91333,1000.);
#28344=VECTOR('',#91346,1000.);
#28345=VECTOR('',#91355,1000.);
#28346=VECTOR('',#91366,1000.);
#28347=VECTOR('',#91375,1000.);
#28348=VECTOR('',#91386,1000.);
#28349=VECTOR('',#91395,1000.);
#28350=VECTOR('',#91406,1000.);
#28351=VECTOR('',#91415,1000.);
#28352=VECTOR('',#91426,1000.);
#28353=VECTOR('',#91435,1000.);
#28354=VECTOR('',#91446,1000.);
#28355=VECTOR('',#91455,1000.);
#28356=VECTOR('',#91466,1000.);
#28357=VECTOR('',#91475,1000.);
#28358=VECTOR('',#91486,1000.);
#28359=VECTOR('',#91495,1000.);
#28360=VECTOR('',#91506,1000.);
#28361=VECTOR('',#91515,1000.);
#28362=VECTOR('',#91526,1000.);
#28363=VECTOR('',#91535,1000.);
#28364=VECTOR('',#91546,1000.);
#28365=VECTOR('',#91569,1000.);
#28366=VECTOR('',#91746,1000.);
#28367=VECTOR('',#91749,1000.);
#28368=VECTOR('',#91750,1000.);
#28369=VECTOR('',#91753,1000.);
#28370=VECTOR('',#91754,1000.);
#28371=VECTOR('',#91757,1000.);
#28372=VECTOR('',#91758,1000.);
#28373=VECTOR('',#91761,1000.);
#28374=VECTOR('',#91762,1000.);
#28375=VECTOR('',#91765,1000.);
#28376=VECTOR('',#91766,1000.);
#28377=VECTOR('',#91769,1000.);
#28378=VECTOR('',#91770,1000.);
#28379=VECTOR('',#91773,1000.);
#28380=VECTOR('',#91774,1000.);
#28381=VECTOR('',#91777,1000.);
#28382=VECTOR('',#91778,1000.);
#28383=VECTOR('',#91781,1000.);
#28384=VECTOR('',#91782,1000.);
#28385=VECTOR('',#91785,1000.);
#28386=VECTOR('',#91786,1000.);
#28387=VECTOR('',#91789,1000.);
#28388=VECTOR('',#91790,1000.);
#28389=VECTOR('',#91793,1000.);
#28390=VECTOR('',#91794,1000.);
#28391=VECTOR('',#91797,1000.);
#28392=VECTOR('',#91798,1000.);
#28393=VECTOR('',#91801,1000.);
#28394=VECTOR('',#91802,1000.);
#28395=VECTOR('',#91805,1000.);
#28396=VECTOR('',#91806,1000.);
#28397=VECTOR('',#91809,1000.);
#28398=VECTOR('',#91810,1000.);
#28399=VECTOR('',#91813,1000.);
#28400=VECTOR('',#91814,1000.);
#28401=VECTOR('',#91817,1000.);
#28402=VECTOR('',#91818,1000.);
#28403=VECTOR('',#91821,1000.);
#28404=VECTOR('',#91822,1000.);
#28405=VECTOR('',#91825,1000.);
#28406=VECTOR('',#91826,1000.);
#28407=VECTOR('',#91829,1000.);
#28408=VECTOR('',#91830,1000.);
#28409=VECTOR('',#91831,1000.);
#28410=VECTOR('',#91832,1000.);
#28411=VECTOR('',#91835,1000.);
#28412=VECTOR('',#91836,1000.);
#28413=VECTOR('',#91839,1000.);
#28414=VECTOR('',#91840,1000.);
#28415=VECTOR('',#91843,1000.);
#28416=VECTOR('',#91844,1000.);
#28417=VECTOR('',#91847,1000.);
#28418=VECTOR('',#91848,1000.);
#28419=VECTOR('',#91851,1000.);
#28420=VECTOR('',#91852,1000.);
#28421=VECTOR('',#91855,1000.);
#28422=VECTOR('',#91856,1000.);
#28423=VECTOR('',#91857,1000.);
#28424=VECTOR('',#92020,1000.);
#28425=VECTOR('',#92023,1000.);
#28426=VECTOR('',#92024,1000.);
#28427=VECTOR('',#92027,1000.);
#28428=VECTOR('',#92028,1000.);
#28429=VECTOR('',#92031,1000.);
#28430=VECTOR('',#92032,1000.);
#28431=VECTOR('',#92035,1000.);
#28432=VECTOR('',#92036,1000.);
#28433=VECTOR('',#92039,1000.);
#28434=VECTOR('',#92040,1000.);
#28435=VECTOR('',#92043,1000.);
#28436=VECTOR('',#92044,1000.);
#28437=VECTOR('',#92047,1000.);
#28438=VECTOR('',#92048,1000.);
#28439=VECTOR('',#92051,1000.);
#28440=VECTOR('',#92052,1000.);
#28441=VECTOR('',#92055,1000.);
#28442=VECTOR('',#92056,1000.);
#28443=VECTOR('',#92059,1000.);
#28444=VECTOR('',#92060,1000.);
#28445=VECTOR('',#92063,1000.);
#28446=VECTOR('',#92064,1000.);
#28447=VECTOR('',#92067,1000.);
#28448=VECTOR('',#92068,1000.);
#28449=VECTOR('',#92071,1000.);
#28450=VECTOR('',#92072,1000.);
#28451=VECTOR('',#92075,1000.);
#28452=VECTOR('',#92076,1000.);
#28453=VECTOR('',#92079,1000.);
#28454=VECTOR('',#92080,1000.);
#28455=VECTOR('',#92083,1000.);
#28456=VECTOR('',#92084,1000.);
#28457=VECTOR('',#92087,1000.);
#28458=VECTOR('',#92088,1000.);
#28459=VECTOR('',#92091,1000.);
#28460=VECTOR('',#92092,1000.);
#28461=VECTOR('',#92095,1000.);
#28462=VECTOR('',#92096,1000.);
#28463=VECTOR('',#92099,1000.);
#28464=VECTOR('',#92100,1000.);
#28465=VECTOR('',#92103,1000.);
#28466=VECTOR('',#92104,1000.);
#28467=VECTOR('',#92107,1000.);
#28468=VECTOR('',#92108,1000.);
#28469=VECTOR('',#92111,1000.);
#28470=VECTOR('',#92112,1000.);
#28471=VECTOR('',#92115,1000.);
#28472=VECTOR('',#92116,1000.);
#28473=VECTOR('',#92119,1000.);
#28474=VECTOR('',#92120,1000.);
#28475=VECTOR('',#92123,1000.);
#28476=VECTOR('',#92124,1000.);
#28477=VECTOR('',#92127,1000.);
#28478=VECTOR('',#92128,1000.);
#28479=VECTOR('',#92131,1000.);
#28480=VECTOR('',#92132,1000.);
#28481=VECTOR('',#92135,1000.);
#28533=VERTEX_POINT('',#92438);
#28534=VERTEX_POINT('',#92439);
#28535=VERTEX_POINT('',#92441);
#28536=VERTEX_POINT('',#92448);
#28537=VERTEX_POINT('',#92459);
#28538=VERTEX_POINT('',#92461);
#28539=VERTEX_POINT('',#92463);
#28540=VERTEX_POINT('',#92470);
#28541=VERTEX_POINT('',#92481);
#28542=VERTEX_POINT('',#92488);
#28543=VERTEX_POINT('',#92499);
#28544=VERTEX_POINT('',#92501);
#28545=VERTEX_POINT('',#92503);
#28546=VERTEX_POINT('',#92510);
#28547=VERTEX_POINT('',#92521);
#28548=VERTEX_POINT('',#92528);
#28549=VERTEX_POINT('',#92539);
#28550=VERTEX_POINT('',#92541);
#28551=VERTEX_POINT('',#92543);
#28552=VERTEX_POINT('',#92550);
#28553=VERTEX_POINT('',#92561);
#28554=VERTEX_POINT('',#92568);
#28555=VERTEX_POINT('',#92579);
#28556=VERTEX_POINT('',#92581);
#28557=VERTEX_POINT('',#92583);
#28558=VERTEX_POINT('',#92590);
#28559=VERTEX_POINT('',#92601);
#28560=VERTEX_POINT('',#92608);
#28561=VERTEX_POINT('',#92619);
#28562=VERTEX_POINT('',#92621);
#28563=VERTEX_POINT('',#92623);
#28564=VERTEX_POINT('',#92630);
#28565=VERTEX_POINT('',#92641);
#28566=VERTEX_POINT('',#92648);
#28567=VERTEX_POINT('',#92659);
#28568=VERTEX_POINT('',#92661);
#28569=VERTEX_POINT('',#92663);
#28570=VERTEX_POINT('',#92670);
#28571=VERTEX_POINT('',#92681);
#28572=VERTEX_POINT('',#92688);
#28573=VERTEX_POINT('',#92699);
#28574=VERTEX_POINT('',#92701);
#28575=VERTEX_POINT('',#92703);
#28576=VERTEX_POINT('',#92710);
#28577=VERTEX_POINT('',#92721);
#28578=VERTEX_POINT('',#92728);
#28579=VERTEX_POINT('',#92739);
#28580=VERTEX_POINT('',#92741);
#28581=VERTEX_POINT('',#92743);
#28582=VERTEX_POINT('',#92750);
#28583=VERTEX_POINT('',#92761);
#28584=VERTEX_POINT('',#92768);
#28585=VERTEX_POINT('',#92779);
#28586=VERTEX_POINT('',#92781);
#28587=VERTEX_POINT('',#92783);
#28588=VERTEX_POINT('',#92790);
#28589=VERTEX_POINT('',#92801);
#28590=VERTEX_POINT('',#92808);
#28591=VERTEX_POINT('',#92819);
#28592=VERTEX_POINT('',#92821);
#28593=VERTEX_POINT('',#92823);
#28594=VERTEX_POINT('',#92830);
#28595=VERTEX_POINT('',#92841);
#28596=VERTEX_POINT('',#92848);
#28597=VERTEX_POINT('',#92859);
#28598=VERTEX_POINT('',#92861);
#28599=VERTEX_POINT('',#92863);
#28600=VERTEX_POINT('',#92870);
#28601=VERTEX_POINT('',#92881);
#28602=VERTEX_POINT('',#92888);
#28603=VERTEX_POINT('',#92899);
#28604=VERTEX_POINT('',#92901);
#28605=VERTEX_POINT('',#92903);
#28606=VERTEX_POINT('',#92910);
#28607=VERTEX_POINT('',#92921);
#28608=VERTEX_POINT('',#92928);
#28609=VERTEX_POINT('',#92939);
#28610=VERTEX_POINT('',#92941);
#28611=VERTEX_POINT('',#92943);
#28612=VERTEX_POINT('',#92950);
#28613=VERTEX_POINT('',#92961);
#28614=VERTEX_POINT('',#92968);
#28615=VERTEX_POINT('',#92979);
#28616=VERTEX_POINT('',#92981);
#28617=VERTEX_POINT('',#92983);
#28618=VERTEX_POINT('',#92990);
#28619=VERTEX_POINT('',#93001);
#28620=VERTEX_POINT('',#93008);
#28621=VERTEX_POINT('',#93019);
#28622=VERTEX_POINT('',#93021);
#28623=VERTEX_POINT('',#93023);
#28624=VERTEX_POINT('',#93030);
#28625=VERTEX_POINT('',#93041);
#28626=VERTEX_POINT('',#93048);
#28627=VERTEX_POINT('',#93059);
#28628=VERTEX_POINT('',#93061);
#28629=VERTEX_POINT('',#93063);
#28630=VERTEX_POINT('',#93070);
#28631=VERTEX_POINT('',#93081);
#28632=VERTEX_POINT('',#93088);
#28633=VERTEX_POINT('',#93099);
#28634=VERTEX_POINT('',#93101);
#28635=VERTEX_POINT('',#93103);
#28636=VERTEX_POINT('',#93110);
#28637=VERTEX_POINT('',#93121);
#28638=VERTEX_POINT('',#93128);
#28639=VERTEX_POINT('',#93139);
#28640=VERTEX_POINT('',#93141);
#28641=VERTEX_POINT('',#93143);
#28642=VERTEX_POINT('',#93150);
#28643=VERTEX_POINT('',#93161);
#28644=VERTEX_POINT('',#93168);
#28645=VERTEX_POINT('',#93179);
#28646=VERTEX_POINT('',#93181);
#28647=VERTEX_POINT('',#93183);
#28648=VERTEX_POINT('',#93190);
#28649=VERTEX_POINT('',#93201);
#28650=VERTEX_POINT('',#93208);
#28651=VERTEX_POINT('',#93219);
#28652=VERTEX_POINT('',#93221);
#28653=VERTEX_POINT('',#93223);
#28654=VERTEX_POINT('',#93230);
#28655=VERTEX_POINT('',#93241);
#28656=VERTEX_POINT('',#93248);
#28657=VERTEX_POINT('',#93259);
#28658=VERTEX_POINT('',#93261);
#28659=VERTEX_POINT('',#93263);
#28660=VERTEX_POINT('',#93270);
#28661=VERTEX_POINT('',#93281);
#28662=VERTEX_POINT('',#93288);
#28663=VERTEX_POINT('',#93299);
#28664=VERTEX_POINT('',#93301);
#28665=VERTEX_POINT('',#93303);
#28666=VERTEX_POINT('',#93310);
#28667=VERTEX_POINT('',#93321);
#28668=VERTEX_POINT('',#93328);
#28669=VERTEX_POINT('',#93339);
#28670=VERTEX_POINT('',#93341);
#28671=VERTEX_POINT('',#93343);
#28672=VERTEX_POINT('',#93350);
#28673=VERTEX_POINT('',#93361);
#28674=VERTEX_POINT('',#93368);
#28675=VERTEX_POINT('',#93379);
#28676=VERTEX_POINT('',#93381);
#28677=VERTEX_POINT('',#93383);
#28678=VERTEX_POINT('',#93390);
#28679=VERTEX_POINT('',#93401);
#28680=VERTEX_POINT('',#93408);
#28681=VERTEX_POINT('',#93419);
#28682=VERTEX_POINT('',#93421);
#28683=VERTEX_POINT('',#93423);
#28684=VERTEX_POINT('',#93430);
#28685=VERTEX_POINT('',#93441);
#28686=VERTEX_POINT('',#93448);
#28687=VERTEX_POINT('',#93459);
#28688=VERTEX_POINT('',#93461);
#28689=VERTEX_POINT('',#93463);
#28690=VERTEX_POINT('',#93470);
#28691=VERTEX_POINT('',#93481);
#28692=VERTEX_POINT('',#93488);
#28693=VERTEX_POINT('',#93499);
#28694=VERTEX_POINT('',#93501);
#28695=VERTEX_POINT('',#93503);
#28696=VERTEX_POINT('',#93510);
#28697=VERTEX_POINT('',#93521);
#28698=VERTEX_POINT('',#93528);
#28699=VERTEX_POINT('',#93539);
#28700=VERTEX_POINT('',#93541);
#28701=VERTEX_POINT('',#93543);
#28702=VERTEX_POINT('',#93550);
#28703=VERTEX_POINT('',#93561);
#28704=VERTEX_POINT('',#93568);
#28705=VERTEX_POINT('',#93579);
#28706=VERTEX_POINT('',#93581);
#28707=VERTEX_POINT('',#93583);
#28708=VERTEX_POINT('',#93590);
#28709=VERTEX_POINT('',#93593);
#28710=VERTEX_POINT('',#93605);
#28711=VERTEX_POINT('',#93607);
#28712=VERTEX_POINT('',#93611);
#28713=VERTEX_POINT('',#93623);
#28714=VERTEX_POINT('',#93625);
#28715=VERTEX_POINT('',#93629);
#28716=VERTEX_POINT('',#93630);
#28717=VERTEX_POINT('',#93632);
#28718=VERTEX_POINT('',#93637);
#28719=VERTEX_POINT('',#93641);
#28720=VERTEX_POINT('',#93642);
#28721=VERTEX_POINT('',#93649);
#28722=VERTEX_POINT('',#93651);
#28723=VERTEX_POINT('',#93653);
#28724=VERTEX_POINT('',#93664);
#28725=VERTEX_POINT('',#93671);
#28726=VERTEX_POINT('',#93678);
#28727=VERTEX_POINT('',#93685);
#28728=VERTEX_POINT('',#93687);
#28729=VERTEX_POINT('',#93689);
#28730=VERTEX_POINT('',#93700);
#28731=VERTEX_POINT('',#93707);
#28732=VERTEX_POINT('',#93714);
#28733=VERTEX_POINT('',#93721);
#28734=VERTEX_POINT('',#93723);
#28735=VERTEX_POINT('',#93725);
#28736=VERTEX_POINT('',#93736);
#28737=VERTEX_POINT('',#93743);
#28738=VERTEX_POINT('',#93750);
#28739=VERTEX_POINT('',#93757);
#28740=VERTEX_POINT('',#93759);
#28741=VERTEX_POINT('',#93761);
#28742=VERTEX_POINT('',#93772);
#28743=VERTEX_POINT('',#93779);
#28744=VERTEX_POINT('',#93786);
#28745=VERTEX_POINT('',#93793);
#28746=VERTEX_POINT('',#93795);
#28747=VERTEX_POINT('',#93797);
#28748=VERTEX_POINT('',#93808);
#28749=VERTEX_POINT('',#93815);
#28750=VERTEX_POINT('',#93822);
#28751=VERTEX_POINT('',#93829);
#28752=VERTEX_POINT('',#93831);
#28753=VERTEX_POINT('',#93833);
#28754=VERTEX_POINT('',#93844);
#28755=VERTEX_POINT('',#93851);
#28756=VERTEX_POINT('',#93858);
#28757=VERTEX_POINT('',#93865);
#28758=VERTEX_POINT('',#93867);
#28759=VERTEX_POINT('',#93869);
#28760=VERTEX_POINT('',#93880);
#28761=VERTEX_POINT('',#93887);
#28762=VERTEX_POINT('',#93894);
#28763=VERTEX_POINT('',#93901);
#28764=VERTEX_POINT('',#93903);
#28765=VERTEX_POINT('',#93905);
#28766=VERTEX_POINT('',#93916);
#28767=VERTEX_POINT('',#93923);
#28768=VERTEX_POINT('',#93930);
#28769=VERTEX_POINT('',#93937);
#28770=VERTEX_POINT('',#93939);
#28771=VERTEX_POINT('',#93941);
#28772=VERTEX_POINT('',#93952);
#28773=VERTEX_POINT('',#93959);
#28774=VERTEX_POINT('',#93966);
#28775=VERTEX_POINT('',#93973);
#28776=VERTEX_POINT('',#93975);
#28777=VERTEX_POINT('',#93977);
#28778=VERTEX_POINT('',#93988);
#28779=VERTEX_POINT('',#93995);
#28780=VERTEX_POINT('',#94002);
#28781=VERTEX_POINT('',#94009);
#28782=VERTEX_POINT('',#94011);
#28783=VERTEX_POINT('',#94013);
#28784=VERTEX_POINT('',#94024);
#28785=VERTEX_POINT('',#94031);
#28786=VERTEX_POINT('',#94038);
#28787=VERTEX_POINT('',#94045);
#28788=VERTEX_POINT('',#94047);
#28789=VERTEX_POINT('',#94049);
#28790=VERTEX_POINT('',#94060);
#28791=VERTEX_POINT('',#94067);
#28792=VERTEX_POINT('',#94074);
#28793=VERTEX_POINT('',#94081);
#28794=VERTEX_POINT('',#94083);
#28795=VERTEX_POINT('',#94085);
#28796=VERTEX_POINT('',#94096);
#28797=VERTEX_POINT('',#94103);
#28798=VERTEX_POINT('',#94110);
#28799=VERTEX_POINT('',#94117);
#28800=VERTEX_POINT('',#94119);
#28801=VERTEX_POINT('',#94121);
#28802=VERTEX_POINT('',#94132);
#28803=VERTEX_POINT('',#94139);
#28804=VERTEX_POINT('',#94146);
#28805=VERTEX_POINT('',#94153);
#28806=VERTEX_POINT('',#94155);
#28807=VERTEX_POINT('',#94157);
#28808=VERTEX_POINT('',#94168);
#28809=VERTEX_POINT('',#94171);
#28810=VERTEX_POINT('',#94176);
#28811=VERTEX_POINT('',#94183);
#28812=VERTEX_POINT('',#94190);
#28813=VERTEX_POINT('',#94197);
#28814=VERTEX_POINT('',#94199);
#28815=VERTEX_POINT('',#94201);
#28816=VERTEX_POINT('',#94212);
#28817=VERTEX_POINT('',#94219);
#28818=VERTEX_POINT('',#94226);
#28819=VERTEX_POINT('',#94233);
#28820=VERTEX_POINT('',#94235);
#28821=VERTEX_POINT('',#94237);
#28822=VERTEX_POINT('',#94248);
#28823=VERTEX_POINT('',#94255);
#28824=VERTEX_POINT('',#94262);
#28825=VERTEX_POINT('',#94269);
#28826=VERTEX_POINT('',#94271);
#28827=VERTEX_POINT('',#94273);
#28828=VERTEX_POINT('',#94284);
#28829=VERTEX_POINT('',#94291);
#28830=VERTEX_POINT('',#94298);
#28831=VERTEX_POINT('',#94305);
#28832=VERTEX_POINT('',#94307);
#28833=VERTEX_POINT('',#94309);
#28834=VERTEX_POINT('',#94320);
#28835=VERTEX_POINT('',#94327);
#28836=VERTEX_POINT('',#94334);
#28837=VERTEX_POINT('',#94341);
#28838=VERTEX_POINT('',#94343);
#28839=VERTEX_POINT('',#94345);
#28840=VERTEX_POINT('',#94356);
#28841=VERTEX_POINT('',#94363);
#28842=VERTEX_POINT('',#94370);
#28843=VERTEX_POINT('',#94377);
#28844=VERTEX_POINT('',#94379);
#28845=VERTEX_POINT('',#94381);
#28846=VERTEX_POINT('',#94392);
#28847=VERTEX_POINT('',#94399);
#28848=VERTEX_POINT('',#94406);
#28849=VERTEX_POINT('',#94413);
#28850=VERTEX_POINT('',#94415);
#28851=VERTEX_POINT('',#94417);
#28852=VERTEX_POINT('',#94428);
#28853=VERTEX_POINT('',#94435);
#28854=VERTEX_POINT('',#94442);
#28855=VERTEX_POINT('',#94449);
#28856=VERTEX_POINT('',#94451);
#28857=VERTEX_POINT('',#94453);
#28858=VERTEX_POINT('',#94464);
#28859=VERTEX_POINT('',#94471);
#28860=VERTEX_POINT('',#94478);
#28861=VERTEX_POINT('',#94485);
#28862=VERTEX_POINT('',#94487);
#28863=VERTEX_POINT('',#94489);
#28864=VERTEX_POINT('',#94500);
#28865=VERTEX_POINT('',#94507);
#28866=VERTEX_POINT('',#94514);
#28867=VERTEX_POINT('',#94521);
#28868=VERTEX_POINT('',#94523);
#28869=VERTEX_POINT('',#94525);
#28870=VERTEX_POINT('',#94536);
#28871=VERTEX_POINT('',#94543);
#28872=VERTEX_POINT('',#94550);
#28873=VERTEX_POINT('',#94557);
#28874=VERTEX_POINT('',#94559);
#28875=VERTEX_POINT('',#94561);
#28876=VERTEX_POINT('',#94572);
#28877=VERTEX_POINT('',#94579);
#28878=VERTEX_POINT('',#94586);
#28879=VERTEX_POINT('',#94593);
#28880=VERTEX_POINT('',#94595);
#28881=VERTEX_POINT('',#94597);
#28882=VERTEX_POINT('',#94608);
#28883=VERTEX_POINT('',#94615);
#28884=VERTEX_POINT('',#94622);
#28885=VERTEX_POINT('',#94629);
#28886=VERTEX_POINT('',#94631);
#28887=VERTEX_POINT('',#94633);
#28888=VERTEX_POINT('',#94644);
#28889=VERTEX_POINT('',#94651);
#28890=VERTEX_POINT('',#94658);
#28891=VERTEX_POINT('',#94665);
#28892=VERTEX_POINT('',#94667);
#28893=VERTEX_POINT('',#94669);
#28894=VERTEX_POINT('',#94680);
#28895=VERTEX_POINT('',#94694);
#28896=VERTEX_POINT('',#94695);
#28897=VERTEX_POINT('',#94697);
#28898=VERTEX_POINT('',#94699);
#28899=VERTEX_POINT('',#94715);
#28900=VERTEX_POINT('',#94716);
#28901=VERTEX_POINT('',#94725);
#28902=VERTEX_POINT('',#94727);
#28903=VERTEX_POINT('',#94743);
#28904=VERTEX_POINT('',#94744);
#28905=VERTEX_POINT('',#94757);
#28906=VERTEX_POINT('',#94759);
#28907=VERTEX_POINT('',#94761);
#28908=VERTEX_POINT('',#94765);
#28909=VERTEX_POINT('',#94766);
#28910=VERTEX_POINT('',#94773);
#28911=VERTEX_POINT('',#94780);
#28912=VERTEX_POINT('',#94784);
#28913=VERTEX_POINT('',#94785);
#28914=VERTEX_POINT('',#94794);
#28915=VERTEX_POINT('',#94796);
#28916=VERTEX_POINT('',#94812);
#28917=VERTEX_POINT('',#94813);
#28918=VERTEX_POINT('',#94822);
#28919=VERTEX_POINT('',#94824);
#28920=VERTEX_POINT('',#94840);
#28921=VERTEX_POINT('',#94841);
#28922=VERTEX_POINT('',#94848);
#28923=VERTEX_POINT('',#94850);
#28924=VERTEX_POINT('',#94859);
#28925=VERTEX_POINT('',#94860);
#28926=VERTEX_POINT('',#94862);
#28927=VERTEX_POINT('',#94864);
#28928=VERTEX_POINT('',#94866);
#28929=VERTEX_POINT('',#94881);
#28930=VERTEX_POINT('',#94890);
#28931=VERTEX_POINT('',#94891);
#28932=VERTEX_POINT('',#94904);
#28933=VERTEX_POINT('',#94917);
#28934=VERTEX_POINT('',#94927);
#28935=VERTEX_POINT('',#94928);
#28936=VERTEX_POINT('',#94935);
#28937=VERTEX_POINT('',#94942);
#28938=VERTEX_POINT('',#94946);
#28939=VERTEX_POINT('',#94947);
#28940=VERTEX_POINT('',#94954);
#28941=VERTEX_POINT('',#94956);
#28942=VERTEX_POINT('',#94971);
#28943=VERTEX_POINT('',#94972);
#28944=VERTEX_POINT('',#94979);
#28945=VERTEX_POINT('',#94981);
#28946=VERTEX_POINT('',#94990);
#28947=VERTEX_POINT('',#94991);
#28948=VERTEX_POINT('',#94998);
#28949=VERTEX_POINT('',#95005);
#28950=VERTEX_POINT('',#95009);
#28951=VERTEX_POINT('',#95010);
#28952=VERTEX_POINT('',#95017);
#28953=VERTEX_POINT('',#95024);
#28954=VERTEX_POINT('',#95034);
#28955=VERTEX_POINT('',#95035);
#28956=VERTEX_POINT('',#95048);
#28957=VERTEX_POINT('',#95056);
#28958=VERTEX_POINT('',#95071);
#28959=VERTEX_POINT('',#95072);
#28960=VERTEX_POINT('',#95079);
#28961=VERTEX_POINT('',#95086);
#28962=VERTEX_POINT('',#95096);
#28963=VERTEX_POINT('',#95097);
#28964=VERTEX_POINT('',#95104);
#28965=VERTEX_POINT('',#95111);
#28966=VERTEX_POINT('',#95115);
#28967=VERTEX_POINT('',#95116);
#28968=VERTEX_POINT('',#95129);
#28969=VERTEX_POINT('',#95131);
#28970=VERTEX_POINT('',#95140);
#28971=VERTEX_POINT('',#95141);
#28972=VERTEX_POINT('',#95154);
#28973=VERTEX_POINT('',#95156);
#28974=VERTEX_POINT('',#95177);
#28975=VERTEX_POINT('',#95178);
#28976=VERTEX_POINT('',#95191);
#28977=VERTEX_POINT('',#95204);
#28978=VERTEX_POINT('',#95208);
#28979=VERTEX_POINT('',#95209);
#28980=VERTEX_POINT('',#95216);
#28981=VERTEX_POINT('',#95223);
#28982=VERTEX_POINT('',#95233);
#28983=VERTEX_POINT('',#95234);
#28984=VERTEX_POINT('',#95241);
#28985=VERTEX_POINT('',#95249);
#28986=VERTEX_POINT('',#95258);
#28987=VERTEX_POINT('',#95259);
#28988=VERTEX_POINT('',#95266);
#28989=VERTEX_POINT('',#95268);
#28990=VERTEX_POINT('',#95283);
#28991=VERTEX_POINT('',#95284);
#28992=VERTEX_POINT('',#95297);
#28993=VERTEX_POINT('',#95304);
#28994=VERTEX_POINT('',#95314);
#28995=VERTEX_POINT('',#95315);
#28996=VERTEX_POINT('',#95328);
#28997=VERTEX_POINT('',#95341);
#28998=VERTEX_POINT('',#95345);
#28999=VERTEX_POINT('',#95346);
#29000=VERTEX_POINT('',#95359);
#29001=VERTEX_POINT('',#95361);
#29002=VERTEX_POINT('',#95379);
#29003=VERTEX_POINT('',#95380);
#29004=VERTEX_POINT('',#95393);
#29005=VERTEX_POINT('',#95406);
#29006=VERTEX_POINT('',#95410);
#29007=VERTEX_POINT('',#95411);
#29008=VERTEX_POINT('',#95418);
#29009=VERTEX_POINT('',#95431);
#29010=VERTEX_POINT('',#95441);
#29011=VERTEX_POINT('',#95442);
#29012=VERTEX_POINT('',#95449);
#29013=VERTEX_POINT('',#95457);
#29014=VERTEX_POINT('',#95466);
#29015=VERTEX_POINT('',#95467);
#29016=VERTEX_POINT('',#95474);
#29017=VERTEX_POINT('',#95480);
#29018=VERTEX_POINT('',#95495);
#29019=VERTEX_POINT('',#95496);
#29020=VERTEX_POINT('',#95503);
#29021=VERTEX_POINT('',#95510);
#29022=VERTEX_POINT('',#95526);
#29023=VERTEX_POINT('',#95527);
#29024=VERTEX_POINT('',#95540);
#29025=VERTEX_POINT('',#95553);
#29026=VERTEX_POINT('',#95557);
#29027=VERTEX_POINT('',#95558);
#29028=VERTEX_POINT('',#95565);
#29029=VERTEX_POINT('',#95567);
#29030=VERTEX_POINT('',#95587);
#29031=VERTEX_POINT('',#95588);
#29032=VERTEX_POINT('',#95590);
#29033=VERTEX_POINT('',#95592);
#29034=VERTEX_POINT('',#95615);
#29035=VERTEX_POINT('',#95616);
#29036=VERTEX_POINT('',#95618);
#29037=VERTEX_POINT('',#95628);
#29038=VERTEX_POINT('',#95636);
#29039=VERTEX_POINT('',#95645);
#29040=VERTEX_POINT('',#95663);
#29041=VERTEX_POINT('',#95664);
#29042=VERTEX_POINT('',#95666);
#29043=VERTEX_POINT('',#95676);
#29044=VERTEX_POINT('',#95684);
#29045=VERTEX_POINT('',#95693);
#29046=VERTEX_POINT('',#95711);
#29047=VERTEX_POINT('',#95712);
#29048=VERTEX_POINT('',#95714);
#29049=VERTEX_POINT('',#95724);
#29050=VERTEX_POINT('',#95732);
#29051=VERTEX_POINT('',#95741);
#29052=VERTEX_POINT('',#95759);
#29053=VERTEX_POINT('',#95760);
#29054=VERTEX_POINT('',#95762);
#29055=VERTEX_POINT('',#95772);
#29056=VERTEX_POINT('',#95780);
#29057=VERTEX_POINT('',#95789);
#29058=VERTEX_POINT('',#95807);
#29059=VERTEX_POINT('',#95808);
#29060=VERTEX_POINT('',#95810);
#29061=VERTEX_POINT('',#95820);
#29062=VERTEX_POINT('',#95828);
#29063=VERTEX_POINT('',#95837);
#29064=VERTEX_POINT('',#95855);
#29065=VERTEX_POINT('',#95856);
#29066=VERTEX_POINT('',#95858);
#29067=VERTEX_POINT('',#95868);
#29068=VERTEX_POINT('',#95876);
#29069=VERTEX_POINT('',#95885);
#29070=VERTEX_POINT('',#95903);
#29071=VERTEX_POINT('',#95918);
#29072=VERTEX_POINT('',#95936);
#29073=VERTEX_POINT('',#95937);
#29074=VERTEX_POINT('',#95939);
#29075=VERTEX_POINT('',#95949);
#29076=VERTEX_POINT('',#95957);
#29077=VERTEX_POINT('',#95966);
#29078=VERTEX_POINT('',#95984);
#29079=VERTEX_POINT('',#95985);
#29080=VERTEX_POINT('',#95987);
#29081=VERTEX_POINT('',#95997);
#29082=VERTEX_POINT('',#96005);
#29083=VERTEX_POINT('',#96014);
#29084=VERTEX_POINT('',#96032);
#29085=VERTEX_POINT('',#96033);
#29086=VERTEX_POINT('',#96035);
#29087=VERTEX_POINT('',#96045);
#29088=VERTEX_POINT('',#96053);
#29089=VERTEX_POINT('',#96062);
#29090=VERTEX_POINT('',#96080);
#29091=VERTEX_POINT('',#96081);
#29092=VERTEX_POINT('',#96083);
#29093=VERTEX_POINT('',#96093);
#29094=VERTEX_POINT('',#96101);
#29095=VERTEX_POINT('',#96110);
#29096=VERTEX_POINT('',#96128);
#29097=VERTEX_POINT('',#96129);
#29098=VERTEX_POINT('',#96131);
#29099=VERTEX_POINT('',#96141);
#29100=VERTEX_POINT('',#96149);
#29101=VERTEX_POINT('',#96158);
#29102=VERTEX_POINT('',#96176);
#29103=VERTEX_POINT('',#96177);
#29104=VERTEX_POINT('',#96179);
#29105=VERTEX_POINT('',#96189);
#29106=VERTEX_POINT('',#96197);
#29107=VERTEX_POINT('',#96206);
#29108=VERTEX_POINT('',#96224);
#29109=VERTEX_POINT('',#96225);
#29110=VERTEX_POINT('',#96227);
#29111=VERTEX_POINT('',#96237);
#29112=VERTEX_POINT('',#96245);
#29113=VERTEX_POINT('',#96254);
#29114=VERTEX_POINT('',#96272);
#29115=VERTEX_POINT('',#96273);
#29116=VERTEX_POINT('',#96275);
#29117=VERTEX_POINT('',#96285);
#29118=VERTEX_POINT('',#96293);
#29119=VERTEX_POINT('',#96302);
#29120=VERTEX_POINT('',#96320);
#29121=VERTEX_POINT('',#96321);
#29122=VERTEX_POINT('',#96323);
#29123=VERTEX_POINT('',#96333);
#29124=VERTEX_POINT('',#96341);
#29125=VERTEX_POINT('',#96350);
#29126=VERTEX_POINT('',#96368);
#29127=VERTEX_POINT('',#96369);
#29128=VERTEX_POINT('',#96371);
#29129=VERTEX_POINT('',#96381);
#29130=VERTEX_POINT('',#96389);
#29131=VERTEX_POINT('',#96398);
#29132=VERTEX_POINT('',#96416);
#29133=VERTEX_POINT('',#96417);
#29134=VERTEX_POINT('',#96419);
#29135=VERTEX_POINT('',#96429);
#29136=VERTEX_POINT('',#96437);
#29137=VERTEX_POINT('',#96446);
#29138=VERTEX_POINT('',#96464);
#29139=VERTEX_POINT('',#96465);
#29140=VERTEX_POINT('',#96467);
#29141=VERTEX_POINT('',#96477);
#29142=VERTEX_POINT('',#96485);
#29143=VERTEX_POINT('',#96494);
#29144=VERTEX_POINT('',#96512);
#29145=VERTEX_POINT('',#96513);
#29146=VERTEX_POINT('',#96515);
#29147=VERTEX_POINT('',#96525);
#29148=VERTEX_POINT('',#96533);
#29149=VERTEX_POINT('',#96542);
#29150=VERTEX_POINT('',#96560);
#29151=VERTEX_POINT('',#96561);
#29152=VERTEX_POINT('',#96563);
#29153=VERTEX_POINT('',#96573);
#29154=VERTEX_POINT('',#96581);
#29155=VERTEX_POINT('',#96590);
#29156=VERTEX_POINT('',#96608);
#29157=VERTEX_POINT('',#96609);
#29158=VERTEX_POINT('',#96611);
#29159=VERTEX_POINT('',#96621);
#29160=VERTEX_POINT('',#96629);
#29161=VERTEX_POINT('',#96638);
#29162=VERTEX_POINT('',#96656);
#29163=VERTEX_POINT('',#96657);
#29164=VERTEX_POINT('',#96659);
#29165=VERTEX_POINT('',#96669);
#29166=VERTEX_POINT('',#96677);
#29167=VERTEX_POINT('',#96686);
#29168=VERTEX_POINT('',#96704);
#29169=VERTEX_POINT('',#96705);
#29170=VERTEX_POINT('',#96707);
#29171=VERTEX_POINT('',#96717);
#29172=VERTEX_POINT('',#96725);
#29173=VERTEX_POINT('',#96734);
#29174=VERTEX_POINT('',#96752);
#29175=VERTEX_POINT('',#96753);
#29176=VERTEX_POINT('',#96755);
#29177=VERTEX_POINT('',#96770);
#29178=VERTEX_POINT('',#96772);
#29179=VERTEX_POINT('',#96776);
#29180=VERTEX_POINT('',#96800);
#29181=VERTEX_POINT('',#96801);
#29182=VERTEX_POINT('',#96803);
#29183=VERTEX_POINT('',#96813);
#29184=VERTEX_POINT('',#96815);
#29185=VERTEX_POINT('',#96830);
#29186=VERTEX_POINT('',#96848);
#29187=VERTEX_POINT('',#96849);
#29188=VERTEX_POINT('',#96851);
#29189=VERTEX_POINT('',#96861);
#29190=VERTEX_POINT('',#96869);
#29191=VERTEX_POINT('',#96878);
#29192=VERTEX_POINT('',#96896);
#29193=VERTEX_POINT('',#96897);
#29194=VERTEX_POINT('',#96899);
#29195=VERTEX_POINT('',#96909);
#29196=VERTEX_POINT('',#96917);
#29197=VERTEX_POINT('',#96926);
#29198=VERTEX_POINT('',#96930);
#29199=VERTEX_POINT('',#96931);
#29200=VERTEX_POINT('',#96968);
#29201=VERTEX_POINT('',#96975);
#29202=VERTEX_POINT('',#96987);
#29203=VERTEX_POINT('',#96989);
#29204=VERTEX_POINT('',#97007);
#29205=VERTEX_POINT('',#97011);
#29206=VERTEX_POINT('',#97023);
#29207=VERTEX_POINT('',#97025);
#29208=VERTEX_POINT('',#97043);
#29209=VERTEX_POINT('',#97047);
#29210=VERTEX_POINT('',#97059);
#29211=VERTEX_POINT('',#97061);
#29212=VERTEX_POINT('',#97079);
#29213=VERTEX_POINT('',#97083);
#29214=VERTEX_POINT('',#97095);
#29215=VERTEX_POINT('',#97097);
#29216=VERTEX_POINT('',#97115);
#29217=VERTEX_POINT('',#97119);
#29218=VERTEX_POINT('',#97131);
#29219=VERTEX_POINT('',#97133);
#29220=VERTEX_POINT('',#97151);
#29221=VERTEX_POINT('',#97155);
#29222=VERTEX_POINT('',#97167);
#29223=VERTEX_POINT('',#97169);
#29224=VERTEX_POINT('',#97187);
#29225=VERTEX_POINT('',#97191);
#29226=VERTEX_POINT('',#97203);
#29227=VERTEX_POINT('',#97205);
#29228=VERTEX_POINT('',#97223);
#29229=VERTEX_POINT('',#97227);
#29230=VERTEX_POINT('',#97239);
#29231=VERTEX_POINT('',#97241);
#29232=VERTEX_POINT('',#97259);
#29233=VERTEX_POINT('',#97263);
#29234=VERTEX_POINT('',#97275);
#29235=VERTEX_POINT('',#97277);
#29236=VERTEX_POINT('',#97295);
#29237=VERTEX_POINT('',#97299);
#29238=VERTEX_POINT('',#97311);
#29239=VERTEX_POINT('',#97313);
#29240=VERTEX_POINT('',#97331);
#29241=VERTEX_POINT('',#97335);
#29242=VERTEX_POINT('',#97347);
#29243=VERTEX_POINT('',#97349);
#29244=VERTEX_POINT('',#97367);
#29245=VERTEX_POINT('',#97371);
#29246=VERTEX_POINT('',#97383);
#29247=VERTEX_POINT('',#97385);
#29248=VERTEX_POINT('',#97403);
#29249=VERTEX_POINT('',#97407);
#29250=VERTEX_POINT('',#97419);
#29251=VERTEX_POINT('',#97421);
#29252=VERTEX_POINT('',#97439);
#29253=VERTEX_POINT('',#97443);
#29254=VERTEX_POINT('',#97482);
#29255=VERTEX_POINT('',#97484);
#29256=VERTEX_POINT('',#97502);
#29257=VERTEX_POINT('',#97506);
#29258=VERTEX_POINT('',#97518);
#29259=VERTEX_POINT('',#97520);
#29260=VERTEX_POINT('',#97538);
#29261=VERTEX_POINT('',#97542);
#29262=VERTEX_POINT('',#97554);
#29263=VERTEX_POINT('',#97556);
#29264=VERTEX_POINT('',#97574);
#29265=VERTEX_POINT('',#97578);
#29266=VERTEX_POINT('',#97590);
#29267=VERTEX_POINT('',#97592);
#29268=VERTEX_POINT('',#97610);
#29269=VERTEX_POINT('',#97614);
#29270=VERTEX_POINT('',#97626);
#29271=VERTEX_POINT('',#97628);
#29272=VERTEX_POINT('',#97646);
#29273=VERTEX_POINT('',#97650);
#29274=VERTEX_POINT('',#97662);
#29275=VERTEX_POINT('',#97664);
#29276=VERTEX_POINT('',#97682);
#29277=VERTEX_POINT('',#97686);
#29278=VERTEX_POINT('',#97698);
#29279=VERTEX_POINT('',#97700);
#29280=VERTEX_POINT('',#97718);
#29281=VERTEX_POINT('',#97722);
#29282=VERTEX_POINT('',#97734);
#29283=VERTEX_POINT('',#97736);
#29284=VERTEX_POINT('',#97754);
#29285=VERTEX_POINT('',#97758);
#29286=VERTEX_POINT('',#97770);
#29287=VERTEX_POINT('',#97772);
#29288=VERTEX_POINT('',#97790);
#29289=VERTEX_POINT('',#97794);
#29290=VERTEX_POINT('',#97806);
#29291=VERTEX_POINT('',#97808);
#29292=VERTEX_POINT('',#97826);
#29293=VERTEX_POINT('',#97830);
#29294=VERTEX_POINT('',#97842);
#29295=VERTEX_POINT('',#97844);
#29296=VERTEX_POINT('',#97862);
#29297=VERTEX_POINT('',#97866);
#29298=VERTEX_POINT('',#97878);
#29299=VERTEX_POINT('',#97880);
#29300=VERTEX_POINT('',#97898);
#29301=VERTEX_POINT('',#97902);
#29302=VERTEX_POINT('',#97914);
#29303=VERTEX_POINT('',#97916);
#29304=VERTEX_POINT('',#97934);
#29305=VERTEX_POINT('',#97938);
#29306=VERTEX_POINT('',#97950);
#29307=VERTEX_POINT('',#97952);
#29308=VERTEX_POINT('',#97970);
#29309=VERTEX_POINT('',#97974);
#29310=VERTEX_POINT('',#97978);
#29311=VERTEX_POINT('',#97980);
#29312=VERTEX_POINT('',#97999);
#29313=VERTEX_POINT('',#98021);
#29314=VERTEX_POINT('',#98054);
#29315=VERTEX_POINT('',#98087);
#29316=VERTEX_POINT('',#98120);
#29317=VERTEX_POINT('',#98153);
#29318=VERTEX_POINT('',#98186);
#29319=VERTEX_POINT('',#98219);
#29320=VERTEX_POINT('',#98252);
#29321=VERTEX_POINT('',#98287);
#29322=VERTEX_POINT('',#98320);
#29323=VERTEX_POINT('',#98353);
#29324=VERTEX_POINT('',#98386);
#29325=VERTEX_POINT('',#98419);
#29326=VERTEX_POINT('',#98454);
#29327=VERTEX_POINT('',#98489);
#29328=VERTEX_POINT('',#98522);
#29329=VERTEX_POINT('',#98555);
#29330=VERTEX_POINT('',#98590);
#29331=VERTEX_POINT('',#98623);
#29332=VERTEX_POINT('',#98656);
#29333=VERTEX_POINT('',#98689);
#29334=VERTEX_POINT('',#98722);
#29335=VERTEX_POINT('',#98755);
#29336=VERTEX_POINT('',#98790);
#29337=VERTEX_POINT('',#98825);
#29338=VERTEX_POINT('',#98860);
#29339=VERTEX_POINT('',#98893);
#29340=VERTEX_POINT('',#98926);
#29341=VERTEX_POINT('',#98976);
#29342=VERTEX_POINT('',#98990);
#29343=VERTEX_POINT('',#99015);
#29344=VERTEX_POINT('',#99040);
#29345=VERTEX_POINT('',#99065);
#29346=VERTEX_POINT('',#99090);
#29347=VERTEX_POINT('',#99115);
#29348=VERTEX_POINT('',#99140);
#29349=VERTEX_POINT('',#99165);
#29350=VERTEX_POINT('',#99190);
#29351=VERTEX_POINT('',#99215);
#29352=VERTEX_POINT('',#99240);
#29353=VERTEX_POINT('',#99265);
#29354=VERTEX_POINT('',#99290);
#29355=VERTEX_POINT('',#99315);
#29356=VERTEX_POINT('',#99340);
#29357=VERTEX_POINT('',#99365);
#29358=VERTEX_POINT('',#99390);
#29359=VERTEX_POINT('',#99415);
#29360=VERTEX_POINT('',#99440);
#29361=VERTEX_POINT('',#99465);
#29362=VERTEX_POINT('',#99490);
#29363=VERTEX_POINT('',#99515);
#29364=VERTEX_POINT('',#99540);
#29365=VERTEX_POINT('',#99565);
#29366=VERTEX_POINT('',#99590);
#29367=VERTEX_POINT('',#99615);
#29368=VERTEX_POINT('',#99640);
#29369=VERTEX_POINT('',#99665);
#29370=VERTEX_POINT('',#99697);
#29371=VERTEX_POINT('',#99698);
#29372=VERTEX_POINT('',#99708);
#29373=VERTEX_POINT('',#99710);
#29374=VERTEX_POINT('',#99746);
#29375=VERTEX_POINT('',#99747);
#29376=VERTEX_POINT('',#99757);
#29377=VERTEX_POINT('',#99759);
#29378=VERTEX_POINT('',#99795);
#29379=VERTEX_POINT('',#99796);
#29380=VERTEX_POINT('',#99806);
#29381=VERTEX_POINT('',#99808);
#29382=VERTEX_POINT('',#99844);
#29383=VERTEX_POINT('',#99845);
#29384=VERTEX_POINT('',#99855);
#29385=VERTEX_POINT('',#99857);
#29386=VERTEX_POINT('',#99893);
#29387=VERTEX_POINT('',#99894);
#29388=VERTEX_POINT('',#99904);
#29389=VERTEX_POINT('',#99906);
#29390=VERTEX_POINT('',#99942);
#29391=VERTEX_POINT('',#99943);
#29392=VERTEX_POINT('',#99953);
#29393=VERTEX_POINT('',#99955);
#29394=VERTEX_POINT('',#99991);
#29395=VERTEX_POINT('',#99992);
#29396=VERTEX_POINT('',#100002);
#29397=VERTEX_POINT('',#100004);
#29398=VERTEX_POINT('',#100040);
#29399=VERTEX_POINT('',#100041);
#29400=VERTEX_POINT('',#100051);
#29401=VERTEX_POINT('',#100053);
#29402=VERTEX_POINT('',#100089);
#29403=VERTEX_POINT('',#100090);
#29404=VERTEX_POINT('',#100100);
#29405=VERTEX_POINT('',#100102);
#29406=VERTEX_POINT('',#100138);
#29407=VERTEX_POINT('',#100139);
#29408=VERTEX_POINT('',#100149);
#29409=VERTEX_POINT('',#100151);
#29410=VERTEX_POINT('',#100187);
#29411=VERTEX_POINT('',#100188);
#29412=VERTEX_POINT('',#100198);
#29413=VERTEX_POINT('',#100200);
#29414=VERTEX_POINT('',#100236);
#29415=VERTEX_POINT('',#100237);
#29416=VERTEX_POINT('',#100247);
#29417=VERTEX_POINT('',#100249);
#29418=VERTEX_POINT('',#100285);
#29419=VERTEX_POINT('',#100286);
#29420=VERTEX_POINT('',#100296);
#29421=VERTEX_POINT('',#100298);
#29422=VERTEX_POINT('',#100334);
#29423=VERTEX_POINT('',#100335);
#29424=VERTEX_POINT('',#100345);
#29425=VERTEX_POINT('',#100347);
#29426=VERTEX_POINT('',#100411);
#29427=VERTEX_POINT('',#100412);
#29428=VERTEX_POINT('',#100422);
#29429=VERTEX_POINT('',#100424);
#29430=VERTEX_POINT('',#100460);
#29431=VERTEX_POINT('',#100461);
#29432=VERTEX_POINT('',#100471);
#29433=VERTEX_POINT('',#100473);
#29434=VERTEX_POINT('',#100509);
#29435=VERTEX_POINT('',#100510);
#29436=VERTEX_POINT('',#100520);
#29437=VERTEX_POINT('',#100522);
#29438=VERTEX_POINT('',#100558);
#29439=VERTEX_POINT('',#100559);
#29440=VERTEX_POINT('',#100569);
#29441=VERTEX_POINT('',#100571);
#29442=VERTEX_POINT('',#100607);
#29443=VERTEX_POINT('',#100608);
#29444=VERTEX_POINT('',#100618);
#29445=VERTEX_POINT('',#100620);
#29446=VERTEX_POINT('',#100656);
#29447=VERTEX_POINT('',#100657);
#29448=VERTEX_POINT('',#100667);
#29449=VERTEX_POINT('',#100669);
#29450=VERTEX_POINT('',#100705);
#29451=VERTEX_POINT('',#100706);
#29452=VERTEX_POINT('',#100716);
#29453=VERTEX_POINT('',#100718);
#29454=VERTEX_POINT('',#100754);
#29455=VERTEX_POINT('',#100755);
#29456=VERTEX_POINT('',#100765);
#29457=VERTEX_POINT('',#100767);
#29458=VERTEX_POINT('',#100803);
#29459=VERTEX_POINT('',#100804);
#29460=VERTEX_POINT('',#100814);
#29461=VERTEX_POINT('',#100816);
#29462=VERTEX_POINT('',#100852);
#29463=VERTEX_POINT('',#100853);
#29464=VERTEX_POINT('',#100876);
#29465=VERTEX_POINT('',#100886);
#29466=VERTEX_POINT('',#100901);
#29467=VERTEX_POINT('',#100903);
#29468=VERTEX_POINT('',#100912);
#29469=VERTEX_POINT('',#100920);
#29470=VERTEX_POINT('',#100950);
#29471=VERTEX_POINT('',#100951);
#29472=VERTEX_POINT('',#100961);
#29473=VERTEX_POINT('',#100963);
#29474=VERTEX_POINT('',#100999);
#29475=VERTEX_POINT('',#101000);
#29476=VERTEX_POINT('',#101010);
#29477=VERTEX_POINT('',#101012);
#29478=VERTEX_POINT('',#101048);
#29479=VERTEX_POINT('',#101049);
#29480=VERTEX_POINT('',#101059);
#29481=VERTEX_POINT('',#101061);
#29482=VERTEX_POINT('',#101101);
#29483=VERTEX_POINT('',#101103);
#29484=VERTEX_POINT('',#101121);
#29485=VERTEX_POINT('',#101125);
#29486=VERTEX_POINT('',#101142);
#29487=VERTEX_POINT('',#101144);
#29488=VERTEX_POINT('',#101162);
#29489=VERTEX_POINT('',#101166);
#29490=VERTEX_POINT('',#101183);
#29491=VERTEX_POINT('',#101185);
#29492=VERTEX_POINT('',#101203);
#29493=VERTEX_POINT('',#101207);
#29494=VERTEX_POINT('',#101224);
#29495=VERTEX_POINT('',#101226);
#29496=VERTEX_POINT('',#101244);
#29497=VERTEX_POINT('',#101248);
#29498=VERTEX_POINT('',#101265);
#29499=VERTEX_POINT('',#101267);
#29500=VERTEX_POINT('',#101285);
#29501=VERTEX_POINT('',#101289);
#29502=VERTEX_POINT('',#101306);
#29503=VERTEX_POINT('',#101308);
#29504=VERTEX_POINT('',#101326);
#29505=VERTEX_POINT('',#101330);
#29506=VERTEX_POINT('',#101347);
#29507=VERTEX_POINT('',#101349);
#29508=VERTEX_POINT('',#101367);
#29509=VERTEX_POINT('',#101371);
#29510=VERTEX_POINT('',#101388);
#29511=VERTEX_POINT('',#101390);
#29512=VERTEX_POINT('',#101408);
#29513=VERTEX_POINT('',#101412);
#29514=VERTEX_POINT('',#101429);
#29515=VERTEX_POINT('',#101431);
#29516=VERTEX_POINT('',#101449);
#29517=VERTEX_POINT('',#101453);
#29518=VERTEX_POINT('',#101470);
#29519=VERTEX_POINT('',#101472);
#29520=VERTEX_POINT('',#101490);
#29521=VERTEX_POINT('',#101494);
#29522=VERTEX_POINT('',#101511);
#29523=VERTEX_POINT('',#101513);
#29524=VERTEX_POINT('',#101531);
#29525=VERTEX_POINT('',#101535);
#29526=VERTEX_POINT('',#101552);
#29527=VERTEX_POINT('',#101554);
#29528=VERTEX_POINT('',#101572);
#29529=VERTEX_POINT('',#101576);
#29530=VERTEX_POINT('',#101593);
#29531=VERTEX_POINT('',#101595);
#29532=VERTEX_POINT('',#101613);
#29533=VERTEX_POINT('',#101617);
#29534=VERTEX_POINT('',#101634);
#29535=VERTEX_POINT('',#101636);
#29536=VERTEX_POINT('',#101654);
#29537=VERTEX_POINT('',#101658);
#29538=VERTEX_POINT('',#101675);
#29539=VERTEX_POINT('',#101677);
#29540=VERTEX_POINT('',#101695);
#29541=VERTEX_POINT('',#101699);
#29542=VERTEX_POINT('',#101716);
#29543=VERTEX_POINT('',#101718);
#29544=VERTEX_POINT('',#101736);
#29545=VERTEX_POINT('',#101740);
#29546=VERTEX_POINT('',#101757);
#29547=VERTEX_POINT('',#101759);
#29548=VERTEX_POINT('',#101777);
#29549=VERTEX_POINT('',#101781);
#29550=VERTEX_POINT('',#101798);
#29551=VERTEX_POINT('',#101800);
#29552=VERTEX_POINT('',#101818);
#29553=VERTEX_POINT('',#101822);
#29554=VERTEX_POINT('',#101839);
#29555=VERTEX_POINT('',#101841);
#29556=VERTEX_POINT('',#101859);
#29557=VERTEX_POINT('',#101863);
#29558=VERTEX_POINT('',#101880);
#29559=VERTEX_POINT('',#101882);
#29560=VERTEX_POINT('',#101900);
#29561=VERTEX_POINT('',#101904);
#29562=VERTEX_POINT('',#101921);
#29563=VERTEX_POINT('',#101923);
#29564=VERTEX_POINT('',#101941);
#29565=VERTEX_POINT('',#101945);
#29566=VERTEX_POINT('',#101990);
#29567=VERTEX_POINT('',#101992);
#29568=VERTEX_POINT('',#102010);
#29569=VERTEX_POINT('',#102014);
#29570=VERTEX_POINT('',#102031);
#29571=VERTEX_POINT('',#102033);
#29572=VERTEX_POINT('',#102051);
#29573=VERTEX_POINT('',#102055);
#29574=VERTEX_POINT('',#102072);
#29575=VERTEX_POINT('',#102074);
#29576=VERTEX_POINT('',#102092);
#29577=VERTEX_POINT('',#102096);
#29578=VERTEX_POINT('',#102113);
#29579=VERTEX_POINT('',#102115);
#29580=VERTEX_POINT('',#102133);
#29581=VERTEX_POINT('',#102137);
#29582=VERTEX_POINT('',#102154);
#29583=VERTEX_POINT('',#102156);
#29584=VERTEX_POINT('',#102174);
#29585=VERTEX_POINT('',#102178);
#29586=VERTEX_POINT('',#102195);
#29587=VERTEX_POINT('',#102197);
#29588=VERTEX_POINT('',#102215);
#29589=VERTEX_POINT('',#102219);
#29590=VERTEX_POINT('',#102236);
#29591=VERTEX_POINT('',#102238);
#29592=VERTEX_POINT('',#102256);
#29593=VERTEX_POINT('',#102260);
#29594=VERTEX_POINT('',#102273);
#29595=VERTEX_POINT('',#102308);
#29596=VERTEX_POINT('',#102343);
#29597=VERTEX_POINT('',#102378);
#29598=VERTEX_POINT('',#102413);
#29599=VERTEX_POINT('',#102448);
#29600=VERTEX_POINT('',#102483);
#29601=VERTEX_POINT('',#102518);
#29602=VERTEX_POINT('',#102553);
#29603=VERTEX_POINT('',#102588);
#29604=VERTEX_POINT('',#102623);
#29605=VERTEX_POINT('',#102658);
#29606=VERTEX_POINT('',#102693);
#29607=VERTEX_POINT('',#102728);
#29608=VERTEX_POINT('',#102763);
#29609=VERTEX_POINT('',#102798);
#29610=VERTEX_POINT('',#102833);
#29611=VERTEX_POINT('',#102868);
#29612=VERTEX_POINT('',#102903);
#29613=VERTEX_POINT('',#102938);
#29614=VERTEX_POINT('',#102973);
#29615=VERTEX_POINT('',#103008);
#29616=VERTEX_POINT('',#103043);
#29617=VERTEX_POINT('',#103078);
#29618=VERTEX_POINT('',#103113);
#29619=VERTEX_POINT('',#103148);
#29620=VERTEX_POINT('',#103183);
#29621=VERTEX_POINT('',#103218);
#29622=VERTEX_POINT('',#103253);
#29623=VERTEX_POINT('',#103288);
#29624=VERTEX_POINT('',#103319);
#29625=VERTEX_POINT('',#103350);
#29626=VERTEX_POINT('',#103381);
#29627=VERTEX_POINT('',#103412);
#29628=VERTEX_POINT('',#103443);
#29629=VERTEX_POINT('',#103474);
#29630=VERTEX_POINT('',#103505);
#29631=VERTEX_POINT('',#103536);
#29632=VERTEX_POINT('',#103567);
#29633=VERTEX_POINT('',#103598);
#29634=VERTEX_POINT('',#103629);
#29635=VERTEX_POINT('',#103660);
#29636=VERTEX_POINT('',#103691);
#29637=VERTEX_POINT('',#103722);
#29638=VERTEX_POINT('',#103753);
#29639=VERTEX_POINT('',#103784);
#29640=VERTEX_POINT('',#103815);
#29641=VERTEX_POINT('',#103846);
#29642=VERTEX_POINT('',#103877);
#29643=VERTEX_POINT('',#103908);
#29644=VERTEX_POINT('',#103939);
#29645=VERTEX_POINT('',#103970);
#29646=VERTEX_POINT('',#104001);
#29647=VERTEX_POINT('',#104032);
#29648=VERTEX_POINT('',#104063);
#29649=VERTEX_POINT('',#104094);
#29650=VERTEX_POINT('',#104125);
#29651=VERTEX_POINT('',#104156);
#29652=VERTEX_POINT('',#104187);
#29653=VERTEX_POINT('',#104188);
#29654=VERTEX_POINT('',#104211);
#29655=VERTEX_POINT('',#104212);
#29656=VERTEX_POINT('',#104228);
#29657=VERTEX_POINT('',#104230);
#29658=VERTEX_POINT('',#104254);
#29659=VERTEX_POINT('',#104255);
#29660=VERTEX_POINT('',#104271);
#29661=VERTEX_POINT('',#104273);
#29662=VERTEX_POINT('',#104297);
#29663=VERTEX_POINT('',#104298);
#29664=VERTEX_POINT('',#104314);
#29665=VERTEX_POINT('',#104316);
#29666=VERTEX_POINT('',#104340);
#29667=VERTEX_POINT('',#104341);
#29668=VERTEX_POINT('',#104357);
#29669=VERTEX_POINT('',#104359);
#29670=VERTEX_POINT('',#104383);
#29671=VERTEX_POINT('',#104384);
#29672=VERTEX_POINT('',#104400);
#29673=VERTEX_POINT('',#104402);
#29674=VERTEX_POINT('',#104426);
#29675=VERTEX_POINT('',#104427);
#29676=VERTEX_POINT('',#104443);
#29677=VERTEX_POINT('',#104445);
#29678=VERTEX_POINT('',#104497);
#29679=VERTEX_POINT('',#104498);
#29680=VERTEX_POINT('',#104514);
#29681=VERTEX_POINT('',#104516);
#29682=VERTEX_POINT('',#104540);
#29683=VERTEX_POINT('',#104541);
#29684=VERTEX_POINT('',#104557);
#29685=VERTEX_POINT('',#104559);
#29686=VERTEX_POINT('',#104583);
#29687=VERTEX_POINT('',#104584);
#29688=VERTEX_POINT('',#104600);
#29689=VERTEX_POINT('',#104602);
#29690=VERTEX_POINT('',#104626);
#29691=VERTEX_POINT('',#104627);
#29692=VERTEX_POINT('',#104643);
#29693=VERTEX_POINT('',#104645);
#29694=VERTEX_POINT('',#104669);
#29695=VERTEX_POINT('',#104670);
#29696=VERTEX_POINT('',#104686);
#29697=VERTEX_POINT('',#104688);
#29698=VERTEX_POINT('',#104712);
#29699=VERTEX_POINT('',#104713);
#29700=VERTEX_POINT('',#104729);
#29701=VERTEX_POINT('',#104731);
#29702=VERTEX_POINT('',#104755);
#29703=VERTEX_POINT('',#104756);
#29704=VERTEX_POINT('',#104772);
#29705=VERTEX_POINT('',#104774);
#29706=VERTEX_POINT('',#104798);
#29707=VERTEX_POINT('',#104799);
#29708=VERTEX_POINT('',#104815);
#29709=VERTEX_POINT('',#104817);
#29710=VERTEX_POINT('',#104841);
#29711=VERTEX_POINT('',#104842);
#29712=VERTEX_POINT('',#104858);
#29713=VERTEX_POINT('',#104860);
#29714=VERTEX_POINT('',#104884);
#29715=VERTEX_POINT('',#104885);
#29716=VERTEX_POINT('',#104901);
#29717=VERTEX_POINT('',#104903);
#29718=VERTEX_POINT('',#104927);
#29719=VERTEX_POINT('',#104928);
#29720=VERTEX_POINT('',#104944);
#29721=VERTEX_POINT('',#104946);
#29722=VERTEX_POINT('',#104970);
#29723=VERTEX_POINT('',#104971);
#29724=VERTEX_POINT('',#104987);
#29725=VERTEX_POINT('',#104989);
#29726=VERTEX_POINT('',#105013);
#29727=VERTEX_POINT('',#105014);
#29728=VERTEX_POINT('',#105030);
#29729=VERTEX_POINT('',#105032);
#29730=VERTEX_POINT('',#105056);
#29731=VERTEX_POINT('',#105057);
#29732=VERTEX_POINT('',#105073);
#29733=VERTEX_POINT('',#105075);
#29734=VERTEX_POINT('',#105099);
#29735=VERTEX_POINT('',#105100);
#29736=VERTEX_POINT('',#105116);
#29737=VERTEX_POINT('',#105118);
#29738=VERTEX_POINT('',#105142);
#29739=VERTEX_POINT('',#105143);
#29740=VERTEX_POINT('',#105159);
#29741=VERTEX_POINT('',#105161);
#29742=VERTEX_POINT('',#105185);
#29743=VERTEX_POINT('',#105186);
#29744=VERTEX_POINT('',#105207);
#29745=VERTEX_POINT('',#105211);
#29746=VERTEX_POINT('',#105228);
#29747=VERTEX_POINT('',#105230);
#29748=VERTEX_POINT('',#105245);
#29749=VERTEX_POINT('',#105247);
#29750=VERTEX_POINT('',#105271);
#29751=VERTEX_POINT('',#105272);
#29752=VERTEX_POINT('',#105288);
#29753=VERTEX_POINT('',#105290);
#29754=VERTEX_POINT('',#105314);
#29755=VERTEX_POINT('',#105315);
#29756=VERTEX_POINT('',#105331);
#29757=VERTEX_POINT('',#105333);
#29758=VERTEX_POINT('',#105357);
#29759=VERTEX_POINT('',#105358);
#29760=VERTEX_POINT('',#105374);
#29761=VERTEX_POINT('',#105376);
#29762=VERTEX_POINT('',#105387);
#29763=VERTEX_POINT('',#105388);
#29764=VERTEX_POINT('',#105423);
#29765=VERTEX_POINT('',#105430);
#29766=VERTEX_POINT('',#105447);
#29767=VERTEX_POINT('',#105449);
#29768=VERTEX_POINT('',#105473);
#29769=VERTEX_POINT('',#105477);
#29770=VERTEX_POINT('',#105494);
#29771=VERTEX_POINT('',#105496);
#29772=VERTEX_POINT('',#105520);
#29773=VERTEX_POINT('',#105524);
#29774=VERTEX_POINT('',#105541);
#29775=VERTEX_POINT('',#105543);
#29776=VERTEX_POINT('',#105567);
#29777=VERTEX_POINT('',#105571);
#29778=VERTEX_POINT('',#105588);
#29779=VERTEX_POINT('',#105590);
#29780=VERTEX_POINT('',#105614);
#29781=VERTEX_POINT('',#105618);
#29782=VERTEX_POINT('',#105635);
#29783=VERTEX_POINT('',#105637);
#29784=VERTEX_POINT('',#105661);
#29785=VERTEX_POINT('',#105665);
#29786=VERTEX_POINT('',#105682);
#29787=VERTEX_POINT('',#105684);
#29788=VERTEX_POINT('',#105708);
#29789=VERTEX_POINT('',#105712);
#29790=VERTEX_POINT('',#105729);
#29791=VERTEX_POINT('',#105731);
#29792=VERTEX_POINT('',#105755);
#29793=VERTEX_POINT('',#105759);
#29794=VERTEX_POINT('',#105776);
#29795=VERTEX_POINT('',#105778);
#29796=VERTEX_POINT('',#105802);
#29797=VERTEX_POINT('',#105806);
#29798=VERTEX_POINT('',#105823);
#29799=VERTEX_POINT('',#105825);
#29800=VERTEX_POINT('',#105849);
#29801=VERTEX_POINT('',#105853);
#29802=VERTEX_POINT('',#105870);
#29803=VERTEX_POINT('',#105872);
#29804=VERTEX_POINT('',#105896);
#29805=VERTEX_POINT('',#105900);
#29806=VERTEX_POINT('',#105917);
#29807=VERTEX_POINT('',#105919);
#29808=VERTEX_POINT('',#105943);
#29809=VERTEX_POINT('',#105947);
#29810=VERTEX_POINT('',#105964);
#29811=VERTEX_POINT('',#105966);
#29812=VERTEX_POINT('',#105990);
#29813=VERTEX_POINT('',#105994);
#29814=VERTEX_POINT('',#106011);
#29815=VERTEX_POINT('',#106013);
#29816=VERTEX_POINT('',#106037);
#29817=VERTEX_POINT('',#106041);
#29818=VERTEX_POINT('',#106090);
#29819=VERTEX_POINT('',#106092);
#29820=VERTEX_POINT('',#106116);
#29821=VERTEX_POINT('',#106120);
#29822=VERTEX_POINT('',#106137);
#29823=VERTEX_POINT('',#106139);
#29824=VERTEX_POINT('',#106163);
#29825=VERTEX_POINT('',#106167);
#29826=VERTEX_POINT('',#106184);
#29827=VERTEX_POINT('',#106186);
#29828=VERTEX_POINT('',#106210);
#29829=VERTEX_POINT('',#106214);
#29830=VERTEX_POINT('',#106231);
#29831=VERTEX_POINT('',#106233);
#29832=VERTEX_POINT('',#106257);
#29833=VERTEX_POINT('',#106261);
#29834=VERTEX_POINT('',#106278);
#29835=VERTEX_POINT('',#106280);
#29836=VERTEX_POINT('',#106304);
#29837=VERTEX_POINT('',#106308);
#29838=VERTEX_POINT('',#106325);
#29839=VERTEX_POINT('',#106327);
#29840=VERTEX_POINT('',#106351);
#29841=VERTEX_POINT('',#106355);
#29842=VERTEX_POINT('',#106372);
#29843=VERTEX_POINT('',#106374);
#29844=VERTEX_POINT('',#106398);
#29845=VERTEX_POINT('',#106402);
#29846=VERTEX_POINT('',#106419);
#29847=VERTEX_POINT('',#106421);
#29848=VERTEX_POINT('',#106445);
#29849=VERTEX_POINT('',#106449);
#29850=VERTEX_POINT('',#106466);
#29851=VERTEX_POINT('',#106468);
#29852=VERTEX_POINT('',#106492);
#29853=VERTEX_POINT('',#106496);
#29854=VERTEX_POINT('',#106513);
#29855=VERTEX_POINT('',#106515);
#29856=VERTEX_POINT('',#106539);
#29857=VERTEX_POINT('',#106543);
#29858=VERTEX_POINT('',#106560);
#29859=VERTEX_POINT('',#106562);
#29860=VERTEX_POINT('',#106586);
#29861=VERTEX_POINT('',#106590);
#29862=VERTEX_POINT('',#106607);
#29863=VERTEX_POINT('',#106609);
#29864=VERTEX_POINT('',#106633);
#29865=VERTEX_POINT('',#106637);
#29866=VERTEX_POINT('',#106654);
#29867=VERTEX_POINT('',#106656);
#29868=VERTEX_POINT('',#106680);
#29869=VERTEX_POINT('',#106684);
#29870=VERTEX_POINT('',#106701);
#29871=VERTEX_POINT('',#106703);
#29872=VERTEX_POINT('',#106727);
#29873=VERTEX_POINT('',#106731);
#29874=VERTEX_POINT('',#106735);
#29875=VERTEX_POINT('',#106743);
#29876=VERTEX_POINT('',#106767);
#29877=VERTEX_POINT('',#106790);
#29878=VERTEX_POINT('',#106820);
#29879=VERTEX_POINT('',#106850);
#29880=VERTEX_POINT('',#106880);
#29881=VERTEX_POINT('',#106910);
#29882=VERTEX_POINT('',#106940);
#29883=VERTEX_POINT('',#106970);
#29884=VERTEX_POINT('',#107000);
#29885=VERTEX_POINT('',#107030);
#29886=VERTEX_POINT('',#107060);
#29887=VERTEX_POINT('',#107090);
#29888=VERTEX_POINT('',#107120);
#29889=VERTEX_POINT('',#107150);
#29890=VERTEX_POINT('',#107180);
#29891=VERTEX_POINT('',#107210);
#29892=VERTEX_POINT('',#107240);
#29893=VERTEX_POINT('',#107270);
#29894=VERTEX_POINT('',#107300);
#29895=VERTEX_POINT('',#107330);
#29896=VERTEX_POINT('',#107360);
#29897=VERTEX_POINT('',#107390);
#29898=VERTEX_POINT('',#107420);
#29899=VERTEX_POINT('',#107450);
#29900=VERTEX_POINT('',#107480);
#29901=VERTEX_POINT('',#107510);
#29902=VERTEX_POINT('',#107540);
#29903=VERTEX_POINT('',#107570);
#29904=VERTEX_POINT('',#107600);
#29905=VERTEX_POINT('',#107637);
#29906=VERTEX_POINT('',#107655);
#29907=VERTEX_POINT('',#107689);
#29908=VERTEX_POINT('',#107723);
#29909=VERTEX_POINT('',#107757);
#29910=VERTEX_POINT('',#107791);
#29911=VERTEX_POINT('',#107825);
#29912=VERTEX_POINT('',#107859);
#29913=VERTEX_POINT('',#107893);
#29914=VERTEX_POINT('',#107927);
#29915=VERTEX_POINT('',#107961);
#29916=VERTEX_POINT('',#107995);
#29917=VERTEX_POINT('',#108029);
#29918=VERTEX_POINT('',#108063);
#29919=VERTEX_POINT('',#108097);
#29920=VERTEX_POINT('',#108131);
#29921=VERTEX_POINT('',#108165);
#29922=VERTEX_POINT('',#108199);
#29923=VERTEX_POINT('',#108233);
#29924=VERTEX_POINT('',#108267);
#29925=VERTEX_POINT('',#108301);
#29926=VERTEX_POINT('',#108335);
#29927=VERTEX_POINT('',#108369);
#29928=VERTEX_POINT('',#108403);
#29929=VERTEX_POINT('',#108437);
#29930=VERTEX_POINT('',#108471);
#29931=VERTEX_POINT('',#108505);
#29932=VERTEX_POINT('',#108539);
#29933=VERTEX_POINT('',#108573);
#29934=VERTEX_POINT('',#108622);
#29935=VERTEX_POINT('',#108623);
#29936=VERTEX_POINT('',#108633);
#29937=VERTEX_POINT('',#108635);
#29938=VERTEX_POINT('',#108658);
#29939=VERTEX_POINT('',#108659);
#29940=VERTEX_POINT('',#108669);
#29941=VERTEX_POINT('',#108671);
#29942=VERTEX_POINT('',#108694);
#29943=VERTEX_POINT('',#108695);
#29944=VERTEX_POINT('',#108705);
#29945=VERTEX_POINT('',#108707);
#29946=VERTEX_POINT('',#108730);
#29947=VERTEX_POINT('',#108731);
#29948=VERTEX_POINT('',#108741);
#29949=VERTEX_POINT('',#108743);
#29950=VERTEX_POINT('',#108766);
#29951=VERTEX_POINT('',#108767);
#29952=VERTEX_POINT('',#108777);
#29953=VERTEX_POINT('',#108779);
#29954=VERTEX_POINT('',#108802);
#29955=VERTEX_POINT('',#108803);
#29956=VERTEX_POINT('',#108813);
#29957=VERTEX_POINT('',#108815);
#29958=VERTEX_POINT('',#108838);
#29959=VERTEX_POINT('',#108839);
#29960=VERTEX_POINT('',#108849);
#29961=VERTEX_POINT('',#108851);
#29962=VERTEX_POINT('',#108874);
#29963=VERTEX_POINT('',#108875);
#29964=VERTEX_POINT('',#108885);
#29965=VERTEX_POINT('',#108887);
#29966=VERTEX_POINT('',#108910);
#29967=VERTEX_POINT('',#108911);
#29968=VERTEX_POINT('',#108921);
#29969=VERTEX_POINT('',#108923);
#29970=VERTEX_POINT('',#108946);
#29971=VERTEX_POINT('',#108947);
#29972=VERTEX_POINT('',#108957);
#29973=VERTEX_POINT('',#108959);
#29974=VERTEX_POINT('',#108982);
#29975=VERTEX_POINT('',#108983);
#29976=VERTEX_POINT('',#108993);
#29977=VERTEX_POINT('',#108995);
#29978=VERTEX_POINT('',#109018);
#29979=VERTEX_POINT('',#109019);
#29980=VERTEX_POINT('',#109029);
#29981=VERTEX_POINT('',#109031);
#29982=VERTEX_POINT('',#109054);
#29983=VERTEX_POINT('',#109055);
#29984=VERTEX_POINT('',#109065);
#29985=VERTEX_POINT('',#109067);
#29986=VERTEX_POINT('',#109090);
#29987=VERTEX_POINT('',#109091);
#29988=VERTEX_POINT('',#109101);
#29989=VERTEX_POINT('',#109103);
#29990=VERTEX_POINT('',#109153);
#29991=VERTEX_POINT('',#109154);
#29992=VERTEX_POINT('',#109164);
#29993=VERTEX_POINT('',#109166);
#29994=VERTEX_POINT('',#109189);
#29995=VERTEX_POINT('',#109190);
#29996=VERTEX_POINT('',#109200);
#29997=VERTEX_POINT('',#109202);
#29998=VERTEX_POINT('',#109225);
#29999=VERTEX_POINT('',#109226);
#30000=VERTEX_POINT('',#109236);
#30001=VERTEX_POINT('',#109238);
#30002=VERTEX_POINT('',#109261);
#30003=VERTEX_POINT('',#109262);
#30004=VERTEX_POINT('',#109272);
#30005=VERTEX_POINT('',#109274);
#30006=VERTEX_POINT('',#109297);
#30007=VERTEX_POINT('',#109298);
#30008=VERTEX_POINT('',#109308);
#30009=VERTEX_POINT('',#109310);
#30010=VERTEX_POINT('',#109333);
#30011=VERTEX_POINT('',#109334);
#30012=VERTEX_POINT('',#109344);
#30013=VERTEX_POINT('',#109346);
#30014=VERTEX_POINT('',#109369);
#30015=VERTEX_POINT('',#109370);
#30016=VERTEX_POINT('',#109380);
#30017=VERTEX_POINT('',#109382);
#30018=VERTEX_POINT('',#109405);
#30019=VERTEX_POINT('',#109406);
#30020=VERTEX_POINT('',#109416);
#30021=VERTEX_POINT('',#109418);
#30022=VERTEX_POINT('',#109441);
#30023=VERTEX_POINT('',#109442);
#30024=VERTEX_POINT('',#109460);
#30025=VERTEX_POINT('',#109464);
#30026=VERTEX_POINT('',#109477);
#30027=VERTEX_POINT('',#109479);
#30028=VERTEX_POINT('',#109488);
#30029=VERTEX_POINT('',#109490);
#30030=VERTEX_POINT('',#109513);
#30031=VERTEX_POINT('',#109514);
#30032=VERTEX_POINT('',#109524);
#30033=VERTEX_POINT('',#109526);
#30034=VERTEX_POINT('',#109549);
#30035=VERTEX_POINT('',#109550);
#30036=VERTEX_POINT('',#109560);
#30037=VERTEX_POINT('',#109562);
#30038=VERTEX_POINT('',#109585);
#30039=VERTEX_POINT('',#109586);
#30040=VERTEX_POINT('',#109596);
#30041=VERTEX_POINT('',#109598);
#30042=VERTEX_POINT('',#109621);
#30043=VERTEX_POINT('',#109622);
#30044=VERTEX_POINT('',#109632);
#30045=VERTEX_POINT('',#109634);
#30046=VERTEX_POINT('',#109653);
#30047=VERTEX_POINT('',#109655);
#30048=VERTEX_POINT('',#109677);
#30049=VERTEX_POINT('',#109687);
#30050=VERTEX_POINT('',#109696);
#30051=VERTEX_POINT('',#109698);
#30052=VERTEX_POINT('',#109720);
#30053=VERTEX_POINT('',#109730);
#30054=VERTEX_POINT('',#109739);
#30055=VERTEX_POINT('',#109741);
#30056=VERTEX_POINT('',#109763);
#30057=VERTEX_POINT('',#109773);
#30058=VERTEX_POINT('',#109782);
#30059=VERTEX_POINT('',#109784);
#30060=VERTEX_POINT('',#109806);
#30061=VERTEX_POINT('',#109816);
#30062=VERTEX_POINT('',#109825);
#30063=VERTEX_POINT('',#109827);
#30064=VERTEX_POINT('',#109849);
#30065=VERTEX_POINT('',#109859);
#30066=VERTEX_POINT('',#109868);
#30067=VERTEX_POINT('',#109870);
#30068=VERTEX_POINT('',#109892);
#30069=VERTEX_POINT('',#109902);
#30070=VERTEX_POINT('',#109911);
#30071=VERTEX_POINT('',#109913);
#30072=VERTEX_POINT('',#109935);
#30073=VERTEX_POINT('',#109945);
#30074=VERTEX_POINT('',#109954);
#30075=VERTEX_POINT('',#109956);
#30076=VERTEX_POINT('',#109978);
#30077=VERTEX_POINT('',#109988);
#30078=VERTEX_POINT('',#109997);
#30079=VERTEX_POINT('',#109999);
#30080=VERTEX_POINT('',#110021);
#30081=VERTEX_POINT('',#110031);
#30082=VERTEX_POINT('',#110040);
#30083=VERTEX_POINT('',#110042);
#30084=VERTEX_POINT('',#110064);
#30085=VERTEX_POINT('',#110074);
#30086=VERTEX_POINT('',#110083);
#30087=VERTEX_POINT('',#110085);
#30088=VERTEX_POINT('',#110107);
#30089=VERTEX_POINT('',#110117);
#30090=VERTEX_POINT('',#110126);
#30091=VERTEX_POINT('',#110128);
#30092=VERTEX_POINT('',#110150);
#30093=VERTEX_POINT('',#110160);
#30094=VERTEX_POINT('',#110169);
#30095=VERTEX_POINT('',#110171);
#30096=VERTEX_POINT('',#110193);
#30097=VERTEX_POINT('',#110203);
#30098=VERTEX_POINT('',#110212);
#30099=VERTEX_POINT('',#110214);
#30100=VERTEX_POINT('',#110236);
#30101=VERTEX_POINT('',#110246);
#30102=VERTEX_POINT('',#110255);
#30103=VERTEX_POINT('',#110257);
#30104=VERTEX_POINT('',#110279);
#30105=VERTEX_POINT('',#110289);
#30106=VERTEX_POINT('',#110298);
#30107=VERTEX_POINT('',#110300);
#30108=VERTEX_POINT('',#110322);
#30109=VERTEX_POINT('',#110332);
#30110=VERTEX_POINT('',#110341);
#30111=VERTEX_POINT('',#110343);
#30112=VERTEX_POINT('',#110365);
#30113=VERTEX_POINT('',#110375);
#30114=VERTEX_POINT('',#110384);
#30115=VERTEX_POINT('',#110386);
#30116=VERTEX_POINT('',#110408);
#30117=VERTEX_POINT('',#110418);
#30118=VERTEX_POINT('',#110427);
#30119=VERTEX_POINT('',#110429);
#30120=VERTEX_POINT('',#110451);
#30121=VERTEX_POINT('',#110461);
#30122=VERTEX_POINT('',#110470);
#30123=VERTEX_POINT('',#110472);
#30124=VERTEX_POINT('',#110494);
#30125=VERTEX_POINT('',#110504);
#30126=VERTEX_POINT('',#110513);
#30127=VERTEX_POINT('',#110515);
#30128=VERTEX_POINT('',#110537);
#30129=VERTEX_POINT('',#110547);
#30130=VERTEX_POINT('',#110556);
#30131=VERTEX_POINT('',#110558);
#30132=VERTEX_POINT('',#110580);
#30133=VERTEX_POINT('',#110590);
#30134=VERTEX_POINT('',#110599);
#30135=VERTEX_POINT('',#110601);
#30136=VERTEX_POINT('',#110623);
#30137=VERTEX_POINT('',#110633);
#30138=VERTEX_POINT('',#110642);
#30139=VERTEX_POINT('',#110644);
#30140=VERTEX_POINT('',#110666);
#30141=VERTEX_POINT('',#110676);
#30142=VERTEX_POINT('',#110685);
#30143=VERTEX_POINT('',#110687);
#30144=VERTEX_POINT('',#110709);
#30145=VERTEX_POINT('',#110719);
#30146=VERTEX_POINT('',#110728);
#30147=VERTEX_POINT('',#110730);
#30148=VERTEX_POINT('',#110752);
#30149=VERTEX_POINT('',#110762);
#30150=VERTEX_POINT('',#110771);
#30151=VERTEX_POINT('',#110773);
#30152=VERTEX_POINT('',#110795);
#30153=VERTEX_POINT('',#110805);
#30154=VERTEX_POINT('',#110814);
#30155=VERTEX_POINT('',#110816);
#30156=VERTEX_POINT('',#110838);
#30157=VERTEX_POINT('',#110848);
#30158=VERTEX_POINT('',#110857);
#30159=VERTEX_POINT('',#110859);
#30160=VERTEX_POINT('',#110881);
#30161=VERTEX_POINT('',#110891);
#30162=VERTEX_POINT('',#110904);
#30163=VERTEX_POINT('',#110929);
#30164=VERTEX_POINT('',#110954);
#30165=VERTEX_POINT('',#110979);
#30166=VERTEX_POINT('',#111004);
#30167=VERTEX_POINT('',#111029);
#30168=VERTEX_POINT('',#111054);
#30169=VERTEX_POINT('',#111079);
#30170=VERTEX_POINT('',#111104);
#30171=VERTEX_POINT('',#111129);
#30172=VERTEX_POINT('',#111154);
#30173=VERTEX_POINT('',#111179);
#30174=VERTEX_POINT('',#111204);
#30175=VERTEX_POINT('',#111229);
#30176=VERTEX_POINT('',#111254);
#30177=VERTEX_POINT('',#111279);
#30178=VERTEX_POINT('',#111304);
#30179=VERTEX_POINT('',#111329);
#30180=VERTEX_POINT('',#111354);
#30181=VERTEX_POINT('',#111379);
#30182=VERTEX_POINT('',#111404);
#30183=VERTEX_POINT('',#111429);
#30184=VERTEX_POINT('',#111454);
#30185=VERTEX_POINT('',#111479);
#30186=VERTEX_POINT('',#111504);
#30187=VERTEX_POINT('',#111529);
#30188=VERTEX_POINT('',#111554);
#30189=VERTEX_POINT('',#111579);
#30190=VERTEX_POINT('',#111604);
#30191=VERTEX_POINT('',#111625);
#30192=VERTEX_POINT('',#111650);
#30193=VERTEX_POINT('',#111675);
#30194=VERTEX_POINT('',#111700);
#30195=VERTEX_POINT('',#111725);
#30196=VERTEX_POINT('',#111750);
#30197=VERTEX_POINT('',#111775);
#30198=VERTEX_POINT('',#111800);
#30199=VERTEX_POINT('',#111825);
#30200=VERTEX_POINT('',#111850);
#30201=VERTEX_POINT('',#111875);
#30202=VERTEX_POINT('',#111900);
#30203=VERTEX_POINT('',#111925);
#30204=VERTEX_POINT('',#111950);
#30205=VERTEX_POINT('',#111975);
#30206=VERTEX_POINT('',#112000);
#30207=VERTEX_POINT('',#112025);
#30208=VERTEX_POINT('',#112050);
#30209=VERTEX_POINT('',#112075);
#30210=VERTEX_POINT('',#112100);
#30211=VERTEX_POINT('',#112125);
#30212=VERTEX_POINT('',#112150);
#30213=VERTEX_POINT('',#112175);
#30214=VERTEX_POINT('',#112200);
#30215=VERTEX_POINT('',#112225);
#30216=VERTEX_POINT('',#112250);
#30217=VERTEX_POINT('',#112275);
#30218=VERTEX_POINT('',#112300);
#30219=VERTEX_POINT('',#112325);
#30220=VERTEX_POINT('',#112354);
#30221=VERTEX_POINT('',#112355);
#30222=VERTEX_POINT('',#112374);
#30223=VERTEX_POINT('',#112375);
#30224=VERTEX_POINT('',#112385);
#30225=VERTEX_POINT('',#112396);
#30226=VERTEX_POINT('',#112420);
#30227=VERTEX_POINT('',#112421);
#30228=VERTEX_POINT('',#112431);
#30229=VERTEX_POINT('',#112442);
#30230=VERTEX_POINT('',#112466);
#30231=VERTEX_POINT('',#112467);
#30232=VERTEX_POINT('',#112477);
#30233=VERTEX_POINT('',#112488);
#30234=VERTEX_POINT('',#112512);
#30235=VERTEX_POINT('',#112513);
#30236=VERTEX_POINT('',#112523);
#30237=VERTEX_POINT('',#112534);
#30238=VERTEX_POINT('',#112558);
#30239=VERTEX_POINT('',#112559);
#30240=VERTEX_POINT('',#112569);
#30241=VERTEX_POINT('',#112580);
#30242=VERTEX_POINT('',#112604);
#30243=VERTEX_POINT('',#112605);
#30244=VERTEX_POINT('',#112615);
#30245=VERTEX_POINT('',#112626);
#30246=VERTEX_POINT('',#112678);
#30247=VERTEX_POINT('',#112679);
#30248=VERTEX_POINT('',#112689);
#30249=VERTEX_POINT('',#112700);
#30250=VERTEX_POINT('',#112724);
#30251=VERTEX_POINT('',#112725);
#30252=VERTEX_POINT('',#112735);
#30253=VERTEX_POINT('',#112746);
#30254=VERTEX_POINT('',#112770);
#30255=VERTEX_POINT('',#112771);
#30256=VERTEX_POINT('',#112781);
#30257=VERTEX_POINT('',#112792);
#30258=VERTEX_POINT('',#112816);
#30259=VERTEX_POINT('',#112817);
#30260=VERTEX_POINT('',#112827);
#30261=VERTEX_POINT('',#112838);
#30262=VERTEX_POINT('',#112862);
#30263=VERTEX_POINT('',#112863);
#30264=VERTEX_POINT('',#112873);
#30265=VERTEX_POINT('',#112884);
#30266=VERTEX_POINT('',#112908);
#30267=VERTEX_POINT('',#112909);
#30268=VERTEX_POINT('',#112919);
#30269=VERTEX_POINT('',#112930);
#30270=VERTEX_POINT('',#112954);
#30271=VERTEX_POINT('',#112955);
#30272=VERTEX_POINT('',#112965);
#30273=VERTEX_POINT('',#112976);
#30274=VERTEX_POINT('',#113000);
#30275=VERTEX_POINT('',#113001);
#30276=VERTEX_POINT('',#113011);
#30277=VERTEX_POINT('',#113022);
#30278=VERTEX_POINT('',#113046);
#30279=VERTEX_POINT('',#113047);
#30280=VERTEX_POINT('',#113057);
#30281=VERTEX_POINT('',#113068);
#30282=VERTEX_POINT('',#113092);
#30283=VERTEX_POINT('',#113093);
#30284=VERTEX_POINT('',#113103);
#30285=VERTEX_POINT('',#113114);
#30286=VERTEX_POINT('',#113138);
#30287=VERTEX_POINT('',#113139);
#30288=VERTEX_POINT('',#113149);
#30289=VERTEX_POINT('',#113160);
#30290=VERTEX_POINT('',#113184);
#30291=VERTEX_POINT('',#113185);
#30292=VERTEX_POINT('',#113195);
#30293=VERTEX_POINT('',#113206);
#30294=VERTEX_POINT('',#113230);
#30295=VERTEX_POINT('',#113231);
#30296=VERTEX_POINT('',#113241);
#30297=VERTEX_POINT('',#113252);
#30298=VERTEX_POINT('',#113276);
#30299=VERTEX_POINT('',#113277);
#30300=VERTEX_POINT('',#113287);
#30301=VERTEX_POINT('',#113298);
#30302=VERTEX_POINT('',#113322);
#30303=VERTEX_POINT('',#113323);
#30304=VERTEX_POINT('',#113333);
#30305=VERTEX_POINT('',#113344);
#30306=VERTEX_POINT('',#113368);
#30307=VERTEX_POINT('',#113369);
#30308=VERTEX_POINT('',#113388);
#30309=VERTEX_POINT('',#113392);
#30310=VERTEX_POINT('',#113414);
#30311=VERTEX_POINT('',#113416);
#30312=VERTEX_POINT('',#113425);
#30313=VERTEX_POINT('',#113427);
#30314=VERTEX_POINT('',#113460);
#30315=VERTEX_POINT('',#113461);
#30316=VERTEX_POINT('',#113471);
#30317=VERTEX_POINT('',#113482);
#30318=VERTEX_POINT('',#113506);
#30319=VERTEX_POINT('',#113507);
#30320=VERTEX_POINT('',#113517);
#30321=VERTEX_POINT('',#113528);
#30322=VERTEX_POINT('',#113552);
#30323=VERTEX_POINT('',#113553);
#30324=VERTEX_POINT('',#113563);
#30325=VERTEX_POINT('',#113574);
#30326=VERTEX_POINT('',#113598);
#30327=VERTEX_POINT('',#113599);
#30328=VERTEX_POINT('',#113609);
#30329=VERTEX_POINT('',#113620);
#30330=VERTEX_POINT('',#113635);
#30331=VERTEX_POINT('',#113636);
#30332=VERTEX_POINT('',#113670);
#30333=VERTEX_POINT('',#113671);
#30334=VERTEX_POINT('',#113686);
#30335=VERTEX_POINT('',#113688);
#30336=VERTEX_POINT('',#113706);
#30337=VERTEX_POINT('',#113710);
#30338=VERTEX_POINT('',#113719);
#30339=VERTEX_POINT('',#113721);
#30340=VERTEX_POINT('',#113739);
#30341=VERTEX_POINT('',#113743);
#30342=VERTEX_POINT('',#113752);
#30343=VERTEX_POINT('',#113754);
#30344=VERTEX_POINT('',#113772);
#30345=VERTEX_POINT('',#113776);
#30346=VERTEX_POINT('',#113785);
#30347=VERTEX_POINT('',#113787);
#30348=VERTEX_POINT('',#113805);
#30349=VERTEX_POINT('',#113809);
#30350=VERTEX_POINT('',#113818);
#30351=VERTEX_POINT('',#113820);
#30352=VERTEX_POINT('',#113838);
#30353=VERTEX_POINT('',#113842);
#30354=VERTEX_POINT('',#113851);
#30355=VERTEX_POINT('',#113853);
#30356=VERTEX_POINT('',#113871);
#30357=VERTEX_POINT('',#113875);
#30358=VERTEX_POINT('',#113884);
#30359=VERTEX_POINT('',#113886);
#30360=VERTEX_POINT('',#113904);
#30361=VERTEX_POINT('',#113908);
#30362=VERTEX_POINT('',#113917);
#30363=VERTEX_POINT('',#113919);
#30364=VERTEX_POINT('',#113937);
#30365=VERTEX_POINT('',#113941);
#30366=VERTEX_POINT('',#113950);
#30367=VERTEX_POINT('',#113952);
#30368=VERTEX_POINT('',#113970);
#30369=VERTEX_POINT('',#113974);
#30370=VERTEX_POINT('',#113983);
#30371=VERTEX_POINT('',#113985);
#30372=VERTEX_POINT('',#114003);
#30373=VERTEX_POINT('',#114007);
#30374=VERTEX_POINT('',#114016);
#30375=VERTEX_POINT('',#114018);
#30376=VERTEX_POINT('',#114036);
#30377=VERTEX_POINT('',#114040);
#30378=VERTEX_POINT('',#114049);
#30379=VERTEX_POINT('',#114051);
#30380=VERTEX_POINT('',#114069);
#30381=VERTEX_POINT('',#114073);
#30382=VERTEX_POINT('',#114082);
#30383=VERTEX_POINT('',#114084);
#30384=VERTEX_POINT('',#114102);
#30385=VERTEX_POINT('',#114106);
#30386=VERTEX_POINT('',#114139);
#30387=VERTEX_POINT('',#114141);
#30388=VERTEX_POINT('',#114159);
#30389=VERTEX_POINT('',#114163);
#30390=VERTEX_POINT('',#114172);
#30391=VERTEX_POINT('',#114174);
#30392=VERTEX_POINT('',#114192);
#30393=VERTEX_POINT('',#114196);
#30394=VERTEX_POINT('',#114205);
#30395=VERTEX_POINT('',#114207);
#30396=VERTEX_POINT('',#114225);
#30397=VERTEX_POINT('',#114229);
#30398=VERTEX_POINT('',#114238);
#30399=VERTEX_POINT('',#114240);
#30400=VERTEX_POINT('',#114258);
#30401=VERTEX_POINT('',#114262);
#30402=VERTEX_POINT('',#114271);
#30403=VERTEX_POINT('',#114273);
#30404=VERTEX_POINT('',#114291);
#30405=VERTEX_POINT('',#114295);
#30406=VERTEX_POINT('',#114304);
#30407=VERTEX_POINT('',#114306);
#30408=VERTEX_POINT('',#114324);
#30409=VERTEX_POINT('',#114328);
#30410=VERTEX_POINT('',#114337);
#30411=VERTEX_POINT('',#114339);
#30412=VERTEX_POINT('',#114357);
#30413=VERTEX_POINT('',#114361);
#30414=VERTEX_POINT('',#114370);
#30415=VERTEX_POINT('',#114372);
#30416=VERTEX_POINT('',#114390);
#30417=VERTEX_POINT('',#114394);
#30418=VERTEX_POINT('',#114403);
#30419=VERTEX_POINT('',#114405);
#30420=VERTEX_POINT('',#114423);
#30421=VERTEX_POINT('',#114427);
#30422=VERTEX_POINT('',#114436);
#30423=VERTEX_POINT('',#114438);
#30424=VERTEX_POINT('',#114456);
#30425=VERTEX_POINT('',#114460);
#30426=VERTEX_POINT('',#114469);
#30427=VERTEX_POINT('',#114471);
#30428=VERTEX_POINT('',#114489);
#30429=VERTEX_POINT('',#114493);
#30430=VERTEX_POINT('',#114502);
#30431=VERTEX_POINT('',#114504);
#30432=VERTEX_POINT('',#114522);
#30433=VERTEX_POINT('',#114526);
#30434=VERTEX_POINT('',#114535);
#30435=VERTEX_POINT('',#114537);
#30436=VERTEX_POINT('',#114555);
#30437=VERTEX_POINT('',#114559);
#30438=VERTEX_POINT('',#114568);
#30439=VERTEX_POINT('',#114570);
#30440=VERTEX_POINT('',#114588);
#30441=VERTEX_POINT('',#114592);
#30442=VERTEX_POINT('',#114596);
#30443=VERTEX_POINT('',#114597);
#30444=VERTEX_POINT('',#114614);
#30445=VERTEX_POINT('',#114632);
#30446=VERTEX_POINT('',#114663);
#30447=VERTEX_POINT('',#114694);
#30448=VERTEX_POINT('',#114725);
#30449=VERTEX_POINT('',#114756);
#30450=VERTEX_POINT('',#114787);
#30451=VERTEX_POINT('',#114818);
#30452=VERTEX_POINT('',#114849);
#30453=VERTEX_POINT('',#114880);
#30454=VERTEX_POINT('',#114911);
#30455=VERTEX_POINT('',#114942);
#30456=VERTEX_POINT('',#114973);
#30457=VERTEX_POINT('',#115004);
#30458=VERTEX_POINT('',#115035);
#30459=VERTEX_POINT('',#115066);
#30460=VERTEX_POINT('',#115097);
#30461=VERTEX_POINT('',#115128);
#30462=VERTEX_POINT('',#115159);
#30463=VERTEX_POINT('',#115190);
#30464=VERTEX_POINT('',#115221);
#30465=VERTEX_POINT('',#115252);
#30466=VERTEX_POINT('',#115283);
#30467=VERTEX_POINT('',#115314);
#30468=VERTEX_POINT('',#115345);
#30469=VERTEX_POINT('',#115376);
#30470=VERTEX_POINT('',#115407);
#30471=VERTEX_POINT('',#115438);
#30472=VERTEX_POINT('',#115469);
#30473=VERTEX_POINT('',#115517);
#30474=VERTEX_POINT('',#115531);
#30475=VERTEX_POINT('',#115556);
#30476=VERTEX_POINT('',#115581);
#30477=VERTEX_POINT('',#115606);
#30478=VERTEX_POINT('',#115631);
#30479=VERTEX_POINT('',#115656);
#30480=VERTEX_POINT('',#115681);
#30481=VERTEX_POINT('',#115706);
#30482=VERTEX_POINT('',#115731);
#30483=VERTEX_POINT('',#115756);
#30484=VERTEX_POINT('',#115781);
#30485=VERTEX_POINT('',#115806);
#30486=VERTEX_POINT('',#115831);
#30487=VERTEX_POINT('',#115856);
#30488=VERTEX_POINT('',#115881);
#30489=VERTEX_POINT('',#115906);
#30490=VERTEX_POINT('',#115931);
#30491=VERTEX_POINT('',#115956);
#30492=VERTEX_POINT('',#115981);
#30493=VERTEX_POINT('',#116006);
#30494=VERTEX_POINT('',#116031);
#30495=VERTEX_POINT('',#116056);
#30496=VERTEX_POINT('',#116081);
#30497=VERTEX_POINT('',#116106);
#30498=VERTEX_POINT('',#116131);
#30499=VERTEX_POINT('',#116156);
#30500=VERTEX_POINT('',#116181);
#30501=VERTEX_POINT('',#116206);
#30502=VERTEX_POINT('',#116242);
#30503=VERTEX_POINT('',#116243);
#30504=VERTEX_POINT('',#116253);
#30505=VERTEX_POINT('',#116255);
#30506=VERTEX_POINT('',#116289);
#30507=VERTEX_POINT('',#116290);
#30508=VERTEX_POINT('',#116300);
#30509=VERTEX_POINT('',#116302);
#30510=VERTEX_POINT('',#116336);
#30511=VERTEX_POINT('',#116337);
#30512=VERTEX_POINT('',#116347);
#30513=VERTEX_POINT('',#116349);
#30514=VERTEX_POINT('',#116383);
#30515=VERTEX_POINT('',#116384);
#30516=VERTEX_POINT('',#116394);
#30517=VERTEX_POINT('',#116396);
#30518=VERTEX_POINT('',#116430);
#30519=VERTEX_POINT('',#116431);
#30520=VERTEX_POINT('',#116441);
#30521=VERTEX_POINT('',#116443);
#30522=VERTEX_POINT('',#116477);
#30523=VERTEX_POINT('',#116478);
#30524=VERTEX_POINT('',#116488);
#30525=VERTEX_POINT('',#116490);
#30526=VERTEX_POINT('',#116524);
#30527=VERTEX_POINT('',#116525);
#30528=VERTEX_POINT('',#116535);
#30529=VERTEX_POINT('',#116537);
#30530=VERTEX_POINT('',#116571);
#30531=VERTEX_POINT('',#116572);
#30532=VERTEX_POINT('',#116582);
#30533=VERTEX_POINT('',#116584);
#30534=VERTEX_POINT('',#116618);
#30535=VERTEX_POINT('',#116619);
#30536=VERTEX_POINT('',#116629);
#30537=VERTEX_POINT('',#116631);
#30538=VERTEX_POINT('',#116665);
#30539=VERTEX_POINT('',#116666);
#30540=VERTEX_POINT('',#116676);
#30541=VERTEX_POINT('',#116678);
#30542=VERTEX_POINT('',#116712);
#30543=VERTEX_POINT('',#116713);
#30544=VERTEX_POINT('',#116723);
#30545=VERTEX_POINT('',#116725);
#30546=VERTEX_POINT('',#116759);
#30547=VERTEX_POINT('',#116760);
#30548=VERTEX_POINT('',#116770);
#30549=VERTEX_POINT('',#116772);
#30550=VERTEX_POINT('',#116806);
#30551=VERTEX_POINT('',#116807);
#30552=VERTEX_POINT('',#116817);
#30553=VERTEX_POINT('',#116819);
#30554=VERTEX_POINT('',#116853);
#30555=VERTEX_POINT('',#116854);
#30556=VERTEX_POINT('',#116864);
#30557=VERTEX_POINT('',#116866);
#30558=VERTEX_POINT('',#116932);
#30559=VERTEX_POINT('',#116933);
#30560=VERTEX_POINT('',#116943);
#30561=VERTEX_POINT('',#116945);
#30562=VERTEX_POINT('',#116979);
#30563=VERTEX_POINT('',#116980);
#30564=VERTEX_POINT('',#116990);
#30565=VERTEX_POINT('',#116992);
#30566=VERTEX_POINT('',#117026);
#30567=VERTEX_POINT('',#117027);
#30568=VERTEX_POINT('',#117037);
#30569=VERTEX_POINT('',#117039);
#30570=VERTEX_POINT('',#117073);
#30571=VERTEX_POINT('',#117074);
#30572=VERTEX_POINT('',#117084);
#30573=VERTEX_POINT('',#117086);
#30574=VERTEX_POINT('',#117120);
#30575=VERTEX_POINT('',#117121);
#30576=VERTEX_POINT('',#117131);
#30577=VERTEX_POINT('',#117133);
#30578=VERTEX_POINT('',#117167);
#30579=VERTEX_POINT('',#117168);
#30580=VERTEX_POINT('',#117178);
#30581=VERTEX_POINT('',#117180);
#30582=VERTEX_POINT('',#117214);
#30583=VERTEX_POINT('',#117215);
#30584=VERTEX_POINT('',#117225);
#30585=VERTEX_POINT('',#117227);
#30586=VERTEX_POINT('',#117261);
#30587=VERTEX_POINT('',#117262);
#30588=VERTEX_POINT('',#117285);
#30589=VERTEX_POINT('',#117295);
#30590=VERTEX_POINT('',#117308);
#30591=VERTEX_POINT('',#117310);
#30592=VERTEX_POINT('',#117319);
#30593=VERTEX_POINT('',#117327);
#30594=VERTEX_POINT('',#117355);
#30595=VERTEX_POINT('',#117356);
#30596=VERTEX_POINT('',#117366);
#30597=VERTEX_POINT('',#117368);
#30598=VERTEX_POINT('',#117402);
#30599=VERTEX_POINT('',#117403);
#30600=VERTEX_POINT('',#117413);
#30601=VERTEX_POINT('',#117415);
#30602=VERTEX_POINT('',#117449);
#30603=VERTEX_POINT('',#117450);
#30604=VERTEX_POINT('',#117460);
#30605=VERTEX_POINT('',#117462);
#30606=VERTEX_POINT('',#117496);
#30607=VERTEX_POINT('',#117497);
#30608=VERTEX_POINT('',#117507);
#30609=VERTEX_POINT('',#117509);
#30610=VERTEX_POINT('',#117543);
#30611=VERTEX_POINT('',#117544);
#30612=VERTEX_POINT('',#117554);
#30613=VERTEX_POINT('',#117556);
#30614=VERTEX_POINT('',#117590);
#30615=VERTEX_POINT('',#117592);
#30616=VERTEX_POINT('',#117610);
#30617=VERTEX_POINT('',#117614);
#30618=VERTEX_POINT('',#117627);
#30619=VERTEX_POINT('',#117629);
#30620=VERTEX_POINT('',#117647);
#30621=VERTEX_POINT('',#117651);
#30622=VERTEX_POINT('',#117664);
#30623=VERTEX_POINT('',#117666);
#30624=VERTEX_POINT('',#117684);
#30625=VERTEX_POINT('',#117688);
#30626=VERTEX_POINT('',#117701);
#30627=VERTEX_POINT('',#117703);
#30628=VERTEX_POINT('',#117721);
#30629=VERTEX_POINT('',#117725);
#30630=VERTEX_POINT('',#117738);
#30631=VERTEX_POINT('',#117740);
#30632=VERTEX_POINT('',#117758);
#30633=VERTEX_POINT('',#117762);
#30634=VERTEX_POINT('',#117775);
#30635=VERTEX_POINT('',#117777);
#30636=VERTEX_POINT('',#117795);
#30637=VERTEX_POINT('',#117799);
#30638=VERTEX_POINT('',#117812);
#30639=VERTEX_POINT('',#117814);
#30640=VERTEX_POINT('',#117832);
#30641=VERTEX_POINT('',#117836);
#30642=VERTEX_POINT('',#117849);
#30643=VERTEX_POINT('',#117851);
#30644=VERTEX_POINT('',#117869);
#30645=VERTEX_POINT('',#117873);
#30646=VERTEX_POINT('',#117886);
#30647=VERTEX_POINT('',#117888);
#30648=VERTEX_POINT('',#117906);
#30649=VERTEX_POINT('',#117910);
#30650=VERTEX_POINT('',#117923);
#30651=VERTEX_POINT('',#117925);
#30652=VERTEX_POINT('',#117943);
#30653=VERTEX_POINT('',#117947);
#30654=VERTEX_POINT('',#117960);
#30655=VERTEX_POINT('',#117962);
#30656=VERTEX_POINT('',#117980);
#30657=VERTEX_POINT('',#117984);
#30658=VERTEX_POINT('',#117997);
#30659=VERTEX_POINT('',#117999);
#30660=VERTEX_POINT('',#118017);
#30661=VERTEX_POINT('',#118021);
#30662=VERTEX_POINT('',#118034);
#30663=VERTEX_POINT('',#118036);
#30664=VERTEX_POINT('',#118054);
#30665=VERTEX_POINT('',#118058);
#30666=VERTEX_POINT('',#118071);
#30667=VERTEX_POINT('',#118073);
#30668=VERTEX_POINT('',#118091);
#30669=VERTEX_POINT('',#118095);
#30670=VERTEX_POINT('',#118108);
#30671=VERTEX_POINT('',#118110);
#30672=VERTEX_POINT('',#118128);
#30673=VERTEX_POINT('',#118132);
#30674=VERTEX_POINT('',#118145);
#30675=VERTEX_POINT('',#118147);
#30676=VERTEX_POINT('',#118165);
#30677=VERTEX_POINT('',#118169);
#30678=VERTEX_POINT('',#118182);
#30679=VERTEX_POINT('',#118184);
#30680=VERTEX_POINT('',#118202);
#30681=VERTEX_POINT('',#118206);
#30682=VERTEX_POINT('',#118219);
#30683=VERTEX_POINT('',#118221);
#30684=VERTEX_POINT('',#118239);
#30685=VERTEX_POINT('',#118243);
#30686=VERTEX_POINT('',#118256);
#30687=VERTEX_POINT('',#118258);
#30688=VERTEX_POINT('',#118276);
#30689=VERTEX_POINT('',#118280);
#30690=VERTEX_POINT('',#118293);
#30691=VERTEX_POINT('',#118295);
#30692=VERTEX_POINT('',#118313);
#30693=VERTEX_POINT('',#118317);
#30694=VERTEX_POINT('',#118330);
#30695=VERTEX_POINT('',#118332);
#30696=VERTEX_POINT('',#118350);
#30697=VERTEX_POINT('',#118354);
#30698=VERTEX_POINT('',#118395);
#30699=VERTEX_POINT('',#118397);
#30700=VERTEX_POINT('',#118415);
#30701=VERTEX_POINT('',#118419);
#30702=VERTEX_POINT('',#118432);
#30703=VERTEX_POINT('',#118434);
#30704=VERTEX_POINT('',#118452);
#30705=VERTEX_POINT('',#118456);
#30706=VERTEX_POINT('',#118469);
#30707=VERTEX_POINT('',#118471);
#30708=VERTEX_POINT('',#118489);
#30709=VERTEX_POINT('',#118493);
#30710=VERTEX_POINT('',#118506);
#30711=VERTEX_POINT('',#118508);
#30712=VERTEX_POINT('',#118526);
#30713=VERTEX_POINT('',#118530);
#30714=VERTEX_POINT('',#118543);
#30715=VERTEX_POINT('',#118545);
#30716=VERTEX_POINT('',#118563);
#30717=VERTEX_POINT('',#118567);
#30718=VERTEX_POINT('',#118580);
#30719=VERTEX_POINT('',#118582);
#30720=VERTEX_POINT('',#118600);
#30721=VERTEX_POINT('',#118604);
#30722=VERTEX_POINT('',#118617);
#30723=VERTEX_POINT('',#118619);
#30724=VERTEX_POINT('',#118637);
#30725=VERTEX_POINT('',#118641);
#30726=VERTEX_POINT('',#118650);
#30727=VERTEX_POINT('',#118684);
#30728=VERTEX_POINT('',#118718);
#30729=VERTEX_POINT('',#118752);
#30730=VERTEX_POINT('',#118786);
#30731=VERTEX_POINT('',#118820);
#30732=VERTEX_POINT('',#118854);
#30733=VERTEX_POINT('',#118888);
#30734=VERTEX_POINT('',#118922);
#30735=VERTEX_POINT('',#118956);
#30736=VERTEX_POINT('',#118990);
#30737=VERTEX_POINT('',#119024);
#30738=VERTEX_POINT('',#119058);
#30739=VERTEX_POINT('',#119092);
#30740=VERTEX_POINT('',#119126);
#30741=VERTEX_POINT('',#119160);
#30742=VERTEX_POINT('',#119194);
#30743=VERTEX_POINT('',#119228);
#30744=VERTEX_POINT('',#119262);
#30745=VERTEX_POINT('',#119296);
#30746=VERTEX_POINT('',#119330);
#30747=VERTEX_POINT('',#119364);
#30748=VERTEX_POINT('',#119398);
#30749=VERTEX_POINT('',#119432);
#30750=VERTEX_POINT('',#119466);
#30751=VERTEX_POINT('',#119500);
#30752=VERTEX_POINT('',#119534);
#30753=VERTEX_POINT('',#119568);
#30754=VERTEX_POINT('',#119602);
#30755=VERTEX_POINT('',#119636);
#30756=VERTEX_POINT('',#119674);
#30757=VERTEX_POINT('',#119712);
#30758=VERTEX_POINT('',#119750);
#30759=VERTEX_POINT('',#119788);
#30760=VERTEX_POINT('',#119826);
#30761=VERTEX_POINT('',#119864);
#30762=VERTEX_POINT('',#119902);
#30763=VERTEX_POINT('',#119940);
#30764=VERTEX_POINT('',#119978);
#30765=VERTEX_POINT('',#120016);
#30766=VERTEX_POINT('',#120054);
#30767=VERTEX_POINT('',#120092);
#30768=VERTEX_POINT('',#120130);
#30769=VERTEX_POINT('',#120168);
#30770=VERTEX_POINT('',#120206);
#30771=VERTEX_POINT('',#120244);
#30772=VERTEX_POINT('',#120282);
#30773=VERTEX_POINT('',#120320);
#30774=VERTEX_POINT('',#120358);
#30775=VERTEX_POINT('',#120396);
#30776=VERTEX_POINT('',#120434);
#30777=VERTEX_POINT('',#120472);
#30778=VERTEX_POINT('',#120510);
#30779=VERTEX_POINT('',#120548);
#30780=VERTEX_POINT('',#120586);
#30781=VERTEX_POINT('',#120624);
#30782=VERTEX_POINT('',#120662);
#30783=VERTEX_POINT('',#120700);
#30784=VERTEX_POINT('',#120738);
#30785=VERTEX_POINT('',#120739);
#30786=VERTEX_POINT('',#120762);
#30787=VERTEX_POINT('',#120763);
#30788=VERTEX_POINT('',#120779);
#30789=VERTEX_POINT('',#120781);
#30790=VERTEX_POINT('',#120805);
#30791=VERTEX_POINT('',#120806);
#30792=VERTEX_POINT('',#120822);
#30793=VERTEX_POINT('',#120824);
#30794=VERTEX_POINT('',#120848);
#30795=VERTEX_POINT('',#120849);
#30796=VERTEX_POINT('',#120865);
#30797=VERTEX_POINT('',#120867);
#30798=VERTEX_POINT('',#120891);
#30799=VERTEX_POINT('',#120892);
#30800=VERTEX_POINT('',#120908);
#30801=VERTEX_POINT('',#120910);
#30802=VERTEX_POINT('',#120934);
#30803=VERTEX_POINT('',#120935);
#30804=VERTEX_POINT('',#120951);
#30805=VERTEX_POINT('',#120953);
#30806=VERTEX_POINT('',#120977);
#30807=VERTEX_POINT('',#120978);
#30808=VERTEX_POINT('',#120994);
#30809=VERTEX_POINT('',#120996);
#30810=VERTEX_POINT('',#121048);
#30811=VERTEX_POINT('',#121049);
#30812=VERTEX_POINT('',#121065);
#30813=VERTEX_POINT('',#121067);
#30814=VERTEX_POINT('',#121091);
#30815=VERTEX_POINT('',#121092);
#30816=VERTEX_POINT('',#121108);
#30817=VERTEX_POINT('',#121110);
#30818=VERTEX_POINT('',#121134);
#30819=VERTEX_POINT('',#121135);
#30820=VERTEX_POINT('',#121151);
#30821=VERTEX_POINT('',#121153);
#30822=VERTEX_POINT('',#121177);
#30823=VERTEX_POINT('',#121178);
#30824=VERTEX_POINT('',#121194);
#30825=VERTEX_POINT('',#121196);
#30826=VERTEX_POINT('',#121220);
#30827=VERTEX_POINT('',#121221);
#30828=VERTEX_POINT('',#121237);
#30829=VERTEX_POINT('',#121239);
#30830=VERTEX_POINT('',#121263);
#30831=VERTEX_POINT('',#121264);
#30832=VERTEX_POINT('',#121280);
#30833=VERTEX_POINT('',#121282);
#30834=VERTEX_POINT('',#121306);
#30835=VERTEX_POINT('',#121307);
#30836=VERTEX_POINT('',#121323);
#30837=VERTEX_POINT('',#121325);
#30838=VERTEX_POINT('',#121349);
#30839=VERTEX_POINT('',#121350);
#30840=VERTEX_POINT('',#121366);
#30841=VERTEX_POINT('',#121368);
#30842=VERTEX_POINT('',#121392);
#30843=VERTEX_POINT('',#121393);
#30844=VERTEX_POINT('',#121409);
#30845=VERTEX_POINT('',#121411);
#30846=VERTEX_POINT('',#121435);
#30847=VERTEX_POINT('',#121436);
#30848=VERTEX_POINT('',#121452);
#30849=VERTEX_POINT('',#121454);
#30850=VERTEX_POINT('',#121478);
#30851=VERTEX_POINT('',#121479);
#30852=VERTEX_POINT('',#121495);
#30853=VERTEX_POINT('',#121497);
#30854=VERTEX_POINT('',#121521);
#30855=VERTEX_POINT('',#121522);
#30856=VERTEX_POINT('',#121538);
#30857=VERTEX_POINT('',#121540);
#30858=VERTEX_POINT('',#121564);
#30859=VERTEX_POINT('',#121565);
#30860=VERTEX_POINT('',#121581);
#30861=VERTEX_POINT('',#121583);
#30862=VERTEX_POINT('',#121607);
#30863=VERTEX_POINT('',#121608);
#30864=VERTEX_POINT('',#121624);
#30865=VERTEX_POINT('',#121626);
#30866=VERTEX_POINT('',#121650);
#30867=VERTEX_POINT('',#121651);
#30868=VERTEX_POINT('',#121672);
#30869=VERTEX_POINT('',#121676);
#30870=VERTEX_POINT('',#121693);
#30871=VERTEX_POINT('',#121695);
#30872=VERTEX_POINT('',#121710);
#30873=VERTEX_POINT('',#121712);
#30874=VERTEX_POINT('',#121736);
#30875=VERTEX_POINT('',#121737);
#30876=VERTEX_POINT('',#121753);
#30877=VERTEX_POINT('',#121755);
#30878=VERTEX_POINT('',#121779);
#30879=VERTEX_POINT('',#121780);
#30880=VERTEX_POINT('',#121796);
#30881=VERTEX_POINT('',#121798);
#30882=VERTEX_POINT('',#121822);
#30883=VERTEX_POINT('',#121823);
#30884=VERTEX_POINT('',#121839);
#30885=VERTEX_POINT('',#121841);
#30886=VERTEX_POINT('',#121865);
#30887=VERTEX_POINT('',#121866);
#30888=VERTEX_POINT('',#121882);
#30889=VERTEX_POINT('',#121884);
#30890=VERTEX_POINT('',#121908);
#30891=VERTEX_POINT('',#121909);
#30892=VERTEX_POINT('',#121925);
#30893=VERTEX_POINT('',#121927);
#30894=VERTEX_POINT('',#121938);
#30895=VERTEX_POINT('',#121939);
#30896=VERTEX_POINT('',#121970);
#30897=VERTEX_POINT('',#121977);
#30898=VERTEX_POINT('',#121990);
#30899=VERTEX_POINT('',#121992);
#30900=VERTEX_POINT('',#122012);
#30901=VERTEX_POINT('',#122016);
#30902=VERTEX_POINT('',#122029);
#30903=VERTEX_POINT('',#122031);
#30904=VERTEX_POINT('',#122051);
#30905=VERTEX_POINT('',#122055);
#30906=VERTEX_POINT('',#122068);
#30907=VERTEX_POINT('',#122070);
#30908=VERTEX_POINT('',#122090);
#30909=VERTEX_POINT('',#122094);
#30910=VERTEX_POINT('',#122107);
#30911=VERTEX_POINT('',#122109);
#30912=VERTEX_POINT('',#122129);
#30913=VERTEX_POINT('',#122133);
#30914=VERTEX_POINT('',#122146);
#30915=VERTEX_POINT('',#122148);
#30916=VERTEX_POINT('',#122168);
#30917=VERTEX_POINT('',#122172);
#30918=VERTEX_POINT('',#122185);
#30919=VERTEX_POINT('',#122187);
#30920=VERTEX_POINT('',#122207);
#30921=VERTEX_POINT('',#122211);
#30922=VERTEX_POINT('',#122224);
#30923=VERTEX_POINT('',#122226);
#30924=VERTEX_POINT('',#122246);
#30925=VERTEX_POINT('',#122250);
#30926=VERTEX_POINT('',#122263);
#30927=VERTEX_POINT('',#122265);
#30928=VERTEX_POINT('',#122285);
#30929=VERTEX_POINT('',#122289);
#30930=VERTEX_POINT('',#122302);
#30931=VERTEX_POINT('',#122304);
#30932=VERTEX_POINT('',#122324);
#30933=VERTEX_POINT('',#122328);
#30934=VERTEX_POINT('',#122341);
#30935=VERTEX_POINT('',#122343);
#30936=VERTEX_POINT('',#122363);
#30937=VERTEX_POINT('',#122367);
#30938=VERTEX_POINT('',#122380);
#30939=VERTEX_POINT('',#122382);
#30940=VERTEX_POINT('',#122402);
#30941=VERTEX_POINT('',#122406);
#30942=VERTEX_POINT('',#122419);
#30943=VERTEX_POINT('',#122421);
#30944=VERTEX_POINT('',#122441);
#30945=VERTEX_POINT('',#122445);
#30946=VERTEX_POINT('',#122458);
#30947=VERTEX_POINT('',#122460);
#30948=VERTEX_POINT('',#122480);
#30949=VERTEX_POINT('',#122484);
#30950=VERTEX_POINT('',#122521);
#30951=VERTEX_POINT('',#122523);
#30952=VERTEX_POINT('',#122543);
#30953=VERTEX_POINT('',#122547);
#30954=VERTEX_POINT('',#122560);
#30955=VERTEX_POINT('',#122562);
#30956=VERTEX_POINT('',#122582);
#30957=VERTEX_POINT('',#122586);
#30958=VERTEX_POINT('',#122599);
#30959=VERTEX_POINT('',#122601);
#30960=VERTEX_POINT('',#122621);
#30961=VERTEX_POINT('',#122625);
#30962=VERTEX_POINT('',#122638);
#30963=VERTEX_POINT('',#122640);
#30964=VERTEX_POINT('',#122660);
#30965=VERTEX_POINT('',#122664);
#30966=VERTEX_POINT('',#122677);
#30967=VERTEX_POINT('',#122679);
#30968=VERTEX_POINT('',#122699);
#30969=VERTEX_POINT('',#122703);
#30970=VERTEX_POINT('',#122716);
#30971=VERTEX_POINT('',#122718);
#30972=VERTEX_POINT('',#122738);
#30973=VERTEX_POINT('',#122742);
#30974=VERTEX_POINT('',#122755);
#30975=VERTEX_POINT('',#122757);
#30976=VERTEX_POINT('',#122777);
#30977=VERTEX_POINT('',#122781);
#30978=VERTEX_POINT('',#122794);
#30979=VERTEX_POINT('',#122796);
#30980=VERTEX_POINT('',#122816);
#30981=VERTEX_POINT('',#122820);
#30982=VERTEX_POINT('',#122833);
#30983=VERTEX_POINT('',#122835);
#30984=VERTEX_POINT('',#122855);
#30985=VERTEX_POINT('',#122859);
#30986=VERTEX_POINT('',#122872);
#30987=VERTEX_POINT('',#122874);
#30988=VERTEX_POINT('',#122894);
#30989=VERTEX_POINT('',#122898);
#30990=VERTEX_POINT('',#122911);
#30991=VERTEX_POINT('',#122913);
#30992=VERTEX_POINT('',#122933);
#30993=VERTEX_POINT('',#122937);
#30994=VERTEX_POINT('',#122950);
#30995=VERTEX_POINT('',#122952);
#30996=VERTEX_POINT('',#122972);
#30997=VERTEX_POINT('',#122976);
#30998=VERTEX_POINT('',#122989);
#30999=VERTEX_POINT('',#122991);
#31000=VERTEX_POINT('',#123011);
#31001=VERTEX_POINT('',#123015);
#31002=VERTEX_POINT('',#123028);
#31003=VERTEX_POINT('',#123030);
#31004=VERTEX_POINT('',#123050);
#31005=VERTEX_POINT('',#123054);
#31006=VERTEX_POINT('',#123058);
#31007=VERTEX_POINT('',#123066);
#31008=VERTEX_POINT('',#123086);
#31009=VERTEX_POINT('',#123104);
#31010=VERTEX_POINT('',#123129);
#31011=VERTEX_POINT('',#123154);
#31012=VERTEX_POINT('',#123179);
#31013=VERTEX_POINT('',#123204);
#31014=VERTEX_POINT('',#123229);
#31015=VERTEX_POINT('',#123254);
#31016=VERTEX_POINT('',#123279);
#31017=VERTEX_POINT('',#123304);
#31018=VERTEX_POINT('',#123329);
#31019=VERTEX_POINT('',#123354);
#31020=VERTEX_POINT('',#123379);
#31021=VERTEX_POINT('',#123404);
#31022=VERTEX_POINT('',#123429);
#31023=VERTEX_POINT('',#123454);
#31024=VERTEX_POINT('',#123479);
#31025=VERTEX_POINT('',#123504);
#31026=VERTEX_POINT('',#123529);
#31027=VERTEX_POINT('',#123554);
#31028=VERTEX_POINT('',#123579);
#31029=VERTEX_POINT('',#123604);
#31030=VERTEX_POINT('',#123629);
#31031=VERTEX_POINT('',#123654);
#31032=VERTEX_POINT('',#123679);
#31033=VERTEX_POINT('',#123704);
#31034=VERTEX_POINT('',#123729);
#31035=VERTEX_POINT('',#123754);
#31036=VERTEX_POINT('',#123779);
#31037=VERTEX_POINT('',#123815);
#31038=VERTEX_POINT('',#123841);
#31039=VERTEX_POINT('',#123887);
#31040=VERTEX_POINT('',#123928);
#31041=VERTEX_POINT('',#123969);
#31042=VERTEX_POINT('',#124015);
#31043=VERTEX_POINT('',#124061);
#31044=VERTEX_POINT('',#124102);
#31045=VERTEX_POINT('',#124143);
#31046=VERTEX_POINT('',#124184);
#31047=VERTEX_POINT('',#124225);
#31048=VERTEX_POINT('',#124271);
#31049=VERTEX_POINT('',#124312);
#31050=VERTEX_POINT('',#124353);
#31051=VERTEX_POINT('',#124394);
#31052=VERTEX_POINT('',#124444);
#31053=VERTEX_POINT('',#124494);
#31054=VERTEX_POINT('',#124544);
#31055=VERTEX_POINT('',#124585);
#31056=VERTEX_POINT('',#124626);
#31057=VERTEX_POINT('',#124672);
#31058=VERTEX_POINT('',#124713);
#31059=VERTEX_POINT('',#124754);
#31060=VERTEX_POINT('',#124800);
#31061=VERTEX_POINT('',#124850);
#31062=VERTEX_POINT('',#124891);
#31063=VERTEX_POINT('',#124932);
#31064=VERTEX_POINT('',#124973);
#31065=VERTEX_POINT('',#125019);
#31066=VERTEX_POINT('',#125089);
#31067=VERTEX_POINT('',#125090);
#31068=VERTEX_POINT('',#125100);
#31069=VERTEX_POINT('',#125102);
#31070=VERTEX_POINT('',#125122);
#31071=VERTEX_POINT('',#125123);
#31072=VERTEX_POINT('',#125133);
#31073=VERTEX_POINT('',#125135);
#31074=VERTEX_POINT('',#125155);
#31075=VERTEX_POINT('',#125156);
#31076=VERTEX_POINT('',#125166);
#31077=VERTEX_POINT('',#125168);
#31078=VERTEX_POINT('',#125188);
#31079=VERTEX_POINT('',#125189);
#31080=VERTEX_POINT('',#125199);
#31081=VERTEX_POINT('',#125201);
#31082=VERTEX_POINT('',#125221);
#31083=VERTEX_POINT('',#125222);
#31084=VERTEX_POINT('',#125232);
#31085=VERTEX_POINT('',#125234);
#31086=VERTEX_POINT('',#125254);
#31087=VERTEX_POINT('',#125255);
#31088=VERTEX_POINT('',#125265);
#31089=VERTEX_POINT('',#125267);
#31090=VERTEX_POINT('',#125287);
#31091=VERTEX_POINT('',#125288);
#31092=VERTEX_POINT('',#125298);
#31093=VERTEX_POINT('',#125300);
#31094=VERTEX_POINT('',#125320);
#31095=VERTEX_POINT('',#125321);
#31096=VERTEX_POINT('',#125331);
#31097=VERTEX_POINT('',#125333);
#31098=VERTEX_POINT('',#125353);
#31099=VERTEX_POINT('',#125354);
#31100=VERTEX_POINT('',#125364);
#31101=VERTEX_POINT('',#125366);
#31102=VERTEX_POINT('',#125386);
#31103=VERTEX_POINT('',#125387);
#31104=VERTEX_POINT('',#125397);
#31105=VERTEX_POINT('',#125399);
#31106=VERTEX_POINT('',#125419);
#31107=VERTEX_POINT('',#125420);
#31108=VERTEX_POINT('',#125430);
#31109=VERTEX_POINT('',#125432);
#31110=VERTEX_POINT('',#125452);
#31111=VERTEX_POINT('',#125453);
#31112=VERTEX_POINT('',#125463);
#31113=VERTEX_POINT('',#125465);
#31114=VERTEX_POINT('',#125485);
#31115=VERTEX_POINT('',#125486);
#31116=VERTEX_POINT('',#125496);
#31117=VERTEX_POINT('',#125498);
#31118=VERTEX_POINT('',#125518);
#31119=VERTEX_POINT('',#125519);
#31120=VERTEX_POINT('',#125529);
#31121=VERTEX_POINT('',#125531);
#31122=VERTEX_POINT('',#125575);
#31123=VERTEX_POINT('',#125576);
#31124=VERTEX_POINT('',#125586);
#31125=VERTEX_POINT('',#125588);
#31126=VERTEX_POINT('',#125608);
#31127=VERTEX_POINT('',#125609);
#31128=VERTEX_POINT('',#125619);
#31129=VERTEX_POINT('',#125621);
#31130=VERTEX_POINT('',#125641);
#31131=VERTEX_POINT('',#125642);
#31132=VERTEX_POINT('',#125652);
#31133=VERTEX_POINT('',#125654);
#31134=VERTEX_POINT('',#125674);
#31135=VERTEX_POINT('',#125675);
#31136=VERTEX_POINT('',#125685);
#31137=VERTEX_POINT('',#125687);
#31138=VERTEX_POINT('',#125707);
#31139=VERTEX_POINT('',#125708);
#31140=VERTEX_POINT('',#125718);
#31141=VERTEX_POINT('',#125720);
#31142=VERTEX_POINT('',#125740);
#31143=VERTEX_POINT('',#125741);
#31144=VERTEX_POINT('',#125751);
#31145=VERTEX_POINT('',#125753);
#31146=VERTEX_POINT('',#125773);
#31147=VERTEX_POINT('',#125774);
#31148=VERTEX_POINT('',#125789);
#31149=VERTEX_POINT('',#125793);
#31150=VERTEX_POINT('',#125806);
#31151=VERTEX_POINT('',#125808);
#31152=VERTEX_POINT('',#125817);
#31153=VERTEX_POINT('',#125819);
#31154=VERTEX_POINT('',#125839);
#31155=VERTEX_POINT('',#125840);
#31156=VERTEX_POINT('',#125850);
#31157=VERTEX_POINT('',#125852);
#31158=VERTEX_POINT('',#125872);
#31159=VERTEX_POINT('',#125873);
#31160=VERTEX_POINT('',#125883);
#31161=VERTEX_POINT('',#125885);
#31162=VERTEX_POINT('',#125905);
#31163=VERTEX_POINT('',#125906);
#31164=VERTEX_POINT('',#125916);
#31165=VERTEX_POINT('',#125918);
#31166=VERTEX_POINT('',#125938);
#31167=VERTEX_POINT('',#125939);
#31168=VERTEX_POINT('',#125949);
#31169=VERTEX_POINT('',#125951);
#31170=VERTEX_POINT('',#125971);
#31171=VERTEX_POINT('',#125972);
#31172=VERTEX_POINT('',#125982);
#31173=VERTEX_POINT('',#125984);
#31174=VERTEX_POINT('',#126004);
#31175=VERTEX_POINT('',#126005);
#31176=VERTEX_POINT('',#126015);
#31177=VERTEX_POINT('',#126017);
#31178=VERTEX_POINT('',#126037);
#31179=VERTEX_POINT('',#126039);
#31180=VERTEX_POINT('',#126057);
#31181=VERTEX_POINT('',#126067);
#31182=VERTEX_POINT('',#126080);
#31183=VERTEX_POINT('',#126082);
#31184=VERTEX_POINT('',#126100);
#31185=VERTEX_POINT('',#126110);
#31186=VERTEX_POINT('',#126123);
#31187=VERTEX_POINT('',#126125);
#31188=VERTEX_POINT('',#126143);
#31189=VERTEX_POINT('',#126153);
#31190=VERTEX_POINT('',#126166);
#31191=VERTEX_POINT('',#126168);
#31192=VERTEX_POINT('',#126186);
#31193=VERTEX_POINT('',#126196);
#31194=VERTEX_POINT('',#126209);
#31195=VERTEX_POINT('',#126211);
#31196=VERTEX_POINT('',#126229);
#31197=VERTEX_POINT('',#126239);
#31198=VERTEX_POINT('',#126252);
#31199=VERTEX_POINT('',#126254);
#31200=VERTEX_POINT('',#126272);
#31201=VERTEX_POINT('',#126282);
#31202=VERTEX_POINT('',#126295);
#31203=VERTEX_POINT('',#126297);
#31204=VERTEX_POINT('',#126315);
#31205=VERTEX_POINT('',#126325);
#31206=VERTEX_POINT('',#126338);
#31207=VERTEX_POINT('',#126340);
#31208=VERTEX_POINT('',#126358);
#31209=VERTEX_POINT('',#126368);
#31210=VERTEX_POINT('',#126381);
#31211=VERTEX_POINT('',#126383);
#31212=VERTEX_POINT('',#126401);
#31213=VERTEX_POINT('',#126411);
#31214=VERTEX_POINT('',#126424);
#31215=VERTEX_POINT('',#126426);
#31216=VERTEX_POINT('',#126444);
#31217=VERTEX_POINT('',#126454);
#31218=VERTEX_POINT('',#126467);
#31219=VERTEX_POINT('',#126469);
#31220=VERTEX_POINT('',#126487);
#31221=VERTEX_POINT('',#126497);
#31222=VERTEX_POINT('',#126510);
#31223=VERTEX_POINT('',#126512);
#31224=VERTEX_POINT('',#126530);
#31225=VERTEX_POINT('',#126540);
#31226=VERTEX_POINT('',#126553);
#31227=VERTEX_POINT('',#126555);
#31228=VERTEX_POINT('',#126573);
#31229=VERTEX_POINT('',#126583);
#31230=VERTEX_POINT('',#126596);
#31231=VERTEX_POINT('',#126598);
#31232=VERTEX_POINT('',#126616);
#31233=VERTEX_POINT('',#126626);
#31234=VERTEX_POINT('',#126639);
#31235=VERTEX_POINT('',#126641);
#31236=VERTEX_POINT('',#126659);
#31237=VERTEX_POINT('',#126669);
#31238=VERTEX_POINT('',#126682);
#31239=VERTEX_POINT('',#126684);
#31240=VERTEX_POINT('',#126702);
#31241=VERTEX_POINT('',#126712);
#31242=VERTEX_POINT('',#126725);
#31243=VERTEX_POINT('',#126727);
#31244=VERTEX_POINT('',#126745);
#31245=VERTEX_POINT('',#126755);
#31246=VERTEX_POINT('',#126768);
#31247=VERTEX_POINT('',#126770);
#31248=VERTEX_POINT('',#126788);
#31249=VERTEX_POINT('',#126798);
#31250=VERTEX_POINT('',#126811);
#31251=VERTEX_POINT('',#126813);
#31252=VERTEX_POINT('',#126831);
#31253=VERTEX_POINT('',#126841);
#31254=VERTEX_POINT('',#126854);
#31255=VERTEX_POINT('',#126856);
#31256=VERTEX_POINT('',#126874);
#31257=VERTEX_POINT('',#126884);
#31258=VERTEX_POINT('',#126897);
#31259=VERTEX_POINT('',#126899);
#31260=VERTEX_POINT('',#126917);
#31261=VERTEX_POINT('',#126927);
#31262=VERTEX_POINT('',#126968);
#31263=VERTEX_POINT('',#126970);
#31264=VERTEX_POINT('',#126988);
#31265=VERTEX_POINT('',#126998);
#31266=VERTEX_POINT('',#127011);
#31267=VERTEX_POINT('',#127013);
#31268=VERTEX_POINT('',#127031);
#31269=VERTEX_POINT('',#127041);
#31270=VERTEX_POINT('',#127054);
#31271=VERTEX_POINT('',#127056);
#31272=VERTEX_POINT('',#127074);
#31273=VERTEX_POINT('',#127084);
#31274=VERTEX_POINT('',#127097);
#31275=VERTEX_POINT('',#127099);
#31276=VERTEX_POINT('',#127117);
#31277=VERTEX_POINT('',#127127);
#31278=VERTEX_POINT('',#127140);
#31279=VERTEX_POINT('',#127142);
#31280=VERTEX_POINT('',#127160);
#31281=VERTEX_POINT('',#127170);
#31282=VERTEX_POINT('',#127183);
#31283=VERTEX_POINT('',#127185);
#31284=VERTEX_POINT('',#127203);
#31285=VERTEX_POINT('',#127213);
#31286=VERTEX_POINT('',#127226);
#31287=VERTEX_POINT('',#127228);
#31288=VERTEX_POINT('',#127246);
#31289=VERTEX_POINT('',#127256);
#31290=VERTEX_POINT('',#127269);
#31291=VERTEX_POINT('',#127294);
#31292=VERTEX_POINT('',#127319);
#31293=VERTEX_POINT('',#127344);
#31294=VERTEX_POINT('',#127369);
#31295=VERTEX_POINT('',#127394);
#31296=VERTEX_POINT('',#127419);
#31297=VERTEX_POINT('',#127444);
#31298=VERTEX_POINT('',#127469);
#31299=VERTEX_POINT('',#127494);
#31300=VERTEX_POINT('',#127519);
#31301=VERTEX_POINT('',#127544);
#31302=VERTEX_POINT('',#127569);
#31303=VERTEX_POINT('',#127594);
#31304=VERTEX_POINT('',#127619);
#31305=VERTEX_POINT('',#127644);
#31306=VERTEX_POINT('',#127669);
#31307=VERTEX_POINT('',#127694);
#31308=VERTEX_POINT('',#127719);
#31309=VERTEX_POINT('',#127744);
#31310=VERTEX_POINT('',#127769);
#31311=VERTEX_POINT('',#127794);
#31312=VERTEX_POINT('',#127819);
#31313=VERTEX_POINT('',#127844);
#31314=VERTEX_POINT('',#127869);
#31315=VERTEX_POINT('',#127894);
#31316=VERTEX_POINT('',#127919);
#31317=VERTEX_POINT('',#127944);
#31318=VERTEX_POINT('',#127969);
#31319=VERTEX_POINT('',#127994);
#31320=VERTEX_POINT('',#128019);
#31321=VERTEX_POINT('',#128044);
#31322=VERTEX_POINT('',#128069);
#31323=VERTEX_POINT('',#128094);
#31324=VERTEX_POINT('',#128119);
#31325=VERTEX_POINT('',#128144);
#31326=VERTEX_POINT('',#128169);
#31327=VERTEX_POINT('',#128194);
#31328=VERTEX_POINT('',#128219);
#31329=VERTEX_POINT('',#128244);
#31330=VERTEX_POINT('',#128269);
#31331=VERTEX_POINT('',#128294);
#31332=VERTEX_POINT('',#128319);
#31333=VERTEX_POINT('',#128344);
#31334=VERTEX_POINT('',#128369);
#31335=VERTEX_POINT('',#128394);
#31336=VERTEX_POINT('',#128419);
#31337=VERTEX_POINT('',#128444);
#31338=VERTEX_POINT('',#128469);
#31339=VERTEX_POINT('',#128494);
#31340=VERTEX_POINT('',#128519);
#31341=VERTEX_POINT('',#128544);
#31342=VERTEX_POINT('',#128569);
#31343=VERTEX_POINT('',#128594);
#31344=VERTEX_POINT('',#128619);
#31345=VERTEX_POINT('',#128644);
#31346=VERTEX_POINT('',#128669);
#31347=VERTEX_POINT('',#128694);
#31348=VERTEX_POINT('',#128719);
#31349=VERTEX_POINT('',#128720);
#31350=VERTEX_POINT('',#128739);
#31351=VERTEX_POINT('',#128740);
#31352=VERTEX_POINT('',#128750);
#31353=VERTEX_POINT('',#128752);
#31354=VERTEX_POINT('',#128776);
#31355=VERTEX_POINT('',#128777);
#31356=VERTEX_POINT('',#128787);
#31357=VERTEX_POINT('',#128789);
#31358=VERTEX_POINT('',#128813);
#31359=VERTEX_POINT('',#128814);
#31360=VERTEX_POINT('',#128824);
#31361=VERTEX_POINT('',#128826);
#31362=VERTEX_POINT('',#128850);
#31363=VERTEX_POINT('',#128851);
#31364=VERTEX_POINT('',#128861);
#31365=VERTEX_POINT('',#128863);
#31366=VERTEX_POINT('',#128887);
#31367=VERTEX_POINT('',#128888);
#31368=VERTEX_POINT('',#128898);
#31369=VERTEX_POINT('',#128900);
#31370=VERTEX_POINT('',#128924);
#31371=VERTEX_POINT('',#128925);
#31372=VERTEX_POINT('',#128935);
#31373=VERTEX_POINT('',#128937);
#31374=VERTEX_POINT('',#128989);
#31375=VERTEX_POINT('',#128990);
#31376=VERTEX_POINT('',#129000);
#31377=VERTEX_POINT('',#129002);
#31378=VERTEX_POINT('',#129026);
#31379=VERTEX_POINT('',#129027);
#31380=VERTEX_POINT('',#129037);
#31381=VERTEX_POINT('',#129039);
#31382=VERTEX_POINT('',#129063);
#31383=VERTEX_POINT('',#129064);
#31384=VERTEX_POINT('',#129074);
#31385=VERTEX_POINT('',#129076);
#31386=VERTEX_POINT('',#129100);
#31387=VERTEX_POINT('',#129101);
#31388=VERTEX_POINT('',#129111);
#31389=VERTEX_POINT('',#129113);
#31390=VERTEX_POINT('',#129137);
#31391=VERTEX_POINT('',#129138);
#31392=VERTEX_POINT('',#129148);
#31393=VERTEX_POINT('',#129150);
#31394=VERTEX_POINT('',#129174);
#31395=VERTEX_POINT('',#129175);
#31396=VERTEX_POINT('',#129185);
#31397=VERTEX_POINT('',#129187);
#31398=VERTEX_POINT('',#129211);
#31399=VERTEX_POINT('',#129212);
#31400=VERTEX_POINT('',#129222);
#31401=VERTEX_POINT('',#129224);
#31402=VERTEX_POINT('',#129248);
#31403=VERTEX_POINT('',#129249);
#31404=VERTEX_POINT('',#129259);
#31405=VERTEX_POINT('',#129261);
#31406=VERTEX_POINT('',#129285);
#31407=VERTEX_POINT('',#129286);
#31408=VERTEX_POINT('',#129296);
#31409=VERTEX_POINT('',#129298);
#31410=VERTEX_POINT('',#129322);
#31411=VERTEX_POINT('',#129323);
#31412=VERTEX_POINT('',#129333);
#31413=VERTEX_POINT('',#129335);
#31414=VERTEX_POINT('',#129359);
#31415=VERTEX_POINT('',#129360);
#31416=VERTEX_POINT('',#129370);
#31417=VERTEX_POINT('',#129372);
#31418=VERTEX_POINT('',#129396);
#31419=VERTEX_POINT('',#129397);
#31420=VERTEX_POINT('',#129407);
#31421=VERTEX_POINT('',#129409);
#31422=VERTEX_POINT('',#129433);
#31423=VERTEX_POINT('',#129434);
#31424=VERTEX_POINT('',#129444);
#31425=VERTEX_POINT('',#129446);
#31426=VERTEX_POINT('',#129470);
#31427=VERTEX_POINT('',#129471);
#31428=VERTEX_POINT('',#129490);
#31429=VERTEX_POINT('',#129494);
#31430=VERTEX_POINT('',#129507);
#31431=VERTEX_POINT('',#129509);
#31432=VERTEX_POINT('',#129518);
#31433=VERTEX_POINT('',#129520);
#31434=VERTEX_POINT('',#129544);
#31435=VERTEX_POINT('',#129545);
#31436=VERTEX_POINT('',#129555);
#31437=VERTEX_POINT('',#129557);
#31438=VERTEX_POINT('',#129581);
#31439=VERTEX_POINT('',#129582);
#31440=VERTEX_POINT('',#129592);
#31441=VERTEX_POINT('',#129594);
#31442=VERTEX_POINT('',#129618);
#31443=VERTEX_POINT('',#129619);
#31444=VERTEX_POINT('',#129629);
#31445=VERTEX_POINT('',#129631);
#31446=VERTEX_POINT('',#129655);
#31447=VERTEX_POINT('',#129656);
#31448=VERTEX_POINT('',#129666);
#31449=VERTEX_POINT('',#129668);
#31450=VERTEX_POINT('',#129692);
#31451=VERTEX_POINT('',#129693);
#31452=VERTEX_POINT('',#129703);
#31453=VERTEX_POINT('',#129705);
#31454=VERTEX_POINT('',#129729);
#31455=VERTEX_POINT('',#129730);
#31456=VERTEX_POINT('',#129740);
#31457=VERTEX_POINT('',#129742);
#31458=VERTEX_POINT('',#129757);
#31459=VERTEX_POINT('',#129758);
#31460=VERTEX_POINT('',#129779);
#31461=VERTEX_POINT('',#129786);
#31462=VERTEX_POINT('',#129799);
#31463=VERTEX_POINT('',#129801);
#31464=VERTEX_POINT('',#129815);
#31465=VERTEX_POINT('',#129819);
#31466=VERTEX_POINT('',#129832);
#31467=VERTEX_POINT('',#129834);
#31468=VERTEX_POINT('',#129848);
#31469=VERTEX_POINT('',#129852);
#31470=VERTEX_POINT('',#129865);
#31471=VERTEX_POINT('',#129867);
#31472=VERTEX_POINT('',#129881);
#31473=VERTEX_POINT('',#129885);
#31474=VERTEX_POINT('',#129898);
#31475=VERTEX_POINT('',#129900);
#31476=VERTEX_POINT('',#129914);
#31477=VERTEX_POINT('',#129918);
#31478=VERTEX_POINT('',#129931);
#31479=VERTEX_POINT('',#129933);
#31480=VERTEX_POINT('',#129947);
#31481=VERTEX_POINT('',#129951);
#31482=VERTEX_POINT('',#129964);
#31483=VERTEX_POINT('',#129966);
#31484=VERTEX_POINT('',#129980);
#31485=VERTEX_POINT('',#129984);
#31486=VERTEX_POINT('',#129997);
#31487=VERTEX_POINT('',#129999);
#31488=VERTEX_POINT('',#130013);
#31489=VERTEX_POINT('',#130017);
#31490=VERTEX_POINT('',#130030);
#31491=VERTEX_POINT('',#130032);
#31492=VERTEX_POINT('',#130046);
#31493=VERTEX_POINT('',#130050);
#31494=VERTEX_POINT('',#130063);
#31495=VERTEX_POINT('',#130065);
#31496=VERTEX_POINT('',#130079);
#31497=VERTEX_POINT('',#130083);
#31498=VERTEX_POINT('',#130096);
#31499=VERTEX_POINT('',#130098);
#31500=VERTEX_POINT('',#130112);
#31501=VERTEX_POINT('',#130116);
#31502=VERTEX_POINT('',#130129);
#31503=VERTEX_POINT('',#130131);
#31504=VERTEX_POINT('',#130145);
#31505=VERTEX_POINT('',#130149);
#31506=VERTEX_POINT('',#130162);
#31507=VERTEX_POINT('',#130164);
#31508=VERTEX_POINT('',#130178);
#31509=VERTEX_POINT('',#130182);
#31510=VERTEX_POINT('',#130195);
#31511=VERTEX_POINT('',#130197);
#31512=VERTEX_POINT('',#130211);
#31513=VERTEX_POINT('',#130215);
#31514=VERTEX_POINT('',#130252);
#31515=VERTEX_POINT('',#130254);
#31516=VERTEX_POINT('',#130268);
#31517=VERTEX_POINT('',#130272);
#31518=VERTEX_POINT('',#130285);
#31519=VERTEX_POINT('',#130287);
#31520=VERTEX_POINT('',#130301);
#31521=VERTEX_POINT('',#130305);
#31522=VERTEX_POINT('',#130318);
#31523=VERTEX_POINT('',#130320);
#31524=VERTEX_POINT('',#130334);
#31525=VERTEX_POINT('',#130338);
#31526=VERTEX_POINT('',#130351);
#31527=VERTEX_POINT('',#130353);
#31528=VERTEX_POINT('',#130367);
#31529=VERTEX_POINT('',#130371);
#31530=VERTEX_POINT('',#130384);
#31531=VERTEX_POINT('',#130386);
#31532=VERTEX_POINT('',#130400);
#31533=VERTEX_POINT('',#130404);
#31534=VERTEX_POINT('',#130417);
#31535=VERTEX_POINT('',#130419);
#31536=VERTEX_POINT('',#130433);
#31537=VERTEX_POINT('',#130437);
#31538=VERTEX_POINT('',#130450);
#31539=VERTEX_POINT('',#130452);
#31540=VERTEX_POINT('',#130466);
#31541=VERTEX_POINT('',#130470);
#31542=VERTEX_POINT('',#130483);
#31543=VERTEX_POINT('',#130485);
#31544=VERTEX_POINT('',#130499);
#31545=VERTEX_POINT('',#130503);
#31546=VERTEX_POINT('',#130516);
#31547=VERTEX_POINT('',#130518);
#31548=VERTEX_POINT('',#130532);
#31549=VERTEX_POINT('',#130536);
#31550=VERTEX_POINT('',#130549);
#31551=VERTEX_POINT('',#130551);
#31552=VERTEX_POINT('',#130565);
#31553=VERTEX_POINT('',#130569);
#31554=VERTEX_POINT('',#130582);
#31555=VERTEX_POINT('',#130584);
#31556=VERTEX_POINT('',#130598);
#31557=VERTEX_POINT('',#130602);
#31558=VERTEX_POINT('',#130615);
#31559=VERTEX_POINT('',#130617);
#31560=VERTEX_POINT('',#130631);
#31561=VERTEX_POINT('',#130635);
#31562=VERTEX_POINT('',#130648);
#31563=VERTEX_POINT('',#130650);
#31564=VERTEX_POINT('',#130664);
#31565=VERTEX_POINT('',#130668);
#31566=VERTEX_POINT('',#130681);
#31567=VERTEX_POINT('',#130683);
#31568=VERTEX_POINT('',#130697);
#31569=VERTEX_POINT('',#130701);
#31570=VERTEX_POINT('',#130705);
#31571=VERTEX_POINT('',#130707);
#31572=VERTEX_POINT('',#130727);
#31573=VERTEX_POINT('',#130749);
#31574=VERTEX_POINT('',#130787);
#31575=VERTEX_POINT('',#130825);
#31576=VERTEX_POINT('',#130863);
#31577=VERTEX_POINT('',#130901);
#31578=VERTEX_POINT('',#130939);
#31579=VERTEX_POINT('',#130977);
#31580=VERTEX_POINT('',#131015);
#31581=VERTEX_POINT('',#131053);
#31582=VERTEX_POINT('',#131091);
#31583=VERTEX_POINT('',#131129);
#31584=VERTEX_POINT('',#131167);
#31585=VERTEX_POINT('',#131205);
#31586=VERTEX_POINT('',#131243);
#31587=VERTEX_POINT('',#131281);
#31588=VERTEX_POINT('',#131319);
#31589=VERTEX_POINT('',#131357);
#31590=VERTEX_POINT('',#131395);
#31591=VERTEX_POINT('',#131433);
#31592=VERTEX_POINT('',#131471);
#31593=VERTEX_POINT('',#131509);
#31594=VERTEX_POINT('',#131547);
#31595=VERTEX_POINT('',#131585);
#31596=VERTEX_POINT('',#131623);
#31597=VERTEX_POINT('',#131661);
#31598=VERTEX_POINT('',#131699);
#31599=VERTEX_POINT('',#131737);
#31600=VERTEX_POINT('',#131775);
#31601=VERTEX_POINT('',#131829);
#31602=VERTEX_POINT('',#131847);
#31603=VERTEX_POINT('',#131875);
#31604=VERTEX_POINT('',#131903);
#31605=VERTEX_POINT('',#131931);
#31606=VERTEX_POINT('',#131959);
#31607=VERTEX_POINT('',#131987);
#31608=VERTEX_POINT('',#132015);
#31609=VERTEX_POINT('',#132043);
#31610=VERTEX_POINT('',#132071);
#31611=VERTEX_POINT('',#132099);
#31612=VERTEX_POINT('',#132127);
#31613=VERTEX_POINT('',#132155);
#31614=VERTEX_POINT('',#132183);
#31615=VERTEX_POINT('',#132211);
#31616=VERTEX_POINT('',#132239);
#31617=VERTEX_POINT('',#132267);
#31618=VERTEX_POINT('',#132295);
#31619=VERTEX_POINT('',#132323);
#31620=VERTEX_POINT('',#132351);
#31621=VERTEX_POINT('',#132379);
#31622=VERTEX_POINT('',#132407);
#31623=VERTEX_POINT('',#132435);
#31624=VERTEX_POINT('',#132463);
#31625=VERTEX_POINT('',#132491);
#31626=VERTEX_POINT('',#132519);
#31627=VERTEX_POINT('',#132547);
#31628=VERTEX_POINT('',#132575);
#31629=VERTEX_POINT('',#132603);
#31630=VERTEX_POINT('',#132643);
#31631=VERTEX_POINT('',#132644);
#31632=VERTEX_POINT('',#132654);
#31633=VERTEX_POINT('',#132656);
#31634=VERTEX_POINT('',#132682);
#31635=VERTEX_POINT('',#132683);
#31636=VERTEX_POINT('',#132693);
#31637=VERTEX_POINT('',#132695);
#31638=VERTEX_POINT('',#132721);
#31639=VERTEX_POINT('',#132722);
#31640=VERTEX_POINT('',#132732);
#31641=VERTEX_POINT('',#132734);
#31642=VERTEX_POINT('',#132760);
#31643=VERTEX_POINT('',#132761);
#31644=VERTEX_POINT('',#132771);
#31645=VERTEX_POINT('',#132773);
#31646=VERTEX_POINT('',#132799);
#31647=VERTEX_POINT('',#132800);
#31648=VERTEX_POINT('',#132810);
#31649=VERTEX_POINT('',#132812);
#31650=VERTEX_POINT('',#132838);
#31651=VERTEX_POINT('',#132839);
#31652=VERTEX_POINT('',#132849);
#31653=VERTEX_POINT('',#132851);
#31654=VERTEX_POINT('',#132877);
#31655=VERTEX_POINT('',#132878);
#31656=VERTEX_POINT('',#132888);
#31657=VERTEX_POINT('',#132890);
#31658=VERTEX_POINT('',#132916);
#31659=VERTEX_POINT('',#132917);
#31660=VERTEX_POINT('',#132927);
#31661=VERTEX_POINT('',#132929);
#31662=VERTEX_POINT('',#132955);
#31663=VERTEX_POINT('',#132956);
#31664=VERTEX_POINT('',#132966);
#31665=VERTEX_POINT('',#132968);
#31666=VERTEX_POINT('',#132992);
#31667=VERTEX_POINT('',#132993);
#31668=VERTEX_POINT('',#133003);
#31669=VERTEX_POINT('',#133005);
#31670=VERTEX_POINT('',#133031);
#31671=VERTEX_POINT('',#133032);
#31672=VERTEX_POINT('',#133042);
#31673=VERTEX_POINT('',#133044);
#31674=VERTEX_POINT('',#133070);
#31675=VERTEX_POINT('',#133071);
#31676=VERTEX_POINT('',#133081);
#31677=VERTEX_POINT('',#133083);
#31678=VERTEX_POINT('',#133109);
#31679=VERTEX_POINT('',#133110);
#31680=VERTEX_POINT('',#133120);
#31681=VERTEX_POINT('',#133122);
#31682=VERTEX_POINT('',#133148);
#31683=VERTEX_POINT('',#133149);
#31684=VERTEX_POINT('',#133159);
#31685=VERTEX_POINT('',#133161);
#31686=VERTEX_POINT('',#133211);
#31687=VERTEX_POINT('',#133212);
#31688=VERTEX_POINT('',#133222);
#31689=VERTEX_POINT('',#133224);
#31690=VERTEX_POINT('',#133250);
#31691=VERTEX_POINT('',#133251);
#31692=VERTEX_POINT('',#133261);
#31693=VERTEX_POINT('',#133263);
#31694=VERTEX_POINT('',#133289);
#31695=VERTEX_POINT('',#133290);
#31696=VERTEX_POINT('',#133300);
#31697=VERTEX_POINT('',#133302);
#31698=VERTEX_POINT('',#133328);
#31699=VERTEX_POINT('',#133329);
#31700=VERTEX_POINT('',#133339);
#31701=VERTEX_POINT('',#133341);
#31702=VERTEX_POINT('',#133367);
#31703=VERTEX_POINT('',#133368);
#31704=VERTEX_POINT('',#133378);
#31705=VERTEX_POINT('',#133380);
#31706=VERTEX_POINT('',#133406);
#31707=VERTEX_POINT('',#133407);
#31708=VERTEX_POINT('',#133426);
#31709=VERTEX_POINT('',#133436);
#31710=VERTEX_POINT('',#133445);
#31711=VERTEX_POINT('',#133447);
#31712=VERTEX_POINT('',#133456);
#31713=VERTEX_POINT('',#133464);
#31714=VERTEX_POINT('',#133484);
#31715=VERTEX_POINT('',#133485);
#31716=VERTEX_POINT('',#133495);
#31717=VERTEX_POINT('',#133497);
#31718=VERTEX_POINT('',#133523);
#31719=VERTEX_POINT('',#133524);
#31720=VERTEX_POINT('',#133534);
#31721=VERTEX_POINT('',#133536);
#31722=VERTEX_POINT('',#133562);
#31723=VERTEX_POINT('',#133563);
#31724=VERTEX_POINT('',#133573);
#31725=VERTEX_POINT('',#133575);
#31726=VERTEX_POINT('',#133601);
#31727=VERTEX_POINT('',#133602);
#31728=VERTEX_POINT('',#133612);
#31729=VERTEX_POINT('',#133614);
#31730=VERTEX_POINT('',#133640);
#31731=VERTEX_POINT('',#133641);
#31732=VERTEX_POINT('',#133651);
#31733=VERTEX_POINT('',#133653);
#31734=VERTEX_POINT('',#133679);
#31735=VERTEX_POINT('',#133680);
#31736=VERTEX_POINT('',#133690);
#31737=VERTEX_POINT('',#133692);
#31738=VERTEX_POINT('',#133718);
#31739=VERTEX_POINT('',#133719);
#31740=VERTEX_POINT('',#133729);
#31741=VERTEX_POINT('',#133731);
#31742=VERTEX_POINT('',#133757);
#31743=VERTEX_POINT('',#133759);
#31744=VERTEX_POINT('',#133773);
#31745=VERTEX_POINT('',#133777);
#31746=VERTEX_POINT('',#133786);
#31747=VERTEX_POINT('',#133788);
#31748=VERTEX_POINT('',#133802);
#31749=VERTEX_POINT('',#133806);
#31750=VERTEX_POINT('',#133815);
#31751=VERTEX_POINT('',#133817);
#31752=VERTEX_POINT('',#133831);
#31753=VERTEX_POINT('',#133835);
#31754=VERTEX_POINT('',#133844);
#31755=VERTEX_POINT('',#133846);
#31756=VERTEX_POINT('',#133860);
#31757=VERTEX_POINT('',#133864);
#31758=VERTEX_POINT('',#133873);
#31759=VERTEX_POINT('',#133875);
#31760=VERTEX_POINT('',#133889);
#31761=VERTEX_POINT('',#133893);
#31762=VERTEX_POINT('',#133902);
#31763=VERTEX_POINT('',#133904);
#31764=VERTEX_POINT('',#133918);
#31765=VERTEX_POINT('',#133922);
#31766=VERTEX_POINT('',#133931);
#31767=VERTEX_POINT('',#133933);
#31768=VERTEX_POINT('',#133947);
#31769=VERTEX_POINT('',#133951);
#31770=VERTEX_POINT('',#133960);
#31771=VERTEX_POINT('',#133962);
#31772=VERTEX_POINT('',#133976);
#31773=VERTEX_POINT('',#133980);
#31774=VERTEX_POINT('',#133989);
#31775=VERTEX_POINT('',#133991);
#31776=VERTEX_POINT('',#134005);
#31777=VERTEX_POINT('',#134009);
#31778=VERTEX_POINT('',#134018);
#31779=VERTEX_POINT('',#134020);
#31780=VERTEX_POINT('',#134034);
#31781=VERTEX_POINT('',#134038);
#31782=VERTEX_POINT('',#134047);
#31783=VERTEX_POINT('',#134049);
#31784=VERTEX_POINT('',#134063);
#31785=VERTEX_POINT('',#134067);
#31786=VERTEX_POINT('',#134076);
#31787=VERTEX_POINT('',#134078);
#31788=VERTEX_POINT('',#134092);
#31789=VERTEX_POINT('',#134096);
#31790=VERTEX_POINT('',#134105);
#31791=VERTEX_POINT('',#134107);
#31792=VERTEX_POINT('',#134121);
#31793=VERTEX_POINT('',#134125);
#31794=VERTEX_POINT('',#134134);
#31795=VERTEX_POINT('',#134136);
#31796=VERTEX_POINT('',#134150);
#31797=VERTEX_POINT('',#134154);
#31798=VERTEX_POINT('',#134163);
#31799=VERTEX_POINT('',#134165);
#31800=VERTEX_POINT('',#134179);
#31801=VERTEX_POINT('',#134183);
#31802=VERTEX_POINT('',#134192);
#31803=VERTEX_POINT('',#134194);
#31804=VERTEX_POINT('',#134208);
#31805=VERTEX_POINT('',#134212);
#31806=VERTEX_POINT('',#134221);
#31807=VERTEX_POINT('',#134223);
#31808=VERTEX_POINT('',#134237);
#31809=VERTEX_POINT('',#134241);
#31810=VERTEX_POINT('',#134250);
#31811=VERTEX_POINT('',#134252);
#31812=VERTEX_POINT('',#134266);
#31813=VERTEX_POINT('',#134270);
#31814=VERTEX_POINT('',#134279);
#31815=VERTEX_POINT('',#134281);
#31816=VERTEX_POINT('',#134295);
#31817=VERTEX_POINT('',#134299);
#31818=VERTEX_POINT('',#134308);
#31819=VERTEX_POINT('',#134310);
#31820=VERTEX_POINT('',#134324);
#31821=VERTEX_POINT('',#134328);
#31822=VERTEX_POINT('',#134337);
#31823=VERTEX_POINT('',#134339);
#31824=VERTEX_POINT('',#134353);
#31825=VERTEX_POINT('',#134357);
#31826=VERTEX_POINT('',#134366);
#31827=VERTEX_POINT('',#134368);
#31828=VERTEX_POINT('',#134382);
#31829=VERTEX_POINT('',#134386);
#31830=VERTEX_POINT('',#134395);
#31831=VERTEX_POINT('',#134397);
#31832=VERTEX_POINT('',#134411);
#31833=VERTEX_POINT('',#134415);
#31834=VERTEX_POINT('',#134424);
#31835=VERTEX_POINT('',#134426);
#31836=VERTEX_POINT('',#134440);
#31837=VERTEX_POINT('',#134444);
#31838=VERTEX_POINT('',#134453);
#31839=VERTEX_POINT('',#134455);
#31840=VERTEX_POINT('',#134469);
#31841=VERTEX_POINT('',#134473);
#31842=VERTEX_POINT('',#134482);
#31843=VERTEX_POINT('',#134484);
#31844=VERTEX_POINT('',#134498);
#31845=VERTEX_POINT('',#134502);
#31846=VERTEX_POINT('',#134511);
#31847=VERTEX_POINT('',#134513);
#31848=VERTEX_POINT('',#134527);
#31849=VERTEX_POINT('',#134531);
#31850=VERTEX_POINT('',#134540);
#31851=VERTEX_POINT('',#134542);
#31852=VERTEX_POINT('',#134556);
#31853=VERTEX_POINT('',#134560);
#31854=VERTEX_POINT('',#134569);
#31855=VERTEX_POINT('',#134571);
#31856=VERTEX_POINT('',#134585);
#31857=VERTEX_POINT('',#134589);
#31858=VERTEX_POINT('',#134602);
#31859=VERTEX_POINT('',#134648);
#31860=VERTEX_POINT('',#134694);
#31861=VERTEX_POINT('',#134740);
#31862=VERTEX_POINT('',#134786);
#31863=VERTEX_POINT('',#134832);
#31864=VERTEX_POINT('',#134882);
#31865=VERTEX_POINT('',#134928);
#31866=VERTEX_POINT('',#134974);
#31867=VERTEX_POINT('',#135020);
#31868=VERTEX_POINT('',#135066);
#31869=VERTEX_POINT('',#135112);
#31870=VERTEX_POINT('',#135158);
#31871=VERTEX_POINT('',#135208);
#31872=VERTEX_POINT('',#135258);
#31873=VERTEX_POINT('',#135308);
#31874=VERTEX_POINT('',#135354);
#31875=VERTEX_POINT('',#135400);
#31876=VERTEX_POINT('',#135446);
#31877=VERTEX_POINT('',#135492);
#31878=VERTEX_POINT('',#135538);
#31879=VERTEX_POINT('',#135584);
#31880=VERTEX_POINT('',#135630);
#31881=VERTEX_POINT('',#135676);
#31882=VERTEX_POINT('',#135722);
#31883=VERTEX_POINT('',#135768);
#31884=VERTEX_POINT('',#135814);
#31885=VERTEX_POINT('',#135860);
#31886=VERTEX_POINT('',#135906);
#31887=VERTEX_POINT('',#135956);
#31888=VERTEX_POINT('',#136006);
#31889=VERTEX_POINT('',#136052);
#31890=VERTEX_POINT('',#136102);
#31891=VERTEX_POINT('',#136151);
#31892=VERTEX_POINT('',#136201);
#31893=VERTEX_POINT('',#136247);
#31894=VERTEX_POINT('',#136297);
#31895=VERTEX_POINT('',#136343);
#31896=VERTEX_POINT('',#136389);
#31897=VERTEX_POINT('',#136439);
#31898=VERTEX_POINT('',#136480);
#31899=VERTEX_POINT('',#136521);
#31900=VERTEX_POINT('',#136567);
#31901=VERTEX_POINT('',#136617);
#31902=VERTEX_POINT('',#136663);
#31903=VERTEX_POINT('',#136707);
#31904=VERTEX_POINT('',#136757);
#31905=VERTEX_POINT('',#136798);
#31906=VERTEX_POINT('',#136848);
#31907=VERTEX_POINT('',#136897);
#31908=VERTEX_POINT('',#136946);
#31909=VERTEX_POINT('',#136996);
#31910=VERTEX_POINT('',#137046);
#31911=VERTEX_POINT('',#137087);
#31912=VERTEX_POINT('',#137128);
#31913=VERTEX_POINT('',#137178);
#31914=VERTEX_POINT('',#137219);
#31915=VERTEX_POINT('',#137265);
#31916=VERTEX_POINT('',#137318);
#31917=VERTEX_POINT('',#137319);
#31918=VERTEX_POINT('',#137338);
#31919=VERTEX_POINT('',#137339);
#31920=VERTEX_POINT('',#137355);
#31921=VERTEX_POINT('',#137357);
#31922=VERTEX_POINT('',#137381);
#31923=VERTEX_POINT('',#137382);
#31924=VERTEX_POINT('',#137398);
#31925=VERTEX_POINT('',#137400);
#31926=VERTEX_POINT('',#137424);
#31927=VERTEX_POINT('',#137425);
#31928=VERTEX_POINT('',#137441);
#31929=VERTEX_POINT('',#137443);
#31930=VERTEX_POINT('',#137467);
#31931=VERTEX_POINT('',#137468);
#31932=VERTEX_POINT('',#137484);
#31933=VERTEX_POINT('',#137486);
#31934=VERTEX_POINT('',#137510);
#31935=VERTEX_POINT('',#137511);
#31936=VERTEX_POINT('',#137527);
#31937=VERTEX_POINT('',#137529);
#31938=VERTEX_POINT('',#137553);
#31939=VERTEX_POINT('',#137554);
#31940=VERTEX_POINT('',#137570);
#31941=VERTEX_POINT('',#137572);
#31942=VERTEX_POINT('',#137624);
#31943=VERTEX_POINT('',#137625);
#31944=VERTEX_POINT('',#137641);
#31945=VERTEX_POINT('',#137643);
#31946=VERTEX_POINT('',#137667);
#31947=VERTEX_POINT('',#137668);
#31948=VERTEX_POINT('',#137684);
#31949=VERTEX_POINT('',#137686);
#31950=VERTEX_POINT('',#137710);
#31951=VERTEX_POINT('',#137711);
#31952=VERTEX_POINT('',#137727);
#31953=VERTEX_POINT('',#137729);
#31954=VERTEX_POINT('',#137753);
#31955=VERTEX_POINT('',#137754);
#31956=VERTEX_POINT('',#137770);
#31957=VERTEX_POINT('',#137772);
#31958=VERTEX_POINT('',#137796);
#31959=VERTEX_POINT('',#137797);
#31960=VERTEX_POINT('',#137813);
#31961=VERTEX_POINT('',#137815);
#31962=VERTEX_POINT('',#137839);
#31963=VERTEX_POINT('',#137840);
#31964=VERTEX_POINT('',#137856);
#31965=VERTEX_POINT('',#137858);
#31966=VERTEX_POINT('',#137882);
#31967=VERTEX_POINT('',#137883);
#31968=VERTEX_POINT('',#137899);
#31969=VERTEX_POINT('',#137901);
#31970=VERTEX_POINT('',#137925);
#31971=VERTEX_POINT('',#137926);
#31972=VERTEX_POINT('',#137942);
#31973=VERTEX_POINT('',#137944);
#31974=VERTEX_POINT('',#137968);
#31975=VERTEX_POINT('',#137969);
#31976=VERTEX_POINT('',#137985);
#31977=VERTEX_POINT('',#137987);
#31978=VERTEX_POINT('',#138011);
#31979=VERTEX_POINT('',#138012);
#31980=VERTEX_POINT('',#138028);
#31981=VERTEX_POINT('',#138030);
#31982=VERTEX_POINT('',#138054);
#31983=VERTEX_POINT('',#138055);
#31984=VERTEX_POINT('',#138071);
#31985=VERTEX_POINT('',#138073);
#31986=VERTEX_POINT('',#138097);
#31987=VERTEX_POINT('',#138098);
#31988=VERTEX_POINT('',#138114);
#31989=VERTEX_POINT('',#138116);
#31990=VERTEX_POINT('',#138140);
#31991=VERTEX_POINT('',#138141);
#31992=VERTEX_POINT('',#138166);
#31993=VERTEX_POINT('',#138170);
#31994=VERTEX_POINT('',#138183);
#31995=VERTEX_POINT('',#138185);
#31996=VERTEX_POINT('',#138200);
#31997=VERTEX_POINT('',#138202);
#31998=VERTEX_POINT('',#138226);
#31999=VERTEX_POINT('',#138227);
#32000=VERTEX_POINT('',#138243);
#32001=VERTEX_POINT('',#138245);
#32002=VERTEX_POINT('',#138269);
#32003=VERTEX_POINT('',#138270);
#32004=VERTEX_POINT('',#138286);
#32005=VERTEX_POINT('',#138288);
#32006=VERTEX_POINT('',#138312);
#32007=VERTEX_POINT('',#138313);
#32008=VERTEX_POINT('',#138329);
#32009=VERTEX_POINT('',#138331);
#32010=VERTEX_POINT('',#138355);
#32011=VERTEX_POINT('',#138356);
#32012=VERTEX_POINT('',#138372);
#32013=VERTEX_POINT('',#138374);
#32014=VERTEX_POINT('',#138398);
#32015=VERTEX_POINT('',#138399);
#32016=VERTEX_POINT('',#138415);
#32017=VERTEX_POINT('',#138417);
#32018=VERTEX_POINT('',#138441);
#32019=VERTEX_POINT('',#138442);
#32020=VERTEX_POINT('',#138458);
#32021=VERTEX_POINT('',#138460);
#32022=VERTEX_POINT('',#138484);
#32023=VERTEX_POINT('',#138485);
#32024=VERTEX_POINT('',#138501);
#32025=VERTEX_POINT('',#138503);
#32026=VERTEX_POINT('',#138518);
#32027=VERTEX_POINT('',#138519);
#32028=VERTEX_POINT('',#138550);
#32029=VERTEX_POINT('',#138557);
#32030=VERTEX_POINT('',#138570);
#32031=VERTEX_POINT('',#138572);
#32032=VERTEX_POINT('',#138596);
#32033=VERTEX_POINT('',#138600);
#32034=VERTEX_POINT('',#138613);
#32035=VERTEX_POINT('',#138615);
#32036=VERTEX_POINT('',#138639);
#32037=VERTEX_POINT('',#138643);
#32038=VERTEX_POINT('',#138656);
#32039=VERTEX_POINT('',#138658);
#32040=VERTEX_POINT('',#138682);
#32041=VERTEX_POINT('',#138686);
#32042=VERTEX_POINT('',#138699);
#32043=VERTEX_POINT('',#138701);
#32044=VERTEX_POINT('',#138725);
#32045=VERTEX_POINT('',#138729);
#32046=VERTEX_POINT('',#138742);
#32047=VERTEX_POINT('',#138744);
#32048=VERTEX_POINT('',#138768);
#32049=VERTEX_POINT('',#138772);
#32050=VERTEX_POINT('',#138785);
#32051=VERTEX_POINT('',#138787);
#32052=VERTEX_POINT('',#138811);
#32053=VERTEX_POINT('',#138815);
#32054=VERTEX_POINT('',#138828);
#32055=VERTEX_POINT('',#138830);
#32056=VERTEX_POINT('',#138854);
#32057=VERTEX_POINT('',#138858);
#32058=VERTEX_POINT('',#138871);
#32059=VERTEX_POINT('',#138873);
#32060=VERTEX_POINT('',#138897);
#32061=VERTEX_POINT('',#138901);
#32062=VERTEX_POINT('',#138914);
#32063=VERTEX_POINT('',#138916);
#32064=VERTEX_POINT('',#138940);
#32065=VERTEX_POINT('',#138944);
#32066=VERTEX_POINT('',#138957);
#32067=VERTEX_POINT('',#138959);
#32068=VERTEX_POINT('',#138983);
#32069=VERTEX_POINT('',#138987);
#32070=VERTEX_POINT('',#139000);
#32071=VERTEX_POINT('',#139002);
#32072=VERTEX_POINT('',#139026);
#32073=VERTEX_POINT('',#139030);
#32074=VERTEX_POINT('',#139043);
#32075=VERTEX_POINT('',#139045);
#32076=VERTEX_POINT('',#139069);
#32077=VERTEX_POINT('',#139073);
#32078=VERTEX_POINT('',#139086);
#32079=VERTEX_POINT('',#139088);
#32080=VERTEX_POINT('',#139112);
#32081=VERTEX_POINT('',#139116);
#32082=VERTEX_POINT('',#139157);
#32083=VERTEX_POINT('',#139159);
#32084=VERTEX_POINT('',#139183);
#32085=VERTEX_POINT('',#139187);
#32086=VERTEX_POINT('',#139200);
#32087=VERTEX_POINT('',#139202);
#32088=VERTEX_POINT('',#139226);
#32089=VERTEX_POINT('',#139230);
#32090=VERTEX_POINT('',#139243);
#32091=VERTEX_POINT('',#139245);
#32092=VERTEX_POINT('',#139269);
#32093=VERTEX_POINT('',#139273);
#32094=VERTEX_POINT('',#139286);
#32095=VERTEX_POINT('',#139288);
#32096=VERTEX_POINT('',#139312);
#32097=VERTEX_POINT('',#139316);
#32098=VERTEX_POINT('',#139329);
#32099=VERTEX_POINT('',#139331);
#32100=VERTEX_POINT('',#139355);
#32101=VERTEX_POINT('',#139359);
#32102=VERTEX_POINT('',#139372);
#32103=VERTEX_POINT('',#139374);
#32104=VERTEX_POINT('',#139398);
#32105=VERTEX_POINT('',#139402);
#32106=VERTEX_POINT('',#139415);
#32107=VERTEX_POINT('',#139417);
#32108=VERTEX_POINT('',#139441);
#32109=VERTEX_POINT('',#139445);
#32110=VERTEX_POINT('',#139458);
#32111=VERTEX_POINT('',#139460);
#32112=VERTEX_POINT('',#139484);
#32113=VERTEX_POINT('',#139488);
#32114=VERTEX_POINT('',#139501);
#32115=VERTEX_POINT('',#139503);
#32116=VERTEX_POINT('',#139527);
#32117=VERTEX_POINT('',#139531);
#32118=VERTEX_POINT('',#139544);
#32119=VERTEX_POINT('',#139546);
#32120=VERTEX_POINT('',#139570);
#32121=VERTEX_POINT('',#139574);
#32122=VERTEX_POINT('',#139587);
#32123=VERTEX_POINT('',#139589);
#32124=VERTEX_POINT('',#139613);
#32125=VERTEX_POINT('',#139617);
#32126=VERTEX_POINT('',#139630);
#32127=VERTEX_POINT('',#139632);
#32128=VERTEX_POINT('',#139656);
#32129=VERTEX_POINT('',#139660);
#32130=VERTEX_POINT('',#139673);
#32131=VERTEX_POINT('',#139675);
#32132=VERTEX_POINT('',#139699);
#32133=VERTEX_POINT('',#139703);
#32134=VERTEX_POINT('',#139716);
#32135=VERTEX_POINT('',#139718);
#32136=VERTEX_POINT('',#139742);
#32137=VERTEX_POINT('',#139746);
#32138=VERTEX_POINT('',#139750);
#32139=VERTEX_POINT('',#139758);
#32140=VERTEX_POINT('',#139782);
#32141=VERTEX_POINT('',#139796);
#32142=VERTEX_POINT('',#139821);
#32143=VERTEX_POINT('',#139846);
#32144=VERTEX_POINT('',#139871);
#32145=VERTEX_POINT('',#139896);
#32146=VERTEX_POINT('',#139921);
#32147=VERTEX_POINT('',#139946);
#32148=VERTEX_POINT('',#139971);
#32149=VERTEX_POINT('',#139996);
#32150=VERTEX_POINT('',#140021);
#32151=VERTEX_POINT('',#140046);
#32152=VERTEX_POINT('',#140071);
#32153=VERTEX_POINT('',#140096);
#32154=VERTEX_POINT('',#140121);
#32155=VERTEX_POINT('',#140146);
#32156=VERTEX_POINT('',#140171);
#32157=VERTEX_POINT('',#140196);
#32158=VERTEX_POINT('',#140221);
#32159=VERTEX_POINT('',#140246);
#32160=VERTEX_POINT('',#140271);
#32161=VERTEX_POINT('',#140296);
#32162=VERTEX_POINT('',#140321);
#32163=VERTEX_POINT('',#140346);
#32164=VERTEX_POINT('',#140371);
#32165=VERTEX_POINT('',#140396);
#32166=VERTEX_POINT('',#140421);
#32167=VERTEX_POINT('',#140446);
#32168=VERTEX_POINT('',#140471);
#32169=VERTEX_POINT('',#140507);
#32170=VERTEX_POINT('',#140525);
#32171=VERTEX_POINT('',#140554);
#32172=VERTEX_POINT('',#140583);
#32173=VERTEX_POINT('',#140612);
#32174=VERTEX_POINT('',#140646);
#32175=VERTEX_POINT('',#140675);
#32176=VERTEX_POINT('',#140704);
#32177=VERTEX_POINT('',#140733);
#32178=VERTEX_POINT('',#140762);
#32179=VERTEX_POINT('',#140791);
#32180=VERTEX_POINT('',#140820);
#32181=VERTEX_POINT('',#140849);
#32182=VERTEX_POINT('',#140878);
#32183=VERTEX_POINT('',#140912);
#32184=VERTEX_POINT('',#140941);
#32185=VERTEX_POINT('',#140970);
#32186=VERTEX_POINT('',#140999);
#32187=VERTEX_POINT('',#141033);
#32188=VERTEX_POINT('',#141062);
#32189=VERTEX_POINT('',#141091);
#32190=VERTEX_POINT('',#141120);
#32191=VERTEX_POINT('',#141149);
#32192=VERTEX_POINT('',#141178);
#32193=VERTEX_POINT('',#141212);
#32194=VERTEX_POINT('',#141246);
#32195=VERTEX_POINT('',#141275);
#32196=VERTEX_POINT('',#141304);
#32197=VERTEX_POINT('',#141333);
#32198=VERTEX_POINT('',#141374);
#32199=VERTEX_POINT('',#141375);
#32200=VERTEX_POINT('',#141385);
#32201=VERTEX_POINT('',#141387);
#32202=VERTEX_POINT('',#141407);
#32203=VERTEX_POINT('',#141408);
#32204=VERTEX_POINT('',#141418);
#32205=VERTEX_POINT('',#141420);
#32206=VERTEX_POINT('',#141440);
#32207=VERTEX_POINT('',#141441);
#32208=VERTEX_POINT('',#141451);
#32209=VERTEX_POINT('',#141453);
#32210=VERTEX_POINT('',#141473);
#32211=VERTEX_POINT('',#141474);
#32212=VERTEX_POINT('',#141484);
#32213=VERTEX_POINT('',#141486);
#32214=VERTEX_POINT('',#141506);
#32215=VERTEX_POINT('',#141507);
#32216=VERTEX_POINT('',#141517);
#32217=VERTEX_POINT('',#141519);
#32218=VERTEX_POINT('',#141539);
#32219=VERTEX_POINT('',#141540);
#32220=VERTEX_POINT('',#141550);
#32221=VERTEX_POINT('',#141552);
#32222=VERTEX_POINT('',#141572);
#32223=VERTEX_POINT('',#141573);
#32224=VERTEX_POINT('',#141583);
#32225=VERTEX_POINT('',#141585);
#32226=VERTEX_POINT('',#141605);
#32227=VERTEX_POINT('',#141606);
#32228=VERTEX_POINT('',#141616);
#32229=VERTEX_POINT('',#141618);
#32230=VERTEX_POINT('',#141638);
#32231=VERTEX_POINT('',#141639);
#32232=VERTEX_POINT('',#141649);
#32233=VERTEX_POINT('',#141651);
#32234=VERTEX_POINT('',#141671);
#32235=VERTEX_POINT('',#141672);
#32236=VERTEX_POINT('',#141682);
#32237=VERTEX_POINT('',#141684);
#32238=VERTEX_POINT('',#141704);
#32239=VERTEX_POINT('',#141705);
#32240=VERTEX_POINT('',#141715);
#32241=VERTEX_POINT('',#141717);
#32242=VERTEX_POINT('',#141737);
#32243=VERTEX_POINT('',#141738);
#32244=VERTEX_POINT('',#141748);
#32245=VERTEX_POINT('',#141750);
#32246=VERTEX_POINT('',#141770);
#32247=VERTEX_POINT('',#141771);
#32248=VERTEX_POINT('',#141781);
#32249=VERTEX_POINT('',#141783);
#32250=VERTEX_POINT('',#141803);
#32251=VERTEX_POINT('',#141804);
#32252=VERTEX_POINT('',#141814);
#32253=VERTEX_POINT('',#141816);
#32254=VERTEX_POINT('',#141860);
#32255=VERTEX_POINT('',#141861);
#32256=VERTEX_POINT('',#141871);
#32257=VERTEX_POINT('',#141873);
#32258=VERTEX_POINT('',#141893);
#32259=VERTEX_POINT('',#141894);
#32260=VERTEX_POINT('',#141904);
#32261=VERTEX_POINT('',#141906);
#32262=VERTEX_POINT('',#141926);
#32263=VERTEX_POINT('',#141927);
#32264=VERTEX_POINT('',#141937);
#32265=VERTEX_POINT('',#141939);
#32266=VERTEX_POINT('',#141959);
#32267=VERTEX_POINT('',#141960);
#32268=VERTEX_POINT('',#141970);
#32269=VERTEX_POINT('',#141972);
#32270=VERTEX_POINT('',#141992);
#32271=VERTEX_POINT('',#141993);
#32272=VERTEX_POINT('',#142012);
#32273=VERTEX_POINT('',#142016);
#32274=VERTEX_POINT('',#142025);
#32275=VERTEX_POINT('',#142027);
#32276=VERTEX_POINT('',#142036);
#32277=VERTEX_POINT('',#142038);
#32278=VERTEX_POINT('',#142058);
#32279=VERTEX_POINT('',#142059);
#32280=VERTEX_POINT('',#142069);
#32281=VERTEX_POINT('',#142071);
#32282=VERTEX_POINT('',#142091);
#32283=VERTEX_POINT('',#142092);
#32284=VERTEX_POINT('',#142102);
#32285=VERTEX_POINT('',#142104);
#32286=VERTEX_POINT('',#142124);
#32287=VERTEX_POINT('',#142125);
#32288=VERTEX_POINT('',#142135);
#32289=VERTEX_POINT('',#142137);
#32290=VERTEX_POINT('',#142157);
#32291=VERTEX_POINT('',#142158);
#32292=VERTEX_POINT('',#142168);
#32293=VERTEX_POINT('',#142170);
#32294=VERTEX_POINT('',#142190);
#32295=VERTEX_POINT('',#142191);
#32296=VERTEX_POINT('',#142201);
#32297=VERTEX_POINT('',#142203);
#32298=VERTEX_POINT('',#142223);
#32299=VERTEX_POINT('',#142224);
#32300=VERTEX_POINT('',#142234);
#32301=VERTEX_POINT('',#142236);
#32302=VERTEX_POINT('',#142256);
#32303=VERTEX_POINT('',#142257);
#32304=VERTEX_POINT('',#142267);
#32305=VERTEX_POINT('',#142269);
#32306=VERTEX_POINT('',#142289);
#32307=VERTEX_POINT('',#142290);
#32308=VERTEX_POINT('',#142300);
#32309=VERTEX_POINT('',#142302);
#32310=VERTEX_POINT('',#142326);
#32311=VERTEX_POINT('',#142328);
#32312=VERTEX_POINT('',#142350);
#32313=VERTEX_POINT('',#142354);
#32314=VERTEX_POINT('',#142367);
#32315=VERTEX_POINT('',#142369);
#32316=VERTEX_POINT('',#142391);
#32317=VERTEX_POINT('',#142395);
#32318=VERTEX_POINT('',#142408);
#32319=VERTEX_POINT('',#142410);
#32320=VERTEX_POINT('',#142432);
#32321=VERTEX_POINT('',#142436);
#32322=VERTEX_POINT('',#142449);
#32323=VERTEX_POINT('',#142451);
#32324=VERTEX_POINT('',#142473);
#32325=VERTEX_POINT('',#142477);
#32326=VERTEX_POINT('',#142490);
#32327=VERTEX_POINT('',#142492);
#32328=VERTEX_POINT('',#142514);
#32329=VERTEX_POINT('',#142518);
#32330=VERTEX_POINT('',#142531);
#32331=VERTEX_POINT('',#142533);
#32332=VERTEX_POINT('',#142555);
#32333=VERTEX_POINT('',#142559);
#32334=VERTEX_POINT('',#142572);
#32335=VERTEX_POINT('',#142574);
#32336=VERTEX_POINT('',#142596);
#32337=VERTEX_POINT('',#142600);
#32338=VERTEX_POINT('',#142613);
#32339=VERTEX_POINT('',#142615);
#32340=VERTEX_POINT('',#142637);
#32341=VERTEX_POINT('',#142641);
#32342=VERTEX_POINT('',#142654);
#32343=VERTEX_POINT('',#142656);
#32344=VERTEX_POINT('',#142678);
#32345=VERTEX_POINT('',#142682);
#32346=VERTEX_POINT('',#142695);
#32347=VERTEX_POINT('',#142697);
#32348=VERTEX_POINT('',#142719);
#32349=VERTEX_POINT('',#142723);
#32350=VERTEX_POINT('',#142736);
#32351=VERTEX_POINT('',#142738);
#32352=VERTEX_POINT('',#142760);
#32353=VERTEX_POINT('',#142764);
#32354=VERTEX_POINT('',#142777);
#32355=VERTEX_POINT('',#142779);
#32356=VERTEX_POINT('',#142801);
#32357=VERTEX_POINT('',#142805);
#32358=VERTEX_POINT('',#142818);
#32359=VERTEX_POINT('',#142820);
#32360=VERTEX_POINT('',#142842);
#32361=VERTEX_POINT('',#142846);
#32362=VERTEX_POINT('',#142859);
#32363=VERTEX_POINT('',#142861);
#32364=VERTEX_POINT('',#142883);
#32365=VERTEX_POINT('',#142887);
#32366=VERTEX_POINT('',#142900);
#32367=VERTEX_POINT('',#142902);
#32368=VERTEX_POINT('',#142924);
#32369=VERTEX_POINT('',#142928);
#32370=VERTEX_POINT('',#142941);
#32371=VERTEX_POINT('',#142943);
#32372=VERTEX_POINT('',#142965);
#32373=VERTEX_POINT('',#142969);
#32374=VERTEX_POINT('',#142982);
#32375=VERTEX_POINT('',#142984);
#32376=VERTEX_POINT('',#143006);
#32377=VERTEX_POINT('',#143010);
#32378=VERTEX_POINT('',#143023);
#32379=VERTEX_POINT('',#143025);
#32380=VERTEX_POINT('',#143047);
#32381=VERTEX_POINT('',#143051);
#32382=VERTEX_POINT('',#143064);
#32383=VERTEX_POINT('',#143066);
#32384=VERTEX_POINT('',#143088);
#32385=VERTEX_POINT('',#143092);
#32386=VERTEX_POINT('',#143105);
#32387=VERTEX_POINT('',#143107);
#32388=VERTEX_POINT('',#143129);
#32389=VERTEX_POINT('',#143133);
#32390=VERTEX_POINT('',#143146);
#32391=VERTEX_POINT('',#143148);
#32392=VERTEX_POINT('',#143170);
#32393=VERTEX_POINT('',#143174);
#32394=VERTEX_POINT('',#143219);
#32395=VERTEX_POINT('',#143221);
#32396=VERTEX_POINT('',#143243);
#32397=VERTEX_POINT('',#143247);
#32398=VERTEX_POINT('',#143260);
#32399=VERTEX_POINT('',#143262);
#32400=VERTEX_POINT('',#143284);
#32401=VERTEX_POINT('',#143288);
#32402=VERTEX_POINT('',#143301);
#32403=VERTEX_POINT('',#143303);
#32404=VERTEX_POINT('',#143325);
#32405=VERTEX_POINT('',#143329);
#32406=VERTEX_POINT('',#143342);
#32407=VERTEX_POINT('',#143344);
#32408=VERTEX_POINT('',#143366);
#32409=VERTEX_POINT('',#143370);
#32410=VERTEX_POINT('',#143383);
#32411=VERTEX_POINT('',#143385);
#32412=VERTEX_POINT('',#143407);
#32413=VERTEX_POINT('',#143411);
#32414=VERTEX_POINT('',#143424);
#32415=VERTEX_POINT('',#143426);
#32416=VERTEX_POINT('',#143448);
#32417=VERTEX_POINT('',#143452);
#32418=VERTEX_POINT('',#143465);
#32419=VERTEX_POINT('',#143467);
#32420=VERTEX_POINT('',#143489);
#32421=VERTEX_POINT('',#143493);
#32422=VERTEX_POINT('',#143502);
#32423=VERTEX_POINT('',#143527);
#32424=VERTEX_POINT('',#143552);
#32425=VERTEX_POINT('',#143577);
#32426=VERTEX_POINT('',#143602);
#32427=VERTEX_POINT('',#143627);
#32428=VERTEX_POINT('',#143652);
#32429=VERTEX_POINT('',#143677);
#32430=VERTEX_POINT('',#143702);
#32431=VERTEX_POINT('',#143727);
#32432=VERTEX_POINT('',#143752);
#32433=VERTEX_POINT('',#143777);
#32434=VERTEX_POINT('',#143802);
#32435=VERTEX_POINT('',#143827);
#32436=VERTEX_POINT('',#143852);
#32437=VERTEX_POINT('',#143877);
#32438=VERTEX_POINT('',#143902);
#32439=VERTEX_POINT('',#143927);
#32440=VERTEX_POINT('',#143952);
#32441=VERTEX_POINT('',#143977);
#32442=VERTEX_POINT('',#144002);
#32443=VERTEX_POINT('',#144027);
#32444=VERTEX_POINT('',#144052);
#32445=VERTEX_POINT('',#144077);
#32446=VERTEX_POINT('',#144102);
#32447=VERTEX_POINT('',#144127);
#32448=VERTEX_POINT('',#144152);
#32449=VERTEX_POINT('',#144177);
#32450=VERTEX_POINT('',#144202);
#32451=VERTEX_POINT('',#144227);
#32452=VERTEX_POINT('',#144248);
#32453=VERTEX_POINT('',#144269);
#32454=VERTEX_POINT('',#144290);
#32455=VERTEX_POINT('',#144311);
#32456=VERTEX_POINT('',#144332);
#32457=VERTEX_POINT('',#144353);
#32458=VERTEX_POINT('',#144374);
#32459=VERTEX_POINT('',#144395);
#32460=VERTEX_POINT('',#144416);
#32461=VERTEX_POINT('',#144437);
#32462=VERTEX_POINT('',#144458);
#32463=VERTEX_POINT('',#144479);
#32464=VERTEX_POINT('',#144500);
#32465=VERTEX_POINT('',#144521);
#32466=VERTEX_POINT('',#144542);
#32467=VERTEX_POINT('',#144563);
#32468=VERTEX_POINT('',#144584);
#32469=VERTEX_POINT('',#144605);
#32470=VERTEX_POINT('',#144626);
#32471=VERTEX_POINT('',#144647);
#32472=VERTEX_POINT('',#144668);
#32473=VERTEX_POINT('',#144689);
#32474=VERTEX_POINT('',#144710);
#32475=VERTEX_POINT('',#144731);
#32476=VERTEX_POINT('',#144752);
#32477=VERTEX_POINT('',#144773);
#32478=VERTEX_POINT('',#144794);
#32479=VERTEX_POINT('',#144815);
#32480=VERTEX_POINT('',#144836);
#32481=VERTEX_POINT('',#144837);
#32482=VERTEX_POINT('',#144852);
#32483=VERTEX_POINT('',#144853);
#32484=VERTEX_POINT('',#144863);
#32485=VERTEX_POINT('',#144865);
#32486=VERTEX_POINT('',#144881);
#32487=VERTEX_POINT('',#144882);
#32488=VERTEX_POINT('',#144892);
#32489=VERTEX_POINT('',#144894);
#32490=VERTEX_POINT('',#144910);
#32491=VERTEX_POINT('',#144911);
#32492=VERTEX_POINT('',#144921);
#32493=VERTEX_POINT('',#144923);
#32494=VERTEX_POINT('',#144939);
#32495=VERTEX_POINT('',#144940);
#32496=VERTEX_POINT('',#144950);
#32497=VERTEX_POINT('',#144952);
#32498=VERTEX_POINT('',#144968);
#32499=VERTEX_POINT('',#144969);
#32500=VERTEX_POINT('',#144979);
#32501=VERTEX_POINT('',#144981);
#32502=VERTEX_POINT('',#144997);
#32503=VERTEX_POINT('',#144998);
#32504=VERTEX_POINT('',#145008);
#32505=VERTEX_POINT('',#145010);
#32506=VERTEX_POINT('',#145046);
#32507=VERTEX_POINT('',#145047);
#32508=VERTEX_POINT('',#145057);
#32509=VERTEX_POINT('',#145059);
#32510=VERTEX_POINT('',#145075);
#32511=VERTEX_POINT('',#145076);
#32512=VERTEX_POINT('',#145086);
#32513=VERTEX_POINT('',#145088);
#32514=VERTEX_POINT('',#145104);
#32515=VERTEX_POINT('',#145105);
#32516=VERTEX_POINT('',#145115);
#32517=VERTEX_POINT('',#145117);
#32518=VERTEX_POINT('',#145133);
#32519=VERTEX_POINT('',#145134);
#32520=VERTEX_POINT('',#145144);
#32521=VERTEX_POINT('',#145146);
#32522=VERTEX_POINT('',#145162);
#32523=VERTEX_POINT('',#145163);
#32524=VERTEX_POINT('',#145173);
#32525=VERTEX_POINT('',#145175);
#32526=VERTEX_POINT('',#145191);
#32527=VERTEX_POINT('',#145192);
#32528=VERTEX_POINT('',#145202);
#32529=VERTEX_POINT('',#145204);
#32530=VERTEX_POINT('',#145220);
#32531=VERTEX_POINT('',#145221);
#32532=VERTEX_POINT('',#145231);
#32533=VERTEX_POINT('',#145233);
#32534=VERTEX_POINT('',#145249);
#32535=VERTEX_POINT('',#145250);
#32536=VERTEX_POINT('',#145260);
#32537=VERTEX_POINT('',#145262);
#32538=VERTEX_POINT('',#145278);
#32539=VERTEX_POINT('',#145279);
#32540=VERTEX_POINT('',#145289);
#32541=VERTEX_POINT('',#145291);
#32542=VERTEX_POINT('',#145307);
#32543=VERTEX_POINT('',#145308);
#32544=VERTEX_POINT('',#145318);
#32545=VERTEX_POINT('',#145320);
#32546=VERTEX_POINT('',#145336);
#32547=VERTEX_POINT('',#145337);
#32548=VERTEX_POINT('',#145347);
#32549=VERTEX_POINT('',#145349);
#32550=VERTEX_POINT('',#145365);
#32551=VERTEX_POINT('',#145366);
#32552=VERTEX_POINT('',#145381);
#32553=VERTEX_POINT('',#145385);
#32554=VERTEX_POINT('',#145394);
#32555=VERTEX_POINT('',#145396);
#32556=VERTEX_POINT('',#145405);
#32557=VERTEX_POINT('',#145407);
#32558=VERTEX_POINT('',#145423);
#32559=VERTEX_POINT('',#145424);
#32560=VERTEX_POINT('',#145434);
#32561=VERTEX_POINT('',#145436);
#32562=VERTEX_POINT('',#145452);
#32563=VERTEX_POINT('',#145453);
#32564=VERTEX_POINT('',#145463);
#32565=VERTEX_POINT('',#145465);
#32566=VERTEX_POINT('',#145481);
#32567=VERTEX_POINT('',#145482);
#32568=VERTEX_POINT('',#145492);
#32569=VERTEX_POINT('',#145494);
#32570=VERTEX_POINT('',#145510);
#32571=VERTEX_POINT('',#145511);
#32572=VERTEX_POINT('',#145521);
#32573=VERTEX_POINT('',#145523);
#32574=VERTEX_POINT('',#145539);
#32575=VERTEX_POINT('',#145540);
#32576=VERTEX_POINT('',#145550);
#32577=VERTEX_POINT('',#145552);
#32578=VERTEX_POINT('',#145568);
#32579=VERTEX_POINT('',#145569);
#32580=VERTEX_POINT('',#145579);
#32581=VERTEX_POINT('',#145581);
#32582=VERTEX_POINT('',#145597);
#32583=VERTEX_POINT('',#145598);
#32584=VERTEX_POINT('',#145608);
#32585=VERTEX_POINT('',#145610);
#32586=VERTEX_POINT('',#145626);
#32587=VERTEX_POINT('',#145627);
#32588=VERTEX_POINT('',#145637);
#32589=VERTEX_POINT('',#145639);
#32590=VERTEX_POINT('',#145650);
#32591=VERTEX_POINT('',#145651);
#32592=VERTEX_POINT('',#145668);
#32593=VERTEX_POINT('',#145675);
#32594=VERTEX_POINT('',#145688);
#32595=VERTEX_POINT('',#145690);
#32596=VERTEX_POINT('',#145704);
#32597=VERTEX_POINT('',#145708);
#32598=VERTEX_POINT('',#145721);
#32599=VERTEX_POINT('',#145723);
#32600=VERTEX_POINT('',#145737);
#32601=VERTEX_POINT('',#145741);
#32602=VERTEX_POINT('',#145754);
#32603=VERTEX_POINT('',#145756);
#32604=VERTEX_POINT('',#145770);
#32605=VERTEX_POINT('',#145774);
#32606=VERTEX_POINT('',#145787);
#32607=VERTEX_POINT('',#145789);
#32608=VERTEX_POINT('',#145803);
#32609=VERTEX_POINT('',#145807);
#32610=VERTEX_POINT('',#145820);
#32611=VERTEX_POINT('',#145822);
#32612=VERTEX_POINT('',#145836);
#32613=VERTEX_POINT('',#145840);
#32614=VERTEX_POINT('',#145853);
#32615=VERTEX_POINT('',#145855);
#32616=VERTEX_POINT('',#145869);
#32617=VERTEX_POINT('',#145873);
#32618=VERTEX_POINT('',#145886);
#32619=VERTEX_POINT('',#145888);
#32620=VERTEX_POINT('',#145902);
#32621=VERTEX_POINT('',#145906);
#32622=VERTEX_POINT('',#145919);
#32623=VERTEX_POINT('',#145921);
#32624=VERTEX_POINT('',#145935);
#32625=VERTEX_POINT('',#145939);
#32626=VERTEX_POINT('',#145952);
#32627=VERTEX_POINT('',#145954);
#32628=VERTEX_POINT('',#145968);
#32629=VERTEX_POINT('',#145972);
#32630=VERTEX_POINT('',#145985);
#32631=VERTEX_POINT('',#145987);
#32632=VERTEX_POINT('',#146001);
#32633=VERTEX_POINT('',#146005);
#32634=VERTEX_POINT('',#146018);
#32635=VERTEX_POINT('',#146020);
#32636=VERTEX_POINT('',#146034);
#32637=VERTEX_POINT('',#146038);
#32638=VERTEX_POINT('',#146051);
#32639=VERTEX_POINT('',#146053);
#32640=VERTEX_POINT('',#146067);
#32641=VERTEX_POINT('',#146071);
#32642=VERTEX_POINT('',#146084);
#32643=VERTEX_POINT('',#146086);
#32644=VERTEX_POINT('',#146100);
#32645=VERTEX_POINT('',#146104);
#32646=VERTEX_POINT('',#146141);
#32647=VERTEX_POINT('',#146143);
#32648=VERTEX_POINT('',#146157);
#32649=VERTEX_POINT('',#146161);
#32650=VERTEX_POINT('',#146174);
#32651=VERTEX_POINT('',#146176);
#32652=VERTEX_POINT('',#146190);
#32653=VERTEX_POINT('',#146194);
#32654=VERTEX_POINT('',#146207);
#32655=VERTEX_POINT('',#146209);
#32656=VERTEX_POINT('',#146223);
#32657=VERTEX_POINT('',#146227);
#32658=VERTEX_POINT('',#146240);
#32659=VERTEX_POINT('',#146242);
#32660=VERTEX_POINT('',#146256);
#32661=VERTEX_POINT('',#146260);
#32662=VERTEX_POINT('',#146273);
#32663=VERTEX_POINT('',#146275);
#32664=VERTEX_POINT('',#146289);
#32665=VERTEX_POINT('',#146293);
#32666=VERTEX_POINT('',#146306);
#32667=VERTEX_POINT('',#146308);
#32668=VERTEX_POINT('',#146322);
#32669=VERTEX_POINT('',#146326);
#32670=VERTEX_POINT('',#146339);
#32671=VERTEX_POINT('',#146341);
#32672=VERTEX_POINT('',#146355);
#32673=VERTEX_POINT('',#146359);
#32674=VERTEX_POINT('',#146372);
#32675=VERTEX_POINT('',#146374);
#32676=VERTEX_POINT('',#146388);
#32677=VERTEX_POINT('',#146392);
#32678=VERTEX_POINT('',#146405);
#32679=VERTEX_POINT('',#146407);
#32680=VERTEX_POINT('',#146421);
#32681=VERTEX_POINT('',#146425);
#32682=VERTEX_POINT('',#146438);
#32683=VERTEX_POINT('',#146440);
#32684=VERTEX_POINT('',#146454);
#32685=VERTEX_POINT('',#146458);
#32686=VERTEX_POINT('',#146471);
#32687=VERTEX_POINT('',#146473);
#32688=VERTEX_POINT('',#146487);
#32689=VERTEX_POINT('',#146491);
#32690=VERTEX_POINT('',#146504);
#32691=VERTEX_POINT('',#146506);
#32692=VERTEX_POINT('',#146520);
#32693=VERTEX_POINT('',#146524);
#32694=VERTEX_POINT('',#146537);
#32695=VERTEX_POINT('',#146539);
#32696=VERTEX_POINT('',#146553);
#32697=VERTEX_POINT('',#146557);
#32698=VERTEX_POINT('',#146570);
#32699=VERTEX_POINT('',#146572);
#32700=VERTEX_POINT('',#146586);
#32701=VERTEX_POINT('',#146590);
#32702=VERTEX_POINT('',#146594);
#32703=VERTEX_POINT('',#146596);
#32704=VERTEX_POINT('',#146620);
#32705=VERTEX_POINT('',#146649);
#32706=VERTEX_POINT('',#146695);
#32707=VERTEX_POINT('',#146736);
#32708=VERTEX_POINT('',#146786);
#32709=VERTEX_POINT('',#146827);
#32710=VERTEX_POINT('',#146868);
#32711=VERTEX_POINT('',#146918);
#32712=VERTEX_POINT('',#146968);
#32713=VERTEX_POINT('',#147017);
#32714=VERTEX_POINT('',#147066);
#32715=VERTEX_POINT('',#147116);
#32716=VERTEX_POINT('',#147157);
#32717=VERTEX_POINT('',#147207);
#32718=VERTEX_POINT('',#147251);
#32719=VERTEX_POINT('',#147297);
#32720=VERTEX_POINT('',#147347);
#32721=VERTEX_POINT('',#147393);
#32722=VERTEX_POINT('',#147434);
#32723=VERTEX_POINT('',#147480);
#32724=VERTEX_POINT('',#147530);
#32725=VERTEX_POINT('',#147576);
#32726=VERTEX_POINT('',#147622);
#32727=VERTEX_POINT('',#147672);
#32728=VERTEX_POINT('',#147718);
#32729=VERTEX_POINT('',#147768);
#32730=VERTEX_POINT('',#147817);
#32731=VERTEX_POINT('',#147867);
#32732=VERTEX_POINT('',#147913);
#32733=VERTEX_POINT('',#147983);
#32734=VERTEX_POINT('',#148001);
#32735=VERTEX_POINT('',#148026);
#32736=VERTEX_POINT('',#148051);
#32737=VERTEX_POINT('',#148076);
#32738=VERTEX_POINT('',#148101);
#32739=VERTEX_POINT('',#148126);
#32740=VERTEX_POINT('',#148151);
#32741=VERTEX_POINT('',#148176);
#32742=VERTEX_POINT('',#148201);
#32743=VERTEX_POINT('',#148226);
#32744=VERTEX_POINT('',#148251);
#32745=VERTEX_POINT('',#148276);
#32746=VERTEX_POINT('',#148301);
#32747=VERTEX_POINT('',#148326);
#32748=VERTEX_POINT('',#148351);
#32749=VERTEX_POINT('',#148376);
#32750=VERTEX_POINT('',#148401);
#32751=VERTEX_POINT('',#148426);
#32752=VERTEX_POINT('',#148451);
#32753=VERTEX_POINT('',#148476);
#32754=VERTEX_POINT('',#148501);
#32755=VERTEX_POINT('',#148526);
#32756=VERTEX_POINT('',#148551);
#32757=VERTEX_POINT('',#148576);
#32758=VERTEX_POINT('',#148601);
#32759=VERTEX_POINT('',#148626);
#32760=VERTEX_POINT('',#148651);
#32761=VERTEX_POINT('',#148676);
#32762=VERTEX_POINT('',#148712);
#32763=VERTEX_POINT('',#148713);
#32764=VERTEX_POINT('',#148723);
#32765=VERTEX_POINT('',#148725);
#32766=VERTEX_POINT('',#148755);
#32767=VERTEX_POINT('',#148756);
#32768=VERTEX_POINT('',#148766);
#32769=VERTEX_POINT('',#148768);
#32770=VERTEX_POINT('',#148798);
#32771=VERTEX_POINT('',#148799);
#32772=VERTEX_POINT('',#148809);
#32773=VERTEX_POINT('',#148811);
#32774=VERTEX_POINT('',#148841);
#32775=VERTEX_POINT('',#148842);
#32776=VERTEX_POINT('',#148852);
#32777=VERTEX_POINT('',#148854);
#32778=VERTEX_POINT('',#148884);
#32779=VERTEX_POINT('',#148885);
#32780=VERTEX_POINT('',#148895);
#32781=VERTEX_POINT('',#148897);
#32782=VERTEX_POINT('',#148927);
#32783=VERTEX_POINT('',#148928);
#32784=VERTEX_POINT('',#148938);
#32785=VERTEX_POINT('',#148940);
#32786=VERTEX_POINT('',#148970);
#32787=VERTEX_POINT('',#148971);
#32788=VERTEX_POINT('',#148981);
#32789=VERTEX_POINT('',#148983);
#32790=VERTEX_POINT('',#149013);
#32791=VERTEX_POINT('',#149014);
#32792=VERTEX_POINT('',#149024);
#32793=VERTEX_POINT('',#149026);
#32794=VERTEX_POINT('',#149056);
#32795=VERTEX_POINT('',#149057);
#32796=VERTEX_POINT('',#149067);
#32797=VERTEX_POINT('',#149069);
#32798=VERTEX_POINT('',#149099);
#32799=VERTEX_POINT('',#149100);
#32800=VERTEX_POINT('',#149110);
#32801=VERTEX_POINT('',#149112);
#32802=VERTEX_POINT('',#149142);
#32803=VERTEX_POINT('',#149143);
#32804=VERTEX_POINT('',#149153);
#32805=VERTEX_POINT('',#149155);
#32806=VERTEX_POINT('',#149185);
#32807=VERTEX_POINT('',#149186);
#32808=VERTEX_POINT('',#149196);
#32809=VERTEX_POINT('',#149198);
#32810=VERTEX_POINT('',#149228);
#32811=VERTEX_POINT('',#149229);
#32812=VERTEX_POINT('',#149239);
#32813=VERTEX_POINT('',#149241);
#32814=VERTEX_POINT('',#149271);
#32815=VERTEX_POINT('',#149272);
#32816=VERTEX_POINT('',#149282);
#32817=VERTEX_POINT('',#149284);
#32818=VERTEX_POINT('',#149342);
#32819=VERTEX_POINT('',#149343);
#32820=VERTEX_POINT('',#149353);
#32821=VERTEX_POINT('',#149355);
#32822=VERTEX_POINT('',#149385);
#32823=VERTEX_POINT('',#149386);
#32824=VERTEX_POINT('',#149396);
#32825=VERTEX_POINT('',#149398);
#32826=VERTEX_POINT('',#149428);
#32827=VERTEX_POINT('',#149429);
#32828=VERTEX_POINT('',#149439);
#32829=VERTEX_POINT('',#149441);
#32830=VERTEX_POINT('',#149471);
#32831=VERTEX_POINT('',#149472);
#32832=VERTEX_POINT('',#149491);
#32833=VERTEX_POINT('',#149501);
#32834=VERTEX_POINT('',#149514);
#32835=VERTEX_POINT('',#149516);
#32836=VERTEX_POINT('',#149525);
#32837=VERTEX_POINT('',#149533);
#32838=VERTEX_POINT('',#149557);
#32839=VERTEX_POINT('',#149558);
#32840=VERTEX_POINT('',#149568);
#32841=VERTEX_POINT('',#149570);
#32842=VERTEX_POINT('',#149600);
#32843=VERTEX_POINT('',#149601);
#32844=VERTEX_POINT('',#149611);
#32845=VERTEX_POINT('',#149613);
#32846=VERTEX_POINT('',#149643);
#32847=VERTEX_POINT('',#149644);
#32848=VERTEX_POINT('',#149654);
#32849=VERTEX_POINT('',#149656);
#32850=VERTEX_POINT('',#149686);
#32851=VERTEX_POINT('',#149687);
#32852=VERTEX_POINT('',#149697);
#32853=VERTEX_POINT('',#149699);
#32854=VERTEX_POINT('',#149729);
#32855=VERTEX_POINT('',#149730);
#32856=VERTEX_POINT('',#149740);
#32857=VERTEX_POINT('',#149742);
#32858=VERTEX_POINT('',#149772);
#32859=VERTEX_POINT('',#149773);
#32860=VERTEX_POINT('',#149783);
#32861=VERTEX_POINT('',#149785);
#32862=VERTEX_POINT('',#149815);
#32863=VERTEX_POINT('',#149816);
#32864=VERTEX_POINT('',#149826);
#32865=VERTEX_POINT('',#149828);
#32866=VERTEX_POINT('',#149858);
#32867=VERTEX_POINT('',#149859);
#32868=VERTEX_POINT('',#149869);
#32869=VERTEX_POINT('',#149871);
#32870=VERTEX_POINT('',#149901);
#32871=VERTEX_POINT('',#149902);
#32872=VERTEX_POINT('',#149912);
#32873=VERTEX_POINT('',#149914);
#32874=VERTEX_POINT('',#149944);
#32875=VERTEX_POINT('',#149946);
#32876=VERTEX_POINT('',#149955);
#32877=VERTEX_POINT('',#149956);
#32878=VERTEX_POINT('',#149958);
#32879=VERTEX_POINT('',#149967);
#32880=VERTEX_POINT('',#149983);
#32881=VERTEX_POINT('',#149985);
#32882=VERTEX_POINT('',#149994);
#32883=VERTEX_POINT('',#149995);
#32884=VERTEX_POINT('',#149997);
#32885=VERTEX_POINT('',#150006);
#32886=VERTEX_POINT('',#150022);
#32887=VERTEX_POINT('',#150024);
#32888=VERTEX_POINT('',#150033);
#32889=VERTEX_POINT('',#150034);
#32890=VERTEX_POINT('',#150036);
#32891=VERTEX_POINT('',#150045);
#32892=VERTEX_POINT('',#150061);
#32893=VERTEX_POINT('',#150063);
#32894=VERTEX_POINT('',#150072);
#32895=VERTEX_POINT('',#150073);
#32896=VERTEX_POINT('',#150075);
#32897=VERTEX_POINT('',#150084);
#32898=VERTEX_POINT('',#150100);
#32899=VERTEX_POINT('',#150102);
#32900=VERTEX_POINT('',#150111);
#32901=VERTEX_POINT('',#150112);
#32902=VERTEX_POINT('',#150114);
#32903=VERTEX_POINT('',#150123);
#32904=VERTEX_POINT('',#150139);
#32905=VERTEX_POINT('',#150141);
#32906=VERTEX_POINT('',#150150);
#32907=VERTEX_POINT('',#150151);
#32908=VERTEX_POINT('',#150153);
#32909=VERTEX_POINT('',#150162);
#32910=VERTEX_POINT('',#150178);
#32911=VERTEX_POINT('',#150180);
#32912=VERTEX_POINT('',#150189);
#32913=VERTEX_POINT('',#150190);
#32914=VERTEX_POINT('',#150192);
#32915=VERTEX_POINT('',#150201);
#32916=VERTEX_POINT('',#150217);
#32917=VERTEX_POINT('',#150219);
#32918=VERTEX_POINT('',#150228);
#32919=VERTEX_POINT('',#150229);
#32920=VERTEX_POINT('',#150231);
#32921=VERTEX_POINT('',#150240);
#32922=VERTEX_POINT('',#150256);
#32923=VERTEX_POINT('',#150258);
#32924=VERTEX_POINT('',#150267);
#32925=VERTEX_POINT('',#150268);
#32926=VERTEX_POINT('',#150270);
#32927=VERTEX_POINT('',#150279);
#32928=VERTEX_POINT('',#150295);
#32929=VERTEX_POINT('',#150297);
#32930=VERTEX_POINT('',#150306);
#32931=VERTEX_POINT('',#150307);
#32932=VERTEX_POINT('',#150309);
#32933=VERTEX_POINT('',#150318);
#32934=VERTEX_POINT('',#150334);
#32935=VERTEX_POINT('',#150336);
#32936=VERTEX_POINT('',#150345);
#32937=VERTEX_POINT('',#150346);
#32938=VERTEX_POINT('',#150348);
#32939=VERTEX_POINT('',#150357);
#32940=VERTEX_POINT('',#150373);
#32941=VERTEX_POINT('',#150375);
#32942=VERTEX_POINT('',#150384);
#32943=VERTEX_POINT('',#150385);
#32944=VERTEX_POINT('',#150387);
#32945=VERTEX_POINT('',#150396);
#32946=VERTEX_POINT('',#150412);
#32947=VERTEX_POINT('',#150414);
#32948=VERTEX_POINT('',#150423);
#32949=VERTEX_POINT('',#150424);
#32950=VERTEX_POINT('',#150426);
#32951=VERTEX_POINT('',#150435);
#32952=VERTEX_POINT('',#150451);
#32953=VERTEX_POINT('',#150453);
#32954=VERTEX_POINT('',#150462);
#32955=VERTEX_POINT('',#150463);
#32956=VERTEX_POINT('',#150465);
#32957=VERTEX_POINT('',#150474);
#32958=VERTEX_POINT('',#150490);
#32959=VERTEX_POINT('',#150492);
#32960=VERTEX_POINT('',#150501);
#32961=VERTEX_POINT('',#150502);
#32962=VERTEX_POINT('',#150504);
#32963=VERTEX_POINT('',#150513);
#32964=VERTEX_POINT('',#150529);
#32965=VERTEX_POINT('',#150531);
#32966=VERTEX_POINT('',#150540);
#32967=VERTEX_POINT('',#150541);
#32968=VERTEX_POINT('',#150543);
#32969=VERTEX_POINT('',#150552);
#32970=VERTEX_POINT('',#150568);
#32971=VERTEX_POINT('',#150570);
#32972=VERTEX_POINT('',#150579);
#32973=VERTEX_POINT('',#150580);
#32974=VERTEX_POINT('',#150582);
#32975=VERTEX_POINT('',#150591);
#32976=VERTEX_POINT('',#150607);
#32977=VERTEX_POINT('',#150609);
#32978=VERTEX_POINT('',#150618);
#32979=VERTEX_POINT('',#150619);
#32980=VERTEX_POINT('',#150621);
#32981=VERTEX_POINT('',#150630);
#32982=VERTEX_POINT('',#150646);
#32983=VERTEX_POINT('',#150648);
#32984=VERTEX_POINT('',#150657);
#32985=VERTEX_POINT('',#150658);
#32986=VERTEX_POINT('',#150660);
#32987=VERTEX_POINT('',#150669);
#32988=VERTEX_POINT('',#150685);
#32989=VERTEX_POINT('',#150687);
#32990=VERTEX_POINT('',#150696);
#32991=VERTEX_POINT('',#150697);
#32992=VERTEX_POINT('',#150699);
#32993=VERTEX_POINT('',#150708);
#32994=VERTEX_POINT('',#150724);
#32995=VERTEX_POINT('',#150726);
#32996=VERTEX_POINT('',#150735);
#32997=VERTEX_POINT('',#150736);
#32998=VERTEX_POINT('',#150738);
#32999=VERTEX_POINT('',#150747);
#33000=VERTEX_POINT('',#150787);
#33001=VERTEX_POINT('',#150789);
#33002=VERTEX_POINT('',#150798);
#33003=VERTEX_POINT('',#150799);
#33004=VERTEX_POINT('',#150801);
#33005=VERTEX_POINT('',#150810);
#33006=VERTEX_POINT('',#150826);
#33007=VERTEX_POINT('',#150828);
#33008=VERTEX_POINT('',#150837);
#33009=VERTEX_POINT('',#150838);
#33010=VERTEX_POINT('',#150840);
#33011=VERTEX_POINT('',#150849);
#33012=VERTEX_POINT('',#150865);
#33013=VERTEX_POINT('',#150867);
#33014=VERTEX_POINT('',#150876);
#33015=VERTEX_POINT('',#150877);
#33016=VERTEX_POINT('',#150879);
#33017=VERTEX_POINT('',#150888);
#33018=VERTEX_POINT('',#150904);
#33019=VERTEX_POINT('',#150906);
#33020=VERTEX_POINT('',#150915);
#33021=VERTEX_POINT('',#150916);
#33022=VERTEX_POINT('',#150918);
#33023=VERTEX_POINT('',#150927);
#33024=VERTEX_POINT('',#150943);
#33025=VERTEX_POINT('',#150945);
#33026=VERTEX_POINT('',#150954);
#33027=VERTEX_POINT('',#150955);
#33028=VERTEX_POINT('',#150957);
#33029=VERTEX_POINT('',#150966);
#33030=VERTEX_POINT('',#150982);
#33031=VERTEX_POINT('',#150984);
#33032=VERTEX_POINT('',#150993);
#33033=VERTEX_POINT('',#150994);
#33034=VERTEX_POINT('',#150996);
#33035=VERTEX_POINT('',#151005);
#33036=VERTEX_POINT('',#151021);
#33037=VERTEX_POINT('',#151023);
#33038=VERTEX_POINT('',#151032);
#33039=VERTEX_POINT('',#151033);
#33040=VERTEX_POINT('',#151035);
#33041=VERTEX_POINT('',#151044);
#33042=VERTEX_POINT('',#151060);
#33043=VERTEX_POINT('',#151089);
#33044=VERTEX_POINT('',#151118);
#33045=VERTEX_POINT('',#151147);
#33046=VERTEX_POINT('',#151181);
#33047=VERTEX_POINT('',#151215);
#33048=VERTEX_POINT('',#151244);
#33049=VERTEX_POINT('',#151273);
#33050=VERTEX_POINT('',#151302);
#33051=VERTEX_POINT('',#151331);
#33052=VERTEX_POINT('',#151360);
#33053=VERTEX_POINT('',#151394);
#33054=VERTEX_POINT('',#151423);
#33055=VERTEX_POINT('',#151452);
#33056=VERTEX_POINT('',#151481);
#33057=VERTEX_POINT('',#151515);
#33058=VERTEX_POINT('',#151544);
#33059=VERTEX_POINT('',#151573);
#33060=VERTEX_POINT('',#151602);
#33061=VERTEX_POINT('',#151631);
#33062=VERTEX_POINT('',#151660);
#33063=VERTEX_POINT('',#151689);
#33064=VERTEX_POINT('',#151718);
#33065=VERTEX_POINT('',#151747);
#33066=VERTEX_POINT('',#151781);
#33067=VERTEX_POINT('',#151810);
#33068=VERTEX_POINT('',#151839);
#33069=VERTEX_POINT('',#151868);
#33070=VERTEX_POINT('',#151897);
#33071=VERTEX_POINT('',#151931);
#33072=VERTEX_POINT('',#151951);
#33073=VERTEX_POINT('',#151971);
#33074=VERTEX_POINT('',#151991);
#33075=VERTEX_POINT('',#152011);
#33076=VERTEX_POINT('',#152031);
#33077=VERTEX_POINT('',#152051);
#33078=VERTEX_POINT('',#152071);
#33079=VERTEX_POINT('',#152091);
#33080=VERTEX_POINT('',#152111);
#33081=VERTEX_POINT('',#152131);
#33082=VERTEX_POINT('',#152151);
#33083=VERTEX_POINT('',#152171);
#33084=VERTEX_POINT('',#152191);
#33085=VERTEX_POINT('',#152211);
#33086=VERTEX_POINT('',#152231);
#33087=VERTEX_POINT('',#152251);
#33088=VERTEX_POINT('',#152271);
#33089=VERTEX_POINT('',#152291);
#33090=VERTEX_POINT('',#152311);
#33091=VERTEX_POINT('',#152331);
#33092=VERTEX_POINT('',#152351);
#33093=VERTEX_POINT('',#152371);
#33094=VERTEX_POINT('',#152391);
#33095=VERTEX_POINT('',#152411);
#33096=VERTEX_POINT('',#152431);
#33097=VERTEX_POINT('',#152451);
#33098=VERTEX_POINT('',#152471);
#33099=VERTEX_POINT('',#152491);
#33100=VERTEX_POINT('',#152511);
#33101=VERTEX_POINT('',#152512);
#33102=VERTEX_POINT('',#152535);
#33103=VERTEX_POINT('',#152536);
#33104=VERTEX_POINT('',#152546);
#33105=VERTEX_POINT('',#152548);
#33106=VERTEX_POINT('',#152576);
#33107=VERTEX_POINT('',#152577);
#33108=VERTEX_POINT('',#152587);
#33109=VERTEX_POINT('',#152589);
#33110=VERTEX_POINT('',#152617);
#33111=VERTEX_POINT('',#152618);
#33112=VERTEX_POINT('',#152628);
#33113=VERTEX_POINT('',#152630);
#33114=VERTEX_POINT('',#152658);
#33115=VERTEX_POINT('',#152659);
#33116=VERTEX_POINT('',#152669);
#33117=VERTEX_POINT('',#152671);
#33118=VERTEX_POINT('',#152699);
#33119=VERTEX_POINT('',#152700);
#33120=VERTEX_POINT('',#152710);
#33121=VERTEX_POINT('',#152712);
#33122=VERTEX_POINT('',#152740);
#33123=VERTEX_POINT('',#152741);
#33124=VERTEX_POINT('',#152751);
#33125=VERTEX_POINT('',#152753);
#33126=VERTEX_POINT('',#152813);
#33127=VERTEX_POINT('',#152814);
#33128=VERTEX_POINT('',#152824);
#33129=VERTEX_POINT('',#152826);
#33130=VERTEX_POINT('',#152854);
#33131=VERTEX_POINT('',#152855);
#33132=VERTEX_POINT('',#152865);
#33133=VERTEX_POINT('',#152867);
#33134=VERTEX_POINT('',#152895);
#33135=VERTEX_POINT('',#152896);
#33136=VERTEX_POINT('',#152906);
#33137=VERTEX_POINT('',#152908);
#33138=VERTEX_POINT('',#152936);
#33139=VERTEX_POINT('',#152937);
#33140=VERTEX_POINT('',#152947);
#33141=VERTEX_POINT('',#152949);
#33142=VERTEX_POINT('',#152977);
#33143=VERTEX_POINT('',#152978);
#33144=VERTEX_POINT('',#152988);
#33145=VERTEX_POINT('',#152990);
#33146=VERTEX_POINT('',#153018);
#33147=VERTEX_POINT('',#153019);
#33148=VERTEX_POINT('',#153029);
#33149=VERTEX_POINT('',#153031);
#33150=VERTEX_POINT('',#153059);
#33151=VERTEX_POINT('',#153060);
#33152=VERTEX_POINT('',#153070);
#33153=VERTEX_POINT('',#153072);
#33154=VERTEX_POINT('',#153100);
#33155=VERTEX_POINT('',#153101);
#33156=VERTEX_POINT('',#153111);
#33157=VERTEX_POINT('',#153113);
#33158=VERTEX_POINT('',#153141);
#33159=VERTEX_POINT('',#153142);
#33160=VERTEX_POINT('',#153152);
#33161=VERTEX_POINT('',#153154);
#33162=VERTEX_POINT('',#153182);
#33163=VERTEX_POINT('',#153183);
#33164=VERTEX_POINT('',#153193);
#33165=VERTEX_POINT('',#153195);
#33166=VERTEX_POINT('',#153223);
#33167=VERTEX_POINT('',#153224);
#33168=VERTEX_POINT('',#153243);
#33169=VERTEX_POINT('',#153247);
#33170=VERTEX_POINT('',#153264);
#33171=VERTEX_POINT('',#153266);
#33172=VERTEX_POINT('',#153275);
#33173=VERTEX_POINT('',#153277);
#33174=VERTEX_POINT('',#153305);
#33175=VERTEX_POINT('',#153306);
#33176=VERTEX_POINT('',#153316);
#33177=VERTEX_POINT('',#153318);
#33178=VERTEX_POINT('',#153346);
#33179=VERTEX_POINT('',#153347);
#33180=VERTEX_POINT('',#153357);
#33181=VERTEX_POINT('',#153359);
#33182=VERTEX_POINT('',#153387);
#33183=VERTEX_POINT('',#153388);
#33184=VERTEX_POINT('',#153398);
#33185=VERTEX_POINT('',#153400);
#33186=VERTEX_POINT('',#153428);
#33187=VERTEX_POINT('',#153429);
#33188=VERTEX_POINT('',#153439);
#33189=VERTEX_POINT('',#153441);
#33190=VERTEX_POINT('',#153469);
#33191=VERTEX_POINT('',#153470);
#33192=VERTEX_POINT('',#153480);
#33193=VERTEX_POINT('',#153482);
#33194=VERTEX_POINT('',#153510);
#33195=VERTEX_POINT('',#153511);
#33196=VERTEX_POINT('',#153521);
#33197=VERTEX_POINT('',#153523);
#33198=VERTEX_POINT('',#153551);
#33199=VERTEX_POINT('',#153552);
#33200=VERTEX_POINT('',#153562);
#33201=VERTEX_POINT('',#153564);
#33202=VERTEX_POINT('',#153592);
#33203=VERTEX_POINT('',#153593);
#33204=VERTEX_POINT('',#153603);
#33205=VERTEX_POINT('',#153605);
#33206=VERTEX_POINT('',#153633);
#33207=VERTEX_POINT('',#153634);
#33208=VERTEX_POINT('',#153644);
#33209=VERTEX_POINT('',#153646);
#33210=VERTEX_POINT('',#153661);
#33211=VERTEX_POINT('',#153662);
#33212=VERTEX_POINT('',#153690);
#33213=VERTEX_POINT('',#153697);
#33214=VERTEX_POINT('',#153714);
#33215=VERTEX_POINT('',#153716);
#33216=VERTEX_POINT('',#153730);
#33217=VERTEX_POINT('',#153739);
#33218=VERTEX_POINT('',#153773);
#33219=VERTEX_POINT('',#153775);
#33220=VERTEX_POINT('',#153789);
#33221=VERTEX_POINT('',#153798);
#33222=VERTEX_POINT('',#153832);
#33223=VERTEX_POINT('',#153834);
#33224=VERTEX_POINT('',#153848);
#33225=VERTEX_POINT('',#153857);
#33226=VERTEX_POINT('',#153891);
#33227=VERTEX_POINT('',#153893);
#33228=VERTEX_POINT('',#153907);
#33229=VERTEX_POINT('',#153916);
#33230=VERTEX_POINT('',#153950);
#33231=VERTEX_POINT('',#153952);
#33232=VERTEX_POINT('',#153966);
#33233=VERTEX_POINT('',#153975);
#33234=VERTEX_POINT('',#154009);
#33235=VERTEX_POINT('',#154011);
#33236=VERTEX_POINT('',#154025);
#33237=VERTEX_POINT('',#154034);
#33238=VERTEX_POINT('',#154068);
#33239=VERTEX_POINT('',#154070);
#33240=VERTEX_POINT('',#154084);
#33241=VERTEX_POINT('',#154093);
#33242=VERTEX_POINT('',#154127);
#33243=VERTEX_POINT('',#154129);
#33244=VERTEX_POINT('',#154143);
#33245=VERTEX_POINT('',#154152);
#33246=VERTEX_POINT('',#154186);
#33247=VERTEX_POINT('',#154188);
#33248=VERTEX_POINT('',#154202);
#33249=VERTEX_POINT('',#154211);
#33250=VERTEX_POINT('',#154245);
#33251=VERTEX_POINT('',#154247);
#33252=VERTEX_POINT('',#154261);
#33253=VERTEX_POINT('',#154270);
#33254=VERTEX_POINT('',#154304);
#33255=VERTEX_POINT('',#154306);
#33256=VERTEX_POINT('',#154320);
#33257=VERTEX_POINT('',#154329);
#33258=VERTEX_POINT('',#154363);
#33259=VERTEX_POINT('',#154365);
#33260=VERTEX_POINT('',#154379);
#33261=VERTEX_POINT('',#154388);
#33262=VERTEX_POINT('',#154422);
#33263=VERTEX_POINT('',#154424);
#33264=VERTEX_POINT('',#154438);
#33265=VERTEX_POINT('',#154447);
#33266=VERTEX_POINT('',#154507);
#33267=VERTEX_POINT('',#154509);
#33268=VERTEX_POINT('',#154523);
#33269=VERTEX_POINT('',#154532);
#33270=VERTEX_POINT('',#154566);
#33271=VERTEX_POINT('',#154568);
#33272=VERTEX_POINT('',#154582);
#33273=VERTEX_POINT('',#154591);
#33274=VERTEX_POINT('',#154625);
#33275=VERTEX_POINT('',#154627);
#33276=VERTEX_POINT('',#154641);
#33277=VERTEX_POINT('',#154650);
#33278=VERTEX_POINT('',#154684);
#33279=VERTEX_POINT('',#154686);
#33280=VERTEX_POINT('',#154700);
#33281=VERTEX_POINT('',#154709);
#33282=VERTEX_POINT('',#154743);
#33283=VERTEX_POINT('',#154745);
#33284=VERTEX_POINT('',#154759);
#33285=VERTEX_POINT('',#154768);
#33286=VERTEX_POINT('',#154802);
#33287=VERTEX_POINT('',#154804);
#33288=VERTEX_POINT('',#154818);
#33289=VERTEX_POINT('',#154827);
#33290=VERTEX_POINT('',#154887);
#33291=VERTEX_POINT('',#154889);
#33292=VERTEX_POINT('',#154903);
#33293=VERTEX_POINT('',#154912);
#33294=VERTEX_POINT('',#154946);
#33295=VERTEX_POINT('',#154948);
#33296=VERTEX_POINT('',#154962);
#33297=VERTEX_POINT('',#154971);
#33298=VERTEX_POINT('',#155005);
#33299=VERTEX_POINT('',#155007);
#33300=VERTEX_POINT('',#155021);
#33301=VERTEX_POINT('',#155030);
#33302=VERTEX_POINT('',#155064);
#33303=VERTEX_POINT('',#155066);
#33304=VERTEX_POINT('',#155080);
#33305=VERTEX_POINT('',#155089);
#33306=VERTEX_POINT('',#155123);
#33307=VERTEX_POINT('',#155125);
#33308=VERTEX_POINT('',#155139);
#33309=VERTEX_POINT('',#155148);
#33310=VERTEX_POINT('',#155182);
#33311=VERTEX_POINT('',#155184);
#33312=VERTEX_POINT('',#155198);
#33313=VERTEX_POINT('',#155207);
#33314=VERTEX_POINT('',#155241);
#33315=VERTEX_POINT('',#155243);
#33316=VERTEX_POINT('',#155257);
#33317=VERTEX_POINT('',#155266);
#33318=VERTEX_POINT('',#155292);
#33319=VERTEX_POINT('',#155299);
#33320=VERTEX_POINT('',#155332);
#33321=VERTEX_POINT('',#155346);
#33322=VERTEX_POINT('',#155367);
#33323=VERTEX_POINT('',#155388);
#33324=VERTEX_POINT('',#155409);
#33325=VERTEX_POINT('',#155430);
#33326=VERTEX_POINT('',#155451);
#33327=VERTEX_POINT('',#155472);
#33328=VERTEX_POINT('',#155493);
#33329=VERTEX_POINT('',#155514);
#33330=VERTEX_POINT('',#155535);
#33331=VERTEX_POINT('',#155556);
#33332=VERTEX_POINT('',#155577);
#33333=VERTEX_POINT('',#155598);
#33334=VERTEX_POINT('',#155619);
#33335=VERTEX_POINT('',#155640);
#33336=VERTEX_POINT('',#155661);
#33337=VERTEX_POINT('',#155682);
#33338=VERTEX_POINT('',#155703);
#33339=VERTEX_POINT('',#155724);
#33340=VERTEX_POINT('',#155745);
#33341=VERTEX_POINT('',#155766);
#33342=VERTEX_POINT('',#155787);
#33343=VERTEX_POINT('',#155808);
#33344=VERTEX_POINT('',#155829);
#33345=VERTEX_POINT('',#155850);
#33346=VERTEX_POINT('',#155871);
#33347=VERTEX_POINT('',#155892);
#33348=VERTEX_POINT('',#155913);
#33349=VERTEX_POINT('',#155949);
#33350=VERTEX_POINT('',#155970);
#33351=VERTEX_POINT('',#156013);
#33352=VERTEX_POINT('',#156056);
#33353=VERTEX_POINT('',#156099);
#33354=VERTEX_POINT('',#156142);
#33355=VERTEX_POINT('',#156185);
#33356=VERTEX_POINT('',#156228);
#33357=VERTEX_POINT('',#156271);
#33358=VERTEX_POINT('',#156314);
#33359=VERTEX_POINT('',#156357);
#33360=VERTEX_POINT('',#156400);
#33361=VERTEX_POINT('',#156443);
#33362=VERTEX_POINT('',#156486);
#33363=VERTEX_POINT('',#156529);
#33364=VERTEX_POINT('',#156572);
#33365=VERTEX_POINT('',#156615);
#33366=VERTEX_POINT('',#156658);
#33367=VERTEX_POINT('',#156701);
#33368=VERTEX_POINT('',#156744);
#33369=VERTEX_POINT('',#156787);
#33370=VERTEX_POINT('',#156830);
#33371=VERTEX_POINT('',#156873);
#33372=VERTEX_POINT('',#156916);
#33373=VERTEX_POINT('',#156959);
#33374=VERTEX_POINT('',#157002);
#33375=VERTEX_POINT('',#157045);
#33376=VERTEX_POINT('',#157088);
#33377=VERTEX_POINT('',#157131);
#33378=VERTEX_POINT('',#157176);
#33379=VERTEX_POINT('',#157177);
#33380=VERTEX_POINT('',#157187);
#33381=VERTEX_POINT('',#157189);
#33382=VERTEX_POINT('',#157209);
#33383=VERTEX_POINT('',#157210);
#33384=VERTEX_POINT('',#157220);
#33385=VERTEX_POINT('',#157222);
#33386=VERTEX_POINT('',#157242);
#33387=VERTEX_POINT('',#157243);
#33388=VERTEX_POINT('',#157253);
#33389=VERTEX_POINT('',#157255);
#33390=VERTEX_POINT('',#157275);
#33391=VERTEX_POINT('',#157276);
#33392=VERTEX_POINT('',#157286);
#33393=VERTEX_POINT('',#157288);
#33394=VERTEX_POINT('',#157308);
#33395=VERTEX_POINT('',#157309);
#33396=VERTEX_POINT('',#157319);
#33397=VERTEX_POINT('',#157321);
#33398=VERTEX_POINT('',#157341);
#33399=VERTEX_POINT('',#157342);
#33400=VERTEX_POINT('',#157352);
#33401=VERTEX_POINT('',#157354);
#33402=VERTEX_POINT('',#157374);
#33403=VERTEX_POINT('',#157375);
#33404=VERTEX_POINT('',#157385);
#33405=VERTEX_POINT('',#157387);
#33406=VERTEX_POINT('',#157407);
#33407=VERTEX_POINT('',#157408);
#33408=VERTEX_POINT('',#157418);
#33409=VERTEX_POINT('',#157420);
#33410=VERTEX_POINT('',#157440);
#33411=VERTEX_POINT('',#157441);
#33412=VERTEX_POINT('',#157451);
#33413=VERTEX_POINT('',#157453);
#33414=VERTEX_POINT('',#157473);
#33415=VERTEX_POINT('',#157474);
#33416=VERTEX_POINT('',#157484);
#33417=VERTEX_POINT('',#157486);
#33418=VERTEX_POINT('',#157506);
#33419=VERTEX_POINT('',#157507);
#33420=VERTEX_POINT('',#157517);
#33421=VERTEX_POINT('',#157519);
#33422=VERTEX_POINT('',#157539);
#33423=VERTEX_POINT('',#157540);
#33424=VERTEX_POINT('',#157550);
#33425=VERTEX_POINT('',#157552);
#33426=VERTEX_POINT('',#157572);
#33427=VERTEX_POINT('',#157573);
#33428=VERTEX_POINT('',#157583);
#33429=VERTEX_POINT('',#157585);
#33430=VERTEX_POINT('',#157605);
#33431=VERTEX_POINT('',#157606);
#33432=VERTEX_POINT('',#157616);
#33433=VERTEX_POINT('',#157618);
#33434=VERTEX_POINT('',#157662);
#33435=VERTEX_POINT('',#157663);
#33436=VERTEX_POINT('',#157673);
#33437=VERTEX_POINT('',#157675);
#33438=VERTEX_POINT('',#157695);
#33439=VERTEX_POINT('',#157696);
#33440=VERTEX_POINT('',#157706);
#33441=VERTEX_POINT('',#157708);
#33442=VERTEX_POINT('',#157728);
#33443=VERTEX_POINT('',#157729);
#33444=VERTEX_POINT('',#157748);
#33445=VERTEX_POINT('',#157752);
#33446=VERTEX_POINT('',#157761);
#33447=VERTEX_POINT('',#157763);
#33448=VERTEX_POINT('',#157772);
#33449=VERTEX_POINT('',#157774);
#33450=VERTEX_POINT('',#157794);
#33451=VERTEX_POINT('',#157795);
#33452=VERTEX_POINT('',#157805);
#33453=VERTEX_POINT('',#157807);
#33454=VERTEX_POINT('',#157827);
#33455=VERTEX_POINT('',#157828);
#33456=VERTEX_POINT('',#157838);
#33457=VERTEX_POINT('',#157840);
#33458=VERTEX_POINT('',#157860);
#33459=VERTEX_POINT('',#157861);
#33460=VERTEX_POINT('',#157871);
#33461=VERTEX_POINT('',#157873);
#33462=VERTEX_POINT('',#157893);
#33463=VERTEX_POINT('',#157894);
#33464=VERTEX_POINT('',#157904);
#33465=VERTEX_POINT('',#157906);
#33466=VERTEX_POINT('',#157926);
#33467=VERTEX_POINT('',#157927);
#33468=VERTEX_POINT('',#157937);
#33469=VERTEX_POINT('',#157939);
#33470=VERTEX_POINT('',#157959);
#33471=VERTEX_POINT('',#157960);
#33472=VERTEX_POINT('',#157970);
#33473=VERTEX_POINT('',#157972);
#33474=VERTEX_POINT('',#157992);
#33475=VERTEX_POINT('',#157993);
#33476=VERTEX_POINT('',#158003);
#33477=VERTEX_POINT('',#158005);
#33478=VERTEX_POINT('',#158025);
#33479=VERTEX_POINT('',#158026);
#33480=VERTEX_POINT('',#158036);
#33481=VERTEX_POINT('',#158038);
#33482=VERTEX_POINT('',#158058);
#33483=VERTEX_POINT('',#158059);
#33484=VERTEX_POINT('',#158069);
#33485=VERTEX_POINT('',#158071);
#33486=VERTEX_POINT('',#158091);
#33487=VERTEX_POINT('',#158092);
#33488=VERTEX_POINT('',#158102);
#33489=VERTEX_POINT('',#158104);
#33490=VERTEX_POINT('',#160607);
#33491=VERTEX_POINT('',#160632);
#33492=VERTEX_POINT('',#160657);
#33493=VERTEX_POINT('',#160682);
#33494=VERTEX_POINT('',#160707);
#33495=VERTEX_POINT('',#160732);
#33496=VERTEX_POINT('',#160757);
#33497=VERTEX_POINT('',#160782);
#33498=VERTEX_POINT('',#160807);
#33499=VERTEX_POINT('',#160832);
#33500=VERTEX_POINT('',#160857);
#33501=VERTEX_POINT('',#160882);
#33502=VERTEX_POINT('',#160907);
#33503=VERTEX_POINT('',#160932);
#33504=VERTEX_POINT('',#160957);
#33505=VERTEX_POINT('',#160982);
#33506=VERTEX_POINT('',#161007);
#33507=VERTEX_POINT('',#161032);
#33508=VERTEX_POINT('',#161057);
#33509=VERTEX_POINT('',#161082);
#33510=VERTEX_POINT('',#161107);
#33511=VERTEX_POINT('',#161132);
#33512=VERTEX_POINT('',#161157);
#33513=VERTEX_POINT('',#161182);
#33514=VERTEX_POINT('',#161207);
#33515=VERTEX_POINT('',#161232);
#33516=VERTEX_POINT('',#161257);
#33517=VERTEX_POINT('',#161282);
#33518=VERTEX_POINT('',#161307);
#33519=VERTEX_POINT('',#161336);
#33520=VERTEX_POINT('',#161337);
#33521=VERTEX_POINT('',#161352);
#33522=VERTEX_POINT('',#161353);
#33523=VERTEX_POINT('',#161363);
#33524=VERTEX_POINT('',#161364);
#33525=VERTEX_POINT('',#161366);
#33526=VERTEX_POINT('',#161379);
#33527=VERTEX_POINT('',#161391);
#33528=VERTEX_POINT('',#161392);
#33529=VERTEX_POINT('',#161402);
#33530=VERTEX_POINT('',#161403);
#33531=VERTEX_POINT('',#161405);
#33532=VERTEX_POINT('',#161418);
#33533=VERTEX_POINT('',#161430);
#33534=VERTEX_POINT('',#161431);
#33535=VERTEX_POINT('',#161441);
#33536=VERTEX_POINT('',#161442);
#33537=VERTEX_POINT('',#161444);
#33538=VERTEX_POINT('',#161457);
#33539=VERTEX_POINT('',#161469);
#33540=VERTEX_POINT('',#161470);
#33541=VERTEX_POINT('',#161480);
#33542=VERTEX_POINT('',#161481);
#33543=VERTEX_POINT('',#161483);
#33544=VERTEX_POINT('',#161496);
#33545=VERTEX_POINT('',#161508);
#33546=VERTEX_POINT('',#161509);
#33547=VERTEX_POINT('',#161519);
#33548=VERTEX_POINT('',#161520);
#33549=VERTEX_POINT('',#161522);
#33550=VERTEX_POINT('',#161535);
#33551=VERTEX_POINT('',#161547);
#33552=VERTEX_POINT('',#161548);
#33553=VERTEX_POINT('',#161558);
#33554=VERTEX_POINT('',#161559);
#33555=VERTEX_POINT('',#161561);
#33556=VERTEX_POINT('',#161574);
#33557=VERTEX_POINT('',#161594);
#33558=VERTEX_POINT('',#161614);
#33559=VERTEX_POINT('',#161615);
#33560=VERTEX_POINT('',#161625);
#33561=VERTEX_POINT('',#161626);
#33562=VERTEX_POINT('',#161628);
#33563=VERTEX_POINT('',#161641);
#33564=VERTEX_POINT('',#161653);
#33565=VERTEX_POINT('',#161654);
#33566=VERTEX_POINT('',#161664);
#33567=VERTEX_POINT('',#161665);
#33568=VERTEX_POINT('',#161667);
#33569=VERTEX_POINT('',#161680);
#33570=VERTEX_POINT('',#161692);
#33571=VERTEX_POINT('',#161693);
#33572=VERTEX_POINT('',#161703);
#33573=VERTEX_POINT('',#161704);
#33574=VERTEX_POINT('',#161706);
#33575=VERTEX_POINT('',#161719);
#33576=VERTEX_POINT('',#161731);
#33577=VERTEX_POINT('',#161732);
#33578=VERTEX_POINT('',#161742);
#33579=VERTEX_POINT('',#161743);
#33580=VERTEX_POINT('',#161745);
#33581=VERTEX_POINT('',#161758);
#33582=VERTEX_POINT('',#161770);
#33583=VERTEX_POINT('',#161771);
#33584=VERTEX_POINT('',#161781);
#33585=VERTEX_POINT('',#161782);
#33586=VERTEX_POINT('',#161784);
#33587=VERTEX_POINT('',#161797);
#33588=VERTEX_POINT('',#161809);
#33589=VERTEX_POINT('',#161810);
#33590=VERTEX_POINT('',#161820);
#33591=VERTEX_POINT('',#161821);
#33592=VERTEX_POINT('',#161823);
#33593=VERTEX_POINT('',#161836);
#33594=VERTEX_POINT('',#161848);
#33595=VERTEX_POINT('',#161849);
#33596=VERTEX_POINT('',#161859);
#33597=VERTEX_POINT('',#161860);
#33598=VERTEX_POINT('',#161862);
#33599=VERTEX_POINT('',#161875);
#33600=VERTEX_POINT('',#161887);
#33601=VERTEX_POINT('',#161888);
#33602=VERTEX_POINT('',#161898);
#33603=VERTEX_POINT('',#161899);
#33604=VERTEX_POINT('',#161901);
#33605=VERTEX_POINT('',#161914);
#33606=VERTEX_POINT('',#161926);
#33607=VERTEX_POINT('',#161927);
#33608=VERTEX_POINT('',#161937);
#33609=VERTEX_POINT('',#161938);
#33610=VERTEX_POINT('',#161940);
#33611=VERTEX_POINT('',#161953);
#33612=VERTEX_POINT('',#161965);
#33613=VERTEX_POINT('',#161966);
#33614=VERTEX_POINT('',#161976);
#33615=VERTEX_POINT('',#161977);
#33616=VERTEX_POINT('',#161979);
#33617=VERTEX_POINT('',#161992);
#33618=VERTEX_POINT('',#162004);
#33619=VERTEX_POINT('',#162006);
#33620=VERTEX_POINT('',#162015);
#33621=VERTEX_POINT('',#162016);
#33622=VERTEX_POINT('',#162018);
#33623=VERTEX_POINT('',#162031);
#33624=VERTEX_POINT('',#162043);
#33625=VERTEX_POINT('',#162044);
#33626=VERTEX_POINT('',#162054);
#33627=VERTEX_POINT('',#162055);
#33628=VERTEX_POINT('',#162057);
#33629=VERTEX_POINT('',#162070);
#33630=VERTEX_POINT('',#162082);
#33631=VERTEX_POINT('',#162083);
#33632=VERTEX_POINT('',#162093);
#33633=VERTEX_POINT('',#162094);
#33634=VERTEX_POINT('',#162096);
#33635=VERTEX_POINT('',#162109);
#33636=VERTEX_POINT('',#162121);
#33637=VERTEX_POINT('',#162122);
#33638=VERTEX_POINT('',#162132);
#33639=VERTEX_POINT('',#162133);
#33640=VERTEX_POINT('',#162135);
#33641=VERTEX_POINT('',#162148);
#33642=VERTEX_POINT('',#162160);
#33643=VERTEX_POINT('',#162161);
#33644=VERTEX_POINT('',#162171);
#33645=VERTEX_POINT('',#162172);
#33646=VERTEX_POINT('',#162174);
#33647=VERTEX_POINT('',#162187);
#33648=VERTEX_POINT('',#162199);
#33649=VERTEX_POINT('',#162200);
#33650=VERTEX_POINT('',#162210);
#33651=VERTEX_POINT('',#162211);
#33652=VERTEX_POINT('',#162213);
#33653=VERTEX_POINT('',#162226);
#33654=VERTEX_POINT('',#162238);
#33655=VERTEX_POINT('',#162239);
#33656=VERTEX_POINT('',#162249);
#33657=VERTEX_POINT('',#162250);
#33658=VERTEX_POINT('',#162252);
#33659=VERTEX_POINT('',#162265);
#33660=VERTEX_POINT('',#162277);
#33661=VERTEX_POINT('',#162278);
#33662=VERTEX_POINT('',#162288);
#33663=VERTEX_POINT('',#162289);
#33664=VERTEX_POINT('',#162291);
#33665=VERTEX_POINT('',#162304);
#33666=VERTEX_POINT('',#162316);
#33667=VERTEX_POINT('',#162317);
#33668=VERTEX_POINT('',#162327);
#33669=VERTEX_POINT('',#162328);
#33670=VERTEX_POINT('',#162330);
#33671=VERTEX_POINT('',#162343);
#33672=VERTEX_POINT('',#162355);
#33673=VERTEX_POINT('',#162356);
#33674=VERTEX_POINT('',#162366);
#33675=VERTEX_POINT('',#162367);
#33676=VERTEX_POINT('',#162369);
#33677=VERTEX_POINT('',#162382);
#33678=VERTEX_POINT('',#162394);
#33679=VERTEX_POINT('',#162395);
#33680=VERTEX_POINT('',#162405);
#33681=VERTEX_POINT('',#162406);
#33682=VERTEX_POINT('',#162408);
#33683=VERTEX_POINT('',#162421);
#33684=VERTEX_POINT('',#162428);
#33685=VERTEX_POINT('',#162429);
#33686=VERTEX_POINT('',#162431);
#33687=VERTEX_POINT('',#162436);
#33688=VERTEX_POINT('',#162457);
#33689=VERTEX_POINT('',#162466);
#33690=VERTEX_POINT('',#162486);
#33691=VERTEX_POINT('',#162506);
#33692=VERTEX_POINT('',#162526);
#33693=VERTEX_POINT('',#162546);
#33694=VERTEX_POINT('',#162566);
#33695=VERTEX_POINT('',#162586);
#33696=VERTEX_POINT('',#162606);
#33697=VERTEX_POINT('',#162626);
#33698=VERTEX_POINT('',#162646);
#33699=VERTEX_POINT('',#162666);
#33700=VERTEX_POINT('',#162686);
#33701=VERTEX_POINT('',#162706);
#33702=VERTEX_POINT('',#162726);
#33703=VERTEX_POINT('',#162746);
#33704=VERTEX_POINT('',#162766);
#33705=VERTEX_POINT('',#162786);
#33706=VERTEX_POINT('',#162806);
#33707=VERTEX_POINT('',#162826);
#33708=VERTEX_POINT('',#162846);
#33709=VERTEX_POINT('',#162866);
#33710=VERTEX_POINT('',#162886);
#33711=VERTEX_POINT('',#162906);
#33712=VERTEX_POINT('',#162926);
#33713=VERTEX_POINT('',#162946);
#33714=VERTEX_POINT('',#162966);
#33715=VERTEX_POINT('',#162986);
#33716=VERTEX_POINT('',#163006);
#33717=VERTEX_POINT('',#163036);
#33718=VERTEX_POINT('',#163038);
#33719=VERTEX_POINT('',#163052);
#33720=VERTEX_POINT('',#163053);
#33721=VERTEX_POINT('',#163095);
#33722=VERTEX_POINT('',#163097);
#33723=VERTEX_POINT('',#163111);
#33724=VERTEX_POINT('',#163112);
#33725=VERTEX_POINT('',#163154);
#33726=VERTEX_POINT('',#163156);
#33727=VERTEX_POINT('',#163170);
#33728=VERTEX_POINT('',#163171);
#33729=VERTEX_POINT('',#163213);
#33730=VERTEX_POINT('',#163215);
#33731=VERTEX_POINT('',#163229);
#33732=VERTEX_POINT('',#163230);
#33733=VERTEX_POINT('',#163272);
#33734=VERTEX_POINT('',#163274);
#33735=VERTEX_POINT('',#163288);
#33736=VERTEX_POINT('',#163289);
#33737=VERTEX_POINT('',#163331);
#33738=VERTEX_POINT('',#163333);
#33739=VERTEX_POINT('',#163347);
#33740=VERTEX_POINT('',#163348);
#33741=VERTEX_POINT('',#163390);
#33742=VERTEX_POINT('',#163392);
#33743=VERTEX_POINT('',#163406);
#33744=VERTEX_POINT('',#163407);
#33745=VERTEX_POINT('',#163449);
#33746=VERTEX_POINT('',#163451);
#33747=VERTEX_POINT('',#163465);
#33748=VERTEX_POINT('',#163466);
#33749=VERTEX_POINT('',#163508);
#33750=VERTEX_POINT('',#163510);
#33751=VERTEX_POINT('',#163524);
#33752=VERTEX_POINT('',#163525);
#33753=VERTEX_POINT('',#163567);
#33754=VERTEX_POINT('',#163569);
#33755=VERTEX_POINT('',#163583);
#33756=VERTEX_POINT('',#163584);
#33757=VERTEX_POINT('',#163626);
#33758=VERTEX_POINT('',#163628);
#33759=VERTEX_POINT('',#163642);
#33760=VERTEX_POINT('',#163643);
#33761=VERTEX_POINT('',#163685);
#33762=VERTEX_POINT('',#163687);
#33763=VERTEX_POINT('',#163701);
#33764=VERTEX_POINT('',#163702);
#33765=VERTEX_POINT('',#163744);
#33766=VERTEX_POINT('',#163746);
#33767=VERTEX_POINT('',#163760);
#33768=VERTEX_POINT('',#163761);
#33769=VERTEX_POINT('',#163803);
#33770=VERTEX_POINT('',#163805);
#33771=VERTEX_POINT('',#163819);
#33772=VERTEX_POINT('',#163820);
#33773=VERTEX_POINT('',#163862);
#33774=VERTEX_POINT('',#163864);
#33775=VERTEX_POINT('',#163878);
#33776=VERTEX_POINT('',#163879);
#33777=VERTEX_POINT('',#163921);
#33778=VERTEX_POINT('',#163923);
#33779=VERTEX_POINT('',#163937);
#33780=VERTEX_POINT('',#163938);
#33781=VERTEX_POINT('',#163980);
#33782=VERTEX_POINT('',#163982);
#33783=VERTEX_POINT('',#163996);
#33784=VERTEX_POINT('',#163997);
#33785=VERTEX_POINT('',#164039);
#33786=VERTEX_POINT('',#164041);
#33787=VERTEX_POINT('',#164055);
#33788=VERTEX_POINT('',#164064);
#33789=VERTEX_POINT('',#164098);
#33790=VERTEX_POINT('',#164100);
#33791=VERTEX_POINT('',#164114);
#33792=VERTEX_POINT('',#164115);
#33793=VERTEX_POINT('',#164157);
#33794=VERTEX_POINT('',#164159);
#33795=VERTEX_POINT('',#164173);
#33796=VERTEX_POINT('',#164174);
#33797=VERTEX_POINT('',#164216);
#33798=VERTEX_POINT('',#164218);
#33799=VERTEX_POINT('',#164232);
#33800=VERTEX_POINT('',#164233);
#33801=VERTEX_POINT('',#164301);
#33802=VERTEX_POINT('',#164303);
#33803=VERTEX_POINT('',#164317);
#33804=VERTEX_POINT('',#164318);
#33805=VERTEX_POINT('',#164360);
#33806=VERTEX_POINT('',#164362);
#33807=VERTEX_POINT('',#164376);
#33808=VERTEX_POINT('',#164377);
#33809=VERTEX_POINT('',#164419);
#33810=VERTEX_POINT('',#164421);
#33811=VERTEX_POINT('',#164435);
#33812=VERTEX_POINT('',#164436);
#33813=VERTEX_POINT('',#164478);
#33814=VERTEX_POINT('',#164480);
#33815=VERTEX_POINT('',#164494);
#33816=VERTEX_POINT('',#164495);
#33817=VERTEX_POINT('',#164537);
#33818=VERTEX_POINT('',#164539);
#33819=VERTEX_POINT('',#164553);
#33820=VERTEX_POINT('',#164554);
#33821=VERTEX_POINT('',#164596);
#33822=VERTEX_POINT('',#164598);
#33823=VERTEX_POINT('',#164612);
#33824=VERTEX_POINT('',#164613);
#33825=VERTEX_POINT('',#164686);
#33826=VERTEX_POINT('',#164721);
#33827=VERTEX_POINT('',#164752);
#33828=VERTEX_POINT('',#164780);
#33829=VERTEX_POINT('',#164808);
#33830=VERTEX_POINT('',#164836);
#33831=VERTEX_POINT('',#164864);
#33832=VERTEX_POINT('',#164899);
#33833=VERTEX_POINT('',#164930);
#33834=VERTEX_POINT('',#164958);
#33835=VERTEX_POINT('',#164986);
#33836=VERTEX_POINT('',#165014);
#33837=VERTEX_POINT('',#165049);
#33838=VERTEX_POINT('',#165080);
#33839=VERTEX_POINT('',#165108);
#33840=VERTEX_POINT('',#165143);
#33841=VERTEX_POINT('',#165174);
#33842=VERTEX_POINT('',#165209);
#33843=VERTEX_POINT('',#165240);
#33844=VERTEX_POINT('',#165268);
#33845=VERTEX_POINT('',#165303);
#33846=VERTEX_POINT('',#165341);
#33847=VERTEX_POINT('',#165372);
#33848=VERTEX_POINT('',#165400);
#33849=VERTEX_POINT('',#165428);
#33850=VERTEX_POINT('',#165456);
#33851=VERTEX_POINT('',#165484);
#33852=VERTEX_POINT('',#165512);
#33853=VERTEX_POINT('',#165540);
#33964=EDGE_CURVE('',#28533,#28534,#24357,.T.);
#33965=EDGE_CURVE('',#28535,#28533,#21046,.F.);
#33966=EDGE_CURVE('',#28536,#28535,#21047,.T.);
#33967=EDGE_CURVE('',#28537,#28536,#15929,.T.);
#33968=EDGE_CURVE('',#28538,#28537,#15930,.T.);
#33969=EDGE_CURVE('',#28539,#28538,#21048,.T.);
#33970=EDGE_CURVE('',#28540,#28539,#21049,.T.);
#33971=EDGE_CURVE('',#28541,#28540,#21050,.T.);
#33972=EDGE_CURVE('',#28542,#28541,#21051,.T.);
#33973=EDGE_CURVE('',#28543,#28542,#15931,.T.);
#33974=EDGE_CURVE('',#28544,#28543,#15932,.T.);
#33975=EDGE_CURVE('',#28545,#28544,#21052,.T.);
#33976=EDGE_CURVE('',#28546,#28545,#21053,.T.);
#33977=EDGE_CURVE('',#28547,#28546,#21054,.T.);
#33978=EDGE_CURVE('',#28548,#28547,#21055,.T.);
#33979=EDGE_CURVE('',#28549,#28548,#15933,.T.);
#33980=EDGE_CURVE('',#28550,#28549,#15934,.T.);
#33981=EDGE_CURVE('',#28551,#28550,#21056,.T.);
#33982=EDGE_CURVE('',#28552,#28551,#21057,.T.);
#33983=EDGE_CURVE('',#28553,#28552,#21058,.T.);
#33984=EDGE_CURVE('',#28554,#28553,#21059,.T.);
#33985=EDGE_CURVE('',#28555,#28554,#15935,.T.);
#33986=EDGE_CURVE('',#28556,#28555,#15936,.T.);
#33987=EDGE_CURVE('',#28557,#28556,#21060,.T.);
#33988=EDGE_CURVE('',#28558,#28557,#21061,.T.);
#33989=EDGE_CURVE('',#28559,#28558,#21062,.T.);
#33990=EDGE_CURVE('',#28560,#28559,#21063,.T.);
#33991=EDGE_CURVE('',#28561,#28560,#15937,.T.);
#33992=EDGE_CURVE('',#28562,#28561,#15938,.T.);
#33993=EDGE_CURVE('',#28563,#28562,#21064,.T.);
#33994=EDGE_CURVE('',#28564,#28563,#21065,.T.);
#33995=EDGE_CURVE('',#28565,#28564,#21066,.T.);
#33996=EDGE_CURVE('',#28566,#28565,#21067,.T.);
#33997=EDGE_CURVE('',#28567,#28566,#15939,.T.);
#33998=EDGE_CURVE('',#28568,#28567,#15940,.T.);
#33999=EDGE_CURVE('',#28569,#28568,#21068,.T.);
#34000=EDGE_CURVE('',#28570,#28569,#21069,.T.);
#34001=EDGE_CURVE('',#28571,#28570,#21070,.T.);
#34002=EDGE_CURVE('',#28572,#28571,#21071,.T.);
#34003=EDGE_CURVE('',#28573,#28572,#15941,.T.);
#34004=EDGE_CURVE('',#28574,#28573,#15942,.T.);
#34005=EDGE_CURVE('',#28575,#28574,#21072,.T.);
#34006=EDGE_CURVE('',#28576,#28575,#21073,.T.);
#34007=EDGE_CURVE('',#28577,#28576,#21074,.T.);
#34008=EDGE_CURVE('',#28578,#28577,#21075,.T.);
#34009=EDGE_CURVE('',#28579,#28578,#15943,.T.);
#34010=EDGE_CURVE('',#28580,#28579,#15944,.T.);
#34011=EDGE_CURVE('',#28581,#28580,#21076,.T.);
#34012=EDGE_CURVE('',#28582,#28581,#21077,.T.);
#34013=EDGE_CURVE('',#28583,#28582,#21078,.T.);
#34014=EDGE_CURVE('',#28584,#28583,#21079,.T.);
#34015=EDGE_CURVE('',#28585,#28584,#15945,.T.);
#34016=EDGE_CURVE('',#28586,#28585,#15946,.T.);
#34017=EDGE_CURVE('',#28587,#28586,#21080,.T.);
#34018=EDGE_CURVE('',#28588,#28587,#21081,.T.);
#34019=EDGE_CURVE('',#28589,#28588,#21082,.T.);
#34020=EDGE_CURVE('',#28590,#28589,#21083,.T.);
#34021=EDGE_CURVE('',#28591,#28590,#15947,.T.);
#34022=EDGE_CURVE('',#28592,#28591,#15948,.T.);
#34023=EDGE_CURVE('',#28593,#28592,#21084,.T.);
#34024=EDGE_CURVE('',#28594,#28593,#21085,.T.);
#34025=EDGE_CURVE('',#28595,#28594,#21086,.T.);
#34026=EDGE_CURVE('',#28596,#28595,#21087,.T.);
#34027=EDGE_CURVE('',#28597,#28596,#15949,.T.);
#34028=EDGE_CURVE('',#28598,#28597,#15950,.T.);
#34029=EDGE_CURVE('',#28599,#28598,#21088,.T.);
#34030=EDGE_CURVE('',#28600,#28599,#21089,.T.);
#34031=EDGE_CURVE('',#28601,#28600,#21090,.T.);
#34032=EDGE_CURVE('',#28602,#28601,#21091,.T.);
#34033=EDGE_CURVE('',#28603,#28602,#15951,.T.);
#34034=EDGE_CURVE('',#28604,#28603,#15952,.T.);
#34035=EDGE_CURVE('',#28605,#28604,#21092,.T.);
#34036=EDGE_CURVE('',#28606,#28605,#21093,.T.);
#34037=EDGE_CURVE('',#28607,#28606,#21094,.T.);
#34038=EDGE_CURVE('',#28608,#28607,#21095,.T.);
#34039=EDGE_CURVE('',#28609,#28608,#15953,.T.);
#34040=EDGE_CURVE('',#28610,#28609,#15954,.T.);
#34041=EDGE_CURVE('',#28611,#28610,#21096,.T.);
#34042=EDGE_CURVE('',#28612,#28611,#21097,.T.);
#34043=EDGE_CURVE('',#28613,#28612,#21098,.T.);
#34044=EDGE_CURVE('',#28614,#28613,#21099,.T.);
#34045=EDGE_CURVE('',#28615,#28614,#15955,.T.);
#34046=EDGE_CURVE('',#28616,#28615,#15956,.T.);
#34047=EDGE_CURVE('',#28617,#28616,#21100,.T.);
#34048=EDGE_CURVE('',#28618,#28617,#21101,.T.);
#34049=EDGE_CURVE('',#28619,#28618,#21102,.T.);
#34050=EDGE_CURVE('',#28620,#28619,#21103,.T.);
#34051=EDGE_CURVE('',#28621,#28620,#15957,.T.);
#34052=EDGE_CURVE('',#28622,#28621,#15958,.T.);
#34053=EDGE_CURVE('',#28623,#28622,#21104,.T.);
#34054=EDGE_CURVE('',#28624,#28623,#21105,.T.);
#34055=EDGE_CURVE('',#28625,#28624,#21106,.T.);
#34056=EDGE_CURVE('',#28626,#28625,#21107,.T.);
#34057=EDGE_CURVE('',#28627,#28626,#15959,.T.);
#34058=EDGE_CURVE('',#28628,#28627,#15960,.T.);
#34059=EDGE_CURVE('',#28629,#28628,#21108,.T.);
#34060=EDGE_CURVE('',#28630,#28629,#21109,.T.);
#34061=EDGE_CURVE('',#28631,#28630,#21110,.T.);
#34062=EDGE_CURVE('',#28632,#28631,#21111,.T.);
#34063=EDGE_CURVE('',#28633,#28632,#15961,.T.);
#34064=EDGE_CURVE('',#28634,#28633,#15962,.T.);
#34065=EDGE_CURVE('',#28635,#28634,#21112,.T.);
#34066=EDGE_CURVE('',#28636,#28635,#21113,.T.);
#34067=EDGE_CURVE('',#28637,#28636,#21114,.T.);
#34068=EDGE_CURVE('',#28638,#28637,#21115,.T.);
#34069=EDGE_CURVE('',#28639,#28638,#15963,.T.);
#34070=EDGE_CURVE('',#28640,#28639,#15964,.T.);
#34071=EDGE_CURVE('',#28641,#28640,#21116,.T.);
#34072=EDGE_CURVE('',#28642,#28641,#21117,.T.);
#34073=EDGE_CURVE('',#28643,#28642,#21118,.T.);
#34074=EDGE_CURVE('',#28644,#28643,#21119,.T.);
#34075=EDGE_CURVE('',#28645,#28644,#15965,.T.);
#34076=EDGE_CURVE('',#28646,#28645,#15966,.T.);
#34077=EDGE_CURVE('',#28647,#28646,#21120,.T.);
#34078=EDGE_CURVE('',#28648,#28647,#21121,.T.);
#34079=EDGE_CURVE('',#28649,#28648,#21122,.T.);
#34080=EDGE_CURVE('',#28650,#28649,#21123,.T.);
#34081=EDGE_CURVE('',#28651,#28650,#15967,.T.);
#34082=EDGE_CURVE('',#28652,#28651,#15968,.T.);
#34083=EDGE_CURVE('',#28653,#28652,#21124,.T.);
#34084=EDGE_CURVE('',#28654,#28653,#21125,.T.);
#34085=EDGE_CURVE('',#28655,#28654,#21126,.T.);
#34086=EDGE_CURVE('',#28656,#28655,#21127,.T.);
#34087=EDGE_CURVE('',#28657,#28656,#15969,.T.);
#34088=EDGE_CURVE('',#28658,#28657,#15970,.T.);
#34089=EDGE_CURVE('',#28659,#28658,#21128,.T.);
#34090=EDGE_CURVE('',#28660,#28659,#21129,.T.);
#34091=EDGE_CURVE('',#28661,#28660,#21130,.T.);
#34092=EDGE_CURVE('',#28662,#28661,#21131,.T.);
#34093=EDGE_CURVE('',#28663,#28662,#15971,.T.);
#34094=EDGE_CURVE('',#28664,#28663,#15972,.T.);
#34095=EDGE_CURVE('',#28665,#28664,#21132,.T.);
#34096=EDGE_CURVE('',#28666,#28665,#21133,.T.);
#34097=EDGE_CURVE('',#28667,#28666,#21134,.T.);
#34098=EDGE_CURVE('',#28668,#28667,#21135,.T.);
#34099=EDGE_CURVE('',#28669,#28668,#15973,.T.);
#34100=EDGE_CURVE('',#28670,#28669,#15974,.T.);
#34101=EDGE_CURVE('',#28671,#28670,#21136,.T.);
#34102=EDGE_CURVE('',#28672,#28671,#21137,.T.);
#34103=EDGE_CURVE('',#28673,#28672,#21138,.T.);
#34104=EDGE_CURVE('',#28674,#28673,#21139,.T.);
#34105=EDGE_CURVE('',#28675,#28674,#15975,.T.);
#34106=EDGE_CURVE('',#28676,#28675,#15976,.T.);
#34107=EDGE_CURVE('',#28677,#28676,#21140,.T.);
#34108=EDGE_CURVE('',#28678,#28677,#21141,.T.);
#34109=EDGE_CURVE('',#28679,#28678,#21142,.T.);
#34110=EDGE_CURVE('',#28680,#28679,#21143,.T.);
#34111=EDGE_CURVE('',#28681,#28680,#15977,.T.);
#34112=EDGE_CURVE('',#28682,#28681,#15978,.T.);
#34113=EDGE_CURVE('',#28683,#28682,#21144,.T.);
#34114=EDGE_CURVE('',#28684,#28683,#21145,.T.);
#34115=EDGE_CURVE('',#28685,#28684,#21146,.T.);
#34116=EDGE_CURVE('',#28686,#28685,#21147,.T.);
#34117=EDGE_CURVE('',#28687,#28686,#15979,.T.);
#34118=EDGE_CURVE('',#28688,#28687,#15980,.T.);
#34119=EDGE_CURVE('',#28689,#28688,#21148,.T.);
#34120=EDGE_CURVE('',#28690,#28689,#21149,.T.);
#34121=EDGE_CURVE('',#28691,#28690,#21150,.T.);
#34122=EDGE_CURVE('',#28692,#28691,#21151,.T.);
#34123=EDGE_CURVE('',#28693,#28692,#15981,.T.);
#34124=EDGE_CURVE('',#28694,#28693,#15982,.T.);
#34125=EDGE_CURVE('',#28695,#28694,#21152,.T.);
#34126=EDGE_CURVE('',#28696,#28695,#21153,.T.);
#34127=EDGE_CURVE('',#28697,#28696,#21154,.T.);
#34128=EDGE_CURVE('',#28698,#28697,#21155,.T.);
#34129=EDGE_CURVE('',#28699,#28698,#15983,.T.);
#34130=EDGE_CURVE('',#28700,#28699,#15984,.T.);
#34131=EDGE_CURVE('',#28701,#28700,#21156,.T.);
#34132=EDGE_CURVE('',#28702,#28701,#21157,.T.);
#34133=EDGE_CURVE('',#28703,#28702,#21158,.T.);
#34134=EDGE_CURVE('',#28704,#28703,#21159,.T.);
#34135=EDGE_CURVE('',#28705,#28704,#15985,.T.);
#34136=EDGE_CURVE('',#28706,#28705,#15986,.T.);
#34137=EDGE_CURVE('',#28707,#28706,#21160,.F.);
#34138=EDGE_CURVE('',#28707,#28708,#24358,.T.);
#34139=EDGE_CURVE('',#28708,#28708,#15987,.T.);
#34140=EDGE_CURVE('',#28709,#28707,#21161,.F.);
#34141=EDGE_CURVE('',#28534,#28709,#21162,.F.);
#34142=EDGE_CURVE('',#28710,#28710,#15988,.T.);
#34143=EDGE_CURVE('',#28710,#28711,#24359,.T.);
#34144=EDGE_CURVE('',#28711,#28711,#15989,.T.);
#34145=EDGE_CURVE('',#28712,#28534,#21163,.F.);
#34146=EDGE_CURVE('',#28533,#28712,#21164,.F.);
#34147=EDGE_CURVE('',#28713,#28713,#15990,.T.);
#34148=EDGE_CURVE('',#28713,#28714,#24360,.T.);
#34149=EDGE_CURVE('',#28714,#28714,#15991,.T.);
#34150=EDGE_CURVE('',#28715,#28716,#15992,.T.);
#34151=EDGE_CURVE('',#28716,#28717,#24361,.T.);
#34152=EDGE_CURVE('',#28717,#28717,#15993,.T.);
#34153=EDGE_CURVE('',#28716,#28715,#15994,.T.);
#34154=EDGE_CURVE('',#28715,#28718,#24362,.T.);
#34155=EDGE_CURVE('',#28718,#28718,#15995,.T.);
#34156=EDGE_CURVE('',#28719,#28720,#21165,.T.);
#34157=EDGE_CURVE('',#28721,#28719,#15996,.T.);
#34158=EDGE_CURVE('',#28722,#28721,#15997,.T.);
#34159=EDGE_CURVE('',#28723,#28722,#21166,.T.);
#34160=EDGE_CURVE('',#28724,#28723,#21167,.T.);
#34161=EDGE_CURVE('',#28725,#28724,#21168,.T.);
#34162=EDGE_CURVE('',#28726,#28725,#21169,.T.);
#34163=EDGE_CURVE('',#28727,#28726,#15998,.T.);
#34164=EDGE_CURVE('',#28728,#28727,#15999,.T.);
#34165=EDGE_CURVE('',#28729,#28728,#21170,.T.);
#34166=EDGE_CURVE('',#28730,#28729,#21171,.T.);
#34167=EDGE_CURVE('',#28731,#28730,#21172,.T.);
#34168=EDGE_CURVE('',#28732,#28731,#21173,.T.);
#34169=EDGE_CURVE('',#28733,#28732,#16000,.T.);
#34170=EDGE_CURVE('',#28734,#28733,#16001,.T.);
#34171=EDGE_CURVE('',#28735,#28734,#21174,.T.);
#34172=EDGE_CURVE('',#28736,#28735,#21175,.T.);
#34173=EDGE_CURVE('',#28737,#28736,#21176,.T.);
#34174=EDGE_CURVE('',#28738,#28737,#21177,.T.);
#34175=EDGE_CURVE('',#28739,#28738,#16002,.T.);
#34176=EDGE_CURVE('',#28740,#28739,#16003,.T.);
#34177=EDGE_CURVE('',#28741,#28740,#21178,.T.);
#34178=EDGE_CURVE('',#28742,#28741,#21179,.T.);
#34179=EDGE_CURVE('',#28743,#28742,#21180,.T.);
#34180=EDGE_CURVE('',#28744,#28743,#21181,.T.);
#34181=EDGE_CURVE('',#28745,#28744,#16004,.T.);
#34182=EDGE_CURVE('',#28746,#28745,#16005,.T.);
#34183=EDGE_CURVE('',#28747,#28746,#21182,.T.);
#34184=EDGE_CURVE('',#28748,#28747,#21183,.T.);
#34185=EDGE_CURVE('',#28749,#28748,#21184,.T.);
#34186=EDGE_CURVE('',#28750,#28749,#21185,.T.);
#34187=EDGE_CURVE('',#28751,#28750,#16006,.T.);
#34188=EDGE_CURVE('',#28752,#28751,#16007,.T.);
#34189=EDGE_CURVE('',#28753,#28752,#21186,.T.);
#34190=EDGE_CURVE('',#28754,#28753,#21187,.T.);
#34191=EDGE_CURVE('',#28755,#28754,#21188,.T.);
#34192=EDGE_CURVE('',#28756,#28755,#21189,.T.);
#34193=EDGE_CURVE('',#28757,#28756,#16008,.T.);
#34194=EDGE_CURVE('',#28758,#28757,#16009,.T.);
#34195=EDGE_CURVE('',#28759,#28758,#21190,.T.);
#34196=EDGE_CURVE('',#28760,#28759,#21191,.T.);
#34197=EDGE_CURVE('',#28761,#28760,#21192,.T.);
#34198=EDGE_CURVE('',#28762,#28761,#21193,.T.);
#34199=EDGE_CURVE('',#28763,#28762,#16010,.T.);
#34200=EDGE_CURVE('',#28764,#28763,#16011,.T.);
#34201=EDGE_CURVE('',#28765,#28764,#21194,.T.);
#34202=EDGE_CURVE('',#28766,#28765,#21195,.T.);
#34203=EDGE_CURVE('',#28767,#28766,#21196,.T.);
#34204=EDGE_CURVE('',#28768,#28767,#21197,.T.);
#34205=EDGE_CURVE('',#28769,#28768,#16012,.T.);
#34206=EDGE_CURVE('',#28770,#28769,#16013,.T.);
#34207=EDGE_CURVE('',#28771,#28770,#21198,.T.);
#34208=EDGE_CURVE('',#28772,#28771,#21199,.T.);
#34209=EDGE_CURVE('',#28773,#28772,#21200,.T.);
#34210=EDGE_CURVE('',#28774,#28773,#21201,.T.);
#34211=EDGE_CURVE('',#28775,#28774,#16014,.T.);
#34212=EDGE_CURVE('',#28776,#28775,#16015,.T.);
#34213=EDGE_CURVE('',#28777,#28776,#21202,.T.);
#34214=EDGE_CURVE('',#28778,#28777,#21203,.T.);
#34215=EDGE_CURVE('',#28779,#28778,#21204,.T.);
#34216=EDGE_CURVE('',#28780,#28779,#21205,.T.);
#34217=EDGE_CURVE('',#28781,#28780,#16016,.T.);
#34218=EDGE_CURVE('',#28782,#28781,#16017,.T.);
#34219=EDGE_CURVE('',#28783,#28782,#21206,.T.);
#34220=EDGE_CURVE('',#28784,#28783,#21207,.T.);
#34221=EDGE_CURVE('',#28785,#28784,#21208,.T.);
#34222=EDGE_CURVE('',#28786,#28785,#21209,.T.);
#34223=EDGE_CURVE('',#28787,#28786,#16018,.T.);
#34224=EDGE_CURVE('',#28788,#28787,#16019,.T.);
#34225=EDGE_CURVE('',#28789,#28788,#21210,.T.);
#34226=EDGE_CURVE('',#28790,#28789,#21211,.T.);
#34227=EDGE_CURVE('',#28791,#28790,#21212,.T.);
#34228=EDGE_CURVE('',#28792,#28791,#21213,.T.);
#34229=EDGE_CURVE('',#28793,#28792,#16020,.T.);
#34230=EDGE_CURVE('',#28794,#28793,#16021,.T.);
#34231=EDGE_CURVE('',#28795,#28794,#21214,.T.);
#34232=EDGE_CURVE('',#28796,#28795,#21215,.T.);
#34233=EDGE_CURVE('',#28797,#28796,#21216,.T.);
#34234=EDGE_CURVE('',#28798,#28797,#21217,.T.);
#34235=EDGE_CURVE('',#28799,#28798,#16022,.T.);
#34236=EDGE_CURVE('',#28800,#28799,#16023,.T.);
#34237=EDGE_CURVE('',#28801,#28800,#21218,.T.);
#34238=EDGE_CURVE('',#28802,#28801,#21219,.T.);
#34239=EDGE_CURVE('',#28803,#28802,#21220,.T.);
#34240=EDGE_CURVE('',#28804,#28803,#21221,.T.);
#34241=EDGE_CURVE('',#28805,#28804,#16024,.T.);
#34242=EDGE_CURVE('',#28806,#28805,#16025,.T.);
#34243=EDGE_CURVE('',#28807,#28806,#21222,.F.);
#34244=EDGE_CURVE('',#28807,#28808,#24363,.T.);
#34245=EDGE_CURVE('',#28808,#28808,#16026,.T.);
#34246=EDGE_CURVE('',#28809,#28807,#21223,.F.);
#34247=EDGE_CURVE('',#28810,#28809,#21224,.T.);
#34248=EDGE_CURVE('',#28811,#28810,#21225,.T.);
#34249=EDGE_CURVE('',#28812,#28811,#21226,.T.);
#34250=EDGE_CURVE('',#28813,#28812,#16027,.T.);
#34251=EDGE_CURVE('',#28814,#28813,#16028,.T.);
#34252=EDGE_CURVE('',#28815,#28814,#21227,.T.);
#34253=EDGE_CURVE('',#28816,#28815,#21228,.T.);
#34254=EDGE_CURVE('',#28817,#28816,#21229,.T.);
#34255=EDGE_CURVE('',#28818,#28817,#21230,.T.);
#34256=EDGE_CURVE('',#28819,#28818,#16029,.T.);
#34257=EDGE_CURVE('',#28820,#28819,#16030,.T.);
#34258=EDGE_CURVE('',#28821,#28820,#21231,.T.);
#34259=EDGE_CURVE('',#28822,#28821,#21232,.T.);
#34260=EDGE_CURVE('',#28823,#28822,#21233,.T.);
#34261=EDGE_CURVE('',#28824,#28823,#21234,.T.);
#34262=EDGE_CURVE('',#28825,#28824,#16031,.T.);
#34263=EDGE_CURVE('',#28826,#28825,#16032,.T.);
#34264=EDGE_CURVE('',#28827,#28826,#21235,.T.);
#34265=EDGE_CURVE('',#28828,#28827,#21236,.T.);
#34266=EDGE_CURVE('',#28829,#28828,#21237,.T.);
#34267=EDGE_CURVE('',#28830,#28829,#21238,.T.);
#34268=EDGE_CURVE('',#28831,#28830,#16033,.T.);
#34269=EDGE_CURVE('',#28832,#28831,#16034,.T.);
#34270=EDGE_CURVE('',#28833,#28832,#21239,.T.);
#34271=EDGE_CURVE('',#28834,#28833,#21240,.T.);
#34272=EDGE_CURVE('',#28835,#28834,#21241,.T.);
#34273=EDGE_CURVE('',#28836,#28835,#21242,.T.);
#34274=EDGE_CURVE('',#28837,#28836,#16035,.T.);
#34275=EDGE_CURVE('',#28838,#28837,#16036,.T.);
#34276=EDGE_CURVE('',#28839,#28838,#21243,.T.);
#34277=EDGE_CURVE('',#28840,#28839,#21244,.T.);
#34278=EDGE_CURVE('',#28841,#28840,#21245,.T.);
#34279=EDGE_CURVE('',#28842,#28841,#21246,.T.);
#34280=EDGE_CURVE('',#28843,#28842,#16037,.T.);
#34281=EDGE_CURVE('',#28844,#28843,#16038,.T.);
#34282=EDGE_CURVE('',#28845,#28844,#21247,.T.);
#34283=EDGE_CURVE('',#28846,#28845,#21248,.T.);
#34284=EDGE_CURVE('',#28847,#28846,#21249,.T.);
#34285=EDGE_CURVE('',#28848,#28847,#21250,.T.);
#34286=EDGE_CURVE('',#28849,#28848,#16039,.T.);
#34287=EDGE_CURVE('',#28850,#28849,#16040,.T.);
#34288=EDGE_CURVE('',#28851,#28850,#21251,.T.);
#34289=EDGE_CURVE('',#28852,#28851,#21252,.T.);
#34290=EDGE_CURVE('',#28853,#28852,#21253,.T.);
#34291=EDGE_CURVE('',#28854,#28853,#21254,.T.);
#34292=EDGE_CURVE('',#28855,#28854,#16041,.T.);
#34293=EDGE_CURVE('',#28856,#28855,#16042,.T.);
#34294=EDGE_CURVE('',#28857,#28856,#21255,.T.);
#34295=EDGE_CURVE('',#28858,#28857,#21256,.T.);
#34296=EDGE_CURVE('',#28859,#28858,#21257,.T.);
#34297=EDGE_CURVE('',#28860,#28859,#21258,.T.);
#34298=EDGE_CURVE('',#28861,#28860,#16043,.T.);
#34299=EDGE_CURVE('',#28862,#28861,#16044,.T.);
#34300=EDGE_CURVE('',#28863,#28862,#21259,.T.);
#34301=EDGE_CURVE('',#28864,#28863,#21260,.T.);
#34302=EDGE_CURVE('',#28865,#28864,#21261,.T.);
#34303=EDGE_CURVE('',#28866,#28865,#21262,.T.);
#34304=EDGE_CURVE('',#28867,#28866,#16045,.T.);
#34305=EDGE_CURVE('',#28868,#28867,#16046,.T.);
#34306=EDGE_CURVE('',#28869,#28868,#21263,.T.);
#34307=EDGE_CURVE('',#28870,#28869,#21264,.T.);
#34308=EDGE_CURVE('',#28871,#28870,#21265,.T.);
#34309=EDGE_CURVE('',#28872,#28871,#21266,.T.);
#34310=EDGE_CURVE('',#28873,#28872,#16047,.T.);
#34311=EDGE_CURVE('',#28874,#28873,#16048,.T.);
#34312=EDGE_CURVE('',#28875,#28874,#21267,.T.);
#34313=EDGE_CURVE('',#28876,#28875,#21268,.T.);
#34314=EDGE_CURVE('',#28877,#28876,#21269,.T.);
#34315=EDGE_CURVE('',#28878,#28877,#21270,.T.);
#34316=EDGE_CURVE('',#28879,#28878,#16049,.T.);
#34317=EDGE_CURVE('',#28880,#28879,#16050,.T.);
#34318=EDGE_CURVE('',#28881,#28880,#21271,.T.);
#34319=EDGE_CURVE('',#28882,#28881,#21272,.T.);
#34320=EDGE_CURVE('',#28883,#28882,#21273,.T.);
#34321=EDGE_CURVE('',#28884,#28883,#21274,.T.);
#34322=EDGE_CURVE('',#28885,#28884,#16051,.T.);
#34323=EDGE_CURVE('',#28886,#28885,#16052,.T.);
#34324=EDGE_CURVE('',#28887,#28886,#21275,.T.);
#34325=EDGE_CURVE('',#28888,#28887,#21276,.T.);
#34326=EDGE_CURVE('',#28889,#28888,#21277,.T.);
#34327=EDGE_CURVE('',#28890,#28889,#21278,.T.);
#34328=EDGE_CURVE('',#28891,#28890,#16053,.T.);
#34329=EDGE_CURVE('',#28892,#28891,#16054,.T.);
#34330=EDGE_CURVE('',#28893,#28892,#21279,.T.);
#34331=EDGE_CURVE('',#28894,#28893,#21280,.F.);
#34332=EDGE_CURVE('',#28720,#28894,#21281,.F.);
#34333=EDGE_CURVE('',#28895,#28896,#16055,.F.);
#34334=EDGE_CURVE('',#28897,#28895,#16056,.F.);
#34335=EDGE_CURVE('',#28898,#28897,#21282,.T.);
#34336=EDGE_CURVE('',#28896,#28898,#21283,.T.);
#34337=EDGE_CURVE('',#28899,#28900,#21284,.F.);
#34338=EDGE_CURVE('',#28901,#28899,#16057,.F.);
#34339=EDGE_CURVE('',#28902,#28901,#21285,.T.);
#34340=EDGE_CURVE('',#28900,#28902,#21286,.T.);
#34341=EDGE_CURVE('',#28903,#28904,#21287,.F.);
#34342=EDGE_CURVE('',#28905,#28903,#16058,.T.);
#34343=EDGE_CURVE('',#28906,#28905,#16059,.T.);
#34344=EDGE_CURVE('',#28907,#28906,#16060,.T.);
#34345=EDGE_CURVE('',#28904,#28907,#16061,.T.);
#34346=EDGE_CURVE('',#28908,#28909,#21288,.F.);
#34347=EDGE_CURVE('',#28910,#28908,#21289,.F.);
#34348=EDGE_CURVE('',#28911,#28910,#16062,.T.);
#34349=EDGE_CURVE('',#28909,#28911,#16063,.T.);
#34350=EDGE_CURVE('',#28912,#28913,#21290,.F.);
#34351=EDGE_CURVE('',#28914,#28912,#16064,.F.);
#34352=EDGE_CURVE('',#28915,#28914,#21291,.T.);
#34353=EDGE_CURVE('',#28913,#28915,#21292,.T.);
#34354=EDGE_CURVE('',#28916,#28917,#21293,.F.);
#34355=EDGE_CURVE('',#28918,#28916,#16065,.F.);
#34356=EDGE_CURVE('',#28919,#28918,#21294,.T.);
#34357=EDGE_CURVE('',#28917,#28919,#21295,.T.);
#34358=EDGE_CURVE('',#28920,#28921,#21296,.F.);
#34359=EDGE_CURVE('',#28922,#28920,#16066,.T.);
#34360=EDGE_CURVE('',#28923,#28922,#16067,.T.);
#34361=EDGE_CURVE('',#28921,#28923,#21297,.F.);
#34362=EDGE_CURVE('',#28924,#28925,#16068,.T.);
#34363=EDGE_CURVE('',#28926,#28924,#16069,.T.);
#34364=EDGE_CURVE('',#28927,#28926,#16070,.T.);
#34365=EDGE_CURVE('',#28928,#28927,#21298,.F.);
#34366=EDGE_CURVE('',#28925,#28928,#16071,.T.);
#34367=EDGE_CURVE('',#28929,#28925,#21299,.F.);
#34368=EDGE_CURVE('',#28924,#28929,#16072,.T.);
#34369=EDGE_CURVE('',#28930,#28931,#21300,.F.);
#34370=EDGE_CURVE('',#28932,#28930,#21301,.F.);
#34371=EDGE_CURVE('',#28933,#28932,#16073,.T.);
#34372=EDGE_CURVE('',#28931,#28933,#21302,.T.);
#34373=EDGE_CURVE('',#28934,#28935,#21303,.F.);
#34374=EDGE_CURVE('',#28936,#28934,#21304,.F.);
#34375=EDGE_CURVE('',#28937,#28936,#16074,.T.);
#34376=EDGE_CURVE('',#28935,#28937,#16075,.T.);
#34377=EDGE_CURVE('',#28938,#28939,#21305,.F.);
#34378=EDGE_CURVE('',#28940,#28938,#16076,.T.);
#34379=EDGE_CURVE('',#28941,#28940,#16077,.T.);
#34380=EDGE_CURVE('',#28939,#28941,#21306,.F.);
#34381=EDGE_CURVE('',#28942,#28943,#21307,.F.);
#34382=EDGE_CURVE('',#28944,#28942,#16078,.T.);
#34383=EDGE_CURVE('',#28945,#28944,#16079,.T.);
#34384=EDGE_CURVE('',#28943,#28945,#21308,.F.);
#34385=EDGE_CURVE('',#28946,#28947,#21309,.F.);
#34386=EDGE_CURVE('',#28948,#28946,#21310,.F.);
#34387=EDGE_CURVE('',#28949,#28948,#16080,.T.);
#34388=EDGE_CURVE('',#28947,#28949,#16081,.T.);
#34389=EDGE_CURVE('',#28950,#28951,#21311,.F.);
#34390=EDGE_CURVE('',#28952,#28950,#21312,.F.);
#34391=EDGE_CURVE('',#28953,#28952,#21313,.T.);
#34392=EDGE_CURVE('',#28951,#28953,#16082,.T.);
#34393=EDGE_CURVE('',#28954,#28955,#21314,.F.);
#34394=EDGE_CURVE('',#28956,#28954,#21315,.T.);
#34395=EDGE_CURVE('',#28957,#28956,#16083,.T.);
#34396=EDGE_CURVE('',#28955,#28957,#21316,.F.);
#34397=EDGE_CURVE('',#28958,#28959,#21317,.F.);
#34398=EDGE_CURVE('',#28960,#28958,#21318,.F.);
#34399=EDGE_CURVE('',#28961,#28960,#16084,.T.);
#34400=EDGE_CURVE('',#28959,#28961,#21319,.T.);
#34401=EDGE_CURVE('',#28962,#28963,#21320,.F.);
#34402=EDGE_CURVE('',#28964,#28962,#21321,.F.);
#34403=EDGE_CURVE('',#28965,#28964,#16085,.T.);
#34404=EDGE_CURVE('',#28963,#28965,#16086,.T.);
#34405=EDGE_CURVE('',#28966,#28967,#21322,.F.);
#34406=EDGE_CURVE('',#28968,#28966,#16087,.T.);
#34407=EDGE_CURVE('',#28969,#28968,#16088,.T.);
#34408=EDGE_CURVE('',#28967,#28969,#21323,.F.);
#34409=EDGE_CURVE('',#28970,#28971,#21324,.F.);
#34410=EDGE_CURVE('',#28972,#28970,#16089,.T.);
#34411=EDGE_CURVE('',#28973,#28972,#21325,.T.);
#34412=EDGE_CURVE('',#28971,#28973,#21326,.F.);
#34413=EDGE_CURVE('',#28974,#28975,#21327,.F.);
#34414=EDGE_CURVE('',#28976,#28974,#21328,.F.);
#34415=EDGE_CURVE('',#28977,#28976,#16090,.T.);
#34416=EDGE_CURVE('',#28975,#28977,#16091,.T.);
#34417=EDGE_CURVE('',#28978,#28979,#21329,.F.);
#34418=EDGE_CURVE('',#28980,#28978,#21330,.F.);
#34419=EDGE_CURVE('',#28981,#28980,#21331,.T.);
#34420=EDGE_CURVE('',#28979,#28981,#16092,.T.);
#34421=EDGE_CURVE('',#28982,#28983,#21332,.F.);
#34422=EDGE_CURVE('',#28984,#28982,#21333,.T.);
#34423=EDGE_CURVE('',#28985,#28984,#16093,.T.);
#34424=EDGE_CURVE('',#28983,#28985,#21334,.F.);
#34425=EDGE_CURVE('',#28986,#28987,#21335,.F.);
#34426=EDGE_CURVE('',#28988,#28986,#16094,.T.);
#34427=EDGE_CURVE('',#28989,#28988,#16095,.T.);
#34428=EDGE_CURVE('',#28987,#28989,#21336,.F.);
#34429=EDGE_CURVE('',#28990,#28991,#21337,.F.);
#34430=EDGE_CURVE('',#28992,#28990,#21338,.F.);
#34431=EDGE_CURVE('',#28993,#28992,#16096,.T.);
#34432=EDGE_CURVE('',#28991,#28993,#21339,.T.);
#34433=EDGE_CURVE('',#28994,#28995,#21340,.F.);
#34434=EDGE_CURVE('',#28996,#28994,#21341,.F.);
#34435=EDGE_CURVE('',#28997,#28996,#16097,.T.);
#34436=EDGE_CURVE('',#28995,#28997,#16098,.T.);
#34437=EDGE_CURVE('',#28998,#28999,#21342,.F.);
#34438=EDGE_CURVE('',#29000,#28998,#16099,.T.);
#34439=EDGE_CURVE('',#29001,#29000,#21343,.T.);
#34440=EDGE_CURVE('',#28999,#29001,#21344,.F.);
#34441=EDGE_CURVE('',#29002,#29003,#21345,.F.);
#34442=EDGE_CURVE('',#29004,#29002,#21346,.F.);
#34443=EDGE_CURVE('',#29005,#29004,#16100,.T.);
#34444=EDGE_CURVE('',#29003,#29005,#16101,.T.);
#34445=EDGE_CURVE('',#29006,#29007,#21347,.F.);
#34446=EDGE_CURVE('',#29008,#29006,#21348,.F.);
#34447=EDGE_CURVE('',#29009,#29008,#21349,.T.);
#34448=EDGE_CURVE('',#29007,#29009,#16102,.T.);
#34449=EDGE_CURVE('',#29010,#29011,#21350,.F.);
#34450=EDGE_CURVE('',#29012,#29010,#21351,.T.);
#34451=EDGE_CURVE('',#29013,#29012,#16103,.T.);
#34452=EDGE_CURVE('',#29011,#29013,#21352,.F.);
#34453=EDGE_CURVE('',#29014,#29015,#21353,.F.);
#34454=EDGE_CURVE('',#29016,#29014,#4375,.T.);
#34455=EDGE_CURVE('',#29017,#29016,#16104,.T.);
#34456=EDGE_CURVE('',#29015,#29017,#21354,.F.);
#34457=EDGE_CURVE('',#29018,#29019,#21355,.F.);
#34458=EDGE_CURVE('',#29020,#29018,#21356,.F.);
#34459=EDGE_CURVE('',#29021,#29020,#21357,.T.);
#34460=EDGE_CURVE('',#29019,#29021,#21358,.T.);
#34461=EDGE_CURVE('',#29022,#29023,#21359,.F.);
#34462=EDGE_CURVE('',#29024,#29022,#21360,.F.);
#34463=EDGE_CURVE('',#29025,#29024,#16105,.T.);
#34464=EDGE_CURVE('',#29023,#29025,#16106,.T.);
#34465=EDGE_CURVE('',#29026,#29027,#21361,.F.);
#34466=EDGE_CURVE('',#29028,#29026,#16107,.T.);
#34467=EDGE_CURVE('',#29029,#29028,#21362,.T.);
#34468=EDGE_CURVE('',#29027,#29029,#21363,.F.);
#34469=EDGE_CURVE('',#29030,#29031,#16108,.T.);
#34470=EDGE_CURVE('',#29032,#29031,#24364,.T.);
#34471=EDGE_CURVE('',#29033,#29032,#16109,.T.);
#34472=EDGE_CURVE('',#29030,#29033,#21364,.T.);
#34473=EDGE_CURVE('',#29034,#29035,#16110,.T.);
#34474=EDGE_CURVE('',#29036,#29035,#21365,.T.);
#34475=EDGE_CURVE('',#29032,#29036,#16111,.T.);
#34476=EDGE_CURVE('',#29034,#29032,#24365,.T.);
#34477=EDGE_CURVE('',#29037,#29034,#21366,.T.);
#34478=EDGE_CURVE('',#29038,#29037,#16112,.T.);
#34479=EDGE_CURVE('',#29035,#29038,#16113,.T.);
#34480=EDGE_CURVE('',#29039,#29038,#24366,.T.);
#34481=EDGE_CURVE('',#29036,#29039,#16114,.T.);
#34482=EDGE_CURVE('',#29040,#29041,#16115,.T.);
#34483=EDGE_CURVE('',#29042,#29041,#21367,.T.);
#34484=EDGE_CURVE('',#29039,#29042,#16116,.T.);
#34485=EDGE_CURVE('',#29040,#29039,#24367,.T.);
#34486=EDGE_CURVE('',#29043,#29040,#21368,.T.);
#34487=EDGE_CURVE('',#29044,#29043,#16117,.T.);
#34488=EDGE_CURVE('',#29041,#29044,#16118,.T.);
#34489=EDGE_CURVE('',#29045,#29044,#24368,.T.);
#34490=EDGE_CURVE('',#29042,#29045,#16119,.T.);
#34491=EDGE_CURVE('',#29046,#29047,#16120,.T.);
#34492=EDGE_CURVE('',#29048,#29047,#21369,.T.);
#34493=EDGE_CURVE('',#29045,#29048,#16121,.T.);
#34494=EDGE_CURVE('',#29046,#29045,#24369,.T.);
#34495=EDGE_CURVE('',#29049,#29046,#21370,.T.);
#34496=EDGE_CURVE('',#29050,#29049,#16122,.T.);
#34497=EDGE_CURVE('',#29047,#29050,#16123,.T.);
#34498=EDGE_CURVE('',#29051,#29050,#24370,.T.);
#34499=EDGE_CURVE('',#29048,#29051,#16124,.T.);
#34500=EDGE_CURVE('',#29052,#29053,#16125,.T.);
#34501=EDGE_CURVE('',#29054,#29053,#21371,.T.);
#34502=EDGE_CURVE('',#29051,#29054,#16126,.T.);
#34503=EDGE_CURVE('',#29052,#29051,#24371,.T.);
#34504=EDGE_CURVE('',#29055,#29052,#21372,.T.);
#34505=EDGE_CURVE('',#29056,#29055,#16127,.T.);
#34506=EDGE_CURVE('',#29053,#29056,#16128,.T.);
#34507=EDGE_CURVE('',#29057,#29056,#24372,.T.);
#34508=EDGE_CURVE('',#29054,#29057,#16129,.T.);
#34509=EDGE_CURVE('',#29058,#29059,#16130,.T.);
#34510=EDGE_CURVE('',#29060,#29059,#21373,.T.);
#34511=EDGE_CURVE('',#29057,#29060,#16131,.T.);
#34512=EDGE_CURVE('',#29058,#29057,#24373,.T.);
#34513=EDGE_CURVE('',#29061,#29058,#21374,.T.);
#34514=EDGE_CURVE('',#29062,#29061,#16132,.T.);
#34515=EDGE_CURVE('',#29059,#29062,#16133,.T.);
#34516=EDGE_CURVE('',#29063,#29062,#24374,.T.);
#34517=EDGE_CURVE('',#29060,#29063,#16134,.T.);
#34518=EDGE_CURVE('',#29064,#29065,#16135,.T.);
#34519=EDGE_CURVE('',#29066,#29065,#21375,.T.);
#34520=EDGE_CURVE('',#29063,#29066,#16136,.T.);
#34521=EDGE_CURVE('',#29064,#29063,#24375,.T.);
#34522=EDGE_CURVE('',#29067,#29064,#21376,.T.);
#34523=EDGE_CURVE('',#29068,#29067,#16137,.T.);
#34524=EDGE_CURVE('',#29065,#29068,#16138,.T.);
#34525=EDGE_CURVE('',#29069,#29068,#24376,.T.);
#34526=EDGE_CURVE('',#29066,#29069,#16139,.T.);
#34527=EDGE_CURVE('',#29070,#29026,#21377,.T.);
#34528=EDGE_CURVE('',#29069,#29070,#16140,.T.);
#34529=EDGE_CURVE('',#29028,#29069,#24377,.T.);
#34530=EDGE_CURVE('',#29071,#29027,#24378,.T.);
#34531=EDGE_CURVE('',#29070,#29071,#16141,.T.);
#34532=EDGE_CURVE('',#29072,#29073,#16142,.T.);
#34533=EDGE_CURVE('',#29074,#29073,#21378,.T.);
#34534=EDGE_CURVE('',#29071,#29074,#16143,.T.);
#34535=EDGE_CURVE('',#29072,#29071,#24379,.T.);
#34536=EDGE_CURVE('',#29075,#29072,#21379,.T.);
#34537=EDGE_CURVE('',#29076,#29075,#16144,.T.);
#34538=EDGE_CURVE('',#29073,#29076,#16145,.T.);
#34539=EDGE_CURVE('',#29077,#29076,#24380,.T.);
#34540=EDGE_CURVE('',#29074,#29077,#16146,.T.);
#34541=EDGE_CURVE('',#29078,#29079,#16147,.T.);
#34542=EDGE_CURVE('',#29080,#29079,#21380,.T.);
#34543=EDGE_CURVE('',#29077,#29080,#16148,.T.);
#34544=EDGE_CURVE('',#29078,#29077,#24381,.T.);
#34545=EDGE_CURVE('',#29081,#29078,#21381,.T.);
#34546=EDGE_CURVE('',#29082,#29081,#16149,.T.);
#34547=EDGE_CURVE('',#29079,#29082,#16150,.T.);
#34548=EDGE_CURVE('',#29083,#29082,#24382,.T.);
#34549=EDGE_CURVE('',#29080,#29083,#16151,.T.);
#34550=EDGE_CURVE('',#29084,#29085,#16152,.T.);
#34551=EDGE_CURVE('',#29086,#29085,#21382,.T.);
#34552=EDGE_CURVE('',#29083,#29086,#16153,.T.);
#34553=EDGE_CURVE('',#29084,#29083,#24383,.T.);
#34554=EDGE_CURVE('',#29087,#29084,#21383,.T.);
#34555=EDGE_CURVE('',#29088,#29087,#16154,.T.);
#34556=EDGE_CURVE('',#29085,#29088,#16155,.T.);
#34557=EDGE_CURVE('',#29089,#29088,#24384,.T.);
#34558=EDGE_CURVE('',#29086,#29089,#16156,.T.);
#34559=EDGE_CURVE('',#29090,#29091,#16157,.T.);
#34560=EDGE_CURVE('',#29092,#29091,#21384,.T.);
#34561=EDGE_CURVE('',#29089,#29092,#16158,.T.);
#34562=EDGE_CURVE('',#29090,#29089,#24385,.T.);
#34563=EDGE_CURVE('',#29093,#29090,#21385,.T.);
#34564=EDGE_CURVE('',#29094,#29093,#16159,.T.);
#34565=EDGE_CURVE('',#29091,#29094,#16160,.T.);
#34566=EDGE_CURVE('',#29095,#29094,#24386,.T.);
#34567=EDGE_CURVE('',#29092,#29095,#16161,.T.);
#34568=EDGE_CURVE('',#29096,#29097,#16162,.T.);
#34569=EDGE_CURVE('',#29098,#29097,#21386,.T.);
#34570=EDGE_CURVE('',#29095,#29098,#16163,.T.);
#34571=EDGE_CURVE('',#29096,#29095,#24387,.T.);
#34572=EDGE_CURVE('',#29099,#29096,#21387,.T.);
#34573=EDGE_CURVE('',#29100,#29099,#16164,.T.);
#34574=EDGE_CURVE('',#29097,#29100,#16165,.T.);
#34575=EDGE_CURVE('',#29101,#29100,#24388,.T.);
#34576=EDGE_CURVE('',#29098,#29101,#16166,.T.);
#34577=EDGE_CURVE('',#29102,#29103,#16167,.T.);
#34578=EDGE_CURVE('',#29104,#29103,#21388,.T.);
#34579=EDGE_CURVE('',#29101,#29104,#16168,.T.);
#34580=EDGE_CURVE('',#29102,#29101,#24389,.T.);
#34581=EDGE_CURVE('',#29105,#29102,#21389,.T.);
#34582=EDGE_CURVE('',#29106,#29105,#16169,.T.);
#34583=EDGE_CURVE('',#29103,#29106,#16170,.T.);
#34584=EDGE_CURVE('',#29107,#29106,#24390,.T.);
#34585=EDGE_CURVE('',#29104,#29107,#16171,.T.);
#34586=EDGE_CURVE('',#29108,#29109,#16172,.T.);
#34587=EDGE_CURVE('',#29110,#29109,#21390,.T.);
#34588=EDGE_CURVE('',#29107,#29110,#16173,.T.);
#34589=EDGE_CURVE('',#29108,#29107,#24391,.T.);
#34590=EDGE_CURVE('',#29111,#29108,#21391,.T.);
#34591=EDGE_CURVE('',#29112,#29111,#16174,.T.);
#34592=EDGE_CURVE('',#29109,#29112,#16175,.T.);
#34593=EDGE_CURVE('',#29113,#29112,#24392,.T.);
#34594=EDGE_CURVE('',#29110,#29113,#16176,.T.);
#34595=EDGE_CURVE('',#29114,#29115,#16177,.T.);
#34596=EDGE_CURVE('',#29116,#29115,#21392,.T.);
#34597=EDGE_CURVE('',#29113,#29116,#16178,.T.);
#34598=EDGE_CURVE('',#29114,#29113,#24393,.T.);
#34599=EDGE_CURVE('',#29117,#29114,#21393,.T.);
#34600=EDGE_CURVE('',#29118,#29117,#16179,.T.);
#34601=EDGE_CURVE('',#29115,#29118,#16180,.T.);
#34602=EDGE_CURVE('',#29119,#29118,#24394,.T.);
#34603=EDGE_CURVE('',#29116,#29119,#16181,.T.);
#34604=EDGE_CURVE('',#29120,#29121,#16182,.T.);
#34605=EDGE_CURVE('',#29122,#29121,#21394,.T.);
#34606=EDGE_CURVE('',#29119,#29122,#16183,.T.);
#34607=EDGE_CURVE('',#29120,#29119,#24395,.T.);
#34608=EDGE_CURVE('',#29123,#29120,#21395,.T.);
#34609=EDGE_CURVE('',#29124,#29123,#16184,.T.);
#34610=EDGE_CURVE('',#29121,#29124,#16185,.T.);
#34611=EDGE_CURVE('',#29125,#29124,#24396,.T.);
#34612=EDGE_CURVE('',#29122,#29125,#16186,.T.);
#34613=EDGE_CURVE('',#29126,#29127,#16187,.T.);
#34614=EDGE_CURVE('',#29128,#29127,#21396,.T.);
#34615=EDGE_CURVE('',#29125,#29128,#16188,.T.);
#34616=EDGE_CURVE('',#29126,#29125,#24397,.T.);
#34617=EDGE_CURVE('',#29129,#29126,#21397,.T.);
#34618=EDGE_CURVE('',#29130,#29129,#16189,.T.);
#34619=EDGE_CURVE('',#29127,#29130,#16190,.T.);
#34620=EDGE_CURVE('',#29131,#29130,#24398,.T.);
#34621=EDGE_CURVE('',#29128,#29131,#16191,.T.);
#34622=EDGE_CURVE('',#29132,#29133,#16192,.T.);
#34623=EDGE_CURVE('',#29134,#29133,#21398,.T.);
#34624=EDGE_CURVE('',#29131,#29134,#16193,.T.);
#34625=EDGE_CURVE('',#29132,#29131,#24399,.T.);
#34626=EDGE_CURVE('',#29135,#29132,#21399,.T.);
#34627=EDGE_CURVE('',#29136,#29135,#16194,.T.);
#34628=EDGE_CURVE('',#29133,#29136,#16195,.T.);
#34629=EDGE_CURVE('',#29137,#29136,#24400,.T.);
#34630=EDGE_CURVE('',#29134,#29137,#16196,.T.);
#34631=EDGE_CURVE('',#29138,#29139,#16197,.T.);
#34632=EDGE_CURVE('',#29140,#29139,#21400,.T.);
#34633=EDGE_CURVE('',#29137,#29140,#16198,.T.);
#34634=EDGE_CURVE('',#29138,#29137,#24401,.T.);
#34635=EDGE_CURVE('',#29141,#29138,#21401,.T.);
#34636=EDGE_CURVE('',#29142,#29141,#16199,.T.);
#34637=EDGE_CURVE('',#29139,#29142,#16200,.T.);
#34638=EDGE_CURVE('',#29143,#29142,#24402,.T.);
#34639=EDGE_CURVE('',#29140,#29143,#16201,.T.);
#34640=EDGE_CURVE('',#29144,#29145,#16202,.T.);
#34641=EDGE_CURVE('',#29146,#29145,#21402,.T.);
#34642=EDGE_CURVE('',#29143,#29146,#16203,.T.);
#34643=EDGE_CURVE('',#29144,#29143,#24403,.T.);
#34644=EDGE_CURVE('',#29147,#29144,#21403,.T.);
#34645=EDGE_CURVE('',#29148,#29147,#16204,.T.);
#34646=EDGE_CURVE('',#29145,#29148,#16205,.T.);
#34647=EDGE_CURVE('',#29149,#29148,#24404,.T.);
#34648=EDGE_CURVE('',#29146,#29149,#16206,.T.);
#34649=EDGE_CURVE('',#29150,#29151,#16207,.T.);
#34650=EDGE_CURVE('',#29152,#29151,#21404,.T.);
#34651=EDGE_CURVE('',#29149,#29152,#16208,.T.);
#34652=EDGE_CURVE('',#29150,#29149,#24405,.T.);
#34653=EDGE_CURVE('',#29153,#29150,#21405,.T.);
#34654=EDGE_CURVE('',#29154,#29153,#16209,.T.);
#34655=EDGE_CURVE('',#29151,#29154,#16210,.T.);
#34656=EDGE_CURVE('',#29155,#29154,#24406,.T.);
#34657=EDGE_CURVE('',#29152,#29155,#16211,.T.);
#34658=EDGE_CURVE('',#29156,#29157,#16212,.T.);
#34659=EDGE_CURVE('',#29158,#29157,#21406,.T.);
#34660=EDGE_CURVE('',#29155,#29158,#16213,.T.);
#34661=EDGE_CURVE('',#29156,#29155,#24407,.T.);
#34662=EDGE_CURVE('',#29159,#29156,#21407,.T.);
#34663=EDGE_CURVE('',#29160,#29159,#16214,.T.);
#34664=EDGE_CURVE('',#29157,#29160,#16215,.T.);
#34665=EDGE_CURVE('',#29161,#29160,#24408,.T.);
#34666=EDGE_CURVE('',#29158,#29161,#16216,.T.);
#34667=EDGE_CURVE('',#29162,#29163,#16217,.T.);
#34668=EDGE_CURVE('',#29164,#29163,#21408,.T.);
#34669=EDGE_CURVE('',#29161,#29164,#16218,.T.);
#34670=EDGE_CURVE('',#29162,#29161,#24409,.T.);
#34671=EDGE_CURVE('',#29165,#29162,#21409,.T.);
#34672=EDGE_CURVE('',#29166,#29165,#16219,.T.);
#34673=EDGE_CURVE('',#29163,#29166,#16220,.T.);
#34674=EDGE_CURVE('',#29167,#29166,#24410,.T.);
#34675=EDGE_CURVE('',#29164,#29167,#16221,.T.);
#34676=EDGE_CURVE('',#29168,#29169,#16222,.T.);
#34677=EDGE_CURVE('',#29170,#29169,#21410,.T.);
#34678=EDGE_CURVE('',#29167,#29170,#16223,.T.);
#34679=EDGE_CURVE('',#29168,#29167,#24411,.T.);
#34680=EDGE_CURVE('',#29171,#29168,#21411,.T.);
#34681=EDGE_CURVE('',#29172,#29171,#16224,.T.);
#34682=EDGE_CURVE('',#29169,#29172,#16225,.T.);
#34683=EDGE_CURVE('',#29173,#29172,#24412,.T.);
#34684=EDGE_CURVE('',#29170,#29173,#16226,.T.);
#34685=EDGE_CURVE('',#29174,#29175,#16227,.T.);
#34686=EDGE_CURVE('',#29176,#29175,#21412,.T.);
#34687=EDGE_CURVE('',#29173,#29176,#16228,.T.);
#34688=EDGE_CURVE('',#29174,#29173,#24413,.T.);
#34689=EDGE_CURVE('',#29175,#29177,#16229,.T.);
#34690=EDGE_CURVE('',#29178,#29177,#24414,.T.);
#34691=EDGE_CURVE('',#29176,#29178,#16230,.T.);
#34692=EDGE_CURVE('',#29179,#29174,#21413,.T.);
#34693=EDGE_CURVE('',#29177,#29179,#16231,.T.);
#34694=EDGE_CURVE('',#29180,#29181,#16232,.T.);
#34695=EDGE_CURVE('',#29182,#29181,#21414,.T.);
#34696=EDGE_CURVE('',#29178,#29182,#16233,.T.);
#34697=EDGE_CURVE('',#29180,#29178,#24415,.T.);
#34698=EDGE_CURVE('',#29181,#29183,#16234,.T.);
#34699=EDGE_CURVE('',#29184,#29180,#21415,.T.);
#34700=EDGE_CURVE('',#29183,#29184,#16235,.T.);
#34701=EDGE_CURVE('',#29182,#29185,#16236,.T.);
#34702=EDGE_CURVE('',#29185,#29183,#24416,.T.);
#34703=EDGE_CURVE('',#29186,#29187,#16237,.T.);
#34704=EDGE_CURVE('',#29188,#29187,#21416,.T.);
#34705=EDGE_CURVE('',#29185,#29188,#16238,.T.);
#34706=EDGE_CURVE('',#29186,#29185,#24417,.T.);
#34707=EDGE_CURVE('',#29189,#29186,#21417,.T.);
#34708=EDGE_CURVE('',#29190,#29189,#16239,.T.);
#34709=EDGE_CURVE('',#29187,#29190,#16240,.T.);
#34710=EDGE_CURVE('',#29191,#29190,#24418,.T.);
#34711=EDGE_CURVE('',#29188,#29191,#16241,.T.);
#34712=EDGE_CURVE('',#29192,#29193,#16242,.T.);
#34713=EDGE_CURVE('',#29194,#29193,#21418,.T.);
#34714=EDGE_CURVE('',#29191,#29194,#16243,.T.);
#34715=EDGE_CURVE('',#29192,#29191,#24419,.T.);
#34716=EDGE_CURVE('',#29195,#29192,#21419,.T.);
#34717=EDGE_CURVE('',#29196,#29195,#16244,.T.);
#34718=EDGE_CURVE('',#29193,#29196,#16245,.T.);
#34719=EDGE_CURVE('',#29197,#29196,#24420,.T.);
#34720=EDGE_CURVE('',#29194,#29197,#16246,.T.);
#34721=EDGE_CURVE('',#29198,#29199,#21420,.T.);
#34722=EDGE_CURVE('',#29031,#29198,#16247,.T.);
#34723=EDGE_CURVE('',#29199,#29030,#16248,.T.);
#34724=EDGE_CURVE('',#29197,#29033,#16249,.T.);
#34725=EDGE_CURVE('',#29199,#29197,#24421,.T.);
#34726=EDGE_CURVE('',#29200,#29197,#21421,.T.);
#34727=EDGE_CURVE('',#29200,#29201,#16250,.T.);
#34728=EDGE_CURVE('',#29194,#29201,#24422,.T.);
#34729=EDGE_CURVE('',#29202,#29194,#24423,.T.);
#34730=EDGE_CURVE('',#29202,#29203,#16251,.T.);
#34731=EDGE_CURVE('',#29191,#29203,#21422,.T.);
#34732=EDGE_CURVE('',#29203,#29204,#16252,.T.);
#34733=EDGE_CURVE('',#29188,#29204,#24424,.T.);
#34734=EDGE_CURVE('',#29205,#29202,#16253,.T.);
#34735=EDGE_CURVE('',#29204,#29205,#16254,.T.);
#34736=EDGE_CURVE('',#29206,#29188,#24425,.T.);
#34737=EDGE_CURVE('',#29206,#29207,#16255,.T.);
#34738=EDGE_CURVE('',#29185,#29207,#21423,.T.);
#34739=EDGE_CURVE('',#29207,#29208,#16256,.T.);
#34740=EDGE_CURVE('',#29182,#29208,#24426,.T.);
#34741=EDGE_CURVE('',#29209,#29206,#16257,.T.);
#34742=EDGE_CURVE('',#29208,#29209,#16258,.T.);
#34743=EDGE_CURVE('',#29210,#29182,#24427,.T.);
#34744=EDGE_CURVE('',#29210,#29211,#16259,.T.);
#34745=EDGE_CURVE('',#29178,#29211,#21424,.T.);
#34746=EDGE_CURVE('',#29211,#29212,#16260,.T.);
#34747=EDGE_CURVE('',#29176,#29212,#24428,.T.);
#34748=EDGE_CURVE('',#29213,#29210,#16261,.T.);
#34749=EDGE_CURVE('',#29212,#29213,#16262,.T.);
#34750=EDGE_CURVE('',#29214,#29176,#24429,.T.);
#34751=EDGE_CURVE('',#29214,#29215,#16263,.T.);
#34752=EDGE_CURVE('',#29173,#29215,#21425,.T.);
#34753=EDGE_CURVE('',#29215,#29216,#16264,.T.);
#34754=EDGE_CURVE('',#29170,#29216,#24430,.T.);
#34755=EDGE_CURVE('',#29217,#29214,#16265,.T.);
#34756=EDGE_CURVE('',#29216,#29217,#16266,.T.);
#34757=EDGE_CURVE('',#29218,#29170,#24431,.T.);
#34758=EDGE_CURVE('',#29218,#29219,#16267,.T.);
#34759=EDGE_CURVE('',#29167,#29219,#21426,.T.);
#34760=EDGE_CURVE('',#29219,#29220,#16268,.T.);
#34761=EDGE_CURVE('',#29164,#29220,#24432,.T.);
#34762=EDGE_CURVE('',#29221,#29218,#16269,.T.);
#34763=EDGE_CURVE('',#29220,#29221,#16270,.T.);
#34764=EDGE_CURVE('',#29222,#29164,#24433,.T.);
#34765=EDGE_CURVE('',#29222,#29223,#16271,.T.);
#34766=EDGE_CURVE('',#29161,#29223,#21427,.T.);
#34767=EDGE_CURVE('',#29223,#29224,#16272,.T.);
#34768=EDGE_CURVE('',#29158,#29224,#24434,.T.);
#34769=EDGE_CURVE('',#29225,#29222,#16273,.T.);
#34770=EDGE_CURVE('',#29224,#29225,#16274,.T.);
#34771=EDGE_CURVE('',#29226,#29158,#24435,.T.);
#34772=EDGE_CURVE('',#29226,#29227,#16275,.T.);
#34773=EDGE_CURVE('',#29155,#29227,#21428,.T.);
#34774=EDGE_CURVE('',#29227,#29228,#16276,.T.);
#34775=EDGE_CURVE('',#29152,#29228,#24436,.T.);
#34776=EDGE_CURVE('',#29229,#29226,#16277,.T.);
#34777=EDGE_CURVE('',#29228,#29229,#16278,.T.);
#34778=EDGE_CURVE('',#29230,#29152,#24437,.T.);
#34779=EDGE_CURVE('',#29230,#29231,#16279,.T.);
#34780=EDGE_CURVE('',#29149,#29231,#21429,.T.);
#34781=EDGE_CURVE('',#29231,#29232,#16280,.T.);
#34782=EDGE_CURVE('',#29146,#29232,#24438,.T.);
#34783=EDGE_CURVE('',#29233,#29230,#16281,.T.);
#34784=EDGE_CURVE('',#29232,#29233,#16282,.T.);
#34785=EDGE_CURVE('',#29234,#29146,#24439,.T.);
#34786=EDGE_CURVE('',#29234,#29235,#16283,.T.);
#34787=EDGE_CURVE('',#29143,#29235,#21430,.T.);
#34788=EDGE_CURVE('',#29235,#29236,#16284,.T.);
#34789=EDGE_CURVE('',#29140,#29236,#24440,.T.);
#34790=EDGE_CURVE('',#29237,#29234,#16285,.T.);
#34791=EDGE_CURVE('',#29236,#29237,#16286,.T.);
#34792=EDGE_CURVE('',#29238,#29140,#24441,.T.);
#34793=EDGE_CURVE('',#29238,#29239,#16287,.T.);
#34794=EDGE_CURVE('',#29137,#29239,#21431,.T.);
#34795=EDGE_CURVE('',#29239,#29240,#16288,.T.);
#34796=EDGE_CURVE('',#29134,#29240,#24442,.T.);
#34797=EDGE_CURVE('',#29241,#29238,#16289,.T.);
#34798=EDGE_CURVE('',#29240,#29241,#16290,.T.);
#34799=EDGE_CURVE('',#29242,#29134,#24443,.T.);
#34800=EDGE_CURVE('',#29242,#29243,#16291,.T.);
#34801=EDGE_CURVE('',#29131,#29243,#21432,.T.);
#34802=EDGE_CURVE('',#29243,#29244,#16292,.T.);
#34803=EDGE_CURVE('',#29128,#29244,#24444,.T.);
#34804=EDGE_CURVE('',#29245,#29242,#16293,.T.);
#34805=EDGE_CURVE('',#29244,#29245,#16294,.T.);
#34806=EDGE_CURVE('',#29246,#29128,#24445,.T.);
#34807=EDGE_CURVE('',#29246,#29247,#16295,.T.);
#34808=EDGE_CURVE('',#29125,#29247,#21433,.T.);
#34809=EDGE_CURVE('',#29247,#29248,#16296,.T.);
#34810=EDGE_CURVE('',#29122,#29248,#24446,.T.);
#34811=EDGE_CURVE('',#29249,#29246,#16297,.T.);
#34812=EDGE_CURVE('',#29248,#29249,#16298,.T.);
#34813=EDGE_CURVE('',#29250,#29122,#24447,.T.);
#34814=EDGE_CURVE('',#29250,#29251,#16299,.T.);
#34815=EDGE_CURVE('',#29119,#29251,#21434,.T.);
#34816=EDGE_CURVE('',#29251,#29252,#16300,.T.);
#34817=EDGE_CURVE('',#29116,#29252,#24448,.T.);
#34818=EDGE_CURVE('',#29253,#29250,#16301,.T.);
#34819=EDGE_CURVE('',#29252,#29253,#16302,.T.);
#34820=EDGE_CURVE('',#29025,#29116,#24449,.T.);
#34821=EDGE_CURVE('',#29113,#29024,#21435,.T.);
#34822=EDGE_CURVE('',#29110,#29022,#24450,.T.);
#34823=EDGE_CURVE('',#29254,#29110,#24451,.T.);
#34824=EDGE_CURVE('',#29254,#29255,#16303,.T.);
#34825=EDGE_CURVE('',#29107,#29255,#21436,.T.);
#34826=EDGE_CURVE('',#29255,#29256,#16304,.T.);
#34827=EDGE_CURVE('',#29104,#29256,#24452,.T.);
#34828=EDGE_CURVE('',#29257,#29254,#16305,.T.);
#34829=EDGE_CURVE('',#29256,#29257,#16306,.T.);
#34830=EDGE_CURVE('',#29258,#29104,#24453,.T.);
#34831=EDGE_CURVE('',#29258,#29259,#16307,.T.);
#34832=EDGE_CURVE('',#29101,#29259,#21437,.T.);
#34833=EDGE_CURVE('',#29259,#29260,#16308,.T.);
#34834=EDGE_CURVE('',#29098,#29260,#24454,.T.);
#34835=EDGE_CURVE('',#29261,#29258,#16309,.T.);
#34836=EDGE_CURVE('',#29260,#29261,#16310,.T.);
#34837=EDGE_CURVE('',#29262,#29098,#24455,.T.);
#34838=EDGE_CURVE('',#29262,#29263,#16311,.T.);
#34839=EDGE_CURVE('',#29095,#29263,#21438,.T.);
#34840=EDGE_CURVE('',#29263,#29264,#16312,.T.);
#34841=EDGE_CURVE('',#29092,#29264,#24456,.T.);
#34842=EDGE_CURVE('',#29265,#29262,#16313,.T.);
#34843=EDGE_CURVE('',#29264,#29265,#16314,.T.);
#34844=EDGE_CURVE('',#29266,#29092,#24457,.T.);
#34845=EDGE_CURVE('',#29266,#29267,#16315,.T.);
#34846=EDGE_CURVE('',#29089,#29267,#21439,.T.);
#34847=EDGE_CURVE('',#29267,#29268,#16316,.T.);
#34848=EDGE_CURVE('',#29086,#29268,#24458,.T.);
#34849=EDGE_CURVE('',#29269,#29266,#16317,.T.);
#34850=EDGE_CURVE('',#29268,#29269,#16318,.T.);
#34851=EDGE_CURVE('',#29270,#29086,#24459,.T.);
#34852=EDGE_CURVE('',#29270,#29271,#16319,.T.);
#34853=EDGE_CURVE('',#29083,#29271,#21440,.T.);
#34854=EDGE_CURVE('',#29271,#29272,#16320,.T.);
#34855=EDGE_CURVE('',#29080,#29272,#24460,.T.);
#34856=EDGE_CURVE('',#29273,#29270,#16321,.T.);
#34857=EDGE_CURVE('',#29272,#29273,#16322,.T.);
#34858=EDGE_CURVE('',#29274,#29080,#24461,.T.);
#34859=EDGE_CURVE('',#29274,#29275,#16323,.T.);
#34860=EDGE_CURVE('',#29077,#29275,#21441,.T.);
#34861=EDGE_CURVE('',#29275,#29276,#16324,.T.);
#34862=EDGE_CURVE('',#29074,#29276,#24462,.T.);
#34863=EDGE_CURVE('',#29277,#29274,#16325,.T.);
#34864=EDGE_CURVE('',#29276,#29277,#16326,.T.);
#34865=EDGE_CURVE('',#29278,#29074,#24463,.T.);
#34866=EDGE_CURVE('',#29278,#29279,#16327,.T.);
#34867=EDGE_CURVE('',#29071,#29279,#21442,.T.);
#34868=EDGE_CURVE('',#29279,#29280,#16328,.T.);
#34869=EDGE_CURVE('',#29070,#29280,#24464,.T.);
#34870=EDGE_CURVE('',#29281,#29278,#16329,.T.);
#34871=EDGE_CURVE('',#29280,#29281,#16330,.T.);
#34872=EDGE_CURVE('',#29282,#29070,#24465,.T.);
#34873=EDGE_CURVE('',#29282,#29283,#16331,.T.);
#34874=EDGE_CURVE('',#29069,#29283,#21443,.T.);
#34875=EDGE_CURVE('',#29283,#29284,#16332,.T.);
#34876=EDGE_CURVE('',#29066,#29284,#24466,.T.);
#34877=EDGE_CURVE('',#29285,#29282,#16333,.T.);
#34878=EDGE_CURVE('',#29284,#29285,#16334,.T.);
#34879=EDGE_CURVE('',#29286,#29066,#24467,.T.);
#34880=EDGE_CURVE('',#29286,#29287,#16335,.T.);
#34881=EDGE_CURVE('',#29063,#29287,#21444,.T.);
#34882=EDGE_CURVE('',#29287,#29288,#16336,.T.);
#34883=EDGE_CURVE('',#29060,#29288,#24468,.T.);
#34884=EDGE_CURVE('',#29289,#29286,#16337,.T.);
#34885=EDGE_CURVE('',#29288,#29289,#16338,.T.);
#34886=EDGE_CURVE('',#29290,#29060,#24469,.T.);
#34887=EDGE_CURVE('',#29290,#29291,#16339,.T.);
#34888=EDGE_CURVE('',#29057,#29291,#21445,.T.);
#34889=EDGE_CURVE('',#29291,#29292,#16340,.T.);
#34890=EDGE_CURVE('',#29054,#29292,#24470,.T.);
#34891=EDGE_CURVE('',#29293,#29290,#16341,.T.);
#34892=EDGE_CURVE('',#29292,#29293,#16342,.T.);
#34893=EDGE_CURVE('',#29294,#29054,#24471,.T.);
#34894=EDGE_CURVE('',#29294,#29295,#16343,.T.);
#34895=EDGE_CURVE('',#29051,#29295,#21446,.T.);
#34896=EDGE_CURVE('',#29295,#29296,#16344,.T.);
#34897=EDGE_CURVE('',#29048,#29296,#24472,.T.);
#34898=EDGE_CURVE('',#29297,#29294,#16345,.T.);
#34899=EDGE_CURVE('',#29296,#29297,#16346,.T.);
#34900=EDGE_CURVE('',#29298,#29048,#24473,.T.);
#34901=EDGE_CURVE('',#29298,#29299,#16347,.T.);
#34902=EDGE_CURVE('',#29045,#29299,#21447,.T.);
#34903=EDGE_CURVE('',#29299,#29300,#16348,.T.);
#34904=EDGE_CURVE('',#29042,#29300,#24474,.T.);
#34905=EDGE_CURVE('',#29301,#29298,#16349,.T.);
#34906=EDGE_CURVE('',#29300,#29301,#16350,.T.);
#34907=EDGE_CURVE('',#29302,#29042,#24475,.T.);
#34908=EDGE_CURVE('',#29302,#29303,#16351,.T.);
#34909=EDGE_CURVE('',#29039,#29303,#21448,.T.);
#34910=EDGE_CURVE('',#29303,#29304,#16352,.T.);
#34911=EDGE_CURVE('',#29036,#29304,#24476,.T.);
#34912=EDGE_CURVE('',#29305,#29302,#16353,.T.);
#34913=EDGE_CURVE('',#29304,#29305,#16354,.T.);
#34914=EDGE_CURVE('',#29306,#29036,#24477,.T.);
#34915=EDGE_CURVE('',#29306,#29307,#16355,.T.);
#34916=EDGE_CURVE('',#29032,#29307,#21449,.T.);
#34917=EDGE_CURVE('',#29307,#29308,#16356,.T.);
#34918=EDGE_CURVE('',#29033,#29308,#24478,.T.);
#34919=EDGE_CURVE('',#29309,#29306,#16357,.T.);
#34920=EDGE_CURVE('',#29308,#29309,#16358,.T.);
#34921=EDGE_CURVE('',#29310,#29200,#16359,.T.);
#34922=EDGE_CURVE('',#29311,#29310,#16360,.T.);
#34923=EDGE_CURVE('',#29201,#29311,#16361,.T.);
#34924=EDGE_CURVE('',#29310,#29033,#24479,.T.);
#34925=EDGE_CURVE('',#29032,#29312,#16362,.T.);
#34926=EDGE_CURVE('',#29312,#29198,#21450,.T.);
#34927=EDGE_CURVE('',#29313,#29032,#4376,.T.);
#34928=EDGE_CURVE('',#29037,#29313,#21451,.T.);
#34929=EDGE_CURVE('',#29039,#29313,#16363,.T.);
#34930=EDGE_CURVE('',#29314,#29039,#4377,.T.);
#34931=EDGE_CURVE('',#29043,#29314,#21452,.T.);
#34932=EDGE_CURVE('',#29045,#29314,#16364,.T.);
#34933=EDGE_CURVE('',#29315,#29045,#4378,.T.);
#34934=EDGE_CURVE('',#29049,#29315,#21453,.T.);
#34935=EDGE_CURVE('',#29051,#29315,#16365,.T.);
#34936=EDGE_CURVE('',#29316,#29051,#4379,.T.);
#34937=EDGE_CURVE('',#29055,#29316,#21454,.T.);
#34938=EDGE_CURVE('',#29057,#29316,#16366,.T.);
#34939=EDGE_CURVE('',#29317,#29057,#4380,.T.);
#34940=EDGE_CURVE('',#29061,#29317,#21455,.T.);
#34941=EDGE_CURVE('',#29063,#29317,#16367,.T.);
#34942=EDGE_CURVE('',#29318,#29063,#4381,.T.);
#34943=EDGE_CURVE('',#29067,#29318,#21456,.T.);
#34944=EDGE_CURVE('',#29069,#29318,#16368,.T.);
#34945=EDGE_CURVE('',#29319,#29069,#4382,.T.);
#34946=EDGE_CURVE('',#29029,#29319,#21457,.T.);
#34947=EDGE_CURVE('',#29071,#29319,#16369,.T.);
#34948=EDGE_CURVE('',#29320,#29071,#21458,.T.);
#34949=EDGE_CURVE('',#29075,#29320,#21459,.T.);
#34950=EDGE_CURVE('',#29077,#29320,#16370,.T.);
#34951=EDGE_CURVE('',#29321,#29077,#4383,.T.);
#34952=EDGE_CURVE('',#29081,#29321,#21460,.T.);
#34953=EDGE_CURVE('',#29083,#29321,#16371,.T.);
#34954=EDGE_CURVE('',#29322,#29083,#4384,.T.);
#34955=EDGE_CURVE('',#29087,#29322,#21461,.T.);
#34956=EDGE_CURVE('',#29089,#29322,#16372,.T.);
#34957=EDGE_CURVE('',#29323,#29089,#4385,.T.);
#34958=EDGE_CURVE('',#29093,#29323,#21462,.T.);
#34959=EDGE_CURVE('',#29095,#29323,#16373,.T.);
#34960=EDGE_CURVE('',#29324,#29095,#4386,.T.);
#34961=EDGE_CURVE('',#29099,#29324,#21463,.T.);
#34962=EDGE_CURVE('',#29101,#29324,#16374,.T.);
#34963=EDGE_CURVE('',#29325,#29101,#21464,.T.);
#34964=EDGE_CURVE('',#29105,#29325,#21465,.T.);
#34965=EDGE_CURVE('',#29107,#29325,#16375,.T.);
#34966=EDGE_CURVE('',#29326,#29107,#21466,.T.);
#34967=EDGE_CURVE('',#29111,#29326,#21467,.T.);
#34968=EDGE_CURVE('',#29113,#29326,#16376,.T.);
#34969=EDGE_CURVE('',#29327,#29113,#4387,.T.);
#34970=EDGE_CURVE('',#29117,#29327,#21468,.T.);
#34971=EDGE_CURVE('',#29119,#29327,#16377,.T.);
#34972=EDGE_CURVE('',#29328,#29119,#4388,.T.);
#34973=EDGE_CURVE('',#29123,#29328,#21469,.T.);
#34974=EDGE_CURVE('',#29125,#29328,#16378,.T.);
#34975=EDGE_CURVE('',#29329,#29125,#21470,.T.);
#34976=EDGE_CURVE('',#29129,#29329,#21471,.T.);
#34977=EDGE_CURVE('',#29131,#29329,#16379,.T.);
#34978=EDGE_CURVE('',#29330,#29131,#4389,.T.);
#34979=EDGE_CURVE('',#29135,#29330,#21472,.T.);
#34980=EDGE_CURVE('',#29137,#29330,#16380,.T.);
#34981=EDGE_CURVE('',#29331,#29137,#4390,.T.);
#34982=EDGE_CURVE('',#29141,#29331,#21473,.T.);
#34983=EDGE_CURVE('',#29143,#29331,#16381,.T.);
#34984=EDGE_CURVE('',#29332,#29143,#4391,.T.);
#34985=EDGE_CURVE('',#29147,#29332,#21474,.T.);
#34986=EDGE_CURVE('',#29149,#29332,#16382,.T.);
#34987=EDGE_CURVE('',#29333,#29149,#4392,.T.);
#34988=EDGE_CURVE('',#29153,#29333,#21475,.T.);
#34989=EDGE_CURVE('',#29155,#29333,#16383,.T.);
#34990=EDGE_CURVE('',#29334,#29155,#4393,.T.);
#34991=EDGE_CURVE('',#29159,#29334,#21476,.T.);
#34992=EDGE_CURVE('',#29161,#29334,#16384,.T.);
#34993=EDGE_CURVE('',#29335,#29161,#21477,.T.);
#34994=EDGE_CURVE('',#29165,#29335,#21478,.T.);
#34995=EDGE_CURVE('',#29167,#29335,#16385,.T.);
#34996=EDGE_CURVE('',#29336,#29167,#21479,.T.);
#34997=EDGE_CURVE('',#29171,#29336,#21480,.T.);
#34998=EDGE_CURVE('',#29173,#29336,#16386,.T.);
#34999=EDGE_CURVE('',#29337,#29173,#21481,.T.);
#35000=EDGE_CURVE('',#29179,#29337,#21482,.T.);
#35001=EDGE_CURVE('',#29178,#29337,#16387,.T.);
#35002=EDGE_CURVE('',#29338,#29178,#4394,.T.);
#35003=EDGE_CURVE('',#29184,#29338,#21483,.T.);
#35004=EDGE_CURVE('',#29185,#29338,#16388,.T.);
#35005=EDGE_CURVE('',#29339,#29185,#4395,.T.);
#35006=EDGE_CURVE('',#29189,#29339,#21484,.T.);
#35007=EDGE_CURVE('',#29191,#29339,#16389,.T.);
#35008=EDGE_CURVE('',#29340,#29191,#4396,.T.);
#35009=EDGE_CURVE('',#29195,#29340,#21485,.T.);
#35010=EDGE_CURVE('',#29197,#29340,#16390,.T.);
#35011=EDGE_CURVE('',#29312,#29197,#21486,.T.);
#35012=EDGE_CURVE('',#29341,#29311,#21487,.T.);
#35013=EDGE_CURVE('',#29194,#29341,#16391,.T.);
#35014=EDGE_CURVE('',#29342,#29194,#16392,.T.);
#35015=EDGE_CURVE('',#29205,#29342,#21488,.T.);
#35016=EDGE_CURVE('',#29188,#29342,#16393,.T.);
#35017=EDGE_CURVE('',#29343,#29188,#16394,.T.);
#35018=EDGE_CURVE('',#29209,#29343,#21489,.T.);
#35019=EDGE_CURVE('',#29182,#29343,#16395,.T.);
#35020=EDGE_CURVE('',#29344,#29182,#16396,.T.);
#35021=EDGE_CURVE('',#29213,#29344,#21490,.T.);
#35022=EDGE_CURVE('',#29176,#29344,#16397,.T.);
#35023=EDGE_CURVE('',#29345,#29176,#16398,.T.);
#35024=EDGE_CURVE('',#29217,#29345,#21491,.T.);
#35025=EDGE_CURVE('',#29170,#29345,#16399,.T.);
#35026=EDGE_CURVE('',#29346,#29170,#16400,.T.);
#35027=EDGE_CURVE('',#29221,#29346,#21492,.T.);
#35028=EDGE_CURVE('',#29164,#29346,#16401,.T.);
#35029=EDGE_CURVE('',#29347,#29164,#16402,.T.);
#35030=EDGE_CURVE('',#29225,#29347,#21493,.T.);
#35031=EDGE_CURVE('',#29158,#29347,#16403,.T.);
#35032=EDGE_CURVE('',#29348,#29158,#16404,.T.);
#35033=EDGE_CURVE('',#29229,#29348,#21494,.T.);
#35034=EDGE_CURVE('',#29152,#29348,#16405,.T.);
#35035=EDGE_CURVE('',#29349,#29152,#16406,.T.);
#35036=EDGE_CURVE('',#29233,#29349,#21495,.T.);
#35037=EDGE_CURVE('',#29146,#29349,#16407,.T.);
#35038=EDGE_CURVE('',#29350,#29146,#16408,.T.);
#35039=EDGE_CURVE('',#29237,#29350,#21496,.T.);
#35040=EDGE_CURVE('',#29140,#29350,#16409,.T.);
#35041=EDGE_CURVE('',#29351,#29140,#16410,.T.);
#35042=EDGE_CURVE('',#29241,#29351,#21497,.T.);
#35043=EDGE_CURVE('',#29134,#29351,#16411,.T.);
#35044=EDGE_CURVE('',#29352,#29134,#16412,.T.);
#35045=EDGE_CURVE('',#29245,#29352,#21498,.T.);
#35046=EDGE_CURVE('',#29128,#29352,#16413,.T.);
#35047=EDGE_CURVE('',#29353,#29128,#16414,.T.);
#35048=EDGE_CURVE('',#29249,#29353,#21499,.T.);
#35049=EDGE_CURVE('',#29122,#29353,#16415,.T.);
#35050=EDGE_CURVE('',#29354,#29122,#16416,.T.);
#35051=EDGE_CURVE('',#29253,#29354,#21500,.T.);
#35052=EDGE_CURVE('',#29116,#29354,#16417,.T.);
#35053=EDGE_CURVE('',#29355,#29116,#16418,.T.);
#35054=EDGE_CURVE('',#29023,#29355,#21501,.T.);
#35055=EDGE_CURVE('',#29110,#29355,#16419,.T.);
#35056=EDGE_CURVE('',#29356,#29110,#16420,.T.);
#35057=EDGE_CURVE('',#29257,#29356,#21502,.T.);
#35058=EDGE_CURVE('',#29104,#29356,#16421,.T.);
#35059=EDGE_CURVE('',#29357,#29104,#16422,.T.);
#35060=EDGE_CURVE('',#29261,#29357,#21503,.T.);
#35061=EDGE_CURVE('',#29098,#29357,#16423,.T.);
#35062=EDGE_CURVE('',#29358,#29098,#16424,.T.);
#35063=EDGE_CURVE('',#29265,#29358,#21504,.T.);
#35064=EDGE_CURVE('',#29092,#29358,#16425,.T.);
#35065=EDGE_CURVE('',#29359,#29092,#16426,.T.);
#35066=EDGE_CURVE('',#29269,#29359,#21505,.T.);
#35067=EDGE_CURVE('',#29086,#29359,#16427,.T.);
#35068=EDGE_CURVE('',#29360,#29086,#16428,.T.);
#35069=EDGE_CURVE('',#29273,#29360,#21506,.T.);
#35070=EDGE_CURVE('',#29080,#29360,#16429,.T.);
#35071=EDGE_CURVE('',#29361,#29080,#16430,.T.);
#35072=EDGE_CURVE('',#29277,#29361,#21507,.T.);
#35073=EDGE_CURVE('',#29074,#29361,#16431,.T.);
#35074=EDGE_CURVE('',#29362,#29074,#16432,.T.);
#35075=EDGE_CURVE('',#29281,#29362,#21508,.T.);
#35076=EDGE_CURVE('',#29070,#29362,#16433,.T.);
#35077=EDGE_CURVE('',#29363,#29070,#16434,.T.);
#35078=EDGE_CURVE('',#29285,#29363,#21509,.T.);
#35079=EDGE_CURVE('',#29066,#29363,#16435,.T.);
#35080=EDGE_CURVE('',#29364,#29066,#16436,.T.);
#35081=EDGE_CURVE('',#29289,#29364,#21510,.T.);
#35082=EDGE_CURVE('',#29060,#29364,#16437,.T.);
#35083=EDGE_CURVE('',#29365,#29060,#16438,.T.);
#35084=EDGE_CURVE('',#29293,#29365,#21511,.T.);
#35085=EDGE_CURVE('',#29054,#29365,#16439,.T.);
#35086=EDGE_CURVE('',#29366,#29054,#16440,.T.);
#35087=EDGE_CURVE('',#29297,#29366,#21512,.T.);
#35088=EDGE_CURVE('',#29048,#29366,#16441,.T.);
#35089=EDGE_CURVE('',#29367,#29048,#16442,.T.);
#35090=EDGE_CURVE('',#29301,#29367,#21513,.T.);
#35091=EDGE_CURVE('',#29042,#29367,#16443,.T.);
#35092=EDGE_CURVE('',#29368,#29042,#16444,.T.);
#35093=EDGE_CURVE('',#29305,#29368,#21514,.T.);
#35094=EDGE_CURVE('',#29036,#29368,#16445,.T.);
#35095=EDGE_CURVE('',#29369,#29036,#16446,.T.);
#35096=EDGE_CURVE('',#29309,#29369,#21515,.T.);
#35097=EDGE_CURVE('',#29033,#29369,#16447,.T.);
#35098=EDGE_CURVE('',#29341,#29033,#16448,.T.);
#35099=EDGE_CURVE('',#29370,#29371,#16449,.T.);
#35100=EDGE_CURVE('',#29032,#29371,#21516,.T.);
#35101=EDGE_CURVE('',#29370,#29312,#24480,.T.);
#35102=EDGE_CURVE('',#29372,#29370,#16450,.T.);
#35103=EDGE_CURVE('',#29373,#29372,#21517,.T.);
#35104=EDGE_CURVE('',#29371,#29373,#21518,.T.);
#35105=EDGE_CURVE('',#29313,#29373,#24481,.T.);
#35106=EDGE_CURVE('',#29374,#29375,#16451,.T.);
#35107=EDGE_CURVE('',#29039,#29375,#21519,.T.);
#35108=EDGE_CURVE('',#29374,#29313,#24482,.T.);
#35109=EDGE_CURVE('',#29376,#29374,#16452,.T.);
#35110=EDGE_CURVE('',#29377,#29376,#21520,.T.);
#35111=EDGE_CURVE('',#29375,#29377,#21521,.T.);
#35112=EDGE_CURVE('',#29314,#29377,#24483,.T.);
#35113=EDGE_CURVE('',#29378,#29379,#16453,.T.);
#35114=EDGE_CURVE('',#29045,#29379,#21522,.T.);
#35115=EDGE_CURVE('',#29378,#29314,#24484,.T.);
#35116=EDGE_CURVE('',#29380,#29378,#16454,.T.);
#35117=EDGE_CURVE('',#29381,#29380,#21523,.T.);
#35118=EDGE_CURVE('',#29379,#29381,#21524,.T.);
#35119=EDGE_CURVE('',#29315,#29381,#24485,.T.);
#35120=EDGE_CURVE('',#29382,#29383,#16455,.T.);
#35121=EDGE_CURVE('',#29051,#29383,#21525,.T.);
#35122=EDGE_CURVE('',#29382,#29315,#24486,.T.);
#35123=EDGE_CURVE('',#29384,#29382,#16456,.T.);
#35124=EDGE_CURVE('',#29385,#29384,#21526,.T.);
#35125=EDGE_CURVE('',#29383,#29385,#21527,.T.);
#35126=EDGE_CURVE('',#29316,#29385,#24487,.T.);
#35127=EDGE_CURVE('',#29386,#29387,#16457,.T.);
#35128=EDGE_CURVE('',#29057,#29387,#21528,.T.);
#35129=EDGE_CURVE('',#29386,#29316,#24488,.T.);
#35130=EDGE_CURVE('',#29388,#29386,#16458,.T.);
#35131=EDGE_CURVE('',#29389,#29388,#21529,.T.);
#35132=EDGE_CURVE('',#29387,#29389,#21530,.T.);
#35133=EDGE_CURVE('',#29317,#29389,#24489,.T.);
#35134=EDGE_CURVE('',#29390,#29391,#16459,.T.);
#35135=EDGE_CURVE('',#29063,#29391,#21531,.T.);
#35136=EDGE_CURVE('',#29390,#29317,#24490,.T.);
#35137=EDGE_CURVE('',#29392,#29390,#16460,.T.);
#35138=EDGE_CURVE('',#29393,#29392,#21532,.T.);
#35139=EDGE_CURVE('',#29391,#29393,#21533,.T.);
#35140=EDGE_CURVE('',#29318,#29393,#24491,.T.);
#35141=EDGE_CURVE('',#29394,#29395,#16461,.T.);
#35142=EDGE_CURVE('',#29069,#29395,#21534,.T.);
#35143=EDGE_CURVE('',#29394,#29318,#24492,.T.);
#35144=EDGE_CURVE('',#29396,#29394,#16462,.T.);
#35145=EDGE_CURVE('',#29397,#29396,#21535,.T.);
#35146=EDGE_CURVE('',#29395,#29397,#21536,.T.);
#35147=EDGE_CURVE('',#29319,#29397,#24493,.T.);
#35148=EDGE_CURVE('',#29398,#29399,#16463,.T.);
#35149=EDGE_CURVE('',#29071,#29399,#21537,.T.);
#35150=EDGE_CURVE('',#29398,#29319,#24494,.T.);
#35151=EDGE_CURVE('',#29400,#29398,#16464,.T.);
#35152=EDGE_CURVE('',#29401,#29400,#21538,.T.);
#35153=EDGE_CURVE('',#29399,#29401,#21539,.T.);
#35154=EDGE_CURVE('',#29320,#29401,#24495,.T.);
#35155=EDGE_CURVE('',#29402,#29403,#16465,.T.);
#35156=EDGE_CURVE('',#29077,#29403,#21540,.T.);
#35157=EDGE_CURVE('',#29402,#29320,#24496,.T.);
#35158=EDGE_CURVE('',#29404,#29402,#16466,.T.);
#35159=EDGE_CURVE('',#29405,#29404,#21541,.T.);
#35160=EDGE_CURVE('',#29403,#29405,#21542,.T.);
#35161=EDGE_CURVE('',#29321,#29405,#24497,.T.);
#35162=EDGE_CURVE('',#29406,#29407,#16467,.T.);
#35163=EDGE_CURVE('',#29083,#29407,#21543,.T.);
#35164=EDGE_CURVE('',#29406,#29321,#24498,.T.);
#35165=EDGE_CURVE('',#29408,#29406,#16468,.T.);
#35166=EDGE_CURVE('',#29409,#29408,#21544,.T.);
#35167=EDGE_CURVE('',#29407,#29409,#21545,.T.);
#35168=EDGE_CURVE('',#29322,#29409,#24499,.T.);
#35169=EDGE_CURVE('',#29410,#29411,#16469,.T.);
#35170=EDGE_CURVE('',#29089,#29411,#21546,.T.);
#35171=EDGE_CURVE('',#29410,#29322,#24500,.T.);
#35172=EDGE_CURVE('',#29412,#29410,#16470,.T.);
#35173=EDGE_CURVE('',#29413,#29412,#21547,.T.);
#35174=EDGE_CURVE('',#29411,#29413,#21548,.T.);
#35175=EDGE_CURVE('',#29323,#29413,#24501,.T.);
#35176=EDGE_CURVE('',#29414,#29415,#16471,.T.);
#35177=EDGE_CURVE('',#29095,#29415,#21549,.T.);
#35178=EDGE_CURVE('',#29414,#29323,#24502,.T.);
#35179=EDGE_CURVE('',#29416,#29414,#16472,.T.);
#35180=EDGE_CURVE('',#29417,#29416,#21550,.T.);
#35181=EDGE_CURVE('',#29415,#29417,#21551,.T.);
#35182=EDGE_CURVE('',#29324,#29417,#24503,.T.);
#35183=EDGE_CURVE('',#29418,#29419,#16473,.T.);
#35184=EDGE_CURVE('',#29101,#29419,#21552,.T.);
#35185=EDGE_CURVE('',#29418,#29324,#24504,.T.);
#35186=EDGE_CURVE('',#29420,#29418,#16474,.T.);
#35187=EDGE_CURVE('',#29421,#29420,#21553,.T.);
#35188=EDGE_CURVE('',#29419,#29421,#21554,.T.);
#35189=EDGE_CURVE('',#29325,#29421,#24505,.T.);
#35190=EDGE_CURVE('',#29422,#29423,#16475,.T.);
#35191=EDGE_CURVE('',#29107,#29423,#21555,.T.);
#35192=EDGE_CURVE('',#29422,#29325,#24506,.T.);
#35193=EDGE_CURVE('',#29424,#29422,#16476,.T.);
#35194=EDGE_CURVE('',#29425,#29424,#21556,.T.);
#35195=EDGE_CURVE('',#29423,#29425,#21557,.T.);
#35196=EDGE_CURVE('',#29326,#29425,#24507,.T.);
#35197=EDGE_CURVE('',#29113,#29019,#21558,.T.);
#35198=EDGE_CURVE('',#29018,#29326,#24508,.T.);
#35199=EDGE_CURVE('',#29327,#29021,#24509,.T.);
#35200=EDGE_CURVE('',#29426,#29427,#16477,.T.);
#35201=EDGE_CURVE('',#29119,#29427,#21559,.T.);
#35202=EDGE_CURVE('',#29426,#29327,#24510,.T.);
#35203=EDGE_CURVE('',#29428,#29426,#16478,.T.);
#35204=EDGE_CURVE('',#29429,#29428,#21560,.T.);
#35205=EDGE_CURVE('',#29427,#29429,#21561,.T.);
#35206=EDGE_CURVE('',#29328,#29429,#24511,.T.);
#35207=EDGE_CURVE('',#29430,#29431,#16479,.T.);
#35208=EDGE_CURVE('',#29125,#29431,#21562,.T.);
#35209=EDGE_CURVE('',#29430,#29328,#24512,.T.);
#35210=EDGE_CURVE('',#29432,#29430,#16480,.T.);
#35211=EDGE_CURVE('',#29433,#29432,#21563,.T.);
#35212=EDGE_CURVE('',#29431,#29433,#21564,.T.);
#35213=EDGE_CURVE('',#29329,#29433,#24513,.T.);
#35214=EDGE_CURVE('',#29434,#29435,#16481,.T.);
#35215=EDGE_CURVE('',#29131,#29435,#21565,.T.);
#35216=EDGE_CURVE('',#29434,#29329,#24514,.T.);
#35217=EDGE_CURVE('',#29436,#29434,#16482,.T.);
#35218=EDGE_CURVE('',#29437,#29436,#21566,.T.);
#35219=EDGE_CURVE('',#29435,#29437,#21567,.T.);
#35220=EDGE_CURVE('',#29330,#29437,#24515,.T.);
#35221=EDGE_CURVE('',#29438,#29439,#16483,.T.);
#35222=EDGE_CURVE('',#29137,#29439,#21568,.T.);
#35223=EDGE_CURVE('',#29438,#29330,#24516,.T.);
#35224=EDGE_CURVE('',#29440,#29438,#16484,.T.);
#35225=EDGE_CURVE('',#29441,#29440,#21569,.T.);
#35226=EDGE_CURVE('',#29439,#29441,#21570,.T.);
#35227=EDGE_CURVE('',#29331,#29441,#24517,.T.);
#35228=EDGE_CURVE('',#29442,#29443,#16485,.T.);
#35229=EDGE_CURVE('',#29143,#29443,#21571,.T.);
#35230=EDGE_CURVE('',#29442,#29331,#24518,.T.);
#35231=EDGE_CURVE('',#29444,#29442,#16486,.T.);
#35232=EDGE_CURVE('',#29445,#29444,#21572,.T.);
#35233=EDGE_CURVE('',#29443,#29445,#21573,.T.);
#35234=EDGE_CURVE('',#29332,#29445,#24519,.T.);
#35235=EDGE_CURVE('',#29446,#29447,#16487,.T.);
#35236=EDGE_CURVE('',#29149,#29447,#21574,.T.);
#35237=EDGE_CURVE('',#29446,#29332,#24520,.T.);
#35238=EDGE_CURVE('',#29448,#29446,#16488,.T.);
#35239=EDGE_CURVE('',#29449,#29448,#21575,.T.);
#35240=EDGE_CURVE('',#29447,#29449,#21576,.T.);
#35241=EDGE_CURVE('',#29333,#29449,#24521,.T.);
#35242=EDGE_CURVE('',#29450,#29451,#16489,.T.);
#35243=EDGE_CURVE('',#29155,#29451,#21577,.T.);
#35244=EDGE_CURVE('',#29450,#29333,#24522,.T.);
#35245=EDGE_CURVE('',#29452,#29450,#16490,.T.);
#35246=EDGE_CURVE('',#29453,#29452,#21578,.T.);
#35247=EDGE_CURVE('',#29451,#29453,#21579,.T.);
#35248=EDGE_CURVE('',#29334,#29453,#24523,.T.);
#35249=EDGE_CURVE('',#29454,#29455,#16491,.T.);
#35250=EDGE_CURVE('',#29161,#29455,#21580,.T.);
#35251=EDGE_CURVE('',#29454,#29334,#24524,.T.);
#35252=EDGE_CURVE('',#29456,#29454,#16492,.T.);
#35253=EDGE_CURVE('',#29457,#29456,#21581,.T.);
#35254=EDGE_CURVE('',#29455,#29457,#21582,.T.);
#35255=EDGE_CURVE('',#29335,#29457,#24525,.T.);
#35256=EDGE_CURVE('',#29458,#29459,#16493,.T.);
#35257=EDGE_CURVE('',#29167,#29459,#21583,.T.);
#35258=EDGE_CURVE('',#29458,#29335,#24526,.T.);
#35259=EDGE_CURVE('',#29460,#29458,#16494,.T.);
#35260=EDGE_CURVE('',#29461,#29460,#21584,.T.);
#35261=EDGE_CURVE('',#29459,#29461,#21585,.T.);
#35262=EDGE_CURVE('',#29336,#29461,#24527,.T.);
#35263=EDGE_CURVE('',#29462,#29463,#16495,.T.);
#35264=EDGE_CURVE('',#29173,#29463,#21586,.T.);
#35265=EDGE_CURVE('',#29462,#29336,#24528,.T.);
#35266=EDGE_CURVE('',#29463,#29464,#21587,.T.);
#35267=EDGE_CURVE('',#29337,#29464,#24529,.T.);
#35268=EDGE_CURVE('',#29465,#29462,#16496,.T.);
#35269=EDGE_CURVE('',#29464,#29465,#21588,.T.);
#35270=EDGE_CURVE('',#29466,#29337,#24530,.T.);
#35271=EDGE_CURVE('',#29466,#29467,#16497,.T.);
#35272=EDGE_CURVE('',#29178,#29467,#21589,.T.);
#35273=EDGE_CURVE('',#29467,#29468,#21590,.T.);
#35274=EDGE_CURVE('',#29469,#29466,#16498,.T.);
#35275=EDGE_CURVE('',#29468,#29469,#21591,.T.);
#35276=EDGE_CURVE('',#29338,#29468,#24531,.T.);
#35277=EDGE_CURVE('',#29470,#29471,#16499,.T.);
#35278=EDGE_CURVE('',#29185,#29471,#21592,.T.);
#35279=EDGE_CURVE('',#29470,#29338,#24532,.T.);
#35280=EDGE_CURVE('',#29472,#29470,#16500,.T.);
#35281=EDGE_CURVE('',#29473,#29472,#21593,.T.);
#35282=EDGE_CURVE('',#29471,#29473,#21594,.T.);
#35283=EDGE_CURVE('',#29339,#29473,#24533,.T.);
#35284=EDGE_CURVE('',#29474,#29475,#16501,.T.);
#35285=EDGE_CURVE('',#29191,#29475,#21595,.T.);
#35286=EDGE_CURVE('',#29474,#29339,#24534,.T.);
#35287=EDGE_CURVE('',#29476,#29474,#16502,.T.);
#35288=EDGE_CURVE('',#29477,#29476,#21596,.T.);
#35289=EDGE_CURVE('',#29475,#29477,#21597,.T.);
#35290=EDGE_CURVE('',#29340,#29477,#24535,.T.);
#35291=EDGE_CURVE('',#29478,#29479,#16503,.T.);
#35292=EDGE_CURVE('',#29197,#29479,#21598,.T.);
#35293=EDGE_CURVE('',#29478,#29340,#24536,.T.);
#35294=EDGE_CURVE('',#29480,#29478,#16504,.T.);
#35295=EDGE_CURVE('',#29481,#29480,#21599,.T.);
#35296=EDGE_CURVE('',#29479,#29481,#21600,.T.);
#35297=EDGE_CURVE('',#29312,#29481,#24537,.T.);
#35298=EDGE_CURVE('',#29482,#29341,#24538,.T.);
#35299=EDGE_CURVE('',#29482,#29483,#16505,.T.);
#35300=EDGE_CURVE('',#29194,#29483,#21601,.T.);
#35301=EDGE_CURVE('',#29483,#29484,#16506,.T.);
#35302=EDGE_CURVE('',#29342,#29484,#24539,.T.);
#35303=EDGE_CURVE('',#29485,#29482,#16507,.T.);
#35304=EDGE_CURVE('',#29484,#29485,#4397,.T.);
#35305=EDGE_CURVE('',#29486,#29342,#24540,.T.);
#35306=EDGE_CURVE('',#29486,#29487,#16508,.T.);
#35307=EDGE_CURVE('',#29188,#29487,#21602,.T.);
#35308=EDGE_CURVE('',#29487,#29488,#16509,.T.);
#35309=EDGE_CURVE('',#29343,#29488,#24541,.T.);
#35310=EDGE_CURVE('',#29489,#29486,#16510,.T.);
#35311=EDGE_CURVE('',#29488,#29489,#4398,.T.);
#35312=EDGE_CURVE('',#29490,#29343,#24542,.T.);
#35313=EDGE_CURVE('',#29490,#29491,#16511,.T.);
#35314=EDGE_CURVE('',#29182,#29491,#21603,.T.);
#35315=EDGE_CURVE('',#29491,#29492,#16512,.T.);
#35316=EDGE_CURVE('',#29344,#29492,#24543,.T.);
#35317=EDGE_CURVE('',#29493,#29490,#16513,.T.);
#35318=EDGE_CURVE('',#29492,#29493,#4399,.T.);
#35319=EDGE_CURVE('',#29494,#29344,#24544,.T.);
#35320=EDGE_CURVE('',#29494,#29495,#16514,.T.);
#35321=EDGE_CURVE('',#29176,#29495,#21604,.T.);
#35322=EDGE_CURVE('',#29495,#29496,#16515,.T.);
#35323=EDGE_CURVE('',#29345,#29496,#24545,.T.);
#35324=EDGE_CURVE('',#29497,#29494,#16516,.T.);
#35325=EDGE_CURVE('',#29496,#29497,#4400,.T.);
#35326=EDGE_CURVE('',#29498,#29345,#24546,.T.);
#35327=EDGE_CURVE('',#29498,#29499,#16517,.T.);
#35328=EDGE_CURVE('',#29170,#29499,#21605,.T.);
#35329=EDGE_CURVE('',#29499,#29500,#16518,.T.);
#35330=EDGE_CURVE('',#29346,#29500,#24547,.T.);
#35331=EDGE_CURVE('',#29501,#29498,#16519,.T.);
#35332=EDGE_CURVE('',#29500,#29501,#4401,.T.);
#35333=EDGE_CURVE('',#29502,#29346,#24548,.T.);
#35334=EDGE_CURVE('',#29502,#29503,#16520,.T.);
#35335=EDGE_CURVE('',#29164,#29503,#21606,.T.);
#35336=EDGE_CURVE('',#29503,#29504,#16521,.T.);
#35337=EDGE_CURVE('',#29347,#29504,#24549,.T.);
#35338=EDGE_CURVE('',#29505,#29502,#16522,.T.);
#35339=EDGE_CURVE('',#29504,#29505,#4402,.T.);
#35340=EDGE_CURVE('',#29506,#29347,#24550,.T.);
#35341=EDGE_CURVE('',#29506,#29507,#16523,.T.);
#35342=EDGE_CURVE('',#29158,#29507,#21607,.T.);
#35343=EDGE_CURVE('',#29507,#29508,#16524,.T.);
#35344=EDGE_CURVE('',#29348,#29508,#24551,.T.);
#35345=EDGE_CURVE('',#29509,#29506,#16525,.T.);
#35346=EDGE_CURVE('',#29508,#29509,#4403,.T.);
#35347=EDGE_CURVE('',#29510,#29348,#24552,.T.);
#35348=EDGE_CURVE('',#29510,#29511,#16526,.T.);
#35349=EDGE_CURVE('',#29152,#29511,#21608,.T.);
#35350=EDGE_CURVE('',#29511,#29512,#16527,.T.);
#35351=EDGE_CURVE('',#29349,#29512,#24553,.T.);
#35352=EDGE_CURVE('',#29513,#29510,#16528,.T.);
#35353=EDGE_CURVE('',#29512,#29513,#4404,.T.);
#35354=EDGE_CURVE('',#29514,#29349,#24554,.T.);
#35355=EDGE_CURVE('',#29514,#29515,#16529,.T.);
#35356=EDGE_CURVE('',#29146,#29515,#21609,.T.);
#35357=EDGE_CURVE('',#29515,#29516,#16530,.T.);
#35358=EDGE_CURVE('',#29350,#29516,#24555,.T.);
#35359=EDGE_CURVE('',#29517,#29514,#16531,.T.);
#35360=EDGE_CURVE('',#29516,#29517,#4405,.T.);
#35361=EDGE_CURVE('',#29518,#29350,#24556,.T.);
#35362=EDGE_CURVE('',#29518,#29519,#16532,.T.);
#35363=EDGE_CURVE('',#29140,#29519,#21610,.T.);
#35364=EDGE_CURVE('',#29519,#29520,#16533,.T.);
#35365=EDGE_CURVE('',#29351,#29520,#24557,.T.);
#35366=EDGE_CURVE('',#29521,#29518,#16534,.T.);
#35367=EDGE_CURVE('',#29520,#29521,#4406,.T.);
#35368=EDGE_CURVE('',#29522,#29351,#24558,.T.);
#35369=EDGE_CURVE('',#29522,#29523,#16535,.T.);
#35370=EDGE_CURVE('',#29134,#29523,#21611,.T.);
#35371=EDGE_CURVE('',#29523,#29524,#16536,.T.);
#35372=EDGE_CURVE('',#29352,#29524,#24559,.T.);
#35373=EDGE_CURVE('',#29525,#29522,#16537,.T.);
#35374=EDGE_CURVE('',#29524,#29525,#4407,.T.);
#35375=EDGE_CURVE('',#29526,#29352,#24560,.T.);
#35376=EDGE_CURVE('',#29526,#29527,#16538,.T.);
#35377=EDGE_CURVE('',#29128,#29527,#21612,.T.);
#35378=EDGE_CURVE('',#29527,#29528,#16539,.T.);
#35379=EDGE_CURVE('',#29353,#29528,#24561,.T.);
#35380=EDGE_CURVE('',#29529,#29526,#16540,.T.);
#35381=EDGE_CURVE('',#29528,#29529,#4408,.T.);
#35382=EDGE_CURVE('',#29530,#29353,#24562,.T.);
#35383=EDGE_CURVE('',#29530,#29531,#16541,.T.);
#35384=EDGE_CURVE('',#29122,#29531,#21613,.T.);
#35385=EDGE_CURVE('',#29531,#29532,#16542,.T.);
#35386=EDGE_CURVE('',#29354,#29532,#24563,.T.);
#35387=EDGE_CURVE('',#29533,#29530,#16543,.T.);
#35388=EDGE_CURVE('',#29532,#29533,#4409,.T.);
#35389=EDGE_CURVE('',#29534,#29354,#24564,.T.);
#35390=EDGE_CURVE('',#29534,#29535,#16544,.T.);
#35391=EDGE_CURVE('',#29116,#29535,#21614,.T.);
#35392=EDGE_CURVE('',#29535,#29536,#16545,.T.);
#35393=EDGE_CURVE('',#29355,#29536,#24565,.T.);
#35394=EDGE_CURVE('',#29537,#29534,#16546,.T.);
#35395=EDGE_CURVE('',#29536,#29537,#4410,.T.);
#35396=EDGE_CURVE('',#29538,#29355,#24566,.T.);
#35397=EDGE_CURVE('',#29538,#29539,#16547,.T.);
#35398=EDGE_CURVE('',#29110,#29539,#21615,.T.);
#35399=EDGE_CURVE('',#29539,#29540,#16548,.T.);
#35400=EDGE_CURVE('',#29356,#29540,#24567,.T.);
#35401=EDGE_CURVE('',#29541,#29538,#16549,.T.);
#35402=EDGE_CURVE('',#29540,#29541,#4411,.T.);
#35403=EDGE_CURVE('',#29542,#29356,#24568,.T.);
#35404=EDGE_CURVE('',#29542,#29543,#16550,.T.);
#35405=EDGE_CURVE('',#29104,#29543,#21616,.T.);
#35406=EDGE_CURVE('',#29543,#29544,#16551,.T.);
#35407=EDGE_CURVE('',#29357,#29544,#24569,.T.);
#35408=EDGE_CURVE('',#29545,#29542,#16552,.T.);
#35409=EDGE_CURVE('',#29544,#29545,#4412,.T.);
#35410=EDGE_CURVE('',#29546,#29357,#24570,.T.);
#35411=EDGE_CURVE('',#29546,#29547,#16553,.T.);
#35412=EDGE_CURVE('',#29098,#29547,#21617,.T.);
#35413=EDGE_CURVE('',#29547,#29548,#16554,.T.);
#35414=EDGE_CURVE('',#29358,#29548,#24571,.T.);
#35415=EDGE_CURVE('',#29549,#29546,#16555,.T.);
#35416=EDGE_CURVE('',#29548,#29549,#4413,.T.);
#35417=EDGE_CURVE('',#29550,#29358,#24572,.T.);
#35418=EDGE_CURVE('',#29550,#29551,#16556,.T.);
#35419=EDGE_CURVE('',#29092,#29551,#21618,.T.);
#35420=EDGE_CURVE('',#29551,#29552,#16557,.T.);
#35421=EDGE_CURVE('',#29359,#29552,#24573,.T.);
#35422=EDGE_CURVE('',#29553,#29550,#16558,.T.);
#35423=EDGE_CURVE('',#29552,#29553,#4414,.T.);
#35424=EDGE_CURVE('',#29554,#29359,#24574,.T.);
#35425=EDGE_CURVE('',#29554,#29555,#16559,.T.);
#35426=EDGE_CURVE('',#29086,#29555,#21619,.T.);
#35427=EDGE_CURVE('',#29555,#29556,#16560,.T.);
#35428=EDGE_CURVE('',#29360,#29556,#24575,.T.);
#35429=EDGE_CURVE('',#29557,#29554,#16561,.T.);
#35430=EDGE_CURVE('',#29556,#29557,#4415,.T.);
#35431=EDGE_CURVE('',#29558,#29360,#24576,.T.);
#35432=EDGE_CURVE('',#29558,#29559,#16562,.T.);
#35433=EDGE_CURVE('',#29080,#29559,#21620,.T.);
#35434=EDGE_CURVE('',#29559,#29560,#16563,.T.);
#35435=EDGE_CURVE('',#29361,#29560,#24577,.T.);
#35436=EDGE_CURVE('',#29561,#29558,#16564,.T.);
#35437=EDGE_CURVE('',#29560,#29561,#4416,.T.);
#35438=EDGE_CURVE('',#29562,#29361,#24578,.T.);
#35439=EDGE_CURVE('',#29562,#29563,#16565,.T.);
#35440=EDGE_CURVE('',#29074,#29563,#21621,.T.);
#35441=EDGE_CURVE('',#29563,#29564,#16566,.T.);
#35442=EDGE_CURVE('',#29362,#29564,#24579,.T.);
#35443=EDGE_CURVE('',#29565,#29562,#16567,.T.);
#35444=EDGE_CURVE('',#29564,#29565,#4417,.T.);
#35445=EDGE_CURVE('',#29015,#29362,#24580,.T.);
#35446=EDGE_CURVE('',#29070,#29017,#21622,.T.);
#35447=EDGE_CURVE('',#29363,#29016,#24581,.T.);
#35448=EDGE_CURVE('',#29566,#29363,#24582,.T.);
#35449=EDGE_CURVE('',#29566,#29567,#16568,.T.);
#35450=EDGE_CURVE('',#29066,#29567,#21623,.T.);
#35451=EDGE_CURVE('',#29567,#29568,#16569,.T.);
#35452=EDGE_CURVE('',#29364,#29568,#24583,.T.);
#35453=EDGE_CURVE('',#29569,#29566,#16570,.T.);
#35454=EDGE_CURVE('',#29568,#29569,#4418,.T.);
#35455=EDGE_CURVE('',#29570,#29364,#24584,.T.);
#35456=EDGE_CURVE('',#29570,#29571,#16571,.T.);
#35457=EDGE_CURVE('',#29060,#29571,#21624,.T.);
#35458=EDGE_CURVE('',#29571,#29572,#16572,.T.);
#35459=EDGE_CURVE('',#29365,#29572,#24585,.T.);
#35460=EDGE_CURVE('',#29573,#29570,#16573,.T.);
#35461=EDGE_CURVE('',#29572,#29573,#4419,.T.);
#35462=EDGE_CURVE('',#29574,#29365,#24586,.T.);
#35463=EDGE_CURVE('',#29574,#29575,#16574,.T.);
#35464=EDGE_CURVE('',#29054,#29575,#21625,.T.);
#35465=EDGE_CURVE('',#29575,#29576,#16575,.T.);
#35466=EDGE_CURVE('',#29366,#29576,#24587,.T.);
#35467=EDGE_CURVE('',#29577,#29574,#16576,.T.);
#35468=EDGE_CURVE('',#29576,#29577,#4420,.T.);
#35469=EDGE_CURVE('',#29578,#29366,#24588,.T.);
#35470=EDGE_CURVE('',#29578,#29579,#16577,.T.);
#35471=EDGE_CURVE('',#29048,#29579,#21626,.T.);
#35472=EDGE_CURVE('',#29579,#29580,#16578,.T.);
#35473=EDGE_CURVE('',#29367,#29580,#24589,.T.);
#35474=EDGE_CURVE('',#29581,#29578,#16579,.T.);
#35475=EDGE_CURVE('',#29580,#29581,#4421,.T.);
#35476=EDGE_CURVE('',#29582,#29367,#24590,.T.);
#35477=EDGE_CURVE('',#29582,#29583,#16580,.T.);
#35478=EDGE_CURVE('',#29042,#29583,#21627,.T.);
#35479=EDGE_CURVE('',#29583,#29584,#16581,.T.);
#35480=EDGE_CURVE('',#29368,#29584,#24591,.T.);
#35481=EDGE_CURVE('',#29585,#29582,#16582,.T.);
#35482=EDGE_CURVE('',#29584,#29585,#4422,.T.);
#35483=EDGE_CURVE('',#29586,#29368,#24592,.T.);
#35484=EDGE_CURVE('',#29586,#29587,#16583,.T.);
#35485=EDGE_CURVE('',#29036,#29587,#21628,.T.);
#35486=EDGE_CURVE('',#29587,#29588,#16584,.T.);
#35487=EDGE_CURVE('',#29369,#29588,#24593,.T.);
#35488=EDGE_CURVE('',#29589,#29586,#16585,.T.);
#35489=EDGE_CURVE('',#29588,#29589,#4423,.T.);
#35490=EDGE_CURVE('',#29590,#29369,#24594,.T.);
#35491=EDGE_CURVE('',#29590,#29591,#16586,.T.);
#35492=EDGE_CURVE('',#29033,#29591,#21629,.T.);
#35493=EDGE_CURVE('',#29591,#29592,#16587,.T.);
#35494=EDGE_CURVE('',#29341,#29592,#24595,.T.);
#35495=EDGE_CURVE('',#29593,#29590,#16588,.T.);
#35496=EDGE_CURVE('',#29592,#29593,#4424,.T.);
#35497=EDGE_CURVE('',#29594,#29312,#16589,.T.);
#35498=EDGE_CURVE('',#29372,#29594,#21630,.T.);
#35499=EDGE_CURVE('',#29313,#29594,#21631,.T.);
#35500=EDGE_CURVE('',#29595,#29313,#16590,.T.);
#35501=EDGE_CURVE('',#29376,#29595,#21632,.T.);
#35502=EDGE_CURVE('',#29314,#29595,#21633,.T.);
#35503=EDGE_CURVE('',#29596,#29314,#16591,.T.);
#35504=EDGE_CURVE('',#29380,#29596,#21634,.T.);
#35505=EDGE_CURVE('',#29315,#29596,#21635,.T.);
#35506=EDGE_CURVE('',#29597,#29315,#16592,.T.);
#35507=EDGE_CURVE('',#29384,#29597,#21636,.T.);
#35508=EDGE_CURVE('',#29316,#29597,#21637,.T.);
#35509=EDGE_CURVE('',#29598,#29316,#16593,.T.);
#35510=EDGE_CURVE('',#29388,#29598,#21638,.T.);
#35511=EDGE_CURVE('',#29317,#29598,#21639,.T.);
#35512=EDGE_CURVE('',#29599,#29317,#16594,.T.);
#35513=EDGE_CURVE('',#29392,#29599,#21640,.T.);
#35514=EDGE_CURVE('',#29318,#29599,#21641,.T.);
#35515=EDGE_CURVE('',#29600,#29318,#16595,.T.);
#35516=EDGE_CURVE('',#29396,#29600,#21642,.T.);
#35517=EDGE_CURVE('',#29319,#29600,#21643,.T.);
#35518=EDGE_CURVE('',#29601,#29319,#16596,.T.);
#35519=EDGE_CURVE('',#29400,#29601,#21644,.T.);
#35520=EDGE_CURVE('',#29320,#29601,#21645,.T.);
#35521=EDGE_CURVE('',#29602,#29320,#16597,.T.);
#35522=EDGE_CURVE('',#29404,#29602,#21646,.T.);
#35523=EDGE_CURVE('',#29321,#29602,#21647,.T.);
#35524=EDGE_CURVE('',#29603,#29321,#16598,.T.);
#35525=EDGE_CURVE('',#29408,#29603,#21648,.T.);
#35526=EDGE_CURVE('',#29322,#29603,#21649,.T.);
#35527=EDGE_CURVE('',#29604,#29322,#16599,.T.);
#35528=EDGE_CURVE('',#29412,#29604,#21650,.T.);
#35529=EDGE_CURVE('',#29323,#29604,#21651,.T.);
#35530=EDGE_CURVE('',#29605,#29323,#16600,.T.);
#35531=EDGE_CURVE('',#29416,#29605,#21652,.T.);
#35532=EDGE_CURVE('',#29324,#29605,#21653,.T.);
#35533=EDGE_CURVE('',#29606,#29324,#16601,.T.);
#35534=EDGE_CURVE('',#29420,#29606,#21654,.T.);
#35535=EDGE_CURVE('',#29325,#29606,#21655,.T.);
#35536=EDGE_CURVE('',#29607,#29325,#16602,.T.);
#35537=EDGE_CURVE('',#29424,#29607,#21656,.T.);
#35538=EDGE_CURVE('',#29326,#29607,#21657,.T.);
#35539=EDGE_CURVE('',#29608,#29326,#16603,.T.);
#35540=EDGE_CURVE('',#29020,#29608,#21658,.T.);
#35541=EDGE_CURVE('',#29327,#29608,#21659,.T.);
#35542=EDGE_CURVE('',#29609,#29327,#16604,.T.);
#35543=EDGE_CURVE('',#29428,#29609,#21660,.T.);
#35544=EDGE_CURVE('',#29328,#29609,#21661,.T.);
#35545=EDGE_CURVE('',#29610,#29328,#16605,.T.);
#35546=EDGE_CURVE('',#29432,#29610,#21662,.T.);
#35547=EDGE_CURVE('',#29329,#29610,#21663,.T.);
#35548=EDGE_CURVE('',#29611,#29329,#16606,.T.);
#35549=EDGE_CURVE('',#29436,#29611,#21664,.T.);
#35550=EDGE_CURVE('',#29330,#29611,#21665,.T.);
#35551=EDGE_CURVE('',#29612,#29330,#16607,.T.);
#35552=EDGE_CURVE('',#29440,#29612,#21666,.T.);
#35553=EDGE_CURVE('',#29331,#29612,#21667,.T.);
#35554=EDGE_CURVE('',#29613,#29331,#16608,.T.);
#35555=EDGE_CURVE('',#29444,#29613,#21668,.T.);
#35556=EDGE_CURVE('',#29332,#29613,#21669,.T.);
#35557=EDGE_CURVE('',#29614,#29332,#16609,.T.);
#35558=EDGE_CURVE('',#29448,#29614,#21670,.T.);
#35559=EDGE_CURVE('',#29333,#29614,#21671,.T.);
#35560=EDGE_CURVE('',#29615,#29333,#16610,.T.);
#35561=EDGE_CURVE('',#29452,#29615,#21672,.T.);
#35562=EDGE_CURVE('',#29334,#29615,#21673,.T.);
#35563=EDGE_CURVE('',#29616,#29334,#16611,.T.);
#35564=EDGE_CURVE('',#29456,#29616,#21674,.T.);
#35565=EDGE_CURVE('',#29335,#29616,#21675,.T.);
#35566=EDGE_CURVE('',#29617,#29335,#16612,.T.);
#35567=EDGE_CURVE('',#29460,#29617,#21676,.T.);
#35568=EDGE_CURVE('',#29336,#29617,#21677,.T.);
#35569=EDGE_CURVE('',#29618,#29336,#16613,.T.);
#35570=EDGE_CURVE('',#29465,#29618,#21678,.T.);
#35571=EDGE_CURVE('',#29337,#29618,#21679,.T.);
#35572=EDGE_CURVE('',#29619,#29337,#16614,.T.);
#35573=EDGE_CURVE('',#29469,#29619,#21680,.T.);
#35574=EDGE_CURVE('',#29338,#29619,#21681,.T.);
#35575=EDGE_CURVE('',#29620,#29338,#16615,.T.);
#35576=EDGE_CURVE('',#29472,#29620,#21682,.T.);
#35577=EDGE_CURVE('',#29339,#29620,#21683,.T.);
#35578=EDGE_CURVE('',#29621,#29339,#16616,.T.);
#35579=EDGE_CURVE('',#29476,#29621,#21684,.T.);
#35580=EDGE_CURVE('',#29340,#29621,#21685,.T.);
#35581=EDGE_CURVE('',#29622,#29340,#16617,.T.);
#35582=EDGE_CURVE('',#29480,#29622,#21686,.T.);
#35583=EDGE_CURVE('',#29312,#29622,#21687,.T.);
#35584=EDGE_CURVE('',#29623,#29341,#16618,.T.);
#35585=EDGE_CURVE('',#29485,#29623,#21688,.T.);
#35586=EDGE_CURVE('',#29342,#29623,#21689,.T.);
#35587=EDGE_CURVE('',#29624,#29342,#16619,.T.);
#35588=EDGE_CURVE('',#29489,#29624,#21690,.T.);
#35589=EDGE_CURVE('',#29343,#29624,#21691,.T.);
#35590=EDGE_CURVE('',#29625,#29343,#16620,.T.);
#35591=EDGE_CURVE('',#29493,#29625,#21692,.T.);
#35592=EDGE_CURVE('',#29344,#29625,#21693,.T.);
#35593=EDGE_CURVE('',#29626,#29344,#16621,.T.);
#35594=EDGE_CURVE('',#29497,#29626,#21694,.T.);
#35595=EDGE_CURVE('',#29345,#29626,#21695,.T.);
#35596=EDGE_CURVE('',#29627,#29345,#16622,.T.);
#35597=EDGE_CURVE('',#29501,#29627,#21696,.T.);
#35598=EDGE_CURVE('',#29346,#29627,#21697,.T.);
#35599=EDGE_CURVE('',#29628,#29346,#16623,.T.);
#35600=EDGE_CURVE('',#29505,#29628,#21698,.T.);
#35601=EDGE_CURVE('',#29347,#29628,#21699,.T.);
#35602=EDGE_CURVE('',#29629,#29347,#16624,.T.);
#35603=EDGE_CURVE('',#29509,#29629,#21700,.T.);
#35604=EDGE_CURVE('',#29348,#29629,#21701,.T.);
#35605=EDGE_CURVE('',#29630,#29348,#16625,.T.);
#35606=EDGE_CURVE('',#29513,#29630,#21702,.T.);
#35607=EDGE_CURVE('',#29349,#29630,#21703,.T.);
#35608=EDGE_CURVE('',#29631,#29349,#16626,.T.);
#35609=EDGE_CURVE('',#29517,#29631,#21704,.T.);
#35610=EDGE_CURVE('',#29350,#29631,#21705,.T.);
#35611=EDGE_CURVE('',#29632,#29350,#16627,.T.);
#35612=EDGE_CURVE('',#29521,#29632,#21706,.T.);
#35613=EDGE_CURVE('',#29351,#29632,#21707,.T.);
#35614=EDGE_CURVE('',#29633,#29351,#16628,.T.);
#35615=EDGE_CURVE('',#29525,#29633,#21708,.T.);
#35616=EDGE_CURVE('',#29352,#29633,#21709,.T.);
#35617=EDGE_CURVE('',#29634,#29352,#16629,.T.);
#35618=EDGE_CURVE('',#29529,#29634,#21710,.T.);
#35619=EDGE_CURVE('',#29353,#29634,#21711,.T.);
#35620=EDGE_CURVE('',#29635,#29353,#16630,.T.);
#35621=EDGE_CURVE('',#29533,#29635,#21712,.T.);
#35622=EDGE_CURVE('',#29354,#29635,#21713,.T.);
#35623=EDGE_CURVE('',#29636,#29354,#16631,.T.);
#35624=EDGE_CURVE('',#29537,#29636,#21714,.T.);
#35625=EDGE_CURVE('',#29355,#29636,#21715,.T.);
#35626=EDGE_CURVE('',#29637,#29355,#16632,.T.);
#35627=EDGE_CURVE('',#29541,#29637,#21716,.T.);
#35628=EDGE_CURVE('',#29356,#29637,#21717,.T.);
#35629=EDGE_CURVE('',#29638,#29356,#16633,.T.);
#35630=EDGE_CURVE('',#29545,#29638,#21718,.T.);
#35631=EDGE_CURVE('',#29357,#29638,#21719,.T.);
#35632=EDGE_CURVE('',#29639,#29357,#16634,.T.);
#35633=EDGE_CURVE('',#29549,#29639,#21720,.T.);
#35634=EDGE_CURVE('',#29358,#29639,#21721,.T.);
#35635=EDGE_CURVE('',#29640,#29358,#16635,.T.);
#35636=EDGE_CURVE('',#29553,#29640,#21722,.T.);
#35637=EDGE_CURVE('',#29359,#29640,#21723,.T.);
#35638=EDGE_CURVE('',#29641,#29359,#16636,.T.);
#35639=EDGE_CURVE('',#29557,#29641,#21724,.T.);
#35640=EDGE_CURVE('',#29360,#29641,#21725,.T.);
#35641=EDGE_CURVE('',#29642,#29360,#16637,.T.);
#35642=EDGE_CURVE('',#29561,#29642,#21726,.T.);
#35643=EDGE_CURVE('',#29361,#29642,#21727,.T.);
#35644=EDGE_CURVE('',#29643,#29361,#16638,.T.);
#35645=EDGE_CURVE('',#29565,#29643,#21728,.T.);
#35646=EDGE_CURVE('',#29362,#29643,#21729,.T.);
#35647=EDGE_CURVE('',#29644,#29362,#16639,.T.);
#35648=EDGE_CURVE('',#29014,#29644,#21730,.T.);
#35649=EDGE_CURVE('',#29363,#29644,#21731,.T.);
#35650=EDGE_CURVE('',#29645,#29363,#16640,.T.);
#35651=EDGE_CURVE('',#29569,#29645,#21732,.T.);
#35652=EDGE_CURVE('',#29364,#29645,#21733,.T.);
#35653=EDGE_CURVE('',#29646,#29364,#16641,.T.);
#35654=EDGE_CURVE('',#29573,#29646,#21734,.T.);
#35655=EDGE_CURVE('',#29365,#29646,#21735,.T.);
#35656=EDGE_CURVE('',#29647,#29365,#16642,.T.);
#35657=EDGE_CURVE('',#29577,#29647,#21736,.T.);
#35658=EDGE_CURVE('',#29366,#29647,#21737,.T.);
#35659=EDGE_CURVE('',#29648,#29366,#16643,.T.);
#35660=EDGE_CURVE('',#29581,#29648,#21738,.T.);
#35661=EDGE_CURVE('',#29367,#29648,#21739,.T.);
#35662=EDGE_CURVE('',#29649,#29367,#16644,.T.);
#35663=EDGE_CURVE('',#29585,#29649,#21740,.T.);
#35664=EDGE_CURVE('',#29368,#29649,#21741,.T.);
#35665=EDGE_CURVE('',#29650,#29368,#16645,.T.);
#35666=EDGE_CURVE('',#29589,#29650,#21742,.T.);
#35667=EDGE_CURVE('',#29369,#29650,#21743,.T.);
#35668=EDGE_CURVE('',#29651,#29369,#16646,.T.);
#35669=EDGE_CURVE('',#29593,#29651,#21744,.T.);
#35670=EDGE_CURVE('',#29341,#29651,#21745,.T.);
#35671=EDGE_CURVE('',#29652,#29653,#16647,.T.);
#35672=EDGE_CURVE('',#29594,#29653,#24596,.T.);
#35673=EDGE_CURVE('',#29652,#29312,#21746,.T.);
#35674=EDGE_CURVE('',#29654,#29655,#21747,.T.);
#35675=EDGE_CURVE('',#29313,#29655,#21748,.T.);
#35676=EDGE_CURVE('',#29654,#29594,#24597,.T.);
#35677=EDGE_CURVE('',#29656,#29654,#16648,.T.);
#35678=EDGE_CURVE('',#29657,#29656,#16649,.T.);
#35679=EDGE_CURVE('',#29655,#29657,#16650,.T.);
#35680=EDGE_CURVE('',#29595,#29657,#24598,.T.);
#35681=EDGE_CURVE('',#29658,#29659,#21749,.T.);
#35682=EDGE_CURVE('',#29314,#29659,#21750,.T.);
#35683=EDGE_CURVE('',#29658,#29595,#24599,.T.);
#35684=EDGE_CURVE('',#29660,#29658,#16651,.T.);
#35685=EDGE_CURVE('',#29661,#29660,#16652,.T.);
#35686=EDGE_CURVE('',#29659,#29661,#16653,.T.);
#35687=EDGE_CURVE('',#29596,#29661,#24600,.T.);
#35688=EDGE_CURVE('',#29662,#29663,#21751,.T.);
#35689=EDGE_CURVE('',#29315,#29663,#21752,.T.);
#35690=EDGE_CURVE('',#29662,#29596,#24601,.T.);
#35691=EDGE_CURVE('',#29664,#29662,#16654,.T.);
#35692=EDGE_CURVE('',#29665,#29664,#16655,.T.);
#35693=EDGE_CURVE('',#29663,#29665,#16656,.T.);
#35694=EDGE_CURVE('',#29597,#29665,#24602,.T.);
#35695=EDGE_CURVE('',#29666,#29667,#21753,.T.);
#35696=EDGE_CURVE('',#29316,#29667,#21754,.T.);
#35697=EDGE_CURVE('',#29666,#29597,#24603,.T.);
#35698=EDGE_CURVE('',#29668,#29666,#16657,.T.);
#35699=EDGE_CURVE('',#29669,#29668,#16658,.T.);
#35700=EDGE_CURVE('',#29667,#29669,#16659,.T.);
#35701=EDGE_CURVE('',#29598,#29669,#24604,.T.);
#35702=EDGE_CURVE('',#29670,#29671,#21755,.T.);
#35703=EDGE_CURVE('',#29317,#29671,#21756,.T.);
#35704=EDGE_CURVE('',#29670,#29598,#24605,.T.);
#35705=EDGE_CURVE('',#29672,#29670,#16660,.T.);
#35706=EDGE_CURVE('',#29673,#29672,#16661,.T.);
#35707=EDGE_CURVE('',#29671,#29673,#16662,.T.);
#35708=EDGE_CURVE('',#29599,#29673,#24606,.T.);
#35709=EDGE_CURVE('',#29674,#29675,#21757,.T.);
#35710=EDGE_CURVE('',#29318,#29675,#21758,.T.);
#35711=EDGE_CURVE('',#29674,#29599,#24607,.T.);
#35712=EDGE_CURVE('',#29676,#29674,#16663,.T.);
#35713=EDGE_CURVE('',#29677,#29676,#16664,.T.);
#35714=EDGE_CURVE('',#29675,#29677,#16665,.T.);
#35715=EDGE_CURVE('',#29600,#29677,#24608,.T.);
#35716=EDGE_CURVE('',#29319,#29010,#21759,.T.);
#35717=EDGE_CURVE('',#29012,#29600,#24609,.T.);
#35718=EDGE_CURVE('',#29601,#29011,#24610,.T.);
#35719=EDGE_CURVE('',#29678,#29679,#21760,.T.);
#35720=EDGE_CURVE('',#29320,#29679,#21761,.T.);
#35721=EDGE_CURVE('',#29678,#29601,#24611,.T.);
#35722=EDGE_CURVE('',#29680,#29678,#16666,.T.);
#35723=EDGE_CURVE('',#29681,#29680,#16667,.T.);
#35724=EDGE_CURVE('',#29679,#29681,#16668,.T.);
#35725=EDGE_CURVE('',#29602,#29681,#24612,.T.);
#35726=EDGE_CURVE('',#29682,#29683,#21762,.T.);
#35727=EDGE_CURVE('',#29321,#29683,#21763,.T.);
#35728=EDGE_CURVE('',#29682,#29602,#24613,.T.);
#35729=EDGE_CURVE('',#29684,#29682,#16669,.T.);
#35730=EDGE_CURVE('',#29685,#29684,#16670,.T.);
#35731=EDGE_CURVE('',#29683,#29685,#16671,.T.);
#35732=EDGE_CURVE('',#29603,#29685,#24614,.T.);
#35733=EDGE_CURVE('',#29686,#29687,#21764,.T.);
#35734=EDGE_CURVE('',#29322,#29687,#21765,.T.);
#35735=EDGE_CURVE('',#29686,#29603,#24615,.T.);
#35736=EDGE_CURVE('',#29688,#29686,#16672,.T.);
#35737=EDGE_CURVE('',#29689,#29688,#16673,.T.);
#35738=EDGE_CURVE('',#29687,#29689,#16674,.T.);
#35739=EDGE_CURVE('',#29604,#29689,#24616,.T.);
#35740=EDGE_CURVE('',#29690,#29691,#21766,.T.);
#35741=EDGE_CURVE('',#29323,#29691,#21767,.T.);
#35742=EDGE_CURVE('',#29690,#29604,#24617,.T.);
#35743=EDGE_CURVE('',#29692,#29690,#16675,.T.);
#35744=EDGE_CURVE('',#29693,#29692,#16676,.T.);
#35745=EDGE_CURVE('',#29691,#29693,#16677,.T.);
#35746=EDGE_CURVE('',#29605,#29693,#24618,.T.);
#35747=EDGE_CURVE('',#29694,#29695,#21768,.T.);
#35748=EDGE_CURVE('',#29324,#29695,#21769,.T.);
#35749=EDGE_CURVE('',#29694,#29605,#24619,.T.);
#35750=EDGE_CURVE('',#29696,#29694,#16678,.T.);
#35751=EDGE_CURVE('',#29697,#29696,#16679,.T.);
#35752=EDGE_CURVE('',#29695,#29697,#16680,.T.);
#35753=EDGE_CURVE('',#29606,#29697,#24620,.T.);
#35754=EDGE_CURVE('',#29698,#29699,#21770,.T.);
#35755=EDGE_CURVE('',#29325,#29699,#21771,.T.);
#35756=EDGE_CURVE('',#29698,#29606,#24621,.T.);
#35757=EDGE_CURVE('',#29700,#29698,#16681,.T.);
#35758=EDGE_CURVE('',#29701,#29700,#16682,.T.);
#35759=EDGE_CURVE('',#29699,#29701,#16683,.T.);
#35760=EDGE_CURVE('',#29607,#29701,#24622,.T.);
#35761=EDGE_CURVE('',#29702,#29703,#21772,.T.);
#35762=EDGE_CURVE('',#29326,#29703,#21773,.T.);
#35763=EDGE_CURVE('',#29702,#29607,#24623,.T.);
#35764=EDGE_CURVE('',#29704,#29702,#16684,.T.);
#35765=EDGE_CURVE('',#29705,#29704,#16685,.T.);
#35766=EDGE_CURVE('',#29703,#29705,#16686,.T.);
#35767=EDGE_CURVE('',#29608,#29705,#24624,.T.);
#35768=EDGE_CURVE('',#29706,#29707,#21774,.T.);
#35769=EDGE_CURVE('',#29327,#29707,#21775,.T.);
#35770=EDGE_CURVE('',#29706,#29608,#24625,.T.);
#35771=EDGE_CURVE('',#29708,#29706,#16687,.T.);
#35772=EDGE_CURVE('',#29709,#29708,#16688,.T.);
#35773=EDGE_CURVE('',#29707,#29709,#16689,.T.);
#35774=EDGE_CURVE('',#29609,#29709,#24626,.T.);
#35775=EDGE_CURVE('',#29710,#29711,#21776,.T.);
#35776=EDGE_CURVE('',#29328,#29711,#21777,.T.);
#35777=EDGE_CURVE('',#29710,#29609,#24627,.T.);
#35778=EDGE_CURVE('',#29712,#29710,#16690,.T.);
#35779=EDGE_CURVE('',#29713,#29712,#16691,.T.);
#35780=EDGE_CURVE('',#29711,#29713,#16692,.T.);
#35781=EDGE_CURVE('',#29610,#29713,#24628,.T.);
#35782=EDGE_CURVE('',#29714,#29715,#21778,.T.);
#35783=EDGE_CURVE('',#29329,#29715,#21779,.T.);
#35784=EDGE_CURVE('',#29714,#29610,#24629,.T.);
#35785=EDGE_CURVE('',#29716,#29714,#16693,.T.);
#35786=EDGE_CURVE('',#29717,#29716,#16694,.T.);
#35787=EDGE_CURVE('',#29715,#29717,#16695,.T.);
#35788=EDGE_CURVE('',#29611,#29717,#24630,.T.);
#35789=EDGE_CURVE('',#29718,#29719,#21780,.T.);
#35790=EDGE_CURVE('',#29330,#29719,#21781,.T.);
#35791=EDGE_CURVE('',#29718,#29611,#24631,.T.);
#35792=EDGE_CURVE('',#29720,#29718,#16696,.T.);
#35793=EDGE_CURVE('',#29721,#29720,#16697,.T.);
#35794=EDGE_CURVE('',#29719,#29721,#16698,.T.);
#35795=EDGE_CURVE('',#29612,#29721,#24632,.T.);
#35796=EDGE_CURVE('',#29722,#29723,#21782,.T.);
#35797=EDGE_CURVE('',#29331,#29723,#21783,.T.);
#35798=EDGE_CURVE('',#29722,#29612,#24633,.T.);
#35799=EDGE_CURVE('',#29724,#29722,#16699,.T.);
#35800=EDGE_CURVE('',#29725,#29724,#16700,.T.);
#35801=EDGE_CURVE('',#29723,#29725,#16701,.T.);
#35802=EDGE_CURVE('',#29613,#29725,#24634,.T.);
#35803=EDGE_CURVE('',#29726,#29727,#21784,.T.);
#35804=EDGE_CURVE('',#29332,#29727,#21785,.T.);
#35805=EDGE_CURVE('',#29726,#29613,#24635,.T.);
#35806=EDGE_CURVE('',#29728,#29726,#16702,.T.);
#35807=EDGE_CURVE('',#29729,#29728,#16703,.T.);
#35808=EDGE_CURVE('',#29727,#29729,#16704,.T.);
#35809=EDGE_CURVE('',#29614,#29729,#24636,.T.);
#35810=EDGE_CURVE('',#29730,#29731,#21786,.T.);
#35811=EDGE_CURVE('',#29333,#29731,#21787,.T.);
#35812=EDGE_CURVE('',#29730,#29614,#24637,.T.);
#35813=EDGE_CURVE('',#29732,#29730,#16705,.T.);
#35814=EDGE_CURVE('',#29733,#29732,#16706,.T.);
#35815=EDGE_CURVE('',#29731,#29733,#16707,.T.);
#35816=EDGE_CURVE('',#29615,#29733,#24638,.T.);
#35817=EDGE_CURVE('',#29734,#29735,#21788,.T.);
#35818=EDGE_CURVE('',#29334,#29735,#21789,.T.);
#35819=EDGE_CURVE('',#29734,#29615,#24639,.T.);
#35820=EDGE_CURVE('',#29736,#29734,#16708,.T.);
#35821=EDGE_CURVE('',#29737,#29736,#16709,.T.);
#35822=EDGE_CURVE('',#29735,#29737,#16710,.T.);
#35823=EDGE_CURVE('',#29616,#29737,#24640,.T.);
#35824=EDGE_CURVE('',#29738,#29739,#21790,.T.);
#35825=EDGE_CURVE('',#29335,#29739,#21791,.T.);
#35826=EDGE_CURVE('',#29738,#29616,#24641,.T.);
#35827=EDGE_CURVE('',#29740,#29738,#16711,.T.);
#35828=EDGE_CURVE('',#29741,#29740,#16712,.T.);
#35829=EDGE_CURVE('',#29739,#29741,#16713,.T.);
#35830=EDGE_CURVE('',#29617,#29741,#24642,.T.);
#35831=EDGE_CURVE('',#29742,#29743,#21792,.T.);
#35832=EDGE_CURVE('',#29336,#29743,#21793,.T.);
#35833=EDGE_CURVE('',#29742,#29617,#24643,.T.);
#35834=EDGE_CURVE('',#29743,#29744,#16714,.T.);
#35835=EDGE_CURVE('',#29618,#29744,#24644,.T.);
#35836=EDGE_CURVE('',#29745,#29742,#16715,.T.);
#35837=EDGE_CURVE('',#29744,#29745,#16716,.T.);
#35838=EDGE_CURVE('',#29746,#29618,#24645,.T.);
#35839=EDGE_CURVE('',#29746,#29747,#21794,.T.);
#35840=EDGE_CURVE('',#29337,#29747,#21795,.T.);
#35841=EDGE_CURVE('',#29747,#29748,#16717,.T.);
#35842=EDGE_CURVE('',#29749,#29746,#16718,.T.);
#35843=EDGE_CURVE('',#29748,#29749,#16719,.T.);
#35844=EDGE_CURVE('',#29619,#29748,#24646,.T.);
#35845=EDGE_CURVE('',#29750,#29751,#21796,.T.);
#35846=EDGE_CURVE('',#29338,#29751,#21797,.T.);
#35847=EDGE_CURVE('',#29750,#29619,#24647,.T.);
#35848=EDGE_CURVE('',#29752,#29750,#16720,.T.);
#35849=EDGE_CURVE('',#29753,#29752,#16721,.T.);
#35850=EDGE_CURVE('',#29751,#29753,#16722,.T.);
#35851=EDGE_CURVE('',#29620,#29753,#24648,.T.);
#35852=EDGE_CURVE('',#29754,#29755,#21798,.T.);
#35853=EDGE_CURVE('',#29339,#29755,#21799,.T.);
#35854=EDGE_CURVE('',#29754,#29620,#24649,.T.);
#35855=EDGE_CURVE('',#29756,#29754,#16723,.T.);
#35856=EDGE_CURVE('',#29757,#29756,#16724,.T.);
#35857=EDGE_CURVE('',#29755,#29757,#16725,.T.);
#35858=EDGE_CURVE('',#29621,#29757,#24650,.T.);
#35859=EDGE_CURVE('',#29758,#29759,#21800,.T.);
#35860=EDGE_CURVE('',#29340,#29759,#21801,.T.);
#35861=EDGE_CURVE('',#29758,#29621,#24651,.T.);
#35862=EDGE_CURVE('',#29760,#29758,#16726,.T.);
#35863=EDGE_CURVE('',#29761,#29760,#16727,.T.);
#35864=EDGE_CURVE('',#29759,#29761,#16728,.T.);
#35865=EDGE_CURVE('',#29622,#29761,#24652,.T.);
#35866=EDGE_CURVE('',#29762,#29763,#16729,.T.);
#35867=EDGE_CURVE('',#29653,#29762,#16730,.T.);
#35868=EDGE_CURVE('',#29763,#29652,#21802,.T.);
#35869=EDGE_CURVE('',#29763,#29622,#24653,.T.);
#35870=EDGE_CURVE('',#29764,#29341,#21803,.T.);
#35871=EDGE_CURVE('',#29764,#29765,#16731,.T.);
#35872=EDGE_CURVE('',#29623,#29765,#24654,.T.);
#35873=EDGE_CURVE('',#29766,#29623,#24655,.T.);
#35874=EDGE_CURVE('',#29766,#29767,#21804,.T.);
#35875=EDGE_CURVE('',#29342,#29767,#21805,.T.);
#35876=EDGE_CURVE('',#29767,#29768,#16732,.T.);
#35877=EDGE_CURVE('',#29624,#29768,#24656,.T.);
#35878=EDGE_CURVE('',#29769,#29766,#16733,.T.);
#35879=EDGE_CURVE('',#29768,#29769,#16734,.T.);
#35880=EDGE_CURVE('',#29770,#29624,#24657,.T.);
#35881=EDGE_CURVE('',#29770,#29771,#21806,.T.);
#35882=EDGE_CURVE('',#29343,#29771,#21807,.T.);
#35883=EDGE_CURVE('',#29771,#29772,#16735,.T.);
#35884=EDGE_CURVE('',#29625,#29772,#24658,.T.);
#35885=EDGE_CURVE('',#29773,#29770,#16736,.T.);
#35886=EDGE_CURVE('',#29772,#29773,#16737,.T.);
#35887=EDGE_CURVE('',#29774,#29625,#24659,.T.);
#35888=EDGE_CURVE('',#29774,#29775,#21808,.T.);
#35889=EDGE_CURVE('',#29344,#29775,#21809,.T.);
#35890=EDGE_CURVE('',#29775,#29776,#16738,.T.);
#35891=EDGE_CURVE('',#29626,#29776,#24660,.T.);
#35892=EDGE_CURVE('',#29777,#29774,#16739,.T.);
#35893=EDGE_CURVE('',#29776,#29777,#16740,.T.);
#35894=EDGE_CURVE('',#29778,#29626,#24661,.T.);
#35895=EDGE_CURVE('',#29778,#29779,#21810,.T.);
#35896=EDGE_CURVE('',#29345,#29779,#21811,.T.);
#35897=EDGE_CURVE('',#29779,#29780,#16741,.T.);
#35898=EDGE_CURVE('',#29627,#29780,#24662,.T.);
#35899=EDGE_CURVE('',#29781,#29778,#16742,.T.);
#35900=EDGE_CURVE('',#29780,#29781,#16743,.T.);
#35901=EDGE_CURVE('',#29782,#29627,#24663,.T.);
#35902=EDGE_CURVE('',#29782,#29783,#21812,.T.);
#35903=EDGE_CURVE('',#29346,#29783,#21813,.T.);
#35904=EDGE_CURVE('',#29783,#29784,#16744,.T.);
#35905=EDGE_CURVE('',#29628,#29784,#24664,.T.);
#35906=EDGE_CURVE('',#29785,#29782,#16745,.T.);
#35907=EDGE_CURVE('',#29784,#29785,#16746,.T.);
#35908=EDGE_CURVE('',#29786,#29628,#24665,.T.);
#35909=EDGE_CURVE('',#29786,#29787,#21814,.T.);
#35910=EDGE_CURVE('',#29347,#29787,#21815,.T.);
#35911=EDGE_CURVE('',#29787,#29788,#16747,.T.);
#35912=EDGE_CURVE('',#29629,#29788,#24666,.T.);
#35913=EDGE_CURVE('',#29789,#29786,#16748,.T.);
#35914=EDGE_CURVE('',#29788,#29789,#16749,.T.);
#35915=EDGE_CURVE('',#29790,#29629,#24667,.T.);
#35916=EDGE_CURVE('',#29790,#29791,#21816,.T.);
#35917=EDGE_CURVE('',#29348,#29791,#21817,.T.);
#35918=EDGE_CURVE('',#29791,#29792,#16750,.T.);
#35919=EDGE_CURVE('',#29630,#29792,#24668,.T.);
#35920=EDGE_CURVE('',#29793,#29790,#16751,.T.);
#35921=EDGE_CURVE('',#29792,#29793,#16752,.T.);
#35922=EDGE_CURVE('',#29794,#29630,#24669,.T.);
#35923=EDGE_CURVE('',#29794,#29795,#21818,.T.);
#35924=EDGE_CURVE('',#29349,#29795,#21819,.T.);
#35925=EDGE_CURVE('',#29795,#29796,#16753,.T.);
#35926=EDGE_CURVE('',#29631,#29796,#24670,.T.);
#35927=EDGE_CURVE('',#29797,#29794,#16754,.T.);
#35928=EDGE_CURVE('',#29796,#29797,#16755,.T.);
#35929=EDGE_CURVE('',#29798,#29631,#24671,.T.);
#35930=EDGE_CURVE('',#29798,#29799,#21820,.T.);
#35931=EDGE_CURVE('',#29350,#29799,#21821,.T.);
#35932=EDGE_CURVE('',#29799,#29800,#16756,.T.);
#35933=EDGE_CURVE('',#29632,#29800,#24672,.T.);
#35934=EDGE_CURVE('',#29801,#29798,#16757,.T.);
#35935=EDGE_CURVE('',#29800,#29801,#16758,.T.);
#35936=EDGE_CURVE('',#29802,#29632,#24673,.T.);
#35937=EDGE_CURVE('',#29802,#29803,#21822,.T.);
#35938=EDGE_CURVE('',#29351,#29803,#21823,.T.);
#35939=EDGE_CURVE('',#29803,#29804,#16759,.T.);
#35940=EDGE_CURVE('',#29633,#29804,#24674,.T.);
#35941=EDGE_CURVE('',#29805,#29802,#16760,.T.);
#35942=EDGE_CURVE('',#29804,#29805,#16761,.T.);
#35943=EDGE_CURVE('',#29806,#29633,#24675,.T.);
#35944=EDGE_CURVE('',#29806,#29807,#21824,.T.);
#35945=EDGE_CURVE('',#29352,#29807,#21825,.T.);
#35946=EDGE_CURVE('',#29807,#29808,#16762,.T.);
#35947=EDGE_CURVE('',#29634,#29808,#24676,.T.);
#35948=EDGE_CURVE('',#29809,#29806,#16763,.T.);
#35949=EDGE_CURVE('',#29808,#29809,#16764,.T.);
#35950=EDGE_CURVE('',#29810,#29634,#24677,.T.);
#35951=EDGE_CURVE('',#29810,#29811,#21826,.T.);
#35952=EDGE_CURVE('',#29353,#29811,#21827,.T.);
#35953=EDGE_CURVE('',#29811,#29812,#16765,.T.);
#35954=EDGE_CURVE('',#29635,#29812,#24678,.T.);
#35955=EDGE_CURVE('',#29813,#29810,#16766,.T.);
#35956=EDGE_CURVE('',#29812,#29813,#16767,.T.);
#35957=EDGE_CURVE('',#29814,#29635,#24679,.T.);
#35958=EDGE_CURVE('',#29814,#29815,#21828,.T.);
#35959=EDGE_CURVE('',#29354,#29815,#21829,.T.);
#35960=EDGE_CURVE('',#29815,#29816,#16768,.T.);
#35961=EDGE_CURVE('',#29636,#29816,#24680,.T.);
#35962=EDGE_CURVE('',#29817,#29814,#16769,.T.);
#35963=EDGE_CURVE('',#29816,#29817,#16770,.T.);
#35964=EDGE_CURVE('',#29009,#29636,#24681,.T.);
#35965=EDGE_CURVE('',#29355,#29008,#21830,.T.);
#35966=EDGE_CURVE('',#29637,#29006,#24682,.T.);
#35967=EDGE_CURVE('',#29818,#29637,#24683,.T.);
#35968=EDGE_CURVE('',#29818,#29819,#21831,.T.);
#35969=EDGE_CURVE('',#29356,#29819,#21832,.T.);
#35970=EDGE_CURVE('',#29819,#29820,#16771,.T.);
#35971=EDGE_CURVE('',#29638,#29820,#24684,.T.);
#35972=EDGE_CURVE('',#29821,#29818,#16772,.T.);
#35973=EDGE_CURVE('',#29820,#29821,#16773,.T.);
#35974=EDGE_CURVE('',#29822,#29638,#24685,.T.);
#35975=EDGE_CURVE('',#29822,#29823,#21833,.T.);
#35976=EDGE_CURVE('',#29357,#29823,#21834,.T.);
#35977=EDGE_CURVE('',#29823,#29824,#16774,.T.);
#35978=EDGE_CURVE('',#29639,#29824,#24686,.T.);
#35979=EDGE_CURVE('',#29825,#29822,#16775,.T.);
#35980=EDGE_CURVE('',#29824,#29825,#16776,.T.);
#35981=EDGE_CURVE('',#29826,#29639,#24687,.T.);
#35982=EDGE_CURVE('',#29826,#29827,#21835,.T.);
#35983=EDGE_CURVE('',#29358,#29827,#21836,.T.);
#35984=EDGE_CURVE('',#29827,#29828,#16777,.T.);
#35985=EDGE_CURVE('',#29640,#29828,#24688,.T.);
#35986=EDGE_CURVE('',#29829,#29826,#16778,.T.);
#35987=EDGE_CURVE('',#29828,#29829,#16779,.T.);
#35988=EDGE_CURVE('',#29830,#29640,#24689,.T.);
#35989=EDGE_CURVE('',#29830,#29831,#21837,.T.);
#35990=EDGE_CURVE('',#29359,#29831,#21838,.T.);
#35991=EDGE_CURVE('',#29831,#29832,#16780,.T.);
#35992=EDGE_CURVE('',#29641,#29832,#24690,.T.);
#35993=EDGE_CURVE('',#29833,#29830,#16781,.T.);
#35994=EDGE_CURVE('',#29832,#29833,#16782,.T.);
#35995=EDGE_CURVE('',#29834,#29641,#24691,.T.);
#35996=EDGE_CURVE('',#29834,#29835,#21839,.T.);
#35997=EDGE_CURVE('',#29360,#29835,#21840,.T.);
#35998=EDGE_CURVE('',#29835,#29836,#16783,.T.);
#35999=EDGE_CURVE('',#29642,#29836,#24692,.T.);
#36000=EDGE_CURVE('',#29837,#29834,#16784,.T.);
#36001=EDGE_CURVE('',#29836,#29837,#16785,.T.);
#36002=EDGE_CURVE('',#29838,#29642,#24693,.T.);
#36003=EDGE_CURVE('',#29838,#29839,#21841,.T.);
#36004=EDGE_CURVE('',#29361,#29839,#21842,.T.);
#36005=EDGE_CURVE('',#29839,#29840,#16786,.T.);
#36006=EDGE_CURVE('',#29643,#29840,#24694,.T.);
#36007=EDGE_CURVE('',#29841,#29838,#16787,.T.);
#36008=EDGE_CURVE('',#29840,#29841,#16788,.T.);
#36009=EDGE_CURVE('',#29842,#29643,#24695,.T.);
#36010=EDGE_CURVE('',#29842,#29843,#21843,.T.);
#36011=EDGE_CURVE('',#29362,#29843,#21844,.T.);
#36012=EDGE_CURVE('',#29843,#29844,#16789,.T.);
#36013=EDGE_CURVE('',#29644,#29844,#24696,.T.);
#36014=EDGE_CURVE('',#29845,#29842,#16790,.T.);
#36015=EDGE_CURVE('',#29844,#29845,#16791,.T.);
#36016=EDGE_CURVE('',#29846,#29644,#24697,.T.);
#36017=EDGE_CURVE('',#29846,#29847,#21845,.T.);
#36018=EDGE_CURVE('',#29363,#29847,#21846,.T.);
#36019=EDGE_CURVE('',#29847,#29848,#16792,.T.);
#36020=EDGE_CURVE('',#29645,#29848,#24698,.T.);
#36021=EDGE_CURVE('',#29849,#29846,#16793,.T.);
#36022=EDGE_CURVE('',#29848,#29849,#16794,.T.);
#36023=EDGE_CURVE('',#29850,#29645,#24699,.T.);
#36024=EDGE_CURVE('',#29850,#29851,#21847,.T.);
#36025=EDGE_CURVE('',#29364,#29851,#21848,.T.);
#36026=EDGE_CURVE('',#29851,#29852,#16795,.T.);
#36027=EDGE_CURVE('',#29646,#29852,#24700,.T.);
#36028=EDGE_CURVE('',#29853,#29850,#16796,.T.);
#36029=EDGE_CURVE('',#29852,#29853,#16797,.T.);
#36030=EDGE_CURVE('',#29854,#29646,#24701,.T.);
#36031=EDGE_CURVE('',#29854,#29855,#21849,.T.);
#36032=EDGE_CURVE('',#29365,#29855,#21850,.T.);
#36033=EDGE_CURVE('',#29855,#29856,#16798,.T.);
#36034=EDGE_CURVE('',#29647,#29856,#24702,.T.);
#36035=EDGE_CURVE('',#29857,#29854,#16799,.T.);
#36036=EDGE_CURVE('',#29856,#29857,#16800,.T.);
#36037=EDGE_CURVE('',#29858,#29647,#24703,.T.);
#36038=EDGE_CURVE('',#29858,#29859,#21851,.T.);
#36039=EDGE_CURVE('',#29366,#29859,#21852,.T.);
#36040=EDGE_CURVE('',#29859,#29860,#16801,.T.);
#36041=EDGE_CURVE('',#29648,#29860,#24704,.T.);
#36042=EDGE_CURVE('',#29861,#29858,#16802,.T.);
#36043=EDGE_CURVE('',#29860,#29861,#16803,.T.);
#36044=EDGE_CURVE('',#29862,#29648,#24705,.T.);
#36045=EDGE_CURVE('',#29862,#29863,#21853,.T.);
#36046=EDGE_CURVE('',#29367,#29863,#21854,.T.);
#36047=EDGE_CURVE('',#29863,#29864,#16804,.T.);
#36048=EDGE_CURVE('',#29649,#29864,#24706,.T.);
#36049=EDGE_CURVE('',#29865,#29862,#16805,.T.);
#36050=EDGE_CURVE('',#29864,#29865,#16806,.T.);
#36051=EDGE_CURVE('',#29866,#29649,#24707,.T.);
#36052=EDGE_CURVE('',#29866,#29867,#21855,.T.);
#36053=EDGE_CURVE('',#29368,#29867,#21856,.T.);
#36054=EDGE_CURVE('',#29867,#29868,#16807,.T.);
#36055=EDGE_CURVE('',#29650,#29868,#24708,.T.);
#36056=EDGE_CURVE('',#29869,#29866,#16808,.T.);
#36057=EDGE_CURVE('',#29868,#29869,#16809,.T.);
#36058=EDGE_CURVE('',#29870,#29650,#24709,.T.);
#36059=EDGE_CURVE('',#29870,#29871,#21857,.T.);
#36060=EDGE_CURVE('',#29369,#29871,#21858,.T.);
#36061=EDGE_CURVE('',#29871,#29872,#16810,.T.);
#36062=EDGE_CURVE('',#29651,#29872,#24710,.T.);
#36063=EDGE_CURVE('',#29873,#29870,#16811,.T.);
#36064=EDGE_CURVE('',#29872,#29873,#16812,.T.);
#36065=EDGE_CURVE('',#29874,#29764,#21859,.T.);
#36066=EDGE_CURVE('',#29875,#29874,#16813,.T.);
#36067=EDGE_CURVE('',#29765,#29875,#16814,.T.);
#36068=EDGE_CURVE('',#29874,#29651,#24711,.T.);
#36069=EDGE_CURVE('',#29594,#29876,#16815,.T.);
#36070=EDGE_CURVE('',#29876,#29762,#21860,.T.);
#36071=EDGE_CURVE('',#29877,#29594,#16816,.T.);
#36072=EDGE_CURVE('',#29656,#29877,#21861,.T.);
#36073=EDGE_CURVE('',#29595,#29877,#16817,.T.);
#36074=EDGE_CURVE('',#29878,#29595,#16818,.T.);
#36075=EDGE_CURVE('',#29660,#29878,#21862,.T.);
#36076=EDGE_CURVE('',#29596,#29878,#16819,.T.);
#36077=EDGE_CURVE('',#29879,#29596,#16820,.T.);
#36078=EDGE_CURVE('',#29664,#29879,#21863,.T.);
#36079=EDGE_CURVE('',#29597,#29879,#16821,.T.);
#36080=EDGE_CURVE('',#29880,#29597,#16822,.T.);
#36081=EDGE_CURVE('',#29668,#29880,#21864,.T.);
#36082=EDGE_CURVE('',#29598,#29880,#16823,.T.);
#36083=EDGE_CURVE('',#29881,#29598,#16824,.T.);
#36084=EDGE_CURVE('',#29672,#29881,#21865,.T.);
#36085=EDGE_CURVE('',#29599,#29881,#16825,.T.);
#36086=EDGE_CURVE('',#29882,#29599,#16826,.T.);
#36087=EDGE_CURVE('',#29676,#29882,#21866,.T.);
#36088=EDGE_CURVE('',#29600,#29882,#16827,.T.);
#36089=EDGE_CURVE('',#29883,#29600,#16828,.T.);
#36090=EDGE_CURVE('',#29013,#29883,#21867,.T.);
#36091=EDGE_CURVE('',#29601,#29883,#16829,.T.);
#36092=EDGE_CURVE('',#29884,#29601,#16830,.T.);
#36093=EDGE_CURVE('',#29680,#29884,#21868,.T.);
#36094=EDGE_CURVE('',#29602,#29884,#16831,.T.);
#36095=EDGE_CURVE('',#29885,#29602,#16832,.T.);
#36096=EDGE_CURVE('',#29684,#29885,#21869,.T.);
#36097=EDGE_CURVE('',#29603,#29885,#16833,.T.);
#36098=EDGE_CURVE('',#29886,#29603,#16834,.T.);
#36099=EDGE_CURVE('',#29688,#29886,#21870,.T.);
#36100=EDGE_CURVE('',#29604,#29886,#16835,.T.);
#36101=EDGE_CURVE('',#29887,#29604,#16836,.T.);
#36102=EDGE_CURVE('',#29692,#29887,#21871,.T.);
#36103=EDGE_CURVE('',#29605,#29887,#16837,.T.);
#36104=EDGE_CURVE('',#29888,#29605,#16838,.T.);
#36105=EDGE_CURVE('',#29696,#29888,#21872,.T.);
#36106=EDGE_CURVE('',#29606,#29888,#16839,.T.);
#36107=EDGE_CURVE('',#29889,#29606,#16840,.T.);
#36108=EDGE_CURVE('',#29700,#29889,#21873,.T.);
#36109=EDGE_CURVE('',#29607,#29889,#16841,.T.);
#36110=EDGE_CURVE('',#29890,#29607,#16842,.T.);
#36111=EDGE_CURVE('',#29704,#29890,#21874,.T.);
#36112=EDGE_CURVE('',#29608,#29890,#16843,.T.);
#36113=EDGE_CURVE('',#29891,#29608,#16844,.T.);
#36114=EDGE_CURVE('',#29708,#29891,#21875,.T.);
#36115=EDGE_CURVE('',#29609,#29891,#16845,.T.);
#36116=EDGE_CURVE('',#29892,#29609,#16846,.T.);
#36117=EDGE_CURVE('',#29712,#29892,#21876,.T.);
#36118=EDGE_CURVE('',#29610,#29892,#16847,.T.);
#36119=EDGE_CURVE('',#29893,#29610,#16848,.T.);
#36120=EDGE_CURVE('',#29716,#29893,#21877,.T.);
#36121=EDGE_CURVE('',#29611,#29893,#16849,.T.);
#36122=EDGE_CURVE('',#29894,#29611,#16850,.T.);
#36123=EDGE_CURVE('',#29720,#29894,#21878,.T.);
#36124=EDGE_CURVE('',#29612,#29894,#16851,.T.);
#36125=EDGE_CURVE('',#29895,#29612,#16852,.T.);
#36126=EDGE_CURVE('',#29724,#29895,#21879,.T.);
#36127=EDGE_CURVE('',#29613,#29895,#16853,.T.);
#36128=EDGE_CURVE('',#29896,#29613,#16854,.T.);
#36129=EDGE_CURVE('',#29728,#29896,#21880,.T.);
#36130=EDGE_CURVE('',#29614,#29896,#16855,.T.);
#36131=EDGE_CURVE('',#29897,#29614,#16856,.T.);
#36132=EDGE_CURVE('',#29732,#29897,#21881,.T.);
#36133=EDGE_CURVE('',#29615,#29897,#16857,.T.);
#36134=EDGE_CURVE('',#29898,#29615,#16858,.T.);
#36135=EDGE_CURVE('',#29736,#29898,#21882,.T.);
#36136=EDGE_CURVE('',#29616,#29898,#16859,.T.);
#36137=EDGE_CURVE('',#29899,#29616,#16860,.T.);
#36138=EDGE_CURVE('',#29740,#29899,#21883,.T.);
#36139=EDGE_CURVE('',#29617,#29899,#16861,.T.);
#36140=EDGE_CURVE('',#29900,#29617,#16862,.T.);
#36141=EDGE_CURVE('',#29745,#29900,#21884,.T.);
#36142=EDGE_CURVE('',#29618,#29900,#16863,.T.);
#36143=EDGE_CURVE('',#29901,#29618,#16864,.T.);
#36144=EDGE_CURVE('',#29749,#29901,#21885,.T.);
#36145=EDGE_CURVE('',#29619,#29901,#16865,.T.);
#36146=EDGE_CURVE('',#29902,#29619,#16866,.T.);
#36147=EDGE_CURVE('',#29752,#29902,#21886,.T.);
#36148=EDGE_CURVE('',#29620,#29902,#16867,.T.);
#36149=EDGE_CURVE('',#29903,#29620,#16868,.T.);
#36150=EDGE_CURVE('',#29756,#29903,#21887,.T.);
#36151=EDGE_CURVE('',#29621,#29903,#16869,.T.);
#36152=EDGE_CURVE('',#29904,#29621,#16870,.T.);
#36153=EDGE_CURVE('',#29760,#29904,#21888,.T.);
#36154=EDGE_CURVE('',#29622,#29904,#16871,.T.);
#36155=EDGE_CURVE('',#29876,#29622,#16872,.T.);
#36156=EDGE_CURVE('',#29905,#29875,#21889,.T.);
#36157=EDGE_CURVE('',#29623,#29905,#16873,.T.);
#36158=EDGE_CURVE('',#29906,#29623,#21890,.T.);
#36159=EDGE_CURVE('',#29769,#29906,#21891,.T.);
#36160=EDGE_CURVE('',#29624,#29906,#16874,.T.);
#36161=EDGE_CURVE('',#29907,#29624,#21892,.T.);
#36162=EDGE_CURVE('',#29773,#29907,#21893,.T.);
#36163=EDGE_CURVE('',#29625,#29907,#16875,.T.);
#36164=EDGE_CURVE('',#29908,#29625,#21894,.T.);
#36165=EDGE_CURVE('',#29777,#29908,#21895,.T.);
#36166=EDGE_CURVE('',#29626,#29908,#16876,.T.);
#36167=EDGE_CURVE('',#29909,#29626,#21896,.T.);
#36168=EDGE_CURVE('',#29781,#29909,#21897,.T.);
#36169=EDGE_CURVE('',#29627,#29909,#16877,.T.);
#36170=EDGE_CURVE('',#29910,#29627,#21898,.T.);
#36171=EDGE_CURVE('',#29785,#29910,#21899,.T.);
#36172=EDGE_CURVE('',#29628,#29910,#16878,.T.);
#36173=EDGE_CURVE('',#29911,#29628,#21900,.T.);
#36174=EDGE_CURVE('',#29789,#29911,#21901,.T.);
#36175=EDGE_CURVE('',#29629,#29911,#16879,.T.);
#36176=EDGE_CURVE('',#29912,#29629,#21902,.T.);
#36177=EDGE_CURVE('',#29793,#29912,#21903,.T.);
#36178=EDGE_CURVE('',#29630,#29912,#16880,.T.);
#36179=EDGE_CURVE('',#29913,#29630,#21904,.T.);
#36180=EDGE_CURVE('',#29797,#29913,#21905,.T.);
#36181=EDGE_CURVE('',#29631,#29913,#16881,.T.);
#36182=EDGE_CURVE('',#29914,#29631,#21906,.T.);
#36183=EDGE_CURVE('',#29801,#29914,#21907,.T.);
#36184=EDGE_CURVE('',#29632,#29914,#16882,.T.);
#36185=EDGE_CURVE('',#29915,#29632,#21908,.T.);
#36186=EDGE_CURVE('',#29805,#29915,#21909,.T.);
#36187=EDGE_CURVE('',#29633,#29915,#16883,.T.);
#36188=EDGE_CURVE('',#29916,#29633,#21910,.T.);
#36189=EDGE_CURVE('',#29809,#29916,#21911,.T.);
#36190=EDGE_CURVE('',#29634,#29916,#16884,.T.);
#36191=EDGE_CURVE('',#29917,#29634,#21912,.T.);
#36192=EDGE_CURVE('',#29813,#29917,#21913,.T.);
#36193=EDGE_CURVE('',#29635,#29917,#16885,.T.);
#36194=EDGE_CURVE('',#29918,#29635,#21914,.T.);
#36195=EDGE_CURVE('',#29817,#29918,#21915,.T.);
#36196=EDGE_CURVE('',#29636,#29918,#16886,.T.);
#36197=EDGE_CURVE('',#29919,#29636,#21916,.T.);
#36198=EDGE_CURVE('',#29007,#29919,#21917,.T.);
#36199=EDGE_CURVE('',#29637,#29919,#16887,.T.);
#36200=EDGE_CURVE('',#29920,#29637,#21918,.T.);
#36201=EDGE_CURVE('',#29821,#29920,#21919,.T.);
#36202=EDGE_CURVE('',#29638,#29920,#16888,.T.);
#36203=EDGE_CURVE('',#29921,#29638,#21920,.T.);
#36204=EDGE_CURVE('',#29825,#29921,#21921,.T.);
#36205=EDGE_CURVE('',#29639,#29921,#16889,.T.);
#36206=EDGE_CURVE('',#29922,#29639,#21922,.T.);
#36207=EDGE_CURVE('',#29829,#29922,#21923,.T.);
#36208=EDGE_CURVE('',#29640,#29922,#16890,.T.);
#36209=EDGE_CURVE('',#29923,#29640,#21924,.T.);
#36210=EDGE_CURVE('',#29833,#29923,#21925,.T.);
#36211=EDGE_CURVE('',#29641,#29923,#16891,.T.);
#36212=EDGE_CURVE('',#29924,#29641,#21926,.T.);
#36213=EDGE_CURVE('',#29837,#29924,#21927,.T.);
#36214=EDGE_CURVE('',#29642,#29924,#16892,.T.);
#36215=EDGE_CURVE('',#29925,#29642,#21928,.T.);
#36216=EDGE_CURVE('',#29841,#29925,#21929,.T.);
#36217=EDGE_CURVE('',#29643,#29925,#16893,.T.);
#36218=EDGE_CURVE('',#29926,#29643,#21930,.T.);
#36219=EDGE_CURVE('',#29845,#29926,#21931,.T.);
#36220=EDGE_CURVE('',#29644,#29926,#16894,.T.);
#36221=EDGE_CURVE('',#29927,#29644,#21932,.T.);
#36222=EDGE_CURVE('',#29849,#29927,#21933,.T.);
#36223=EDGE_CURVE('',#29645,#29927,#16895,.T.);
#36224=EDGE_CURVE('',#29928,#29645,#21934,.T.);
#36225=EDGE_CURVE('',#29853,#29928,#21935,.T.);
#36226=EDGE_CURVE('',#29646,#29928,#16896,.T.);
#36227=EDGE_CURVE('',#29929,#29646,#21936,.T.);
#36228=EDGE_CURVE('',#29857,#29929,#21937,.T.);
#36229=EDGE_CURVE('',#29647,#29929,#16897,.T.);
#36230=EDGE_CURVE('',#29930,#29647,#21938,.T.);
#36231=EDGE_CURVE('',#29861,#29930,#21939,.T.);
#36232=EDGE_CURVE('',#29648,#29930,#16898,.T.);
#36233=EDGE_CURVE('',#29931,#29648,#21940,.T.);
#36234=EDGE_CURVE('',#29865,#29931,#21941,.T.);
#36235=EDGE_CURVE('',#29649,#29931,#16899,.T.);
#36236=EDGE_CURVE('',#29932,#29649,#21942,.T.);
#36237=EDGE_CURVE('',#29869,#29932,#21943,.T.);
#36238=EDGE_CURVE('',#29650,#29932,#16900,.T.);
#36239=EDGE_CURVE('',#29933,#29650,#21944,.T.);
#36240=EDGE_CURVE('',#29873,#29933,#21945,.T.);
#36241=EDGE_CURVE('',#29651,#29933,#16901,.T.);
#36242=EDGE_CURVE('',#29905,#29651,#4425,.T.);
#36243=EDGE_CURVE('',#29934,#29935,#16902,.T.);
#36244=EDGE_CURVE('',#29594,#29935,#21946,.T.);
#36245=EDGE_CURVE('',#29934,#29876,#24712,.T.);
#36246=EDGE_CURVE('',#29936,#29934,#16903,.T.);
#36247=EDGE_CURVE('',#29937,#29936,#16904,.T.);
#36248=EDGE_CURVE('',#29935,#29937,#16905,.T.);
#36249=EDGE_CURVE('',#29877,#29937,#24713,.T.);
#36250=EDGE_CURVE('',#29938,#29939,#16906,.T.);
#36251=EDGE_CURVE('',#29595,#29939,#21947,.T.);
#36252=EDGE_CURVE('',#29938,#29877,#24714,.T.);
#36253=EDGE_CURVE('',#29940,#29938,#16907,.T.);
#36254=EDGE_CURVE('',#29941,#29940,#16908,.T.);
#36255=EDGE_CURVE('',#29939,#29941,#16909,.T.);
#36256=EDGE_CURVE('',#29878,#29941,#24715,.T.);
#36257=EDGE_CURVE('',#29942,#29943,#16910,.T.);
#36258=EDGE_CURVE('',#29596,#29943,#21948,.T.);
#36259=EDGE_CURVE('',#29942,#29878,#24716,.T.);
#36260=EDGE_CURVE('',#29944,#29942,#16911,.T.);
#36261=EDGE_CURVE('',#29945,#29944,#16912,.T.);
#36262=EDGE_CURVE('',#29943,#29945,#16913,.T.);
#36263=EDGE_CURVE('',#29879,#29945,#24717,.T.);
#36264=EDGE_CURVE('',#29946,#29947,#16914,.T.);
#36265=EDGE_CURVE('',#29597,#29947,#21949,.T.);
#36266=EDGE_CURVE('',#29946,#29879,#24718,.T.);
#36267=EDGE_CURVE('',#29948,#29946,#16915,.T.);
#36268=EDGE_CURVE('',#29949,#29948,#16916,.T.);
#36269=EDGE_CURVE('',#29947,#29949,#16917,.T.);
#36270=EDGE_CURVE('',#29880,#29949,#24719,.T.);
#36271=EDGE_CURVE('',#29950,#29951,#16918,.T.);
#36272=EDGE_CURVE('',#29598,#29951,#21950,.T.);
#36273=EDGE_CURVE('',#29950,#29880,#24720,.T.);
#36274=EDGE_CURVE('',#29952,#29950,#16919,.T.);
#36275=EDGE_CURVE('',#29953,#29952,#16920,.T.);
#36276=EDGE_CURVE('',#29951,#29953,#16921,.T.);
#36277=EDGE_CURVE('',#29881,#29953,#24721,.T.);
#36278=EDGE_CURVE('',#29954,#29955,#16922,.T.);
#36279=EDGE_CURVE('',#29599,#29955,#21951,.T.);
#36280=EDGE_CURVE('',#29954,#29881,#24722,.T.);
#36281=EDGE_CURVE('',#29956,#29954,#16923,.T.);
#36282=EDGE_CURVE('',#29957,#29956,#16924,.T.);
#36283=EDGE_CURVE('',#29955,#29957,#16925,.T.);
#36284=EDGE_CURVE('',#29882,#29957,#24723,.T.);
#36285=EDGE_CURVE('',#29958,#29959,#16926,.T.);
#36286=EDGE_CURVE('',#29600,#29959,#21952,.T.);
#36287=EDGE_CURVE('',#29958,#29882,#24724,.T.);
#36288=EDGE_CURVE('',#29960,#29958,#16927,.T.);
#36289=EDGE_CURVE('',#29961,#29960,#16928,.T.);
#36290=EDGE_CURVE('',#29959,#29961,#16929,.T.);
#36291=EDGE_CURVE('',#29883,#29961,#24725,.T.);
#36292=EDGE_CURVE('',#29962,#29963,#16930,.T.);
#36293=EDGE_CURVE('',#29601,#29963,#21953,.T.);
#36294=EDGE_CURVE('',#29962,#29883,#24726,.T.);
#36295=EDGE_CURVE('',#29964,#29962,#16931,.T.);
#36296=EDGE_CURVE('',#29965,#29964,#16932,.T.);
#36297=EDGE_CURVE('',#29963,#29965,#16933,.T.);
#36298=EDGE_CURVE('',#29884,#29965,#24727,.T.);
#36299=EDGE_CURVE('',#29966,#29967,#16934,.T.);
#36300=EDGE_CURVE('',#29602,#29967,#21954,.T.);
#36301=EDGE_CURVE('',#29966,#29884,#24728,.T.);
#36302=EDGE_CURVE('',#29968,#29966,#16935,.T.);
#36303=EDGE_CURVE('',#29969,#29968,#16936,.T.);
#36304=EDGE_CURVE('',#29967,#29969,#16937,.T.);
#36305=EDGE_CURVE('',#29885,#29969,#24729,.T.);
#36306=EDGE_CURVE('',#29970,#29971,#16938,.T.);
#36307=EDGE_CURVE('',#29603,#29971,#21955,.T.);
#36308=EDGE_CURVE('',#29970,#29885,#24730,.T.);
#36309=EDGE_CURVE('',#29972,#29970,#16939,.T.);
#36310=EDGE_CURVE('',#29973,#29972,#16940,.T.);
#36311=EDGE_CURVE('',#29971,#29973,#16941,.T.);
#36312=EDGE_CURVE('',#29886,#29973,#24731,.T.);
#36313=EDGE_CURVE('',#29974,#29975,#16942,.T.);
#36314=EDGE_CURVE('',#29604,#29975,#21956,.T.);
#36315=EDGE_CURVE('',#29974,#29886,#24732,.T.);
#36316=EDGE_CURVE('',#29976,#29974,#16943,.T.);
#36317=EDGE_CURVE('',#29977,#29976,#16944,.T.);
#36318=EDGE_CURVE('',#29975,#29977,#16945,.T.);
#36319=EDGE_CURVE('',#29887,#29977,#24733,.T.);
#36320=EDGE_CURVE('',#29978,#29979,#16946,.T.);
#36321=EDGE_CURVE('',#29605,#29979,#21957,.T.);
#36322=EDGE_CURVE('',#29978,#29887,#24734,.T.);
#36323=EDGE_CURVE('',#29980,#29978,#16947,.T.);
#36324=EDGE_CURVE('',#29981,#29980,#16948,.T.);
#36325=EDGE_CURVE('',#29979,#29981,#16949,.T.);
#36326=EDGE_CURVE('',#29888,#29981,#24735,.T.);
#36327=EDGE_CURVE('',#29982,#29983,#16950,.T.);
#36328=EDGE_CURVE('',#29606,#29983,#21958,.T.);
#36329=EDGE_CURVE('',#29982,#29888,#24736,.T.);
#36330=EDGE_CURVE('',#29984,#29982,#16951,.T.);
#36331=EDGE_CURVE('',#29985,#29984,#16952,.T.);
#36332=EDGE_CURVE('',#29983,#29985,#16953,.T.);
#36333=EDGE_CURVE('',#29889,#29985,#24737,.T.);
#36334=EDGE_CURVE('',#29986,#29987,#16954,.T.);
#36335=EDGE_CURVE('',#29607,#29987,#21959,.T.);
#36336=EDGE_CURVE('',#29986,#29889,#24738,.T.);
#36337=EDGE_CURVE('',#29988,#29986,#16955,.T.);
#36338=EDGE_CURVE('',#29989,#29988,#16956,.T.);
#36339=EDGE_CURVE('',#29987,#29989,#16957,.T.);
#36340=EDGE_CURVE('',#29890,#29989,#24739,.T.);
#36341=EDGE_CURVE('',#29608,#29003,#21960,.T.);
#36342=EDGE_CURVE('',#29002,#29890,#24740,.T.);
#36343=EDGE_CURVE('',#29891,#29005,#24741,.T.);
#36344=EDGE_CURVE('',#29990,#29991,#16958,.T.);
#36345=EDGE_CURVE('',#29609,#29991,#21961,.T.);
#36346=EDGE_CURVE('',#29990,#29891,#24742,.T.);
#36347=EDGE_CURVE('',#29992,#29990,#16959,.T.);
#36348=EDGE_CURVE('',#29993,#29992,#16960,.T.);
#36349=EDGE_CURVE('',#29991,#29993,#16961,.T.);
#36350=EDGE_CURVE('',#29892,#29993,#24743,.T.);
#36351=EDGE_CURVE('',#29994,#29995,#16962,.T.);
#36352=EDGE_CURVE('',#29610,#29995,#21962,.T.);
#36353=EDGE_CURVE('',#29994,#29892,#24744,.T.);
#36354=EDGE_CURVE('',#29996,#29994,#16963,.T.);
#36355=EDGE_CURVE('',#29997,#29996,#16964,.T.);
#36356=EDGE_CURVE('',#29995,#29997,#16965,.T.);
#36357=EDGE_CURVE('',#29893,#29997,#24745,.T.);
#36358=EDGE_CURVE('',#29998,#29999,#16966,.T.);
#36359=EDGE_CURVE('',#29611,#29999,#21963,.T.);
#36360=EDGE_CURVE('',#29998,#29893,#24746,.T.);
#36361=EDGE_CURVE('',#30000,#29998,#16967,.T.);
#36362=EDGE_CURVE('',#30001,#30000,#16968,.T.);
#36363=EDGE_CURVE('',#29999,#30001,#16969,.T.);
#36364=EDGE_CURVE('',#29894,#30001,#24747,.T.);
#36365=EDGE_CURVE('',#30002,#30003,#16970,.T.);
#36366=EDGE_CURVE('',#29612,#30003,#21964,.T.);
#36367=EDGE_CURVE('',#30002,#29894,#24748,.T.);
#36368=EDGE_CURVE('',#30004,#30002,#16971,.T.);
#36369=EDGE_CURVE('',#30005,#30004,#16972,.T.);
#36370=EDGE_CURVE('',#30003,#30005,#16973,.T.);
#36371=EDGE_CURVE('',#29895,#30005,#24749,.T.);
#36372=EDGE_CURVE('',#30006,#30007,#16974,.T.);
#36373=EDGE_CURVE('',#29613,#30007,#21965,.T.);
#36374=EDGE_CURVE('',#30006,#29895,#24750,.T.);
#36375=EDGE_CURVE('',#30008,#30006,#16975,.T.);
#36376=EDGE_CURVE('',#30009,#30008,#16976,.T.);
#36377=EDGE_CURVE('',#30007,#30009,#16977,.T.);
#36378=EDGE_CURVE('',#29896,#30009,#24751,.T.);
#36379=EDGE_CURVE('',#30010,#30011,#16978,.T.);
#36380=EDGE_CURVE('',#29614,#30011,#21966,.T.);
#36381=EDGE_CURVE('',#30010,#29896,#24752,.T.);
#36382=EDGE_CURVE('',#30012,#30010,#16979,.T.);
#36383=EDGE_CURVE('',#30013,#30012,#16980,.T.);
#36384=EDGE_CURVE('',#30011,#30013,#16981,.T.);
#36385=EDGE_CURVE('',#29897,#30013,#24753,.T.);
#36386=EDGE_CURVE('',#30014,#30015,#16982,.T.);
#36387=EDGE_CURVE('',#29615,#30015,#21967,.T.);
#36388=EDGE_CURVE('',#30014,#29897,#24754,.T.);
#36389=EDGE_CURVE('',#30016,#30014,#16983,.T.);
#36390=EDGE_CURVE('',#30017,#30016,#16984,.T.);
#36391=EDGE_CURVE('',#30015,#30017,#16985,.T.);
#36392=EDGE_CURVE('',#29898,#30017,#24755,.T.);
#36393=EDGE_CURVE('',#30018,#30019,#16986,.T.);
#36394=EDGE_CURVE('',#29616,#30019,#21968,.T.);
#36395=EDGE_CURVE('',#30018,#29898,#24756,.T.);
#36396=EDGE_CURVE('',#30020,#30018,#16987,.T.);
#36397=EDGE_CURVE('',#30021,#30020,#16988,.T.);
#36398=EDGE_CURVE('',#30019,#30021,#16989,.T.);
#36399=EDGE_CURVE('',#29899,#30021,#24757,.T.);
#36400=EDGE_CURVE('',#30022,#30023,#16990,.T.);
#36401=EDGE_CURVE('',#29617,#30023,#21969,.T.);
#36402=EDGE_CURVE('',#30022,#29899,#24758,.T.);
#36403=EDGE_CURVE('',#30023,#30024,#16991,.T.);
#36404=EDGE_CURVE('',#29900,#30024,#24759,.T.);
#36405=EDGE_CURVE('',#30025,#30022,#16992,.T.);
#36406=EDGE_CURVE('',#30024,#30025,#16993,.T.);
#36407=EDGE_CURVE('',#30026,#29900,#24760,.T.);
#36408=EDGE_CURVE('',#30026,#30027,#16994,.T.);
#36409=EDGE_CURVE('',#29618,#30027,#21970,.T.);
#36410=EDGE_CURVE('',#30027,#30028,#16995,.T.);
#36411=EDGE_CURVE('',#30029,#30026,#16996,.T.);
#36412=EDGE_CURVE('',#30028,#30029,#16997,.T.);
#36413=EDGE_CURVE('',#29901,#30028,#24761,.T.);
#36414=EDGE_CURVE('',#30030,#30031,#16998,.T.);
#36415=EDGE_CURVE('',#29619,#30031,#21971,.T.);
#36416=EDGE_CURVE('',#30030,#29901,#24762,.T.);
#36417=EDGE_CURVE('',#30032,#30030,#16999,.T.);
#36418=EDGE_CURVE('',#30033,#30032,#17000,.T.);
#36419=EDGE_CURVE('',#30031,#30033,#17001,.T.);
#36420=EDGE_CURVE('',#29902,#30033,#24763,.T.);
#36421=EDGE_CURVE('',#30034,#30035,#17002,.T.);
#36422=EDGE_CURVE('',#29620,#30035,#21972,.T.);
#36423=EDGE_CURVE('',#30034,#29902,#24764,.T.);
#36424=EDGE_CURVE('',#30036,#30034,#17003,.T.);
#36425=EDGE_CURVE('',#30037,#30036,#17004,.T.);
#36426=EDGE_CURVE('',#30035,#30037,#17005,.T.);
#36427=EDGE_CURVE('',#29903,#30037,#24765,.T.);
#36428=EDGE_CURVE('',#30038,#30039,#17006,.T.);
#36429=EDGE_CURVE('',#29621,#30039,#21973,.T.);
#36430=EDGE_CURVE('',#30038,#29903,#24766,.T.);
#36431=EDGE_CURVE('',#30040,#30038,#17007,.T.);
#36432=EDGE_CURVE('',#30041,#30040,#17008,.T.);
#36433=EDGE_CURVE('',#30039,#30041,#17009,.T.);
#36434=EDGE_CURVE('',#29904,#30041,#24767,.T.);
#36435=EDGE_CURVE('',#30042,#30043,#17010,.T.);
#36436=EDGE_CURVE('',#29622,#30043,#21974,.T.);
#36437=EDGE_CURVE('',#30042,#29904,#24768,.T.);
#36438=EDGE_CURVE('',#30044,#30042,#17011,.T.);
#36439=EDGE_CURVE('',#30045,#30044,#17012,.T.);
#36440=EDGE_CURVE('',#30043,#30045,#17013,.T.);
#36441=EDGE_CURVE('',#29876,#30045,#24769,.T.);
#36442=EDGE_CURVE('',#30046,#29905,#24770,.T.);
#36443=EDGE_CURVE('',#30046,#30047,#17014,.T.);
#36444=EDGE_CURVE('',#29623,#30047,#21975,.T.);
#36445=EDGE_CURVE('',#30047,#30048,#21976,.T.);
#36446=EDGE_CURVE('',#29906,#30048,#24771,.T.);
#36447=EDGE_CURVE('',#30049,#30046,#17015,.T.);
#36448=EDGE_CURVE('',#30048,#30049,#17016,.T.);
#36449=EDGE_CURVE('',#30050,#29906,#24772,.T.);
#36450=EDGE_CURVE('',#30050,#30051,#17017,.T.);
#36451=EDGE_CURVE('',#29624,#30051,#21977,.T.);
#36452=EDGE_CURVE('',#30051,#30052,#21978,.T.);
#36453=EDGE_CURVE('',#29907,#30052,#24773,.T.);
#36454=EDGE_CURVE('',#30053,#30050,#17018,.T.);
#36455=EDGE_CURVE('',#30052,#30053,#17019,.T.);
#36456=EDGE_CURVE('',#30054,#29907,#24774,.T.);
#36457=EDGE_CURVE('',#30054,#30055,#17020,.T.);
#36458=EDGE_CURVE('',#29625,#30055,#21979,.T.);
#36459=EDGE_CURVE('',#30055,#30056,#21980,.T.);
#36460=EDGE_CURVE('',#29908,#30056,#24775,.T.);
#36461=EDGE_CURVE('',#30057,#30054,#17021,.T.);
#36462=EDGE_CURVE('',#30056,#30057,#17022,.T.);
#36463=EDGE_CURVE('',#30058,#29908,#24776,.T.);
#36464=EDGE_CURVE('',#30058,#30059,#17023,.T.);
#36465=EDGE_CURVE('',#29626,#30059,#21981,.T.);
#36466=EDGE_CURVE('',#30059,#30060,#21982,.T.);
#36467=EDGE_CURVE('',#29909,#30060,#24777,.T.);
#36468=EDGE_CURVE('',#30061,#30058,#17024,.T.);
#36469=EDGE_CURVE('',#30060,#30061,#17025,.T.);
#36470=EDGE_CURVE('',#30062,#29909,#24778,.T.);
#36471=EDGE_CURVE('',#30062,#30063,#17026,.T.);
#36472=EDGE_CURVE('',#29627,#30063,#21983,.T.);
#36473=EDGE_CURVE('',#30063,#30064,#21984,.T.);
#36474=EDGE_CURVE('',#29910,#30064,#24779,.T.);
#36475=EDGE_CURVE('',#30065,#30062,#17027,.T.);
#36476=EDGE_CURVE('',#30064,#30065,#17028,.T.);
#36477=EDGE_CURVE('',#30066,#29910,#24780,.T.);
#36478=EDGE_CURVE('',#30066,#30067,#17029,.T.);
#36479=EDGE_CURVE('',#29628,#30067,#21985,.T.);
#36480=EDGE_CURVE('',#30067,#30068,#21986,.T.);
#36481=EDGE_CURVE('',#29911,#30068,#24781,.T.);
#36482=EDGE_CURVE('',#30069,#30066,#17030,.T.);
#36483=EDGE_CURVE('',#30068,#30069,#17031,.T.);
#36484=EDGE_CURVE('',#30070,#29911,#24782,.T.);
#36485=EDGE_CURVE('',#30070,#30071,#17032,.T.);
#36486=EDGE_CURVE('',#29629,#30071,#21987,.T.);
#36487=EDGE_CURVE('',#30071,#30072,#21988,.T.);
#36488=EDGE_CURVE('',#29912,#30072,#24783,.T.);
#36489=EDGE_CURVE('',#30073,#30070,#17033,.T.);
#36490=EDGE_CURVE('',#30072,#30073,#17034,.T.);
#36491=EDGE_CURVE('',#30074,#29912,#24784,.T.);
#36492=EDGE_CURVE('',#30074,#30075,#17035,.T.);
#36493=EDGE_CURVE('',#29630,#30075,#21989,.T.);
#36494=EDGE_CURVE('',#30075,#30076,#21990,.T.);
#36495=EDGE_CURVE('',#29913,#30076,#24785,.T.);
#36496=EDGE_CURVE('',#30077,#30074,#17036,.T.);
#36497=EDGE_CURVE('',#30076,#30077,#17037,.T.);
#36498=EDGE_CURVE('',#30078,#29913,#24786,.T.);
#36499=EDGE_CURVE('',#30078,#30079,#17038,.T.);
#36500=EDGE_CURVE('',#29631,#30079,#21991,.T.);
#36501=EDGE_CURVE('',#30079,#30080,#21992,.T.);
#36502=EDGE_CURVE('',#29914,#30080,#24787,.T.);
#36503=EDGE_CURVE('',#30081,#30078,#17039,.T.);
#36504=EDGE_CURVE('',#30080,#30081,#17040,.T.);
#36505=EDGE_CURVE('',#30082,#29914,#24788,.T.);
#36506=EDGE_CURVE('',#30082,#30083,#17041,.T.);
#36507=EDGE_CURVE('',#29632,#30083,#21993,.T.);
#36508=EDGE_CURVE('',#30083,#30084,#21994,.T.);
#36509=EDGE_CURVE('',#29915,#30084,#24789,.T.);
#36510=EDGE_CURVE('',#30085,#30082,#17042,.T.);
#36511=EDGE_CURVE('',#30084,#30085,#17043,.T.);
#36512=EDGE_CURVE('',#30086,#29915,#24790,.T.);
#36513=EDGE_CURVE('',#30086,#30087,#17044,.T.);
#36514=EDGE_CURVE('',#29633,#30087,#21995,.T.);
#36515=EDGE_CURVE('',#30087,#30088,#21996,.T.);
#36516=EDGE_CURVE('',#29916,#30088,#24791,.T.);
#36517=EDGE_CURVE('',#30089,#30086,#17045,.T.);
#36518=EDGE_CURVE('',#30088,#30089,#17046,.T.);
#36519=EDGE_CURVE('',#30090,#29916,#24792,.T.);
#36520=EDGE_CURVE('',#30090,#30091,#17047,.T.);
#36521=EDGE_CURVE('',#29634,#30091,#21997,.T.);
#36522=EDGE_CURVE('',#30091,#30092,#21998,.T.);
#36523=EDGE_CURVE('',#29917,#30092,#24793,.T.);
#36524=EDGE_CURVE('',#30093,#30090,#17048,.T.);
#36525=EDGE_CURVE('',#30092,#30093,#17049,.T.);
#36526=EDGE_CURVE('',#30094,#29917,#24794,.T.);
#36527=EDGE_CURVE('',#30094,#30095,#17050,.T.);
#36528=EDGE_CURVE('',#29635,#30095,#21999,.T.);
#36529=EDGE_CURVE('',#30095,#30096,#22000,.T.);
#36530=EDGE_CURVE('',#29918,#30096,#24795,.T.);
#36531=EDGE_CURVE('',#30097,#30094,#17051,.T.);
#36532=EDGE_CURVE('',#30096,#30097,#17052,.T.);
#36533=EDGE_CURVE('',#30098,#29918,#24796,.T.);
#36534=EDGE_CURVE('',#30098,#30099,#17053,.T.);
#36535=EDGE_CURVE('',#29636,#30099,#22001,.T.);
#36536=EDGE_CURVE('',#30099,#30100,#22002,.T.);
#36537=EDGE_CURVE('',#29919,#30100,#24797,.T.);
#36538=EDGE_CURVE('',#30101,#30098,#17054,.T.);
#36539=EDGE_CURVE('',#30100,#30101,#17055,.T.);
#36540=EDGE_CURVE('',#30102,#29919,#24798,.T.);
#36541=EDGE_CURVE('',#30102,#30103,#17056,.T.);
#36542=EDGE_CURVE('',#29637,#30103,#22003,.T.);
#36543=EDGE_CURVE('',#30103,#30104,#22004,.T.);
#36544=EDGE_CURVE('',#29920,#30104,#24799,.T.);
#36545=EDGE_CURVE('',#30105,#30102,#17057,.T.);
#36546=EDGE_CURVE('',#30104,#30105,#17058,.T.);
#36547=EDGE_CURVE('',#30106,#29920,#24800,.T.);
#36548=EDGE_CURVE('',#30106,#30107,#17059,.T.);
#36549=EDGE_CURVE('',#29638,#30107,#22005,.T.);
#36550=EDGE_CURVE('',#30107,#30108,#22006,.T.);
#36551=EDGE_CURVE('',#29921,#30108,#24801,.T.);
#36552=EDGE_CURVE('',#30109,#30106,#17060,.T.);
#36553=EDGE_CURVE('',#30108,#30109,#17061,.T.);
#36554=EDGE_CURVE('',#30110,#29921,#24802,.T.);
#36555=EDGE_CURVE('',#30110,#30111,#17062,.T.);
#36556=EDGE_CURVE('',#29639,#30111,#22007,.T.);
#36557=EDGE_CURVE('',#30111,#30112,#22008,.T.);
#36558=EDGE_CURVE('',#29922,#30112,#24803,.T.);
#36559=EDGE_CURVE('',#30113,#30110,#17063,.T.);
#36560=EDGE_CURVE('',#30112,#30113,#17064,.T.);
#36561=EDGE_CURVE('',#30114,#29922,#24804,.T.);
#36562=EDGE_CURVE('',#30114,#30115,#17065,.T.);
#36563=EDGE_CURVE('',#29640,#30115,#22009,.T.);
#36564=EDGE_CURVE('',#30115,#30116,#22010,.T.);
#36565=EDGE_CURVE('',#29923,#30116,#24805,.T.);
#36566=EDGE_CURVE('',#30117,#30114,#17066,.T.);
#36567=EDGE_CURVE('',#30116,#30117,#17067,.T.);
#36568=EDGE_CURVE('',#30118,#29923,#24806,.T.);
#36569=EDGE_CURVE('',#30118,#30119,#17068,.T.);
#36570=EDGE_CURVE('',#29641,#30119,#22011,.T.);
#36571=EDGE_CURVE('',#30119,#30120,#22012,.T.);
#36572=EDGE_CURVE('',#29924,#30120,#24807,.T.);
#36573=EDGE_CURVE('',#30121,#30118,#17069,.T.);
#36574=EDGE_CURVE('',#30120,#30121,#17070,.T.);
#36575=EDGE_CURVE('',#30122,#29924,#24808,.T.);
#36576=EDGE_CURVE('',#30122,#30123,#17071,.T.);
#36577=EDGE_CURVE('',#29642,#30123,#22013,.T.);
#36578=EDGE_CURVE('',#30123,#30124,#22014,.T.);
#36579=EDGE_CURVE('',#29925,#30124,#24809,.T.);
#36580=EDGE_CURVE('',#30125,#30122,#17072,.T.);
#36581=EDGE_CURVE('',#30124,#30125,#17073,.T.);
#36582=EDGE_CURVE('',#30126,#29925,#24810,.T.);
#36583=EDGE_CURVE('',#30126,#30127,#17074,.T.);
#36584=EDGE_CURVE('',#29643,#30127,#22015,.T.);
#36585=EDGE_CURVE('',#30127,#30128,#22016,.T.);
#36586=EDGE_CURVE('',#29926,#30128,#24811,.T.);
#36587=EDGE_CURVE('',#30129,#30126,#17075,.T.);
#36588=EDGE_CURVE('',#30128,#30129,#17076,.T.);
#36589=EDGE_CURVE('',#30130,#29926,#24812,.T.);
#36590=EDGE_CURVE('',#30130,#30131,#17077,.T.);
#36591=EDGE_CURVE('',#29644,#30131,#22017,.T.);
#36592=EDGE_CURVE('',#30131,#30132,#22018,.T.);
#36593=EDGE_CURVE('',#29927,#30132,#24813,.T.);
#36594=EDGE_CURVE('',#30133,#30130,#17078,.T.);
#36595=EDGE_CURVE('',#30132,#30133,#17079,.T.);
#36596=EDGE_CURVE('',#30134,#29927,#24814,.T.);
#36597=EDGE_CURVE('',#30134,#30135,#17080,.T.);
#36598=EDGE_CURVE('',#29645,#30135,#22019,.T.);
#36599=EDGE_CURVE('',#30135,#30136,#22020,.T.);
#36600=EDGE_CURVE('',#29928,#30136,#24815,.T.);
#36601=EDGE_CURVE('',#30137,#30134,#17081,.T.);
#36602=EDGE_CURVE('',#30136,#30137,#17082,.T.);
#36603=EDGE_CURVE('',#30138,#29928,#24816,.T.);
#36604=EDGE_CURVE('',#30138,#30139,#17083,.T.);
#36605=EDGE_CURVE('',#29646,#30139,#22021,.T.);
#36606=EDGE_CURVE('',#30139,#30140,#22022,.T.);
#36607=EDGE_CURVE('',#29929,#30140,#24817,.T.);
#36608=EDGE_CURVE('',#30141,#30138,#17084,.T.);
#36609=EDGE_CURVE('',#30140,#30141,#17085,.T.);
#36610=EDGE_CURVE('',#30142,#29929,#24818,.T.);
#36611=EDGE_CURVE('',#30142,#30143,#17086,.T.);
#36612=EDGE_CURVE('',#29647,#30143,#22023,.T.);
#36613=EDGE_CURVE('',#30143,#30144,#22024,.T.);
#36614=EDGE_CURVE('',#29930,#30144,#24819,.T.);
#36615=EDGE_CURVE('',#30145,#30142,#17087,.T.);
#36616=EDGE_CURVE('',#30144,#30145,#17088,.T.);
#36617=EDGE_CURVE('',#30146,#29930,#24820,.T.);
#36618=EDGE_CURVE('',#30146,#30147,#17089,.T.);
#36619=EDGE_CURVE('',#29648,#30147,#22025,.T.);
#36620=EDGE_CURVE('',#30147,#30148,#22026,.T.);
#36621=EDGE_CURVE('',#29931,#30148,#24821,.T.);
#36622=EDGE_CURVE('',#30149,#30146,#17090,.T.);
#36623=EDGE_CURVE('',#30148,#30149,#17091,.T.);
#36624=EDGE_CURVE('',#30150,#29931,#24822,.T.);
#36625=EDGE_CURVE('',#30150,#30151,#17092,.T.);
#36626=EDGE_CURVE('',#29649,#30151,#22027,.T.);
#36627=EDGE_CURVE('',#30151,#30152,#22028,.T.);
#36628=EDGE_CURVE('',#29932,#30152,#24823,.T.);
#36629=EDGE_CURVE('',#30153,#30150,#17093,.T.);
#36630=EDGE_CURVE('',#30152,#30153,#17094,.T.);
#36631=EDGE_CURVE('',#30154,#29932,#24824,.T.);
#36632=EDGE_CURVE('',#30154,#30155,#17095,.T.);
#36633=EDGE_CURVE('',#29650,#30155,#22029,.T.);
#36634=EDGE_CURVE('',#30155,#30156,#22030,.T.);
#36635=EDGE_CURVE('',#29933,#30156,#24825,.T.);
#36636=EDGE_CURVE('',#30157,#30154,#17096,.T.);
#36637=EDGE_CURVE('',#30156,#30157,#17097,.T.);
#36638=EDGE_CURVE('',#30158,#29933,#24826,.T.);
#36639=EDGE_CURVE('',#30158,#30159,#17098,.T.);
#36640=EDGE_CURVE('',#29651,#30159,#22031,.T.);
#36641=EDGE_CURVE('',#30159,#30160,#22032,.T.);
#36642=EDGE_CURVE('',#29905,#30160,#24827,.T.);
#36643=EDGE_CURVE('',#30161,#30158,#17099,.T.);
#36644=EDGE_CURVE('',#30160,#30161,#17100,.T.);
#36645=EDGE_CURVE('',#30162,#29876,#17101,.T.);
#36646=EDGE_CURVE('',#29936,#30162,#22033,.T.);
#36647=EDGE_CURVE('',#29877,#30162,#17102,.T.);
#36648=EDGE_CURVE('',#30163,#29877,#17103,.T.);
#36649=EDGE_CURVE('',#29940,#30163,#22034,.T.);
#36650=EDGE_CURVE('',#29878,#30163,#17104,.T.);
#36651=EDGE_CURVE('',#30164,#29878,#17105,.T.);
#36652=EDGE_CURVE('',#29944,#30164,#22035,.T.);
#36653=EDGE_CURVE('',#29879,#30164,#17106,.T.);
#36654=EDGE_CURVE('',#30165,#29879,#17107,.T.);
#36655=EDGE_CURVE('',#29948,#30165,#22036,.T.);
#36656=EDGE_CURVE('',#29880,#30165,#17108,.T.);
#36657=EDGE_CURVE('',#30166,#29880,#17109,.T.);
#36658=EDGE_CURVE('',#29952,#30166,#22037,.T.);
#36659=EDGE_CURVE('',#29881,#30166,#17110,.T.);
#36660=EDGE_CURVE('',#30167,#29881,#17111,.T.);
#36661=EDGE_CURVE('',#29956,#30167,#22038,.T.);
#36662=EDGE_CURVE('',#29882,#30167,#17112,.T.);
#36663=EDGE_CURVE('',#30168,#29882,#17113,.T.);
#36664=EDGE_CURVE('',#29960,#30168,#22039,.T.);
#36665=EDGE_CURVE('',#29883,#30168,#17114,.T.);
#36666=EDGE_CURVE('',#30169,#29883,#17115,.T.);
#36667=EDGE_CURVE('',#29964,#30169,#22040,.T.);
#36668=EDGE_CURVE('',#29884,#30169,#17116,.T.);
#36669=EDGE_CURVE('',#30170,#29884,#17117,.T.);
#36670=EDGE_CURVE('',#29968,#30170,#22041,.T.);
#36671=EDGE_CURVE('',#29885,#30170,#17118,.T.);
#36672=EDGE_CURVE('',#30171,#29885,#17119,.T.);
#36673=EDGE_CURVE('',#29972,#30171,#22042,.T.);
#36674=EDGE_CURVE('',#29886,#30171,#17120,.T.);
#36675=EDGE_CURVE('',#30172,#29886,#17121,.T.);
#36676=EDGE_CURVE('',#29976,#30172,#22043,.T.);
#36677=EDGE_CURVE('',#29887,#30172,#17122,.T.);
#36678=EDGE_CURVE('',#30173,#29887,#17123,.T.);
#36679=EDGE_CURVE('',#29980,#30173,#22044,.T.);
#36680=EDGE_CURVE('',#29888,#30173,#17124,.T.);
#36681=EDGE_CURVE('',#30174,#29888,#17125,.T.);
#36682=EDGE_CURVE('',#29984,#30174,#22045,.T.);
#36683=EDGE_CURVE('',#29889,#30174,#17126,.T.);
#36684=EDGE_CURVE('',#30175,#29889,#17127,.T.);
#36685=EDGE_CURVE('',#29988,#30175,#22046,.T.);
#36686=EDGE_CURVE('',#29890,#30175,#17128,.T.);
#36687=EDGE_CURVE('',#30176,#29890,#17129,.T.);
#36688=EDGE_CURVE('',#29004,#30176,#22047,.T.);
#36689=EDGE_CURVE('',#29891,#30176,#17130,.T.);
#36690=EDGE_CURVE('',#30177,#29891,#17131,.T.);
#36691=EDGE_CURVE('',#29992,#30177,#22048,.T.);
#36692=EDGE_CURVE('',#29892,#30177,#17132,.T.);
#36693=EDGE_CURVE('',#30178,#29892,#17133,.T.);
#36694=EDGE_CURVE('',#29996,#30178,#22049,.T.);
#36695=EDGE_CURVE('',#29893,#30178,#17134,.T.);
#36696=EDGE_CURVE('',#30179,#29893,#17135,.T.);
#36697=EDGE_CURVE('',#30000,#30179,#22050,.T.);
#36698=EDGE_CURVE('',#29894,#30179,#17136,.T.);
#36699=EDGE_CURVE('',#30180,#29894,#17137,.T.);
#36700=EDGE_CURVE('',#30004,#30180,#22051,.T.);
#36701=EDGE_CURVE('',#29895,#30180,#17138,.T.);
#36702=EDGE_CURVE('',#30181,#29895,#17139,.T.);
#36703=EDGE_CURVE('',#30008,#30181,#22052,.T.);
#36704=EDGE_CURVE('',#29896,#30181,#17140,.T.);
#36705=EDGE_CURVE('',#30182,#29896,#17141,.T.);
#36706=EDGE_CURVE('',#30012,#30182,#22053,.T.);
#36707=EDGE_CURVE('',#29897,#30182,#17142,.T.);
#36708=EDGE_CURVE('',#30183,#29897,#17143,.T.);
#36709=EDGE_CURVE('',#30016,#30183,#22054,.T.);
#36710=EDGE_CURVE('',#29898,#30183,#17144,.T.);
#36711=EDGE_CURVE('',#30184,#29898,#17145,.T.);
#36712=EDGE_CURVE('',#30020,#30184,#22055,.T.);
#36713=EDGE_CURVE('',#29899,#30184,#17146,.T.);
#36714=EDGE_CURVE('',#30185,#29899,#17147,.T.);
#36715=EDGE_CURVE('',#30025,#30185,#22056,.T.);
#36716=EDGE_CURVE('',#29900,#30185,#17148,.T.);
#36717=EDGE_CURVE('',#30186,#29900,#17149,.T.);
#36718=EDGE_CURVE('',#30029,#30186,#22057,.T.);
#36719=EDGE_CURVE('',#29901,#30186,#17150,.T.);
#36720=EDGE_CURVE('',#30187,#29901,#17151,.T.);
#36721=EDGE_CURVE('',#30032,#30187,#22058,.T.);
#36722=EDGE_CURVE('',#29902,#30187,#17152,.T.);
#36723=EDGE_CURVE('',#30188,#29902,#17153,.T.);
#36724=EDGE_CURVE('',#30036,#30188,#22059,.T.);
#36725=EDGE_CURVE('',#29903,#30188,#17154,.T.);
#36726=EDGE_CURVE('',#30189,#29903,#17155,.T.);
#36727=EDGE_CURVE('',#30040,#30189,#22060,.T.);
#36728=EDGE_CURVE('',#29904,#30189,#17156,.T.);
#36729=EDGE_CURVE('',#30190,#29904,#17157,.T.);
#36730=EDGE_CURVE('',#30044,#30190,#22061,.T.);
#36731=EDGE_CURVE('',#29876,#30190,#17158,.T.);
#36732=EDGE_CURVE('',#30191,#29905,#17159,.T.);
#36733=EDGE_CURVE('',#30049,#30191,#22062,.T.);
#36734=EDGE_CURVE('',#29906,#30191,#17160,.T.);
#36735=EDGE_CURVE('',#30192,#29906,#17161,.T.);
#36736=EDGE_CURVE('',#30053,#30192,#22063,.T.);
#36737=EDGE_CURVE('',#29907,#30192,#17162,.T.);
#36738=EDGE_CURVE('',#30193,#29907,#17163,.T.);
#36739=EDGE_CURVE('',#30057,#30193,#22064,.T.);
#36740=EDGE_CURVE('',#29908,#30193,#17164,.T.);
#36741=EDGE_CURVE('',#30194,#29908,#17165,.T.);
#36742=EDGE_CURVE('',#30061,#30194,#22065,.T.);
#36743=EDGE_CURVE('',#29909,#30194,#17166,.T.);
#36744=EDGE_CURVE('',#30195,#29909,#17167,.T.);
#36745=EDGE_CURVE('',#30065,#30195,#22066,.T.);
#36746=EDGE_CURVE('',#29910,#30195,#17168,.T.);
#36747=EDGE_CURVE('',#30196,#29910,#17169,.T.);
#36748=EDGE_CURVE('',#30069,#30196,#22067,.T.);
#36749=EDGE_CURVE('',#29911,#30196,#17170,.T.);
#36750=EDGE_CURVE('',#30197,#29911,#17171,.T.);
#36751=EDGE_CURVE('',#30073,#30197,#22068,.T.);
#36752=EDGE_CURVE('',#29912,#30197,#17172,.T.);
#36753=EDGE_CURVE('',#30198,#29912,#17173,.T.);
#36754=EDGE_CURVE('',#30077,#30198,#22069,.T.);
#36755=EDGE_CURVE('',#29913,#30198,#17174,.T.);
#36756=EDGE_CURVE('',#30199,#29913,#17175,.T.);
#36757=EDGE_CURVE('',#30081,#30199,#22070,.T.);
#36758=EDGE_CURVE('',#29914,#30199,#17176,.T.);
#36759=EDGE_CURVE('',#30200,#29914,#17177,.T.);
#36760=EDGE_CURVE('',#30085,#30200,#22071,.T.);
#36761=EDGE_CURVE('',#29915,#30200,#17178,.T.);
#36762=EDGE_CURVE('',#30201,#29915,#17179,.T.);
#36763=EDGE_CURVE('',#30089,#30201,#22072,.T.);
#36764=EDGE_CURVE('',#29916,#30201,#17180,.T.);
#36765=EDGE_CURVE('',#30202,#29916,#17181,.T.);
#36766=EDGE_CURVE('',#30093,#30202,#22073,.T.);
#36767=EDGE_CURVE('',#29917,#30202,#17182,.T.);
#36768=EDGE_CURVE('',#30203,#29917,#17183,.T.);
#36769=EDGE_CURVE('',#30097,#30203,#22074,.T.);
#36770=EDGE_CURVE('',#29918,#30203,#17184,.T.);
#36771=EDGE_CURVE('',#30204,#29918,#17185,.T.);
#36772=EDGE_CURVE('',#30101,#30204,#22075,.T.);
#36773=EDGE_CURVE('',#29919,#30204,#17186,.T.);
#36774=EDGE_CURVE('',#30205,#29919,#17187,.T.);
#36775=EDGE_CURVE('',#30105,#30205,#22076,.T.);
#36776=EDGE_CURVE('',#29920,#30205,#17188,.T.);
#36777=EDGE_CURVE('',#30206,#29920,#17189,.T.);
#36778=EDGE_CURVE('',#30109,#30206,#22077,.T.);
#36779=EDGE_CURVE('',#29921,#30206,#17190,.T.);
#36780=EDGE_CURVE('',#30207,#29921,#17191,.T.);
#36781=EDGE_CURVE('',#30113,#30207,#22078,.T.);
#36782=EDGE_CURVE('',#29922,#30207,#17192,.T.);
#36783=EDGE_CURVE('',#30208,#29922,#17193,.T.);
#36784=EDGE_CURVE('',#30117,#30208,#22079,.T.);
#36785=EDGE_CURVE('',#29923,#30208,#17194,.T.);
#36786=EDGE_CURVE('',#30209,#29923,#17195,.T.);
#36787=EDGE_CURVE('',#30121,#30209,#22080,.T.);
#36788=EDGE_CURVE('',#29924,#30209,#17196,.T.);
#36789=EDGE_CURVE('',#30210,#29924,#17197,.T.);
#36790=EDGE_CURVE('',#30125,#30210,#22081,.T.);
#36791=EDGE_CURVE('',#29925,#30210,#17198,.T.);
#36792=EDGE_CURVE('',#30211,#29925,#17199,.T.);
#36793=EDGE_CURVE('',#30129,#30211,#22082,.T.);
#36794=EDGE_CURVE('',#29926,#30211,#17200,.T.);
#36795=EDGE_CURVE('',#30212,#29926,#17201,.T.);
#36796=EDGE_CURVE('',#30133,#30212,#22083,.T.);
#36797=EDGE_CURVE('',#29927,#30212,#17202,.T.);
#36798=EDGE_CURVE('',#30213,#29927,#17203,.T.);
#36799=EDGE_CURVE('',#30137,#30213,#22084,.T.);
#36800=EDGE_CURVE('',#29928,#30213,#17204,.T.);
#36801=EDGE_CURVE('',#30214,#29928,#17205,.T.);
#36802=EDGE_CURVE('',#30141,#30214,#22085,.T.);
#36803=EDGE_CURVE('',#29929,#30214,#17206,.T.);
#36804=EDGE_CURVE('',#30215,#29929,#17207,.T.);
#36805=EDGE_CURVE('',#30145,#30215,#22086,.T.);
#36806=EDGE_CURVE('',#29930,#30215,#17208,.T.);
#36807=EDGE_CURVE('',#30216,#29930,#17209,.T.);
#36808=EDGE_CURVE('',#30149,#30216,#22087,.T.);
#36809=EDGE_CURVE('',#29931,#30216,#17210,.T.);
#36810=EDGE_CURVE('',#30217,#29931,#17211,.T.);
#36811=EDGE_CURVE('',#30153,#30217,#22088,.T.);
#36812=EDGE_CURVE('',#29932,#30217,#17212,.T.);
#36813=EDGE_CURVE('',#30218,#29932,#17213,.T.);
#36814=EDGE_CURVE('',#30157,#30218,#22089,.T.);
#36815=EDGE_CURVE('',#29933,#30218,#17214,.T.);
#36816=EDGE_CURVE('',#30219,#29933,#17215,.T.);
#36817=EDGE_CURVE('',#30161,#30219,#22090,.T.);
#36818=EDGE_CURVE('',#29905,#30219,#17216,.T.);
#36819=EDGE_CURVE('',#30220,#30221,#17217,.T.);
#36820=EDGE_CURVE('',#30162,#30221,#24828,.T.);
#36821=EDGE_CURVE('',#30220,#29876,#22091,.T.);
#36822=EDGE_CURVE('',#30222,#30223,#17218,.T.);
#36823=EDGE_CURVE('',#29877,#30223,#22092,.T.);
#36824=EDGE_CURVE('',#30222,#30162,#24829,.T.);
#36825=EDGE_CURVE('',#30224,#30222,#22093,.T.);
#36826=EDGE_CURVE('',#30225,#30224,#17219,.T.);
#36827=EDGE_CURVE('',#30223,#30225,#17220,.T.);
#36828=EDGE_CURVE('',#30163,#30225,#24830,.T.);
#36829=EDGE_CURVE('',#30226,#30227,#17221,.T.);
#36830=EDGE_CURVE('',#29878,#30227,#22094,.T.);
#36831=EDGE_CURVE('',#30226,#30163,#24831,.T.);
#36832=EDGE_CURVE('',#30228,#30226,#22095,.T.);
#36833=EDGE_CURVE('',#30229,#30228,#17222,.T.);
#36834=EDGE_CURVE('',#30227,#30229,#17223,.T.);
#36835=EDGE_CURVE('',#30164,#30229,#24832,.T.);
#36836=EDGE_CURVE('',#30230,#30231,#17224,.T.);
#36837=EDGE_CURVE('',#29879,#30231,#22096,.T.);
#36838=EDGE_CURVE('',#30230,#30164,#24833,.T.);
#36839=EDGE_CURVE('',#30232,#30230,#22097,.T.);
#36840=EDGE_CURVE('',#30233,#30232,#17225,.T.);
#36841=EDGE_CURVE('',#30231,#30233,#17226,.T.);
#36842=EDGE_CURVE('',#30165,#30233,#24834,.T.);
#36843=EDGE_CURVE('',#30234,#30235,#17227,.T.);
#36844=EDGE_CURVE('',#29880,#30235,#22098,.T.);
#36845=EDGE_CURVE('',#30234,#30165,#24835,.T.);
#36846=EDGE_CURVE('',#30236,#30234,#22099,.T.);
#36847=EDGE_CURVE('',#30237,#30236,#17228,.T.);
#36848=EDGE_CURVE('',#30235,#30237,#17229,.T.);
#36849=EDGE_CURVE('',#30166,#30237,#24836,.T.);
#36850=EDGE_CURVE('',#30238,#30239,#17230,.T.);
#36851=EDGE_CURVE('',#29881,#30239,#22100,.T.);
#36852=EDGE_CURVE('',#30238,#30166,#24837,.T.);
#36853=EDGE_CURVE('',#30240,#30238,#22101,.T.);
#36854=EDGE_CURVE('',#30241,#30240,#17231,.T.);
#36855=EDGE_CURVE('',#30239,#30241,#17232,.T.);
#36856=EDGE_CURVE('',#30167,#30241,#24838,.T.);
#36857=EDGE_CURVE('',#30242,#30243,#17233,.T.);
#36858=EDGE_CURVE('',#29882,#30243,#22102,.T.);
#36859=EDGE_CURVE('',#30242,#30167,#24839,.T.);
#36860=EDGE_CURVE('',#30244,#30242,#22103,.T.);
#36861=EDGE_CURVE('',#30245,#30244,#17234,.T.);
#36862=EDGE_CURVE('',#30243,#30245,#17235,.T.);
#36863=EDGE_CURVE('',#30168,#30245,#24840,.T.);
#36864=EDGE_CURVE('',#29883,#28998,#22104,.T.);
#36865=EDGE_CURVE('',#29000,#30168,#24841,.T.);
#36866=EDGE_CURVE('',#30169,#28999,#24842,.T.);
#36867=EDGE_CURVE('',#30246,#30247,#17236,.T.);
#36868=EDGE_CURVE('',#29884,#30247,#22105,.T.);
#36869=EDGE_CURVE('',#30246,#30169,#24843,.T.);
#36870=EDGE_CURVE('',#30248,#30246,#22106,.T.);
#36871=EDGE_CURVE('',#30249,#30248,#17237,.T.);
#36872=EDGE_CURVE('',#30247,#30249,#17238,.T.);
#36873=EDGE_CURVE('',#30170,#30249,#24844,.T.);
#36874=EDGE_CURVE('',#30250,#30251,#17239,.T.);
#36875=EDGE_CURVE('',#29885,#30251,#22107,.T.);
#36876=EDGE_CURVE('',#30250,#30170,#24845,.T.);
#36877=EDGE_CURVE('',#30252,#30250,#22108,.T.);
#36878=EDGE_CURVE('',#30253,#30252,#17240,.T.);
#36879=EDGE_CURVE('',#30251,#30253,#17241,.T.);
#36880=EDGE_CURVE('',#30171,#30253,#24846,.T.);
#36881=EDGE_CURVE('',#30254,#30255,#17242,.T.);
#36882=EDGE_CURVE('',#29886,#30255,#22109,.T.);
#36883=EDGE_CURVE('',#30254,#30171,#24847,.T.);
#36884=EDGE_CURVE('',#30256,#30254,#22110,.T.);
#36885=EDGE_CURVE('',#30257,#30256,#17243,.T.);
#36886=EDGE_CURVE('',#30255,#30257,#17244,.T.);
#36887=EDGE_CURVE('',#30172,#30257,#24848,.T.);
#36888=EDGE_CURVE('',#30258,#30259,#17245,.T.);
#36889=EDGE_CURVE('',#29887,#30259,#22111,.T.);
#36890=EDGE_CURVE('',#30258,#30172,#24849,.T.);
#36891=EDGE_CURVE('',#30260,#30258,#22112,.T.);
#36892=EDGE_CURVE('',#30261,#30260,#17246,.T.);
#36893=EDGE_CURVE('',#30259,#30261,#17247,.T.);
#36894=EDGE_CURVE('',#30173,#30261,#24850,.T.);
#36895=EDGE_CURVE('',#30262,#30263,#17248,.T.);
#36896=EDGE_CURVE('',#29888,#30263,#22113,.T.);
#36897=EDGE_CURVE('',#30262,#30173,#24851,.T.);
#36898=EDGE_CURVE('',#30264,#30262,#22114,.T.);
#36899=EDGE_CURVE('',#30265,#30264,#17249,.T.);
#36900=EDGE_CURVE('',#30263,#30265,#17250,.T.);
#36901=EDGE_CURVE('',#30174,#30265,#24852,.T.);
#36902=EDGE_CURVE('',#30266,#30267,#17251,.T.);
#36903=EDGE_CURVE('',#29889,#30267,#22115,.T.);
#36904=EDGE_CURVE('',#30266,#30174,#24853,.T.);
#36905=EDGE_CURVE('',#30268,#30266,#22116,.T.);
#36906=EDGE_CURVE('',#30269,#30268,#17252,.T.);
#36907=EDGE_CURVE('',#30267,#30269,#17253,.T.);
#36908=EDGE_CURVE('',#30175,#30269,#24854,.T.);
#36909=EDGE_CURVE('',#30270,#30271,#17254,.T.);
#36910=EDGE_CURVE('',#29890,#30271,#22117,.T.);
#36911=EDGE_CURVE('',#30270,#30175,#24855,.T.);
#36912=EDGE_CURVE('',#30272,#30270,#22118,.T.);
#36913=EDGE_CURVE('',#30273,#30272,#17255,.T.);
#36914=EDGE_CURVE('',#30271,#30273,#17256,.T.);
#36915=EDGE_CURVE('',#30176,#30273,#24856,.T.);
#36916=EDGE_CURVE('',#30274,#30275,#17257,.T.);
#36917=EDGE_CURVE('',#29891,#30275,#22119,.T.);
#36918=EDGE_CURVE('',#30274,#30176,#24857,.T.);
#36919=EDGE_CURVE('',#30276,#30274,#22120,.T.);
#36920=EDGE_CURVE('',#30277,#30276,#17258,.T.);
#36921=EDGE_CURVE('',#30275,#30277,#17259,.T.);
#36922=EDGE_CURVE('',#30177,#30277,#24858,.T.);
#36923=EDGE_CURVE('',#30278,#30279,#17260,.T.);
#36924=EDGE_CURVE('',#29892,#30279,#22121,.T.);
#36925=EDGE_CURVE('',#30278,#30177,#24859,.T.);
#36926=EDGE_CURVE('',#30280,#30278,#22122,.T.);
#36927=EDGE_CURVE('',#30281,#30280,#17261,.T.);
#36928=EDGE_CURVE('',#30279,#30281,#17262,.T.);
#36929=EDGE_CURVE('',#30178,#30281,#24860,.T.);
#36930=EDGE_CURVE('',#30282,#30283,#17263,.T.);
#36931=EDGE_CURVE('',#29893,#30283,#22123,.T.);
#36932=EDGE_CURVE('',#30282,#30178,#24861,.T.);
#36933=EDGE_CURVE('',#30284,#30282,#22124,.T.);
#36934=EDGE_CURVE('',#30285,#30284,#17264,.T.);
#36935=EDGE_CURVE('',#30283,#30285,#17265,.T.);
#36936=EDGE_CURVE('',#30179,#30285,#24862,.T.);
#36937=EDGE_CURVE('',#30286,#30287,#17266,.T.);
#36938=EDGE_CURVE('',#29894,#30287,#22125,.T.);
#36939=EDGE_CURVE('',#30286,#30179,#24863,.T.);
#36940=EDGE_CURVE('',#30288,#30286,#22126,.T.);
#36941=EDGE_CURVE('',#30289,#30288,#17267,.T.);
#36942=EDGE_CURVE('',#30287,#30289,#17268,.T.);
#36943=EDGE_CURVE('',#30180,#30289,#24864,.T.);
#36944=EDGE_CURVE('',#30290,#30291,#17269,.T.);
#36945=EDGE_CURVE('',#29895,#30291,#22127,.T.);
#36946=EDGE_CURVE('',#30290,#30180,#24865,.T.);
#36947=EDGE_CURVE('',#30292,#30290,#22128,.T.);
#36948=EDGE_CURVE('',#30293,#30292,#17270,.T.);
#36949=EDGE_CURVE('',#30291,#30293,#17271,.T.);
#36950=EDGE_CURVE('',#30181,#30293,#24866,.T.);
#36951=EDGE_CURVE('',#30294,#30295,#17272,.T.);
#36952=EDGE_CURVE('',#29896,#30295,#22129,.T.);
#36953=EDGE_CURVE('',#30294,#30181,#24867,.T.);
#36954=EDGE_CURVE('',#30296,#30294,#22130,.T.);
#36955=EDGE_CURVE('',#30297,#30296,#17273,.T.);
#36956=EDGE_CURVE('',#30295,#30297,#17274,.T.);
#36957=EDGE_CURVE('',#30182,#30297,#24868,.T.);
#36958=EDGE_CURVE('',#30298,#30299,#17275,.T.);
#36959=EDGE_CURVE('',#29897,#30299,#22131,.T.);
#36960=EDGE_CURVE('',#30298,#30182,#24869,.T.);
#36961=EDGE_CURVE('',#30300,#30298,#22132,.T.);
#36962=EDGE_CURVE('',#30301,#30300,#17276,.T.);
#36963=EDGE_CURVE('',#30299,#30301,#17277,.T.);
#36964=EDGE_CURVE('',#30183,#30301,#24870,.T.);
#36965=EDGE_CURVE('',#30302,#30303,#17278,.T.);
#36966=EDGE_CURVE('',#29898,#30303,#22133,.T.);
#36967=EDGE_CURVE('',#30302,#30183,#24871,.T.);
#36968=EDGE_CURVE('',#30304,#30302,#22134,.T.);
#36969=EDGE_CURVE('',#30305,#30304,#17279,.T.);
#36970=EDGE_CURVE('',#30303,#30305,#17280,.T.);
#36971=EDGE_CURVE('',#30184,#30305,#24872,.T.);
#36972=EDGE_CURVE('',#30306,#30307,#17281,.T.);
#36973=EDGE_CURVE('',#29899,#30307,#22135,.T.);
#36974=EDGE_CURVE('',#30306,#30184,#24873,.T.);
#36975=EDGE_CURVE('',#30307,#30308,#17282,.T.);
#36976=EDGE_CURVE('',#30185,#30308,#24874,.T.);
#36977=EDGE_CURVE('',#30309,#30306,#22136,.T.);
#36978=EDGE_CURVE('',#30308,#30309,#17283,.T.);
#36979=EDGE_CURVE('',#30310,#30185,#24875,.T.);
#36980=EDGE_CURVE('',#30310,#30311,#17284,.T.);
#36981=EDGE_CURVE('',#29900,#30311,#22137,.T.);
#36982=EDGE_CURVE('',#30311,#30312,#17285,.T.);
#36983=EDGE_CURVE('',#30313,#30310,#22138,.T.);
#36984=EDGE_CURVE('',#30312,#30313,#17286,.T.);
#36985=EDGE_CURVE('',#30186,#30312,#24876,.T.);
#36986=EDGE_CURVE('',#30314,#30315,#17287,.T.);
#36987=EDGE_CURVE('',#29901,#30315,#22139,.T.);
#36988=EDGE_CURVE('',#30314,#30186,#24877,.T.);
#36989=EDGE_CURVE('',#30316,#30314,#22140,.T.);
#36990=EDGE_CURVE('',#30317,#30316,#17288,.T.);
#36991=EDGE_CURVE('',#30315,#30317,#17289,.T.);
#36992=EDGE_CURVE('',#30187,#30317,#24878,.T.);
#36993=EDGE_CURVE('',#30318,#30319,#17290,.T.);
#36994=EDGE_CURVE('',#29902,#30319,#22141,.T.);
#36995=EDGE_CURVE('',#30318,#30187,#24879,.T.);
#36996=EDGE_CURVE('',#30320,#30318,#22142,.T.);
#36997=EDGE_CURVE('',#30321,#30320,#17291,.T.);
#36998=EDGE_CURVE('',#30319,#30321,#17292,.T.);
#36999=EDGE_CURVE('',#30188,#30321,#24880,.T.);
#37000=EDGE_CURVE('',#30322,#30323,#17293,.T.);
#37001=EDGE_CURVE('',#29903,#30323,#22143,.T.);
#37002=EDGE_CURVE('',#30322,#30188,#24881,.T.);
#37003=EDGE_CURVE('',#30324,#30322,#22144,.T.);
#37004=EDGE_CURVE('',#30325,#30324,#17294,.T.);
#37005=EDGE_CURVE('',#30323,#30325,#17295,.T.);
#37006=EDGE_CURVE('',#30189,#30325,#24882,.T.);
#37007=EDGE_CURVE('',#30326,#30327,#17296,.T.);
#37008=EDGE_CURVE('',#29904,#30327,#22145,.T.);
#37009=EDGE_CURVE('',#30326,#30189,#24883,.T.);
#37010=EDGE_CURVE('',#30328,#30326,#22146,.T.);
#37011=EDGE_CURVE('',#30329,#30328,#17297,.T.);
#37012=EDGE_CURVE('',#30327,#30329,#17298,.T.);
#37013=EDGE_CURVE('',#30190,#30329,#24884,.T.);
#37014=EDGE_CURVE('',#30330,#30331,#22147,.T.);
#37015=EDGE_CURVE('',#30221,#30330,#17299,.T.);
#37016=EDGE_CURVE('',#30331,#30220,#17300,.T.);
#37017=EDGE_CURVE('',#30331,#30190,#24885,.T.);
#37018=EDGE_CURVE('',#30332,#30333,#17301,.T.);
#37019=EDGE_CURVE('',#30191,#30333,#24886,.T.);
#37020=EDGE_CURVE('',#30332,#29905,#22148,.T.);
#37021=EDGE_CURVE('',#30334,#30191,#24887,.T.);
#37022=EDGE_CURVE('',#30334,#30335,#17302,.T.);
#37023=EDGE_CURVE('',#29906,#30335,#22149,.T.);
#37024=EDGE_CURVE('',#30335,#30336,#17303,.T.);
#37025=EDGE_CURVE('',#30192,#30336,#24888,.T.);
#37026=EDGE_CURVE('',#30337,#30334,#17304,.T.);
#37027=EDGE_CURVE('',#30336,#30337,#17305,.T.);
#37028=EDGE_CURVE('',#30338,#30192,#24889,.T.);
#37029=EDGE_CURVE('',#30338,#30339,#17306,.T.);
#37030=EDGE_CURVE('',#29907,#30339,#22150,.T.);
#37031=EDGE_CURVE('',#30339,#30340,#17307,.T.);
#37032=EDGE_CURVE('',#30193,#30340,#24890,.T.);
#37033=EDGE_CURVE('',#30341,#30338,#17308,.T.);
#37034=EDGE_CURVE('',#30340,#30341,#17309,.T.);
#37035=EDGE_CURVE('',#30342,#30193,#24891,.T.);
#37036=EDGE_CURVE('',#30342,#30343,#17310,.T.);
#37037=EDGE_CURVE('',#29908,#30343,#22151,.T.);
#37038=EDGE_CURVE('',#30343,#30344,#17311,.T.);
#37039=EDGE_CURVE('',#30194,#30344,#24892,.T.);
#37040=EDGE_CURVE('',#30345,#30342,#17312,.T.);
#37041=EDGE_CURVE('',#30344,#30345,#17313,.T.);
#37042=EDGE_CURVE('',#30346,#30194,#24893,.T.);
#37043=EDGE_CURVE('',#30346,#30347,#17314,.T.);
#37044=EDGE_CURVE('',#29909,#30347,#22152,.T.);
#37045=EDGE_CURVE('',#30347,#30348,#17315,.T.);
#37046=EDGE_CURVE('',#30195,#30348,#24894,.T.);
#37047=EDGE_CURVE('',#30349,#30346,#17316,.T.);
#37048=EDGE_CURVE('',#30348,#30349,#17317,.T.);
#37049=EDGE_CURVE('',#30350,#30195,#24895,.T.);
#37050=EDGE_CURVE('',#30350,#30351,#17318,.T.);
#37051=EDGE_CURVE('',#29910,#30351,#22153,.T.);
#37052=EDGE_CURVE('',#30351,#30352,#17319,.T.);
#37053=EDGE_CURVE('',#30196,#30352,#24896,.T.);
#37054=EDGE_CURVE('',#30353,#30350,#17320,.T.);
#37055=EDGE_CURVE('',#30352,#30353,#17321,.T.);
#37056=EDGE_CURVE('',#30354,#30196,#24897,.T.);
#37057=EDGE_CURVE('',#30354,#30355,#17322,.T.);
#37058=EDGE_CURVE('',#29911,#30355,#22154,.T.);
#37059=EDGE_CURVE('',#30355,#30356,#17323,.T.);
#37060=EDGE_CURVE('',#30197,#30356,#24898,.T.);
#37061=EDGE_CURVE('',#30357,#30354,#17324,.T.);
#37062=EDGE_CURVE('',#30356,#30357,#17325,.T.);
#37063=EDGE_CURVE('',#30358,#30197,#24899,.T.);
#37064=EDGE_CURVE('',#30358,#30359,#17326,.T.);
#37065=EDGE_CURVE('',#29912,#30359,#22155,.T.);
#37066=EDGE_CURVE('',#30359,#30360,#17327,.T.);
#37067=EDGE_CURVE('',#30198,#30360,#24900,.T.);
#37068=EDGE_CURVE('',#30361,#30358,#17328,.T.);
#37069=EDGE_CURVE('',#30360,#30361,#17329,.T.);
#37070=EDGE_CURVE('',#30362,#30198,#24901,.T.);
#37071=EDGE_CURVE('',#30362,#30363,#17330,.T.);
#37072=EDGE_CURVE('',#29913,#30363,#22156,.T.);
#37073=EDGE_CURVE('',#30363,#30364,#17331,.T.);
#37074=EDGE_CURVE('',#30199,#30364,#24902,.T.);
#37075=EDGE_CURVE('',#30365,#30362,#17332,.T.);
#37076=EDGE_CURVE('',#30364,#30365,#17333,.T.);
#37077=EDGE_CURVE('',#30366,#30199,#24903,.T.);
#37078=EDGE_CURVE('',#30366,#30367,#17334,.T.);
#37079=EDGE_CURVE('',#29914,#30367,#22157,.T.);
#37080=EDGE_CURVE('',#30367,#30368,#17335,.T.);
#37081=EDGE_CURVE('',#30200,#30368,#24904,.T.);
#37082=EDGE_CURVE('',#30369,#30366,#17336,.T.);
#37083=EDGE_CURVE('',#30368,#30369,#17337,.T.);
#37084=EDGE_CURVE('',#30370,#30200,#24905,.T.);
#37085=EDGE_CURVE('',#30370,#30371,#17338,.T.);
#37086=EDGE_CURVE('',#29915,#30371,#22158,.T.);
#37087=EDGE_CURVE('',#30371,#30372,#17339,.T.);
#37088=EDGE_CURVE('',#30201,#30372,#24906,.T.);
#37089=EDGE_CURVE('',#30373,#30370,#17340,.T.);
#37090=EDGE_CURVE('',#30372,#30373,#17341,.T.);
#37091=EDGE_CURVE('',#30374,#30201,#24907,.T.);
#37092=EDGE_CURVE('',#30374,#30375,#17342,.T.);
#37093=EDGE_CURVE('',#29916,#30375,#22159,.T.);
#37094=EDGE_CURVE('',#30375,#30376,#17343,.T.);
#37095=EDGE_CURVE('',#30202,#30376,#24908,.T.);
#37096=EDGE_CURVE('',#30377,#30374,#17344,.T.);
#37097=EDGE_CURVE('',#30376,#30377,#17345,.T.);
#37098=EDGE_CURVE('',#30378,#30202,#24909,.T.);
#37099=EDGE_CURVE('',#30378,#30379,#17346,.T.);
#37100=EDGE_CURVE('',#29917,#30379,#22160,.T.);
#37101=EDGE_CURVE('',#30379,#30380,#17347,.T.);
#37102=EDGE_CURVE('',#30203,#30380,#24910,.T.);
#37103=EDGE_CURVE('',#30381,#30378,#17348,.T.);
#37104=EDGE_CURVE('',#30380,#30381,#17349,.T.);
#37105=EDGE_CURVE('',#30382,#30203,#24911,.T.);
#37106=EDGE_CURVE('',#30382,#30383,#17350,.T.);
#37107=EDGE_CURVE('',#29918,#30383,#22161,.T.);
#37108=EDGE_CURVE('',#30383,#30384,#17351,.T.);
#37109=EDGE_CURVE('',#30204,#30384,#24912,.T.);
#37110=EDGE_CURVE('',#30385,#30382,#17352,.T.);
#37111=EDGE_CURVE('',#30384,#30385,#17353,.T.);
#37112=EDGE_CURVE('',#28997,#30204,#24913,.T.);
#37113=EDGE_CURVE('',#29919,#28996,#22162,.T.);
#37114=EDGE_CURVE('',#30205,#28994,#24914,.T.);
#37115=EDGE_CURVE('',#30386,#30205,#24915,.T.);
#37116=EDGE_CURVE('',#30386,#30387,#17354,.T.);
#37117=EDGE_CURVE('',#29920,#30387,#22163,.T.);
#37118=EDGE_CURVE('',#30387,#30388,#17355,.T.);
#37119=EDGE_CURVE('',#30206,#30388,#24916,.T.);
#37120=EDGE_CURVE('',#30389,#30386,#17356,.T.);
#37121=EDGE_CURVE('',#30388,#30389,#17357,.T.);
#37122=EDGE_CURVE('',#30390,#30206,#24917,.T.);
#37123=EDGE_CURVE('',#30390,#30391,#17358,.T.);
#37124=EDGE_CURVE('',#29921,#30391,#22164,.T.);
#37125=EDGE_CURVE('',#30391,#30392,#17359,.T.);
#37126=EDGE_CURVE('',#30207,#30392,#24918,.T.);
#37127=EDGE_CURVE('',#30393,#30390,#17360,.T.);
#37128=EDGE_CURVE('',#30392,#30393,#17361,.T.);
#37129=EDGE_CURVE('',#30394,#30207,#24919,.T.);
#37130=EDGE_CURVE('',#30394,#30395,#17362,.T.);
#37131=EDGE_CURVE('',#29922,#30395,#22165,.T.);
#37132=EDGE_CURVE('',#30395,#30396,#17363,.T.);
#37133=EDGE_CURVE('',#30208,#30396,#24920,.T.);
#37134=EDGE_CURVE('',#30397,#30394,#17364,.T.);
#37135=EDGE_CURVE('',#30396,#30397,#17365,.T.);
#37136=EDGE_CURVE('',#30398,#30208,#24921,.T.);
#37137=EDGE_CURVE('',#30398,#30399,#17366,.T.);
#37138=EDGE_CURVE('',#29923,#30399,#22166,.T.);
#37139=EDGE_CURVE('',#30399,#30400,#17367,.T.);
#37140=EDGE_CURVE('',#30209,#30400,#24922,.T.);
#37141=EDGE_CURVE('',#30401,#30398,#17368,.T.);
#37142=EDGE_CURVE('',#30400,#30401,#17369,.T.);
#37143=EDGE_CURVE('',#30402,#30209,#24923,.T.);
#37144=EDGE_CURVE('',#30402,#30403,#17370,.T.);
#37145=EDGE_CURVE('',#29924,#30403,#22167,.T.);
#37146=EDGE_CURVE('',#30403,#30404,#17371,.T.);
#37147=EDGE_CURVE('',#30210,#30404,#24924,.T.);
#37148=EDGE_CURVE('',#30405,#30402,#17372,.T.);
#37149=EDGE_CURVE('',#30404,#30405,#17373,.T.);
#37150=EDGE_CURVE('',#30406,#30210,#24925,.T.);
#37151=EDGE_CURVE('',#30406,#30407,#17374,.T.);
#37152=EDGE_CURVE('',#29925,#30407,#22168,.T.);
#37153=EDGE_CURVE('',#30407,#30408,#17375,.T.);
#37154=EDGE_CURVE('',#30211,#30408,#24926,.T.);
#37155=EDGE_CURVE('',#30409,#30406,#17376,.T.);
#37156=EDGE_CURVE('',#30408,#30409,#17377,.T.);
#37157=EDGE_CURVE('',#30410,#30211,#24927,.T.);
#37158=EDGE_CURVE('',#30410,#30411,#17378,.T.);
#37159=EDGE_CURVE('',#29926,#30411,#22169,.T.);
#37160=EDGE_CURVE('',#30411,#30412,#17379,.T.);
#37161=EDGE_CURVE('',#30212,#30412,#24928,.T.);
#37162=EDGE_CURVE('',#30413,#30410,#17380,.T.);
#37163=EDGE_CURVE('',#30412,#30413,#17381,.T.);
#37164=EDGE_CURVE('',#30414,#30212,#24929,.T.);
#37165=EDGE_CURVE('',#30414,#30415,#17382,.T.);
#37166=EDGE_CURVE('',#29927,#30415,#22170,.T.);
#37167=EDGE_CURVE('',#30415,#30416,#17383,.T.);
#37168=EDGE_CURVE('',#30213,#30416,#24930,.T.);
#37169=EDGE_CURVE('',#30417,#30414,#17384,.T.);
#37170=EDGE_CURVE('',#30416,#30417,#17385,.T.);
#37171=EDGE_CURVE('',#30418,#30213,#24931,.T.);
#37172=EDGE_CURVE('',#30418,#30419,#17386,.T.);
#37173=EDGE_CURVE('',#29928,#30419,#22171,.T.);
#37174=EDGE_CURVE('',#30419,#30420,#17387,.T.);
#37175=EDGE_CURVE('',#30214,#30420,#24932,.T.);
#37176=EDGE_CURVE('',#30421,#30418,#17388,.T.);
#37177=EDGE_CURVE('',#30420,#30421,#17389,.T.);
#37178=EDGE_CURVE('',#30422,#30214,#24933,.T.);
#37179=EDGE_CURVE('',#30422,#30423,#17390,.T.);
#37180=EDGE_CURVE('',#29929,#30423,#22172,.T.);
#37181=EDGE_CURVE('',#30423,#30424,#17391,.T.);
#37182=EDGE_CURVE('',#30215,#30424,#24934,.T.);
#37183=EDGE_CURVE('',#30425,#30422,#17392,.T.);
#37184=EDGE_CURVE('',#30424,#30425,#17393,.T.);
#37185=EDGE_CURVE('',#30426,#30215,#24935,.T.);
#37186=EDGE_CURVE('',#30426,#30427,#17394,.T.);
#37187=EDGE_CURVE('',#29930,#30427,#22173,.T.);
#37188=EDGE_CURVE('',#30427,#30428,#17395,.T.);
#37189=EDGE_CURVE('',#30216,#30428,#24936,.T.);
#37190=EDGE_CURVE('',#30429,#30426,#17396,.T.);
#37191=EDGE_CURVE('',#30428,#30429,#17397,.T.);
#37192=EDGE_CURVE('',#30430,#30216,#24937,.T.);
#37193=EDGE_CURVE('',#30430,#30431,#17398,.T.);
#37194=EDGE_CURVE('',#29931,#30431,#22174,.T.);
#37195=EDGE_CURVE('',#30431,#30432,#17399,.T.);
#37196=EDGE_CURVE('',#30217,#30432,#24938,.T.);
#37197=EDGE_CURVE('',#30433,#30430,#17400,.T.);
#37198=EDGE_CURVE('',#30432,#30433,#17401,.T.);
#37199=EDGE_CURVE('',#30434,#30217,#24939,.T.);
#37200=EDGE_CURVE('',#30434,#30435,#17402,.T.);
#37201=EDGE_CURVE('',#29932,#30435,#22175,.T.);
#37202=EDGE_CURVE('',#30435,#30436,#17403,.T.);
#37203=EDGE_CURVE('',#30218,#30436,#24940,.T.);
#37204=EDGE_CURVE('',#30437,#30434,#17404,.T.);
#37205=EDGE_CURVE('',#30436,#30437,#17405,.T.);
#37206=EDGE_CURVE('',#30438,#30218,#24941,.T.);
#37207=EDGE_CURVE('',#30438,#30439,#17406,.T.);
#37208=EDGE_CURVE('',#29933,#30439,#22176,.T.);
#37209=EDGE_CURVE('',#30439,#30440,#17407,.T.);
#37210=EDGE_CURVE('',#30219,#30440,#24942,.T.);
#37211=EDGE_CURVE('',#30441,#30438,#17408,.T.);
#37212=EDGE_CURVE('',#30440,#30441,#17409,.T.);
#37213=EDGE_CURVE('',#30442,#30443,#17410,.T.);
#37214=EDGE_CURVE('',#30333,#30442,#17411,.T.);
#37215=EDGE_CURVE('',#30443,#30332,#17412,.T.);
#37216=EDGE_CURVE('',#30443,#30219,#24943,.T.);
#37217=EDGE_CURVE('',#30162,#30444,#17413,.T.);
#37218=EDGE_CURVE('',#30444,#30330,#22177,.T.);
#37219=EDGE_CURVE('',#30445,#30162,#22178,.T.);
#37220=EDGE_CURVE('',#30224,#30445,#22179,.T.);
#37221=EDGE_CURVE('',#30163,#30445,#17414,.T.);
#37222=EDGE_CURVE('',#30446,#30163,#22180,.T.);
#37223=EDGE_CURVE('',#30228,#30446,#22181,.T.);
#37224=EDGE_CURVE('',#30164,#30446,#17415,.T.);
#37225=EDGE_CURVE('',#30447,#30164,#22182,.T.);
#37226=EDGE_CURVE('',#30232,#30447,#22183,.T.);
#37227=EDGE_CURVE('',#30165,#30447,#17416,.T.);
#37228=EDGE_CURVE('',#30448,#30165,#22184,.T.);
#37229=EDGE_CURVE('',#30236,#30448,#22185,.T.);
#37230=EDGE_CURVE('',#30166,#30448,#17417,.T.);
#37231=EDGE_CURVE('',#30449,#30166,#22186,.T.);
#37232=EDGE_CURVE('',#30240,#30449,#22187,.T.);
#37233=EDGE_CURVE('',#30167,#30449,#17418,.T.);
#37234=EDGE_CURVE('',#30450,#30167,#22188,.T.);
#37235=EDGE_CURVE('',#30244,#30450,#22189,.T.);
#37236=EDGE_CURVE('',#30168,#30450,#17419,.T.);
#37237=EDGE_CURVE('',#30451,#30168,#22190,.T.);
#37238=EDGE_CURVE('',#29001,#30451,#22191,.T.);
#37239=EDGE_CURVE('',#30169,#30451,#17420,.T.);
#37240=EDGE_CURVE('',#30452,#30169,#22192,.T.);
#37241=EDGE_CURVE('',#30248,#30452,#22193,.T.);
#37242=EDGE_CURVE('',#30170,#30452,#17421,.T.);
#37243=EDGE_CURVE('',#30453,#30170,#22194,.T.);
#37244=EDGE_CURVE('',#30252,#30453,#22195,.T.);
#37245=EDGE_CURVE('',#30171,#30453,#17422,.T.);
#37246=EDGE_CURVE('',#30454,#30171,#22196,.T.);
#37247=EDGE_CURVE('',#30256,#30454,#22197,.T.);
#37248=EDGE_CURVE('',#30172,#30454,#17423,.T.);
#37249=EDGE_CURVE('',#30455,#30172,#22198,.T.);
#37250=EDGE_CURVE('',#30260,#30455,#22199,.T.);
#37251=EDGE_CURVE('',#30173,#30455,#17424,.T.);
#37252=EDGE_CURVE('',#30456,#30173,#22200,.T.);
#37253=EDGE_CURVE('',#30264,#30456,#22201,.T.);
#37254=EDGE_CURVE('',#30174,#30456,#17425,.T.);
#37255=EDGE_CURVE('',#30457,#30174,#22202,.T.);
#37256=EDGE_CURVE('',#30268,#30457,#22203,.T.);
#37257=EDGE_CURVE('',#30175,#30457,#17426,.T.);
#37258=EDGE_CURVE('',#30458,#30175,#22204,.T.);
#37259=EDGE_CURVE('',#30272,#30458,#22205,.T.);
#37260=EDGE_CURVE('',#30176,#30458,#17427,.T.);
#37261=EDGE_CURVE('',#30459,#30176,#22206,.T.);
#37262=EDGE_CURVE('',#30276,#30459,#22207,.T.);
#37263=EDGE_CURVE('',#30177,#30459,#17428,.T.);
#37264=EDGE_CURVE('',#30460,#30177,#22208,.T.);
#37265=EDGE_CURVE('',#30280,#30460,#22209,.T.);
#37266=EDGE_CURVE('',#30178,#30460,#17429,.T.);
#37267=EDGE_CURVE('',#30461,#30178,#22210,.T.);
#37268=EDGE_CURVE('',#30284,#30461,#22211,.T.);
#37269=EDGE_CURVE('',#30179,#30461,#17430,.T.);
#37270=EDGE_CURVE('',#30462,#30179,#22212,.T.);
#37271=EDGE_CURVE('',#30288,#30462,#22213,.T.);
#37272=EDGE_CURVE('',#30180,#30462,#17431,.T.);
#37273=EDGE_CURVE('',#30463,#30180,#22214,.T.);
#37274=EDGE_CURVE('',#30292,#30463,#22215,.T.);
#37275=EDGE_CURVE('',#30181,#30463,#17432,.T.);
#37276=EDGE_CURVE('',#30464,#30181,#22216,.T.);
#37277=EDGE_CURVE('',#30296,#30464,#22217,.T.);
#37278=EDGE_CURVE('',#30182,#30464,#17433,.T.);
#37279=EDGE_CURVE('',#30465,#30182,#22218,.T.);
#37280=EDGE_CURVE('',#30300,#30465,#22219,.T.);
#37281=EDGE_CURVE('',#30183,#30465,#17434,.T.);
#37282=EDGE_CURVE('',#30466,#30183,#22220,.T.);
#37283=EDGE_CURVE('',#30304,#30466,#22221,.T.);
#37284=EDGE_CURVE('',#30184,#30466,#17435,.T.);
#37285=EDGE_CURVE('',#30467,#30184,#22222,.T.);
#37286=EDGE_CURVE('',#30309,#30467,#22223,.T.);
#37287=EDGE_CURVE('',#30185,#30467,#17436,.T.);
#37288=EDGE_CURVE('',#30468,#30185,#22224,.T.);
#37289=EDGE_CURVE('',#30313,#30468,#22225,.T.);
#37290=EDGE_CURVE('',#30186,#30468,#17437,.T.);
#37291=EDGE_CURVE('',#30469,#30186,#22226,.T.);
#37292=EDGE_CURVE('',#30316,#30469,#22227,.T.);
#37293=EDGE_CURVE('',#30187,#30469,#17438,.T.);
#37294=EDGE_CURVE('',#30470,#30187,#22228,.T.);
#37295=EDGE_CURVE('',#30320,#30470,#22229,.T.);
#37296=EDGE_CURVE('',#30188,#30470,#17439,.T.);
#37297=EDGE_CURVE('',#30471,#30188,#22230,.T.);
#37298=EDGE_CURVE('',#30324,#30471,#22231,.T.);
#37299=EDGE_CURVE('',#30189,#30471,#17440,.T.);
#37300=EDGE_CURVE('',#30472,#30189,#22232,.T.);
#37301=EDGE_CURVE('',#30328,#30472,#22233,.T.);
#37302=EDGE_CURVE('',#30190,#30472,#17441,.T.);
#37303=EDGE_CURVE('',#30444,#30190,#22234,.T.);
#37304=EDGE_CURVE('',#30473,#30442,#22235,.T.);
#37305=EDGE_CURVE('',#30191,#30473,#17442,.T.);
#37306=EDGE_CURVE('',#30474,#30191,#17443,.T.);
#37307=EDGE_CURVE('',#30337,#30474,#22236,.T.);
#37308=EDGE_CURVE('',#30192,#30474,#17444,.T.);
#37309=EDGE_CURVE('',#30475,#30192,#17445,.T.);
#37310=EDGE_CURVE('',#30341,#30475,#22237,.T.);
#37311=EDGE_CURVE('',#30193,#30475,#17446,.T.);
#37312=EDGE_CURVE('',#30476,#30193,#17447,.T.);
#37313=EDGE_CURVE('',#30345,#30476,#22238,.T.);
#37314=EDGE_CURVE('',#30194,#30476,#17448,.T.);
#37315=EDGE_CURVE('',#30477,#30194,#17449,.T.);
#37316=EDGE_CURVE('',#30349,#30477,#22239,.T.);
#37317=EDGE_CURVE('',#30195,#30477,#17450,.T.);
#37318=EDGE_CURVE('',#30478,#30195,#17451,.T.);
#37319=EDGE_CURVE('',#30353,#30478,#22240,.T.);
#37320=EDGE_CURVE('',#30196,#30478,#17452,.T.);
#37321=EDGE_CURVE('',#30479,#30196,#17453,.T.);
#37322=EDGE_CURVE('',#30357,#30479,#22241,.T.);
#37323=EDGE_CURVE('',#30197,#30479,#17454,.T.);
#37324=EDGE_CURVE('',#30480,#30197,#17455,.T.);
#37325=EDGE_CURVE('',#30361,#30480,#22242,.T.);
#37326=EDGE_CURVE('',#30198,#30480,#17456,.T.);
#37327=EDGE_CURVE('',#30481,#30198,#17457,.T.);
#37328=EDGE_CURVE('',#30365,#30481,#22243,.T.);
#37329=EDGE_CURVE('',#30199,#30481,#17458,.T.);
#37330=EDGE_CURVE('',#30482,#30199,#17459,.T.);
#37331=EDGE_CURVE('',#30369,#30482,#22244,.T.);
#37332=EDGE_CURVE('',#30200,#30482,#17460,.T.);
#37333=EDGE_CURVE('',#30483,#30200,#17461,.T.);
#37334=EDGE_CURVE('',#30373,#30483,#22245,.T.);
#37335=EDGE_CURVE('',#30201,#30483,#17462,.T.);
#37336=EDGE_CURVE('',#30484,#30201,#17463,.T.);
#37337=EDGE_CURVE('',#30377,#30484,#22246,.T.);
#37338=EDGE_CURVE('',#30202,#30484,#17464,.T.);
#37339=EDGE_CURVE('',#30485,#30202,#17465,.T.);
#37340=EDGE_CURVE('',#30381,#30485,#22247,.T.);
#37341=EDGE_CURVE('',#30203,#30485,#17466,.T.);
#37342=EDGE_CURVE('',#30486,#30203,#17467,.T.);
#37343=EDGE_CURVE('',#30385,#30486,#22248,.T.);
#37344=EDGE_CURVE('',#30204,#30486,#17468,.T.);
#37345=EDGE_CURVE('',#30487,#30204,#17469,.T.);
#37346=EDGE_CURVE('',#28995,#30487,#22249,.T.);
#37347=EDGE_CURVE('',#30205,#30487,#17470,.T.);
#37348=EDGE_CURVE('',#30488,#30205,#17471,.T.);
#37349=EDGE_CURVE('',#30389,#30488,#22250,.T.);
#37350=EDGE_CURVE('',#30206,#30488,#17472,.T.);
#37351=EDGE_CURVE('',#30489,#30206,#17473,.T.);
#37352=EDGE_CURVE('',#30393,#30489,#22251,.T.);
#37353=EDGE_CURVE('',#30207,#30489,#17474,.T.);
#37354=EDGE_CURVE('',#30490,#30207,#17475,.T.);
#37355=EDGE_CURVE('',#30397,#30490,#22252,.T.);
#37356=EDGE_CURVE('',#30208,#30490,#17476,.T.);
#37357=EDGE_CURVE('',#30491,#30208,#17477,.T.);
#37358=EDGE_CURVE('',#30401,#30491,#22253,.T.);
#37359=EDGE_CURVE('',#30209,#30491,#17478,.T.);
#37360=EDGE_CURVE('',#30492,#30209,#17479,.T.);
#37361=EDGE_CURVE('',#30405,#30492,#22254,.T.);
#37362=EDGE_CURVE('',#30210,#30492,#17480,.T.);
#37363=EDGE_CURVE('',#30493,#30210,#17481,.T.);
#37364=EDGE_CURVE('',#30409,#30493,#22255,.T.);
#37365=EDGE_CURVE('',#30211,#30493,#17482,.T.);
#37366=EDGE_CURVE('',#30494,#30211,#17483,.T.);
#37367=EDGE_CURVE('',#30413,#30494,#22256,.T.);
#37368=EDGE_CURVE('',#30212,#30494,#17484,.T.);
#37369=EDGE_CURVE('',#30495,#30212,#17485,.T.);
#37370=EDGE_CURVE('',#30417,#30495,#22257,.T.);
#37371=EDGE_CURVE('',#30213,#30495,#17486,.T.);
#37372=EDGE_CURVE('',#30496,#30213,#17487,.T.);
#37373=EDGE_CURVE('',#30421,#30496,#22258,.T.);
#37374=EDGE_CURVE('',#30214,#30496,#17488,.T.);
#37375=EDGE_CURVE('',#30497,#30214,#17489,.T.);
#37376=EDGE_CURVE('',#30425,#30497,#22259,.T.);
#37377=EDGE_CURVE('',#30215,#30497,#17490,.T.);
#37378=EDGE_CURVE('',#30498,#30215,#17491,.T.);
#37379=EDGE_CURVE('',#30429,#30498,#22260,.T.);
#37380=EDGE_CURVE('',#30216,#30498,#17492,.T.);
#37381=EDGE_CURVE('',#30499,#30216,#17493,.T.);
#37382=EDGE_CURVE('',#30433,#30499,#22261,.T.);
#37383=EDGE_CURVE('',#30217,#30499,#17494,.T.);
#37384=EDGE_CURVE('',#30500,#30217,#17495,.T.);
#37385=EDGE_CURVE('',#30437,#30500,#22262,.T.);
#37386=EDGE_CURVE('',#30218,#30500,#17496,.T.);
#37387=EDGE_CURVE('',#30501,#30218,#17497,.T.);
#37388=EDGE_CURVE('',#30441,#30501,#22263,.T.);
#37389=EDGE_CURVE('',#30219,#30501,#17498,.T.);
#37390=EDGE_CURVE('',#30473,#30219,#17499,.T.);
#37391=EDGE_CURVE('',#30502,#30503,#17500,.T.);
#37392=EDGE_CURVE('',#30162,#30503,#22264,.T.);
#37393=EDGE_CURVE('',#30502,#30444,#24944,.T.);
#37394=EDGE_CURVE('',#30504,#30502,#17501,.T.);
#37395=EDGE_CURVE('',#30505,#30504,#17502,.T.);
#37396=EDGE_CURVE('',#30503,#30505,#22265,.T.);
#37397=EDGE_CURVE('',#30445,#30505,#24945,.T.);
#37398=EDGE_CURVE('',#30506,#30507,#17503,.T.);
#37399=EDGE_CURVE('',#30163,#30507,#22266,.T.);
#37400=EDGE_CURVE('',#30506,#30445,#24946,.T.);
#37401=EDGE_CURVE('',#30508,#30506,#17504,.T.);
#37402=EDGE_CURVE('',#30509,#30508,#17505,.T.);
#37403=EDGE_CURVE('',#30507,#30509,#22267,.T.);
#37404=EDGE_CURVE('',#30446,#30509,#24947,.T.);
#37405=EDGE_CURVE('',#30510,#30511,#17506,.T.);
#37406=EDGE_CURVE('',#30164,#30511,#22268,.T.);
#37407=EDGE_CURVE('',#30510,#30446,#24948,.T.);
#37408=EDGE_CURVE('',#30512,#30510,#17507,.T.);
#37409=EDGE_CURVE('',#30513,#30512,#17508,.T.);
#37410=EDGE_CURVE('',#30511,#30513,#22269,.T.);
#37411=EDGE_CURVE('',#30447,#30513,#24949,.T.);
#37412=EDGE_CURVE('',#30514,#30515,#17509,.T.);
#37413=EDGE_CURVE('',#30165,#30515,#22270,.T.);
#37414=EDGE_CURVE('',#30514,#30447,#24950,.T.);
#37415=EDGE_CURVE('',#30516,#30514,#17510,.T.);
#37416=EDGE_CURVE('',#30517,#30516,#17511,.T.);
#37417=EDGE_CURVE('',#30515,#30517,#22271,.T.);
#37418=EDGE_CURVE('',#30448,#30517,#24951,.T.);
#37419=EDGE_CURVE('',#30518,#30519,#17512,.T.);
#37420=EDGE_CURVE('',#30166,#30519,#22272,.T.);
#37421=EDGE_CURVE('',#30518,#30448,#24952,.T.);
#37422=EDGE_CURVE('',#30520,#30518,#17513,.T.);
#37423=EDGE_CURVE('',#30521,#30520,#17514,.T.);
#37424=EDGE_CURVE('',#30519,#30521,#22273,.T.);
#37425=EDGE_CURVE('',#30449,#30521,#24953,.T.);
#37426=EDGE_CURVE('',#30522,#30523,#17515,.T.);
#37427=EDGE_CURVE('',#30167,#30523,#22274,.T.);
#37428=EDGE_CURVE('',#30522,#30449,#24954,.T.);
#37429=EDGE_CURVE('',#30524,#30522,#17516,.T.);
#37430=EDGE_CURVE('',#30525,#30524,#17517,.T.);
#37431=EDGE_CURVE('',#30523,#30525,#22275,.T.);
#37432=EDGE_CURVE('',#30450,#30525,#24955,.T.);
#37433=EDGE_CURVE('',#30526,#30527,#17518,.T.);
#37434=EDGE_CURVE('',#30168,#30527,#22276,.T.);
#37435=EDGE_CURVE('',#30526,#30450,#24956,.T.);
#37436=EDGE_CURVE('',#30528,#30526,#17519,.T.);
#37437=EDGE_CURVE('',#30529,#30528,#17520,.T.);
#37438=EDGE_CURVE('',#30527,#30529,#22277,.T.);
#37439=EDGE_CURVE('',#30451,#30529,#24957,.T.);
#37440=EDGE_CURVE('',#30530,#30531,#17521,.T.);
#37441=EDGE_CURVE('',#30169,#30531,#22278,.T.);
#37442=EDGE_CURVE('',#30530,#30451,#24958,.T.);
#37443=EDGE_CURVE('',#30532,#30530,#17522,.T.);
#37444=EDGE_CURVE('',#30533,#30532,#17523,.T.);
#37445=EDGE_CURVE('',#30531,#30533,#22279,.T.);
#37446=EDGE_CURVE('',#30452,#30533,#24959,.T.);
#37447=EDGE_CURVE('',#30534,#30535,#17524,.T.);
#37448=EDGE_CURVE('',#30170,#30535,#22280,.T.);
#37449=EDGE_CURVE('',#30534,#30452,#24960,.T.);
#37450=EDGE_CURVE('',#30536,#30534,#17525,.T.);
#37451=EDGE_CURVE('',#30537,#30536,#17526,.T.);
#37452=EDGE_CURVE('',#30535,#30537,#22281,.T.);
#37453=EDGE_CURVE('',#30453,#30537,#24961,.T.);
#37454=EDGE_CURVE('',#30538,#30539,#17527,.T.);
#37455=EDGE_CURVE('',#30171,#30539,#22282,.T.);
#37456=EDGE_CURVE('',#30538,#30453,#24962,.T.);
#37457=EDGE_CURVE('',#30540,#30538,#17528,.T.);
#37458=EDGE_CURVE('',#30541,#30540,#17529,.T.);
#37459=EDGE_CURVE('',#30539,#30541,#22283,.T.);
#37460=EDGE_CURVE('',#30454,#30541,#24963,.T.);
#37461=EDGE_CURVE('',#30542,#30543,#17530,.T.);
#37462=EDGE_CURVE('',#30172,#30543,#22284,.T.);
#37463=EDGE_CURVE('',#30542,#30454,#24964,.T.);
#37464=EDGE_CURVE('',#30544,#30542,#17531,.T.);
#37465=EDGE_CURVE('',#30545,#30544,#17532,.T.);
#37466=EDGE_CURVE('',#30543,#30545,#22285,.T.);
#37467=EDGE_CURVE('',#30455,#30545,#24965,.T.);
#37468=EDGE_CURVE('',#30546,#30547,#17533,.T.);
#37469=EDGE_CURVE('',#30173,#30547,#22286,.T.);
#37470=EDGE_CURVE('',#30546,#30455,#24966,.T.);
#37471=EDGE_CURVE('',#30548,#30546,#17534,.T.);
#37472=EDGE_CURVE('',#30549,#30548,#17535,.T.);
#37473=EDGE_CURVE('',#30547,#30549,#22287,.T.);
#37474=EDGE_CURVE('',#30456,#30549,#24967,.T.);
#37475=EDGE_CURVE('',#30550,#30551,#17536,.T.);
#37476=EDGE_CURVE('',#30174,#30551,#22288,.T.);
#37477=EDGE_CURVE('',#30550,#30456,#24968,.T.);
#37478=EDGE_CURVE('',#30552,#30550,#17537,.T.);
#37479=EDGE_CURVE('',#30553,#30552,#17538,.T.);
#37480=EDGE_CURVE('',#30551,#30553,#22289,.T.);
#37481=EDGE_CURVE('',#30457,#30553,#24969,.T.);
#37482=EDGE_CURVE('',#30554,#30555,#17539,.T.);
#37483=EDGE_CURVE('',#30175,#30555,#22290,.T.);
#37484=EDGE_CURVE('',#30554,#30457,#24970,.T.);
#37485=EDGE_CURVE('',#30556,#30554,#17540,.T.);
#37486=EDGE_CURVE('',#30557,#30556,#17541,.T.);
#37487=EDGE_CURVE('',#30555,#30557,#22291,.T.);
#37488=EDGE_CURVE('',#30458,#30557,#24971,.T.);
#37489=EDGE_CURVE('',#30176,#28991,#22292,.T.);
#37490=EDGE_CURVE('',#28990,#30458,#24972,.T.);
#37491=EDGE_CURVE('',#30459,#28993,#24973,.T.);
#37492=EDGE_CURVE('',#30558,#30559,#17542,.T.);
#37493=EDGE_CURVE('',#30177,#30559,#22293,.T.);
#37494=EDGE_CURVE('',#30558,#30459,#24974,.T.);
#37495=EDGE_CURVE('',#30560,#30558,#17543,.T.);
#37496=EDGE_CURVE('',#30561,#30560,#17544,.T.);
#37497=EDGE_CURVE('',#30559,#30561,#22294,.T.);
#37498=EDGE_CURVE('',#30460,#30561,#24975,.T.);
#37499=EDGE_CURVE('',#30562,#30563,#17545,.T.);
#37500=EDGE_CURVE('',#30178,#30563,#22295,.T.);
#37501=EDGE_CURVE('',#30562,#30460,#24976,.T.);
#37502=EDGE_CURVE('',#30564,#30562,#17546,.T.);
#37503=EDGE_CURVE('',#30565,#30564,#17547,.T.);
#37504=EDGE_CURVE('',#30563,#30565,#22296,.T.);
#37505=EDGE_CURVE('',#30461,#30565,#24977,.T.);
#37506=EDGE_CURVE('',#30566,#30567,#17548,.T.);
#37507=EDGE_CURVE('',#30179,#30567,#22297,.T.);
#37508=EDGE_CURVE('',#30566,#30461,#24978,.T.);
#37509=EDGE_CURVE('',#30568,#30566,#17549,.T.);
#37510=EDGE_CURVE('',#30569,#30568,#17550,.T.);
#37511=EDGE_CURVE('',#30567,#30569,#22298,.T.);
#37512=EDGE_CURVE('',#30462,#30569,#24979,.T.);
#37513=EDGE_CURVE('',#30570,#30571,#17551,.T.);
#37514=EDGE_CURVE('',#30180,#30571,#22299,.T.);
#37515=EDGE_CURVE('',#30570,#30462,#24980,.T.);
#37516=EDGE_CURVE('',#30572,#30570,#17552,.T.);
#37517=EDGE_CURVE('',#30573,#30572,#17553,.T.);
#37518=EDGE_CURVE('',#30571,#30573,#22300,.T.);
#37519=EDGE_CURVE('',#30463,#30573,#24981,.T.);
#37520=EDGE_CURVE('',#30574,#30575,#17554,.T.);
#37521=EDGE_CURVE('',#30181,#30575,#22301,.T.);
#37522=EDGE_CURVE('',#30574,#30463,#24982,.T.);
#37523=EDGE_CURVE('',#30576,#30574,#17555,.T.);
#37524=EDGE_CURVE('',#30577,#30576,#17556,.T.);
#37525=EDGE_CURVE('',#30575,#30577,#22302,.T.);
#37526=EDGE_CURVE('',#30464,#30577,#24983,.T.);
#37527=EDGE_CURVE('',#30578,#30579,#17557,.T.);
#37528=EDGE_CURVE('',#30182,#30579,#22303,.T.);
#37529=EDGE_CURVE('',#30578,#30464,#24984,.T.);
#37530=EDGE_CURVE('',#30580,#30578,#17558,.T.);
#37531=EDGE_CURVE('',#30581,#30580,#17559,.T.);
#37532=EDGE_CURVE('',#30579,#30581,#22304,.T.);
#37533=EDGE_CURVE('',#30465,#30581,#24985,.T.);
#37534=EDGE_CURVE('',#30582,#30583,#17560,.T.);
#37535=EDGE_CURVE('',#30183,#30583,#22305,.T.);
#37536=EDGE_CURVE('',#30582,#30465,#24986,.T.);
#37537=EDGE_CURVE('',#30584,#30582,#17561,.T.);
#37538=EDGE_CURVE('',#30585,#30584,#17562,.T.);
#37539=EDGE_CURVE('',#30583,#30585,#22306,.T.);
#37540=EDGE_CURVE('',#30466,#30585,#24987,.T.);
#37541=EDGE_CURVE('',#30586,#30587,#17563,.T.);
#37542=EDGE_CURVE('',#30184,#30587,#22307,.T.);
#37543=EDGE_CURVE('',#30586,#30466,#24988,.T.);
#37544=EDGE_CURVE('',#30587,#30588,#22308,.T.);
#37545=EDGE_CURVE('',#30467,#30588,#24989,.T.);
#37546=EDGE_CURVE('',#30589,#30586,#17564,.T.);
#37547=EDGE_CURVE('',#30588,#30589,#17565,.T.);
#37548=EDGE_CURVE('',#30590,#30467,#24990,.T.);
#37549=EDGE_CURVE('',#30590,#30591,#17566,.T.);
#37550=EDGE_CURVE('',#30185,#30591,#22309,.T.);
#37551=EDGE_CURVE('',#30591,#30592,#22310,.T.);
#37552=EDGE_CURVE('',#30593,#30590,#17567,.T.);
#37553=EDGE_CURVE('',#30592,#30593,#17568,.T.);
#37554=EDGE_CURVE('',#30468,#30592,#24991,.T.);
#37555=EDGE_CURVE('',#30594,#30595,#17569,.T.);
#37556=EDGE_CURVE('',#30186,#30595,#22311,.T.);
#37557=EDGE_CURVE('',#30594,#30468,#24992,.T.);
#37558=EDGE_CURVE('',#30596,#30594,#17570,.T.);
#37559=EDGE_CURVE('',#30597,#30596,#17571,.T.);
#37560=EDGE_CURVE('',#30595,#30597,#22312,.T.);
#37561=EDGE_CURVE('',#30469,#30597,#24993,.T.);
#37562=EDGE_CURVE('',#30598,#30599,#17572,.T.);
#37563=EDGE_CURVE('',#30187,#30599,#22313,.T.);
#37564=EDGE_CURVE('',#30598,#30469,#24994,.T.);
#37565=EDGE_CURVE('',#30600,#30598,#17573,.T.);
#37566=EDGE_CURVE('',#30601,#30600,#17574,.T.);
#37567=EDGE_CURVE('',#30599,#30601,#22314,.T.);
#37568=EDGE_CURVE('',#30470,#30601,#24995,.T.);
#37569=EDGE_CURVE('',#30602,#30603,#17575,.T.);
#37570=EDGE_CURVE('',#30188,#30603,#22315,.T.);
#37571=EDGE_CURVE('',#30602,#30470,#24996,.T.);
#37572=EDGE_CURVE('',#30604,#30602,#17576,.T.);
#37573=EDGE_CURVE('',#30605,#30604,#17577,.T.);
#37574=EDGE_CURVE('',#30603,#30605,#22316,.T.);
#37575=EDGE_CURVE('',#30471,#30605,#24997,.T.);
#37576=EDGE_CURVE('',#30606,#30607,#17578,.T.);
#37577=EDGE_CURVE('',#30189,#30607,#22317,.T.);
#37578=EDGE_CURVE('',#30606,#30471,#24998,.T.);
#37579=EDGE_CURVE('',#30608,#30606,#17579,.T.);
#37580=EDGE_CURVE('',#30609,#30608,#17580,.T.);
#37581=EDGE_CURVE('',#30607,#30609,#22318,.T.);
#37582=EDGE_CURVE('',#30472,#30609,#24999,.T.);
#37583=EDGE_CURVE('',#30610,#30611,#17581,.T.);
#37584=EDGE_CURVE('',#30190,#30611,#22319,.T.);
#37585=EDGE_CURVE('',#30610,#30472,#25000,.T.);
#37586=EDGE_CURVE('',#30612,#30610,#17582,.T.);
#37587=EDGE_CURVE('',#30613,#30612,#17583,.T.);
#37588=EDGE_CURVE('',#30611,#30613,#22320,.T.);
#37589=EDGE_CURVE('',#30444,#30613,#25001,.T.);
#37590=EDGE_CURVE('',#30614,#30473,#25002,.T.);
#37591=EDGE_CURVE('',#30614,#30615,#17584,.T.);
#37592=EDGE_CURVE('',#30191,#30615,#22321,.T.);
#37593=EDGE_CURVE('',#30615,#30616,#17585,.T.);
#37594=EDGE_CURVE('',#30474,#30616,#25003,.T.);
#37595=EDGE_CURVE('',#30617,#30614,#17586,.T.);
#37596=EDGE_CURVE('',#30616,#30617,#17587,.T.);
#37597=EDGE_CURVE('',#30618,#30474,#25004,.T.);
#37598=EDGE_CURVE('',#30618,#30619,#17588,.T.);
#37599=EDGE_CURVE('',#30192,#30619,#22322,.T.);
#37600=EDGE_CURVE('',#30619,#30620,#17589,.T.);
#37601=EDGE_CURVE('',#30475,#30620,#25005,.T.);
#37602=EDGE_CURVE('',#30621,#30618,#17590,.T.);
#37603=EDGE_CURVE('',#30620,#30621,#17591,.T.);
#37604=EDGE_CURVE('',#30622,#30475,#25006,.T.);
#37605=EDGE_CURVE('',#30622,#30623,#17592,.T.);
#37606=EDGE_CURVE('',#30193,#30623,#22323,.T.);
#37607=EDGE_CURVE('',#30623,#30624,#17593,.T.);
#37608=EDGE_CURVE('',#30476,#30624,#25007,.T.);
#37609=EDGE_CURVE('',#30625,#30622,#17594,.T.);
#37610=EDGE_CURVE('',#30624,#30625,#17595,.T.);
#37611=EDGE_CURVE('',#30626,#30476,#25008,.T.);
#37612=EDGE_CURVE('',#30626,#30627,#17596,.T.);
#37613=EDGE_CURVE('',#30194,#30627,#22324,.T.);
#37614=EDGE_CURVE('',#30627,#30628,#17597,.T.);
#37615=EDGE_CURVE('',#30477,#30628,#25009,.T.);
#37616=EDGE_CURVE('',#30629,#30626,#17598,.T.);
#37617=EDGE_CURVE('',#30628,#30629,#17599,.T.);
#37618=EDGE_CURVE('',#30630,#30477,#25010,.T.);
#37619=EDGE_CURVE('',#30630,#30631,#17600,.T.);
#37620=EDGE_CURVE('',#30195,#30631,#22325,.T.);
#37621=EDGE_CURVE('',#30631,#30632,#17601,.T.);
#37622=EDGE_CURVE('',#30478,#30632,#25011,.T.);
#37623=EDGE_CURVE('',#30633,#30630,#17602,.T.);
#37624=EDGE_CURVE('',#30632,#30633,#17603,.T.);
#37625=EDGE_CURVE('',#30634,#30478,#25012,.T.);
#37626=EDGE_CURVE('',#30634,#30635,#17604,.T.);
#37627=EDGE_CURVE('',#30196,#30635,#22326,.T.);
#37628=EDGE_CURVE('',#30635,#30636,#17605,.T.);
#37629=EDGE_CURVE('',#30479,#30636,#25013,.T.);
#37630=EDGE_CURVE('',#30637,#30634,#17606,.T.);
#37631=EDGE_CURVE('',#30636,#30637,#17607,.T.);
#37632=EDGE_CURVE('',#30638,#30479,#25014,.T.);
#37633=EDGE_CURVE('',#30638,#30639,#17608,.T.);
#37634=EDGE_CURVE('',#30197,#30639,#22327,.T.);
#37635=EDGE_CURVE('',#30639,#30640,#17609,.T.);
#37636=EDGE_CURVE('',#30480,#30640,#25015,.T.);
#37637=EDGE_CURVE('',#30641,#30638,#17610,.T.);
#37638=EDGE_CURVE('',#30640,#30641,#17611,.T.);
#37639=EDGE_CURVE('',#30642,#30480,#25016,.T.);
#37640=EDGE_CURVE('',#30642,#30643,#17612,.T.);
#37641=EDGE_CURVE('',#30198,#30643,#22328,.T.);
#37642=EDGE_CURVE('',#30643,#30644,#17613,.T.);
#37643=EDGE_CURVE('',#30481,#30644,#25017,.T.);
#37644=EDGE_CURVE('',#30645,#30642,#17614,.T.);
#37645=EDGE_CURVE('',#30644,#30645,#17615,.T.);
#37646=EDGE_CURVE('',#30646,#30481,#25018,.T.);
#37647=EDGE_CURVE('',#30646,#30647,#17616,.T.);
#37648=EDGE_CURVE('',#30199,#30647,#22329,.T.);
#37649=EDGE_CURVE('',#30647,#30648,#17617,.T.);
#37650=EDGE_CURVE('',#30482,#30648,#25019,.T.);
#37651=EDGE_CURVE('',#30649,#30646,#17618,.T.);
#37652=EDGE_CURVE('',#30648,#30649,#17619,.T.);
#37653=EDGE_CURVE('',#30650,#30482,#25020,.T.);
#37654=EDGE_CURVE('',#30650,#30651,#17620,.T.);
#37655=EDGE_CURVE('',#30200,#30651,#22330,.T.);
#37656=EDGE_CURVE('',#30651,#30652,#17621,.T.);
#37657=EDGE_CURVE('',#30483,#30652,#25021,.T.);
#37658=EDGE_CURVE('',#30653,#30650,#17622,.T.);
#37659=EDGE_CURVE('',#30652,#30653,#17623,.T.);
#37660=EDGE_CURVE('',#30654,#30483,#25022,.T.);
#37661=EDGE_CURVE('',#30654,#30655,#17624,.T.);
#37662=EDGE_CURVE('',#30201,#30655,#22331,.T.);
#37663=EDGE_CURVE('',#30655,#30656,#17625,.T.);
#37664=EDGE_CURVE('',#30484,#30656,#25023,.T.);
#37665=EDGE_CURVE('',#30657,#30654,#17626,.T.);
#37666=EDGE_CURVE('',#30656,#30657,#17627,.T.);
#37667=EDGE_CURVE('',#30658,#30484,#25024,.T.);
#37668=EDGE_CURVE('',#30658,#30659,#17628,.T.);
#37669=EDGE_CURVE('',#30202,#30659,#22332,.T.);
#37670=EDGE_CURVE('',#30659,#30660,#17629,.T.);
#37671=EDGE_CURVE('',#30485,#30660,#25025,.T.);
#37672=EDGE_CURVE('',#30661,#30658,#17630,.T.);
#37673=EDGE_CURVE('',#30660,#30661,#17631,.T.);
#37674=EDGE_CURVE('',#30662,#30485,#25026,.T.);
#37675=EDGE_CURVE('',#30662,#30663,#17632,.T.);
#37676=EDGE_CURVE('',#30203,#30663,#22333,.T.);
#37677=EDGE_CURVE('',#30663,#30664,#17633,.T.);
#37678=EDGE_CURVE('',#30486,#30664,#25027,.T.);
#37679=EDGE_CURVE('',#30665,#30662,#17634,.T.);
#37680=EDGE_CURVE('',#30664,#30665,#17635,.T.);
#37681=EDGE_CURVE('',#30666,#30486,#25028,.T.);
#37682=EDGE_CURVE('',#30666,#30667,#17636,.T.);
#37683=EDGE_CURVE('',#30204,#30667,#22334,.T.);
#37684=EDGE_CURVE('',#30667,#30668,#17637,.T.);
#37685=EDGE_CURVE('',#30487,#30668,#25029,.T.);
#37686=EDGE_CURVE('',#30669,#30666,#17638,.T.);
#37687=EDGE_CURVE('',#30668,#30669,#17639,.T.);
#37688=EDGE_CURVE('',#30670,#30487,#25030,.T.);
#37689=EDGE_CURVE('',#30670,#30671,#17640,.T.);
#37690=EDGE_CURVE('',#30205,#30671,#22335,.T.);
#37691=EDGE_CURVE('',#30671,#30672,#17641,.T.);
#37692=EDGE_CURVE('',#30488,#30672,#25031,.T.);
#37693=EDGE_CURVE('',#30673,#30670,#17642,.T.);
#37694=EDGE_CURVE('',#30672,#30673,#17643,.T.);
#37695=EDGE_CURVE('',#30674,#30488,#25032,.T.);
#37696=EDGE_CURVE('',#30674,#30675,#17644,.T.);
#37697=EDGE_CURVE('',#30206,#30675,#22336,.T.);
#37698=EDGE_CURVE('',#30675,#30676,#17645,.T.);
#37699=EDGE_CURVE('',#30489,#30676,#25033,.T.);
#37700=EDGE_CURVE('',#30677,#30674,#17646,.T.);
#37701=EDGE_CURVE('',#30676,#30677,#17647,.T.);
#37702=EDGE_CURVE('',#30678,#30489,#25034,.T.);
#37703=EDGE_CURVE('',#30678,#30679,#17648,.T.);
#37704=EDGE_CURVE('',#30207,#30679,#22337,.T.);
#37705=EDGE_CURVE('',#30679,#30680,#17649,.T.);
#37706=EDGE_CURVE('',#30490,#30680,#25035,.T.);
#37707=EDGE_CURVE('',#30681,#30678,#17650,.T.);
#37708=EDGE_CURVE('',#30680,#30681,#17651,.T.);
#37709=EDGE_CURVE('',#30682,#30490,#25036,.T.);
#37710=EDGE_CURVE('',#30682,#30683,#17652,.T.);
#37711=EDGE_CURVE('',#30208,#30683,#22338,.T.);
#37712=EDGE_CURVE('',#30683,#30684,#17653,.T.);
#37713=EDGE_CURVE('',#30491,#30684,#25037,.T.);
#37714=EDGE_CURVE('',#30685,#30682,#17654,.T.);
#37715=EDGE_CURVE('',#30684,#30685,#17655,.T.);
#37716=EDGE_CURVE('',#30686,#30491,#25038,.T.);
#37717=EDGE_CURVE('',#30686,#30687,#17656,.T.);
#37718=EDGE_CURVE('',#30209,#30687,#22339,.T.);
#37719=EDGE_CURVE('',#30687,#30688,#17657,.T.);
#37720=EDGE_CURVE('',#30492,#30688,#25039,.T.);
#37721=EDGE_CURVE('',#30689,#30686,#17658,.T.);
#37722=EDGE_CURVE('',#30688,#30689,#17659,.T.);
#37723=EDGE_CURVE('',#30690,#30492,#25040,.T.);
#37724=EDGE_CURVE('',#30690,#30691,#17660,.T.);
#37725=EDGE_CURVE('',#30210,#30691,#22340,.T.);
#37726=EDGE_CURVE('',#30691,#30692,#17661,.T.);
#37727=EDGE_CURVE('',#30493,#30692,#25041,.T.);
#37728=EDGE_CURVE('',#30693,#30690,#17662,.T.);
#37729=EDGE_CURVE('',#30692,#30693,#17663,.T.);
#37730=EDGE_CURVE('',#30694,#30493,#25042,.T.);
#37731=EDGE_CURVE('',#30694,#30695,#17664,.T.);
#37732=EDGE_CURVE('',#30211,#30695,#22341,.T.);
#37733=EDGE_CURVE('',#30695,#30696,#17665,.T.);
#37734=EDGE_CURVE('',#30494,#30696,#25043,.T.);
#37735=EDGE_CURVE('',#30697,#30694,#17666,.T.);
#37736=EDGE_CURVE('',#30696,#30697,#17667,.T.);
#37737=EDGE_CURVE('',#28987,#30494,#25044,.T.);
#37738=EDGE_CURVE('',#30212,#28989,#22342,.T.);
#37739=EDGE_CURVE('',#30495,#28988,#25045,.T.);
#37740=EDGE_CURVE('',#30698,#30495,#25046,.T.);
#37741=EDGE_CURVE('',#30698,#30699,#17668,.T.);
#37742=EDGE_CURVE('',#30213,#30699,#22343,.T.);
#37743=EDGE_CURVE('',#30699,#30700,#17669,.T.);
#37744=EDGE_CURVE('',#30496,#30700,#25047,.T.);
#37745=EDGE_CURVE('',#30701,#30698,#17670,.T.);
#37746=EDGE_CURVE('',#30700,#30701,#17671,.T.);
#37747=EDGE_CURVE('',#30702,#30496,#25048,.T.);
#37748=EDGE_CURVE('',#30702,#30703,#17672,.T.);
#37749=EDGE_CURVE('',#30214,#30703,#22344,.T.);
#37750=EDGE_CURVE('',#30703,#30704,#17673,.T.);
#37751=EDGE_CURVE('',#30497,#30704,#25049,.T.);
#37752=EDGE_CURVE('',#30705,#30702,#17674,.T.);
#37753=EDGE_CURVE('',#30704,#30705,#17675,.T.);
#37754=EDGE_CURVE('',#30706,#30497,#25050,.T.);
#37755=EDGE_CURVE('',#30706,#30707,#17676,.T.);
#37756=EDGE_CURVE('',#30215,#30707,#22345,.T.);
#37757=EDGE_CURVE('',#30707,#30708,#17677,.T.);
#37758=EDGE_CURVE('',#30498,#30708,#25051,.T.);
#37759=EDGE_CURVE('',#30709,#30706,#17678,.T.);
#37760=EDGE_CURVE('',#30708,#30709,#17679,.T.);
#37761=EDGE_CURVE('',#30710,#30498,#25052,.T.);
#37762=EDGE_CURVE('',#30710,#30711,#17680,.T.);
#37763=EDGE_CURVE('',#30216,#30711,#22346,.T.);
#37764=EDGE_CURVE('',#30711,#30712,#17681,.T.);
#37765=EDGE_CURVE('',#30499,#30712,#25053,.T.);
#37766=EDGE_CURVE('',#30713,#30710,#17682,.T.);
#37767=EDGE_CURVE('',#30712,#30713,#17683,.T.);
#37768=EDGE_CURVE('',#30714,#30499,#25054,.T.);
#37769=EDGE_CURVE('',#30714,#30715,#17684,.T.);
#37770=EDGE_CURVE('',#30217,#30715,#22347,.T.);
#37771=EDGE_CURVE('',#30715,#30716,#17685,.T.);
#37772=EDGE_CURVE('',#30500,#30716,#25055,.T.);
#37773=EDGE_CURVE('',#30717,#30714,#17686,.T.);
#37774=EDGE_CURVE('',#30716,#30717,#17687,.T.);
#37775=EDGE_CURVE('',#30718,#30500,#25056,.T.);
#37776=EDGE_CURVE('',#30718,#30719,#17688,.T.);
#37777=EDGE_CURVE('',#30218,#30719,#22348,.T.);
#37778=EDGE_CURVE('',#30719,#30720,#17689,.T.);
#37779=EDGE_CURVE('',#30501,#30720,#25057,.T.);
#37780=EDGE_CURVE('',#30721,#30718,#17690,.T.);
#37781=EDGE_CURVE('',#30720,#30721,#17691,.T.);
#37782=EDGE_CURVE('',#30722,#30501,#25058,.T.);
#37783=EDGE_CURVE('',#30722,#30723,#17692,.T.);
#37784=EDGE_CURVE('',#30219,#30723,#22349,.T.);
#37785=EDGE_CURVE('',#30723,#30724,#17693,.T.);
#37786=EDGE_CURVE('',#30473,#30724,#25059,.T.);
#37787=EDGE_CURVE('',#30725,#30722,#17694,.T.);
#37788=EDGE_CURVE('',#30724,#30725,#17695,.T.);
#37789=EDGE_CURVE('',#30726,#30444,#17696,.T.);
#37790=EDGE_CURVE('',#30504,#30726,#22350,.T.);
#37791=EDGE_CURVE('',#30445,#30726,#22351,.T.);
#37792=EDGE_CURVE('',#30727,#30445,#17697,.T.);
#37793=EDGE_CURVE('',#30508,#30727,#22352,.T.);
#37794=EDGE_CURVE('',#30446,#30727,#22353,.T.);
#37795=EDGE_CURVE('',#30728,#30446,#17698,.T.);
#37796=EDGE_CURVE('',#30512,#30728,#22354,.T.);
#37797=EDGE_CURVE('',#30447,#30728,#22355,.T.);
#37798=EDGE_CURVE('',#30729,#30447,#17699,.T.);
#37799=EDGE_CURVE('',#30516,#30729,#22356,.T.);
#37800=EDGE_CURVE('',#30448,#30729,#22357,.T.);
#37801=EDGE_CURVE('',#30730,#30448,#17700,.T.);
#37802=EDGE_CURVE('',#30520,#30730,#22358,.T.);
#37803=EDGE_CURVE('',#30449,#30730,#22359,.T.);
#37804=EDGE_CURVE('',#30731,#30449,#17701,.T.);
#37805=EDGE_CURVE('',#30524,#30731,#22360,.T.);
#37806=EDGE_CURVE('',#30450,#30731,#22361,.T.);
#37807=EDGE_CURVE('',#30732,#30450,#17702,.T.);
#37808=EDGE_CURVE('',#30528,#30732,#22362,.T.);
#37809=EDGE_CURVE('',#30451,#30732,#22363,.T.);
#37810=EDGE_CURVE('',#30733,#30451,#17703,.T.);
#37811=EDGE_CURVE('',#30532,#30733,#22364,.T.);
#37812=EDGE_CURVE('',#30452,#30733,#22365,.T.);
#37813=EDGE_CURVE('',#30734,#30452,#17704,.T.);
#37814=EDGE_CURVE('',#30536,#30734,#22366,.T.);
#37815=EDGE_CURVE('',#30453,#30734,#22367,.T.);
#37816=EDGE_CURVE('',#30735,#30453,#17705,.T.);
#37817=EDGE_CURVE('',#30540,#30735,#22368,.T.);
#37818=EDGE_CURVE('',#30454,#30735,#22369,.T.);
#37819=EDGE_CURVE('',#30736,#30454,#17706,.T.);
#37820=EDGE_CURVE('',#30544,#30736,#22370,.T.);
#37821=EDGE_CURVE('',#30455,#30736,#22371,.T.);
#37822=EDGE_CURVE('',#30737,#30455,#17707,.T.);
#37823=EDGE_CURVE('',#30548,#30737,#22372,.T.);
#37824=EDGE_CURVE('',#30456,#30737,#22373,.T.);
#37825=EDGE_CURVE('',#30738,#30456,#17708,.T.);
#37826=EDGE_CURVE('',#30552,#30738,#22374,.T.);
#37827=EDGE_CURVE('',#30457,#30738,#22375,.T.);
#37828=EDGE_CURVE('',#30739,#30457,#17709,.T.);
#37829=EDGE_CURVE('',#30556,#30739,#22376,.T.);
#37830=EDGE_CURVE('',#30458,#30739,#22377,.T.);
#37831=EDGE_CURVE('',#30740,#30458,#17710,.T.);
#37832=EDGE_CURVE('',#28992,#30740,#22378,.T.);
#37833=EDGE_CURVE('',#30459,#30740,#22379,.T.);
#37834=EDGE_CURVE('',#30741,#30459,#17711,.T.);
#37835=EDGE_CURVE('',#30560,#30741,#22380,.T.);
#37836=EDGE_CURVE('',#30460,#30741,#22381,.T.);
#37837=EDGE_CURVE('',#30742,#30460,#17712,.T.);
#37838=EDGE_CURVE('',#30564,#30742,#22382,.T.);
#37839=EDGE_CURVE('',#30461,#30742,#22383,.T.);
#37840=EDGE_CURVE('',#30743,#30461,#17713,.T.);
#37841=EDGE_CURVE('',#30568,#30743,#22384,.T.);
#37842=EDGE_CURVE('',#30462,#30743,#22385,.T.);
#37843=EDGE_CURVE('',#30744,#30462,#17714,.T.);
#37844=EDGE_CURVE('',#30572,#30744,#22386,.T.);
#37845=EDGE_CURVE('',#30463,#30744,#22387,.T.);
#37846=EDGE_CURVE('',#30745,#30463,#17715,.T.);
#37847=EDGE_CURVE('',#30576,#30745,#22388,.T.);
#37848=EDGE_CURVE('',#30464,#30745,#22389,.T.);
#37849=EDGE_CURVE('',#30746,#30464,#17716,.T.);
#37850=EDGE_CURVE('',#30580,#30746,#22390,.T.);
#37851=EDGE_CURVE('',#30465,#30746,#22391,.T.);
#37852=EDGE_CURVE('',#30747,#30465,#17717,.T.);
#37853=EDGE_CURVE('',#30584,#30747,#22392,.T.);
#37854=EDGE_CURVE('',#30466,#30747,#22393,.T.);
#37855=EDGE_CURVE('',#30748,#30466,#17718,.T.);
#37856=EDGE_CURVE('',#30589,#30748,#22394,.T.);
#37857=EDGE_CURVE('',#30467,#30748,#22395,.T.);
#37858=EDGE_CURVE('',#30749,#30467,#17719,.T.);
#37859=EDGE_CURVE('',#30593,#30749,#22396,.T.);
#37860=EDGE_CURVE('',#30468,#30749,#22397,.T.);
#37861=EDGE_CURVE('',#30750,#30468,#17720,.T.);
#37862=EDGE_CURVE('',#30596,#30750,#22398,.T.);
#37863=EDGE_CURVE('',#30469,#30750,#22399,.T.);
#37864=EDGE_CURVE('',#30751,#30469,#17721,.T.);
#37865=EDGE_CURVE('',#30600,#30751,#22400,.T.);
#37866=EDGE_CURVE('',#30470,#30751,#22401,.T.);
#37867=EDGE_CURVE('',#30752,#30470,#17722,.T.);
#37868=EDGE_CURVE('',#30604,#30752,#22402,.T.);
#37869=EDGE_CURVE('',#30471,#30752,#22403,.T.);
#37870=EDGE_CURVE('',#30753,#30471,#17723,.T.);
#37871=EDGE_CURVE('',#30608,#30753,#22404,.T.);
#37872=EDGE_CURVE('',#30472,#30753,#22405,.T.);
#37873=EDGE_CURVE('',#30754,#30472,#17724,.T.);
#37874=EDGE_CURVE('',#30612,#30754,#22406,.T.);
#37875=EDGE_CURVE('',#30444,#30754,#22407,.T.);
#37876=EDGE_CURVE('',#30755,#30473,#17725,.T.);
#37877=EDGE_CURVE('',#30617,#30755,#22408,.T.);
#37878=EDGE_CURVE('',#30474,#30755,#22409,.T.);
#37879=EDGE_CURVE('',#30756,#30474,#17726,.T.);
#37880=EDGE_CURVE('',#30621,#30756,#22410,.T.);
#37881=EDGE_CURVE('',#30475,#30756,#22411,.T.);
#37882=EDGE_CURVE('',#30757,#30475,#17727,.T.);
#37883=EDGE_CURVE('',#30625,#30757,#22412,.T.);
#37884=EDGE_CURVE('',#30476,#30757,#22413,.T.);
#37885=EDGE_CURVE('',#30758,#30476,#17728,.T.);
#37886=EDGE_CURVE('',#30629,#30758,#22414,.T.);
#37887=EDGE_CURVE('',#30477,#30758,#22415,.T.);
#37888=EDGE_CURVE('',#30759,#30477,#17729,.T.);
#37889=EDGE_CURVE('',#30633,#30759,#22416,.T.);
#37890=EDGE_CURVE('',#30478,#30759,#22417,.T.);
#37891=EDGE_CURVE('',#30760,#30478,#17730,.T.);
#37892=EDGE_CURVE('',#30637,#30760,#22418,.T.);
#37893=EDGE_CURVE('',#30479,#30760,#22419,.T.);
#37894=EDGE_CURVE('',#30761,#30479,#17731,.T.);
#37895=EDGE_CURVE('',#30641,#30761,#22420,.T.);
#37896=EDGE_CURVE('',#30480,#30761,#22421,.T.);
#37897=EDGE_CURVE('',#30762,#30480,#17732,.T.);
#37898=EDGE_CURVE('',#30645,#30762,#22422,.T.);
#37899=EDGE_CURVE('',#30481,#30762,#22423,.T.);
#37900=EDGE_CURVE('',#30763,#30481,#17733,.T.);
#37901=EDGE_CURVE('',#30649,#30763,#22424,.T.);
#37902=EDGE_CURVE('',#30482,#30763,#22425,.T.);
#37903=EDGE_CURVE('',#30764,#30482,#17734,.T.);
#37904=EDGE_CURVE('',#30653,#30764,#22426,.T.);
#37905=EDGE_CURVE('',#30483,#30764,#22427,.T.);
#37906=EDGE_CURVE('',#30765,#30483,#17735,.T.);
#37907=EDGE_CURVE('',#30657,#30765,#22428,.T.);
#37908=EDGE_CURVE('',#30484,#30765,#22429,.T.);
#37909=EDGE_CURVE('',#30766,#30484,#17736,.T.);
#37910=EDGE_CURVE('',#30661,#30766,#22430,.T.);
#37911=EDGE_CURVE('',#30485,#30766,#22431,.T.);
#37912=EDGE_CURVE('',#30767,#30485,#17737,.T.);
#37913=EDGE_CURVE('',#30665,#30767,#22432,.T.);
#37914=EDGE_CURVE('',#30486,#30767,#22433,.T.);
#37915=EDGE_CURVE('',#30768,#30486,#17738,.T.);
#37916=EDGE_CURVE('',#30669,#30768,#22434,.T.);
#37917=EDGE_CURVE('',#30487,#30768,#22435,.T.);
#37918=EDGE_CURVE('',#30769,#30487,#17739,.T.);
#37919=EDGE_CURVE('',#30673,#30769,#22436,.T.);
#37920=EDGE_CURVE('',#30488,#30769,#22437,.T.);
#37921=EDGE_CURVE('',#30770,#30488,#17740,.T.);
#37922=EDGE_CURVE('',#30677,#30770,#22438,.T.);
#37923=EDGE_CURVE('',#30489,#30770,#22439,.T.);
#37924=EDGE_CURVE('',#30771,#30489,#17741,.T.);
#37925=EDGE_CURVE('',#30681,#30771,#22440,.T.);
#37926=EDGE_CURVE('',#30490,#30771,#22441,.T.);
#37927=EDGE_CURVE('',#30772,#30490,#17742,.T.);
#37928=EDGE_CURVE('',#30685,#30772,#22442,.T.);
#37929=EDGE_CURVE('',#30491,#30772,#22443,.T.);
#37930=EDGE_CURVE('',#30773,#30491,#17743,.T.);
#37931=EDGE_CURVE('',#30689,#30773,#22444,.T.);
#37932=EDGE_CURVE('',#30492,#30773,#22445,.T.);
#37933=EDGE_CURVE('',#30774,#30492,#17744,.T.);
#37934=EDGE_CURVE('',#30693,#30774,#22446,.T.);
#37935=EDGE_CURVE('',#30493,#30774,#22447,.T.);
#37936=EDGE_CURVE('',#30775,#30493,#17745,.T.);
#37937=EDGE_CURVE('',#30697,#30775,#22448,.T.);
#37938=EDGE_CURVE('',#30494,#30775,#22449,.T.);
#37939=EDGE_CURVE('',#30776,#30494,#17746,.T.);
#37940=EDGE_CURVE('',#28986,#30776,#22450,.T.);
#37941=EDGE_CURVE('',#30495,#30776,#22451,.T.);
#37942=EDGE_CURVE('',#30777,#30495,#17747,.T.);
#37943=EDGE_CURVE('',#30701,#30777,#22452,.T.);
#37944=EDGE_CURVE('',#30496,#30777,#22453,.T.);
#37945=EDGE_CURVE('',#30778,#30496,#17748,.T.);
#37946=EDGE_CURVE('',#30705,#30778,#22454,.T.);
#37947=EDGE_CURVE('',#30497,#30778,#22455,.T.);
#37948=EDGE_CURVE('',#30779,#30497,#17749,.T.);
#37949=EDGE_CURVE('',#30709,#30779,#22456,.T.);
#37950=EDGE_CURVE('',#30498,#30779,#22457,.T.);
#37951=EDGE_CURVE('',#30780,#30498,#17750,.T.);
#37952=EDGE_CURVE('',#30713,#30780,#22458,.T.);
#37953=EDGE_CURVE('',#30499,#30780,#22459,.T.);
#37954=EDGE_CURVE('',#30781,#30499,#17751,.T.);
#37955=EDGE_CURVE('',#30717,#30781,#22460,.T.);
#37956=EDGE_CURVE('',#30500,#30781,#22461,.T.);
#37957=EDGE_CURVE('',#30782,#30500,#17752,.T.);
#37958=EDGE_CURVE('',#30721,#30782,#22462,.T.);
#37959=EDGE_CURVE('',#30501,#30782,#22463,.T.);
#37960=EDGE_CURVE('',#30783,#30501,#17753,.T.);
#37961=EDGE_CURVE('',#30725,#30783,#22464,.T.);
#37962=EDGE_CURVE('',#30473,#30783,#22465,.T.);
#37963=EDGE_CURVE('',#30784,#30785,#17754,.T.);
#37964=EDGE_CURVE('',#30726,#30785,#25060,.T.);
#37965=EDGE_CURVE('',#30784,#30444,#22466,.T.);
#37966=EDGE_CURVE('',#30786,#30787,#22467,.T.);
#37967=EDGE_CURVE('',#30445,#30787,#22468,.T.);
#37968=EDGE_CURVE('',#30786,#30726,#25061,.T.);
#37969=EDGE_CURVE('',#30788,#30786,#17755,.T.);
#37970=EDGE_CURVE('',#30789,#30788,#17756,.T.);
#37971=EDGE_CURVE('',#30787,#30789,#17757,.T.);
#37972=EDGE_CURVE('',#30727,#30789,#25062,.T.);
#37973=EDGE_CURVE('',#30790,#30791,#22469,.T.);
#37974=EDGE_CURVE('',#30446,#30791,#22470,.T.);
#37975=EDGE_CURVE('',#30790,#30727,#25063,.T.);
#37976=EDGE_CURVE('',#30792,#30790,#17758,.T.);
#37977=EDGE_CURVE('',#30793,#30792,#17759,.T.);
#37978=EDGE_CURVE('',#30791,#30793,#17760,.T.);
#37979=EDGE_CURVE('',#30728,#30793,#25064,.T.);
#37980=EDGE_CURVE('',#30794,#30795,#22471,.T.);
#37981=EDGE_CURVE('',#30447,#30795,#22472,.T.);
#37982=EDGE_CURVE('',#30794,#30728,#25065,.T.);
#37983=EDGE_CURVE('',#30796,#30794,#17761,.T.);
#37984=EDGE_CURVE('',#30797,#30796,#17762,.T.);
#37985=EDGE_CURVE('',#30795,#30797,#17763,.T.);
#37986=EDGE_CURVE('',#30729,#30797,#25066,.T.);
#37987=EDGE_CURVE('',#30798,#30799,#22473,.T.);
#37988=EDGE_CURVE('',#30448,#30799,#22474,.T.);
#37989=EDGE_CURVE('',#30798,#30729,#25067,.T.);
#37990=EDGE_CURVE('',#30800,#30798,#17764,.T.);
#37991=EDGE_CURVE('',#30801,#30800,#17765,.T.);
#37992=EDGE_CURVE('',#30799,#30801,#17766,.T.);
#37993=EDGE_CURVE('',#30730,#30801,#25068,.T.);
#37994=EDGE_CURVE('',#30802,#30803,#22475,.T.);
#37995=EDGE_CURVE('',#30449,#30803,#22476,.T.);
#37996=EDGE_CURVE('',#30802,#30730,#25069,.T.);
#37997=EDGE_CURVE('',#30804,#30802,#17767,.T.);
#37998=EDGE_CURVE('',#30805,#30804,#17768,.T.);
#37999=EDGE_CURVE('',#30803,#30805,#17769,.T.);
#38000=EDGE_CURVE('',#30731,#30805,#25070,.T.);
#38001=EDGE_CURVE('',#30806,#30807,#22477,.T.);
#38002=EDGE_CURVE('',#30450,#30807,#22478,.T.);
#38003=EDGE_CURVE('',#30806,#30731,#25071,.T.);
#38004=EDGE_CURVE('',#30808,#30806,#17770,.T.);
#38005=EDGE_CURVE('',#30809,#30808,#17771,.T.);
#38006=EDGE_CURVE('',#30807,#30809,#17772,.T.);
#38007=EDGE_CURVE('',#30732,#30809,#25072,.T.);
#38008=EDGE_CURVE('',#30451,#28982,#22479,.T.);
#38009=EDGE_CURVE('',#28984,#30732,#25073,.T.);
#38010=EDGE_CURVE('',#30733,#28983,#25074,.T.);
#38011=EDGE_CURVE('',#30810,#30811,#22480,.T.);
#38012=EDGE_CURVE('',#30452,#30811,#22481,.T.);
#38013=EDGE_CURVE('',#30810,#30733,#25075,.T.);
#38014=EDGE_CURVE('',#30812,#30810,#17773,.T.);
#38015=EDGE_CURVE('',#30813,#30812,#17774,.T.);
#38016=EDGE_CURVE('',#30811,#30813,#17775,.T.);
#38017=EDGE_CURVE('',#30734,#30813,#25076,.T.);
#38018=EDGE_CURVE('',#30814,#30815,#22482,.T.);
#38019=EDGE_CURVE('',#30453,#30815,#22483,.T.);
#38020=EDGE_CURVE('',#30814,#30734,#25077,.T.);
#38021=EDGE_CURVE('',#30816,#30814,#17776,.T.);
#38022=EDGE_CURVE('',#30817,#30816,#17777,.T.);
#38023=EDGE_CURVE('',#30815,#30817,#17778,.T.);
#38024=EDGE_CURVE('',#30735,#30817,#25078,.T.);
#38025=EDGE_CURVE('',#30818,#30819,#22484,.T.);
#38026=EDGE_CURVE('',#30454,#30819,#22485,.T.);
#38027=EDGE_CURVE('',#30818,#30735,#25079,.T.);
#38028=EDGE_CURVE('',#30820,#30818,#17779,.T.);
#38029=EDGE_CURVE('',#30821,#30820,#17780,.T.);
#38030=EDGE_CURVE('',#30819,#30821,#17781,.T.);
#38031=EDGE_CURVE('',#30736,#30821,#25080,.T.);
#38032=EDGE_CURVE('',#30822,#30823,#22486,.T.);
#38033=EDGE_CURVE('',#30455,#30823,#22487,.T.);
#38034=EDGE_CURVE('',#30822,#30736,#25081,.T.);
#38035=EDGE_CURVE('',#30824,#30822,#17782,.T.);
#38036=EDGE_CURVE('',#30825,#30824,#17783,.T.);
#38037=EDGE_CURVE('',#30823,#30825,#17784,.T.);
#38038=EDGE_CURVE('',#30737,#30825,#25082,.T.);
#38039=EDGE_CURVE('',#30826,#30827,#22488,.T.);
#38040=EDGE_CURVE('',#30456,#30827,#22489,.T.);
#38041=EDGE_CURVE('',#30826,#30737,#25083,.T.);
#38042=EDGE_CURVE('',#30828,#30826,#17785,.T.);
#38043=EDGE_CURVE('',#30829,#30828,#17786,.T.);
#38044=EDGE_CURVE('',#30827,#30829,#17787,.T.);
#38045=EDGE_CURVE('',#30738,#30829,#25084,.T.);
#38046=EDGE_CURVE('',#30830,#30831,#22490,.T.);
#38047=EDGE_CURVE('',#30457,#30831,#22491,.T.);
#38048=EDGE_CURVE('',#30830,#30738,#25085,.T.);
#38049=EDGE_CURVE('',#30832,#30830,#17788,.T.);
#38050=EDGE_CURVE('',#30833,#30832,#17789,.T.);
#38051=EDGE_CURVE('',#30831,#30833,#17790,.T.);
#38052=EDGE_CURVE('',#30739,#30833,#25086,.T.);
#38053=EDGE_CURVE('',#30834,#30835,#22492,.T.);
#38054=EDGE_CURVE('',#30458,#30835,#22493,.T.);
#38055=EDGE_CURVE('',#30834,#30739,#25087,.T.);
#38056=EDGE_CURVE('',#30836,#30834,#17791,.T.);
#38057=EDGE_CURVE('',#30837,#30836,#17792,.T.);
#38058=EDGE_CURVE('',#30835,#30837,#17793,.T.);
#38059=EDGE_CURVE('',#30740,#30837,#25088,.T.);
#38060=EDGE_CURVE('',#30838,#30839,#22494,.T.);
#38061=EDGE_CURVE('',#30459,#30839,#22495,.T.);
#38062=EDGE_CURVE('',#30838,#30740,#25089,.T.);
#38063=EDGE_CURVE('',#30840,#30838,#17794,.T.);
#38064=EDGE_CURVE('',#30841,#30840,#17795,.T.);
#38065=EDGE_CURVE('',#30839,#30841,#17796,.T.);
#38066=EDGE_CURVE('',#30741,#30841,#25090,.T.);
#38067=EDGE_CURVE('',#30842,#30843,#22496,.T.);
#38068=EDGE_CURVE('',#30460,#30843,#22497,.T.);
#38069=EDGE_CURVE('',#30842,#30741,#25091,.T.);
#38070=EDGE_CURVE('',#30844,#30842,#17797,.T.);
#38071=EDGE_CURVE('',#30845,#30844,#17798,.T.);
#38072=EDGE_CURVE('',#30843,#30845,#17799,.T.);
#38073=EDGE_CURVE('',#30742,#30845,#25092,.T.);
#38074=EDGE_CURVE('',#30846,#30847,#22498,.T.);
#38075=EDGE_CURVE('',#30461,#30847,#22499,.T.);
#38076=EDGE_CURVE('',#30846,#30742,#25093,.T.);
#38077=EDGE_CURVE('',#30848,#30846,#17800,.T.);
#38078=EDGE_CURVE('',#30849,#30848,#17801,.T.);
#38079=EDGE_CURVE('',#30847,#30849,#17802,.T.);
#38080=EDGE_CURVE('',#30743,#30849,#25094,.T.);
#38081=EDGE_CURVE('',#30850,#30851,#22500,.T.);
#38082=EDGE_CURVE('',#30462,#30851,#22501,.T.);
#38083=EDGE_CURVE('',#30850,#30743,#25095,.T.);
#38084=EDGE_CURVE('',#30852,#30850,#17803,.T.);
#38085=EDGE_CURVE('',#30853,#30852,#17804,.T.);
#38086=EDGE_CURVE('',#30851,#30853,#17805,.T.);
#38087=EDGE_CURVE('',#30744,#30853,#25096,.T.);
#38088=EDGE_CURVE('',#30854,#30855,#22502,.T.);
#38089=EDGE_CURVE('',#30463,#30855,#22503,.T.);
#38090=EDGE_CURVE('',#30854,#30744,#25097,.T.);
#38091=EDGE_CURVE('',#30856,#30854,#17806,.T.);
#38092=EDGE_CURVE('',#30857,#30856,#17807,.T.);
#38093=EDGE_CURVE('',#30855,#30857,#17808,.T.);
#38094=EDGE_CURVE('',#30745,#30857,#25098,.T.);
#38095=EDGE_CURVE('',#30858,#30859,#22504,.T.);
#38096=EDGE_CURVE('',#30464,#30859,#22505,.T.);
#38097=EDGE_CURVE('',#30858,#30745,#25099,.T.);
#38098=EDGE_CURVE('',#30860,#30858,#17809,.T.);
#38099=EDGE_CURVE('',#30861,#30860,#17810,.T.);
#38100=EDGE_CURVE('',#30859,#30861,#17811,.T.);
#38101=EDGE_CURVE('',#30746,#30861,#25100,.T.);
#38102=EDGE_CURVE('',#30862,#30863,#22506,.T.);
#38103=EDGE_CURVE('',#30465,#30863,#22507,.T.);
#38104=EDGE_CURVE('',#30862,#30746,#25101,.T.);
#38105=EDGE_CURVE('',#30864,#30862,#17812,.T.);
#38106=EDGE_CURVE('',#30865,#30864,#17813,.T.);
#38107=EDGE_CURVE('',#30863,#30865,#17814,.T.);
#38108=EDGE_CURVE('',#30747,#30865,#25102,.T.);
#38109=EDGE_CURVE('',#30866,#30867,#22508,.T.);
#38110=EDGE_CURVE('',#30466,#30867,#22509,.T.);
#38111=EDGE_CURVE('',#30866,#30747,#25103,.T.);
#38112=EDGE_CURVE('',#30867,#30868,#17815,.T.);
#38113=EDGE_CURVE('',#30748,#30868,#25104,.T.);
#38114=EDGE_CURVE('',#30869,#30866,#17816,.T.);
#38115=EDGE_CURVE('',#30868,#30869,#17817,.T.);
#38116=EDGE_CURVE('',#30870,#30748,#25105,.T.);
#38117=EDGE_CURVE('',#30870,#30871,#22510,.T.);
#38118=EDGE_CURVE('',#30467,#30871,#22511,.T.);
#38119=EDGE_CURVE('',#30871,#30872,#17818,.T.);
#38120=EDGE_CURVE('',#30873,#30870,#17819,.T.);
#38121=EDGE_CURVE('',#30872,#30873,#17820,.T.);
#38122=EDGE_CURVE('',#30749,#30872,#25106,.T.);
#38123=EDGE_CURVE('',#30874,#30875,#22512,.T.);
#38124=EDGE_CURVE('',#30468,#30875,#22513,.T.);
#38125=EDGE_CURVE('',#30874,#30749,#25107,.T.);
#38126=EDGE_CURVE('',#30876,#30874,#17821,.T.);
#38127=EDGE_CURVE('',#30877,#30876,#17822,.T.);
#38128=EDGE_CURVE('',#30875,#30877,#17823,.T.);
#38129=EDGE_CURVE('',#30750,#30877,#25108,.T.);
#38130=EDGE_CURVE('',#30878,#30879,#22514,.T.);
#38131=EDGE_CURVE('',#30469,#30879,#22515,.T.);
#38132=EDGE_CURVE('',#30878,#30750,#25109,.T.);
#38133=EDGE_CURVE('',#30880,#30878,#17824,.T.);
#38134=EDGE_CURVE('',#30881,#30880,#17825,.T.);
#38135=EDGE_CURVE('',#30879,#30881,#17826,.T.);
#38136=EDGE_CURVE('',#30751,#30881,#25110,.T.);
#38137=EDGE_CURVE('',#30882,#30883,#22516,.T.);
#38138=EDGE_CURVE('',#30470,#30883,#22517,.T.);
#38139=EDGE_CURVE('',#30882,#30751,#25111,.T.);
#38140=EDGE_CURVE('',#30884,#30882,#17827,.T.);
#38141=EDGE_CURVE('',#30885,#30884,#17828,.T.);
#38142=EDGE_CURVE('',#30883,#30885,#17829,.T.);
#38143=EDGE_CURVE('',#30752,#30885,#25112,.T.);
#38144=EDGE_CURVE('',#30886,#30887,#22518,.T.);
#38145=EDGE_CURVE('',#30471,#30887,#22519,.T.);
#38146=EDGE_CURVE('',#30886,#30752,#25113,.T.);
#38147=EDGE_CURVE('',#30888,#30886,#17830,.T.);
#38148=EDGE_CURVE('',#30889,#30888,#17831,.T.);
#38149=EDGE_CURVE('',#30887,#30889,#17832,.T.);
#38150=EDGE_CURVE('',#30753,#30889,#25114,.T.);
#38151=EDGE_CURVE('',#30890,#30891,#22520,.T.);
#38152=EDGE_CURVE('',#30472,#30891,#22521,.T.);
#38153=EDGE_CURVE('',#30890,#30753,#25115,.T.);
#38154=EDGE_CURVE('',#30892,#30890,#17833,.T.);
#38155=EDGE_CURVE('',#30893,#30892,#17834,.T.);
#38156=EDGE_CURVE('',#30891,#30893,#17835,.T.);
#38157=EDGE_CURVE('',#30754,#30893,#25116,.T.);
#38158=EDGE_CURVE('',#30894,#30895,#17836,.T.);
#38159=EDGE_CURVE('',#30785,#30894,#17837,.T.);
#38160=EDGE_CURVE('',#30895,#30784,#22522,.T.);
#38161=EDGE_CURVE('',#30895,#30754,#25117,.T.);
#38162=EDGE_CURVE('',#30896,#30473,#22523,.T.);
#38163=EDGE_CURVE('',#30896,#30897,#17838,.T.);
#38164=EDGE_CURVE('',#30755,#30897,#25118,.T.);
#38165=EDGE_CURVE('',#30898,#30755,#25119,.T.);
#38166=EDGE_CURVE('',#30898,#30899,#22524,.T.);
#38167=EDGE_CURVE('',#30474,#30899,#22525,.T.);
#38168=EDGE_CURVE('',#30899,#30900,#17839,.T.);
#38169=EDGE_CURVE('',#30756,#30900,#25120,.T.);
#38170=EDGE_CURVE('',#30901,#30898,#17840,.T.);
#38171=EDGE_CURVE('',#30900,#30901,#17841,.T.);
#38172=EDGE_CURVE('',#30902,#30756,#25121,.T.);
#38173=EDGE_CURVE('',#30902,#30903,#22526,.T.);
#38174=EDGE_CURVE('',#30475,#30903,#22527,.T.);
#38175=EDGE_CURVE('',#30903,#30904,#17842,.T.);
#38176=EDGE_CURVE('',#30757,#30904,#25122,.T.);
#38177=EDGE_CURVE('',#30905,#30902,#17843,.T.);
#38178=EDGE_CURVE('',#30904,#30905,#17844,.T.);
#38179=EDGE_CURVE('',#30906,#30757,#25123,.T.);
#38180=EDGE_CURVE('',#30906,#30907,#22528,.T.);
#38181=EDGE_CURVE('',#30476,#30907,#22529,.T.);
#38182=EDGE_CURVE('',#30907,#30908,#17845,.T.);
#38183=EDGE_CURVE('',#30758,#30908,#25124,.T.);
#38184=EDGE_CURVE('',#30909,#30906,#17846,.T.);
#38185=EDGE_CURVE('',#30908,#30909,#17847,.T.);
#38186=EDGE_CURVE('',#30910,#30758,#25125,.T.);
#38187=EDGE_CURVE('',#30910,#30911,#22530,.T.);
#38188=EDGE_CURVE('',#30477,#30911,#22531,.T.);
#38189=EDGE_CURVE('',#30911,#30912,#17848,.T.);
#38190=EDGE_CURVE('',#30759,#30912,#25126,.T.);
#38191=EDGE_CURVE('',#30913,#30910,#17849,.T.);
#38192=EDGE_CURVE('',#30912,#30913,#17850,.T.);
#38193=EDGE_CURVE('',#30914,#30759,#25127,.T.);
#38194=EDGE_CURVE('',#30914,#30915,#22532,.T.);
#38195=EDGE_CURVE('',#30478,#30915,#22533,.T.);
#38196=EDGE_CURVE('',#30915,#30916,#17851,.T.);
#38197=EDGE_CURVE('',#30760,#30916,#25128,.T.);
#38198=EDGE_CURVE('',#30917,#30914,#17852,.T.);
#38199=EDGE_CURVE('',#30916,#30917,#17853,.T.);
#38200=EDGE_CURVE('',#30918,#30760,#25129,.T.);
#38201=EDGE_CURVE('',#30918,#30919,#22534,.T.);
#38202=EDGE_CURVE('',#30479,#30919,#22535,.T.);
#38203=EDGE_CURVE('',#30919,#30920,#17854,.T.);
#38204=EDGE_CURVE('',#30761,#30920,#25130,.T.);
#38205=EDGE_CURVE('',#30921,#30918,#17855,.T.);
#38206=EDGE_CURVE('',#30920,#30921,#17856,.T.);
#38207=EDGE_CURVE('',#30922,#30761,#25131,.T.);
#38208=EDGE_CURVE('',#30922,#30923,#22536,.T.);
#38209=EDGE_CURVE('',#30480,#30923,#22537,.T.);
#38210=EDGE_CURVE('',#30923,#30924,#17857,.T.);
#38211=EDGE_CURVE('',#30762,#30924,#25132,.T.);
#38212=EDGE_CURVE('',#30925,#30922,#17858,.T.);
#38213=EDGE_CURVE('',#30924,#30925,#17859,.T.);
#38214=EDGE_CURVE('',#30926,#30762,#25133,.T.);
#38215=EDGE_CURVE('',#30926,#30927,#22538,.T.);
#38216=EDGE_CURVE('',#30481,#30927,#22539,.T.);
#38217=EDGE_CURVE('',#30927,#30928,#17860,.T.);
#38218=EDGE_CURVE('',#30763,#30928,#25134,.T.);
#38219=EDGE_CURVE('',#30929,#30926,#17861,.T.);
#38220=EDGE_CURVE('',#30928,#30929,#17862,.T.);
#38221=EDGE_CURVE('',#30930,#30763,#25135,.T.);
#38222=EDGE_CURVE('',#30930,#30931,#22540,.T.);
#38223=EDGE_CURVE('',#30482,#30931,#22541,.T.);
#38224=EDGE_CURVE('',#30931,#30932,#17863,.T.);
#38225=EDGE_CURVE('',#30764,#30932,#25136,.T.);
#38226=EDGE_CURVE('',#30933,#30930,#17864,.T.);
#38227=EDGE_CURVE('',#30932,#30933,#17865,.T.);
#38228=EDGE_CURVE('',#30934,#30764,#25137,.T.);
#38229=EDGE_CURVE('',#30934,#30935,#22542,.T.);
#38230=EDGE_CURVE('',#30483,#30935,#22543,.T.);
#38231=EDGE_CURVE('',#30935,#30936,#17866,.T.);
#38232=EDGE_CURVE('',#30765,#30936,#25138,.T.);
#38233=EDGE_CURVE('',#30937,#30934,#17867,.T.);
#38234=EDGE_CURVE('',#30936,#30937,#17868,.T.);
#38235=EDGE_CURVE('',#30938,#30765,#25139,.T.);
#38236=EDGE_CURVE('',#30938,#30939,#22544,.T.);
#38237=EDGE_CURVE('',#30484,#30939,#22545,.T.);
#38238=EDGE_CURVE('',#30939,#30940,#17869,.T.);
#38239=EDGE_CURVE('',#30766,#30940,#25140,.T.);
#38240=EDGE_CURVE('',#30941,#30938,#17870,.T.);
#38241=EDGE_CURVE('',#30940,#30941,#17871,.T.);
#38242=EDGE_CURVE('',#30942,#30766,#25141,.T.);
#38243=EDGE_CURVE('',#30942,#30943,#22546,.T.);
#38244=EDGE_CURVE('',#30485,#30943,#22547,.T.);
#38245=EDGE_CURVE('',#30943,#30944,#17872,.T.);
#38246=EDGE_CURVE('',#30767,#30944,#25142,.T.);
#38247=EDGE_CURVE('',#30945,#30942,#17873,.T.);
#38248=EDGE_CURVE('',#30944,#30945,#17874,.T.);
#38249=EDGE_CURVE('',#30946,#30767,#25143,.T.);
#38250=EDGE_CURVE('',#30946,#30947,#22548,.T.);
#38251=EDGE_CURVE('',#30486,#30947,#22549,.T.);
#38252=EDGE_CURVE('',#30947,#30948,#17875,.T.);
#38253=EDGE_CURVE('',#30768,#30948,#25144,.T.);
#38254=EDGE_CURVE('',#30949,#30946,#17876,.T.);
#38255=EDGE_CURVE('',#30948,#30949,#17877,.T.);
#38256=EDGE_CURVE('',#28981,#30768,#25145,.T.);
#38257=EDGE_CURVE('',#30487,#28980,#22550,.T.);
#38258=EDGE_CURVE('',#30769,#28978,#25146,.T.);
#38259=EDGE_CURVE('',#30950,#30769,#25147,.T.);
#38260=EDGE_CURVE('',#30950,#30951,#22551,.T.);
#38261=EDGE_CURVE('',#30488,#30951,#22552,.T.);
#38262=EDGE_CURVE('',#30951,#30952,#17878,.T.);
#38263=EDGE_CURVE('',#30770,#30952,#25148,.T.);
#38264=EDGE_CURVE('',#30953,#30950,#17879,.T.);
#38265=EDGE_CURVE('',#30952,#30953,#17880,.T.);
#38266=EDGE_CURVE('',#30954,#30770,#25149,.T.);
#38267=EDGE_CURVE('',#30954,#30955,#22553,.T.);
#38268=EDGE_CURVE('',#30489,#30955,#22554,.T.);
#38269=EDGE_CURVE('',#30955,#30956,#17881,.T.);
#38270=EDGE_CURVE('',#30771,#30956,#25150,.T.);
#38271=EDGE_CURVE('',#30957,#30954,#17882,.T.);
#38272=EDGE_CURVE('',#30956,#30957,#17883,.T.);
#38273=EDGE_CURVE('',#30958,#30771,#25151,.T.);
#38274=EDGE_CURVE('',#30958,#30959,#22555,.T.);
#38275=EDGE_CURVE('',#30490,#30959,#22556,.T.);
#38276=EDGE_CURVE('',#30959,#30960,#17884,.T.);
#38277=EDGE_CURVE('',#30772,#30960,#25152,.T.);
#38278=EDGE_CURVE('',#30961,#30958,#17885,.T.);
#38279=EDGE_CURVE('',#30960,#30961,#17886,.T.);
#38280=EDGE_CURVE('',#30962,#30772,#25153,.T.);
#38281=EDGE_CURVE('',#30962,#30963,#22557,.T.);
#38282=EDGE_CURVE('',#30491,#30963,#22558,.T.);
#38283=EDGE_CURVE('',#30963,#30964,#17887,.T.);
#38284=EDGE_CURVE('',#30773,#30964,#25154,.T.);
#38285=EDGE_CURVE('',#30965,#30962,#17888,.T.);
#38286=EDGE_CURVE('',#30964,#30965,#17889,.T.);
#38287=EDGE_CURVE('',#30966,#30773,#25155,.T.);
#38288=EDGE_CURVE('',#30966,#30967,#22559,.T.);
#38289=EDGE_CURVE('',#30492,#30967,#22560,.T.);
#38290=EDGE_CURVE('',#30967,#30968,#17890,.T.);
#38291=EDGE_CURVE('',#30774,#30968,#25156,.T.);
#38292=EDGE_CURVE('',#30969,#30966,#17891,.T.);
#38293=EDGE_CURVE('',#30968,#30969,#17892,.T.);
#38294=EDGE_CURVE('',#30970,#30774,#25157,.T.);
#38295=EDGE_CURVE('',#30970,#30971,#22561,.T.);
#38296=EDGE_CURVE('',#30493,#30971,#22562,.T.);
#38297=EDGE_CURVE('',#30971,#30972,#17893,.T.);
#38298=EDGE_CURVE('',#30775,#30972,#25158,.T.);
#38299=EDGE_CURVE('',#30973,#30970,#17894,.T.);
#38300=EDGE_CURVE('',#30972,#30973,#17895,.T.);
#38301=EDGE_CURVE('',#30974,#30775,#25159,.T.);
#38302=EDGE_CURVE('',#30974,#30975,#22563,.T.);
#38303=EDGE_CURVE('',#30494,#30975,#22564,.T.);
#38304=EDGE_CURVE('',#30975,#30976,#17896,.T.);
#38305=EDGE_CURVE('',#30776,#30976,#25160,.T.);
#38306=EDGE_CURVE('',#30977,#30974,#17897,.T.);
#38307=EDGE_CURVE('',#30976,#30977,#17898,.T.);
#38308=EDGE_CURVE('',#30978,#30776,#25161,.T.);
#38309=EDGE_CURVE('',#30978,#30979,#22565,.T.);
#38310=EDGE_CURVE('',#30495,#30979,#22566,.T.);
#38311=EDGE_CURVE('',#30979,#30980,#17899,.T.);
#38312=EDGE_CURVE('',#30777,#30980,#25162,.T.);
#38313=EDGE_CURVE('',#30981,#30978,#17900,.T.);
#38314=EDGE_CURVE('',#30980,#30981,#17901,.T.);
#38315=EDGE_CURVE('',#30982,#30777,#25163,.T.);
#38316=EDGE_CURVE('',#30982,#30983,#22567,.T.);
#38317=EDGE_CURVE('',#30496,#30983,#22568,.T.);
#38318=EDGE_CURVE('',#30983,#30984,#17902,.T.);
#38319=EDGE_CURVE('',#30778,#30984,#25164,.T.);
#38320=EDGE_CURVE('',#30985,#30982,#17903,.T.);
#38321=EDGE_CURVE('',#30984,#30985,#17904,.T.);
#38322=EDGE_CURVE('',#30986,#30778,#25165,.T.);
#38323=EDGE_CURVE('',#30986,#30987,#22569,.T.);
#38324=EDGE_CURVE('',#30497,#30987,#22570,.T.);
#38325=EDGE_CURVE('',#30987,#30988,#17905,.T.);
#38326=EDGE_CURVE('',#30779,#30988,#25166,.T.);
#38327=EDGE_CURVE('',#30989,#30986,#17906,.T.);
#38328=EDGE_CURVE('',#30988,#30989,#17907,.T.);
#38329=EDGE_CURVE('',#30990,#30779,#25167,.T.);
#38330=EDGE_CURVE('',#30990,#30991,#22571,.T.);
#38331=EDGE_CURVE('',#30498,#30991,#22572,.T.);
#38332=EDGE_CURVE('',#30991,#30992,#17908,.T.);
#38333=EDGE_CURVE('',#30780,#30992,#25168,.T.);
#38334=EDGE_CURVE('',#30993,#30990,#17909,.T.);
#38335=EDGE_CURVE('',#30992,#30993,#17910,.T.);
#38336=EDGE_CURVE('',#30994,#30780,#25169,.T.);
#38337=EDGE_CURVE('',#30994,#30995,#22573,.T.);
#38338=EDGE_CURVE('',#30499,#30995,#22574,.T.);
#38339=EDGE_CURVE('',#30995,#30996,#17911,.T.);
#38340=EDGE_CURVE('',#30781,#30996,#25170,.T.);
#38341=EDGE_CURVE('',#30997,#30994,#17912,.T.);
#38342=EDGE_CURVE('',#30996,#30997,#17913,.T.);
#38343=EDGE_CURVE('',#30998,#30781,#25171,.T.);
#38344=EDGE_CURVE('',#30998,#30999,#22575,.T.);
#38345=EDGE_CURVE('',#30500,#30999,#22576,.T.);
#38346=EDGE_CURVE('',#30999,#31000,#17914,.T.);
#38347=EDGE_CURVE('',#30782,#31000,#25172,.T.);
#38348=EDGE_CURVE('',#31001,#30998,#17915,.T.);
#38349=EDGE_CURVE('',#31000,#31001,#17916,.T.);
#38350=EDGE_CURVE('',#31002,#30782,#25173,.T.);
#38351=EDGE_CURVE('',#31002,#31003,#22577,.T.);
#38352=EDGE_CURVE('',#30501,#31003,#22578,.T.);
#38353=EDGE_CURVE('',#31003,#31004,#17917,.T.);
#38354=EDGE_CURVE('',#30783,#31004,#25174,.T.);
#38355=EDGE_CURVE('',#31005,#31002,#17918,.T.);
#38356=EDGE_CURVE('',#31004,#31005,#17919,.T.);
#38357=EDGE_CURVE('',#31006,#30896,#22579,.T.);
#38358=EDGE_CURVE('',#31007,#31006,#17920,.T.);
#38359=EDGE_CURVE('',#30897,#31007,#17921,.T.);
#38360=EDGE_CURVE('',#31006,#30783,#25175,.T.);
#38361=EDGE_CURVE('',#30726,#31008,#17922,.T.);
#38362=EDGE_CURVE('',#31008,#30894,#22580,.T.);
#38363=EDGE_CURVE('',#31009,#30726,#17923,.T.);
#38364=EDGE_CURVE('',#30788,#31009,#22581,.T.);
#38365=EDGE_CURVE('',#30727,#31009,#17924,.T.);
#38366=EDGE_CURVE('',#31010,#30727,#17925,.T.);
#38367=EDGE_CURVE('',#30792,#31010,#22582,.T.);
#38368=EDGE_CURVE('',#30728,#31010,#17926,.T.);
#38369=EDGE_CURVE('',#31011,#30728,#17927,.T.);
#38370=EDGE_CURVE('',#30796,#31011,#22583,.T.);
#38371=EDGE_CURVE('',#30729,#31011,#17928,.T.);
#38372=EDGE_CURVE('',#31012,#30729,#17929,.T.);
#38373=EDGE_CURVE('',#30800,#31012,#22584,.T.);
#38374=EDGE_CURVE('',#30730,#31012,#17930,.T.);
#38375=EDGE_CURVE('',#31013,#30730,#17931,.T.);
#38376=EDGE_CURVE('',#30804,#31013,#22585,.T.);
#38377=EDGE_CURVE('',#30731,#31013,#17932,.T.);
#38378=EDGE_CURVE('',#31014,#30731,#17933,.T.);
#38379=EDGE_CURVE('',#30808,#31014,#22586,.T.);
#38380=EDGE_CURVE('',#30732,#31014,#17934,.T.);
#38381=EDGE_CURVE('',#31015,#30732,#17935,.T.);
#38382=EDGE_CURVE('',#28985,#31015,#22587,.T.);
#38383=EDGE_CURVE('',#30733,#31015,#17936,.T.);
#38384=EDGE_CURVE('',#31016,#30733,#17937,.T.);
#38385=EDGE_CURVE('',#30812,#31016,#22588,.T.);
#38386=EDGE_CURVE('',#30734,#31016,#17938,.T.);
#38387=EDGE_CURVE('',#31017,#30734,#17939,.T.);
#38388=EDGE_CURVE('',#30816,#31017,#22589,.T.);
#38389=EDGE_CURVE('',#30735,#31017,#17940,.T.);
#38390=EDGE_CURVE('',#31018,#30735,#17941,.T.);
#38391=EDGE_CURVE('',#30820,#31018,#22590,.T.);
#38392=EDGE_CURVE('',#30736,#31018,#17942,.T.);
#38393=EDGE_CURVE('',#31019,#30736,#17943,.T.);
#38394=EDGE_CURVE('',#30824,#31019,#22591,.T.);
#38395=EDGE_CURVE('',#30737,#31019,#17944,.T.);
#38396=EDGE_CURVE('',#31020,#30737,#17945,.T.);
#38397=EDGE_CURVE('',#30828,#31020,#22592,.T.);
#38398=EDGE_CURVE('',#30738,#31020,#17946,.T.);
#38399=EDGE_CURVE('',#31021,#30738,#17947,.T.);
#38400=EDGE_CURVE('',#30832,#31021,#22593,.T.);
#38401=EDGE_CURVE('',#30739,#31021,#17948,.T.);
#38402=EDGE_CURVE('',#31022,#30739,#17949,.T.);
#38403=EDGE_CURVE('',#30836,#31022,#22594,.T.);
#38404=EDGE_CURVE('',#30740,#31022,#17950,.T.);
#38405=EDGE_CURVE('',#31023,#30740,#17951,.T.);
#38406=EDGE_CURVE('',#30840,#31023,#22595,.T.);
#38407=EDGE_CURVE('',#30741,#31023,#17952,.T.);
#38408=EDGE_CURVE('',#31024,#30741,#17953,.T.);
#38409=EDGE_CURVE('',#30844,#31024,#22596,.T.);
#38410=EDGE_CURVE('',#30742,#31024,#17954,.T.);
#38411=EDGE_CURVE('',#31025,#30742,#17955,.T.);
#38412=EDGE_CURVE('',#30848,#31025,#22597,.T.);
#38413=EDGE_CURVE('',#30743,#31025,#17956,.T.);
#38414=EDGE_CURVE('',#31026,#30743,#17957,.T.);
#38415=EDGE_CURVE('',#30852,#31026,#22598,.T.);
#38416=EDGE_CURVE('',#30744,#31026,#17958,.T.);
#38417=EDGE_CURVE('',#31027,#30744,#17959,.T.);
#38418=EDGE_CURVE('',#30856,#31027,#22599,.T.);
#38419=EDGE_CURVE('',#30745,#31027,#17960,.T.);
#38420=EDGE_CURVE('',#31028,#30745,#17961,.T.);
#38421=EDGE_CURVE('',#30860,#31028,#22600,.T.);
#38422=EDGE_CURVE('',#30746,#31028,#17962,.T.);
#38423=EDGE_CURVE('',#31029,#30746,#17963,.T.);
#38424=EDGE_CURVE('',#30864,#31029,#22601,.T.);
#38425=EDGE_CURVE('',#30747,#31029,#17964,.T.);
#38426=EDGE_CURVE('',#31030,#30747,#17965,.T.);
#38427=EDGE_CURVE('',#30869,#31030,#22602,.T.);
#38428=EDGE_CURVE('',#30748,#31030,#17966,.T.);
#38429=EDGE_CURVE('',#31031,#30748,#17967,.T.);
#38430=EDGE_CURVE('',#30873,#31031,#22603,.T.);
#38431=EDGE_CURVE('',#30749,#31031,#17968,.T.);
#38432=EDGE_CURVE('',#31032,#30749,#17969,.T.);
#38433=EDGE_CURVE('',#30876,#31032,#22604,.T.);
#38434=EDGE_CURVE('',#30750,#31032,#17970,.T.);
#38435=EDGE_CURVE('',#31033,#30750,#17971,.T.);
#38436=EDGE_CURVE('',#30880,#31033,#22605,.T.);
#38437=EDGE_CURVE('',#30751,#31033,#17972,.T.);
#38438=EDGE_CURVE('',#31034,#30751,#17973,.T.);
#38439=EDGE_CURVE('',#30884,#31034,#22606,.T.);
#38440=EDGE_CURVE('',#30752,#31034,#17974,.T.);
#38441=EDGE_CURVE('',#31035,#30752,#17975,.T.);
#38442=EDGE_CURVE('',#30888,#31035,#22607,.T.);
#38443=EDGE_CURVE('',#30753,#31035,#17976,.T.);
#38444=EDGE_CURVE('',#31036,#30753,#17977,.T.);
#38445=EDGE_CURVE('',#30892,#31036,#22608,.T.);
#38446=EDGE_CURVE('',#30754,#31036,#17978,.T.);
#38447=EDGE_CURVE('',#31008,#30754,#17979,.T.);
#38448=EDGE_CURVE('',#31037,#31007,#22609,.T.);
#38449=EDGE_CURVE('',#30755,#31037,#17980,.T.);
#38450=EDGE_CURVE('',#31038,#30755,#22610,.T.);
#38451=EDGE_CURVE('',#30901,#31038,#22611,.T.);
#38452=EDGE_CURVE('',#30756,#31038,#17981,.T.);
#38453=EDGE_CURVE('',#31039,#30756,#4426,.T.);
#38454=EDGE_CURVE('',#30905,#31039,#22612,.T.);
#38455=EDGE_CURVE('',#30757,#31039,#17982,.T.);
#38456=EDGE_CURVE('',#31040,#30757,#4427,.T.);
#38457=EDGE_CURVE('',#30909,#31040,#22613,.T.);
#38458=EDGE_CURVE('',#30758,#31040,#17983,.T.);
#38459=EDGE_CURVE('',#31041,#30758,#22614,.T.);
#38460=EDGE_CURVE('',#30913,#31041,#22615,.T.);
#38461=EDGE_CURVE('',#30759,#31041,#17984,.T.);
#38462=EDGE_CURVE('',#31042,#30759,#22616,.T.);
#38463=EDGE_CURVE('',#30917,#31042,#22617,.T.);
#38464=EDGE_CURVE('',#30760,#31042,#17985,.T.);
#38465=EDGE_CURVE('',#31043,#30760,#4428,.T.);
#38466=EDGE_CURVE('',#30921,#31043,#22618,.T.);
#38467=EDGE_CURVE('',#30761,#31043,#17986,.T.);
#38468=EDGE_CURVE('',#31044,#30761,#4429,.T.);
#38469=EDGE_CURVE('',#30925,#31044,#22619,.T.);
#38470=EDGE_CURVE('',#30762,#31044,#17987,.T.);
#38471=EDGE_CURVE('',#31045,#30762,#4430,.T.);
#38472=EDGE_CURVE('',#30929,#31045,#22620,.T.);
#38473=EDGE_CURVE('',#30763,#31045,#17988,.T.);
#38474=EDGE_CURVE('',#31046,#30763,#4431,.T.);
#38475=EDGE_CURVE('',#30933,#31046,#22621,.T.);
#38476=EDGE_CURVE('',#30764,#31046,#17989,.T.);
#38477=EDGE_CURVE('',#31047,#30764,#22622,.T.);
#38478=EDGE_CURVE('',#30937,#31047,#22623,.T.);
#38479=EDGE_CURVE('',#30765,#31047,#17990,.T.);
#38480=EDGE_CURVE('',#31048,#30765,#4432,.T.);
#38481=EDGE_CURVE('',#30941,#31048,#22624,.T.);
#38482=EDGE_CURVE('',#30766,#31048,#17991,.T.);
#38483=EDGE_CURVE('',#31049,#30766,#4433,.T.);
#38484=EDGE_CURVE('',#30945,#31049,#22625,.T.);
#38485=EDGE_CURVE('',#30767,#31049,#17992,.T.);
#38486=EDGE_CURVE('',#31050,#30767,#4434,.T.);
#38487=EDGE_CURVE('',#30949,#31050,#22626,.T.);
#38488=EDGE_CURVE('',#30768,#31050,#17993,.T.);
#38489=EDGE_CURVE('',#31051,#30768,#22627,.T.);
#38490=EDGE_CURVE('',#28979,#31051,#22628,.T.);
#38491=EDGE_CURVE('',#30769,#31051,#17994,.T.);
#38492=EDGE_CURVE('',#31052,#30769,#22629,.T.);
#38493=EDGE_CURVE('',#30953,#31052,#22630,.T.);
#38494=EDGE_CURVE('',#30770,#31052,#17995,.T.);
#38495=EDGE_CURVE('',#31053,#30770,#22631,.T.);
#38496=EDGE_CURVE('',#30957,#31053,#22632,.T.);
#38497=EDGE_CURVE('',#30771,#31053,#17996,.T.);
#38498=EDGE_CURVE('',#31054,#30771,#4435,.T.);
#38499=EDGE_CURVE('',#30961,#31054,#22633,.T.);
#38500=EDGE_CURVE('',#30772,#31054,#17997,.T.);
#38501=EDGE_CURVE('',#31055,#30772,#4436,.T.);
#38502=EDGE_CURVE('',#30965,#31055,#22634,.T.);
#38503=EDGE_CURVE('',#30773,#31055,#17998,.T.);
#38504=EDGE_CURVE('',#31056,#30773,#22635,.T.);
#38505=EDGE_CURVE('',#30969,#31056,#22636,.T.);
#38506=EDGE_CURVE('',#30774,#31056,#17999,.T.);
#38507=EDGE_CURVE('',#31057,#30774,#4437,.T.);
#38508=EDGE_CURVE('',#30973,#31057,#22637,.T.);
#38509=EDGE_CURVE('',#30775,#31057,#18000,.T.);
#38510=EDGE_CURVE('',#31058,#30775,#4438,.T.);
#38511=EDGE_CURVE('',#30977,#31058,#22638,.T.);
#38512=EDGE_CURVE('',#30776,#31058,#18001,.T.);
#38513=EDGE_CURVE('',#31059,#30776,#22639,.T.);
#38514=EDGE_CURVE('',#30981,#31059,#22640,.T.);
#38515=EDGE_CURVE('',#30777,#31059,#18002,.T.);
#38516=EDGE_CURVE('',#31060,#30777,#22641,.T.);
#38517=EDGE_CURVE('',#30985,#31060,#22642,.T.);
#38518=EDGE_CURVE('',#30778,#31060,#18003,.T.);
#38519=EDGE_CURVE('',#31061,#30778,#4439,.T.);
#38520=EDGE_CURVE('',#30989,#31061,#22643,.T.);
#38521=EDGE_CURVE('',#30779,#31061,#18004,.T.);
#38522=EDGE_CURVE('',#31062,#30779,#4440,.T.);
#38523=EDGE_CURVE('',#30993,#31062,#22644,.T.);
#38524=EDGE_CURVE('',#30780,#31062,#18005,.T.);
#38525=EDGE_CURVE('',#31063,#30780,#4441,.T.);
#38526=EDGE_CURVE('',#30997,#31063,#22645,.T.);
#38527=EDGE_CURVE('',#30781,#31063,#18006,.T.);
#38528=EDGE_CURVE('',#31064,#30781,#22646,.T.);
#38529=EDGE_CURVE('',#31001,#31064,#22647,.T.);
#38530=EDGE_CURVE('',#30782,#31064,#18007,.T.);
#38531=EDGE_CURVE('',#31065,#30782,#22648,.T.);
#38532=EDGE_CURVE('',#31005,#31065,#22649,.T.);
#38533=EDGE_CURVE('',#30783,#31065,#18008,.T.);
#38534=EDGE_CURVE('',#31037,#30783,#22650,.T.);
#38535=EDGE_CURVE('',#31066,#31067,#18009,.T.);
#38536=EDGE_CURVE('',#30726,#31067,#22651,.T.);
#38537=EDGE_CURVE('',#31066,#31008,#25176,.T.);
#38538=EDGE_CURVE('',#31068,#31066,#18010,.T.);
#38539=EDGE_CURVE('',#31069,#31068,#18011,.T.);
#38540=EDGE_CURVE('',#31067,#31069,#18012,.T.);
#38541=EDGE_CURVE('',#31009,#31069,#25177,.T.);
#38542=EDGE_CURVE('',#31070,#31071,#18013,.T.);
#38543=EDGE_CURVE('',#30727,#31071,#22652,.T.);
#38544=EDGE_CURVE('',#31070,#31009,#25178,.T.);
#38545=EDGE_CURVE('',#31072,#31070,#18014,.T.);
#38546=EDGE_CURVE('',#31073,#31072,#18015,.T.);
#38547=EDGE_CURVE('',#31071,#31073,#18016,.T.);
#38548=EDGE_CURVE('',#31010,#31073,#25179,.T.);
#38549=EDGE_CURVE('',#31074,#31075,#18017,.T.);
#38550=EDGE_CURVE('',#30728,#31075,#22653,.T.);
#38551=EDGE_CURVE('',#31074,#31010,#25180,.T.);
#38552=EDGE_CURVE('',#31076,#31074,#18018,.T.);
#38553=EDGE_CURVE('',#31077,#31076,#18019,.T.);
#38554=EDGE_CURVE('',#31075,#31077,#18020,.T.);
#38555=EDGE_CURVE('',#31011,#31077,#25181,.T.);
#38556=EDGE_CURVE('',#31078,#31079,#18021,.T.);
#38557=EDGE_CURVE('',#30729,#31079,#22654,.T.);
#38558=EDGE_CURVE('',#31078,#31011,#25182,.T.);
#38559=EDGE_CURVE('',#31080,#31078,#18022,.T.);
#38560=EDGE_CURVE('',#31081,#31080,#18023,.T.);
#38561=EDGE_CURVE('',#31079,#31081,#18024,.T.);
#38562=EDGE_CURVE('',#31012,#31081,#25183,.T.);
#38563=EDGE_CURVE('',#31082,#31083,#18025,.T.);
#38564=EDGE_CURVE('',#30730,#31083,#22655,.T.);
#38565=EDGE_CURVE('',#31082,#31012,#25184,.T.);
#38566=EDGE_CURVE('',#31084,#31082,#18026,.T.);
#38567=EDGE_CURVE('',#31085,#31084,#18027,.T.);
#38568=EDGE_CURVE('',#31083,#31085,#18028,.T.);
#38569=EDGE_CURVE('',#31013,#31085,#25185,.T.);
#38570=EDGE_CURVE('',#31086,#31087,#18029,.T.);
#38571=EDGE_CURVE('',#30731,#31087,#22656,.T.);
#38572=EDGE_CURVE('',#31086,#31013,#25186,.T.);
#38573=EDGE_CURVE('',#31088,#31086,#18030,.T.);
#38574=EDGE_CURVE('',#31089,#31088,#18031,.T.);
#38575=EDGE_CURVE('',#31087,#31089,#18032,.T.);
#38576=EDGE_CURVE('',#31014,#31089,#25187,.T.);
#38577=EDGE_CURVE('',#31090,#31091,#18033,.T.);
#38578=EDGE_CURVE('',#30732,#31091,#22657,.T.);
#38579=EDGE_CURVE('',#31090,#31014,#25188,.T.);
#38580=EDGE_CURVE('',#31092,#31090,#18034,.T.);
#38581=EDGE_CURVE('',#31093,#31092,#18035,.T.);
#38582=EDGE_CURVE('',#31091,#31093,#18036,.T.);
#38583=EDGE_CURVE('',#31015,#31093,#25189,.T.);
#38584=EDGE_CURVE('',#31094,#31095,#18037,.T.);
#38585=EDGE_CURVE('',#30733,#31095,#22658,.T.);
#38586=EDGE_CURVE('',#31094,#31015,#25190,.T.);
#38587=EDGE_CURVE('',#31096,#31094,#18038,.T.);
#38588=EDGE_CURVE('',#31097,#31096,#18039,.T.);
#38589=EDGE_CURVE('',#31095,#31097,#18040,.T.);
#38590=EDGE_CURVE('',#31016,#31097,#25191,.T.);
#38591=EDGE_CURVE('',#31098,#31099,#18041,.T.);
#38592=EDGE_CURVE('',#30734,#31099,#22659,.T.);
#38593=EDGE_CURVE('',#31098,#31016,#25192,.T.);
#38594=EDGE_CURVE('',#31100,#31098,#18042,.T.);
#38595=EDGE_CURVE('',#31101,#31100,#18043,.T.);
#38596=EDGE_CURVE('',#31099,#31101,#18044,.T.);
#38597=EDGE_CURVE('',#31017,#31101,#25193,.T.);
#38598=EDGE_CURVE('',#31102,#31103,#18045,.T.);
#38599=EDGE_CURVE('',#30735,#31103,#22660,.T.);
#38600=EDGE_CURVE('',#31102,#31017,#25194,.T.);
#38601=EDGE_CURVE('',#31104,#31102,#18046,.T.);
#38602=EDGE_CURVE('',#31105,#31104,#18047,.T.);
#38603=EDGE_CURVE('',#31103,#31105,#18048,.T.);
#38604=EDGE_CURVE('',#31018,#31105,#25195,.T.);
#38605=EDGE_CURVE('',#31106,#31107,#18049,.T.);
#38606=EDGE_CURVE('',#30736,#31107,#22661,.T.);
#38607=EDGE_CURVE('',#31106,#31018,#25196,.T.);
#38608=EDGE_CURVE('',#31108,#31106,#18050,.T.);
#38609=EDGE_CURVE('',#31109,#31108,#18051,.T.);
#38610=EDGE_CURVE('',#31107,#31109,#18052,.T.);
#38611=EDGE_CURVE('',#31019,#31109,#25197,.T.);
#38612=EDGE_CURVE('',#31110,#31111,#18053,.T.);
#38613=EDGE_CURVE('',#30737,#31111,#22662,.T.);
#38614=EDGE_CURVE('',#31110,#31019,#25198,.T.);
#38615=EDGE_CURVE('',#31112,#31110,#18054,.T.);
#38616=EDGE_CURVE('',#31113,#31112,#18055,.T.);
#38617=EDGE_CURVE('',#31111,#31113,#18056,.T.);
#38618=EDGE_CURVE('',#31020,#31113,#25199,.T.);
#38619=EDGE_CURVE('',#31114,#31115,#18057,.T.);
#38620=EDGE_CURVE('',#30738,#31115,#22663,.T.);
#38621=EDGE_CURVE('',#31114,#31020,#25200,.T.);
#38622=EDGE_CURVE('',#31116,#31114,#18058,.T.);
#38623=EDGE_CURVE('',#31117,#31116,#18059,.T.);
#38624=EDGE_CURVE('',#31115,#31117,#18060,.T.);
#38625=EDGE_CURVE('',#31021,#31117,#25201,.T.);
#38626=EDGE_CURVE('',#31118,#31119,#18061,.T.);
#38627=EDGE_CURVE('',#30739,#31119,#22664,.T.);
#38628=EDGE_CURVE('',#31118,#31021,#25202,.T.);
#38629=EDGE_CURVE('',#31120,#31118,#18062,.T.);
#38630=EDGE_CURVE('',#31121,#31120,#18063,.T.);
#38631=EDGE_CURVE('',#31119,#31121,#18064,.T.);
#38632=EDGE_CURVE('',#31022,#31121,#25203,.T.);
#38633=EDGE_CURVE('',#30740,#28975,#22665,.T.);
#38634=EDGE_CURVE('',#28974,#31022,#25204,.T.);
#38635=EDGE_CURVE('',#31023,#28977,#25205,.T.);
#38636=EDGE_CURVE('',#31122,#31123,#18065,.T.);
#38637=EDGE_CURVE('',#30741,#31123,#22666,.T.);
#38638=EDGE_CURVE('',#31122,#31023,#25206,.T.);
#38639=EDGE_CURVE('',#31124,#31122,#18066,.T.);
#38640=EDGE_CURVE('',#31125,#31124,#18067,.T.);
#38641=EDGE_CURVE('',#31123,#31125,#18068,.T.);
#38642=EDGE_CURVE('',#31024,#31125,#25207,.T.);
#38643=EDGE_CURVE('',#31126,#31127,#18069,.T.);
#38644=EDGE_CURVE('',#30742,#31127,#22667,.T.);
#38645=EDGE_CURVE('',#31126,#31024,#25208,.T.);
#38646=EDGE_CURVE('',#31128,#31126,#18070,.T.);
#38647=EDGE_CURVE('',#31129,#31128,#18071,.T.);
#38648=EDGE_CURVE('',#31127,#31129,#18072,.T.);
#38649=EDGE_CURVE('',#31025,#31129,#25209,.T.);
#38650=EDGE_CURVE('',#31130,#31131,#18073,.T.);
#38651=EDGE_CURVE('',#30743,#31131,#22668,.T.);
#38652=EDGE_CURVE('',#31130,#31025,#25210,.T.);
#38653=EDGE_CURVE('',#31132,#31130,#18074,.T.);
#38654=EDGE_CURVE('',#31133,#31132,#18075,.T.);
#38655=EDGE_CURVE('',#31131,#31133,#18076,.T.);
#38656=EDGE_CURVE('',#31026,#31133,#25211,.T.);
#38657=EDGE_CURVE('',#31134,#31135,#18077,.T.);
#38658=EDGE_CURVE('',#30744,#31135,#22669,.T.);
#38659=EDGE_CURVE('',#31134,#31026,#25212,.T.);
#38660=EDGE_CURVE('',#31136,#31134,#18078,.T.);
#38661=EDGE_CURVE('',#31137,#31136,#18079,.T.);
#38662=EDGE_CURVE('',#31135,#31137,#18080,.T.);
#38663=EDGE_CURVE('',#31027,#31137,#25213,.T.);
#38664=EDGE_CURVE('',#31138,#31139,#18081,.T.);
#38665=EDGE_CURVE('',#30745,#31139,#22670,.T.);
#38666=EDGE_CURVE('',#31138,#31027,#25214,.T.);
#38667=EDGE_CURVE('',#31140,#31138,#18082,.T.);
#38668=EDGE_CURVE('',#31141,#31140,#18083,.T.);
#38669=EDGE_CURVE('',#31139,#31141,#18084,.T.);
#38670=EDGE_CURVE('',#31028,#31141,#25215,.T.);
#38671=EDGE_CURVE('',#31142,#31143,#18085,.T.);
#38672=EDGE_CURVE('',#30746,#31143,#22671,.T.);
#38673=EDGE_CURVE('',#31142,#31028,#25216,.T.);
#38674=EDGE_CURVE('',#31144,#31142,#18086,.T.);
#38675=EDGE_CURVE('',#31145,#31144,#18087,.T.);
#38676=EDGE_CURVE('',#31143,#31145,#18088,.T.);
#38677=EDGE_CURVE('',#31029,#31145,#25217,.T.);
#38678=EDGE_CURVE('',#31146,#31147,#18089,.T.);
#38679=EDGE_CURVE('',#30747,#31147,#22672,.T.);
#38680=EDGE_CURVE('',#31146,#31029,#25218,.T.);
#38681=EDGE_CURVE('',#31147,#31148,#18090,.T.);
#38682=EDGE_CURVE('',#31030,#31148,#25219,.T.);
#38683=EDGE_CURVE('',#31149,#31146,#18091,.T.);
#38684=EDGE_CURVE('',#31148,#31149,#18092,.T.);
#38685=EDGE_CURVE('',#31150,#31030,#25220,.T.);
#38686=EDGE_CURVE('',#31150,#31151,#18093,.T.);
#38687=EDGE_CURVE('',#30748,#31151,#22673,.T.);
#38688=EDGE_CURVE('',#31151,#31152,#18094,.T.);
#38689=EDGE_CURVE('',#31153,#31150,#18095,.T.);
#38690=EDGE_CURVE('',#31152,#31153,#18096,.T.);
#38691=EDGE_CURVE('',#31031,#31152,#25221,.T.);
#38692=EDGE_CURVE('',#31154,#31155,#18097,.T.);
#38693=EDGE_CURVE('',#30749,#31155,#22674,.T.);
#38694=EDGE_CURVE('',#31154,#31031,#25222,.T.);
#38695=EDGE_CURVE('',#31156,#31154,#18098,.T.);
#38696=EDGE_CURVE('',#31157,#31156,#18099,.T.);
#38697=EDGE_CURVE('',#31155,#31157,#18100,.T.);
#38698=EDGE_CURVE('',#31032,#31157,#25223,.T.);
#38699=EDGE_CURVE('',#31158,#31159,#18101,.T.);
#38700=EDGE_CURVE('',#30750,#31159,#22675,.T.);
#38701=EDGE_CURVE('',#31158,#31032,#25224,.T.);
#38702=EDGE_CURVE('',#31160,#31158,#18102,.T.);
#38703=EDGE_CURVE('',#31161,#31160,#18103,.T.);
#38704=EDGE_CURVE('',#31159,#31161,#18104,.T.);
#38705=EDGE_CURVE('',#31033,#31161,#25225,.T.);
#38706=EDGE_CURVE('',#31162,#31163,#18105,.T.);
#38707=EDGE_CURVE('',#30751,#31163,#22676,.T.);
#38708=EDGE_CURVE('',#31162,#31033,#25226,.T.);
#38709=EDGE_CURVE('',#31164,#31162,#18106,.T.);
#38710=EDGE_CURVE('',#31165,#31164,#18107,.T.);
#38711=EDGE_CURVE('',#31163,#31165,#18108,.T.);
#38712=EDGE_CURVE('',#31034,#31165,#25227,.T.);
#38713=EDGE_CURVE('',#31166,#31167,#18109,.T.);
#38714=EDGE_CURVE('',#30752,#31167,#22677,.T.);
#38715=EDGE_CURVE('',#31166,#31034,#25228,.T.);
#38716=EDGE_CURVE('',#31168,#31166,#18110,.T.);
#38717=EDGE_CURVE('',#31169,#31168,#18111,.T.);
#38718=EDGE_CURVE('',#31167,#31169,#18112,.T.);
#38719=EDGE_CURVE('',#31035,#31169,#25229,.T.);
#38720=EDGE_CURVE('',#31170,#31171,#18113,.T.);
#38721=EDGE_CURVE('',#30753,#31171,#22678,.T.);
#38722=EDGE_CURVE('',#31170,#31035,#25230,.T.);
#38723=EDGE_CURVE('',#31172,#31170,#18114,.T.);
#38724=EDGE_CURVE('',#31173,#31172,#18115,.T.);
#38725=EDGE_CURVE('',#31171,#31173,#18116,.T.);
#38726=EDGE_CURVE('',#31036,#31173,#25231,.T.);
#38727=EDGE_CURVE('',#31174,#31175,#18117,.T.);
#38728=EDGE_CURVE('',#30754,#31175,#22679,.T.);
#38729=EDGE_CURVE('',#31174,#31036,#25232,.T.);
#38730=EDGE_CURVE('',#31176,#31174,#18118,.T.);
#38731=EDGE_CURVE('',#31177,#31176,#18119,.T.);
#38732=EDGE_CURVE('',#31175,#31177,#18120,.T.);
#38733=EDGE_CURVE('',#31008,#31177,#25233,.T.);
#38734=EDGE_CURVE('',#31178,#31037,#25234,.T.);
#38735=EDGE_CURVE('',#31178,#31179,#18121,.T.);
#38736=EDGE_CURVE('',#30755,#31179,#22680,.T.);
#38737=EDGE_CURVE('',#31179,#31180,#22681,.T.);
#38738=EDGE_CURVE('',#31038,#31180,#25235,.T.);
#38739=EDGE_CURVE('',#31181,#31178,#18122,.T.);
#38740=EDGE_CURVE('',#31180,#31181,#18123,.T.);
#38741=EDGE_CURVE('',#31182,#31038,#25236,.T.);
#38742=EDGE_CURVE('',#31182,#31183,#18124,.T.);
#38743=EDGE_CURVE('',#30756,#31183,#22682,.T.);
#38744=EDGE_CURVE('',#31183,#31184,#22683,.T.);
#38745=EDGE_CURVE('',#31039,#31184,#25237,.T.);
#38746=EDGE_CURVE('',#31185,#31182,#18125,.T.);
#38747=EDGE_CURVE('',#31184,#31185,#18126,.T.);
#38748=EDGE_CURVE('',#31186,#31039,#25238,.T.);
#38749=EDGE_CURVE('',#31186,#31187,#18127,.T.);
#38750=EDGE_CURVE('',#30757,#31187,#22684,.T.);
#38751=EDGE_CURVE('',#31187,#31188,#22685,.T.);
#38752=EDGE_CURVE('',#31040,#31188,#25239,.T.);
#38753=EDGE_CURVE('',#31189,#31186,#18128,.T.);
#38754=EDGE_CURVE('',#31188,#31189,#18129,.T.);
#38755=EDGE_CURVE('',#31190,#31040,#25240,.T.);
#38756=EDGE_CURVE('',#31190,#31191,#18130,.T.);
#38757=EDGE_CURVE('',#30758,#31191,#22686,.T.);
#38758=EDGE_CURVE('',#31191,#31192,#22687,.T.);
#38759=EDGE_CURVE('',#31041,#31192,#25241,.T.);
#38760=EDGE_CURVE('',#31193,#31190,#18131,.T.);
#38761=EDGE_CURVE('',#31192,#31193,#18132,.T.);
#38762=EDGE_CURVE('',#31194,#31041,#25242,.T.);
#38763=EDGE_CURVE('',#31194,#31195,#18133,.T.);
#38764=EDGE_CURVE('',#30759,#31195,#22688,.T.);
#38765=EDGE_CURVE('',#31195,#31196,#22689,.T.);
#38766=EDGE_CURVE('',#31042,#31196,#25243,.T.);
#38767=EDGE_CURVE('',#31197,#31194,#18134,.T.);
#38768=EDGE_CURVE('',#31196,#31197,#18135,.T.);
#38769=EDGE_CURVE('',#31198,#31042,#25244,.T.);
#38770=EDGE_CURVE('',#31198,#31199,#18136,.T.);
#38771=EDGE_CURVE('',#30760,#31199,#22690,.T.);
#38772=EDGE_CURVE('',#31199,#31200,#22691,.T.);
#38773=EDGE_CURVE('',#31043,#31200,#25245,.T.);
#38774=EDGE_CURVE('',#31201,#31198,#18137,.T.);
#38775=EDGE_CURVE('',#31200,#31201,#18138,.T.);
#38776=EDGE_CURVE('',#31202,#31043,#25246,.T.);
#38777=EDGE_CURVE('',#31202,#31203,#18139,.T.);
#38778=EDGE_CURVE('',#30761,#31203,#22692,.T.);
#38779=EDGE_CURVE('',#31203,#31204,#22693,.T.);
#38780=EDGE_CURVE('',#31044,#31204,#25247,.T.);
#38781=EDGE_CURVE('',#31205,#31202,#18140,.T.);
#38782=EDGE_CURVE('',#31204,#31205,#18141,.T.);
#38783=EDGE_CURVE('',#31206,#31044,#25248,.T.);
#38784=EDGE_CURVE('',#31206,#31207,#18142,.T.);
#38785=EDGE_CURVE('',#30762,#31207,#22694,.T.);
#38786=EDGE_CURVE('',#31207,#31208,#22695,.T.);
#38787=EDGE_CURVE('',#31045,#31208,#25249,.T.);
#38788=EDGE_CURVE('',#31209,#31206,#18143,.T.);
#38789=EDGE_CURVE('',#31208,#31209,#18144,.T.);
#38790=EDGE_CURVE('',#31210,#31045,#25250,.T.);
#38791=EDGE_CURVE('',#31210,#31211,#18145,.T.);
#38792=EDGE_CURVE('',#30763,#31211,#22696,.T.);
#38793=EDGE_CURVE('',#31211,#31212,#22697,.T.);
#38794=EDGE_CURVE('',#31046,#31212,#25251,.T.);
#38795=EDGE_CURVE('',#31213,#31210,#18146,.T.);
#38796=EDGE_CURVE('',#31212,#31213,#18147,.T.);
#38797=EDGE_CURVE('',#31214,#31046,#25252,.T.);
#38798=EDGE_CURVE('',#31214,#31215,#18148,.T.);
#38799=EDGE_CURVE('',#30764,#31215,#22698,.T.);
#38800=EDGE_CURVE('',#31215,#31216,#22699,.T.);
#38801=EDGE_CURVE('',#31047,#31216,#25253,.T.);
#38802=EDGE_CURVE('',#31217,#31214,#18149,.T.);
#38803=EDGE_CURVE('',#31216,#31217,#18150,.T.);
#38804=EDGE_CURVE('',#31218,#31047,#25254,.T.);
#38805=EDGE_CURVE('',#31218,#31219,#18151,.T.);
#38806=EDGE_CURVE('',#30765,#31219,#22700,.T.);
#38807=EDGE_CURVE('',#31219,#31220,#22701,.T.);
#38808=EDGE_CURVE('',#31048,#31220,#25255,.T.);
#38809=EDGE_CURVE('',#31221,#31218,#18152,.T.);
#38810=EDGE_CURVE('',#31220,#31221,#18153,.T.);
#38811=EDGE_CURVE('',#31222,#31048,#25256,.T.);
#38812=EDGE_CURVE('',#31222,#31223,#18154,.T.);
#38813=EDGE_CURVE('',#30766,#31223,#22702,.T.);
#38814=EDGE_CURVE('',#31223,#31224,#22703,.T.);
#38815=EDGE_CURVE('',#31049,#31224,#25257,.T.);
#38816=EDGE_CURVE('',#31225,#31222,#18155,.T.);
#38817=EDGE_CURVE('',#31224,#31225,#18156,.T.);
#38818=EDGE_CURVE('',#31226,#31049,#25258,.T.);
#38819=EDGE_CURVE('',#31226,#31227,#18157,.T.);
#38820=EDGE_CURVE('',#30767,#31227,#22704,.T.);
#38821=EDGE_CURVE('',#31227,#31228,#22705,.T.);
#38822=EDGE_CURVE('',#31050,#31228,#25259,.T.);
#38823=EDGE_CURVE('',#31229,#31226,#18158,.T.);
#38824=EDGE_CURVE('',#31228,#31229,#18159,.T.);
#38825=EDGE_CURVE('',#31230,#31050,#25260,.T.);
#38826=EDGE_CURVE('',#31230,#31231,#18160,.T.);
#38827=EDGE_CURVE('',#30768,#31231,#22706,.T.);
#38828=EDGE_CURVE('',#31231,#31232,#22707,.T.);
#38829=EDGE_CURVE('',#31051,#31232,#25261,.T.);
#38830=EDGE_CURVE('',#31233,#31230,#18161,.T.);
#38831=EDGE_CURVE('',#31232,#31233,#18162,.T.);
#38832=EDGE_CURVE('',#31234,#31051,#25262,.T.);
#38833=EDGE_CURVE('',#31234,#31235,#18163,.T.);
#38834=EDGE_CURVE('',#30769,#31235,#22708,.T.);
#38835=EDGE_CURVE('',#31235,#31236,#22709,.T.);
#38836=EDGE_CURVE('',#31052,#31236,#25263,.T.);
#38837=EDGE_CURVE('',#31237,#31234,#18164,.T.);
#38838=EDGE_CURVE('',#31236,#31237,#18165,.T.);
#38839=EDGE_CURVE('',#31238,#31052,#25264,.T.);
#38840=EDGE_CURVE('',#31238,#31239,#18166,.T.);
#38841=EDGE_CURVE('',#30770,#31239,#22710,.T.);
#38842=EDGE_CURVE('',#31239,#31240,#22711,.T.);
#38843=EDGE_CURVE('',#31053,#31240,#25265,.T.);
#38844=EDGE_CURVE('',#31241,#31238,#18167,.T.);
#38845=EDGE_CURVE('',#31240,#31241,#18168,.T.);
#38846=EDGE_CURVE('',#31242,#31053,#25266,.T.);
#38847=EDGE_CURVE('',#31242,#31243,#18169,.T.);
#38848=EDGE_CURVE('',#30771,#31243,#22712,.T.);
#38849=EDGE_CURVE('',#31243,#31244,#22713,.T.);
#38850=EDGE_CURVE('',#31054,#31244,#25267,.T.);
#38851=EDGE_CURVE('',#31245,#31242,#18170,.T.);
#38852=EDGE_CURVE('',#31244,#31245,#18171,.T.);
#38853=EDGE_CURVE('',#31246,#31054,#25268,.T.);
#38854=EDGE_CURVE('',#31246,#31247,#18172,.T.);
#38855=EDGE_CURVE('',#30772,#31247,#22714,.T.);
#38856=EDGE_CURVE('',#31247,#31248,#22715,.T.);
#38857=EDGE_CURVE('',#31055,#31248,#25269,.T.);
#38858=EDGE_CURVE('',#31249,#31246,#18173,.T.);
#38859=EDGE_CURVE('',#31248,#31249,#18174,.T.);
#38860=EDGE_CURVE('',#31250,#31055,#25270,.T.);
#38861=EDGE_CURVE('',#31250,#31251,#18175,.T.);
#38862=EDGE_CURVE('',#30773,#31251,#22716,.T.);
#38863=EDGE_CURVE('',#31251,#31252,#22717,.T.);
#38864=EDGE_CURVE('',#31056,#31252,#25271,.T.);
#38865=EDGE_CURVE('',#31253,#31250,#18176,.T.);
#38866=EDGE_CURVE('',#31252,#31253,#18177,.T.);
#38867=EDGE_CURVE('',#31254,#31056,#25272,.T.);
#38868=EDGE_CURVE('',#31254,#31255,#18178,.T.);
#38869=EDGE_CURVE('',#30774,#31255,#22718,.T.);
#38870=EDGE_CURVE('',#31255,#31256,#22719,.T.);
#38871=EDGE_CURVE('',#31057,#31256,#25273,.T.);
#38872=EDGE_CURVE('',#31257,#31254,#18179,.T.);
#38873=EDGE_CURVE('',#31256,#31257,#18180,.T.);
#38874=EDGE_CURVE('',#31258,#31057,#25274,.T.);
#38875=EDGE_CURVE('',#31258,#31259,#18181,.T.);
#38876=EDGE_CURVE('',#30775,#31259,#22720,.T.);
#38877=EDGE_CURVE('',#31259,#31260,#22721,.T.);
#38878=EDGE_CURVE('',#31058,#31260,#25275,.T.);
#38879=EDGE_CURVE('',#31261,#31258,#18182,.T.);
#38880=EDGE_CURVE('',#31260,#31261,#18183,.T.);
#38881=EDGE_CURVE('',#28971,#31058,#25276,.T.);
#38882=EDGE_CURVE('',#30776,#28973,#22722,.T.);
#38883=EDGE_CURVE('',#31059,#28972,#25277,.T.);
#38884=EDGE_CURVE('',#31262,#31059,#25278,.T.);
#38885=EDGE_CURVE('',#31262,#31263,#18184,.T.);
#38886=EDGE_CURVE('',#30777,#31263,#22723,.T.);
#38887=EDGE_CURVE('',#31263,#31264,#22724,.T.);
#38888=EDGE_CURVE('',#31060,#31264,#25279,.T.);
#38889=EDGE_CURVE('',#31265,#31262,#18185,.T.);
#38890=EDGE_CURVE('',#31264,#31265,#18186,.T.);
#38891=EDGE_CURVE('',#31266,#31060,#25280,.T.);
#38892=EDGE_CURVE('',#31266,#31267,#18187,.T.);
#38893=EDGE_CURVE('',#30778,#31267,#22725,.T.);
#38894=EDGE_CURVE('',#31267,#31268,#22726,.T.);
#38895=EDGE_CURVE('',#31061,#31268,#25281,.T.);
#38896=EDGE_CURVE('',#31269,#31266,#18188,.T.);
#38897=EDGE_CURVE('',#31268,#31269,#18189,.T.);
#38898=EDGE_CURVE('',#31270,#31061,#25282,.T.);
#38899=EDGE_CURVE('',#31270,#31271,#18190,.T.);
#38900=EDGE_CURVE('',#30779,#31271,#22727,.T.);
#38901=EDGE_CURVE('',#31271,#31272,#22728,.T.);
#38902=EDGE_CURVE('',#31062,#31272,#25283,.T.);
#38903=EDGE_CURVE('',#31273,#31270,#18191,.T.);
#38904=EDGE_CURVE('',#31272,#31273,#18192,.T.);
#38905=EDGE_CURVE('',#31274,#31062,#25284,.T.);
#38906=EDGE_CURVE('',#31274,#31275,#18193,.T.);
#38907=EDGE_CURVE('',#30780,#31275,#22729,.T.);
#38908=EDGE_CURVE('',#31275,#31276,#22730,.T.);
#38909=EDGE_CURVE('',#31063,#31276,#25285,.T.);
#38910=EDGE_CURVE('',#31277,#31274,#18194,.T.);
#38911=EDGE_CURVE('',#31276,#31277,#18195,.T.);
#38912=EDGE_CURVE('',#31278,#31063,#25286,.T.);
#38913=EDGE_CURVE('',#31278,#31279,#18196,.T.);
#38914=EDGE_CURVE('',#30781,#31279,#22731,.T.);
#38915=EDGE_CURVE('',#31279,#31280,#22732,.T.);
#38916=EDGE_CURVE('',#31064,#31280,#25287,.T.);
#38917=EDGE_CURVE('',#31281,#31278,#18197,.T.);
#38918=EDGE_CURVE('',#31280,#31281,#18198,.T.);
#38919=EDGE_CURVE('',#31282,#31064,#25288,.T.);
#38920=EDGE_CURVE('',#31282,#31283,#18199,.T.);
#38921=EDGE_CURVE('',#30782,#31283,#22733,.T.);
#38922=EDGE_CURVE('',#31283,#31284,#22734,.T.);
#38923=EDGE_CURVE('',#31065,#31284,#25289,.T.);
#38924=EDGE_CURVE('',#31285,#31282,#18200,.T.);
#38925=EDGE_CURVE('',#31284,#31285,#18201,.T.);
#38926=EDGE_CURVE('',#31286,#31065,#25290,.T.);
#38927=EDGE_CURVE('',#31286,#31287,#18202,.T.);
#38928=EDGE_CURVE('',#30783,#31287,#22735,.T.);
#38929=EDGE_CURVE('',#31287,#31288,#22736,.T.);
#38930=EDGE_CURVE('',#31037,#31288,#25291,.T.);
#38931=EDGE_CURVE('',#31289,#31286,#18203,.T.);
#38932=EDGE_CURVE('',#31288,#31289,#18204,.T.);
#38933=EDGE_CURVE('',#31290,#31008,#18205,.T.);
#38934=EDGE_CURVE('',#31068,#31290,#22737,.T.);
#38935=EDGE_CURVE('',#31009,#31290,#18206,.T.);
#38936=EDGE_CURVE('',#31291,#31009,#18207,.T.);
#38937=EDGE_CURVE('',#31072,#31291,#22738,.T.);
#38938=EDGE_CURVE('',#31010,#31291,#18208,.T.);
#38939=EDGE_CURVE('',#31292,#31010,#18209,.T.);
#38940=EDGE_CURVE('',#31076,#31292,#22739,.T.);
#38941=EDGE_CURVE('',#31011,#31292,#18210,.T.);
#38942=EDGE_CURVE('',#31293,#31011,#18211,.T.);
#38943=EDGE_CURVE('',#31080,#31293,#22740,.T.);
#38944=EDGE_CURVE('',#31012,#31293,#18212,.T.);
#38945=EDGE_CURVE('',#31294,#31012,#18213,.T.);
#38946=EDGE_CURVE('',#31084,#31294,#22741,.T.);
#38947=EDGE_CURVE('',#31013,#31294,#18214,.T.);
#38948=EDGE_CURVE('',#31295,#31013,#18215,.T.);
#38949=EDGE_CURVE('',#31088,#31295,#22742,.T.);
#38950=EDGE_CURVE('',#31014,#31295,#18216,.T.);
#38951=EDGE_CURVE('',#31296,#31014,#18217,.T.);
#38952=EDGE_CURVE('',#31092,#31296,#22743,.T.);
#38953=EDGE_CURVE('',#31015,#31296,#18218,.T.);
#38954=EDGE_CURVE('',#31297,#31015,#18219,.T.);
#38955=EDGE_CURVE('',#31096,#31297,#22744,.T.);
#38956=EDGE_CURVE('',#31016,#31297,#18220,.T.);
#38957=EDGE_CURVE('',#31298,#31016,#18221,.T.);
#38958=EDGE_CURVE('',#31100,#31298,#22745,.T.);
#38959=EDGE_CURVE('',#31017,#31298,#18222,.T.);
#38960=EDGE_CURVE('',#31299,#31017,#18223,.T.);
#38961=EDGE_CURVE('',#31104,#31299,#22746,.T.);
#38962=EDGE_CURVE('',#31018,#31299,#18224,.T.);
#38963=EDGE_CURVE('',#31300,#31018,#18225,.T.);
#38964=EDGE_CURVE('',#31108,#31300,#22747,.T.);
#38965=EDGE_CURVE('',#31019,#31300,#18226,.T.);
#38966=EDGE_CURVE('',#31301,#31019,#18227,.T.);
#38967=EDGE_CURVE('',#31112,#31301,#22748,.T.);
#38968=EDGE_CURVE('',#31020,#31301,#18228,.T.);
#38969=EDGE_CURVE('',#31302,#31020,#18229,.T.);
#38970=EDGE_CURVE('',#31116,#31302,#22749,.T.);
#38971=EDGE_CURVE('',#31021,#31302,#18230,.T.);
#38972=EDGE_CURVE('',#31303,#31021,#18231,.T.);
#38973=EDGE_CURVE('',#31120,#31303,#22750,.T.);
#38974=EDGE_CURVE('',#31022,#31303,#18232,.T.);
#38975=EDGE_CURVE('',#31304,#31022,#18233,.T.);
#38976=EDGE_CURVE('',#28976,#31304,#22751,.T.);
#38977=EDGE_CURVE('',#31023,#31304,#18234,.T.);
#38978=EDGE_CURVE('',#31305,#31023,#18235,.T.);
#38979=EDGE_CURVE('',#31124,#31305,#22752,.T.);
#38980=EDGE_CURVE('',#31024,#31305,#18236,.T.);
#38981=EDGE_CURVE('',#31306,#31024,#18237,.T.);
#38982=EDGE_CURVE('',#31128,#31306,#22753,.T.);
#38983=EDGE_CURVE('',#31025,#31306,#18238,.T.);
#38984=EDGE_CURVE('',#31307,#31025,#18239,.T.);
#38985=EDGE_CURVE('',#31132,#31307,#22754,.T.);
#38986=EDGE_CURVE('',#31026,#31307,#18240,.T.);
#38987=EDGE_CURVE('',#31308,#31026,#18241,.T.);
#38988=EDGE_CURVE('',#31136,#31308,#22755,.T.);
#38989=EDGE_CURVE('',#31027,#31308,#18242,.T.);
#38990=EDGE_CURVE('',#31309,#31027,#18243,.T.);
#38991=EDGE_CURVE('',#31140,#31309,#22756,.T.);
#38992=EDGE_CURVE('',#31028,#31309,#18244,.T.);
#38993=EDGE_CURVE('',#31310,#31028,#18245,.T.);
#38994=EDGE_CURVE('',#31144,#31310,#22757,.T.);
#38995=EDGE_CURVE('',#31029,#31310,#18246,.T.);
#38996=EDGE_CURVE('',#31311,#31029,#18247,.T.);
#38997=EDGE_CURVE('',#31149,#31311,#22758,.T.);
#38998=EDGE_CURVE('',#31030,#31311,#18248,.T.);
#38999=EDGE_CURVE('',#31312,#31030,#18249,.T.);
#39000=EDGE_CURVE('',#31153,#31312,#22759,.T.);
#39001=EDGE_CURVE('',#31031,#31312,#18250,.T.);
#39002=EDGE_CURVE('',#31313,#31031,#18251,.T.);
#39003=EDGE_CURVE('',#31156,#31313,#22760,.T.);
#39004=EDGE_CURVE('',#31032,#31313,#18252,.T.);
#39005=EDGE_CURVE('',#31314,#31032,#18253,.T.);
#39006=EDGE_CURVE('',#31160,#31314,#22761,.T.);
#39007=EDGE_CURVE('',#31033,#31314,#18254,.T.);
#39008=EDGE_CURVE('',#31315,#31033,#18255,.T.);
#39009=EDGE_CURVE('',#31164,#31315,#22762,.T.);
#39010=EDGE_CURVE('',#31034,#31315,#18256,.T.);
#39011=EDGE_CURVE('',#31316,#31034,#18257,.T.);
#39012=EDGE_CURVE('',#31168,#31316,#22763,.T.);
#39013=EDGE_CURVE('',#31035,#31316,#18258,.T.);
#39014=EDGE_CURVE('',#31317,#31035,#18259,.T.);
#39015=EDGE_CURVE('',#31172,#31317,#22764,.T.);
#39016=EDGE_CURVE('',#31036,#31317,#18260,.T.);
#39017=EDGE_CURVE('',#31318,#31036,#18261,.T.);
#39018=EDGE_CURVE('',#31176,#31318,#22765,.T.);
#39019=EDGE_CURVE('',#31008,#31318,#18262,.T.);
#39020=EDGE_CURVE('',#31319,#31037,#18263,.T.);
#39021=EDGE_CURVE('',#31181,#31319,#22766,.T.);
#39022=EDGE_CURVE('',#31038,#31319,#18264,.T.);
#39023=EDGE_CURVE('',#31320,#31038,#18265,.T.);
#39024=EDGE_CURVE('',#31185,#31320,#22767,.T.);
#39025=EDGE_CURVE('',#31039,#31320,#18266,.T.);
#39026=EDGE_CURVE('',#31321,#31039,#18267,.T.);
#39027=EDGE_CURVE('',#31189,#31321,#22768,.T.);
#39028=EDGE_CURVE('',#31040,#31321,#18268,.T.);
#39029=EDGE_CURVE('',#31322,#31040,#18269,.T.);
#39030=EDGE_CURVE('',#31193,#31322,#22769,.T.);
#39031=EDGE_CURVE('',#31041,#31322,#18270,.T.);
#39032=EDGE_CURVE('',#31323,#31041,#18271,.T.);
#39033=EDGE_CURVE('',#31197,#31323,#22770,.T.);
#39034=EDGE_CURVE('',#31042,#31323,#18272,.T.);
#39035=EDGE_CURVE('',#31324,#31042,#18273,.T.);
#39036=EDGE_CURVE('',#31201,#31324,#22771,.T.);
#39037=EDGE_CURVE('',#31043,#31324,#18274,.T.);
#39038=EDGE_CURVE('',#31325,#31043,#18275,.T.);
#39039=EDGE_CURVE('',#31205,#31325,#22772,.T.);
#39040=EDGE_CURVE('',#31044,#31325,#18276,.T.);
#39041=EDGE_CURVE('',#31326,#31044,#18277,.T.);
#39042=EDGE_CURVE('',#31209,#31326,#22773,.T.);
#39043=EDGE_CURVE('',#31045,#31326,#18278,.T.);
#39044=EDGE_CURVE('',#31327,#31045,#18279,.T.);
#39045=EDGE_CURVE('',#31213,#31327,#22774,.T.);
#39046=EDGE_CURVE('',#31046,#31327,#18280,.T.);
#39047=EDGE_CURVE('',#31328,#31046,#18281,.T.);
#39048=EDGE_CURVE('',#31217,#31328,#22775,.T.);
#39049=EDGE_CURVE('',#31047,#31328,#18282,.T.);
#39050=EDGE_CURVE('',#31329,#31047,#18283,.T.);
#39051=EDGE_CURVE('',#31221,#31329,#22776,.T.);
#39052=EDGE_CURVE('',#31048,#31329,#18284,.T.);
#39053=EDGE_CURVE('',#31330,#31048,#18285,.T.);
#39054=EDGE_CURVE('',#31225,#31330,#22777,.T.);
#39055=EDGE_CURVE('',#31049,#31330,#18286,.T.);
#39056=EDGE_CURVE('',#31331,#31049,#18287,.T.);
#39057=EDGE_CURVE('',#31229,#31331,#22778,.T.);
#39058=EDGE_CURVE('',#31050,#31331,#18288,.T.);
#39059=EDGE_CURVE('',#31332,#31050,#18289,.T.);
#39060=EDGE_CURVE('',#31233,#31332,#22779,.T.);
#39061=EDGE_CURVE('',#31051,#31332,#18290,.T.);
#39062=EDGE_CURVE('',#31333,#31051,#18291,.T.);
#39063=EDGE_CURVE('',#31237,#31333,#22780,.T.);
#39064=EDGE_CURVE('',#31052,#31333,#18292,.T.);
#39065=EDGE_CURVE('',#31334,#31052,#18293,.T.);
#39066=EDGE_CURVE('',#31241,#31334,#22781,.T.);
#39067=EDGE_CURVE('',#31053,#31334,#18294,.T.);
#39068=EDGE_CURVE('',#31335,#31053,#18295,.T.);
#39069=EDGE_CURVE('',#31245,#31335,#22782,.T.);
#39070=EDGE_CURVE('',#31054,#31335,#18296,.T.);
#39071=EDGE_CURVE('',#31336,#31054,#18297,.T.);
#39072=EDGE_CURVE('',#31249,#31336,#22783,.T.);
#39073=EDGE_CURVE('',#31055,#31336,#18298,.T.);
#39074=EDGE_CURVE('',#31337,#31055,#18299,.T.);
#39075=EDGE_CURVE('',#31253,#31337,#22784,.T.);
#39076=EDGE_CURVE('',#31056,#31337,#18300,.T.);
#39077=EDGE_CURVE('',#31338,#31056,#18301,.T.);
#39078=EDGE_CURVE('',#31257,#31338,#22785,.T.);
#39079=EDGE_CURVE('',#31057,#31338,#18302,.T.);
#39080=EDGE_CURVE('',#31339,#31057,#18303,.T.);
#39081=EDGE_CURVE('',#31261,#31339,#22786,.T.);
#39082=EDGE_CURVE('',#31058,#31339,#18304,.T.);
#39083=EDGE_CURVE('',#31340,#31058,#18305,.T.);
#39084=EDGE_CURVE('',#28970,#31340,#22787,.T.);
#39085=EDGE_CURVE('',#31059,#31340,#18306,.T.);
#39086=EDGE_CURVE('',#31341,#31059,#18307,.T.);
#39087=EDGE_CURVE('',#31265,#31341,#22788,.T.);
#39088=EDGE_CURVE('',#31060,#31341,#18308,.T.);
#39089=EDGE_CURVE('',#31342,#31060,#18309,.T.);
#39090=EDGE_CURVE('',#31269,#31342,#22789,.T.);
#39091=EDGE_CURVE('',#31061,#31342,#18310,.T.);
#39092=EDGE_CURVE('',#31343,#31061,#18311,.T.);
#39093=EDGE_CURVE('',#31273,#31343,#22790,.T.);
#39094=EDGE_CURVE('',#31062,#31343,#18312,.T.);
#39095=EDGE_CURVE('',#31344,#31062,#18313,.T.);
#39096=EDGE_CURVE('',#31277,#31344,#22791,.T.);
#39097=EDGE_CURVE('',#31063,#31344,#18314,.T.);
#39098=EDGE_CURVE('',#31345,#31063,#18315,.T.);
#39099=EDGE_CURVE('',#31281,#31345,#22792,.T.);
#39100=EDGE_CURVE('',#31064,#31345,#18316,.T.);
#39101=EDGE_CURVE('',#31346,#31064,#18317,.T.);
#39102=EDGE_CURVE('',#31285,#31346,#22793,.T.);
#39103=EDGE_CURVE('',#31065,#31346,#18318,.T.);
#39104=EDGE_CURVE('',#31347,#31065,#18319,.T.);
#39105=EDGE_CURVE('',#31289,#31347,#22794,.T.);
#39106=EDGE_CURVE('',#31037,#31347,#18320,.T.);
#39107=EDGE_CURVE('',#31348,#31349,#18321,.T.);
#39108=EDGE_CURVE('',#31290,#31349,#25292,.T.);
#39109=EDGE_CURVE('',#31348,#31008,#22795,.T.);
#39110=EDGE_CURVE('',#31350,#31351,#18322,.T.);
#39111=EDGE_CURVE('',#31009,#31351,#22796,.T.);
#39112=EDGE_CURVE('',#31350,#31290,#25293,.T.);
#39113=EDGE_CURVE('',#31352,#31350,#18323,.T.);
#39114=EDGE_CURVE('',#31353,#31352,#18324,.T.);
#39115=EDGE_CURVE('',#31351,#31353,#18325,.T.);
#39116=EDGE_CURVE('',#31291,#31353,#25294,.T.);
#39117=EDGE_CURVE('',#31354,#31355,#18326,.T.);
#39118=EDGE_CURVE('',#31010,#31355,#22797,.T.);
#39119=EDGE_CURVE('',#31354,#31291,#25295,.T.);
#39120=EDGE_CURVE('',#31356,#31354,#18327,.T.);
#39121=EDGE_CURVE('',#31357,#31356,#18328,.T.);
#39122=EDGE_CURVE('',#31355,#31357,#18329,.T.);
#39123=EDGE_CURVE('',#31292,#31357,#25296,.T.);
#39124=EDGE_CURVE('',#31358,#31359,#18330,.T.);
#39125=EDGE_CURVE('',#31011,#31359,#22798,.T.);
#39126=EDGE_CURVE('',#31358,#31292,#25297,.T.);
#39127=EDGE_CURVE('',#31360,#31358,#18331,.T.);
#39128=EDGE_CURVE('',#31361,#31360,#18332,.T.);
#39129=EDGE_CURVE('',#31359,#31361,#18333,.T.);
#39130=EDGE_CURVE('',#31293,#31361,#25298,.T.);
#39131=EDGE_CURVE('',#31362,#31363,#18334,.T.);
#39132=EDGE_CURVE('',#31012,#31363,#22799,.T.);
#39133=EDGE_CURVE('',#31362,#31293,#25299,.T.);
#39134=EDGE_CURVE('',#31364,#31362,#18335,.T.);
#39135=EDGE_CURVE('',#31365,#31364,#18336,.T.);
#39136=EDGE_CURVE('',#31363,#31365,#18337,.T.);
#39137=EDGE_CURVE('',#31294,#31365,#25300,.T.);
#39138=EDGE_CURVE('',#31366,#31367,#18338,.T.);
#39139=EDGE_CURVE('',#31013,#31367,#22800,.T.);
#39140=EDGE_CURVE('',#31366,#31294,#25301,.T.);
#39141=EDGE_CURVE('',#31368,#31366,#18339,.T.);
#39142=EDGE_CURVE('',#31369,#31368,#18340,.T.);
#39143=EDGE_CURVE('',#31367,#31369,#18341,.T.);
#39144=EDGE_CURVE('',#31295,#31369,#25302,.T.);
#39145=EDGE_CURVE('',#31370,#31371,#18342,.T.);
#39146=EDGE_CURVE('',#31014,#31371,#22801,.T.);
#39147=EDGE_CURVE('',#31370,#31295,#25303,.T.);
#39148=EDGE_CURVE('',#31372,#31370,#18343,.T.);
#39149=EDGE_CURVE('',#31373,#31372,#18344,.T.);
#39150=EDGE_CURVE('',#31371,#31373,#18345,.T.);
#39151=EDGE_CURVE('',#31296,#31373,#25304,.T.);
#39152=EDGE_CURVE('',#31015,#28966,#22802,.T.);
#39153=EDGE_CURVE('',#28968,#31296,#25305,.T.);
#39154=EDGE_CURVE('',#31297,#28967,#25306,.T.);
#39155=EDGE_CURVE('',#31374,#31375,#18346,.T.);
#39156=EDGE_CURVE('',#31016,#31375,#22803,.T.);
#39157=EDGE_CURVE('',#31374,#31297,#25307,.T.);
#39158=EDGE_CURVE('',#31376,#31374,#18347,.T.);
#39159=EDGE_CURVE('',#31377,#31376,#18348,.T.);
#39160=EDGE_CURVE('',#31375,#31377,#18349,.T.);
#39161=EDGE_CURVE('',#31298,#31377,#25308,.T.);
#39162=EDGE_CURVE('',#31378,#31379,#18350,.T.);
#39163=EDGE_CURVE('',#31017,#31379,#22804,.T.);
#39164=EDGE_CURVE('',#31378,#31298,#25309,.T.);
#39165=EDGE_CURVE('',#31380,#31378,#18351,.T.);
#39166=EDGE_CURVE('',#31381,#31380,#18352,.T.);
#39167=EDGE_CURVE('',#31379,#31381,#18353,.T.);
#39168=EDGE_CURVE('',#31299,#31381,#25310,.T.);
#39169=EDGE_CURVE('',#31382,#31383,#18354,.T.);
#39170=EDGE_CURVE('',#31018,#31383,#22805,.T.);
#39171=EDGE_CURVE('',#31382,#31299,#25311,.T.);
#39172=EDGE_CURVE('',#31384,#31382,#18355,.T.);
#39173=EDGE_CURVE('',#31385,#31384,#18356,.T.);
#39174=EDGE_CURVE('',#31383,#31385,#18357,.T.);
#39175=EDGE_CURVE('',#31300,#31385,#25312,.T.);
#39176=EDGE_CURVE('',#31386,#31387,#18358,.T.);
#39177=EDGE_CURVE('',#31019,#31387,#22806,.T.);
#39178=EDGE_CURVE('',#31386,#31300,#25313,.T.);
#39179=EDGE_CURVE('',#31388,#31386,#18359,.T.);
#39180=EDGE_CURVE('',#31389,#31388,#18360,.T.);
#39181=EDGE_CURVE('',#31387,#31389,#18361,.T.);
#39182=EDGE_CURVE('',#31301,#31389,#25314,.T.);
#39183=EDGE_CURVE('',#31390,#31391,#18362,.T.);
#39184=EDGE_CURVE('',#31020,#31391,#22807,.T.);
#39185=EDGE_CURVE('',#31390,#31301,#25315,.T.);
#39186=EDGE_CURVE('',#31392,#31390,#18363,.T.);
#39187=EDGE_CURVE('',#31393,#31392,#18364,.T.);
#39188=EDGE_CURVE('',#31391,#31393,#18365,.T.);
#39189=EDGE_CURVE('',#31302,#31393,#25316,.T.);
#39190=EDGE_CURVE('',#31394,#31395,#18366,.T.);
#39191=EDGE_CURVE('',#31021,#31395,#22808,.T.);
#39192=EDGE_CURVE('',#31394,#31302,#25317,.T.);
#39193=EDGE_CURVE('',#31396,#31394,#18367,.T.);
#39194=EDGE_CURVE('',#31397,#31396,#18368,.T.);
#39195=EDGE_CURVE('',#31395,#31397,#18369,.T.);
#39196=EDGE_CURVE('',#31303,#31397,#25318,.T.);
#39197=EDGE_CURVE('',#31398,#31399,#18370,.T.);
#39198=EDGE_CURVE('',#31022,#31399,#22809,.T.);
#39199=EDGE_CURVE('',#31398,#31303,#25319,.T.);
#39200=EDGE_CURVE('',#31400,#31398,#18371,.T.);
#39201=EDGE_CURVE('',#31401,#31400,#18372,.T.);
#39202=EDGE_CURVE('',#31399,#31401,#18373,.T.);
#39203=EDGE_CURVE('',#31304,#31401,#25320,.T.);
#39204=EDGE_CURVE('',#31402,#31403,#18374,.T.);
#39205=EDGE_CURVE('',#31023,#31403,#22810,.T.);
#39206=EDGE_CURVE('',#31402,#31304,#25321,.T.);
#39207=EDGE_CURVE('',#31404,#31402,#18375,.T.);
#39208=EDGE_CURVE('',#31405,#31404,#18376,.T.);
#39209=EDGE_CURVE('',#31403,#31405,#18377,.T.);
#39210=EDGE_CURVE('',#31305,#31405,#25322,.T.);
#39211=EDGE_CURVE('',#31406,#31407,#18378,.T.);
#39212=EDGE_CURVE('',#31024,#31407,#22811,.T.);
#39213=EDGE_CURVE('',#31406,#31305,#25323,.T.);
#39214=EDGE_CURVE('',#31408,#31406,#18379,.T.);
#39215=EDGE_CURVE('',#31409,#31408,#18380,.T.);
#39216=EDGE_CURVE('',#31407,#31409,#18381,.T.);
#39217=EDGE_CURVE('',#31306,#31409,#25324,.T.);
#39218=EDGE_CURVE('',#31410,#31411,#18382,.T.);
#39219=EDGE_CURVE('',#31025,#31411,#22812,.T.);
#39220=EDGE_CURVE('',#31410,#31306,#25325,.T.);
#39221=EDGE_CURVE('',#31412,#31410,#18383,.T.);
#39222=EDGE_CURVE('',#31413,#31412,#18384,.T.);
#39223=EDGE_CURVE('',#31411,#31413,#18385,.T.);
#39224=EDGE_CURVE('',#31307,#31413,#25326,.T.);
#39225=EDGE_CURVE('',#31414,#31415,#18386,.T.);
#39226=EDGE_CURVE('',#31026,#31415,#22813,.T.);
#39227=EDGE_CURVE('',#31414,#31307,#25327,.T.);
#39228=EDGE_CURVE('',#31416,#31414,#18387,.T.);
#39229=EDGE_CURVE('',#31417,#31416,#18388,.T.);
#39230=EDGE_CURVE('',#31415,#31417,#18389,.T.);
#39231=EDGE_CURVE('',#31308,#31417,#25328,.T.);
#39232=EDGE_CURVE('',#31418,#31419,#18390,.T.);
#39233=EDGE_CURVE('',#31027,#31419,#22814,.T.);
#39234=EDGE_CURVE('',#31418,#31308,#25329,.T.);
#39235=EDGE_CURVE('',#31420,#31418,#18391,.T.);
#39236=EDGE_CURVE('',#31421,#31420,#18392,.T.);
#39237=EDGE_CURVE('',#31419,#31421,#18393,.T.);
#39238=EDGE_CURVE('',#31309,#31421,#25330,.T.);
#39239=EDGE_CURVE('',#31422,#31423,#18394,.T.);
#39240=EDGE_CURVE('',#31028,#31423,#22815,.T.);
#39241=EDGE_CURVE('',#31422,#31309,#25331,.T.);
#39242=EDGE_CURVE('',#31424,#31422,#18395,.T.);
#39243=EDGE_CURVE('',#31425,#31424,#18396,.T.);
#39244=EDGE_CURVE('',#31423,#31425,#18397,.T.);
#39245=EDGE_CURVE('',#31310,#31425,#25332,.T.);
#39246=EDGE_CURVE('',#31426,#31427,#18398,.T.);
#39247=EDGE_CURVE('',#31029,#31427,#22816,.T.);
#39248=EDGE_CURVE('',#31426,#31310,#25333,.T.);
#39249=EDGE_CURVE('',#31427,#31428,#18399,.T.);
#39250=EDGE_CURVE('',#31311,#31428,#25334,.T.);
#39251=EDGE_CURVE('',#31429,#31426,#18400,.T.);
#39252=EDGE_CURVE('',#31428,#31429,#18401,.T.);
#39253=EDGE_CURVE('',#31430,#31311,#25335,.T.);
#39254=EDGE_CURVE('',#31430,#31431,#18402,.T.);
#39255=EDGE_CURVE('',#31030,#31431,#22817,.T.);
#39256=EDGE_CURVE('',#31431,#31432,#18403,.T.);
#39257=EDGE_CURVE('',#31433,#31430,#18404,.T.);
#39258=EDGE_CURVE('',#31432,#31433,#18405,.T.);
#39259=EDGE_CURVE('',#31312,#31432,#25336,.T.);
#39260=EDGE_CURVE('',#31434,#31435,#18406,.T.);
#39261=EDGE_CURVE('',#31031,#31435,#22818,.T.);
#39262=EDGE_CURVE('',#31434,#31312,#25337,.T.);
#39263=EDGE_CURVE('',#31436,#31434,#18407,.T.);
#39264=EDGE_CURVE('',#31437,#31436,#18408,.T.);
#39265=EDGE_CURVE('',#31435,#31437,#18409,.T.);
#39266=EDGE_CURVE('',#31313,#31437,#25338,.T.);
#39267=EDGE_CURVE('',#31438,#31439,#18410,.T.);
#39268=EDGE_CURVE('',#31032,#31439,#22819,.T.);
#39269=EDGE_CURVE('',#31438,#31313,#25339,.T.);
#39270=EDGE_CURVE('',#31440,#31438,#18411,.T.);
#39271=EDGE_CURVE('',#31441,#31440,#18412,.T.);
#39272=EDGE_CURVE('',#31439,#31441,#18413,.T.);
#39273=EDGE_CURVE('',#31314,#31441,#25340,.T.);
#39274=EDGE_CURVE('',#31442,#31443,#18414,.T.);
#39275=EDGE_CURVE('',#31033,#31443,#22820,.T.);
#39276=EDGE_CURVE('',#31442,#31314,#25341,.T.);
#39277=EDGE_CURVE('',#31444,#31442,#18415,.T.);
#39278=EDGE_CURVE('',#31445,#31444,#18416,.T.);
#39279=EDGE_CURVE('',#31443,#31445,#18417,.T.);
#39280=EDGE_CURVE('',#31315,#31445,#25342,.T.);
#39281=EDGE_CURVE('',#31446,#31447,#18418,.T.);
#39282=EDGE_CURVE('',#31034,#31447,#22821,.T.);
#39283=EDGE_CURVE('',#31446,#31315,#25343,.T.);
#39284=EDGE_CURVE('',#31448,#31446,#18419,.T.);
#39285=EDGE_CURVE('',#31449,#31448,#18420,.T.);
#39286=EDGE_CURVE('',#31447,#31449,#18421,.T.);
#39287=EDGE_CURVE('',#31316,#31449,#25344,.T.);
#39288=EDGE_CURVE('',#31450,#31451,#18422,.T.);
#39289=EDGE_CURVE('',#31035,#31451,#22822,.T.);
#39290=EDGE_CURVE('',#31450,#31316,#25345,.T.);
#39291=EDGE_CURVE('',#31452,#31450,#18423,.T.);
#39292=EDGE_CURVE('',#31453,#31452,#18424,.T.);
#39293=EDGE_CURVE('',#31451,#31453,#18425,.T.);
#39294=EDGE_CURVE('',#31317,#31453,#25346,.T.);
#39295=EDGE_CURVE('',#31454,#31455,#18426,.T.);
#39296=EDGE_CURVE('',#31036,#31455,#22823,.T.);
#39297=EDGE_CURVE('',#31454,#31317,#25347,.T.);
#39298=EDGE_CURVE('',#31456,#31454,#18427,.T.);
#39299=EDGE_CURVE('',#31457,#31456,#18428,.T.);
#39300=EDGE_CURVE('',#31455,#31457,#18429,.T.);
#39301=EDGE_CURVE('',#31318,#31457,#25348,.T.);
#39302=EDGE_CURVE('',#31458,#31459,#18430,.T.);
#39303=EDGE_CURVE('',#31349,#31458,#18431,.T.);
#39304=EDGE_CURVE('',#31459,#31348,#18432,.T.);
#39305=EDGE_CURVE('',#31459,#31318,#25349,.T.);
#39306=EDGE_CURVE('',#31460,#31037,#22824,.T.);
#39307=EDGE_CURVE('',#31460,#31461,#18433,.T.);
#39308=EDGE_CURVE('',#31319,#31461,#25350,.T.);
#39309=EDGE_CURVE('',#31462,#31319,#25351,.T.);
#39310=EDGE_CURVE('',#31462,#31463,#18434,.T.);
#39311=EDGE_CURVE('',#31038,#31463,#22825,.T.);
#39312=EDGE_CURVE('',#31463,#31464,#18435,.T.);
#39313=EDGE_CURVE('',#31320,#31464,#25352,.T.);
#39314=EDGE_CURVE('',#31465,#31462,#18436,.T.);
#39315=EDGE_CURVE('',#31464,#31465,#18437,.T.);
#39316=EDGE_CURVE('',#31466,#31320,#25353,.T.);
#39317=EDGE_CURVE('',#31466,#31467,#18438,.T.);
#39318=EDGE_CURVE('',#31039,#31467,#22826,.T.);
#39319=EDGE_CURVE('',#31467,#31468,#18439,.T.);
#39320=EDGE_CURVE('',#31321,#31468,#25354,.T.);
#39321=EDGE_CURVE('',#31469,#31466,#18440,.T.);
#39322=EDGE_CURVE('',#31468,#31469,#18441,.T.);
#39323=EDGE_CURVE('',#31470,#31321,#25355,.T.);
#39324=EDGE_CURVE('',#31470,#31471,#18442,.T.);
#39325=EDGE_CURVE('',#31040,#31471,#22827,.T.);
#39326=EDGE_CURVE('',#31471,#31472,#18443,.T.);
#39327=EDGE_CURVE('',#31322,#31472,#25356,.T.);
#39328=EDGE_CURVE('',#31473,#31470,#18444,.T.);
#39329=EDGE_CURVE('',#31472,#31473,#18445,.T.);
#39330=EDGE_CURVE('',#31474,#31322,#25357,.T.);
#39331=EDGE_CURVE('',#31474,#31475,#18446,.T.);
#39332=EDGE_CURVE('',#31041,#31475,#22828,.T.);
#39333=EDGE_CURVE('',#31475,#31476,#18447,.T.);
#39334=EDGE_CURVE('',#31323,#31476,#25358,.T.);
#39335=EDGE_CURVE('',#31477,#31474,#18448,.T.);
#39336=EDGE_CURVE('',#31476,#31477,#18449,.T.);
#39337=EDGE_CURVE('',#31478,#31323,#25359,.T.);
#39338=EDGE_CURVE('',#31478,#31479,#18450,.T.);
#39339=EDGE_CURVE('',#31042,#31479,#22829,.T.);
#39340=EDGE_CURVE('',#31479,#31480,#18451,.T.);
#39341=EDGE_CURVE('',#31324,#31480,#25360,.T.);
#39342=EDGE_CURVE('',#31481,#31478,#18452,.T.);
#39343=EDGE_CURVE('',#31480,#31481,#18453,.T.);
#39344=EDGE_CURVE('',#31482,#31324,#25361,.T.);
#39345=EDGE_CURVE('',#31482,#31483,#18454,.T.);
#39346=EDGE_CURVE('',#31043,#31483,#22830,.T.);
#39347=EDGE_CURVE('',#31483,#31484,#18455,.T.);
#39348=EDGE_CURVE('',#31325,#31484,#25362,.T.);
#39349=EDGE_CURVE('',#31485,#31482,#18456,.T.);
#39350=EDGE_CURVE('',#31484,#31485,#18457,.T.);
#39351=EDGE_CURVE('',#31486,#31325,#25363,.T.);
#39352=EDGE_CURVE('',#31486,#31487,#18458,.T.);
#39353=EDGE_CURVE('',#31044,#31487,#22831,.T.);
#39354=EDGE_CURVE('',#31487,#31488,#18459,.T.);
#39355=EDGE_CURVE('',#31326,#31488,#25364,.T.);
#39356=EDGE_CURVE('',#31489,#31486,#18460,.T.);
#39357=EDGE_CURVE('',#31488,#31489,#18461,.T.);
#39358=EDGE_CURVE('',#31490,#31326,#25365,.T.);
#39359=EDGE_CURVE('',#31490,#31491,#18462,.T.);
#39360=EDGE_CURVE('',#31045,#31491,#22832,.T.);
#39361=EDGE_CURVE('',#31491,#31492,#18463,.T.);
#39362=EDGE_CURVE('',#31327,#31492,#25366,.T.);
#39363=EDGE_CURVE('',#31493,#31490,#18464,.T.);
#39364=EDGE_CURVE('',#31492,#31493,#18465,.T.);
#39365=EDGE_CURVE('',#31494,#31327,#25367,.T.);
#39366=EDGE_CURVE('',#31494,#31495,#18466,.T.);
#39367=EDGE_CURVE('',#31046,#31495,#22833,.T.);
#39368=EDGE_CURVE('',#31495,#31496,#18467,.T.);
#39369=EDGE_CURVE('',#31328,#31496,#25368,.T.);
#39370=EDGE_CURVE('',#31497,#31494,#18468,.T.);
#39371=EDGE_CURVE('',#31496,#31497,#18469,.T.);
#39372=EDGE_CURVE('',#31498,#31328,#25369,.T.);
#39373=EDGE_CURVE('',#31498,#31499,#18470,.T.);
#39374=EDGE_CURVE('',#31047,#31499,#22834,.T.);
#39375=EDGE_CURVE('',#31499,#31500,#18471,.T.);
#39376=EDGE_CURVE('',#31329,#31500,#25370,.T.);
#39377=EDGE_CURVE('',#31501,#31498,#18472,.T.);
#39378=EDGE_CURVE('',#31500,#31501,#18473,.T.);
#39379=EDGE_CURVE('',#31502,#31329,#25371,.T.);
#39380=EDGE_CURVE('',#31502,#31503,#18474,.T.);
#39381=EDGE_CURVE('',#31048,#31503,#22835,.T.);
#39382=EDGE_CURVE('',#31503,#31504,#18475,.T.);
#39383=EDGE_CURVE('',#31330,#31504,#25372,.T.);
#39384=EDGE_CURVE('',#31505,#31502,#18476,.T.);
#39385=EDGE_CURVE('',#31504,#31505,#18477,.T.);
#39386=EDGE_CURVE('',#31506,#31330,#25373,.T.);
#39387=EDGE_CURVE('',#31506,#31507,#18478,.T.);
#39388=EDGE_CURVE('',#31049,#31507,#22836,.T.);
#39389=EDGE_CURVE('',#31507,#31508,#18479,.T.);
#39390=EDGE_CURVE('',#31331,#31508,#25374,.T.);
#39391=EDGE_CURVE('',#31509,#31506,#18480,.T.);
#39392=EDGE_CURVE('',#31508,#31509,#18481,.T.);
#39393=EDGE_CURVE('',#31510,#31331,#25375,.T.);
#39394=EDGE_CURVE('',#31510,#31511,#18482,.T.);
#39395=EDGE_CURVE('',#31050,#31511,#22837,.T.);
#39396=EDGE_CURVE('',#31511,#31512,#18483,.T.);
#39397=EDGE_CURVE('',#31332,#31512,#25376,.T.);
#39398=EDGE_CURVE('',#31513,#31510,#18484,.T.);
#39399=EDGE_CURVE('',#31512,#31513,#18485,.T.);
#39400=EDGE_CURVE('',#28965,#31332,#25377,.T.);
#39401=EDGE_CURVE('',#31051,#28964,#22838,.T.);
#39402=EDGE_CURVE('',#31333,#28962,#25378,.T.);
#39403=EDGE_CURVE('',#31514,#31333,#25379,.T.);
#39404=EDGE_CURVE('',#31514,#31515,#18486,.T.);
#39405=EDGE_CURVE('',#31052,#31515,#22839,.T.);
#39406=EDGE_CURVE('',#31515,#31516,#18487,.T.);
#39407=EDGE_CURVE('',#31334,#31516,#25380,.T.);
#39408=EDGE_CURVE('',#31517,#31514,#18488,.T.);
#39409=EDGE_CURVE('',#31516,#31517,#18489,.T.);
#39410=EDGE_CURVE('',#31518,#31334,#25381,.T.);
#39411=EDGE_CURVE('',#31518,#31519,#18490,.T.);
#39412=EDGE_CURVE('',#31053,#31519,#22840,.T.);
#39413=EDGE_CURVE('',#31519,#31520,#18491,.T.);
#39414=EDGE_CURVE('',#31335,#31520,#25382,.T.);
#39415=EDGE_CURVE('',#31521,#31518,#18492,.T.);
#39416=EDGE_CURVE('',#31520,#31521,#18493,.T.);
#39417=EDGE_CURVE('',#31522,#31335,#25383,.T.);
#39418=EDGE_CURVE('',#31522,#31523,#18494,.T.);
#39419=EDGE_CURVE('',#31054,#31523,#22841,.T.);
#39420=EDGE_CURVE('',#31523,#31524,#18495,.T.);
#39421=EDGE_CURVE('',#31336,#31524,#25384,.T.);
#39422=EDGE_CURVE('',#31525,#31522,#18496,.T.);
#39423=EDGE_CURVE('',#31524,#31525,#18497,.T.);
#39424=EDGE_CURVE('',#31526,#31336,#25385,.T.);
#39425=EDGE_CURVE('',#31526,#31527,#18498,.T.);
#39426=EDGE_CURVE('',#31055,#31527,#22842,.T.);
#39427=EDGE_CURVE('',#31527,#31528,#18499,.T.);
#39428=EDGE_CURVE('',#31337,#31528,#25386,.T.);
#39429=EDGE_CURVE('',#31529,#31526,#18500,.T.);
#39430=EDGE_CURVE('',#31528,#31529,#18501,.T.);
#39431=EDGE_CURVE('',#31530,#31337,#25387,.T.);
#39432=EDGE_CURVE('',#31530,#31531,#18502,.T.);
#39433=EDGE_CURVE('',#31056,#31531,#22843,.T.);
#39434=EDGE_CURVE('',#31531,#31532,#18503,.T.);
#39435=EDGE_CURVE('',#31338,#31532,#25388,.T.);
#39436=EDGE_CURVE('',#31533,#31530,#18504,.T.);
#39437=EDGE_CURVE('',#31532,#31533,#18505,.T.);
#39438=EDGE_CURVE('',#31534,#31338,#25389,.T.);
#39439=EDGE_CURVE('',#31534,#31535,#18506,.T.);
#39440=EDGE_CURVE('',#31057,#31535,#22844,.T.);
#39441=EDGE_CURVE('',#31535,#31536,#18507,.T.);
#39442=EDGE_CURVE('',#31339,#31536,#25390,.T.);
#39443=EDGE_CURVE('',#31537,#31534,#18508,.T.);
#39444=EDGE_CURVE('',#31536,#31537,#18509,.T.);
#39445=EDGE_CURVE('',#31538,#31339,#25391,.T.);
#39446=EDGE_CURVE('',#31538,#31539,#18510,.T.);
#39447=EDGE_CURVE('',#31058,#31539,#22845,.T.);
#39448=EDGE_CURVE('',#31539,#31540,#18511,.T.);
#39449=EDGE_CURVE('',#31340,#31540,#25392,.T.);
#39450=EDGE_CURVE('',#31541,#31538,#18512,.T.);
#39451=EDGE_CURVE('',#31540,#31541,#18513,.T.);
#39452=EDGE_CURVE('',#31542,#31340,#25393,.T.);
#39453=EDGE_CURVE('',#31542,#31543,#18514,.T.);
#39454=EDGE_CURVE('',#31059,#31543,#22846,.T.);
#39455=EDGE_CURVE('',#31543,#31544,#18515,.T.);
#39456=EDGE_CURVE('',#31341,#31544,#25394,.T.);
#39457=EDGE_CURVE('',#31545,#31542,#18516,.T.);
#39458=EDGE_CURVE('',#31544,#31545,#18517,.T.);
#39459=EDGE_CURVE('',#31546,#31341,#25395,.T.);
#39460=EDGE_CURVE('',#31546,#31547,#18518,.T.);
#39461=EDGE_CURVE('',#31060,#31547,#22847,.T.);
#39462=EDGE_CURVE('',#31547,#31548,#18519,.T.);
#39463=EDGE_CURVE('',#31342,#31548,#25396,.T.);
#39464=EDGE_CURVE('',#31549,#31546,#18520,.T.);
#39465=EDGE_CURVE('',#31548,#31549,#18521,.T.);
#39466=EDGE_CURVE('',#31550,#31342,#25397,.T.);
#39467=EDGE_CURVE('',#31550,#31551,#18522,.T.);
#39468=EDGE_CURVE('',#31061,#31551,#22848,.T.);
#39469=EDGE_CURVE('',#31551,#31552,#18523,.T.);
#39470=EDGE_CURVE('',#31343,#31552,#25398,.T.);
#39471=EDGE_CURVE('',#31553,#31550,#18524,.T.);
#39472=EDGE_CURVE('',#31552,#31553,#18525,.T.);
#39473=EDGE_CURVE('',#31554,#31343,#25399,.T.);
#39474=EDGE_CURVE('',#31554,#31555,#18526,.T.);
#39475=EDGE_CURVE('',#31062,#31555,#22849,.T.);
#39476=EDGE_CURVE('',#31555,#31556,#18527,.T.);
#39477=EDGE_CURVE('',#31344,#31556,#25400,.T.);
#39478=EDGE_CURVE('',#31557,#31554,#18528,.T.);
#39479=EDGE_CURVE('',#31556,#31557,#18529,.T.);
#39480=EDGE_CURVE('',#31558,#31344,#25401,.T.);
#39481=EDGE_CURVE('',#31558,#31559,#18530,.T.);
#39482=EDGE_CURVE('',#31063,#31559,#22850,.T.);
#39483=EDGE_CURVE('',#31559,#31560,#18531,.T.);
#39484=EDGE_CURVE('',#31345,#31560,#25402,.T.);
#39485=EDGE_CURVE('',#31561,#31558,#18532,.T.);
#39486=EDGE_CURVE('',#31560,#31561,#18533,.T.);
#39487=EDGE_CURVE('',#31562,#31345,#25403,.T.);
#39488=EDGE_CURVE('',#31562,#31563,#18534,.T.);
#39489=EDGE_CURVE('',#31064,#31563,#22851,.T.);
#39490=EDGE_CURVE('',#31563,#31564,#18535,.T.);
#39491=EDGE_CURVE('',#31346,#31564,#25404,.T.);
#39492=EDGE_CURVE('',#31565,#31562,#18536,.T.);
#39493=EDGE_CURVE('',#31564,#31565,#18537,.T.);
#39494=EDGE_CURVE('',#31566,#31346,#25405,.T.);
#39495=EDGE_CURVE('',#31566,#31567,#18538,.T.);
#39496=EDGE_CURVE('',#31065,#31567,#22852,.T.);
#39497=EDGE_CURVE('',#31567,#31568,#18539,.T.);
#39498=EDGE_CURVE('',#31347,#31568,#25406,.T.);
#39499=EDGE_CURVE('',#31569,#31566,#18540,.T.);
#39500=EDGE_CURVE('',#31568,#31569,#18541,.T.);
#39501=EDGE_CURVE('',#31570,#31460,#18542,.T.);
#39502=EDGE_CURVE('',#31571,#31570,#18543,.T.);
#39503=EDGE_CURVE('',#31461,#31571,#18544,.T.);
#39504=EDGE_CURVE('',#31570,#31347,#25407,.T.);
#39505=EDGE_CURVE('',#31290,#31572,#18545,.T.);
#39506=EDGE_CURVE('',#31572,#31458,#22853,.T.);
#39507=EDGE_CURVE('',#31573,#31290,#22854,.T.);
#39508=EDGE_CURVE('',#31352,#31573,#22855,.T.);
#39509=EDGE_CURVE('',#31291,#31573,#18546,.T.);
#39510=EDGE_CURVE('',#31574,#31291,#22856,.T.);
#39511=EDGE_CURVE('',#31356,#31574,#22857,.T.);
#39512=EDGE_CURVE('',#31292,#31574,#18547,.T.);
#39513=EDGE_CURVE('',#31575,#31292,#22858,.T.);
#39514=EDGE_CURVE('',#31360,#31575,#22859,.T.);
#39515=EDGE_CURVE('',#31293,#31575,#18548,.T.);
#39516=EDGE_CURVE('',#31576,#31293,#22860,.T.);
#39517=EDGE_CURVE('',#31364,#31576,#22861,.T.);
#39518=EDGE_CURVE('',#31294,#31576,#18549,.T.);
#39519=EDGE_CURVE('',#31577,#31294,#22862,.T.);
#39520=EDGE_CURVE('',#31368,#31577,#22863,.T.);
#39521=EDGE_CURVE('',#31295,#31577,#18550,.T.);
#39522=EDGE_CURVE('',#31578,#31295,#22864,.T.);
#39523=EDGE_CURVE('',#31372,#31578,#22865,.T.);
#39524=EDGE_CURVE('',#31296,#31578,#18551,.T.);
#39525=EDGE_CURVE('',#31579,#31296,#22866,.T.);
#39526=EDGE_CURVE('',#28969,#31579,#22867,.T.);
#39527=EDGE_CURVE('',#31297,#31579,#18552,.T.);
#39528=EDGE_CURVE('',#31580,#31297,#22868,.T.);
#39529=EDGE_CURVE('',#31376,#31580,#22869,.T.);
#39530=EDGE_CURVE('',#31298,#31580,#18553,.T.);
#39531=EDGE_CURVE('',#31581,#31298,#22870,.T.);
#39532=EDGE_CURVE('',#31380,#31581,#22871,.T.);
#39533=EDGE_CURVE('',#31299,#31581,#18554,.T.);
#39534=EDGE_CURVE('',#31582,#31299,#22872,.T.);
#39535=EDGE_CURVE('',#31384,#31582,#22873,.T.);
#39536=EDGE_CURVE('',#31300,#31582,#18555,.T.);
#39537=EDGE_CURVE('',#31583,#31300,#22874,.T.);
#39538=EDGE_CURVE('',#31388,#31583,#22875,.T.);
#39539=EDGE_CURVE('',#31301,#31583,#18556,.T.);
#39540=EDGE_CURVE('',#31584,#31301,#22876,.T.);
#39541=EDGE_CURVE('',#31392,#31584,#22877,.T.);
#39542=EDGE_CURVE('',#31302,#31584,#18557,.T.);
#39543=EDGE_CURVE('',#31585,#31302,#22878,.T.);
#39544=EDGE_CURVE('',#31396,#31585,#22879,.T.);
#39545=EDGE_CURVE('',#31303,#31585,#18558,.T.);
#39546=EDGE_CURVE('',#31586,#31303,#22880,.T.);
#39547=EDGE_CURVE('',#31400,#31586,#22881,.T.);
#39548=EDGE_CURVE('',#31304,#31586,#18559,.T.);
#39549=EDGE_CURVE('',#31587,#31304,#22882,.T.);
#39550=EDGE_CURVE('',#31404,#31587,#22883,.T.);
#39551=EDGE_CURVE('',#31305,#31587,#18560,.T.);
#39552=EDGE_CURVE('',#31588,#31305,#22884,.T.);
#39553=EDGE_CURVE('',#31408,#31588,#22885,.T.);
#39554=EDGE_CURVE('',#31306,#31588,#18561,.T.);
#39555=EDGE_CURVE('',#31589,#31306,#22886,.T.);
#39556=EDGE_CURVE('',#31412,#31589,#22887,.T.);
#39557=EDGE_CURVE('',#31307,#31589,#18562,.T.);
#39558=EDGE_CURVE('',#31590,#31307,#22888,.T.);
#39559=EDGE_CURVE('',#31416,#31590,#22889,.T.);
#39560=EDGE_CURVE('',#31308,#31590,#18563,.T.);
#39561=EDGE_CURVE('',#31591,#31308,#22890,.T.);
#39562=EDGE_CURVE('',#31420,#31591,#22891,.T.);
#39563=EDGE_CURVE('',#31309,#31591,#18564,.T.);
#39564=EDGE_CURVE('',#31592,#31309,#22892,.T.);
#39565=EDGE_CURVE('',#31424,#31592,#22893,.T.);
#39566=EDGE_CURVE('',#31310,#31592,#18565,.T.);
#39567=EDGE_CURVE('',#31593,#31310,#22894,.T.);
#39568=EDGE_CURVE('',#31429,#31593,#22895,.T.);
#39569=EDGE_CURVE('',#31311,#31593,#18566,.T.);
#39570=EDGE_CURVE('',#31594,#31311,#22896,.T.);
#39571=EDGE_CURVE('',#31433,#31594,#22897,.T.);
#39572=EDGE_CURVE('',#31312,#31594,#18567,.T.);
#39573=EDGE_CURVE('',#31595,#31312,#22898,.T.);
#39574=EDGE_CURVE('',#31436,#31595,#22899,.T.);
#39575=EDGE_CURVE('',#31313,#31595,#18568,.T.);
#39576=EDGE_CURVE('',#31596,#31313,#22900,.T.);
#39577=EDGE_CURVE('',#31440,#31596,#22901,.T.);
#39578=EDGE_CURVE('',#31314,#31596,#18569,.T.);
#39579=EDGE_CURVE('',#31597,#31314,#22902,.T.);
#39580=EDGE_CURVE('',#31444,#31597,#22903,.T.);
#39581=EDGE_CURVE('',#31315,#31597,#18570,.T.);
#39582=EDGE_CURVE('',#31598,#31315,#22904,.T.);
#39583=EDGE_CURVE('',#31448,#31598,#22905,.T.);
#39584=EDGE_CURVE('',#31316,#31598,#18571,.T.);
#39585=EDGE_CURVE('',#31599,#31316,#22906,.T.);
#39586=EDGE_CURVE('',#31452,#31599,#22907,.T.);
#39587=EDGE_CURVE('',#31317,#31599,#18572,.T.);
#39588=EDGE_CURVE('',#31600,#31317,#22908,.T.);
#39589=EDGE_CURVE('',#31456,#31600,#22909,.T.);
#39590=EDGE_CURVE('',#31318,#31600,#18573,.T.);
#39591=EDGE_CURVE('',#31572,#31318,#22910,.T.);
#39592=EDGE_CURVE('',#31601,#31571,#22911,.T.);
#39593=EDGE_CURVE('',#31319,#31601,#18574,.T.);
#39594=EDGE_CURVE('',#31602,#31319,#18575,.T.);
#39595=EDGE_CURVE('',#31465,#31602,#22912,.T.);
#39596=EDGE_CURVE('',#31320,#31602,#18576,.T.);
#39597=EDGE_CURVE('',#31603,#31320,#18577,.T.);
#39598=EDGE_CURVE('',#31469,#31603,#22913,.T.);
#39599=EDGE_CURVE('',#31321,#31603,#18578,.T.);
#39600=EDGE_CURVE('',#31604,#31321,#18579,.T.);
#39601=EDGE_CURVE('',#31473,#31604,#22914,.T.);
#39602=EDGE_CURVE('',#31322,#31604,#18580,.T.);
#39603=EDGE_CURVE('',#31605,#31322,#18581,.T.);
#39604=EDGE_CURVE('',#31477,#31605,#22915,.T.);
#39605=EDGE_CURVE('',#31323,#31605,#18582,.T.);
#39606=EDGE_CURVE('',#31606,#31323,#18583,.T.);
#39607=EDGE_CURVE('',#31481,#31606,#22916,.T.);
#39608=EDGE_CURVE('',#31324,#31606,#18584,.T.);
#39609=EDGE_CURVE('',#31607,#31324,#18585,.T.);
#39610=EDGE_CURVE('',#31485,#31607,#22917,.T.);
#39611=EDGE_CURVE('',#31325,#31607,#18586,.T.);
#39612=EDGE_CURVE('',#31608,#31325,#18587,.T.);
#39613=EDGE_CURVE('',#31489,#31608,#22918,.T.);
#39614=EDGE_CURVE('',#31326,#31608,#18588,.T.);
#39615=EDGE_CURVE('',#31609,#31326,#18589,.T.);
#39616=EDGE_CURVE('',#31493,#31609,#22919,.T.);
#39617=EDGE_CURVE('',#31327,#31609,#18590,.T.);
#39618=EDGE_CURVE('',#31610,#31327,#18591,.T.);
#39619=EDGE_CURVE('',#31497,#31610,#22920,.T.);
#39620=EDGE_CURVE('',#31328,#31610,#18592,.T.);
#39621=EDGE_CURVE('',#31611,#31328,#18593,.T.);
#39622=EDGE_CURVE('',#31501,#31611,#22921,.T.);
#39623=EDGE_CURVE('',#31329,#31611,#18594,.T.);
#39624=EDGE_CURVE('',#31612,#31329,#18595,.T.);
#39625=EDGE_CURVE('',#31505,#31612,#22922,.T.);
#39626=EDGE_CURVE('',#31330,#31612,#18596,.T.);
#39627=EDGE_CURVE('',#31613,#31330,#18597,.T.);
#39628=EDGE_CURVE('',#31509,#31613,#22923,.T.);
#39629=EDGE_CURVE('',#31331,#31613,#18598,.T.);
#39630=EDGE_CURVE('',#31614,#31331,#18599,.T.);
#39631=EDGE_CURVE('',#31513,#31614,#22924,.T.);
#39632=EDGE_CURVE('',#31332,#31614,#18600,.T.);
#39633=EDGE_CURVE('',#31615,#31332,#18601,.T.);
#39634=EDGE_CURVE('',#28963,#31615,#22925,.T.);
#39635=EDGE_CURVE('',#31333,#31615,#18602,.T.);
#39636=EDGE_CURVE('',#31616,#31333,#18603,.T.);
#39637=EDGE_CURVE('',#31517,#31616,#22926,.T.);
#39638=EDGE_CURVE('',#31334,#31616,#18604,.T.);
#39639=EDGE_CURVE('',#31617,#31334,#18605,.T.);
#39640=EDGE_CURVE('',#31521,#31617,#22927,.T.);
#39641=EDGE_CURVE('',#31335,#31617,#18606,.T.);
#39642=EDGE_CURVE('',#31618,#31335,#18607,.T.);
#39643=EDGE_CURVE('',#31525,#31618,#22928,.T.);
#39644=EDGE_CURVE('',#31336,#31618,#18608,.T.);
#39645=EDGE_CURVE('',#31619,#31336,#18609,.T.);
#39646=EDGE_CURVE('',#31529,#31619,#22929,.T.);
#39647=EDGE_CURVE('',#31337,#31619,#18610,.T.);
#39648=EDGE_CURVE('',#31620,#31337,#18611,.T.);
#39649=EDGE_CURVE('',#31533,#31620,#22930,.T.);
#39650=EDGE_CURVE('',#31338,#31620,#18612,.T.);
#39651=EDGE_CURVE('',#31621,#31338,#18613,.T.);
#39652=EDGE_CURVE('',#31537,#31621,#22931,.T.);
#39653=EDGE_CURVE('',#31339,#31621,#18614,.T.);
#39654=EDGE_CURVE('',#31622,#31339,#18615,.T.);
#39655=EDGE_CURVE('',#31541,#31622,#22932,.T.);
#39656=EDGE_CURVE('',#31340,#31622,#18616,.T.);
#39657=EDGE_CURVE('',#31623,#31340,#18617,.T.);
#39658=EDGE_CURVE('',#31545,#31623,#22933,.T.);
#39659=EDGE_CURVE('',#31341,#31623,#18618,.T.);
#39660=EDGE_CURVE('',#31624,#31341,#18619,.T.);
#39661=EDGE_CURVE('',#31549,#31624,#22934,.T.);
#39662=EDGE_CURVE('',#31342,#31624,#18620,.T.);
#39663=EDGE_CURVE('',#31625,#31342,#18621,.T.);
#39664=EDGE_CURVE('',#31553,#31625,#22935,.T.);
#39665=EDGE_CURVE('',#31343,#31625,#18622,.T.);
#39666=EDGE_CURVE('',#31626,#31343,#18623,.T.);
#39667=EDGE_CURVE('',#31557,#31626,#22936,.T.);
#39668=EDGE_CURVE('',#31344,#31626,#18624,.T.);
#39669=EDGE_CURVE('',#31627,#31344,#18625,.T.);
#39670=EDGE_CURVE('',#31561,#31627,#22937,.T.);
#39671=EDGE_CURVE('',#31345,#31627,#18626,.T.);
#39672=EDGE_CURVE('',#31628,#31345,#18627,.T.);
#39673=EDGE_CURVE('',#31565,#31628,#22938,.T.);
#39674=EDGE_CURVE('',#31346,#31628,#18628,.T.);
#39675=EDGE_CURVE('',#31629,#31346,#18629,.T.);
#39676=EDGE_CURVE('',#31569,#31629,#22939,.T.);
#39677=EDGE_CURVE('',#31347,#31629,#18630,.T.);
#39678=EDGE_CURVE('',#31601,#31347,#18631,.T.);
#39679=EDGE_CURVE('',#31630,#31631,#18632,.T.);
#39680=EDGE_CURVE('',#31290,#31631,#22940,.T.);
#39681=EDGE_CURVE('',#31630,#31572,#25408,.T.);
#39682=EDGE_CURVE('',#31632,#31630,#18633,.T.);
#39683=EDGE_CURVE('',#31633,#31632,#18634,.T.);
#39684=EDGE_CURVE('',#31631,#31633,#22941,.T.);
#39685=EDGE_CURVE('',#31573,#31633,#25409,.T.);
#39686=EDGE_CURVE('',#31634,#31635,#18635,.T.);
#39687=EDGE_CURVE('',#31291,#31635,#22942,.T.);
#39688=EDGE_CURVE('',#31634,#31573,#25410,.T.);
#39689=EDGE_CURVE('',#31636,#31634,#18636,.T.);
#39690=EDGE_CURVE('',#31637,#31636,#18637,.T.);
#39691=EDGE_CURVE('',#31635,#31637,#22943,.T.);
#39692=EDGE_CURVE('',#31574,#31637,#25411,.T.);
#39693=EDGE_CURVE('',#31638,#31639,#18638,.T.);
#39694=EDGE_CURVE('',#31292,#31639,#22944,.T.);
#39695=EDGE_CURVE('',#31638,#31574,#25412,.T.);
#39696=EDGE_CURVE('',#31640,#31638,#18639,.T.);
#39697=EDGE_CURVE('',#31641,#31640,#18640,.T.);
#39698=EDGE_CURVE('',#31639,#31641,#22945,.T.);
#39699=EDGE_CURVE('',#31575,#31641,#25413,.T.);
#39700=EDGE_CURVE('',#31642,#31643,#18641,.T.);
#39701=EDGE_CURVE('',#31293,#31643,#22946,.T.);
#39702=EDGE_CURVE('',#31642,#31575,#25414,.T.);
#39703=EDGE_CURVE('',#31644,#31642,#18642,.T.);
#39704=EDGE_CURVE('',#31645,#31644,#18643,.T.);
#39705=EDGE_CURVE('',#31643,#31645,#22947,.T.);
#39706=EDGE_CURVE('',#31576,#31645,#25415,.T.);
#39707=EDGE_CURVE('',#31646,#31647,#18644,.T.);
#39708=EDGE_CURVE('',#31294,#31647,#22948,.T.);
#39709=EDGE_CURVE('',#31646,#31576,#25416,.T.);
#39710=EDGE_CURVE('',#31648,#31646,#18645,.T.);
#39711=EDGE_CURVE('',#31649,#31648,#18646,.T.);
#39712=EDGE_CURVE('',#31647,#31649,#22949,.T.);
#39713=EDGE_CURVE('',#31577,#31649,#25417,.T.);
#39714=EDGE_CURVE('',#31650,#31651,#18647,.T.);
#39715=EDGE_CURVE('',#31295,#31651,#22950,.T.);
#39716=EDGE_CURVE('',#31650,#31577,#25418,.T.);
#39717=EDGE_CURVE('',#31652,#31650,#18648,.T.);
#39718=EDGE_CURVE('',#31653,#31652,#18649,.T.);
#39719=EDGE_CURVE('',#31651,#31653,#22951,.T.);
#39720=EDGE_CURVE('',#31578,#31653,#25419,.T.);
#39721=EDGE_CURVE('',#31654,#31655,#18650,.T.);
#39722=EDGE_CURVE('',#31296,#31655,#22952,.T.);
#39723=EDGE_CURVE('',#31654,#31578,#25420,.T.);
#39724=EDGE_CURVE('',#31656,#31654,#18651,.T.);
#39725=EDGE_CURVE('',#31657,#31656,#18652,.T.);
#39726=EDGE_CURVE('',#31655,#31657,#22953,.T.);
#39727=EDGE_CURVE('',#31579,#31657,#25421,.T.);
#39728=EDGE_CURVE('',#31658,#31659,#18653,.T.);
#39729=EDGE_CURVE('',#31297,#31659,#22954,.T.);
#39730=EDGE_CURVE('',#31658,#31579,#25422,.T.);
#39731=EDGE_CURVE('',#31660,#31658,#18654,.T.);
#39732=EDGE_CURVE('',#31661,#31660,#18655,.T.);
#39733=EDGE_CURVE('',#31659,#31661,#22955,.T.);
#39734=EDGE_CURVE('',#31580,#31661,#25423,.T.);
#39735=EDGE_CURVE('',#31662,#31663,#18656,.T.);
#39736=EDGE_CURVE('',#31298,#31663,#22956,.T.);
#39737=EDGE_CURVE('',#31662,#31580,#25424,.T.);
#39738=EDGE_CURVE('',#31664,#31662,#18657,.T.);
#39739=EDGE_CURVE('',#31665,#31664,#18658,.T.);
#39740=EDGE_CURVE('',#31663,#31665,#4442,.T.);
#39741=EDGE_CURVE('',#31581,#31665,#25425,.T.);
#39742=EDGE_CURVE('',#31666,#31667,#18659,.T.);
#39743=EDGE_CURVE('',#31299,#31667,#22957,.T.);
#39744=EDGE_CURVE('',#31666,#31581,#25426,.T.);
#39745=EDGE_CURVE('',#31668,#31666,#18660,.T.);
#39746=EDGE_CURVE('',#31669,#31668,#18661,.T.);
#39747=EDGE_CURVE('',#31667,#31669,#22958,.T.);
#39748=EDGE_CURVE('',#31582,#31669,#25427,.T.);
#39749=EDGE_CURVE('',#31670,#31671,#18662,.T.);
#39750=EDGE_CURVE('',#31300,#31671,#22959,.T.);
#39751=EDGE_CURVE('',#31670,#31582,#25428,.T.);
#39752=EDGE_CURVE('',#31672,#31670,#18663,.T.);
#39753=EDGE_CURVE('',#31673,#31672,#18664,.T.);
#39754=EDGE_CURVE('',#31671,#31673,#22960,.T.);
#39755=EDGE_CURVE('',#31583,#31673,#25429,.T.);
#39756=EDGE_CURVE('',#31674,#31675,#18665,.T.);
#39757=EDGE_CURVE('',#31301,#31675,#22961,.T.);
#39758=EDGE_CURVE('',#31674,#31583,#25430,.T.);
#39759=EDGE_CURVE('',#31676,#31674,#18666,.T.);
#39760=EDGE_CURVE('',#31677,#31676,#18667,.T.);
#39761=EDGE_CURVE('',#31675,#31677,#22962,.T.);
#39762=EDGE_CURVE('',#31584,#31677,#25431,.T.);
#39763=EDGE_CURVE('',#31678,#31679,#18668,.T.);
#39764=EDGE_CURVE('',#31302,#31679,#22963,.T.);
#39765=EDGE_CURVE('',#31678,#31584,#25432,.T.);
#39766=EDGE_CURVE('',#31680,#31678,#18669,.T.);
#39767=EDGE_CURVE('',#31681,#31680,#18670,.T.);
#39768=EDGE_CURVE('',#31679,#31681,#22964,.T.);
#39769=EDGE_CURVE('',#31585,#31681,#25433,.T.);
#39770=EDGE_CURVE('',#31682,#31683,#18671,.T.);
#39771=EDGE_CURVE('',#31303,#31683,#22965,.T.);
#39772=EDGE_CURVE('',#31682,#31585,#25434,.T.);
#39773=EDGE_CURVE('',#31684,#31682,#18672,.T.);
#39774=EDGE_CURVE('',#31685,#31684,#18673,.T.);
#39775=EDGE_CURVE('',#31683,#31685,#22966,.T.);
#39776=EDGE_CURVE('',#31586,#31685,#25435,.T.);
#39777=EDGE_CURVE('',#31304,#28959,#22967,.T.);
#39778=EDGE_CURVE('',#28958,#31586,#25436,.T.);
#39779=EDGE_CURVE('',#31587,#28961,#25437,.T.);
#39780=EDGE_CURVE('',#31686,#31687,#18674,.T.);
#39781=EDGE_CURVE('',#31305,#31687,#22968,.T.);
#39782=EDGE_CURVE('',#31686,#31587,#25438,.T.);
#39783=EDGE_CURVE('',#31688,#31686,#18675,.T.);
#39784=EDGE_CURVE('',#31689,#31688,#18676,.T.);
#39785=EDGE_CURVE('',#31687,#31689,#22969,.T.);
#39786=EDGE_CURVE('',#31588,#31689,#25439,.T.);
#39787=EDGE_CURVE('',#31690,#31691,#18677,.T.);
#39788=EDGE_CURVE('',#31306,#31691,#22970,.T.);
#39789=EDGE_CURVE('',#31690,#31588,#25440,.T.);
#39790=EDGE_CURVE('',#31692,#31690,#18678,.T.);
#39791=EDGE_CURVE('',#31693,#31692,#18679,.T.);
#39792=EDGE_CURVE('',#31691,#31693,#22971,.T.);
#39793=EDGE_CURVE('',#31589,#31693,#25441,.T.);
#39794=EDGE_CURVE('',#31694,#31695,#18680,.T.);
#39795=EDGE_CURVE('',#31307,#31695,#22972,.T.);
#39796=EDGE_CURVE('',#31694,#31589,#25442,.T.);
#39797=EDGE_CURVE('',#31696,#31694,#18681,.T.);
#39798=EDGE_CURVE('',#31697,#31696,#18682,.T.);
#39799=EDGE_CURVE('',#31695,#31697,#22973,.T.);
#39800=EDGE_CURVE('',#31590,#31697,#25443,.T.);
#39801=EDGE_CURVE('',#31698,#31699,#18683,.T.);
#39802=EDGE_CURVE('',#31308,#31699,#22974,.T.);
#39803=EDGE_CURVE('',#31698,#31590,#25444,.T.);
#39804=EDGE_CURVE('',#31700,#31698,#18684,.T.);
#39805=EDGE_CURVE('',#31701,#31700,#18685,.T.);
#39806=EDGE_CURVE('',#31699,#31701,#22975,.T.);
#39807=EDGE_CURVE('',#31591,#31701,#25445,.T.);
#39808=EDGE_CURVE('',#31702,#31703,#18686,.T.);
#39809=EDGE_CURVE('',#31309,#31703,#22976,.T.);
#39810=EDGE_CURVE('',#31702,#31591,#25446,.T.);
#39811=EDGE_CURVE('',#31704,#31702,#18687,.T.);
#39812=EDGE_CURVE('',#31705,#31704,#18688,.T.);
#39813=EDGE_CURVE('',#31703,#31705,#22977,.T.);
#39814=EDGE_CURVE('',#31592,#31705,#25447,.T.);
#39815=EDGE_CURVE('',#31706,#31707,#18689,.T.);
#39816=EDGE_CURVE('',#31310,#31707,#22978,.T.);
#39817=EDGE_CURVE('',#31706,#31592,#25448,.T.);
#39818=EDGE_CURVE('',#31707,#31708,#22979,.T.);
#39819=EDGE_CURVE('',#31593,#31708,#25449,.T.);
#39820=EDGE_CURVE('',#31709,#31706,#18690,.T.);
#39821=EDGE_CURVE('',#31708,#31709,#18691,.T.);
#39822=EDGE_CURVE('',#31710,#31593,#25450,.T.);
#39823=EDGE_CURVE('',#31710,#31711,#18692,.T.);
#39824=EDGE_CURVE('',#31311,#31711,#22980,.T.);
#39825=EDGE_CURVE('',#31711,#31712,#22981,.T.);
#39826=EDGE_CURVE('',#31713,#31710,#18693,.T.);
#39827=EDGE_CURVE('',#31712,#31713,#18694,.T.);
#39828=EDGE_CURVE('',#31594,#31712,#25451,.T.);
#39829=EDGE_CURVE('',#31714,#31715,#18695,.T.);
#39830=EDGE_CURVE('',#31312,#31715,#22982,.T.);
#39831=EDGE_CURVE('',#31714,#31594,#25452,.T.);
#39832=EDGE_CURVE('',#31716,#31714,#18696,.T.);
#39833=EDGE_CURVE('',#31717,#31716,#18697,.T.);
#39834=EDGE_CURVE('',#31715,#31717,#22983,.T.);
#39835=EDGE_CURVE('',#31595,#31717,#25453,.T.);
#39836=EDGE_CURVE('',#31718,#31719,#18698,.T.);
#39837=EDGE_CURVE('',#31313,#31719,#22984,.T.);
#39838=EDGE_CURVE('',#31718,#31595,#25454,.T.);
#39839=EDGE_CURVE('',#31720,#31718,#18699,.T.);
#39840=EDGE_CURVE('',#31721,#31720,#18700,.T.);
#39841=EDGE_CURVE('',#31719,#31721,#22985,.T.);
#39842=EDGE_CURVE('',#31596,#31721,#25455,.T.);
#39843=EDGE_CURVE('',#31722,#31723,#18701,.T.);
#39844=EDGE_CURVE('',#31314,#31723,#22986,.T.);
#39845=EDGE_CURVE('',#31722,#31596,#25456,.T.);
#39846=EDGE_CURVE('',#31724,#31722,#18702,.T.);
#39847=EDGE_CURVE('',#31725,#31724,#18703,.T.);
#39848=EDGE_CURVE('',#31723,#31725,#22987,.T.);
#39849=EDGE_CURVE('',#31597,#31725,#25457,.T.);
#39850=EDGE_CURVE('',#31726,#31727,#18704,.T.);
#39851=EDGE_CURVE('',#31315,#31727,#22988,.T.);
#39852=EDGE_CURVE('',#31726,#31597,#25458,.T.);
#39853=EDGE_CURVE('',#31728,#31726,#18705,.T.);
#39854=EDGE_CURVE('',#31729,#31728,#18706,.T.);
#39855=EDGE_CURVE('',#31727,#31729,#22989,.T.);
#39856=EDGE_CURVE('',#31598,#31729,#25459,.T.);
#39857=EDGE_CURVE('',#31730,#31731,#18707,.T.);
#39858=EDGE_CURVE('',#31316,#31731,#22990,.T.);
#39859=EDGE_CURVE('',#31730,#31598,#25460,.T.);
#39860=EDGE_CURVE('',#31732,#31730,#18708,.T.);
#39861=EDGE_CURVE('',#31733,#31732,#18709,.T.);
#39862=EDGE_CURVE('',#31731,#31733,#22991,.T.);
#39863=EDGE_CURVE('',#31599,#31733,#25461,.T.);
#39864=EDGE_CURVE('',#31734,#31735,#18710,.T.);
#39865=EDGE_CURVE('',#31317,#31735,#22992,.T.);
#39866=EDGE_CURVE('',#31734,#31599,#25462,.T.);
#39867=EDGE_CURVE('',#31736,#31734,#18711,.T.);
#39868=EDGE_CURVE('',#31737,#31736,#18712,.T.);
#39869=EDGE_CURVE('',#31735,#31737,#22993,.T.);
#39870=EDGE_CURVE('',#31600,#31737,#25463,.T.);
#39871=EDGE_CURVE('',#31738,#31739,#18713,.T.);
#39872=EDGE_CURVE('',#31318,#31739,#22994,.T.);
#39873=EDGE_CURVE('',#31738,#31600,#25464,.T.);
#39874=EDGE_CURVE('',#31740,#31738,#18714,.T.);
#39875=EDGE_CURVE('',#31741,#31740,#18715,.T.);
#39876=EDGE_CURVE('',#31739,#31741,#22995,.T.);
#39877=EDGE_CURVE('',#31572,#31741,#25465,.T.);
#39878=EDGE_CURVE('',#31742,#31601,#25466,.T.);
#39879=EDGE_CURVE('',#31742,#31743,#18716,.T.);
#39880=EDGE_CURVE('',#31319,#31743,#22996,.T.);
#39881=EDGE_CURVE('',#31743,#31744,#18717,.T.);
#39882=EDGE_CURVE('',#31602,#31744,#25467,.T.);
#39883=EDGE_CURVE('',#31745,#31742,#18718,.T.);
#39884=EDGE_CURVE('',#31744,#31745,#18719,.T.);
#39885=EDGE_CURVE('',#31746,#31602,#25468,.T.);
#39886=EDGE_CURVE('',#31746,#31747,#18720,.T.);
#39887=EDGE_CURVE('',#31320,#31747,#22997,.T.);
#39888=EDGE_CURVE('',#31747,#31748,#18721,.T.);
#39889=EDGE_CURVE('',#31603,#31748,#25469,.T.);
#39890=EDGE_CURVE('',#31749,#31746,#18722,.T.);
#39891=EDGE_CURVE('',#31748,#31749,#18723,.T.);
#39892=EDGE_CURVE('',#31750,#31603,#25470,.T.);
#39893=EDGE_CURVE('',#31750,#31751,#18724,.T.);
#39894=EDGE_CURVE('',#31321,#31751,#22998,.T.);
#39895=EDGE_CURVE('',#31751,#31752,#18725,.T.);
#39896=EDGE_CURVE('',#31604,#31752,#25471,.T.);
#39897=EDGE_CURVE('',#31753,#31750,#18726,.T.);
#39898=EDGE_CURVE('',#31752,#31753,#18727,.T.);
#39899=EDGE_CURVE('',#31754,#31604,#25472,.T.);
#39900=EDGE_CURVE('',#31754,#31755,#18728,.T.);
#39901=EDGE_CURVE('',#31322,#31755,#22999,.T.);
#39902=EDGE_CURVE('',#31755,#31756,#18729,.T.);
#39903=EDGE_CURVE('',#31605,#31756,#25473,.T.);
#39904=EDGE_CURVE('',#31757,#31754,#18730,.T.);
#39905=EDGE_CURVE('',#31756,#31757,#18731,.T.);
#39906=EDGE_CURVE('',#31758,#31605,#25474,.T.);
#39907=EDGE_CURVE('',#31758,#31759,#18732,.T.);
#39908=EDGE_CURVE('',#31323,#31759,#23000,.T.);
#39909=EDGE_CURVE('',#31759,#31760,#18733,.T.);
#39910=EDGE_CURVE('',#31606,#31760,#25475,.T.);
#39911=EDGE_CURVE('',#31761,#31758,#18734,.T.);
#39912=EDGE_CURVE('',#31760,#31761,#18735,.T.);
#39913=EDGE_CURVE('',#31762,#31606,#25476,.T.);
#39914=EDGE_CURVE('',#31762,#31763,#18736,.T.);
#39915=EDGE_CURVE('',#31324,#31763,#23001,.T.);
#39916=EDGE_CURVE('',#31763,#31764,#18737,.T.);
#39917=EDGE_CURVE('',#31607,#31764,#25477,.T.);
#39918=EDGE_CURVE('',#31765,#31762,#18738,.T.);
#39919=EDGE_CURVE('',#31764,#31765,#18739,.T.);
#39920=EDGE_CURVE('',#31766,#31607,#25478,.T.);
#39921=EDGE_CURVE('',#31766,#31767,#18740,.T.);
#39922=EDGE_CURVE('',#31325,#31767,#23002,.T.);
#39923=EDGE_CURVE('',#31767,#31768,#18741,.T.);
#39924=EDGE_CURVE('',#31608,#31768,#25479,.T.);
#39925=EDGE_CURVE('',#31769,#31766,#18742,.T.);
#39926=EDGE_CURVE('',#31768,#31769,#18743,.T.);
#39927=EDGE_CURVE('',#31770,#31608,#25480,.T.);
#39928=EDGE_CURVE('',#31770,#31771,#18744,.T.);
#39929=EDGE_CURVE('',#31326,#31771,#23003,.T.);
#39930=EDGE_CURVE('',#31771,#31772,#18745,.T.);
#39931=EDGE_CURVE('',#31609,#31772,#25481,.T.);
#39932=EDGE_CURVE('',#31773,#31770,#18746,.T.);
#39933=EDGE_CURVE('',#31772,#31773,#18747,.T.);
#39934=EDGE_CURVE('',#31774,#31609,#25482,.T.);
#39935=EDGE_CURVE('',#31774,#31775,#18748,.T.);
#39936=EDGE_CURVE('',#31327,#31775,#23004,.T.);
#39937=EDGE_CURVE('',#31775,#31776,#18749,.T.);
#39938=EDGE_CURVE('',#31610,#31776,#25483,.T.);
#39939=EDGE_CURVE('',#31777,#31774,#18750,.T.);
#39940=EDGE_CURVE('',#31776,#31777,#18751,.T.);
#39941=EDGE_CURVE('',#31778,#31610,#25484,.T.);
#39942=EDGE_CURVE('',#31778,#31779,#18752,.T.);
#39943=EDGE_CURVE('',#31328,#31779,#23005,.T.);
#39944=EDGE_CURVE('',#31779,#31780,#18753,.T.);
#39945=EDGE_CURVE('',#31611,#31780,#25485,.T.);
#39946=EDGE_CURVE('',#31781,#31778,#18754,.T.);
#39947=EDGE_CURVE('',#31780,#31781,#18755,.T.);
#39948=EDGE_CURVE('',#31782,#31611,#25486,.T.);
#39949=EDGE_CURVE('',#31782,#31783,#18756,.T.);
#39950=EDGE_CURVE('',#31329,#31783,#23006,.T.);
#39951=EDGE_CURVE('',#31783,#31784,#18757,.T.);
#39952=EDGE_CURVE('',#31612,#31784,#25487,.T.);
#39953=EDGE_CURVE('',#31785,#31782,#18758,.T.);
#39954=EDGE_CURVE('',#31784,#31785,#18759,.T.);
#39955=EDGE_CURVE('',#31786,#31612,#25488,.T.);
#39956=EDGE_CURVE('',#31786,#31787,#18760,.T.);
#39957=EDGE_CURVE('',#31330,#31787,#23007,.T.);
#39958=EDGE_CURVE('',#31787,#31788,#18761,.T.);
#39959=EDGE_CURVE('',#31613,#31788,#25489,.T.);
#39960=EDGE_CURVE('',#31789,#31786,#18762,.T.);
#39961=EDGE_CURVE('',#31788,#31789,#18763,.T.);
#39962=EDGE_CURVE('',#31790,#31613,#25490,.T.);
#39963=EDGE_CURVE('',#31790,#31791,#18764,.T.);
#39964=EDGE_CURVE('',#31331,#31791,#23008,.T.);
#39965=EDGE_CURVE('',#31791,#31792,#18765,.T.);
#39966=EDGE_CURVE('',#31614,#31792,#25491,.T.);
#39967=EDGE_CURVE('',#31793,#31790,#18766,.T.);
#39968=EDGE_CURVE('',#31792,#31793,#18767,.T.);
#39969=EDGE_CURVE('',#31794,#31614,#25492,.T.);
#39970=EDGE_CURVE('',#31794,#31795,#18768,.T.);
#39971=EDGE_CURVE('',#31332,#31795,#23009,.T.);
#39972=EDGE_CURVE('',#31795,#31796,#18769,.T.);
#39973=EDGE_CURVE('',#31615,#31796,#25493,.T.);
#39974=EDGE_CURVE('',#31797,#31794,#18770,.T.);
#39975=EDGE_CURVE('',#31796,#31797,#18771,.T.);
#39976=EDGE_CURVE('',#31798,#31615,#25494,.T.);
#39977=EDGE_CURVE('',#31798,#31799,#18772,.T.);
#39978=EDGE_CURVE('',#31333,#31799,#23010,.T.);
#39979=EDGE_CURVE('',#31799,#31800,#18773,.T.);
#39980=EDGE_CURVE('',#31616,#31800,#25495,.T.);
#39981=EDGE_CURVE('',#31801,#31798,#18774,.T.);
#39982=EDGE_CURVE('',#31800,#31801,#18775,.T.);
#39983=EDGE_CURVE('',#31802,#31616,#25496,.T.);
#39984=EDGE_CURVE('',#31802,#31803,#18776,.T.);
#39985=EDGE_CURVE('',#31334,#31803,#23011,.T.);
#39986=EDGE_CURVE('',#31803,#31804,#18777,.T.);
#39987=EDGE_CURVE('',#31617,#31804,#25497,.T.);
#39988=EDGE_CURVE('',#31805,#31802,#18778,.T.);
#39989=EDGE_CURVE('',#31804,#31805,#18779,.T.);
#39990=EDGE_CURVE('',#31806,#31617,#25498,.T.);
#39991=EDGE_CURVE('',#31806,#31807,#18780,.T.);
#39992=EDGE_CURVE('',#31335,#31807,#23012,.T.);
#39993=EDGE_CURVE('',#31807,#31808,#18781,.T.);
#39994=EDGE_CURVE('',#31618,#31808,#25499,.T.);
#39995=EDGE_CURVE('',#31809,#31806,#18782,.T.);
#39996=EDGE_CURVE('',#31808,#31809,#18783,.T.);
#39997=EDGE_CURVE('',#31810,#31618,#25500,.T.);
#39998=EDGE_CURVE('',#31810,#31811,#18784,.T.);
#39999=EDGE_CURVE('',#31336,#31811,#23013,.T.);
#40000=EDGE_CURVE('',#31811,#31812,#18785,.T.);
#40001=EDGE_CURVE('',#31619,#31812,#25501,.T.);
#40002=EDGE_CURVE('',#31813,#31810,#18786,.T.);
#40003=EDGE_CURVE('',#31812,#31813,#18787,.T.);
#40004=EDGE_CURVE('',#31814,#31619,#25502,.T.);
#40005=EDGE_CURVE('',#31814,#31815,#18788,.T.);
#40006=EDGE_CURVE('',#31337,#31815,#23014,.T.);
#40007=EDGE_CURVE('',#31815,#31816,#18789,.T.);
#40008=EDGE_CURVE('',#31620,#31816,#25503,.T.);
#40009=EDGE_CURVE('',#31817,#31814,#18790,.T.);
#40010=EDGE_CURVE('',#31816,#31817,#18791,.T.);
#40011=EDGE_CURVE('',#31818,#31620,#25504,.T.);
#40012=EDGE_CURVE('',#31818,#31819,#18792,.T.);
#40013=EDGE_CURVE('',#31338,#31819,#23015,.T.);
#40014=EDGE_CURVE('',#31819,#31820,#18793,.T.);
#40015=EDGE_CURVE('',#31621,#31820,#25505,.T.);
#40016=EDGE_CURVE('',#31821,#31818,#18794,.T.);
#40017=EDGE_CURVE('',#31820,#31821,#18795,.T.);
#40018=EDGE_CURVE('',#31822,#31621,#25506,.T.);
#40019=EDGE_CURVE('',#31822,#31823,#18796,.T.);
#40020=EDGE_CURVE('',#31339,#31823,#23016,.T.);
#40021=EDGE_CURVE('',#31823,#31824,#18797,.T.);
#40022=EDGE_CURVE('',#31622,#31824,#25507,.T.);
#40023=EDGE_CURVE('',#31825,#31822,#18798,.T.);
#40024=EDGE_CURVE('',#31824,#31825,#18799,.T.);
#40025=EDGE_CURVE('',#31826,#31622,#25508,.T.);
#40026=EDGE_CURVE('',#31826,#31827,#18800,.T.);
#40027=EDGE_CURVE('',#31340,#31827,#23017,.T.);
#40028=EDGE_CURVE('',#31827,#31828,#18801,.T.);
#40029=EDGE_CURVE('',#31623,#31828,#25509,.T.);
#40030=EDGE_CURVE('',#31829,#31826,#18802,.T.);
#40031=EDGE_CURVE('',#31828,#31829,#18803,.T.);
#40032=EDGE_CURVE('',#31830,#31623,#25510,.T.);
#40033=EDGE_CURVE('',#31830,#31831,#18804,.T.);
#40034=EDGE_CURVE('',#31341,#31831,#23018,.T.);
#40035=EDGE_CURVE('',#31831,#31832,#18805,.T.);
#40036=EDGE_CURVE('',#31624,#31832,#25511,.T.);
#40037=EDGE_CURVE('',#31833,#31830,#18806,.T.);
#40038=EDGE_CURVE('',#31832,#31833,#18807,.T.);
#40039=EDGE_CURVE('',#31834,#31624,#25512,.T.);
#40040=EDGE_CURVE('',#31834,#31835,#18808,.T.);
#40041=EDGE_CURVE('',#31342,#31835,#23019,.T.);
#40042=EDGE_CURVE('',#31835,#31836,#18809,.T.);
#40043=EDGE_CURVE('',#31625,#31836,#25513,.T.);
#40044=EDGE_CURVE('',#31837,#31834,#18810,.T.);
#40045=EDGE_CURVE('',#31836,#31837,#18811,.T.);
#40046=EDGE_CURVE('',#31838,#31625,#25514,.T.);
#40047=EDGE_CURVE('',#31838,#31839,#18812,.T.);
#40048=EDGE_CURVE('',#31343,#31839,#23020,.T.);
#40049=EDGE_CURVE('',#31839,#31840,#18813,.T.);
#40050=EDGE_CURVE('',#31626,#31840,#25515,.T.);
#40051=EDGE_CURVE('',#31841,#31838,#18814,.T.);
#40052=EDGE_CURVE('',#31840,#31841,#18815,.T.);
#40053=EDGE_CURVE('',#31842,#31626,#25516,.T.);
#40054=EDGE_CURVE('',#31842,#31843,#18816,.T.);
#40055=EDGE_CURVE('',#31344,#31843,#23021,.T.);
#40056=EDGE_CURVE('',#31843,#31844,#18817,.T.);
#40057=EDGE_CURVE('',#31627,#31844,#25517,.T.);
#40058=EDGE_CURVE('',#31845,#31842,#18818,.T.);
#40059=EDGE_CURVE('',#31844,#31845,#18819,.T.);
#40060=EDGE_CURVE('',#31846,#31627,#25518,.T.);
#40061=EDGE_CURVE('',#31846,#31847,#18820,.T.);
#40062=EDGE_CURVE('',#31345,#31847,#23022,.T.);
#40063=EDGE_CURVE('',#31847,#31848,#18821,.T.);
#40064=EDGE_CURVE('',#31628,#31848,#25519,.T.);
#40065=EDGE_CURVE('',#31849,#31846,#18822,.T.);
#40066=EDGE_CURVE('',#31848,#31849,#18823,.T.);
#40067=EDGE_CURVE('',#31850,#31628,#25520,.T.);
#40068=EDGE_CURVE('',#31850,#31851,#18824,.T.);
#40069=EDGE_CURVE('',#31346,#31851,#23023,.T.);
#40070=EDGE_CURVE('',#31851,#31852,#18825,.T.);
#40071=EDGE_CURVE('',#31629,#31852,#25521,.T.);
#40072=EDGE_CURVE('',#31853,#31850,#18826,.T.);
#40073=EDGE_CURVE('',#31852,#31853,#18827,.T.);
#40074=EDGE_CURVE('',#31854,#31629,#25522,.T.);
#40075=EDGE_CURVE('',#31854,#31855,#18828,.T.);
#40076=EDGE_CURVE('',#31347,#31855,#23024,.T.);
#40077=EDGE_CURVE('',#31855,#31856,#18829,.T.);
#40078=EDGE_CURVE('',#31601,#31856,#25523,.T.);
#40079=EDGE_CURVE('',#31857,#31854,#18830,.T.);
#40080=EDGE_CURVE('',#31856,#31857,#18831,.T.);
#40081=EDGE_CURVE('',#31858,#31572,#18832,.T.);
#40082=EDGE_CURVE('',#31632,#31858,#23025,.T.);
#40083=EDGE_CURVE('',#31573,#31858,#23026,.T.);
#40084=EDGE_CURVE('',#31859,#31573,#18833,.T.);
#40085=EDGE_CURVE('',#31636,#31859,#23027,.T.);
#40086=EDGE_CURVE('',#31574,#31859,#23028,.T.);
#40087=EDGE_CURVE('',#31860,#31574,#18834,.T.);
#40088=EDGE_CURVE('',#31640,#31860,#23029,.T.);
#40089=EDGE_CURVE('',#31575,#31860,#23030,.T.);
#40090=EDGE_CURVE('',#31861,#31575,#18835,.T.);
#40091=EDGE_CURVE('',#31644,#31861,#23031,.T.);
#40092=EDGE_CURVE('',#31576,#31861,#23032,.T.);
#40093=EDGE_CURVE('',#31862,#31576,#18836,.T.);
#40094=EDGE_CURVE('',#31648,#31862,#23033,.T.);
#40095=EDGE_CURVE('',#31577,#31862,#23034,.T.);
#40096=EDGE_CURVE('',#31863,#31577,#18837,.T.);
#40097=EDGE_CURVE('',#31652,#31863,#23035,.T.);
#40098=EDGE_CURVE('',#31578,#31863,#23036,.T.);
#40099=EDGE_CURVE('',#31864,#31578,#18838,.T.);
#40100=EDGE_CURVE('',#31656,#31864,#23037,.T.);
#40101=EDGE_CURVE('',#31579,#31864,#23038,.T.);
#40102=EDGE_CURVE('',#31865,#31579,#18839,.T.);
#40103=EDGE_CURVE('',#31660,#31865,#23039,.T.);
#40104=EDGE_CURVE('',#31580,#31865,#23040,.T.);
#40105=EDGE_CURVE('',#31866,#31580,#18840,.T.);
#40106=EDGE_CURVE('',#31664,#31866,#23041,.T.);
#40107=EDGE_CURVE('',#31581,#31866,#23042,.T.);
#40108=EDGE_CURVE('',#31867,#31581,#18841,.T.);
#40109=EDGE_CURVE('',#31668,#31867,#23043,.T.);
#40110=EDGE_CURVE('',#31582,#31867,#23044,.T.);
#40111=EDGE_CURVE('',#31868,#31582,#18842,.T.);
#40112=EDGE_CURVE('',#31672,#31868,#23045,.T.);
#40113=EDGE_CURVE('',#31583,#31868,#23046,.T.);
#40114=EDGE_CURVE('',#31869,#31583,#18843,.T.);
#40115=EDGE_CURVE('',#31676,#31869,#23047,.T.);
#40116=EDGE_CURVE('',#31584,#31869,#23048,.T.);
#40117=EDGE_CURVE('',#31870,#31584,#18844,.T.);
#40118=EDGE_CURVE('',#31680,#31870,#23049,.T.);
#40119=EDGE_CURVE('',#31585,#31870,#23050,.T.);
#40120=EDGE_CURVE('',#31871,#31585,#18845,.T.);
#40121=EDGE_CURVE('',#31684,#31871,#23051,.T.);
#40122=EDGE_CURVE('',#31586,#31871,#23052,.T.);
#40123=EDGE_CURVE('',#31872,#31586,#18846,.T.);
#40124=EDGE_CURVE('',#28960,#31872,#23053,.T.);
#40125=EDGE_CURVE('',#31587,#31872,#23054,.T.);
#40126=EDGE_CURVE('',#31873,#31587,#18847,.T.);
#40127=EDGE_CURVE('',#31688,#31873,#23055,.T.);
#40128=EDGE_CURVE('',#31588,#31873,#23056,.T.);
#40129=EDGE_CURVE('',#31874,#31588,#18848,.T.);
#40130=EDGE_CURVE('',#31692,#31874,#23057,.T.);
#40131=EDGE_CURVE('',#31589,#31874,#23058,.T.);
#40132=EDGE_CURVE('',#31875,#31589,#18849,.T.);
#40133=EDGE_CURVE('',#31696,#31875,#23059,.T.);
#40134=EDGE_CURVE('',#31590,#31875,#23060,.T.);
#40135=EDGE_CURVE('',#31876,#31590,#18850,.T.);
#40136=EDGE_CURVE('',#31700,#31876,#23061,.T.);
#40137=EDGE_CURVE('',#31591,#31876,#23062,.T.);
#40138=EDGE_CURVE('',#31877,#31591,#18851,.T.);
#40139=EDGE_CURVE('',#31704,#31877,#23063,.T.);
#40140=EDGE_CURVE('',#31592,#31877,#23064,.T.);
#40141=EDGE_CURVE('',#31878,#31592,#18852,.T.);
#40142=EDGE_CURVE('',#31709,#31878,#23065,.T.);
#40143=EDGE_CURVE('',#31593,#31878,#23066,.T.);
#40144=EDGE_CURVE('',#31879,#31593,#18853,.T.);
#40145=EDGE_CURVE('',#31713,#31879,#23067,.T.);
#40146=EDGE_CURVE('',#31594,#31879,#23068,.T.);
#40147=EDGE_CURVE('',#31880,#31594,#18854,.T.);
#40148=EDGE_CURVE('',#31716,#31880,#23069,.T.);
#40149=EDGE_CURVE('',#31595,#31880,#23070,.T.);
#40150=EDGE_CURVE('',#31881,#31595,#18855,.T.);
#40151=EDGE_CURVE('',#31720,#31881,#23071,.T.);
#40152=EDGE_CURVE('',#31596,#31881,#23072,.T.);
#40153=EDGE_CURVE('',#31882,#31596,#18856,.T.);
#40154=EDGE_CURVE('',#31724,#31882,#23073,.T.);
#40155=EDGE_CURVE('',#31597,#31882,#23074,.T.);
#40156=EDGE_CURVE('',#31883,#31597,#18857,.T.);
#40157=EDGE_CURVE('',#31728,#31883,#23075,.T.);
#40158=EDGE_CURVE('',#31598,#31883,#23076,.T.);
#40159=EDGE_CURVE('',#31884,#31598,#18858,.T.);
#40160=EDGE_CURVE('',#31732,#31884,#23077,.T.);
#40161=EDGE_CURVE('',#31599,#31884,#23078,.T.);
#40162=EDGE_CURVE('',#31885,#31599,#18859,.T.);
#40163=EDGE_CURVE('',#31736,#31885,#23079,.T.);
#40164=EDGE_CURVE('',#31600,#31885,#23080,.T.);
#40165=EDGE_CURVE('',#31886,#31600,#18860,.T.);
#40166=EDGE_CURVE('',#31740,#31886,#23081,.T.);
#40167=EDGE_CURVE('',#31572,#31886,#23082,.T.);
#40168=EDGE_CURVE('',#31887,#31601,#18861,.T.);
#40169=EDGE_CURVE('',#31745,#31887,#23083,.T.);
#40170=EDGE_CURVE('',#31602,#31887,#23084,.T.);
#40171=EDGE_CURVE('',#31888,#31602,#18862,.T.);
#40172=EDGE_CURVE('',#31749,#31888,#23085,.T.);
#40173=EDGE_CURVE('',#31603,#31888,#23086,.T.);
#40174=EDGE_CURVE('',#31889,#31603,#18863,.T.);
#40175=EDGE_CURVE('',#31753,#31889,#23087,.T.);
#40176=EDGE_CURVE('',#31604,#31889,#23088,.T.);
#40177=EDGE_CURVE('',#31890,#31604,#18864,.T.);
#40178=EDGE_CURVE('',#31757,#31890,#23089,.T.);
#40179=EDGE_CURVE('',#31605,#31890,#23090,.T.);
#40180=EDGE_CURVE('',#31891,#31605,#18865,.T.);
#40181=EDGE_CURVE('',#31761,#31891,#23091,.T.);
#40182=EDGE_CURVE('',#31606,#31891,#23092,.T.);
#40183=EDGE_CURVE('',#31892,#31606,#18866,.T.);
#40184=EDGE_CURVE('',#31765,#31892,#23093,.T.);
#40185=EDGE_CURVE('',#31607,#31892,#23094,.T.);
#40186=EDGE_CURVE('',#31893,#31607,#18867,.T.);
#40187=EDGE_CURVE('',#31769,#31893,#23095,.T.);
#40188=EDGE_CURVE('',#31608,#31893,#23096,.T.);
#40189=EDGE_CURVE('',#31894,#31608,#18868,.T.);
#40190=EDGE_CURVE('',#31773,#31894,#23097,.T.);
#40191=EDGE_CURVE('',#31609,#31894,#23098,.T.);
#40192=EDGE_CURVE('',#31895,#31609,#18869,.T.);
#40193=EDGE_CURVE('',#31777,#31895,#23099,.T.);
#40194=EDGE_CURVE('',#31610,#31895,#23100,.T.);
#40195=EDGE_CURVE('',#31896,#31610,#18870,.T.);
#40196=EDGE_CURVE('',#31781,#31896,#23101,.T.);
#40197=EDGE_CURVE('',#31611,#31896,#23102,.T.);
#40198=EDGE_CURVE('',#31897,#31611,#18871,.T.);
#40199=EDGE_CURVE('',#31785,#31897,#23103,.T.);
#40200=EDGE_CURVE('',#31612,#31897,#4443,.T.);
#40201=EDGE_CURVE('',#31898,#31612,#18872,.T.);
#40202=EDGE_CURVE('',#31789,#31898,#23104,.T.);
#40203=EDGE_CURVE('',#31613,#31898,#4444,.T.);
#40204=EDGE_CURVE('',#31899,#31613,#18873,.T.);
#40205=EDGE_CURVE('',#31793,#31899,#23105,.T.);
#40206=EDGE_CURVE('',#31614,#31899,#23106,.T.);
#40207=EDGE_CURVE('',#31900,#31614,#18874,.T.);
#40208=EDGE_CURVE('',#31797,#31900,#23107,.T.);
#40209=EDGE_CURVE('',#31615,#31900,#23108,.T.);
#40210=EDGE_CURVE('',#31901,#31615,#18875,.T.);
#40211=EDGE_CURVE('',#31801,#31901,#23109,.T.);
#40212=EDGE_CURVE('',#31616,#31901,#23110,.T.);
#40213=EDGE_CURVE('',#31902,#31616,#18876,.T.);
#40214=EDGE_CURVE('',#31805,#31902,#23111,.T.);
#40215=EDGE_CURVE('',#31617,#31902,#4445,.T.);
#40216=EDGE_CURVE('',#31903,#31617,#18877,.T.);
#40217=EDGE_CURVE('',#31809,#31903,#23112,.T.);
#40218=EDGE_CURVE('',#31618,#31903,#23113,.T.);
#40219=EDGE_CURVE('',#31904,#31618,#18878,.T.);
#40220=EDGE_CURVE('',#31813,#31904,#23114,.T.);
#40221=EDGE_CURVE('',#31619,#31904,#4446,.T.);
#40222=EDGE_CURVE('',#31905,#31619,#18879,.T.);
#40223=EDGE_CURVE('',#31817,#31905,#23115,.T.);
#40224=EDGE_CURVE('',#31620,#31905,#23116,.T.);
#40225=EDGE_CURVE('',#31906,#31620,#18880,.T.);
#40226=EDGE_CURVE('',#31821,#31906,#23117,.T.);
#40227=EDGE_CURVE('',#31621,#31906,#23118,.T.);
#40228=EDGE_CURVE('',#31907,#31621,#18881,.T.);
#40229=EDGE_CURVE('',#31825,#31907,#23119,.T.);
#40230=EDGE_CURVE('',#31622,#31907,#23120,.T.);
#40231=EDGE_CURVE('',#31908,#31622,#18882,.T.);
#40232=EDGE_CURVE('',#31829,#31908,#23121,.T.);
#40233=EDGE_CURVE('',#31623,#31908,#23122,.T.);
#40234=EDGE_CURVE('',#31909,#31623,#18883,.T.);
#40235=EDGE_CURVE('',#31833,#31909,#23123,.T.);
#40236=EDGE_CURVE('',#31624,#31909,#23124,.T.);
#40237=EDGE_CURVE('',#31910,#31624,#18884,.T.);
#40238=EDGE_CURVE('',#31837,#31910,#23125,.T.);
#40239=EDGE_CURVE('',#31625,#31910,#4447,.T.);
#40240=EDGE_CURVE('',#31911,#31625,#18885,.T.);
#40241=EDGE_CURVE('',#31841,#31911,#23126,.T.);
#40242=EDGE_CURVE('',#31626,#31911,#4448,.T.);
#40243=EDGE_CURVE('',#31912,#31626,#18886,.T.);
#40244=EDGE_CURVE('',#31845,#31912,#23127,.T.);
#40245=EDGE_CURVE('',#31627,#31912,#23128,.T.);
#40246=EDGE_CURVE('',#31913,#31627,#18887,.T.);
#40247=EDGE_CURVE('',#31849,#31913,#23129,.T.);
#40248=EDGE_CURVE('',#31628,#31913,#4449,.T.);
#40249=EDGE_CURVE('',#31914,#31628,#18888,.T.);
#40250=EDGE_CURVE('',#31853,#31914,#23130,.T.);
#40251=EDGE_CURVE('',#31629,#31914,#23131,.T.);
#40252=EDGE_CURVE('',#31915,#31629,#18889,.T.);
#40253=EDGE_CURVE('',#31857,#31915,#23132,.T.);
#40254=EDGE_CURVE('',#31601,#31915,#23133,.T.);
#40255=EDGE_CURVE('',#31916,#31917,#18890,.T.);
#40256=EDGE_CURVE('',#31858,#31917,#25524,.T.);
#40257=EDGE_CURVE('',#31916,#31572,#23134,.T.);
#40258=EDGE_CURVE('',#31918,#31919,#23135,.T.);
#40259=EDGE_CURVE('',#31573,#31919,#23136,.T.);
#40260=EDGE_CURVE('',#31918,#31858,#25525,.T.);
#40261=EDGE_CURVE('',#31920,#31918,#18891,.T.);
#40262=EDGE_CURVE('',#31921,#31920,#18892,.T.);
#40263=EDGE_CURVE('',#31919,#31921,#18893,.T.);
#40264=EDGE_CURVE('',#31859,#31921,#25526,.T.);
#40265=EDGE_CURVE('',#31922,#31923,#23137,.T.);
#40266=EDGE_CURVE('',#31574,#31923,#23138,.T.);
#40267=EDGE_CURVE('',#31922,#31859,#25527,.T.);
#40268=EDGE_CURVE('',#31924,#31922,#18894,.T.);
#40269=EDGE_CURVE('',#31925,#31924,#18895,.T.);
#40270=EDGE_CURVE('',#31923,#31925,#18896,.T.);
#40271=EDGE_CURVE('',#31860,#31925,#25528,.T.);
#40272=EDGE_CURVE('',#31926,#31927,#23139,.T.);
#40273=EDGE_CURVE('',#31575,#31927,#23140,.T.);
#40274=EDGE_CURVE('',#31926,#31860,#25529,.T.);
#40275=EDGE_CURVE('',#31928,#31926,#18897,.T.);
#40276=EDGE_CURVE('',#31929,#31928,#18898,.T.);
#40277=EDGE_CURVE('',#31927,#31929,#18899,.T.);
#40278=EDGE_CURVE('',#31861,#31929,#25530,.T.);
#40279=EDGE_CURVE('',#31930,#31931,#23141,.T.);
#40280=EDGE_CURVE('',#31576,#31931,#23142,.T.);
#40281=EDGE_CURVE('',#31930,#31861,#25531,.T.);
#40282=EDGE_CURVE('',#31932,#31930,#18900,.T.);
#40283=EDGE_CURVE('',#31933,#31932,#18901,.T.);
#40284=EDGE_CURVE('',#31931,#31933,#18902,.T.);
#40285=EDGE_CURVE('',#31862,#31933,#25532,.T.);
#40286=EDGE_CURVE('',#31934,#31935,#23143,.T.);
#40287=EDGE_CURVE('',#31577,#31935,#23144,.T.);
#40288=EDGE_CURVE('',#31934,#31862,#25533,.T.);
#40289=EDGE_CURVE('',#31936,#31934,#18903,.T.);
#40290=EDGE_CURVE('',#31937,#31936,#18904,.T.);
#40291=EDGE_CURVE('',#31935,#31937,#18905,.T.);
#40292=EDGE_CURVE('',#31863,#31937,#25534,.T.);
#40293=EDGE_CURVE('',#31938,#31939,#23145,.T.);
#40294=EDGE_CURVE('',#31578,#31939,#23146,.T.);
#40295=EDGE_CURVE('',#31938,#31863,#25535,.T.);
#40296=EDGE_CURVE('',#31940,#31938,#18906,.T.);
#40297=EDGE_CURVE('',#31941,#31940,#18907,.T.);
#40298=EDGE_CURVE('',#31939,#31941,#18908,.T.);
#40299=EDGE_CURVE('',#31864,#31941,#25536,.T.);
#40300=EDGE_CURVE('',#31579,#28954,#23147,.T.);
#40301=EDGE_CURVE('',#28956,#31864,#25537,.T.);
#40302=EDGE_CURVE('',#31865,#28955,#25538,.T.);
#40303=EDGE_CURVE('',#31942,#31943,#23148,.T.);
#40304=EDGE_CURVE('',#31580,#31943,#23149,.T.);
#40305=EDGE_CURVE('',#31942,#31865,#25539,.T.);
#40306=EDGE_CURVE('',#31944,#31942,#18909,.T.);
#40307=EDGE_CURVE('',#31945,#31944,#18910,.T.);
#40308=EDGE_CURVE('',#31943,#31945,#18911,.T.);
#40309=EDGE_CURVE('',#31866,#31945,#25540,.T.);
#40310=EDGE_CURVE('',#31946,#31947,#23150,.T.);
#40311=EDGE_CURVE('',#31581,#31947,#23151,.T.);
#40312=EDGE_CURVE('',#31946,#31866,#25541,.T.);
#40313=EDGE_CURVE('',#31948,#31946,#18912,.T.);
#40314=EDGE_CURVE('',#31949,#31948,#18913,.T.);
#40315=EDGE_CURVE('',#31947,#31949,#18914,.T.);
#40316=EDGE_CURVE('',#31867,#31949,#25542,.T.);
#40317=EDGE_CURVE('',#31950,#31951,#23152,.T.);
#40318=EDGE_CURVE('',#31582,#31951,#23153,.T.);
#40319=EDGE_CURVE('',#31950,#31867,#25543,.T.);
#40320=EDGE_CURVE('',#31952,#31950,#18915,.T.);
#40321=EDGE_CURVE('',#31953,#31952,#18916,.T.);
#40322=EDGE_CURVE('',#31951,#31953,#18917,.T.);
#40323=EDGE_CURVE('',#31868,#31953,#25544,.T.);
#40324=EDGE_CURVE('',#31954,#31955,#23154,.T.);
#40325=EDGE_CURVE('',#31583,#31955,#23155,.T.);
#40326=EDGE_CURVE('',#31954,#31868,#25545,.T.);
#40327=EDGE_CURVE('',#31956,#31954,#18918,.T.);
#40328=EDGE_CURVE('',#31957,#31956,#18919,.T.);
#40329=EDGE_CURVE('',#31955,#31957,#18920,.T.);
#40330=EDGE_CURVE('',#31869,#31957,#25546,.T.);
#40331=EDGE_CURVE('',#31958,#31959,#23156,.T.);
#40332=EDGE_CURVE('',#31584,#31959,#23157,.T.);
#40333=EDGE_CURVE('',#31958,#31869,#25547,.T.);
#40334=EDGE_CURVE('',#31960,#31958,#18921,.T.);
#40335=EDGE_CURVE('',#31961,#31960,#18922,.T.);
#40336=EDGE_CURVE('',#31959,#31961,#18923,.T.);
#40337=EDGE_CURVE('',#31870,#31961,#25548,.T.);
#40338=EDGE_CURVE('',#31962,#31963,#23158,.T.);
#40339=EDGE_CURVE('',#31585,#31963,#23159,.T.);
#40340=EDGE_CURVE('',#31962,#31870,#25549,.T.);
#40341=EDGE_CURVE('',#31964,#31962,#18924,.T.);
#40342=EDGE_CURVE('',#31965,#31964,#18925,.T.);
#40343=EDGE_CURVE('',#31963,#31965,#18926,.T.);
#40344=EDGE_CURVE('',#31871,#31965,#25550,.T.);
#40345=EDGE_CURVE('',#31966,#31967,#23160,.T.);
#40346=EDGE_CURVE('',#31586,#31967,#23161,.T.);
#40347=EDGE_CURVE('',#31966,#31871,#25551,.T.);
#40348=EDGE_CURVE('',#31968,#31966,#18927,.T.);
#40349=EDGE_CURVE('',#31969,#31968,#18928,.T.);
#40350=EDGE_CURVE('',#31967,#31969,#18929,.T.);
#40351=EDGE_CURVE('',#31872,#31969,#25552,.T.);
#40352=EDGE_CURVE('',#31970,#31971,#23162,.T.);
#40353=EDGE_CURVE('',#31587,#31971,#23163,.T.);
#40354=EDGE_CURVE('',#31970,#31872,#25553,.T.);
#40355=EDGE_CURVE('',#31972,#31970,#18930,.T.);
#40356=EDGE_CURVE('',#31973,#31972,#18931,.T.);
#40357=EDGE_CURVE('',#31971,#31973,#18932,.T.);
#40358=EDGE_CURVE('',#31873,#31973,#25554,.T.);
#40359=EDGE_CURVE('',#31974,#31975,#23164,.T.);
#40360=EDGE_CURVE('',#31588,#31975,#23165,.T.);
#40361=EDGE_CURVE('',#31974,#31873,#25555,.T.);
#40362=EDGE_CURVE('',#31976,#31974,#18933,.T.);
#40363=EDGE_CURVE('',#31977,#31976,#18934,.T.);
#40364=EDGE_CURVE('',#31975,#31977,#18935,.T.);
#40365=EDGE_CURVE('',#31874,#31977,#25556,.T.);
#40366=EDGE_CURVE('',#31978,#31979,#23166,.T.);
#40367=EDGE_CURVE('',#31589,#31979,#23167,.T.);
#40368=EDGE_CURVE('',#31978,#31874,#25557,.T.);
#40369=EDGE_CURVE('',#31980,#31978,#18936,.T.);
#40370=EDGE_CURVE('',#31981,#31980,#18937,.T.);
#40371=EDGE_CURVE('',#31979,#31981,#18938,.T.);
#40372=EDGE_CURVE('',#31875,#31981,#25558,.T.);
#40373=EDGE_CURVE('',#31982,#31983,#23168,.T.);
#40374=EDGE_CURVE('',#31590,#31983,#23169,.T.);
#40375=EDGE_CURVE('',#31982,#31875,#25559,.T.);
#40376=EDGE_CURVE('',#31984,#31982,#18939,.T.);
#40377=EDGE_CURVE('',#31985,#31984,#18940,.T.);
#40378=EDGE_CURVE('',#31983,#31985,#18941,.T.);
#40379=EDGE_CURVE('',#31876,#31985,#25560,.T.);
#40380=EDGE_CURVE('',#31986,#31987,#23170,.T.);
#40381=EDGE_CURVE('',#31591,#31987,#23171,.T.);
#40382=EDGE_CURVE('',#31986,#31876,#25561,.T.);
#40383=EDGE_CURVE('',#31988,#31986,#18942,.T.);
#40384=EDGE_CURVE('',#31989,#31988,#18943,.T.);
#40385=EDGE_CURVE('',#31987,#31989,#18944,.T.);
#40386=EDGE_CURVE('',#31877,#31989,#25562,.T.);
#40387=EDGE_CURVE('',#31990,#31991,#23172,.T.);
#40388=EDGE_CURVE('',#31592,#31991,#23173,.T.);
#40389=EDGE_CURVE('',#31990,#31877,#25563,.T.);
#40390=EDGE_CURVE('',#31991,#31992,#18945,.T.);
#40391=EDGE_CURVE('',#31878,#31992,#25564,.T.);
#40392=EDGE_CURVE('',#31993,#31990,#18946,.T.);
#40393=EDGE_CURVE('',#31992,#31993,#18947,.T.);
#40394=EDGE_CURVE('',#31994,#31878,#25565,.T.);
#40395=EDGE_CURVE('',#31994,#31995,#23174,.T.);
#40396=EDGE_CURVE('',#31593,#31995,#23175,.T.);
#40397=EDGE_CURVE('',#31995,#31996,#18948,.T.);
#40398=EDGE_CURVE('',#31997,#31994,#18949,.T.);
#40399=EDGE_CURVE('',#31996,#31997,#18950,.T.);
#40400=EDGE_CURVE('',#31879,#31996,#25566,.T.);
#40401=EDGE_CURVE('',#31998,#31999,#23176,.T.);
#40402=EDGE_CURVE('',#31594,#31999,#23177,.T.);
#40403=EDGE_CURVE('',#31998,#31879,#25567,.T.);
#40404=EDGE_CURVE('',#32000,#31998,#18951,.T.);
#40405=EDGE_CURVE('',#32001,#32000,#18952,.T.);
#40406=EDGE_CURVE('',#31999,#32001,#18953,.T.);
#40407=EDGE_CURVE('',#31880,#32001,#25568,.T.);
#40408=EDGE_CURVE('',#32002,#32003,#23178,.T.);
#40409=EDGE_CURVE('',#31595,#32003,#23179,.T.);
#40410=EDGE_CURVE('',#32002,#31880,#25569,.T.);
#40411=EDGE_CURVE('',#32004,#32002,#18954,.T.);
#40412=EDGE_CURVE('',#32005,#32004,#18955,.T.);
#40413=EDGE_CURVE('',#32003,#32005,#18956,.T.);
#40414=EDGE_CURVE('',#31881,#32005,#25570,.T.);
#40415=EDGE_CURVE('',#32006,#32007,#23180,.T.);
#40416=EDGE_CURVE('',#31596,#32007,#23181,.T.);
#40417=EDGE_CURVE('',#32006,#31881,#25571,.T.);
#40418=EDGE_CURVE('',#32008,#32006,#18957,.T.);
#40419=EDGE_CURVE('',#32009,#32008,#18958,.T.);
#40420=EDGE_CURVE('',#32007,#32009,#18959,.T.);
#40421=EDGE_CURVE('',#31882,#32009,#25572,.T.);
#40422=EDGE_CURVE('',#32010,#32011,#23182,.T.);
#40423=EDGE_CURVE('',#31597,#32011,#23183,.T.);
#40424=EDGE_CURVE('',#32010,#31882,#25573,.T.);
#40425=EDGE_CURVE('',#32012,#32010,#18960,.T.);
#40426=EDGE_CURVE('',#32013,#32012,#18961,.T.);
#40427=EDGE_CURVE('',#32011,#32013,#18962,.T.);
#40428=EDGE_CURVE('',#31883,#32013,#25574,.T.);
#40429=EDGE_CURVE('',#32014,#32015,#23184,.T.);
#40430=EDGE_CURVE('',#31598,#32015,#23185,.T.);
#40431=EDGE_CURVE('',#32014,#31883,#25575,.T.);
#40432=EDGE_CURVE('',#32016,#32014,#18963,.T.);
#40433=EDGE_CURVE('',#32017,#32016,#18964,.T.);
#40434=EDGE_CURVE('',#32015,#32017,#18965,.T.);
#40435=EDGE_CURVE('',#31884,#32017,#25576,.T.);
#40436=EDGE_CURVE('',#32018,#32019,#23186,.T.);
#40437=EDGE_CURVE('',#31599,#32019,#23187,.T.);
#40438=EDGE_CURVE('',#32018,#31884,#25577,.T.);
#40439=EDGE_CURVE('',#32020,#32018,#18966,.T.);
#40440=EDGE_CURVE('',#32021,#32020,#18967,.T.);
#40441=EDGE_CURVE('',#32019,#32021,#18968,.T.);
#40442=EDGE_CURVE('',#31885,#32021,#25578,.T.);
#40443=EDGE_CURVE('',#32022,#32023,#23188,.T.);
#40444=EDGE_CURVE('',#31600,#32023,#23189,.T.);
#40445=EDGE_CURVE('',#32022,#31885,#25579,.T.);
#40446=EDGE_CURVE('',#32024,#32022,#18969,.T.);
#40447=EDGE_CURVE('',#32025,#32024,#18970,.T.);
#40448=EDGE_CURVE('',#32023,#32025,#18971,.T.);
#40449=EDGE_CURVE('',#31886,#32025,#25580,.T.);
#40450=EDGE_CURVE('',#32026,#32027,#18972,.T.);
#40451=EDGE_CURVE('',#31917,#32026,#18973,.T.);
#40452=EDGE_CURVE('',#32027,#31916,#23190,.T.);
#40453=EDGE_CURVE('',#32027,#31886,#25581,.T.);
#40454=EDGE_CURVE('',#32028,#31601,#23191,.T.);
#40455=EDGE_CURVE('',#32028,#32029,#18974,.T.);
#40456=EDGE_CURVE('',#31887,#32029,#25582,.T.);
#40457=EDGE_CURVE('',#32030,#31887,#25583,.T.);
#40458=EDGE_CURVE('',#32030,#32031,#23192,.T.);
#40459=EDGE_CURVE('',#31602,#32031,#23193,.T.);
#40460=EDGE_CURVE('',#32031,#32032,#18975,.T.);
#40461=EDGE_CURVE('',#31888,#32032,#25584,.T.);
#40462=EDGE_CURVE('',#32033,#32030,#18976,.T.);
#40463=EDGE_CURVE('',#32032,#32033,#18977,.T.);
#40464=EDGE_CURVE('',#32034,#31888,#25585,.T.);
#40465=EDGE_CURVE('',#32034,#32035,#23194,.T.);
#40466=EDGE_CURVE('',#31603,#32035,#23195,.T.);
#40467=EDGE_CURVE('',#32035,#32036,#18978,.T.);
#40468=EDGE_CURVE('',#31889,#32036,#25586,.T.);
#40469=EDGE_CURVE('',#32037,#32034,#18979,.T.);
#40470=EDGE_CURVE('',#32036,#32037,#18980,.T.);
#40471=EDGE_CURVE('',#32038,#31889,#25587,.T.);
#40472=EDGE_CURVE('',#32038,#32039,#23196,.T.);
#40473=EDGE_CURVE('',#31604,#32039,#23197,.T.);
#40474=EDGE_CURVE('',#32039,#32040,#18981,.T.);
#40475=EDGE_CURVE('',#31890,#32040,#25588,.T.);
#40476=EDGE_CURVE('',#32041,#32038,#18982,.T.);
#40477=EDGE_CURVE('',#32040,#32041,#18983,.T.);
#40478=EDGE_CURVE('',#32042,#31890,#25589,.T.);
#40479=EDGE_CURVE('',#32042,#32043,#23198,.T.);
#40480=EDGE_CURVE('',#31605,#32043,#23199,.T.);
#40481=EDGE_CURVE('',#32043,#32044,#18984,.T.);
#40482=EDGE_CURVE('',#31891,#32044,#25590,.T.);
#40483=EDGE_CURVE('',#32045,#32042,#18985,.T.);
#40484=EDGE_CURVE('',#32044,#32045,#18986,.T.);
#40485=EDGE_CURVE('',#32046,#31891,#25591,.T.);
#40486=EDGE_CURVE('',#32046,#32047,#23200,.T.);
#40487=EDGE_CURVE('',#31606,#32047,#23201,.T.);
#40488=EDGE_CURVE('',#32047,#32048,#18987,.T.);
#40489=EDGE_CURVE('',#31892,#32048,#25592,.T.);
#40490=EDGE_CURVE('',#32049,#32046,#18988,.T.);
#40491=EDGE_CURVE('',#32048,#32049,#18989,.T.);
#40492=EDGE_CURVE('',#32050,#31892,#25593,.T.);
#40493=EDGE_CURVE('',#32050,#32051,#23202,.T.);
#40494=EDGE_CURVE('',#31607,#32051,#23203,.T.);
#40495=EDGE_CURVE('',#32051,#32052,#18990,.T.);
#40496=EDGE_CURVE('',#31893,#32052,#25594,.T.);
#40497=EDGE_CURVE('',#32053,#32050,#18991,.T.);
#40498=EDGE_CURVE('',#32052,#32053,#18992,.T.);
#40499=EDGE_CURVE('',#32054,#31893,#25595,.T.);
#40500=EDGE_CURVE('',#32054,#32055,#23204,.T.);
#40501=EDGE_CURVE('',#31608,#32055,#23205,.T.);
#40502=EDGE_CURVE('',#32055,#32056,#18993,.T.);
#40503=EDGE_CURVE('',#31894,#32056,#25596,.T.);
#40504=EDGE_CURVE('',#32057,#32054,#18994,.T.);
#40505=EDGE_CURVE('',#32056,#32057,#18995,.T.);
#40506=EDGE_CURVE('',#32058,#31894,#25597,.T.);
#40507=EDGE_CURVE('',#32058,#32059,#23206,.T.);
#40508=EDGE_CURVE('',#31609,#32059,#23207,.T.);
#40509=EDGE_CURVE('',#32059,#32060,#18996,.T.);
#40510=EDGE_CURVE('',#31895,#32060,#25598,.T.);
#40511=EDGE_CURVE('',#32061,#32058,#18997,.T.);
#40512=EDGE_CURVE('',#32060,#32061,#18998,.T.);
#40513=EDGE_CURVE('',#32062,#31895,#25599,.T.);
#40514=EDGE_CURVE('',#32062,#32063,#23208,.T.);
#40515=EDGE_CURVE('',#31610,#32063,#23209,.T.);
#40516=EDGE_CURVE('',#32063,#32064,#18999,.T.);
#40517=EDGE_CURVE('',#31896,#32064,#25600,.T.);
#40518=EDGE_CURVE('',#32065,#32062,#19000,.T.);
#40519=EDGE_CURVE('',#32064,#32065,#19001,.T.);
#40520=EDGE_CURVE('',#32066,#31896,#25601,.T.);
#40521=EDGE_CURVE('',#32066,#32067,#23210,.T.);
#40522=EDGE_CURVE('',#31611,#32067,#23211,.T.);
#40523=EDGE_CURVE('',#32067,#32068,#19002,.T.);
#40524=EDGE_CURVE('',#31897,#32068,#25602,.T.);
#40525=EDGE_CURVE('',#32069,#32066,#19003,.T.);
#40526=EDGE_CURVE('',#32068,#32069,#19004,.T.);
#40527=EDGE_CURVE('',#32070,#31897,#25603,.T.);
#40528=EDGE_CURVE('',#32070,#32071,#23212,.T.);
#40529=EDGE_CURVE('',#31612,#32071,#23213,.T.);
#40530=EDGE_CURVE('',#32071,#32072,#19005,.T.);
#40531=EDGE_CURVE('',#31898,#32072,#25604,.T.);
#40532=EDGE_CURVE('',#32073,#32070,#19006,.T.);
#40533=EDGE_CURVE('',#32072,#32073,#19007,.T.);
#40534=EDGE_CURVE('',#32074,#31898,#25605,.T.);
#40535=EDGE_CURVE('',#32074,#32075,#23214,.T.);
#40536=EDGE_CURVE('',#31613,#32075,#23215,.T.);
#40537=EDGE_CURVE('',#32075,#32076,#19008,.T.);
#40538=EDGE_CURVE('',#31899,#32076,#25606,.T.);
#40539=EDGE_CURVE('',#32077,#32074,#19009,.T.);
#40540=EDGE_CURVE('',#32076,#32077,#19010,.T.);
#40541=EDGE_CURVE('',#32078,#31899,#25607,.T.);
#40542=EDGE_CURVE('',#32078,#32079,#23216,.T.);
#40543=EDGE_CURVE('',#31614,#32079,#23217,.T.);
#40544=EDGE_CURVE('',#32079,#32080,#19011,.T.);
#40545=EDGE_CURVE('',#31900,#32080,#25608,.T.);
#40546=EDGE_CURVE('',#32081,#32078,#19012,.T.);
#40547=EDGE_CURVE('',#32080,#32081,#19013,.T.);
#40548=EDGE_CURVE('',#28953,#31900,#25609,.T.);
#40549=EDGE_CURVE('',#31615,#28952,#23218,.T.);
#40550=EDGE_CURVE('',#31901,#28950,#25610,.T.);
#40551=EDGE_CURVE('',#32082,#31901,#25611,.T.);
#40552=EDGE_CURVE('',#32082,#32083,#23219,.T.);
#40553=EDGE_CURVE('',#31616,#32083,#23220,.T.);
#40554=EDGE_CURVE('',#32083,#32084,#19014,.T.);
#40555=EDGE_CURVE('',#31902,#32084,#25612,.T.);
#40556=EDGE_CURVE('',#32085,#32082,#19015,.T.);
#40557=EDGE_CURVE('',#32084,#32085,#19016,.T.);
#40558=EDGE_CURVE('',#32086,#31902,#25613,.T.);
#40559=EDGE_CURVE('',#32086,#32087,#23221,.T.);
#40560=EDGE_CURVE('',#31617,#32087,#23222,.T.);
#40561=EDGE_CURVE('',#32087,#32088,#19017,.T.);
#40562=EDGE_CURVE('',#31903,#32088,#25614,.T.);
#40563=EDGE_CURVE('',#32089,#32086,#19018,.T.);
#40564=EDGE_CURVE('',#32088,#32089,#19019,.T.);
#40565=EDGE_CURVE('',#32090,#31903,#25615,.T.);
#40566=EDGE_CURVE('',#32090,#32091,#23223,.T.);
#40567=EDGE_CURVE('',#31618,#32091,#23224,.T.);
#40568=EDGE_CURVE('',#32091,#32092,#19020,.T.);
#40569=EDGE_CURVE('',#31904,#32092,#25616,.T.);
#40570=EDGE_CURVE('',#32093,#32090,#19021,.T.);
#40571=EDGE_CURVE('',#32092,#32093,#19022,.T.);
#40572=EDGE_CURVE('',#32094,#31904,#25617,.T.);
#40573=EDGE_CURVE('',#32094,#32095,#23225,.T.);
#40574=EDGE_CURVE('',#31619,#32095,#23226,.T.);
#40575=EDGE_CURVE('',#32095,#32096,#19023,.T.);
#40576=EDGE_CURVE('',#31905,#32096,#25618,.T.);
#40577=EDGE_CURVE('',#32097,#32094,#19024,.T.);
#40578=EDGE_CURVE('',#32096,#32097,#19025,.T.);
#40579=EDGE_CURVE('',#32098,#31905,#25619,.T.);
#40580=EDGE_CURVE('',#32098,#32099,#23227,.T.);
#40581=EDGE_CURVE('',#31620,#32099,#23228,.T.);
#40582=EDGE_CURVE('',#32099,#32100,#19026,.T.);
#40583=EDGE_CURVE('',#31906,#32100,#25620,.T.);
#40584=EDGE_CURVE('',#32101,#32098,#19027,.T.);
#40585=EDGE_CURVE('',#32100,#32101,#19028,.T.);
#40586=EDGE_CURVE('',#32102,#31906,#25621,.T.);
#40587=EDGE_CURVE('',#32102,#32103,#23229,.T.);
#40588=EDGE_CURVE('',#31621,#32103,#23230,.T.);
#40589=EDGE_CURVE('',#32103,#32104,#19029,.T.);
#40590=EDGE_CURVE('',#31907,#32104,#25622,.T.);
#40591=EDGE_CURVE('',#32105,#32102,#19030,.T.);
#40592=EDGE_CURVE('',#32104,#32105,#19031,.T.);
#40593=EDGE_CURVE('',#32106,#31907,#25623,.T.);
#40594=EDGE_CURVE('',#32106,#32107,#23231,.T.);
#40595=EDGE_CURVE('',#31622,#32107,#23232,.T.);
#40596=EDGE_CURVE('',#32107,#32108,#19032,.T.);
#40597=EDGE_CURVE('',#31908,#32108,#25624,.T.);
#40598=EDGE_CURVE('',#32109,#32106,#19033,.T.);
#40599=EDGE_CURVE('',#32108,#32109,#19034,.T.);
#40600=EDGE_CURVE('',#32110,#31908,#25625,.T.);
#40601=EDGE_CURVE('',#32110,#32111,#23233,.T.);
#40602=EDGE_CURVE('',#31623,#32111,#23234,.T.);
#40603=EDGE_CURVE('',#32111,#32112,#19035,.T.);
#40604=EDGE_CURVE('',#31909,#32112,#25626,.T.);
#40605=EDGE_CURVE('',#32113,#32110,#19036,.T.);
#40606=EDGE_CURVE('',#32112,#32113,#19037,.T.);
#40607=EDGE_CURVE('',#32114,#31909,#25627,.T.);
#40608=EDGE_CURVE('',#32114,#32115,#23235,.T.);
#40609=EDGE_CURVE('',#31624,#32115,#23236,.T.);
#40610=EDGE_CURVE('',#32115,#32116,#19038,.T.);
#40611=EDGE_CURVE('',#31910,#32116,#25628,.T.);
#40612=EDGE_CURVE('',#32117,#32114,#19039,.T.);
#40613=EDGE_CURVE('',#32116,#32117,#19040,.T.);
#40614=EDGE_CURVE('',#32118,#31910,#25629,.T.);
#40615=EDGE_CURVE('',#32118,#32119,#23237,.T.);
#40616=EDGE_CURVE('',#31625,#32119,#23238,.T.);
#40617=EDGE_CURVE('',#32119,#32120,#19041,.T.);
#40618=EDGE_CURVE('',#31911,#32120,#25630,.T.);
#40619=EDGE_CURVE('',#32121,#32118,#19042,.T.);
#40620=EDGE_CURVE('',#32120,#32121,#19043,.T.);
#40621=EDGE_CURVE('',#32122,#31911,#25631,.T.);
#40622=EDGE_CURVE('',#32122,#32123,#23239,.T.);
#40623=EDGE_CURVE('',#31626,#32123,#23240,.T.);
#40624=EDGE_CURVE('',#32123,#32124,#19044,.T.);
#40625=EDGE_CURVE('',#31912,#32124,#25632,.T.);
#40626=EDGE_CURVE('',#32125,#32122,#19045,.T.);
#40627=EDGE_CURVE('',#32124,#32125,#19046,.T.);
#40628=EDGE_CURVE('',#32126,#31912,#25633,.T.);
#40629=EDGE_CURVE('',#32126,#32127,#23241,.T.);
#40630=EDGE_CURVE('',#31627,#32127,#23242,.T.);
#40631=EDGE_CURVE('',#32127,#32128,#19047,.T.);
#40632=EDGE_CURVE('',#31913,#32128,#25634,.T.);
#40633=EDGE_CURVE('',#32129,#32126,#19048,.T.);
#40634=EDGE_CURVE('',#32128,#32129,#19049,.T.);
#40635=EDGE_CURVE('',#32130,#31913,#25635,.T.);
#40636=EDGE_CURVE('',#32130,#32131,#23243,.T.);
#40637=EDGE_CURVE('',#31628,#32131,#23244,.T.);
#40638=EDGE_CURVE('',#32131,#32132,#19050,.T.);
#40639=EDGE_CURVE('',#31914,#32132,#25636,.T.);
#40640=EDGE_CURVE('',#32133,#32130,#19051,.T.);
#40641=EDGE_CURVE('',#32132,#32133,#19052,.T.);
#40642=EDGE_CURVE('',#32134,#31914,#25637,.T.);
#40643=EDGE_CURVE('',#32134,#32135,#23245,.T.);
#40644=EDGE_CURVE('',#31629,#32135,#23246,.T.);
#40645=EDGE_CURVE('',#32135,#32136,#19053,.T.);
#40646=EDGE_CURVE('',#31915,#32136,#25638,.T.);
#40647=EDGE_CURVE('',#32137,#32134,#19054,.T.);
#40648=EDGE_CURVE('',#32136,#32137,#19055,.T.);
#40649=EDGE_CURVE('',#32138,#32028,#23247,.T.);
#40650=EDGE_CURVE('',#32139,#32138,#19056,.T.);
#40651=EDGE_CURVE('',#32029,#32139,#19057,.T.);
#40652=EDGE_CURVE('',#32138,#31915,#25639,.T.);
#40653=EDGE_CURVE('',#31858,#32140,#19058,.T.);
#40654=EDGE_CURVE('',#32140,#32026,#23248,.T.);
#40655=EDGE_CURVE('',#32141,#31858,#19059,.T.);
#40656=EDGE_CURVE('',#31920,#32141,#23249,.T.);
#40657=EDGE_CURVE('',#31859,#32141,#19060,.T.);
#40658=EDGE_CURVE('',#32142,#31859,#19061,.T.);
#40659=EDGE_CURVE('',#31924,#32142,#23250,.T.);
#40660=EDGE_CURVE('',#31860,#32142,#19062,.T.);
#40661=EDGE_CURVE('',#32143,#31860,#19063,.T.);
#40662=EDGE_CURVE('',#31928,#32143,#23251,.T.);
#40663=EDGE_CURVE('',#31861,#32143,#19064,.T.);
#40664=EDGE_CURVE('',#32144,#31861,#19065,.T.);
#40665=EDGE_CURVE('',#31932,#32144,#23252,.T.);
#40666=EDGE_CURVE('',#31862,#32144,#19066,.T.);
#40667=EDGE_CURVE('',#32145,#31862,#19067,.T.);
#40668=EDGE_CURVE('',#31936,#32145,#23253,.T.);
#40669=EDGE_CURVE('',#31863,#32145,#19068,.T.);
#40670=EDGE_CURVE('',#32146,#31863,#19069,.T.);
#40671=EDGE_CURVE('',#31940,#32146,#23254,.T.);
#40672=EDGE_CURVE('',#31864,#32146,#19070,.T.);
#40673=EDGE_CURVE('',#32147,#31864,#19071,.T.);
#40674=EDGE_CURVE('',#28957,#32147,#23255,.T.);
#40675=EDGE_CURVE('',#31865,#32147,#19072,.T.);
#40676=EDGE_CURVE('',#32148,#31865,#19073,.T.);
#40677=EDGE_CURVE('',#31944,#32148,#23256,.T.);
#40678=EDGE_CURVE('',#31866,#32148,#19074,.T.);
#40679=EDGE_CURVE('',#32149,#31866,#19075,.T.);
#40680=EDGE_CURVE('',#31948,#32149,#23257,.T.);
#40681=EDGE_CURVE('',#31867,#32149,#19076,.T.);
#40682=EDGE_CURVE('',#32150,#31867,#19077,.T.);
#40683=EDGE_CURVE('',#31952,#32150,#23258,.T.);
#40684=EDGE_CURVE('',#31868,#32150,#19078,.T.);
#40685=EDGE_CURVE('',#32151,#31868,#19079,.T.);
#40686=EDGE_CURVE('',#31956,#32151,#23259,.T.);
#40687=EDGE_CURVE('',#31869,#32151,#19080,.T.);
#40688=EDGE_CURVE('',#32152,#31869,#19081,.T.);
#40689=EDGE_CURVE('',#31960,#32152,#23260,.T.);
#40690=EDGE_CURVE('',#31870,#32152,#19082,.T.);
#40691=EDGE_CURVE('',#32153,#31870,#19083,.T.);
#40692=EDGE_CURVE('',#31964,#32153,#23261,.T.);
#40693=EDGE_CURVE('',#31871,#32153,#19084,.T.);
#40694=EDGE_CURVE('',#32154,#31871,#19085,.T.);
#40695=EDGE_CURVE('',#31968,#32154,#23262,.T.);
#40696=EDGE_CURVE('',#31872,#32154,#19086,.T.);
#40697=EDGE_CURVE('',#32155,#31872,#19087,.T.);
#40698=EDGE_CURVE('',#31972,#32155,#23263,.T.);
#40699=EDGE_CURVE('',#31873,#32155,#19088,.T.);
#40700=EDGE_CURVE('',#32156,#31873,#19089,.T.);
#40701=EDGE_CURVE('',#31976,#32156,#23264,.T.);
#40702=EDGE_CURVE('',#31874,#32156,#19090,.T.);
#40703=EDGE_CURVE('',#32157,#31874,#19091,.T.);
#40704=EDGE_CURVE('',#31980,#32157,#23265,.T.);
#40705=EDGE_CURVE('',#31875,#32157,#19092,.T.);
#40706=EDGE_CURVE('',#32158,#31875,#19093,.T.);
#40707=EDGE_CURVE('',#31984,#32158,#23266,.T.);
#40708=EDGE_CURVE('',#31876,#32158,#19094,.T.);
#40709=EDGE_CURVE('',#32159,#31876,#19095,.T.);
#40710=EDGE_CURVE('',#31988,#32159,#23267,.T.);
#40711=EDGE_CURVE('',#31877,#32159,#19096,.T.);
#40712=EDGE_CURVE('',#32160,#31877,#19097,.T.);
#40713=EDGE_CURVE('',#31993,#32160,#23268,.T.);
#40714=EDGE_CURVE('',#31878,#32160,#19098,.T.);
#40715=EDGE_CURVE('',#32161,#31878,#19099,.T.);
#40716=EDGE_CURVE('',#31997,#32161,#23269,.T.);
#40717=EDGE_CURVE('',#31879,#32161,#19100,.T.);
#40718=EDGE_CURVE('',#32162,#31879,#19101,.T.);
#40719=EDGE_CURVE('',#32000,#32162,#23270,.T.);
#40720=EDGE_CURVE('',#31880,#32162,#19102,.T.);
#40721=EDGE_CURVE('',#32163,#31880,#19103,.T.);
#40722=EDGE_CURVE('',#32004,#32163,#23271,.T.);
#40723=EDGE_CURVE('',#31881,#32163,#19104,.T.);
#40724=EDGE_CURVE('',#32164,#31881,#19105,.T.);
#40725=EDGE_CURVE('',#32008,#32164,#23272,.T.);
#40726=EDGE_CURVE('',#31882,#32164,#19106,.T.);
#40727=EDGE_CURVE('',#32165,#31882,#19107,.T.);
#40728=EDGE_CURVE('',#32012,#32165,#23273,.T.);
#40729=EDGE_CURVE('',#31883,#32165,#19108,.T.);
#40730=EDGE_CURVE('',#32166,#31883,#19109,.T.);
#40731=EDGE_CURVE('',#32016,#32166,#23274,.T.);
#40732=EDGE_CURVE('',#31884,#32166,#19110,.T.);
#40733=EDGE_CURVE('',#32167,#31884,#19111,.T.);
#40734=EDGE_CURVE('',#32020,#32167,#23275,.T.);
#40735=EDGE_CURVE('',#31885,#32167,#19112,.T.);
#40736=EDGE_CURVE('',#32168,#31885,#19113,.T.);
#40737=EDGE_CURVE('',#32024,#32168,#23276,.T.);
#40738=EDGE_CURVE('',#31886,#32168,#19114,.T.);
#40739=EDGE_CURVE('',#32140,#31886,#19115,.T.);
#40740=EDGE_CURVE('',#32169,#32139,#23277,.T.);
#40741=EDGE_CURVE('',#31887,#32169,#19116,.T.);
#40742=EDGE_CURVE('',#32170,#31887,#19117,.T.);
#40743=EDGE_CURVE('',#32033,#32170,#23278,.T.);
#40744=EDGE_CURVE('',#31888,#32170,#19118,.T.);
#40745=EDGE_CURVE('',#32171,#31888,#19119,.T.);
#40746=EDGE_CURVE('',#32037,#32171,#23279,.T.);
#40747=EDGE_CURVE('',#31889,#32171,#19120,.T.);
#40748=EDGE_CURVE('',#32172,#31889,#19121,.T.);
#40749=EDGE_CURVE('',#32041,#32172,#23280,.T.);
#40750=EDGE_CURVE('',#31890,#32172,#19122,.T.);
#40751=EDGE_CURVE('',#32173,#31890,#19123,.T.);
#40752=EDGE_CURVE('',#32045,#32173,#23281,.T.);
#40753=EDGE_CURVE('',#31891,#32173,#19124,.T.);
#40754=EDGE_CURVE('',#32174,#31891,#19125,.T.);
#40755=EDGE_CURVE('',#32049,#32174,#23282,.T.);
#40756=EDGE_CURVE('',#31892,#32174,#19126,.T.);
#40757=EDGE_CURVE('',#32175,#31892,#19127,.T.);
#40758=EDGE_CURVE('',#32053,#32175,#23283,.T.);
#40759=EDGE_CURVE('',#31893,#32175,#19128,.T.);
#40760=EDGE_CURVE('',#32176,#31893,#19129,.T.);
#40761=EDGE_CURVE('',#32057,#32176,#23284,.T.);
#40762=EDGE_CURVE('',#31894,#32176,#19130,.T.);
#40763=EDGE_CURVE('',#32177,#31894,#19131,.T.);
#40764=EDGE_CURVE('',#32061,#32177,#23285,.T.);
#40765=EDGE_CURVE('',#31895,#32177,#19132,.T.);
#40766=EDGE_CURVE('',#32178,#31895,#19133,.T.);
#40767=EDGE_CURVE('',#32065,#32178,#23286,.T.);
#40768=EDGE_CURVE('',#31896,#32178,#19134,.T.);
#40769=EDGE_CURVE('',#32179,#31896,#19135,.T.);
#40770=EDGE_CURVE('',#32069,#32179,#23287,.T.);
#40771=EDGE_CURVE('',#31897,#32179,#19136,.T.);
#40772=EDGE_CURVE('',#32180,#31897,#19137,.T.);
#40773=EDGE_CURVE('',#32073,#32180,#23288,.T.);
#40774=EDGE_CURVE('',#31898,#32180,#19138,.T.);
#40775=EDGE_CURVE('',#32181,#31898,#19139,.T.);
#40776=EDGE_CURVE('',#32077,#32181,#23289,.T.);
#40777=EDGE_CURVE('',#31899,#32181,#19140,.T.);
#40778=EDGE_CURVE('',#32182,#31899,#19141,.T.);
#40779=EDGE_CURVE('',#32081,#32182,#23290,.T.);
#40780=EDGE_CURVE('',#31900,#32182,#19142,.T.);
#40781=EDGE_CURVE('',#32183,#31900,#19143,.T.);
#40782=EDGE_CURVE('',#28951,#32183,#23291,.T.);
#40783=EDGE_CURVE('',#31901,#32183,#19144,.T.);
#40784=EDGE_CURVE('',#32184,#31901,#19145,.T.);
#40785=EDGE_CURVE('',#32085,#32184,#23292,.T.);
#40786=EDGE_CURVE('',#31902,#32184,#19146,.T.);
#40787=EDGE_CURVE('',#32185,#31902,#19147,.T.);
#40788=EDGE_CURVE('',#32089,#32185,#23293,.T.);
#40789=EDGE_CURVE('',#31903,#32185,#19148,.T.);
#40790=EDGE_CURVE('',#32186,#31903,#19149,.T.);
#40791=EDGE_CURVE('',#32093,#32186,#23294,.T.);
#40792=EDGE_CURVE('',#31904,#32186,#19150,.T.);
#40793=EDGE_CURVE('',#32187,#31904,#19151,.T.);
#40794=EDGE_CURVE('',#32097,#32187,#23295,.T.);
#40795=EDGE_CURVE('',#31905,#32187,#19152,.T.);
#40796=EDGE_CURVE('',#32188,#31905,#19153,.T.);
#40797=EDGE_CURVE('',#32101,#32188,#23296,.T.);
#40798=EDGE_CURVE('',#31906,#32188,#19154,.T.);
#40799=EDGE_CURVE('',#32189,#31906,#19155,.T.);
#40800=EDGE_CURVE('',#32105,#32189,#23297,.T.);
#40801=EDGE_CURVE('',#31907,#32189,#19156,.T.);
#40802=EDGE_CURVE('',#32190,#31907,#19157,.T.);
#40803=EDGE_CURVE('',#32109,#32190,#23298,.T.);
#40804=EDGE_CURVE('',#31908,#32190,#19158,.T.);
#40805=EDGE_CURVE('',#32191,#31908,#19159,.T.);
#40806=EDGE_CURVE('',#32113,#32191,#23299,.T.);
#40807=EDGE_CURVE('',#31909,#32191,#19160,.T.);
#40808=EDGE_CURVE('',#32192,#31909,#19161,.T.);
#40809=EDGE_CURVE('',#32117,#32192,#23300,.T.);
#40810=EDGE_CURVE('',#31910,#32192,#19162,.T.);
#40811=EDGE_CURVE('',#32193,#31910,#19163,.T.);
#40812=EDGE_CURVE('',#32121,#32193,#23301,.T.);
#40813=EDGE_CURVE('',#31911,#32193,#19164,.T.);
#40814=EDGE_CURVE('',#32194,#31911,#19165,.T.);
#40815=EDGE_CURVE('',#32125,#32194,#23302,.T.);
#40816=EDGE_CURVE('',#31912,#32194,#19166,.T.);
#40817=EDGE_CURVE('',#32195,#31912,#19167,.T.);
#40818=EDGE_CURVE('',#32129,#32195,#23303,.T.);
#40819=EDGE_CURVE('',#31913,#32195,#19168,.T.);
#40820=EDGE_CURVE('',#32196,#31913,#19169,.T.);
#40821=EDGE_CURVE('',#32133,#32196,#23304,.T.);
#40822=EDGE_CURVE('',#31914,#32196,#19170,.T.);
#40823=EDGE_CURVE('',#32197,#31914,#19171,.T.);
#40824=EDGE_CURVE('',#32137,#32197,#23305,.T.);
#40825=EDGE_CURVE('',#31915,#32197,#19172,.T.);
#40826=EDGE_CURVE('',#32169,#31915,#19173,.T.);
#40827=EDGE_CURVE('',#32198,#32199,#19174,.T.);
#40828=EDGE_CURVE('',#31858,#32199,#23306,.T.);
#40829=EDGE_CURVE('',#32198,#32140,#25640,.T.);
#40830=EDGE_CURVE('',#32200,#32198,#19175,.T.);
#40831=EDGE_CURVE('',#32201,#32200,#19176,.T.);
#40832=EDGE_CURVE('',#32199,#32201,#19177,.T.);
#40833=EDGE_CURVE('',#32141,#32201,#25641,.T.);
#40834=EDGE_CURVE('',#32202,#32203,#19178,.T.);
#40835=EDGE_CURVE('',#31859,#32203,#23307,.T.);
#40836=EDGE_CURVE('',#32202,#32141,#25642,.T.);
#40837=EDGE_CURVE('',#32204,#32202,#19179,.T.);
#40838=EDGE_CURVE('',#32205,#32204,#19180,.T.);
#40839=EDGE_CURVE('',#32203,#32205,#19181,.T.);
#40840=EDGE_CURVE('',#32142,#32205,#25643,.T.);
#40841=EDGE_CURVE('',#32206,#32207,#19182,.T.);
#40842=EDGE_CURVE('',#31860,#32207,#23308,.T.);
#40843=EDGE_CURVE('',#32206,#32142,#25644,.T.);
#40844=EDGE_CURVE('',#32208,#32206,#19183,.T.);
#40845=EDGE_CURVE('',#32209,#32208,#19184,.T.);
#40846=EDGE_CURVE('',#32207,#32209,#19185,.T.);
#40847=EDGE_CURVE('',#32143,#32209,#25645,.T.);
#40848=EDGE_CURVE('',#32210,#32211,#19186,.T.);
#40849=EDGE_CURVE('',#31861,#32211,#23309,.T.);
#40850=EDGE_CURVE('',#32210,#32143,#25646,.T.);
#40851=EDGE_CURVE('',#32212,#32210,#19187,.T.);
#40852=EDGE_CURVE('',#32213,#32212,#19188,.T.);
#40853=EDGE_CURVE('',#32211,#32213,#19189,.T.);
#40854=EDGE_CURVE('',#32144,#32213,#25647,.T.);
#40855=EDGE_CURVE('',#32214,#32215,#19190,.T.);
#40856=EDGE_CURVE('',#31862,#32215,#23310,.T.);
#40857=EDGE_CURVE('',#32214,#32144,#25648,.T.);
#40858=EDGE_CURVE('',#32216,#32214,#19191,.T.);
#40859=EDGE_CURVE('',#32217,#32216,#19192,.T.);
#40860=EDGE_CURVE('',#32215,#32217,#19193,.T.);
#40861=EDGE_CURVE('',#32145,#32217,#25649,.T.);
#40862=EDGE_CURVE('',#32218,#32219,#19194,.T.);
#40863=EDGE_CURVE('',#31863,#32219,#23311,.T.);
#40864=EDGE_CURVE('',#32218,#32145,#25650,.T.);
#40865=EDGE_CURVE('',#32220,#32218,#19195,.T.);
#40866=EDGE_CURVE('',#32221,#32220,#19196,.T.);
#40867=EDGE_CURVE('',#32219,#32221,#19197,.T.);
#40868=EDGE_CURVE('',#32146,#32221,#25651,.T.);
#40869=EDGE_CURVE('',#32222,#32223,#19198,.T.);
#40870=EDGE_CURVE('',#31864,#32223,#23312,.T.);
#40871=EDGE_CURVE('',#32222,#32146,#25652,.T.);
#40872=EDGE_CURVE('',#32224,#32222,#19199,.T.);
#40873=EDGE_CURVE('',#32225,#32224,#19200,.T.);
#40874=EDGE_CURVE('',#32223,#32225,#19201,.T.);
#40875=EDGE_CURVE('',#32147,#32225,#25653,.T.);
#40876=EDGE_CURVE('',#32226,#32227,#19202,.T.);
#40877=EDGE_CURVE('',#31865,#32227,#23313,.T.);
#40878=EDGE_CURVE('',#32226,#32147,#25654,.T.);
#40879=EDGE_CURVE('',#32228,#32226,#19203,.T.);
#40880=EDGE_CURVE('',#32229,#32228,#19204,.T.);
#40881=EDGE_CURVE('',#32227,#32229,#19205,.T.);
#40882=EDGE_CURVE('',#32148,#32229,#25655,.T.);
#40883=EDGE_CURVE('',#32230,#32231,#19206,.T.);
#40884=EDGE_CURVE('',#31866,#32231,#23314,.T.);
#40885=EDGE_CURVE('',#32230,#32148,#25656,.T.);
#40886=EDGE_CURVE('',#32232,#32230,#19207,.T.);
#40887=EDGE_CURVE('',#32233,#32232,#19208,.T.);
#40888=EDGE_CURVE('',#32231,#32233,#19209,.T.);
#40889=EDGE_CURVE('',#32149,#32233,#25657,.T.);
#40890=EDGE_CURVE('',#32234,#32235,#19210,.T.);
#40891=EDGE_CURVE('',#31867,#32235,#23315,.T.);
#40892=EDGE_CURVE('',#32234,#32149,#25658,.T.);
#40893=EDGE_CURVE('',#32236,#32234,#19211,.T.);
#40894=EDGE_CURVE('',#32237,#32236,#19212,.T.);
#40895=EDGE_CURVE('',#32235,#32237,#19213,.T.);
#40896=EDGE_CURVE('',#32150,#32237,#25659,.T.);
#40897=EDGE_CURVE('',#32238,#32239,#19214,.T.);
#40898=EDGE_CURVE('',#31868,#32239,#23316,.T.);
#40899=EDGE_CURVE('',#32238,#32150,#25660,.T.);
#40900=EDGE_CURVE('',#32240,#32238,#19215,.T.);
#40901=EDGE_CURVE('',#32241,#32240,#19216,.T.);
#40902=EDGE_CURVE('',#32239,#32241,#19217,.T.);
#40903=EDGE_CURVE('',#32151,#32241,#25661,.T.);
#40904=EDGE_CURVE('',#32242,#32243,#19218,.T.);
#40905=EDGE_CURVE('',#31869,#32243,#23317,.T.);
#40906=EDGE_CURVE('',#32242,#32151,#25662,.T.);
#40907=EDGE_CURVE('',#32244,#32242,#19219,.T.);
#40908=EDGE_CURVE('',#32245,#32244,#19220,.T.);
#40909=EDGE_CURVE('',#32243,#32245,#19221,.T.);
#40910=EDGE_CURVE('',#32152,#32245,#25663,.T.);
#40911=EDGE_CURVE('',#32246,#32247,#19222,.T.);
#40912=EDGE_CURVE('',#31870,#32247,#23318,.T.);
#40913=EDGE_CURVE('',#32246,#32152,#25664,.T.);
#40914=EDGE_CURVE('',#32248,#32246,#19223,.T.);
#40915=EDGE_CURVE('',#32249,#32248,#19224,.T.);
#40916=EDGE_CURVE('',#32247,#32249,#19225,.T.);
#40917=EDGE_CURVE('',#32153,#32249,#25665,.T.);
#40918=EDGE_CURVE('',#32250,#32251,#19226,.T.);
#40919=EDGE_CURVE('',#31871,#32251,#23319,.T.);
#40920=EDGE_CURVE('',#32250,#32153,#25666,.T.);
#40921=EDGE_CURVE('',#32252,#32250,#19227,.T.);
#40922=EDGE_CURVE('',#32253,#32252,#19228,.T.);
#40923=EDGE_CURVE('',#32251,#32253,#19229,.T.);
#40924=EDGE_CURVE('',#32154,#32253,#25667,.T.);
#40925=EDGE_CURVE('',#31872,#28947,#23320,.T.);
#40926=EDGE_CURVE('',#28946,#32154,#25668,.T.);
#40927=EDGE_CURVE('',#32155,#28949,#25669,.T.);
#40928=EDGE_CURVE('',#32254,#32255,#19230,.T.);
#40929=EDGE_CURVE('',#31873,#32255,#23321,.T.);
#40930=EDGE_CURVE('',#32254,#32155,#25670,.T.);
#40931=EDGE_CURVE('',#32256,#32254,#19231,.T.);
#40932=EDGE_CURVE('',#32257,#32256,#19232,.T.);
#40933=EDGE_CURVE('',#32255,#32257,#19233,.T.);
#40934=EDGE_CURVE('',#32156,#32257,#25671,.T.);
#40935=EDGE_CURVE('',#32258,#32259,#19234,.T.);
#40936=EDGE_CURVE('',#31874,#32259,#23322,.T.);
#40937=EDGE_CURVE('',#32258,#32156,#25672,.T.);
#40938=EDGE_CURVE('',#32260,#32258,#19235,.T.);
#40939=EDGE_CURVE('',#32261,#32260,#19236,.T.);
#40940=EDGE_CURVE('',#32259,#32261,#19237,.T.);
#40941=EDGE_CURVE('',#32157,#32261,#25673,.T.);
#40942=EDGE_CURVE('',#32262,#32263,#19238,.T.);
#40943=EDGE_CURVE('',#31875,#32263,#23323,.T.);
#40944=EDGE_CURVE('',#32262,#32157,#25674,.T.);
#40945=EDGE_CURVE('',#32264,#32262,#19239,.T.);
#40946=EDGE_CURVE('',#32265,#32264,#19240,.T.);
#40947=EDGE_CURVE('',#32263,#32265,#19241,.T.);
#40948=EDGE_CURVE('',#32158,#32265,#25675,.T.);
#40949=EDGE_CURVE('',#32266,#32267,#19242,.T.);
#40950=EDGE_CURVE('',#31876,#32267,#23324,.T.);
#40951=EDGE_CURVE('',#32266,#32158,#25676,.T.);
#40952=EDGE_CURVE('',#32268,#32266,#19243,.T.);
#40953=EDGE_CURVE('',#32269,#32268,#19244,.T.);
#40954=EDGE_CURVE('',#32267,#32269,#19245,.T.);
#40955=EDGE_CURVE('',#32159,#32269,#25677,.T.);
#40956=EDGE_CURVE('',#32270,#32271,#19246,.T.);
#40957=EDGE_CURVE('',#31877,#32271,#23325,.T.);
#40958=EDGE_CURVE('',#32270,#32159,#25678,.T.);
#40959=EDGE_CURVE('',#32271,#32272,#19247,.T.);
#40960=EDGE_CURVE('',#32160,#32272,#25679,.T.);
#40961=EDGE_CURVE('',#32273,#32270,#19248,.T.);
#40962=EDGE_CURVE('',#32272,#32273,#19249,.T.);
#40963=EDGE_CURVE('',#32274,#32160,#25680,.T.);
#40964=EDGE_CURVE('',#32274,#32275,#19250,.T.);
#40965=EDGE_CURVE('',#31878,#32275,#23326,.T.);
#40966=EDGE_CURVE('',#32275,#32276,#19251,.T.);
#40967=EDGE_CURVE('',#32277,#32274,#19252,.T.);
#40968=EDGE_CURVE('',#32276,#32277,#19253,.T.);
#40969=EDGE_CURVE('',#32161,#32276,#25681,.T.);
#40970=EDGE_CURVE('',#32278,#32279,#19254,.T.);
#40971=EDGE_CURVE('',#31879,#32279,#23327,.T.);
#40972=EDGE_CURVE('',#32278,#32161,#25682,.T.);
#40973=EDGE_CURVE('',#32280,#32278,#19255,.T.);
#40974=EDGE_CURVE('',#32281,#32280,#19256,.T.);
#40975=EDGE_CURVE('',#32279,#32281,#19257,.T.);
#40976=EDGE_CURVE('',#32162,#32281,#25683,.T.);
#40977=EDGE_CURVE('',#32282,#32283,#19258,.T.);
#40978=EDGE_CURVE('',#31880,#32283,#23328,.T.);
#40979=EDGE_CURVE('',#32282,#32162,#25684,.T.);
#40980=EDGE_CURVE('',#32284,#32282,#19259,.T.);
#40981=EDGE_CURVE('',#32285,#32284,#19260,.T.);
#40982=EDGE_CURVE('',#32283,#32285,#19261,.T.);
#40983=EDGE_CURVE('',#32163,#32285,#25685,.T.);
#40984=EDGE_CURVE('',#32286,#32287,#19262,.T.);
#40985=EDGE_CURVE('',#31881,#32287,#23329,.T.);
#40986=EDGE_CURVE('',#32286,#32163,#25686,.T.);
#40987=EDGE_CURVE('',#32288,#32286,#19263,.T.);
#40988=EDGE_CURVE('',#32289,#32288,#19264,.T.);
#40989=EDGE_CURVE('',#32287,#32289,#19265,.T.);
#40990=EDGE_CURVE('',#32164,#32289,#25687,.T.);
#40991=EDGE_CURVE('',#32290,#32291,#19266,.T.);
#40992=EDGE_CURVE('',#31882,#32291,#23330,.T.);
#40993=EDGE_CURVE('',#32290,#32164,#25688,.T.);
#40994=EDGE_CURVE('',#32292,#32290,#19267,.T.);
#40995=EDGE_CURVE('',#32293,#32292,#19268,.T.);
#40996=EDGE_CURVE('',#32291,#32293,#19269,.T.);
#40997=EDGE_CURVE('',#32165,#32293,#25689,.T.);
#40998=EDGE_CURVE('',#32294,#32295,#19270,.T.);
#40999=EDGE_CURVE('',#31883,#32295,#23331,.T.);
#41000=EDGE_CURVE('',#32294,#32165,#25690,.T.);
#41001=EDGE_CURVE('',#32296,#32294,#19271,.T.);
#41002=EDGE_CURVE('',#32297,#32296,#19272,.T.);
#41003=EDGE_CURVE('',#32295,#32297,#19273,.T.);
#41004=EDGE_CURVE('',#32166,#32297,#25691,.T.);
#41005=EDGE_CURVE('',#32298,#32299,#19274,.T.);
#41006=EDGE_CURVE('',#31884,#32299,#23332,.T.);
#41007=EDGE_CURVE('',#32298,#32166,#25692,.T.);
#41008=EDGE_CURVE('',#32300,#32298,#19275,.T.);
#41009=EDGE_CURVE('',#32301,#32300,#19276,.T.);
#41010=EDGE_CURVE('',#32299,#32301,#19277,.T.);
#41011=EDGE_CURVE('',#32167,#32301,#25693,.T.);
#41012=EDGE_CURVE('',#32302,#32303,#19278,.T.);
#41013=EDGE_CURVE('',#31885,#32303,#23333,.T.);
#41014=EDGE_CURVE('',#32302,#32167,#25694,.T.);
#41015=EDGE_CURVE('',#32304,#32302,#19279,.T.);
#41016=EDGE_CURVE('',#32305,#32304,#19280,.T.);
#41017=EDGE_CURVE('',#32303,#32305,#19281,.T.);
#41018=EDGE_CURVE('',#32168,#32305,#25695,.T.);
#41019=EDGE_CURVE('',#32306,#32307,#19282,.T.);
#41020=EDGE_CURVE('',#31886,#32307,#23334,.T.);
#41021=EDGE_CURVE('',#32306,#32168,#25696,.T.);
#41022=EDGE_CURVE('',#32308,#32306,#19283,.T.);
#41023=EDGE_CURVE('',#32309,#32308,#19284,.T.);
#41024=EDGE_CURVE('',#32307,#32309,#19285,.T.);
#41025=EDGE_CURVE('',#32140,#32309,#25697,.T.);
#41026=EDGE_CURVE('',#32310,#32169,#25698,.T.);
#41027=EDGE_CURVE('',#32310,#32311,#19286,.T.);
#41028=EDGE_CURVE('',#31887,#32311,#23335,.T.);
#41029=EDGE_CURVE('',#32311,#32312,#19287,.T.);
#41030=EDGE_CURVE('',#32170,#32312,#25699,.T.);
#41031=EDGE_CURVE('',#32313,#32310,#19288,.T.);
#41032=EDGE_CURVE('',#32312,#32313,#19289,.T.);
#41033=EDGE_CURVE('',#32314,#32170,#25700,.T.);
#41034=EDGE_CURVE('',#32314,#32315,#19290,.T.);
#41035=EDGE_CURVE('',#31888,#32315,#23336,.T.);
#41036=EDGE_CURVE('',#32315,#32316,#19291,.T.);
#41037=EDGE_CURVE('',#32171,#32316,#25701,.T.);
#41038=EDGE_CURVE('',#32317,#32314,#19292,.T.);
#41039=EDGE_CURVE('',#32316,#32317,#19293,.T.);
#41040=EDGE_CURVE('',#32318,#32171,#25702,.T.);
#41041=EDGE_CURVE('',#32318,#32319,#19294,.T.);
#41042=EDGE_CURVE('',#31889,#32319,#23337,.T.);
#41043=EDGE_CURVE('',#32319,#32320,#19295,.T.);
#41044=EDGE_CURVE('',#32172,#32320,#25703,.T.);
#41045=EDGE_CURVE('',#32321,#32318,#19296,.T.);
#41046=EDGE_CURVE('',#32320,#32321,#19297,.T.);
#41047=EDGE_CURVE('',#32322,#32172,#25704,.T.);
#41048=EDGE_CURVE('',#32322,#32323,#19298,.T.);
#41049=EDGE_CURVE('',#31890,#32323,#23338,.T.);
#41050=EDGE_CURVE('',#32323,#32324,#19299,.T.);
#41051=EDGE_CURVE('',#32173,#32324,#25705,.T.);
#41052=EDGE_CURVE('',#32325,#32322,#19300,.T.);
#41053=EDGE_CURVE('',#32324,#32325,#19301,.T.);
#41054=EDGE_CURVE('',#32326,#32173,#25706,.T.);
#41055=EDGE_CURVE('',#32326,#32327,#19302,.T.);
#41056=EDGE_CURVE('',#31891,#32327,#23339,.T.);
#41057=EDGE_CURVE('',#32327,#32328,#19303,.T.);
#41058=EDGE_CURVE('',#32174,#32328,#25707,.T.);
#41059=EDGE_CURVE('',#32329,#32326,#19304,.T.);
#41060=EDGE_CURVE('',#32328,#32329,#19305,.T.);
#41061=EDGE_CURVE('',#32330,#32174,#25708,.T.);
#41062=EDGE_CURVE('',#32330,#32331,#19306,.T.);
#41063=EDGE_CURVE('',#31892,#32331,#23340,.T.);
#41064=EDGE_CURVE('',#32331,#32332,#19307,.T.);
#41065=EDGE_CURVE('',#32175,#32332,#25709,.T.);
#41066=EDGE_CURVE('',#32333,#32330,#19308,.T.);
#41067=EDGE_CURVE('',#32332,#32333,#19309,.T.);
#41068=EDGE_CURVE('',#32334,#32175,#25710,.T.);
#41069=EDGE_CURVE('',#32334,#32335,#19310,.T.);
#41070=EDGE_CURVE('',#31893,#32335,#23341,.T.);
#41071=EDGE_CURVE('',#32335,#32336,#19311,.T.);
#41072=EDGE_CURVE('',#32176,#32336,#25711,.T.);
#41073=EDGE_CURVE('',#32337,#32334,#19312,.T.);
#41074=EDGE_CURVE('',#32336,#32337,#19313,.T.);
#41075=EDGE_CURVE('',#32338,#32176,#25712,.T.);
#41076=EDGE_CURVE('',#32338,#32339,#19314,.T.);
#41077=EDGE_CURVE('',#31894,#32339,#23342,.T.);
#41078=EDGE_CURVE('',#32339,#32340,#19315,.T.);
#41079=EDGE_CURVE('',#32177,#32340,#25713,.T.);
#41080=EDGE_CURVE('',#32341,#32338,#19316,.T.);
#41081=EDGE_CURVE('',#32340,#32341,#19317,.T.);
#41082=EDGE_CURVE('',#32342,#32177,#25714,.T.);
#41083=EDGE_CURVE('',#32342,#32343,#19318,.T.);
#41084=EDGE_CURVE('',#31895,#32343,#23343,.T.);
#41085=EDGE_CURVE('',#32343,#32344,#19319,.T.);
#41086=EDGE_CURVE('',#32178,#32344,#25715,.T.);
#41087=EDGE_CURVE('',#32345,#32342,#19320,.T.);
#41088=EDGE_CURVE('',#32344,#32345,#19321,.T.);
#41089=EDGE_CURVE('',#32346,#32178,#25716,.T.);
#41090=EDGE_CURVE('',#32346,#32347,#19322,.T.);
#41091=EDGE_CURVE('',#31896,#32347,#23344,.T.);
#41092=EDGE_CURVE('',#32347,#32348,#19323,.T.);
#41093=EDGE_CURVE('',#32179,#32348,#25717,.T.);
#41094=EDGE_CURVE('',#32349,#32346,#19324,.T.);
#41095=EDGE_CURVE('',#32348,#32349,#19325,.T.);
#41096=EDGE_CURVE('',#32350,#32179,#25718,.T.);
#41097=EDGE_CURVE('',#32350,#32351,#19326,.T.);
#41098=EDGE_CURVE('',#31897,#32351,#23345,.T.);
#41099=EDGE_CURVE('',#32351,#32352,#19327,.T.);
#41100=EDGE_CURVE('',#32180,#32352,#25719,.T.);
#41101=EDGE_CURVE('',#32353,#32350,#19328,.T.);
#41102=EDGE_CURVE('',#32352,#32353,#19329,.T.);
#41103=EDGE_CURVE('',#32354,#32180,#25720,.T.);
#41104=EDGE_CURVE('',#32354,#32355,#19330,.T.);
#41105=EDGE_CURVE('',#31898,#32355,#23346,.T.);
#41106=EDGE_CURVE('',#32355,#32356,#19331,.T.);
#41107=EDGE_CURVE('',#32181,#32356,#25721,.T.);
#41108=EDGE_CURVE('',#32357,#32354,#19332,.T.);
#41109=EDGE_CURVE('',#32356,#32357,#19333,.T.);
#41110=EDGE_CURVE('',#32358,#32181,#25722,.T.);
#41111=EDGE_CURVE('',#32358,#32359,#19334,.T.);
#41112=EDGE_CURVE('',#31899,#32359,#23347,.T.);
#41113=EDGE_CURVE('',#32359,#32360,#19335,.T.);
#41114=EDGE_CURVE('',#32182,#32360,#25723,.T.);
#41115=EDGE_CURVE('',#32361,#32358,#19336,.T.);
#41116=EDGE_CURVE('',#32360,#32361,#19337,.T.);
#41117=EDGE_CURVE('',#32362,#32182,#25724,.T.);
#41118=EDGE_CURVE('',#32362,#32363,#19338,.T.);
#41119=EDGE_CURVE('',#31900,#32363,#23348,.T.);
#41120=EDGE_CURVE('',#32363,#32364,#19339,.T.);
#41121=EDGE_CURVE('',#32183,#32364,#25725,.T.);
#41122=EDGE_CURVE('',#32365,#32362,#19340,.T.);
#41123=EDGE_CURVE('',#32364,#32365,#19341,.T.);
#41124=EDGE_CURVE('',#32366,#32183,#25726,.T.);
#41125=EDGE_CURVE('',#32366,#32367,#19342,.T.);
#41126=EDGE_CURVE('',#31901,#32367,#23349,.T.);
#41127=EDGE_CURVE('',#32367,#32368,#19343,.T.);
#41128=EDGE_CURVE('',#32184,#32368,#25727,.T.);
#41129=EDGE_CURVE('',#32369,#32366,#19344,.T.);
#41130=EDGE_CURVE('',#32368,#32369,#19345,.T.);
#41131=EDGE_CURVE('',#32370,#32184,#25728,.T.);
#41132=EDGE_CURVE('',#32370,#32371,#19346,.T.);
#41133=EDGE_CURVE('',#31902,#32371,#23350,.T.);
#41134=EDGE_CURVE('',#32371,#32372,#19347,.T.);
#41135=EDGE_CURVE('',#32185,#32372,#25729,.T.);
#41136=EDGE_CURVE('',#32373,#32370,#19348,.T.);
#41137=EDGE_CURVE('',#32372,#32373,#19349,.T.);
#41138=EDGE_CURVE('',#32374,#32185,#25730,.T.);
#41139=EDGE_CURVE('',#32374,#32375,#19350,.T.);
#41140=EDGE_CURVE('',#31903,#32375,#23351,.T.);
#41141=EDGE_CURVE('',#32375,#32376,#19351,.T.);
#41142=EDGE_CURVE('',#32186,#32376,#25731,.T.);
#41143=EDGE_CURVE('',#32377,#32374,#19352,.T.);
#41144=EDGE_CURVE('',#32376,#32377,#19353,.T.);
#41145=EDGE_CURVE('',#32378,#32186,#25732,.T.);
#41146=EDGE_CURVE('',#32378,#32379,#19354,.T.);
#41147=EDGE_CURVE('',#31904,#32379,#23352,.T.);
#41148=EDGE_CURVE('',#32379,#32380,#19355,.T.);
#41149=EDGE_CURVE('',#32187,#32380,#25733,.T.);
#41150=EDGE_CURVE('',#32381,#32378,#19356,.T.);
#41151=EDGE_CURVE('',#32380,#32381,#19357,.T.);
#41152=EDGE_CURVE('',#32382,#32187,#25734,.T.);
#41153=EDGE_CURVE('',#32382,#32383,#19358,.T.);
#41154=EDGE_CURVE('',#31905,#32383,#23353,.T.);
#41155=EDGE_CURVE('',#32383,#32384,#19359,.T.);
#41156=EDGE_CURVE('',#32188,#32384,#25735,.T.);
#41157=EDGE_CURVE('',#32385,#32382,#19360,.T.);
#41158=EDGE_CURVE('',#32384,#32385,#19361,.T.);
#41159=EDGE_CURVE('',#32386,#32188,#25736,.T.);
#41160=EDGE_CURVE('',#32386,#32387,#19362,.T.);
#41161=EDGE_CURVE('',#31906,#32387,#23354,.T.);
#41162=EDGE_CURVE('',#32387,#32388,#19363,.T.);
#41163=EDGE_CURVE('',#32189,#32388,#25737,.T.);
#41164=EDGE_CURVE('',#32389,#32386,#19364,.T.);
#41165=EDGE_CURVE('',#32388,#32389,#19365,.T.);
#41166=EDGE_CURVE('',#32390,#32189,#25738,.T.);
#41167=EDGE_CURVE('',#32390,#32391,#19366,.T.);
#41168=EDGE_CURVE('',#31907,#32391,#23355,.T.);
#41169=EDGE_CURVE('',#32391,#32392,#19367,.T.);
#41170=EDGE_CURVE('',#32190,#32392,#25739,.T.);
#41171=EDGE_CURVE('',#32393,#32390,#19368,.T.);
#41172=EDGE_CURVE('',#32392,#32393,#19369,.T.);
#41173=EDGE_CURVE('',#28943,#32190,#25740,.T.);
#41174=EDGE_CURVE('',#31908,#28945,#23356,.T.);
#41175=EDGE_CURVE('',#32191,#28944,#25741,.T.);
#41176=EDGE_CURVE('',#32394,#32191,#25742,.T.);
#41177=EDGE_CURVE('',#32394,#32395,#19370,.T.);
#41178=EDGE_CURVE('',#31909,#32395,#23357,.T.);
#41179=EDGE_CURVE('',#32395,#32396,#19371,.T.);
#41180=EDGE_CURVE('',#32192,#32396,#25743,.T.);
#41181=EDGE_CURVE('',#32397,#32394,#19372,.T.);
#41182=EDGE_CURVE('',#32396,#32397,#19373,.T.);
#41183=EDGE_CURVE('',#32398,#32192,#25744,.T.);
#41184=EDGE_CURVE('',#32398,#32399,#19374,.T.);
#41185=EDGE_CURVE('',#31910,#32399,#23358,.T.);
#41186=EDGE_CURVE('',#32399,#32400,#19375,.T.);
#41187=EDGE_CURVE('',#32193,#32400,#25745,.T.);
#41188=EDGE_CURVE('',#32401,#32398,#19376,.T.);
#41189=EDGE_CURVE('',#32400,#32401,#19377,.T.);
#41190=EDGE_CURVE('',#32402,#32193,#25746,.T.);
#41191=EDGE_CURVE('',#32402,#32403,#19378,.T.);
#41192=EDGE_CURVE('',#31911,#32403,#23359,.T.);
#41193=EDGE_CURVE('',#32403,#32404,#19379,.T.);
#41194=EDGE_CURVE('',#32194,#32404,#25747,.T.);
#41195=EDGE_CURVE('',#32405,#32402,#19380,.T.);
#41196=EDGE_CURVE('',#32404,#32405,#19381,.T.);
#41197=EDGE_CURVE('',#32406,#32194,#25748,.T.);
#41198=EDGE_CURVE('',#32406,#32407,#19382,.T.);
#41199=EDGE_CURVE('',#31912,#32407,#23360,.T.);
#41200=EDGE_CURVE('',#32407,#32408,#19383,.T.);
#41201=EDGE_CURVE('',#32195,#32408,#25749,.T.);
#41202=EDGE_CURVE('',#32409,#32406,#19384,.T.);
#41203=EDGE_CURVE('',#32408,#32409,#19385,.T.);
#41204=EDGE_CURVE('',#32410,#32195,#25750,.T.);
#41205=EDGE_CURVE('',#32410,#32411,#19386,.T.);
#41206=EDGE_CURVE('',#31913,#32411,#23361,.T.);
#41207=EDGE_CURVE('',#32411,#32412,#19387,.T.);
#41208=EDGE_CURVE('',#32196,#32412,#25751,.T.);
#41209=EDGE_CURVE('',#32413,#32410,#19388,.T.);
#41210=EDGE_CURVE('',#32412,#32413,#19389,.T.);
#41211=EDGE_CURVE('',#32414,#32196,#25752,.T.);
#41212=EDGE_CURVE('',#32414,#32415,#19390,.T.);
#41213=EDGE_CURVE('',#31914,#32415,#23362,.T.);
#41214=EDGE_CURVE('',#32415,#32416,#19391,.T.);
#41215=EDGE_CURVE('',#32197,#32416,#25753,.T.);
#41216=EDGE_CURVE('',#32417,#32414,#19392,.T.);
#41217=EDGE_CURVE('',#32416,#32417,#19393,.T.);
#41218=EDGE_CURVE('',#32418,#32197,#25754,.T.);
#41219=EDGE_CURVE('',#32418,#32419,#19394,.T.);
#41220=EDGE_CURVE('',#31915,#32419,#23363,.T.);
#41221=EDGE_CURVE('',#32419,#32420,#19395,.T.);
#41222=EDGE_CURVE('',#32169,#32420,#25755,.T.);
#41223=EDGE_CURVE('',#32421,#32418,#19396,.T.);
#41224=EDGE_CURVE('',#32420,#32421,#19397,.T.);
#41225=EDGE_CURVE('',#32422,#32140,#19398,.T.);
#41226=EDGE_CURVE('',#32200,#32422,#23364,.T.);
#41227=EDGE_CURVE('',#32141,#32422,#19399,.T.);
#41228=EDGE_CURVE('',#32423,#32141,#19400,.T.);
#41229=EDGE_CURVE('',#32204,#32423,#23365,.T.);
#41230=EDGE_CURVE('',#32142,#32423,#19401,.T.);
#41231=EDGE_CURVE('',#32424,#32142,#19402,.T.);
#41232=EDGE_CURVE('',#32208,#32424,#23366,.T.);
#41233=EDGE_CURVE('',#32143,#32424,#19403,.T.);
#41234=EDGE_CURVE('',#32425,#32143,#19404,.T.);
#41235=EDGE_CURVE('',#32212,#32425,#23367,.T.);
#41236=EDGE_CURVE('',#32144,#32425,#19405,.T.);
#41237=EDGE_CURVE('',#32426,#32144,#19406,.T.);
#41238=EDGE_CURVE('',#32216,#32426,#23368,.T.);
#41239=EDGE_CURVE('',#32145,#32426,#19407,.T.);
#41240=EDGE_CURVE('',#32427,#32145,#19408,.T.);
#41241=EDGE_CURVE('',#32220,#32427,#23369,.T.);
#41242=EDGE_CURVE('',#32146,#32427,#19409,.T.);
#41243=EDGE_CURVE('',#32428,#32146,#19410,.T.);
#41244=EDGE_CURVE('',#32224,#32428,#23370,.T.);
#41245=EDGE_CURVE('',#32147,#32428,#19411,.T.);
#41246=EDGE_CURVE('',#32429,#32147,#19412,.T.);
#41247=EDGE_CURVE('',#32228,#32429,#23371,.T.);
#41248=EDGE_CURVE('',#32148,#32429,#19413,.T.);
#41249=EDGE_CURVE('',#32430,#32148,#19414,.T.);
#41250=EDGE_CURVE('',#32232,#32430,#23372,.T.);
#41251=EDGE_CURVE('',#32149,#32430,#19415,.T.);
#41252=EDGE_CURVE('',#32431,#32149,#19416,.T.);
#41253=EDGE_CURVE('',#32236,#32431,#23373,.T.);
#41254=EDGE_CURVE('',#32150,#32431,#19417,.T.);
#41255=EDGE_CURVE('',#32432,#32150,#19418,.T.);
#41256=EDGE_CURVE('',#32240,#32432,#23374,.T.);
#41257=EDGE_CURVE('',#32151,#32432,#19419,.T.);
#41258=EDGE_CURVE('',#32433,#32151,#19420,.T.);
#41259=EDGE_CURVE('',#32244,#32433,#23375,.T.);
#41260=EDGE_CURVE('',#32152,#32433,#19421,.T.);
#41261=EDGE_CURVE('',#32434,#32152,#19422,.T.);
#41262=EDGE_CURVE('',#32248,#32434,#23376,.T.);
#41263=EDGE_CURVE('',#32153,#32434,#19423,.T.);
#41264=EDGE_CURVE('',#32435,#32153,#19424,.T.);
#41265=EDGE_CURVE('',#32252,#32435,#23377,.T.);
#41266=EDGE_CURVE('',#32154,#32435,#19425,.T.);
#41267=EDGE_CURVE('',#32436,#32154,#19426,.T.);
#41268=EDGE_CURVE('',#28948,#32436,#23378,.T.);
#41269=EDGE_CURVE('',#32155,#32436,#19427,.T.);
#41270=EDGE_CURVE('',#32437,#32155,#19428,.T.);
#41271=EDGE_CURVE('',#32256,#32437,#23379,.T.);
#41272=EDGE_CURVE('',#32156,#32437,#19429,.T.);
#41273=EDGE_CURVE('',#32438,#32156,#19430,.T.);
#41274=EDGE_CURVE('',#32260,#32438,#23380,.T.);
#41275=EDGE_CURVE('',#32157,#32438,#19431,.T.);
#41276=EDGE_CURVE('',#32439,#32157,#19432,.T.);
#41277=EDGE_CURVE('',#32264,#32439,#23381,.T.);
#41278=EDGE_CURVE('',#32158,#32439,#19433,.T.);
#41279=EDGE_CURVE('',#32440,#32158,#19434,.T.);
#41280=EDGE_CURVE('',#32268,#32440,#23382,.T.);
#41281=EDGE_CURVE('',#32159,#32440,#19435,.T.);
#41282=EDGE_CURVE('',#32441,#32159,#19436,.T.);
#41283=EDGE_CURVE('',#32273,#32441,#23383,.T.);
#41284=EDGE_CURVE('',#32160,#32441,#19437,.T.);
#41285=EDGE_CURVE('',#32442,#32160,#19438,.T.);
#41286=EDGE_CURVE('',#32277,#32442,#23384,.T.);
#41287=EDGE_CURVE('',#32161,#32442,#19439,.T.);
#41288=EDGE_CURVE('',#32443,#32161,#19440,.T.);
#41289=EDGE_CURVE('',#32280,#32443,#23385,.T.);
#41290=EDGE_CURVE('',#32162,#32443,#19441,.T.);
#41291=EDGE_CURVE('',#32444,#32162,#19442,.T.);
#41292=EDGE_CURVE('',#32284,#32444,#23386,.T.);
#41293=EDGE_CURVE('',#32163,#32444,#19443,.T.);
#41294=EDGE_CURVE('',#32445,#32163,#19444,.T.);
#41295=EDGE_CURVE('',#32288,#32445,#23387,.T.);
#41296=EDGE_CURVE('',#32164,#32445,#19445,.T.);
#41297=EDGE_CURVE('',#32446,#32164,#19446,.T.);
#41298=EDGE_CURVE('',#32292,#32446,#23388,.T.);
#41299=EDGE_CURVE('',#32165,#32446,#19447,.T.);
#41300=EDGE_CURVE('',#32447,#32165,#19448,.T.);
#41301=EDGE_CURVE('',#32296,#32447,#23389,.T.);
#41302=EDGE_CURVE('',#32166,#32447,#19449,.T.);
#41303=EDGE_CURVE('',#32448,#32166,#19450,.T.);
#41304=EDGE_CURVE('',#32300,#32448,#23390,.T.);
#41305=EDGE_CURVE('',#32167,#32448,#19451,.T.);
#41306=EDGE_CURVE('',#32449,#32167,#19452,.T.);
#41307=EDGE_CURVE('',#32304,#32449,#23391,.T.);
#41308=EDGE_CURVE('',#32168,#32449,#19453,.T.);
#41309=EDGE_CURVE('',#32450,#32168,#19454,.T.);
#41310=EDGE_CURVE('',#32308,#32450,#23392,.T.);
#41311=EDGE_CURVE('',#32140,#32450,#19455,.T.);
#41312=EDGE_CURVE('',#32451,#32169,#19456,.T.);
#41313=EDGE_CURVE('',#32313,#32451,#23393,.T.);
#41314=EDGE_CURVE('',#32170,#32451,#19457,.T.);
#41315=EDGE_CURVE('',#32452,#32170,#19458,.T.);
#41316=EDGE_CURVE('',#32317,#32452,#23394,.T.);
#41317=EDGE_CURVE('',#32171,#32452,#19459,.T.);
#41318=EDGE_CURVE('',#32453,#32171,#19460,.T.);
#41319=EDGE_CURVE('',#32321,#32453,#23395,.T.);
#41320=EDGE_CURVE('',#32172,#32453,#19461,.T.);
#41321=EDGE_CURVE('',#32454,#32172,#19462,.T.);
#41322=EDGE_CURVE('',#32325,#32454,#23396,.T.);
#41323=EDGE_CURVE('',#32173,#32454,#19463,.T.);
#41324=EDGE_CURVE('',#32455,#32173,#19464,.T.);
#41325=EDGE_CURVE('',#32329,#32455,#23397,.T.);
#41326=EDGE_CURVE('',#32174,#32455,#19465,.T.);
#41327=EDGE_CURVE('',#32456,#32174,#19466,.T.);
#41328=EDGE_CURVE('',#32333,#32456,#23398,.T.);
#41329=EDGE_CURVE('',#32175,#32456,#19467,.T.);
#41330=EDGE_CURVE('',#32457,#32175,#19468,.T.);
#41331=EDGE_CURVE('',#32337,#32457,#23399,.T.);
#41332=EDGE_CURVE('',#32176,#32457,#19469,.T.);
#41333=EDGE_CURVE('',#32458,#32176,#19470,.T.);
#41334=EDGE_CURVE('',#32341,#32458,#23400,.T.);
#41335=EDGE_CURVE('',#32177,#32458,#19471,.T.);
#41336=EDGE_CURVE('',#32459,#32177,#19472,.T.);
#41337=EDGE_CURVE('',#32345,#32459,#23401,.T.);
#41338=EDGE_CURVE('',#32178,#32459,#19473,.T.);
#41339=EDGE_CURVE('',#32460,#32178,#19474,.T.);
#41340=EDGE_CURVE('',#32349,#32460,#23402,.T.);
#41341=EDGE_CURVE('',#32179,#32460,#19475,.T.);
#41342=EDGE_CURVE('',#32461,#32179,#19476,.T.);
#41343=EDGE_CURVE('',#32353,#32461,#23403,.T.);
#41344=EDGE_CURVE('',#32180,#32461,#19477,.T.);
#41345=EDGE_CURVE('',#32462,#32180,#19478,.T.);
#41346=EDGE_CURVE('',#32357,#32462,#23404,.T.);
#41347=EDGE_CURVE('',#32181,#32462,#19479,.T.);
#41348=EDGE_CURVE('',#32463,#32181,#19480,.T.);
#41349=EDGE_CURVE('',#32361,#32463,#23405,.T.);
#41350=EDGE_CURVE('',#32182,#32463,#19481,.T.);
#41351=EDGE_CURVE('',#32464,#32182,#19482,.T.);
#41352=EDGE_CURVE('',#32365,#32464,#23406,.T.);
#41353=EDGE_CURVE('',#32183,#32464,#19483,.T.);
#41354=EDGE_CURVE('',#32465,#32183,#19484,.T.);
#41355=EDGE_CURVE('',#32369,#32465,#23407,.T.);
#41356=EDGE_CURVE('',#32184,#32465,#19485,.T.);
#41357=EDGE_CURVE('',#32466,#32184,#19486,.T.);
#41358=EDGE_CURVE('',#32373,#32466,#23408,.T.);
#41359=EDGE_CURVE('',#32185,#32466,#19487,.T.);
#41360=EDGE_CURVE('',#32467,#32185,#19488,.T.);
#41361=EDGE_CURVE('',#32377,#32467,#23409,.T.);
#41362=EDGE_CURVE('',#32186,#32467,#19489,.T.);
#41363=EDGE_CURVE('',#32468,#32186,#19490,.T.);
#41364=EDGE_CURVE('',#32381,#32468,#23410,.T.);
#41365=EDGE_CURVE('',#32187,#32468,#19491,.T.);
#41366=EDGE_CURVE('',#32469,#32187,#19492,.T.);
#41367=EDGE_CURVE('',#32385,#32469,#23411,.T.);
#41368=EDGE_CURVE('',#32188,#32469,#19493,.T.);
#41369=EDGE_CURVE('',#32470,#32188,#19494,.T.);
#41370=EDGE_CURVE('',#32389,#32470,#23412,.T.);
#41371=EDGE_CURVE('',#32189,#32470,#19495,.T.);
#41372=EDGE_CURVE('',#32471,#32189,#19496,.T.);
#41373=EDGE_CURVE('',#32393,#32471,#23413,.T.);
#41374=EDGE_CURVE('',#32190,#32471,#19497,.T.);
#41375=EDGE_CURVE('',#32472,#32190,#19498,.T.);
#41376=EDGE_CURVE('',#28942,#32472,#23414,.T.);
#41377=EDGE_CURVE('',#32191,#32472,#19499,.T.);
#41378=EDGE_CURVE('',#32473,#32191,#19500,.T.);
#41379=EDGE_CURVE('',#32397,#32473,#23415,.T.);
#41380=EDGE_CURVE('',#32192,#32473,#19501,.T.);
#41381=EDGE_CURVE('',#32474,#32192,#19502,.T.);
#41382=EDGE_CURVE('',#32401,#32474,#23416,.T.);
#41383=EDGE_CURVE('',#32193,#32474,#19503,.T.);
#41384=EDGE_CURVE('',#32475,#32193,#19504,.T.);
#41385=EDGE_CURVE('',#32405,#32475,#23417,.T.);
#41386=EDGE_CURVE('',#32194,#32475,#19505,.T.);
#41387=EDGE_CURVE('',#32476,#32194,#19506,.T.);
#41388=EDGE_CURVE('',#32409,#32476,#23418,.T.);
#41389=EDGE_CURVE('',#32195,#32476,#19507,.T.);
#41390=EDGE_CURVE('',#32477,#32195,#19508,.T.);
#41391=EDGE_CURVE('',#32413,#32477,#23419,.T.);
#41392=EDGE_CURVE('',#32196,#32477,#19509,.T.);
#41393=EDGE_CURVE('',#32478,#32196,#19510,.T.);
#41394=EDGE_CURVE('',#32417,#32478,#23420,.T.);
#41395=EDGE_CURVE('',#32197,#32478,#19511,.T.);
#41396=EDGE_CURVE('',#32479,#32197,#19512,.T.);
#41397=EDGE_CURVE('',#32421,#32479,#23421,.T.);
#41398=EDGE_CURVE('',#32169,#32479,#19513,.T.);
#41399=EDGE_CURVE('',#32480,#32481,#19514,.T.);
#41400=EDGE_CURVE('',#32422,#32481,#25756,.T.);
#41401=EDGE_CURVE('',#32480,#32140,#23422,.T.);
#41402=EDGE_CURVE('',#32482,#32483,#19515,.T.);
#41403=EDGE_CURVE('',#32141,#32483,#23423,.T.);
#41404=EDGE_CURVE('',#32482,#32422,#25757,.T.);
#41405=EDGE_CURVE('',#32484,#32482,#19516,.T.);
#41406=EDGE_CURVE('',#32485,#32484,#19517,.T.);
#41407=EDGE_CURVE('',#32483,#32485,#19518,.T.);
#41408=EDGE_CURVE('',#32423,#32485,#25758,.T.);
#41409=EDGE_CURVE('',#32486,#32487,#19519,.T.);
#41410=EDGE_CURVE('',#32142,#32487,#23424,.T.);
#41411=EDGE_CURVE('',#32486,#32423,#25759,.T.);
#41412=EDGE_CURVE('',#32488,#32486,#19520,.T.);
#41413=EDGE_CURVE('',#32489,#32488,#19521,.T.);
#41414=EDGE_CURVE('',#32487,#32489,#19522,.T.);
#41415=EDGE_CURVE('',#32424,#32489,#25760,.T.);
#41416=EDGE_CURVE('',#32490,#32491,#19523,.T.);
#41417=EDGE_CURVE('',#32143,#32491,#23425,.T.);
#41418=EDGE_CURVE('',#32490,#32424,#25761,.T.);
#41419=EDGE_CURVE('',#32492,#32490,#19524,.T.);
#41420=EDGE_CURVE('',#32493,#32492,#19525,.T.);
#41421=EDGE_CURVE('',#32491,#32493,#19526,.T.);
#41422=EDGE_CURVE('',#32425,#32493,#25762,.T.);
#41423=EDGE_CURVE('',#32494,#32495,#19527,.T.);
#41424=EDGE_CURVE('',#32144,#32495,#23426,.T.);
#41425=EDGE_CURVE('',#32494,#32425,#25763,.T.);
#41426=EDGE_CURVE('',#32496,#32494,#19528,.T.);
#41427=EDGE_CURVE('',#32497,#32496,#19529,.T.);
#41428=EDGE_CURVE('',#32495,#32497,#19530,.T.);
#41429=EDGE_CURVE('',#32426,#32497,#25764,.T.);
#41430=EDGE_CURVE('',#32498,#32499,#19531,.T.);
#41431=EDGE_CURVE('',#32145,#32499,#23427,.T.);
#41432=EDGE_CURVE('',#32498,#32426,#25765,.T.);
#41433=EDGE_CURVE('',#32500,#32498,#19532,.T.);
#41434=EDGE_CURVE('',#32501,#32500,#19533,.T.);
#41435=EDGE_CURVE('',#32499,#32501,#19534,.T.);
#41436=EDGE_CURVE('',#32427,#32501,#25766,.T.);
#41437=EDGE_CURVE('',#32502,#32503,#19535,.T.);
#41438=EDGE_CURVE('',#32146,#32503,#23428,.T.);
#41439=EDGE_CURVE('',#32502,#32427,#25767,.T.);
#41440=EDGE_CURVE('',#32504,#32502,#19536,.T.);
#41441=EDGE_CURVE('',#32505,#32504,#19537,.T.);
#41442=EDGE_CURVE('',#32503,#32505,#19538,.T.);
#41443=EDGE_CURVE('',#32428,#32505,#25768,.T.);
#41444=EDGE_CURVE('',#32147,#28938,#23429,.T.);
#41445=EDGE_CURVE('',#28940,#32428,#25769,.T.);
#41446=EDGE_CURVE('',#32429,#28939,#25770,.T.);
#41447=EDGE_CURVE('',#32506,#32507,#19539,.T.);
#41448=EDGE_CURVE('',#32148,#32507,#23430,.T.);
#41449=EDGE_CURVE('',#32506,#32429,#25771,.T.);
#41450=EDGE_CURVE('',#32508,#32506,#19540,.T.);
#41451=EDGE_CURVE('',#32509,#32508,#19541,.T.);
#41452=EDGE_CURVE('',#32507,#32509,#19542,.T.);
#41453=EDGE_CURVE('',#32430,#32509,#25772,.T.);
#41454=EDGE_CURVE('',#32510,#32511,#19543,.T.);
#41455=EDGE_CURVE('',#32149,#32511,#23431,.T.);
#41456=EDGE_CURVE('',#32510,#32430,#25773,.T.);
#41457=EDGE_CURVE('',#32512,#32510,#19544,.T.);
#41458=EDGE_CURVE('',#32513,#32512,#19545,.T.);
#41459=EDGE_CURVE('',#32511,#32513,#19546,.T.);
#41460=EDGE_CURVE('',#32431,#32513,#25774,.T.);
#41461=EDGE_CURVE('',#32514,#32515,#19547,.T.);
#41462=EDGE_CURVE('',#32150,#32515,#23432,.T.);
#41463=EDGE_CURVE('',#32514,#32431,#25775,.T.);
#41464=EDGE_CURVE('',#32516,#32514,#19548,.T.);
#41465=EDGE_CURVE('',#32517,#32516,#19549,.T.);
#41466=EDGE_CURVE('',#32515,#32517,#19550,.T.);
#41467=EDGE_CURVE('',#32432,#32517,#25776,.T.);
#41468=EDGE_CURVE('',#32518,#32519,#19551,.T.);
#41469=EDGE_CURVE('',#32151,#32519,#23433,.T.);
#41470=EDGE_CURVE('',#32518,#32432,#25777,.T.);
#41471=EDGE_CURVE('',#32520,#32518,#19552,.T.);
#41472=EDGE_CURVE('',#32521,#32520,#19553,.T.);
#41473=EDGE_CURVE('',#32519,#32521,#19554,.T.);
#41474=EDGE_CURVE('',#32433,#32521,#25778,.T.);
#41475=EDGE_CURVE('',#32522,#32523,#19555,.T.);
#41476=EDGE_CURVE('',#32152,#32523,#23434,.T.);
#41477=EDGE_CURVE('',#32522,#32433,#25779,.T.);
#41478=EDGE_CURVE('',#32524,#32522,#19556,.T.);
#41479=EDGE_CURVE('',#32525,#32524,#19557,.T.);
#41480=EDGE_CURVE('',#32523,#32525,#19558,.T.);
#41481=EDGE_CURVE('',#32434,#32525,#25780,.T.);
#41482=EDGE_CURVE('',#32526,#32527,#19559,.T.);
#41483=EDGE_CURVE('',#32153,#32527,#23435,.T.);
#41484=EDGE_CURVE('',#32526,#32434,#25781,.T.);
#41485=EDGE_CURVE('',#32528,#32526,#19560,.T.);
#41486=EDGE_CURVE('',#32529,#32528,#19561,.T.);
#41487=EDGE_CURVE('',#32527,#32529,#19562,.T.);
#41488=EDGE_CURVE('',#32435,#32529,#25782,.T.);
#41489=EDGE_CURVE('',#32530,#32531,#19563,.T.);
#41490=EDGE_CURVE('',#32154,#32531,#23436,.T.);
#41491=EDGE_CURVE('',#32530,#32435,#25783,.T.);
#41492=EDGE_CURVE('',#32532,#32530,#19564,.T.);
#41493=EDGE_CURVE('',#32533,#32532,#19565,.T.);
#41494=EDGE_CURVE('',#32531,#32533,#19566,.T.);
#41495=EDGE_CURVE('',#32436,#32533,#25784,.T.);
#41496=EDGE_CURVE('',#32534,#32535,#19567,.T.);
#41497=EDGE_CURVE('',#32155,#32535,#23437,.T.);
#41498=EDGE_CURVE('',#32534,#32436,#25785,.T.);
#41499=EDGE_CURVE('',#32536,#32534,#19568,.T.);
#41500=EDGE_CURVE('',#32537,#32536,#19569,.T.);
#41501=EDGE_CURVE('',#32535,#32537,#19570,.T.);
#41502=EDGE_CURVE('',#32437,#32537,#25786,.T.);
#41503=EDGE_CURVE('',#32538,#32539,#19571,.T.);
#41504=EDGE_CURVE('',#32156,#32539,#23438,.T.);
#41505=EDGE_CURVE('',#32538,#32437,#25787,.T.);
#41506=EDGE_CURVE('',#32540,#32538,#19572,.T.);
#41507=EDGE_CURVE('',#32541,#32540,#19573,.T.);
#41508=EDGE_CURVE('',#32539,#32541,#19574,.T.);
#41509=EDGE_CURVE('',#32438,#32541,#25788,.T.);
#41510=EDGE_CURVE('',#32542,#32543,#19575,.T.);
#41511=EDGE_CURVE('',#32157,#32543,#23439,.T.);
#41512=EDGE_CURVE('',#32542,#32438,#25789,.T.);
#41513=EDGE_CURVE('',#32544,#32542,#19576,.T.);
#41514=EDGE_CURVE('',#32545,#32544,#19577,.T.);
#41515=EDGE_CURVE('',#32543,#32545,#19578,.T.);
#41516=EDGE_CURVE('',#32439,#32545,#25790,.T.);
#41517=EDGE_CURVE('',#32546,#32547,#19579,.T.);
#41518=EDGE_CURVE('',#32158,#32547,#23440,.T.);
#41519=EDGE_CURVE('',#32546,#32439,#25791,.T.);
#41520=EDGE_CURVE('',#32548,#32546,#19580,.T.);
#41521=EDGE_CURVE('',#32549,#32548,#19581,.T.);
#41522=EDGE_CURVE('',#32547,#32549,#19582,.T.);
#41523=EDGE_CURVE('',#32440,#32549,#25792,.T.);
#41524=EDGE_CURVE('',#32550,#32551,#19583,.T.);
#41525=EDGE_CURVE('',#32159,#32551,#23441,.T.);
#41526=EDGE_CURVE('',#32550,#32440,#25793,.T.);
#41527=EDGE_CURVE('',#32551,#32552,#19584,.T.);
#41528=EDGE_CURVE('',#32441,#32552,#25794,.T.);
#41529=EDGE_CURVE('',#32553,#32550,#19585,.T.);
#41530=EDGE_CURVE('',#32552,#32553,#19586,.T.);
#41531=EDGE_CURVE('',#32554,#32441,#25795,.T.);
#41532=EDGE_CURVE('',#32554,#32555,#19587,.T.);
#41533=EDGE_CURVE('',#32160,#32555,#23442,.T.);
#41534=EDGE_CURVE('',#32555,#32556,#19588,.T.);
#41535=EDGE_CURVE('',#32557,#32554,#19589,.T.);
#41536=EDGE_CURVE('',#32556,#32557,#19590,.T.);
#41537=EDGE_CURVE('',#32442,#32556,#25796,.T.);
#41538=EDGE_CURVE('',#32558,#32559,#19591,.T.);
#41539=EDGE_CURVE('',#32161,#32559,#23443,.T.);
#41540=EDGE_CURVE('',#32558,#32442,#25797,.T.);
#41541=EDGE_CURVE('',#32560,#32558,#19592,.T.);
#41542=EDGE_CURVE('',#32561,#32560,#19593,.T.);
#41543=EDGE_CURVE('',#32559,#32561,#19594,.T.);
#41544=EDGE_CURVE('',#32443,#32561,#25798,.T.);
#41545=EDGE_CURVE('',#32562,#32563,#19595,.T.);
#41546=EDGE_CURVE('',#32162,#32563,#23444,.T.);
#41547=EDGE_CURVE('',#32562,#32443,#25799,.T.);
#41548=EDGE_CURVE('',#32564,#32562,#19596,.T.);
#41549=EDGE_CURVE('',#32565,#32564,#19597,.T.);
#41550=EDGE_CURVE('',#32563,#32565,#19598,.T.);
#41551=EDGE_CURVE('',#32444,#32565,#25800,.T.);
#41552=EDGE_CURVE('',#32566,#32567,#19599,.T.);
#41553=EDGE_CURVE('',#32163,#32567,#23445,.T.);
#41554=EDGE_CURVE('',#32566,#32444,#25801,.T.);
#41555=EDGE_CURVE('',#32568,#32566,#19600,.T.);
#41556=EDGE_CURVE('',#32569,#32568,#19601,.T.);
#41557=EDGE_CURVE('',#32567,#32569,#19602,.T.);
#41558=EDGE_CURVE('',#32445,#32569,#25802,.T.);
#41559=EDGE_CURVE('',#32570,#32571,#19603,.T.);
#41560=EDGE_CURVE('',#32164,#32571,#23446,.T.);
#41561=EDGE_CURVE('',#32570,#32445,#25803,.T.);
#41562=EDGE_CURVE('',#32572,#32570,#19604,.T.);
#41563=EDGE_CURVE('',#32573,#32572,#19605,.T.);
#41564=EDGE_CURVE('',#32571,#32573,#19606,.T.);
#41565=EDGE_CURVE('',#32446,#32573,#25804,.T.);
#41566=EDGE_CURVE('',#32574,#32575,#19607,.T.);
#41567=EDGE_CURVE('',#32165,#32575,#23447,.T.);
#41568=EDGE_CURVE('',#32574,#32446,#25805,.T.);
#41569=EDGE_CURVE('',#32576,#32574,#19608,.T.);
#41570=EDGE_CURVE('',#32577,#32576,#19609,.T.);
#41571=EDGE_CURVE('',#32575,#32577,#19610,.T.);
#41572=EDGE_CURVE('',#32447,#32577,#25806,.T.);
#41573=EDGE_CURVE('',#32578,#32579,#19611,.T.);
#41574=EDGE_CURVE('',#32166,#32579,#23448,.T.);
#41575=EDGE_CURVE('',#32578,#32447,#25807,.T.);
#41576=EDGE_CURVE('',#32580,#32578,#19612,.T.);
#41577=EDGE_CURVE('',#32581,#32580,#19613,.T.);
#41578=EDGE_CURVE('',#32579,#32581,#19614,.T.);
#41579=EDGE_CURVE('',#32448,#32581,#25808,.T.);
#41580=EDGE_CURVE('',#32582,#32583,#19615,.T.);
#41581=EDGE_CURVE('',#32167,#32583,#23449,.T.);
#41582=EDGE_CURVE('',#32582,#32448,#25809,.T.);
#41583=EDGE_CURVE('',#32584,#32582,#19616,.T.);
#41584=EDGE_CURVE('',#32585,#32584,#19617,.T.);
#41585=EDGE_CURVE('',#32583,#32585,#19618,.T.);
#41586=EDGE_CURVE('',#32449,#32585,#25810,.T.);
#41587=EDGE_CURVE('',#32586,#32587,#19619,.T.);
#41588=EDGE_CURVE('',#32168,#32587,#23450,.T.);
#41589=EDGE_CURVE('',#32586,#32449,#25811,.T.);
#41590=EDGE_CURVE('',#32588,#32586,#19620,.T.);
#41591=EDGE_CURVE('',#32589,#32588,#19621,.T.);
#41592=EDGE_CURVE('',#32587,#32589,#19622,.T.);
#41593=EDGE_CURVE('',#32450,#32589,#25812,.T.);
#41594=EDGE_CURVE('',#32590,#32591,#19623,.T.);
#41595=EDGE_CURVE('',#32481,#32590,#19624,.T.);
#41596=EDGE_CURVE('',#32591,#32480,#19625,.T.);
#41597=EDGE_CURVE('',#32591,#32450,#25813,.T.);
#41598=EDGE_CURVE('',#32592,#32169,#23451,.T.);
#41599=EDGE_CURVE('',#32592,#32593,#19626,.T.);
#41600=EDGE_CURVE('',#32451,#32593,#25814,.T.);
#41601=EDGE_CURVE('',#32594,#32451,#25815,.T.);
#41602=EDGE_CURVE('',#32594,#32595,#19627,.T.);
#41603=EDGE_CURVE('',#32170,#32595,#23452,.T.);
#41604=EDGE_CURVE('',#32595,#32596,#19628,.T.);
#41605=EDGE_CURVE('',#32452,#32596,#25816,.T.);
#41606=EDGE_CURVE('',#32597,#32594,#19629,.T.);
#41607=EDGE_CURVE('',#32596,#32597,#19630,.T.);
#41608=EDGE_CURVE('',#32598,#32452,#25817,.T.);
#41609=EDGE_CURVE('',#32598,#32599,#19631,.T.);
#41610=EDGE_CURVE('',#32171,#32599,#23453,.T.);
#41611=EDGE_CURVE('',#32599,#32600,#19632,.T.);
#41612=EDGE_CURVE('',#32453,#32600,#25818,.T.);
#41613=EDGE_CURVE('',#32601,#32598,#19633,.T.);
#41614=EDGE_CURVE('',#32600,#32601,#19634,.T.);
#41615=EDGE_CURVE('',#32602,#32453,#25819,.T.);
#41616=EDGE_CURVE('',#32602,#32603,#19635,.T.);
#41617=EDGE_CURVE('',#32172,#32603,#23454,.T.);
#41618=EDGE_CURVE('',#32603,#32604,#19636,.T.);
#41619=EDGE_CURVE('',#32454,#32604,#25820,.T.);
#41620=EDGE_CURVE('',#32605,#32602,#19637,.T.);
#41621=EDGE_CURVE('',#32604,#32605,#19638,.T.);
#41622=EDGE_CURVE('',#32606,#32454,#25821,.T.);
#41623=EDGE_CURVE('',#32606,#32607,#19639,.T.);
#41624=EDGE_CURVE('',#32173,#32607,#23455,.T.);
#41625=EDGE_CURVE('',#32607,#32608,#19640,.T.);
#41626=EDGE_CURVE('',#32455,#32608,#25822,.T.);
#41627=EDGE_CURVE('',#32609,#32606,#19641,.T.);
#41628=EDGE_CURVE('',#32608,#32609,#19642,.T.);
#41629=EDGE_CURVE('',#32610,#32455,#25823,.T.);
#41630=EDGE_CURVE('',#32610,#32611,#19643,.T.);
#41631=EDGE_CURVE('',#32174,#32611,#23456,.T.);
#41632=EDGE_CURVE('',#32611,#32612,#19644,.T.);
#41633=EDGE_CURVE('',#32456,#32612,#25824,.T.);
#41634=EDGE_CURVE('',#32613,#32610,#19645,.T.);
#41635=EDGE_CURVE('',#32612,#32613,#19646,.T.);
#41636=EDGE_CURVE('',#32614,#32456,#25825,.T.);
#41637=EDGE_CURVE('',#32614,#32615,#19647,.T.);
#41638=EDGE_CURVE('',#32175,#32615,#23457,.T.);
#41639=EDGE_CURVE('',#32615,#32616,#19648,.T.);
#41640=EDGE_CURVE('',#32457,#32616,#25826,.T.);
#41641=EDGE_CURVE('',#32617,#32614,#19649,.T.);
#41642=EDGE_CURVE('',#32616,#32617,#19650,.T.);
#41643=EDGE_CURVE('',#32618,#32457,#25827,.T.);
#41644=EDGE_CURVE('',#32618,#32619,#19651,.T.);
#41645=EDGE_CURVE('',#32176,#32619,#23458,.T.);
#41646=EDGE_CURVE('',#32619,#32620,#19652,.T.);
#41647=EDGE_CURVE('',#32458,#32620,#25828,.T.);
#41648=EDGE_CURVE('',#32621,#32618,#19653,.T.);
#41649=EDGE_CURVE('',#32620,#32621,#19654,.T.);
#41650=EDGE_CURVE('',#32622,#32458,#25829,.T.);
#41651=EDGE_CURVE('',#32622,#32623,#19655,.T.);
#41652=EDGE_CURVE('',#32177,#32623,#23459,.T.);
#41653=EDGE_CURVE('',#32623,#32624,#19656,.T.);
#41654=EDGE_CURVE('',#32459,#32624,#25830,.T.);
#41655=EDGE_CURVE('',#32625,#32622,#19657,.T.);
#41656=EDGE_CURVE('',#32624,#32625,#19658,.T.);
#41657=EDGE_CURVE('',#32626,#32459,#25831,.T.);
#41658=EDGE_CURVE('',#32626,#32627,#19659,.T.);
#41659=EDGE_CURVE('',#32178,#32627,#23460,.T.);
#41660=EDGE_CURVE('',#32627,#32628,#19660,.T.);
#41661=EDGE_CURVE('',#32460,#32628,#25832,.T.);
#41662=EDGE_CURVE('',#32629,#32626,#19661,.T.);
#41663=EDGE_CURVE('',#32628,#32629,#19662,.T.);
#41664=EDGE_CURVE('',#32630,#32460,#25833,.T.);
#41665=EDGE_CURVE('',#32630,#32631,#19663,.T.);
#41666=EDGE_CURVE('',#32179,#32631,#23461,.T.);
#41667=EDGE_CURVE('',#32631,#32632,#19664,.T.);
#41668=EDGE_CURVE('',#32461,#32632,#25834,.T.);
#41669=EDGE_CURVE('',#32633,#32630,#19665,.T.);
#41670=EDGE_CURVE('',#32632,#32633,#19666,.T.);
#41671=EDGE_CURVE('',#32634,#32461,#25835,.T.);
#41672=EDGE_CURVE('',#32634,#32635,#19667,.T.);
#41673=EDGE_CURVE('',#32180,#32635,#23462,.T.);
#41674=EDGE_CURVE('',#32635,#32636,#19668,.T.);
#41675=EDGE_CURVE('',#32462,#32636,#25836,.T.);
#41676=EDGE_CURVE('',#32637,#32634,#19669,.T.);
#41677=EDGE_CURVE('',#32636,#32637,#19670,.T.);
#41678=EDGE_CURVE('',#32638,#32462,#25837,.T.);
#41679=EDGE_CURVE('',#32638,#32639,#19671,.T.);
#41680=EDGE_CURVE('',#32181,#32639,#23463,.T.);
#41681=EDGE_CURVE('',#32639,#32640,#19672,.T.);
#41682=EDGE_CURVE('',#32463,#32640,#25838,.T.);
#41683=EDGE_CURVE('',#32641,#32638,#19673,.T.);
#41684=EDGE_CURVE('',#32640,#32641,#19674,.T.);
#41685=EDGE_CURVE('',#32642,#32463,#25839,.T.);
#41686=EDGE_CURVE('',#32642,#32643,#19675,.T.);
#41687=EDGE_CURVE('',#32182,#32643,#23464,.T.);
#41688=EDGE_CURVE('',#32643,#32644,#19676,.T.);
#41689=EDGE_CURVE('',#32464,#32644,#25840,.T.);
#41690=EDGE_CURVE('',#32645,#32642,#19677,.T.);
#41691=EDGE_CURVE('',#32644,#32645,#19678,.T.);
#41692=EDGE_CURVE('',#28937,#32464,#25841,.T.);
#41693=EDGE_CURVE('',#32183,#28936,#23465,.T.);
#41694=EDGE_CURVE('',#32465,#28934,#25842,.T.);
#41695=EDGE_CURVE('',#32646,#32465,#25843,.T.);
#41696=EDGE_CURVE('',#32646,#32647,#19679,.T.);
#41697=EDGE_CURVE('',#32184,#32647,#23466,.T.);
#41698=EDGE_CURVE('',#32647,#32648,#19680,.T.);
#41699=EDGE_CURVE('',#32466,#32648,#25844,.T.);
#41700=EDGE_CURVE('',#32649,#32646,#19681,.T.);
#41701=EDGE_CURVE('',#32648,#32649,#19682,.T.);
#41702=EDGE_CURVE('',#32650,#32466,#25845,.T.);
#41703=EDGE_CURVE('',#32650,#32651,#19683,.T.);
#41704=EDGE_CURVE('',#32185,#32651,#23467,.T.);
#41705=EDGE_CURVE('',#32651,#32652,#19684,.T.);
#41706=EDGE_CURVE('',#32467,#32652,#25846,.T.);
#41707=EDGE_CURVE('',#32653,#32650,#19685,.T.);
#41708=EDGE_CURVE('',#32652,#32653,#19686,.T.);
#41709=EDGE_CURVE('',#32654,#32467,#25847,.T.);
#41710=EDGE_CURVE('',#32654,#32655,#19687,.T.);
#41711=EDGE_CURVE('',#32186,#32655,#23468,.T.);
#41712=EDGE_CURVE('',#32655,#32656,#19688,.T.);
#41713=EDGE_CURVE('',#32468,#32656,#25848,.T.);
#41714=EDGE_CURVE('',#32657,#32654,#19689,.T.);
#41715=EDGE_CURVE('',#32656,#32657,#19690,.T.);
#41716=EDGE_CURVE('',#32658,#32468,#25849,.T.);
#41717=EDGE_CURVE('',#32658,#32659,#19691,.T.);
#41718=EDGE_CURVE('',#32187,#32659,#23469,.T.);
#41719=EDGE_CURVE('',#32659,#32660,#19692,.T.);
#41720=EDGE_CURVE('',#32469,#32660,#25850,.T.);
#41721=EDGE_CURVE('',#32661,#32658,#19693,.T.);
#41722=EDGE_CURVE('',#32660,#32661,#19694,.T.);
#41723=EDGE_CURVE('',#32662,#32469,#25851,.T.);
#41724=EDGE_CURVE('',#32662,#32663,#19695,.T.);
#41725=EDGE_CURVE('',#32188,#32663,#23470,.T.);
#41726=EDGE_CURVE('',#32663,#32664,#19696,.T.);
#41727=EDGE_CURVE('',#32470,#32664,#25852,.T.);
#41728=EDGE_CURVE('',#32665,#32662,#19697,.T.);
#41729=EDGE_CURVE('',#32664,#32665,#19698,.T.);
#41730=EDGE_CURVE('',#32666,#32470,#25853,.T.);
#41731=EDGE_CURVE('',#32666,#32667,#19699,.T.);
#41732=EDGE_CURVE('',#32189,#32667,#23471,.T.);
#41733=EDGE_CURVE('',#32667,#32668,#19700,.T.);
#41734=EDGE_CURVE('',#32471,#32668,#25854,.T.);
#41735=EDGE_CURVE('',#32669,#32666,#19701,.T.);
#41736=EDGE_CURVE('',#32668,#32669,#19702,.T.);
#41737=EDGE_CURVE('',#32670,#32471,#25855,.T.);
#41738=EDGE_CURVE('',#32670,#32671,#19703,.T.);
#41739=EDGE_CURVE('',#32190,#32671,#23472,.T.);
#41740=EDGE_CURVE('',#32671,#32672,#19704,.T.);
#41741=EDGE_CURVE('',#32472,#32672,#25856,.T.);
#41742=EDGE_CURVE('',#32673,#32670,#19705,.T.);
#41743=EDGE_CURVE('',#32672,#32673,#19706,.T.);
#41744=EDGE_CURVE('',#32674,#32472,#25857,.T.);
#41745=EDGE_CURVE('',#32674,#32675,#19707,.T.);
#41746=EDGE_CURVE('',#32191,#32675,#23473,.T.);
#41747=EDGE_CURVE('',#32675,#32676,#19708,.T.);
#41748=EDGE_CURVE('',#32473,#32676,#25858,.T.);
#41749=EDGE_CURVE('',#32677,#32674,#19709,.T.);
#41750=EDGE_CURVE('',#32676,#32677,#19710,.T.);
#41751=EDGE_CURVE('',#32678,#32473,#25859,.T.);
#41752=EDGE_CURVE('',#32678,#32679,#19711,.T.);
#41753=EDGE_CURVE('',#32192,#32679,#23474,.T.);
#41754=EDGE_CURVE('',#32679,#32680,#19712,.T.);
#41755=EDGE_CURVE('',#32474,#32680,#25860,.T.);
#41756=EDGE_CURVE('',#32681,#32678,#19713,.T.);
#41757=EDGE_CURVE('',#32680,#32681,#19714,.T.);
#41758=EDGE_CURVE('',#32682,#32474,#25861,.T.);
#41759=EDGE_CURVE('',#32682,#32683,#19715,.T.);
#41760=EDGE_CURVE('',#32193,#32683,#23475,.T.);
#41761=EDGE_CURVE('',#32683,#32684,#19716,.T.);
#41762=EDGE_CURVE('',#32475,#32684,#25862,.T.);
#41763=EDGE_CURVE('',#32685,#32682,#19717,.T.);
#41764=EDGE_CURVE('',#32684,#32685,#19718,.T.);
#41765=EDGE_CURVE('',#32686,#32475,#25863,.T.);
#41766=EDGE_CURVE('',#32686,#32687,#19719,.T.);
#41767=EDGE_CURVE('',#32194,#32687,#23476,.T.);
#41768=EDGE_CURVE('',#32687,#32688,#19720,.T.);
#41769=EDGE_CURVE('',#32476,#32688,#25864,.T.);
#41770=EDGE_CURVE('',#32689,#32686,#19721,.T.);
#41771=EDGE_CURVE('',#32688,#32689,#19722,.T.);
#41772=EDGE_CURVE('',#32690,#32476,#25865,.T.);
#41773=EDGE_CURVE('',#32690,#32691,#19723,.T.);
#41774=EDGE_CURVE('',#32195,#32691,#23477,.T.);
#41775=EDGE_CURVE('',#32691,#32692,#19724,.T.);
#41776=EDGE_CURVE('',#32477,#32692,#25866,.T.);
#41777=EDGE_CURVE('',#32693,#32690,#19725,.T.);
#41778=EDGE_CURVE('',#32692,#32693,#19726,.T.);
#41779=EDGE_CURVE('',#32694,#32477,#25867,.T.);
#41780=EDGE_CURVE('',#32694,#32695,#19727,.T.);
#41781=EDGE_CURVE('',#32196,#32695,#23478,.T.);
#41782=EDGE_CURVE('',#32695,#32696,#19728,.T.);
#41783=EDGE_CURVE('',#32478,#32696,#25868,.T.);
#41784=EDGE_CURVE('',#32697,#32694,#19729,.T.);
#41785=EDGE_CURVE('',#32696,#32697,#19730,.T.);
#41786=EDGE_CURVE('',#32698,#32478,#25869,.T.);
#41787=EDGE_CURVE('',#32698,#32699,#19731,.T.);
#41788=EDGE_CURVE('',#32197,#32699,#23479,.T.);
#41789=EDGE_CURVE('',#32699,#32700,#19732,.T.);
#41790=EDGE_CURVE('',#32479,#32700,#25870,.T.);
#41791=EDGE_CURVE('',#32701,#32698,#19733,.T.);
#41792=EDGE_CURVE('',#32700,#32701,#19734,.T.);
#41793=EDGE_CURVE('',#32702,#32592,#19735,.T.);
#41794=EDGE_CURVE('',#32703,#32702,#19736,.T.);
#41795=EDGE_CURVE('',#32593,#32703,#19737,.T.);
#41796=EDGE_CURVE('',#32702,#32479,#25871,.T.);
#41797=EDGE_CURVE('',#32422,#32704,#19738,.T.);
#41798=EDGE_CURVE('',#32704,#32590,#23480,.T.);
#41799=EDGE_CURVE('',#32705,#32422,#23481,.T.);
#41800=EDGE_CURVE('',#32484,#32705,#23482,.T.);
#41801=EDGE_CURVE('',#32423,#32705,#19739,.T.);
#41802=EDGE_CURVE('',#32706,#32423,#4450,.T.);
#41803=EDGE_CURVE('',#32488,#32706,#23483,.T.);
#41804=EDGE_CURVE('',#32424,#32706,#19740,.T.);
#41805=EDGE_CURVE('',#32707,#32424,#23484,.T.);
#41806=EDGE_CURVE('',#32492,#32707,#23485,.T.);
#41807=EDGE_CURVE('',#32425,#32707,#19741,.T.);
#41808=EDGE_CURVE('',#32708,#32425,#4451,.T.);
#41809=EDGE_CURVE('',#32496,#32708,#23486,.T.);
#41810=EDGE_CURVE('',#32426,#32708,#19742,.T.);
#41811=EDGE_CURVE('',#32709,#32426,#4452,.T.);
#41812=EDGE_CURVE('',#32500,#32709,#23487,.T.);
#41813=EDGE_CURVE('',#32427,#32709,#19743,.T.);
#41814=EDGE_CURVE('',#32710,#32427,#23488,.T.);
#41815=EDGE_CURVE('',#32504,#32710,#23489,.T.);
#41816=EDGE_CURVE('',#32428,#32710,#19744,.T.);
#41817=EDGE_CURVE('',#32711,#32428,#23490,.T.);
#41818=EDGE_CURVE('',#28941,#32711,#23491,.T.);
#41819=EDGE_CURVE('',#32429,#32711,#19745,.T.);
#41820=EDGE_CURVE('',#32712,#32429,#23492,.T.);
#41821=EDGE_CURVE('',#32508,#32712,#23493,.T.);
#41822=EDGE_CURVE('',#32430,#32712,#19746,.T.);
#41823=EDGE_CURVE('',#32713,#32430,#23494,.T.);
#41824=EDGE_CURVE('',#32512,#32713,#23495,.T.);
#41825=EDGE_CURVE('',#32431,#32713,#19747,.T.);
#41826=EDGE_CURVE('',#32714,#32431,#23496,.T.);
#41827=EDGE_CURVE('',#32516,#32714,#23497,.T.);
#41828=EDGE_CURVE('',#32432,#32714,#19748,.T.);
#41829=EDGE_CURVE('',#32715,#32432,#4453,.T.);
#41830=EDGE_CURVE('',#32520,#32715,#23498,.T.);
#41831=EDGE_CURVE('',#32433,#32715,#19749,.T.);
#41832=EDGE_CURVE('',#32716,#32433,#23499,.T.);
#41833=EDGE_CURVE('',#32524,#32716,#23500,.T.);
#41834=EDGE_CURVE('',#32434,#32716,#19750,.T.);
#41835=EDGE_CURVE('',#32717,#32434,#4454,.T.);
#41836=EDGE_CURVE('',#32528,#32717,#23501,.T.);
#41837=EDGE_CURVE('',#32435,#32717,#19751,.T.);
#41838=EDGE_CURVE('',#32718,#32435,#23502,.T.);
#41839=EDGE_CURVE('',#32532,#32718,#23503,.T.);
#41840=EDGE_CURVE('',#32436,#32718,#19752,.T.);
#41841=EDGE_CURVE('',#32719,#32436,#23504,.T.);
#41842=EDGE_CURVE('',#32536,#32719,#23505,.T.);
#41843=EDGE_CURVE('',#32437,#32719,#19753,.T.);
#41844=EDGE_CURVE('',#32720,#32437,#23506,.T.);
#41845=EDGE_CURVE('',#32540,#32720,#23507,.T.);
#41846=EDGE_CURVE('',#32438,#32720,#19754,.T.);
#41847=EDGE_CURVE('',#32721,#32438,#4455,.T.);
#41848=EDGE_CURVE('',#32544,#32721,#23508,.T.);
#41849=EDGE_CURVE('',#32439,#32721,#19755,.T.);
#41850=EDGE_CURVE('',#32722,#32439,#23509,.T.);
#41851=EDGE_CURVE('',#32548,#32722,#23510,.T.);
#41852=EDGE_CURVE('',#32440,#32722,#19756,.T.);
#41853=EDGE_CURVE('',#32723,#32440,#23511,.T.);
#41854=EDGE_CURVE('',#32553,#32723,#23512,.T.);
#41855=EDGE_CURVE('',#32441,#32723,#19757,.T.);
#41856=EDGE_CURVE('',#32724,#32441,#23513,.T.);
#41857=EDGE_CURVE('',#32557,#32724,#23514,.T.);
#41858=EDGE_CURVE('',#32442,#32724,#19758,.T.);
#41859=EDGE_CURVE('',#32725,#32442,#23515,.T.);
#41860=EDGE_CURVE('',#32560,#32725,#23516,.T.);
#41861=EDGE_CURVE('',#32443,#32725,#19759,.T.);
#41862=EDGE_CURVE('',#32726,#32443,#23517,.T.);
#41863=EDGE_CURVE('',#32564,#32726,#23518,.T.);
#41864=EDGE_CURVE('',#32444,#32726,#19760,.T.);
#41865=EDGE_CURVE('',#32727,#32444,#23519,.T.);
#41866=EDGE_CURVE('',#32568,#32727,#23520,.T.);
#41867=EDGE_CURVE('',#32445,#32727,#19761,.T.);
#41868=EDGE_CURVE('',#32728,#32445,#23521,.T.);
#41869=EDGE_CURVE('',#32572,#32728,#23522,.T.);
#41870=EDGE_CURVE('',#32446,#32728,#19762,.T.);
#41871=EDGE_CURVE('',#32729,#32446,#23523,.T.);
#41872=EDGE_CURVE('',#32576,#32729,#23524,.T.);
#41873=EDGE_CURVE('',#32447,#32729,#19763,.T.);
#41874=EDGE_CURVE('',#32730,#32447,#23525,.T.);
#41875=EDGE_CURVE('',#32580,#32730,#23526,.T.);
#41876=EDGE_CURVE('',#32448,#32730,#19764,.T.);
#41877=EDGE_CURVE('',#32731,#32448,#23527,.T.);
#41878=EDGE_CURVE('',#32584,#32731,#23528,.T.);
#41879=EDGE_CURVE('',#32449,#32731,#19765,.T.);
#41880=EDGE_CURVE('',#32732,#32449,#23529,.T.);
#41881=EDGE_CURVE('',#32588,#32732,#23530,.T.);
#41882=EDGE_CURVE('',#32450,#32732,#19766,.T.);
#41883=EDGE_CURVE('',#32704,#32450,#23531,.T.);
#41884=EDGE_CURVE('',#32733,#32703,#23532,.T.);
#41885=EDGE_CURVE('',#32451,#32733,#19767,.T.);
#41886=EDGE_CURVE('',#32734,#32451,#19768,.T.);
#41887=EDGE_CURVE('',#32597,#32734,#23533,.T.);
#41888=EDGE_CURVE('',#32452,#32734,#19769,.T.);
#41889=EDGE_CURVE('',#32735,#32452,#19770,.T.);
#41890=EDGE_CURVE('',#32601,#32735,#23534,.T.);
#41891=EDGE_CURVE('',#32453,#32735,#19771,.T.);
#41892=EDGE_CURVE('',#32736,#32453,#19772,.T.);
#41893=EDGE_CURVE('',#32605,#32736,#23535,.T.);
#41894=EDGE_CURVE('',#32454,#32736,#19773,.T.);
#41895=EDGE_CURVE('',#32737,#32454,#19774,.T.);
#41896=EDGE_CURVE('',#32609,#32737,#23536,.T.);
#41897=EDGE_CURVE('',#32455,#32737,#19775,.T.);
#41898=EDGE_CURVE('',#32738,#32455,#19776,.T.);
#41899=EDGE_CURVE('',#32613,#32738,#23537,.T.);
#41900=EDGE_CURVE('',#32456,#32738,#19777,.T.);
#41901=EDGE_CURVE('',#32739,#32456,#19778,.T.);
#41902=EDGE_CURVE('',#32617,#32739,#23538,.T.);
#41903=EDGE_CURVE('',#32457,#32739,#19779,.T.);
#41904=EDGE_CURVE('',#32740,#32457,#19780,.T.);
#41905=EDGE_CURVE('',#32621,#32740,#23539,.T.);
#41906=EDGE_CURVE('',#32458,#32740,#19781,.T.);
#41907=EDGE_CURVE('',#32741,#32458,#19782,.T.);
#41908=EDGE_CURVE('',#32625,#32741,#23540,.T.);
#41909=EDGE_CURVE('',#32459,#32741,#19783,.T.);
#41910=EDGE_CURVE('',#32742,#32459,#19784,.T.);
#41911=EDGE_CURVE('',#32629,#32742,#23541,.T.);
#41912=EDGE_CURVE('',#32460,#32742,#19785,.T.);
#41913=EDGE_CURVE('',#32743,#32460,#19786,.T.);
#41914=EDGE_CURVE('',#32633,#32743,#23542,.T.);
#41915=EDGE_CURVE('',#32461,#32743,#19787,.T.);
#41916=EDGE_CURVE('',#32744,#32461,#19788,.T.);
#41917=EDGE_CURVE('',#32637,#32744,#23543,.T.);
#41918=EDGE_CURVE('',#32462,#32744,#19789,.T.);
#41919=EDGE_CURVE('',#32745,#32462,#19790,.T.);
#41920=EDGE_CURVE('',#32641,#32745,#23544,.T.);
#41921=EDGE_CURVE('',#32463,#32745,#19791,.T.);
#41922=EDGE_CURVE('',#32746,#32463,#19792,.T.);
#41923=EDGE_CURVE('',#32645,#32746,#23545,.T.);
#41924=EDGE_CURVE('',#32464,#32746,#19793,.T.);
#41925=EDGE_CURVE('',#32747,#32464,#19794,.T.);
#41926=EDGE_CURVE('',#28935,#32747,#23546,.T.);
#41927=EDGE_CURVE('',#32465,#32747,#19795,.T.);
#41928=EDGE_CURVE('',#32748,#32465,#19796,.T.);
#41929=EDGE_CURVE('',#32649,#32748,#23547,.T.);
#41930=EDGE_CURVE('',#32466,#32748,#19797,.T.);
#41931=EDGE_CURVE('',#32749,#32466,#19798,.T.);
#41932=EDGE_CURVE('',#32653,#32749,#23548,.T.);
#41933=EDGE_CURVE('',#32467,#32749,#19799,.T.);
#41934=EDGE_CURVE('',#32750,#32467,#19800,.T.);
#41935=EDGE_CURVE('',#32657,#32750,#23549,.T.);
#41936=EDGE_CURVE('',#32468,#32750,#19801,.T.);
#41937=EDGE_CURVE('',#32751,#32468,#19802,.T.);
#41938=EDGE_CURVE('',#32661,#32751,#23550,.T.);
#41939=EDGE_CURVE('',#32469,#32751,#19803,.T.);
#41940=EDGE_CURVE('',#32752,#32469,#19804,.T.);
#41941=EDGE_CURVE('',#32665,#32752,#23551,.T.);
#41942=EDGE_CURVE('',#32470,#32752,#19805,.T.);
#41943=EDGE_CURVE('',#32753,#32470,#19806,.T.);
#41944=EDGE_CURVE('',#32669,#32753,#23552,.T.);
#41945=EDGE_CURVE('',#32471,#32753,#19807,.T.);
#41946=EDGE_CURVE('',#32754,#32471,#19808,.T.);
#41947=EDGE_CURVE('',#32673,#32754,#23553,.T.);
#41948=EDGE_CURVE('',#32472,#32754,#19809,.T.);
#41949=EDGE_CURVE('',#32755,#32472,#19810,.T.);
#41950=EDGE_CURVE('',#32677,#32755,#23554,.T.);
#41951=EDGE_CURVE('',#32473,#32755,#19811,.T.);
#41952=EDGE_CURVE('',#32756,#32473,#19812,.T.);
#41953=EDGE_CURVE('',#32681,#32756,#23555,.T.);
#41954=EDGE_CURVE('',#32474,#32756,#19813,.T.);
#41955=EDGE_CURVE('',#32757,#32474,#19814,.T.);
#41956=EDGE_CURVE('',#32685,#32757,#23556,.T.);
#41957=EDGE_CURVE('',#32475,#32757,#19815,.T.);
#41958=EDGE_CURVE('',#32758,#32475,#19816,.T.);
#41959=EDGE_CURVE('',#32689,#32758,#23557,.T.);
#41960=EDGE_CURVE('',#32476,#32758,#19817,.T.);
#41961=EDGE_CURVE('',#32759,#32476,#19818,.T.);
#41962=EDGE_CURVE('',#32693,#32759,#23558,.T.);
#41963=EDGE_CURVE('',#32477,#32759,#19819,.T.);
#41964=EDGE_CURVE('',#32760,#32477,#19820,.T.);
#41965=EDGE_CURVE('',#32697,#32760,#23559,.T.);
#41966=EDGE_CURVE('',#32478,#32760,#19821,.T.);
#41967=EDGE_CURVE('',#32761,#32478,#19822,.T.);
#41968=EDGE_CURVE('',#32701,#32761,#23560,.T.);
#41969=EDGE_CURVE('',#32479,#32761,#19823,.T.);
#41970=EDGE_CURVE('',#32733,#32479,#19824,.T.);
#41971=EDGE_CURVE('',#32762,#32763,#19825,.T.);
#41972=EDGE_CURVE('',#32422,#32763,#23561,.T.);
#41973=EDGE_CURVE('',#32762,#32704,#25872,.T.);
#41974=EDGE_CURVE('',#32764,#32762,#19826,.T.);
#41975=EDGE_CURVE('',#32765,#32764,#19827,.T.);
#41976=EDGE_CURVE('',#32763,#32765,#23562,.T.);
#41977=EDGE_CURVE('',#32705,#32765,#25873,.T.);
#41978=EDGE_CURVE('',#32766,#32767,#19828,.T.);
#41979=EDGE_CURVE('',#32423,#32767,#23563,.T.);
#41980=EDGE_CURVE('',#32766,#32705,#25874,.T.);
#41981=EDGE_CURVE('',#32768,#32766,#19829,.T.);
#41982=EDGE_CURVE('',#32769,#32768,#19830,.T.);
#41983=EDGE_CURVE('',#32767,#32769,#23564,.T.);
#41984=EDGE_CURVE('',#32706,#32769,#25875,.T.);
#41985=EDGE_CURVE('',#32770,#32771,#19831,.T.);
#41986=EDGE_CURVE('',#32424,#32771,#23565,.T.);
#41987=EDGE_CURVE('',#32770,#32706,#25876,.T.);
#41988=EDGE_CURVE('',#32772,#32770,#19832,.T.);
#41989=EDGE_CURVE('',#32773,#32772,#19833,.T.);
#41990=EDGE_CURVE('',#32771,#32773,#23566,.T.);
#41991=EDGE_CURVE('',#32707,#32773,#25877,.T.);
#41992=EDGE_CURVE('',#32774,#32775,#19834,.T.);
#41993=EDGE_CURVE('',#32425,#32775,#23567,.T.);
#41994=EDGE_CURVE('',#32774,#32707,#25878,.T.);
#41995=EDGE_CURVE('',#32776,#32774,#19835,.T.);
#41996=EDGE_CURVE('',#32777,#32776,#19836,.T.);
#41997=EDGE_CURVE('',#32775,#32777,#23568,.T.);
#41998=EDGE_CURVE('',#32708,#32777,#25879,.T.);
#41999=EDGE_CURVE('',#32778,#32779,#19837,.T.);
#42000=EDGE_CURVE('',#32426,#32779,#23569,.T.);
#42001=EDGE_CURVE('',#32778,#32708,#25880,.T.);
#42002=EDGE_CURVE('',#32780,#32778,#19838,.T.);
#42003=EDGE_CURVE('',#32781,#32780,#19839,.T.);
#42004=EDGE_CURVE('',#32779,#32781,#23570,.T.);
#42005=EDGE_CURVE('',#32709,#32781,#25881,.T.);
#42006=EDGE_CURVE('',#32782,#32783,#19840,.T.);
#42007=EDGE_CURVE('',#32427,#32783,#23571,.T.);
#42008=EDGE_CURVE('',#32782,#32709,#25882,.T.);
#42009=EDGE_CURVE('',#32784,#32782,#19841,.T.);
#42010=EDGE_CURVE('',#32785,#32784,#19842,.T.);
#42011=EDGE_CURVE('',#32783,#32785,#23572,.T.);
#42012=EDGE_CURVE('',#32710,#32785,#25883,.T.);
#42013=EDGE_CURVE('',#32786,#32787,#19843,.T.);
#42014=EDGE_CURVE('',#32428,#32787,#23573,.T.);
#42015=EDGE_CURVE('',#32786,#32710,#25884,.T.);
#42016=EDGE_CURVE('',#32788,#32786,#19844,.T.);
#42017=EDGE_CURVE('',#32789,#32788,#19845,.T.);
#42018=EDGE_CURVE('',#32787,#32789,#23574,.T.);
#42019=EDGE_CURVE('',#32711,#32789,#25885,.T.);
#42020=EDGE_CURVE('',#32790,#32791,#19846,.T.);
#42021=EDGE_CURVE('',#32429,#32791,#23575,.T.);
#42022=EDGE_CURVE('',#32790,#32711,#25886,.T.);
#42023=EDGE_CURVE('',#32792,#32790,#19847,.T.);
#42024=EDGE_CURVE('',#32793,#32792,#19848,.T.);
#42025=EDGE_CURVE('',#32791,#32793,#23576,.T.);
#42026=EDGE_CURVE('',#32712,#32793,#25887,.T.);
#42027=EDGE_CURVE('',#32794,#32795,#19849,.T.);
#42028=EDGE_CURVE('',#32430,#32795,#23577,.T.);
#42029=EDGE_CURVE('',#32794,#32712,#25888,.T.);
#42030=EDGE_CURVE('',#32796,#32794,#19850,.T.);
#42031=EDGE_CURVE('',#32797,#32796,#19851,.T.);
#42032=EDGE_CURVE('',#32795,#32797,#23578,.T.);
#42033=EDGE_CURVE('',#32713,#32797,#25889,.T.);
#42034=EDGE_CURVE('',#32798,#32799,#19852,.T.);
#42035=EDGE_CURVE('',#32431,#32799,#23579,.T.);
#42036=EDGE_CURVE('',#32798,#32713,#25890,.T.);
#42037=EDGE_CURVE('',#32800,#32798,#19853,.T.);
#42038=EDGE_CURVE('',#32801,#32800,#19854,.T.);
#42039=EDGE_CURVE('',#32799,#32801,#23580,.T.);
#42040=EDGE_CURVE('',#32714,#32801,#25891,.T.);
#42041=EDGE_CURVE('',#32802,#32803,#19855,.T.);
#42042=EDGE_CURVE('',#32432,#32803,#23581,.T.);
#42043=EDGE_CURVE('',#32802,#32714,#25892,.T.);
#42044=EDGE_CURVE('',#32804,#32802,#19856,.T.);
#42045=EDGE_CURVE('',#32805,#32804,#19857,.T.);
#42046=EDGE_CURVE('',#32803,#32805,#23582,.T.);
#42047=EDGE_CURVE('',#32715,#32805,#25893,.T.);
#42048=EDGE_CURVE('',#32806,#32807,#19858,.T.);
#42049=EDGE_CURVE('',#32433,#32807,#23583,.T.);
#42050=EDGE_CURVE('',#32806,#32715,#25894,.T.);
#42051=EDGE_CURVE('',#32808,#32806,#19859,.T.);
#42052=EDGE_CURVE('',#32809,#32808,#19860,.T.);
#42053=EDGE_CURVE('',#32807,#32809,#23584,.T.);
#42054=EDGE_CURVE('',#32716,#32809,#25895,.T.);
#42055=EDGE_CURVE('',#32810,#32811,#19861,.T.);
#42056=EDGE_CURVE('',#32434,#32811,#23585,.T.);
#42057=EDGE_CURVE('',#32810,#32716,#25896,.T.);
#42058=EDGE_CURVE('',#32812,#32810,#19862,.T.);
#42059=EDGE_CURVE('',#32813,#32812,#19863,.T.);
#42060=EDGE_CURVE('',#32811,#32813,#23586,.T.);
#42061=EDGE_CURVE('',#32717,#32813,#25897,.T.);
#42062=EDGE_CURVE('',#32814,#32815,#19864,.T.);
#42063=EDGE_CURVE('',#32435,#32815,#23587,.T.);
#42064=EDGE_CURVE('',#32814,#32717,#25898,.T.);
#42065=EDGE_CURVE('',#32816,#32814,#19865,.T.);
#42066=EDGE_CURVE('',#32817,#32816,#19866,.T.);
#42067=EDGE_CURVE('',#32815,#32817,#23588,.T.);
#42068=EDGE_CURVE('',#32718,#32817,#25899,.T.);
#42069=EDGE_CURVE('',#32436,#28931,#23589,.T.);
#42070=EDGE_CURVE('',#28930,#32718,#25900,.T.);
#42071=EDGE_CURVE('',#32719,#28933,#25901,.T.);
#42072=EDGE_CURVE('',#32818,#32819,#19867,.T.);
#42073=EDGE_CURVE('',#32437,#32819,#23590,.T.);
#42074=EDGE_CURVE('',#32818,#32719,#25902,.T.);
#42075=EDGE_CURVE('',#32820,#32818,#19868,.T.);
#42076=EDGE_CURVE('',#32821,#32820,#19869,.T.);
#42077=EDGE_CURVE('',#32819,#32821,#23591,.T.);
#42078=EDGE_CURVE('',#32720,#32821,#25903,.T.);
#42079=EDGE_CURVE('',#32822,#32823,#19870,.T.);
#42080=EDGE_CURVE('',#32438,#32823,#23592,.T.);
#42081=EDGE_CURVE('',#32822,#32720,#25904,.T.);
#42082=EDGE_CURVE('',#32824,#32822,#19871,.T.);
#42083=EDGE_CURVE('',#32825,#32824,#19872,.T.);
#42084=EDGE_CURVE('',#32823,#32825,#23593,.T.);
#42085=EDGE_CURVE('',#32721,#32825,#25905,.T.);
#42086=EDGE_CURVE('',#32826,#32827,#19873,.T.);
#42087=EDGE_CURVE('',#32439,#32827,#23594,.T.);
#42088=EDGE_CURVE('',#32826,#32721,#25906,.T.);
#42089=EDGE_CURVE('',#32828,#32826,#19874,.T.);
#42090=EDGE_CURVE('',#32829,#32828,#19875,.T.);
#42091=EDGE_CURVE('',#32827,#32829,#23595,.T.);
#42092=EDGE_CURVE('',#32722,#32829,#25907,.T.);
#42093=EDGE_CURVE('',#32830,#32831,#19876,.T.);
#42094=EDGE_CURVE('',#32440,#32831,#23596,.T.);
#42095=EDGE_CURVE('',#32830,#32722,#25908,.T.);
#42096=EDGE_CURVE('',#32831,#32832,#23597,.T.);
#42097=EDGE_CURVE('',#32723,#32832,#25909,.T.);
#42098=EDGE_CURVE('',#32833,#32830,#19877,.T.);
#42099=EDGE_CURVE('',#32832,#32833,#19878,.T.);
#42100=EDGE_CURVE('',#32834,#32723,#25910,.T.);
#42101=EDGE_CURVE('',#32834,#32835,#19879,.T.);
#42102=EDGE_CURVE('',#32441,#32835,#23598,.T.);
#42103=EDGE_CURVE('',#32835,#32836,#23599,.T.);
#42104=EDGE_CURVE('',#32837,#32834,#19880,.T.);
#42105=EDGE_CURVE('',#32836,#32837,#19881,.T.);
#42106=EDGE_CURVE('',#32724,#32836,#25911,.T.);
#42107=EDGE_CURVE('',#32838,#32839,#19882,.T.);
#42108=EDGE_CURVE('',#32442,#32839,#23600,.T.);
#42109=EDGE_CURVE('',#32838,#32724,#25912,.T.);
#42110=EDGE_CURVE('',#32840,#32838,#19883,.T.);
#42111=EDGE_CURVE('',#32841,#32840,#19884,.T.);
#42112=EDGE_CURVE('',#32839,#32841,#23601,.T.);
#42113=EDGE_CURVE('',#32725,#32841,#25913,.T.);
#42114=EDGE_CURVE('',#32842,#32843,#19885,.T.);
#42115=EDGE_CURVE('',#32443,#32843,#23602,.T.);
#42116=EDGE_CURVE('',#32842,#32725,#25914,.T.);
#42117=EDGE_CURVE('',#32844,#32842,#19886,.T.);
#42118=EDGE_CURVE('',#32845,#32844,#19887,.T.);
#42119=EDGE_CURVE('',#32843,#32845,#23603,.T.);
#42120=EDGE_CURVE('',#32726,#32845,#25915,.T.);
#42121=EDGE_CURVE('',#32846,#32847,#19888,.T.);
#42122=EDGE_CURVE('',#32444,#32847,#23604,.T.);
#42123=EDGE_CURVE('',#32846,#32726,#25916,.T.);
#42124=EDGE_CURVE('',#32848,#32846,#19889,.T.);
#42125=EDGE_CURVE('',#32849,#32848,#19890,.T.);
#42126=EDGE_CURVE('',#32847,#32849,#23605,.T.);
#42127=EDGE_CURVE('',#32727,#32849,#25917,.T.);
#42128=EDGE_CURVE('',#32850,#32851,#19891,.T.);
#42129=EDGE_CURVE('',#32445,#32851,#23606,.T.);
#42130=EDGE_CURVE('',#32850,#32727,#25918,.T.);
#42131=EDGE_CURVE('',#32852,#32850,#19892,.T.);
#42132=EDGE_CURVE('',#32853,#32852,#19893,.T.);
#42133=EDGE_CURVE('',#32851,#32853,#23607,.T.);
#42134=EDGE_CURVE('',#32728,#32853,#25919,.T.);
#42135=EDGE_CURVE('',#32854,#32855,#19894,.T.);
#42136=EDGE_CURVE('',#32446,#32855,#23608,.T.);
#42137=EDGE_CURVE('',#32854,#32728,#25920,.T.);
#42138=EDGE_CURVE('',#32856,#32854,#19895,.T.);
#42139=EDGE_CURVE('',#32857,#32856,#19896,.T.);
#42140=EDGE_CURVE('',#32855,#32857,#23609,.T.);
#42141=EDGE_CURVE('',#32729,#32857,#25921,.T.);
#42142=EDGE_CURVE('',#32858,#32859,#19897,.T.);
#42143=EDGE_CURVE('',#32447,#32859,#23610,.T.);
#42144=EDGE_CURVE('',#32858,#32729,#25922,.T.);
#42145=EDGE_CURVE('',#32860,#32858,#19898,.T.);
#42146=EDGE_CURVE('',#32861,#32860,#19899,.T.);
#42147=EDGE_CURVE('',#32859,#32861,#23611,.T.);
#42148=EDGE_CURVE('',#32730,#32861,#25923,.T.);
#42149=EDGE_CURVE('',#32862,#32863,#19900,.T.);
#42150=EDGE_CURVE('',#32448,#32863,#23612,.T.);
#42151=EDGE_CURVE('',#32862,#32730,#25924,.T.);
#42152=EDGE_CURVE('',#32864,#32862,#19901,.T.);
#42153=EDGE_CURVE('',#32865,#32864,#19902,.T.);
#42154=EDGE_CURVE('',#32863,#32865,#23613,.T.);
#42155=EDGE_CURVE('',#32731,#32865,#25925,.T.);
#42156=EDGE_CURVE('',#32866,#32867,#19903,.T.);
#42157=EDGE_CURVE('',#32449,#32867,#23614,.T.);
#42158=EDGE_CURVE('',#32866,#32731,#25926,.T.);
#42159=EDGE_CURVE('',#32868,#32866,#19904,.T.);
#42160=EDGE_CURVE('',#32869,#32868,#19905,.T.);
#42161=EDGE_CURVE('',#32867,#32869,#23615,.T.);
#42162=EDGE_CURVE('',#32732,#32869,#25927,.T.);
#42163=EDGE_CURVE('',#32870,#32871,#19906,.T.);
#42164=EDGE_CURVE('',#32450,#32871,#23616,.T.);
#42165=EDGE_CURVE('',#32870,#32732,#25928,.T.);
#42166=EDGE_CURVE('',#32872,#32870,#19907,.T.);
#42167=EDGE_CURVE('',#32873,#32872,#19908,.T.);
#42168=EDGE_CURVE('',#32871,#32873,#23617,.T.);
#42169=EDGE_CURVE('',#32704,#32873,#25929,.T.);
#42170=EDGE_CURVE('',#32874,#32733,#25930,.T.);
#42171=EDGE_CURVE('',#32874,#32875,#19909,.T.);
#42172=EDGE_CURVE('',#32451,#32875,#23618,.T.);
#42173=EDGE_CURVE('',#32876,#32877,#19910,.T.);
#42174=EDGE_CURVE('',#32876,#32878,#19911,.T.);
#42175=EDGE_CURVE('',#32877,#32878,#19912,.T.);
#42176=EDGE_CURVE('',#32875,#32879,#19913,.T.);
#42177=EDGE_CURVE('',#32734,#32879,#25931,.T.);
#42178=EDGE_CURVE('',#32879,#32876,#19914,.T.);
#42179=EDGE_CURVE('',#32878,#32874,#19915,.T.);
#42180=EDGE_CURVE('',#32880,#32734,#25932,.T.);
#42181=EDGE_CURVE('',#32880,#32881,#19916,.T.);
#42182=EDGE_CURVE('',#32452,#32881,#23619,.T.);
#42183=EDGE_CURVE('',#32882,#32883,#19917,.T.);
#42184=EDGE_CURVE('',#32882,#32884,#19918,.T.);
#42185=EDGE_CURVE('',#32883,#32884,#19919,.T.);
#42186=EDGE_CURVE('',#32881,#32885,#19920,.T.);
#42187=EDGE_CURVE('',#32735,#32885,#25933,.T.);
#42188=EDGE_CURVE('',#32885,#32882,#19921,.T.);
#42189=EDGE_CURVE('',#32884,#32880,#19922,.T.);
#42190=EDGE_CURVE('',#32886,#32735,#25934,.T.);
#42191=EDGE_CURVE('',#32886,#32887,#19923,.T.);
#42192=EDGE_CURVE('',#32453,#32887,#23620,.T.);
#42193=EDGE_CURVE('',#32888,#32889,#19924,.T.);
#42194=EDGE_CURVE('',#32888,#32890,#19925,.T.);
#42195=EDGE_CURVE('',#32889,#32890,#19926,.T.);
#42196=EDGE_CURVE('',#32887,#32891,#19927,.T.);
#42197=EDGE_CURVE('',#32736,#32891,#25935,.T.);
#42198=EDGE_CURVE('',#32891,#32888,#19928,.T.);
#42199=EDGE_CURVE('',#32890,#32886,#19929,.T.);
#42200=EDGE_CURVE('',#32892,#32736,#25936,.T.);
#42201=EDGE_CURVE('',#32892,#32893,#19930,.T.);
#42202=EDGE_CURVE('',#32454,#32893,#23621,.T.);
#42203=EDGE_CURVE('',#32894,#32895,#19931,.T.);
#42204=EDGE_CURVE('',#32894,#32896,#19932,.T.);
#42205=EDGE_CURVE('',#32895,#32896,#19933,.T.);
#42206=EDGE_CURVE('',#32893,#32897,#19934,.T.);
#42207=EDGE_CURVE('',#32737,#32897,#25937,.T.);
#42208=EDGE_CURVE('',#32897,#32894,#19935,.T.);
#42209=EDGE_CURVE('',#32896,#32892,#19936,.T.);
#42210=EDGE_CURVE('',#32898,#32737,#25938,.T.);
#42211=EDGE_CURVE('',#32898,#32899,#19937,.T.);
#42212=EDGE_CURVE('',#32455,#32899,#23622,.T.);
#42213=EDGE_CURVE('',#32900,#32901,#19938,.T.);
#42214=EDGE_CURVE('',#32900,#32902,#19939,.T.);
#42215=EDGE_CURVE('',#32901,#32902,#19940,.T.);
#42216=EDGE_CURVE('',#32899,#32903,#19941,.T.);
#42217=EDGE_CURVE('',#32738,#32903,#25939,.T.);
#42218=EDGE_CURVE('',#32903,#32900,#19942,.T.);
#42219=EDGE_CURVE('',#32902,#32898,#19943,.T.);
#42220=EDGE_CURVE('',#32904,#32738,#25940,.T.);
#42221=EDGE_CURVE('',#32904,#32905,#19944,.T.);
#42222=EDGE_CURVE('',#32456,#32905,#23623,.T.);
#42223=EDGE_CURVE('',#32906,#32907,#19945,.T.);
#42224=EDGE_CURVE('',#32906,#32908,#19946,.T.);
#42225=EDGE_CURVE('',#32907,#32908,#19947,.T.);
#42226=EDGE_CURVE('',#32905,#32909,#19948,.T.);
#42227=EDGE_CURVE('',#32739,#32909,#25941,.T.);
#42228=EDGE_CURVE('',#32909,#32906,#19949,.T.);
#42229=EDGE_CURVE('',#32908,#32904,#19950,.T.);
#42230=EDGE_CURVE('',#32910,#32739,#25942,.T.);
#42231=EDGE_CURVE('',#32910,#32911,#19951,.T.);
#42232=EDGE_CURVE('',#32457,#32911,#23624,.T.);
#42233=EDGE_CURVE('',#32912,#32913,#19952,.T.);
#42234=EDGE_CURVE('',#32912,#32914,#19953,.T.);
#42235=EDGE_CURVE('',#32913,#32914,#19954,.T.);
#42236=EDGE_CURVE('',#32911,#32915,#19955,.T.);
#42237=EDGE_CURVE('',#32740,#32915,#25943,.T.);
#42238=EDGE_CURVE('',#32915,#32912,#19956,.T.);
#42239=EDGE_CURVE('',#32914,#32910,#19957,.T.);
#42240=EDGE_CURVE('',#32916,#32740,#25944,.T.);
#42241=EDGE_CURVE('',#32916,#32917,#19958,.T.);
#42242=EDGE_CURVE('',#32458,#32917,#23625,.T.);
#42243=EDGE_CURVE('',#32918,#32919,#19959,.T.);
#42244=EDGE_CURVE('',#32918,#32920,#19960,.T.);
#42245=EDGE_CURVE('',#32919,#32920,#19961,.T.);
#42246=EDGE_CURVE('',#32917,#32921,#19962,.T.);
#42247=EDGE_CURVE('',#32741,#32921,#25945,.T.);
#42248=EDGE_CURVE('',#32921,#32918,#19963,.T.);
#42249=EDGE_CURVE('',#32920,#32916,#19964,.T.);
#42250=EDGE_CURVE('',#32922,#32741,#25946,.T.);
#42251=EDGE_CURVE('',#32922,#32923,#19965,.T.);
#42252=EDGE_CURVE('',#32459,#32923,#23626,.T.);
#42253=EDGE_CURVE('',#32924,#32925,#19966,.T.);
#42254=EDGE_CURVE('',#32924,#32926,#19967,.T.);
#42255=EDGE_CURVE('',#32925,#32926,#19968,.T.);
#42256=EDGE_CURVE('',#32923,#32927,#19969,.T.);
#42257=EDGE_CURVE('',#32742,#32927,#25947,.T.);
#42258=EDGE_CURVE('',#32927,#32924,#19970,.T.);
#42259=EDGE_CURVE('',#32926,#32922,#19971,.T.);
#42260=EDGE_CURVE('',#32928,#32742,#25948,.T.);
#42261=EDGE_CURVE('',#32928,#32929,#19972,.T.);
#42262=EDGE_CURVE('',#32460,#32929,#23627,.T.);
#42263=EDGE_CURVE('',#32930,#32931,#19973,.T.);
#42264=EDGE_CURVE('',#32930,#32932,#19974,.T.);
#42265=EDGE_CURVE('',#32931,#32932,#19975,.T.);
#42266=EDGE_CURVE('',#32929,#32933,#19976,.T.);
#42267=EDGE_CURVE('',#32743,#32933,#25949,.T.);
#42268=EDGE_CURVE('',#32933,#32930,#19977,.T.);
#42269=EDGE_CURVE('',#32932,#32928,#19978,.T.);
#42270=EDGE_CURVE('',#32934,#32743,#25950,.T.);
#42271=EDGE_CURVE('',#32934,#32935,#19979,.T.);
#42272=EDGE_CURVE('',#32461,#32935,#23628,.T.);
#42273=EDGE_CURVE('',#32936,#32937,#19980,.T.);
#42274=EDGE_CURVE('',#32936,#32938,#19981,.T.);
#42275=EDGE_CURVE('',#32937,#32938,#19982,.T.);
#42276=EDGE_CURVE('',#32935,#32939,#19983,.T.);
#42277=EDGE_CURVE('',#32744,#32939,#25951,.T.);
#42278=EDGE_CURVE('',#32939,#32936,#19984,.T.);
#42279=EDGE_CURVE('',#32938,#32934,#19985,.T.);
#42280=EDGE_CURVE('',#32940,#32744,#25952,.T.);
#42281=EDGE_CURVE('',#32940,#32941,#19986,.T.);
#42282=EDGE_CURVE('',#32462,#32941,#23629,.T.);
#42283=EDGE_CURVE('',#32942,#32943,#19987,.T.);
#42284=EDGE_CURVE('',#32942,#32944,#19988,.T.);
#42285=EDGE_CURVE('',#32943,#32944,#19989,.T.);
#42286=EDGE_CURVE('',#32941,#32945,#19990,.T.);
#42287=EDGE_CURVE('',#32745,#32945,#25953,.T.);
#42288=EDGE_CURVE('',#32945,#32942,#19991,.T.);
#42289=EDGE_CURVE('',#32944,#32940,#19992,.T.);
#42290=EDGE_CURVE('',#32946,#32745,#25954,.T.);
#42291=EDGE_CURVE('',#32946,#32947,#19993,.T.);
#42292=EDGE_CURVE('',#32463,#32947,#23630,.T.);
#42293=EDGE_CURVE('',#32948,#32949,#19994,.T.);
#42294=EDGE_CURVE('',#32948,#32950,#19995,.T.);
#42295=EDGE_CURVE('',#32949,#32950,#19996,.T.);
#42296=EDGE_CURVE('',#32947,#32951,#19997,.T.);
#42297=EDGE_CURVE('',#32746,#32951,#25955,.T.);
#42298=EDGE_CURVE('',#32951,#32948,#19998,.T.);
#42299=EDGE_CURVE('',#32950,#32946,#19999,.T.);
#42300=EDGE_CURVE('',#32952,#32746,#25956,.T.);
#42301=EDGE_CURVE('',#32952,#32953,#20000,.T.);
#42302=EDGE_CURVE('',#32464,#32953,#23631,.T.);
#42303=EDGE_CURVE('',#32954,#32955,#20001,.T.);
#42304=EDGE_CURVE('',#32954,#32956,#20002,.T.);
#42305=EDGE_CURVE('',#32955,#32956,#20003,.T.);
#42306=EDGE_CURVE('',#32953,#32957,#20004,.T.);
#42307=EDGE_CURVE('',#32747,#32957,#25957,.T.);
#42308=EDGE_CURVE('',#32957,#32954,#20005,.T.);
#42309=EDGE_CURVE('',#32956,#32952,#20006,.T.);
#42310=EDGE_CURVE('',#32958,#32747,#25958,.T.);
#42311=EDGE_CURVE('',#32958,#32959,#20007,.T.);
#42312=EDGE_CURVE('',#32465,#32959,#23632,.T.);
#42313=EDGE_CURVE('',#32960,#32961,#20008,.T.);
#42314=EDGE_CURVE('',#32960,#32962,#20009,.T.);
#42315=EDGE_CURVE('',#32961,#32962,#20010,.T.);
#42316=EDGE_CURVE('',#32959,#32963,#20011,.T.);
#42317=EDGE_CURVE('',#32748,#32963,#25959,.T.);
#42318=EDGE_CURVE('',#32963,#32960,#20012,.T.);
#42319=EDGE_CURVE('',#32962,#32958,#20013,.T.);
#42320=EDGE_CURVE('',#32964,#32748,#25960,.T.);
#42321=EDGE_CURVE('',#32964,#32965,#20014,.T.);
#42322=EDGE_CURVE('',#32466,#32965,#23633,.T.);
#42323=EDGE_CURVE('',#32966,#32967,#20015,.T.);
#42324=EDGE_CURVE('',#32966,#32968,#20016,.T.);
#42325=EDGE_CURVE('',#32967,#32968,#20017,.T.);
#42326=EDGE_CURVE('',#32965,#32969,#20018,.T.);
#42327=EDGE_CURVE('',#32749,#32969,#25961,.T.);
#42328=EDGE_CURVE('',#32969,#32966,#20019,.T.);
#42329=EDGE_CURVE('',#32968,#32964,#20020,.T.);
#42330=EDGE_CURVE('',#32970,#32749,#25962,.T.);
#42331=EDGE_CURVE('',#32970,#32971,#20021,.T.);
#42332=EDGE_CURVE('',#32467,#32971,#23634,.T.);
#42333=EDGE_CURVE('',#32972,#32973,#20022,.T.);
#42334=EDGE_CURVE('',#32972,#32974,#20023,.T.);
#42335=EDGE_CURVE('',#32973,#32974,#20024,.T.);
#42336=EDGE_CURVE('',#32971,#32975,#20025,.T.);
#42337=EDGE_CURVE('',#32750,#32975,#25963,.T.);
#42338=EDGE_CURVE('',#32975,#32972,#20026,.T.);
#42339=EDGE_CURVE('',#32974,#32970,#20027,.T.);
#42340=EDGE_CURVE('',#32976,#32750,#25964,.T.);
#42341=EDGE_CURVE('',#32976,#32977,#20028,.T.);
#42342=EDGE_CURVE('',#32468,#32977,#23635,.T.);
#42343=EDGE_CURVE('',#32978,#32979,#20029,.T.);
#42344=EDGE_CURVE('',#32978,#32980,#20030,.T.);
#42345=EDGE_CURVE('',#32979,#32980,#20031,.T.);
#42346=EDGE_CURVE('',#32977,#32981,#20032,.T.);
#42347=EDGE_CURVE('',#32751,#32981,#25965,.T.);
#42348=EDGE_CURVE('',#32981,#32978,#20033,.T.);
#42349=EDGE_CURVE('',#32980,#32976,#20034,.T.);
#42350=EDGE_CURVE('',#32982,#32751,#25966,.T.);
#42351=EDGE_CURVE('',#32982,#32983,#20035,.T.);
#42352=EDGE_CURVE('',#32469,#32983,#23636,.T.);
#42353=EDGE_CURVE('',#32984,#32985,#20036,.T.);
#42354=EDGE_CURVE('',#32984,#32986,#20037,.T.);
#42355=EDGE_CURVE('',#32985,#32986,#20038,.T.);
#42356=EDGE_CURVE('',#32983,#32987,#20039,.T.);
#42357=EDGE_CURVE('',#32752,#32987,#25967,.T.);
#42358=EDGE_CURVE('',#32987,#32984,#20040,.T.);
#42359=EDGE_CURVE('',#32986,#32982,#20041,.T.);
#42360=EDGE_CURVE('',#32988,#32752,#25968,.T.);
#42361=EDGE_CURVE('',#32988,#32989,#20042,.T.);
#42362=EDGE_CURVE('',#32470,#32989,#23637,.T.);
#42363=EDGE_CURVE('',#32990,#32991,#20043,.T.);
#42364=EDGE_CURVE('',#32990,#32992,#20044,.T.);
#42365=EDGE_CURVE('',#32991,#32992,#20045,.T.);
#42366=EDGE_CURVE('',#32989,#32993,#20046,.T.);
#42367=EDGE_CURVE('',#32753,#32993,#25969,.T.);
#42368=EDGE_CURVE('',#32993,#32990,#20047,.T.);
#42369=EDGE_CURVE('',#32992,#32988,#20048,.T.);
#42370=EDGE_CURVE('',#32994,#32753,#25970,.T.);
#42371=EDGE_CURVE('',#32994,#32995,#20049,.T.);
#42372=EDGE_CURVE('',#32471,#32995,#23638,.T.);
#42373=EDGE_CURVE('',#32996,#32997,#20050,.T.);
#42374=EDGE_CURVE('',#32996,#32998,#20051,.T.);
#42375=EDGE_CURVE('',#32997,#32998,#20052,.T.);
#42376=EDGE_CURVE('',#32995,#32999,#20053,.T.);
#42377=EDGE_CURVE('',#32754,#32999,#25971,.T.);
#42378=EDGE_CURVE('',#32999,#32996,#20054,.T.);
#42379=EDGE_CURVE('',#32998,#32994,#20055,.T.);
#42380=EDGE_CURVE('',#28928,#32754,#25972,.T.);
#42381=EDGE_CURVE('',#32472,#28927,#23639,.T.);
#42382=EDGE_CURVE('',#32755,#28926,#25973,.T.);
#42383=EDGE_CURVE('',#33000,#32755,#25974,.T.);
#42384=EDGE_CURVE('',#33000,#33001,#20056,.T.);
#42385=EDGE_CURVE('',#32473,#33001,#23640,.T.);
#42386=EDGE_CURVE('',#33002,#33003,#20057,.T.);
#42387=EDGE_CURVE('',#33002,#33004,#20058,.T.);
#42388=EDGE_CURVE('',#33003,#33004,#20059,.T.);
#42389=EDGE_CURVE('',#33001,#33005,#20060,.T.);
#42390=EDGE_CURVE('',#32756,#33005,#25975,.T.);
#42391=EDGE_CURVE('',#33005,#33002,#20061,.T.);
#42392=EDGE_CURVE('',#33004,#33000,#20062,.T.);
#42393=EDGE_CURVE('',#33006,#32756,#25976,.T.);
#42394=EDGE_CURVE('',#33006,#33007,#20063,.T.);
#42395=EDGE_CURVE('',#32474,#33007,#23641,.T.);
#42396=EDGE_CURVE('',#33008,#33009,#20064,.T.);
#42397=EDGE_CURVE('',#33008,#33010,#20065,.T.);
#42398=EDGE_CURVE('',#33009,#33010,#20066,.T.);
#42399=EDGE_CURVE('',#33007,#33011,#20067,.T.);
#42400=EDGE_CURVE('',#32757,#33011,#25977,.T.);
#42401=EDGE_CURVE('',#33011,#33008,#20068,.T.);
#42402=EDGE_CURVE('',#33010,#33006,#20069,.T.);
#42403=EDGE_CURVE('',#33012,#32757,#25978,.T.);
#42404=EDGE_CURVE('',#33012,#33013,#20070,.T.);
#42405=EDGE_CURVE('',#32475,#33013,#23642,.T.);
#42406=EDGE_CURVE('',#33014,#33015,#20071,.T.);
#42407=EDGE_CURVE('',#33016,#33014,#20072,.T.);
#42408=EDGE_CURVE('',#33016,#33015,#20073,.T.);
#42409=EDGE_CURVE('',#33013,#33017,#20074,.T.);
#42410=EDGE_CURVE('',#32758,#33017,#25979,.T.);
#42411=EDGE_CURVE('',#33017,#33016,#20075,.T.);
#42412=EDGE_CURVE('',#33015,#33012,#20076,.T.);
#42413=EDGE_CURVE('',#33018,#32758,#25980,.T.);
#42414=EDGE_CURVE('',#33018,#33019,#20077,.T.);
#42415=EDGE_CURVE('',#32476,#33019,#23643,.T.);
#42416=EDGE_CURVE('',#33020,#33021,#20078,.T.);
#42417=EDGE_CURVE('',#33020,#33022,#20079,.T.);
#42418=EDGE_CURVE('',#33021,#33022,#20080,.T.);
#42419=EDGE_CURVE('',#33019,#33023,#20081,.T.);
#42420=EDGE_CURVE('',#32759,#33023,#25981,.T.);
#42421=EDGE_CURVE('',#33023,#33020,#20082,.T.);
#42422=EDGE_CURVE('',#33022,#33018,#20083,.T.);
#42423=EDGE_CURVE('',#33024,#32759,#25982,.T.);
#42424=EDGE_CURVE('',#33024,#33025,#20084,.T.);
#42425=EDGE_CURVE('',#32477,#33025,#23644,.T.);
#42426=EDGE_CURVE('',#33026,#33027,#20085,.T.);
#42427=EDGE_CURVE('',#33026,#33028,#20086,.T.);
#42428=EDGE_CURVE('',#33027,#33028,#20087,.T.);
#42429=EDGE_CURVE('',#33025,#33029,#20088,.T.);
#42430=EDGE_CURVE('',#32760,#33029,#25983,.T.);
#42431=EDGE_CURVE('',#33029,#33026,#20089,.T.);
#42432=EDGE_CURVE('',#33028,#33024,#20090,.T.);
#42433=EDGE_CURVE('',#33030,#32760,#25984,.T.);
#42434=EDGE_CURVE('',#33030,#33031,#20091,.T.);
#42435=EDGE_CURVE('',#32478,#33031,#23645,.T.);
#42436=EDGE_CURVE('',#33032,#33033,#20092,.T.);
#42437=EDGE_CURVE('',#33032,#33034,#20093,.T.);
#42438=EDGE_CURVE('',#33033,#33034,#20094,.T.);
#42439=EDGE_CURVE('',#33031,#33035,#20095,.T.);
#42440=EDGE_CURVE('',#32761,#33035,#25985,.T.);
#42441=EDGE_CURVE('',#33035,#33032,#20096,.T.);
#42442=EDGE_CURVE('',#33034,#33030,#20097,.T.);
#42443=EDGE_CURVE('',#33036,#32761,#25986,.T.);
#42444=EDGE_CURVE('',#33036,#33037,#20098,.T.);
#42445=EDGE_CURVE('',#32479,#33037,#23646,.T.);
#42446=EDGE_CURVE('',#33038,#33039,#20099,.T.);
#42447=EDGE_CURVE('',#33038,#33040,#20100,.T.);
#42448=EDGE_CURVE('',#33039,#33040,#20101,.T.);
#42449=EDGE_CURVE('',#33037,#33041,#20102,.T.);
#42450=EDGE_CURVE('',#32733,#33041,#25987,.T.);
#42451=EDGE_CURVE('',#33041,#33038,#20103,.T.);
#42452=EDGE_CURVE('',#33040,#33036,#20104,.T.);
#42453=EDGE_CURVE('',#33042,#32704,#20105,.T.);
#42454=EDGE_CURVE('',#32764,#33042,#23647,.T.);
#42455=EDGE_CURVE('',#32705,#33042,#20106,.T.);
#42456=EDGE_CURVE('',#33043,#32705,#20107,.T.);
#42457=EDGE_CURVE('',#32768,#33043,#23648,.T.);
#42458=EDGE_CURVE('',#32706,#33043,#20108,.T.);
#42459=EDGE_CURVE('',#33044,#32706,#20109,.T.);
#42460=EDGE_CURVE('',#32772,#33044,#23649,.T.);
#42461=EDGE_CURVE('',#32707,#33044,#20110,.T.);
#42462=EDGE_CURVE('',#33045,#32707,#20111,.T.);
#42463=EDGE_CURVE('',#32776,#33045,#23650,.T.);
#42464=EDGE_CURVE('',#32708,#33045,#20112,.T.);
#42465=EDGE_CURVE('',#33046,#32708,#20113,.T.);
#42466=EDGE_CURVE('',#32780,#33046,#23651,.T.);
#42467=EDGE_CURVE('',#32709,#33046,#20114,.T.);
#42468=EDGE_CURVE('',#33047,#32709,#20115,.T.);
#42469=EDGE_CURVE('',#32784,#33047,#23652,.T.);
#42470=EDGE_CURVE('',#32710,#33047,#20116,.T.);
#42471=EDGE_CURVE('',#33048,#32710,#20117,.T.);
#42472=EDGE_CURVE('',#32788,#33048,#23653,.T.);
#42473=EDGE_CURVE('',#32711,#33048,#20118,.T.);
#42474=EDGE_CURVE('',#33049,#32711,#20119,.T.);
#42475=EDGE_CURVE('',#32792,#33049,#23654,.T.);
#42476=EDGE_CURVE('',#32712,#33049,#20120,.T.);
#42477=EDGE_CURVE('',#33050,#32712,#20121,.T.);
#42478=EDGE_CURVE('',#32796,#33050,#23655,.T.);
#42479=EDGE_CURVE('',#32713,#33050,#20122,.T.);
#42480=EDGE_CURVE('',#33051,#32713,#20123,.T.);
#42481=EDGE_CURVE('',#32800,#33051,#23656,.T.);
#42482=EDGE_CURVE('',#32714,#33051,#20124,.T.);
#42483=EDGE_CURVE('',#33052,#32714,#20125,.T.);
#42484=EDGE_CURVE('',#32804,#33052,#23657,.T.);
#42485=EDGE_CURVE('',#32715,#33052,#20126,.T.);
#42486=EDGE_CURVE('',#33053,#32715,#20127,.T.);
#42487=EDGE_CURVE('',#32808,#33053,#23658,.T.);
#42488=EDGE_CURVE('',#32716,#33053,#20128,.T.);
#42489=EDGE_CURVE('',#33054,#32716,#20129,.T.);
#42490=EDGE_CURVE('',#32812,#33054,#23659,.T.);
#42491=EDGE_CURVE('',#32717,#33054,#20130,.T.);
#42492=EDGE_CURVE('',#33055,#32717,#20131,.T.);
#42493=EDGE_CURVE('',#32816,#33055,#23660,.T.);
#42494=EDGE_CURVE('',#32718,#33055,#20132,.T.);
#42495=EDGE_CURVE('',#33056,#32718,#20133,.T.);
#42496=EDGE_CURVE('',#28932,#33056,#23661,.T.);
#42497=EDGE_CURVE('',#32719,#33056,#20134,.T.);
#42498=EDGE_CURVE('',#33057,#32719,#20135,.T.);
#42499=EDGE_CURVE('',#32820,#33057,#23662,.T.);
#42500=EDGE_CURVE('',#32720,#33057,#20136,.T.);
#42501=EDGE_CURVE('',#33058,#32720,#20137,.T.);
#42502=EDGE_CURVE('',#32824,#33058,#23663,.T.);
#42503=EDGE_CURVE('',#32721,#33058,#20138,.T.);
#42504=EDGE_CURVE('',#33059,#32721,#20139,.T.);
#42505=EDGE_CURVE('',#32828,#33059,#23664,.T.);
#42506=EDGE_CURVE('',#32722,#33059,#20140,.T.);
#42507=EDGE_CURVE('',#33060,#32722,#20141,.T.);
#42508=EDGE_CURVE('',#32833,#33060,#23665,.T.);
#42509=EDGE_CURVE('',#32723,#33060,#20142,.T.);
#42510=EDGE_CURVE('',#33061,#32723,#20143,.T.);
#42511=EDGE_CURVE('',#32837,#33061,#23666,.T.);
#42512=EDGE_CURVE('',#32724,#33061,#20144,.T.);
#42513=EDGE_CURVE('',#33062,#32724,#20145,.T.);
#42514=EDGE_CURVE('',#32840,#33062,#23667,.T.);
#42515=EDGE_CURVE('',#32725,#33062,#20146,.T.);
#42516=EDGE_CURVE('',#33063,#32725,#20147,.T.);
#42517=EDGE_CURVE('',#32844,#33063,#23668,.T.);
#42518=EDGE_CURVE('',#32726,#33063,#20148,.T.);
#42519=EDGE_CURVE('',#33064,#32726,#20149,.T.);
#42520=EDGE_CURVE('',#32848,#33064,#23669,.T.);
#42521=EDGE_CURVE('',#32727,#33064,#20150,.T.);
#42522=EDGE_CURVE('',#33065,#32727,#20151,.T.);
#42523=EDGE_CURVE('',#32852,#33065,#23670,.T.);
#42524=EDGE_CURVE('',#32728,#33065,#20152,.T.);
#42525=EDGE_CURVE('',#33066,#32728,#20153,.T.);
#42526=EDGE_CURVE('',#32856,#33066,#23671,.T.);
#42527=EDGE_CURVE('',#32729,#33066,#20154,.T.);
#42528=EDGE_CURVE('',#33067,#32729,#20155,.T.);
#42529=EDGE_CURVE('',#32860,#33067,#23672,.T.);
#42530=EDGE_CURVE('',#32730,#33067,#20156,.T.);
#42531=EDGE_CURVE('',#33068,#32730,#20157,.T.);
#42532=EDGE_CURVE('',#32864,#33068,#23673,.T.);
#42533=EDGE_CURVE('',#32731,#33068,#20158,.T.);
#42534=EDGE_CURVE('',#33069,#32731,#20159,.T.);
#42535=EDGE_CURVE('',#32868,#33069,#23674,.T.);
#42536=EDGE_CURVE('',#32732,#33069,#20160,.T.);
#42537=EDGE_CURVE('',#33070,#32732,#20161,.T.);
#42538=EDGE_CURVE('',#32872,#33070,#23675,.T.);
#42539=EDGE_CURVE('',#32704,#33070,#20162,.T.);
#42540=EDGE_CURVE('',#33071,#32733,#20163,.T.);
#42541=EDGE_CURVE('',#32877,#33071,#112,.T.);
#42542=EDGE_CURVE('',#32734,#33071,#20164,.T.);
#42543=EDGE_CURVE('',#33072,#32734,#20165,.T.);
#42544=EDGE_CURVE('',#32883,#33072,#113,.T.);
#42545=EDGE_CURVE('',#32735,#33072,#20166,.T.);
#42546=EDGE_CURVE('',#33073,#32735,#20167,.T.);
#42547=EDGE_CURVE('',#32889,#33073,#114,.T.);
#42548=EDGE_CURVE('',#32736,#33073,#20168,.T.);
#42549=EDGE_CURVE('',#33074,#32736,#20169,.T.);
#42550=EDGE_CURVE('',#32895,#33074,#115,.T.);
#42551=EDGE_CURVE('',#32737,#33074,#20170,.T.);
#42552=EDGE_CURVE('',#33075,#32737,#20171,.T.);
#42553=EDGE_CURVE('',#32901,#33075,#116,.T.);
#42554=EDGE_CURVE('',#32738,#33075,#20172,.T.);
#42555=EDGE_CURVE('',#33076,#32738,#20173,.T.);
#42556=EDGE_CURVE('',#32907,#33076,#117,.T.);
#42557=EDGE_CURVE('',#32739,#33076,#20174,.T.);
#42558=EDGE_CURVE('',#33077,#32739,#20175,.T.);
#42559=EDGE_CURVE('',#32913,#33077,#118,.T.);
#42560=EDGE_CURVE('',#32740,#33077,#20176,.T.);
#42561=EDGE_CURVE('',#33078,#32740,#20177,.T.);
#42562=EDGE_CURVE('',#32919,#33078,#119,.T.);
#42563=EDGE_CURVE('',#32741,#33078,#20178,.T.);
#42564=EDGE_CURVE('',#33079,#32741,#20179,.T.);
#42565=EDGE_CURVE('',#32925,#33079,#120,.T.);
#42566=EDGE_CURVE('',#32742,#33079,#20180,.T.);
#42567=EDGE_CURVE('',#33080,#32742,#20181,.T.);
#42568=EDGE_CURVE('',#32931,#33080,#121,.T.);
#42569=EDGE_CURVE('',#32743,#33080,#20182,.T.);
#42570=EDGE_CURVE('',#33081,#32743,#20183,.T.);
#42571=EDGE_CURVE('',#32937,#33081,#122,.T.);
#42572=EDGE_CURVE('',#32744,#33081,#20184,.T.);
#42573=EDGE_CURVE('',#33082,#32744,#20185,.T.);
#42574=EDGE_CURVE('',#32943,#33082,#123,.T.);
#42575=EDGE_CURVE('',#32745,#33082,#20186,.T.);
#42576=EDGE_CURVE('',#33083,#32745,#20187,.T.);
#42577=EDGE_CURVE('',#32949,#33083,#124,.T.);
#42578=EDGE_CURVE('',#32746,#33083,#20188,.T.);
#42579=EDGE_CURVE('',#33084,#32746,#20189,.T.);
#42580=EDGE_CURVE('',#32955,#33084,#125,.T.);
#42581=EDGE_CURVE('',#32747,#33084,#20190,.T.);
#42582=EDGE_CURVE('',#33085,#32747,#20191,.T.);
#42583=EDGE_CURVE('',#32961,#33085,#126,.T.);
#42584=EDGE_CURVE('',#32748,#33085,#20192,.T.);
#42585=EDGE_CURVE('',#33086,#32748,#20193,.T.);
#42586=EDGE_CURVE('',#32967,#33086,#127,.T.);
#42587=EDGE_CURVE('',#32749,#33086,#20194,.T.);
#42588=EDGE_CURVE('',#33087,#32749,#20195,.T.);
#42589=EDGE_CURVE('',#32973,#33087,#128,.T.);
#42590=EDGE_CURVE('',#32750,#33087,#20196,.T.);
#42591=EDGE_CURVE('',#33088,#32750,#20197,.T.);
#42592=EDGE_CURVE('',#32979,#33088,#129,.T.);
#42593=EDGE_CURVE('',#32751,#33088,#20198,.T.);
#42594=EDGE_CURVE('',#33089,#32751,#20199,.T.);
#42595=EDGE_CURVE('',#32985,#33089,#130,.T.);
#42596=EDGE_CURVE('',#32752,#33089,#20200,.T.);
#42597=EDGE_CURVE('',#33090,#32752,#20201,.T.);
#42598=EDGE_CURVE('',#32991,#33090,#131,.T.);
#42599=EDGE_CURVE('',#32753,#33090,#20202,.T.);
#42600=EDGE_CURVE('',#33091,#32753,#20203,.T.);
#42601=EDGE_CURVE('',#32997,#33091,#132,.T.);
#42602=EDGE_CURVE('',#32754,#33091,#20204,.T.);
#42603=EDGE_CURVE('',#33092,#32754,#20205,.T.);
#42604=EDGE_CURVE('',#28929,#33092,#133,.T.);
#42605=EDGE_CURVE('',#32755,#33092,#20206,.T.);
#42606=EDGE_CURVE('',#33093,#32755,#20207,.T.);
#42607=EDGE_CURVE('',#33003,#33093,#134,.T.);
#42608=EDGE_CURVE('',#32756,#33093,#20208,.T.);
#42609=EDGE_CURVE('',#33094,#32756,#20209,.T.);
#42610=EDGE_CURVE('',#33009,#33094,#135,.T.);
#42611=EDGE_CURVE('',#32757,#33094,#20210,.T.);
#42612=EDGE_CURVE('',#33095,#32757,#20211,.T.);
#42613=EDGE_CURVE('',#33014,#33095,#136,.T.);
#42614=EDGE_CURVE('',#32758,#33095,#20212,.T.);
#42615=EDGE_CURVE('',#33096,#32758,#20213,.T.);
#42616=EDGE_CURVE('',#33021,#33096,#137,.T.);
#42617=EDGE_CURVE('',#32759,#33096,#20214,.T.);
#42618=EDGE_CURVE('',#33097,#32759,#20215,.T.);
#42619=EDGE_CURVE('',#33027,#33097,#138,.T.);
#42620=EDGE_CURVE('',#32760,#33097,#20216,.T.);
#42621=EDGE_CURVE('',#33098,#32760,#20217,.T.);
#42622=EDGE_CURVE('',#33033,#33098,#139,.T.);
#42623=EDGE_CURVE('',#32761,#33098,#20218,.T.);
#42624=EDGE_CURVE('',#33099,#32761,#20219,.T.);
#42625=EDGE_CURVE('',#33039,#33099,#140,.T.);
#42626=EDGE_CURVE('',#32733,#33099,#20220,.T.);
#42627=EDGE_CURVE('',#33100,#33101,#20221,.T.);
#42628=EDGE_CURVE('',#33042,#33101,#25988,.T.);
#42629=EDGE_CURVE('',#33100,#32704,#23676,.T.);
#42630=EDGE_CURVE('',#33102,#33103,#20222,.T.);
#42631=EDGE_CURVE('',#32705,#33103,#23677,.T.);
#42632=EDGE_CURVE('',#33102,#33042,#25989,.T.);
#42633=EDGE_CURVE('',#33104,#33102,#20223,.T.);
#42634=EDGE_CURVE('',#33105,#33104,#20224,.T.);
#42635=EDGE_CURVE('',#33103,#33105,#20225,.T.);
#42636=EDGE_CURVE('',#33043,#33105,#25990,.T.);
#42637=EDGE_CURVE('',#33106,#33107,#20226,.T.);
#42638=EDGE_CURVE('',#32706,#33107,#23678,.T.);
#42639=EDGE_CURVE('',#33106,#33043,#25991,.T.);
#42640=EDGE_CURVE('',#33108,#33106,#20227,.T.);
#42641=EDGE_CURVE('',#33109,#33108,#20228,.T.);
#42642=EDGE_CURVE('',#33107,#33109,#20229,.T.);
#42643=EDGE_CURVE('',#33044,#33109,#25992,.T.);
#42644=EDGE_CURVE('',#33110,#33111,#20230,.T.);
#42645=EDGE_CURVE('',#32707,#33111,#23679,.T.);
#42646=EDGE_CURVE('',#33110,#33044,#25993,.T.);
#42647=EDGE_CURVE('',#33112,#33110,#20231,.T.);
#42648=EDGE_CURVE('',#33113,#33112,#20232,.T.);
#42649=EDGE_CURVE('',#33111,#33113,#20233,.T.);
#42650=EDGE_CURVE('',#33045,#33113,#25994,.T.);
#42651=EDGE_CURVE('',#33114,#33115,#20234,.T.);
#42652=EDGE_CURVE('',#32708,#33115,#23680,.T.);
#42653=EDGE_CURVE('',#33114,#33045,#25995,.T.);
#42654=EDGE_CURVE('',#33116,#33114,#20235,.T.);
#42655=EDGE_CURVE('',#33117,#33116,#20236,.T.);
#42656=EDGE_CURVE('',#33115,#33117,#20237,.T.);
#42657=EDGE_CURVE('',#33046,#33117,#25996,.T.);
#42658=EDGE_CURVE('',#33118,#33119,#20238,.T.);
#42659=EDGE_CURVE('',#32709,#33119,#23681,.T.);
#42660=EDGE_CURVE('',#33118,#33046,#25997,.T.);
#42661=EDGE_CURVE('',#33120,#33118,#20239,.T.);
#42662=EDGE_CURVE('',#33121,#33120,#20240,.T.);
#42663=EDGE_CURVE('',#33119,#33121,#20241,.T.);
#42664=EDGE_CURVE('',#33047,#33121,#25998,.T.);
#42665=EDGE_CURVE('',#33122,#33123,#20242,.T.);
#42666=EDGE_CURVE('',#32710,#33123,#23682,.T.);
#42667=EDGE_CURVE('',#33122,#33047,#25999,.T.);
#42668=EDGE_CURVE('',#33124,#33122,#20243,.T.);
#42669=EDGE_CURVE('',#33125,#33124,#20244,.T.);
#42670=EDGE_CURVE('',#33123,#33125,#20245,.T.);
#42671=EDGE_CURVE('',#33048,#33125,#26000,.T.);
#42672=EDGE_CURVE('',#32711,#28920,#23683,.T.);
#42673=EDGE_CURVE('',#28922,#33048,#26001,.T.);
#42674=EDGE_CURVE('',#33049,#28921,#26002,.T.);
#42675=EDGE_CURVE('',#33126,#33127,#20246,.T.);
#42676=EDGE_CURVE('',#32712,#33127,#23684,.T.);
#42677=EDGE_CURVE('',#33126,#33049,#26003,.T.);
#42678=EDGE_CURVE('',#33128,#33126,#20247,.T.);
#42679=EDGE_CURVE('',#33129,#33128,#20248,.T.);
#42680=EDGE_CURVE('',#33127,#33129,#20249,.T.);
#42681=EDGE_CURVE('',#33050,#33129,#26004,.T.);
#42682=EDGE_CURVE('',#33130,#33131,#20250,.T.);
#42683=EDGE_CURVE('',#32713,#33131,#23685,.T.);
#42684=EDGE_CURVE('',#33130,#33050,#26005,.T.);
#42685=EDGE_CURVE('',#33132,#33130,#20251,.T.);
#42686=EDGE_CURVE('',#33133,#33132,#20252,.T.);
#42687=EDGE_CURVE('',#33131,#33133,#20253,.T.);
#42688=EDGE_CURVE('',#33051,#33133,#26006,.T.);
#42689=EDGE_CURVE('',#33134,#33135,#20254,.T.);
#42690=EDGE_CURVE('',#32714,#33135,#23686,.T.);
#42691=EDGE_CURVE('',#33134,#33051,#26007,.T.);
#42692=EDGE_CURVE('',#33136,#33134,#20255,.T.);
#42693=EDGE_CURVE('',#33137,#33136,#20256,.T.);
#42694=EDGE_CURVE('',#33135,#33137,#20257,.T.);
#42695=EDGE_CURVE('',#33052,#33137,#26008,.T.);
#42696=EDGE_CURVE('',#33138,#33139,#20258,.T.);
#42697=EDGE_CURVE('',#32715,#33139,#23687,.T.);
#42698=EDGE_CURVE('',#33138,#33052,#26009,.T.);
#42699=EDGE_CURVE('',#33140,#33138,#20259,.T.);
#42700=EDGE_CURVE('',#33141,#33140,#20260,.T.);
#42701=EDGE_CURVE('',#33139,#33141,#20261,.T.);
#42702=EDGE_CURVE('',#33053,#33141,#26010,.T.);
#42703=EDGE_CURVE('',#33142,#33143,#20262,.T.);
#42704=EDGE_CURVE('',#32716,#33143,#23688,.T.);
#42705=EDGE_CURVE('',#33142,#33053,#26011,.T.);
#42706=EDGE_CURVE('',#33144,#33142,#20263,.T.);
#42707=EDGE_CURVE('',#33145,#33144,#20264,.T.);
#42708=EDGE_CURVE('',#33143,#33145,#20265,.T.);
#42709=EDGE_CURVE('',#33054,#33145,#26012,.T.);
#42710=EDGE_CURVE('',#33146,#33147,#20266,.T.);
#42711=EDGE_CURVE('',#32717,#33147,#23689,.T.);
#42712=EDGE_CURVE('',#33146,#33054,#26013,.T.);
#42713=EDGE_CURVE('',#33148,#33146,#20267,.T.);
#42714=EDGE_CURVE('',#33149,#33148,#20268,.T.);
#42715=EDGE_CURVE('',#33147,#33149,#20269,.T.);
#42716=EDGE_CURVE('',#33055,#33149,#26014,.T.);
#42717=EDGE_CURVE('',#33150,#33151,#20270,.T.);
#42718=EDGE_CURVE('',#32718,#33151,#23690,.T.);
#42719=EDGE_CURVE('',#33150,#33055,#26015,.T.);
#42720=EDGE_CURVE('',#33152,#33150,#20271,.T.);
#42721=EDGE_CURVE('',#33153,#33152,#20272,.T.);
#42722=EDGE_CURVE('',#33151,#33153,#20273,.T.);
#42723=EDGE_CURVE('',#33056,#33153,#26016,.T.);
#42724=EDGE_CURVE('',#33154,#33155,#20274,.T.);
#42725=EDGE_CURVE('',#32719,#33155,#23691,.T.);
#42726=EDGE_CURVE('',#33154,#33056,#26017,.T.);
#42727=EDGE_CURVE('',#33156,#33154,#20275,.T.);
#42728=EDGE_CURVE('',#33157,#33156,#20276,.T.);
#42729=EDGE_CURVE('',#33155,#33157,#20277,.T.);
#42730=EDGE_CURVE('',#33057,#33157,#26018,.T.);
#42731=EDGE_CURVE('',#33158,#33159,#20278,.T.);
#42732=EDGE_CURVE('',#32720,#33159,#23692,.T.);
#42733=EDGE_CURVE('',#33158,#33057,#26019,.T.);
#42734=EDGE_CURVE('',#33160,#33158,#20279,.T.);
#42735=EDGE_CURVE('',#33161,#33160,#20280,.T.);
#42736=EDGE_CURVE('',#33159,#33161,#20281,.T.);
#42737=EDGE_CURVE('',#33058,#33161,#26020,.T.);
#42738=EDGE_CURVE('',#33162,#33163,#20282,.T.);
#42739=EDGE_CURVE('',#32721,#33163,#23693,.T.);
#42740=EDGE_CURVE('',#33162,#33058,#26021,.T.);
#42741=EDGE_CURVE('',#33164,#33162,#20283,.T.);
#42742=EDGE_CURVE('',#33165,#33164,#20284,.T.);
#42743=EDGE_CURVE('',#33163,#33165,#20285,.T.);
#42744=EDGE_CURVE('',#33059,#33165,#26022,.T.);
#42745=EDGE_CURVE('',#33166,#33167,#20286,.T.);
#42746=EDGE_CURVE('',#32722,#33167,#23694,.T.);
#42747=EDGE_CURVE('',#33166,#33059,#26023,.T.);
#42748=EDGE_CURVE('',#33167,#33168,#20287,.T.);
#42749=EDGE_CURVE('',#33060,#33168,#26024,.T.);
#42750=EDGE_CURVE('',#33169,#33166,#20288,.T.);
#42751=EDGE_CURVE('',#33168,#33169,#20289,.T.);
#42752=EDGE_CURVE('',#33170,#33060,#26025,.T.);
#42753=EDGE_CURVE('',#33170,#33171,#20290,.T.);
#42754=EDGE_CURVE('',#32723,#33171,#23695,.T.);
#42755=EDGE_CURVE('',#33171,#33172,#20291,.T.);
#42756=EDGE_CURVE('',#33173,#33170,#20292,.T.);
#42757=EDGE_CURVE('',#33172,#33173,#20293,.T.);
#42758=EDGE_CURVE('',#33061,#33172,#26026,.T.);
#42759=EDGE_CURVE('',#33174,#33175,#20294,.T.);
#42760=EDGE_CURVE('',#32724,#33175,#23696,.T.);
#42761=EDGE_CURVE('',#33174,#33061,#26027,.T.);
#42762=EDGE_CURVE('',#33176,#33174,#20295,.T.);
#42763=EDGE_CURVE('',#33177,#33176,#20296,.T.);
#42764=EDGE_CURVE('',#33175,#33177,#20297,.T.);
#42765=EDGE_CURVE('',#33062,#33177,#26028,.T.);
#42766=EDGE_CURVE('',#33178,#33179,#20298,.T.);
#42767=EDGE_CURVE('',#32725,#33179,#23697,.T.);
#42768=EDGE_CURVE('',#33178,#33062,#26029,.T.);
#42769=EDGE_CURVE('',#33180,#33178,#20299,.T.);
#42770=EDGE_CURVE('',#33181,#33180,#20300,.T.);
#42771=EDGE_CURVE('',#33179,#33181,#20301,.T.);
#42772=EDGE_CURVE('',#33063,#33181,#26030,.T.);
#42773=EDGE_CURVE('',#33182,#33183,#20302,.T.);
#42774=EDGE_CURVE('',#32726,#33183,#23698,.T.);
#42775=EDGE_CURVE('',#33182,#33063,#26031,.T.);
#42776=EDGE_CURVE('',#33184,#33182,#20303,.T.);
#42777=EDGE_CURVE('',#33185,#33184,#20304,.T.);
#42778=EDGE_CURVE('',#33183,#33185,#20305,.T.);
#42779=EDGE_CURVE('',#33064,#33185,#26032,.T.);
#42780=EDGE_CURVE('',#33186,#33187,#20306,.T.);
#42781=EDGE_CURVE('',#32727,#33187,#23699,.T.);
#42782=EDGE_CURVE('',#33186,#33064,#26033,.T.);
#42783=EDGE_CURVE('',#33188,#33186,#20307,.T.);
#42784=EDGE_CURVE('',#33189,#33188,#20308,.T.);
#42785=EDGE_CURVE('',#33187,#33189,#20309,.T.);
#42786=EDGE_CURVE('',#33065,#33189,#26034,.T.);
#42787=EDGE_CURVE('',#33190,#33191,#20310,.T.);
#42788=EDGE_CURVE('',#32728,#33191,#23700,.T.);
#42789=EDGE_CURVE('',#33190,#33065,#26035,.T.);
#42790=EDGE_CURVE('',#33192,#33190,#20311,.T.);
#42791=EDGE_CURVE('',#33193,#33192,#20312,.T.);
#42792=EDGE_CURVE('',#33191,#33193,#20313,.T.);
#42793=EDGE_CURVE('',#33066,#33193,#26036,.T.);
#42794=EDGE_CURVE('',#33194,#33195,#20314,.T.);
#42795=EDGE_CURVE('',#32729,#33195,#23701,.T.);
#42796=EDGE_CURVE('',#33194,#33066,#26037,.T.);
#42797=EDGE_CURVE('',#33196,#33194,#20315,.T.);
#42798=EDGE_CURVE('',#33197,#33196,#20316,.T.);
#42799=EDGE_CURVE('',#33195,#33197,#20317,.T.);
#42800=EDGE_CURVE('',#33067,#33197,#26038,.T.);
#42801=EDGE_CURVE('',#33198,#33199,#20318,.T.);
#42802=EDGE_CURVE('',#32730,#33199,#23702,.T.);
#42803=EDGE_CURVE('',#33198,#33067,#26039,.T.);
#42804=EDGE_CURVE('',#33200,#33198,#20319,.T.);
#42805=EDGE_CURVE('',#33201,#33200,#20320,.T.);
#42806=EDGE_CURVE('',#33199,#33201,#20321,.T.);
#42807=EDGE_CURVE('',#33068,#33201,#26040,.T.);
#42808=EDGE_CURVE('',#33202,#33203,#20322,.T.);
#42809=EDGE_CURVE('',#32731,#33203,#23703,.T.);
#42810=EDGE_CURVE('',#33202,#33068,#26041,.T.);
#42811=EDGE_CURVE('',#33204,#33202,#20323,.T.);
#42812=EDGE_CURVE('',#33205,#33204,#20324,.T.);
#42813=EDGE_CURVE('',#33203,#33205,#20325,.T.);
#42814=EDGE_CURVE('',#33069,#33205,#26042,.T.);
#42815=EDGE_CURVE('',#33206,#33207,#20326,.T.);
#42816=EDGE_CURVE('',#32732,#33207,#23704,.T.);
#42817=EDGE_CURVE('',#33206,#33069,#26043,.T.);
#42818=EDGE_CURVE('',#33208,#33206,#20327,.T.);
#42819=EDGE_CURVE('',#33209,#33208,#20328,.T.);
#42820=EDGE_CURVE('',#33207,#33209,#20329,.T.);
#42821=EDGE_CURVE('',#33070,#33209,#26044,.T.);
#42822=EDGE_CURVE('',#33210,#33211,#20330,.T.);
#42823=EDGE_CURVE('',#33101,#33210,#20331,.T.);
#42824=EDGE_CURVE('',#33211,#33100,#20332,.T.);
#42825=EDGE_CURVE('',#33211,#33070,#26045,.T.);
#42826=EDGE_CURVE('',#33212,#32733,#23705,.T.);
#42827=EDGE_CURVE('',#33212,#33213,#23706,.T.);
#42828=EDGE_CURVE('',#33071,#33213,#26046,.T.);
#42829=EDGE_CURVE('',#33214,#33071,#26047,.T.);
#42830=EDGE_CURVE('',#33214,#33215,#23707,.T.);
#42831=EDGE_CURVE('',#32734,#33215,#23708,.T.);
#42832=EDGE_CURVE('',#33216,#33214,#23709,.T.);
#42833=EDGE_CURVE('',#33217,#33216,#23710,.T.);
#42834=EDGE_CURVE('',#33215,#33217,#23711,.T.);
#42835=EDGE_CURVE('',#33072,#33217,#26048,.T.);
#42836=EDGE_CURVE('',#33218,#33072,#26049,.T.);
#42837=EDGE_CURVE('',#33218,#33219,#23712,.T.);
#42838=EDGE_CURVE('',#32735,#33219,#23713,.T.);
#42839=EDGE_CURVE('',#33220,#33218,#23714,.T.);
#42840=EDGE_CURVE('',#33221,#33220,#23715,.T.);
#42841=EDGE_CURVE('',#33219,#33221,#23716,.T.);
#42842=EDGE_CURVE('',#33073,#33221,#26050,.T.);
#42843=EDGE_CURVE('',#33222,#33073,#26051,.T.);
#42844=EDGE_CURVE('',#33222,#33223,#23717,.T.);
#42845=EDGE_CURVE('',#32736,#33223,#23718,.T.);
#42846=EDGE_CURVE('',#33224,#33222,#23719,.T.);
#42847=EDGE_CURVE('',#33225,#33224,#23720,.T.);
#42848=EDGE_CURVE('',#33223,#33225,#23721,.T.);
#42849=EDGE_CURVE('',#33074,#33225,#26052,.T.);
#42850=EDGE_CURVE('',#33226,#33074,#26053,.T.);
#42851=EDGE_CURVE('',#33226,#33227,#23722,.T.);
#42852=EDGE_CURVE('',#32737,#33227,#23723,.T.);
#42853=EDGE_CURVE('',#33228,#33226,#23724,.T.);
#42854=EDGE_CURVE('',#33229,#33228,#23725,.T.);
#42855=EDGE_CURVE('',#33227,#33229,#23726,.T.);
#42856=EDGE_CURVE('',#33075,#33229,#26054,.T.);
#42857=EDGE_CURVE('',#33230,#33075,#26055,.T.);
#42858=EDGE_CURVE('',#33230,#33231,#23727,.T.);
#42859=EDGE_CURVE('',#32738,#33231,#23728,.T.);
#42860=EDGE_CURVE('',#33232,#33230,#23729,.T.);
#42861=EDGE_CURVE('',#33233,#33232,#23730,.T.);
#42862=EDGE_CURVE('',#33231,#33233,#23731,.T.);
#42863=EDGE_CURVE('',#33076,#33233,#26056,.T.);
#42864=EDGE_CURVE('',#33234,#33076,#26057,.T.);
#42865=EDGE_CURVE('',#33234,#33235,#23732,.T.);
#42866=EDGE_CURVE('',#32739,#33235,#23733,.T.);
#42867=EDGE_CURVE('',#33236,#33234,#23734,.T.);
#42868=EDGE_CURVE('',#33237,#33236,#23735,.T.);
#42869=EDGE_CURVE('',#33235,#33237,#23736,.T.);
#42870=EDGE_CURVE('',#33077,#33237,#26058,.T.);
#42871=EDGE_CURVE('',#33238,#33077,#26059,.T.);
#42872=EDGE_CURVE('',#33238,#33239,#23737,.T.);
#42873=EDGE_CURVE('',#32740,#33239,#23738,.T.);
#42874=EDGE_CURVE('',#33240,#33238,#23739,.T.);
#42875=EDGE_CURVE('',#33241,#33240,#23740,.T.);
#42876=EDGE_CURVE('',#33239,#33241,#23741,.T.);
#42877=EDGE_CURVE('',#33078,#33241,#26060,.T.);
#42878=EDGE_CURVE('',#33242,#33078,#26061,.T.);
#42879=EDGE_CURVE('',#33242,#33243,#23742,.T.);
#42880=EDGE_CURVE('',#32741,#33243,#23743,.T.);
#42881=EDGE_CURVE('',#33244,#33242,#23744,.T.);
#42882=EDGE_CURVE('',#33245,#33244,#23745,.T.);
#42883=EDGE_CURVE('',#33243,#33245,#23746,.T.);
#42884=EDGE_CURVE('',#33079,#33245,#26062,.T.);
#42885=EDGE_CURVE('',#33246,#33079,#26063,.T.);
#42886=EDGE_CURVE('',#33246,#33247,#23747,.T.);
#42887=EDGE_CURVE('',#32742,#33247,#23748,.T.);
#42888=EDGE_CURVE('',#33248,#33246,#23749,.T.);
#42889=EDGE_CURVE('',#33249,#33248,#23750,.T.);
#42890=EDGE_CURVE('',#33247,#33249,#23751,.T.);
#42891=EDGE_CURVE('',#33080,#33249,#26064,.T.);
#42892=EDGE_CURVE('',#33250,#33080,#26065,.T.);
#42893=EDGE_CURVE('',#33250,#33251,#23752,.T.);
#42894=EDGE_CURVE('',#32743,#33251,#23753,.T.);
#42895=EDGE_CURVE('',#33252,#33250,#23754,.T.);
#42896=EDGE_CURVE('',#33253,#33252,#23755,.T.);
#42897=EDGE_CURVE('',#33251,#33253,#23756,.T.);
#42898=EDGE_CURVE('',#33081,#33253,#26066,.T.);
#42899=EDGE_CURVE('',#33254,#33081,#26067,.T.);
#42900=EDGE_CURVE('',#33254,#33255,#23757,.T.);
#42901=EDGE_CURVE('',#32744,#33255,#23758,.T.);
#42902=EDGE_CURVE('',#33256,#33254,#23759,.T.);
#42903=EDGE_CURVE('',#33257,#33256,#23760,.T.);
#42904=EDGE_CURVE('',#33255,#33257,#23761,.T.);
#42905=EDGE_CURVE('',#33082,#33257,#26068,.T.);
#42906=EDGE_CURVE('',#33258,#33082,#26069,.T.);
#42907=EDGE_CURVE('',#33258,#33259,#23762,.T.);
#42908=EDGE_CURVE('',#32745,#33259,#23763,.T.);
#42909=EDGE_CURVE('',#33260,#33258,#23764,.T.);
#42910=EDGE_CURVE('',#33261,#33260,#23765,.T.);
#42911=EDGE_CURVE('',#33259,#33261,#23766,.T.);
#42912=EDGE_CURVE('',#33083,#33261,#26070,.T.);
#42913=EDGE_CURVE('',#33262,#33083,#26071,.T.);
#42914=EDGE_CURVE('',#33262,#33263,#23767,.T.);
#42915=EDGE_CURVE('',#32746,#33263,#23768,.T.);
#42916=EDGE_CURVE('',#33264,#33262,#23769,.T.);
#42917=EDGE_CURVE('',#33265,#33264,#23770,.T.);
#42918=EDGE_CURVE('',#33263,#33265,#23771,.T.);
#42919=EDGE_CURVE('',#33084,#33265,#26072,.T.);
#42920=EDGE_CURVE('',#28919,#33084,#26073,.T.);
#42921=EDGE_CURVE('',#32747,#28918,#23772,.T.);
#42922=EDGE_CURVE('',#33085,#28916,#26074,.T.);
#42923=EDGE_CURVE('',#33266,#33085,#26075,.T.);
#42924=EDGE_CURVE('',#33266,#33267,#23773,.T.);
#42925=EDGE_CURVE('',#32748,#33267,#23774,.T.);
#42926=EDGE_CURVE('',#33268,#33266,#23775,.T.);
#42927=EDGE_CURVE('',#33269,#33268,#23776,.T.);
#42928=EDGE_CURVE('',#33267,#33269,#23777,.T.);
#42929=EDGE_CURVE('',#33086,#33269,#26076,.T.);
#42930=EDGE_CURVE('',#33270,#33086,#26077,.T.);
#42931=EDGE_CURVE('',#33270,#33271,#23778,.T.);
#42932=EDGE_CURVE('',#32749,#33271,#23779,.T.);
#42933=EDGE_CURVE('',#33272,#33270,#23780,.T.);
#42934=EDGE_CURVE('',#33273,#33272,#23781,.T.);
#42935=EDGE_CURVE('',#33271,#33273,#23782,.T.);
#42936=EDGE_CURVE('',#33087,#33273,#26078,.T.);
#42937=EDGE_CURVE('',#33274,#33087,#26079,.T.);
#42938=EDGE_CURVE('',#33274,#33275,#23783,.T.);
#42939=EDGE_CURVE('',#32750,#33275,#23784,.T.);
#42940=EDGE_CURVE('',#33276,#33274,#23785,.T.);
#42941=EDGE_CURVE('',#33277,#33276,#23786,.T.);
#42942=EDGE_CURVE('',#33275,#33277,#23787,.T.);
#42943=EDGE_CURVE('',#33088,#33277,#26080,.T.);
#42944=EDGE_CURVE('',#33278,#33088,#26081,.T.);
#42945=EDGE_CURVE('',#33278,#33279,#23788,.T.);
#42946=EDGE_CURVE('',#32751,#33279,#23789,.T.);
#42947=EDGE_CURVE('',#33280,#33278,#23790,.T.);
#42948=EDGE_CURVE('',#33281,#33280,#23791,.T.);
#42949=EDGE_CURVE('',#33279,#33281,#23792,.T.);
#42950=EDGE_CURVE('',#33089,#33281,#26082,.T.);
#42951=EDGE_CURVE('',#33282,#33089,#26083,.T.);
#42952=EDGE_CURVE('',#33282,#33283,#23793,.T.);
#42953=EDGE_CURVE('',#32752,#33283,#23794,.T.);
#42954=EDGE_CURVE('',#33284,#33282,#23795,.T.);
#42955=EDGE_CURVE('',#33285,#33284,#23796,.T.);
#42956=EDGE_CURVE('',#33283,#33285,#23797,.T.);
#42957=EDGE_CURVE('',#33090,#33285,#26084,.T.);
#42958=EDGE_CURVE('',#33286,#33090,#26085,.T.);
#42959=EDGE_CURVE('',#33286,#33287,#23798,.T.);
#42960=EDGE_CURVE('',#32753,#33287,#23799,.T.);
#42961=EDGE_CURVE('',#33288,#33286,#23800,.T.);
#42962=EDGE_CURVE('',#33289,#33288,#23801,.T.);
#42963=EDGE_CURVE('',#33287,#33289,#23802,.T.);
#42964=EDGE_CURVE('',#33091,#33289,#26086,.T.);
#42965=EDGE_CURVE('',#28915,#33091,#26087,.T.);
#42966=EDGE_CURVE('',#32754,#28914,#23803,.T.);
#42967=EDGE_CURVE('',#33092,#28912,#26088,.T.);
#42968=EDGE_CURVE('',#33290,#33092,#26089,.T.);
#42969=EDGE_CURVE('',#33290,#33291,#23804,.T.);
#42970=EDGE_CURVE('',#32755,#33291,#23805,.T.);
#42971=EDGE_CURVE('',#33292,#33290,#23806,.T.);
#42972=EDGE_CURVE('',#33293,#33292,#23807,.T.);
#42973=EDGE_CURVE('',#33291,#33293,#23808,.T.);
#42974=EDGE_CURVE('',#33093,#33293,#26090,.T.);
#42975=EDGE_CURVE('',#33294,#33093,#26091,.T.);
#42976=EDGE_CURVE('',#33294,#33295,#23809,.T.);
#42977=EDGE_CURVE('',#32756,#33295,#23810,.T.);
#42978=EDGE_CURVE('',#33296,#33294,#23811,.T.);
#42979=EDGE_CURVE('',#33297,#33296,#23812,.T.);
#42980=EDGE_CURVE('',#33295,#33297,#23813,.T.);
#42981=EDGE_CURVE('',#33094,#33297,#26092,.T.);
#42982=EDGE_CURVE('',#33298,#33094,#26093,.T.);
#42983=EDGE_CURVE('',#33298,#33299,#23814,.T.);
#42984=EDGE_CURVE('',#32757,#33299,#23815,.T.);
#42985=EDGE_CURVE('',#33300,#33298,#23816,.T.);
#42986=EDGE_CURVE('',#33301,#33300,#23817,.T.);
#42987=EDGE_CURVE('',#33299,#33301,#23818,.T.);
#42988=EDGE_CURVE('',#33095,#33301,#26094,.T.);
#42989=EDGE_CURVE('',#33302,#33095,#26095,.T.);
#42990=EDGE_CURVE('',#33302,#33303,#23819,.T.);
#42991=EDGE_CURVE('',#32758,#33303,#23820,.T.);
#42992=EDGE_CURVE('',#33304,#33302,#23821,.T.);
#42993=EDGE_CURVE('',#33305,#33304,#23822,.T.);
#42994=EDGE_CURVE('',#33303,#33305,#23823,.T.);
#42995=EDGE_CURVE('',#33096,#33305,#26096,.T.);
#42996=EDGE_CURVE('',#33306,#33096,#26097,.T.);
#42997=EDGE_CURVE('',#33306,#33307,#23824,.T.);
#42998=EDGE_CURVE('',#32759,#33307,#23825,.T.);
#42999=EDGE_CURVE('',#33308,#33306,#23826,.T.);
#43000=EDGE_CURVE('',#33309,#33308,#23827,.T.);
#43001=EDGE_CURVE('',#33307,#33309,#23828,.T.);
#43002=EDGE_CURVE('',#33097,#33309,#26098,.T.);
#43003=EDGE_CURVE('',#33310,#33097,#26099,.T.);
#43004=EDGE_CURVE('',#33310,#33311,#23829,.T.);
#43005=EDGE_CURVE('',#32760,#33311,#23830,.T.);
#43006=EDGE_CURVE('',#33312,#33310,#23831,.T.);
#43007=EDGE_CURVE('',#33313,#33312,#23832,.T.);
#43008=EDGE_CURVE('',#33311,#33313,#23833,.T.);
#43009=EDGE_CURVE('',#33098,#33313,#26100,.T.);
#43010=EDGE_CURVE('',#33314,#33098,#26101,.T.);
#43011=EDGE_CURVE('',#33314,#33315,#23834,.T.);
#43012=EDGE_CURVE('',#32761,#33315,#23835,.T.);
#43013=EDGE_CURVE('',#33316,#33314,#23836,.T.);
#43014=EDGE_CURVE('',#33317,#33316,#23837,.T.);
#43015=EDGE_CURVE('',#33315,#33317,#23838,.T.);
#43016=EDGE_CURVE('',#33099,#33317,#26102,.T.);
#43017=EDGE_CURVE('',#33318,#33212,#23839,.T.);
#43018=EDGE_CURVE('',#33319,#33318,#23840,.T.);
#43019=EDGE_CURVE('',#33213,#33319,#23841,.T.);
#43020=EDGE_CURVE('',#33318,#33099,#26103,.T.);
#43021=EDGE_CURVE('',#33042,#33320,#20333,.T.);
#43022=EDGE_CURVE('',#33320,#33210,#23842,.T.);
#43023=EDGE_CURVE('',#33321,#33042,#20334,.T.);
#43024=EDGE_CURVE('',#33104,#33321,#23843,.T.);
#43025=EDGE_CURVE('',#33043,#33321,#20335,.T.);
#43026=EDGE_CURVE('',#33322,#33043,#20336,.T.);
#43027=EDGE_CURVE('',#33108,#33322,#23844,.T.);
#43028=EDGE_CURVE('',#33044,#33322,#20337,.T.);
#43029=EDGE_CURVE('',#33323,#33044,#20338,.T.);
#43030=EDGE_CURVE('',#33112,#33323,#23845,.T.);
#43031=EDGE_CURVE('',#33045,#33323,#20339,.T.);
#43032=EDGE_CURVE('',#33324,#33045,#20340,.T.);
#43033=EDGE_CURVE('',#33116,#33324,#23846,.T.);
#43034=EDGE_CURVE('',#33046,#33324,#20341,.T.);
#43035=EDGE_CURVE('',#33325,#33046,#20342,.T.);
#43036=EDGE_CURVE('',#33120,#33325,#23847,.T.);
#43037=EDGE_CURVE('',#33047,#33325,#20343,.T.);
#43038=EDGE_CURVE('',#33326,#33047,#20344,.T.);
#43039=EDGE_CURVE('',#33124,#33326,#23848,.T.);
#43040=EDGE_CURVE('',#33048,#33326,#20345,.T.);
#43041=EDGE_CURVE('',#33327,#33048,#20346,.T.);
#43042=EDGE_CURVE('',#28923,#33327,#23849,.T.);
#43043=EDGE_CURVE('',#33049,#33327,#20347,.T.);
#43044=EDGE_CURVE('',#33328,#33049,#20348,.T.);
#43045=EDGE_CURVE('',#33128,#33328,#23850,.T.);
#43046=EDGE_CURVE('',#33050,#33328,#20349,.T.);
#43047=EDGE_CURVE('',#33329,#33050,#20350,.T.);
#43048=EDGE_CURVE('',#33132,#33329,#23851,.T.);
#43049=EDGE_CURVE('',#33051,#33329,#20351,.T.);
#43050=EDGE_CURVE('',#33330,#33051,#20352,.T.);
#43051=EDGE_CURVE('',#33136,#33330,#23852,.T.);
#43052=EDGE_CURVE('',#33052,#33330,#20353,.T.);
#43053=EDGE_CURVE('',#33331,#33052,#20354,.T.);
#43054=EDGE_CURVE('',#33140,#33331,#23853,.T.);
#43055=EDGE_CURVE('',#33053,#33331,#20355,.T.);
#43056=EDGE_CURVE('',#33332,#33053,#20356,.T.);
#43057=EDGE_CURVE('',#33144,#33332,#23854,.T.);
#43058=EDGE_CURVE('',#33054,#33332,#20357,.T.);
#43059=EDGE_CURVE('',#33333,#33054,#20358,.T.);
#43060=EDGE_CURVE('',#33148,#33333,#23855,.T.);
#43061=EDGE_CURVE('',#33055,#33333,#20359,.T.);
#43062=EDGE_CURVE('',#33334,#33055,#20360,.T.);
#43063=EDGE_CURVE('',#33152,#33334,#23856,.T.);
#43064=EDGE_CURVE('',#33056,#33334,#20361,.T.);
#43065=EDGE_CURVE('',#33335,#33056,#20362,.T.);
#43066=EDGE_CURVE('',#33156,#33335,#23857,.T.);
#43067=EDGE_CURVE('',#33057,#33335,#20363,.T.);
#43068=EDGE_CURVE('',#33336,#33057,#20364,.T.);
#43069=EDGE_CURVE('',#33160,#33336,#23858,.T.);
#43070=EDGE_CURVE('',#33058,#33336,#20365,.T.);
#43071=EDGE_CURVE('',#33337,#33058,#20366,.T.);
#43072=EDGE_CURVE('',#33164,#33337,#23859,.T.);
#43073=EDGE_CURVE('',#33059,#33337,#20367,.T.);
#43074=EDGE_CURVE('',#33338,#33059,#20368,.T.);
#43075=EDGE_CURVE('',#33169,#33338,#23860,.T.);
#43076=EDGE_CURVE('',#33060,#33338,#20369,.T.);
#43077=EDGE_CURVE('',#33339,#33060,#20370,.T.);
#43078=EDGE_CURVE('',#33173,#33339,#23861,.T.);
#43079=EDGE_CURVE('',#33061,#33339,#20371,.T.);
#43080=EDGE_CURVE('',#33340,#33061,#20372,.T.);
#43081=EDGE_CURVE('',#33176,#33340,#23862,.T.);
#43082=EDGE_CURVE('',#33062,#33340,#20373,.T.);
#43083=EDGE_CURVE('',#33341,#33062,#20374,.T.);
#43084=EDGE_CURVE('',#33180,#33341,#23863,.T.);
#43085=EDGE_CURVE('',#33063,#33341,#20375,.T.);
#43086=EDGE_CURVE('',#33342,#33063,#20376,.T.);
#43087=EDGE_CURVE('',#33184,#33342,#23864,.T.);
#43088=EDGE_CURVE('',#33064,#33342,#20377,.T.);
#43089=EDGE_CURVE('',#33343,#33064,#20378,.T.);
#43090=EDGE_CURVE('',#33188,#33343,#23865,.T.);
#43091=EDGE_CURVE('',#33065,#33343,#20379,.T.);
#43092=EDGE_CURVE('',#33344,#33065,#20380,.T.);
#43093=EDGE_CURVE('',#33192,#33344,#23866,.T.);
#43094=EDGE_CURVE('',#33066,#33344,#20381,.T.);
#43095=EDGE_CURVE('',#33345,#33066,#20382,.T.);
#43096=EDGE_CURVE('',#33196,#33345,#23867,.T.);
#43097=EDGE_CURVE('',#33067,#33345,#20383,.T.);
#43098=EDGE_CURVE('',#33346,#33067,#20384,.T.);
#43099=EDGE_CURVE('',#33200,#33346,#23868,.T.);
#43100=EDGE_CURVE('',#33068,#33346,#20385,.T.);
#43101=EDGE_CURVE('',#33347,#33068,#20386,.T.);
#43102=EDGE_CURVE('',#33204,#33347,#23869,.T.);
#43103=EDGE_CURVE('',#33069,#33347,#20387,.T.);
#43104=EDGE_CURVE('',#33348,#33069,#20388,.T.);
#43105=EDGE_CURVE('',#33208,#33348,#23870,.T.);
#43106=EDGE_CURVE('',#33070,#33348,#20389,.T.);
#43107=EDGE_CURVE('',#33320,#33070,#20390,.T.);
#43108=EDGE_CURVE('',#33071,#33349,#20391,.T.);
#43109=EDGE_CURVE('',#33349,#33319,#23871,.T.);
#43110=EDGE_CURVE('',#33350,#33071,#20392,.T.);
#43111=EDGE_CURVE('',#33216,#33350,#23872,.T.);
#43112=EDGE_CURVE('',#33072,#33350,#20393,.T.);
#43113=EDGE_CURVE('',#33351,#33072,#20394,.T.);
#43114=EDGE_CURVE('',#33220,#33351,#23873,.T.);
#43115=EDGE_CURVE('',#33073,#33351,#20395,.T.);
#43116=EDGE_CURVE('',#33352,#33073,#20396,.T.);
#43117=EDGE_CURVE('',#33224,#33352,#23874,.T.);
#43118=EDGE_CURVE('',#33074,#33352,#20397,.T.);
#43119=EDGE_CURVE('',#33353,#33074,#20398,.T.);
#43120=EDGE_CURVE('',#33228,#33353,#23875,.T.);
#43121=EDGE_CURVE('',#33075,#33353,#20399,.T.);
#43122=EDGE_CURVE('',#33354,#33075,#20400,.T.);
#43123=EDGE_CURVE('',#33232,#33354,#23876,.T.);
#43124=EDGE_CURVE('',#33076,#33354,#20401,.T.);
#43125=EDGE_CURVE('',#33355,#33076,#20402,.T.);
#43126=EDGE_CURVE('',#33236,#33355,#23877,.T.);
#43127=EDGE_CURVE('',#33077,#33355,#20403,.T.);
#43128=EDGE_CURVE('',#33356,#33077,#20404,.T.);
#43129=EDGE_CURVE('',#33240,#33356,#23878,.T.);
#43130=EDGE_CURVE('',#33078,#33356,#20405,.T.);
#43131=EDGE_CURVE('',#33357,#33078,#20406,.T.);
#43132=EDGE_CURVE('',#33244,#33357,#23879,.T.);
#43133=EDGE_CURVE('',#33079,#33357,#20407,.T.);
#43134=EDGE_CURVE('',#33358,#33079,#20408,.T.);
#43135=EDGE_CURVE('',#33248,#33358,#23880,.T.);
#43136=EDGE_CURVE('',#33080,#33358,#20409,.T.);
#43137=EDGE_CURVE('',#33359,#33080,#20410,.T.);
#43138=EDGE_CURVE('',#33252,#33359,#23881,.T.);
#43139=EDGE_CURVE('',#33081,#33359,#20411,.T.);
#43140=EDGE_CURVE('',#33360,#33081,#20412,.T.);
#43141=EDGE_CURVE('',#33256,#33360,#23882,.T.);
#43142=EDGE_CURVE('',#33082,#33360,#20413,.T.);
#43143=EDGE_CURVE('',#33361,#33082,#20414,.T.);
#43144=EDGE_CURVE('',#33260,#33361,#23883,.T.);
#43145=EDGE_CURVE('',#33083,#33361,#20415,.T.);
#43146=EDGE_CURVE('',#33362,#33083,#20416,.T.);
#43147=EDGE_CURVE('',#33264,#33362,#23884,.T.);
#43148=EDGE_CURVE('',#33084,#33362,#20417,.T.);
#43149=EDGE_CURVE('',#33363,#33084,#20418,.T.);
#43150=EDGE_CURVE('',#28917,#33363,#23885,.T.);
#43151=EDGE_CURVE('',#33085,#33363,#20419,.T.);
#43152=EDGE_CURVE('',#33364,#33085,#20420,.T.);
#43153=EDGE_CURVE('',#33268,#33364,#23886,.T.);
#43154=EDGE_CURVE('',#33086,#33364,#20421,.T.);
#43155=EDGE_CURVE('',#33365,#33086,#20422,.T.);
#43156=EDGE_CURVE('',#33272,#33365,#23887,.T.);
#43157=EDGE_CURVE('',#33087,#33365,#20423,.T.);
#43158=EDGE_CURVE('',#33366,#33087,#20424,.T.);
#43159=EDGE_CURVE('',#33276,#33366,#23888,.T.);
#43160=EDGE_CURVE('',#33088,#33366,#20425,.T.);
#43161=EDGE_CURVE('',#33367,#33088,#20426,.T.);
#43162=EDGE_CURVE('',#33280,#33367,#23889,.T.);
#43163=EDGE_CURVE('',#33089,#33367,#20427,.T.);
#43164=EDGE_CURVE('',#33368,#33089,#20428,.T.);
#43165=EDGE_CURVE('',#33284,#33368,#23890,.T.);
#43166=EDGE_CURVE('',#33090,#33368,#20429,.T.);
#43167=EDGE_CURVE('',#33369,#33090,#20430,.T.);
#43168=EDGE_CURVE('',#33288,#33369,#23891,.T.);
#43169=EDGE_CURVE('',#33091,#33369,#20431,.T.);
#43170=EDGE_CURVE('',#33370,#33091,#20432,.T.);
#43171=EDGE_CURVE('',#28913,#33370,#23892,.T.);
#43172=EDGE_CURVE('',#33092,#33370,#20433,.T.);
#43173=EDGE_CURVE('',#33371,#33092,#20434,.T.);
#43174=EDGE_CURVE('',#33292,#33371,#23893,.T.);
#43175=EDGE_CURVE('',#33093,#33371,#20435,.T.);
#43176=EDGE_CURVE('',#33372,#33093,#20436,.T.);
#43177=EDGE_CURVE('',#33296,#33372,#23894,.T.);
#43178=EDGE_CURVE('',#33094,#33372,#20437,.T.);
#43179=EDGE_CURVE('',#33373,#33094,#20438,.T.);
#43180=EDGE_CURVE('',#33300,#33373,#23895,.T.);
#43181=EDGE_CURVE('',#33095,#33373,#20439,.T.);
#43182=EDGE_CURVE('',#33374,#33095,#20440,.T.);
#43183=EDGE_CURVE('',#33304,#33374,#23896,.T.);
#43184=EDGE_CURVE('',#33096,#33374,#20441,.T.);
#43185=EDGE_CURVE('',#33375,#33096,#20442,.T.);
#43186=EDGE_CURVE('',#33308,#33375,#23897,.T.);
#43187=EDGE_CURVE('',#33097,#33375,#20443,.T.);
#43188=EDGE_CURVE('',#33376,#33097,#20444,.T.);
#43189=EDGE_CURVE('',#33312,#33376,#23898,.T.);
#43190=EDGE_CURVE('',#33098,#33376,#20445,.T.);
#43191=EDGE_CURVE('',#33377,#33098,#20446,.T.);
#43192=EDGE_CURVE('',#33316,#33377,#23899,.T.);
#43193=EDGE_CURVE('',#33099,#33377,#20447,.T.);
#43194=EDGE_CURVE('',#33349,#33099,#20448,.T.);
#43195=EDGE_CURVE('',#33378,#33379,#20449,.T.);
#43196=EDGE_CURVE('',#33042,#33379,#23900,.T.);
#43197=EDGE_CURVE('',#33378,#33320,#26104,.T.);
#43198=EDGE_CURVE('',#33380,#33378,#20450,.T.);
#43199=EDGE_CURVE('',#33381,#33380,#20451,.T.);
#43200=EDGE_CURVE('',#33379,#33381,#20452,.T.);
#43201=EDGE_CURVE('',#33321,#33381,#26105,.T.);
#43202=EDGE_CURVE('',#33382,#33383,#20453,.T.);
#43203=EDGE_CURVE('',#33043,#33383,#23901,.T.);
#43204=EDGE_CURVE('',#33382,#33321,#26106,.T.);
#43205=EDGE_CURVE('',#33384,#33382,#20454,.T.);
#43206=EDGE_CURVE('',#33385,#33384,#20455,.T.);
#43207=EDGE_CURVE('',#33383,#33385,#20456,.T.);
#43208=EDGE_CURVE('',#33322,#33385,#26107,.T.);
#43209=EDGE_CURVE('',#33386,#33387,#20457,.T.);
#43210=EDGE_CURVE('',#33044,#33387,#23902,.T.);
#43211=EDGE_CURVE('',#33386,#33322,#26108,.T.);
#43212=EDGE_CURVE('',#33388,#33386,#20458,.T.);
#43213=EDGE_CURVE('',#33389,#33388,#20459,.T.);
#43214=EDGE_CURVE('',#33387,#33389,#20460,.T.);
#43215=EDGE_CURVE('',#33323,#33389,#26109,.T.);
#43216=EDGE_CURVE('',#33390,#33391,#20461,.T.);
#43217=EDGE_CURVE('',#33045,#33391,#23903,.T.);
#43218=EDGE_CURVE('',#33390,#33323,#26110,.T.);
#43219=EDGE_CURVE('',#33392,#33390,#20462,.T.);
#43220=EDGE_CURVE('',#33393,#33392,#20463,.T.);
#43221=EDGE_CURVE('',#33391,#33393,#20464,.T.);
#43222=EDGE_CURVE('',#33324,#33393,#26111,.T.);
#43223=EDGE_CURVE('',#33394,#33395,#20465,.T.);
#43224=EDGE_CURVE('',#33046,#33395,#23904,.T.);
#43225=EDGE_CURVE('',#33394,#33324,#26112,.T.);
#43226=EDGE_CURVE('',#33396,#33394,#20466,.T.);
#43227=EDGE_CURVE('',#33397,#33396,#20467,.T.);
#43228=EDGE_CURVE('',#33395,#33397,#20468,.T.);
#43229=EDGE_CURVE('',#33325,#33397,#26113,.T.);
#43230=EDGE_CURVE('',#33398,#33399,#20469,.T.);
#43231=EDGE_CURVE('',#33047,#33399,#23905,.T.);
#43232=EDGE_CURVE('',#33398,#33325,#26114,.T.);
#43233=EDGE_CURVE('',#33400,#33398,#20470,.T.);
#43234=EDGE_CURVE('',#33401,#33400,#20471,.T.);
#43235=EDGE_CURVE('',#33399,#33401,#20472,.T.);
#43236=EDGE_CURVE('',#33326,#33401,#26115,.T.);
#43237=EDGE_CURVE('',#33402,#33403,#20473,.T.);
#43238=EDGE_CURVE('',#33048,#33403,#23906,.T.);
#43239=EDGE_CURVE('',#33402,#33326,#26116,.T.);
#43240=EDGE_CURVE('',#33404,#33402,#20474,.T.);
#43241=EDGE_CURVE('',#33405,#33404,#20475,.T.);
#43242=EDGE_CURVE('',#33403,#33405,#20476,.T.);
#43243=EDGE_CURVE('',#33327,#33405,#26117,.T.);
#43244=EDGE_CURVE('',#33406,#33407,#20477,.T.);
#43245=EDGE_CURVE('',#33049,#33407,#23907,.T.);
#43246=EDGE_CURVE('',#33406,#33327,#26118,.T.);
#43247=EDGE_CURVE('',#33408,#33406,#20478,.T.);
#43248=EDGE_CURVE('',#33409,#33408,#20479,.T.);
#43249=EDGE_CURVE('',#33407,#33409,#20480,.T.);
#43250=EDGE_CURVE('',#33328,#33409,#26119,.T.);
#43251=EDGE_CURVE('',#33410,#33411,#20481,.T.);
#43252=EDGE_CURVE('',#33050,#33411,#23908,.T.);
#43253=EDGE_CURVE('',#33410,#33328,#26120,.T.);
#43254=EDGE_CURVE('',#33412,#33410,#20482,.T.);
#43255=EDGE_CURVE('',#33413,#33412,#20483,.T.);
#43256=EDGE_CURVE('',#33411,#33413,#20484,.T.);
#43257=EDGE_CURVE('',#33329,#33413,#26121,.T.);
#43258=EDGE_CURVE('',#33414,#33415,#20485,.T.);
#43259=EDGE_CURVE('',#33051,#33415,#23909,.T.);
#43260=EDGE_CURVE('',#33414,#33329,#26122,.T.);
#43261=EDGE_CURVE('',#33416,#33414,#20486,.T.);
#43262=EDGE_CURVE('',#33417,#33416,#20487,.T.);
#43263=EDGE_CURVE('',#33415,#33417,#20488,.T.);
#43264=EDGE_CURVE('',#33330,#33417,#26123,.T.);
#43265=EDGE_CURVE('',#33418,#33419,#20489,.T.);
#43266=EDGE_CURVE('',#33052,#33419,#23910,.T.);
#43267=EDGE_CURVE('',#33418,#33330,#26124,.T.);
#43268=EDGE_CURVE('',#33420,#33418,#20490,.T.);
#43269=EDGE_CURVE('',#33421,#33420,#20491,.T.);
#43270=EDGE_CURVE('',#33419,#33421,#20492,.T.);
#43271=EDGE_CURVE('',#33331,#33421,#26125,.T.);
#43272=EDGE_CURVE('',#33422,#33423,#20493,.T.);
#43273=EDGE_CURVE('',#33053,#33423,#23911,.T.);
#43274=EDGE_CURVE('',#33422,#33331,#26126,.T.);
#43275=EDGE_CURVE('',#33424,#33422,#20494,.T.);
#43276=EDGE_CURVE('',#33425,#33424,#20495,.T.);
#43277=EDGE_CURVE('',#33423,#33425,#20496,.T.);
#43278=EDGE_CURVE('',#33332,#33425,#26127,.T.);
#43279=EDGE_CURVE('',#33426,#33427,#20497,.T.);
#43280=EDGE_CURVE('',#33054,#33427,#23912,.T.);
#43281=EDGE_CURVE('',#33426,#33332,#26128,.T.);
#43282=EDGE_CURVE('',#33428,#33426,#20498,.T.);
#43283=EDGE_CURVE('',#33429,#33428,#20499,.T.);
#43284=EDGE_CURVE('',#33427,#33429,#20500,.T.);
#43285=EDGE_CURVE('',#33333,#33429,#26129,.T.);
#43286=EDGE_CURVE('',#33430,#33431,#20501,.T.);
#43287=EDGE_CURVE('',#33055,#33431,#23913,.T.);
#43288=EDGE_CURVE('',#33430,#33333,#26130,.T.);
#43289=EDGE_CURVE('',#33432,#33430,#20502,.T.);
#43290=EDGE_CURVE('',#33433,#33432,#20503,.T.);
#43291=EDGE_CURVE('',#33431,#33433,#20504,.T.);
#43292=EDGE_CURVE('',#33334,#33433,#26131,.T.);
#43293=EDGE_CURVE('',#33056,#28909,#23914,.T.);
#43294=EDGE_CURVE('',#28908,#33334,#26132,.T.);
#43295=EDGE_CURVE('',#33335,#28911,#26133,.T.);
#43296=EDGE_CURVE('',#33434,#33435,#20505,.T.);
#43297=EDGE_CURVE('',#33057,#33435,#23915,.T.);
#43298=EDGE_CURVE('',#33434,#33335,#26134,.T.);
#43299=EDGE_CURVE('',#33436,#33434,#20506,.T.);
#43300=EDGE_CURVE('',#33437,#33436,#20507,.T.);
#43301=EDGE_CURVE('',#33435,#33437,#20508,.T.);
#43302=EDGE_CURVE('',#33336,#33437,#26135,.T.);
#43303=EDGE_CURVE('',#33438,#33439,#20509,.T.);
#43304=EDGE_CURVE('',#33058,#33439,#23916,.T.);
#43305=EDGE_CURVE('',#33438,#33336,#26136,.T.);
#43306=EDGE_CURVE('',#33440,#33438,#20510,.T.);
#43307=EDGE_CURVE('',#33441,#33440,#20511,.T.);
#43308=EDGE_CURVE('',#33439,#33441,#20512,.T.);
#43309=EDGE_CURVE('',#33337,#33441,#26137,.T.);
#43310=EDGE_CURVE('',#33442,#33443,#20513,.T.);
#43311=EDGE_CURVE('',#33059,#33443,#23917,.T.);
#43312=EDGE_CURVE('',#33442,#33337,#26138,.T.);
#43313=EDGE_CURVE('',#33443,#33444,#20514,.T.);
#43314=EDGE_CURVE('',#33338,#33444,#26139,.T.);
#43315=EDGE_CURVE('',#33445,#33442,#20515,.T.);
#43316=EDGE_CURVE('',#33444,#33445,#20516,.T.);
#43317=EDGE_CURVE('',#33446,#33338,#26140,.T.);
#43318=EDGE_CURVE('',#33446,#33447,#20517,.T.);
#43319=EDGE_CURVE('',#33060,#33447,#23918,.T.);
#43320=EDGE_CURVE('',#33447,#33448,#20518,.T.);
#43321=EDGE_CURVE('',#33449,#33446,#20519,.T.);
#43322=EDGE_CURVE('',#33448,#33449,#20520,.T.);
#43323=EDGE_CURVE('',#33339,#33448,#26141,.T.);
#43324=EDGE_CURVE('',#33450,#33451,#20521,.T.);
#43325=EDGE_CURVE('',#33061,#33451,#23919,.T.);
#43326=EDGE_CURVE('',#33450,#33339,#26142,.T.);
#43327=EDGE_CURVE('',#33452,#33450,#20522,.T.);
#43328=EDGE_CURVE('',#33453,#33452,#20523,.T.);
#43329=EDGE_CURVE('',#33451,#33453,#20524,.T.);
#43330=EDGE_CURVE('',#33340,#33453,#26143,.T.);
#43331=EDGE_CURVE('',#33454,#33455,#20525,.T.);
#43332=EDGE_CURVE('',#33062,#33455,#23920,.T.);
#43333=EDGE_CURVE('',#33454,#33340,#26144,.T.);
#43334=EDGE_CURVE('',#33456,#33454,#20526,.T.);
#43335=EDGE_CURVE('',#33457,#33456,#20527,.T.);
#43336=EDGE_CURVE('',#33455,#33457,#20528,.T.);
#43337=EDGE_CURVE('',#33341,#33457,#26145,.T.);
#43338=EDGE_CURVE('',#33458,#33459,#20529,.T.);
#43339=EDGE_CURVE('',#33063,#33459,#23921,.T.);
#43340=EDGE_CURVE('',#33458,#33341,#26146,.T.);
#43341=EDGE_CURVE('',#33460,#33458,#20530,.T.);
#43342=EDGE_CURVE('',#33461,#33460,#20531,.T.);
#43343=EDGE_CURVE('',#33459,#33461,#20532,.T.);
#43344=EDGE_CURVE('',#33342,#33461,#26147,.T.);
#43345=EDGE_CURVE('',#33462,#33463,#20533,.T.);
#43346=EDGE_CURVE('',#33064,#33463,#23922,.T.);
#43347=EDGE_CURVE('',#33462,#33342,#26148,.T.);
#43348=EDGE_CURVE('',#33464,#33462,#20534,.T.);
#43349=EDGE_CURVE('',#33465,#33464,#20535,.T.);
#43350=EDGE_CURVE('',#33463,#33465,#20536,.T.);
#43351=EDGE_CURVE('',#33343,#33465,#26149,.T.);
#43352=EDGE_CURVE('',#33466,#33467,#20537,.T.);
#43353=EDGE_CURVE('',#33065,#33467,#23923,.T.);
#43354=EDGE_CURVE('',#33466,#33343,#26150,.T.);
#43355=EDGE_CURVE('',#33468,#33466,#20538,.T.);
#43356=EDGE_CURVE('',#33469,#33468,#20539,.T.);
#43357=EDGE_CURVE('',#33467,#33469,#20540,.T.);
#43358=EDGE_CURVE('',#33344,#33469,#26151,.T.);
#43359=EDGE_CURVE('',#33470,#33471,#20541,.T.);
#43360=EDGE_CURVE('',#33066,#33471,#23924,.T.);
#43361=EDGE_CURVE('',#33470,#33344,#26152,.T.);
#43362=EDGE_CURVE('',#33472,#33470,#20542,.T.);
#43363=EDGE_CURVE('',#33473,#33472,#20543,.T.);
#43364=EDGE_CURVE('',#33471,#33473,#20544,.T.);
#43365=EDGE_CURVE('',#33345,#33473,#26153,.T.);
#43366=EDGE_CURVE('',#33474,#33475,#20545,.T.);
#43367=EDGE_CURVE('',#33067,#33475,#23925,.T.);
#43368=EDGE_CURVE('',#33474,#33345,#26154,.T.);
#43369=EDGE_CURVE('',#33476,#33474,#20546,.T.);
#43370=EDGE_CURVE('',#33477,#33476,#20547,.T.);
#43371=EDGE_CURVE('',#33475,#33477,#20548,.T.);
#43372=EDGE_CURVE('',#33346,#33477,#26155,.T.);
#43373=EDGE_CURVE('',#33478,#33479,#20549,.T.);
#43374=EDGE_CURVE('',#33068,#33479,#23926,.T.);
#43375=EDGE_CURVE('',#33478,#33346,#26156,.T.);
#43376=EDGE_CURVE('',#33480,#33478,#20550,.T.);
#43377=EDGE_CURVE('',#33481,#33480,#20551,.T.);
#43378=EDGE_CURVE('',#33479,#33481,#20552,.T.);
#43379=EDGE_CURVE('',#33347,#33481,#26157,.T.);
#43380=EDGE_CURVE('',#33482,#33483,#20553,.T.);
#43381=EDGE_CURVE('',#33069,#33483,#23927,.T.);
#43382=EDGE_CURVE('',#33482,#33347,#26158,.T.);
#43383=EDGE_CURVE('',#33484,#33482,#20554,.T.);
#43384=EDGE_CURVE('',#33485,#33484,#20555,.T.);
#43385=EDGE_CURVE('',#33483,#33485,#20556,.T.);
#43386=EDGE_CURVE('',#33348,#33485,#26159,.T.);
#43387=EDGE_CURVE('',#33486,#33487,#20557,.T.);
#43388=EDGE_CURVE('',#33070,#33487,#23928,.T.);
#43389=EDGE_CURVE('',#33486,#33348,#26160,.T.);
#43390=EDGE_CURVE('',#33488,#33486,#20558,.T.);
#43391=EDGE_CURVE('',#33489,#33488,#20559,.T.);
#43392=EDGE_CURVE('',#33487,#33489,#20560,.T.);
#43393=EDGE_CURVE('',#33320,#33489,#26161,.T.);
#43394=EDGE_CURVE('',#33349,#28805,#20561,.T.);
#43395=EDGE_CURVE('',#28806,#33349,#26162,.T.);
#43396=EDGE_CURVE('',#33349,#28804,#23929,.T.);
#43397=EDGE_CURVE('',#33349,#28803,#23930,.T.);
#43398=EDGE_CURVE('',#33349,#28802,#26163,.T.);
#43399=EDGE_CURVE('',#33071,#28801,#23931,.T.);
#43400=EDGE_CURVE('',#33350,#28800,#26164,.T.);
#43401=EDGE_CURVE('',#33350,#28799,#20562,.T.);
#43402=EDGE_CURVE('',#33350,#28798,#23932,.T.);
#43403=EDGE_CURVE('',#33350,#28797,#23933,.T.);
#43404=EDGE_CURVE('',#33350,#28796,#26165,.T.);
#43405=EDGE_CURVE('',#33072,#28795,#23934,.T.);
#43406=EDGE_CURVE('',#33351,#28794,#26166,.T.);
#43407=EDGE_CURVE('',#33351,#28793,#20563,.T.);
#43408=EDGE_CURVE('',#33351,#28792,#23935,.T.);
#43409=EDGE_CURVE('',#33351,#28791,#23936,.T.);
#43410=EDGE_CURVE('',#33351,#28790,#26167,.T.);
#43411=EDGE_CURVE('',#33073,#28789,#23937,.T.);
#43412=EDGE_CURVE('',#33352,#28788,#26168,.T.);
#43413=EDGE_CURVE('',#33352,#28787,#20564,.T.);
#43414=EDGE_CURVE('',#33352,#28786,#23938,.T.);
#43415=EDGE_CURVE('',#33352,#28785,#23939,.T.);
#43416=EDGE_CURVE('',#33352,#28784,#26169,.T.);
#43417=EDGE_CURVE('',#33074,#28783,#23940,.T.);
#43418=EDGE_CURVE('',#33353,#28782,#26170,.T.);
#43419=EDGE_CURVE('',#33353,#28781,#20565,.T.);
#43420=EDGE_CURVE('',#33353,#28780,#23941,.T.);
#43421=EDGE_CURVE('',#33353,#28779,#4456,.T.);
#43422=EDGE_CURVE('',#33353,#28778,#26171,.T.);
#43423=EDGE_CURVE('',#33075,#28777,#23942,.T.);
#43424=EDGE_CURVE('',#33354,#28776,#26172,.T.);
#43425=EDGE_CURVE('',#33354,#28775,#20566,.T.);
#43426=EDGE_CURVE('',#33354,#28774,#23943,.T.);
#43427=EDGE_CURVE('',#33354,#28773,#23944,.T.);
#43428=EDGE_CURVE('',#33354,#28772,#26173,.T.);
#43429=EDGE_CURVE('',#33076,#28771,#23945,.T.);
#43430=EDGE_CURVE('',#33355,#28770,#26174,.T.);
#43431=EDGE_CURVE('',#33355,#28769,#20567,.T.);
#43432=EDGE_CURVE('',#33355,#28768,#23946,.T.);
#43433=EDGE_CURVE('',#33355,#28767,#23947,.T.);
#43434=EDGE_CURVE('',#33355,#28766,#26175,.T.);
#43435=EDGE_CURVE('',#33077,#28765,#23948,.T.);
#43436=EDGE_CURVE('',#33356,#28764,#26176,.T.);
#43437=EDGE_CURVE('',#33356,#28763,#20568,.T.);
#43438=EDGE_CURVE('',#33356,#28762,#23949,.T.);
#43439=EDGE_CURVE('',#33356,#28761,#23950,.T.);
#43440=EDGE_CURVE('',#33356,#28760,#26177,.T.);
#43441=EDGE_CURVE('',#33078,#28759,#23951,.T.);
#43442=EDGE_CURVE('',#33357,#28758,#26178,.T.);
#43443=EDGE_CURVE('',#33357,#28757,#20569,.T.);
#43444=EDGE_CURVE('',#33357,#28756,#23952,.T.);
#43445=EDGE_CURVE('',#33357,#28755,#23953,.T.);
#43446=EDGE_CURVE('',#33357,#28754,#26179,.T.);
#43447=EDGE_CURVE('',#33079,#28753,#23954,.T.);
#43448=EDGE_CURVE('',#33358,#28752,#26180,.T.);
#43449=EDGE_CURVE('',#33358,#28751,#20570,.T.);
#43450=EDGE_CURVE('',#33358,#28750,#23955,.T.);
#43451=EDGE_CURVE('',#33358,#28749,#23956,.T.);
#43452=EDGE_CURVE('',#33358,#28748,#26181,.T.);
#43453=EDGE_CURVE('',#33080,#28747,#23957,.T.);
#43454=EDGE_CURVE('',#33359,#28746,#26182,.T.);
#43455=EDGE_CURVE('',#33359,#28745,#20571,.T.);
#43456=EDGE_CURVE('',#33359,#28744,#23958,.T.);
#43457=EDGE_CURVE('',#33359,#28743,#23959,.T.);
#43458=EDGE_CURVE('',#33359,#28742,#26183,.T.);
#43459=EDGE_CURVE('',#33081,#28741,#23960,.T.);
#43460=EDGE_CURVE('',#33360,#28740,#26184,.T.);
#43461=EDGE_CURVE('',#33360,#28739,#20572,.T.);
#43462=EDGE_CURVE('',#33360,#28738,#23961,.T.);
#43463=EDGE_CURVE('',#33360,#28737,#23962,.T.);
#43464=EDGE_CURVE('',#33360,#28736,#26185,.T.);
#43465=EDGE_CURVE('',#33082,#28735,#23963,.T.);
#43466=EDGE_CURVE('',#33361,#28734,#26186,.T.);
#43467=EDGE_CURVE('',#33361,#28733,#20573,.T.);
#43468=EDGE_CURVE('',#33361,#28732,#23964,.T.);
#43469=EDGE_CURVE('',#33361,#28731,#23965,.T.);
#43470=EDGE_CURVE('',#33361,#28730,#26187,.T.);
#43471=EDGE_CURVE('',#33083,#28729,#23966,.T.);
#43472=EDGE_CURVE('',#33362,#28728,#26188,.T.);
#43473=EDGE_CURVE('',#33362,#28727,#20574,.T.);
#43474=EDGE_CURVE('',#33362,#28726,#23967,.T.);
#43475=EDGE_CURVE('',#33362,#28725,#23968,.T.);
#43476=EDGE_CURVE('',#33362,#28724,#26189,.T.);
#43477=EDGE_CURVE('',#33084,#28723,#23969,.T.);
#43478=EDGE_CURVE('',#33363,#28722,#26190,.T.);
#43479=EDGE_CURVE('',#33363,#28721,#20575,.T.);
#43480=EDGE_CURVE('',#33363,#28719,#23970,.T.);
#43481=EDGE_CURVE('',#33363,#28720,#23971,.T.);
#43482=EDGE_CURVE('',#33363,#28894,#26191,.T.);
#43483=EDGE_CURVE('',#33085,#28893,#23972,.T.);
#43484=EDGE_CURVE('',#33364,#28892,#26192,.T.);
#43485=EDGE_CURVE('',#33364,#28891,#20576,.T.);
#43486=EDGE_CURVE('',#33364,#28890,#23973,.T.);
#43487=EDGE_CURVE('',#33364,#28889,#23974,.T.);
#43488=EDGE_CURVE('',#33364,#28888,#26193,.T.);
#43489=EDGE_CURVE('',#33086,#28887,#23975,.T.);
#43490=EDGE_CURVE('',#33365,#28886,#26194,.T.);
#43491=EDGE_CURVE('',#33365,#28885,#20577,.T.);
#43492=EDGE_CURVE('',#33365,#28884,#23976,.T.);
#43493=EDGE_CURVE('',#33365,#28883,#23977,.T.);
#43494=EDGE_CURVE('',#33365,#28882,#26195,.T.);
#43495=EDGE_CURVE('',#33087,#28881,#23978,.T.);
#43496=EDGE_CURVE('',#33366,#28880,#26196,.T.);
#43497=EDGE_CURVE('',#33366,#28879,#20578,.T.);
#43498=EDGE_CURVE('',#33366,#28878,#23979,.T.);
#43499=EDGE_CURVE('',#33366,#28877,#23980,.T.);
#43500=EDGE_CURVE('',#33366,#28876,#26197,.T.);
#43501=EDGE_CURVE('',#33088,#28875,#23981,.T.);
#43502=EDGE_CURVE('',#33367,#28874,#26198,.T.);
#43503=EDGE_CURVE('',#33367,#28873,#20579,.T.);
#43504=EDGE_CURVE('',#33367,#28872,#23982,.T.);
#43505=EDGE_CURVE('',#33367,#28871,#23983,.T.);
#43506=EDGE_CURVE('',#33367,#28870,#26199,.T.);
#43507=EDGE_CURVE('',#33089,#28869,#23984,.T.);
#43508=EDGE_CURVE('',#33368,#28868,#26200,.T.);
#43509=EDGE_CURVE('',#33368,#28867,#20580,.T.);
#43510=EDGE_CURVE('',#33368,#28866,#23985,.T.);
#43511=EDGE_CURVE('',#33368,#28865,#23986,.T.);
#43512=EDGE_CURVE('',#33368,#28864,#26201,.T.);
#43513=EDGE_CURVE('',#33090,#28863,#23987,.T.);
#43514=EDGE_CURVE('',#33369,#28862,#26202,.T.);
#43515=EDGE_CURVE('',#33369,#28861,#20581,.T.);
#43516=EDGE_CURVE('',#33369,#28860,#23988,.T.);
#43517=EDGE_CURVE('',#33369,#28859,#23989,.T.);
#43518=EDGE_CURVE('',#33369,#28858,#26203,.T.);
#43519=EDGE_CURVE('',#33091,#28857,#23990,.T.);
#43520=EDGE_CURVE('',#33370,#28856,#26204,.T.);
#43521=EDGE_CURVE('',#33370,#28855,#20582,.T.);
#43522=EDGE_CURVE('',#33370,#28854,#23991,.T.);
#43523=EDGE_CURVE('',#33370,#28853,#23992,.T.);
#43524=EDGE_CURVE('',#33370,#28852,#26205,.T.);
#43525=EDGE_CURVE('',#33092,#28851,#23993,.T.);
#43526=EDGE_CURVE('',#33371,#28850,#26206,.T.);
#43527=EDGE_CURVE('',#33371,#28849,#20583,.T.);
#43528=EDGE_CURVE('',#33371,#28848,#23994,.T.);
#43529=EDGE_CURVE('',#33371,#28847,#23995,.T.);
#43530=EDGE_CURVE('',#33371,#28846,#26207,.T.);
#43531=EDGE_CURVE('',#33093,#28845,#23996,.T.);
#43532=EDGE_CURVE('',#33372,#28844,#26208,.T.);
#43533=EDGE_CURVE('',#33372,#28843,#20584,.T.);
#43534=EDGE_CURVE('',#33372,#28842,#23997,.T.);
#43535=EDGE_CURVE('',#33372,#28841,#23998,.T.);
#43536=EDGE_CURVE('',#33372,#28840,#26209,.T.);
#43537=EDGE_CURVE('',#33094,#28839,#23999,.T.);
#43538=EDGE_CURVE('',#33373,#28838,#26210,.T.);
#43539=EDGE_CURVE('',#33373,#28837,#20585,.T.);
#43540=EDGE_CURVE('',#33373,#28836,#24000,.T.);
#43541=EDGE_CURVE('',#33373,#28835,#24001,.T.);
#43542=EDGE_CURVE('',#33373,#28834,#26211,.T.);
#43543=EDGE_CURVE('',#33095,#28833,#24002,.T.);
#43544=EDGE_CURVE('',#33374,#28832,#26212,.T.);
#43545=EDGE_CURVE('',#33374,#28831,#20586,.T.);
#43546=EDGE_CURVE('',#33374,#28830,#24003,.T.);
#43547=EDGE_CURVE('',#33374,#28829,#24004,.T.);
#43548=EDGE_CURVE('',#33374,#28828,#26213,.T.);
#43549=EDGE_CURVE('',#33096,#28827,#24005,.T.);
#43550=EDGE_CURVE('',#33375,#28826,#26214,.T.);
#43551=EDGE_CURVE('',#33375,#28825,#20587,.T.);
#43552=EDGE_CURVE('',#33375,#28824,#24006,.T.);
#43553=EDGE_CURVE('',#33375,#28823,#24007,.T.);
#43554=EDGE_CURVE('',#33375,#28822,#26215,.T.);
#43555=EDGE_CURVE('',#33097,#28821,#24008,.T.);
#43556=EDGE_CURVE('',#33376,#28820,#26216,.T.);
#43557=EDGE_CURVE('',#33376,#28819,#20588,.T.);
#43558=EDGE_CURVE('',#33376,#28818,#24009,.T.);
#43559=EDGE_CURVE('',#33376,#28817,#24010,.T.);
#43560=EDGE_CURVE('',#33376,#28816,#26217,.T.);
#43561=EDGE_CURVE('',#33098,#28815,#24011,.T.);
#43562=EDGE_CURVE('',#33377,#28814,#26218,.T.);
#43563=EDGE_CURVE('',#33377,#28813,#20589,.T.);
#43564=EDGE_CURVE('',#33377,#28812,#24012,.T.);
#43565=EDGE_CURVE('',#33377,#28811,#24013,.T.);
#43566=EDGE_CURVE('',#33377,#28810,#26219,.T.);
#43567=EDGE_CURVE('',#33099,#28809,#24014,.T.);
#43568=EDGE_CURVE('',#33490,#33320,#20590,.T.);
#43569=EDGE_CURVE('',#33380,#33490,#24015,.T.);
#43570=EDGE_CURVE('',#33321,#33490,#20591,.T.);
#43571=EDGE_CURVE('',#33491,#33321,#20592,.T.);
#43572=EDGE_CURVE('',#33384,#33491,#24016,.T.);
#43573=EDGE_CURVE('',#33322,#33491,#20593,.T.);
#43574=EDGE_CURVE('',#33492,#33322,#20594,.T.);
#43575=EDGE_CURVE('',#33388,#33492,#24017,.T.);
#43576=EDGE_CURVE('',#33323,#33492,#20595,.T.);
#43577=EDGE_CURVE('',#33493,#33323,#20596,.T.);
#43578=EDGE_CURVE('',#33392,#33493,#24018,.T.);
#43579=EDGE_CURVE('',#33324,#33493,#20597,.T.);
#43580=EDGE_CURVE('',#33494,#33324,#20598,.T.);
#43581=EDGE_CURVE('',#33396,#33494,#24019,.T.);
#43582=EDGE_CURVE('',#33325,#33494,#20599,.T.);
#43583=EDGE_CURVE('',#33495,#33325,#20600,.T.);
#43584=EDGE_CURVE('',#33400,#33495,#24020,.T.);
#43585=EDGE_CURVE('',#33326,#33495,#20601,.T.);
#43586=EDGE_CURVE('',#33496,#33326,#20602,.T.);
#43587=EDGE_CURVE('',#33404,#33496,#24021,.T.);
#43588=EDGE_CURVE('',#33327,#33496,#20603,.T.);
#43589=EDGE_CURVE('',#33497,#33327,#20604,.T.);
#43590=EDGE_CURVE('',#33408,#33497,#24022,.T.);
#43591=EDGE_CURVE('',#33328,#33497,#20605,.T.);
#43592=EDGE_CURVE('',#33498,#33328,#20606,.T.);
#43593=EDGE_CURVE('',#33412,#33498,#24023,.T.);
#43594=EDGE_CURVE('',#33329,#33498,#20607,.T.);
#43595=EDGE_CURVE('',#33499,#33329,#20608,.T.);
#43596=EDGE_CURVE('',#33416,#33499,#24024,.T.);
#43597=EDGE_CURVE('',#33330,#33499,#20609,.T.);
#43598=EDGE_CURVE('',#33500,#33330,#20610,.T.);
#43599=EDGE_CURVE('',#33420,#33500,#24025,.T.);
#43600=EDGE_CURVE('',#33331,#33500,#20611,.T.);
#43601=EDGE_CURVE('',#33501,#33331,#20612,.T.);
#43602=EDGE_CURVE('',#33424,#33501,#24026,.T.);
#43603=EDGE_CURVE('',#33332,#33501,#20613,.T.);
#43604=EDGE_CURVE('',#33502,#33332,#20614,.T.);
#43605=EDGE_CURVE('',#33428,#33502,#24027,.T.);
#43606=EDGE_CURVE('',#33333,#33502,#20615,.T.);
#43607=EDGE_CURVE('',#33503,#33333,#20616,.T.);
#43608=EDGE_CURVE('',#33432,#33503,#24028,.T.);
#43609=EDGE_CURVE('',#33334,#33503,#20617,.T.);
#43610=EDGE_CURVE('',#33504,#33334,#20618,.T.);
#43611=EDGE_CURVE('',#28910,#33504,#24029,.T.);
#43612=EDGE_CURVE('',#33335,#33504,#20619,.T.);
#43613=EDGE_CURVE('',#33505,#33335,#20620,.T.);
#43614=EDGE_CURVE('',#33436,#33505,#24030,.T.);
#43615=EDGE_CURVE('',#33336,#33505,#20621,.T.);
#43616=EDGE_CURVE('',#33506,#33336,#20622,.T.);
#43617=EDGE_CURVE('',#33440,#33506,#24031,.T.);
#43618=EDGE_CURVE('',#33337,#33506,#20623,.T.);
#43619=EDGE_CURVE('',#33507,#33337,#20624,.T.);
#43620=EDGE_CURVE('',#33445,#33507,#24032,.T.);
#43621=EDGE_CURVE('',#33338,#33507,#20625,.T.);
#43622=EDGE_CURVE('',#33508,#33338,#20626,.T.);
#43623=EDGE_CURVE('',#33449,#33508,#24033,.T.);
#43624=EDGE_CURVE('',#33339,#33508,#20627,.T.);
#43625=EDGE_CURVE('',#33509,#33339,#20628,.T.);
#43626=EDGE_CURVE('',#33452,#33509,#24034,.T.);
#43627=EDGE_CURVE('',#33340,#33509,#20629,.T.);
#43628=EDGE_CURVE('',#33510,#33340,#20630,.T.);
#43629=EDGE_CURVE('',#33456,#33510,#24035,.T.);
#43630=EDGE_CURVE('',#33341,#33510,#20631,.T.);
#43631=EDGE_CURVE('',#33511,#33341,#20632,.T.);
#43632=EDGE_CURVE('',#33460,#33511,#24036,.T.);
#43633=EDGE_CURVE('',#33342,#33511,#20633,.T.);
#43634=EDGE_CURVE('',#33512,#33342,#20634,.T.);
#43635=EDGE_CURVE('',#33464,#33512,#24037,.T.);
#43636=EDGE_CURVE('',#33343,#33512,#20635,.T.);
#43637=EDGE_CURVE('',#33513,#33343,#20636,.T.);
#43638=EDGE_CURVE('',#33468,#33513,#24038,.T.);
#43639=EDGE_CURVE('',#33344,#33513,#20637,.T.);
#43640=EDGE_CURVE('',#33514,#33344,#20638,.T.);
#43641=EDGE_CURVE('',#33472,#33514,#24039,.T.);
#43642=EDGE_CURVE('',#33345,#33514,#20639,.T.);
#43643=EDGE_CURVE('',#33515,#33345,#20640,.T.);
#43644=EDGE_CURVE('',#33476,#33515,#24040,.T.);
#43645=EDGE_CURVE('',#33346,#33515,#20641,.T.);
#43646=EDGE_CURVE('',#33516,#33346,#20642,.T.);
#43647=EDGE_CURVE('',#33480,#33516,#24041,.T.);
#43648=EDGE_CURVE('',#33347,#33516,#20643,.T.);
#43649=EDGE_CURVE('',#33517,#33347,#20644,.T.);
#43650=EDGE_CURVE('',#33484,#33517,#24042,.T.);
#43651=EDGE_CURVE('',#33348,#33517,#20645,.T.);
#43652=EDGE_CURVE('',#33518,#33348,#20646,.T.);
#43653=EDGE_CURVE('',#33488,#33518,#24043,.T.);
#43654=EDGE_CURVE('',#33320,#33518,#20647,.T.);
#43655=EDGE_CURVE('',#33519,#33520,#20648,.T.);
#43656=EDGE_CURVE('',#33490,#33520,#26220,.T.);
#43657=EDGE_CURVE('',#33519,#33320,#24044,.T.);
#43658=EDGE_CURVE('',#33521,#33522,#20649,.T.);
#43659=EDGE_CURVE('',#33321,#33522,#24045,.T.);
#43660=EDGE_CURVE('',#33521,#33490,#26221,.T.);
#43661=EDGE_CURVE('',#33523,#33524,#20650,.T.);
#43662=EDGE_CURVE('',#33523,#33525,#20651,.T.);
#43663=EDGE_CURVE('',#33524,#33525,#20652,.T.);
#43664=EDGE_CURVE('',#33522,#33526,#20653,.T.);
#43665=EDGE_CURVE('',#33491,#33526,#26222,.T.);
#43666=EDGE_CURVE('',#33526,#33523,#20654,.T.);
#43667=EDGE_CURVE('',#33525,#33521,#20655,.T.);
#43668=EDGE_CURVE('',#33527,#33528,#20656,.T.);
#43669=EDGE_CURVE('',#33322,#33528,#24046,.T.);
#43670=EDGE_CURVE('',#33527,#33491,#26223,.T.);
#43671=EDGE_CURVE('',#33529,#33530,#20657,.T.);
#43672=EDGE_CURVE('',#33529,#33531,#20658,.T.);
#43673=EDGE_CURVE('',#33530,#33531,#20659,.T.);
#43674=EDGE_CURVE('',#33528,#33532,#20660,.T.);
#43675=EDGE_CURVE('',#33492,#33532,#26224,.T.);
#43676=EDGE_CURVE('',#33532,#33529,#20661,.T.);
#43677=EDGE_CURVE('',#33531,#33527,#20662,.T.);
#43678=EDGE_CURVE('',#33533,#33534,#20663,.T.);
#43679=EDGE_CURVE('',#33323,#33534,#24047,.T.);
#43680=EDGE_CURVE('',#33533,#33492,#26225,.T.);
#43681=EDGE_CURVE('',#33535,#33536,#20664,.T.);
#43682=EDGE_CURVE('',#33535,#33537,#20665,.T.);
#43683=EDGE_CURVE('',#33536,#33537,#20666,.T.);
#43684=EDGE_CURVE('',#33534,#33538,#20667,.T.);
#43685=EDGE_CURVE('',#33493,#33538,#26226,.T.);
#43686=EDGE_CURVE('',#33538,#33535,#20668,.T.);
#43687=EDGE_CURVE('',#33537,#33533,#20669,.T.);
#43688=EDGE_CURVE('',#33539,#33540,#20670,.T.);
#43689=EDGE_CURVE('',#33324,#33540,#24048,.T.);
#43690=EDGE_CURVE('',#33539,#33493,#26227,.T.);
#43691=EDGE_CURVE('',#33541,#33542,#20671,.T.);
#43692=EDGE_CURVE('',#33541,#33543,#20672,.T.);
#43693=EDGE_CURVE('',#33542,#33543,#20673,.T.);
#43694=EDGE_CURVE('',#33540,#33544,#20674,.T.);
#43695=EDGE_CURVE('',#33494,#33544,#26228,.T.);
#43696=EDGE_CURVE('',#33544,#33541,#20675,.T.);
#43697=EDGE_CURVE('',#33543,#33539,#20676,.T.);
#43698=EDGE_CURVE('',#33545,#33546,#20677,.T.);
#43699=EDGE_CURVE('',#33325,#33546,#24049,.T.);
#43700=EDGE_CURVE('',#33545,#33494,#26229,.T.);
#43701=EDGE_CURVE('',#33547,#33548,#20678,.T.);
#43702=EDGE_CURVE('',#33547,#33549,#20679,.T.);
#43703=EDGE_CURVE('',#33548,#33549,#20680,.T.);
#43704=EDGE_CURVE('',#33546,#33550,#20681,.T.);
#43705=EDGE_CURVE('',#33495,#33550,#26230,.T.);
#43706=EDGE_CURVE('',#33550,#33547,#20682,.T.);
#43707=EDGE_CURVE('',#33549,#33545,#20683,.T.);
#43708=EDGE_CURVE('',#33551,#33552,#20684,.T.);
#43709=EDGE_CURVE('',#33326,#33552,#24050,.T.);
#43710=EDGE_CURVE('',#33551,#33495,#26231,.T.);
#43711=EDGE_CURVE('',#33553,#33554,#20685,.T.);
#43712=EDGE_CURVE('',#33553,#33555,#20686,.T.);
#43713=EDGE_CURVE('',#33554,#33555,#20687,.T.);
#43714=EDGE_CURVE('',#33552,#33556,#20688,.T.);
#43715=EDGE_CURVE('',#33496,#33556,#26232,.T.);
#43716=EDGE_CURVE('',#33556,#33553,#20689,.T.);
#43717=EDGE_CURVE('',#33555,#33551,#20690,.T.);
#43718=EDGE_CURVE('',#33327,#28903,#24051,.T.);
#43719=EDGE_CURVE('',#28905,#33496,#26233,.T.);
#43720=EDGE_CURVE('',#28907,#33557,#20691,.T.);
#43721=EDGE_CURVE('',#33557,#28906,#20692,.T.);
#43722=EDGE_CURVE('',#33497,#28904,#26234,.T.);
#43723=EDGE_CURVE('',#33558,#33559,#20693,.T.);
#43724=EDGE_CURVE('',#33328,#33559,#24052,.T.);
#43725=EDGE_CURVE('',#33558,#33497,#26235,.T.);
#43726=EDGE_CURVE('',#33560,#33561,#20694,.T.);
#43727=EDGE_CURVE('',#33560,#33562,#20695,.T.);
#43728=EDGE_CURVE('',#33561,#33562,#20696,.T.);
#43729=EDGE_CURVE('',#33559,#33563,#20697,.T.);
#43730=EDGE_CURVE('',#33498,#33563,#26236,.T.);
#43731=EDGE_CURVE('',#33563,#33560,#20698,.T.);
#43732=EDGE_CURVE('',#33562,#33558,#20699,.T.);
#43733=EDGE_CURVE('',#33564,#33565,#20700,.T.);
#43734=EDGE_CURVE('',#33329,#33565,#24053,.T.);
#43735=EDGE_CURVE('',#33564,#33498,#26237,.T.);
#43736=EDGE_CURVE('',#33566,#33567,#20701,.T.);
#43737=EDGE_CURVE('',#33566,#33568,#20702,.T.);
#43738=EDGE_CURVE('',#33567,#33568,#20703,.T.);
#43739=EDGE_CURVE('',#33565,#33569,#20704,.T.);
#43740=EDGE_CURVE('',#33499,#33569,#26238,.T.);
#43741=EDGE_CURVE('',#33569,#33566,#20705,.T.);
#43742=EDGE_CURVE('',#33568,#33564,#20706,.T.);
#43743=EDGE_CURVE('',#33570,#33571,#20707,.T.);
#43744=EDGE_CURVE('',#33330,#33571,#24054,.T.);
#43745=EDGE_CURVE('',#33570,#33499,#26239,.T.);
#43746=EDGE_CURVE('',#33572,#33573,#20708,.T.);
#43747=EDGE_CURVE('',#33572,#33574,#20709,.T.);
#43748=EDGE_CURVE('',#33573,#33574,#20710,.T.);
#43749=EDGE_CURVE('',#33571,#33575,#20711,.T.);
#43750=EDGE_CURVE('',#33500,#33575,#26240,.T.);
#43751=EDGE_CURVE('',#33575,#33572,#20712,.T.);
#43752=EDGE_CURVE('',#33574,#33570,#20713,.T.);
#43753=EDGE_CURVE('',#33576,#33577,#20714,.T.);
#43754=EDGE_CURVE('',#33331,#33577,#24055,.T.);
#43755=EDGE_CURVE('',#33576,#33500,#26241,.T.);
#43756=EDGE_CURVE('',#33578,#33579,#20715,.T.);
#43757=EDGE_CURVE('',#33578,#33580,#20716,.T.);
#43758=EDGE_CURVE('',#33579,#33580,#20717,.T.);
#43759=EDGE_CURVE('',#33577,#33581,#20718,.T.);
#43760=EDGE_CURVE('',#33501,#33581,#26242,.T.);
#43761=EDGE_CURVE('',#33581,#33578,#20719,.T.);
#43762=EDGE_CURVE('',#33580,#33576,#20720,.T.);
#43763=EDGE_CURVE('',#33582,#33583,#20721,.T.);
#43764=EDGE_CURVE('',#33332,#33583,#24056,.T.);
#43765=EDGE_CURVE('',#33582,#33501,#26243,.T.);
#43766=EDGE_CURVE('',#33584,#33585,#20722,.T.);
#43767=EDGE_CURVE('',#33584,#33586,#20723,.T.);
#43768=EDGE_CURVE('',#33585,#33586,#20724,.T.);
#43769=EDGE_CURVE('',#33583,#33587,#20725,.T.);
#43770=EDGE_CURVE('',#33502,#33587,#26244,.T.);
#43771=EDGE_CURVE('',#33587,#33584,#20726,.T.);
#43772=EDGE_CURVE('',#33586,#33582,#20727,.T.);
#43773=EDGE_CURVE('',#33588,#33589,#20728,.T.);
#43774=EDGE_CURVE('',#33333,#33589,#24057,.T.);
#43775=EDGE_CURVE('',#33588,#33502,#26245,.T.);
#43776=EDGE_CURVE('',#33590,#33591,#20729,.T.);
#43777=EDGE_CURVE('',#33590,#33592,#20730,.T.);
#43778=EDGE_CURVE('',#33591,#33592,#20731,.T.);
#43779=EDGE_CURVE('',#33589,#33593,#20732,.T.);
#43780=EDGE_CURVE('',#33503,#33593,#26246,.T.);
#43781=EDGE_CURVE('',#33593,#33590,#20733,.T.);
#43782=EDGE_CURVE('',#33592,#33588,#20734,.T.);
#43783=EDGE_CURVE('',#33594,#33595,#20735,.T.);
#43784=EDGE_CURVE('',#33334,#33595,#24058,.T.);
#43785=EDGE_CURVE('',#33594,#33503,#26247,.T.);
#43786=EDGE_CURVE('',#33596,#33597,#20736,.T.);
#43787=EDGE_CURVE('',#33596,#33598,#20737,.T.);
#43788=EDGE_CURVE('',#33597,#33598,#20738,.T.);
#43789=EDGE_CURVE('',#33595,#33599,#20739,.T.);
#43790=EDGE_CURVE('',#33504,#33599,#26248,.T.);
#43791=EDGE_CURVE('',#33599,#33596,#20740,.T.);
#43792=EDGE_CURVE('',#33598,#33594,#20741,.T.);
#43793=EDGE_CURVE('',#33600,#33601,#20742,.T.);
#43794=EDGE_CURVE('',#33335,#33601,#24059,.T.);
#43795=EDGE_CURVE('',#33600,#33504,#26249,.T.);
#43796=EDGE_CURVE('',#33602,#33603,#20743,.T.);
#43797=EDGE_CURVE('',#33602,#33604,#20744,.T.);
#43798=EDGE_CURVE('',#33603,#33604,#20745,.T.);
#43799=EDGE_CURVE('',#33601,#33605,#20746,.T.);
#43800=EDGE_CURVE('',#33505,#33605,#26250,.T.);
#43801=EDGE_CURVE('',#33605,#33602,#20747,.T.);
#43802=EDGE_CURVE('',#33604,#33600,#20748,.T.);
#43803=EDGE_CURVE('',#33606,#33607,#20749,.T.);
#43804=EDGE_CURVE('',#33336,#33607,#24060,.T.);
#43805=EDGE_CURVE('',#33606,#33505,#26251,.T.);
#43806=EDGE_CURVE('',#33608,#33609,#20750,.T.);
#43807=EDGE_CURVE('',#33608,#33610,#20751,.T.);
#43808=EDGE_CURVE('',#33609,#33610,#20752,.T.);
#43809=EDGE_CURVE('',#33607,#33611,#20753,.T.);
#43810=EDGE_CURVE('',#33506,#33611,#26252,.T.);
#43811=EDGE_CURVE('',#33611,#33608,#20754,.T.);
#43812=EDGE_CURVE('',#33610,#33606,#20755,.T.);
#43813=EDGE_CURVE('',#33612,#33613,#20756,.T.);
#43814=EDGE_CURVE('',#33337,#33613,#24061,.T.);
#43815=EDGE_CURVE('',#33612,#33506,#26253,.T.);
#43816=EDGE_CURVE('',#33614,#33615,#20757,.T.);
#43817=EDGE_CURVE('',#33614,#33616,#20758,.T.);
#43818=EDGE_CURVE('',#33615,#33616,#20759,.T.);
#43819=EDGE_CURVE('',#33613,#33617,#20760,.T.);
#43820=EDGE_CURVE('',#33507,#33617,#26254,.T.);
#43821=EDGE_CURVE('',#33617,#33614,#20761,.T.);
#43822=EDGE_CURVE('',#33616,#33612,#20762,.T.);
#43823=EDGE_CURVE('',#33618,#33507,#26255,.T.);
#43824=EDGE_CURVE('',#33618,#33619,#20763,.T.);
#43825=EDGE_CURVE('',#33338,#33619,#24062,.T.);
#43826=EDGE_CURVE('',#33620,#33621,#20764,.T.);
#43827=EDGE_CURVE('',#33620,#33622,#20765,.T.);
#43828=EDGE_CURVE('',#33621,#33622,#20766,.T.);
#43829=EDGE_CURVE('',#33619,#33623,#20767,.T.);
#43830=EDGE_CURVE('',#33508,#33623,#26256,.T.);
#43831=EDGE_CURVE('',#33623,#33620,#20768,.T.);
#43832=EDGE_CURVE('',#33622,#33618,#20769,.T.);
#43833=EDGE_CURVE('',#33624,#33625,#20770,.T.);
#43834=EDGE_CURVE('',#33339,#33625,#24063,.T.);
#43835=EDGE_CURVE('',#33624,#33508,#26257,.T.);
#43836=EDGE_CURVE('',#33626,#33627,#20771,.T.);
#43837=EDGE_CURVE('',#33626,#33628,#20772,.T.);
#43838=EDGE_CURVE('',#33627,#33628,#20773,.T.);
#43839=EDGE_CURVE('',#33625,#33629,#20774,.T.);
#43840=EDGE_CURVE('',#33509,#33629,#26258,.T.);
#43841=EDGE_CURVE('',#33629,#33626,#20775,.T.);
#43842=EDGE_CURVE('',#33628,#33624,#20776,.T.);
#43843=EDGE_CURVE('',#33630,#33631,#20777,.T.);
#43844=EDGE_CURVE('',#33340,#33631,#24064,.T.);
#43845=EDGE_CURVE('',#33630,#33509,#26259,.T.);
#43846=EDGE_CURVE('',#33632,#33633,#20778,.T.);
#43847=EDGE_CURVE('',#33632,#33634,#20779,.T.);
#43848=EDGE_CURVE('',#33633,#33634,#20780,.T.);
#43849=EDGE_CURVE('',#33631,#33635,#20781,.T.);
#43850=EDGE_CURVE('',#33510,#33635,#26260,.T.);
#43851=EDGE_CURVE('',#33635,#33632,#20782,.T.);
#43852=EDGE_CURVE('',#33634,#33630,#20783,.T.);
#43853=EDGE_CURVE('',#33636,#33637,#20784,.T.);
#43854=EDGE_CURVE('',#33341,#33637,#24065,.T.);
#43855=EDGE_CURVE('',#33636,#33510,#26261,.T.);
#43856=EDGE_CURVE('',#33638,#33639,#20785,.T.);
#43857=EDGE_CURVE('',#33638,#33640,#20786,.T.);
#43858=EDGE_CURVE('',#33639,#33640,#20787,.T.);
#43859=EDGE_CURVE('',#33637,#33641,#20788,.T.);
#43860=EDGE_CURVE('',#33511,#33641,#26262,.T.);
#43861=EDGE_CURVE('',#33641,#33638,#20789,.T.);
#43862=EDGE_CURVE('',#33640,#33636,#20790,.T.);
#43863=EDGE_CURVE('',#33642,#33643,#20791,.T.);
#43864=EDGE_CURVE('',#33342,#33643,#24066,.T.);
#43865=EDGE_CURVE('',#33642,#33511,#26263,.T.);
#43866=EDGE_CURVE('',#33644,#33645,#20792,.T.);
#43867=EDGE_CURVE('',#33644,#33646,#20793,.T.);
#43868=EDGE_CURVE('',#33645,#33646,#20794,.T.);
#43869=EDGE_CURVE('',#33643,#33647,#20795,.T.);
#43870=EDGE_CURVE('',#33512,#33647,#26264,.T.);
#43871=EDGE_CURVE('',#33647,#33644,#20796,.T.);
#43872=EDGE_CURVE('',#33646,#33642,#20797,.T.);
#43873=EDGE_CURVE('',#33648,#33649,#20798,.T.);
#43874=EDGE_CURVE('',#33343,#33649,#24067,.T.);
#43875=EDGE_CURVE('',#33648,#33512,#26265,.T.);
#43876=EDGE_CURVE('',#33650,#33651,#20799,.T.);
#43877=EDGE_CURVE('',#33650,#33652,#20800,.T.);
#43878=EDGE_CURVE('',#33651,#33652,#20801,.T.);
#43879=EDGE_CURVE('',#33649,#33653,#20802,.T.);
#43880=EDGE_CURVE('',#33513,#33653,#26266,.T.);
#43881=EDGE_CURVE('',#33653,#33650,#20803,.T.);
#43882=EDGE_CURVE('',#33652,#33648,#20804,.T.);
#43883=EDGE_CURVE('',#33654,#33655,#20805,.T.);
#43884=EDGE_CURVE('',#33344,#33655,#24068,.T.);
#43885=EDGE_CURVE('',#33654,#33513,#26267,.T.);
#43886=EDGE_CURVE('',#33656,#33657,#20806,.T.);
#43887=EDGE_CURVE('',#33656,#33658,#20807,.T.);
#43888=EDGE_CURVE('',#33657,#33658,#20808,.T.);
#43889=EDGE_CURVE('',#33655,#33659,#20809,.T.);
#43890=EDGE_CURVE('',#33514,#33659,#26268,.T.);
#43891=EDGE_CURVE('',#33659,#33656,#20810,.T.);
#43892=EDGE_CURVE('',#33658,#33654,#20811,.T.);
#43893=EDGE_CURVE('',#33660,#33661,#20812,.T.);
#43894=EDGE_CURVE('',#33345,#33661,#24069,.T.);
#43895=EDGE_CURVE('',#33660,#33514,#26269,.T.);
#43896=EDGE_CURVE('',#33662,#33663,#20813,.T.);
#43897=EDGE_CURVE('',#33662,#33664,#20814,.T.);
#43898=EDGE_CURVE('',#33663,#33664,#20815,.T.);
#43899=EDGE_CURVE('',#33661,#33665,#20816,.T.);
#43900=EDGE_CURVE('',#33515,#33665,#26270,.T.);
#43901=EDGE_CURVE('',#33665,#33662,#20817,.T.);
#43902=EDGE_CURVE('',#33664,#33660,#20818,.T.);
#43903=EDGE_CURVE('',#33666,#33667,#20819,.T.);
#43904=EDGE_CURVE('',#33346,#33667,#24070,.T.);
#43905=EDGE_CURVE('',#33666,#33515,#26271,.T.);
#43906=EDGE_CURVE('',#33668,#33669,#20820,.T.);
#43907=EDGE_CURVE('',#33668,#33670,#20821,.T.);
#43908=EDGE_CURVE('',#33669,#33670,#20822,.T.);
#43909=EDGE_CURVE('',#33667,#33671,#20823,.T.);
#43910=EDGE_CURVE('',#33516,#33671,#26272,.T.);
#43911=EDGE_CURVE('',#33671,#33668,#20824,.T.);
#43912=EDGE_CURVE('',#33670,#33666,#20825,.T.);
#43913=EDGE_CURVE('',#33672,#33673,#20826,.T.);
#43914=EDGE_CURVE('',#33347,#33673,#24071,.T.);
#43915=EDGE_CURVE('',#33672,#33516,#26273,.T.);
#43916=EDGE_CURVE('',#33674,#33675,#20827,.T.);
#43917=EDGE_CURVE('',#33674,#33676,#20828,.T.);
#43918=EDGE_CURVE('',#33675,#33676,#20829,.T.);
#43919=EDGE_CURVE('',#33673,#33677,#20830,.T.);
#43920=EDGE_CURVE('',#33517,#33677,#26274,.T.);
#43921=EDGE_CURVE('',#33677,#33674,#20831,.T.);
#43922=EDGE_CURVE('',#33676,#33672,#20832,.T.);
#43923=EDGE_CURVE('',#33678,#33679,#20833,.T.);
#43924=EDGE_CURVE('',#33348,#33679,#24072,.T.);
#43925=EDGE_CURVE('',#33678,#33517,#26275,.T.);
#43926=EDGE_CURVE('',#33680,#33681,#20834,.T.);
#43927=EDGE_CURVE('',#33680,#33682,#20835,.T.);
#43928=EDGE_CURVE('',#33681,#33682,#20836,.T.);
#43929=EDGE_CURVE('',#33679,#33683,#20837,.T.);
#43930=EDGE_CURVE('',#33518,#33683,#26276,.T.);
#43931=EDGE_CURVE('',#33683,#33680,#20838,.T.);
#43932=EDGE_CURVE('',#33682,#33678,#20839,.T.);
#43933=EDGE_CURVE('',#33684,#33685,#20840,.T.);
#43934=EDGE_CURVE('',#33684,#33686,#20841,.T.);
#43935=EDGE_CURVE('',#33685,#33686,#20842,.T.);
#43936=EDGE_CURVE('',#33520,#33684,#20843,.T.);
#43937=EDGE_CURVE('',#33687,#33519,#20844,.T.);
#43938=EDGE_CURVE('',#33686,#33687,#20845,.T.);
#43939=EDGE_CURVE('',#33687,#33518,#26277,.T.);
#43940=EDGE_CURVE('',#33688,#33685,#141,.T.);
#43941=EDGE_CURVE('',#33490,#33688,#20846,.T.);
#43942=EDGE_CURVE('',#33689,#33490,#20847,.T.);
#43943=EDGE_CURVE('',#33524,#33689,#142,.T.);
#43944=EDGE_CURVE('',#33491,#33689,#20848,.T.);
#43945=EDGE_CURVE('',#33690,#33491,#20849,.T.);
#43946=EDGE_CURVE('',#33530,#33690,#143,.T.);
#43947=EDGE_CURVE('',#33492,#33690,#20850,.T.);
#43948=EDGE_CURVE('',#33691,#33492,#20851,.T.);
#43949=EDGE_CURVE('',#33536,#33691,#144,.T.);
#43950=EDGE_CURVE('',#33493,#33691,#20852,.T.);
#43951=EDGE_CURVE('',#33692,#33493,#20853,.T.);
#43952=EDGE_CURVE('',#33542,#33692,#145,.T.);
#43953=EDGE_CURVE('',#33494,#33692,#20854,.T.);
#43954=EDGE_CURVE('',#33693,#33494,#20855,.T.);
#43955=EDGE_CURVE('',#33548,#33693,#146,.T.);
#43956=EDGE_CURVE('',#33495,#33693,#20856,.T.);
#43957=EDGE_CURVE('',#33694,#33495,#20857,.T.);
#43958=EDGE_CURVE('',#33554,#33694,#147,.T.);
#43959=EDGE_CURVE('',#33496,#33694,#20858,.T.);
#43960=EDGE_CURVE('',#33695,#33496,#20859,.T.);
#43961=EDGE_CURVE('',#33557,#33695,#148,.T.);
#43962=EDGE_CURVE('',#33497,#33695,#20860,.T.);
#43963=EDGE_CURVE('',#33696,#33497,#20861,.T.);
#43964=EDGE_CURVE('',#33561,#33696,#149,.T.);
#43965=EDGE_CURVE('',#33498,#33696,#20862,.T.);
#43966=EDGE_CURVE('',#33697,#33498,#20863,.T.);
#43967=EDGE_CURVE('',#33567,#33697,#150,.T.);
#43968=EDGE_CURVE('',#33499,#33697,#20864,.T.);
#43969=EDGE_CURVE('',#33698,#33499,#20865,.T.);
#43970=EDGE_CURVE('',#33573,#33698,#151,.T.);
#43971=EDGE_CURVE('',#33500,#33698,#20866,.T.);
#43972=EDGE_CURVE('',#33699,#33500,#20867,.T.);
#43973=EDGE_CURVE('',#33579,#33699,#152,.T.);
#43974=EDGE_CURVE('',#33501,#33699,#20868,.T.);
#43975=EDGE_CURVE('',#33700,#33501,#20869,.T.);
#43976=EDGE_CURVE('',#33585,#33700,#153,.T.);
#43977=EDGE_CURVE('',#33502,#33700,#20870,.T.);
#43978=EDGE_CURVE('',#33701,#33502,#20871,.T.);
#43979=EDGE_CURVE('',#33591,#33701,#154,.T.);
#43980=EDGE_CURVE('',#33503,#33701,#20872,.T.);
#43981=EDGE_CURVE('',#33702,#33503,#20873,.T.);
#43982=EDGE_CURVE('',#33597,#33702,#155,.T.);
#43983=EDGE_CURVE('',#33504,#33702,#20874,.T.);
#43984=EDGE_CURVE('',#33703,#33504,#20875,.T.);
#43985=EDGE_CURVE('',#33603,#33703,#156,.T.);
#43986=EDGE_CURVE('',#33505,#33703,#20876,.T.);
#43987=EDGE_CURVE('',#33704,#33505,#20877,.T.);
#43988=EDGE_CURVE('',#33609,#33704,#157,.T.);
#43989=EDGE_CURVE('',#33506,#33704,#20878,.T.);
#43990=EDGE_CURVE('',#33705,#33506,#20879,.T.);
#43991=EDGE_CURVE('',#33615,#33705,#158,.T.);
#43992=EDGE_CURVE('',#33507,#33705,#20880,.T.);
#43993=EDGE_CURVE('',#33706,#33507,#20881,.T.);
#43994=EDGE_CURVE('',#33621,#33706,#159,.T.);
#43995=EDGE_CURVE('',#33508,#33706,#20882,.T.);
#43996=EDGE_CURVE('',#33707,#33508,#20883,.T.);
#43997=EDGE_CURVE('',#33627,#33707,#160,.T.);
#43998=EDGE_CURVE('',#33509,#33707,#20884,.T.);
#43999=EDGE_CURVE('',#33708,#33509,#20885,.T.);
#44000=EDGE_CURVE('',#33633,#33708,#161,.T.);
#44001=EDGE_CURVE('',#33510,#33708,#20886,.T.);
#44002=EDGE_CURVE('',#33709,#33510,#20887,.T.);
#44003=EDGE_CURVE('',#33639,#33709,#162,.T.);
#44004=EDGE_CURVE('',#33511,#33709,#20888,.T.);
#44005=EDGE_CURVE('',#33710,#33511,#20889,.T.);
#44006=EDGE_CURVE('',#33645,#33710,#163,.T.);
#44007=EDGE_CURVE('',#33512,#33710,#20890,.T.);
#44008=EDGE_CURVE('',#33711,#33512,#20891,.T.);
#44009=EDGE_CURVE('',#33651,#33711,#164,.T.);
#44010=EDGE_CURVE('',#33513,#33711,#20892,.T.);
#44011=EDGE_CURVE('',#33712,#33513,#20893,.T.);
#44012=EDGE_CURVE('',#33657,#33712,#165,.T.);
#44013=EDGE_CURVE('',#33514,#33712,#20894,.T.);
#44014=EDGE_CURVE('',#33713,#33514,#20895,.T.);
#44015=EDGE_CURVE('',#33663,#33713,#166,.T.);
#44016=EDGE_CURVE('',#33515,#33713,#20896,.T.);
#44017=EDGE_CURVE('',#33714,#33515,#20897,.T.);
#44018=EDGE_CURVE('',#33669,#33714,#167,.T.);
#44019=EDGE_CURVE('',#33516,#33714,#20898,.T.);
#44020=EDGE_CURVE('',#33715,#33516,#20899,.T.);
#44021=EDGE_CURVE('',#33675,#33715,#168,.T.);
#44022=EDGE_CURVE('',#33517,#33715,#20900,.T.);
#44023=EDGE_CURVE('',#33716,#33517,#20901,.T.);
#44024=EDGE_CURVE('',#33681,#33716,#169,.T.);
#44025=EDGE_CURVE('',#33518,#33716,#20902,.T.);
#44026=EDGE_CURVE('',#33688,#33518,#20903,.T.);
#44027=EDGE_CURVE('',#33717,#33688,#26278,.T.);
#44028=EDGE_CURVE('',#33717,#33718,#24073,.T.);
#44029=EDGE_CURVE('',#33490,#33718,#24074,.T.);
#44030=EDGE_CURVE('',#33719,#33720,#24075,.T.);
#44031=EDGE_CURVE('',#33718,#33719,#24076,.T.);
#44032=EDGE_CURVE('',#33720,#33717,#24077,.T.);
#44033=EDGE_CURVE('',#33689,#33719,#26279,.T.);
#44034=EDGE_CURVE('',#33721,#33689,#26280,.T.);
#44035=EDGE_CURVE('',#33721,#33722,#24078,.T.);
#44036=EDGE_CURVE('',#33491,#33722,#24079,.T.);
#44037=EDGE_CURVE('',#33723,#33724,#24080,.T.);
#44038=EDGE_CURVE('',#33722,#33723,#24081,.T.);
#44039=EDGE_CURVE('',#33724,#33721,#24082,.T.);
#44040=EDGE_CURVE('',#33690,#33723,#26281,.T.);
#44041=EDGE_CURVE('',#33725,#33690,#26282,.T.);
#44042=EDGE_CURVE('',#33725,#33726,#24083,.T.);
#44043=EDGE_CURVE('',#33492,#33726,#24084,.T.);
#44044=EDGE_CURVE('',#33727,#33728,#24085,.T.);
#44045=EDGE_CURVE('',#33726,#33727,#24086,.T.);
#44046=EDGE_CURVE('',#33728,#33725,#24087,.T.);
#44047=EDGE_CURVE('',#33691,#33727,#26283,.T.);
#44048=EDGE_CURVE('',#33729,#33691,#26284,.T.);
#44049=EDGE_CURVE('',#33729,#33730,#24088,.T.);
#44050=EDGE_CURVE('',#33493,#33730,#24089,.T.);
#44051=EDGE_CURVE('',#33731,#33732,#24090,.T.);
#44052=EDGE_CURVE('',#33730,#33731,#24091,.T.);
#44053=EDGE_CURVE('',#33732,#33729,#24092,.T.);
#44054=EDGE_CURVE('',#33692,#33731,#26285,.T.);
#44055=EDGE_CURVE('',#33733,#33692,#26286,.T.);
#44056=EDGE_CURVE('',#33733,#33734,#24093,.T.);
#44057=EDGE_CURVE('',#33494,#33734,#24094,.T.);
#44058=EDGE_CURVE('',#33735,#33736,#24095,.T.);
#44059=EDGE_CURVE('',#33734,#33735,#24096,.T.);
#44060=EDGE_CURVE('',#33736,#33733,#24097,.T.);
#44061=EDGE_CURVE('',#33693,#33735,#26287,.T.);
#44062=EDGE_CURVE('',#33737,#33693,#26288,.T.);
#44063=EDGE_CURVE('',#33737,#33738,#24098,.T.);
#44064=EDGE_CURVE('',#33495,#33738,#24099,.T.);
#44065=EDGE_CURVE('',#33739,#33740,#24100,.T.);
#44066=EDGE_CURVE('',#33738,#33739,#24101,.T.);
#44067=EDGE_CURVE('',#33740,#33737,#24102,.T.);
#44068=EDGE_CURVE('',#33694,#33739,#26289,.T.);
#44069=EDGE_CURVE('',#33741,#33694,#26290,.T.);
#44070=EDGE_CURVE('',#33741,#33742,#24103,.T.);
#44071=EDGE_CURVE('',#33496,#33742,#24104,.T.);
#44072=EDGE_CURVE('',#33743,#33744,#24105,.T.);
#44073=EDGE_CURVE('',#33742,#33743,#24106,.T.);
#44074=EDGE_CURVE('',#33744,#33741,#24107,.T.);
#44075=EDGE_CURVE('',#33695,#33743,#26291,.T.);
#44076=EDGE_CURVE('',#33745,#33695,#26292,.T.);
#44077=EDGE_CURVE('',#33745,#33746,#24108,.T.);
#44078=EDGE_CURVE('',#33497,#33746,#24109,.T.);
#44079=EDGE_CURVE('',#33747,#33748,#24110,.T.);
#44080=EDGE_CURVE('',#33746,#33747,#24111,.T.);
#44081=EDGE_CURVE('',#33748,#33745,#24112,.T.);
#44082=EDGE_CURVE('',#33696,#33747,#26293,.T.);
#44083=EDGE_CURVE('',#33749,#33696,#26294,.T.);
#44084=EDGE_CURVE('',#33749,#33750,#24113,.T.);
#44085=EDGE_CURVE('',#33498,#33750,#24114,.T.);
#44086=EDGE_CURVE('',#33751,#33752,#24115,.T.);
#44087=EDGE_CURVE('',#33750,#33751,#24116,.T.);
#44088=EDGE_CURVE('',#33752,#33749,#24117,.T.);
#44089=EDGE_CURVE('',#33697,#33751,#26295,.T.);
#44090=EDGE_CURVE('',#33753,#33697,#26296,.T.);
#44091=EDGE_CURVE('',#33753,#33754,#24118,.T.);
#44092=EDGE_CURVE('',#33499,#33754,#24119,.T.);
#44093=EDGE_CURVE('',#33755,#33756,#24120,.T.);
#44094=EDGE_CURVE('',#33754,#33755,#24121,.T.);
#44095=EDGE_CURVE('',#33756,#33753,#24122,.T.);
#44096=EDGE_CURVE('',#33698,#33755,#26297,.T.);
#44097=EDGE_CURVE('',#33757,#33698,#26298,.T.);
#44098=EDGE_CURVE('',#33757,#33758,#24123,.T.);
#44099=EDGE_CURVE('',#33500,#33758,#24124,.T.);
#44100=EDGE_CURVE('',#33759,#33760,#24125,.T.);
#44101=EDGE_CURVE('',#33758,#33759,#24126,.T.);
#44102=EDGE_CURVE('',#33760,#33757,#24127,.T.);
#44103=EDGE_CURVE('',#33699,#33759,#26299,.T.);
#44104=EDGE_CURVE('',#33761,#33699,#26300,.T.);
#44105=EDGE_CURVE('',#33761,#33762,#24128,.T.);
#44106=EDGE_CURVE('',#33501,#33762,#24129,.T.);
#44107=EDGE_CURVE('',#33763,#33764,#24130,.T.);
#44108=EDGE_CURVE('',#33762,#33763,#24131,.T.);
#44109=EDGE_CURVE('',#33764,#33761,#24132,.T.);
#44110=EDGE_CURVE('',#33700,#33763,#26301,.T.);
#44111=EDGE_CURVE('',#33765,#33700,#26302,.T.);
#44112=EDGE_CURVE('',#33765,#33766,#24133,.T.);
#44113=EDGE_CURVE('',#33502,#33766,#24134,.T.);
#44114=EDGE_CURVE('',#33767,#33768,#24135,.T.);
#44115=EDGE_CURVE('',#33766,#33767,#24136,.T.);
#44116=EDGE_CURVE('',#33768,#33765,#24137,.T.);
#44117=EDGE_CURVE('',#33701,#33767,#26303,.T.);
#44118=EDGE_CURVE('',#33769,#33701,#26304,.T.);
#44119=EDGE_CURVE('',#33769,#33770,#24138,.T.);
#44120=EDGE_CURVE('',#33503,#33770,#24139,.T.);
#44121=EDGE_CURVE('',#33771,#33772,#24140,.T.);
#44122=EDGE_CURVE('',#33770,#33771,#24141,.T.);
#44123=EDGE_CURVE('',#33772,#33769,#24142,.T.);
#44124=EDGE_CURVE('',#33702,#33771,#26305,.T.);
#44125=EDGE_CURVE('',#33773,#33702,#26306,.T.);
#44126=EDGE_CURVE('',#33773,#33774,#24143,.T.);
#44127=EDGE_CURVE('',#33504,#33774,#24144,.T.);
#44128=EDGE_CURVE('',#33775,#33776,#24145,.T.);
#44129=EDGE_CURVE('',#33774,#33775,#24146,.T.);
#44130=EDGE_CURVE('',#33776,#33773,#24147,.T.);
#44131=EDGE_CURVE('',#33703,#33775,#26307,.T.);
#44132=EDGE_CURVE('',#33777,#33703,#26308,.T.);
#44133=EDGE_CURVE('',#33777,#33778,#24148,.T.);
#44134=EDGE_CURVE('',#33505,#33778,#24149,.T.);
#44135=EDGE_CURVE('',#33779,#33780,#24150,.T.);
#44136=EDGE_CURVE('',#33778,#33779,#24151,.T.);
#44137=EDGE_CURVE('',#33780,#33777,#24152,.T.);
#44138=EDGE_CURVE('',#33704,#33779,#26309,.T.);
#44139=EDGE_CURVE('',#33781,#33704,#26310,.T.);
#44140=EDGE_CURVE('',#33781,#33782,#24153,.T.);
#44141=EDGE_CURVE('',#33506,#33782,#24154,.T.);
#44142=EDGE_CURVE('',#33783,#33784,#24155,.T.);
#44143=EDGE_CURVE('',#33782,#33783,#24156,.T.);
#44144=EDGE_CURVE('',#33784,#33781,#24157,.T.);
#44145=EDGE_CURVE('',#33705,#33783,#26311,.T.);
#44146=EDGE_CURVE('',#33785,#33705,#26312,.T.);
#44147=EDGE_CURVE('',#33785,#33786,#24158,.T.);
#44148=EDGE_CURVE('',#33507,#33786,#24159,.T.);
#44149=EDGE_CURVE('',#33787,#33785,#24160,.T.);
#44150=EDGE_CURVE('',#33788,#33787,#24161,.T.);
#44151=EDGE_CURVE('',#33786,#33788,#24162,.T.);
#44152=EDGE_CURVE('',#33706,#33788,#26313,.T.);
#44153=EDGE_CURVE('',#33789,#33706,#26314,.T.);
#44154=EDGE_CURVE('',#33789,#33790,#24163,.T.);
#44155=EDGE_CURVE('',#33508,#33790,#24164,.T.);
#44156=EDGE_CURVE('',#33791,#33792,#24165,.T.);
#44157=EDGE_CURVE('',#33790,#33791,#24166,.T.);
#44158=EDGE_CURVE('',#33792,#33789,#24167,.T.);
#44159=EDGE_CURVE('',#33707,#33791,#26315,.T.);
#44160=EDGE_CURVE('',#33793,#33707,#26316,.T.);
#44161=EDGE_CURVE('',#33793,#33794,#24168,.T.);
#44162=EDGE_CURVE('',#33509,#33794,#24169,.T.);
#44163=EDGE_CURVE('',#33795,#33796,#24170,.T.);
#44164=EDGE_CURVE('',#33794,#33795,#24171,.T.);
#44165=EDGE_CURVE('',#33796,#33793,#24172,.T.);
#44166=EDGE_CURVE('',#33708,#33795,#26317,.T.);
#44167=EDGE_CURVE('',#33797,#33708,#26318,.T.);
#44168=EDGE_CURVE('',#33797,#33798,#24173,.T.);
#44169=EDGE_CURVE('',#33510,#33798,#24174,.T.);
#44170=EDGE_CURVE('',#33799,#33800,#24175,.T.);
#44171=EDGE_CURVE('',#33798,#33799,#24176,.T.);
#44172=EDGE_CURVE('',#33800,#33797,#24177,.T.);
#44173=EDGE_CURVE('',#33709,#33799,#26319,.T.);
#44174=EDGE_CURVE('',#28902,#33709,#26320,.T.);
#44175=EDGE_CURVE('',#33511,#28901,#24178,.T.);
#44176=EDGE_CURVE('',#33710,#28899,#26321,.T.);
#44177=EDGE_CURVE('',#33801,#33710,#26322,.T.);
#44178=EDGE_CURVE('',#33801,#33802,#24179,.T.);
#44179=EDGE_CURVE('',#33512,#33802,#24180,.T.);
#44180=EDGE_CURVE('',#33803,#33804,#24181,.T.);
#44181=EDGE_CURVE('',#33802,#33803,#24182,.T.);
#44182=EDGE_CURVE('',#33804,#33801,#24183,.T.);
#44183=EDGE_CURVE('',#33711,#33803,#26323,.T.);
#44184=EDGE_CURVE('',#33805,#33711,#26324,.T.);
#44185=EDGE_CURVE('',#33805,#33806,#24184,.T.);
#44186=EDGE_CURVE('',#33513,#33806,#24185,.T.);
#44187=EDGE_CURVE('',#33807,#33808,#24186,.T.);
#44188=EDGE_CURVE('',#33806,#33807,#24187,.T.);
#44189=EDGE_CURVE('',#33808,#33805,#24188,.T.);
#44190=EDGE_CURVE('',#33712,#33807,#26325,.T.);
#44191=EDGE_CURVE('',#33809,#33712,#26326,.T.);
#44192=EDGE_CURVE('',#33809,#33810,#24189,.T.);
#44193=EDGE_CURVE('',#33514,#33810,#24190,.T.);
#44194=EDGE_CURVE('',#33811,#33812,#24191,.T.);
#44195=EDGE_CURVE('',#33810,#33811,#24192,.T.);
#44196=EDGE_CURVE('',#33812,#33809,#24193,.T.);
#44197=EDGE_CURVE('',#33713,#33811,#26327,.T.);
#44198=EDGE_CURVE('',#33813,#33713,#26328,.T.);
#44199=EDGE_CURVE('',#33813,#33814,#24194,.T.);
#44200=EDGE_CURVE('',#33515,#33814,#24195,.T.);
#44201=EDGE_CURVE('',#33815,#33816,#24196,.T.);
#44202=EDGE_CURVE('',#33814,#33815,#24197,.T.);
#44203=EDGE_CURVE('',#33816,#33813,#24198,.T.);
#44204=EDGE_CURVE('',#33714,#33815,#26329,.T.);
#44205=EDGE_CURVE('',#33817,#33714,#26330,.T.);
#44206=EDGE_CURVE('',#33817,#33818,#24199,.T.);
#44207=EDGE_CURVE('',#33516,#33818,#24200,.T.);
#44208=EDGE_CURVE('',#33819,#33820,#24201,.T.);
#44209=EDGE_CURVE('',#33818,#33819,#24202,.T.);
#44210=EDGE_CURVE('',#33820,#33817,#24203,.T.);
#44211=EDGE_CURVE('',#33715,#33819,#26331,.T.);
#44212=EDGE_CURVE('',#33821,#33715,#26332,.T.);
#44213=EDGE_CURVE('',#33821,#33822,#24204,.T.);
#44214=EDGE_CURVE('',#33517,#33822,#24205,.T.);
#44215=EDGE_CURVE('',#33823,#33824,#24206,.T.);
#44216=EDGE_CURVE('',#33822,#33823,#24207,.T.);
#44217=EDGE_CURVE('',#33824,#33821,#24208,.T.);
#44218=EDGE_CURVE('',#33716,#33823,#26333,.T.);
#44219=EDGE_CURVE('',#28898,#33716,#26334,.T.);
#44220=EDGE_CURVE('',#33518,#28897,#24209,.T.);
#44221=EDGE_CURVE('',#33688,#28895,#26335,.T.);
#44222=EDGE_CURVE('',#33825,#33688,#20904,.T.);
#44223=EDGE_CURVE('',#33720,#33825,#170,.T.);
#44224=EDGE_CURVE('',#33689,#33825,#20905,.T.);
#44225=EDGE_CURVE('',#33826,#33689,#20906,.T.);
#44226=EDGE_CURVE('',#33724,#33826,#24210,.T.);
#44227=EDGE_CURVE('',#33690,#33826,#20907,.T.);
#44228=EDGE_CURVE('',#33827,#33690,#20908,.T.);
#44229=EDGE_CURVE('',#33728,#33827,#171,.T.);
#44230=EDGE_CURVE('',#33691,#33827,#20909,.T.);
#44231=EDGE_CURVE('',#33828,#33691,#20910,.T.);
#44232=EDGE_CURVE('',#33732,#33828,#172,.T.);
#44233=EDGE_CURVE('',#33692,#33828,#20911,.T.);
#44234=EDGE_CURVE('',#33829,#33692,#20912,.T.);
#44235=EDGE_CURVE('',#33736,#33829,#173,.T.);
#44236=EDGE_CURVE('',#33693,#33829,#20913,.T.);
#44237=EDGE_CURVE('',#33830,#33693,#20914,.T.);
#44238=EDGE_CURVE('',#33740,#33830,#174,.T.);
#44239=EDGE_CURVE('',#33694,#33830,#20915,.T.);
#44240=EDGE_CURVE('',#33831,#33694,#20916,.T.);
#44241=EDGE_CURVE('',#33744,#33831,#175,.T.);
#44242=EDGE_CURVE('',#33695,#33831,#20917,.T.);
#44243=EDGE_CURVE('',#33832,#33695,#20918,.T.);
#44244=EDGE_CURVE('',#33748,#33832,#24211,.T.);
#44245=EDGE_CURVE('',#33696,#33832,#20919,.T.);
#44246=EDGE_CURVE('',#33833,#33696,#20920,.T.);
#44247=EDGE_CURVE('',#33752,#33833,#176,.T.);
#44248=EDGE_CURVE('',#33697,#33833,#20921,.T.);
#44249=EDGE_CURVE('',#33834,#33697,#20922,.T.);
#44250=EDGE_CURVE('',#33756,#33834,#177,.T.);
#44251=EDGE_CURVE('',#33698,#33834,#20923,.T.);
#44252=EDGE_CURVE('',#33835,#33698,#20924,.T.);
#44253=EDGE_CURVE('',#33760,#33835,#178,.T.);
#44254=EDGE_CURVE('',#33699,#33835,#20925,.T.);
#44255=EDGE_CURVE('',#33836,#33699,#20926,.T.);
#44256=EDGE_CURVE('',#33764,#33836,#179,.T.);
#44257=EDGE_CURVE('',#33700,#33836,#20927,.T.);
#44258=EDGE_CURVE('',#33837,#33700,#20928,.T.);
#44259=EDGE_CURVE('',#33768,#33837,#24212,.T.);
#44260=EDGE_CURVE('',#33701,#33837,#20929,.T.);
#44261=EDGE_CURVE('',#33838,#33701,#20930,.T.);
#44262=EDGE_CURVE('',#33772,#33838,#180,.T.);
#44263=EDGE_CURVE('',#33702,#33838,#20931,.T.);
#44264=EDGE_CURVE('',#33839,#33702,#20932,.T.);
#44265=EDGE_CURVE('',#33776,#33839,#181,.T.);
#44266=EDGE_CURVE('',#33703,#33839,#20933,.T.);
#44267=EDGE_CURVE('',#33840,#33703,#20934,.T.);
#44268=EDGE_CURVE('',#33780,#33840,#24213,.T.);
#44269=EDGE_CURVE('',#33704,#33840,#20935,.T.);
#44270=EDGE_CURVE('',#33841,#33704,#20936,.T.);
#44271=EDGE_CURVE('',#33784,#33841,#182,.T.);
#44272=EDGE_CURVE('',#33705,#33841,#20937,.T.);
#44273=EDGE_CURVE('',#33842,#33705,#20938,.T.);
#44274=EDGE_CURVE('',#33787,#33842,#24214,.T.);
#44275=EDGE_CURVE('',#33706,#33842,#20939,.T.);
#44276=EDGE_CURVE('',#33843,#33706,#20940,.T.);
#44277=EDGE_CURVE('',#33792,#33843,#183,.T.);
#44278=EDGE_CURVE('',#33707,#33843,#20941,.T.);
#44279=EDGE_CURVE('',#33844,#33707,#20942,.T.);
#44280=EDGE_CURVE('',#33796,#33844,#184,.T.);
#44281=EDGE_CURVE('',#33708,#33844,#20943,.T.);
#44282=EDGE_CURVE('',#33845,#33708,#20944,.T.);
#44283=EDGE_CURVE('',#33800,#33845,#24215,.T.);
#44284=EDGE_CURVE('',#33709,#33845,#20945,.T.);
#44285=EDGE_CURVE('',#33846,#33709,#20946,.T.);
#44286=EDGE_CURVE('',#28900,#33846,#24216,.T.);
#44287=EDGE_CURVE('',#33710,#33846,#20947,.T.);
#44288=EDGE_CURVE('',#33847,#33710,#20948,.T.);
#44289=EDGE_CURVE('',#33804,#33847,#185,.T.);
#44290=EDGE_CURVE('',#33711,#33847,#20949,.T.);
#44291=EDGE_CURVE('',#33848,#33711,#20950,.T.);
#44292=EDGE_CURVE('',#33808,#33848,#186,.T.);
#44293=EDGE_CURVE('',#33712,#33848,#20951,.T.);
#44294=EDGE_CURVE('',#33849,#33712,#20952,.T.);
#44295=EDGE_CURVE('',#33812,#33849,#187,.T.);
#44296=EDGE_CURVE('',#33713,#33849,#20953,.T.);
#44297=EDGE_CURVE('',#33850,#33713,#20954,.T.);
#44298=EDGE_CURVE('',#33816,#33850,#188,.T.);
#44299=EDGE_CURVE('',#33714,#33850,#20955,.T.);
#44300=EDGE_CURVE('',#33851,#33714,#20956,.T.);
#44301=EDGE_CURVE('',#33820,#33851,#189,.T.);
#44302=EDGE_CURVE('',#33715,#33851,#20957,.T.);
#44303=EDGE_CURVE('',#33852,#33715,#20958,.T.);
#44304=EDGE_CURVE('',#33824,#33852,#190,.T.);
#44305=EDGE_CURVE('',#33716,#33852,#20959,.T.);
#44306=EDGE_CURVE('',#33853,#33716,#20960,.T.);
#44307=EDGE_CURVE('',#28896,#33853,#191,.T.);
#44308=EDGE_CURVE('',#33688,#33853,#20961,.T.);
#44309=EDGE_CURVE('',#28619,#33688,#24217,.T.);
#44310=EDGE_CURVE('',#33825,#28618,#26336,.T.);
#44311=EDGE_CURVE('',#33825,#28617,#24218,.T.);
#44312=EDGE_CURVE('',#33825,#28616,#24219,.T.);
#44313=EDGE_CURVE('',#33825,#28615,#20962,.T.);
#44314=EDGE_CURVE('',#33825,#28614,#26337,.T.);
#44315=EDGE_CURVE('',#33689,#28613,#24220,.T.);
#44316=EDGE_CURVE('',#33826,#28612,#26338,.T.);
#44317=EDGE_CURVE('',#33826,#28611,#24221,.T.);
#44318=EDGE_CURVE('',#33826,#28610,#24222,.T.);
#44319=EDGE_CURVE('',#33826,#28609,#20963,.T.);
#44320=EDGE_CURVE('',#33826,#28608,#26339,.T.);
#44321=EDGE_CURVE('',#33690,#28607,#24223,.T.);
#44322=EDGE_CURVE('',#33827,#28606,#26340,.T.);
#44323=EDGE_CURVE('',#33827,#28605,#24224,.T.);
#44324=EDGE_CURVE('',#33827,#28604,#24225,.T.);
#44325=EDGE_CURVE('',#33827,#28603,#20964,.T.);
#44326=EDGE_CURVE('',#33827,#28602,#26341,.T.);
#44327=EDGE_CURVE('',#33691,#28601,#24226,.T.);
#44328=EDGE_CURVE('',#33828,#28600,#26342,.T.);
#44329=EDGE_CURVE('',#33828,#28599,#24227,.T.);
#44330=EDGE_CURVE('',#33828,#28598,#24228,.T.);
#44331=EDGE_CURVE('',#33828,#28597,#20965,.T.);
#44332=EDGE_CURVE('',#33828,#28596,#26343,.T.);
#44333=EDGE_CURVE('',#33692,#28595,#24229,.T.);
#44334=EDGE_CURVE('',#33829,#28594,#26344,.T.);
#44335=EDGE_CURVE('',#33829,#28593,#24230,.T.);
#44336=EDGE_CURVE('',#33829,#28592,#24231,.T.);
#44337=EDGE_CURVE('',#33829,#28591,#20966,.T.);
#44338=EDGE_CURVE('',#33829,#28590,#26345,.T.);
#44339=EDGE_CURVE('',#33693,#28589,#24232,.T.);
#44340=EDGE_CURVE('',#33830,#28588,#26346,.T.);
#44341=EDGE_CURVE('',#33830,#28587,#24233,.T.);
#44342=EDGE_CURVE('',#33830,#28586,#24234,.T.);
#44343=EDGE_CURVE('',#33830,#28585,#20967,.T.);
#44344=EDGE_CURVE('',#33830,#28584,#26347,.T.);
#44345=EDGE_CURVE('',#33694,#28583,#24235,.T.);
#44346=EDGE_CURVE('',#33831,#28582,#26348,.T.);
#44347=EDGE_CURVE('',#33831,#28581,#24236,.T.);
#44348=EDGE_CURVE('',#33831,#28580,#24237,.T.);
#44349=EDGE_CURVE('',#33831,#28579,#20968,.T.);
#44350=EDGE_CURVE('',#33831,#28578,#26349,.T.);
#44351=EDGE_CURVE('',#33695,#28577,#24238,.T.);
#44352=EDGE_CURVE('',#33832,#28576,#26350,.T.);
#44353=EDGE_CURVE('',#33832,#28575,#24239,.T.);
#44354=EDGE_CURVE('',#33832,#28574,#24240,.T.);
#44355=EDGE_CURVE('',#33832,#28573,#20969,.T.);
#44356=EDGE_CURVE('',#33832,#28572,#26351,.T.);
#44357=EDGE_CURVE('',#33696,#28571,#24241,.T.);
#44358=EDGE_CURVE('',#33833,#28570,#26352,.T.);
#44359=EDGE_CURVE('',#33833,#28569,#24242,.T.);
#44360=EDGE_CURVE('',#33833,#28568,#24243,.T.);
#44361=EDGE_CURVE('',#33833,#28567,#20970,.T.);
#44362=EDGE_CURVE('',#33833,#28566,#26353,.T.);
#44363=EDGE_CURVE('',#33697,#28565,#24244,.T.);
#44364=EDGE_CURVE('',#33834,#28564,#26354,.T.);
#44365=EDGE_CURVE('',#33834,#28563,#24245,.T.);
#44366=EDGE_CURVE('',#33834,#28562,#24246,.T.);
#44367=EDGE_CURVE('',#33834,#28561,#20971,.T.);
#44368=EDGE_CURVE('',#33834,#28560,#26355,.T.);
#44369=EDGE_CURVE('',#33698,#28559,#24247,.T.);
#44370=EDGE_CURVE('',#33835,#28558,#26356,.T.);
#44371=EDGE_CURVE('',#33835,#28557,#24248,.T.);
#44372=EDGE_CURVE('',#33835,#28556,#24249,.T.);
#44373=EDGE_CURVE('',#33835,#28555,#20972,.T.);
#44374=EDGE_CURVE('',#33835,#28554,#26357,.T.);
#44375=EDGE_CURVE('',#33699,#28553,#24250,.T.);
#44376=EDGE_CURVE('',#33836,#28552,#26358,.T.);
#44377=EDGE_CURVE('',#33836,#28551,#24251,.T.);
#44378=EDGE_CURVE('',#33836,#28550,#24252,.T.);
#44379=EDGE_CURVE('',#33836,#28549,#20973,.T.);
#44380=EDGE_CURVE('',#33836,#28548,#26359,.T.);
#44381=EDGE_CURVE('',#33700,#28547,#24253,.T.);
#44382=EDGE_CURVE('',#33837,#28546,#26360,.T.);
#44383=EDGE_CURVE('',#33837,#28545,#24254,.T.);
#44384=EDGE_CURVE('',#33837,#28544,#24255,.T.);
#44385=EDGE_CURVE('',#33837,#28543,#20974,.T.);
#44386=EDGE_CURVE('',#33837,#28542,#26361,.T.);
#44387=EDGE_CURVE('',#33701,#28541,#24256,.T.);
#44388=EDGE_CURVE('',#33838,#28540,#26362,.T.);
#44389=EDGE_CURVE('',#33838,#28539,#24257,.T.);
#44390=EDGE_CURVE('',#33838,#28538,#24258,.T.);
#44391=EDGE_CURVE('',#33838,#28537,#20975,.T.);
#44392=EDGE_CURVE('',#33838,#28536,#26363,.T.);
#44393=EDGE_CURVE('',#33702,#28535,#24259,.T.);
#44394=EDGE_CURVE('',#33839,#28712,#26364,.T.);
#44395=EDGE_CURVE('',#33839,#28709,#24260,.T.);
#44396=EDGE_CURVE('',#33839,#28706,#24261,.T.);
#44397=EDGE_CURVE('',#33839,#28705,#20976,.T.);
#44398=EDGE_CURVE('',#33839,#28704,#26365,.T.);
#44399=EDGE_CURVE('',#33703,#28703,#24262,.T.);
#44400=EDGE_CURVE('',#33840,#28702,#26366,.T.);
#44401=EDGE_CURVE('',#33840,#28701,#24263,.T.);
#44402=EDGE_CURVE('',#33840,#28700,#24264,.T.);
#44403=EDGE_CURVE('',#33840,#28699,#20977,.T.);
#44404=EDGE_CURVE('',#33840,#28698,#26367,.T.);
#44405=EDGE_CURVE('',#33704,#28697,#24265,.T.);
#44406=EDGE_CURVE('',#33841,#28696,#26368,.T.);
#44407=EDGE_CURVE('',#33841,#28695,#24266,.T.);
#44408=EDGE_CURVE('',#33841,#28694,#24267,.T.);
#44409=EDGE_CURVE('',#33841,#28693,#20978,.T.);
#44410=EDGE_CURVE('',#33841,#28692,#26369,.T.);
#44411=EDGE_CURVE('',#33705,#28691,#24268,.T.);
#44412=EDGE_CURVE('',#33842,#28690,#26370,.T.);
#44413=EDGE_CURVE('',#33842,#28689,#24269,.T.);
#44414=EDGE_CURVE('',#33842,#28688,#24270,.T.);
#44415=EDGE_CURVE('',#33842,#28687,#20979,.T.);
#44416=EDGE_CURVE('',#33842,#28686,#26371,.T.);
#44417=EDGE_CURVE('',#33706,#28685,#24271,.T.);
#44418=EDGE_CURVE('',#33843,#28684,#26372,.T.);
#44419=EDGE_CURVE('',#33843,#28683,#24272,.T.);
#44420=EDGE_CURVE('',#33843,#28682,#24273,.T.);
#44421=EDGE_CURVE('',#33843,#28681,#20980,.T.);
#44422=EDGE_CURVE('',#33843,#28680,#26373,.T.);
#44423=EDGE_CURVE('',#33707,#28679,#24274,.T.);
#44424=EDGE_CURVE('',#33844,#28678,#26374,.T.);
#44425=EDGE_CURVE('',#33844,#28677,#24275,.T.);
#44426=EDGE_CURVE('',#33844,#28676,#24276,.T.);
#44427=EDGE_CURVE('',#33844,#28675,#20981,.T.);
#44428=EDGE_CURVE('',#33844,#28674,#26375,.T.);
#44429=EDGE_CURVE('',#33708,#28673,#24277,.T.);
#44430=EDGE_CURVE('',#33845,#28672,#26376,.T.);
#44431=EDGE_CURVE('',#33845,#28671,#24278,.T.);
#44432=EDGE_CURVE('',#33845,#28670,#24279,.T.);
#44433=EDGE_CURVE('',#33845,#28669,#20982,.T.);
#44434=EDGE_CURVE('',#33845,#28668,#26377,.T.);
#44435=EDGE_CURVE('',#33709,#28667,#24280,.T.);
#44436=EDGE_CURVE('',#33846,#28666,#26378,.T.);
#44437=EDGE_CURVE('',#33846,#28665,#24281,.T.);
#44438=EDGE_CURVE('',#33846,#28664,#24282,.T.);
#44439=EDGE_CURVE('',#33846,#28663,#20983,.T.);
#44440=EDGE_CURVE('',#33846,#28662,#26379,.T.);
#44441=EDGE_CURVE('',#33710,#28661,#24283,.T.);
#44442=EDGE_CURVE('',#33847,#28660,#26380,.T.);
#44443=EDGE_CURVE('',#33847,#28659,#24284,.T.);
#44444=EDGE_CURVE('',#33847,#28658,#24285,.T.);
#44445=EDGE_CURVE('',#33847,#28657,#20984,.T.);
#44446=EDGE_CURVE('',#33847,#28656,#26381,.T.);
#44447=EDGE_CURVE('',#33711,#28655,#24286,.T.);
#44448=EDGE_CURVE('',#33848,#28654,#26382,.T.);
#44449=EDGE_CURVE('',#33848,#28653,#24287,.T.);
#44450=EDGE_CURVE('',#33848,#28652,#24288,.T.);
#44451=EDGE_CURVE('',#33848,#28651,#20985,.T.);
#44452=EDGE_CURVE('',#33848,#28650,#26383,.T.);
#44453=EDGE_CURVE('',#33712,#28649,#24289,.T.);
#44454=EDGE_CURVE('',#33849,#28648,#26384,.T.);
#44455=EDGE_CURVE('',#33849,#28647,#4457,.T.);
#44456=EDGE_CURVE('',#33849,#28646,#24290,.T.);
#44457=EDGE_CURVE('',#33849,#28645,#20986,.T.);
#44458=EDGE_CURVE('',#33849,#28644,#26385,.T.);
#44459=EDGE_CURVE('',#33713,#28643,#24291,.T.);
#44460=EDGE_CURVE('',#33850,#28642,#26386,.T.);
#44461=EDGE_CURVE('',#33850,#28641,#24292,.T.);
#44462=EDGE_CURVE('',#33850,#28640,#24293,.T.);
#44463=EDGE_CURVE('',#33850,#28639,#20987,.T.);
#44464=EDGE_CURVE('',#33850,#28638,#26387,.T.);
#44465=EDGE_CURVE('',#33714,#28637,#24294,.T.);
#44466=EDGE_CURVE('',#33851,#28636,#26388,.T.);
#44467=EDGE_CURVE('',#33851,#28635,#24295,.T.);
#44468=EDGE_CURVE('',#33851,#28634,#24296,.T.);
#44469=EDGE_CURVE('',#33851,#28633,#20988,.T.);
#44470=EDGE_CURVE('',#33851,#28632,#26389,.T.);
#44471=EDGE_CURVE('',#33715,#28631,#24297,.T.);
#44472=EDGE_CURVE('',#33852,#28630,#26390,.T.);
#44473=EDGE_CURVE('',#33852,#28629,#24298,.T.);
#44474=EDGE_CURVE('',#33852,#28628,#24299,.T.);
#44475=EDGE_CURVE('',#33852,#28627,#20989,.T.);
#44476=EDGE_CURVE('',#33852,#28626,#26391,.T.);
#44477=EDGE_CURVE('',#33716,#28625,#24300,.T.);
#44478=EDGE_CURVE('',#33853,#28624,#26392,.T.);
#44479=EDGE_CURVE('',#33853,#28623,#24301,.T.);
#44480=EDGE_CURVE('',#33853,#28622,#24302,.T.);
#44481=EDGE_CURVE('',#33853,#28621,#20990,.T.);
#44482=EDGE_CURVE('',#33853,#28620,#26393,.T.);
#44646=ORIENTED_EDGE('',*,*,#33964,.F.);
#44647=ORIENTED_EDGE('',*,*,#33965,.F.);
#44648=ORIENTED_EDGE('',*,*,#33966,.F.);
#44649=ORIENTED_EDGE('',*,*,#33967,.F.);
#44650=ORIENTED_EDGE('',*,*,#33968,.F.);
#44651=ORIENTED_EDGE('',*,*,#33969,.F.);
#44652=ORIENTED_EDGE('',*,*,#33970,.F.);
#44653=ORIENTED_EDGE('',*,*,#33971,.F.);
#44654=ORIENTED_EDGE('',*,*,#33972,.F.);
#44655=ORIENTED_EDGE('',*,*,#33973,.F.);
#44656=ORIENTED_EDGE('',*,*,#33974,.F.);
#44657=ORIENTED_EDGE('',*,*,#33975,.F.);
#44658=ORIENTED_EDGE('',*,*,#33976,.F.);
#44659=ORIENTED_EDGE('',*,*,#33977,.F.);
#44660=ORIENTED_EDGE('',*,*,#33978,.F.);
#44661=ORIENTED_EDGE('',*,*,#33979,.F.);
#44662=ORIENTED_EDGE('',*,*,#33980,.F.);
#44663=ORIENTED_EDGE('',*,*,#33981,.F.);
#44664=ORIENTED_EDGE('',*,*,#33982,.F.);
#44665=ORIENTED_EDGE('',*,*,#33983,.F.);
#44666=ORIENTED_EDGE('',*,*,#33984,.F.);
#44667=ORIENTED_EDGE('',*,*,#33985,.F.);
#44668=ORIENTED_EDGE('',*,*,#33986,.F.);
#44669=ORIENTED_EDGE('',*,*,#33987,.F.);
#44670=ORIENTED_EDGE('',*,*,#33988,.F.);
#44671=ORIENTED_EDGE('',*,*,#33989,.F.);
#44672=ORIENTED_EDGE('',*,*,#33990,.F.);
#44673=ORIENTED_EDGE('',*,*,#33991,.F.);
#44674=ORIENTED_EDGE('',*,*,#33992,.F.);
#44675=ORIENTED_EDGE('',*,*,#33993,.F.);
#44676=ORIENTED_EDGE('',*,*,#33994,.F.);
#44677=ORIENTED_EDGE('',*,*,#33995,.F.);
#44678=ORIENTED_EDGE('',*,*,#33996,.F.);
#44679=ORIENTED_EDGE('',*,*,#33997,.F.);
#44680=ORIENTED_EDGE('',*,*,#33998,.F.);
#44681=ORIENTED_EDGE('',*,*,#33999,.F.);
#44682=ORIENTED_EDGE('',*,*,#34000,.F.);
#44683=ORIENTED_EDGE('',*,*,#34001,.F.);
#44684=ORIENTED_EDGE('',*,*,#34002,.F.);
#44685=ORIENTED_EDGE('',*,*,#34003,.F.);
#44686=ORIENTED_EDGE('',*,*,#34004,.F.);
#44687=ORIENTED_EDGE('',*,*,#34005,.F.);
#44688=ORIENTED_EDGE('',*,*,#34006,.F.);
#44689=ORIENTED_EDGE('',*,*,#34007,.F.);
#44690=ORIENTED_EDGE('',*,*,#34008,.F.);
#44691=ORIENTED_EDGE('',*,*,#34009,.F.);
#44692=ORIENTED_EDGE('',*,*,#34010,.F.);
#44693=ORIENTED_EDGE('',*,*,#34011,.F.);
#44694=ORIENTED_EDGE('',*,*,#34012,.F.);
#44695=ORIENTED_EDGE('',*,*,#34013,.F.);
#44696=ORIENTED_EDGE('',*,*,#34014,.F.);
#44697=ORIENTED_EDGE('',*,*,#34015,.F.);
#44698=ORIENTED_EDGE('',*,*,#34016,.F.);
#44699=ORIENTED_EDGE('',*,*,#34017,.F.);
#44700=ORIENTED_EDGE('',*,*,#34018,.F.);
#44701=ORIENTED_EDGE('',*,*,#34019,.F.);
#44702=ORIENTED_EDGE('',*,*,#34020,.F.);
#44703=ORIENTED_EDGE('',*,*,#34021,.F.);
#44704=ORIENTED_EDGE('',*,*,#34022,.F.);
#44705=ORIENTED_EDGE('',*,*,#34023,.F.);
#44706=ORIENTED_EDGE('',*,*,#34024,.F.);
#44707=ORIENTED_EDGE('',*,*,#34025,.F.);
#44708=ORIENTED_EDGE('',*,*,#34026,.F.);
#44709=ORIENTED_EDGE('',*,*,#34027,.F.);
#44710=ORIENTED_EDGE('',*,*,#34028,.F.);
#44711=ORIENTED_EDGE('',*,*,#34029,.F.);
#44712=ORIENTED_EDGE('',*,*,#34030,.F.);
#44713=ORIENTED_EDGE('',*,*,#34031,.F.);
#44714=ORIENTED_EDGE('',*,*,#34032,.F.);
#44715=ORIENTED_EDGE('',*,*,#34033,.F.);
#44716=ORIENTED_EDGE('',*,*,#34034,.F.);
#44717=ORIENTED_EDGE('',*,*,#34035,.F.);
#44718=ORIENTED_EDGE('',*,*,#34036,.F.);
#44719=ORIENTED_EDGE('',*,*,#34037,.F.);
#44720=ORIENTED_EDGE('',*,*,#34038,.F.);
#44721=ORIENTED_EDGE('',*,*,#34039,.F.);
#44722=ORIENTED_EDGE('',*,*,#34040,.F.);
#44723=ORIENTED_EDGE('',*,*,#34041,.F.);
#44724=ORIENTED_EDGE('',*,*,#34042,.F.);
#44725=ORIENTED_EDGE('',*,*,#34043,.F.);
#44726=ORIENTED_EDGE('',*,*,#34044,.F.);
#44727=ORIENTED_EDGE('',*,*,#34045,.F.);
#44728=ORIENTED_EDGE('',*,*,#34046,.F.);
#44729=ORIENTED_EDGE('',*,*,#34047,.F.);
#44730=ORIENTED_EDGE('',*,*,#34048,.F.);
#44731=ORIENTED_EDGE('',*,*,#34049,.F.);
#44732=ORIENTED_EDGE('',*,*,#34050,.F.);
#44733=ORIENTED_EDGE('',*,*,#34051,.F.);
#44734=ORIENTED_EDGE('',*,*,#34052,.F.);
#44735=ORIENTED_EDGE('',*,*,#34053,.F.);
#44736=ORIENTED_EDGE('',*,*,#34054,.F.);
#44737=ORIENTED_EDGE('',*,*,#34055,.F.);
#44738=ORIENTED_EDGE('',*,*,#34056,.F.);
#44739=ORIENTED_EDGE('',*,*,#34057,.F.);
#44740=ORIENTED_EDGE('',*,*,#34058,.F.);
#44741=ORIENTED_EDGE('',*,*,#34059,.F.);
#44742=ORIENTED_EDGE('',*,*,#34060,.F.);
#44743=ORIENTED_EDGE('',*,*,#34061,.F.);
#44744=ORIENTED_EDGE('',*,*,#34062,.F.);
#44745=ORIENTED_EDGE('',*,*,#34063,.F.);
#44746=ORIENTED_EDGE('',*,*,#34064,.F.);
#44747=ORIENTED_EDGE('',*,*,#34065,.F.);
#44748=ORIENTED_EDGE('',*,*,#34066,.F.);
#44749=ORIENTED_EDGE('',*,*,#34067,.F.);
#44750=ORIENTED_EDGE('',*,*,#34068,.F.);
#44751=ORIENTED_EDGE('',*,*,#34069,.F.);
#44752=ORIENTED_EDGE('',*,*,#34070,.F.);
#44753=ORIENTED_EDGE('',*,*,#34071,.F.);
#44754=ORIENTED_EDGE('',*,*,#34072,.F.);
#44755=ORIENTED_EDGE('',*,*,#34073,.F.);
#44756=ORIENTED_EDGE('',*,*,#34074,.F.);
#44757=ORIENTED_EDGE('',*,*,#34075,.F.);
#44758=ORIENTED_EDGE('',*,*,#34076,.F.);
#44759=ORIENTED_EDGE('',*,*,#34077,.F.);
#44760=ORIENTED_EDGE('',*,*,#34078,.F.);
#44761=ORIENTED_EDGE('',*,*,#34079,.F.);
#44762=ORIENTED_EDGE('',*,*,#34080,.F.);
#44763=ORIENTED_EDGE('',*,*,#34081,.F.);
#44764=ORIENTED_EDGE('',*,*,#34082,.F.);
#44765=ORIENTED_EDGE('',*,*,#34083,.F.);
#44766=ORIENTED_EDGE('',*,*,#34084,.F.);
#44767=ORIENTED_EDGE('',*,*,#34085,.F.);
#44768=ORIENTED_EDGE('',*,*,#34086,.F.);
#44769=ORIENTED_EDGE('',*,*,#34087,.F.);
#44770=ORIENTED_EDGE('',*,*,#34088,.F.);
#44771=ORIENTED_EDGE('',*,*,#34089,.F.);
#44772=ORIENTED_EDGE('',*,*,#34090,.F.);
#44773=ORIENTED_EDGE('',*,*,#34091,.F.);
#44774=ORIENTED_EDGE('',*,*,#34092,.F.);
#44775=ORIENTED_EDGE('',*,*,#34093,.F.);
#44776=ORIENTED_EDGE('',*,*,#34094,.F.);
#44777=ORIENTED_EDGE('',*,*,#34095,.F.);
#44778=ORIENTED_EDGE('',*,*,#34096,.F.);
#44779=ORIENTED_EDGE('',*,*,#34097,.F.);
#44780=ORIENTED_EDGE('',*,*,#34098,.F.);
#44781=ORIENTED_EDGE('',*,*,#34099,.F.);
#44782=ORIENTED_EDGE('',*,*,#34100,.F.);
#44783=ORIENTED_EDGE('',*,*,#34101,.F.);
#44784=ORIENTED_EDGE('',*,*,#34102,.F.);
#44785=ORIENTED_EDGE('',*,*,#34103,.F.);
#44786=ORIENTED_EDGE('',*,*,#34104,.F.);
#44787=ORIENTED_EDGE('',*,*,#34105,.F.);
#44788=ORIENTED_EDGE('',*,*,#34106,.F.);
#44789=ORIENTED_EDGE('',*,*,#34107,.F.);
#44790=ORIENTED_EDGE('',*,*,#34108,.F.);
#44791=ORIENTED_EDGE('',*,*,#34109,.F.);
#44792=ORIENTED_EDGE('',*,*,#34110,.F.);
#44793=ORIENTED_EDGE('',*,*,#34111,.F.);
#44794=ORIENTED_EDGE('',*,*,#34112,.F.);
#44795=ORIENTED_EDGE('',*,*,#34113,.F.);
#44796=ORIENTED_EDGE('',*,*,#34114,.F.);
#44797=ORIENTED_EDGE('',*,*,#34115,.F.);
#44798=ORIENTED_EDGE('',*,*,#34116,.F.);
#44799=ORIENTED_EDGE('',*,*,#34117,.F.);
#44800=ORIENTED_EDGE('',*,*,#34118,.F.);
#44801=ORIENTED_EDGE('',*,*,#34119,.F.);
#44802=ORIENTED_EDGE('',*,*,#34120,.F.);
#44803=ORIENTED_EDGE('',*,*,#34121,.F.);
#44804=ORIENTED_EDGE('',*,*,#34122,.F.);
#44805=ORIENTED_EDGE('',*,*,#34123,.F.);
#44806=ORIENTED_EDGE('',*,*,#34124,.F.);
#44807=ORIENTED_EDGE('',*,*,#34125,.F.);
#44808=ORIENTED_EDGE('',*,*,#34126,.F.);
#44809=ORIENTED_EDGE('',*,*,#34127,.F.);
#44810=ORIENTED_EDGE('',*,*,#34128,.F.);
#44811=ORIENTED_EDGE('',*,*,#34129,.F.);
#44812=ORIENTED_EDGE('',*,*,#34130,.F.);
#44813=ORIENTED_EDGE('',*,*,#34131,.F.);
#44814=ORIENTED_EDGE('',*,*,#34132,.F.);
#44815=ORIENTED_EDGE('',*,*,#34133,.F.);
#44816=ORIENTED_EDGE('',*,*,#34134,.F.);
#44817=ORIENTED_EDGE('',*,*,#34135,.F.);
#44818=ORIENTED_EDGE('',*,*,#34136,.F.);
#44819=ORIENTED_EDGE('',*,*,#34137,.F.);
#44820=ORIENTED_EDGE('',*,*,#34138,.T.);
#44821=ORIENTED_EDGE('',*,*,#34139,.F.);
#44822=ORIENTED_EDGE('',*,*,#34138,.F.);
#44823=ORIENTED_EDGE('',*,*,#34140,.F.);
#44824=ORIENTED_EDGE('',*,*,#34141,.F.);
#44825=ORIENTED_EDGE('',*,*,#34142,.T.);
#44826=ORIENTED_EDGE('',*,*,#34143,.T.);
#44827=ORIENTED_EDGE('',*,*,#34144,.T.);
#44828=ORIENTED_EDGE('',*,*,#34143,.F.);
#44829=ORIENTED_EDGE('',*,*,#33964,.T.);
#44830=ORIENTED_EDGE('',*,*,#34145,.F.);
#44831=ORIENTED_EDGE('',*,*,#34146,.F.);
#44832=ORIENTED_EDGE('',*,*,#34147,.T.);
#44833=ORIENTED_EDGE('',*,*,#34148,.T.);
#44834=ORIENTED_EDGE('',*,*,#34149,.F.);
#44835=ORIENTED_EDGE('',*,*,#34148,.F.);
#44836=ORIENTED_EDGE('',*,*,#34150,.T.);
#44837=ORIENTED_EDGE('',*,*,#34151,.T.);
#44838=ORIENTED_EDGE('',*,*,#34152,.F.);
#44839=ORIENTED_EDGE('',*,*,#34151,.F.);
#44840=ORIENTED_EDGE('',*,*,#34153,.T.);
#44841=ORIENTED_EDGE('',*,*,#34150,.F.);
#44842=ORIENTED_EDGE('',*,*,#34154,.T.);
#44843=ORIENTED_EDGE('',*,*,#34155,.T.);
#44844=ORIENTED_EDGE('',*,*,#34154,.F.);
#44845=ORIENTED_EDGE('',*,*,#34153,.F.);
#44846=ORIENTED_EDGE('',*,*,#34156,.F.);
#44847=ORIENTED_EDGE('',*,*,#34157,.F.);
#44848=ORIENTED_EDGE('',*,*,#34158,.F.);
#44849=ORIENTED_EDGE('',*,*,#34159,.F.);
#44850=ORIENTED_EDGE('',*,*,#34160,.F.);
#44851=ORIENTED_EDGE('',*,*,#34161,.F.);
#44852=ORIENTED_EDGE('',*,*,#34162,.F.);
#44853=ORIENTED_EDGE('',*,*,#34163,.F.);
#44854=ORIENTED_EDGE('',*,*,#34164,.F.);
#44855=ORIENTED_EDGE('',*,*,#34165,.F.);
#44856=ORIENTED_EDGE('',*,*,#34166,.F.);
#44857=ORIENTED_EDGE('',*,*,#34167,.F.);
#44858=ORIENTED_EDGE('',*,*,#34168,.F.);
#44859=ORIENTED_EDGE('',*,*,#34169,.F.);
#44860=ORIENTED_EDGE('',*,*,#34170,.F.);
#44861=ORIENTED_EDGE('',*,*,#34171,.F.);
#44862=ORIENTED_EDGE('',*,*,#34172,.F.);
#44863=ORIENTED_EDGE('',*,*,#34173,.F.);
#44864=ORIENTED_EDGE('',*,*,#34174,.F.);
#44865=ORIENTED_EDGE('',*,*,#34175,.F.);
#44866=ORIENTED_EDGE('',*,*,#34176,.F.);
#44867=ORIENTED_EDGE('',*,*,#34177,.F.);
#44868=ORIENTED_EDGE('',*,*,#34178,.F.);
#44869=ORIENTED_EDGE('',*,*,#34179,.F.);
#44870=ORIENTED_EDGE('',*,*,#34180,.F.);
#44871=ORIENTED_EDGE('',*,*,#34181,.F.);
#44872=ORIENTED_EDGE('',*,*,#34182,.F.);
#44873=ORIENTED_EDGE('',*,*,#34183,.F.);
#44874=ORIENTED_EDGE('',*,*,#34184,.F.);
#44875=ORIENTED_EDGE('',*,*,#34185,.F.);
#44876=ORIENTED_EDGE('',*,*,#34186,.F.);
#44877=ORIENTED_EDGE('',*,*,#34187,.F.);
#44878=ORIENTED_EDGE('',*,*,#34188,.F.);
#44879=ORIENTED_EDGE('',*,*,#34189,.F.);
#44880=ORIENTED_EDGE('',*,*,#34190,.F.);
#44881=ORIENTED_EDGE('',*,*,#34191,.F.);
#44882=ORIENTED_EDGE('',*,*,#34192,.F.);
#44883=ORIENTED_EDGE('',*,*,#34193,.F.);
#44884=ORIENTED_EDGE('',*,*,#34194,.F.);
#44885=ORIENTED_EDGE('',*,*,#34195,.F.);
#44886=ORIENTED_EDGE('',*,*,#34196,.F.);
#44887=ORIENTED_EDGE('',*,*,#34197,.F.);
#44888=ORIENTED_EDGE('',*,*,#34198,.F.);
#44889=ORIENTED_EDGE('',*,*,#34199,.F.);
#44890=ORIENTED_EDGE('',*,*,#34200,.F.);
#44891=ORIENTED_EDGE('',*,*,#34201,.F.);
#44892=ORIENTED_EDGE('',*,*,#34202,.F.);
#44893=ORIENTED_EDGE('',*,*,#34203,.F.);
#44894=ORIENTED_EDGE('',*,*,#34204,.F.);
#44895=ORIENTED_EDGE('',*,*,#34205,.F.);
#44896=ORIENTED_EDGE('',*,*,#34206,.F.);
#44897=ORIENTED_EDGE('',*,*,#34207,.F.);
#44898=ORIENTED_EDGE('',*,*,#34208,.F.);
#44899=ORIENTED_EDGE('',*,*,#34209,.F.);
#44900=ORIENTED_EDGE('',*,*,#34210,.F.);
#44901=ORIENTED_EDGE('',*,*,#34211,.F.);
#44902=ORIENTED_EDGE('',*,*,#34212,.F.);
#44903=ORIENTED_EDGE('',*,*,#34213,.F.);
#44904=ORIENTED_EDGE('',*,*,#34214,.F.);
#44905=ORIENTED_EDGE('',*,*,#34215,.F.);
#44906=ORIENTED_EDGE('',*,*,#34216,.F.);
#44907=ORIENTED_EDGE('',*,*,#34217,.F.);
#44908=ORIENTED_EDGE('',*,*,#34218,.F.);
#44909=ORIENTED_EDGE('',*,*,#34219,.F.);
#44910=ORIENTED_EDGE('',*,*,#34220,.F.);
#44911=ORIENTED_EDGE('',*,*,#34221,.F.);
#44912=ORIENTED_EDGE('',*,*,#34222,.F.);
#44913=ORIENTED_EDGE('',*,*,#34223,.F.);
#44914=ORIENTED_EDGE('',*,*,#34224,.F.);
#44915=ORIENTED_EDGE('',*,*,#34225,.F.);
#44916=ORIENTED_EDGE('',*,*,#34226,.F.);
#44917=ORIENTED_EDGE('',*,*,#34227,.F.);
#44918=ORIENTED_EDGE('',*,*,#34228,.F.);
#44919=ORIENTED_EDGE('',*,*,#34229,.F.);
#44920=ORIENTED_EDGE('',*,*,#34230,.F.);
#44921=ORIENTED_EDGE('',*,*,#34231,.F.);
#44922=ORIENTED_EDGE('',*,*,#34232,.F.);
#44923=ORIENTED_EDGE('',*,*,#34233,.F.);
#44924=ORIENTED_EDGE('',*,*,#34234,.F.);
#44925=ORIENTED_EDGE('',*,*,#34235,.F.);
#44926=ORIENTED_EDGE('',*,*,#34236,.F.);
#44927=ORIENTED_EDGE('',*,*,#34237,.F.);
#44928=ORIENTED_EDGE('',*,*,#34238,.F.);
#44929=ORIENTED_EDGE('',*,*,#34239,.F.);
#44930=ORIENTED_EDGE('',*,*,#34240,.F.);
#44931=ORIENTED_EDGE('',*,*,#34241,.F.);
#44932=ORIENTED_EDGE('',*,*,#34242,.F.);
#44933=ORIENTED_EDGE('',*,*,#34243,.F.);
#44934=ORIENTED_EDGE('',*,*,#34244,.T.);
#44935=ORIENTED_EDGE('',*,*,#34245,.F.);
#44936=ORIENTED_EDGE('',*,*,#34244,.F.);
#44937=ORIENTED_EDGE('',*,*,#34246,.F.);
#44938=ORIENTED_EDGE('',*,*,#34247,.F.);
#44939=ORIENTED_EDGE('',*,*,#34248,.F.);
#44940=ORIENTED_EDGE('',*,*,#34249,.F.);
#44941=ORIENTED_EDGE('',*,*,#34250,.F.);
#44942=ORIENTED_EDGE('',*,*,#34251,.F.);
#44943=ORIENTED_EDGE('',*,*,#34252,.F.);
#44944=ORIENTED_EDGE('',*,*,#34253,.F.);
#44945=ORIENTED_EDGE('',*,*,#34254,.F.);
#44946=ORIENTED_EDGE('',*,*,#34255,.F.);
#44947=ORIENTED_EDGE('',*,*,#34256,.F.);
#44948=ORIENTED_EDGE('',*,*,#34257,.F.);
#44949=ORIENTED_EDGE('',*,*,#34258,.F.);
#44950=ORIENTED_EDGE('',*,*,#34259,.F.);
#44951=ORIENTED_EDGE('',*,*,#34260,.F.);
#44952=ORIENTED_EDGE('',*,*,#34261,.F.);
#44953=ORIENTED_EDGE('',*,*,#34262,.F.);
#44954=ORIENTED_EDGE('',*,*,#34263,.F.);
#44955=ORIENTED_EDGE('',*,*,#34264,.F.);
#44956=ORIENTED_EDGE('',*,*,#34265,.F.);
#44957=ORIENTED_EDGE('',*,*,#34266,.F.);
#44958=ORIENTED_EDGE('',*,*,#34267,.F.);
#44959=ORIENTED_EDGE('',*,*,#34268,.F.);
#44960=ORIENTED_EDGE('',*,*,#34269,.F.);
#44961=ORIENTED_EDGE('',*,*,#34270,.F.);
#44962=ORIENTED_EDGE('',*,*,#34271,.F.);
#44963=ORIENTED_EDGE('',*,*,#34272,.F.);
#44964=ORIENTED_EDGE('',*,*,#34273,.F.);
#44965=ORIENTED_EDGE('',*,*,#34274,.F.);
#44966=ORIENTED_EDGE('',*,*,#34275,.F.);
#44967=ORIENTED_EDGE('',*,*,#34276,.F.);
#44968=ORIENTED_EDGE('',*,*,#34277,.F.);
#44969=ORIENTED_EDGE('',*,*,#34278,.F.);
#44970=ORIENTED_EDGE('',*,*,#34279,.F.);
#44971=ORIENTED_EDGE('',*,*,#34280,.F.);
#44972=ORIENTED_EDGE('',*,*,#34281,.F.);
#44973=ORIENTED_EDGE('',*,*,#34282,.F.);
#44974=ORIENTED_EDGE('',*,*,#34283,.F.);
#44975=ORIENTED_EDGE('',*,*,#34284,.F.);
#44976=ORIENTED_EDGE('',*,*,#34285,.F.);
#44977=ORIENTED_EDGE('',*,*,#34286,.F.);
#44978=ORIENTED_EDGE('',*,*,#34287,.F.);
#44979=ORIENTED_EDGE('',*,*,#34288,.F.);
#44980=ORIENTED_EDGE('',*,*,#34289,.F.);
#44981=ORIENTED_EDGE('',*,*,#34290,.F.);
#44982=ORIENTED_EDGE('',*,*,#34291,.F.);
#44983=ORIENTED_EDGE('',*,*,#34292,.F.);
#44984=ORIENTED_EDGE('',*,*,#34293,.F.);
#44985=ORIENTED_EDGE('',*,*,#34294,.F.);
#44986=ORIENTED_EDGE('',*,*,#34295,.F.);
#44987=ORIENTED_EDGE('',*,*,#34296,.F.);
#44988=ORIENTED_EDGE('',*,*,#34297,.F.);
#44989=ORIENTED_EDGE('',*,*,#34298,.F.);
#44990=ORIENTED_EDGE('',*,*,#34299,.F.);
#44991=ORIENTED_EDGE('',*,*,#34300,.F.);
#44992=ORIENTED_EDGE('',*,*,#34301,.F.);
#44993=ORIENTED_EDGE('',*,*,#34302,.F.);
#44994=ORIENTED_EDGE('',*,*,#34303,.F.);
#44995=ORIENTED_EDGE('',*,*,#34304,.F.);
#44996=ORIENTED_EDGE('',*,*,#34305,.F.);
#44997=ORIENTED_EDGE('',*,*,#34306,.F.);
#44998=ORIENTED_EDGE('',*,*,#34307,.F.);
#44999=ORIENTED_EDGE('',*,*,#34308,.F.);
#45000=ORIENTED_EDGE('',*,*,#34309,.F.);
#45001=ORIENTED_EDGE('',*,*,#34310,.F.);
#45002=ORIENTED_EDGE('',*,*,#34311,.F.);
#45003=ORIENTED_EDGE('',*,*,#34312,.F.);
#45004=ORIENTED_EDGE('',*,*,#34313,.F.);
#45005=ORIENTED_EDGE('',*,*,#34314,.F.);
#45006=ORIENTED_EDGE('',*,*,#34315,.F.);
#45007=ORIENTED_EDGE('',*,*,#34316,.F.);
#45008=ORIENTED_EDGE('',*,*,#34317,.F.);
#45009=ORIENTED_EDGE('',*,*,#34318,.F.);
#45010=ORIENTED_EDGE('',*,*,#34319,.F.);
#45011=ORIENTED_EDGE('',*,*,#34320,.F.);
#45012=ORIENTED_EDGE('',*,*,#34321,.F.);
#45013=ORIENTED_EDGE('',*,*,#34322,.F.);
#45014=ORIENTED_EDGE('',*,*,#34323,.F.);
#45015=ORIENTED_EDGE('',*,*,#34324,.F.);
#45016=ORIENTED_EDGE('',*,*,#34325,.F.);
#45017=ORIENTED_EDGE('',*,*,#34326,.F.);
#45018=ORIENTED_EDGE('',*,*,#34327,.F.);
#45019=ORIENTED_EDGE('',*,*,#34328,.F.);
#45020=ORIENTED_EDGE('',*,*,#34329,.F.);
#45021=ORIENTED_EDGE('',*,*,#34330,.F.);
#45022=ORIENTED_EDGE('',*,*,#34331,.F.);
#45023=ORIENTED_EDGE('',*,*,#34332,.F.);
#45024=ORIENTED_EDGE('',*,*,#34333,.F.);
#45025=ORIENTED_EDGE('',*,*,#34334,.F.);
#45026=ORIENTED_EDGE('',*,*,#34335,.F.);
#45027=ORIENTED_EDGE('',*,*,#34336,.F.);
#45028=ORIENTED_EDGE('',*,*,#34337,.F.);
#45029=ORIENTED_EDGE('',*,*,#34338,.F.);
#45030=ORIENTED_EDGE('',*,*,#34339,.F.);
#45031=ORIENTED_EDGE('',*,*,#34340,.F.);
#45032=ORIENTED_EDGE('',*,*,#34341,.F.);
#45033=ORIENTED_EDGE('',*,*,#34342,.F.);
#45034=ORIENTED_EDGE('',*,*,#34343,.F.);
#45035=ORIENTED_EDGE('',*,*,#34344,.F.);
#45036=ORIENTED_EDGE('',*,*,#34345,.F.);
#45037=ORIENTED_EDGE('',*,*,#34346,.F.);
#45038=ORIENTED_EDGE('',*,*,#34347,.F.);
#45039=ORIENTED_EDGE('',*,*,#34348,.F.);
#45040=ORIENTED_EDGE('',*,*,#34349,.F.);
#45041=ORIENTED_EDGE('',*,*,#34350,.F.);
#45042=ORIENTED_EDGE('',*,*,#34351,.F.);
#45043=ORIENTED_EDGE('',*,*,#34352,.F.);
#45044=ORIENTED_EDGE('',*,*,#34353,.F.);
#45045=ORIENTED_EDGE('',*,*,#34354,.F.);
#45046=ORIENTED_EDGE('',*,*,#34355,.F.);
#45047=ORIENTED_EDGE('',*,*,#34356,.F.);
#45048=ORIENTED_EDGE('',*,*,#34357,.F.);
#45049=ORIENTED_EDGE('',*,*,#34358,.F.);
#45050=ORIENTED_EDGE('',*,*,#34359,.F.);
#45051=ORIENTED_EDGE('',*,*,#34360,.F.);
#45052=ORIENTED_EDGE('',*,*,#34361,.F.);
#45053=ORIENTED_EDGE('',*,*,#34362,.F.);
#45054=ORIENTED_EDGE('',*,*,#34363,.F.);
#45055=ORIENTED_EDGE('',*,*,#34364,.F.);
#45056=ORIENTED_EDGE('',*,*,#34365,.F.);
#45057=ORIENTED_EDGE('',*,*,#34366,.F.);
#45058=ORIENTED_EDGE('',*,*,#34367,.F.);
#45059=ORIENTED_EDGE('',*,*,#34368,.F.);
#45060=ORIENTED_EDGE('',*,*,#34362,.T.);
#45061=ORIENTED_EDGE('',*,*,#34369,.F.);
#45062=ORIENTED_EDGE('',*,*,#34370,.F.);
#45063=ORIENTED_EDGE('',*,*,#34371,.F.);
#45064=ORIENTED_EDGE('',*,*,#34372,.F.);
#45065=ORIENTED_EDGE('',*,*,#34373,.F.);
#45066=ORIENTED_EDGE('',*,*,#34374,.F.);
#45067=ORIENTED_EDGE('',*,*,#34375,.F.);
#45068=ORIENTED_EDGE('',*,*,#34376,.F.);
#45069=ORIENTED_EDGE('',*,*,#34377,.F.);
#45070=ORIENTED_EDGE('',*,*,#34378,.F.);
#45071=ORIENTED_EDGE('',*,*,#34379,.F.);
#45072=ORIENTED_EDGE('',*,*,#34380,.F.);
#45073=ORIENTED_EDGE('',*,*,#34381,.F.);
#45074=ORIENTED_EDGE('',*,*,#34382,.F.);
#45075=ORIENTED_EDGE('',*,*,#34383,.F.);
#45076=ORIENTED_EDGE('',*,*,#34384,.F.);
#45077=ORIENTED_EDGE('',*,*,#34385,.F.);
#45078=ORIENTED_EDGE('',*,*,#34386,.F.);
#45079=ORIENTED_EDGE('',*,*,#34387,.F.);
#45080=ORIENTED_EDGE('',*,*,#34388,.F.);
#45081=ORIENTED_EDGE('',*,*,#34389,.F.);
#45082=ORIENTED_EDGE('',*,*,#34390,.F.);
#45083=ORIENTED_EDGE('',*,*,#34391,.F.);
#45084=ORIENTED_EDGE('',*,*,#34392,.F.);
#45085=ORIENTED_EDGE('',*,*,#34393,.F.);
#45086=ORIENTED_EDGE('',*,*,#34394,.F.);
#45087=ORIENTED_EDGE('',*,*,#34395,.F.);
#45088=ORIENTED_EDGE('',*,*,#34396,.F.);
#45089=ORIENTED_EDGE('',*,*,#34397,.F.);
#45090=ORIENTED_EDGE('',*,*,#34398,.F.);
#45091=ORIENTED_EDGE('',*,*,#34399,.F.);
#45092=ORIENTED_EDGE('',*,*,#34400,.F.);
#45093=ORIENTED_EDGE('',*,*,#34401,.F.);
#45094=ORIENTED_EDGE('',*,*,#34402,.F.);
#45095=ORIENTED_EDGE('',*,*,#34403,.F.);
#45096=ORIENTED_EDGE('',*,*,#34404,.F.);
#45097=ORIENTED_EDGE('',*,*,#34405,.F.);
#45098=ORIENTED_EDGE('',*,*,#34406,.F.);
#45099=ORIENTED_EDGE('',*,*,#34407,.F.);
#45100=ORIENTED_EDGE('',*,*,#34408,.F.);
#45101=ORIENTED_EDGE('',*,*,#34409,.F.);
#45102=ORIENTED_EDGE('',*,*,#34410,.F.);
#45103=ORIENTED_EDGE('',*,*,#34411,.F.);
#45104=ORIENTED_EDGE('',*,*,#34412,.F.);
#45105=ORIENTED_EDGE('',*,*,#34413,.F.);
#45106=ORIENTED_EDGE('',*,*,#34414,.F.);
#45107=ORIENTED_EDGE('',*,*,#34415,.F.);
#45108=ORIENTED_EDGE('',*,*,#34416,.F.);
#45109=ORIENTED_EDGE('',*,*,#34417,.F.);
#45110=ORIENTED_EDGE('',*,*,#34418,.F.);
#45111=ORIENTED_EDGE('',*,*,#34419,.F.);
#45112=ORIENTED_EDGE('',*,*,#34420,.F.);
#45113=ORIENTED_EDGE('',*,*,#34421,.F.);
#45114=ORIENTED_EDGE('',*,*,#34422,.F.);
#45115=ORIENTED_EDGE('',*,*,#34423,.F.);
#45116=ORIENTED_EDGE('',*,*,#34424,.F.);
#45117=ORIENTED_EDGE('',*,*,#34425,.F.);
#45118=ORIENTED_EDGE('',*,*,#34426,.F.);
#45119=ORIENTED_EDGE('',*,*,#34427,.F.);
#45120=ORIENTED_EDGE('',*,*,#34428,.F.);
#45121=ORIENTED_EDGE('',*,*,#34429,.F.);
#45122=ORIENTED_EDGE('',*,*,#34430,.F.);
#45123=ORIENTED_EDGE('',*,*,#34431,.F.);
#45124=ORIENTED_EDGE('',*,*,#34432,.F.);
#45125=ORIENTED_EDGE('',*,*,#34433,.F.);
#45126=ORIENTED_EDGE('',*,*,#34434,.F.);
#45127=ORIENTED_EDGE('',*,*,#34435,.F.);
#45128=ORIENTED_EDGE('',*,*,#34436,.F.);
#45129=ORIENTED_EDGE('',*,*,#34437,.F.);
#45130=ORIENTED_EDGE('',*,*,#34438,.F.);
#45131=ORIENTED_EDGE('',*,*,#34439,.F.);
#45132=ORIENTED_EDGE('',*,*,#34440,.F.);
#45133=ORIENTED_EDGE('',*,*,#34441,.F.);
#45134=ORIENTED_EDGE('',*,*,#34442,.F.);
#45135=ORIENTED_EDGE('',*,*,#34443,.F.);
#45136=ORIENTED_EDGE('',*,*,#34444,.F.);
#45137=ORIENTED_EDGE('',*,*,#34445,.F.);
#45138=ORIENTED_EDGE('',*,*,#34446,.F.);
#45139=ORIENTED_EDGE('',*,*,#34447,.F.);
#45140=ORIENTED_EDGE('',*,*,#34448,.F.);
#45141=ORIENTED_EDGE('',*,*,#34449,.F.);
#45142=ORIENTED_EDGE('',*,*,#34450,.F.);
#45143=ORIENTED_EDGE('',*,*,#34451,.F.);
#45144=ORIENTED_EDGE('',*,*,#34452,.F.);
#45145=ORIENTED_EDGE('',*,*,#34453,.F.);
#45146=ORIENTED_EDGE('',*,*,#34454,.F.);
#45147=ORIENTED_EDGE('',*,*,#34455,.F.);
#45148=ORIENTED_EDGE('',*,*,#34456,.F.);
#45149=ORIENTED_EDGE('',*,*,#34457,.F.);
#45150=ORIENTED_EDGE('',*,*,#34458,.F.);
#45151=ORIENTED_EDGE('',*,*,#34459,.F.);
#45152=ORIENTED_EDGE('',*,*,#34460,.F.);
#45153=ORIENTED_EDGE('',*,*,#34461,.F.);
#45154=ORIENTED_EDGE('',*,*,#34462,.F.);
#45155=ORIENTED_EDGE('',*,*,#34463,.F.);
#45156=ORIENTED_EDGE('',*,*,#34464,.F.);
#45157=ORIENTED_EDGE('',*,*,#34465,.F.);
#45158=ORIENTED_EDGE('',*,*,#34466,.F.);
#45159=ORIENTED_EDGE('',*,*,#34467,.F.);
#45160=ORIENTED_EDGE('',*,*,#34468,.F.);
#45161=ORIENTED_EDGE('',*,*,#34469,.T.);
#45162=ORIENTED_EDGE('',*,*,#34470,.F.);
#45163=ORIENTED_EDGE('',*,*,#34471,.F.);
#45164=ORIENTED_EDGE('',*,*,#34472,.F.);
#45165=ORIENTED_EDGE('',*,*,#34473,.T.);
#45166=ORIENTED_EDGE('',*,*,#34474,.F.);
#45167=ORIENTED_EDGE('',*,*,#34475,.F.);
#45168=ORIENTED_EDGE('',*,*,#34476,.F.);
#45169=ORIENTED_EDGE('',*,*,#34477,.F.);
#45170=ORIENTED_EDGE('',*,*,#34478,.F.);
#45171=ORIENTED_EDGE('',*,*,#34479,.F.);
#45172=ORIENTED_EDGE('',*,*,#34473,.F.);
#45173=ORIENTED_EDGE('',*,*,#34479,.T.);
#45174=ORIENTED_EDGE('',*,*,#34480,.F.);
#45175=ORIENTED_EDGE('',*,*,#34481,.F.);
#45176=ORIENTED_EDGE('',*,*,#34474,.T.);
#45177=ORIENTED_EDGE('',*,*,#34482,.T.);
#45178=ORIENTED_EDGE('',*,*,#34483,.F.);
#45179=ORIENTED_EDGE('',*,*,#34484,.F.);
#45180=ORIENTED_EDGE('',*,*,#34485,.F.);
#45181=ORIENTED_EDGE('',*,*,#34486,.F.);
#45182=ORIENTED_EDGE('',*,*,#34487,.F.);
#45183=ORIENTED_EDGE('',*,*,#34488,.F.);
#45184=ORIENTED_EDGE('',*,*,#34482,.F.);
#45185=ORIENTED_EDGE('',*,*,#34488,.T.);
#45186=ORIENTED_EDGE('',*,*,#34489,.F.);
#45187=ORIENTED_EDGE('',*,*,#34490,.F.);
#45188=ORIENTED_EDGE('',*,*,#34483,.T.);
#45189=ORIENTED_EDGE('',*,*,#34491,.T.);
#45190=ORIENTED_EDGE('',*,*,#34492,.F.);
#45191=ORIENTED_EDGE('',*,*,#34493,.F.);
#45192=ORIENTED_EDGE('',*,*,#34494,.F.);
#45193=ORIENTED_EDGE('',*,*,#34495,.F.);
#45194=ORIENTED_EDGE('',*,*,#34496,.F.);
#45195=ORIENTED_EDGE('',*,*,#34497,.F.);
#45196=ORIENTED_EDGE('',*,*,#34491,.F.);
#45197=ORIENTED_EDGE('',*,*,#34497,.T.);
#45198=ORIENTED_EDGE('',*,*,#34498,.F.);
#45199=ORIENTED_EDGE('',*,*,#34499,.F.);
#45200=ORIENTED_EDGE('',*,*,#34492,.T.);
#45201=ORIENTED_EDGE('',*,*,#34500,.T.);
#45202=ORIENTED_EDGE('',*,*,#34501,.F.);
#45203=ORIENTED_EDGE('',*,*,#34502,.F.);
#45204=ORIENTED_EDGE('',*,*,#34503,.F.);
#45205=ORIENTED_EDGE('',*,*,#34504,.F.);
#45206=ORIENTED_EDGE('',*,*,#34505,.F.);
#45207=ORIENTED_EDGE('',*,*,#34506,.F.);
#45208=ORIENTED_EDGE('',*,*,#34500,.F.);
#45209=ORIENTED_EDGE('',*,*,#34506,.T.);
#45210=ORIENTED_EDGE('',*,*,#34507,.F.);
#45211=ORIENTED_EDGE('',*,*,#34508,.F.);
#45212=ORIENTED_EDGE('',*,*,#34501,.T.);
#45213=ORIENTED_EDGE('',*,*,#34509,.T.);
#45214=ORIENTED_EDGE('',*,*,#34510,.F.);
#45215=ORIENTED_EDGE('',*,*,#34511,.F.);
#45216=ORIENTED_EDGE('',*,*,#34512,.F.);
#45217=ORIENTED_EDGE('',*,*,#34513,.F.);
#45218=ORIENTED_EDGE('',*,*,#34514,.F.);
#45219=ORIENTED_EDGE('',*,*,#34515,.F.);
#45220=ORIENTED_EDGE('',*,*,#34509,.F.);
#45221=ORIENTED_EDGE('',*,*,#34515,.T.);
#45222=ORIENTED_EDGE('',*,*,#34516,.F.);
#45223=ORIENTED_EDGE('',*,*,#34517,.F.);
#45224=ORIENTED_EDGE('',*,*,#34510,.T.);
#45225=ORIENTED_EDGE('',*,*,#34518,.T.);
#45226=ORIENTED_EDGE('',*,*,#34519,.F.);
#45227=ORIENTED_EDGE('',*,*,#34520,.F.);
#45228=ORIENTED_EDGE('',*,*,#34521,.F.);
#45229=ORIENTED_EDGE('',*,*,#34522,.F.);
#45230=ORIENTED_EDGE('',*,*,#34523,.F.);
#45231=ORIENTED_EDGE('',*,*,#34524,.F.);
#45232=ORIENTED_EDGE('',*,*,#34518,.F.);
#45233=ORIENTED_EDGE('',*,*,#34524,.T.);
#45234=ORIENTED_EDGE('',*,*,#34525,.F.);
#45235=ORIENTED_EDGE('',*,*,#34526,.F.);
#45236=ORIENTED_EDGE('',*,*,#34519,.T.);
#45237=ORIENTED_EDGE('',*,*,#34466,.T.);
#45238=ORIENTED_EDGE('',*,*,#34527,.F.);
#45239=ORIENTED_EDGE('',*,*,#34528,.F.);
#45240=ORIENTED_EDGE('',*,*,#34529,.F.);
#45241=ORIENTED_EDGE('',*,*,#34465,.T.);
#45242=ORIENTED_EDGE('',*,*,#34530,.F.);
#45243=ORIENTED_EDGE('',*,*,#34531,.F.);
#45244=ORIENTED_EDGE('',*,*,#34527,.T.);
#45245=ORIENTED_EDGE('',*,*,#34532,.T.);
#45246=ORIENTED_EDGE('',*,*,#34533,.F.);
#45247=ORIENTED_EDGE('',*,*,#34534,.F.);
#45248=ORIENTED_EDGE('',*,*,#34535,.F.);
#45249=ORIENTED_EDGE('',*,*,#34536,.F.);
#45250=ORIENTED_EDGE('',*,*,#34537,.F.);
#45251=ORIENTED_EDGE('',*,*,#34538,.F.);
#45252=ORIENTED_EDGE('',*,*,#34532,.F.);
#45253=ORIENTED_EDGE('',*,*,#34538,.T.);
#45254=ORIENTED_EDGE('',*,*,#34539,.F.);
#45255=ORIENTED_EDGE('',*,*,#34540,.F.);
#45256=ORIENTED_EDGE('',*,*,#34533,.T.);
#45257=ORIENTED_EDGE('',*,*,#34541,.T.);
#45258=ORIENTED_EDGE('',*,*,#34542,.F.);
#45259=ORIENTED_EDGE('',*,*,#34543,.F.);
#45260=ORIENTED_EDGE('',*,*,#34544,.F.);
#45261=ORIENTED_EDGE('',*,*,#34545,.F.);
#45262=ORIENTED_EDGE('',*,*,#34546,.F.);
#45263=ORIENTED_EDGE('',*,*,#34547,.F.);
#45264=ORIENTED_EDGE('',*,*,#34541,.F.);
#45265=ORIENTED_EDGE('',*,*,#34547,.T.);
#45266=ORIENTED_EDGE('',*,*,#34548,.F.);
#45267=ORIENTED_EDGE('',*,*,#34549,.F.);
#45268=ORIENTED_EDGE('',*,*,#34542,.T.);
#45269=ORIENTED_EDGE('',*,*,#34550,.T.);
#45270=ORIENTED_EDGE('',*,*,#34551,.F.);
#45271=ORIENTED_EDGE('',*,*,#34552,.F.);
#45272=ORIENTED_EDGE('',*,*,#34553,.F.);
#45273=ORIENTED_EDGE('',*,*,#34554,.F.);
#45274=ORIENTED_EDGE('',*,*,#34555,.F.);
#45275=ORIENTED_EDGE('',*,*,#34556,.F.);
#45276=ORIENTED_EDGE('',*,*,#34550,.F.);
#45277=ORIENTED_EDGE('',*,*,#34556,.T.);
#45278=ORIENTED_EDGE('',*,*,#34557,.F.);
#45279=ORIENTED_EDGE('',*,*,#34558,.F.);
#45280=ORIENTED_EDGE('',*,*,#34551,.T.);
#45281=ORIENTED_EDGE('',*,*,#34559,.T.);
#45282=ORIENTED_EDGE('',*,*,#34560,.F.);
#45283=ORIENTED_EDGE('',*,*,#34561,.F.);
#45284=ORIENTED_EDGE('',*,*,#34562,.F.);
#45285=ORIENTED_EDGE('',*,*,#34563,.F.);
#45286=ORIENTED_EDGE('',*,*,#34564,.F.);
#45287=ORIENTED_EDGE('',*,*,#34565,.F.);
#45288=ORIENTED_EDGE('',*,*,#34559,.F.);
#45289=ORIENTED_EDGE('',*,*,#34565,.T.);
#45290=ORIENTED_EDGE('',*,*,#34566,.F.);
#45291=ORIENTED_EDGE('',*,*,#34567,.F.);
#45292=ORIENTED_EDGE('',*,*,#34560,.T.);
#45293=ORIENTED_EDGE('',*,*,#34568,.T.);
#45294=ORIENTED_EDGE('',*,*,#34569,.F.);
#45295=ORIENTED_EDGE('',*,*,#34570,.F.);
#45296=ORIENTED_EDGE('',*,*,#34571,.F.);
#45297=ORIENTED_EDGE('',*,*,#34572,.F.);
#45298=ORIENTED_EDGE('',*,*,#34573,.F.);
#45299=ORIENTED_EDGE('',*,*,#34574,.F.);
#45300=ORIENTED_EDGE('',*,*,#34568,.F.);
#45301=ORIENTED_EDGE('',*,*,#34574,.T.);
#45302=ORIENTED_EDGE('',*,*,#34575,.F.);
#45303=ORIENTED_EDGE('',*,*,#34576,.F.);
#45304=ORIENTED_EDGE('',*,*,#34569,.T.);
#45305=ORIENTED_EDGE('',*,*,#34577,.T.);
#45306=ORIENTED_EDGE('',*,*,#34578,.F.);
#45307=ORIENTED_EDGE('',*,*,#34579,.F.);
#45308=ORIENTED_EDGE('',*,*,#34580,.F.);
#45309=ORIENTED_EDGE('',*,*,#34581,.F.);
#45310=ORIENTED_EDGE('',*,*,#34582,.F.);
#45311=ORIENTED_EDGE('',*,*,#34583,.F.);
#45312=ORIENTED_EDGE('',*,*,#34577,.F.);
#45313=ORIENTED_EDGE('',*,*,#34583,.T.);
#45314=ORIENTED_EDGE('',*,*,#34584,.F.);
#45315=ORIENTED_EDGE('',*,*,#34585,.F.);
#45316=ORIENTED_EDGE('',*,*,#34578,.T.);
#45317=ORIENTED_EDGE('',*,*,#34586,.T.);
#45318=ORIENTED_EDGE('',*,*,#34587,.F.);
#45319=ORIENTED_EDGE('',*,*,#34588,.F.);
#45320=ORIENTED_EDGE('',*,*,#34589,.F.);
#45321=ORIENTED_EDGE('',*,*,#34590,.F.);
#45322=ORIENTED_EDGE('',*,*,#34591,.F.);
#45323=ORIENTED_EDGE('',*,*,#34592,.F.);
#45324=ORIENTED_EDGE('',*,*,#34586,.F.);
#45325=ORIENTED_EDGE('',*,*,#34592,.T.);
#45326=ORIENTED_EDGE('',*,*,#34593,.F.);
#45327=ORIENTED_EDGE('',*,*,#34594,.F.);
#45328=ORIENTED_EDGE('',*,*,#34587,.T.);
#45329=ORIENTED_EDGE('',*,*,#34595,.T.);
#45330=ORIENTED_EDGE('',*,*,#34596,.F.);
#45331=ORIENTED_EDGE('',*,*,#34597,.F.);
#45332=ORIENTED_EDGE('',*,*,#34598,.F.);
#45333=ORIENTED_EDGE('',*,*,#34599,.F.);
#45334=ORIENTED_EDGE('',*,*,#34600,.F.);
#45335=ORIENTED_EDGE('',*,*,#34601,.F.);
#45336=ORIENTED_EDGE('',*,*,#34595,.F.);
#45337=ORIENTED_EDGE('',*,*,#34601,.T.);
#45338=ORIENTED_EDGE('',*,*,#34602,.F.);
#45339=ORIENTED_EDGE('',*,*,#34603,.F.);
#45340=ORIENTED_EDGE('',*,*,#34596,.T.);
#45341=ORIENTED_EDGE('',*,*,#34604,.T.);
#45342=ORIENTED_EDGE('',*,*,#34605,.F.);
#45343=ORIENTED_EDGE('',*,*,#34606,.F.);
#45344=ORIENTED_EDGE('',*,*,#34607,.F.);
#45345=ORIENTED_EDGE('',*,*,#34608,.F.);
#45346=ORIENTED_EDGE('',*,*,#34609,.F.);
#45347=ORIENTED_EDGE('',*,*,#34610,.F.);
#45348=ORIENTED_EDGE('',*,*,#34604,.F.);
#45349=ORIENTED_EDGE('',*,*,#34610,.T.);
#45350=ORIENTED_EDGE('',*,*,#34611,.F.);
#45351=ORIENTED_EDGE('',*,*,#34612,.F.);
#45352=ORIENTED_EDGE('',*,*,#34605,.T.);
#45353=ORIENTED_EDGE('',*,*,#34613,.T.);
#45354=ORIENTED_EDGE('',*,*,#34614,.F.);
#45355=ORIENTED_EDGE('',*,*,#34615,.F.);
#45356=ORIENTED_EDGE('',*,*,#34616,.F.);
#45357=ORIENTED_EDGE('',*,*,#34617,.F.);
#45358=ORIENTED_EDGE('',*,*,#34618,.F.);
#45359=ORIENTED_EDGE('',*,*,#34619,.F.);
#45360=ORIENTED_EDGE('',*,*,#34613,.F.);
#45361=ORIENTED_EDGE('',*,*,#34619,.T.);
#45362=ORIENTED_EDGE('',*,*,#34620,.F.);
#45363=ORIENTED_EDGE('',*,*,#34621,.F.);
#45364=ORIENTED_EDGE('',*,*,#34614,.T.);
#45365=ORIENTED_EDGE('',*,*,#34622,.T.);
#45366=ORIENTED_EDGE('',*,*,#34623,.F.);
#45367=ORIENTED_EDGE('',*,*,#34624,.F.);
#45368=ORIENTED_EDGE('',*,*,#34625,.F.);
#45369=ORIENTED_EDGE('',*,*,#34626,.F.);
#45370=ORIENTED_EDGE('',*,*,#34627,.F.);
#45371=ORIENTED_EDGE('',*,*,#34628,.F.);
#45372=ORIENTED_EDGE('',*,*,#34622,.F.);
#45373=ORIENTED_EDGE('',*,*,#34628,.T.);
#45374=ORIENTED_EDGE('',*,*,#34629,.F.);
#45375=ORIENTED_EDGE('',*,*,#34630,.F.);
#45376=ORIENTED_EDGE('',*,*,#34623,.T.);
#45377=ORIENTED_EDGE('',*,*,#34631,.T.);
#45378=ORIENTED_EDGE('',*,*,#34632,.F.);
#45379=ORIENTED_EDGE('',*,*,#34633,.F.);
#45380=ORIENTED_EDGE('',*,*,#34634,.F.);
#45381=ORIENTED_EDGE('',*,*,#34635,.F.);
#45382=ORIENTED_EDGE('',*,*,#34636,.F.);
#45383=ORIENTED_EDGE('',*,*,#34637,.F.);
#45384=ORIENTED_EDGE('',*,*,#34631,.F.);
#45385=ORIENTED_EDGE('',*,*,#34637,.T.);
#45386=ORIENTED_EDGE('',*,*,#34638,.F.);
#45387=ORIENTED_EDGE('',*,*,#34639,.F.);
#45388=ORIENTED_EDGE('',*,*,#34632,.T.);
#45389=ORIENTED_EDGE('',*,*,#34640,.T.);
#45390=ORIENTED_EDGE('',*,*,#34641,.F.);
#45391=ORIENTED_EDGE('',*,*,#34642,.F.);
#45392=ORIENTED_EDGE('',*,*,#34643,.F.);
#45393=ORIENTED_EDGE('',*,*,#34644,.F.);
#45394=ORIENTED_EDGE('',*,*,#34645,.F.);
#45395=ORIENTED_EDGE('',*,*,#34646,.F.);
#45396=ORIENTED_EDGE('',*,*,#34640,.F.);
#45397=ORIENTED_EDGE('',*,*,#34646,.T.);
#45398=ORIENTED_EDGE('',*,*,#34647,.F.);
#45399=ORIENTED_EDGE('',*,*,#34648,.F.);
#45400=ORIENTED_EDGE('',*,*,#34641,.T.);
#45401=ORIENTED_EDGE('',*,*,#34649,.T.);
#45402=ORIENTED_EDGE('',*,*,#34650,.F.);
#45403=ORIENTED_EDGE('',*,*,#34651,.F.);
#45404=ORIENTED_EDGE('',*,*,#34652,.F.);
#45405=ORIENTED_EDGE('',*,*,#34653,.F.);
#45406=ORIENTED_EDGE('',*,*,#34654,.F.);
#45407=ORIENTED_EDGE('',*,*,#34655,.F.);
#45408=ORIENTED_EDGE('',*,*,#34649,.F.);
#45409=ORIENTED_EDGE('',*,*,#34655,.T.);
#45410=ORIENTED_EDGE('',*,*,#34656,.F.);
#45411=ORIENTED_EDGE('',*,*,#34657,.F.);
#45412=ORIENTED_EDGE('',*,*,#34650,.T.);
#45413=ORIENTED_EDGE('',*,*,#34658,.T.);
#45414=ORIENTED_EDGE('',*,*,#34659,.F.);
#45415=ORIENTED_EDGE('',*,*,#34660,.F.);
#45416=ORIENTED_EDGE('',*,*,#34661,.F.);
#45417=ORIENTED_EDGE('',*,*,#34662,.F.);
#45418=ORIENTED_EDGE('',*,*,#34663,.F.);
#45419=ORIENTED_EDGE('',*,*,#34664,.F.);
#45420=ORIENTED_EDGE('',*,*,#34658,.F.);
#45421=ORIENTED_EDGE('',*,*,#34664,.T.);
#45422=ORIENTED_EDGE('',*,*,#34665,.F.);
#45423=ORIENTED_EDGE('',*,*,#34666,.F.);
#45424=ORIENTED_EDGE('',*,*,#34659,.T.);
#45425=ORIENTED_EDGE('',*,*,#34667,.T.);
#45426=ORIENTED_EDGE('',*,*,#34668,.F.);
#45427=ORIENTED_EDGE('',*,*,#34669,.F.);
#45428=ORIENTED_EDGE('',*,*,#34670,.F.);
#45429=ORIENTED_EDGE('',*,*,#34671,.F.);
#45430=ORIENTED_EDGE('',*,*,#34672,.F.);
#45431=ORIENTED_EDGE('',*,*,#34673,.F.);
#45432=ORIENTED_EDGE('',*,*,#34667,.F.);
#45433=ORIENTED_EDGE('',*,*,#34673,.T.);
#45434=ORIENTED_EDGE('',*,*,#34674,.F.);
#45435=ORIENTED_EDGE('',*,*,#34675,.F.);
#45436=ORIENTED_EDGE('',*,*,#34668,.T.);
#45437=ORIENTED_EDGE('',*,*,#34676,.T.);
#45438=ORIENTED_EDGE('',*,*,#34677,.F.);
#45439=ORIENTED_EDGE('',*,*,#34678,.F.);
#45440=ORIENTED_EDGE('',*,*,#34679,.F.);
#45441=ORIENTED_EDGE('',*,*,#34680,.F.);
#45442=ORIENTED_EDGE('',*,*,#34681,.F.);
#45443=ORIENTED_EDGE('',*,*,#34682,.F.);
#45444=ORIENTED_EDGE('',*,*,#34676,.F.);
#45445=ORIENTED_EDGE('',*,*,#34682,.T.);
#45446=ORIENTED_EDGE('',*,*,#34683,.F.);
#45447=ORIENTED_EDGE('',*,*,#34684,.F.);
#45448=ORIENTED_EDGE('',*,*,#34677,.T.);
#45449=ORIENTED_EDGE('',*,*,#34685,.T.);
#45450=ORIENTED_EDGE('',*,*,#34686,.F.);
#45451=ORIENTED_EDGE('',*,*,#34687,.F.);
#45452=ORIENTED_EDGE('',*,*,#34688,.F.);
#45453=ORIENTED_EDGE('',*,*,#34689,.T.);
#45454=ORIENTED_EDGE('',*,*,#34690,.F.);
#45455=ORIENTED_EDGE('',*,*,#34691,.F.);
#45456=ORIENTED_EDGE('',*,*,#34686,.T.);
#45457=ORIENTED_EDGE('',*,*,#34692,.F.);
#45458=ORIENTED_EDGE('',*,*,#34693,.F.);
#45459=ORIENTED_EDGE('',*,*,#34689,.F.);
#45460=ORIENTED_EDGE('',*,*,#34685,.F.);
#45461=ORIENTED_EDGE('',*,*,#34694,.T.);
#45462=ORIENTED_EDGE('',*,*,#34695,.F.);
#45463=ORIENTED_EDGE('',*,*,#34696,.F.);
#45464=ORIENTED_EDGE('',*,*,#34697,.F.);
#45465=ORIENTED_EDGE('',*,*,#34698,.F.);
#45466=ORIENTED_EDGE('',*,*,#34694,.F.);
#45467=ORIENTED_EDGE('',*,*,#34699,.F.);
#45468=ORIENTED_EDGE('',*,*,#34700,.F.);
#45469=ORIENTED_EDGE('',*,*,#34701,.F.);
#45470=ORIENTED_EDGE('',*,*,#34695,.T.);
#45471=ORIENTED_EDGE('',*,*,#34698,.T.);
#45472=ORIENTED_EDGE('',*,*,#34702,.F.);
#45473=ORIENTED_EDGE('',*,*,#34703,.T.);
#45474=ORIENTED_EDGE('',*,*,#34704,.F.);
#45475=ORIENTED_EDGE('',*,*,#34705,.F.);
#45476=ORIENTED_EDGE('',*,*,#34706,.F.);
#45477=ORIENTED_EDGE('',*,*,#34707,.F.);
#45478=ORIENTED_EDGE('',*,*,#34708,.F.);
#45479=ORIENTED_EDGE('',*,*,#34709,.F.);
#45480=ORIENTED_EDGE('',*,*,#34703,.F.);
#45481=ORIENTED_EDGE('',*,*,#34709,.T.);
#45482=ORIENTED_EDGE('',*,*,#34710,.F.);
#45483=ORIENTED_EDGE('',*,*,#34711,.F.);
#45484=ORIENTED_EDGE('',*,*,#34704,.T.);
#45485=ORIENTED_EDGE('',*,*,#34712,.T.);
#45486=ORIENTED_EDGE('',*,*,#34713,.F.);
#45487=ORIENTED_EDGE('',*,*,#34714,.F.);
#45488=ORIENTED_EDGE('',*,*,#34715,.F.);
#45489=ORIENTED_EDGE('',*,*,#34716,.F.);
#45490=ORIENTED_EDGE('',*,*,#34717,.F.);
#45491=ORIENTED_EDGE('',*,*,#34718,.F.);
#45492=ORIENTED_EDGE('',*,*,#34712,.F.);
#45493=ORIENTED_EDGE('',*,*,#34718,.T.);
#45494=ORIENTED_EDGE('',*,*,#34719,.F.);
#45495=ORIENTED_EDGE('',*,*,#34720,.F.);
#45496=ORIENTED_EDGE('',*,*,#34713,.T.);
#45497=ORIENTED_EDGE('',*,*,#34721,.F.);
#45498=ORIENTED_EDGE('',*,*,#34722,.F.);
#45499=ORIENTED_EDGE('',*,*,#34469,.F.);
#45500=ORIENTED_EDGE('',*,*,#34723,.F.);
#45501=ORIENTED_EDGE('',*,*,#34723,.T.);
#45502=ORIENTED_EDGE('',*,*,#34472,.T.);
#45503=ORIENTED_EDGE('',*,*,#34724,.F.);
#45504=ORIENTED_EDGE('',*,*,#34725,.F.);
#45505=ORIENTED_EDGE('',*,*,#34720,.T.);
#45506=ORIENTED_EDGE('',*,*,#34726,.F.);
#45507=ORIENTED_EDGE('',*,*,#34727,.T.);
#45508=ORIENTED_EDGE('',*,*,#34728,.F.);
#45509=ORIENTED_EDGE('',*,*,#34714,.T.);
#45510=ORIENTED_EDGE('',*,*,#34729,.F.);
#45511=ORIENTED_EDGE('',*,*,#34730,.T.);
#45512=ORIENTED_EDGE('',*,*,#34731,.F.);
#45513=ORIENTED_EDGE('',*,*,#34711,.T.);
#45514=ORIENTED_EDGE('',*,*,#34731,.T.);
#45515=ORIENTED_EDGE('',*,*,#34732,.T.);
#45516=ORIENTED_EDGE('',*,*,#34733,.F.);
#45517=ORIENTED_EDGE('',*,*,#34732,.F.);
#45518=ORIENTED_EDGE('',*,*,#34730,.F.);
#45519=ORIENTED_EDGE('',*,*,#34734,.F.);
#45520=ORIENTED_EDGE('',*,*,#34735,.F.);
#45521=ORIENTED_EDGE('',*,*,#34705,.T.);
#45522=ORIENTED_EDGE('',*,*,#34736,.F.);
#45523=ORIENTED_EDGE('',*,*,#34737,.T.);
#45524=ORIENTED_EDGE('',*,*,#34738,.F.);
#45525=ORIENTED_EDGE('',*,*,#34739,.T.);
#45526=ORIENTED_EDGE('',*,*,#34740,.F.);
#45527=ORIENTED_EDGE('',*,*,#34701,.T.);
#45528=ORIENTED_EDGE('',*,*,#34738,.T.);
#45529=ORIENTED_EDGE('',*,*,#34741,.F.);
#45530=ORIENTED_EDGE('',*,*,#34742,.F.);
#45531=ORIENTED_EDGE('',*,*,#34739,.F.);
#45532=ORIENTED_EDGE('',*,*,#34737,.F.);
#45533=ORIENTED_EDGE('',*,*,#34696,.T.);
#45534=ORIENTED_EDGE('',*,*,#34743,.F.);
#45535=ORIENTED_EDGE('',*,*,#34744,.T.);
#45536=ORIENTED_EDGE('',*,*,#34745,.F.);
#45537=ORIENTED_EDGE('',*,*,#34691,.T.);
#45538=ORIENTED_EDGE('',*,*,#34745,.T.);
#45539=ORIENTED_EDGE('',*,*,#34746,.T.);
#45540=ORIENTED_EDGE('',*,*,#34747,.F.);
#45541=ORIENTED_EDGE('',*,*,#34746,.F.);
#45542=ORIENTED_EDGE('',*,*,#34744,.F.);
#45543=ORIENTED_EDGE('',*,*,#34748,.F.);
#45544=ORIENTED_EDGE('',*,*,#34749,.F.);
#45545=ORIENTED_EDGE('',*,*,#34687,.T.);
#45546=ORIENTED_EDGE('',*,*,#34750,.F.);
#45547=ORIENTED_EDGE('',*,*,#34751,.T.);
#45548=ORIENTED_EDGE('',*,*,#34752,.F.);
#45549=ORIENTED_EDGE('',*,*,#34684,.T.);
#45550=ORIENTED_EDGE('',*,*,#34752,.T.);
#45551=ORIENTED_EDGE('',*,*,#34753,.T.);
#45552=ORIENTED_EDGE('',*,*,#34754,.F.);
#45553=ORIENTED_EDGE('',*,*,#34753,.F.);
#45554=ORIENTED_EDGE('',*,*,#34751,.F.);
#45555=ORIENTED_EDGE('',*,*,#34755,.F.);
#45556=ORIENTED_EDGE('',*,*,#34756,.F.);
#45557=ORIENTED_EDGE('',*,*,#34678,.T.);
#45558=ORIENTED_EDGE('',*,*,#34757,.F.);
#45559=ORIENTED_EDGE('',*,*,#34758,.T.);
#45560=ORIENTED_EDGE('',*,*,#34759,.F.);
#45561=ORIENTED_EDGE('',*,*,#34675,.T.);
#45562=ORIENTED_EDGE('',*,*,#34759,.T.);
#45563=ORIENTED_EDGE('',*,*,#34760,.T.);
#45564=ORIENTED_EDGE('',*,*,#34761,.F.);
#45565=ORIENTED_EDGE('',*,*,#34760,.F.);
#45566=ORIENTED_EDGE('',*,*,#34758,.F.);
#45567=ORIENTED_EDGE('',*,*,#34762,.F.);
#45568=ORIENTED_EDGE('',*,*,#34763,.F.);
#45569=ORIENTED_EDGE('',*,*,#34669,.T.);
#45570=ORIENTED_EDGE('',*,*,#34764,.F.);
#45571=ORIENTED_EDGE('',*,*,#34765,.T.);
#45572=ORIENTED_EDGE('',*,*,#34766,.F.);
#45573=ORIENTED_EDGE('',*,*,#34666,.T.);
#45574=ORIENTED_EDGE('',*,*,#34766,.T.);
#45575=ORIENTED_EDGE('',*,*,#34767,.T.);
#45576=ORIENTED_EDGE('',*,*,#34768,.F.);
#45577=ORIENTED_EDGE('',*,*,#34767,.F.);
#45578=ORIENTED_EDGE('',*,*,#34765,.F.);
#45579=ORIENTED_EDGE('',*,*,#34769,.F.);
#45580=ORIENTED_EDGE('',*,*,#34770,.F.);
#45581=ORIENTED_EDGE('',*,*,#34660,.T.);
#45582=ORIENTED_EDGE('',*,*,#34771,.F.);
#45583=ORIENTED_EDGE('',*,*,#34772,.T.);
#45584=ORIENTED_EDGE('',*,*,#34773,.F.);
#45585=ORIENTED_EDGE('',*,*,#34657,.T.);
#45586=ORIENTED_EDGE('',*,*,#34773,.T.);
#45587=ORIENTED_EDGE('',*,*,#34774,.T.);
#45588=ORIENTED_EDGE('',*,*,#34775,.F.);
#45589=ORIENTED_EDGE('',*,*,#34774,.F.);
#45590=ORIENTED_EDGE('',*,*,#34772,.F.);
#45591=ORIENTED_EDGE('',*,*,#34776,.F.);
#45592=ORIENTED_EDGE('',*,*,#34777,.F.);
#45593=ORIENTED_EDGE('',*,*,#34651,.T.);
#45594=ORIENTED_EDGE('',*,*,#34778,.F.);
#45595=ORIENTED_EDGE('',*,*,#34779,.T.);
#45596=ORIENTED_EDGE('',*,*,#34780,.F.);
#45597=ORIENTED_EDGE('',*,*,#34648,.T.);
#45598=ORIENTED_EDGE('',*,*,#34780,.T.);
#45599=ORIENTED_EDGE('',*,*,#34781,.T.);
#45600=ORIENTED_EDGE('',*,*,#34782,.F.);
#45601=ORIENTED_EDGE('',*,*,#34781,.F.);
#45602=ORIENTED_EDGE('',*,*,#34779,.F.);
#45603=ORIENTED_EDGE('',*,*,#34783,.F.);
#45604=ORIENTED_EDGE('',*,*,#34784,.F.);
#45605=ORIENTED_EDGE('',*,*,#34642,.T.);
#45606=ORIENTED_EDGE('',*,*,#34785,.F.);
#45607=ORIENTED_EDGE('',*,*,#34786,.T.);
#45608=ORIENTED_EDGE('',*,*,#34787,.F.);
#45609=ORIENTED_EDGE('',*,*,#34639,.T.);
#45610=ORIENTED_EDGE('',*,*,#34787,.T.);
#45611=ORIENTED_EDGE('',*,*,#34788,.T.);
#45612=ORIENTED_EDGE('',*,*,#34789,.F.);
#45613=ORIENTED_EDGE('',*,*,#34788,.F.);
#45614=ORIENTED_EDGE('',*,*,#34786,.F.);
#45615=ORIENTED_EDGE('',*,*,#34790,.F.);
#45616=ORIENTED_EDGE('',*,*,#34791,.F.);
#45617=ORIENTED_EDGE('',*,*,#34633,.T.);
#45618=ORIENTED_EDGE('',*,*,#34792,.F.);
#45619=ORIENTED_EDGE('',*,*,#34793,.T.);
#45620=ORIENTED_EDGE('',*,*,#34794,.F.);
#45621=ORIENTED_EDGE('',*,*,#34630,.T.);
#45622=ORIENTED_EDGE('',*,*,#34794,.T.);
#45623=ORIENTED_EDGE('',*,*,#34795,.T.);
#45624=ORIENTED_EDGE('',*,*,#34796,.F.);
#45625=ORIENTED_EDGE('',*,*,#34795,.F.);
#45626=ORIENTED_EDGE('',*,*,#34793,.F.);
#45627=ORIENTED_EDGE('',*,*,#34797,.F.);
#45628=ORIENTED_EDGE('',*,*,#34798,.F.);
#45629=ORIENTED_EDGE('',*,*,#34624,.T.);
#45630=ORIENTED_EDGE('',*,*,#34799,.F.);
#45631=ORIENTED_EDGE('',*,*,#34800,.T.);
#45632=ORIENTED_EDGE('',*,*,#34801,.F.);
#45633=ORIENTED_EDGE('',*,*,#34621,.T.);
#45634=ORIENTED_EDGE('',*,*,#34801,.T.);
#45635=ORIENTED_EDGE('',*,*,#34802,.T.);
#45636=ORIENTED_EDGE('',*,*,#34803,.F.);
#45637=ORIENTED_EDGE('',*,*,#34802,.F.);
#45638=ORIENTED_EDGE('',*,*,#34800,.F.);
#45639=ORIENTED_EDGE('',*,*,#34804,.F.);
#45640=ORIENTED_EDGE('',*,*,#34805,.F.);
#45641=ORIENTED_EDGE('',*,*,#34615,.T.);
#45642=ORIENTED_EDGE('',*,*,#34806,.F.);
#45643=ORIENTED_EDGE('',*,*,#34807,.T.);
#45644=ORIENTED_EDGE('',*,*,#34808,.F.);
#45645=ORIENTED_EDGE('',*,*,#34612,.T.);
#45646=ORIENTED_EDGE('',*,*,#34808,.T.);
#45647=ORIENTED_EDGE('',*,*,#34809,.T.);
#45648=ORIENTED_EDGE('',*,*,#34810,.F.);
#45649=ORIENTED_EDGE('',*,*,#34809,.F.);
#45650=ORIENTED_EDGE('',*,*,#34807,.F.);
#45651=ORIENTED_EDGE('',*,*,#34811,.F.);
#45652=ORIENTED_EDGE('',*,*,#34812,.F.);
#45653=ORIENTED_EDGE('',*,*,#34606,.T.);
#45654=ORIENTED_EDGE('',*,*,#34813,.F.);
#45655=ORIENTED_EDGE('',*,*,#34814,.T.);
#45656=ORIENTED_EDGE('',*,*,#34815,.F.);
#45657=ORIENTED_EDGE('',*,*,#34603,.T.);
#45658=ORIENTED_EDGE('',*,*,#34815,.T.);
#45659=ORIENTED_EDGE('',*,*,#34816,.T.);
#45660=ORIENTED_EDGE('',*,*,#34817,.F.);
#45661=ORIENTED_EDGE('',*,*,#34816,.F.);
#45662=ORIENTED_EDGE('',*,*,#34814,.F.);
#45663=ORIENTED_EDGE('',*,*,#34818,.F.);
#45664=ORIENTED_EDGE('',*,*,#34819,.F.);
#45665=ORIENTED_EDGE('',*,*,#34597,.T.);
#45666=ORIENTED_EDGE('',*,*,#34820,.F.);
#45667=ORIENTED_EDGE('',*,*,#34463,.T.);
#45668=ORIENTED_EDGE('',*,*,#34821,.F.);
#45669=ORIENTED_EDGE('',*,*,#34594,.T.);
#45670=ORIENTED_EDGE('',*,*,#34821,.T.);
#45671=ORIENTED_EDGE('',*,*,#34462,.T.);
#45672=ORIENTED_EDGE('',*,*,#34822,.F.);
#45673=ORIENTED_EDGE('',*,*,#34588,.T.);
#45674=ORIENTED_EDGE('',*,*,#34823,.F.);
#45675=ORIENTED_EDGE('',*,*,#34824,.T.);
#45676=ORIENTED_EDGE('',*,*,#34825,.F.);
#45677=ORIENTED_EDGE('',*,*,#34585,.T.);
#45678=ORIENTED_EDGE('',*,*,#34825,.T.);
#45679=ORIENTED_EDGE('',*,*,#34826,.T.);
#45680=ORIENTED_EDGE('',*,*,#34827,.F.);
#45681=ORIENTED_EDGE('',*,*,#34826,.F.);
#45682=ORIENTED_EDGE('',*,*,#34824,.F.);
#45683=ORIENTED_EDGE('',*,*,#34828,.F.);
#45684=ORIENTED_EDGE('',*,*,#34829,.F.);
#45685=ORIENTED_EDGE('',*,*,#34579,.T.);
#45686=ORIENTED_EDGE('',*,*,#34830,.F.);
#45687=ORIENTED_EDGE('',*,*,#34831,.T.);
#45688=ORIENTED_EDGE('',*,*,#34832,.F.);
#45689=ORIENTED_EDGE('',*,*,#34576,.T.);
#45690=ORIENTED_EDGE('',*,*,#34832,.T.);
#45691=ORIENTED_EDGE('',*,*,#34833,.T.);
#45692=ORIENTED_EDGE('',*,*,#34834,.F.);
#45693=ORIENTED_EDGE('',*,*,#34833,.F.);
#45694=ORIENTED_EDGE('',*,*,#34831,.F.);
#45695=ORIENTED_EDGE('',*,*,#34835,.F.);
#45696=ORIENTED_EDGE('',*,*,#34836,.F.);
#45697=ORIENTED_EDGE('',*,*,#34570,.T.);
#45698=ORIENTED_EDGE('',*,*,#34837,.F.);
#45699=ORIENTED_EDGE('',*,*,#34838,.T.);
#45700=ORIENTED_EDGE('',*,*,#34839,.F.);
#45701=ORIENTED_EDGE('',*,*,#34567,.T.);
#45702=ORIENTED_EDGE('',*,*,#34839,.T.);
#45703=ORIENTED_EDGE('',*,*,#34840,.T.);
#45704=ORIENTED_EDGE('',*,*,#34841,.F.);
#45705=ORIENTED_EDGE('',*,*,#34840,.F.);
#45706=ORIENTED_EDGE('',*,*,#34838,.F.);
#45707=ORIENTED_EDGE('',*,*,#34842,.F.);
#45708=ORIENTED_EDGE('',*,*,#34843,.F.);
#45709=ORIENTED_EDGE('',*,*,#34561,.T.);
#45710=ORIENTED_EDGE('',*,*,#34844,.F.);
#45711=ORIENTED_EDGE('',*,*,#34845,.T.);
#45712=ORIENTED_EDGE('',*,*,#34846,.F.);
#45713=ORIENTED_EDGE('',*,*,#34558,.T.);
#45714=ORIENTED_EDGE('',*,*,#34846,.T.);
#45715=ORIENTED_EDGE('',*,*,#34847,.T.);
#45716=ORIENTED_EDGE('',*,*,#34848,.F.);
#45717=ORIENTED_EDGE('',*,*,#34847,.F.);
#45718=ORIENTED_EDGE('',*,*,#34845,.F.);
#45719=ORIENTED_EDGE('',*,*,#34849,.F.);
#45720=ORIENTED_EDGE('',*,*,#34850,.F.);
#45721=ORIENTED_EDGE('',*,*,#34552,.T.);
#45722=ORIENTED_EDGE('',*,*,#34851,.F.);
#45723=ORIENTED_EDGE('',*,*,#34852,.T.);
#45724=ORIENTED_EDGE('',*,*,#34853,.F.);
#45725=ORIENTED_EDGE('',*,*,#34549,.T.);
#45726=ORIENTED_EDGE('',*,*,#34853,.T.);
#45727=ORIENTED_EDGE('',*,*,#34854,.T.);
#45728=ORIENTED_EDGE('',*,*,#34855,.F.);
#45729=ORIENTED_EDGE('',*,*,#34854,.F.);
#45730=ORIENTED_EDGE('',*,*,#34852,.F.);
#45731=ORIENTED_EDGE('',*,*,#34856,.F.);
#45732=ORIENTED_EDGE('',*,*,#34857,.F.);
#45733=ORIENTED_EDGE('',*,*,#34543,.T.);
#45734=ORIENTED_EDGE('',*,*,#34858,.F.);
#45735=ORIENTED_EDGE('',*,*,#34859,.T.);
#45736=ORIENTED_EDGE('',*,*,#34860,.F.);
#45737=ORIENTED_EDGE('',*,*,#34540,.T.);
#45738=ORIENTED_EDGE('',*,*,#34860,.T.);
#45739=ORIENTED_EDGE('',*,*,#34861,.T.);
#45740=ORIENTED_EDGE('',*,*,#34862,.F.);
#45741=ORIENTED_EDGE('',*,*,#34861,.F.);
#45742=ORIENTED_EDGE('',*,*,#34859,.F.);
#45743=ORIENTED_EDGE('',*,*,#34863,.F.);
#45744=ORIENTED_EDGE('',*,*,#34864,.F.);
#45745=ORIENTED_EDGE('',*,*,#34534,.T.);
#45746=ORIENTED_EDGE('',*,*,#34865,.F.);
#45747=ORIENTED_EDGE('',*,*,#34866,.T.);
#45748=ORIENTED_EDGE('',*,*,#34867,.F.);
#45749=ORIENTED_EDGE('',*,*,#34531,.T.);
#45750=ORIENTED_EDGE('',*,*,#34867,.T.);
#45751=ORIENTED_EDGE('',*,*,#34868,.T.);
#45752=ORIENTED_EDGE('',*,*,#34869,.F.);
#45753=ORIENTED_EDGE('',*,*,#34868,.F.);
#45754=ORIENTED_EDGE('',*,*,#34866,.F.);
#45755=ORIENTED_EDGE('',*,*,#34870,.F.);
#45756=ORIENTED_EDGE('',*,*,#34871,.F.);
#45757=ORIENTED_EDGE('',*,*,#34528,.T.);
#45758=ORIENTED_EDGE('',*,*,#34872,.F.);
#45759=ORIENTED_EDGE('',*,*,#34873,.T.);
#45760=ORIENTED_EDGE('',*,*,#34874,.F.);
#45761=ORIENTED_EDGE('',*,*,#34526,.T.);
#45762=ORIENTED_EDGE('',*,*,#34874,.T.);
#45763=ORIENTED_EDGE('',*,*,#34875,.T.);
#45764=ORIENTED_EDGE('',*,*,#34876,.F.);
#45765=ORIENTED_EDGE('',*,*,#34875,.F.);
#45766=ORIENTED_EDGE('',*,*,#34873,.F.);
#45767=ORIENTED_EDGE('',*,*,#34877,.F.);
#45768=ORIENTED_EDGE('',*,*,#34878,.F.);
#45769=ORIENTED_EDGE('',*,*,#34520,.T.);
#45770=ORIENTED_EDGE('',*,*,#34879,.F.);
#45771=ORIENTED_EDGE('',*,*,#34880,.T.);
#45772=ORIENTED_EDGE('',*,*,#34881,.F.);
#45773=ORIENTED_EDGE('',*,*,#34517,.T.);
#45774=ORIENTED_EDGE('',*,*,#34881,.T.);
#45775=ORIENTED_EDGE('',*,*,#34882,.T.);
#45776=ORIENTED_EDGE('',*,*,#34883,.F.);
#45777=ORIENTED_EDGE('',*,*,#34882,.F.);
#45778=ORIENTED_EDGE('',*,*,#34880,.F.);
#45779=ORIENTED_EDGE('',*,*,#34884,.F.);
#45780=ORIENTED_EDGE('',*,*,#34885,.F.);
#45781=ORIENTED_EDGE('',*,*,#34511,.T.);
#45782=ORIENTED_EDGE('',*,*,#34886,.F.);
#45783=ORIENTED_EDGE('',*,*,#34887,.T.);
#45784=ORIENTED_EDGE('',*,*,#34888,.F.);
#45785=ORIENTED_EDGE('',*,*,#34508,.T.);
#45786=ORIENTED_EDGE('',*,*,#34888,.T.);
#45787=ORIENTED_EDGE('',*,*,#34889,.T.);
#45788=ORIENTED_EDGE('',*,*,#34890,.F.);
#45789=ORIENTED_EDGE('',*,*,#34889,.F.);
#45790=ORIENTED_EDGE('',*,*,#34887,.F.);
#45791=ORIENTED_EDGE('',*,*,#34891,.F.);
#45792=ORIENTED_EDGE('',*,*,#34892,.F.);
#45793=ORIENTED_EDGE('',*,*,#34502,.T.);
#45794=ORIENTED_EDGE('',*,*,#34893,.F.);
#45795=ORIENTED_EDGE('',*,*,#34894,.T.);
#45796=ORIENTED_EDGE('',*,*,#34895,.F.);
#45797=ORIENTED_EDGE('',*,*,#34499,.T.);
#45798=ORIENTED_EDGE('',*,*,#34895,.T.);
#45799=ORIENTED_EDGE('',*,*,#34896,.T.);
#45800=ORIENTED_EDGE('',*,*,#34897,.F.);
#45801=ORIENTED_EDGE('',*,*,#34896,.F.);
#45802=ORIENTED_EDGE('',*,*,#34894,.F.);
#45803=ORIENTED_EDGE('',*,*,#34898,.F.);
#45804=ORIENTED_EDGE('',*,*,#34899,.F.);
#45805=ORIENTED_EDGE('',*,*,#34493,.T.);
#45806=ORIENTED_EDGE('',*,*,#34900,.F.);
#45807=ORIENTED_EDGE('',*,*,#34901,.T.);
#45808=ORIENTED_EDGE('',*,*,#34902,.F.);
#45809=ORIENTED_EDGE('',*,*,#34490,.T.);
#45810=ORIENTED_EDGE('',*,*,#34902,.T.);
#45811=ORIENTED_EDGE('',*,*,#34903,.T.);
#45812=ORIENTED_EDGE('',*,*,#34904,.F.);
#45813=ORIENTED_EDGE('',*,*,#34903,.F.);
#45814=ORIENTED_EDGE('',*,*,#34901,.F.);
#45815=ORIENTED_EDGE('',*,*,#34905,.F.);
#45816=ORIENTED_EDGE('',*,*,#34906,.F.);
#45817=ORIENTED_EDGE('',*,*,#34484,.T.);
#45818=ORIENTED_EDGE('',*,*,#34907,.F.);
#45819=ORIENTED_EDGE('',*,*,#34908,.T.);
#45820=ORIENTED_EDGE('',*,*,#34909,.F.);
#45821=ORIENTED_EDGE('',*,*,#34481,.T.);
#45822=ORIENTED_EDGE('',*,*,#34909,.T.);
#45823=ORIENTED_EDGE('',*,*,#34910,.T.);
#45824=ORIENTED_EDGE('',*,*,#34911,.F.);
#45825=ORIENTED_EDGE('',*,*,#34910,.F.);
#45826=ORIENTED_EDGE('',*,*,#34908,.F.);
#45827=ORIENTED_EDGE('',*,*,#34912,.F.);
#45828=ORIENTED_EDGE('',*,*,#34913,.F.);
#45829=ORIENTED_EDGE('',*,*,#34475,.T.);
#45830=ORIENTED_EDGE('',*,*,#34914,.F.);
#45831=ORIENTED_EDGE('',*,*,#34915,.T.);
#45832=ORIENTED_EDGE('',*,*,#34916,.F.);
#45833=ORIENTED_EDGE('',*,*,#34471,.T.);
#45834=ORIENTED_EDGE('',*,*,#34916,.T.);
#45835=ORIENTED_EDGE('',*,*,#34917,.T.);
#45836=ORIENTED_EDGE('',*,*,#34918,.F.);
#45837=ORIENTED_EDGE('',*,*,#34917,.F.);
#45838=ORIENTED_EDGE('',*,*,#34915,.F.);
#45839=ORIENTED_EDGE('',*,*,#34919,.F.);
#45840=ORIENTED_EDGE('',*,*,#34920,.F.);
#45841=ORIENTED_EDGE('',*,*,#34727,.F.);
#45842=ORIENTED_EDGE('',*,*,#34921,.F.);
#45843=ORIENTED_EDGE('',*,*,#34922,.F.);
#45844=ORIENTED_EDGE('',*,*,#34923,.F.);
#45845=ORIENTED_EDGE('',*,*,#34724,.T.);
#45846=ORIENTED_EDGE('',*,*,#34924,.F.);
#45847=ORIENTED_EDGE('',*,*,#34921,.T.);
#45848=ORIENTED_EDGE('',*,*,#34726,.T.);
#45849=ORIENTED_EDGE('',*,*,#34925,.F.);
#45850=ORIENTED_EDGE('',*,*,#34470,.T.);
#45851=ORIENTED_EDGE('',*,*,#34722,.T.);
#45852=ORIENTED_EDGE('',*,*,#34926,.F.);
#45853=ORIENTED_EDGE('',*,*,#34927,.F.);
#45854=ORIENTED_EDGE('',*,*,#34928,.F.);
#45855=ORIENTED_EDGE('',*,*,#34477,.T.);
#45856=ORIENTED_EDGE('',*,*,#34476,.T.);
#45857=ORIENTED_EDGE('',*,*,#34929,.F.);
#45858=ORIENTED_EDGE('',*,*,#34480,.T.);
#45859=ORIENTED_EDGE('',*,*,#34478,.T.);
#45860=ORIENTED_EDGE('',*,*,#34928,.T.);
#45861=ORIENTED_EDGE('',*,*,#34930,.F.);
#45862=ORIENTED_EDGE('',*,*,#34931,.F.);
#45863=ORIENTED_EDGE('',*,*,#34486,.T.);
#45864=ORIENTED_EDGE('',*,*,#34485,.T.);
#45865=ORIENTED_EDGE('',*,*,#34932,.F.);
#45866=ORIENTED_EDGE('',*,*,#34489,.T.);
#45867=ORIENTED_EDGE('',*,*,#34487,.T.);
#45868=ORIENTED_EDGE('',*,*,#34931,.T.);
#45869=ORIENTED_EDGE('',*,*,#34933,.F.);
#45870=ORIENTED_EDGE('',*,*,#34934,.F.);
#45871=ORIENTED_EDGE('',*,*,#34495,.T.);
#45872=ORIENTED_EDGE('',*,*,#34494,.T.);
#45873=ORIENTED_EDGE('',*,*,#34935,.F.);
#45874=ORIENTED_EDGE('',*,*,#34498,.T.);
#45875=ORIENTED_EDGE('',*,*,#34496,.T.);
#45876=ORIENTED_EDGE('',*,*,#34934,.T.);
#45877=ORIENTED_EDGE('',*,*,#34936,.F.);
#45878=ORIENTED_EDGE('',*,*,#34937,.F.);
#45879=ORIENTED_EDGE('',*,*,#34504,.T.);
#45880=ORIENTED_EDGE('',*,*,#34503,.T.);
#45881=ORIENTED_EDGE('',*,*,#34938,.F.);
#45882=ORIENTED_EDGE('',*,*,#34507,.T.);
#45883=ORIENTED_EDGE('',*,*,#34505,.T.);
#45884=ORIENTED_EDGE('',*,*,#34937,.T.);
#45885=ORIENTED_EDGE('',*,*,#34939,.F.);
#45886=ORIENTED_EDGE('',*,*,#34940,.F.);
#45887=ORIENTED_EDGE('',*,*,#34513,.T.);
#45888=ORIENTED_EDGE('',*,*,#34512,.T.);
#45889=ORIENTED_EDGE('',*,*,#34941,.F.);
#45890=ORIENTED_EDGE('',*,*,#34516,.T.);
#45891=ORIENTED_EDGE('',*,*,#34514,.T.);
#45892=ORIENTED_EDGE('',*,*,#34940,.T.);
#45893=ORIENTED_EDGE('',*,*,#34942,.F.);
#45894=ORIENTED_EDGE('',*,*,#34943,.F.);
#45895=ORIENTED_EDGE('',*,*,#34522,.T.);
#45896=ORIENTED_EDGE('',*,*,#34521,.T.);
#45897=ORIENTED_EDGE('',*,*,#34944,.F.);
#45898=ORIENTED_EDGE('',*,*,#34525,.T.);
#45899=ORIENTED_EDGE('',*,*,#34523,.T.);
#45900=ORIENTED_EDGE('',*,*,#34943,.T.);
#45901=ORIENTED_EDGE('',*,*,#34945,.F.);
#45902=ORIENTED_EDGE('',*,*,#34946,.F.);
#45903=ORIENTED_EDGE('',*,*,#34467,.T.);
#45904=ORIENTED_EDGE('',*,*,#34529,.T.);
#45905=ORIENTED_EDGE('',*,*,#34947,.F.);
#45906=ORIENTED_EDGE('',*,*,#34530,.T.);
#45907=ORIENTED_EDGE('',*,*,#34468,.T.);
#45908=ORIENTED_EDGE('',*,*,#34946,.T.);
#45909=ORIENTED_EDGE('',*,*,#34948,.F.);
#45910=ORIENTED_EDGE('',*,*,#34949,.F.);
#45911=ORIENTED_EDGE('',*,*,#34536,.T.);
#45912=ORIENTED_EDGE('',*,*,#34535,.T.);
#45913=ORIENTED_EDGE('',*,*,#34950,.F.);
#45914=ORIENTED_EDGE('',*,*,#34539,.T.);
#45915=ORIENTED_EDGE('',*,*,#34537,.T.);
#45916=ORIENTED_EDGE('',*,*,#34949,.T.);
#45917=ORIENTED_EDGE('',*,*,#34951,.F.);
#45918=ORIENTED_EDGE('',*,*,#34952,.F.);
#45919=ORIENTED_EDGE('',*,*,#34545,.T.);
#45920=ORIENTED_EDGE('',*,*,#34544,.T.);
#45921=ORIENTED_EDGE('',*,*,#34953,.F.);
#45922=ORIENTED_EDGE('',*,*,#34548,.T.);
#45923=ORIENTED_EDGE('',*,*,#34546,.T.);
#45924=ORIENTED_EDGE('',*,*,#34952,.T.);
#45925=ORIENTED_EDGE('',*,*,#34954,.F.);
#45926=ORIENTED_EDGE('',*,*,#34955,.F.);
#45927=ORIENTED_EDGE('',*,*,#34554,.T.);
#45928=ORIENTED_EDGE('',*,*,#34553,.T.);
#45929=ORIENTED_EDGE('',*,*,#34956,.F.);
#45930=ORIENTED_EDGE('',*,*,#34557,.T.);
#45931=ORIENTED_EDGE('',*,*,#34555,.T.);
#45932=ORIENTED_EDGE('',*,*,#34955,.T.);
#45933=ORIENTED_EDGE('',*,*,#34957,.F.);
#45934=ORIENTED_EDGE('',*,*,#34958,.F.);
#45935=ORIENTED_EDGE('',*,*,#34563,.T.);
#45936=ORIENTED_EDGE('',*,*,#34562,.T.);
#45937=ORIENTED_EDGE('',*,*,#34959,.F.);
#45938=ORIENTED_EDGE('',*,*,#34566,.T.);
#45939=ORIENTED_EDGE('',*,*,#34564,.T.);
#45940=ORIENTED_EDGE('',*,*,#34958,.T.);
#45941=ORIENTED_EDGE('',*,*,#34960,.F.);
#45942=ORIENTED_EDGE('',*,*,#34961,.F.);
#45943=ORIENTED_EDGE('',*,*,#34572,.T.);
#45944=ORIENTED_EDGE('',*,*,#34571,.T.);
#45945=ORIENTED_EDGE('',*,*,#34962,.F.);
#45946=ORIENTED_EDGE('',*,*,#34575,.T.);
#45947=ORIENTED_EDGE('',*,*,#34573,.T.);
#45948=ORIENTED_EDGE('',*,*,#34961,.T.);
#45949=ORIENTED_EDGE('',*,*,#34963,.F.);
#45950=ORIENTED_EDGE('',*,*,#34964,.F.);
#45951=ORIENTED_EDGE('',*,*,#34581,.T.);
#45952=ORIENTED_EDGE('',*,*,#34580,.T.);
#45953=ORIENTED_EDGE('',*,*,#34965,.F.);
#45954=ORIENTED_EDGE('',*,*,#34584,.T.);
#45955=ORIENTED_EDGE('',*,*,#34582,.T.);
#45956=ORIENTED_EDGE('',*,*,#34964,.T.);
#45957=ORIENTED_EDGE('',*,*,#34966,.F.);
#45958=ORIENTED_EDGE('',*,*,#34967,.F.);
#45959=ORIENTED_EDGE('',*,*,#34590,.T.);
#45960=ORIENTED_EDGE('',*,*,#34589,.T.);
#45961=ORIENTED_EDGE('',*,*,#34968,.F.);
#45962=ORIENTED_EDGE('',*,*,#34593,.T.);
#45963=ORIENTED_EDGE('',*,*,#34591,.T.);
#45964=ORIENTED_EDGE('',*,*,#34967,.T.);
#45965=ORIENTED_EDGE('',*,*,#34969,.F.);
#45966=ORIENTED_EDGE('',*,*,#34970,.F.);
#45967=ORIENTED_EDGE('',*,*,#34599,.T.);
#45968=ORIENTED_EDGE('',*,*,#34598,.T.);
#45969=ORIENTED_EDGE('',*,*,#34971,.F.);
#45970=ORIENTED_EDGE('',*,*,#34602,.T.);
#45971=ORIENTED_EDGE('',*,*,#34600,.T.);
#45972=ORIENTED_EDGE('',*,*,#34970,.T.);
#45973=ORIENTED_EDGE('',*,*,#34972,.F.);
#45974=ORIENTED_EDGE('',*,*,#34973,.F.);
#45975=ORIENTED_EDGE('',*,*,#34608,.T.);
#45976=ORIENTED_EDGE('',*,*,#34607,.T.);
#45977=ORIENTED_EDGE('',*,*,#34974,.F.);
#45978=ORIENTED_EDGE('',*,*,#34611,.T.);
#45979=ORIENTED_EDGE('',*,*,#34609,.T.);
#45980=ORIENTED_EDGE('',*,*,#34973,.T.);
#45981=ORIENTED_EDGE('',*,*,#34975,.F.);
#45982=ORIENTED_EDGE('',*,*,#34976,.F.);
#45983=ORIENTED_EDGE('',*,*,#34617,.T.);
#45984=ORIENTED_EDGE('',*,*,#34616,.T.);
#45985=ORIENTED_EDGE('',*,*,#34977,.F.);
#45986=ORIENTED_EDGE('',*,*,#34620,.T.);
#45987=ORIENTED_EDGE('',*,*,#34618,.T.);
#45988=ORIENTED_EDGE('',*,*,#34976,.T.);
#45989=ORIENTED_EDGE('',*,*,#34978,.F.);
#45990=ORIENTED_EDGE('',*,*,#34979,.F.);
#45991=ORIENTED_EDGE('',*,*,#34626,.T.);
#45992=ORIENTED_EDGE('',*,*,#34625,.T.);
#45993=ORIENTED_EDGE('',*,*,#34980,.F.);
#45994=ORIENTED_EDGE('',*,*,#34629,.T.);
#45995=ORIENTED_EDGE('',*,*,#34627,.T.);
#45996=ORIENTED_EDGE('',*,*,#34979,.T.);
#45997=ORIENTED_EDGE('',*,*,#34981,.F.);
#45998=ORIENTED_EDGE('',*,*,#34982,.F.);
#45999=ORIENTED_EDGE('',*,*,#34635,.T.);
#46000=ORIENTED_EDGE('',*,*,#34634,.T.);
#46001=ORIENTED_EDGE('',*,*,#34983,.F.);
#46002=ORIENTED_EDGE('',*,*,#34638,.T.);
#46003=ORIENTED_EDGE('',*,*,#34636,.T.);
#46004=ORIENTED_EDGE('',*,*,#34982,.T.);
#46005=ORIENTED_EDGE('',*,*,#34984,.F.);
#46006=ORIENTED_EDGE('',*,*,#34985,.F.);
#46007=ORIENTED_EDGE('',*,*,#34644,.T.);
#46008=ORIENTED_EDGE('',*,*,#34643,.T.);
#46009=ORIENTED_EDGE('',*,*,#34986,.F.);
#46010=ORIENTED_EDGE('',*,*,#34647,.T.);
#46011=ORIENTED_EDGE('',*,*,#34645,.T.);
#46012=ORIENTED_EDGE('',*,*,#34985,.T.);
#46013=ORIENTED_EDGE('',*,*,#34987,.F.);
#46014=ORIENTED_EDGE('',*,*,#34988,.F.);
#46015=ORIENTED_EDGE('',*,*,#34653,.T.);
#46016=ORIENTED_EDGE('',*,*,#34652,.T.);
#46017=ORIENTED_EDGE('',*,*,#34989,.F.);
#46018=ORIENTED_EDGE('',*,*,#34656,.T.);
#46019=ORIENTED_EDGE('',*,*,#34654,.T.);
#46020=ORIENTED_EDGE('',*,*,#34988,.T.);
#46021=ORIENTED_EDGE('',*,*,#34990,.F.);
#46022=ORIENTED_EDGE('',*,*,#34991,.F.);
#46023=ORIENTED_EDGE('',*,*,#34662,.T.);
#46024=ORIENTED_EDGE('',*,*,#34661,.T.);
#46025=ORIENTED_EDGE('',*,*,#34992,.F.);
#46026=ORIENTED_EDGE('',*,*,#34665,.T.);
#46027=ORIENTED_EDGE('',*,*,#34663,.T.);
#46028=ORIENTED_EDGE('',*,*,#34991,.T.);
#46029=ORIENTED_EDGE('',*,*,#34993,.F.);
#46030=ORIENTED_EDGE('',*,*,#34994,.F.);
#46031=ORIENTED_EDGE('',*,*,#34671,.T.);
#46032=ORIENTED_EDGE('',*,*,#34670,.T.);
#46033=ORIENTED_EDGE('',*,*,#34995,.F.);
#46034=ORIENTED_EDGE('',*,*,#34674,.T.);
#46035=ORIENTED_EDGE('',*,*,#34672,.T.);
#46036=ORIENTED_EDGE('',*,*,#34994,.T.);
#46037=ORIENTED_EDGE('',*,*,#34996,.F.);
#46038=ORIENTED_EDGE('',*,*,#34997,.F.);
#46039=ORIENTED_EDGE('',*,*,#34680,.T.);
#46040=ORIENTED_EDGE('',*,*,#34679,.T.);
#46041=ORIENTED_EDGE('',*,*,#34998,.F.);
#46042=ORIENTED_EDGE('',*,*,#34683,.T.);
#46043=ORIENTED_EDGE('',*,*,#34681,.T.);
#46044=ORIENTED_EDGE('',*,*,#34997,.T.);
#46045=ORIENTED_EDGE('',*,*,#34999,.F.);
#46046=ORIENTED_EDGE('',*,*,#35000,.F.);
#46047=ORIENTED_EDGE('',*,*,#34692,.T.);
#46048=ORIENTED_EDGE('',*,*,#34688,.T.);
#46049=ORIENTED_EDGE('',*,*,#34693,.T.);
#46050=ORIENTED_EDGE('',*,*,#35000,.T.);
#46051=ORIENTED_EDGE('',*,*,#35001,.F.);
#46052=ORIENTED_EDGE('',*,*,#34690,.T.);
#46053=ORIENTED_EDGE('',*,*,#34699,.T.);
#46054=ORIENTED_EDGE('',*,*,#34697,.T.);
#46055=ORIENTED_EDGE('',*,*,#35002,.F.);
#46056=ORIENTED_EDGE('',*,*,#35003,.F.);
#46057=ORIENTED_EDGE('',*,*,#35004,.F.);
#46058=ORIENTED_EDGE('',*,*,#34702,.T.);
#46059=ORIENTED_EDGE('',*,*,#34700,.T.);
#46060=ORIENTED_EDGE('',*,*,#35003,.T.);
#46061=ORIENTED_EDGE('',*,*,#35005,.F.);
#46062=ORIENTED_EDGE('',*,*,#35006,.F.);
#46063=ORIENTED_EDGE('',*,*,#34707,.T.);
#46064=ORIENTED_EDGE('',*,*,#34706,.T.);
#46065=ORIENTED_EDGE('',*,*,#35007,.F.);
#46066=ORIENTED_EDGE('',*,*,#34710,.T.);
#46067=ORIENTED_EDGE('',*,*,#34708,.T.);
#46068=ORIENTED_EDGE('',*,*,#35006,.T.);
#46069=ORIENTED_EDGE('',*,*,#35008,.F.);
#46070=ORIENTED_EDGE('',*,*,#35009,.F.);
#46071=ORIENTED_EDGE('',*,*,#34716,.T.);
#46072=ORIENTED_EDGE('',*,*,#34715,.T.);
#46073=ORIENTED_EDGE('',*,*,#35010,.F.);
#46074=ORIENTED_EDGE('',*,*,#34719,.T.);
#46075=ORIENTED_EDGE('',*,*,#34717,.T.);
#46076=ORIENTED_EDGE('',*,*,#35009,.T.);
#46077=ORIENTED_EDGE('',*,*,#35011,.F.);
#46078=ORIENTED_EDGE('',*,*,#34926,.T.);
#46079=ORIENTED_EDGE('',*,*,#34721,.T.);
#46080=ORIENTED_EDGE('',*,*,#34725,.T.);
#46081=ORIENTED_EDGE('',*,*,#34923,.T.);
#46082=ORIENTED_EDGE('',*,*,#35012,.F.);
#46083=ORIENTED_EDGE('',*,*,#35013,.F.);
#46084=ORIENTED_EDGE('',*,*,#34728,.T.);
#46085=ORIENTED_EDGE('',*,*,#34734,.T.);
#46086=ORIENTED_EDGE('',*,*,#34729,.T.);
#46087=ORIENTED_EDGE('',*,*,#35014,.F.);
#46088=ORIENTED_EDGE('',*,*,#35015,.F.);
#46089=ORIENTED_EDGE('',*,*,#34735,.T.);
#46090=ORIENTED_EDGE('',*,*,#35015,.T.);
#46091=ORIENTED_EDGE('',*,*,#35016,.F.);
#46092=ORIENTED_EDGE('',*,*,#34733,.T.);
#46093=ORIENTED_EDGE('',*,*,#35017,.F.);
#46094=ORIENTED_EDGE('',*,*,#35018,.F.);
#46095=ORIENTED_EDGE('',*,*,#34741,.T.);
#46096=ORIENTED_EDGE('',*,*,#34736,.T.);
#46097=ORIENTED_EDGE('',*,*,#34742,.T.);
#46098=ORIENTED_EDGE('',*,*,#35018,.T.);
#46099=ORIENTED_EDGE('',*,*,#35019,.F.);
#46100=ORIENTED_EDGE('',*,*,#34740,.T.);
#46101=ORIENTED_EDGE('',*,*,#34748,.T.);
#46102=ORIENTED_EDGE('',*,*,#34743,.T.);
#46103=ORIENTED_EDGE('',*,*,#35020,.F.);
#46104=ORIENTED_EDGE('',*,*,#35021,.F.);
#46105=ORIENTED_EDGE('',*,*,#34749,.T.);
#46106=ORIENTED_EDGE('',*,*,#35021,.T.);
#46107=ORIENTED_EDGE('',*,*,#35022,.F.);
#46108=ORIENTED_EDGE('',*,*,#34747,.T.);
#46109=ORIENTED_EDGE('',*,*,#34755,.T.);
#46110=ORIENTED_EDGE('',*,*,#34750,.T.);
#46111=ORIENTED_EDGE('',*,*,#35023,.F.);
#46112=ORIENTED_EDGE('',*,*,#35024,.F.);
#46113=ORIENTED_EDGE('',*,*,#34756,.T.);
#46114=ORIENTED_EDGE('',*,*,#35024,.T.);
#46115=ORIENTED_EDGE('',*,*,#35025,.F.);
#46116=ORIENTED_EDGE('',*,*,#34754,.T.);
#46117=ORIENTED_EDGE('',*,*,#34762,.T.);
#46118=ORIENTED_EDGE('',*,*,#34757,.T.);
#46119=ORIENTED_EDGE('',*,*,#35026,.F.);
#46120=ORIENTED_EDGE('',*,*,#35027,.F.);
#46121=ORIENTED_EDGE('',*,*,#34763,.T.);
#46122=ORIENTED_EDGE('',*,*,#35027,.T.);
#46123=ORIENTED_EDGE('',*,*,#35028,.F.);
#46124=ORIENTED_EDGE('',*,*,#34761,.T.);
#46125=ORIENTED_EDGE('',*,*,#34769,.T.);
#46126=ORIENTED_EDGE('',*,*,#34764,.T.);
#46127=ORIENTED_EDGE('',*,*,#35029,.F.);
#46128=ORIENTED_EDGE('',*,*,#35030,.F.);
#46129=ORIENTED_EDGE('',*,*,#34770,.T.);
#46130=ORIENTED_EDGE('',*,*,#35030,.T.);
#46131=ORIENTED_EDGE('',*,*,#35031,.F.);
#46132=ORIENTED_EDGE('',*,*,#34768,.T.);
#46133=ORIENTED_EDGE('',*,*,#34776,.T.);
#46134=ORIENTED_EDGE('',*,*,#34771,.T.);
#46135=ORIENTED_EDGE('',*,*,#35032,.F.);
#46136=ORIENTED_EDGE('',*,*,#35033,.F.);
#46137=ORIENTED_EDGE('',*,*,#34777,.T.);
#46138=ORIENTED_EDGE('',*,*,#35033,.T.);
#46139=ORIENTED_EDGE('',*,*,#35034,.F.);
#46140=ORIENTED_EDGE('',*,*,#34775,.T.);
#46141=ORIENTED_EDGE('',*,*,#34783,.T.);
#46142=ORIENTED_EDGE('',*,*,#34778,.T.);
#46143=ORIENTED_EDGE('',*,*,#35035,.F.);
#46144=ORIENTED_EDGE('',*,*,#35036,.F.);
#46145=ORIENTED_EDGE('',*,*,#34784,.T.);
#46146=ORIENTED_EDGE('',*,*,#35036,.T.);
#46147=ORIENTED_EDGE('',*,*,#35037,.F.);
#46148=ORIENTED_EDGE('',*,*,#34782,.T.);
#46149=ORIENTED_EDGE('',*,*,#34790,.T.);
#46150=ORIENTED_EDGE('',*,*,#34785,.T.);
#46151=ORIENTED_EDGE('',*,*,#35038,.F.);
#46152=ORIENTED_EDGE('',*,*,#35039,.F.);
#46153=ORIENTED_EDGE('',*,*,#34791,.T.);
#46154=ORIENTED_EDGE('',*,*,#35039,.T.);
#46155=ORIENTED_EDGE('',*,*,#35040,.F.);
#46156=ORIENTED_EDGE('',*,*,#34789,.T.);
#46157=ORIENTED_EDGE('',*,*,#34797,.T.);
#46158=ORIENTED_EDGE('',*,*,#34792,.T.);
#46159=ORIENTED_EDGE('',*,*,#35041,.F.);
#46160=ORIENTED_EDGE('',*,*,#35042,.F.);
#46161=ORIENTED_EDGE('',*,*,#34798,.T.);
#46162=ORIENTED_EDGE('',*,*,#35042,.T.);
#46163=ORIENTED_EDGE('',*,*,#35043,.F.);
#46164=ORIENTED_EDGE('',*,*,#34796,.T.);
#46165=ORIENTED_EDGE('',*,*,#34804,.T.);
#46166=ORIENTED_EDGE('',*,*,#34799,.T.);
#46167=ORIENTED_EDGE('',*,*,#35044,.F.);
#46168=ORIENTED_EDGE('',*,*,#35045,.F.);
#46169=ORIENTED_EDGE('',*,*,#34805,.T.);
#46170=ORIENTED_EDGE('',*,*,#35045,.T.);
#46171=ORIENTED_EDGE('',*,*,#35046,.F.);
#46172=ORIENTED_EDGE('',*,*,#34803,.T.);
#46173=ORIENTED_EDGE('',*,*,#34811,.T.);
#46174=ORIENTED_EDGE('',*,*,#34806,.T.);
#46175=ORIENTED_EDGE('',*,*,#35047,.F.);
#46176=ORIENTED_EDGE('',*,*,#35048,.F.);
#46177=ORIENTED_EDGE('',*,*,#34812,.T.);
#46178=ORIENTED_EDGE('',*,*,#35048,.T.);
#46179=ORIENTED_EDGE('',*,*,#35049,.F.);
#46180=ORIENTED_EDGE('',*,*,#34810,.T.);
#46181=ORIENTED_EDGE('',*,*,#34818,.T.);
#46182=ORIENTED_EDGE('',*,*,#34813,.T.);
#46183=ORIENTED_EDGE('',*,*,#35050,.F.);
#46184=ORIENTED_EDGE('',*,*,#35051,.F.);
#46185=ORIENTED_EDGE('',*,*,#34819,.T.);
#46186=ORIENTED_EDGE('',*,*,#35051,.T.);
#46187=ORIENTED_EDGE('',*,*,#35052,.F.);
#46188=ORIENTED_EDGE('',*,*,#34817,.T.);
#46189=ORIENTED_EDGE('',*,*,#34464,.T.);
#46190=ORIENTED_EDGE('',*,*,#34820,.T.);
#46191=ORIENTED_EDGE('',*,*,#35053,.F.);
#46192=ORIENTED_EDGE('',*,*,#35054,.F.);
#46193=ORIENTED_EDGE('',*,*,#34461,.T.);
#46194=ORIENTED_EDGE('',*,*,#35054,.T.);
#46195=ORIENTED_EDGE('',*,*,#35055,.F.);
#46196=ORIENTED_EDGE('',*,*,#34822,.T.);
#46197=ORIENTED_EDGE('',*,*,#34828,.T.);
#46198=ORIENTED_EDGE('',*,*,#34823,.T.);
#46199=ORIENTED_EDGE('',*,*,#35056,.F.);
#46200=ORIENTED_EDGE('',*,*,#35057,.F.);
#46201=ORIENTED_EDGE('',*,*,#34829,.T.);
#46202=ORIENTED_EDGE('',*,*,#35057,.T.);
#46203=ORIENTED_EDGE('',*,*,#35058,.F.);
#46204=ORIENTED_EDGE('',*,*,#34827,.T.);
#46205=ORIENTED_EDGE('',*,*,#34835,.T.);
#46206=ORIENTED_EDGE('',*,*,#34830,.T.);
#46207=ORIENTED_EDGE('',*,*,#35059,.F.);
#46208=ORIENTED_EDGE('',*,*,#35060,.F.);
#46209=ORIENTED_EDGE('',*,*,#34836,.T.);
#46210=ORIENTED_EDGE('',*,*,#35060,.T.);
#46211=ORIENTED_EDGE('',*,*,#35061,.F.);
#46212=ORIENTED_EDGE('',*,*,#34834,.T.);
#46213=ORIENTED_EDGE('',*,*,#34842,.T.);
#46214=ORIENTED_EDGE('',*,*,#34837,.T.);
#46215=ORIENTED_EDGE('',*,*,#35062,.F.);
#46216=ORIENTED_EDGE('',*,*,#35063,.F.);
#46217=ORIENTED_EDGE('',*,*,#34843,.T.);
#46218=ORIENTED_EDGE('',*,*,#35063,.T.);
#46219=ORIENTED_EDGE('',*,*,#35064,.F.);
#46220=ORIENTED_EDGE('',*,*,#34841,.T.);
#46221=ORIENTED_EDGE('',*,*,#34849,.T.);
#46222=ORIENTED_EDGE('',*,*,#34844,.T.);
#46223=ORIENTED_EDGE('',*,*,#35065,.F.);
#46224=ORIENTED_EDGE('',*,*,#35066,.F.);
#46225=ORIENTED_EDGE('',*,*,#34850,.T.);
#46226=ORIENTED_EDGE('',*,*,#35066,.T.);
#46227=ORIENTED_EDGE('',*,*,#35067,.F.);
#46228=ORIENTED_EDGE('',*,*,#34848,.T.);
#46229=ORIENTED_EDGE('',*,*,#34856,.T.);
#46230=ORIENTED_EDGE('',*,*,#34851,.T.);
#46231=ORIENTED_EDGE('',*,*,#35068,.F.);
#46232=ORIENTED_EDGE('',*,*,#35069,.F.);
#46233=ORIENTED_EDGE('',*,*,#34857,.T.);
#46234=ORIENTED_EDGE('',*,*,#35069,.T.);
#46235=ORIENTED_EDGE('',*,*,#35070,.F.);
#46236=ORIENTED_EDGE('',*,*,#34855,.T.);
#46237=ORIENTED_EDGE('',*,*,#34863,.T.);
#46238=ORIENTED_EDGE('',*,*,#34858,.T.);
#46239=ORIENTED_EDGE('',*,*,#35071,.F.);
#46240=ORIENTED_EDGE('',*,*,#35072,.F.);
#46241=ORIENTED_EDGE('',*,*,#34864,.T.);
#46242=ORIENTED_EDGE('',*,*,#35072,.T.);
#46243=ORIENTED_EDGE('',*,*,#35073,.F.);
#46244=ORIENTED_EDGE('',*,*,#34862,.T.);
#46245=ORIENTED_EDGE('',*,*,#34870,.T.);
#46246=ORIENTED_EDGE('',*,*,#34865,.T.);
#46247=ORIENTED_EDGE('',*,*,#35074,.F.);
#46248=ORIENTED_EDGE('',*,*,#35075,.F.);
#46249=ORIENTED_EDGE('',*,*,#34871,.T.);
#46250=ORIENTED_EDGE('',*,*,#35075,.T.);
#46251=ORIENTED_EDGE('',*,*,#35076,.F.);
#46252=ORIENTED_EDGE('',*,*,#34869,.T.);
#46253=ORIENTED_EDGE('',*,*,#34877,.T.);
#46254=ORIENTED_EDGE('',*,*,#34872,.T.);
#46255=ORIENTED_EDGE('',*,*,#35077,.F.);
#46256=ORIENTED_EDGE('',*,*,#35078,.F.);
#46257=ORIENTED_EDGE('',*,*,#34878,.T.);
#46258=ORIENTED_EDGE('',*,*,#35078,.T.);
#46259=ORIENTED_EDGE('',*,*,#35079,.F.);
#46260=ORIENTED_EDGE('',*,*,#34876,.T.);
#46261=ORIENTED_EDGE('',*,*,#34884,.T.);
#46262=ORIENTED_EDGE('',*,*,#34879,.T.);
#46263=ORIENTED_EDGE('',*,*,#35080,.F.);
#46264=ORIENTED_EDGE('',*,*,#35081,.F.);
#46265=ORIENTED_EDGE('',*,*,#34885,.T.);
#46266=ORIENTED_EDGE('',*,*,#35081,.T.);
#46267=ORIENTED_EDGE('',*,*,#35082,.F.);
#46268=ORIENTED_EDGE('',*,*,#34883,.T.);
#46269=ORIENTED_EDGE('',*,*,#34891,.T.);
#46270=ORIENTED_EDGE('',*,*,#34886,.T.);
#46271=ORIENTED_EDGE('',*,*,#35083,.F.);
#46272=ORIENTED_EDGE('',*,*,#35084,.F.);
#46273=ORIENTED_EDGE('',*,*,#34892,.T.);
#46274=ORIENTED_EDGE('',*,*,#35084,.T.);
#46275=ORIENTED_EDGE('',*,*,#35085,.F.);
#46276=ORIENTED_EDGE('',*,*,#34890,.T.);
#46277=ORIENTED_EDGE('',*,*,#34898,.T.);
#46278=ORIENTED_EDGE('',*,*,#34893,.T.);
#46279=ORIENTED_EDGE('',*,*,#35086,.F.);
#46280=ORIENTED_EDGE('',*,*,#35087,.F.);
#46281=ORIENTED_EDGE('',*,*,#34899,.T.);
#46282=ORIENTED_EDGE('',*,*,#35087,.T.);
#46283=ORIENTED_EDGE('',*,*,#35088,.F.);
#46284=ORIENTED_EDGE('',*,*,#34897,.T.);
#46285=ORIENTED_EDGE('',*,*,#34905,.T.);
#46286=ORIENTED_EDGE('',*,*,#34900,.T.);
#46287=ORIENTED_EDGE('',*,*,#35089,.F.);
#46288=ORIENTED_EDGE('',*,*,#35090,.F.);
#46289=ORIENTED_EDGE('',*,*,#34906,.T.);
#46290=ORIENTED_EDGE('',*,*,#35090,.T.);
#46291=ORIENTED_EDGE('',*,*,#35091,.F.);
#46292=ORIENTED_EDGE('',*,*,#34904,.T.);
#46293=ORIENTED_EDGE('',*,*,#34912,.T.);
#46294=ORIENTED_EDGE('',*,*,#34907,.T.);
#46295=ORIENTED_EDGE('',*,*,#35092,.F.);
#46296=ORIENTED_EDGE('',*,*,#35093,.F.);
#46297=ORIENTED_EDGE('',*,*,#34913,.T.);
#46298=ORIENTED_EDGE('',*,*,#35093,.T.);
#46299=ORIENTED_EDGE('',*,*,#35094,.F.);
#46300=ORIENTED_EDGE('',*,*,#34911,.T.);
#46301=ORIENTED_EDGE('',*,*,#34919,.T.);
#46302=ORIENTED_EDGE('',*,*,#34914,.T.);
#46303=ORIENTED_EDGE('',*,*,#35095,.F.);
#46304=ORIENTED_EDGE('',*,*,#35096,.F.);
#46305=ORIENTED_EDGE('',*,*,#34920,.T.);
#46306=ORIENTED_EDGE('',*,*,#35096,.T.);
#46307=ORIENTED_EDGE('',*,*,#35097,.F.);
#46308=ORIENTED_EDGE('',*,*,#34918,.T.);
#46309=ORIENTED_EDGE('',*,*,#34922,.T.);
#46310=ORIENTED_EDGE('',*,*,#34924,.T.);
#46311=ORIENTED_EDGE('',*,*,#35098,.F.);
#46312=ORIENTED_EDGE('',*,*,#35012,.T.);
#46313=ORIENTED_EDGE('',*,*,#35099,.T.);
#46314=ORIENTED_EDGE('',*,*,#35100,.F.);
#46315=ORIENTED_EDGE('',*,*,#34925,.T.);
#46316=ORIENTED_EDGE('',*,*,#35101,.F.);
#46317=ORIENTED_EDGE('',*,*,#35102,.F.);
#46318=ORIENTED_EDGE('',*,*,#35103,.F.);
#46319=ORIENTED_EDGE('',*,*,#35104,.F.);
#46320=ORIENTED_EDGE('',*,*,#35099,.F.);
#46321=ORIENTED_EDGE('',*,*,#35104,.T.);
#46322=ORIENTED_EDGE('',*,*,#35105,.F.);
#46323=ORIENTED_EDGE('',*,*,#34927,.T.);
#46324=ORIENTED_EDGE('',*,*,#35100,.T.);
#46325=ORIENTED_EDGE('',*,*,#35106,.T.);
#46326=ORIENTED_EDGE('',*,*,#35107,.F.);
#46327=ORIENTED_EDGE('',*,*,#34929,.T.);
#46328=ORIENTED_EDGE('',*,*,#35108,.F.);
#46329=ORIENTED_EDGE('',*,*,#35109,.F.);
#46330=ORIENTED_EDGE('',*,*,#35110,.F.);
#46331=ORIENTED_EDGE('',*,*,#35111,.F.);
#46332=ORIENTED_EDGE('',*,*,#35106,.F.);
#46333=ORIENTED_EDGE('',*,*,#35111,.T.);
#46334=ORIENTED_EDGE('',*,*,#35112,.F.);
#46335=ORIENTED_EDGE('',*,*,#34930,.T.);
#46336=ORIENTED_EDGE('',*,*,#35107,.T.);
#46337=ORIENTED_EDGE('',*,*,#35113,.T.);
#46338=ORIENTED_EDGE('',*,*,#35114,.F.);
#46339=ORIENTED_EDGE('',*,*,#34932,.T.);
#46340=ORIENTED_EDGE('',*,*,#35115,.F.);
#46341=ORIENTED_EDGE('',*,*,#35116,.F.);
#46342=ORIENTED_EDGE('',*,*,#35117,.F.);
#46343=ORIENTED_EDGE('',*,*,#35118,.F.);
#46344=ORIENTED_EDGE('',*,*,#35113,.F.);
#46345=ORIENTED_EDGE('',*,*,#35118,.T.);
#46346=ORIENTED_EDGE('',*,*,#35119,.F.);
#46347=ORIENTED_EDGE('',*,*,#34933,.T.);
#46348=ORIENTED_EDGE('',*,*,#35114,.T.);
#46349=ORIENTED_EDGE('',*,*,#35120,.T.);
#46350=ORIENTED_EDGE('',*,*,#35121,.F.);
#46351=ORIENTED_EDGE('',*,*,#34935,.T.);
#46352=ORIENTED_EDGE('',*,*,#35122,.F.);
#46353=ORIENTED_EDGE('',*,*,#35123,.F.);
#46354=ORIENTED_EDGE('',*,*,#35124,.F.);
#46355=ORIENTED_EDGE('',*,*,#35125,.F.);
#46356=ORIENTED_EDGE('',*,*,#35120,.F.);
#46357=ORIENTED_EDGE('',*,*,#35125,.T.);
#46358=ORIENTED_EDGE('',*,*,#35126,.F.);
#46359=ORIENTED_EDGE('',*,*,#34936,.T.);
#46360=ORIENTED_EDGE('',*,*,#35121,.T.);
#46361=ORIENTED_EDGE('',*,*,#35127,.T.);
#46362=ORIENTED_EDGE('',*,*,#35128,.F.);
#46363=ORIENTED_EDGE('',*,*,#34938,.T.);
#46364=ORIENTED_EDGE('',*,*,#35129,.F.);
#46365=ORIENTED_EDGE('',*,*,#35130,.F.);
#46366=ORIENTED_EDGE('',*,*,#35131,.F.);
#46367=ORIENTED_EDGE('',*,*,#35132,.F.);
#46368=ORIENTED_EDGE('',*,*,#35127,.F.);
#46369=ORIENTED_EDGE('',*,*,#35132,.T.);
#46370=ORIENTED_EDGE('',*,*,#35133,.F.);
#46371=ORIENTED_EDGE('',*,*,#34939,.T.);
#46372=ORIENTED_EDGE('',*,*,#35128,.T.);
#46373=ORIENTED_EDGE('',*,*,#35134,.T.);
#46374=ORIENTED_EDGE('',*,*,#35135,.F.);
#46375=ORIENTED_EDGE('',*,*,#34941,.T.);
#46376=ORIENTED_EDGE('',*,*,#35136,.F.);
#46377=ORIENTED_EDGE('',*,*,#35137,.F.);
#46378=ORIENTED_EDGE('',*,*,#35138,.F.);
#46379=ORIENTED_EDGE('',*,*,#35139,.F.);
#46380=ORIENTED_EDGE('',*,*,#35134,.F.);
#46381=ORIENTED_EDGE('',*,*,#35139,.T.);
#46382=ORIENTED_EDGE('',*,*,#35140,.F.);
#46383=ORIENTED_EDGE('',*,*,#34942,.T.);
#46384=ORIENTED_EDGE('',*,*,#35135,.T.);
#46385=ORIENTED_EDGE('',*,*,#35141,.T.);
#46386=ORIENTED_EDGE('',*,*,#35142,.F.);
#46387=ORIENTED_EDGE('',*,*,#34944,.T.);
#46388=ORIENTED_EDGE('',*,*,#35143,.F.);
#46389=ORIENTED_EDGE('',*,*,#35144,.F.);
#46390=ORIENTED_EDGE('',*,*,#35145,.F.);
#46391=ORIENTED_EDGE('',*,*,#35146,.F.);
#46392=ORIENTED_EDGE('',*,*,#35141,.F.);
#46393=ORIENTED_EDGE('',*,*,#35146,.T.);
#46394=ORIENTED_EDGE('',*,*,#35147,.F.);
#46395=ORIENTED_EDGE('',*,*,#34945,.T.);
#46396=ORIENTED_EDGE('',*,*,#35142,.T.);
#46397=ORIENTED_EDGE('',*,*,#35148,.T.);
#46398=ORIENTED_EDGE('',*,*,#35149,.F.);
#46399=ORIENTED_EDGE('',*,*,#34947,.T.);
#46400=ORIENTED_EDGE('',*,*,#35150,.F.);
#46401=ORIENTED_EDGE('',*,*,#35151,.F.);
#46402=ORIENTED_EDGE('',*,*,#35152,.F.);
#46403=ORIENTED_EDGE('',*,*,#35153,.F.);
#46404=ORIENTED_EDGE('',*,*,#35148,.F.);
#46405=ORIENTED_EDGE('',*,*,#35153,.T.);
#46406=ORIENTED_EDGE('',*,*,#35154,.F.);
#46407=ORIENTED_EDGE('',*,*,#34948,.T.);
#46408=ORIENTED_EDGE('',*,*,#35149,.T.);
#46409=ORIENTED_EDGE('',*,*,#35155,.T.);
#46410=ORIENTED_EDGE('',*,*,#35156,.F.);
#46411=ORIENTED_EDGE('',*,*,#34950,.T.);
#46412=ORIENTED_EDGE('',*,*,#35157,.F.);
#46413=ORIENTED_EDGE('',*,*,#35158,.F.);
#46414=ORIENTED_EDGE('',*,*,#35159,.F.);
#46415=ORIENTED_EDGE('',*,*,#35160,.F.);
#46416=ORIENTED_EDGE('',*,*,#35155,.F.);
#46417=ORIENTED_EDGE('',*,*,#35160,.T.);
#46418=ORIENTED_EDGE('',*,*,#35161,.F.);
#46419=ORIENTED_EDGE('',*,*,#34951,.T.);
#46420=ORIENTED_EDGE('',*,*,#35156,.T.);
#46421=ORIENTED_EDGE('',*,*,#35162,.T.);
#46422=ORIENTED_EDGE('',*,*,#35163,.F.);
#46423=ORIENTED_EDGE('',*,*,#34953,.T.);
#46424=ORIENTED_EDGE('',*,*,#35164,.F.);
#46425=ORIENTED_EDGE('',*,*,#35165,.F.);
#46426=ORIENTED_EDGE('',*,*,#35166,.F.);
#46427=ORIENTED_EDGE('',*,*,#35167,.F.);
#46428=ORIENTED_EDGE('',*,*,#35162,.F.);
#46429=ORIENTED_EDGE('',*,*,#35167,.T.);
#46430=ORIENTED_EDGE('',*,*,#35168,.F.);
#46431=ORIENTED_EDGE('',*,*,#34954,.T.);
#46432=ORIENTED_EDGE('',*,*,#35163,.T.);
#46433=ORIENTED_EDGE('',*,*,#35169,.T.);
#46434=ORIENTED_EDGE('',*,*,#35170,.F.);
#46435=ORIENTED_EDGE('',*,*,#34956,.T.);
#46436=ORIENTED_EDGE('',*,*,#35171,.F.);
#46437=ORIENTED_EDGE('',*,*,#35172,.F.);
#46438=ORIENTED_EDGE('',*,*,#35173,.F.);
#46439=ORIENTED_EDGE('',*,*,#35174,.F.);
#46440=ORIENTED_EDGE('',*,*,#35169,.F.);
#46441=ORIENTED_EDGE('',*,*,#35174,.T.);
#46442=ORIENTED_EDGE('',*,*,#35175,.F.);
#46443=ORIENTED_EDGE('',*,*,#34957,.T.);
#46444=ORIENTED_EDGE('',*,*,#35170,.T.);
#46445=ORIENTED_EDGE('',*,*,#35176,.T.);
#46446=ORIENTED_EDGE('',*,*,#35177,.F.);
#46447=ORIENTED_EDGE('',*,*,#34959,.T.);
#46448=ORIENTED_EDGE('',*,*,#35178,.F.);
#46449=ORIENTED_EDGE('',*,*,#35179,.F.);
#46450=ORIENTED_EDGE('',*,*,#35180,.F.);
#46451=ORIENTED_EDGE('',*,*,#35181,.F.);
#46452=ORIENTED_EDGE('',*,*,#35176,.F.);
#46453=ORIENTED_EDGE('',*,*,#35181,.T.);
#46454=ORIENTED_EDGE('',*,*,#35182,.F.);
#46455=ORIENTED_EDGE('',*,*,#34960,.T.);
#46456=ORIENTED_EDGE('',*,*,#35177,.T.);
#46457=ORIENTED_EDGE('',*,*,#35183,.T.);
#46458=ORIENTED_EDGE('',*,*,#35184,.F.);
#46459=ORIENTED_EDGE('',*,*,#34962,.T.);
#46460=ORIENTED_EDGE('',*,*,#35185,.F.);
#46461=ORIENTED_EDGE('',*,*,#35186,.F.);
#46462=ORIENTED_EDGE('',*,*,#35187,.F.);
#46463=ORIENTED_EDGE('',*,*,#35188,.F.);
#46464=ORIENTED_EDGE('',*,*,#35183,.F.);
#46465=ORIENTED_EDGE('',*,*,#35188,.T.);
#46466=ORIENTED_EDGE('',*,*,#35189,.F.);
#46467=ORIENTED_EDGE('',*,*,#34963,.T.);
#46468=ORIENTED_EDGE('',*,*,#35184,.T.);
#46469=ORIENTED_EDGE('',*,*,#35190,.T.);
#46470=ORIENTED_EDGE('',*,*,#35191,.F.);
#46471=ORIENTED_EDGE('',*,*,#34965,.T.);
#46472=ORIENTED_EDGE('',*,*,#35192,.F.);
#46473=ORIENTED_EDGE('',*,*,#35193,.F.);
#46474=ORIENTED_EDGE('',*,*,#35194,.F.);
#46475=ORIENTED_EDGE('',*,*,#35195,.F.);
#46476=ORIENTED_EDGE('',*,*,#35190,.F.);
#46477=ORIENTED_EDGE('',*,*,#35195,.T.);
#46478=ORIENTED_EDGE('',*,*,#35196,.F.);
#46479=ORIENTED_EDGE('',*,*,#34966,.T.);
#46480=ORIENTED_EDGE('',*,*,#35191,.T.);
#46481=ORIENTED_EDGE('',*,*,#34457,.T.);
#46482=ORIENTED_EDGE('',*,*,#35197,.F.);
#46483=ORIENTED_EDGE('',*,*,#34968,.T.);
#46484=ORIENTED_EDGE('',*,*,#35198,.F.);
#46485=ORIENTED_EDGE('',*,*,#34460,.T.);
#46486=ORIENTED_EDGE('',*,*,#35199,.F.);
#46487=ORIENTED_EDGE('',*,*,#34969,.T.);
#46488=ORIENTED_EDGE('',*,*,#35197,.T.);
#46489=ORIENTED_EDGE('',*,*,#35200,.T.);
#46490=ORIENTED_EDGE('',*,*,#35201,.F.);
#46491=ORIENTED_EDGE('',*,*,#34971,.T.);
#46492=ORIENTED_EDGE('',*,*,#35202,.F.);
#46493=ORIENTED_EDGE('',*,*,#35203,.F.);
#46494=ORIENTED_EDGE('',*,*,#35204,.F.);
#46495=ORIENTED_EDGE('',*,*,#35205,.F.);
#46496=ORIENTED_EDGE('',*,*,#35200,.F.);
#46497=ORIENTED_EDGE('',*,*,#35205,.T.);
#46498=ORIENTED_EDGE('',*,*,#35206,.F.);
#46499=ORIENTED_EDGE('',*,*,#34972,.T.);
#46500=ORIENTED_EDGE('',*,*,#35201,.T.);
#46501=ORIENTED_EDGE('',*,*,#35207,.T.);
#46502=ORIENTED_EDGE('',*,*,#35208,.F.);
#46503=ORIENTED_EDGE('',*,*,#34974,.T.);
#46504=ORIENTED_EDGE('',*,*,#35209,.F.);
#46505=ORIENTED_EDGE('',*,*,#35210,.F.);
#46506=ORIENTED_EDGE('',*,*,#35211,.F.);
#46507=ORIENTED_EDGE('',*,*,#35212,.F.);
#46508=ORIENTED_EDGE('',*,*,#35207,.F.);
#46509=ORIENTED_EDGE('',*,*,#35212,.T.);
#46510=ORIENTED_EDGE('',*,*,#35213,.F.);
#46511=ORIENTED_EDGE('',*,*,#34975,.T.);
#46512=ORIENTED_EDGE('',*,*,#35208,.T.);
#46513=ORIENTED_EDGE('',*,*,#35214,.T.);
#46514=ORIENTED_EDGE('',*,*,#35215,.F.);
#46515=ORIENTED_EDGE('',*,*,#34977,.T.);
#46516=ORIENTED_EDGE('',*,*,#35216,.F.);
#46517=ORIENTED_EDGE('',*,*,#35217,.F.);
#46518=ORIENTED_EDGE('',*,*,#35218,.F.);
#46519=ORIENTED_EDGE('',*,*,#35219,.F.);
#46520=ORIENTED_EDGE('',*,*,#35214,.F.);
#46521=ORIENTED_EDGE('',*,*,#35219,.T.);
#46522=ORIENTED_EDGE('',*,*,#35220,.F.);
#46523=ORIENTED_EDGE('',*,*,#34978,.T.);
#46524=ORIENTED_EDGE('',*,*,#35215,.T.);
#46525=ORIENTED_EDGE('',*,*,#35221,.T.);
#46526=ORIENTED_EDGE('',*,*,#35222,.F.);
#46527=ORIENTED_EDGE('',*,*,#34980,.T.);
#46528=ORIENTED_EDGE('',*,*,#35223,.F.);
#46529=ORIENTED_EDGE('',*,*,#35224,.F.);
#46530=ORIENTED_EDGE('',*,*,#35225,.F.);
#46531=ORIENTED_EDGE('',*,*,#35226,.F.);
#46532=ORIENTED_EDGE('',*,*,#35221,.F.);
#46533=ORIENTED_EDGE('',*,*,#35226,.T.);
#46534=ORIENTED_EDGE('',*,*,#35227,.F.);
#46535=ORIENTED_EDGE('',*,*,#34981,.T.);
#46536=ORIENTED_EDGE('',*,*,#35222,.T.);
#46537=ORIENTED_EDGE('',*,*,#35228,.T.);
#46538=ORIENTED_EDGE('',*,*,#35229,.F.);
#46539=ORIENTED_EDGE('',*,*,#34983,.T.);
#46540=ORIENTED_EDGE('',*,*,#35230,.F.);
#46541=ORIENTED_EDGE('',*,*,#35231,.F.);
#46542=ORIENTED_EDGE('',*,*,#35232,.F.);
#46543=ORIENTED_EDGE('',*,*,#35233,.F.);
#46544=ORIENTED_EDGE('',*,*,#35228,.F.);
#46545=ORIENTED_EDGE('',*,*,#35233,.T.);
#46546=ORIENTED_EDGE('',*,*,#35234,.F.);
#46547=ORIENTED_EDGE('',*,*,#34984,.T.);
#46548=ORIENTED_EDGE('',*,*,#35229,.T.);
#46549=ORIENTED_EDGE('',*,*,#35235,.T.);
#46550=ORIENTED_EDGE('',*,*,#35236,.F.);
#46551=ORIENTED_EDGE('',*,*,#34986,.T.);
#46552=ORIENTED_EDGE('',*,*,#35237,.F.);
#46553=ORIENTED_EDGE('',*,*,#35238,.F.);
#46554=ORIENTED_EDGE('',*,*,#35239,.F.);
#46555=ORIENTED_EDGE('',*,*,#35240,.F.);
#46556=ORIENTED_EDGE('',*,*,#35235,.F.);
#46557=ORIENTED_EDGE('',*,*,#35240,.T.);
#46558=ORIENTED_EDGE('',*,*,#35241,.F.);
#46559=ORIENTED_EDGE('',*,*,#34987,.T.);
#46560=ORIENTED_EDGE('',*,*,#35236,.T.);
#46561=ORIENTED_EDGE('',*,*,#35242,.T.);
#46562=ORIENTED_EDGE('',*,*,#35243,.F.);
#46563=ORIENTED_EDGE('',*,*,#34989,.T.);
#46564=ORIENTED_EDGE('',*,*,#35244,.F.);
#46565=ORIENTED_EDGE('',*,*,#35245,.F.);
#46566=ORIENTED_EDGE('',*,*,#35246,.F.);
#46567=ORIENTED_EDGE('',*,*,#35247,.F.);
#46568=ORIENTED_EDGE('',*,*,#35242,.F.);
#46569=ORIENTED_EDGE('',*,*,#35247,.T.);
#46570=ORIENTED_EDGE('',*,*,#35248,.F.);
#46571=ORIENTED_EDGE('',*,*,#34990,.T.);
#46572=ORIENTED_EDGE('',*,*,#35243,.T.);
#46573=ORIENTED_EDGE('',*,*,#35249,.T.);
#46574=ORIENTED_EDGE('',*,*,#35250,.F.);
#46575=ORIENTED_EDGE('',*,*,#34992,.T.);
#46576=ORIENTED_EDGE('',*,*,#35251,.F.);
#46577=ORIENTED_EDGE('',*,*,#35252,.F.);
#46578=ORIENTED_EDGE('',*,*,#35253,.F.);
#46579=ORIENTED_EDGE('',*,*,#35254,.F.);
#46580=ORIENTED_EDGE('',*,*,#35249,.F.);
#46581=ORIENTED_EDGE('',*,*,#35254,.T.);
#46582=ORIENTED_EDGE('',*,*,#35255,.F.);
#46583=ORIENTED_EDGE('',*,*,#34993,.T.);
#46584=ORIENTED_EDGE('',*,*,#35250,.T.);
#46585=ORIENTED_EDGE('',*,*,#35256,.T.);
#46586=ORIENTED_EDGE('',*,*,#35257,.F.);
#46587=ORIENTED_EDGE('',*,*,#34995,.T.);
#46588=ORIENTED_EDGE('',*,*,#35258,.F.);
#46589=ORIENTED_EDGE('',*,*,#35259,.F.);
#46590=ORIENTED_EDGE('',*,*,#35260,.F.);
#46591=ORIENTED_EDGE('',*,*,#35261,.F.);
#46592=ORIENTED_EDGE('',*,*,#35256,.F.);
#46593=ORIENTED_EDGE('',*,*,#35261,.T.);
#46594=ORIENTED_EDGE('',*,*,#35262,.F.);
#46595=ORIENTED_EDGE('',*,*,#34996,.T.);
#46596=ORIENTED_EDGE('',*,*,#35257,.T.);
#46597=ORIENTED_EDGE('',*,*,#35263,.T.);
#46598=ORIENTED_EDGE('',*,*,#35264,.F.);
#46599=ORIENTED_EDGE('',*,*,#34998,.T.);
#46600=ORIENTED_EDGE('',*,*,#35265,.F.);
#46601=ORIENTED_EDGE('',*,*,#35266,.T.);
#46602=ORIENTED_EDGE('',*,*,#35267,.F.);
#46603=ORIENTED_EDGE('',*,*,#34999,.T.);
#46604=ORIENTED_EDGE('',*,*,#35264,.T.);
#46605=ORIENTED_EDGE('',*,*,#35268,.F.);
#46606=ORIENTED_EDGE('',*,*,#35269,.F.);
#46607=ORIENTED_EDGE('',*,*,#35266,.F.);
#46608=ORIENTED_EDGE('',*,*,#35263,.F.);
#46609=ORIENTED_EDGE('',*,*,#35001,.T.);
#46610=ORIENTED_EDGE('',*,*,#35270,.F.);
#46611=ORIENTED_EDGE('',*,*,#35271,.T.);
#46612=ORIENTED_EDGE('',*,*,#35272,.F.);
#46613=ORIENTED_EDGE('',*,*,#35273,.F.);
#46614=ORIENTED_EDGE('',*,*,#35271,.F.);
#46615=ORIENTED_EDGE('',*,*,#35274,.F.);
#46616=ORIENTED_EDGE('',*,*,#35275,.F.);
#46617=ORIENTED_EDGE('',*,*,#35002,.T.);
#46618=ORIENTED_EDGE('',*,*,#35272,.T.);
#46619=ORIENTED_EDGE('',*,*,#35273,.T.);
#46620=ORIENTED_EDGE('',*,*,#35276,.F.);
#46621=ORIENTED_EDGE('',*,*,#35277,.T.);
#46622=ORIENTED_EDGE('',*,*,#35278,.F.);
#46623=ORIENTED_EDGE('',*,*,#35004,.T.);
#46624=ORIENTED_EDGE('',*,*,#35279,.F.);
#46625=ORIENTED_EDGE('',*,*,#35280,.F.);
#46626=ORIENTED_EDGE('',*,*,#35281,.F.);
#46627=ORIENTED_EDGE('',*,*,#35282,.F.);
#46628=ORIENTED_EDGE('',*,*,#35277,.F.);
#46629=ORIENTED_EDGE('',*,*,#35282,.T.);
#46630=ORIENTED_EDGE('',*,*,#35283,.F.);
#46631=ORIENTED_EDGE('',*,*,#35005,.T.);
#46632=ORIENTED_EDGE('',*,*,#35278,.T.);
#46633=ORIENTED_EDGE('',*,*,#35284,.T.);
#46634=ORIENTED_EDGE('',*,*,#35285,.F.);
#46635=ORIENTED_EDGE('',*,*,#35007,.T.);
#46636=ORIENTED_EDGE('',*,*,#35286,.F.);
#46637=ORIENTED_EDGE('',*,*,#35287,.F.);
#46638=ORIENTED_EDGE('',*,*,#35288,.F.);
#46639=ORIENTED_EDGE('',*,*,#35289,.F.);
#46640=ORIENTED_EDGE('',*,*,#35284,.F.);
#46641=ORIENTED_EDGE('',*,*,#35289,.T.);
#46642=ORIENTED_EDGE('',*,*,#35290,.F.);
#46643=ORIENTED_EDGE('',*,*,#35008,.T.);
#46644=ORIENTED_EDGE('',*,*,#35285,.T.);
#46645=ORIENTED_EDGE('',*,*,#35291,.T.);
#46646=ORIENTED_EDGE('',*,*,#35292,.F.);
#46647=ORIENTED_EDGE('',*,*,#35010,.T.);
#46648=ORIENTED_EDGE('',*,*,#35293,.F.);
#46649=ORIENTED_EDGE('',*,*,#35294,.F.);
#46650=ORIENTED_EDGE('',*,*,#35295,.F.);
#46651=ORIENTED_EDGE('',*,*,#35296,.F.);
#46652=ORIENTED_EDGE('',*,*,#35291,.F.);
#46653=ORIENTED_EDGE('',*,*,#35296,.T.);
#46654=ORIENTED_EDGE('',*,*,#35297,.F.);
#46655=ORIENTED_EDGE('',*,*,#35011,.T.);
#46656=ORIENTED_EDGE('',*,*,#35292,.T.);
#46657=ORIENTED_EDGE('',*,*,#35013,.T.);
#46658=ORIENTED_EDGE('',*,*,#35298,.F.);
#46659=ORIENTED_EDGE('',*,*,#35299,.T.);
#46660=ORIENTED_EDGE('',*,*,#35300,.F.);
#46661=ORIENTED_EDGE('',*,*,#35014,.T.);
#46662=ORIENTED_EDGE('',*,*,#35300,.T.);
#46663=ORIENTED_EDGE('',*,*,#35301,.T.);
#46664=ORIENTED_EDGE('',*,*,#35302,.F.);
#46665=ORIENTED_EDGE('',*,*,#35301,.F.);
#46666=ORIENTED_EDGE('',*,*,#35299,.F.);
#46667=ORIENTED_EDGE('',*,*,#35303,.F.);
#46668=ORIENTED_EDGE('',*,*,#35304,.F.);
#46669=ORIENTED_EDGE('',*,*,#35016,.T.);
#46670=ORIENTED_EDGE('',*,*,#35305,.F.);
#46671=ORIENTED_EDGE('',*,*,#35306,.T.);
#46672=ORIENTED_EDGE('',*,*,#35307,.F.);
#46673=ORIENTED_EDGE('',*,*,#35308,.T.);
#46674=ORIENTED_EDGE('',*,*,#35309,.F.);
#46675=ORIENTED_EDGE('',*,*,#35017,.T.);
#46676=ORIENTED_EDGE('',*,*,#35307,.T.);
#46677=ORIENTED_EDGE('',*,*,#35310,.F.);
#46678=ORIENTED_EDGE('',*,*,#35311,.F.);
#46679=ORIENTED_EDGE('',*,*,#35308,.F.);
#46680=ORIENTED_EDGE('',*,*,#35306,.F.);
#46681=ORIENTED_EDGE('',*,*,#35019,.T.);
#46682=ORIENTED_EDGE('',*,*,#35312,.F.);
#46683=ORIENTED_EDGE('',*,*,#35313,.T.);
#46684=ORIENTED_EDGE('',*,*,#35314,.F.);
#46685=ORIENTED_EDGE('',*,*,#35020,.T.);
#46686=ORIENTED_EDGE('',*,*,#35314,.T.);
#46687=ORIENTED_EDGE('',*,*,#35315,.T.);
#46688=ORIENTED_EDGE('',*,*,#35316,.F.);
#46689=ORIENTED_EDGE('',*,*,#35315,.F.);
#46690=ORIENTED_EDGE('',*,*,#35313,.F.);
#46691=ORIENTED_EDGE('',*,*,#35317,.F.);
#46692=ORIENTED_EDGE('',*,*,#35318,.F.);
#46693=ORIENTED_EDGE('',*,*,#35022,.T.);
#46694=ORIENTED_EDGE('',*,*,#35319,.F.);
#46695=ORIENTED_EDGE('',*,*,#35320,.T.);
#46696=ORIENTED_EDGE('',*,*,#35321,.F.);
#46697=ORIENTED_EDGE('',*,*,#35023,.T.);
#46698=ORIENTED_EDGE('',*,*,#35321,.T.);
#46699=ORIENTED_EDGE('',*,*,#35322,.T.);
#46700=ORIENTED_EDGE('',*,*,#35323,.F.);
#46701=ORIENTED_EDGE('',*,*,#35322,.F.);
#46702=ORIENTED_EDGE('',*,*,#35320,.F.);
#46703=ORIENTED_EDGE('',*,*,#35324,.F.);
#46704=ORIENTED_EDGE('',*,*,#35325,.F.);
#46705=ORIENTED_EDGE('',*,*,#35025,.T.);
#46706=ORIENTED_EDGE('',*,*,#35326,.F.);
#46707=ORIENTED_EDGE('',*,*,#35327,.T.);
#46708=ORIENTED_EDGE('',*,*,#35328,.F.);
#46709=ORIENTED_EDGE('',*,*,#35026,.T.);
#46710=ORIENTED_EDGE('',*,*,#35328,.T.);
#46711=ORIENTED_EDGE('',*,*,#35329,.T.);
#46712=ORIENTED_EDGE('',*,*,#35330,.F.);
#46713=ORIENTED_EDGE('',*,*,#35329,.F.);
#46714=ORIENTED_EDGE('',*,*,#35327,.F.);
#46715=ORIENTED_EDGE('',*,*,#35331,.F.);
#46716=ORIENTED_EDGE('',*,*,#35332,.F.);
#46717=ORIENTED_EDGE('',*,*,#35028,.T.);
#46718=ORIENTED_EDGE('',*,*,#35333,.F.);
#46719=ORIENTED_EDGE('',*,*,#35334,.T.);
#46720=ORIENTED_EDGE('',*,*,#35335,.F.);
#46721=ORIENTED_EDGE('',*,*,#35029,.T.);
#46722=ORIENTED_EDGE('',*,*,#35335,.T.);
#46723=ORIENTED_EDGE('',*,*,#35336,.T.);
#46724=ORIENTED_EDGE('',*,*,#35337,.F.);
#46725=ORIENTED_EDGE('',*,*,#35336,.F.);
#46726=ORIENTED_EDGE('',*,*,#35334,.F.);
#46727=ORIENTED_EDGE('',*,*,#35338,.F.);
#46728=ORIENTED_EDGE('',*,*,#35339,.F.);
#46729=ORIENTED_EDGE('',*,*,#35031,.T.);
#46730=ORIENTED_EDGE('',*,*,#35340,.F.);
#46731=ORIENTED_EDGE('',*,*,#35341,.T.);
#46732=ORIENTED_EDGE('',*,*,#35342,.F.);
#46733=ORIENTED_EDGE('',*,*,#35032,.T.);
#46734=ORIENTED_EDGE('',*,*,#35342,.T.);
#46735=ORIENTED_EDGE('',*,*,#35343,.T.);
#46736=ORIENTED_EDGE('',*,*,#35344,.F.);
#46737=ORIENTED_EDGE('',*,*,#35343,.F.);
#46738=ORIENTED_EDGE('',*,*,#35341,.F.);
#46739=ORIENTED_EDGE('',*,*,#35345,.F.);
#46740=ORIENTED_EDGE('',*,*,#35346,.F.);
#46741=ORIENTED_EDGE('',*,*,#35034,.T.);
#46742=ORIENTED_EDGE('',*,*,#35347,.F.);
#46743=ORIENTED_EDGE('',*,*,#35348,.T.);
#46744=ORIENTED_EDGE('',*,*,#35349,.F.);
#46745=ORIENTED_EDGE('',*,*,#35035,.T.);
#46746=ORIENTED_EDGE('',*,*,#35349,.T.);
#46747=ORIENTED_EDGE('',*,*,#35350,.T.);
#46748=ORIENTED_EDGE('',*,*,#35351,.F.);
#46749=ORIENTED_EDGE('',*,*,#35350,.F.);
#46750=ORIENTED_EDGE('',*,*,#35348,.F.);
#46751=ORIENTED_EDGE('',*,*,#35352,.F.);
#46752=ORIENTED_EDGE('',*,*,#35353,.F.);
#46753=ORIENTED_EDGE('',*,*,#35037,.T.);
#46754=ORIENTED_EDGE('',*,*,#35354,.F.);
#46755=ORIENTED_EDGE('',*,*,#35355,.T.);
#46756=ORIENTED_EDGE('',*,*,#35356,.F.);
#46757=ORIENTED_EDGE('',*,*,#35038,.T.);
#46758=ORIENTED_EDGE('',*,*,#35356,.T.);
#46759=ORIENTED_EDGE('',*,*,#35357,.T.);
#46760=ORIENTED_EDGE('',*,*,#35358,.F.);
#46761=ORIENTED_EDGE('',*,*,#35357,.F.);
#46762=ORIENTED_EDGE('',*,*,#35355,.F.);
#46763=ORIENTED_EDGE('',*,*,#35359,.F.);
#46764=ORIENTED_EDGE('',*,*,#35360,.F.);
#46765=ORIENTED_EDGE('',*,*,#35040,.T.);
#46766=ORIENTED_EDGE('',*,*,#35361,.F.);
#46767=ORIENTED_EDGE('',*,*,#35362,.T.);
#46768=ORIENTED_EDGE('',*,*,#35363,.F.);
#46769=ORIENTED_EDGE('',*,*,#35041,.T.);
#46770=ORIENTED_EDGE('',*,*,#35363,.T.);
#46771=ORIENTED_EDGE('',*,*,#35364,.T.);
#46772=ORIENTED_EDGE('',*,*,#35365,.F.);
#46773=ORIENTED_EDGE('',*,*,#35364,.F.);
#46774=ORIENTED_EDGE('',*,*,#35362,.F.);
#46775=ORIENTED_EDGE('',*,*,#35366,.F.);
#46776=ORIENTED_EDGE('',*,*,#35367,.F.);
#46777=ORIENTED_EDGE('',*,*,#35043,.T.);
#46778=ORIENTED_EDGE('',*,*,#35368,.F.);
#46779=ORIENTED_EDGE('',*,*,#35369,.T.);
#46780=ORIENTED_EDGE('',*,*,#35370,.F.);
#46781=ORIENTED_EDGE('',*,*,#35044,.T.);
#46782=ORIENTED_EDGE('',*,*,#35370,.T.);
#46783=ORIENTED_EDGE('',*,*,#35371,.T.);
#46784=ORIENTED_EDGE('',*,*,#35372,.F.);
#46785=ORIENTED_EDGE('',*,*,#35371,.F.);
#46786=ORIENTED_EDGE('',*,*,#35369,.F.);
#46787=ORIENTED_EDGE('',*,*,#35373,.F.);
#46788=ORIENTED_EDGE('',*,*,#35374,.F.);
#46789=ORIENTED_EDGE('',*,*,#35046,.T.);
#46790=ORIENTED_EDGE('',*,*,#35375,.F.);
#46791=ORIENTED_EDGE('',*,*,#35376,.T.);
#46792=ORIENTED_EDGE('',*,*,#35377,.F.);
#46793=ORIENTED_EDGE('',*,*,#35047,.T.);
#46794=ORIENTED_EDGE('',*,*,#35377,.T.);
#46795=ORIENTED_EDGE('',*,*,#35378,.T.);
#46796=ORIENTED_EDGE('',*,*,#35379,.F.);
#46797=ORIENTED_EDGE('',*,*,#35378,.F.);
#46798=ORIENTED_EDGE('',*,*,#35376,.F.);
#46799=ORIENTED_EDGE('',*,*,#35380,.F.);
#46800=ORIENTED_EDGE('',*,*,#35381,.F.);
#46801=ORIENTED_EDGE('',*,*,#35049,.T.);
#46802=ORIENTED_EDGE('',*,*,#35382,.F.);
#46803=ORIENTED_EDGE('',*,*,#35383,.T.);
#46804=ORIENTED_EDGE('',*,*,#35384,.F.);
#46805=ORIENTED_EDGE('',*,*,#35050,.T.);
#46806=ORIENTED_EDGE('',*,*,#35384,.T.);
#46807=ORIENTED_EDGE('',*,*,#35385,.T.);
#46808=ORIENTED_EDGE('',*,*,#35386,.F.);
#46809=ORIENTED_EDGE('',*,*,#35385,.F.);
#46810=ORIENTED_EDGE('',*,*,#35383,.F.);
#46811=ORIENTED_EDGE('',*,*,#35387,.F.);
#46812=ORIENTED_EDGE('',*,*,#35388,.F.);
#46813=ORIENTED_EDGE('',*,*,#35052,.T.);
#46814=ORIENTED_EDGE('',*,*,#35389,.F.);
#46815=ORIENTED_EDGE('',*,*,#35390,.T.);
#46816=ORIENTED_EDGE('',*,*,#35391,.F.);
#46817=ORIENTED_EDGE('',*,*,#35053,.T.);
#46818=ORIENTED_EDGE('',*,*,#35391,.T.);
#46819=ORIENTED_EDGE('',*,*,#35392,.T.);
#46820=ORIENTED_EDGE('',*,*,#35393,.F.);
#46821=ORIENTED_EDGE('',*,*,#35392,.F.);
#46822=ORIENTED_EDGE('',*,*,#35390,.F.);
#46823=ORIENTED_EDGE('',*,*,#35394,.F.);
#46824=ORIENTED_EDGE('',*,*,#35395,.F.);
#46825=ORIENTED_EDGE('',*,*,#35055,.T.);
#46826=ORIENTED_EDGE('',*,*,#35396,.F.);
#46827=ORIENTED_EDGE('',*,*,#35397,.T.);
#46828=ORIENTED_EDGE('',*,*,#35398,.F.);
#46829=ORIENTED_EDGE('',*,*,#35056,.T.);
#46830=ORIENTED_EDGE('',*,*,#35398,.T.);
#46831=ORIENTED_EDGE('',*,*,#35399,.T.);
#46832=ORIENTED_EDGE('',*,*,#35400,.F.);
#46833=ORIENTED_EDGE('',*,*,#35399,.F.);
#46834=ORIENTED_EDGE('',*,*,#35397,.F.);
#46835=ORIENTED_EDGE('',*,*,#35401,.F.);
#46836=ORIENTED_EDGE('',*,*,#35402,.F.);
#46837=ORIENTED_EDGE('',*,*,#35058,.T.);
#46838=ORIENTED_EDGE('',*,*,#35403,.F.);
#46839=ORIENTED_EDGE('',*,*,#35404,.T.);
#46840=ORIENTED_EDGE('',*,*,#35405,.F.);
#46841=ORIENTED_EDGE('',*,*,#35059,.T.);
#46842=ORIENTED_EDGE('',*,*,#35405,.T.);
#46843=ORIENTED_EDGE('',*,*,#35406,.T.);
#46844=ORIENTED_EDGE('',*,*,#35407,.F.);
#46845=ORIENTED_EDGE('',*,*,#35406,.F.);
#46846=ORIENTED_EDGE('',*,*,#35404,.F.);
#46847=ORIENTED_EDGE('',*,*,#35408,.F.);
#46848=ORIENTED_EDGE('',*,*,#35409,.F.);
#46849=ORIENTED_EDGE('',*,*,#35061,.T.);
#46850=ORIENTED_EDGE('',*,*,#35410,.F.);
#46851=ORIENTED_EDGE('',*,*,#35411,.T.);
#46852=ORIENTED_EDGE('',*,*,#35412,.F.);
#46853=ORIENTED_EDGE('',*,*,#35062,.T.);
#46854=ORIENTED_EDGE('',*,*,#35412,.T.);
#46855=ORIENTED_EDGE('',*,*,#35413,.T.);
#46856=ORIENTED_EDGE('',*,*,#35414,.F.);
#46857=ORIENTED_EDGE('',*,*,#35413,.F.);
#46858=ORIENTED_EDGE('',*,*,#35411,.F.);
#46859=ORIENTED_EDGE('',*,*,#35415,.F.);
#46860=ORIENTED_EDGE('',*,*,#35416,.F.);
#46861=ORIENTED_EDGE('',*,*,#35064,.T.);
#46862=ORIENTED_EDGE('',*,*,#35417,.F.);
#46863=ORIENTED_EDGE('',*,*,#35418,.T.);
#46864=ORIENTED_EDGE('',*,*,#35419,.F.);
#46865=ORIENTED_EDGE('',*,*,#35065,.T.);
#46866=ORIENTED_EDGE('',*,*,#35419,.T.);
#46867=ORIENTED_EDGE('',*,*,#35420,.T.);
#46868=ORIENTED_EDGE('',*,*,#35421,.F.);
#46869=ORIENTED_EDGE('',*,*,#35420,.F.);
#46870=ORIENTED_EDGE('',*,*,#35418,.F.);
#46871=ORIENTED_EDGE('',*,*,#35422,.F.);
#46872=ORIENTED_EDGE('',*,*,#35423,.F.);
#46873=ORIENTED_EDGE('',*,*,#35067,.T.);
#46874=ORIENTED_EDGE('',*,*,#35424,.F.);
#46875=ORIENTED_EDGE('',*,*,#35425,.T.);
#46876=ORIENTED_EDGE('',*,*,#35426,.F.);
#46877=ORIENTED_EDGE('',*,*,#35068,.T.);
#46878=ORIENTED_EDGE('',*,*,#35426,.T.);
#46879=ORIENTED_EDGE('',*,*,#35427,.T.);
#46880=ORIENTED_EDGE('',*,*,#35428,.F.);
#46881=ORIENTED_EDGE('',*,*,#35427,.F.);
#46882=ORIENTED_EDGE('',*,*,#35425,.F.);
#46883=ORIENTED_EDGE('',*,*,#35429,.F.);
#46884=ORIENTED_EDGE('',*,*,#35430,.F.);
#46885=ORIENTED_EDGE('',*,*,#35070,.T.);
#46886=ORIENTED_EDGE('',*,*,#35431,.F.);
#46887=ORIENTED_EDGE('',*,*,#35432,.T.);
#46888=ORIENTED_EDGE('',*,*,#35433,.F.);
#46889=ORIENTED_EDGE('',*,*,#35071,.T.);
#46890=ORIENTED_EDGE('',*,*,#35433,.T.);
#46891=ORIENTED_EDGE('',*,*,#35434,.T.);
#46892=ORIENTED_EDGE('',*,*,#35435,.F.);
#46893=ORIENTED_EDGE('',*,*,#35434,.F.);
#46894=ORIENTED_EDGE('',*,*,#35432,.F.);
#46895=ORIENTED_EDGE('',*,*,#35436,.F.);
#46896=ORIENTED_EDGE('',*,*,#35437,.F.);
#46897=ORIENTED_EDGE('',*,*,#35073,.T.);
#46898=ORIENTED_EDGE('',*,*,#35438,.F.);
#46899=ORIENTED_EDGE('',*,*,#35439,.T.);
#46900=ORIENTED_EDGE('',*,*,#35440,.F.);
#46901=ORIENTED_EDGE('',*,*,#35074,.T.);
#46902=ORIENTED_EDGE('',*,*,#35440,.T.);
#46903=ORIENTED_EDGE('',*,*,#35441,.T.);
#46904=ORIENTED_EDGE('',*,*,#35442,.F.);
#46905=ORIENTED_EDGE('',*,*,#35441,.F.);
#46906=ORIENTED_EDGE('',*,*,#35439,.F.);
#46907=ORIENTED_EDGE('',*,*,#35443,.F.);
#46908=ORIENTED_EDGE('',*,*,#35444,.F.);
#46909=ORIENTED_EDGE('',*,*,#35076,.T.);
#46910=ORIENTED_EDGE('',*,*,#35445,.F.);
#46911=ORIENTED_EDGE('',*,*,#34456,.T.);
#46912=ORIENTED_EDGE('',*,*,#35446,.F.);
#46913=ORIENTED_EDGE('',*,*,#35077,.T.);
#46914=ORIENTED_EDGE('',*,*,#35446,.T.);
#46915=ORIENTED_EDGE('',*,*,#34455,.T.);
#46916=ORIENTED_EDGE('',*,*,#35447,.F.);
#46917=ORIENTED_EDGE('',*,*,#35079,.T.);
#46918=ORIENTED_EDGE('',*,*,#35448,.F.);
#46919=ORIENTED_EDGE('',*,*,#35449,.T.);
#46920=ORIENTED_EDGE('',*,*,#35450,.F.);
#46921=ORIENTED_EDGE('',*,*,#35080,.T.);
#46922=ORIENTED_EDGE('',*,*,#35450,.T.);
#46923=ORIENTED_EDGE('',*,*,#35451,.T.);
#46924=ORIENTED_EDGE('',*,*,#35452,.F.);
#46925=ORIENTED_EDGE('',*,*,#35451,.F.);
#46926=ORIENTED_EDGE('',*,*,#35449,.F.);
#46927=ORIENTED_EDGE('',*,*,#35453,.F.);
#46928=ORIENTED_EDGE('',*,*,#35454,.F.);
#46929=ORIENTED_EDGE('',*,*,#35082,.T.);
#46930=ORIENTED_EDGE('',*,*,#35455,.F.);
#46931=ORIENTED_EDGE('',*,*,#35456,.T.);
#46932=ORIENTED_EDGE('',*,*,#35457,.F.);
#46933=ORIENTED_EDGE('',*,*,#35083,.T.);
#46934=ORIENTED_EDGE('',*,*,#35457,.T.);
#46935=ORIENTED_EDGE('',*,*,#35458,.T.);
#46936=ORIENTED_EDGE('',*,*,#35459,.F.);
#46937=ORIENTED_EDGE('',*,*,#35458,.F.);
#46938=ORIENTED_EDGE('',*,*,#35456,.F.);
#46939=ORIENTED_EDGE('',*,*,#35460,.F.);
#46940=ORIENTED_EDGE('',*,*,#35461,.F.);
#46941=ORIENTED_EDGE('',*,*,#35085,.T.);
#46942=ORIENTED_EDGE('',*,*,#35462,.F.);
#46943=ORIENTED_EDGE('',*,*,#35463,.T.);
#46944=ORIENTED_EDGE('',*,*,#35464,.F.);
#46945=ORIENTED_EDGE('',*,*,#35086,.T.);
#46946=ORIENTED_EDGE('',*,*,#35464,.T.);
#46947=ORIENTED_EDGE('',*,*,#35465,.T.);
#46948=ORIENTED_EDGE('',*,*,#35466,.F.);
#46949=ORIENTED_EDGE('',*,*,#35465,.F.);
#46950=ORIENTED_EDGE('',*,*,#35463,.F.);
#46951=ORIENTED_EDGE('',*,*,#35467,.F.);
#46952=ORIENTED_EDGE('',*,*,#35468,.F.);
#46953=ORIENTED_EDGE('',*,*,#35088,.T.);
#46954=ORIENTED_EDGE('',*,*,#35469,.F.);
#46955=ORIENTED_EDGE('',*,*,#35470,.T.);
#46956=ORIENTED_EDGE('',*,*,#35471,.F.);
#46957=ORIENTED_EDGE('',*,*,#35089,.T.);
#46958=ORIENTED_EDGE('',*,*,#35471,.T.);
#46959=ORIENTED_EDGE('',*,*,#35472,.T.);
#46960=ORIENTED_EDGE('',*,*,#35473,.F.);
#46961=ORIENTED_EDGE('',*,*,#35472,.F.);
#46962=ORIENTED_EDGE('',*,*,#35470,.F.);
#46963=ORIENTED_EDGE('',*,*,#35474,.F.);
#46964=ORIENTED_EDGE('',*,*,#35475,.F.);
#46965=ORIENTED_EDGE('',*,*,#35091,.T.);
#46966=ORIENTED_EDGE('',*,*,#35476,.F.);
#46967=ORIENTED_EDGE('',*,*,#35477,.T.);
#46968=ORIENTED_EDGE('',*,*,#35478,.F.);
#46969=ORIENTED_EDGE('',*,*,#35092,.T.);
#46970=ORIENTED_EDGE('',*,*,#35478,.T.);
#46971=ORIENTED_EDGE('',*,*,#35479,.T.);
#46972=ORIENTED_EDGE('',*,*,#35480,.F.);
#46973=ORIENTED_EDGE('',*,*,#35479,.F.);
#46974=ORIENTED_EDGE('',*,*,#35477,.F.);
#46975=ORIENTED_EDGE('',*,*,#35481,.F.);
#46976=ORIENTED_EDGE('',*,*,#35482,.F.);
#46977=ORIENTED_EDGE('',*,*,#35094,.T.);
#46978=ORIENTED_EDGE('',*,*,#35483,.F.);
#46979=ORIENTED_EDGE('',*,*,#35484,.T.);
#46980=ORIENTED_EDGE('',*,*,#35485,.F.);
#46981=ORIENTED_EDGE('',*,*,#35095,.T.);
#46982=ORIENTED_EDGE('',*,*,#35485,.T.);
#46983=ORIENTED_EDGE('',*,*,#35486,.T.);
#46984=ORIENTED_EDGE('',*,*,#35487,.F.);
#46985=ORIENTED_EDGE('',*,*,#35486,.F.);
#46986=ORIENTED_EDGE('',*,*,#35484,.F.);
#46987=ORIENTED_EDGE('',*,*,#35488,.F.);
#46988=ORIENTED_EDGE('',*,*,#35489,.F.);
#46989=ORIENTED_EDGE('',*,*,#35097,.T.);
#46990=ORIENTED_EDGE('',*,*,#35490,.F.);
#46991=ORIENTED_EDGE('',*,*,#35491,.T.);
#46992=ORIENTED_EDGE('',*,*,#35492,.F.);
#46993=ORIENTED_EDGE('',*,*,#35098,.T.);
#46994=ORIENTED_EDGE('',*,*,#35492,.T.);
#46995=ORIENTED_EDGE('',*,*,#35493,.T.);
#46996=ORIENTED_EDGE('',*,*,#35494,.F.);
#46997=ORIENTED_EDGE('',*,*,#35493,.F.);
#46998=ORIENTED_EDGE('',*,*,#35491,.F.);
#46999=ORIENTED_EDGE('',*,*,#35495,.F.);
#47000=ORIENTED_EDGE('',*,*,#35496,.F.);
#47001=ORIENTED_EDGE('',*,*,#35497,.F.);
#47002=ORIENTED_EDGE('',*,*,#35498,.F.);
#47003=ORIENTED_EDGE('',*,*,#35102,.T.);
#47004=ORIENTED_EDGE('',*,*,#35101,.T.);
#47005=ORIENTED_EDGE('',*,*,#35499,.F.);
#47006=ORIENTED_EDGE('',*,*,#35105,.T.);
#47007=ORIENTED_EDGE('',*,*,#35103,.T.);
#47008=ORIENTED_EDGE('',*,*,#35498,.T.);
#47009=ORIENTED_EDGE('',*,*,#35500,.F.);
#47010=ORIENTED_EDGE('',*,*,#35501,.F.);
#47011=ORIENTED_EDGE('',*,*,#35109,.T.);
#47012=ORIENTED_EDGE('',*,*,#35108,.T.);
#47013=ORIENTED_EDGE('',*,*,#35502,.F.);
#47014=ORIENTED_EDGE('',*,*,#35112,.T.);
#47015=ORIENTED_EDGE('',*,*,#35110,.T.);
#47016=ORIENTED_EDGE('',*,*,#35501,.T.);
#47017=ORIENTED_EDGE('',*,*,#35503,.F.);
#47018=ORIENTED_EDGE('',*,*,#35504,.F.);
#47019=ORIENTED_EDGE('',*,*,#35116,.T.);
#47020=ORIENTED_EDGE('',*,*,#35115,.T.);
#47021=ORIENTED_EDGE('',*,*,#35505,.F.);
#47022=ORIENTED_EDGE('',*,*,#35119,.T.);
#47023=ORIENTED_EDGE('',*,*,#35117,.T.);
#47024=ORIENTED_EDGE('',*,*,#35504,.T.);
#47025=ORIENTED_EDGE('',*,*,#35506,.F.);
#47026=ORIENTED_EDGE('',*,*,#35507,.F.);
#47027=ORIENTED_EDGE('',*,*,#35123,.T.);
#47028=ORIENTED_EDGE('',*,*,#35122,.T.);
#47029=ORIENTED_EDGE('',*,*,#35508,.F.);
#47030=ORIENTED_EDGE('',*,*,#35126,.T.);
#47031=ORIENTED_EDGE('',*,*,#35124,.T.);
#47032=ORIENTED_EDGE('',*,*,#35507,.T.);
#47033=ORIENTED_EDGE('',*,*,#35509,.F.);
#47034=ORIENTED_EDGE('',*,*,#35510,.F.);
#47035=ORIENTED_EDGE('',*,*,#35130,.T.);
#47036=ORIENTED_EDGE('',*,*,#35129,.T.);
#47037=ORIENTED_EDGE('',*,*,#35511,.F.);
#47038=ORIENTED_EDGE('',*,*,#35133,.T.);
#47039=ORIENTED_EDGE('',*,*,#35131,.T.);
#47040=ORIENTED_EDGE('',*,*,#35510,.T.);
#47041=ORIENTED_EDGE('',*,*,#35512,.F.);
#47042=ORIENTED_EDGE('',*,*,#35513,.F.);
#47043=ORIENTED_EDGE('',*,*,#35137,.T.);
#47044=ORIENTED_EDGE('',*,*,#35136,.T.);
#47045=ORIENTED_EDGE('',*,*,#35514,.F.);
#47046=ORIENTED_EDGE('',*,*,#35140,.T.);
#47047=ORIENTED_EDGE('',*,*,#35138,.T.);
#47048=ORIENTED_EDGE('',*,*,#35513,.T.);
#47049=ORIENTED_EDGE('',*,*,#35515,.F.);
#47050=ORIENTED_EDGE('',*,*,#35516,.F.);
#47051=ORIENTED_EDGE('',*,*,#35144,.T.);
#47052=ORIENTED_EDGE('',*,*,#35143,.T.);
#47053=ORIENTED_EDGE('',*,*,#35517,.F.);
#47054=ORIENTED_EDGE('',*,*,#35147,.T.);
#47055=ORIENTED_EDGE('',*,*,#35145,.T.);
#47056=ORIENTED_EDGE('',*,*,#35516,.T.);
#47057=ORIENTED_EDGE('',*,*,#35518,.F.);
#47058=ORIENTED_EDGE('',*,*,#35519,.F.);
#47059=ORIENTED_EDGE('',*,*,#35151,.T.);
#47060=ORIENTED_EDGE('',*,*,#35150,.T.);
#47061=ORIENTED_EDGE('',*,*,#35520,.F.);
#47062=ORIENTED_EDGE('',*,*,#35154,.T.);
#47063=ORIENTED_EDGE('',*,*,#35152,.T.);
#47064=ORIENTED_EDGE('',*,*,#35519,.T.);
#47065=ORIENTED_EDGE('',*,*,#35521,.F.);
#47066=ORIENTED_EDGE('',*,*,#35522,.F.);
#47067=ORIENTED_EDGE('',*,*,#35158,.T.);
#47068=ORIENTED_EDGE('',*,*,#35157,.T.);
#47069=ORIENTED_EDGE('',*,*,#35523,.F.);
#47070=ORIENTED_EDGE('',*,*,#35161,.T.);
#47071=ORIENTED_EDGE('',*,*,#35159,.T.);
#47072=ORIENTED_EDGE('',*,*,#35522,.T.);
#47073=ORIENTED_EDGE('',*,*,#35524,.F.);
#47074=ORIENTED_EDGE('',*,*,#35525,.F.);
#47075=ORIENTED_EDGE('',*,*,#35165,.T.);
#47076=ORIENTED_EDGE('',*,*,#35164,.T.);
#47077=ORIENTED_EDGE('',*,*,#35526,.F.);
#47078=ORIENTED_EDGE('',*,*,#35168,.T.);
#47079=ORIENTED_EDGE('',*,*,#35166,.T.);
#47080=ORIENTED_EDGE('',*,*,#35525,.T.);
#47081=ORIENTED_EDGE('',*,*,#35527,.F.);
#47082=ORIENTED_EDGE('',*,*,#35528,.F.);
#47083=ORIENTED_EDGE('',*,*,#35172,.T.);
#47084=ORIENTED_EDGE('',*,*,#35171,.T.);
#47085=ORIENTED_EDGE('',*,*,#35529,.F.);
#47086=ORIENTED_EDGE('',*,*,#35175,.T.);
#47087=ORIENTED_EDGE('',*,*,#35173,.T.);
#47088=ORIENTED_EDGE('',*,*,#35528,.T.);
#47089=ORIENTED_EDGE('',*,*,#35530,.F.);
#47090=ORIENTED_EDGE('',*,*,#35531,.F.);
#47091=ORIENTED_EDGE('',*,*,#35179,.T.);
#47092=ORIENTED_EDGE('',*,*,#35178,.T.);
#47093=ORIENTED_EDGE('',*,*,#35532,.F.);
#47094=ORIENTED_EDGE('',*,*,#35182,.T.);
#47095=ORIENTED_EDGE('',*,*,#35180,.T.);
#47096=ORIENTED_EDGE('',*,*,#35531,.T.);
#47097=ORIENTED_EDGE('',*,*,#35533,.F.);
#47098=ORIENTED_EDGE('',*,*,#35534,.F.);
#47099=ORIENTED_EDGE('',*,*,#35186,.T.);
#47100=ORIENTED_EDGE('',*,*,#35185,.T.);
#47101=ORIENTED_EDGE('',*,*,#35535,.F.);
#47102=ORIENTED_EDGE('',*,*,#35189,.T.);
#47103=ORIENTED_EDGE('',*,*,#35187,.T.);
#47104=ORIENTED_EDGE('',*,*,#35534,.T.);
#47105=ORIENTED_EDGE('',*,*,#35536,.F.);
#47106=ORIENTED_EDGE('',*,*,#35537,.F.);
#47107=ORIENTED_EDGE('',*,*,#35193,.T.);
#47108=ORIENTED_EDGE('',*,*,#35192,.T.);
#47109=ORIENTED_EDGE('',*,*,#35538,.F.);
#47110=ORIENTED_EDGE('',*,*,#35196,.T.);
#47111=ORIENTED_EDGE('',*,*,#35194,.T.);
#47112=ORIENTED_EDGE('',*,*,#35537,.T.);
#47113=ORIENTED_EDGE('',*,*,#35539,.F.);
#47114=ORIENTED_EDGE('',*,*,#35540,.F.);
#47115=ORIENTED_EDGE('',*,*,#34458,.T.);
#47116=ORIENTED_EDGE('',*,*,#35198,.T.);
#47117=ORIENTED_EDGE('',*,*,#35541,.F.);
#47118=ORIENTED_EDGE('',*,*,#35199,.T.);
#47119=ORIENTED_EDGE('',*,*,#34459,.T.);
#47120=ORIENTED_EDGE('',*,*,#35540,.T.);
#47121=ORIENTED_EDGE('',*,*,#35542,.F.);
#47122=ORIENTED_EDGE('',*,*,#35543,.F.);
#47123=ORIENTED_EDGE('',*,*,#35203,.T.);
#47124=ORIENTED_EDGE('',*,*,#35202,.T.);
#47125=ORIENTED_EDGE('',*,*,#35544,.F.);
#47126=ORIENTED_EDGE('',*,*,#35206,.T.);
#47127=ORIENTED_EDGE('',*,*,#35204,.T.);
#47128=ORIENTED_EDGE('',*,*,#35543,.T.);
#47129=ORIENTED_EDGE('',*,*,#35545,.F.);
#47130=ORIENTED_EDGE('',*,*,#35546,.F.);
#47131=ORIENTED_EDGE('',*,*,#35210,.T.);
#47132=ORIENTED_EDGE('',*,*,#35209,.T.);
#47133=ORIENTED_EDGE('',*,*,#35547,.F.);
#47134=ORIENTED_EDGE('',*,*,#35213,.T.);
#47135=ORIENTED_EDGE('',*,*,#35211,.T.);
#47136=ORIENTED_EDGE('',*,*,#35546,.T.);
#47137=ORIENTED_EDGE('',*,*,#35548,.F.);
#47138=ORIENTED_EDGE('',*,*,#35549,.F.);
#47139=ORIENTED_EDGE('',*,*,#35217,.T.);
#47140=ORIENTED_EDGE('',*,*,#35216,.T.);
#47141=ORIENTED_EDGE('',*,*,#35550,.F.);
#47142=ORIENTED_EDGE('',*,*,#35220,.T.);
#47143=ORIENTED_EDGE('',*,*,#35218,.T.);
#47144=ORIENTED_EDGE('',*,*,#35549,.T.);
#47145=ORIENTED_EDGE('',*,*,#35551,.F.);
#47146=ORIENTED_EDGE('',*,*,#35552,.F.);
#47147=ORIENTED_EDGE('',*,*,#35224,.T.);
#47148=ORIENTED_EDGE('',*,*,#35223,.T.);
#47149=ORIENTED_EDGE('',*,*,#35553,.F.);
#47150=ORIENTED_EDGE('',*,*,#35227,.T.);
#47151=ORIENTED_EDGE('',*,*,#35225,.T.);
#47152=ORIENTED_EDGE('',*,*,#35552,.T.);
#47153=ORIENTED_EDGE('',*,*,#35554,.F.);
#47154=ORIENTED_EDGE('',*,*,#35555,.F.);
#47155=ORIENTED_EDGE('',*,*,#35231,.T.);
#47156=ORIENTED_EDGE('',*,*,#35230,.T.);
#47157=ORIENTED_EDGE('',*,*,#35556,.F.);
#47158=ORIENTED_EDGE('',*,*,#35234,.T.);
#47159=ORIENTED_EDGE('',*,*,#35232,.T.);
#47160=ORIENTED_EDGE('',*,*,#35555,.T.);
#47161=ORIENTED_EDGE('',*,*,#35557,.F.);
#47162=ORIENTED_EDGE('',*,*,#35558,.F.);
#47163=ORIENTED_EDGE('',*,*,#35238,.T.);
#47164=ORIENTED_EDGE('',*,*,#35237,.T.);
#47165=ORIENTED_EDGE('',*,*,#35559,.F.);
#47166=ORIENTED_EDGE('',*,*,#35241,.T.);
#47167=ORIENTED_EDGE('',*,*,#35239,.T.);
#47168=ORIENTED_EDGE('',*,*,#35558,.T.);
#47169=ORIENTED_EDGE('',*,*,#35560,.F.);
#47170=ORIENTED_EDGE('',*,*,#35561,.F.);
#47171=ORIENTED_EDGE('',*,*,#35245,.T.);
#47172=ORIENTED_EDGE('',*,*,#35244,.T.);
#47173=ORIENTED_EDGE('',*,*,#35562,.F.);
#47174=ORIENTED_EDGE('',*,*,#35248,.T.);
#47175=ORIENTED_EDGE('',*,*,#35246,.T.);
#47176=ORIENTED_EDGE('',*,*,#35561,.T.);
#47177=ORIENTED_EDGE('',*,*,#35563,.F.);
#47178=ORIENTED_EDGE('',*,*,#35564,.F.);
#47179=ORIENTED_EDGE('',*,*,#35252,.T.);
#47180=ORIENTED_EDGE('',*,*,#35251,.T.);
#47181=ORIENTED_EDGE('',*,*,#35565,.F.);
#47182=ORIENTED_EDGE('',*,*,#35255,.T.);
#47183=ORIENTED_EDGE('',*,*,#35253,.T.);
#47184=ORIENTED_EDGE('',*,*,#35564,.T.);
#47185=ORIENTED_EDGE('',*,*,#35566,.F.);
#47186=ORIENTED_EDGE('',*,*,#35567,.F.);
#47187=ORIENTED_EDGE('',*,*,#35259,.T.);
#47188=ORIENTED_EDGE('',*,*,#35258,.T.);
#47189=ORIENTED_EDGE('',*,*,#35568,.F.);
#47190=ORIENTED_EDGE('',*,*,#35262,.T.);
#47191=ORIENTED_EDGE('',*,*,#35260,.T.);
#47192=ORIENTED_EDGE('',*,*,#35567,.T.);
#47193=ORIENTED_EDGE('',*,*,#35569,.F.);
#47194=ORIENTED_EDGE('',*,*,#35570,.F.);
#47195=ORIENTED_EDGE('',*,*,#35268,.T.);
#47196=ORIENTED_EDGE('',*,*,#35265,.T.);
#47197=ORIENTED_EDGE('',*,*,#35269,.T.);
#47198=ORIENTED_EDGE('',*,*,#35570,.T.);
#47199=ORIENTED_EDGE('',*,*,#35571,.F.);
#47200=ORIENTED_EDGE('',*,*,#35267,.T.);
#47201=ORIENTED_EDGE('',*,*,#35274,.T.);
#47202=ORIENTED_EDGE('',*,*,#35270,.T.);
#47203=ORIENTED_EDGE('',*,*,#35572,.F.);
#47204=ORIENTED_EDGE('',*,*,#35573,.F.);
#47205=ORIENTED_EDGE('',*,*,#35574,.F.);
#47206=ORIENTED_EDGE('',*,*,#35276,.T.);
#47207=ORIENTED_EDGE('',*,*,#35275,.T.);
#47208=ORIENTED_EDGE('',*,*,#35573,.T.);
#47209=ORIENTED_EDGE('',*,*,#35575,.F.);
#47210=ORIENTED_EDGE('',*,*,#35576,.F.);
#47211=ORIENTED_EDGE('',*,*,#35280,.T.);
#47212=ORIENTED_EDGE('',*,*,#35279,.T.);
#47213=ORIENTED_EDGE('',*,*,#35577,.F.);
#47214=ORIENTED_EDGE('',*,*,#35283,.T.);
#47215=ORIENTED_EDGE('',*,*,#35281,.T.);
#47216=ORIENTED_EDGE('',*,*,#35576,.T.);
#47217=ORIENTED_EDGE('',*,*,#35578,.F.);
#47218=ORIENTED_EDGE('',*,*,#35579,.F.);
#47219=ORIENTED_EDGE('',*,*,#35287,.T.);
#47220=ORIENTED_EDGE('',*,*,#35286,.T.);
#47221=ORIENTED_EDGE('',*,*,#35580,.F.);
#47222=ORIENTED_EDGE('',*,*,#35290,.T.);
#47223=ORIENTED_EDGE('',*,*,#35288,.T.);
#47224=ORIENTED_EDGE('',*,*,#35579,.T.);
#47225=ORIENTED_EDGE('',*,*,#35581,.F.);
#47226=ORIENTED_EDGE('',*,*,#35582,.F.);
#47227=ORIENTED_EDGE('',*,*,#35294,.T.);
#47228=ORIENTED_EDGE('',*,*,#35293,.T.);
#47229=ORIENTED_EDGE('',*,*,#35583,.F.);
#47230=ORIENTED_EDGE('',*,*,#35297,.T.);
#47231=ORIENTED_EDGE('',*,*,#35295,.T.);
#47232=ORIENTED_EDGE('',*,*,#35582,.T.);
#47233=ORIENTED_EDGE('',*,*,#35303,.T.);
#47234=ORIENTED_EDGE('',*,*,#35298,.T.);
#47235=ORIENTED_EDGE('',*,*,#35584,.F.);
#47236=ORIENTED_EDGE('',*,*,#35585,.F.);
#47237=ORIENTED_EDGE('',*,*,#35304,.T.);
#47238=ORIENTED_EDGE('',*,*,#35585,.T.);
#47239=ORIENTED_EDGE('',*,*,#35586,.F.);
#47240=ORIENTED_EDGE('',*,*,#35302,.T.);
#47241=ORIENTED_EDGE('',*,*,#35587,.F.);
#47242=ORIENTED_EDGE('',*,*,#35588,.F.);
#47243=ORIENTED_EDGE('',*,*,#35310,.T.);
#47244=ORIENTED_EDGE('',*,*,#35305,.T.);
#47245=ORIENTED_EDGE('',*,*,#35311,.T.);
#47246=ORIENTED_EDGE('',*,*,#35588,.T.);
#47247=ORIENTED_EDGE('',*,*,#35589,.F.);
#47248=ORIENTED_EDGE('',*,*,#35309,.T.);
#47249=ORIENTED_EDGE('',*,*,#35317,.T.);
#47250=ORIENTED_EDGE('',*,*,#35312,.T.);
#47251=ORIENTED_EDGE('',*,*,#35590,.F.);
#47252=ORIENTED_EDGE('',*,*,#35591,.F.);
#47253=ORIENTED_EDGE('',*,*,#35318,.T.);
#47254=ORIENTED_EDGE('',*,*,#35591,.T.);
#47255=ORIENTED_EDGE('',*,*,#35592,.F.);
#47256=ORIENTED_EDGE('',*,*,#35316,.T.);
#47257=ORIENTED_EDGE('',*,*,#35324,.T.);
#47258=ORIENTED_EDGE('',*,*,#35319,.T.);
#47259=ORIENTED_EDGE('',*,*,#35593,.F.);
#47260=ORIENTED_EDGE('',*,*,#35594,.F.);
#47261=ORIENTED_EDGE('',*,*,#35325,.T.);
#47262=ORIENTED_EDGE('',*,*,#35594,.T.);
#47263=ORIENTED_EDGE('',*,*,#35595,.F.);
#47264=ORIENTED_EDGE('',*,*,#35323,.T.);
#47265=ORIENTED_EDGE('',*,*,#35331,.T.);
#47266=ORIENTED_EDGE('',*,*,#35326,.T.);
#47267=ORIENTED_EDGE('',*,*,#35596,.F.);
#47268=ORIENTED_EDGE('',*,*,#35597,.F.);
#47269=ORIENTED_EDGE('',*,*,#35332,.T.);
#47270=ORIENTED_EDGE('',*,*,#35597,.T.);
#47271=ORIENTED_EDGE('',*,*,#35598,.F.);
#47272=ORIENTED_EDGE('',*,*,#35330,.T.);
#47273=ORIENTED_EDGE('',*,*,#35338,.T.);
#47274=ORIENTED_EDGE('',*,*,#35333,.T.);
#47275=ORIENTED_EDGE('',*,*,#35599,.F.);
#47276=ORIENTED_EDGE('',*,*,#35600,.F.);
#47277=ORIENTED_EDGE('',*,*,#35339,.T.);
#47278=ORIENTED_EDGE('',*,*,#35600,.T.);
#47279=ORIENTED_EDGE('',*,*,#35601,.F.);
#47280=ORIENTED_EDGE('',*,*,#35337,.T.);
#47281=ORIENTED_EDGE('',*,*,#35345,.T.);
#47282=ORIENTED_EDGE('',*,*,#35340,.T.);
#47283=ORIENTED_EDGE('',*,*,#35602,.F.);
#47284=ORIENTED_EDGE('',*,*,#35603,.F.);
#47285=ORIENTED_EDGE('',*,*,#35346,.T.);
#47286=ORIENTED_EDGE('',*,*,#35603,.T.);
#47287=ORIENTED_EDGE('',*,*,#35604,.F.);
#47288=ORIENTED_EDGE('',*,*,#35344,.T.);
#47289=ORIENTED_EDGE('',*,*,#35352,.T.);
#47290=ORIENTED_EDGE('',*,*,#35347,.T.);
#47291=ORIENTED_EDGE('',*,*,#35605,.F.);
#47292=ORIENTED_EDGE('',*,*,#35606,.F.);
#47293=ORIENTED_EDGE('',*,*,#35353,.T.);
#47294=ORIENTED_EDGE('',*,*,#35606,.T.);
#47295=ORIENTED_EDGE('',*,*,#35607,.F.);
#47296=ORIENTED_EDGE('',*,*,#35351,.T.);
#47297=ORIENTED_EDGE('',*,*,#35359,.T.);
#47298=ORIENTED_EDGE('',*,*,#35354,.T.);
#47299=ORIENTED_EDGE('',*,*,#35608,.F.);
#47300=ORIENTED_EDGE('',*,*,#35609,.F.);
#47301=ORIENTED_EDGE('',*,*,#35360,.T.);
#47302=ORIENTED_EDGE('',*,*,#35609,.T.);
#47303=ORIENTED_EDGE('',*,*,#35610,.F.);
#47304=ORIENTED_EDGE('',*,*,#35358,.T.);
#47305=ORIENTED_EDGE('',*,*,#35366,.T.);
#47306=ORIENTED_EDGE('',*,*,#35361,.T.);
#47307=ORIENTED_EDGE('',*,*,#35611,.F.);
#47308=ORIENTED_EDGE('',*,*,#35612,.F.);
#47309=ORIENTED_EDGE('',*,*,#35367,.T.);
#47310=ORIENTED_EDGE('',*,*,#35612,.T.);
#47311=ORIENTED_EDGE('',*,*,#35613,.F.);
#47312=ORIENTED_EDGE('',*,*,#35365,.T.);
#47313=ORIENTED_EDGE('',*,*,#35373,.T.);
#47314=ORIENTED_EDGE('',*,*,#35368,.T.);
#47315=ORIENTED_EDGE('',*,*,#35614,.F.);
#47316=ORIENTED_EDGE('',*,*,#35615,.F.);
#47317=ORIENTED_EDGE('',*,*,#35374,.T.);
#47318=ORIENTED_EDGE('',*,*,#35615,.T.);
#47319=ORIENTED_EDGE('',*,*,#35616,.F.);
#47320=ORIENTED_EDGE('',*,*,#35372,.T.);
#47321=ORIENTED_EDGE('',*,*,#35380,.T.);
#47322=ORIENTED_EDGE('',*,*,#35375,.T.);
#47323=ORIENTED_EDGE('',*,*,#35617,.F.);
#47324=ORIENTED_EDGE('',*,*,#35618,.F.);
#47325=ORIENTED_EDGE('',*,*,#35381,.T.);
#47326=ORIENTED_EDGE('',*,*,#35618,.T.);
#47327=ORIENTED_EDGE('',*,*,#35619,.F.);
#47328=ORIENTED_EDGE('',*,*,#35379,.T.);
#47329=ORIENTED_EDGE('',*,*,#35387,.T.);
#47330=ORIENTED_EDGE('',*,*,#35382,.T.);
#47331=ORIENTED_EDGE('',*,*,#35620,.F.);
#47332=ORIENTED_EDGE('',*,*,#35621,.F.);
#47333=ORIENTED_EDGE('',*,*,#35388,.T.);
#47334=ORIENTED_EDGE('',*,*,#35621,.T.);
#47335=ORIENTED_EDGE('',*,*,#35622,.F.);
#47336=ORIENTED_EDGE('',*,*,#35386,.T.);
#47337=ORIENTED_EDGE('',*,*,#35394,.T.);
#47338=ORIENTED_EDGE('',*,*,#35389,.T.);
#47339=ORIENTED_EDGE('',*,*,#35623,.F.);
#47340=ORIENTED_EDGE('',*,*,#35624,.F.);
#47341=ORIENTED_EDGE('',*,*,#35395,.T.);
#47342=ORIENTED_EDGE('',*,*,#35624,.T.);
#47343=ORIENTED_EDGE('',*,*,#35625,.F.);
#47344=ORIENTED_EDGE('',*,*,#35393,.T.);
#47345=ORIENTED_EDGE('',*,*,#35401,.T.);
#47346=ORIENTED_EDGE('',*,*,#35396,.T.);
#47347=ORIENTED_EDGE('',*,*,#35626,.F.);
#47348=ORIENTED_EDGE('',*,*,#35627,.F.);
#47349=ORIENTED_EDGE('',*,*,#35402,.T.);
#47350=ORIENTED_EDGE('',*,*,#35627,.T.);
#47351=ORIENTED_EDGE('',*,*,#35628,.F.);
#47352=ORIENTED_EDGE('',*,*,#35400,.T.);
#47353=ORIENTED_EDGE('',*,*,#35408,.T.);
#47354=ORIENTED_EDGE('',*,*,#35403,.T.);
#47355=ORIENTED_EDGE('',*,*,#35629,.F.);
#47356=ORIENTED_EDGE('',*,*,#35630,.F.);
#47357=ORIENTED_EDGE('',*,*,#35409,.T.);
#47358=ORIENTED_EDGE('',*,*,#35630,.T.);
#47359=ORIENTED_EDGE('',*,*,#35631,.F.);
#47360=ORIENTED_EDGE('',*,*,#35407,.T.);
#47361=ORIENTED_EDGE('',*,*,#35415,.T.);
#47362=ORIENTED_EDGE('',*,*,#35410,.T.);
#47363=ORIENTED_EDGE('',*,*,#35632,.F.);
#47364=ORIENTED_EDGE('',*,*,#35633,.F.);
#47365=ORIENTED_EDGE('',*,*,#35416,.T.);
#47366=ORIENTED_EDGE('',*,*,#35633,.T.);
#47367=ORIENTED_EDGE('',*,*,#35634,.F.);
#47368=ORIENTED_EDGE('',*,*,#35414,.T.);
#47369=ORIENTED_EDGE('',*,*,#35422,.T.);
#47370=ORIENTED_EDGE('',*,*,#35417,.T.);
#47371=ORIENTED_EDGE('',*,*,#35635,.F.);
#47372=ORIENTED_EDGE('',*,*,#35636,.F.);
#47373=ORIENTED_EDGE('',*,*,#35423,.T.);
#47374=ORIENTED_EDGE('',*,*,#35636,.T.);
#47375=ORIENTED_EDGE('',*,*,#35637,.F.);
#47376=ORIENTED_EDGE('',*,*,#35421,.T.);
#47377=ORIENTED_EDGE('',*,*,#35429,.T.);
#47378=ORIENTED_EDGE('',*,*,#35424,.T.);
#47379=ORIENTED_EDGE('',*,*,#35638,.F.);
#47380=ORIENTED_EDGE('',*,*,#35639,.F.);
#47381=ORIENTED_EDGE('',*,*,#35430,.T.);
#47382=ORIENTED_EDGE('',*,*,#35639,.T.);
#47383=ORIENTED_EDGE('',*,*,#35640,.F.);
#47384=ORIENTED_EDGE('',*,*,#35428,.T.);
#47385=ORIENTED_EDGE('',*,*,#35436,.T.);
#47386=ORIENTED_EDGE('',*,*,#35431,.T.);
#47387=ORIENTED_EDGE('',*,*,#35641,.F.);
#47388=ORIENTED_EDGE('',*,*,#35642,.F.);
#47389=ORIENTED_EDGE('',*,*,#35437,.T.);
#47390=ORIENTED_EDGE('',*,*,#35642,.T.);
#47391=ORIENTED_EDGE('',*,*,#35643,.F.);
#47392=ORIENTED_EDGE('',*,*,#35435,.T.);
#47393=ORIENTED_EDGE('',*,*,#35443,.T.);
#47394=ORIENTED_EDGE('',*,*,#35438,.T.);
#47395=ORIENTED_EDGE('',*,*,#35644,.F.);
#47396=ORIENTED_EDGE('',*,*,#35645,.F.);
#47397=ORIENTED_EDGE('',*,*,#35444,.T.);
#47398=ORIENTED_EDGE('',*,*,#35645,.T.);
#47399=ORIENTED_EDGE('',*,*,#35646,.F.);
#47400=ORIENTED_EDGE('',*,*,#35442,.T.);
#47401=ORIENTED_EDGE('',*,*,#34453,.T.);
#47402=ORIENTED_EDGE('',*,*,#35445,.T.);
#47403=ORIENTED_EDGE('',*,*,#35647,.F.);
#47404=ORIENTED_EDGE('',*,*,#35648,.F.);
#47405=ORIENTED_EDGE('',*,*,#34454,.T.);
#47406=ORIENTED_EDGE('',*,*,#35648,.T.);
#47407=ORIENTED_EDGE('',*,*,#35649,.F.);
#47408=ORIENTED_EDGE('',*,*,#35447,.T.);
#47409=ORIENTED_EDGE('',*,*,#35453,.T.);
#47410=ORIENTED_EDGE('',*,*,#35448,.T.);
#47411=ORIENTED_EDGE('',*,*,#35650,.F.);
#47412=ORIENTED_EDGE('',*,*,#35651,.F.);
#47413=ORIENTED_EDGE('',*,*,#35454,.T.);
#47414=ORIENTED_EDGE('',*,*,#35651,.T.);
#47415=ORIENTED_EDGE('',*,*,#35652,.F.);
#47416=ORIENTED_EDGE('',*,*,#35452,.T.);
#47417=ORIENTED_EDGE('',*,*,#35460,.T.);
#47418=ORIENTED_EDGE('',*,*,#35455,.T.);
#47419=ORIENTED_EDGE('',*,*,#35653,.F.);
#47420=ORIENTED_EDGE('',*,*,#35654,.F.);
#47421=ORIENTED_EDGE('',*,*,#35461,.T.);
#47422=ORIENTED_EDGE('',*,*,#35654,.T.);
#47423=ORIENTED_EDGE('',*,*,#35655,.F.);
#47424=ORIENTED_EDGE('',*,*,#35459,.T.);
#47425=ORIENTED_EDGE('',*,*,#35467,.T.);
#47426=ORIENTED_EDGE('',*,*,#35462,.T.);
#47427=ORIENTED_EDGE('',*,*,#35656,.F.);
#47428=ORIENTED_EDGE('',*,*,#35657,.F.);
#47429=ORIENTED_EDGE('',*,*,#35468,.T.);
#47430=ORIENTED_EDGE('',*,*,#35657,.T.);
#47431=ORIENTED_EDGE('',*,*,#35658,.F.);
#47432=ORIENTED_EDGE('',*,*,#35466,.T.);
#47433=ORIENTED_EDGE('',*,*,#35474,.T.);
#47434=ORIENTED_EDGE('',*,*,#35469,.T.);
#47435=ORIENTED_EDGE('',*,*,#35659,.F.);
#47436=ORIENTED_EDGE('',*,*,#35660,.F.);
#47437=ORIENTED_EDGE('',*,*,#35475,.T.);
#47438=ORIENTED_EDGE('',*,*,#35660,.T.);
#47439=ORIENTED_EDGE('',*,*,#35661,.F.);
#47440=ORIENTED_EDGE('',*,*,#35473,.T.);
#47441=ORIENTED_EDGE('',*,*,#35481,.T.);
#47442=ORIENTED_EDGE('',*,*,#35476,.T.);
#47443=ORIENTED_EDGE('',*,*,#35662,.F.);
#47444=ORIENTED_EDGE('',*,*,#35663,.F.);
#47445=ORIENTED_EDGE('',*,*,#35482,.T.);
#47446=ORIENTED_EDGE('',*,*,#35663,.T.);
#47447=ORIENTED_EDGE('',*,*,#35664,.F.);
#47448=ORIENTED_EDGE('',*,*,#35480,.T.);
#47449=ORIENTED_EDGE('',*,*,#35488,.T.);
#47450=ORIENTED_EDGE('',*,*,#35483,.T.);
#47451=ORIENTED_EDGE('',*,*,#35665,.F.);
#47452=ORIENTED_EDGE('',*,*,#35666,.F.);
#47453=ORIENTED_EDGE('',*,*,#35489,.T.);
#47454=ORIENTED_EDGE('',*,*,#35666,.T.);
#47455=ORIENTED_EDGE('',*,*,#35667,.F.);
#47456=ORIENTED_EDGE('',*,*,#35487,.T.);
#47457=ORIENTED_EDGE('',*,*,#35495,.T.);
#47458=ORIENTED_EDGE('',*,*,#35490,.T.);
#47459=ORIENTED_EDGE('',*,*,#35668,.F.);
#47460=ORIENTED_EDGE('',*,*,#35669,.F.);
#47461=ORIENTED_EDGE('',*,*,#35496,.T.);
#47462=ORIENTED_EDGE('',*,*,#35669,.T.);
#47463=ORIENTED_EDGE('',*,*,#35670,.F.);
#47464=ORIENTED_EDGE('',*,*,#35494,.T.);
#47465=ORIENTED_EDGE('',*,*,#35671,.T.);
#47466=ORIENTED_EDGE('',*,*,#35672,.F.);
#47467=ORIENTED_EDGE('',*,*,#35497,.T.);
#47468=ORIENTED_EDGE('',*,*,#35673,.F.);
#47469=ORIENTED_EDGE('',*,*,#35674,.T.);
#47470=ORIENTED_EDGE('',*,*,#35675,.F.);
#47471=ORIENTED_EDGE('',*,*,#35499,.T.);
#47472=ORIENTED_EDGE('',*,*,#35676,.F.);
#47473=ORIENTED_EDGE('',*,*,#35677,.F.);
#47474=ORIENTED_EDGE('',*,*,#35678,.F.);
#47475=ORIENTED_EDGE('',*,*,#35679,.F.);
#47476=ORIENTED_EDGE('',*,*,#35674,.F.);
#47477=ORIENTED_EDGE('',*,*,#35679,.T.);
#47478=ORIENTED_EDGE('',*,*,#35680,.F.);
#47479=ORIENTED_EDGE('',*,*,#35500,.T.);
#47480=ORIENTED_EDGE('',*,*,#35675,.T.);
#47481=ORIENTED_EDGE('',*,*,#35681,.T.);
#47482=ORIENTED_EDGE('',*,*,#35682,.F.);
#47483=ORIENTED_EDGE('',*,*,#35502,.T.);
#47484=ORIENTED_EDGE('',*,*,#35683,.F.);
#47485=ORIENTED_EDGE('',*,*,#35684,.F.);
#47486=ORIENTED_EDGE('',*,*,#35685,.F.);
#47487=ORIENTED_EDGE('',*,*,#35686,.F.);
#47488=ORIENTED_EDGE('',*,*,#35681,.F.);
#47489=ORIENTED_EDGE('',*,*,#35686,.T.);
#47490=ORIENTED_EDGE('',*,*,#35687,.F.);
#47491=ORIENTED_EDGE('',*,*,#35503,.T.);
#47492=ORIENTED_EDGE('',*,*,#35682,.T.);
#47493=ORIENTED_EDGE('',*,*,#35688,.T.);
#47494=ORIENTED_EDGE('',*,*,#35689,.F.);
#47495=ORIENTED_EDGE('',*,*,#35505,.T.);
#47496=ORIENTED_EDGE('',*,*,#35690,.F.);
#47497=ORIENTED_EDGE('',*,*,#35691,.F.);
#47498=ORIENTED_EDGE('',*,*,#35692,.F.);
#47499=ORIENTED_EDGE('',*,*,#35693,.F.);
#47500=ORIENTED_EDGE('',*,*,#35688,.F.);
#47501=ORIENTED_EDGE('',*,*,#35693,.T.);
#47502=ORIENTED_EDGE('',*,*,#35694,.F.);
#47503=ORIENTED_EDGE('',*,*,#35506,.T.);
#47504=ORIENTED_EDGE('',*,*,#35689,.T.);
#47505=ORIENTED_EDGE('',*,*,#35695,.T.);
#47506=ORIENTED_EDGE('',*,*,#35696,.F.);
#47507=ORIENTED_EDGE('',*,*,#35508,.T.);
#47508=ORIENTED_EDGE('',*,*,#35697,.F.);
#47509=ORIENTED_EDGE('',*,*,#35698,.F.);
#47510=ORIENTED_EDGE('',*,*,#35699,.F.);
#47511=ORIENTED_EDGE('',*,*,#35700,.F.);
#47512=ORIENTED_EDGE('',*,*,#35695,.F.);
#47513=ORIENTED_EDGE('',*,*,#35700,.T.);
#47514=ORIENTED_EDGE('',*,*,#35701,.F.);
#47515=ORIENTED_EDGE('',*,*,#35509,.T.);
#47516=ORIENTED_EDGE('',*,*,#35696,.T.);
#47517=ORIENTED_EDGE('',*,*,#35702,.T.);
#47518=ORIENTED_EDGE('',*,*,#35703,.F.);
#47519=ORIENTED_EDGE('',*,*,#35511,.T.);
#47520=ORIENTED_EDGE('',*,*,#35704,.F.);
#47521=ORIENTED_EDGE('',*,*,#35705,.F.);
#47522=ORIENTED_EDGE('',*,*,#35706,.F.);
#47523=ORIENTED_EDGE('',*,*,#35707,.F.);
#47524=ORIENTED_EDGE('',*,*,#35702,.F.);
#47525=ORIENTED_EDGE('',*,*,#35707,.T.);
#47526=ORIENTED_EDGE('',*,*,#35708,.F.);
#47527=ORIENTED_EDGE('',*,*,#35512,.T.);
#47528=ORIENTED_EDGE('',*,*,#35703,.T.);
#47529=ORIENTED_EDGE('',*,*,#35709,.T.);
#47530=ORIENTED_EDGE('',*,*,#35710,.F.);
#47531=ORIENTED_EDGE('',*,*,#35514,.T.);
#47532=ORIENTED_EDGE('',*,*,#35711,.F.);
#47533=ORIENTED_EDGE('',*,*,#35712,.F.);
#47534=ORIENTED_EDGE('',*,*,#35713,.F.);
#47535=ORIENTED_EDGE('',*,*,#35714,.F.);
#47536=ORIENTED_EDGE('',*,*,#35709,.F.);
#47537=ORIENTED_EDGE('',*,*,#35714,.T.);
#47538=ORIENTED_EDGE('',*,*,#35715,.F.);
#47539=ORIENTED_EDGE('',*,*,#35515,.T.);
#47540=ORIENTED_EDGE('',*,*,#35710,.T.);
#47541=ORIENTED_EDGE('',*,*,#34450,.T.);
#47542=ORIENTED_EDGE('',*,*,#35716,.F.);
#47543=ORIENTED_EDGE('',*,*,#35517,.T.);
#47544=ORIENTED_EDGE('',*,*,#35717,.F.);
#47545=ORIENTED_EDGE('',*,*,#34449,.T.);
#47546=ORIENTED_EDGE('',*,*,#35718,.F.);
#47547=ORIENTED_EDGE('',*,*,#35518,.T.);
#47548=ORIENTED_EDGE('',*,*,#35716,.T.);
#47549=ORIENTED_EDGE('',*,*,#35719,.T.);
#47550=ORIENTED_EDGE('',*,*,#35720,.F.);
#47551=ORIENTED_EDGE('',*,*,#35520,.T.);
#47552=ORIENTED_EDGE('',*,*,#35721,.F.);
#47553=ORIENTED_EDGE('',*,*,#35722,.F.);
#47554=ORIENTED_EDGE('',*,*,#35723,.F.);
#47555=ORIENTED_EDGE('',*,*,#35724,.F.);
#47556=ORIENTED_EDGE('',*,*,#35719,.F.);
#47557=ORIENTED_EDGE('',*,*,#35724,.T.);
#47558=ORIENTED_EDGE('',*,*,#35725,.F.);
#47559=ORIENTED_EDGE('',*,*,#35521,.T.);
#47560=ORIENTED_EDGE('',*,*,#35720,.T.);
#47561=ORIENTED_EDGE('',*,*,#35726,.T.);
#47562=ORIENTED_EDGE('',*,*,#35727,.F.);
#47563=ORIENTED_EDGE('',*,*,#35523,.T.);
#47564=ORIENTED_EDGE('',*,*,#35728,.F.);
#47565=ORIENTED_EDGE('',*,*,#35729,.F.);
#47566=ORIENTED_EDGE('',*,*,#35730,.F.);
#47567=ORIENTED_EDGE('',*,*,#35731,.F.);
#47568=ORIENTED_EDGE('',*,*,#35726,.F.);
#47569=ORIENTED_EDGE('',*,*,#35731,.T.);
#47570=ORIENTED_EDGE('',*,*,#35732,.F.);
#47571=ORIENTED_EDGE('',*,*,#35524,.T.);
#47572=ORIENTED_EDGE('',*,*,#35727,.T.);
#47573=ORIENTED_EDGE('',*,*,#35733,.T.);
#47574=ORIENTED_EDGE('',*,*,#35734,.F.);
#47575=ORIENTED_EDGE('',*,*,#35526,.T.);
#47576=ORIENTED_EDGE('',*,*,#35735,.F.);
#47577=ORIENTED_EDGE('',*,*,#35736,.F.);
#47578=ORIENTED_EDGE('',*,*,#35737,.F.);
#47579=ORIENTED_EDGE('',*,*,#35738,.F.);
#47580=ORIENTED_EDGE('',*,*,#35733,.F.);
#47581=ORIENTED_EDGE('',*,*,#35738,.T.);
#47582=ORIENTED_EDGE('',*,*,#35739,.F.);
#47583=ORIENTED_EDGE('',*,*,#35527,.T.);
#47584=ORIENTED_EDGE('',*,*,#35734,.T.);
#47585=ORIENTED_EDGE('',*,*,#35740,.T.);
#47586=ORIENTED_EDGE('',*,*,#35741,.F.);
#47587=ORIENTED_EDGE('',*,*,#35529,.T.);
#47588=ORIENTED_EDGE('',*,*,#35742,.F.);
#47589=ORIENTED_EDGE('',*,*,#35743,.F.);
#47590=ORIENTED_EDGE('',*,*,#35744,.F.);
#47591=ORIENTED_EDGE('',*,*,#35745,.F.);
#47592=ORIENTED_EDGE('',*,*,#35740,.F.);
#47593=ORIENTED_EDGE('',*,*,#35745,.T.);
#47594=ORIENTED_EDGE('',*,*,#35746,.F.);
#47595=ORIENTED_EDGE('',*,*,#35530,.T.);
#47596=ORIENTED_EDGE('',*,*,#35741,.T.);
#47597=ORIENTED_EDGE('',*,*,#35747,.T.);
#47598=ORIENTED_EDGE('',*,*,#35748,.F.);
#47599=ORIENTED_EDGE('',*,*,#35532,.T.);
#47600=ORIENTED_EDGE('',*,*,#35749,.F.);
#47601=ORIENTED_EDGE('',*,*,#35750,.F.);
#47602=ORIENTED_EDGE('',*,*,#35751,.F.);
#47603=ORIENTED_EDGE('',*,*,#35752,.F.);
#47604=ORIENTED_EDGE('',*,*,#35747,.F.);
#47605=ORIENTED_EDGE('',*,*,#35752,.T.);
#47606=ORIENTED_EDGE('',*,*,#35753,.F.);
#47607=ORIENTED_EDGE('',*,*,#35533,.T.);
#47608=ORIENTED_EDGE('',*,*,#35748,.T.);
#47609=ORIENTED_EDGE('',*,*,#35754,.T.);
#47610=ORIENTED_EDGE('',*,*,#35755,.F.);
#47611=ORIENTED_EDGE('',*,*,#35535,.T.);
#47612=ORIENTED_EDGE('',*,*,#35756,.F.);
#47613=ORIENTED_EDGE('',*,*,#35757,.F.);
#47614=ORIENTED_EDGE('',*,*,#35758,.F.);
#47615=ORIENTED_EDGE('',*,*,#35759,.F.);
#47616=ORIENTED_EDGE('',*,*,#35754,.F.);
#47617=ORIENTED_EDGE('',*,*,#35759,.T.);
#47618=ORIENTED_EDGE('',*,*,#35760,.F.);
#47619=ORIENTED_EDGE('',*,*,#35536,.T.);
#47620=ORIENTED_EDGE('',*,*,#35755,.T.);
#47621=ORIENTED_EDGE('',*,*,#35761,.T.);
#47622=ORIENTED_EDGE('',*,*,#35762,.F.);
#47623=ORIENTED_EDGE('',*,*,#35538,.T.);
#47624=ORIENTED_EDGE('',*,*,#35763,.F.);
#47625=ORIENTED_EDGE('',*,*,#35764,.F.);
#47626=ORIENTED_EDGE('',*,*,#35765,.F.);
#47627=ORIENTED_EDGE('',*,*,#35766,.F.);
#47628=ORIENTED_EDGE('',*,*,#35761,.F.);
#47629=ORIENTED_EDGE('',*,*,#35766,.T.);
#47630=ORIENTED_EDGE('',*,*,#35767,.F.);
#47631=ORIENTED_EDGE('',*,*,#35539,.T.);
#47632=ORIENTED_EDGE('',*,*,#35762,.T.);
#47633=ORIENTED_EDGE('',*,*,#35768,.T.);
#47634=ORIENTED_EDGE('',*,*,#35769,.F.);
#47635=ORIENTED_EDGE('',*,*,#35541,.T.);
#47636=ORIENTED_EDGE('',*,*,#35770,.F.);
#47637=ORIENTED_EDGE('',*,*,#35771,.F.);
#47638=ORIENTED_EDGE('',*,*,#35772,.F.);
#47639=ORIENTED_EDGE('',*,*,#35773,.F.);
#47640=ORIENTED_EDGE('',*,*,#35768,.F.);
#47641=ORIENTED_EDGE('',*,*,#35773,.T.);
#47642=ORIENTED_EDGE('',*,*,#35774,.F.);
#47643=ORIENTED_EDGE('',*,*,#35542,.T.);
#47644=ORIENTED_EDGE('',*,*,#35769,.T.);
#47645=ORIENTED_EDGE('',*,*,#35775,.T.);
#47646=ORIENTED_EDGE('',*,*,#35776,.F.);
#47647=ORIENTED_EDGE('',*,*,#35544,.T.);
#47648=ORIENTED_EDGE('',*,*,#35777,.F.);
#47649=ORIENTED_EDGE('',*,*,#35778,.F.);
#47650=ORIENTED_EDGE('',*,*,#35779,.F.);
#47651=ORIENTED_EDGE('',*,*,#35780,.F.);
#47652=ORIENTED_EDGE('',*,*,#35775,.F.);
#47653=ORIENTED_EDGE('',*,*,#35780,.T.);
#47654=ORIENTED_EDGE('',*,*,#35781,.F.);
#47655=ORIENTED_EDGE('',*,*,#35545,.T.);
#47656=ORIENTED_EDGE('',*,*,#35776,.T.);
#47657=ORIENTED_EDGE('',*,*,#35782,.T.);
#47658=ORIENTED_EDGE('',*,*,#35783,.F.);
#47659=ORIENTED_EDGE('',*,*,#35547,.T.);
#47660=ORIENTED_EDGE('',*,*,#35784,.F.);
#47661=ORIENTED_EDGE('',*,*,#35785,.F.);
#47662=ORIENTED_EDGE('',*,*,#35786,.F.);
#47663=ORIENTED_EDGE('',*,*,#35787,.F.);
#47664=ORIENTED_EDGE('',*,*,#35782,.F.);
#47665=ORIENTED_EDGE('',*,*,#35787,.T.);
#47666=ORIENTED_EDGE('',*,*,#35788,.F.);
#47667=ORIENTED_EDGE('',*,*,#35548,.T.);
#47668=ORIENTED_EDGE('',*,*,#35783,.T.);
#47669=ORIENTED_EDGE('',*,*,#35789,.T.);
#47670=ORIENTED_EDGE('',*,*,#35790,.F.);
#47671=ORIENTED_EDGE('',*,*,#35550,.T.);
#47672=ORIENTED_EDGE('',*,*,#35791,.F.);
#47673=ORIENTED_EDGE('',*,*,#35792,.F.);
#47674=ORIENTED_EDGE('',*,*,#35793,.F.);
#47675=ORIENTED_EDGE('',*,*,#35794,.F.);
#47676=ORIENTED_EDGE('',*,*,#35789,.F.);
#47677=ORIENTED_EDGE('',*,*,#35794,.T.);
#47678=ORIENTED_EDGE('',*,*,#35795,.F.);
#47679=ORIENTED_EDGE('',*,*,#35551,.T.);
#47680=ORIENTED_EDGE('',*,*,#35790,.T.);
#47681=ORIENTED_EDGE('',*,*,#35796,.T.);
#47682=ORIENTED_EDGE('',*,*,#35797,.F.);
#47683=ORIENTED_EDGE('',*,*,#35553,.T.);
#47684=ORIENTED_EDGE('',*,*,#35798,.F.);
#47685=ORIENTED_EDGE('',*,*,#35799,.F.);
#47686=ORIENTED_EDGE('',*,*,#35800,.F.);
#47687=ORIENTED_EDGE('',*,*,#35801,.F.);
#47688=ORIENTED_EDGE('',*,*,#35796,.F.);
#47689=ORIENTED_EDGE('',*,*,#35801,.T.);
#47690=ORIENTED_EDGE('',*,*,#35802,.F.);
#47691=ORIENTED_EDGE('',*,*,#35554,.T.);
#47692=ORIENTED_EDGE('',*,*,#35797,.T.);
#47693=ORIENTED_EDGE('',*,*,#35803,.T.);
#47694=ORIENTED_EDGE('',*,*,#35804,.F.);
#47695=ORIENTED_EDGE('',*,*,#35556,.T.);
#47696=ORIENTED_EDGE('',*,*,#35805,.F.);
#47697=ORIENTED_EDGE('',*,*,#35806,.F.);
#47698=ORIENTED_EDGE('',*,*,#35807,.F.);
#47699=ORIENTED_EDGE('',*,*,#35808,.F.);
#47700=ORIENTED_EDGE('',*,*,#35803,.F.);
#47701=ORIENTED_EDGE('',*,*,#35808,.T.);
#47702=ORIENTED_EDGE('',*,*,#35809,.F.);
#47703=ORIENTED_EDGE('',*,*,#35557,.T.);
#47704=ORIENTED_EDGE('',*,*,#35804,.T.);
#47705=ORIENTED_EDGE('',*,*,#35810,.T.);
#47706=ORIENTED_EDGE('',*,*,#35811,.F.);
#47707=ORIENTED_EDGE('',*,*,#35559,.T.);
#47708=ORIENTED_EDGE('',*,*,#35812,.F.);
#47709=ORIENTED_EDGE('',*,*,#35813,.F.);
#47710=ORIENTED_EDGE('',*,*,#35814,.F.);
#47711=ORIENTED_EDGE('',*,*,#35815,.F.);
#47712=ORIENTED_EDGE('',*,*,#35810,.F.);
#47713=ORIENTED_EDGE('',*,*,#35815,.T.);
#47714=ORIENTED_EDGE('',*,*,#35816,.F.);
#47715=ORIENTED_EDGE('',*,*,#35560,.T.);
#47716=ORIENTED_EDGE('',*,*,#35811,.T.);
#47717=ORIENTED_EDGE('',*,*,#35817,.T.);
#47718=ORIENTED_EDGE('',*,*,#35818,.F.);
#47719=ORIENTED_EDGE('',*,*,#35562,.T.);
#47720=ORIENTED_EDGE('',*,*,#35819,.F.);
#47721=ORIENTED_EDGE('',*,*,#35820,.F.);
#47722=ORIENTED_EDGE('',*,*,#35821,.F.);
#47723=ORIENTED_EDGE('',*,*,#35822,.F.);
#47724=ORIENTED_EDGE('',*,*,#35817,.F.);
#47725=ORIENTED_EDGE('',*,*,#35822,.T.);
#47726=ORIENTED_EDGE('',*,*,#35823,.F.);
#47727=ORIENTED_EDGE('',*,*,#35563,.T.);
#47728=ORIENTED_EDGE('',*,*,#35818,.T.);
#47729=ORIENTED_EDGE('',*,*,#35824,.T.);
#47730=ORIENTED_EDGE('',*,*,#35825,.F.);
#47731=ORIENTED_EDGE('',*,*,#35565,.T.);
#47732=ORIENTED_EDGE('',*,*,#35826,.F.);
#47733=ORIENTED_EDGE('',*,*,#35827,.F.);
#47734=ORIENTED_EDGE('',*,*,#35828,.F.);
#47735=ORIENTED_EDGE('',*,*,#35829,.F.);
#47736=ORIENTED_EDGE('',*,*,#35824,.F.);
#47737=ORIENTED_EDGE('',*,*,#35829,.T.);
#47738=ORIENTED_EDGE('',*,*,#35830,.F.);
#47739=ORIENTED_EDGE('',*,*,#35566,.T.);
#47740=ORIENTED_EDGE('',*,*,#35825,.T.);
#47741=ORIENTED_EDGE('',*,*,#35831,.T.);
#47742=ORIENTED_EDGE('',*,*,#35832,.F.);
#47743=ORIENTED_EDGE('',*,*,#35568,.T.);
#47744=ORIENTED_EDGE('',*,*,#35833,.F.);
#47745=ORIENTED_EDGE('',*,*,#35834,.T.);
#47746=ORIENTED_EDGE('',*,*,#35835,.F.);
#47747=ORIENTED_EDGE('',*,*,#35569,.T.);
#47748=ORIENTED_EDGE('',*,*,#35832,.T.);
#47749=ORIENTED_EDGE('',*,*,#35836,.F.);
#47750=ORIENTED_EDGE('',*,*,#35837,.F.);
#47751=ORIENTED_EDGE('',*,*,#35834,.F.);
#47752=ORIENTED_EDGE('',*,*,#35831,.F.);
#47753=ORIENTED_EDGE('',*,*,#35571,.T.);
#47754=ORIENTED_EDGE('',*,*,#35838,.F.);
#47755=ORIENTED_EDGE('',*,*,#35839,.T.);
#47756=ORIENTED_EDGE('',*,*,#35840,.F.);
#47757=ORIENTED_EDGE('',*,*,#35841,.F.);
#47758=ORIENTED_EDGE('',*,*,#35839,.F.);
#47759=ORIENTED_EDGE('',*,*,#35842,.F.);
#47760=ORIENTED_EDGE('',*,*,#35843,.F.);
#47761=ORIENTED_EDGE('',*,*,#35572,.T.);
#47762=ORIENTED_EDGE('',*,*,#35840,.T.);
#47763=ORIENTED_EDGE('',*,*,#35841,.T.);
#47764=ORIENTED_EDGE('',*,*,#35844,.F.);
#47765=ORIENTED_EDGE('',*,*,#35845,.T.);
#47766=ORIENTED_EDGE('',*,*,#35846,.F.);
#47767=ORIENTED_EDGE('',*,*,#35574,.T.);
#47768=ORIENTED_EDGE('',*,*,#35847,.F.);
#47769=ORIENTED_EDGE('',*,*,#35848,.F.);
#47770=ORIENTED_EDGE('',*,*,#35849,.F.);
#47771=ORIENTED_EDGE('',*,*,#35850,.F.);
#47772=ORIENTED_EDGE('',*,*,#35845,.F.);
#47773=ORIENTED_EDGE('',*,*,#35850,.T.);
#47774=ORIENTED_EDGE('',*,*,#35851,.F.);
#47775=ORIENTED_EDGE('',*,*,#35575,.T.);
#47776=ORIENTED_EDGE('',*,*,#35846,.T.);
#47777=ORIENTED_EDGE('',*,*,#35852,.T.);
#47778=ORIENTED_EDGE('',*,*,#35853,.F.);
#47779=ORIENTED_EDGE('',*,*,#35577,.T.);
#47780=ORIENTED_EDGE('',*,*,#35854,.F.);
#47781=ORIENTED_EDGE('',*,*,#35855,.F.);
#47782=ORIENTED_EDGE('',*,*,#35856,.F.);
#47783=ORIENTED_EDGE('',*,*,#35857,.F.);
#47784=ORIENTED_EDGE('',*,*,#35852,.F.);
#47785=ORIENTED_EDGE('',*,*,#35857,.T.);
#47786=ORIENTED_EDGE('',*,*,#35858,.F.);
#47787=ORIENTED_EDGE('',*,*,#35578,.T.);
#47788=ORIENTED_EDGE('',*,*,#35853,.T.);
#47789=ORIENTED_EDGE('',*,*,#35859,.T.);
#47790=ORIENTED_EDGE('',*,*,#35860,.F.);
#47791=ORIENTED_EDGE('',*,*,#35580,.T.);
#47792=ORIENTED_EDGE('',*,*,#35861,.F.);
#47793=ORIENTED_EDGE('',*,*,#35862,.F.);
#47794=ORIENTED_EDGE('',*,*,#35863,.F.);
#47795=ORIENTED_EDGE('',*,*,#35864,.F.);
#47796=ORIENTED_EDGE('',*,*,#35859,.F.);
#47797=ORIENTED_EDGE('',*,*,#35864,.T.);
#47798=ORIENTED_EDGE('',*,*,#35865,.F.);
#47799=ORIENTED_EDGE('',*,*,#35581,.T.);
#47800=ORIENTED_EDGE('',*,*,#35860,.T.);
#47801=ORIENTED_EDGE('',*,*,#35866,.F.);
#47802=ORIENTED_EDGE('',*,*,#35867,.F.);
#47803=ORIENTED_EDGE('',*,*,#35671,.F.);
#47804=ORIENTED_EDGE('',*,*,#35868,.F.);
#47805=ORIENTED_EDGE('',*,*,#35868,.T.);
#47806=ORIENTED_EDGE('',*,*,#35673,.T.);
#47807=ORIENTED_EDGE('',*,*,#35583,.T.);
#47808=ORIENTED_EDGE('',*,*,#35869,.F.);
#47809=ORIENTED_EDGE('',*,*,#35584,.T.);
#47810=ORIENTED_EDGE('',*,*,#35870,.F.);
#47811=ORIENTED_EDGE('',*,*,#35871,.T.);
#47812=ORIENTED_EDGE('',*,*,#35872,.F.);
#47813=ORIENTED_EDGE('',*,*,#35586,.T.);
#47814=ORIENTED_EDGE('',*,*,#35873,.F.);
#47815=ORIENTED_EDGE('',*,*,#35874,.T.);
#47816=ORIENTED_EDGE('',*,*,#35875,.F.);
#47817=ORIENTED_EDGE('',*,*,#35876,.T.);
#47818=ORIENTED_EDGE('',*,*,#35877,.F.);
#47819=ORIENTED_EDGE('',*,*,#35587,.T.);
#47820=ORIENTED_EDGE('',*,*,#35875,.T.);
#47821=ORIENTED_EDGE('',*,*,#35878,.F.);
#47822=ORIENTED_EDGE('',*,*,#35879,.F.);
#47823=ORIENTED_EDGE('',*,*,#35876,.F.);
#47824=ORIENTED_EDGE('',*,*,#35874,.F.);
#47825=ORIENTED_EDGE('',*,*,#35589,.T.);
#47826=ORIENTED_EDGE('',*,*,#35880,.F.);
#47827=ORIENTED_EDGE('',*,*,#35881,.T.);
#47828=ORIENTED_EDGE('',*,*,#35882,.F.);
#47829=ORIENTED_EDGE('',*,*,#35590,.T.);
#47830=ORIENTED_EDGE('',*,*,#35882,.T.);
#47831=ORIENTED_EDGE('',*,*,#35883,.T.);
#47832=ORIENTED_EDGE('',*,*,#35884,.F.);
#47833=ORIENTED_EDGE('',*,*,#35883,.F.);
#47834=ORIENTED_EDGE('',*,*,#35881,.F.);
#47835=ORIENTED_EDGE('',*,*,#35885,.F.);
#47836=ORIENTED_EDGE('',*,*,#35886,.F.);
#47837=ORIENTED_EDGE('',*,*,#35592,.T.);
#47838=ORIENTED_EDGE('',*,*,#35887,.F.);
#47839=ORIENTED_EDGE('',*,*,#35888,.T.);
#47840=ORIENTED_EDGE('',*,*,#35889,.F.);
#47841=ORIENTED_EDGE('',*,*,#35593,.T.);
#47842=ORIENTED_EDGE('',*,*,#35889,.T.);
#47843=ORIENTED_EDGE('',*,*,#35890,.T.);
#47844=ORIENTED_EDGE('',*,*,#35891,.F.);
#47845=ORIENTED_EDGE('',*,*,#35890,.F.);
#47846=ORIENTED_EDGE('',*,*,#35888,.F.);
#47847=ORIENTED_EDGE('',*,*,#35892,.F.);
#47848=ORIENTED_EDGE('',*,*,#35893,.F.);
#47849=ORIENTED_EDGE('',*,*,#35595,.T.);
#47850=ORIENTED_EDGE('',*,*,#35894,.F.);
#47851=ORIENTED_EDGE('',*,*,#35895,.T.);
#47852=ORIENTED_EDGE('',*,*,#35896,.F.);
#47853=ORIENTED_EDGE('',*,*,#35596,.T.);
#47854=ORIENTED_EDGE('',*,*,#35896,.T.);
#47855=ORIENTED_EDGE('',*,*,#35897,.T.);
#47856=ORIENTED_EDGE('',*,*,#35898,.F.);
#47857=ORIENTED_EDGE('',*,*,#35897,.F.);
#47858=ORIENTED_EDGE('',*,*,#35895,.F.);
#47859=ORIENTED_EDGE('',*,*,#35899,.F.);
#47860=ORIENTED_EDGE('',*,*,#35900,.F.);
#47861=ORIENTED_EDGE('',*,*,#35598,.T.);
#47862=ORIENTED_EDGE('',*,*,#35901,.F.);
#47863=ORIENTED_EDGE('',*,*,#35902,.T.);
#47864=ORIENTED_EDGE('',*,*,#35903,.F.);
#47865=ORIENTED_EDGE('',*,*,#35599,.T.);
#47866=ORIENTED_EDGE('',*,*,#35903,.T.);
#47867=ORIENTED_EDGE('',*,*,#35904,.T.);
#47868=ORIENTED_EDGE('',*,*,#35905,.F.);
#47869=ORIENTED_EDGE('',*,*,#35904,.F.);
#47870=ORIENTED_EDGE('',*,*,#35902,.F.);
#47871=ORIENTED_EDGE('',*,*,#35906,.F.);
#47872=ORIENTED_EDGE('',*,*,#35907,.F.);
#47873=ORIENTED_EDGE('',*,*,#35601,.T.);
#47874=ORIENTED_EDGE('',*,*,#35908,.F.);
#47875=ORIENTED_EDGE('',*,*,#35909,.T.);
#47876=ORIENTED_EDGE('',*,*,#35910,.F.);
#47877=ORIENTED_EDGE('',*,*,#35602,.T.);
#47878=ORIENTED_EDGE('',*,*,#35910,.T.);
#47879=ORIENTED_EDGE('',*,*,#35911,.T.);
#47880=ORIENTED_EDGE('',*,*,#35912,.F.);
#47881=ORIENTED_EDGE('',*,*,#35911,.F.);
#47882=ORIENTED_EDGE('',*,*,#35909,.F.);
#47883=ORIENTED_EDGE('',*,*,#35913,.F.);
#47884=ORIENTED_EDGE('',*,*,#35914,.F.);
#47885=ORIENTED_EDGE('',*,*,#35604,.T.);
#47886=ORIENTED_EDGE('',*,*,#35915,.F.);
#47887=ORIENTED_EDGE('',*,*,#35916,.T.);
#47888=ORIENTED_EDGE('',*,*,#35917,.F.);
#47889=ORIENTED_EDGE('',*,*,#35605,.T.);
#47890=ORIENTED_EDGE('',*,*,#35917,.T.);
#47891=ORIENTED_EDGE('',*,*,#35918,.T.);
#47892=ORIENTED_EDGE('',*,*,#35919,.F.);
#47893=ORIENTED_EDGE('',*,*,#35918,.F.);
#47894=ORIENTED_EDGE('',*,*,#35916,.F.);
#47895=ORIENTED_EDGE('',*,*,#35920,.F.);
#47896=ORIENTED_EDGE('',*,*,#35921,.F.);
#47897=ORIENTED_EDGE('',*,*,#35607,.T.);
#47898=ORIENTED_EDGE('',*,*,#35922,.F.);
#47899=ORIENTED_EDGE('',*,*,#35923,.T.);
#47900=ORIENTED_EDGE('',*,*,#35924,.F.);
#47901=ORIENTED_EDGE('',*,*,#35608,.T.);
#47902=ORIENTED_EDGE('',*,*,#35924,.T.);
#47903=ORIENTED_EDGE('',*,*,#35925,.T.);
#47904=ORIENTED_EDGE('',*,*,#35926,.F.);
#47905=ORIENTED_EDGE('',*,*,#35925,.F.);
#47906=ORIENTED_EDGE('',*,*,#35923,.F.);
#47907=ORIENTED_EDGE('',*,*,#35927,.F.);
#47908=ORIENTED_EDGE('',*,*,#35928,.F.);
#47909=ORIENTED_EDGE('',*,*,#35610,.T.);
#47910=ORIENTED_EDGE('',*,*,#35929,.F.);
#47911=ORIENTED_EDGE('',*,*,#35930,.T.);
#47912=ORIENTED_EDGE('',*,*,#35931,.F.);
#47913=ORIENTED_EDGE('',*,*,#35611,.T.);
#47914=ORIENTED_EDGE('',*,*,#35931,.T.);
#47915=ORIENTED_EDGE('',*,*,#35932,.T.);
#47916=ORIENTED_EDGE('',*,*,#35933,.F.);
#47917=ORIENTED_EDGE('',*,*,#35932,.F.);
#47918=ORIENTED_EDGE('',*,*,#35930,.F.);
#47919=ORIENTED_EDGE('',*,*,#35934,.F.);
#47920=ORIENTED_EDGE('',*,*,#35935,.F.);
#47921=ORIENTED_EDGE('',*,*,#35613,.T.);
#47922=ORIENTED_EDGE('',*,*,#35936,.F.);
#47923=ORIENTED_EDGE('',*,*,#35937,.T.);
#47924=ORIENTED_EDGE('',*,*,#35938,.F.);
#47925=ORIENTED_EDGE('',*,*,#35614,.T.);
#47926=ORIENTED_EDGE('',*,*,#35938,.T.);
#47927=ORIENTED_EDGE('',*,*,#35939,.T.);
#47928=ORIENTED_EDGE('',*,*,#35940,.F.);
#47929=ORIENTED_EDGE('',*,*,#35939,.F.);
#47930=ORIENTED_EDGE('',*,*,#35937,.F.);
#47931=ORIENTED_EDGE('',*,*,#35941,.F.);
#47932=ORIENTED_EDGE('',*,*,#35942,.F.);
#47933=ORIENTED_EDGE('',*,*,#35616,.T.);
#47934=ORIENTED_EDGE('',*,*,#35943,.F.);
#47935=ORIENTED_EDGE('',*,*,#35944,.T.);
#47936=ORIENTED_EDGE('',*,*,#35945,.F.);
#47937=ORIENTED_EDGE('',*,*,#35617,.T.);
#47938=ORIENTED_EDGE('',*,*,#35945,.T.);
#47939=ORIENTED_EDGE('',*,*,#35946,.T.);
#47940=ORIENTED_EDGE('',*,*,#35947,.F.);
#47941=ORIENTED_EDGE('',*,*,#35946,.F.);
#47942=ORIENTED_EDGE('',*,*,#35944,.F.);
#47943=ORIENTED_EDGE('',*,*,#35948,.F.);
#47944=ORIENTED_EDGE('',*,*,#35949,.F.);
#47945=ORIENTED_EDGE('',*,*,#35619,.T.);
#47946=ORIENTED_EDGE('',*,*,#35950,.F.);
#47947=ORIENTED_EDGE('',*,*,#35951,.T.);
#47948=ORIENTED_EDGE('',*,*,#35952,.F.);
#47949=ORIENTED_EDGE('',*,*,#35620,.T.);
#47950=ORIENTED_EDGE('',*,*,#35952,.T.);
#47951=ORIENTED_EDGE('',*,*,#35953,.T.);
#47952=ORIENTED_EDGE('',*,*,#35954,.F.);
#47953=ORIENTED_EDGE('',*,*,#35953,.F.);
#47954=ORIENTED_EDGE('',*,*,#35951,.F.);
#47955=ORIENTED_EDGE('',*,*,#35955,.F.);
#47956=ORIENTED_EDGE('',*,*,#35956,.F.);
#47957=ORIENTED_EDGE('',*,*,#35622,.T.);
#47958=ORIENTED_EDGE('',*,*,#35957,.F.);
#47959=ORIENTED_EDGE('',*,*,#35958,.T.);
#47960=ORIENTED_EDGE('',*,*,#35959,.F.);
#47961=ORIENTED_EDGE('',*,*,#35623,.T.);
#47962=ORIENTED_EDGE('',*,*,#35959,.T.);
#47963=ORIENTED_EDGE('',*,*,#35960,.T.);
#47964=ORIENTED_EDGE('',*,*,#35961,.F.);
#47965=ORIENTED_EDGE('',*,*,#35960,.F.);
#47966=ORIENTED_EDGE('',*,*,#35958,.F.);
#47967=ORIENTED_EDGE('',*,*,#35962,.F.);
#47968=ORIENTED_EDGE('',*,*,#35963,.F.);
#47969=ORIENTED_EDGE('',*,*,#35625,.T.);
#47970=ORIENTED_EDGE('',*,*,#35964,.F.);
#47971=ORIENTED_EDGE('',*,*,#34447,.T.);
#47972=ORIENTED_EDGE('',*,*,#35965,.F.);
#47973=ORIENTED_EDGE('',*,*,#35626,.T.);
#47974=ORIENTED_EDGE('',*,*,#35965,.T.);
#47975=ORIENTED_EDGE('',*,*,#34446,.T.);
#47976=ORIENTED_EDGE('',*,*,#35966,.F.);
#47977=ORIENTED_EDGE('',*,*,#35628,.T.);
#47978=ORIENTED_EDGE('',*,*,#35967,.F.);
#47979=ORIENTED_EDGE('',*,*,#35968,.T.);
#47980=ORIENTED_EDGE('',*,*,#35969,.F.);
#47981=ORIENTED_EDGE('',*,*,#35629,.T.);
#47982=ORIENTED_EDGE('',*,*,#35969,.T.);
#47983=ORIENTED_EDGE('',*,*,#35970,.T.);
#47984=ORIENTED_EDGE('',*,*,#35971,.F.);
#47985=ORIENTED_EDGE('',*,*,#35970,.F.);
#47986=ORIENTED_EDGE('',*,*,#35968,.F.);
#47987=ORIENTED_EDGE('',*,*,#35972,.F.);
#47988=ORIENTED_EDGE('',*,*,#35973,.F.);
#47989=ORIENTED_EDGE('',*,*,#35631,.T.);
#47990=ORIENTED_EDGE('',*,*,#35974,.F.);
#47991=ORIENTED_EDGE('',*,*,#35975,.T.);
#47992=ORIENTED_EDGE('',*,*,#35976,.F.);
#47993=ORIENTED_EDGE('',*,*,#35632,.T.);
#47994=ORIENTED_EDGE('',*,*,#35976,.T.);
#47995=ORIENTED_EDGE('',*,*,#35977,.T.);
#47996=ORIENTED_EDGE('',*,*,#35978,.F.);
#47997=ORIENTED_EDGE('',*,*,#35977,.F.);
#47998=ORIENTED_EDGE('',*,*,#35975,.F.);
#47999=ORIENTED_EDGE('',*,*,#35979,.F.);
#48000=ORIENTED_EDGE('',*,*,#35980,.F.);
#48001=ORIENTED_EDGE('',*,*,#35634,.T.);
#48002=ORIENTED_EDGE('',*,*,#35981,.F.);
#48003=ORIENTED_EDGE('',*,*,#35982,.T.);
#48004=ORIENTED_EDGE('',*,*,#35983,.F.);
#48005=ORIENTED_EDGE('',*,*,#35635,.T.);
#48006=ORIENTED_EDGE('',*,*,#35983,.T.);
#48007=ORIENTED_EDGE('',*,*,#35984,.T.);
#48008=ORIENTED_EDGE('',*,*,#35985,.F.);
#48009=ORIENTED_EDGE('',*,*,#35984,.F.);
#48010=ORIENTED_EDGE('',*,*,#35982,.F.);
#48011=ORIENTED_EDGE('',*,*,#35986,.F.);
#48012=ORIENTED_EDGE('',*,*,#35987,.F.);
#48013=ORIENTED_EDGE('',*,*,#35637,.T.);
#48014=ORIENTED_EDGE('',*,*,#35988,.F.);
#48015=ORIENTED_EDGE('',*,*,#35989,.T.);
#48016=ORIENTED_EDGE('',*,*,#35990,.F.);
#48017=ORIENTED_EDGE('',*,*,#35638,.T.);
#48018=ORIENTED_EDGE('',*,*,#35990,.T.);
#48019=ORIENTED_EDGE('',*,*,#35991,.T.);
#48020=ORIENTED_EDGE('',*,*,#35992,.F.);
#48021=ORIENTED_EDGE('',*,*,#35991,.F.);
#48022=ORIENTED_EDGE('',*,*,#35989,.F.);
#48023=ORIENTED_EDGE('',*,*,#35993,.F.);
#48024=ORIENTED_EDGE('',*,*,#35994,.F.);
#48025=ORIENTED_EDGE('',*,*,#35640,.T.);
#48026=ORIENTED_EDGE('',*,*,#35995,.F.);
#48027=ORIENTED_EDGE('',*,*,#35996,.T.);
#48028=ORIENTED_EDGE('',*,*,#35997,.F.);
#48029=ORIENTED_EDGE('',*,*,#35641,.T.);
#48030=ORIENTED_EDGE('',*,*,#35997,.T.);
#48031=ORIENTED_EDGE('',*,*,#35998,.T.);
#48032=ORIENTED_EDGE('',*,*,#35999,.F.);
#48033=ORIENTED_EDGE('',*,*,#35998,.F.);
#48034=ORIENTED_EDGE('',*,*,#35996,.F.);
#48035=ORIENTED_EDGE('',*,*,#36000,.F.);
#48036=ORIENTED_EDGE('',*,*,#36001,.F.);
#48037=ORIENTED_EDGE('',*,*,#35643,.T.);
#48038=ORIENTED_EDGE('',*,*,#36002,.F.);
#48039=ORIENTED_EDGE('',*,*,#36003,.T.);
#48040=ORIENTED_EDGE('',*,*,#36004,.F.);
#48041=ORIENTED_EDGE('',*,*,#35644,.T.);
#48042=ORIENTED_EDGE('',*,*,#36004,.T.);
#48043=ORIENTED_EDGE('',*,*,#36005,.T.);
#48044=ORIENTED_EDGE('',*,*,#36006,.F.);
#48045=ORIENTED_EDGE('',*,*,#36005,.F.);
#48046=ORIENTED_EDGE('',*,*,#36003,.F.);
#48047=ORIENTED_EDGE('',*,*,#36007,.F.);
#48048=ORIENTED_EDGE('',*,*,#36008,.F.);
#48049=ORIENTED_EDGE('',*,*,#35646,.T.);
#48050=ORIENTED_EDGE('',*,*,#36009,.F.);
#48051=ORIENTED_EDGE('',*,*,#36010,.T.);
#48052=ORIENTED_EDGE('',*,*,#36011,.F.);
#48053=ORIENTED_EDGE('',*,*,#35647,.T.);
#48054=ORIENTED_EDGE('',*,*,#36011,.T.);
#48055=ORIENTED_EDGE('',*,*,#36012,.T.);
#48056=ORIENTED_EDGE('',*,*,#36013,.F.);
#48057=ORIENTED_EDGE('',*,*,#36012,.F.);
#48058=ORIENTED_EDGE('',*,*,#36010,.F.);
#48059=ORIENTED_EDGE('',*,*,#36014,.F.);
#48060=ORIENTED_EDGE('',*,*,#36015,.F.);
#48061=ORIENTED_EDGE('',*,*,#35649,.T.);
#48062=ORIENTED_EDGE('',*,*,#36016,.F.);
#48063=ORIENTED_EDGE('',*,*,#36017,.T.);
#48064=ORIENTED_EDGE('',*,*,#36018,.F.);
#48065=ORIENTED_EDGE('',*,*,#35650,.T.);
#48066=ORIENTED_EDGE('',*,*,#36018,.T.);
#48067=ORIENTED_EDGE('',*,*,#36019,.T.);
#48068=ORIENTED_EDGE('',*,*,#36020,.F.);
#48069=ORIENTED_EDGE('',*,*,#36019,.F.);
#48070=ORIENTED_EDGE('',*,*,#36017,.F.);
#48071=ORIENTED_EDGE('',*,*,#36021,.F.);
#48072=ORIENTED_EDGE('',*,*,#36022,.F.);
#48073=ORIENTED_EDGE('',*,*,#35652,.T.);
#48074=ORIENTED_EDGE('',*,*,#36023,.F.);
#48075=ORIENTED_EDGE('',*,*,#36024,.T.);
#48076=ORIENTED_EDGE('',*,*,#36025,.F.);
#48077=ORIENTED_EDGE('',*,*,#35653,.T.);
#48078=ORIENTED_EDGE('',*,*,#36025,.T.);
#48079=ORIENTED_EDGE('',*,*,#36026,.T.);
#48080=ORIENTED_EDGE('',*,*,#36027,.F.);
#48081=ORIENTED_EDGE('',*,*,#36026,.F.);
#48082=ORIENTED_EDGE('',*,*,#36024,.F.);
#48083=ORIENTED_EDGE('',*,*,#36028,.F.);
#48084=ORIENTED_EDGE('',*,*,#36029,.F.);
#48085=ORIENTED_EDGE('',*,*,#35655,.T.);
#48086=ORIENTED_EDGE('',*,*,#36030,.F.);
#48087=ORIENTED_EDGE('',*,*,#36031,.T.);
#48088=ORIENTED_EDGE('',*,*,#36032,.F.);
#48089=ORIENTED_EDGE('',*,*,#35656,.T.);
#48090=ORIENTED_EDGE('',*,*,#36032,.T.);
#48091=ORIENTED_EDGE('',*,*,#36033,.T.);
#48092=ORIENTED_EDGE('',*,*,#36034,.F.);
#48093=ORIENTED_EDGE('',*,*,#36033,.F.);
#48094=ORIENTED_EDGE('',*,*,#36031,.F.);
#48095=ORIENTED_EDGE('',*,*,#36035,.F.);
#48096=ORIENTED_EDGE('',*,*,#36036,.F.);
#48097=ORIENTED_EDGE('',*,*,#35658,.T.);
#48098=ORIENTED_EDGE('',*,*,#36037,.F.);
#48099=ORIENTED_EDGE('',*,*,#36038,.T.);
#48100=ORIENTED_EDGE('',*,*,#36039,.F.);
#48101=ORIENTED_EDGE('',*,*,#35659,.T.);
#48102=ORIENTED_EDGE('',*,*,#36039,.T.);
#48103=ORIENTED_EDGE('',*,*,#36040,.T.);
#48104=ORIENTED_EDGE('',*,*,#36041,.F.);
#48105=ORIENTED_EDGE('',*,*,#36040,.F.);
#48106=ORIENTED_EDGE('',*,*,#36038,.F.);
#48107=ORIENTED_EDGE('',*,*,#36042,.F.);
#48108=ORIENTED_EDGE('',*,*,#36043,.F.);
#48109=ORIENTED_EDGE('',*,*,#35661,.T.);
#48110=ORIENTED_EDGE('',*,*,#36044,.F.);
#48111=ORIENTED_EDGE('',*,*,#36045,.T.);
#48112=ORIENTED_EDGE('',*,*,#36046,.F.);
#48113=ORIENTED_EDGE('',*,*,#35662,.T.);
#48114=ORIENTED_EDGE('',*,*,#36046,.T.);
#48115=ORIENTED_EDGE('',*,*,#36047,.T.);
#48116=ORIENTED_EDGE('',*,*,#36048,.F.);
#48117=ORIENTED_EDGE('',*,*,#36047,.F.);
#48118=ORIENTED_EDGE('',*,*,#36045,.F.);
#48119=ORIENTED_EDGE('',*,*,#36049,.F.);
#48120=ORIENTED_EDGE('',*,*,#36050,.F.);
#48121=ORIENTED_EDGE('',*,*,#35664,.T.);
#48122=ORIENTED_EDGE('',*,*,#36051,.F.);
#48123=ORIENTED_EDGE('',*,*,#36052,.T.);
#48124=ORIENTED_EDGE('',*,*,#36053,.F.);
#48125=ORIENTED_EDGE('',*,*,#35665,.T.);
#48126=ORIENTED_EDGE('',*,*,#36053,.T.);
#48127=ORIENTED_EDGE('',*,*,#36054,.T.);
#48128=ORIENTED_EDGE('',*,*,#36055,.F.);
#48129=ORIENTED_EDGE('',*,*,#36054,.F.);
#48130=ORIENTED_EDGE('',*,*,#36052,.F.);
#48131=ORIENTED_EDGE('',*,*,#36056,.F.);
#48132=ORIENTED_EDGE('',*,*,#36057,.F.);
#48133=ORIENTED_EDGE('',*,*,#35667,.T.);
#48134=ORIENTED_EDGE('',*,*,#36058,.F.);
#48135=ORIENTED_EDGE('',*,*,#36059,.T.);
#48136=ORIENTED_EDGE('',*,*,#36060,.F.);
#48137=ORIENTED_EDGE('',*,*,#35668,.T.);
#48138=ORIENTED_EDGE('',*,*,#36060,.T.);
#48139=ORIENTED_EDGE('',*,*,#36061,.T.);
#48140=ORIENTED_EDGE('',*,*,#36062,.F.);
#48141=ORIENTED_EDGE('',*,*,#36061,.F.);
#48142=ORIENTED_EDGE('',*,*,#36059,.F.);
#48143=ORIENTED_EDGE('',*,*,#36063,.F.);
#48144=ORIENTED_EDGE('',*,*,#36064,.F.);
#48145=ORIENTED_EDGE('',*,*,#35871,.F.);
#48146=ORIENTED_EDGE('',*,*,#36065,.F.);
#48147=ORIENTED_EDGE('',*,*,#36066,.F.);
#48148=ORIENTED_EDGE('',*,*,#36067,.F.);
#48149=ORIENTED_EDGE('',*,*,#35670,.T.);
#48150=ORIENTED_EDGE('',*,*,#36068,.F.);
#48151=ORIENTED_EDGE('',*,*,#36065,.T.);
#48152=ORIENTED_EDGE('',*,*,#35870,.T.);
#48153=ORIENTED_EDGE('',*,*,#36069,.F.);
#48154=ORIENTED_EDGE('',*,*,#35672,.T.);
#48155=ORIENTED_EDGE('',*,*,#35867,.T.);
#48156=ORIENTED_EDGE('',*,*,#36070,.F.);
#48157=ORIENTED_EDGE('',*,*,#36071,.F.);
#48158=ORIENTED_EDGE('',*,*,#36072,.F.);
#48159=ORIENTED_EDGE('',*,*,#35677,.T.);
#48160=ORIENTED_EDGE('',*,*,#35676,.T.);
#48161=ORIENTED_EDGE('',*,*,#36073,.F.);
#48162=ORIENTED_EDGE('',*,*,#35680,.T.);
#48163=ORIENTED_EDGE('',*,*,#35678,.T.);
#48164=ORIENTED_EDGE('',*,*,#36072,.T.);
#48165=ORIENTED_EDGE('',*,*,#36074,.F.);
#48166=ORIENTED_EDGE('',*,*,#36075,.F.);
#48167=ORIENTED_EDGE('',*,*,#35684,.T.);
#48168=ORIENTED_EDGE('',*,*,#35683,.T.);
#48169=ORIENTED_EDGE('',*,*,#36076,.F.);
#48170=ORIENTED_EDGE('',*,*,#35687,.T.);
#48171=ORIENTED_EDGE('',*,*,#35685,.T.);
#48172=ORIENTED_EDGE('',*,*,#36075,.T.);
#48173=ORIENTED_EDGE('',*,*,#36077,.F.);
#48174=ORIENTED_EDGE('',*,*,#36078,.F.);
#48175=ORIENTED_EDGE('',*,*,#35691,.T.);
#48176=ORIENTED_EDGE('',*,*,#35690,.T.);
#48177=ORIENTED_EDGE('',*,*,#36079,.F.);
#48178=ORIENTED_EDGE('',*,*,#35694,.T.);
#48179=ORIENTED_EDGE('',*,*,#35692,.T.);
#48180=ORIENTED_EDGE('',*,*,#36078,.T.);
#48181=ORIENTED_EDGE('',*,*,#36080,.F.);
#48182=ORIENTED_EDGE('',*,*,#36081,.F.);
#48183=ORIENTED_EDGE('',*,*,#35698,.T.);
#48184=ORIENTED_EDGE('',*,*,#35697,.T.);
#48185=ORIENTED_EDGE('',*,*,#36082,.F.);
#48186=ORIENTED_EDGE('',*,*,#35701,.T.);
#48187=ORIENTED_EDGE('',*,*,#35699,.T.);
#48188=ORIENTED_EDGE('',*,*,#36081,.T.);
#48189=ORIENTED_EDGE('',*,*,#36083,.F.);
#48190=ORIENTED_EDGE('',*,*,#36084,.F.);
#48191=ORIENTED_EDGE('',*,*,#35705,.T.);
#48192=ORIENTED_EDGE('',*,*,#35704,.T.);
#48193=ORIENTED_EDGE('',*,*,#36085,.F.);
#48194=ORIENTED_EDGE('',*,*,#35708,.T.);
#48195=ORIENTED_EDGE('',*,*,#35706,.T.);
#48196=ORIENTED_EDGE('',*,*,#36084,.T.);
#48197=ORIENTED_EDGE('',*,*,#36086,.F.);
#48198=ORIENTED_EDGE('',*,*,#36087,.F.);
#48199=ORIENTED_EDGE('',*,*,#35712,.T.);
#48200=ORIENTED_EDGE('',*,*,#35711,.T.);
#48201=ORIENTED_EDGE('',*,*,#36088,.F.);
#48202=ORIENTED_EDGE('',*,*,#35715,.T.);
#48203=ORIENTED_EDGE('',*,*,#35713,.T.);
#48204=ORIENTED_EDGE('',*,*,#36087,.T.);
#48205=ORIENTED_EDGE('',*,*,#36089,.F.);
#48206=ORIENTED_EDGE('',*,*,#36090,.F.);
#48207=ORIENTED_EDGE('',*,*,#34451,.T.);
#48208=ORIENTED_EDGE('',*,*,#35717,.T.);
#48209=ORIENTED_EDGE('',*,*,#36091,.F.);
#48210=ORIENTED_EDGE('',*,*,#35718,.T.);
#48211=ORIENTED_EDGE('',*,*,#34452,.T.);
#48212=ORIENTED_EDGE('',*,*,#36090,.T.);
#48213=ORIENTED_EDGE('',*,*,#36092,.F.);
#48214=ORIENTED_EDGE('',*,*,#36093,.F.);
#48215=ORIENTED_EDGE('',*,*,#35722,.T.);
#48216=ORIENTED_EDGE('',*,*,#35721,.T.);
#48217=ORIENTED_EDGE('',*,*,#36094,.F.);
#48218=ORIENTED_EDGE('',*,*,#35725,.T.);
#48219=ORIENTED_EDGE('',*,*,#35723,.T.);
#48220=ORIENTED_EDGE('',*,*,#36093,.T.);
#48221=ORIENTED_EDGE('',*,*,#36095,.F.);
#48222=ORIENTED_EDGE('',*,*,#36096,.F.);
#48223=ORIENTED_EDGE('',*,*,#35729,.T.);
#48224=ORIENTED_EDGE('',*,*,#35728,.T.);
#48225=ORIENTED_EDGE('',*,*,#36097,.F.);
#48226=ORIENTED_EDGE('',*,*,#35732,.T.);
#48227=ORIENTED_EDGE('',*,*,#35730,.T.);
#48228=ORIENTED_EDGE('',*,*,#36096,.T.);
#48229=ORIENTED_EDGE('',*,*,#36098,.F.);
#48230=ORIENTED_EDGE('',*,*,#36099,.F.);
#48231=ORIENTED_EDGE('',*,*,#35736,.T.);
#48232=ORIENTED_EDGE('',*,*,#35735,.T.);
#48233=ORIENTED_EDGE('',*,*,#36100,.F.);
#48234=ORIENTED_EDGE('',*,*,#35739,.T.);
#48235=ORIENTED_EDGE('',*,*,#35737,.T.);
#48236=ORIENTED_EDGE('',*,*,#36099,.T.);
#48237=ORIENTED_EDGE('',*,*,#36101,.F.);
#48238=ORIENTED_EDGE('',*,*,#36102,.F.);
#48239=ORIENTED_EDGE('',*,*,#35743,.T.);
#48240=ORIENTED_EDGE('',*,*,#35742,.T.);
#48241=ORIENTED_EDGE('',*,*,#36103,.F.);
#48242=ORIENTED_EDGE('',*,*,#35746,.T.);
#48243=ORIENTED_EDGE('',*,*,#35744,.T.);
#48244=ORIENTED_EDGE('',*,*,#36102,.T.);
#48245=ORIENTED_EDGE('',*,*,#36104,.F.);
#48246=ORIENTED_EDGE('',*,*,#36105,.F.);
#48247=ORIENTED_EDGE('',*,*,#35750,.T.);
#48248=ORIENTED_EDGE('',*,*,#35749,.T.);
#48249=ORIENTED_EDGE('',*,*,#36106,.F.);
#48250=ORIENTED_EDGE('',*,*,#35753,.T.);
#48251=ORIENTED_EDGE('',*,*,#35751,.T.);
#48252=ORIENTED_EDGE('',*,*,#36105,.T.);
#48253=ORIENTED_EDGE('',*,*,#36107,.F.);
#48254=ORIENTED_EDGE('',*,*,#36108,.F.);
#48255=ORIENTED_EDGE('',*,*,#35757,.T.);
#48256=ORIENTED_EDGE('',*,*,#35756,.T.);
#48257=ORIENTED_EDGE('',*,*,#36109,.F.);
#48258=ORIENTED_EDGE('',*,*,#35760,.T.);
#48259=ORIENTED_EDGE('',*,*,#35758,.T.);
#48260=ORIENTED_EDGE('',*,*,#36108,.T.);
#48261=ORIENTED_EDGE('',*,*,#36110,.F.);
#48262=ORIENTED_EDGE('',*,*,#36111,.F.);
#48263=ORIENTED_EDGE('',*,*,#35764,.T.);
#48264=ORIENTED_EDGE('',*,*,#35763,.T.);
#48265=ORIENTED_EDGE('',*,*,#36112,.F.);
#48266=ORIENTED_EDGE('',*,*,#35767,.T.);
#48267=ORIENTED_EDGE('',*,*,#35765,.T.);
#48268=ORIENTED_EDGE('',*,*,#36111,.T.);
#48269=ORIENTED_EDGE('',*,*,#36113,.F.);
#48270=ORIENTED_EDGE('',*,*,#36114,.F.);
#48271=ORIENTED_EDGE('',*,*,#35771,.T.);
#48272=ORIENTED_EDGE('',*,*,#35770,.T.);
#48273=ORIENTED_EDGE('',*,*,#36115,.F.);
#48274=ORIENTED_EDGE('',*,*,#35774,.T.);
#48275=ORIENTED_EDGE('',*,*,#35772,.T.);
#48276=ORIENTED_EDGE('',*,*,#36114,.T.);
#48277=ORIENTED_EDGE('',*,*,#36116,.F.);
#48278=ORIENTED_EDGE('',*,*,#36117,.F.);
#48279=ORIENTED_EDGE('',*,*,#35778,.T.);
#48280=ORIENTED_EDGE('',*,*,#35777,.T.);
#48281=ORIENTED_EDGE('',*,*,#36118,.F.);
#48282=ORIENTED_EDGE('',*,*,#35781,.T.);
#48283=ORIENTED_EDGE('',*,*,#35779,.T.);
#48284=ORIENTED_EDGE('',*,*,#36117,.T.);
#48285=ORIENTED_EDGE('',*,*,#36119,.F.);
#48286=ORIENTED_EDGE('',*,*,#36120,.F.);
#48287=ORIENTED_EDGE('',*,*,#35785,.T.);
#48288=ORIENTED_EDGE('',*,*,#35784,.T.);
#48289=ORIENTED_EDGE('',*,*,#36121,.F.);
#48290=ORIENTED_EDGE('',*,*,#35788,.T.);
#48291=ORIENTED_EDGE('',*,*,#35786,.T.);
#48292=ORIENTED_EDGE('',*,*,#36120,.T.);
#48293=ORIENTED_EDGE('',*,*,#36122,.F.);
#48294=ORIENTED_EDGE('',*,*,#36123,.F.);
#48295=ORIENTED_EDGE('',*,*,#35792,.T.);
#48296=ORIENTED_EDGE('',*,*,#35791,.T.);
#48297=ORIENTED_EDGE('',*,*,#36124,.F.);
#48298=ORIENTED_EDGE('',*,*,#35795,.T.);
#48299=ORIENTED_EDGE('',*,*,#35793,.T.);
#48300=ORIENTED_EDGE('',*,*,#36123,.T.);
#48301=ORIENTED_EDGE('',*,*,#36125,.F.);
#48302=ORIENTED_EDGE('',*,*,#36126,.F.);
#48303=ORIENTED_EDGE('',*,*,#35799,.T.);
#48304=ORIENTED_EDGE('',*,*,#35798,.T.);
#48305=ORIENTED_EDGE('',*,*,#36127,.F.);
#48306=ORIENTED_EDGE('',*,*,#35802,.T.);
#48307=ORIENTED_EDGE('',*,*,#35800,.T.);
#48308=ORIENTED_EDGE('',*,*,#36126,.T.);
#48309=ORIENTED_EDGE('',*,*,#36128,.F.);
#48310=ORIENTED_EDGE('',*,*,#36129,.F.);
#48311=ORIENTED_EDGE('',*,*,#35806,.T.);
#48312=ORIENTED_EDGE('',*,*,#35805,.T.);
#48313=ORIENTED_EDGE('',*,*,#36130,.F.);
#48314=ORIENTED_EDGE('',*,*,#35809,.T.);
#48315=ORIENTED_EDGE('',*,*,#35807,.T.);
#48316=ORIENTED_EDGE('',*,*,#36129,.T.);
#48317=ORIENTED_EDGE('',*,*,#36131,.F.);
#48318=ORIENTED_EDGE('',*,*,#36132,.F.);
#48319=ORIENTED_EDGE('',*,*,#35813,.T.);
#48320=ORIENTED_EDGE('',*,*,#35812,.T.);
#48321=ORIENTED_EDGE('',*,*,#36133,.F.);
#48322=ORIENTED_EDGE('',*,*,#35816,.T.);
#48323=ORIENTED_EDGE('',*,*,#35814,.T.);
#48324=ORIENTED_EDGE('',*,*,#36132,.T.);
#48325=ORIENTED_EDGE('',*,*,#36134,.F.);
#48326=ORIENTED_EDGE('',*,*,#36135,.F.);
#48327=ORIENTED_EDGE('',*,*,#35820,.T.);
#48328=ORIENTED_EDGE('',*,*,#35819,.T.);
#48329=ORIENTED_EDGE('',*,*,#36136,.F.);
#48330=ORIENTED_EDGE('',*,*,#35823,.T.);
#48331=ORIENTED_EDGE('',*,*,#35821,.T.);
#48332=ORIENTED_EDGE('',*,*,#36135,.T.);
#48333=ORIENTED_EDGE('',*,*,#36137,.F.);
#48334=ORIENTED_EDGE('',*,*,#36138,.F.);
#48335=ORIENTED_EDGE('',*,*,#35827,.T.);
#48336=ORIENTED_EDGE('',*,*,#35826,.T.);
#48337=ORIENTED_EDGE('',*,*,#36139,.F.);
#48338=ORIENTED_EDGE('',*,*,#35830,.T.);
#48339=ORIENTED_EDGE('',*,*,#35828,.T.);
#48340=ORIENTED_EDGE('',*,*,#36138,.T.);
#48341=ORIENTED_EDGE('',*,*,#36140,.F.);
#48342=ORIENTED_EDGE('',*,*,#36141,.F.);
#48343=ORIENTED_EDGE('',*,*,#35836,.T.);
#48344=ORIENTED_EDGE('',*,*,#35833,.T.);
#48345=ORIENTED_EDGE('',*,*,#35837,.T.);
#48346=ORIENTED_EDGE('',*,*,#36141,.T.);
#48347=ORIENTED_EDGE('',*,*,#36142,.F.);
#48348=ORIENTED_EDGE('',*,*,#35835,.T.);
#48349=ORIENTED_EDGE('',*,*,#35842,.T.);
#48350=ORIENTED_EDGE('',*,*,#35838,.T.);
#48351=ORIENTED_EDGE('',*,*,#36143,.F.);
#48352=ORIENTED_EDGE('',*,*,#36144,.F.);
#48353=ORIENTED_EDGE('',*,*,#36145,.F.);
#48354=ORIENTED_EDGE('',*,*,#35844,.T.);
#48355=ORIENTED_EDGE('',*,*,#35843,.T.);
#48356=ORIENTED_EDGE('',*,*,#36144,.T.);
#48357=ORIENTED_EDGE('',*,*,#36146,.F.);
#48358=ORIENTED_EDGE('',*,*,#36147,.F.);
#48359=ORIENTED_EDGE('',*,*,#35848,.T.);
#48360=ORIENTED_EDGE('',*,*,#35847,.T.);
#48361=ORIENTED_EDGE('',*,*,#36148,.F.);
#48362=ORIENTED_EDGE('',*,*,#35851,.T.);
#48363=ORIENTED_EDGE('',*,*,#35849,.T.);
#48364=ORIENTED_EDGE('',*,*,#36147,.T.);
#48365=ORIENTED_EDGE('',*,*,#36149,.F.);
#48366=ORIENTED_EDGE('',*,*,#36150,.F.);
#48367=ORIENTED_EDGE('',*,*,#35855,.T.);
#48368=ORIENTED_EDGE('',*,*,#35854,.T.);
#48369=ORIENTED_EDGE('',*,*,#36151,.F.);
#48370=ORIENTED_EDGE('',*,*,#35858,.T.);
#48371=ORIENTED_EDGE('',*,*,#35856,.T.);
#48372=ORIENTED_EDGE('',*,*,#36150,.T.);
#48373=ORIENTED_EDGE('',*,*,#36152,.F.);
#48374=ORIENTED_EDGE('',*,*,#36153,.F.);
#48375=ORIENTED_EDGE('',*,*,#35862,.T.);
#48376=ORIENTED_EDGE('',*,*,#35861,.T.);
#48377=ORIENTED_EDGE('',*,*,#36154,.F.);
#48378=ORIENTED_EDGE('',*,*,#35865,.T.);
#48379=ORIENTED_EDGE('',*,*,#35863,.T.);
#48380=ORIENTED_EDGE('',*,*,#36153,.T.);
#48381=ORIENTED_EDGE('',*,*,#36155,.F.);
#48382=ORIENTED_EDGE('',*,*,#36070,.T.);
#48383=ORIENTED_EDGE('',*,*,#35866,.T.);
#48384=ORIENTED_EDGE('',*,*,#35869,.T.);
#48385=ORIENTED_EDGE('',*,*,#36067,.T.);
#48386=ORIENTED_EDGE('',*,*,#36156,.F.);
#48387=ORIENTED_EDGE('',*,*,#36157,.F.);
#48388=ORIENTED_EDGE('',*,*,#35872,.T.);
#48389=ORIENTED_EDGE('',*,*,#36158,.F.);
#48390=ORIENTED_EDGE('',*,*,#36159,.F.);
#48391=ORIENTED_EDGE('',*,*,#35878,.T.);
#48392=ORIENTED_EDGE('',*,*,#35873,.T.);
#48393=ORIENTED_EDGE('',*,*,#35879,.T.);
#48394=ORIENTED_EDGE('',*,*,#36159,.T.);
#48395=ORIENTED_EDGE('',*,*,#36160,.F.);
#48396=ORIENTED_EDGE('',*,*,#35877,.T.);
#48397=ORIENTED_EDGE('',*,*,#35885,.T.);
#48398=ORIENTED_EDGE('',*,*,#35880,.T.);
#48399=ORIENTED_EDGE('',*,*,#36161,.F.);
#48400=ORIENTED_EDGE('',*,*,#36162,.F.);
#48401=ORIENTED_EDGE('',*,*,#35886,.T.);
#48402=ORIENTED_EDGE('',*,*,#36162,.T.);
#48403=ORIENTED_EDGE('',*,*,#36163,.F.);
#48404=ORIENTED_EDGE('',*,*,#35884,.T.);
#48405=ORIENTED_EDGE('',*,*,#35892,.T.);
#48406=ORIENTED_EDGE('',*,*,#35887,.T.);
#48407=ORIENTED_EDGE('',*,*,#36164,.F.);
#48408=ORIENTED_EDGE('',*,*,#36165,.F.);
#48409=ORIENTED_EDGE('',*,*,#35893,.T.);
#48410=ORIENTED_EDGE('',*,*,#36165,.T.);
#48411=ORIENTED_EDGE('',*,*,#36166,.F.);
#48412=ORIENTED_EDGE('',*,*,#35891,.T.);
#48413=ORIENTED_EDGE('',*,*,#35899,.T.);
#48414=ORIENTED_EDGE('',*,*,#35894,.T.);
#48415=ORIENTED_EDGE('',*,*,#36167,.F.);
#48416=ORIENTED_EDGE('',*,*,#36168,.F.);
#48417=ORIENTED_EDGE('',*,*,#35900,.T.);
#48418=ORIENTED_EDGE('',*,*,#36168,.T.);
#48419=ORIENTED_EDGE('',*,*,#36169,.F.);
#48420=ORIENTED_EDGE('',*,*,#35898,.T.);
#48421=ORIENTED_EDGE('',*,*,#35906,.T.);
#48422=ORIENTED_EDGE('',*,*,#35901,.T.);
#48423=ORIENTED_EDGE('',*,*,#36170,.F.);
#48424=ORIENTED_EDGE('',*,*,#36171,.F.);
#48425=ORIENTED_EDGE('',*,*,#35907,.T.);
#48426=ORIENTED_EDGE('',*,*,#36171,.T.);
#48427=ORIENTED_EDGE('',*,*,#36172,.F.);
#48428=ORIENTED_EDGE('',*,*,#35905,.T.);
#48429=ORIENTED_EDGE('',*,*,#35913,.T.);
#48430=ORIENTED_EDGE('',*,*,#35908,.T.);
#48431=ORIENTED_EDGE('',*,*,#36173,.F.);
#48432=ORIENTED_EDGE('',*,*,#36174,.F.);
#48433=ORIENTED_EDGE('',*,*,#35914,.T.);
#48434=ORIENTED_EDGE('',*,*,#36174,.T.);
#48435=ORIENTED_EDGE('',*,*,#36175,.F.);
#48436=ORIENTED_EDGE('',*,*,#35912,.T.);
#48437=ORIENTED_EDGE('',*,*,#35920,.T.);
#48438=ORIENTED_EDGE('',*,*,#35915,.T.);
#48439=ORIENTED_EDGE('',*,*,#36176,.F.);
#48440=ORIENTED_EDGE('',*,*,#36177,.F.);
#48441=ORIENTED_EDGE('',*,*,#35921,.T.);
#48442=ORIENTED_EDGE('',*,*,#36177,.T.);
#48443=ORIENTED_EDGE('',*,*,#36178,.F.);
#48444=ORIENTED_EDGE('',*,*,#35919,.T.);
#48445=ORIENTED_EDGE('',*,*,#35927,.T.);
#48446=ORIENTED_EDGE('',*,*,#35922,.T.);
#48447=ORIENTED_EDGE('',*,*,#36179,.F.);
#48448=ORIENTED_EDGE('',*,*,#36180,.F.);
#48449=ORIENTED_EDGE('',*,*,#35928,.T.);
#48450=ORIENTED_EDGE('',*,*,#36180,.T.);
#48451=ORIENTED_EDGE('',*,*,#36181,.F.);
#48452=ORIENTED_EDGE('',*,*,#35926,.T.);
#48453=ORIENTED_EDGE('',*,*,#35934,.T.);
#48454=ORIENTED_EDGE('',*,*,#35929,.T.);
#48455=ORIENTED_EDGE('',*,*,#36182,.F.);
#48456=ORIENTED_EDGE('',*,*,#36183,.F.);
#48457=ORIENTED_EDGE('',*,*,#35935,.T.);
#48458=ORIENTED_EDGE('',*,*,#36183,.T.);
#48459=ORIENTED_EDGE('',*,*,#36184,.F.);
#48460=ORIENTED_EDGE('',*,*,#35933,.T.);
#48461=ORIENTED_EDGE('',*,*,#35941,.T.);
#48462=ORIENTED_EDGE('',*,*,#35936,.T.);
#48463=ORIENTED_EDGE('',*,*,#36185,.F.);
#48464=ORIENTED_EDGE('',*,*,#36186,.F.);
#48465=ORIENTED_EDGE('',*,*,#35942,.T.);
#48466=ORIENTED_EDGE('',*,*,#36186,.T.);
#48467=ORIENTED_EDGE('',*,*,#36187,.F.);
#48468=ORIENTED_EDGE('',*,*,#35940,.T.);
#48469=ORIENTED_EDGE('',*,*,#35948,.T.);
#48470=ORIENTED_EDGE('',*,*,#35943,.T.);
#48471=ORIENTED_EDGE('',*,*,#36188,.F.);
#48472=ORIENTED_EDGE('',*,*,#36189,.F.);
#48473=ORIENTED_EDGE('',*,*,#35949,.T.);
#48474=ORIENTED_EDGE('',*,*,#36189,.T.);
#48475=ORIENTED_EDGE('',*,*,#36190,.F.);
#48476=ORIENTED_EDGE('',*,*,#35947,.T.);
#48477=ORIENTED_EDGE('',*,*,#35955,.T.);
#48478=ORIENTED_EDGE('',*,*,#35950,.T.);
#48479=ORIENTED_EDGE('',*,*,#36191,.F.);
#48480=ORIENTED_EDGE('',*,*,#36192,.F.);
#48481=ORIENTED_EDGE('',*,*,#35956,.T.);
#48482=ORIENTED_EDGE('',*,*,#36192,.T.);
#48483=ORIENTED_EDGE('',*,*,#36193,.F.);
#48484=ORIENTED_EDGE('',*,*,#35954,.T.);
#48485=ORIENTED_EDGE('',*,*,#35962,.T.);
#48486=ORIENTED_EDGE('',*,*,#35957,.T.);
#48487=ORIENTED_EDGE('',*,*,#36194,.F.);
#48488=ORIENTED_EDGE('',*,*,#36195,.F.);
#48489=ORIENTED_EDGE('',*,*,#35963,.T.);
#48490=ORIENTED_EDGE('',*,*,#36195,.T.);
#48491=ORIENTED_EDGE('',*,*,#36196,.F.);
#48492=ORIENTED_EDGE('',*,*,#35961,.T.);
#48493=ORIENTED_EDGE('',*,*,#34448,.T.);
#48494=ORIENTED_EDGE('',*,*,#35964,.T.);
#48495=ORIENTED_EDGE('',*,*,#36197,.F.);
#48496=ORIENTED_EDGE('',*,*,#36198,.F.);
#48497=ORIENTED_EDGE('',*,*,#34445,.T.);
#48498=ORIENTED_EDGE('',*,*,#36198,.T.);
#48499=ORIENTED_EDGE('',*,*,#36199,.F.);
#48500=ORIENTED_EDGE('',*,*,#35966,.T.);
#48501=ORIENTED_EDGE('',*,*,#35972,.T.);
#48502=ORIENTED_EDGE('',*,*,#35967,.T.);
#48503=ORIENTED_EDGE('',*,*,#36200,.F.);
#48504=ORIENTED_EDGE('',*,*,#36201,.F.);
#48505=ORIENTED_EDGE('',*,*,#35973,.T.);
#48506=ORIENTED_EDGE('',*,*,#36201,.T.);
#48507=ORIENTED_EDGE('',*,*,#36202,.F.);
#48508=ORIENTED_EDGE('',*,*,#35971,.T.);
#48509=ORIENTED_EDGE('',*,*,#35979,.T.);
#48510=ORIENTED_EDGE('',*,*,#35974,.T.);
#48511=ORIENTED_EDGE('',*,*,#36203,.F.);
#48512=ORIENTED_EDGE('',*,*,#36204,.F.);
#48513=ORIENTED_EDGE('',*,*,#35980,.T.);
#48514=ORIENTED_EDGE('',*,*,#36204,.T.);
#48515=ORIENTED_EDGE('',*,*,#36205,.F.);
#48516=ORIENTED_EDGE('',*,*,#35978,.T.);
#48517=ORIENTED_EDGE('',*,*,#35986,.T.);
#48518=ORIENTED_EDGE('',*,*,#35981,.T.);
#48519=ORIENTED_EDGE('',*,*,#36206,.F.);
#48520=ORIENTED_EDGE('',*,*,#36207,.F.);
#48521=ORIENTED_EDGE('',*,*,#35987,.T.);
#48522=ORIENTED_EDGE('',*,*,#36207,.T.);
#48523=ORIENTED_EDGE('',*,*,#36208,.F.);
#48524=ORIENTED_EDGE('',*,*,#35985,.T.);
#48525=ORIENTED_EDGE('',*,*,#35993,.T.);
#48526=ORIENTED_EDGE('',*,*,#35988,.T.);
#48527=ORIENTED_EDGE('',*,*,#36209,.F.);
#48528=ORIENTED_EDGE('',*,*,#36210,.F.);
#48529=ORIENTED_EDGE('',*,*,#35994,.T.);
#48530=ORIENTED_EDGE('',*,*,#36210,.T.);
#48531=ORIENTED_EDGE('',*,*,#36211,.F.);
#48532=ORIENTED_EDGE('',*,*,#35992,.T.);
#48533=ORIENTED_EDGE('',*,*,#36000,.T.);
#48534=ORIENTED_EDGE('',*,*,#35995,.T.);
#48535=ORIENTED_EDGE('',*,*,#36212,.F.);
#48536=ORIENTED_EDGE('',*,*,#36213,.F.);
#48537=ORIENTED_EDGE('',*,*,#36001,.T.);
#48538=ORIENTED_EDGE('',*,*,#36213,.T.);
#48539=ORIENTED_EDGE('',*,*,#36214,.F.);
#48540=ORIENTED_EDGE('',*,*,#35999,.T.);
#48541=ORIENTED_EDGE('',*,*,#36007,.T.);
#48542=ORIENTED_EDGE('',*,*,#36002,.T.);
#48543=ORIENTED_EDGE('',*,*,#36215,.F.);
#48544=ORIENTED_EDGE('',*,*,#36216,.F.);
#48545=ORIENTED_EDGE('',*,*,#36008,.T.);
#48546=ORIENTED_EDGE('',*,*,#36216,.T.);
#48547=ORIENTED_EDGE('',*,*,#36217,.F.);
#48548=ORIENTED_EDGE('',*,*,#36006,.T.);
#48549=ORIENTED_EDGE('',*,*,#36014,.T.);
#48550=ORIENTED_EDGE('',*,*,#36009,.T.);
#48551=ORIENTED_EDGE('',*,*,#36218,.F.);
#48552=ORIENTED_EDGE('',*,*,#36219,.F.);
#48553=ORIENTED_EDGE('',*,*,#36015,.T.);
#48554=ORIENTED_EDGE('',*,*,#36219,.T.);
#48555=ORIENTED_EDGE('',*,*,#36220,.F.);
#48556=ORIENTED_EDGE('',*,*,#36013,.T.);
#48557=ORIENTED_EDGE('',*,*,#36021,.T.);
#48558=ORIENTED_EDGE('',*,*,#36016,.T.);
#48559=ORIENTED_EDGE('',*,*,#36221,.F.);
#48560=ORIENTED_EDGE('',*,*,#36222,.F.);
#48561=ORIENTED_EDGE('',*,*,#36022,.T.);
#48562=ORIENTED_EDGE('',*,*,#36222,.T.);
#48563=ORIENTED_EDGE('',*,*,#36223,.F.);
#48564=ORIENTED_EDGE('',*,*,#36020,.T.);
#48565=ORIENTED_EDGE('',*,*,#36028,.T.);
#48566=ORIENTED_EDGE('',*,*,#36023,.T.);
#48567=ORIENTED_EDGE('',*,*,#36224,.F.);
#48568=ORIENTED_EDGE('',*,*,#36225,.F.);
#48569=ORIENTED_EDGE('',*,*,#36029,.T.);
#48570=ORIENTED_EDGE('',*,*,#36225,.T.);
#48571=ORIENTED_EDGE('',*,*,#36226,.F.);
#48572=ORIENTED_EDGE('',*,*,#36027,.T.);
#48573=ORIENTED_EDGE('',*,*,#36035,.T.);
#48574=ORIENTED_EDGE('',*,*,#36030,.T.);
#48575=ORIENTED_EDGE('',*,*,#36227,.F.);
#48576=ORIENTED_EDGE('',*,*,#36228,.F.);
#48577=ORIENTED_EDGE('',*,*,#36036,.T.);
#48578=ORIENTED_EDGE('',*,*,#36228,.T.);
#48579=ORIENTED_EDGE('',*,*,#36229,.F.);
#48580=ORIENTED_EDGE('',*,*,#36034,.T.);
#48581=ORIENTED_EDGE('',*,*,#36042,.T.);
#48582=ORIENTED_EDGE('',*,*,#36037,.T.);
#48583=ORIENTED_EDGE('',*,*,#36230,.F.);
#48584=ORIENTED_EDGE('',*,*,#36231,.F.);
#48585=ORIENTED_EDGE('',*,*,#36043,.T.);
#48586=ORIENTED_EDGE('',*,*,#36231,.T.);
#48587=ORIENTED_EDGE('',*,*,#36232,.F.);
#48588=ORIENTED_EDGE('',*,*,#36041,.T.);
#48589=ORIENTED_EDGE('',*,*,#36049,.T.);
#48590=ORIENTED_EDGE('',*,*,#36044,.T.);
#48591=ORIENTED_EDGE('',*,*,#36233,.F.);
#48592=ORIENTED_EDGE('',*,*,#36234,.F.);
#48593=ORIENTED_EDGE('',*,*,#36050,.T.);
#48594=ORIENTED_EDGE('',*,*,#36234,.T.);
#48595=ORIENTED_EDGE('',*,*,#36235,.F.);
#48596=ORIENTED_EDGE('',*,*,#36048,.T.);
#48597=ORIENTED_EDGE('',*,*,#36056,.T.);
#48598=ORIENTED_EDGE('',*,*,#36051,.T.);
#48599=ORIENTED_EDGE('',*,*,#36236,.F.);
#48600=ORIENTED_EDGE('',*,*,#36237,.F.);
#48601=ORIENTED_EDGE('',*,*,#36057,.T.);
#48602=ORIENTED_EDGE('',*,*,#36237,.T.);
#48603=ORIENTED_EDGE('',*,*,#36238,.F.);
#48604=ORIENTED_EDGE('',*,*,#36055,.T.);
#48605=ORIENTED_EDGE('',*,*,#36063,.T.);
#48606=ORIENTED_EDGE('',*,*,#36058,.T.);
#48607=ORIENTED_EDGE('',*,*,#36239,.F.);
#48608=ORIENTED_EDGE('',*,*,#36240,.F.);
#48609=ORIENTED_EDGE('',*,*,#36064,.T.);
#48610=ORIENTED_EDGE('',*,*,#36240,.T.);
#48611=ORIENTED_EDGE('',*,*,#36241,.F.);
#48612=ORIENTED_EDGE('',*,*,#36062,.T.);
#48613=ORIENTED_EDGE('',*,*,#36066,.T.);
#48614=ORIENTED_EDGE('',*,*,#36068,.T.);
#48615=ORIENTED_EDGE('',*,*,#36242,.F.);
#48616=ORIENTED_EDGE('',*,*,#36156,.T.);
#48617=ORIENTED_EDGE('',*,*,#36243,.T.);
#48618=ORIENTED_EDGE('',*,*,#36244,.F.);
#48619=ORIENTED_EDGE('',*,*,#36069,.T.);
#48620=ORIENTED_EDGE('',*,*,#36245,.F.);
#48621=ORIENTED_EDGE('',*,*,#36246,.F.);
#48622=ORIENTED_EDGE('',*,*,#36247,.F.);
#48623=ORIENTED_EDGE('',*,*,#36248,.F.);
#48624=ORIENTED_EDGE('',*,*,#36243,.F.);
#48625=ORIENTED_EDGE('',*,*,#36248,.T.);
#48626=ORIENTED_EDGE('',*,*,#36249,.F.);
#48627=ORIENTED_EDGE('',*,*,#36071,.T.);
#48628=ORIENTED_EDGE('',*,*,#36244,.T.);
#48629=ORIENTED_EDGE('',*,*,#36250,.T.);
#48630=ORIENTED_EDGE('',*,*,#36251,.F.);
#48631=ORIENTED_EDGE('',*,*,#36073,.T.);
#48632=ORIENTED_EDGE('',*,*,#36252,.F.);
#48633=ORIENTED_EDGE('',*,*,#36253,.F.);
#48634=ORIENTED_EDGE('',*,*,#36254,.F.);
#48635=ORIENTED_EDGE('',*,*,#36255,.F.);
#48636=ORIENTED_EDGE('',*,*,#36250,.F.);
#48637=ORIENTED_EDGE('',*,*,#36255,.T.);
#48638=ORIENTED_EDGE('',*,*,#36256,.F.);
#48639=ORIENTED_EDGE('',*,*,#36074,.T.);
#48640=ORIENTED_EDGE('',*,*,#36251,.T.);
#48641=ORIENTED_EDGE('',*,*,#36257,.T.);
#48642=ORIENTED_EDGE('',*,*,#36258,.F.);
#48643=ORIENTED_EDGE('',*,*,#36076,.T.);
#48644=ORIENTED_EDGE('',*,*,#36259,.F.);
#48645=ORIENTED_EDGE('',*,*,#36260,.F.);
#48646=ORIENTED_EDGE('',*,*,#36261,.F.);
#48647=ORIENTED_EDGE('',*,*,#36262,.F.);
#48648=ORIENTED_EDGE('',*,*,#36257,.F.);
#48649=ORIENTED_EDGE('',*,*,#36262,.T.);
#48650=ORIENTED_EDGE('',*,*,#36263,.F.);
#48651=ORIENTED_EDGE('',*,*,#36077,.T.);
#48652=ORIENTED_EDGE('',*,*,#36258,.T.);
#48653=ORIENTED_EDGE('',*,*,#36264,.T.);
#48654=ORIENTED_EDGE('',*,*,#36265,.F.);
#48655=ORIENTED_EDGE('',*,*,#36079,.T.);
#48656=ORIENTED_EDGE('',*,*,#36266,.F.);
#48657=ORIENTED_EDGE('',*,*,#36267,.F.);
#48658=ORIENTED_EDGE('',*,*,#36268,.F.);
#48659=ORIENTED_EDGE('',*,*,#36269,.F.);
#48660=ORIENTED_EDGE('',*,*,#36264,.F.);
#48661=ORIENTED_EDGE('',*,*,#36269,.T.);
#48662=ORIENTED_EDGE('',*,*,#36270,.F.);
#48663=ORIENTED_EDGE('',*,*,#36080,.T.);
#48664=ORIENTED_EDGE('',*,*,#36265,.T.);
#48665=ORIENTED_EDGE('',*,*,#36271,.T.);
#48666=ORIENTED_EDGE('',*,*,#36272,.F.);
#48667=ORIENTED_EDGE('',*,*,#36082,.T.);
#48668=ORIENTED_EDGE('',*,*,#36273,.F.);
#48669=ORIENTED_EDGE('',*,*,#36274,.F.);
#48670=ORIENTED_EDGE('',*,*,#36275,.F.);
#48671=ORIENTED_EDGE('',*,*,#36276,.F.);
#48672=ORIENTED_EDGE('',*,*,#36271,.F.);
#48673=ORIENTED_EDGE('',*,*,#36276,.T.);
#48674=ORIENTED_EDGE('',*,*,#36277,.F.);
#48675=ORIENTED_EDGE('',*,*,#36083,.T.);
#48676=ORIENTED_EDGE('',*,*,#36272,.T.);
#48677=ORIENTED_EDGE('',*,*,#36278,.T.);
#48678=ORIENTED_EDGE('',*,*,#36279,.F.);
#48679=ORIENTED_EDGE('',*,*,#36085,.T.);
#48680=ORIENTED_EDGE('',*,*,#36280,.F.);
#48681=ORIENTED_EDGE('',*,*,#36281,.F.);
#48682=ORIENTED_EDGE('',*,*,#36282,.F.);
#48683=ORIENTED_EDGE('',*,*,#36283,.F.);
#48684=ORIENTED_EDGE('',*,*,#36278,.F.);
#48685=ORIENTED_EDGE('',*,*,#36283,.T.);
#48686=ORIENTED_EDGE('',*,*,#36284,.F.);
#48687=ORIENTED_EDGE('',*,*,#36086,.T.);
#48688=ORIENTED_EDGE('',*,*,#36279,.T.);
#48689=ORIENTED_EDGE('',*,*,#36285,.T.);
#48690=ORIENTED_EDGE('',*,*,#36286,.F.);
#48691=ORIENTED_EDGE('',*,*,#36088,.T.);
#48692=ORIENTED_EDGE('',*,*,#36287,.F.);
#48693=ORIENTED_EDGE('',*,*,#36288,.F.);
#48694=ORIENTED_EDGE('',*,*,#36289,.F.);
#48695=ORIENTED_EDGE('',*,*,#36290,.F.);
#48696=ORIENTED_EDGE('',*,*,#36285,.F.);
#48697=ORIENTED_EDGE('',*,*,#36290,.T.);
#48698=ORIENTED_EDGE('',*,*,#36291,.F.);
#48699=ORIENTED_EDGE('',*,*,#36089,.T.);
#48700=ORIENTED_EDGE('',*,*,#36286,.T.);
#48701=ORIENTED_EDGE('',*,*,#36292,.T.);
#48702=ORIENTED_EDGE('',*,*,#36293,.F.);
#48703=ORIENTED_EDGE('',*,*,#36091,.T.);
#48704=ORIENTED_EDGE('',*,*,#36294,.F.);
#48705=ORIENTED_EDGE('',*,*,#36295,.F.);
#48706=ORIENTED_EDGE('',*,*,#36296,.F.);
#48707=ORIENTED_EDGE('',*,*,#36297,.F.);
#48708=ORIENTED_EDGE('',*,*,#36292,.F.);
#48709=ORIENTED_EDGE('',*,*,#36297,.T.);
#48710=ORIENTED_EDGE('',*,*,#36298,.F.);
#48711=ORIENTED_EDGE('',*,*,#36092,.T.);
#48712=ORIENTED_EDGE('',*,*,#36293,.T.);
#48713=ORIENTED_EDGE('',*,*,#36299,.T.);
#48714=ORIENTED_EDGE('',*,*,#36300,.F.);
#48715=ORIENTED_EDGE('',*,*,#36094,.T.);
#48716=ORIENTED_EDGE('',*,*,#36301,.F.);
#48717=ORIENTED_EDGE('',*,*,#36302,.F.);
#48718=ORIENTED_EDGE('',*,*,#36303,.F.);
#48719=ORIENTED_EDGE('',*,*,#36304,.F.);
#48720=ORIENTED_EDGE('',*,*,#36299,.F.);
#48721=ORIENTED_EDGE('',*,*,#36304,.T.);
#48722=ORIENTED_EDGE('',*,*,#36305,.F.);
#48723=ORIENTED_EDGE('',*,*,#36095,.T.);
#48724=ORIENTED_EDGE('',*,*,#36300,.T.);
#48725=ORIENTED_EDGE('',*,*,#36306,.T.);
#48726=ORIENTED_EDGE('',*,*,#36307,.F.);
#48727=ORIENTED_EDGE('',*,*,#36097,.T.);
#48728=ORIENTED_EDGE('',*,*,#36308,.F.);
#48729=ORIENTED_EDGE('',*,*,#36309,.F.);
#48730=ORIENTED_EDGE('',*,*,#36310,.F.);
#48731=ORIENTED_EDGE('',*,*,#36311,.F.);
#48732=ORIENTED_EDGE('',*,*,#36306,.F.);
#48733=ORIENTED_EDGE('',*,*,#36311,.T.);
#48734=ORIENTED_EDGE('',*,*,#36312,.F.);
#48735=ORIENTED_EDGE('',*,*,#36098,.T.);
#48736=ORIENTED_EDGE('',*,*,#36307,.T.);
#48737=ORIENTED_EDGE('',*,*,#36313,.T.);
#48738=ORIENTED_EDGE('',*,*,#36314,.F.);
#48739=ORIENTED_EDGE('',*,*,#36100,.T.);
#48740=ORIENTED_EDGE('',*,*,#36315,.F.);
#48741=ORIENTED_EDGE('',*,*,#36316,.F.);
#48742=ORIENTED_EDGE('',*,*,#36317,.F.);
#48743=ORIENTED_EDGE('',*,*,#36318,.F.);
#48744=ORIENTED_EDGE('',*,*,#36313,.F.);
#48745=ORIENTED_EDGE('',*,*,#36318,.T.);
#48746=ORIENTED_EDGE('',*,*,#36319,.F.);
#48747=ORIENTED_EDGE('',*,*,#36101,.T.);
#48748=ORIENTED_EDGE('',*,*,#36314,.T.);
#48749=ORIENTED_EDGE('',*,*,#36320,.T.);
#48750=ORIENTED_EDGE('',*,*,#36321,.F.);
#48751=ORIENTED_EDGE('',*,*,#36103,.T.);
#48752=ORIENTED_EDGE('',*,*,#36322,.F.);
#48753=ORIENTED_EDGE('',*,*,#36323,.F.);
#48754=ORIENTED_EDGE('',*,*,#36324,.F.);
#48755=ORIENTED_EDGE('',*,*,#36325,.F.);
#48756=ORIENTED_EDGE('',*,*,#36320,.F.);
#48757=ORIENTED_EDGE('',*,*,#36325,.T.);
#48758=ORIENTED_EDGE('',*,*,#36326,.F.);
#48759=ORIENTED_EDGE('',*,*,#36104,.T.);
#48760=ORIENTED_EDGE('',*,*,#36321,.T.);
#48761=ORIENTED_EDGE('',*,*,#36327,.T.);
#48762=ORIENTED_EDGE('',*,*,#36328,.F.);
#48763=ORIENTED_EDGE('',*,*,#36106,.T.);
#48764=ORIENTED_EDGE('',*,*,#36329,.F.);
#48765=ORIENTED_EDGE('',*,*,#36330,.F.);
#48766=ORIENTED_EDGE('',*,*,#36331,.F.);
#48767=ORIENTED_EDGE('',*,*,#36332,.F.);
#48768=ORIENTED_EDGE('',*,*,#36327,.F.);
#48769=ORIENTED_EDGE('',*,*,#36332,.T.);
#48770=ORIENTED_EDGE('',*,*,#36333,.F.);
#48771=ORIENTED_EDGE('',*,*,#36107,.T.);
#48772=ORIENTED_EDGE('',*,*,#36328,.T.);
#48773=ORIENTED_EDGE('',*,*,#36334,.T.);
#48774=ORIENTED_EDGE('',*,*,#36335,.F.);
#48775=ORIENTED_EDGE('',*,*,#36109,.T.);
#48776=ORIENTED_EDGE('',*,*,#36336,.F.);
#48777=ORIENTED_EDGE('',*,*,#36337,.F.);
#48778=ORIENTED_EDGE('',*,*,#36338,.F.);
#48779=ORIENTED_EDGE('',*,*,#36339,.F.);
#48780=ORIENTED_EDGE('',*,*,#36334,.F.);
#48781=ORIENTED_EDGE('',*,*,#36339,.T.);
#48782=ORIENTED_EDGE('',*,*,#36340,.F.);
#48783=ORIENTED_EDGE('',*,*,#36110,.T.);
#48784=ORIENTED_EDGE('',*,*,#36335,.T.);
#48785=ORIENTED_EDGE('',*,*,#34441,.T.);
#48786=ORIENTED_EDGE('',*,*,#36341,.F.);
#48787=ORIENTED_EDGE('',*,*,#36112,.T.);
#48788=ORIENTED_EDGE('',*,*,#36342,.F.);
#48789=ORIENTED_EDGE('',*,*,#34444,.T.);
#48790=ORIENTED_EDGE('',*,*,#36343,.F.);
#48791=ORIENTED_EDGE('',*,*,#36113,.T.);
#48792=ORIENTED_EDGE('',*,*,#36341,.T.);
#48793=ORIENTED_EDGE('',*,*,#36344,.T.);
#48794=ORIENTED_EDGE('',*,*,#36345,.F.);
#48795=ORIENTED_EDGE('',*,*,#36115,.T.);
#48796=ORIENTED_EDGE('',*,*,#36346,.F.);
#48797=ORIENTED_EDGE('',*,*,#36347,.F.);
#48798=ORIENTED_EDGE('',*,*,#36348,.F.);
#48799=ORIENTED_EDGE('',*,*,#36349,.F.);
#48800=ORIENTED_EDGE('',*,*,#36344,.F.);
#48801=ORIENTED_EDGE('',*,*,#36349,.T.);
#48802=ORIENTED_EDGE('',*,*,#36350,.F.);
#48803=ORIENTED_EDGE('',*,*,#36116,.T.);
#48804=ORIENTED_EDGE('',*,*,#36345,.T.);
#48805=ORIENTED_EDGE('',*,*,#36351,.T.);
#48806=ORIENTED_EDGE('',*,*,#36352,.F.);
#48807=ORIENTED_EDGE('',*,*,#36118,.T.);
#48808=ORIENTED_EDGE('',*,*,#36353,.F.);
#48809=ORIENTED_EDGE('',*,*,#36354,.F.);
#48810=ORIENTED_EDGE('',*,*,#36355,.F.);
#48811=ORIENTED_EDGE('',*,*,#36356,.F.);
#48812=ORIENTED_EDGE('',*,*,#36351,.F.);
#48813=ORIENTED_EDGE('',*,*,#36356,.T.);
#48814=ORIENTED_EDGE('',*,*,#36357,.F.);
#48815=ORIENTED_EDGE('',*,*,#36119,.T.);
#48816=ORIENTED_EDGE('',*,*,#36352,.T.);
#48817=ORIENTED_EDGE('',*,*,#36358,.T.);
#48818=ORIENTED_EDGE('',*,*,#36359,.F.);
#48819=ORIENTED_EDGE('',*,*,#36121,.T.);
#48820=ORIENTED_EDGE('',*,*,#36360,.F.);
#48821=ORIENTED_EDGE('',*,*,#36361,.F.);
#48822=ORIENTED_EDGE('',*,*,#36362,.F.);
#48823=ORIENTED_EDGE('',*,*,#36363,.F.);
#48824=ORIENTED_EDGE('',*,*,#36358,.F.);
#48825=ORIENTED_EDGE('',*,*,#36363,.T.);
#48826=ORIENTED_EDGE('',*,*,#36364,.F.);
#48827=ORIENTED_EDGE('',*,*,#36122,.T.);
#48828=ORIENTED_EDGE('',*,*,#36359,.T.);
#48829=ORIENTED_EDGE('',*,*,#36365,.T.);
#48830=ORIENTED_EDGE('',*,*,#36366,.F.);
#48831=ORIENTED_EDGE('',*,*,#36124,.T.);
#48832=ORIENTED_EDGE('',*,*,#36367,.F.);
#48833=ORIENTED_EDGE('',*,*,#36368,.F.);
#48834=ORIENTED_EDGE('',*,*,#36369,.F.);
#48835=ORIENTED_EDGE('',*,*,#36370,.F.);
#48836=ORIENTED_EDGE('',*,*,#36365,.F.);
#48837=ORIENTED_EDGE('',*,*,#36370,.T.);
#48838=ORIENTED_EDGE('',*,*,#36371,.F.);
#48839=ORIENTED_EDGE('',*,*,#36125,.T.);
#48840=ORIENTED_EDGE('',*,*,#36366,.T.);
#48841=ORIENTED_EDGE('',*,*,#36372,.T.);
#48842=ORIENTED_EDGE('',*,*,#36373,.F.);
#48843=ORIENTED_EDGE('',*,*,#36127,.T.);
#48844=ORIENTED_EDGE('',*,*,#36374,.F.);
#48845=ORIENTED_EDGE('',*,*,#36375,.F.);
#48846=ORIENTED_EDGE('',*,*,#36376,.F.);
#48847=ORIENTED_EDGE('',*,*,#36377,.F.);
#48848=ORIENTED_EDGE('',*,*,#36372,.F.);
#48849=ORIENTED_EDGE('',*,*,#36377,.T.);
#48850=ORIENTED_EDGE('',*,*,#36378,.F.);
#48851=ORIENTED_EDGE('',*,*,#36128,.T.);
#48852=ORIENTED_EDGE('',*,*,#36373,.T.);
#48853=ORIENTED_EDGE('',*,*,#36379,.T.);
#48854=ORIENTED_EDGE('',*,*,#36380,.F.);
#48855=ORIENTED_EDGE('',*,*,#36130,.T.);
#48856=ORIENTED_EDGE('',*,*,#36381,.F.);
#48857=ORIENTED_EDGE('',*,*,#36382,.F.);
#48858=ORIENTED_EDGE('',*,*,#36383,.F.);
#48859=ORIENTED_EDGE('',*,*,#36384,.F.);
#48860=ORIENTED_EDGE('',*,*,#36379,.F.);
#48861=ORIENTED_EDGE('',*,*,#36384,.T.);
#48862=ORIENTED_EDGE('',*,*,#36385,.F.);
#48863=ORIENTED_EDGE('',*,*,#36131,.T.);
#48864=ORIENTED_EDGE('',*,*,#36380,.T.);
#48865=ORIENTED_EDGE('',*,*,#36386,.T.);
#48866=ORIENTED_EDGE('',*,*,#36387,.F.);
#48867=ORIENTED_EDGE('',*,*,#36133,.T.);
#48868=ORIENTED_EDGE('',*,*,#36388,.F.);
#48869=ORIENTED_EDGE('',*,*,#36389,.F.);
#48870=ORIENTED_EDGE('',*,*,#36390,.F.);
#48871=ORIENTED_EDGE('',*,*,#36391,.F.);
#48872=ORIENTED_EDGE('',*,*,#36386,.F.);
#48873=ORIENTED_EDGE('',*,*,#36391,.T.);
#48874=ORIENTED_EDGE('',*,*,#36392,.F.);
#48875=ORIENTED_EDGE('',*,*,#36134,.T.);
#48876=ORIENTED_EDGE('',*,*,#36387,.T.);
#48877=ORIENTED_EDGE('',*,*,#36393,.T.);
#48878=ORIENTED_EDGE('',*,*,#36394,.F.);
#48879=ORIENTED_EDGE('',*,*,#36136,.T.);
#48880=ORIENTED_EDGE('',*,*,#36395,.F.);
#48881=ORIENTED_EDGE('',*,*,#36396,.F.);
#48882=ORIENTED_EDGE('',*,*,#36397,.F.);
#48883=ORIENTED_EDGE('',*,*,#36398,.F.);
#48884=ORIENTED_EDGE('',*,*,#36393,.F.);
#48885=ORIENTED_EDGE('',*,*,#36398,.T.);
#48886=ORIENTED_EDGE('',*,*,#36399,.F.);
#48887=ORIENTED_EDGE('',*,*,#36137,.T.);
#48888=ORIENTED_EDGE('',*,*,#36394,.T.);
#48889=ORIENTED_EDGE('',*,*,#36400,.T.);
#48890=ORIENTED_EDGE('',*,*,#36401,.F.);
#48891=ORIENTED_EDGE('',*,*,#36139,.T.);
#48892=ORIENTED_EDGE('',*,*,#36402,.F.);
#48893=ORIENTED_EDGE('',*,*,#36403,.T.);
#48894=ORIENTED_EDGE('',*,*,#36404,.F.);
#48895=ORIENTED_EDGE('',*,*,#36140,.T.);
#48896=ORIENTED_EDGE('',*,*,#36401,.T.);
#48897=ORIENTED_EDGE('',*,*,#36405,.F.);
#48898=ORIENTED_EDGE('',*,*,#36406,.F.);
#48899=ORIENTED_EDGE('',*,*,#36403,.F.);
#48900=ORIENTED_EDGE('',*,*,#36400,.F.);
#48901=ORIENTED_EDGE('',*,*,#36142,.T.);
#48902=ORIENTED_EDGE('',*,*,#36407,.F.);
#48903=ORIENTED_EDGE('',*,*,#36408,.T.);
#48904=ORIENTED_EDGE('',*,*,#36409,.F.);
#48905=ORIENTED_EDGE('',*,*,#36410,.F.);
#48906=ORIENTED_EDGE('',*,*,#36408,.F.);
#48907=ORIENTED_EDGE('',*,*,#36411,.F.);
#48908=ORIENTED_EDGE('',*,*,#36412,.F.);
#48909=ORIENTED_EDGE('',*,*,#36143,.T.);
#48910=ORIENTED_EDGE('',*,*,#36409,.T.);
#48911=ORIENTED_EDGE('',*,*,#36410,.T.);
#48912=ORIENTED_EDGE('',*,*,#36413,.F.);
#48913=ORIENTED_EDGE('',*,*,#36414,.T.);
#48914=ORIENTED_EDGE('',*,*,#36415,.F.);
#48915=ORIENTED_EDGE('',*,*,#36145,.T.);
#48916=ORIENTED_EDGE('',*,*,#36416,.F.);
#48917=ORIENTED_EDGE('',*,*,#36417,.F.);
#48918=ORIENTED_EDGE('',*,*,#36418,.F.);
#48919=ORIENTED_EDGE('',*,*,#36419,.F.);
#48920=ORIENTED_EDGE('',*,*,#36414,.F.);
#48921=ORIENTED_EDGE('',*,*,#36419,.T.);
#48922=ORIENTED_EDGE('',*,*,#36420,.F.);
#48923=ORIENTED_EDGE('',*,*,#36146,.T.);
#48924=ORIENTED_EDGE('',*,*,#36415,.T.);
#48925=ORIENTED_EDGE('',*,*,#36421,.T.);
#48926=ORIENTED_EDGE('',*,*,#36422,.F.);
#48927=ORIENTED_EDGE('',*,*,#36148,.T.);
#48928=ORIENTED_EDGE('',*,*,#36423,.F.);
#48929=ORIENTED_EDGE('',*,*,#36424,.F.);
#48930=ORIENTED_EDGE('',*,*,#36425,.F.);
#48931=ORIENTED_EDGE('',*,*,#36426,.F.);
#48932=ORIENTED_EDGE('',*,*,#36421,.F.);
#48933=ORIENTED_EDGE('',*,*,#36426,.T.);
#48934=ORIENTED_EDGE('',*,*,#36427,.F.);
#48935=ORIENTED_EDGE('',*,*,#36149,.T.);
#48936=ORIENTED_EDGE('',*,*,#36422,.T.);
#48937=ORIENTED_EDGE('',*,*,#36428,.T.);
#48938=ORIENTED_EDGE('',*,*,#36429,.F.);
#48939=ORIENTED_EDGE('',*,*,#36151,.T.);
#48940=ORIENTED_EDGE('',*,*,#36430,.F.);
#48941=ORIENTED_EDGE('',*,*,#36431,.F.);
#48942=ORIENTED_EDGE('',*,*,#36432,.F.);
#48943=ORIENTED_EDGE('',*,*,#36433,.F.);
#48944=ORIENTED_EDGE('',*,*,#36428,.F.);
#48945=ORIENTED_EDGE('',*,*,#36433,.T.);
#48946=ORIENTED_EDGE('',*,*,#36434,.F.);
#48947=ORIENTED_EDGE('',*,*,#36152,.T.);
#48948=ORIENTED_EDGE('',*,*,#36429,.T.);
#48949=ORIENTED_EDGE('',*,*,#36435,.T.);
#48950=ORIENTED_EDGE('',*,*,#36436,.F.);
#48951=ORIENTED_EDGE('',*,*,#36154,.T.);
#48952=ORIENTED_EDGE('',*,*,#36437,.F.);
#48953=ORIENTED_EDGE('',*,*,#36438,.F.);
#48954=ORIENTED_EDGE('',*,*,#36439,.F.);
#48955=ORIENTED_EDGE('',*,*,#36440,.F.);
#48956=ORIENTED_EDGE('',*,*,#36435,.F.);
#48957=ORIENTED_EDGE('',*,*,#36440,.T.);
#48958=ORIENTED_EDGE('',*,*,#36441,.F.);
#48959=ORIENTED_EDGE('',*,*,#36155,.T.);
#48960=ORIENTED_EDGE('',*,*,#36436,.T.);
#48961=ORIENTED_EDGE('',*,*,#36157,.T.);
#48962=ORIENTED_EDGE('',*,*,#36442,.F.);
#48963=ORIENTED_EDGE('',*,*,#36443,.T.);
#48964=ORIENTED_EDGE('',*,*,#36444,.F.);
#48965=ORIENTED_EDGE('',*,*,#36445,.T.);
#48966=ORIENTED_EDGE('',*,*,#36446,.F.);
#48967=ORIENTED_EDGE('',*,*,#36158,.T.);
#48968=ORIENTED_EDGE('',*,*,#36444,.T.);
#48969=ORIENTED_EDGE('',*,*,#36447,.F.);
#48970=ORIENTED_EDGE('',*,*,#36448,.F.);
#48971=ORIENTED_EDGE('',*,*,#36445,.F.);
#48972=ORIENTED_EDGE('',*,*,#36443,.F.);
#48973=ORIENTED_EDGE('',*,*,#36160,.T.);
#48974=ORIENTED_EDGE('',*,*,#36449,.F.);
#48975=ORIENTED_EDGE('',*,*,#36450,.T.);
#48976=ORIENTED_EDGE('',*,*,#36451,.F.);
#48977=ORIENTED_EDGE('',*,*,#36161,.T.);
#48978=ORIENTED_EDGE('',*,*,#36451,.T.);
#48979=ORIENTED_EDGE('',*,*,#36452,.T.);
#48980=ORIENTED_EDGE('',*,*,#36453,.F.);
#48981=ORIENTED_EDGE('',*,*,#36452,.F.);
#48982=ORIENTED_EDGE('',*,*,#36450,.F.);
#48983=ORIENTED_EDGE('',*,*,#36454,.F.);
#48984=ORIENTED_EDGE('',*,*,#36455,.F.);
#48985=ORIENTED_EDGE('',*,*,#36163,.T.);
#48986=ORIENTED_EDGE('',*,*,#36456,.F.);
#48987=ORIENTED_EDGE('',*,*,#36457,.T.);
#48988=ORIENTED_EDGE('',*,*,#36458,.F.);
#48989=ORIENTED_EDGE('',*,*,#36164,.T.);
#48990=ORIENTED_EDGE('',*,*,#36458,.T.);
#48991=ORIENTED_EDGE('',*,*,#36459,.T.);
#48992=ORIENTED_EDGE('',*,*,#36460,.F.);
#48993=ORIENTED_EDGE('',*,*,#36459,.F.);
#48994=ORIENTED_EDGE('',*,*,#36457,.F.);
#48995=ORIENTED_EDGE('',*,*,#36461,.F.);
#48996=ORIENTED_EDGE('',*,*,#36462,.F.);
#48997=ORIENTED_EDGE('',*,*,#36166,.T.);
#48998=ORIENTED_EDGE('',*,*,#36463,.F.);
#48999=ORIENTED_EDGE('',*,*,#36464,.T.);
#49000=ORIENTED_EDGE('',*,*,#36465,.F.);
#49001=ORIENTED_EDGE('',*,*,#36167,.T.);
#49002=ORIENTED_EDGE('',*,*,#36465,.T.);
#49003=ORIENTED_EDGE('',*,*,#36466,.T.);
#49004=ORIENTED_EDGE('',*,*,#36467,.F.);
#49005=ORIENTED_EDGE('',*,*,#36466,.F.);
#49006=ORIENTED_EDGE('',*,*,#36464,.F.);
#49007=ORIENTED_EDGE('',*,*,#36468,.F.);
#49008=ORIENTED_EDGE('',*,*,#36469,.F.);
#49009=ORIENTED_EDGE('',*,*,#36169,.T.);
#49010=ORIENTED_EDGE('',*,*,#36470,.F.);
#49011=ORIENTED_EDGE('',*,*,#36471,.T.);
#49012=ORIENTED_EDGE('',*,*,#36472,.F.);
#49013=ORIENTED_EDGE('',*,*,#36170,.T.);
#49014=ORIENTED_EDGE('',*,*,#36472,.T.);
#49015=ORIENTED_EDGE('',*,*,#36473,.T.);
#49016=ORIENTED_EDGE('',*,*,#36474,.F.);
#49017=ORIENTED_EDGE('',*,*,#36473,.F.);
#49018=ORIENTED_EDGE('',*,*,#36471,.F.);
#49019=ORIENTED_EDGE('',*,*,#36475,.F.);
#49020=ORIENTED_EDGE('',*,*,#36476,.F.);
#49021=ORIENTED_EDGE('',*,*,#36172,.T.);
#49022=ORIENTED_EDGE('',*,*,#36477,.F.);
#49023=ORIENTED_EDGE('',*,*,#36478,.T.);
#49024=ORIENTED_EDGE('',*,*,#36479,.F.);
#49025=ORIENTED_EDGE('',*,*,#36173,.T.);
#49026=ORIENTED_EDGE('',*,*,#36479,.T.);
#49027=ORIENTED_EDGE('',*,*,#36480,.T.);
#49028=ORIENTED_EDGE('',*,*,#36481,.F.);
#49029=ORIENTED_EDGE('',*,*,#36480,.F.);
#49030=ORIENTED_EDGE('',*,*,#36478,.F.);
#49031=ORIENTED_EDGE('',*,*,#36482,.F.);
#49032=ORIENTED_EDGE('',*,*,#36483,.F.);
#49033=ORIENTED_EDGE('',*,*,#36175,.T.);
#49034=ORIENTED_EDGE('',*,*,#36484,.F.);
#49035=ORIENTED_EDGE('',*,*,#36485,.T.);
#49036=ORIENTED_EDGE('',*,*,#36486,.F.);
#49037=ORIENTED_EDGE('',*,*,#36176,.T.);
#49038=ORIENTED_EDGE('',*,*,#36486,.T.);
#49039=ORIENTED_EDGE('',*,*,#36487,.T.);
#49040=ORIENTED_EDGE('',*,*,#36488,.F.);
#49041=ORIENTED_EDGE('',*,*,#36487,.F.);
#49042=ORIENTED_EDGE('',*,*,#36485,.F.);
#49043=ORIENTED_EDGE('',*,*,#36489,.F.);
#49044=ORIENTED_EDGE('',*,*,#36490,.F.);
#49045=ORIENTED_EDGE('',*,*,#36178,.T.);
#49046=ORIENTED_EDGE('',*,*,#36491,.F.);
#49047=ORIENTED_EDGE('',*,*,#36492,.T.);
#49048=ORIENTED_EDGE('',*,*,#36493,.F.);
#49049=ORIENTED_EDGE('',*,*,#36179,.T.);
#49050=ORIENTED_EDGE('',*,*,#36493,.T.);
#49051=ORIENTED_EDGE('',*,*,#36494,.T.);
#49052=ORIENTED_EDGE('',*,*,#36495,.F.);
#49053=ORIENTED_EDGE('',*,*,#36494,.F.);
#49054=ORIENTED_EDGE('',*,*,#36492,.F.);
#49055=ORIENTED_EDGE('',*,*,#36496,.F.);
#49056=ORIENTED_EDGE('',*,*,#36497,.F.);
#49057=ORIENTED_EDGE('',*,*,#36181,.T.);
#49058=ORIENTED_EDGE('',*,*,#36498,.F.);
#49059=ORIENTED_EDGE('',*,*,#36499,.T.);
#49060=ORIENTED_EDGE('',*,*,#36500,.F.);
#49061=ORIENTED_EDGE('',*,*,#36182,.T.);
#49062=ORIENTED_EDGE('',*,*,#36500,.T.);
#49063=ORIENTED_EDGE('',*,*,#36501,.T.);
#49064=ORIENTED_EDGE('',*,*,#36502,.F.);
#49065=ORIENTED_EDGE('',*,*,#36501,.F.);
#49066=ORIENTED_EDGE('',*,*,#36499,.F.);
#49067=ORIENTED_EDGE('',*,*,#36503,.F.);
#49068=ORIENTED_EDGE('',*,*,#36504,.F.);
#49069=ORIENTED_EDGE('',*,*,#36184,.T.);
#49070=ORIENTED_EDGE('',*,*,#36505,.F.);
#49071=ORIENTED_EDGE('',*,*,#36506,.T.);
#49072=ORIENTED_EDGE('',*,*,#36507,.F.);
#49073=ORIENTED_EDGE('',*,*,#36185,.T.);
#49074=ORIENTED_EDGE('',*,*,#36507,.T.);
#49075=ORIENTED_EDGE('',*,*,#36508,.T.);
#49076=ORIENTED_EDGE('',*,*,#36509,.F.);
#49077=ORIENTED_EDGE('',*,*,#36508,.F.);
#49078=ORIENTED_EDGE('',*,*,#36506,.F.);
#49079=ORIENTED_EDGE('',*,*,#36510,.F.);
#49080=ORIENTED_EDGE('',*,*,#36511,.F.);
#49081=ORIENTED_EDGE('',*,*,#36187,.T.);
#49082=ORIENTED_EDGE('',*,*,#36512,.F.);
#49083=ORIENTED_EDGE('',*,*,#36513,.T.);
#49084=ORIENTED_EDGE('',*,*,#36514,.F.);
#49085=ORIENTED_EDGE('',*,*,#36188,.T.);
#49086=ORIENTED_EDGE('',*,*,#36514,.T.);
#49087=ORIENTED_EDGE('',*,*,#36515,.T.);
#49088=ORIENTED_EDGE('',*,*,#36516,.F.);
#49089=ORIENTED_EDGE('',*,*,#36515,.F.);
#49090=ORIENTED_EDGE('',*,*,#36513,.F.);
#49091=ORIENTED_EDGE('',*,*,#36517,.F.);
#49092=ORIENTED_EDGE('',*,*,#36518,.F.);
#49093=ORIENTED_EDGE('',*,*,#36190,.T.);
#49094=ORIENTED_EDGE('',*,*,#36519,.F.);
#49095=ORIENTED_EDGE('',*,*,#36520,.T.);
#49096=ORIENTED_EDGE('',*,*,#36521,.F.);
#49097=ORIENTED_EDGE('',*,*,#36191,.T.);
#49098=ORIENTED_EDGE('',*,*,#36521,.T.);
#49099=ORIENTED_EDGE('',*,*,#36522,.T.);
#49100=ORIENTED_EDGE('',*,*,#36523,.F.);
#49101=ORIENTED_EDGE('',*,*,#36522,.F.);
#49102=ORIENTED_EDGE('',*,*,#36520,.F.);
#49103=ORIENTED_EDGE('',*,*,#36524,.F.);
#49104=ORIENTED_EDGE('',*,*,#36525,.F.);
#49105=ORIENTED_EDGE('',*,*,#36193,.T.);
#49106=ORIENTED_EDGE('',*,*,#36526,.F.);
#49107=ORIENTED_EDGE('',*,*,#36527,.T.);
#49108=ORIENTED_EDGE('',*,*,#36528,.F.);
#49109=ORIENTED_EDGE('',*,*,#36194,.T.);
#49110=ORIENTED_EDGE('',*,*,#36528,.T.);
#49111=ORIENTED_EDGE('',*,*,#36529,.T.);
#49112=ORIENTED_EDGE('',*,*,#36530,.F.);
#49113=ORIENTED_EDGE('',*,*,#36529,.F.);
#49114=ORIENTED_EDGE('',*,*,#36527,.F.);
#49115=ORIENTED_EDGE('',*,*,#36531,.F.);
#49116=ORIENTED_EDGE('',*,*,#36532,.F.);
#49117=ORIENTED_EDGE('',*,*,#36196,.T.);
#49118=ORIENTED_EDGE('',*,*,#36533,.F.);
#49119=ORIENTED_EDGE('',*,*,#36534,.T.);
#49120=ORIENTED_EDGE('',*,*,#36535,.F.);
#49121=ORIENTED_EDGE('',*,*,#36197,.T.);
#49122=ORIENTED_EDGE('',*,*,#36535,.T.);
#49123=ORIENTED_EDGE('',*,*,#36536,.T.);
#49124=ORIENTED_EDGE('',*,*,#36537,.F.);
#49125=ORIENTED_EDGE('',*,*,#36536,.F.);
#49126=ORIENTED_EDGE('',*,*,#36534,.F.);
#49127=ORIENTED_EDGE('',*,*,#36538,.F.);
#49128=ORIENTED_EDGE('',*,*,#36539,.F.);
#49129=ORIENTED_EDGE('',*,*,#36199,.T.);
#49130=ORIENTED_EDGE('',*,*,#36540,.F.);
#49131=ORIENTED_EDGE('',*,*,#36541,.T.);
#49132=ORIENTED_EDGE('',*,*,#36542,.F.);
#49133=ORIENTED_EDGE('',*,*,#36200,.T.);
#49134=ORIENTED_EDGE('',*,*,#36542,.T.);
#49135=ORIENTED_EDGE('',*,*,#36543,.T.);
#49136=ORIENTED_EDGE('',*,*,#36544,.F.);
#49137=ORIENTED_EDGE('',*,*,#36543,.F.);
#49138=ORIENTED_EDGE('',*,*,#36541,.F.);
#49139=ORIENTED_EDGE('',*,*,#36545,.F.);
#49140=ORIENTED_EDGE('',*,*,#36546,.F.);
#49141=ORIENTED_EDGE('',*,*,#36202,.T.);
#49142=ORIENTED_EDGE('',*,*,#36547,.F.);
#49143=ORIENTED_EDGE('',*,*,#36548,.T.);
#49144=ORIENTED_EDGE('',*,*,#36549,.F.);
#49145=ORIENTED_EDGE('',*,*,#36203,.T.);
#49146=ORIENTED_EDGE('',*,*,#36549,.T.);
#49147=ORIENTED_EDGE('',*,*,#36550,.T.);
#49148=ORIENTED_EDGE('',*,*,#36551,.F.);
#49149=ORIENTED_EDGE('',*,*,#36550,.F.);
#49150=ORIENTED_EDGE('',*,*,#36548,.F.);
#49151=ORIENTED_EDGE('',*,*,#36552,.F.);
#49152=ORIENTED_EDGE('',*,*,#36553,.F.);
#49153=ORIENTED_EDGE('',*,*,#36205,.T.);
#49154=ORIENTED_EDGE('',*,*,#36554,.F.);
#49155=ORIENTED_EDGE('',*,*,#36555,.T.);
#49156=ORIENTED_EDGE('',*,*,#36556,.F.);
#49157=ORIENTED_EDGE('',*,*,#36206,.T.);
#49158=ORIENTED_EDGE('',*,*,#36556,.T.);
#49159=ORIENTED_EDGE('',*,*,#36557,.T.);
#49160=ORIENTED_EDGE('',*,*,#36558,.F.);
#49161=ORIENTED_EDGE('',*,*,#36557,.F.);
#49162=ORIENTED_EDGE('',*,*,#36555,.F.);
#49163=ORIENTED_EDGE('',*,*,#36559,.F.);
#49164=ORIENTED_EDGE('',*,*,#36560,.F.);
#49165=ORIENTED_EDGE('',*,*,#36208,.T.);
#49166=ORIENTED_EDGE('',*,*,#36561,.F.);
#49167=ORIENTED_EDGE('',*,*,#36562,.T.);
#49168=ORIENTED_EDGE('',*,*,#36563,.F.);
#49169=ORIENTED_EDGE('',*,*,#36209,.T.);
#49170=ORIENTED_EDGE('',*,*,#36563,.T.);
#49171=ORIENTED_EDGE('',*,*,#36564,.T.);
#49172=ORIENTED_EDGE('',*,*,#36565,.F.);
#49173=ORIENTED_EDGE('',*,*,#36564,.F.);
#49174=ORIENTED_EDGE('',*,*,#36562,.F.);
#49175=ORIENTED_EDGE('',*,*,#36566,.F.);
#49176=ORIENTED_EDGE('',*,*,#36567,.F.);
#49177=ORIENTED_EDGE('',*,*,#36211,.T.);
#49178=ORIENTED_EDGE('',*,*,#36568,.F.);
#49179=ORIENTED_EDGE('',*,*,#36569,.T.);
#49180=ORIENTED_EDGE('',*,*,#36570,.F.);
#49181=ORIENTED_EDGE('',*,*,#36212,.T.);
#49182=ORIENTED_EDGE('',*,*,#36570,.T.);
#49183=ORIENTED_EDGE('',*,*,#36571,.T.);
#49184=ORIENTED_EDGE('',*,*,#36572,.F.);
#49185=ORIENTED_EDGE('',*,*,#36571,.F.);
#49186=ORIENTED_EDGE('',*,*,#36569,.F.);
#49187=ORIENTED_EDGE('',*,*,#36573,.F.);
#49188=ORIENTED_EDGE('',*,*,#36574,.F.);
#49189=ORIENTED_EDGE('',*,*,#36214,.T.);
#49190=ORIENTED_EDGE('',*,*,#36575,.F.);
#49191=ORIENTED_EDGE('',*,*,#36576,.T.);
#49192=ORIENTED_EDGE('',*,*,#36577,.F.);
#49193=ORIENTED_EDGE('',*,*,#36215,.T.);
#49194=ORIENTED_EDGE('',*,*,#36577,.T.);
#49195=ORIENTED_EDGE('',*,*,#36578,.T.);
#49196=ORIENTED_EDGE('',*,*,#36579,.F.);
#49197=ORIENTED_EDGE('',*,*,#36578,.F.);
#49198=ORIENTED_EDGE('',*,*,#36576,.F.);
#49199=ORIENTED_EDGE('',*,*,#36580,.F.);
#49200=ORIENTED_EDGE('',*,*,#36581,.F.);
#49201=ORIENTED_EDGE('',*,*,#36217,.T.);
#49202=ORIENTED_EDGE('',*,*,#36582,.F.);
#49203=ORIENTED_EDGE('',*,*,#36583,.T.);
#49204=ORIENTED_EDGE('',*,*,#36584,.F.);
#49205=ORIENTED_EDGE('',*,*,#36218,.T.);
#49206=ORIENTED_EDGE('',*,*,#36584,.T.);
#49207=ORIENTED_EDGE('',*,*,#36585,.T.);
#49208=ORIENTED_EDGE('',*,*,#36586,.F.);
#49209=ORIENTED_EDGE('',*,*,#36585,.F.);
#49210=ORIENTED_EDGE('',*,*,#36583,.F.);
#49211=ORIENTED_EDGE('',*,*,#36587,.F.);
#49212=ORIENTED_EDGE('',*,*,#36588,.F.);
#49213=ORIENTED_EDGE('',*,*,#36220,.T.);
#49214=ORIENTED_EDGE('',*,*,#36589,.F.);
#49215=ORIENTED_EDGE('',*,*,#36590,.T.);
#49216=ORIENTED_EDGE('',*,*,#36591,.F.);
#49217=ORIENTED_EDGE('',*,*,#36221,.T.);
#49218=ORIENTED_EDGE('',*,*,#36591,.T.);
#49219=ORIENTED_EDGE('',*,*,#36592,.T.);
#49220=ORIENTED_EDGE('',*,*,#36593,.F.);
#49221=ORIENTED_EDGE('',*,*,#36592,.F.);
#49222=ORIENTED_EDGE('',*,*,#36590,.F.);
#49223=ORIENTED_EDGE('',*,*,#36594,.F.);
#49224=ORIENTED_EDGE('',*,*,#36595,.F.);
#49225=ORIENTED_EDGE('',*,*,#36223,.T.);
#49226=ORIENTED_EDGE('',*,*,#36596,.F.);
#49227=ORIENTED_EDGE('',*,*,#36597,.T.);
#49228=ORIENTED_EDGE('',*,*,#36598,.F.);
#49229=ORIENTED_EDGE('',*,*,#36224,.T.);
#49230=ORIENTED_EDGE('',*,*,#36598,.T.);
#49231=ORIENTED_EDGE('',*,*,#36599,.T.);
#49232=ORIENTED_EDGE('',*,*,#36600,.F.);
#49233=ORIENTED_EDGE('',*,*,#36599,.F.);
#49234=ORIENTED_EDGE('',*,*,#36597,.F.);
#49235=ORIENTED_EDGE('',*,*,#36601,.F.);
#49236=ORIENTED_EDGE('',*,*,#36602,.F.);
#49237=ORIENTED_EDGE('',*,*,#36226,.T.);
#49238=ORIENTED_EDGE('',*,*,#36603,.F.);
#49239=ORIENTED_EDGE('',*,*,#36604,.T.);
#49240=ORIENTED_EDGE('',*,*,#36605,.F.);
#49241=ORIENTED_EDGE('',*,*,#36227,.T.);
#49242=ORIENTED_EDGE('',*,*,#36605,.T.);
#49243=ORIENTED_EDGE('',*,*,#36606,.T.);
#49244=ORIENTED_EDGE('',*,*,#36607,.F.);
#49245=ORIENTED_EDGE('',*,*,#36606,.F.);
#49246=ORIENTED_EDGE('',*,*,#36604,.F.);
#49247=ORIENTED_EDGE('',*,*,#36608,.F.);
#49248=ORIENTED_EDGE('',*,*,#36609,.F.);
#49249=ORIENTED_EDGE('',*,*,#36229,.T.);
#49250=ORIENTED_EDGE('',*,*,#36610,.F.);
#49251=ORIENTED_EDGE('',*,*,#36611,.T.);
#49252=ORIENTED_EDGE('',*,*,#36612,.F.);
#49253=ORIENTED_EDGE('',*,*,#36230,.T.);
#49254=ORIENTED_EDGE('',*,*,#36612,.T.);
#49255=ORIENTED_EDGE('',*,*,#36613,.T.);
#49256=ORIENTED_EDGE('',*,*,#36614,.F.);
#49257=ORIENTED_EDGE('',*,*,#36613,.F.);
#49258=ORIENTED_EDGE('',*,*,#36611,.F.);
#49259=ORIENTED_EDGE('',*,*,#36615,.F.);
#49260=ORIENTED_EDGE('',*,*,#36616,.F.);
#49261=ORIENTED_EDGE('',*,*,#36232,.T.);
#49262=ORIENTED_EDGE('',*,*,#36617,.F.);
#49263=ORIENTED_EDGE('',*,*,#36618,.T.);
#49264=ORIENTED_EDGE('',*,*,#36619,.F.);
#49265=ORIENTED_EDGE('',*,*,#36233,.T.);
#49266=ORIENTED_EDGE('',*,*,#36619,.T.);
#49267=ORIENTED_EDGE('',*,*,#36620,.T.);
#49268=ORIENTED_EDGE('',*,*,#36621,.F.);
#49269=ORIENTED_EDGE('',*,*,#36620,.F.);
#49270=ORIENTED_EDGE('',*,*,#36618,.F.);
#49271=ORIENTED_EDGE('',*,*,#36622,.F.);
#49272=ORIENTED_EDGE('',*,*,#36623,.F.);
#49273=ORIENTED_EDGE('',*,*,#36235,.T.);
#49274=ORIENTED_EDGE('',*,*,#36624,.F.);
#49275=ORIENTED_EDGE('',*,*,#36625,.T.);
#49276=ORIENTED_EDGE('',*,*,#36626,.F.);
#49277=ORIENTED_EDGE('',*,*,#36236,.T.);
#49278=ORIENTED_EDGE('',*,*,#36626,.T.);
#49279=ORIENTED_EDGE('',*,*,#36627,.T.);
#49280=ORIENTED_EDGE('',*,*,#36628,.F.);
#49281=ORIENTED_EDGE('',*,*,#36627,.F.);
#49282=ORIENTED_EDGE('',*,*,#36625,.F.);
#49283=ORIENTED_EDGE('',*,*,#36629,.F.);
#49284=ORIENTED_EDGE('',*,*,#36630,.F.);
#49285=ORIENTED_EDGE('',*,*,#36238,.T.);
#49286=ORIENTED_EDGE('',*,*,#36631,.F.);
#49287=ORIENTED_EDGE('',*,*,#36632,.T.);
#49288=ORIENTED_EDGE('',*,*,#36633,.F.);
#49289=ORIENTED_EDGE('',*,*,#36239,.T.);
#49290=ORIENTED_EDGE('',*,*,#36633,.T.);
#49291=ORIENTED_EDGE('',*,*,#36634,.T.);
#49292=ORIENTED_EDGE('',*,*,#36635,.F.);
#49293=ORIENTED_EDGE('',*,*,#36634,.F.);
#49294=ORIENTED_EDGE('',*,*,#36632,.F.);
#49295=ORIENTED_EDGE('',*,*,#36636,.F.);
#49296=ORIENTED_EDGE('',*,*,#36637,.F.);
#49297=ORIENTED_EDGE('',*,*,#36241,.T.);
#49298=ORIENTED_EDGE('',*,*,#36638,.F.);
#49299=ORIENTED_EDGE('',*,*,#36639,.T.);
#49300=ORIENTED_EDGE('',*,*,#36640,.F.);
#49301=ORIENTED_EDGE('',*,*,#36242,.T.);
#49302=ORIENTED_EDGE('',*,*,#36640,.T.);
#49303=ORIENTED_EDGE('',*,*,#36641,.T.);
#49304=ORIENTED_EDGE('',*,*,#36642,.F.);
#49305=ORIENTED_EDGE('',*,*,#36641,.F.);
#49306=ORIENTED_EDGE('',*,*,#36639,.F.);
#49307=ORIENTED_EDGE('',*,*,#36643,.F.);
#49308=ORIENTED_EDGE('',*,*,#36644,.F.);
#49309=ORIENTED_EDGE('',*,*,#36645,.F.);
#49310=ORIENTED_EDGE('',*,*,#36646,.F.);
#49311=ORIENTED_EDGE('',*,*,#36246,.T.);
#49312=ORIENTED_EDGE('',*,*,#36245,.T.);
#49313=ORIENTED_EDGE('',*,*,#36647,.F.);
#49314=ORIENTED_EDGE('',*,*,#36249,.T.);
#49315=ORIENTED_EDGE('',*,*,#36247,.T.);
#49316=ORIENTED_EDGE('',*,*,#36646,.T.);
#49317=ORIENTED_EDGE('',*,*,#36648,.F.);
#49318=ORIENTED_EDGE('',*,*,#36649,.F.);
#49319=ORIENTED_EDGE('',*,*,#36253,.T.);
#49320=ORIENTED_EDGE('',*,*,#36252,.T.);
#49321=ORIENTED_EDGE('',*,*,#36650,.F.);
#49322=ORIENTED_EDGE('',*,*,#36256,.T.);
#49323=ORIENTED_EDGE('',*,*,#36254,.T.);
#49324=ORIENTED_EDGE('',*,*,#36649,.T.);
#49325=ORIENTED_EDGE('',*,*,#36651,.F.);
#49326=ORIENTED_EDGE('',*,*,#36652,.F.);
#49327=ORIENTED_EDGE('',*,*,#36260,.T.);
#49328=ORIENTED_EDGE('',*,*,#36259,.T.);
#49329=ORIENTED_EDGE('',*,*,#36653,.F.);
#49330=ORIENTED_EDGE('',*,*,#36263,.T.);
#49331=ORIENTED_EDGE('',*,*,#36261,.T.);
#49332=ORIENTED_EDGE('',*,*,#36652,.T.);
#49333=ORIENTED_EDGE('',*,*,#36654,.F.);
#49334=ORIENTED_EDGE('',*,*,#36655,.F.);
#49335=ORIENTED_EDGE('',*,*,#36267,.T.);
#49336=ORIENTED_EDGE('',*,*,#36266,.T.);
#49337=ORIENTED_EDGE('',*,*,#36656,.F.);
#49338=ORIENTED_EDGE('',*,*,#36270,.T.);
#49339=ORIENTED_EDGE('',*,*,#36268,.T.);
#49340=ORIENTED_EDGE('',*,*,#36655,.T.);
#49341=ORIENTED_EDGE('',*,*,#36657,.F.);
#49342=ORIENTED_EDGE('',*,*,#36658,.F.);
#49343=ORIENTED_EDGE('',*,*,#36274,.T.);
#49344=ORIENTED_EDGE('',*,*,#36273,.T.);
#49345=ORIENTED_EDGE('',*,*,#36659,.F.);
#49346=ORIENTED_EDGE('',*,*,#36277,.T.);
#49347=ORIENTED_EDGE('',*,*,#36275,.T.);
#49348=ORIENTED_EDGE('',*,*,#36658,.T.);
#49349=ORIENTED_EDGE('',*,*,#36660,.F.);
#49350=ORIENTED_EDGE('',*,*,#36661,.F.);
#49351=ORIENTED_EDGE('',*,*,#36281,.T.);
#49352=ORIENTED_EDGE('',*,*,#36280,.T.);
#49353=ORIENTED_EDGE('',*,*,#36662,.F.);
#49354=ORIENTED_EDGE('',*,*,#36284,.T.);
#49355=ORIENTED_EDGE('',*,*,#36282,.T.);
#49356=ORIENTED_EDGE('',*,*,#36661,.T.);
#49357=ORIENTED_EDGE('',*,*,#36663,.F.);
#49358=ORIENTED_EDGE('',*,*,#36664,.F.);
#49359=ORIENTED_EDGE('',*,*,#36288,.T.);
#49360=ORIENTED_EDGE('',*,*,#36287,.T.);
#49361=ORIENTED_EDGE('',*,*,#36665,.F.);
#49362=ORIENTED_EDGE('',*,*,#36291,.T.);
#49363=ORIENTED_EDGE('',*,*,#36289,.T.);
#49364=ORIENTED_EDGE('',*,*,#36664,.T.);
#49365=ORIENTED_EDGE('',*,*,#36666,.F.);
#49366=ORIENTED_EDGE('',*,*,#36667,.F.);
#49367=ORIENTED_EDGE('',*,*,#36295,.T.);
#49368=ORIENTED_EDGE('',*,*,#36294,.T.);
#49369=ORIENTED_EDGE('',*,*,#36668,.F.);
#49370=ORIENTED_EDGE('',*,*,#36298,.T.);
#49371=ORIENTED_EDGE('',*,*,#36296,.T.);
#49372=ORIENTED_EDGE('',*,*,#36667,.T.);
#49373=ORIENTED_EDGE('',*,*,#36669,.F.);
#49374=ORIENTED_EDGE('',*,*,#36670,.F.);
#49375=ORIENTED_EDGE('',*,*,#36302,.T.);
#49376=ORIENTED_EDGE('',*,*,#36301,.T.);
#49377=ORIENTED_EDGE('',*,*,#36671,.F.);
#49378=ORIENTED_EDGE('',*,*,#36305,.T.);
#49379=ORIENTED_EDGE('',*,*,#36303,.T.);
#49380=ORIENTED_EDGE('',*,*,#36670,.T.);
#49381=ORIENTED_EDGE('',*,*,#36672,.F.);
#49382=ORIENTED_EDGE('',*,*,#36673,.F.);
#49383=ORIENTED_EDGE('',*,*,#36309,.T.);
#49384=ORIENTED_EDGE('',*,*,#36308,.T.);
#49385=ORIENTED_EDGE('',*,*,#36674,.F.);
#49386=ORIENTED_EDGE('',*,*,#36312,.T.);
#49387=ORIENTED_EDGE('',*,*,#36310,.T.);
#49388=ORIENTED_EDGE('',*,*,#36673,.T.);
#49389=ORIENTED_EDGE('',*,*,#36675,.F.);
#49390=ORIENTED_EDGE('',*,*,#36676,.F.);
#49391=ORIENTED_EDGE('',*,*,#36316,.T.);
#49392=ORIENTED_EDGE('',*,*,#36315,.T.);
#49393=ORIENTED_EDGE('',*,*,#36677,.F.);
#49394=ORIENTED_EDGE('',*,*,#36319,.T.);
#49395=ORIENTED_EDGE('',*,*,#36317,.T.);
#49396=ORIENTED_EDGE('',*,*,#36676,.T.);
#49397=ORIENTED_EDGE('',*,*,#36678,.F.);
#49398=ORIENTED_EDGE('',*,*,#36679,.F.);
#49399=ORIENTED_EDGE('',*,*,#36323,.T.);
#49400=ORIENTED_EDGE('',*,*,#36322,.T.);
#49401=ORIENTED_EDGE('',*,*,#36680,.F.);
#49402=ORIENTED_EDGE('',*,*,#36326,.T.);
#49403=ORIENTED_EDGE('',*,*,#36324,.T.);
#49404=ORIENTED_EDGE('',*,*,#36679,.T.);
#49405=ORIENTED_EDGE('',*,*,#36681,.F.);
#49406=ORIENTED_EDGE('',*,*,#36682,.F.);
#49407=ORIENTED_EDGE('',*,*,#36330,.T.);
#49408=ORIENTED_EDGE('',*,*,#36329,.T.);
#49409=ORIENTED_EDGE('',*,*,#36683,.F.);
#49410=ORIENTED_EDGE('',*,*,#36333,.T.);
#49411=ORIENTED_EDGE('',*,*,#36331,.T.);
#49412=ORIENTED_EDGE('',*,*,#36682,.T.);
#49413=ORIENTED_EDGE('',*,*,#36684,.F.);
#49414=ORIENTED_EDGE('',*,*,#36685,.F.);
#49415=ORIENTED_EDGE('',*,*,#36337,.T.);
#49416=ORIENTED_EDGE('',*,*,#36336,.T.);
#49417=ORIENTED_EDGE('',*,*,#36686,.F.);
#49418=ORIENTED_EDGE('',*,*,#36340,.T.);
#49419=ORIENTED_EDGE('',*,*,#36338,.T.);
#49420=ORIENTED_EDGE('',*,*,#36685,.T.);
#49421=ORIENTED_EDGE('',*,*,#36687,.F.);
#49422=ORIENTED_EDGE('',*,*,#36688,.F.);
#49423=ORIENTED_EDGE('',*,*,#34442,.T.);
#49424=ORIENTED_EDGE('',*,*,#36342,.T.);
#49425=ORIENTED_EDGE('',*,*,#36689,.F.);
#49426=ORIENTED_EDGE('',*,*,#36343,.T.);
#49427=ORIENTED_EDGE('',*,*,#34443,.T.);
#49428=ORIENTED_EDGE('',*,*,#36688,.T.);
#49429=ORIENTED_EDGE('',*,*,#36690,.F.);
#49430=ORIENTED_EDGE('',*,*,#36691,.F.);
#49431=ORIENTED_EDGE('',*,*,#36347,.T.);
#49432=ORIENTED_EDGE('',*,*,#36346,.T.);
#49433=ORIENTED_EDGE('',*,*,#36692,.F.);
#49434=ORIENTED_EDGE('',*,*,#36350,.T.);
#49435=ORIENTED_EDGE('',*,*,#36348,.T.);
#49436=ORIENTED_EDGE('',*,*,#36691,.T.);
#49437=ORIENTED_EDGE('',*,*,#36693,.F.);
#49438=ORIENTED_EDGE('',*,*,#36694,.F.);
#49439=ORIENTED_EDGE('',*,*,#36354,.T.);
#49440=ORIENTED_EDGE('',*,*,#36353,.T.);
#49441=ORIENTED_EDGE('',*,*,#36695,.F.);
#49442=ORIENTED_EDGE('',*,*,#36357,.T.);
#49443=ORIENTED_EDGE('',*,*,#36355,.T.);
#49444=ORIENTED_EDGE('',*,*,#36694,.T.);
#49445=ORIENTED_EDGE('',*,*,#36696,.F.);
#49446=ORIENTED_EDGE('',*,*,#36697,.F.);
#49447=ORIENTED_EDGE('',*,*,#36361,.T.);
#49448=ORIENTED_EDGE('',*,*,#36360,.T.);
#49449=ORIENTED_EDGE('',*,*,#36698,.F.);
#49450=ORIENTED_EDGE('',*,*,#36364,.T.);
#49451=ORIENTED_EDGE('',*,*,#36362,.T.);
#49452=ORIENTED_EDGE('',*,*,#36697,.T.);
#49453=ORIENTED_EDGE('',*,*,#36699,.F.);
#49454=ORIENTED_EDGE('',*,*,#36700,.F.);
#49455=ORIENTED_EDGE('',*,*,#36368,.T.);
#49456=ORIENTED_EDGE('',*,*,#36367,.T.);
#49457=ORIENTED_EDGE('',*,*,#36701,.F.);
#49458=ORIENTED_EDGE('',*,*,#36371,.T.);
#49459=ORIENTED_EDGE('',*,*,#36369,.T.);
#49460=ORIENTED_EDGE('',*,*,#36700,.T.);
#49461=ORIENTED_EDGE('',*,*,#36702,.F.);
#49462=ORIENTED_EDGE('',*,*,#36703,.F.);
#49463=ORIENTED_EDGE('',*,*,#36375,.T.);
#49464=ORIENTED_EDGE('',*,*,#36374,.T.);
#49465=ORIENTED_EDGE('',*,*,#36704,.F.);
#49466=ORIENTED_EDGE('',*,*,#36378,.T.);
#49467=ORIENTED_EDGE('',*,*,#36376,.T.);
#49468=ORIENTED_EDGE('',*,*,#36703,.T.);
#49469=ORIENTED_EDGE('',*,*,#36705,.F.);
#49470=ORIENTED_EDGE('',*,*,#36706,.F.);
#49471=ORIENTED_EDGE('',*,*,#36382,.T.);
#49472=ORIENTED_EDGE('',*,*,#36381,.T.);
#49473=ORIENTED_EDGE('',*,*,#36707,.F.);
#49474=ORIENTED_EDGE('',*,*,#36385,.T.);
#49475=ORIENTED_EDGE('',*,*,#36383,.T.);
#49476=ORIENTED_EDGE('',*,*,#36706,.T.);
#49477=ORIENTED_EDGE('',*,*,#36708,.F.);
#49478=ORIENTED_EDGE('',*,*,#36709,.F.);
#49479=ORIENTED_EDGE('',*,*,#36389,.T.);
#49480=ORIENTED_EDGE('',*,*,#36388,.T.);
#49481=ORIENTED_EDGE('',*,*,#36710,.F.);
#49482=ORIENTED_EDGE('',*,*,#36392,.T.);
#49483=ORIENTED_EDGE('',*,*,#36390,.T.);
#49484=ORIENTED_EDGE('',*,*,#36709,.T.);
#49485=ORIENTED_EDGE('',*,*,#36711,.F.);
#49486=ORIENTED_EDGE('',*,*,#36712,.F.);
#49487=ORIENTED_EDGE('',*,*,#36396,.T.);
#49488=ORIENTED_EDGE('',*,*,#36395,.T.);
#49489=ORIENTED_EDGE('',*,*,#36713,.F.);
#49490=ORIENTED_EDGE('',*,*,#36399,.T.);
#49491=ORIENTED_EDGE('',*,*,#36397,.T.);
#49492=ORIENTED_EDGE('',*,*,#36712,.T.);
#49493=ORIENTED_EDGE('',*,*,#36714,.F.);
#49494=ORIENTED_EDGE('',*,*,#36715,.F.);
#49495=ORIENTED_EDGE('',*,*,#36405,.T.);
#49496=ORIENTED_EDGE('',*,*,#36402,.T.);
#49497=ORIENTED_EDGE('',*,*,#36406,.T.);
#49498=ORIENTED_EDGE('',*,*,#36715,.T.);
#49499=ORIENTED_EDGE('',*,*,#36716,.F.);
#49500=ORIENTED_EDGE('',*,*,#36404,.T.);
#49501=ORIENTED_EDGE('',*,*,#36411,.T.);
#49502=ORIENTED_EDGE('',*,*,#36407,.T.);
#49503=ORIENTED_EDGE('',*,*,#36717,.F.);
#49504=ORIENTED_EDGE('',*,*,#36718,.F.);
#49505=ORIENTED_EDGE('',*,*,#36719,.F.);
#49506=ORIENTED_EDGE('',*,*,#36413,.T.);
#49507=ORIENTED_EDGE('',*,*,#36412,.T.);
#49508=ORIENTED_EDGE('',*,*,#36718,.T.);
#49509=ORIENTED_EDGE('',*,*,#36720,.F.);
#49510=ORIENTED_EDGE('',*,*,#36721,.F.);
#49511=ORIENTED_EDGE('',*,*,#36417,.T.);
#49512=ORIENTED_EDGE('',*,*,#36416,.T.);
#49513=ORIENTED_EDGE('',*,*,#36722,.F.);
#49514=ORIENTED_EDGE('',*,*,#36420,.T.);
#49515=ORIENTED_EDGE('',*,*,#36418,.T.);
#49516=ORIENTED_EDGE('',*,*,#36721,.T.);
#49517=ORIENTED_EDGE('',*,*,#36723,.F.);
#49518=ORIENTED_EDGE('',*,*,#36724,.F.);
#49519=ORIENTED_EDGE('',*,*,#36424,.T.);
#49520=ORIENTED_EDGE('',*,*,#36423,.T.);
#49521=ORIENTED_EDGE('',*,*,#36725,.F.);
#49522=ORIENTED_EDGE('',*,*,#36427,.T.);
#49523=ORIENTED_EDGE('',*,*,#36425,.T.);
#49524=ORIENTED_EDGE('',*,*,#36724,.T.);
#49525=ORIENTED_EDGE('',*,*,#36726,.F.);
#49526=ORIENTED_EDGE('',*,*,#36727,.F.);
#49527=ORIENTED_EDGE('',*,*,#36431,.T.);
#49528=ORIENTED_EDGE('',*,*,#36430,.T.);
#49529=ORIENTED_EDGE('',*,*,#36728,.F.);
#49530=ORIENTED_EDGE('',*,*,#36434,.T.);
#49531=ORIENTED_EDGE('',*,*,#36432,.T.);
#49532=ORIENTED_EDGE('',*,*,#36727,.T.);
#49533=ORIENTED_EDGE('',*,*,#36729,.F.);
#49534=ORIENTED_EDGE('',*,*,#36730,.F.);
#49535=ORIENTED_EDGE('',*,*,#36438,.T.);
#49536=ORIENTED_EDGE('',*,*,#36437,.T.);
#49537=ORIENTED_EDGE('',*,*,#36731,.F.);
#49538=ORIENTED_EDGE('',*,*,#36441,.T.);
#49539=ORIENTED_EDGE('',*,*,#36439,.T.);
#49540=ORIENTED_EDGE('',*,*,#36730,.T.);
#49541=ORIENTED_EDGE('',*,*,#36732,.F.);
#49542=ORIENTED_EDGE('',*,*,#36733,.F.);
#49543=ORIENTED_EDGE('',*,*,#36447,.T.);
#49544=ORIENTED_EDGE('',*,*,#36442,.T.);
#49545=ORIENTED_EDGE('',*,*,#36448,.T.);
#49546=ORIENTED_EDGE('',*,*,#36733,.T.);
#49547=ORIENTED_EDGE('',*,*,#36734,.F.);
#49548=ORIENTED_EDGE('',*,*,#36446,.T.);
#49549=ORIENTED_EDGE('',*,*,#36454,.T.);
#49550=ORIENTED_EDGE('',*,*,#36449,.T.);
#49551=ORIENTED_EDGE('',*,*,#36735,.F.);
#49552=ORIENTED_EDGE('',*,*,#36736,.F.);
#49553=ORIENTED_EDGE('',*,*,#36455,.T.);
#49554=ORIENTED_EDGE('',*,*,#36736,.T.);
#49555=ORIENTED_EDGE('',*,*,#36737,.F.);
#49556=ORIENTED_EDGE('',*,*,#36453,.T.);
#49557=ORIENTED_EDGE('',*,*,#36461,.T.);
#49558=ORIENTED_EDGE('',*,*,#36456,.T.);
#49559=ORIENTED_EDGE('',*,*,#36738,.F.);
#49560=ORIENTED_EDGE('',*,*,#36739,.F.);
#49561=ORIENTED_EDGE('',*,*,#36462,.T.);
#49562=ORIENTED_EDGE('',*,*,#36739,.T.);
#49563=ORIENTED_EDGE('',*,*,#36740,.F.);
#49564=ORIENTED_EDGE('',*,*,#36460,.T.);
#49565=ORIENTED_EDGE('',*,*,#36468,.T.);
#49566=ORIENTED_EDGE('',*,*,#36463,.T.);
#49567=ORIENTED_EDGE('',*,*,#36741,.F.);
#49568=ORIENTED_EDGE('',*,*,#36742,.F.);
#49569=ORIENTED_EDGE('',*,*,#36469,.T.);
#49570=ORIENTED_EDGE('',*,*,#36742,.T.);
#49571=ORIENTED_EDGE('',*,*,#36743,.F.);
#49572=ORIENTED_EDGE('',*,*,#36467,.T.);
#49573=ORIENTED_EDGE('',*,*,#36475,.T.);
#49574=ORIENTED_EDGE('',*,*,#36470,.T.);
#49575=ORIENTED_EDGE('',*,*,#36744,.F.);
#49576=ORIENTED_EDGE('',*,*,#36745,.F.);
#49577=ORIENTED_EDGE('',*,*,#36476,.T.);
#49578=ORIENTED_EDGE('',*,*,#36745,.T.);
#49579=ORIENTED_EDGE('',*,*,#36746,.F.);
#49580=ORIENTED_EDGE('',*,*,#36474,.T.);
#49581=ORIENTED_EDGE('',*,*,#36482,.T.);
#49582=ORIENTED_EDGE('',*,*,#36477,.T.);
#49583=ORIENTED_EDGE('',*,*,#36747,.F.);
#49584=ORIENTED_EDGE('',*,*,#36748,.F.);
#49585=ORIENTED_EDGE('',*,*,#36483,.T.);
#49586=ORIENTED_EDGE('',*,*,#36748,.T.);
#49587=ORIENTED_EDGE('',*,*,#36749,.F.);
#49588=ORIENTED_EDGE('',*,*,#36481,.T.);
#49589=ORIENTED_EDGE('',*,*,#36489,.T.);
#49590=ORIENTED_EDGE('',*,*,#36484,.T.);
#49591=ORIENTED_EDGE('',*,*,#36750,.F.);
#49592=ORIENTED_EDGE('',*,*,#36751,.F.);
#49593=ORIENTED_EDGE('',*,*,#36490,.T.);
#49594=ORIENTED_EDGE('',*,*,#36751,.T.);
#49595=ORIENTED_EDGE('',*,*,#36752,.F.);
#49596=ORIENTED_EDGE('',*,*,#36488,.T.);
#49597=ORIENTED_EDGE('',*,*,#36496,.T.);
#49598=ORIENTED_EDGE('',*,*,#36491,.T.);
#49599=ORIENTED_EDGE('',*,*,#36753,.F.);
#49600=ORIENTED_EDGE('',*,*,#36754,.F.);
#49601=ORIENTED_EDGE('',*,*,#36497,.T.);
#49602=ORIENTED_EDGE('',*,*,#36754,.T.);
#49603=ORIENTED_EDGE('',*,*,#36755,.F.);
#49604=ORIENTED_EDGE('',*,*,#36495,.T.);
#49605=ORIENTED_EDGE('',*,*,#36503,.T.);
#49606=ORIENTED_EDGE('',*,*,#36498,.T.);
#49607=ORIENTED_EDGE('',*,*,#36756,.F.);
#49608=ORIENTED_EDGE('',*,*,#36757,.F.);
#49609=ORIENTED_EDGE('',*,*,#36504,.T.);
#49610=ORIENTED_EDGE('',*,*,#36757,.T.);
#49611=ORIENTED_EDGE('',*,*,#36758,.F.);
#49612=ORIENTED_EDGE('',*,*,#36502,.T.);
#49613=ORIENTED_EDGE('',*,*,#36510,.T.);
#49614=ORIENTED_EDGE('',*,*,#36505,.T.);
#49615=ORIENTED_EDGE('',*,*,#36759,.F.);
#49616=ORIENTED_EDGE('',*,*,#36760,.F.);
#49617=ORIENTED_EDGE('',*,*,#36511,.T.);
#49618=ORIENTED_EDGE('',*,*,#36760,.T.);
#49619=ORIENTED_EDGE('',*,*,#36761,.F.);
#49620=ORIENTED_EDGE('',*,*,#36509,.T.);
#49621=ORIENTED_EDGE('',*,*,#36517,.T.);
#49622=ORIENTED_EDGE('',*,*,#36512,.T.);
#49623=ORIENTED_EDGE('',*,*,#36762,.F.);
#49624=ORIENTED_EDGE('',*,*,#36763,.F.);
#49625=ORIENTED_EDGE('',*,*,#36518,.T.);
#49626=ORIENTED_EDGE('',*,*,#36763,.T.);
#49627=ORIENTED_EDGE('',*,*,#36764,.F.);
#49628=ORIENTED_EDGE('',*,*,#36516,.T.);
#49629=ORIENTED_EDGE('',*,*,#36524,.T.);
#49630=ORIENTED_EDGE('',*,*,#36519,.T.);
#49631=ORIENTED_EDGE('',*,*,#36765,.F.);
#49632=ORIENTED_EDGE('',*,*,#36766,.F.);
#49633=ORIENTED_EDGE('',*,*,#36525,.T.);
#49634=ORIENTED_EDGE('',*,*,#36766,.T.);
#49635=ORIENTED_EDGE('',*,*,#36767,.F.);
#49636=ORIENTED_EDGE('',*,*,#36523,.T.);
#49637=ORIENTED_EDGE('',*,*,#36531,.T.);
#49638=ORIENTED_EDGE('',*,*,#36526,.T.);
#49639=ORIENTED_EDGE('',*,*,#36768,.F.);
#49640=ORIENTED_EDGE('',*,*,#36769,.F.);
#49641=ORIENTED_EDGE('',*,*,#36532,.T.);
#49642=ORIENTED_EDGE('',*,*,#36769,.T.);
#49643=ORIENTED_EDGE('',*,*,#36770,.F.);
#49644=ORIENTED_EDGE('',*,*,#36530,.T.);
#49645=ORIENTED_EDGE('',*,*,#36538,.T.);
#49646=ORIENTED_EDGE('',*,*,#36533,.T.);
#49647=ORIENTED_EDGE('',*,*,#36771,.F.);
#49648=ORIENTED_EDGE('',*,*,#36772,.F.);
#49649=ORIENTED_EDGE('',*,*,#36539,.T.);
#49650=ORIENTED_EDGE('',*,*,#36772,.T.);
#49651=ORIENTED_EDGE('',*,*,#36773,.F.);
#49652=ORIENTED_EDGE('',*,*,#36537,.T.);
#49653=ORIENTED_EDGE('',*,*,#36545,.T.);
#49654=ORIENTED_EDGE('',*,*,#36540,.T.);
#49655=ORIENTED_EDGE('',*,*,#36774,.F.);
#49656=ORIENTED_EDGE('',*,*,#36775,.F.);
#49657=ORIENTED_EDGE('',*,*,#36546,.T.);
#49658=ORIENTED_EDGE('',*,*,#36775,.T.);
#49659=ORIENTED_EDGE('',*,*,#36776,.F.);
#49660=ORIENTED_EDGE('',*,*,#36544,.T.);
#49661=ORIENTED_EDGE('',*,*,#36552,.T.);
#49662=ORIENTED_EDGE('',*,*,#36547,.T.);
#49663=ORIENTED_EDGE('',*,*,#36777,.F.);
#49664=ORIENTED_EDGE('',*,*,#36778,.F.);
#49665=ORIENTED_EDGE('',*,*,#36553,.T.);
#49666=ORIENTED_EDGE('',*,*,#36778,.T.);
#49667=ORIENTED_EDGE('',*,*,#36779,.F.);
#49668=ORIENTED_EDGE('',*,*,#36551,.T.);
#49669=ORIENTED_EDGE('',*,*,#36559,.T.);
#49670=ORIENTED_EDGE('',*,*,#36554,.T.);
#49671=ORIENTED_EDGE('',*,*,#36780,.F.);
#49672=ORIENTED_EDGE('',*,*,#36781,.F.);
#49673=ORIENTED_EDGE('',*,*,#36560,.T.);
#49674=ORIENTED_EDGE('',*,*,#36781,.T.);
#49675=ORIENTED_EDGE('',*,*,#36782,.F.);
#49676=ORIENTED_EDGE('',*,*,#36558,.T.);
#49677=ORIENTED_EDGE('',*,*,#36566,.T.);
#49678=ORIENTED_EDGE('',*,*,#36561,.T.);
#49679=ORIENTED_EDGE('',*,*,#36783,.F.);
#49680=ORIENTED_EDGE('',*,*,#36784,.F.);
#49681=ORIENTED_EDGE('',*,*,#36567,.T.);
#49682=ORIENTED_EDGE('',*,*,#36784,.T.);
#49683=ORIENTED_EDGE('',*,*,#36785,.F.);
#49684=ORIENTED_EDGE('',*,*,#36565,.T.);
#49685=ORIENTED_EDGE('',*,*,#36573,.T.);
#49686=ORIENTED_EDGE('',*,*,#36568,.T.);
#49687=ORIENTED_EDGE('',*,*,#36786,.F.);
#49688=ORIENTED_EDGE('',*,*,#36787,.F.);
#49689=ORIENTED_EDGE('',*,*,#36574,.T.);
#49690=ORIENTED_EDGE('',*,*,#36787,.T.);
#49691=ORIENTED_EDGE('',*,*,#36788,.F.);
#49692=ORIENTED_EDGE('',*,*,#36572,.T.);
#49693=ORIENTED_EDGE('',*,*,#36580,.T.);
#49694=ORIENTED_EDGE('',*,*,#36575,.T.);
#49695=ORIENTED_EDGE('',*,*,#36789,.F.);
#49696=ORIENTED_EDGE('',*,*,#36790,.F.);
#49697=ORIENTED_EDGE('',*,*,#36581,.T.);
#49698=ORIENTED_EDGE('',*,*,#36790,.T.);
#49699=ORIENTED_EDGE('',*,*,#36791,.F.);
#49700=ORIENTED_EDGE('',*,*,#36579,.T.);
#49701=ORIENTED_EDGE('',*,*,#36587,.T.);
#49702=ORIENTED_EDGE('',*,*,#36582,.T.);
#49703=ORIENTED_EDGE('',*,*,#36792,.F.);
#49704=ORIENTED_EDGE('',*,*,#36793,.F.);
#49705=ORIENTED_EDGE('',*,*,#36588,.T.);
#49706=ORIENTED_EDGE('',*,*,#36793,.T.);
#49707=ORIENTED_EDGE('',*,*,#36794,.F.);
#49708=ORIENTED_EDGE('',*,*,#36586,.T.);
#49709=ORIENTED_EDGE('',*,*,#36594,.T.);
#49710=ORIENTED_EDGE('',*,*,#36589,.T.);
#49711=ORIENTED_EDGE('',*,*,#36795,.F.);
#49712=ORIENTED_EDGE('',*,*,#36796,.F.);
#49713=ORIENTED_EDGE('',*,*,#36595,.T.);
#49714=ORIENTED_EDGE('',*,*,#36796,.T.);
#49715=ORIENTED_EDGE('',*,*,#36797,.F.);
#49716=ORIENTED_EDGE('',*,*,#36593,.T.);
#49717=ORIENTED_EDGE('',*,*,#36601,.T.);
#49718=ORIENTED_EDGE('',*,*,#36596,.T.);
#49719=ORIENTED_EDGE('',*,*,#36798,.F.);
#49720=ORIENTED_EDGE('',*,*,#36799,.F.);
#49721=ORIENTED_EDGE('',*,*,#36602,.T.);
#49722=ORIENTED_EDGE('',*,*,#36799,.T.);
#49723=ORIENTED_EDGE('',*,*,#36800,.F.);
#49724=ORIENTED_EDGE('',*,*,#36600,.T.);
#49725=ORIENTED_EDGE('',*,*,#36608,.T.);
#49726=ORIENTED_EDGE('',*,*,#36603,.T.);
#49727=ORIENTED_EDGE('',*,*,#36801,.F.);
#49728=ORIENTED_EDGE('',*,*,#36802,.F.);
#49729=ORIENTED_EDGE('',*,*,#36609,.T.);
#49730=ORIENTED_EDGE('',*,*,#36802,.T.);
#49731=ORIENTED_EDGE('',*,*,#36803,.F.);
#49732=ORIENTED_EDGE('',*,*,#36607,.T.);
#49733=ORIENTED_EDGE('',*,*,#36615,.T.);
#49734=ORIENTED_EDGE('',*,*,#36610,.T.);
#49735=ORIENTED_EDGE('',*,*,#36804,.F.);
#49736=ORIENTED_EDGE('',*,*,#36805,.F.);
#49737=ORIENTED_EDGE('',*,*,#36616,.T.);
#49738=ORIENTED_EDGE('',*,*,#36805,.T.);
#49739=ORIENTED_EDGE('',*,*,#36806,.F.);
#49740=ORIENTED_EDGE('',*,*,#36614,.T.);
#49741=ORIENTED_EDGE('',*,*,#36622,.T.);
#49742=ORIENTED_EDGE('',*,*,#36617,.T.);
#49743=ORIENTED_EDGE('',*,*,#36807,.F.);
#49744=ORIENTED_EDGE('',*,*,#36808,.F.);
#49745=ORIENTED_EDGE('',*,*,#36623,.T.);
#49746=ORIENTED_EDGE('',*,*,#36808,.T.);
#49747=ORIENTED_EDGE('',*,*,#36809,.F.);
#49748=ORIENTED_EDGE('',*,*,#36621,.T.);
#49749=ORIENTED_EDGE('',*,*,#36629,.T.);
#49750=ORIENTED_EDGE('',*,*,#36624,.T.);
#49751=ORIENTED_EDGE('',*,*,#36810,.F.);
#49752=ORIENTED_EDGE('',*,*,#36811,.F.);
#49753=ORIENTED_EDGE('',*,*,#36630,.T.);
#49754=ORIENTED_EDGE('',*,*,#36811,.T.);
#49755=ORIENTED_EDGE('',*,*,#36812,.F.);
#49756=ORIENTED_EDGE('',*,*,#36628,.T.);
#49757=ORIENTED_EDGE('',*,*,#36636,.T.);
#49758=ORIENTED_EDGE('',*,*,#36631,.T.);
#49759=ORIENTED_EDGE('',*,*,#36813,.F.);
#49760=ORIENTED_EDGE('',*,*,#36814,.F.);
#49761=ORIENTED_EDGE('',*,*,#36637,.T.);
#49762=ORIENTED_EDGE('',*,*,#36814,.T.);
#49763=ORIENTED_EDGE('',*,*,#36815,.F.);
#49764=ORIENTED_EDGE('',*,*,#36635,.T.);
#49765=ORIENTED_EDGE('',*,*,#36643,.T.);
#49766=ORIENTED_EDGE('',*,*,#36638,.T.);
#49767=ORIENTED_EDGE('',*,*,#36816,.F.);
#49768=ORIENTED_EDGE('',*,*,#36817,.F.);
#49769=ORIENTED_EDGE('',*,*,#36644,.T.);
#49770=ORIENTED_EDGE('',*,*,#36817,.T.);
#49771=ORIENTED_EDGE('',*,*,#36818,.F.);
#49772=ORIENTED_EDGE('',*,*,#36642,.T.);
#49773=ORIENTED_EDGE('',*,*,#36819,.T.);
#49774=ORIENTED_EDGE('',*,*,#36820,.F.);
#49775=ORIENTED_EDGE('',*,*,#36645,.T.);
#49776=ORIENTED_EDGE('',*,*,#36821,.F.);
#49777=ORIENTED_EDGE('',*,*,#36822,.T.);
#49778=ORIENTED_EDGE('',*,*,#36823,.F.);
#49779=ORIENTED_EDGE('',*,*,#36647,.T.);
#49780=ORIENTED_EDGE('',*,*,#36824,.F.);
#49781=ORIENTED_EDGE('',*,*,#36825,.F.);
#49782=ORIENTED_EDGE('',*,*,#36826,.F.);
#49783=ORIENTED_EDGE('',*,*,#36827,.F.);
#49784=ORIENTED_EDGE('',*,*,#36822,.F.);
#49785=ORIENTED_EDGE('',*,*,#36827,.T.);
#49786=ORIENTED_EDGE('',*,*,#36828,.F.);
#49787=ORIENTED_EDGE('',*,*,#36648,.T.);
#49788=ORIENTED_EDGE('',*,*,#36823,.T.);
#49789=ORIENTED_EDGE('',*,*,#36829,.T.);
#49790=ORIENTED_EDGE('',*,*,#36830,.F.);
#49791=ORIENTED_EDGE('',*,*,#36650,.T.);
#49792=ORIENTED_EDGE('',*,*,#36831,.F.);
#49793=ORIENTED_EDGE('',*,*,#36832,.F.);
#49794=ORIENTED_EDGE('',*,*,#36833,.F.);
#49795=ORIENTED_EDGE('',*,*,#36834,.F.);
#49796=ORIENTED_EDGE('',*,*,#36829,.F.);
#49797=ORIENTED_EDGE('',*,*,#36834,.T.);
#49798=ORIENTED_EDGE('',*,*,#36835,.F.);
#49799=ORIENTED_EDGE('',*,*,#36651,.T.);
#49800=ORIENTED_EDGE('',*,*,#36830,.T.);
#49801=ORIENTED_EDGE('',*,*,#36836,.T.);
#49802=ORIENTED_EDGE('',*,*,#36837,.F.);
#49803=ORIENTED_EDGE('',*,*,#36653,.T.);
#49804=ORIENTED_EDGE('',*,*,#36838,.F.);
#49805=ORIENTED_EDGE('',*,*,#36839,.F.);
#49806=ORIENTED_EDGE('',*,*,#36840,.F.);
#49807=ORIENTED_EDGE('',*,*,#36841,.F.);
#49808=ORIENTED_EDGE('',*,*,#36836,.F.);
#49809=ORIENTED_EDGE('',*,*,#36841,.T.);
#49810=ORIENTED_EDGE('',*,*,#36842,.F.);
#49811=ORIENTED_EDGE('',*,*,#36654,.T.);
#49812=ORIENTED_EDGE('',*,*,#36837,.T.);
#49813=ORIENTED_EDGE('',*,*,#36843,.T.);
#49814=ORIENTED_EDGE('',*,*,#36844,.F.);
#49815=ORIENTED_EDGE('',*,*,#36656,.T.);
#49816=ORIENTED_EDGE('',*,*,#36845,.F.);
#49817=ORIENTED_EDGE('',*,*,#36846,.F.);
#49818=ORIENTED_EDGE('',*,*,#36847,.F.);
#49819=ORIENTED_EDGE('',*,*,#36848,.F.);
#49820=ORIENTED_EDGE('',*,*,#36843,.F.);
#49821=ORIENTED_EDGE('',*,*,#36848,.T.);
#49822=ORIENTED_EDGE('',*,*,#36849,.F.);
#49823=ORIENTED_EDGE('',*,*,#36657,.T.);
#49824=ORIENTED_EDGE('',*,*,#36844,.T.);
#49825=ORIENTED_EDGE('',*,*,#36850,.T.);
#49826=ORIENTED_EDGE('',*,*,#36851,.F.);
#49827=ORIENTED_EDGE('',*,*,#36659,.T.);
#49828=ORIENTED_EDGE('',*,*,#36852,.F.);
#49829=ORIENTED_EDGE('',*,*,#36853,.F.);
#49830=ORIENTED_EDGE('',*,*,#36854,.F.);
#49831=ORIENTED_EDGE('',*,*,#36855,.F.);
#49832=ORIENTED_EDGE('',*,*,#36850,.F.);
#49833=ORIENTED_EDGE('',*,*,#36855,.T.);
#49834=ORIENTED_EDGE('',*,*,#36856,.F.);
#49835=ORIENTED_EDGE('',*,*,#36660,.T.);
#49836=ORIENTED_EDGE('',*,*,#36851,.T.);
#49837=ORIENTED_EDGE('',*,*,#36857,.T.);
#49838=ORIENTED_EDGE('',*,*,#36858,.F.);
#49839=ORIENTED_EDGE('',*,*,#36662,.T.);
#49840=ORIENTED_EDGE('',*,*,#36859,.F.);
#49841=ORIENTED_EDGE('',*,*,#36860,.F.);
#49842=ORIENTED_EDGE('',*,*,#36861,.F.);
#49843=ORIENTED_EDGE('',*,*,#36862,.F.);
#49844=ORIENTED_EDGE('',*,*,#36857,.F.);
#49845=ORIENTED_EDGE('',*,*,#36862,.T.);
#49846=ORIENTED_EDGE('',*,*,#36863,.F.);
#49847=ORIENTED_EDGE('',*,*,#36663,.T.);
#49848=ORIENTED_EDGE('',*,*,#36858,.T.);
#49849=ORIENTED_EDGE('',*,*,#34438,.T.);
#49850=ORIENTED_EDGE('',*,*,#36864,.F.);
#49851=ORIENTED_EDGE('',*,*,#36665,.T.);
#49852=ORIENTED_EDGE('',*,*,#36865,.F.);
#49853=ORIENTED_EDGE('',*,*,#34437,.T.);
#49854=ORIENTED_EDGE('',*,*,#36866,.F.);
#49855=ORIENTED_EDGE('',*,*,#36666,.T.);
#49856=ORIENTED_EDGE('',*,*,#36864,.T.);
#49857=ORIENTED_EDGE('',*,*,#36867,.T.);
#49858=ORIENTED_EDGE('',*,*,#36868,.F.);
#49859=ORIENTED_EDGE('',*,*,#36668,.T.);
#49860=ORIENTED_EDGE('',*,*,#36869,.F.);
#49861=ORIENTED_EDGE('',*,*,#36870,.F.);
#49862=ORIENTED_EDGE('',*,*,#36871,.F.);
#49863=ORIENTED_EDGE('',*,*,#36872,.F.);
#49864=ORIENTED_EDGE('',*,*,#36867,.F.);
#49865=ORIENTED_EDGE('',*,*,#36872,.T.);
#49866=ORIENTED_EDGE('',*,*,#36873,.F.);
#49867=ORIENTED_EDGE('',*,*,#36669,.T.);
#49868=ORIENTED_EDGE('',*,*,#36868,.T.);
#49869=ORIENTED_EDGE('',*,*,#36874,.T.);
#49870=ORIENTED_EDGE('',*,*,#36875,.F.);
#49871=ORIENTED_EDGE('',*,*,#36671,.T.);
#49872=ORIENTED_EDGE('',*,*,#36876,.F.);
#49873=ORIENTED_EDGE('',*,*,#36877,.F.);
#49874=ORIENTED_EDGE('',*,*,#36878,.F.);
#49875=ORIENTED_EDGE('',*,*,#36879,.F.);
#49876=ORIENTED_EDGE('',*,*,#36874,.F.);
#49877=ORIENTED_EDGE('',*,*,#36879,.T.);
#49878=ORIENTED_EDGE('',*,*,#36880,.F.);
#49879=ORIENTED_EDGE('',*,*,#36672,.T.);
#49880=ORIENTED_EDGE('',*,*,#36875,.T.);
#49881=ORIENTED_EDGE('',*,*,#36881,.T.);
#49882=ORIENTED_EDGE('',*,*,#36882,.F.);
#49883=ORIENTED_EDGE('',*,*,#36674,.T.);
#49884=ORIENTED_EDGE('',*,*,#36883,.F.);
#49885=ORIENTED_EDGE('',*,*,#36884,.F.);
#49886=ORIENTED_EDGE('',*,*,#36885,.F.);
#49887=ORIENTED_EDGE('',*,*,#36886,.F.);
#49888=ORIENTED_EDGE('',*,*,#36881,.F.);
#49889=ORIENTED_EDGE('',*,*,#36886,.T.);
#49890=ORIENTED_EDGE('',*,*,#36887,.F.);
#49891=ORIENTED_EDGE('',*,*,#36675,.T.);
#49892=ORIENTED_EDGE('',*,*,#36882,.T.);
#49893=ORIENTED_EDGE('',*,*,#36888,.T.);
#49894=ORIENTED_EDGE('',*,*,#36889,.F.);
#49895=ORIENTED_EDGE('',*,*,#36677,.T.);
#49896=ORIENTED_EDGE('',*,*,#36890,.F.);
#49897=ORIENTED_EDGE('',*,*,#36891,.F.);
#49898=ORIENTED_EDGE('',*,*,#36892,.F.);
#49899=ORIENTED_EDGE('',*,*,#36893,.F.);
#49900=ORIENTED_EDGE('',*,*,#36888,.F.);
#49901=ORIENTED_EDGE('',*,*,#36893,.T.);
#49902=ORIENTED_EDGE('',*,*,#36894,.F.);
#49903=ORIENTED_EDGE('',*,*,#36678,.T.);
#49904=ORIENTED_EDGE('',*,*,#36889,.T.);
#49905=ORIENTED_EDGE('',*,*,#36895,.T.);
#49906=ORIENTED_EDGE('',*,*,#36896,.F.);
#49907=ORIENTED_EDGE('',*,*,#36680,.T.);
#49908=ORIENTED_EDGE('',*,*,#36897,.F.);
#49909=ORIENTED_EDGE('',*,*,#36898,.F.);
#49910=ORIENTED_EDGE('',*,*,#36899,.F.);
#49911=ORIENTED_EDGE('',*,*,#36900,.F.);
#49912=ORIENTED_EDGE('',*,*,#36895,.F.);
#49913=ORIENTED_EDGE('',*,*,#36900,.T.);
#49914=ORIENTED_EDGE('',*,*,#36901,.F.);
#49915=ORIENTED_EDGE('',*,*,#36681,.T.);
#49916=ORIENTED_EDGE('',*,*,#36896,.T.);
#49917=ORIENTED_EDGE('',*,*,#36902,.T.);
#49918=ORIENTED_EDGE('',*,*,#36903,.F.);
#49919=ORIENTED_EDGE('',*,*,#36683,.T.);
#49920=ORIENTED_EDGE('',*,*,#36904,.F.);
#49921=ORIENTED_EDGE('',*,*,#36905,.F.);
#49922=ORIENTED_EDGE('',*,*,#36906,.F.);
#49923=ORIENTED_EDGE('',*,*,#36907,.F.);
#49924=ORIENTED_EDGE('',*,*,#36902,.F.);
#49925=ORIENTED_EDGE('',*,*,#36907,.T.);
#49926=ORIENTED_EDGE('',*,*,#36908,.F.);
#49927=ORIENTED_EDGE('',*,*,#36684,.T.);
#49928=ORIENTED_EDGE('',*,*,#36903,.T.);
#49929=ORIENTED_EDGE('',*,*,#36909,.T.);
#49930=ORIENTED_EDGE('',*,*,#36910,.F.);
#49931=ORIENTED_EDGE('',*,*,#36686,.T.);
#49932=ORIENTED_EDGE('',*,*,#36911,.F.);
#49933=ORIENTED_EDGE('',*,*,#36912,.F.);
#49934=ORIENTED_EDGE('',*,*,#36913,.F.);
#49935=ORIENTED_EDGE('',*,*,#36914,.F.);
#49936=ORIENTED_EDGE('',*,*,#36909,.F.);
#49937=ORIENTED_EDGE('',*,*,#36914,.T.);
#49938=ORIENTED_EDGE('',*,*,#36915,.F.);
#49939=ORIENTED_EDGE('',*,*,#36687,.T.);
#49940=ORIENTED_EDGE('',*,*,#36910,.T.);
#49941=ORIENTED_EDGE('',*,*,#36916,.T.);
#49942=ORIENTED_EDGE('',*,*,#36917,.F.);
#49943=ORIENTED_EDGE('',*,*,#36689,.T.);
#49944=ORIENTED_EDGE('',*,*,#36918,.F.);
#49945=ORIENTED_EDGE('',*,*,#36919,.F.);
#49946=ORIENTED_EDGE('',*,*,#36920,.F.);
#49947=ORIENTED_EDGE('',*,*,#36921,.F.);
#49948=ORIENTED_EDGE('',*,*,#36916,.F.);
#49949=ORIENTED_EDGE('',*,*,#36921,.T.);
#49950=ORIENTED_EDGE('',*,*,#36922,.F.);
#49951=ORIENTED_EDGE('',*,*,#36690,.T.);
#49952=ORIENTED_EDGE('',*,*,#36917,.T.);
#49953=ORIENTED_EDGE('',*,*,#36923,.T.);
#49954=ORIENTED_EDGE('',*,*,#36924,.F.);
#49955=ORIENTED_EDGE('',*,*,#36692,.T.);
#49956=ORIENTED_EDGE('',*,*,#36925,.F.);
#49957=ORIENTED_EDGE('',*,*,#36926,.F.);
#49958=ORIENTED_EDGE('',*,*,#36927,.F.);
#49959=ORIENTED_EDGE('',*,*,#36928,.F.);
#49960=ORIENTED_EDGE('',*,*,#36923,.F.);
#49961=ORIENTED_EDGE('',*,*,#36928,.T.);
#49962=ORIENTED_EDGE('',*,*,#36929,.F.);
#49963=ORIENTED_EDGE('',*,*,#36693,.T.);
#49964=ORIENTED_EDGE('',*,*,#36924,.T.);
#49965=ORIENTED_EDGE('',*,*,#36930,.T.);
#49966=ORIENTED_EDGE('',*,*,#36931,.F.);
#49967=ORIENTED_EDGE('',*,*,#36695,.T.);
#49968=ORIENTED_EDGE('',*,*,#36932,.F.);
#49969=ORIENTED_EDGE('',*,*,#36933,.F.);
#49970=ORIENTED_EDGE('',*,*,#36934,.F.);
#49971=ORIENTED_EDGE('',*,*,#36935,.F.);
#49972=ORIENTED_EDGE('',*,*,#36930,.F.);
#49973=ORIENTED_EDGE('',*,*,#36935,.T.);
#49974=ORIENTED_EDGE('',*,*,#36936,.F.);
#49975=ORIENTED_EDGE('',*,*,#36696,.T.);
#49976=ORIENTED_EDGE('',*,*,#36931,.T.);
#49977=ORIENTED_EDGE('',*,*,#36937,.T.);
#49978=ORIENTED_EDGE('',*,*,#36938,.F.);
#49979=ORIENTED_EDGE('',*,*,#36698,.T.);
#49980=ORIENTED_EDGE('',*,*,#36939,.F.);
#49981=ORIENTED_EDGE('',*,*,#36940,.F.);
#49982=ORIENTED_EDGE('',*,*,#36941,.F.);
#49983=ORIENTED_EDGE('',*,*,#36942,.F.);
#49984=ORIENTED_EDGE('',*,*,#36937,.F.);
#49985=ORIENTED_EDGE('',*,*,#36942,.T.);
#49986=ORIENTED_EDGE('',*,*,#36943,.F.);
#49987=ORIENTED_EDGE('',*,*,#36699,.T.);
#49988=ORIENTED_EDGE('',*,*,#36938,.T.);
#49989=ORIENTED_EDGE('',*,*,#36944,.T.);
#49990=ORIENTED_EDGE('',*,*,#36945,.F.);
#49991=ORIENTED_EDGE('',*,*,#36701,.T.);
#49992=ORIENTED_EDGE('',*,*,#36946,.F.);
#49993=ORIENTED_EDGE('',*,*,#36947,.F.);
#49994=ORIENTED_EDGE('',*,*,#36948,.F.);
#49995=ORIENTED_EDGE('',*,*,#36949,.F.);
#49996=ORIENTED_EDGE('',*,*,#36944,.F.);
#49997=ORIENTED_EDGE('',*,*,#36949,.T.);
#49998=ORIENTED_EDGE('',*,*,#36950,.F.);
#49999=ORIENTED_EDGE('',*,*,#36702,.T.);
#50000=ORIENTED_EDGE('',*,*,#36945,.T.);
#50001=ORIENTED_EDGE('',*,*,#36951,.T.);
#50002=ORIENTED_EDGE('',*,*,#36952,.F.);
#50003=ORIENTED_EDGE('',*,*,#36704,.T.);
#50004=ORIENTED_EDGE('',*,*,#36953,.F.);
#50005=ORIENTED_EDGE('',*,*,#36954,.F.);
#50006=ORIENTED_EDGE('',*,*,#36955,.F.);
#50007=ORIENTED_EDGE('',*,*,#36956,.F.);
#50008=ORIENTED_EDGE('',*,*,#36951,.F.);
#50009=ORIENTED_EDGE('',*,*,#36956,.T.);
#50010=ORIENTED_EDGE('',*,*,#36957,.F.);
#50011=ORIENTED_EDGE('',*,*,#36705,.T.);
#50012=ORIENTED_EDGE('',*,*,#36952,.T.);
#50013=ORIENTED_EDGE('',*,*,#36958,.T.);
#50014=ORIENTED_EDGE('',*,*,#36959,.F.);
#50015=ORIENTED_EDGE('',*,*,#36707,.T.);
#50016=ORIENTED_EDGE('',*,*,#36960,.F.);
#50017=ORIENTED_EDGE('',*,*,#36961,.F.);
#50018=ORIENTED_EDGE('',*,*,#36962,.F.);
#50019=ORIENTED_EDGE('',*,*,#36963,.F.);
#50020=ORIENTED_EDGE('',*,*,#36958,.F.);
#50021=ORIENTED_EDGE('',*,*,#36963,.T.);
#50022=ORIENTED_EDGE('',*,*,#36964,.F.);
#50023=ORIENTED_EDGE('',*,*,#36708,.T.);
#50024=ORIENTED_EDGE('',*,*,#36959,.T.);
#50025=ORIENTED_EDGE('',*,*,#36965,.T.);
#50026=ORIENTED_EDGE('',*,*,#36966,.F.);
#50027=ORIENTED_EDGE('',*,*,#36710,.T.);
#50028=ORIENTED_EDGE('',*,*,#36967,.F.);
#50029=ORIENTED_EDGE('',*,*,#36968,.F.);
#50030=ORIENTED_EDGE('',*,*,#36969,.F.);
#50031=ORIENTED_EDGE('',*,*,#36970,.F.);
#50032=ORIENTED_EDGE('',*,*,#36965,.F.);
#50033=ORIENTED_EDGE('',*,*,#36970,.T.);
#50034=ORIENTED_EDGE('',*,*,#36971,.F.);
#50035=ORIENTED_EDGE('',*,*,#36711,.T.);
#50036=ORIENTED_EDGE('',*,*,#36966,.T.);
#50037=ORIENTED_EDGE('',*,*,#36972,.T.);
#50038=ORIENTED_EDGE('',*,*,#36973,.F.);
#50039=ORIENTED_EDGE('',*,*,#36713,.T.);
#50040=ORIENTED_EDGE('',*,*,#36974,.F.);
#50041=ORIENTED_EDGE('',*,*,#36975,.T.);
#50042=ORIENTED_EDGE('',*,*,#36976,.F.);
#50043=ORIENTED_EDGE('',*,*,#36714,.T.);
#50044=ORIENTED_EDGE('',*,*,#36973,.T.);
#50045=ORIENTED_EDGE('',*,*,#36977,.F.);
#50046=ORIENTED_EDGE('',*,*,#36978,.F.);
#50047=ORIENTED_EDGE('',*,*,#36975,.F.);
#50048=ORIENTED_EDGE('',*,*,#36972,.F.);
#50049=ORIENTED_EDGE('',*,*,#36716,.T.);
#50050=ORIENTED_EDGE('',*,*,#36979,.F.);
#50051=ORIENTED_EDGE('',*,*,#36980,.T.);
#50052=ORIENTED_EDGE('',*,*,#36981,.F.);
#50053=ORIENTED_EDGE('',*,*,#36982,.F.);
#50054=ORIENTED_EDGE('',*,*,#36980,.F.);
#50055=ORIENTED_EDGE('',*,*,#36983,.F.);
#50056=ORIENTED_EDGE('',*,*,#36984,.F.);
#50057=ORIENTED_EDGE('',*,*,#36717,.T.);
#50058=ORIENTED_EDGE('',*,*,#36981,.T.);
#50059=ORIENTED_EDGE('',*,*,#36982,.T.);
#50060=ORIENTED_EDGE('',*,*,#36985,.F.);
#50061=ORIENTED_EDGE('',*,*,#36986,.T.);
#50062=ORIENTED_EDGE('',*,*,#36987,.F.);
#50063=ORIENTED_EDGE('',*,*,#36719,.T.);
#50064=ORIENTED_EDGE('',*,*,#36988,.F.);
#50065=ORIENTED_EDGE('',*,*,#36989,.F.);
#50066=ORIENTED_EDGE('',*,*,#36990,.F.);
#50067=ORIENTED_EDGE('',*,*,#36991,.F.);
#50068=ORIENTED_EDGE('',*,*,#36986,.F.);
#50069=ORIENTED_EDGE('',*,*,#36991,.T.);
#50070=ORIENTED_EDGE('',*,*,#36992,.F.);
#50071=ORIENTED_EDGE('',*,*,#36720,.T.);
#50072=ORIENTED_EDGE('',*,*,#36987,.T.);
#50073=ORIENTED_EDGE('',*,*,#36993,.T.);
#50074=ORIENTED_EDGE('',*,*,#36994,.F.);
#50075=ORIENTED_EDGE('',*,*,#36722,.T.);
#50076=ORIENTED_EDGE('',*,*,#36995,.F.);
#50077=ORIENTED_EDGE('',*,*,#36996,.F.);
#50078=ORIENTED_EDGE('',*,*,#36997,.F.);
#50079=ORIENTED_EDGE('',*,*,#36998,.F.);
#50080=ORIENTED_EDGE('',*,*,#36993,.F.);
#50081=ORIENTED_EDGE('',*,*,#36998,.T.);
#50082=ORIENTED_EDGE('',*,*,#36999,.F.);
#50083=ORIENTED_EDGE('',*,*,#36723,.T.);
#50084=ORIENTED_EDGE('',*,*,#36994,.T.);
#50085=ORIENTED_EDGE('',*,*,#37000,.T.);
#50086=ORIENTED_EDGE('',*,*,#37001,.F.);
#50087=ORIENTED_EDGE('',*,*,#36725,.T.);
#50088=ORIENTED_EDGE('',*,*,#37002,.F.);
#50089=ORIENTED_EDGE('',*,*,#37003,.F.);
#50090=ORIENTED_EDGE('',*,*,#37004,.F.);
#50091=ORIENTED_EDGE('',*,*,#37005,.F.);
#50092=ORIENTED_EDGE('',*,*,#37000,.F.);
#50093=ORIENTED_EDGE('',*,*,#37005,.T.);
#50094=ORIENTED_EDGE('',*,*,#37006,.F.);
#50095=ORIENTED_EDGE('',*,*,#36726,.T.);
#50096=ORIENTED_EDGE('',*,*,#37001,.T.);
#50097=ORIENTED_EDGE('',*,*,#37007,.T.);
#50098=ORIENTED_EDGE('',*,*,#37008,.F.);
#50099=ORIENTED_EDGE('',*,*,#36728,.T.);
#50100=ORIENTED_EDGE('',*,*,#37009,.F.);
#50101=ORIENTED_EDGE('',*,*,#37010,.F.);
#50102=ORIENTED_EDGE('',*,*,#37011,.F.);
#50103=ORIENTED_EDGE('',*,*,#37012,.F.);
#50104=ORIENTED_EDGE('',*,*,#37007,.F.);
#50105=ORIENTED_EDGE('',*,*,#37012,.T.);
#50106=ORIENTED_EDGE('',*,*,#37013,.F.);
#50107=ORIENTED_EDGE('',*,*,#36729,.T.);
#50108=ORIENTED_EDGE('',*,*,#37008,.T.);
#50109=ORIENTED_EDGE('',*,*,#37014,.F.);
#50110=ORIENTED_EDGE('',*,*,#37015,.F.);
#50111=ORIENTED_EDGE('',*,*,#36819,.F.);
#50112=ORIENTED_EDGE('',*,*,#37016,.F.);
#50113=ORIENTED_EDGE('',*,*,#37016,.T.);
#50114=ORIENTED_EDGE('',*,*,#36821,.T.);
#50115=ORIENTED_EDGE('',*,*,#36731,.T.);
#50116=ORIENTED_EDGE('',*,*,#37017,.F.);
#50117=ORIENTED_EDGE('',*,*,#37018,.T.);
#50118=ORIENTED_EDGE('',*,*,#37019,.F.);
#50119=ORIENTED_EDGE('',*,*,#36732,.T.);
#50120=ORIENTED_EDGE('',*,*,#37020,.F.);
#50121=ORIENTED_EDGE('',*,*,#36734,.T.);
#50122=ORIENTED_EDGE('',*,*,#37021,.F.);
#50123=ORIENTED_EDGE('',*,*,#37022,.T.);
#50124=ORIENTED_EDGE('',*,*,#37023,.F.);
#50125=ORIENTED_EDGE('',*,*,#36735,.T.);
#50126=ORIENTED_EDGE('',*,*,#37023,.T.);
#50127=ORIENTED_EDGE('',*,*,#37024,.T.);
#50128=ORIENTED_EDGE('',*,*,#37025,.F.);
#50129=ORIENTED_EDGE('',*,*,#37024,.F.);
#50130=ORIENTED_EDGE('',*,*,#37022,.F.);
#50131=ORIENTED_EDGE('',*,*,#37026,.F.);
#50132=ORIENTED_EDGE('',*,*,#37027,.F.);
#50133=ORIENTED_EDGE('',*,*,#36737,.T.);
#50134=ORIENTED_EDGE('',*,*,#37028,.F.);
#50135=ORIENTED_EDGE('',*,*,#37029,.T.);
#50136=ORIENTED_EDGE('',*,*,#37030,.F.);
#50137=ORIENTED_EDGE('',*,*,#36738,.T.);
#50138=ORIENTED_EDGE('',*,*,#37030,.T.);
#50139=ORIENTED_EDGE('',*,*,#37031,.T.);
#50140=ORIENTED_EDGE('',*,*,#37032,.F.);
#50141=ORIENTED_EDGE('',*,*,#37031,.F.);
#50142=ORIENTED_EDGE('',*,*,#37029,.F.);
#50143=ORIENTED_EDGE('',*,*,#37033,.F.);
#50144=ORIENTED_EDGE('',*,*,#37034,.F.);
#50145=ORIENTED_EDGE('',*,*,#36740,.T.);
#50146=ORIENTED_EDGE('',*,*,#37035,.F.);
#50147=ORIENTED_EDGE('',*,*,#37036,.T.);
#50148=ORIENTED_EDGE('',*,*,#37037,.F.);
#50149=ORIENTED_EDGE('',*,*,#36741,.T.);
#50150=ORIENTED_EDGE('',*,*,#37037,.T.);
#50151=ORIENTED_EDGE('',*,*,#37038,.T.);
#50152=ORIENTED_EDGE('',*,*,#37039,.F.);
#50153=ORIENTED_EDGE('',*,*,#37038,.F.);
#50154=ORIENTED_EDGE('',*,*,#37036,.F.);
#50155=ORIENTED_EDGE('',*,*,#37040,.F.);
#50156=ORIENTED_EDGE('',*,*,#37041,.F.);
#50157=ORIENTED_EDGE('',*,*,#36743,.T.);
#50158=ORIENTED_EDGE('',*,*,#37042,.F.);
#50159=ORIENTED_EDGE('',*,*,#37043,.T.);
#50160=ORIENTED_EDGE('',*,*,#37044,.F.);
#50161=ORIENTED_EDGE('',*,*,#36744,.T.);
#50162=ORIENTED_EDGE('',*,*,#37044,.T.);
#50163=ORIENTED_EDGE('',*,*,#37045,.T.);
#50164=ORIENTED_EDGE('',*,*,#37046,.F.);
#50165=ORIENTED_EDGE('',*,*,#37045,.F.);
#50166=ORIENTED_EDGE('',*,*,#37043,.F.);
#50167=ORIENTED_EDGE('',*,*,#37047,.F.);
#50168=ORIENTED_EDGE('',*,*,#37048,.F.);
#50169=ORIENTED_EDGE('',*,*,#36746,.T.);
#50170=ORIENTED_EDGE('',*,*,#37049,.F.);
#50171=ORIENTED_EDGE('',*,*,#37050,.T.);
#50172=ORIENTED_EDGE('',*,*,#37051,.F.);
#50173=ORIENTED_EDGE('',*,*,#36747,.T.);
#50174=ORIENTED_EDGE('',*,*,#37051,.T.);
#50175=ORIENTED_EDGE('',*,*,#37052,.T.);
#50176=ORIENTED_EDGE('',*,*,#37053,.F.);
#50177=ORIENTED_EDGE('',*,*,#37052,.F.);
#50178=ORIENTED_EDGE('',*,*,#37050,.F.);
#50179=ORIENTED_EDGE('',*,*,#37054,.F.);
#50180=ORIENTED_EDGE('',*,*,#37055,.F.);
#50181=ORIENTED_EDGE('',*,*,#36749,.T.);
#50182=ORIENTED_EDGE('',*,*,#37056,.F.);
#50183=ORIENTED_EDGE('',*,*,#37057,.T.);
#50184=ORIENTED_EDGE('',*,*,#37058,.F.);
#50185=ORIENTED_EDGE('',*,*,#36750,.T.);
#50186=ORIENTED_EDGE('',*,*,#37058,.T.);
#50187=ORIENTED_EDGE('',*,*,#37059,.T.);
#50188=ORIENTED_EDGE('',*,*,#37060,.F.);
#50189=ORIENTED_EDGE('',*,*,#37059,.F.);
#50190=ORIENTED_EDGE('',*,*,#37057,.F.);
#50191=ORIENTED_EDGE('',*,*,#37061,.F.);
#50192=ORIENTED_EDGE('',*,*,#37062,.F.);
#50193=ORIENTED_EDGE('',*,*,#36752,.T.);
#50194=ORIENTED_EDGE('',*,*,#37063,.F.);
#50195=ORIENTED_EDGE('',*,*,#37064,.T.);
#50196=ORIENTED_EDGE('',*,*,#37065,.F.);
#50197=ORIENTED_EDGE('',*,*,#36753,.T.);
#50198=ORIENTED_EDGE('',*,*,#37065,.T.);
#50199=ORIENTED_EDGE('',*,*,#37066,.T.);
#50200=ORIENTED_EDGE('',*,*,#37067,.F.);
#50201=ORIENTED_EDGE('',*,*,#37066,.F.);
#50202=ORIENTED_EDGE('',*,*,#37064,.F.);
#50203=ORIENTED_EDGE('',*,*,#37068,.F.);
#50204=ORIENTED_EDGE('',*,*,#37069,.F.);
#50205=ORIENTED_EDGE('',*,*,#36755,.T.);
#50206=ORIENTED_EDGE('',*,*,#37070,.F.);
#50207=ORIENTED_EDGE('',*,*,#37071,.T.);
#50208=ORIENTED_EDGE('',*,*,#37072,.F.);
#50209=ORIENTED_EDGE('',*,*,#36756,.T.);
#50210=ORIENTED_EDGE('',*,*,#37072,.T.);
#50211=ORIENTED_EDGE('',*,*,#37073,.T.);
#50212=ORIENTED_EDGE('',*,*,#37074,.F.);
#50213=ORIENTED_EDGE('',*,*,#37073,.F.);
#50214=ORIENTED_EDGE('',*,*,#37071,.F.);
#50215=ORIENTED_EDGE('',*,*,#37075,.F.);
#50216=ORIENTED_EDGE('',*,*,#37076,.F.);
#50217=ORIENTED_EDGE('',*,*,#36758,.T.);
#50218=ORIENTED_EDGE('',*,*,#37077,.F.);
#50219=ORIENTED_EDGE('',*,*,#37078,.T.);
#50220=ORIENTED_EDGE('',*,*,#37079,.F.);
#50221=ORIENTED_EDGE('',*,*,#36759,.T.);
#50222=ORIENTED_EDGE('',*,*,#37079,.T.);
#50223=ORIENTED_EDGE('',*,*,#37080,.T.);
#50224=ORIENTED_EDGE('',*,*,#37081,.F.);
#50225=ORIENTED_EDGE('',*,*,#37080,.F.);
#50226=ORIENTED_EDGE('',*,*,#37078,.F.);
#50227=ORIENTED_EDGE('',*,*,#37082,.F.);
#50228=ORIENTED_EDGE('',*,*,#37083,.F.);
#50229=ORIENTED_EDGE('',*,*,#36761,.T.);
#50230=ORIENTED_EDGE('',*,*,#37084,.F.);
#50231=ORIENTED_EDGE('',*,*,#37085,.T.);
#50232=ORIENTED_EDGE('',*,*,#37086,.F.);
#50233=ORIENTED_EDGE('',*,*,#36762,.T.);
#50234=ORIENTED_EDGE('',*,*,#37086,.T.);
#50235=ORIENTED_EDGE('',*,*,#37087,.T.);
#50236=ORIENTED_EDGE('',*,*,#37088,.F.);
#50237=ORIENTED_EDGE('',*,*,#37087,.F.);
#50238=ORIENTED_EDGE('',*,*,#37085,.F.);
#50239=ORIENTED_EDGE('',*,*,#37089,.F.);
#50240=ORIENTED_EDGE('',*,*,#37090,.F.);
#50241=ORIENTED_EDGE('',*,*,#36764,.T.);
#50242=ORIENTED_EDGE('',*,*,#37091,.F.);
#50243=ORIENTED_EDGE('',*,*,#37092,.T.);
#50244=ORIENTED_EDGE('',*,*,#37093,.F.);
#50245=ORIENTED_EDGE('',*,*,#36765,.T.);
#50246=ORIENTED_EDGE('',*,*,#37093,.T.);
#50247=ORIENTED_EDGE('',*,*,#37094,.T.);
#50248=ORIENTED_EDGE('',*,*,#37095,.F.);
#50249=ORIENTED_EDGE('',*,*,#37094,.F.);
#50250=ORIENTED_EDGE('',*,*,#37092,.F.);
#50251=ORIENTED_EDGE('',*,*,#37096,.F.);
#50252=ORIENTED_EDGE('',*,*,#37097,.F.);
#50253=ORIENTED_EDGE('',*,*,#36767,.T.);
#50254=ORIENTED_EDGE('',*,*,#37098,.F.);
#50255=ORIENTED_EDGE('',*,*,#37099,.T.);
#50256=ORIENTED_EDGE('',*,*,#37100,.F.);
#50257=ORIENTED_EDGE('',*,*,#36768,.T.);
#50258=ORIENTED_EDGE('',*,*,#37100,.T.);
#50259=ORIENTED_EDGE('',*,*,#37101,.T.);
#50260=ORIENTED_EDGE('',*,*,#37102,.F.);
#50261=ORIENTED_EDGE('',*,*,#37101,.F.);
#50262=ORIENTED_EDGE('',*,*,#37099,.F.);
#50263=ORIENTED_EDGE('',*,*,#37103,.F.);
#50264=ORIENTED_EDGE('',*,*,#37104,.F.);
#50265=ORIENTED_EDGE('',*,*,#36770,.T.);
#50266=ORIENTED_EDGE('',*,*,#37105,.F.);
#50267=ORIENTED_EDGE('',*,*,#37106,.T.);
#50268=ORIENTED_EDGE('',*,*,#37107,.F.);
#50269=ORIENTED_EDGE('',*,*,#36771,.T.);
#50270=ORIENTED_EDGE('',*,*,#37107,.T.);
#50271=ORIENTED_EDGE('',*,*,#37108,.T.);
#50272=ORIENTED_EDGE('',*,*,#37109,.F.);
#50273=ORIENTED_EDGE('',*,*,#37108,.F.);
#50274=ORIENTED_EDGE('',*,*,#37106,.F.);
#50275=ORIENTED_EDGE('',*,*,#37110,.F.);
#50276=ORIENTED_EDGE('',*,*,#37111,.F.);
#50277=ORIENTED_EDGE('',*,*,#36773,.T.);
#50278=ORIENTED_EDGE('',*,*,#37112,.F.);
#50279=ORIENTED_EDGE('',*,*,#34435,.T.);
#50280=ORIENTED_EDGE('',*,*,#37113,.F.);
#50281=ORIENTED_EDGE('',*,*,#36774,.T.);
#50282=ORIENTED_EDGE('',*,*,#37113,.T.);
#50283=ORIENTED_EDGE('',*,*,#34434,.T.);
#50284=ORIENTED_EDGE('',*,*,#37114,.F.);
#50285=ORIENTED_EDGE('',*,*,#36776,.T.);
#50286=ORIENTED_EDGE('',*,*,#37115,.F.);
#50287=ORIENTED_EDGE('',*,*,#37116,.T.);
#50288=ORIENTED_EDGE('',*,*,#37117,.F.);
#50289=ORIENTED_EDGE('',*,*,#36777,.T.);
#50290=ORIENTED_EDGE('',*,*,#37117,.T.);
#50291=ORIENTED_EDGE('',*,*,#37118,.T.);
#50292=ORIENTED_EDGE('',*,*,#37119,.F.);
#50293=ORIENTED_EDGE('',*,*,#37118,.F.);
#50294=ORIENTED_EDGE('',*,*,#37116,.F.);
#50295=ORIENTED_EDGE('',*,*,#37120,.F.);
#50296=ORIENTED_EDGE('',*,*,#37121,.F.);
#50297=ORIENTED_EDGE('',*,*,#36779,.T.);
#50298=ORIENTED_EDGE('',*,*,#37122,.F.);
#50299=ORIENTED_EDGE('',*,*,#37123,.T.);
#50300=ORIENTED_EDGE('',*,*,#37124,.F.);
#50301=ORIENTED_EDGE('',*,*,#36780,.T.);
#50302=ORIENTED_EDGE('',*,*,#37124,.T.);
#50303=ORIENTED_EDGE('',*,*,#37125,.T.);
#50304=ORIENTED_EDGE('',*,*,#37126,.F.);
#50305=ORIENTED_EDGE('',*,*,#37125,.F.);
#50306=ORIENTED_EDGE('',*,*,#37123,.F.);
#50307=ORIENTED_EDGE('',*,*,#37127,.F.);
#50308=ORIENTED_EDGE('',*,*,#37128,.F.);
#50309=ORIENTED_EDGE('',*,*,#36782,.T.);
#50310=ORIENTED_EDGE('',*,*,#37129,.F.);
#50311=ORIENTED_EDGE('',*,*,#37130,.T.);
#50312=ORIENTED_EDGE('',*,*,#37131,.F.);
#50313=ORIENTED_EDGE('',*,*,#36783,.T.);
#50314=ORIENTED_EDGE('',*,*,#37131,.T.);
#50315=ORIENTED_EDGE('',*,*,#37132,.T.);
#50316=ORIENTED_EDGE('',*,*,#37133,.F.);
#50317=ORIENTED_EDGE('',*,*,#37132,.F.);
#50318=ORIENTED_EDGE('',*,*,#37130,.F.);
#50319=ORIENTED_EDGE('',*,*,#37134,.F.);
#50320=ORIENTED_EDGE('',*,*,#37135,.F.);
#50321=ORIENTED_EDGE('',*,*,#36785,.T.);
#50322=ORIENTED_EDGE('',*,*,#37136,.F.);
#50323=ORIENTED_EDGE('',*,*,#37137,.T.);
#50324=ORIENTED_EDGE('',*,*,#37138,.F.);
#50325=ORIENTED_EDGE('',*,*,#36786,.T.);
#50326=ORIENTED_EDGE('',*,*,#37138,.T.);
#50327=ORIENTED_EDGE('',*,*,#37139,.T.);
#50328=ORIENTED_EDGE('',*,*,#37140,.F.);
#50329=ORIENTED_EDGE('',*,*,#37139,.F.);
#50330=ORIENTED_EDGE('',*,*,#37137,.F.);
#50331=ORIENTED_EDGE('',*,*,#37141,.F.);
#50332=ORIENTED_EDGE('',*,*,#37142,.F.);
#50333=ORIENTED_EDGE('',*,*,#36788,.T.);
#50334=ORIENTED_EDGE('',*,*,#37143,.F.);
#50335=ORIENTED_EDGE('',*,*,#37144,.T.);
#50336=ORIENTED_EDGE('',*,*,#37145,.F.);
#50337=ORIENTED_EDGE('',*,*,#36789,.T.);
#50338=ORIENTED_EDGE('',*,*,#37145,.T.);
#50339=ORIENTED_EDGE('',*,*,#37146,.T.);
#50340=ORIENTED_EDGE('',*,*,#37147,.F.);
#50341=ORIENTED_EDGE('',*,*,#37146,.F.);
#50342=ORIENTED_EDGE('',*,*,#37144,.F.);
#50343=ORIENTED_EDGE('',*,*,#37148,.F.);
#50344=ORIENTED_EDGE('',*,*,#37149,.F.);
#50345=ORIENTED_EDGE('',*,*,#36791,.T.);
#50346=ORIENTED_EDGE('',*,*,#37150,.F.);
#50347=ORIENTED_EDGE('',*,*,#37151,.T.);
#50348=ORIENTED_EDGE('',*,*,#37152,.F.);
#50349=ORIENTED_EDGE('',*,*,#36792,.T.);
#50350=ORIENTED_EDGE('',*,*,#37152,.T.);
#50351=ORIENTED_EDGE('',*,*,#37153,.T.);
#50352=ORIENTED_EDGE('',*,*,#37154,.F.);
#50353=ORIENTED_EDGE('',*,*,#37153,.F.);
#50354=ORIENTED_EDGE('',*,*,#37151,.F.);
#50355=ORIENTED_EDGE('',*,*,#37155,.F.);
#50356=ORIENTED_EDGE('',*,*,#37156,.F.);
#50357=ORIENTED_EDGE('',*,*,#36794,.T.);
#50358=ORIENTED_EDGE('',*,*,#37157,.F.);
#50359=ORIENTED_EDGE('',*,*,#37158,.T.);
#50360=ORIENTED_EDGE('',*,*,#37159,.F.);
#50361=ORIENTED_EDGE('',*,*,#36795,.T.);
#50362=ORIENTED_EDGE('',*,*,#37159,.T.);
#50363=ORIENTED_EDGE('',*,*,#37160,.T.);
#50364=ORIENTED_EDGE('',*,*,#37161,.F.);
#50365=ORIENTED_EDGE('',*,*,#37160,.F.);
#50366=ORIENTED_EDGE('',*,*,#37158,.F.);
#50367=ORIENTED_EDGE('',*,*,#37162,.F.);
#50368=ORIENTED_EDGE('',*,*,#37163,.F.);
#50369=ORIENTED_EDGE('',*,*,#36797,.T.);
#50370=ORIENTED_EDGE('',*,*,#37164,.F.);
#50371=ORIENTED_EDGE('',*,*,#37165,.T.);
#50372=ORIENTED_EDGE('',*,*,#37166,.F.);
#50373=ORIENTED_EDGE('',*,*,#36798,.T.);
#50374=ORIENTED_EDGE('',*,*,#37166,.T.);
#50375=ORIENTED_EDGE('',*,*,#37167,.T.);
#50376=ORIENTED_EDGE('',*,*,#37168,.F.);
#50377=ORIENTED_EDGE('',*,*,#37167,.F.);
#50378=ORIENTED_EDGE('',*,*,#37165,.F.);
#50379=ORIENTED_EDGE('',*,*,#37169,.F.);
#50380=ORIENTED_EDGE('',*,*,#37170,.F.);
#50381=ORIENTED_EDGE('',*,*,#36800,.T.);
#50382=ORIENTED_EDGE('',*,*,#37171,.F.);
#50383=ORIENTED_EDGE('',*,*,#37172,.T.);
#50384=ORIENTED_EDGE('',*,*,#37173,.F.);
#50385=ORIENTED_EDGE('',*,*,#36801,.T.);
#50386=ORIENTED_EDGE('',*,*,#37173,.T.);
#50387=ORIENTED_EDGE('',*,*,#37174,.T.);
#50388=ORIENTED_EDGE('',*,*,#37175,.F.);
#50389=ORIENTED_EDGE('',*,*,#37174,.F.);
#50390=ORIENTED_EDGE('',*,*,#37172,.F.);
#50391=ORIENTED_EDGE('',*,*,#37176,.F.);
#50392=ORIENTED_EDGE('',*,*,#37177,.F.);
#50393=ORIENTED_EDGE('',*,*,#36803,.T.);
#50394=ORIENTED_EDGE('',*,*,#37178,.F.);
#50395=ORIENTED_EDGE('',*,*,#37179,.T.);
#50396=ORIENTED_EDGE('',*,*,#37180,.F.);
#50397=ORIENTED_EDGE('',*,*,#36804,.T.);
#50398=ORIENTED_EDGE('',*,*,#37180,.T.);
#50399=ORIENTED_EDGE('',*,*,#37181,.T.);
#50400=ORIENTED_EDGE('',*,*,#37182,.F.);
#50401=ORIENTED_EDGE('',*,*,#37181,.F.);
#50402=ORIENTED_EDGE('',*,*,#37179,.F.);
#50403=ORIENTED_EDGE('',*,*,#37183,.F.);
#50404=ORIENTED_EDGE('',*,*,#37184,.F.);
#50405=ORIENTED_EDGE('',*,*,#36806,.T.);
#50406=ORIENTED_EDGE('',*,*,#37185,.F.);
#50407=ORIENTED_EDGE('',*,*,#37186,.T.);
#50408=ORIENTED_EDGE('',*,*,#37187,.F.);
#50409=ORIENTED_EDGE('',*,*,#36807,.T.);
#50410=ORIENTED_EDGE('',*,*,#37187,.T.);
#50411=ORIENTED_EDGE('',*,*,#37188,.T.);
#50412=ORIENTED_EDGE('',*,*,#37189,.F.);
#50413=ORIENTED_EDGE('',*,*,#37188,.F.);
#50414=ORIENTED_EDGE('',*,*,#37186,.F.);
#50415=ORIENTED_EDGE('',*,*,#37190,.F.);
#50416=ORIENTED_EDGE('',*,*,#37191,.F.);
#50417=ORIENTED_EDGE('',*,*,#36809,.T.);
#50418=ORIENTED_EDGE('',*,*,#37192,.F.);
#50419=ORIENTED_EDGE('',*,*,#37193,.T.);
#50420=ORIENTED_EDGE('',*,*,#37194,.F.);
#50421=ORIENTED_EDGE('',*,*,#36810,.T.);
#50422=ORIENTED_EDGE('',*,*,#37194,.T.);
#50423=ORIENTED_EDGE('',*,*,#37195,.T.);
#50424=ORIENTED_EDGE('',*,*,#37196,.F.);
#50425=ORIENTED_EDGE('',*,*,#37195,.F.);
#50426=ORIENTED_EDGE('',*,*,#37193,.F.);
#50427=ORIENTED_EDGE('',*,*,#37197,.F.);
#50428=ORIENTED_EDGE('',*,*,#37198,.F.);
#50429=ORIENTED_EDGE('',*,*,#36812,.T.);
#50430=ORIENTED_EDGE('',*,*,#37199,.F.);
#50431=ORIENTED_EDGE('',*,*,#37200,.T.);
#50432=ORIENTED_EDGE('',*,*,#37201,.F.);
#50433=ORIENTED_EDGE('',*,*,#36813,.T.);
#50434=ORIENTED_EDGE('',*,*,#37201,.T.);
#50435=ORIENTED_EDGE('',*,*,#37202,.T.);
#50436=ORIENTED_EDGE('',*,*,#37203,.F.);
#50437=ORIENTED_EDGE('',*,*,#37202,.F.);
#50438=ORIENTED_EDGE('',*,*,#37200,.F.);
#50439=ORIENTED_EDGE('',*,*,#37204,.F.);
#50440=ORIENTED_EDGE('',*,*,#37205,.F.);
#50441=ORIENTED_EDGE('',*,*,#36815,.T.);
#50442=ORIENTED_EDGE('',*,*,#37206,.F.);
#50443=ORIENTED_EDGE('',*,*,#37207,.T.);
#50444=ORIENTED_EDGE('',*,*,#37208,.F.);
#50445=ORIENTED_EDGE('',*,*,#36816,.T.);
#50446=ORIENTED_EDGE('',*,*,#37208,.T.);
#50447=ORIENTED_EDGE('',*,*,#37209,.T.);
#50448=ORIENTED_EDGE('',*,*,#37210,.F.);
#50449=ORIENTED_EDGE('',*,*,#37209,.F.);
#50450=ORIENTED_EDGE('',*,*,#37207,.F.);
#50451=ORIENTED_EDGE('',*,*,#37211,.F.);
#50452=ORIENTED_EDGE('',*,*,#37212,.F.);
#50453=ORIENTED_EDGE('',*,*,#37213,.F.);
#50454=ORIENTED_EDGE('',*,*,#37214,.F.);
#50455=ORIENTED_EDGE('',*,*,#37018,.F.);
#50456=ORIENTED_EDGE('',*,*,#37215,.F.);
#50457=ORIENTED_EDGE('',*,*,#36818,.T.);
#50458=ORIENTED_EDGE('',*,*,#37216,.F.);
#50459=ORIENTED_EDGE('',*,*,#37215,.T.);
#50460=ORIENTED_EDGE('',*,*,#37020,.T.);
#50461=ORIENTED_EDGE('',*,*,#37217,.F.);
#50462=ORIENTED_EDGE('',*,*,#36820,.T.);
#50463=ORIENTED_EDGE('',*,*,#37015,.T.);
#50464=ORIENTED_EDGE('',*,*,#37218,.F.);
#50465=ORIENTED_EDGE('',*,*,#37219,.F.);
#50466=ORIENTED_EDGE('',*,*,#37220,.F.);
#50467=ORIENTED_EDGE('',*,*,#36825,.T.);
#50468=ORIENTED_EDGE('',*,*,#36824,.T.);
#50469=ORIENTED_EDGE('',*,*,#37221,.F.);
#50470=ORIENTED_EDGE('',*,*,#36828,.T.);
#50471=ORIENTED_EDGE('',*,*,#36826,.T.);
#50472=ORIENTED_EDGE('',*,*,#37220,.T.);
#50473=ORIENTED_EDGE('',*,*,#37222,.F.);
#50474=ORIENTED_EDGE('',*,*,#37223,.F.);
#50475=ORIENTED_EDGE('',*,*,#36832,.T.);
#50476=ORIENTED_EDGE('',*,*,#36831,.T.);
#50477=ORIENTED_EDGE('',*,*,#37224,.F.);
#50478=ORIENTED_EDGE('',*,*,#36835,.T.);
#50479=ORIENTED_EDGE('',*,*,#36833,.T.);
#50480=ORIENTED_EDGE('',*,*,#37223,.T.);
#50481=ORIENTED_EDGE('',*,*,#37225,.F.);
#50482=ORIENTED_EDGE('',*,*,#37226,.F.);
#50483=ORIENTED_EDGE('',*,*,#36839,.T.);
#50484=ORIENTED_EDGE('',*,*,#36838,.T.);
#50485=ORIENTED_EDGE('',*,*,#37227,.F.);
#50486=ORIENTED_EDGE('',*,*,#36842,.T.);
#50487=ORIENTED_EDGE('',*,*,#36840,.T.);
#50488=ORIENTED_EDGE('',*,*,#37226,.T.);
#50489=ORIENTED_EDGE('',*,*,#37228,.F.);
#50490=ORIENTED_EDGE('',*,*,#37229,.F.);
#50491=ORIENTED_EDGE('',*,*,#36846,.T.);
#50492=ORIENTED_EDGE('',*,*,#36845,.T.);
#50493=ORIENTED_EDGE('',*,*,#37230,.F.);
#50494=ORIENTED_EDGE('',*,*,#36849,.T.);
#50495=ORIENTED_EDGE('',*,*,#36847,.T.);
#50496=ORIENTED_EDGE('',*,*,#37229,.T.);
#50497=ORIENTED_EDGE('',*,*,#37231,.F.);
#50498=ORIENTED_EDGE('',*,*,#37232,.F.);
#50499=ORIENTED_EDGE('',*,*,#36853,.T.);
#50500=ORIENTED_EDGE('',*,*,#36852,.T.);
#50501=ORIENTED_EDGE('',*,*,#37233,.F.);
#50502=ORIENTED_EDGE('',*,*,#36856,.T.);
#50503=ORIENTED_EDGE('',*,*,#36854,.T.);
#50504=ORIENTED_EDGE('',*,*,#37232,.T.);
#50505=ORIENTED_EDGE('',*,*,#37234,.F.);
#50506=ORIENTED_EDGE('',*,*,#37235,.F.);
#50507=ORIENTED_EDGE('',*,*,#36860,.T.);
#50508=ORIENTED_EDGE('',*,*,#36859,.T.);
#50509=ORIENTED_EDGE('',*,*,#37236,.F.);
#50510=ORIENTED_EDGE('',*,*,#36863,.T.);
#50511=ORIENTED_EDGE('',*,*,#36861,.T.);
#50512=ORIENTED_EDGE('',*,*,#37235,.T.);
#50513=ORIENTED_EDGE('',*,*,#37237,.F.);
#50514=ORIENTED_EDGE('',*,*,#37238,.F.);
#50515=ORIENTED_EDGE('',*,*,#34439,.T.);
#50516=ORIENTED_EDGE('',*,*,#36865,.T.);
#50517=ORIENTED_EDGE('',*,*,#37239,.F.);
#50518=ORIENTED_EDGE('',*,*,#36866,.T.);
#50519=ORIENTED_EDGE('',*,*,#34440,.T.);
#50520=ORIENTED_EDGE('',*,*,#37238,.T.);
#50521=ORIENTED_EDGE('',*,*,#37240,.F.);
#50522=ORIENTED_EDGE('',*,*,#37241,.F.);
#50523=ORIENTED_EDGE('',*,*,#36870,.T.);
#50524=ORIENTED_EDGE('',*,*,#36869,.T.);
#50525=ORIENTED_EDGE('',*,*,#37242,.F.);
#50526=ORIENTED_EDGE('',*,*,#36873,.T.);
#50527=ORIENTED_EDGE('',*,*,#36871,.T.);
#50528=ORIENTED_EDGE('',*,*,#37241,.T.);
#50529=ORIENTED_EDGE('',*,*,#37243,.F.);
#50530=ORIENTED_EDGE('',*,*,#37244,.F.);
#50531=ORIENTED_EDGE('',*,*,#36877,.T.);
#50532=ORIENTED_EDGE('',*,*,#36876,.T.);
#50533=ORIENTED_EDGE('',*,*,#37245,.F.);
#50534=ORIENTED_EDGE('',*,*,#36880,.T.);
#50535=ORIENTED_EDGE('',*,*,#36878,.T.);
#50536=ORIENTED_EDGE('',*,*,#37244,.T.);
#50537=ORIENTED_EDGE('',*,*,#37246,.F.);
#50538=ORIENTED_EDGE('',*,*,#37247,.F.);
#50539=ORIENTED_EDGE('',*,*,#36884,.T.);
#50540=ORIENTED_EDGE('',*,*,#36883,.T.);
#50541=ORIENTED_EDGE('',*,*,#37248,.F.);
#50542=ORIENTED_EDGE('',*,*,#36887,.T.);
#50543=ORIENTED_EDGE('',*,*,#36885,.T.);
#50544=ORIENTED_EDGE('',*,*,#37247,.T.);
#50545=ORIENTED_EDGE('',*,*,#37249,.F.);
#50546=ORIENTED_EDGE('',*,*,#37250,.F.);
#50547=ORIENTED_EDGE('',*,*,#36891,.T.);
#50548=ORIENTED_EDGE('',*,*,#36890,.T.);
#50549=ORIENTED_EDGE('',*,*,#37251,.F.);
#50550=ORIENTED_EDGE('',*,*,#36894,.T.);
#50551=ORIENTED_EDGE('',*,*,#36892,.T.);
#50552=ORIENTED_EDGE('',*,*,#37250,.T.);
#50553=ORIENTED_EDGE('',*,*,#37252,.F.);
#50554=ORIENTED_EDGE('',*,*,#37253,.F.);
#50555=ORIENTED_EDGE('',*,*,#36898,.T.);
#50556=ORIENTED_EDGE('',*,*,#36897,.T.);
#50557=ORIENTED_EDGE('',*,*,#37254,.F.);
#50558=ORIENTED_EDGE('',*,*,#36901,.T.);
#50559=ORIENTED_EDGE('',*,*,#36899,.T.);
#50560=ORIENTED_EDGE('',*,*,#37253,.T.);
#50561=ORIENTED_EDGE('',*,*,#37255,.F.);
#50562=ORIENTED_EDGE('',*,*,#37256,.F.);
#50563=ORIENTED_EDGE('',*,*,#36905,.T.);
#50564=ORIENTED_EDGE('',*,*,#36904,.T.);
#50565=ORIENTED_EDGE('',*,*,#37257,.F.);
#50566=ORIENTED_EDGE('',*,*,#36908,.T.);
#50567=ORIENTED_EDGE('',*,*,#36906,.T.);
#50568=ORIENTED_EDGE('',*,*,#37256,.T.);
#50569=ORIENTED_EDGE('',*,*,#37258,.F.);
#50570=ORIENTED_EDGE('',*,*,#37259,.F.);
#50571=ORIENTED_EDGE('',*,*,#36912,.T.);
#50572=ORIENTED_EDGE('',*,*,#36911,.T.);
#50573=ORIENTED_EDGE('',*,*,#37260,.F.);
#50574=ORIENTED_EDGE('',*,*,#36915,.T.);
#50575=ORIENTED_EDGE('',*,*,#36913,.T.);
#50576=ORIENTED_EDGE('',*,*,#37259,.T.);
#50577=ORIENTED_EDGE('',*,*,#37261,.F.);
#50578=ORIENTED_EDGE('',*,*,#37262,.F.);
#50579=ORIENTED_EDGE('',*,*,#36919,.T.);
#50580=ORIENTED_EDGE('',*,*,#36918,.T.);
#50581=ORIENTED_EDGE('',*,*,#37263,.F.);
#50582=ORIENTED_EDGE('',*,*,#36922,.T.);
#50583=ORIENTED_EDGE('',*,*,#36920,.T.);
#50584=ORIENTED_EDGE('',*,*,#37262,.T.);
#50585=ORIENTED_EDGE('',*,*,#37264,.F.);
#50586=ORIENTED_EDGE('',*,*,#37265,.F.);
#50587=ORIENTED_EDGE('',*,*,#36926,.T.);
#50588=ORIENTED_EDGE('',*,*,#36925,.T.);
#50589=ORIENTED_EDGE('',*,*,#37266,.F.);
#50590=ORIENTED_EDGE('',*,*,#36929,.T.);
#50591=ORIENTED_EDGE('',*,*,#36927,.T.);
#50592=ORIENTED_EDGE('',*,*,#37265,.T.);
#50593=ORIENTED_EDGE('',*,*,#37267,.F.);
#50594=ORIENTED_EDGE('',*,*,#37268,.F.);
#50595=ORIENTED_EDGE('',*,*,#36933,.T.);
#50596=ORIENTED_EDGE('',*,*,#36932,.T.);
#50597=ORIENTED_EDGE('',*,*,#37269,.F.);
#50598=ORIENTED_EDGE('',*,*,#36936,.T.);
#50599=ORIENTED_EDGE('',*,*,#36934,.T.);
#50600=ORIENTED_EDGE('',*,*,#37268,.T.);
#50601=ORIENTED_EDGE('',*,*,#37270,.F.);
#50602=ORIENTED_EDGE('',*,*,#37271,.F.);
#50603=ORIENTED_EDGE('',*,*,#36940,.T.);
#50604=ORIENTED_EDGE('',*,*,#36939,.T.);
#50605=ORIENTED_EDGE('',*,*,#37272,.F.);
#50606=ORIENTED_EDGE('',*,*,#36943,.T.);
#50607=ORIENTED_EDGE('',*,*,#36941,.T.);
#50608=ORIENTED_EDGE('',*,*,#37271,.T.);
#50609=ORIENTED_EDGE('',*,*,#37273,.F.);
#50610=ORIENTED_EDGE('',*,*,#37274,.F.);
#50611=ORIENTED_EDGE('',*,*,#36947,.T.);
#50612=ORIENTED_EDGE('',*,*,#36946,.T.);
#50613=ORIENTED_EDGE('',*,*,#37275,.F.);
#50614=ORIENTED_EDGE('',*,*,#36950,.T.);
#50615=ORIENTED_EDGE('',*,*,#36948,.T.);
#50616=ORIENTED_EDGE('',*,*,#37274,.T.);
#50617=ORIENTED_EDGE('',*,*,#37276,.F.);
#50618=ORIENTED_EDGE('',*,*,#37277,.F.);
#50619=ORIENTED_EDGE('',*,*,#36954,.T.);
#50620=ORIENTED_EDGE('',*,*,#36953,.T.);
#50621=ORIENTED_EDGE('',*,*,#37278,.F.);
#50622=ORIENTED_EDGE('',*,*,#36957,.T.);
#50623=ORIENTED_EDGE('',*,*,#36955,.T.);
#50624=ORIENTED_EDGE('',*,*,#37277,.T.);
#50625=ORIENTED_EDGE('',*,*,#37279,.F.);
#50626=ORIENTED_EDGE('',*,*,#37280,.F.);
#50627=ORIENTED_EDGE('',*,*,#36961,.T.);
#50628=ORIENTED_EDGE('',*,*,#36960,.T.);
#50629=ORIENTED_EDGE('',*,*,#37281,.F.);
#50630=ORIENTED_EDGE('',*,*,#36964,.T.);
#50631=ORIENTED_EDGE('',*,*,#36962,.T.);
#50632=ORIENTED_EDGE('',*,*,#37280,.T.);
#50633=ORIENTED_EDGE('',*,*,#37282,.F.);
#50634=ORIENTED_EDGE('',*,*,#37283,.F.);
#50635=ORIENTED_EDGE('',*,*,#36968,.T.);
#50636=ORIENTED_EDGE('',*,*,#36967,.T.);
#50637=ORIENTED_EDGE('',*,*,#37284,.F.);
#50638=ORIENTED_EDGE('',*,*,#36971,.T.);
#50639=ORIENTED_EDGE('',*,*,#36969,.T.);
#50640=ORIENTED_EDGE('',*,*,#37283,.T.);
#50641=ORIENTED_EDGE('',*,*,#37285,.F.);
#50642=ORIENTED_EDGE('',*,*,#37286,.F.);
#50643=ORIENTED_EDGE('',*,*,#36977,.T.);
#50644=ORIENTED_EDGE('',*,*,#36974,.T.);
#50645=ORIENTED_EDGE('',*,*,#36978,.T.);
#50646=ORIENTED_EDGE('',*,*,#37286,.T.);
#50647=ORIENTED_EDGE('',*,*,#37287,.F.);
#50648=ORIENTED_EDGE('',*,*,#36976,.T.);
#50649=ORIENTED_EDGE('',*,*,#36983,.T.);
#50650=ORIENTED_EDGE('',*,*,#36979,.T.);
#50651=ORIENTED_EDGE('',*,*,#37288,.F.);
#50652=ORIENTED_EDGE('',*,*,#37289,.F.);
#50653=ORIENTED_EDGE('',*,*,#37290,.F.);
#50654=ORIENTED_EDGE('',*,*,#36985,.T.);
#50655=ORIENTED_EDGE('',*,*,#36984,.T.);
#50656=ORIENTED_EDGE('',*,*,#37289,.T.);
#50657=ORIENTED_EDGE('',*,*,#37291,.F.);
#50658=ORIENTED_EDGE('',*,*,#37292,.F.);
#50659=ORIENTED_EDGE('',*,*,#36989,.T.);
#50660=ORIENTED_EDGE('',*,*,#36988,.T.);
#50661=ORIENTED_EDGE('',*,*,#37293,.F.);
#50662=ORIENTED_EDGE('',*,*,#36992,.T.);
#50663=ORIENTED_EDGE('',*,*,#36990,.T.);
#50664=ORIENTED_EDGE('',*,*,#37292,.T.);
#50665=ORIENTED_EDGE('',*,*,#37294,.F.);
#50666=ORIENTED_EDGE('',*,*,#37295,.F.);
#50667=ORIENTED_EDGE('',*,*,#36996,.T.);
#50668=ORIENTED_EDGE('',*,*,#36995,.T.);
#50669=ORIENTED_EDGE('',*,*,#37296,.F.);
#50670=ORIENTED_EDGE('',*,*,#36999,.T.);
#50671=ORIENTED_EDGE('',*,*,#36997,.T.);
#50672=ORIENTED_EDGE('',*,*,#37295,.T.);
#50673=ORIENTED_EDGE('',*,*,#37297,.F.);
#50674=ORIENTED_EDGE('',*,*,#37298,.F.);
#50675=ORIENTED_EDGE('',*,*,#37003,.T.);
#50676=ORIENTED_EDGE('',*,*,#37002,.T.);
#50677=ORIENTED_EDGE('',*,*,#37299,.F.);
#50678=ORIENTED_EDGE('',*,*,#37006,.T.);
#50679=ORIENTED_EDGE('',*,*,#37004,.T.);
#50680=ORIENTED_EDGE('',*,*,#37298,.T.);
#50681=ORIENTED_EDGE('',*,*,#37300,.F.);
#50682=ORIENTED_EDGE('',*,*,#37301,.F.);
#50683=ORIENTED_EDGE('',*,*,#37010,.T.);
#50684=ORIENTED_EDGE('',*,*,#37009,.T.);
#50685=ORIENTED_EDGE('',*,*,#37302,.F.);
#50686=ORIENTED_EDGE('',*,*,#37013,.T.);
#50687=ORIENTED_EDGE('',*,*,#37011,.T.);
#50688=ORIENTED_EDGE('',*,*,#37301,.T.);
#50689=ORIENTED_EDGE('',*,*,#37303,.F.);
#50690=ORIENTED_EDGE('',*,*,#37218,.T.);
#50691=ORIENTED_EDGE('',*,*,#37014,.T.);
#50692=ORIENTED_EDGE('',*,*,#37017,.T.);
#50693=ORIENTED_EDGE('',*,*,#37214,.T.);
#50694=ORIENTED_EDGE('',*,*,#37304,.F.);
#50695=ORIENTED_EDGE('',*,*,#37305,.F.);
#50696=ORIENTED_EDGE('',*,*,#37019,.T.);
#50697=ORIENTED_EDGE('',*,*,#37026,.T.);
#50698=ORIENTED_EDGE('',*,*,#37021,.T.);
#50699=ORIENTED_EDGE('',*,*,#37306,.F.);
#50700=ORIENTED_EDGE('',*,*,#37307,.F.);
#50701=ORIENTED_EDGE('',*,*,#37027,.T.);
#50702=ORIENTED_EDGE('',*,*,#37307,.T.);
#50703=ORIENTED_EDGE('',*,*,#37308,.F.);
#50704=ORIENTED_EDGE('',*,*,#37025,.T.);
#50705=ORIENTED_EDGE('',*,*,#37033,.T.);
#50706=ORIENTED_EDGE('',*,*,#37028,.T.);
#50707=ORIENTED_EDGE('',*,*,#37309,.F.);
#50708=ORIENTED_EDGE('',*,*,#37310,.F.);
#50709=ORIENTED_EDGE('',*,*,#37034,.T.);
#50710=ORIENTED_EDGE('',*,*,#37310,.T.);
#50711=ORIENTED_EDGE('',*,*,#37311,.F.);
#50712=ORIENTED_EDGE('',*,*,#37032,.T.);
#50713=ORIENTED_EDGE('',*,*,#37040,.T.);
#50714=ORIENTED_EDGE('',*,*,#37035,.T.);
#50715=ORIENTED_EDGE('',*,*,#37312,.F.);
#50716=ORIENTED_EDGE('',*,*,#37313,.F.);
#50717=ORIENTED_EDGE('',*,*,#37041,.T.);
#50718=ORIENTED_EDGE('',*,*,#37313,.T.);
#50719=ORIENTED_EDGE('',*,*,#37314,.F.);
#50720=ORIENTED_EDGE('',*,*,#37039,.T.);
#50721=ORIENTED_EDGE('',*,*,#37047,.T.);
#50722=ORIENTED_EDGE('',*,*,#37042,.T.);
#50723=ORIENTED_EDGE('',*,*,#37315,.F.);
#50724=ORIENTED_EDGE('',*,*,#37316,.F.);
#50725=ORIENTED_EDGE('',*,*,#37048,.T.);
#50726=ORIENTED_EDGE('',*,*,#37316,.T.);
#50727=ORIENTED_EDGE('',*,*,#37317,.F.);
#50728=ORIENTED_EDGE('',*,*,#37046,.T.);
#50729=ORIENTED_EDGE('',*,*,#37054,.T.);
#50730=ORIENTED_EDGE('',*,*,#37049,.T.);
#50731=ORIENTED_EDGE('',*,*,#37318,.F.);
#50732=ORIENTED_EDGE('',*,*,#37319,.F.);
#50733=ORIENTED_EDGE('',*,*,#37055,.T.);
#50734=ORIENTED_EDGE('',*,*,#37319,.T.);
#50735=ORIENTED_EDGE('',*,*,#37320,.F.);
#50736=ORIENTED_EDGE('',*,*,#37053,.T.);
#50737=ORIENTED_EDGE('',*,*,#37061,.T.);
#50738=ORIENTED_EDGE('',*,*,#37056,.T.);
#50739=ORIENTED_EDGE('',*,*,#37321,.F.);
#50740=ORIENTED_EDGE('',*,*,#37322,.F.);
#50741=ORIENTED_EDGE('',*,*,#37062,.T.);
#50742=ORIENTED_EDGE('',*,*,#37322,.T.);
#50743=ORIENTED_EDGE('',*,*,#37323,.F.);
#50744=ORIENTED_EDGE('',*,*,#37060,.T.);
#50745=ORIENTED_EDGE('',*,*,#37068,.T.);
#50746=ORIENTED_EDGE('',*,*,#37063,.T.);
#50747=ORIENTED_EDGE('',*,*,#37324,.F.);
#50748=ORIENTED_EDGE('',*,*,#37325,.F.);
#50749=ORIENTED_EDGE('',*,*,#37069,.T.);
#50750=ORIENTED_EDGE('',*,*,#37325,.T.);
#50751=ORIENTED_EDGE('',*,*,#37326,.F.);
#50752=ORIENTED_EDGE('',*,*,#37067,.T.);
#50753=ORIENTED_EDGE('',*,*,#37075,.T.);
#50754=ORIENTED_EDGE('',*,*,#37070,.T.);
#50755=ORIENTED_EDGE('',*,*,#37327,.F.);
#50756=ORIENTED_EDGE('',*,*,#37328,.F.);
#50757=ORIENTED_EDGE('',*,*,#37076,.T.);
#50758=ORIENTED_EDGE('',*,*,#37328,.T.);
#50759=ORIENTED_EDGE('',*,*,#37329,.F.);
#50760=ORIENTED_EDGE('',*,*,#37074,.T.);
#50761=ORIENTED_EDGE('',*,*,#37082,.T.);
#50762=ORIENTED_EDGE('',*,*,#37077,.T.);
#50763=ORIENTED_EDGE('',*,*,#37330,.F.);
#50764=ORIENTED_EDGE('',*,*,#37331,.F.);
#50765=ORIENTED_EDGE('',*,*,#37083,.T.);
#50766=ORIENTED_EDGE('',*,*,#37331,.T.);
#50767=ORIENTED_EDGE('',*,*,#37332,.F.);
#50768=ORIENTED_EDGE('',*,*,#37081,.T.);
#50769=ORIENTED_EDGE('',*,*,#37089,.T.);
#50770=ORIENTED_EDGE('',*,*,#37084,.T.);
#50771=ORIENTED_EDGE('',*,*,#37333,.F.);
#50772=ORIENTED_EDGE('',*,*,#37334,.F.);
#50773=ORIENTED_EDGE('',*,*,#37090,.T.);
#50774=ORIENTED_EDGE('',*,*,#37334,.T.);
#50775=ORIENTED_EDGE('',*,*,#37335,.F.);
#50776=ORIENTED_EDGE('',*,*,#37088,.T.);
#50777=ORIENTED_EDGE('',*,*,#37096,.T.);
#50778=ORIENTED_EDGE('',*,*,#37091,.T.);
#50779=ORIENTED_EDGE('',*,*,#37336,.F.);
#50780=ORIENTED_EDGE('',*,*,#37337,.F.);
#50781=ORIENTED_EDGE('',*,*,#37097,.T.);
#50782=ORIENTED_EDGE('',*,*,#37337,.T.);
#50783=ORIENTED_EDGE('',*,*,#37338,.F.);
#50784=ORIENTED_EDGE('',*,*,#37095,.T.);
#50785=ORIENTED_EDGE('',*,*,#37103,.T.);
#50786=ORIENTED_EDGE('',*,*,#37098,.T.);
#50787=ORIENTED_EDGE('',*,*,#37339,.F.);
#50788=ORIENTED_EDGE('',*,*,#37340,.F.);
#50789=ORIENTED_EDGE('',*,*,#37104,.T.);
#50790=ORIENTED_EDGE('',*,*,#37340,.T.);
#50791=ORIENTED_EDGE('',*,*,#37341,.F.);
#50792=ORIENTED_EDGE('',*,*,#37102,.T.);
#50793=ORIENTED_EDGE('',*,*,#37110,.T.);
#50794=ORIENTED_EDGE('',*,*,#37105,.T.);
#50795=ORIENTED_EDGE('',*,*,#37342,.F.);
#50796=ORIENTED_EDGE('',*,*,#37343,.F.);
#50797=ORIENTED_EDGE('',*,*,#37111,.T.);
#50798=ORIENTED_EDGE('',*,*,#37343,.T.);
#50799=ORIENTED_EDGE('',*,*,#37344,.F.);
#50800=ORIENTED_EDGE('',*,*,#37109,.T.);
#50801=ORIENTED_EDGE('',*,*,#34436,.T.);
#50802=ORIENTED_EDGE('',*,*,#37112,.T.);
#50803=ORIENTED_EDGE('',*,*,#37345,.F.);
#50804=ORIENTED_EDGE('',*,*,#37346,.F.);
#50805=ORIENTED_EDGE('',*,*,#34433,.T.);
#50806=ORIENTED_EDGE('',*,*,#37346,.T.);
#50807=ORIENTED_EDGE('',*,*,#37347,.F.);
#50808=ORIENTED_EDGE('',*,*,#37114,.T.);
#50809=ORIENTED_EDGE('',*,*,#37120,.T.);
#50810=ORIENTED_EDGE('',*,*,#37115,.T.);
#50811=ORIENTED_EDGE('',*,*,#37348,.F.);
#50812=ORIENTED_EDGE('',*,*,#37349,.F.);
#50813=ORIENTED_EDGE('',*,*,#37121,.T.);
#50814=ORIENTED_EDGE('',*,*,#37349,.T.);
#50815=ORIENTED_EDGE('',*,*,#37350,.F.);
#50816=ORIENTED_EDGE('',*,*,#37119,.T.);
#50817=ORIENTED_EDGE('',*,*,#37127,.T.);
#50818=ORIENTED_EDGE('',*,*,#37122,.T.);
#50819=ORIENTED_EDGE('',*,*,#37351,.F.);
#50820=ORIENTED_EDGE('',*,*,#37352,.F.);
#50821=ORIENTED_EDGE('',*,*,#37128,.T.);
#50822=ORIENTED_EDGE('',*,*,#37352,.T.);
#50823=ORIENTED_EDGE('',*,*,#37353,.F.);
#50824=ORIENTED_EDGE('',*,*,#37126,.T.);
#50825=ORIENTED_EDGE('',*,*,#37134,.T.);
#50826=ORIENTED_EDGE('',*,*,#37129,.T.);
#50827=ORIENTED_EDGE('',*,*,#37354,.F.);
#50828=ORIENTED_EDGE('',*,*,#37355,.F.);
#50829=ORIENTED_EDGE('',*,*,#37135,.T.);
#50830=ORIENTED_EDGE('',*,*,#37355,.T.);
#50831=ORIENTED_EDGE('',*,*,#37356,.F.);
#50832=ORIENTED_EDGE('',*,*,#37133,.T.);
#50833=ORIENTED_EDGE('',*,*,#37141,.T.);
#50834=ORIENTED_EDGE('',*,*,#37136,.T.);
#50835=ORIENTED_EDGE('',*,*,#37357,.F.);
#50836=ORIENTED_EDGE('',*,*,#37358,.F.);
#50837=ORIENTED_EDGE('',*,*,#37142,.T.);
#50838=ORIENTED_EDGE('',*,*,#37358,.T.);
#50839=ORIENTED_EDGE('',*,*,#37359,.F.);
#50840=ORIENTED_EDGE('',*,*,#37140,.T.);
#50841=ORIENTED_EDGE('',*,*,#37148,.T.);
#50842=ORIENTED_EDGE('',*,*,#37143,.T.);
#50843=ORIENTED_EDGE('',*,*,#37360,.F.);
#50844=ORIENTED_EDGE('',*,*,#37361,.F.);
#50845=ORIENTED_EDGE('',*,*,#37149,.T.);
#50846=ORIENTED_EDGE('',*,*,#37361,.T.);
#50847=ORIENTED_EDGE('',*,*,#37362,.F.);
#50848=ORIENTED_EDGE('',*,*,#37147,.T.);
#50849=ORIENTED_EDGE('',*,*,#37155,.T.);
#50850=ORIENTED_EDGE('',*,*,#37150,.T.);
#50851=ORIENTED_EDGE('',*,*,#37363,.F.);
#50852=ORIENTED_EDGE('',*,*,#37364,.F.);
#50853=ORIENTED_EDGE('',*,*,#37156,.T.);
#50854=ORIENTED_EDGE('',*,*,#37364,.T.);
#50855=ORIENTED_EDGE('',*,*,#37365,.F.);
#50856=ORIENTED_EDGE('',*,*,#37154,.T.);
#50857=ORIENTED_EDGE('',*,*,#37162,.T.);
#50858=ORIENTED_EDGE('',*,*,#37157,.T.);
#50859=ORIENTED_EDGE('',*,*,#37366,.F.);
#50860=ORIENTED_EDGE('',*,*,#37367,.F.);
#50861=ORIENTED_EDGE('',*,*,#37163,.T.);
#50862=ORIENTED_EDGE('',*,*,#37367,.T.);
#50863=ORIENTED_EDGE('',*,*,#37368,.F.);
#50864=ORIENTED_EDGE('',*,*,#37161,.T.);
#50865=ORIENTED_EDGE('',*,*,#37169,.T.);
#50866=ORIENTED_EDGE('',*,*,#37164,.T.);
#50867=ORIENTED_EDGE('',*,*,#37369,.F.);
#50868=ORIENTED_EDGE('',*,*,#37370,.F.);
#50869=ORIENTED_EDGE('',*,*,#37170,.T.);
#50870=ORIENTED_EDGE('',*,*,#37370,.T.);
#50871=ORIENTED_EDGE('',*,*,#37371,.F.);
#50872=ORIENTED_EDGE('',*,*,#37168,.T.);
#50873=ORIENTED_EDGE('',*,*,#37176,.T.);
#50874=ORIENTED_EDGE('',*,*,#37171,.T.);
#50875=ORIENTED_EDGE('',*,*,#37372,.F.);
#50876=ORIENTED_EDGE('',*,*,#37373,.F.);
#50877=ORIENTED_EDGE('',*,*,#37177,.T.);
#50878=ORIENTED_EDGE('',*,*,#37373,.T.);
#50879=ORIENTED_EDGE('',*,*,#37374,.F.);
#50880=ORIENTED_EDGE('',*,*,#37175,.T.);
#50881=ORIENTED_EDGE('',*,*,#37183,.T.);
#50882=ORIENTED_EDGE('',*,*,#37178,.T.);
#50883=ORIENTED_EDGE('',*,*,#37375,.F.);
#50884=ORIENTED_EDGE('',*,*,#37376,.F.);
#50885=ORIENTED_EDGE('',*,*,#37184,.T.);
#50886=ORIENTED_EDGE('',*,*,#37376,.T.);
#50887=ORIENTED_EDGE('',*,*,#37377,.F.);
#50888=ORIENTED_EDGE('',*,*,#37182,.T.);
#50889=ORIENTED_EDGE('',*,*,#37190,.T.);
#50890=ORIENTED_EDGE('',*,*,#37185,.T.);
#50891=ORIENTED_EDGE('',*,*,#37378,.F.);
#50892=ORIENTED_EDGE('',*,*,#37379,.F.);
#50893=ORIENTED_EDGE('',*,*,#37191,.T.);
#50894=ORIENTED_EDGE('',*,*,#37379,.T.);
#50895=ORIENTED_EDGE('',*,*,#37380,.F.);
#50896=ORIENTED_EDGE('',*,*,#37189,.T.);
#50897=ORIENTED_EDGE('',*,*,#37197,.T.);
#50898=ORIENTED_EDGE('',*,*,#37192,.T.);
#50899=ORIENTED_EDGE('',*,*,#37381,.F.);
#50900=ORIENTED_EDGE('',*,*,#37382,.F.);
#50901=ORIENTED_EDGE('',*,*,#37198,.T.);
#50902=ORIENTED_EDGE('',*,*,#37382,.T.);
#50903=ORIENTED_EDGE('',*,*,#37383,.F.);
#50904=ORIENTED_EDGE('',*,*,#37196,.T.);
#50905=ORIENTED_EDGE('',*,*,#37204,.T.);
#50906=ORIENTED_EDGE('',*,*,#37199,.T.);
#50907=ORIENTED_EDGE('',*,*,#37384,.F.);
#50908=ORIENTED_EDGE('',*,*,#37385,.F.);
#50909=ORIENTED_EDGE('',*,*,#37205,.T.);
#50910=ORIENTED_EDGE('',*,*,#37385,.T.);
#50911=ORIENTED_EDGE('',*,*,#37386,.F.);
#50912=ORIENTED_EDGE('',*,*,#37203,.T.);
#50913=ORIENTED_EDGE('',*,*,#37211,.T.);
#50914=ORIENTED_EDGE('',*,*,#37206,.T.);
#50915=ORIENTED_EDGE('',*,*,#37387,.F.);
#50916=ORIENTED_EDGE('',*,*,#37388,.F.);
#50917=ORIENTED_EDGE('',*,*,#37212,.T.);
#50918=ORIENTED_EDGE('',*,*,#37388,.T.);
#50919=ORIENTED_EDGE('',*,*,#37389,.F.);
#50920=ORIENTED_EDGE('',*,*,#37210,.T.);
#50921=ORIENTED_EDGE('',*,*,#37390,.F.);
#50922=ORIENTED_EDGE('',*,*,#37304,.T.);
#50923=ORIENTED_EDGE('',*,*,#37213,.T.);
#50924=ORIENTED_EDGE('',*,*,#37216,.T.);
#50925=ORIENTED_EDGE('',*,*,#37391,.T.);
#50926=ORIENTED_EDGE('',*,*,#37392,.F.);
#50927=ORIENTED_EDGE('',*,*,#37217,.T.);
#50928=ORIENTED_EDGE('',*,*,#37393,.F.);
#50929=ORIENTED_EDGE('',*,*,#37394,.F.);
#50930=ORIENTED_EDGE('',*,*,#37395,.F.);
#50931=ORIENTED_EDGE('',*,*,#37396,.F.);
#50932=ORIENTED_EDGE('',*,*,#37391,.F.);
#50933=ORIENTED_EDGE('',*,*,#37396,.T.);
#50934=ORIENTED_EDGE('',*,*,#37397,.F.);
#50935=ORIENTED_EDGE('',*,*,#37219,.T.);
#50936=ORIENTED_EDGE('',*,*,#37392,.T.);
#50937=ORIENTED_EDGE('',*,*,#37398,.T.);
#50938=ORIENTED_EDGE('',*,*,#37399,.F.);
#50939=ORIENTED_EDGE('',*,*,#37221,.T.);
#50940=ORIENTED_EDGE('',*,*,#37400,.F.);
#50941=ORIENTED_EDGE('',*,*,#37401,.F.);
#50942=ORIENTED_EDGE('',*,*,#37402,.F.);
#50943=ORIENTED_EDGE('',*,*,#37403,.F.);
#50944=ORIENTED_EDGE('',*,*,#37398,.F.);
#50945=ORIENTED_EDGE('',*,*,#37403,.T.);
#50946=ORIENTED_EDGE('',*,*,#37404,.F.);
#50947=ORIENTED_EDGE('',*,*,#37222,.T.);
#50948=ORIENTED_EDGE('',*,*,#37399,.T.);
#50949=ORIENTED_EDGE('',*,*,#37405,.T.);
#50950=ORIENTED_EDGE('',*,*,#37406,.F.);
#50951=ORIENTED_EDGE('',*,*,#37224,.T.);
#50952=ORIENTED_EDGE('',*,*,#37407,.F.);
#50953=ORIENTED_EDGE('',*,*,#37408,.F.);
#50954=ORIENTED_EDGE('',*,*,#37409,.F.);
#50955=ORIENTED_EDGE('',*,*,#37410,.F.);
#50956=ORIENTED_EDGE('',*,*,#37405,.F.);
#50957=ORIENTED_EDGE('',*,*,#37410,.T.);
#50958=ORIENTED_EDGE('',*,*,#37411,.F.);
#50959=ORIENTED_EDGE('',*,*,#37225,.T.);
#50960=ORIENTED_EDGE('',*,*,#37406,.T.);
#50961=ORIENTED_EDGE('',*,*,#37412,.T.);
#50962=ORIENTED_EDGE('',*,*,#37413,.F.);
#50963=ORIENTED_EDGE('',*,*,#37227,.T.);
#50964=ORIENTED_EDGE('',*,*,#37414,.F.);
#50965=ORIENTED_EDGE('',*,*,#37415,.F.);
#50966=ORIENTED_EDGE('',*,*,#37416,.F.);
#50967=ORIENTED_EDGE('',*,*,#37417,.F.);
#50968=ORIENTED_EDGE('',*,*,#37412,.F.);
#50969=ORIENTED_EDGE('',*,*,#37417,.T.);
#50970=ORIENTED_EDGE('',*,*,#37418,.F.);
#50971=ORIENTED_EDGE('',*,*,#37228,.T.);
#50972=ORIENTED_EDGE('',*,*,#37413,.T.);
#50973=ORIENTED_EDGE('',*,*,#37419,.T.);
#50974=ORIENTED_EDGE('',*,*,#37420,.F.);
#50975=ORIENTED_EDGE('',*,*,#37230,.T.);
#50976=ORIENTED_EDGE('',*,*,#37421,.F.);
#50977=ORIENTED_EDGE('',*,*,#37422,.F.);
#50978=ORIENTED_EDGE('',*,*,#37423,.F.);
#50979=ORIENTED_EDGE('',*,*,#37424,.F.);
#50980=ORIENTED_EDGE('',*,*,#37419,.F.);
#50981=ORIENTED_EDGE('',*,*,#37424,.T.);
#50982=ORIENTED_EDGE('',*,*,#37425,.F.);
#50983=ORIENTED_EDGE('',*,*,#37231,.T.);
#50984=ORIENTED_EDGE('',*,*,#37420,.T.);
#50985=ORIENTED_EDGE('',*,*,#37426,.T.);
#50986=ORIENTED_EDGE('',*,*,#37427,.F.);
#50987=ORIENTED_EDGE('',*,*,#37233,.T.);
#50988=ORIENTED_EDGE('',*,*,#37428,.F.);
#50989=ORIENTED_EDGE('',*,*,#37429,.F.);
#50990=ORIENTED_EDGE('',*,*,#37430,.F.);
#50991=ORIENTED_EDGE('',*,*,#37431,.F.);
#50992=ORIENTED_EDGE('',*,*,#37426,.F.);
#50993=ORIENTED_EDGE('',*,*,#37431,.T.);
#50994=ORIENTED_EDGE('',*,*,#37432,.F.);
#50995=ORIENTED_EDGE('',*,*,#37234,.T.);
#50996=ORIENTED_EDGE('',*,*,#37427,.T.);
#50997=ORIENTED_EDGE('',*,*,#37433,.T.);
#50998=ORIENTED_EDGE('',*,*,#37434,.F.);
#50999=ORIENTED_EDGE('',*,*,#37236,.T.);
#51000=ORIENTED_EDGE('',*,*,#37435,.F.);
#51001=ORIENTED_EDGE('',*,*,#37436,.F.);
#51002=ORIENTED_EDGE('',*,*,#37437,.F.);
#51003=ORIENTED_EDGE('',*,*,#37438,.F.);
#51004=ORIENTED_EDGE('',*,*,#37433,.F.);
#51005=ORIENTED_EDGE('',*,*,#37438,.T.);
#51006=ORIENTED_EDGE('',*,*,#37439,.F.);
#51007=ORIENTED_EDGE('',*,*,#37237,.T.);
#51008=ORIENTED_EDGE('',*,*,#37434,.T.);
#51009=ORIENTED_EDGE('',*,*,#37440,.T.);
#51010=ORIENTED_EDGE('',*,*,#37441,.F.);
#51011=ORIENTED_EDGE('',*,*,#37239,.T.);
#51012=ORIENTED_EDGE('',*,*,#37442,.F.);
#51013=ORIENTED_EDGE('',*,*,#37443,.F.);
#51014=ORIENTED_EDGE('',*,*,#37444,.F.);
#51015=ORIENTED_EDGE('',*,*,#37445,.F.);
#51016=ORIENTED_EDGE('',*,*,#37440,.F.);
#51017=ORIENTED_EDGE('',*,*,#37445,.T.);
#51018=ORIENTED_EDGE('',*,*,#37446,.F.);
#51019=ORIENTED_EDGE('',*,*,#37240,.T.);
#51020=ORIENTED_EDGE('',*,*,#37441,.T.);
#51021=ORIENTED_EDGE('',*,*,#37447,.T.);
#51022=ORIENTED_EDGE('',*,*,#37448,.F.);
#51023=ORIENTED_EDGE('',*,*,#37242,.T.);
#51024=ORIENTED_EDGE('',*,*,#37449,.F.);
#51025=ORIENTED_EDGE('',*,*,#37450,.F.);
#51026=ORIENTED_EDGE('',*,*,#37451,.F.);
#51027=ORIENTED_EDGE('',*,*,#37452,.F.);
#51028=ORIENTED_EDGE('',*,*,#37447,.F.);
#51029=ORIENTED_EDGE('',*,*,#37452,.T.);
#51030=ORIENTED_EDGE('',*,*,#37453,.F.);
#51031=ORIENTED_EDGE('',*,*,#37243,.T.);
#51032=ORIENTED_EDGE('',*,*,#37448,.T.);
#51033=ORIENTED_EDGE('',*,*,#37454,.T.);
#51034=ORIENTED_EDGE('',*,*,#37455,.F.);
#51035=ORIENTED_EDGE('',*,*,#37245,.T.);
#51036=ORIENTED_EDGE('',*,*,#37456,.F.);
#51037=ORIENTED_EDGE('',*,*,#37457,.F.);
#51038=ORIENTED_EDGE('',*,*,#37458,.F.);
#51039=ORIENTED_EDGE('',*,*,#37459,.F.);
#51040=ORIENTED_EDGE('',*,*,#37454,.F.);
#51041=ORIENTED_EDGE('',*,*,#37459,.T.);
#51042=ORIENTED_EDGE('',*,*,#37460,.F.);
#51043=ORIENTED_EDGE('',*,*,#37246,.T.);
#51044=ORIENTED_EDGE('',*,*,#37455,.T.);
#51045=ORIENTED_EDGE('',*,*,#37461,.T.);
#51046=ORIENTED_EDGE('',*,*,#37462,.F.);
#51047=ORIENTED_EDGE('',*,*,#37248,.T.);
#51048=ORIENTED_EDGE('',*,*,#37463,.F.);
#51049=ORIENTED_EDGE('',*,*,#37464,.F.);
#51050=ORIENTED_EDGE('',*,*,#37465,.F.);
#51051=ORIENTED_EDGE('',*,*,#37466,.F.);
#51052=ORIENTED_EDGE('',*,*,#37461,.F.);
#51053=ORIENTED_EDGE('',*,*,#37466,.T.);
#51054=ORIENTED_EDGE('',*,*,#37467,.F.);
#51055=ORIENTED_EDGE('',*,*,#37249,.T.);
#51056=ORIENTED_EDGE('',*,*,#37462,.T.);
#51057=ORIENTED_EDGE('',*,*,#37468,.T.);
#51058=ORIENTED_EDGE('',*,*,#37469,.F.);
#51059=ORIENTED_EDGE('',*,*,#37251,.T.);
#51060=ORIENTED_EDGE('',*,*,#37470,.F.);
#51061=ORIENTED_EDGE('',*,*,#37471,.F.);
#51062=ORIENTED_EDGE('',*,*,#37472,.F.);
#51063=ORIENTED_EDGE('',*,*,#37473,.F.);
#51064=ORIENTED_EDGE('',*,*,#37468,.F.);
#51065=ORIENTED_EDGE('',*,*,#37473,.T.);
#51066=ORIENTED_EDGE('',*,*,#37474,.F.);
#51067=ORIENTED_EDGE('',*,*,#37252,.T.);
#51068=ORIENTED_EDGE('',*,*,#37469,.T.);
#51069=ORIENTED_EDGE('',*,*,#37475,.T.);
#51070=ORIENTED_EDGE('',*,*,#37476,.F.);
#51071=ORIENTED_EDGE('',*,*,#37254,.T.);
#51072=ORIENTED_EDGE('',*,*,#37477,.F.);
#51073=ORIENTED_EDGE('',*,*,#37478,.F.);
#51074=ORIENTED_EDGE('',*,*,#37479,.F.);
#51075=ORIENTED_EDGE('',*,*,#37480,.F.);
#51076=ORIENTED_EDGE('',*,*,#37475,.F.);
#51077=ORIENTED_EDGE('',*,*,#37480,.T.);
#51078=ORIENTED_EDGE('',*,*,#37481,.F.);
#51079=ORIENTED_EDGE('',*,*,#37255,.T.);
#51080=ORIENTED_EDGE('',*,*,#37476,.T.);
#51081=ORIENTED_EDGE('',*,*,#37482,.T.);
#51082=ORIENTED_EDGE('',*,*,#37483,.F.);
#51083=ORIENTED_EDGE('',*,*,#37257,.T.);
#51084=ORIENTED_EDGE('',*,*,#37484,.F.);
#51085=ORIENTED_EDGE('',*,*,#37485,.F.);
#51086=ORIENTED_EDGE('',*,*,#37486,.F.);
#51087=ORIENTED_EDGE('',*,*,#37487,.F.);
#51088=ORIENTED_EDGE('',*,*,#37482,.F.);
#51089=ORIENTED_EDGE('',*,*,#37487,.T.);
#51090=ORIENTED_EDGE('',*,*,#37488,.F.);
#51091=ORIENTED_EDGE('',*,*,#37258,.T.);
#51092=ORIENTED_EDGE('',*,*,#37483,.T.);
#51093=ORIENTED_EDGE('',*,*,#34429,.T.);
#51094=ORIENTED_EDGE('',*,*,#37489,.F.);
#51095=ORIENTED_EDGE('',*,*,#37260,.T.);
#51096=ORIENTED_EDGE('',*,*,#37490,.F.);
#51097=ORIENTED_EDGE('',*,*,#34432,.T.);
#51098=ORIENTED_EDGE('',*,*,#37491,.F.);
#51099=ORIENTED_EDGE('',*,*,#37261,.T.);
#51100=ORIENTED_EDGE('',*,*,#37489,.T.);
#51101=ORIENTED_EDGE('',*,*,#37492,.T.);
#51102=ORIENTED_EDGE('',*,*,#37493,.F.);
#51103=ORIENTED_EDGE('',*,*,#37263,.T.);
#51104=ORIENTED_EDGE('',*,*,#37494,.F.);
#51105=ORIENTED_EDGE('',*,*,#37495,.F.);
#51106=ORIENTED_EDGE('',*,*,#37496,.F.);
#51107=ORIENTED_EDGE('',*,*,#37497,.F.);
#51108=ORIENTED_EDGE('',*,*,#37492,.F.);
#51109=ORIENTED_EDGE('',*,*,#37497,.T.);
#51110=ORIENTED_EDGE('',*,*,#37498,.F.);
#51111=ORIENTED_EDGE('',*,*,#37264,.T.);
#51112=ORIENTED_EDGE('',*,*,#37493,.T.);
#51113=ORIENTED_EDGE('',*,*,#37499,.T.);
#51114=ORIENTED_EDGE('',*,*,#37500,.F.);
#51115=ORIENTED_EDGE('',*,*,#37266,.T.);
#51116=ORIENTED_EDGE('',*,*,#37501,.F.);
#51117=ORIENTED_EDGE('',*,*,#37502,.F.);
#51118=ORIENTED_EDGE('',*,*,#37503,.F.);
#51119=ORIENTED_EDGE('',*,*,#37504,.F.);
#51120=ORIENTED_EDGE('',*,*,#37499,.F.);
#51121=ORIENTED_EDGE('',*,*,#37504,.T.);
#51122=ORIENTED_EDGE('',*,*,#37505,.F.);
#51123=ORIENTED_EDGE('',*,*,#37267,.T.);
#51124=ORIENTED_EDGE('',*,*,#37500,.T.);
#51125=ORIENTED_EDGE('',*,*,#37506,.T.);
#51126=ORIENTED_EDGE('',*,*,#37507,.F.);
#51127=ORIENTED_EDGE('',*,*,#37269,.T.);
#51128=ORIENTED_EDGE('',*,*,#37508,.F.);
#51129=ORIENTED_EDGE('',*,*,#37509,.F.);
#51130=ORIENTED_EDGE('',*,*,#37510,.F.);
#51131=ORIENTED_EDGE('',*,*,#37511,.F.);
#51132=ORIENTED_EDGE('',*,*,#37506,.F.);
#51133=ORIENTED_EDGE('',*,*,#37511,.T.);
#51134=ORIENTED_EDGE('',*,*,#37512,.F.);
#51135=ORIENTED_EDGE('',*,*,#37270,.T.);
#51136=ORIENTED_EDGE('',*,*,#37507,.T.);
#51137=ORIENTED_EDGE('',*,*,#37513,.T.);
#51138=ORIENTED_EDGE('',*,*,#37514,.F.);
#51139=ORIENTED_EDGE('',*,*,#37272,.T.);
#51140=ORIENTED_EDGE('',*,*,#37515,.F.);
#51141=ORIENTED_EDGE('',*,*,#37516,.F.);
#51142=ORIENTED_EDGE('',*,*,#37517,.F.);
#51143=ORIENTED_EDGE('',*,*,#37518,.F.);
#51144=ORIENTED_EDGE('',*,*,#37513,.F.);
#51145=ORIENTED_EDGE('',*,*,#37518,.T.);
#51146=ORIENTED_EDGE('',*,*,#37519,.F.);
#51147=ORIENTED_EDGE('',*,*,#37273,.T.);
#51148=ORIENTED_EDGE('',*,*,#37514,.T.);
#51149=ORIENTED_EDGE('',*,*,#37520,.T.);
#51150=ORIENTED_EDGE('',*,*,#37521,.F.);
#51151=ORIENTED_EDGE('',*,*,#37275,.T.);
#51152=ORIENTED_EDGE('',*,*,#37522,.F.);
#51153=ORIENTED_EDGE('',*,*,#37523,.F.);
#51154=ORIENTED_EDGE('',*,*,#37524,.F.);
#51155=ORIENTED_EDGE('',*,*,#37525,.F.);
#51156=ORIENTED_EDGE('',*,*,#37520,.F.);
#51157=ORIENTED_EDGE('',*,*,#37525,.T.);
#51158=ORIENTED_EDGE('',*,*,#37526,.F.);
#51159=ORIENTED_EDGE('',*,*,#37276,.T.);
#51160=ORIENTED_EDGE('',*,*,#37521,.T.);
#51161=ORIENTED_EDGE('',*,*,#37527,.T.);
#51162=ORIENTED_EDGE('',*,*,#37528,.F.);
#51163=ORIENTED_EDGE('',*,*,#37278,.T.);
#51164=ORIENTED_EDGE('',*,*,#37529,.F.);
#51165=ORIENTED_EDGE('',*,*,#37530,.F.);
#51166=ORIENTED_EDGE('',*,*,#37531,.F.);
#51167=ORIENTED_EDGE('',*,*,#37532,.F.);
#51168=ORIENTED_EDGE('',*,*,#37527,.F.);
#51169=ORIENTED_EDGE('',*,*,#37532,.T.);
#51170=ORIENTED_EDGE('',*,*,#37533,.F.);
#51171=ORIENTED_EDGE('',*,*,#37279,.T.);
#51172=ORIENTED_EDGE('',*,*,#37528,.T.);
#51173=ORIENTED_EDGE('',*,*,#37534,.T.);
#51174=ORIENTED_EDGE('',*,*,#37535,.F.);
#51175=ORIENTED_EDGE('',*,*,#37281,.T.);
#51176=ORIENTED_EDGE('',*,*,#37536,.F.);
#51177=ORIENTED_EDGE('',*,*,#37537,.F.);
#51178=ORIENTED_EDGE('',*,*,#37538,.F.);
#51179=ORIENTED_EDGE('',*,*,#37539,.F.);
#51180=ORIENTED_EDGE('',*,*,#37534,.F.);
#51181=ORIENTED_EDGE('',*,*,#37539,.T.);
#51182=ORIENTED_EDGE('',*,*,#37540,.F.);
#51183=ORIENTED_EDGE('',*,*,#37282,.T.);
#51184=ORIENTED_EDGE('',*,*,#37535,.T.);
#51185=ORIENTED_EDGE('',*,*,#37541,.T.);
#51186=ORIENTED_EDGE('',*,*,#37542,.F.);
#51187=ORIENTED_EDGE('',*,*,#37284,.T.);
#51188=ORIENTED_EDGE('',*,*,#37543,.F.);
#51189=ORIENTED_EDGE('',*,*,#37544,.T.);
#51190=ORIENTED_EDGE('',*,*,#37545,.F.);
#51191=ORIENTED_EDGE('',*,*,#37285,.T.);
#51192=ORIENTED_EDGE('',*,*,#37542,.T.);
#51193=ORIENTED_EDGE('',*,*,#37546,.F.);
#51194=ORIENTED_EDGE('',*,*,#37547,.F.);
#51195=ORIENTED_EDGE('',*,*,#37544,.F.);
#51196=ORIENTED_EDGE('',*,*,#37541,.F.);
#51197=ORIENTED_EDGE('',*,*,#37287,.T.);
#51198=ORIENTED_EDGE('',*,*,#37548,.F.);
#51199=ORIENTED_EDGE('',*,*,#37549,.T.);
#51200=ORIENTED_EDGE('',*,*,#37550,.F.);
#51201=ORIENTED_EDGE('',*,*,#37551,.F.);
#51202=ORIENTED_EDGE('',*,*,#37549,.F.);
#51203=ORIENTED_EDGE('',*,*,#37552,.F.);
#51204=ORIENTED_EDGE('',*,*,#37553,.F.);
#51205=ORIENTED_EDGE('',*,*,#37288,.T.);
#51206=ORIENTED_EDGE('',*,*,#37550,.T.);
#51207=ORIENTED_EDGE('',*,*,#37551,.T.);
#51208=ORIENTED_EDGE('',*,*,#37554,.F.);
#51209=ORIENTED_EDGE('',*,*,#37555,.T.);
#51210=ORIENTED_EDGE('',*,*,#37556,.F.);
#51211=ORIENTED_EDGE('',*,*,#37290,.T.);
#51212=ORIENTED_EDGE('',*,*,#37557,.F.);
#51213=ORIENTED_EDGE('',*,*,#37558,.F.);
#51214=ORIENTED_EDGE('',*,*,#37559,.F.);
#51215=ORIENTED_EDGE('',*,*,#37560,.F.);
#51216=ORIENTED_EDGE('',*,*,#37555,.F.);
#51217=ORIENTED_EDGE('',*,*,#37560,.T.);
#51218=ORIENTED_EDGE('',*,*,#37561,.F.);
#51219=ORIENTED_EDGE('',*,*,#37291,.T.);
#51220=ORIENTED_EDGE('',*,*,#37556,.T.);
#51221=ORIENTED_EDGE('',*,*,#37562,.T.);
#51222=ORIENTED_EDGE('',*,*,#37563,.F.);
#51223=ORIENTED_EDGE('',*,*,#37293,.T.);
#51224=ORIENTED_EDGE('',*,*,#37564,.F.);
#51225=ORIENTED_EDGE('',*,*,#37565,.F.);
#51226=ORIENTED_EDGE('',*,*,#37566,.F.);
#51227=ORIENTED_EDGE('',*,*,#37567,.F.);
#51228=ORIENTED_EDGE('',*,*,#37562,.F.);
#51229=ORIENTED_EDGE('',*,*,#37567,.T.);
#51230=ORIENTED_EDGE('',*,*,#37568,.F.);
#51231=ORIENTED_EDGE('',*,*,#37294,.T.);
#51232=ORIENTED_EDGE('',*,*,#37563,.T.);
#51233=ORIENTED_EDGE('',*,*,#37569,.T.);
#51234=ORIENTED_EDGE('',*,*,#37570,.F.);
#51235=ORIENTED_EDGE('',*,*,#37296,.T.);
#51236=ORIENTED_EDGE('',*,*,#37571,.F.);
#51237=ORIENTED_EDGE('',*,*,#37572,.F.);
#51238=ORIENTED_EDGE('',*,*,#37573,.F.);
#51239=ORIENTED_EDGE('',*,*,#37574,.F.);
#51240=ORIENTED_EDGE('',*,*,#37569,.F.);
#51241=ORIENTED_EDGE('',*,*,#37574,.T.);
#51242=ORIENTED_EDGE('',*,*,#37575,.F.);
#51243=ORIENTED_EDGE('',*,*,#37297,.T.);
#51244=ORIENTED_EDGE('',*,*,#37570,.T.);
#51245=ORIENTED_EDGE('',*,*,#37576,.T.);
#51246=ORIENTED_EDGE('',*,*,#37577,.F.);
#51247=ORIENTED_EDGE('',*,*,#37299,.T.);
#51248=ORIENTED_EDGE('',*,*,#37578,.F.);
#51249=ORIENTED_EDGE('',*,*,#37579,.F.);
#51250=ORIENTED_EDGE('',*,*,#37580,.F.);
#51251=ORIENTED_EDGE('',*,*,#37581,.F.);
#51252=ORIENTED_EDGE('',*,*,#37576,.F.);
#51253=ORIENTED_EDGE('',*,*,#37581,.T.);
#51254=ORIENTED_EDGE('',*,*,#37582,.F.);
#51255=ORIENTED_EDGE('',*,*,#37300,.T.);
#51256=ORIENTED_EDGE('',*,*,#37577,.T.);
#51257=ORIENTED_EDGE('',*,*,#37583,.T.);
#51258=ORIENTED_EDGE('',*,*,#37584,.F.);
#51259=ORIENTED_EDGE('',*,*,#37302,.T.);
#51260=ORIENTED_EDGE('',*,*,#37585,.F.);
#51261=ORIENTED_EDGE('',*,*,#37586,.F.);
#51262=ORIENTED_EDGE('',*,*,#37587,.F.);
#51263=ORIENTED_EDGE('',*,*,#37588,.F.);
#51264=ORIENTED_EDGE('',*,*,#37583,.F.);
#51265=ORIENTED_EDGE('',*,*,#37588,.T.);
#51266=ORIENTED_EDGE('',*,*,#37589,.F.);
#51267=ORIENTED_EDGE('',*,*,#37303,.T.);
#51268=ORIENTED_EDGE('',*,*,#37584,.T.);
#51269=ORIENTED_EDGE('',*,*,#37305,.T.);
#51270=ORIENTED_EDGE('',*,*,#37590,.F.);
#51271=ORIENTED_EDGE('',*,*,#37591,.T.);
#51272=ORIENTED_EDGE('',*,*,#37592,.F.);
#51273=ORIENTED_EDGE('',*,*,#37306,.T.);
#51274=ORIENTED_EDGE('',*,*,#37592,.T.);
#51275=ORIENTED_EDGE('',*,*,#37593,.T.);
#51276=ORIENTED_EDGE('',*,*,#37594,.F.);
#51277=ORIENTED_EDGE('',*,*,#37593,.F.);
#51278=ORIENTED_EDGE('',*,*,#37591,.F.);
#51279=ORIENTED_EDGE('',*,*,#37595,.F.);
#51280=ORIENTED_EDGE('',*,*,#37596,.F.);
#51281=ORIENTED_EDGE('',*,*,#37308,.T.);
#51282=ORIENTED_EDGE('',*,*,#37597,.F.);
#51283=ORIENTED_EDGE('',*,*,#37598,.T.);
#51284=ORIENTED_EDGE('',*,*,#37599,.F.);
#51285=ORIENTED_EDGE('',*,*,#37309,.T.);
#51286=ORIENTED_EDGE('',*,*,#37599,.T.);
#51287=ORIENTED_EDGE('',*,*,#37600,.T.);
#51288=ORIENTED_EDGE('',*,*,#37601,.F.);
#51289=ORIENTED_EDGE('',*,*,#37600,.F.);
#51290=ORIENTED_EDGE('',*,*,#37598,.F.);
#51291=ORIENTED_EDGE('',*,*,#37602,.F.);
#51292=ORIENTED_EDGE('',*,*,#37603,.F.);
#51293=ORIENTED_EDGE('',*,*,#37311,.T.);
#51294=ORIENTED_EDGE('',*,*,#37604,.F.);
#51295=ORIENTED_EDGE('',*,*,#37605,.T.);
#51296=ORIENTED_EDGE('',*,*,#37606,.F.);
#51297=ORIENTED_EDGE('',*,*,#37312,.T.);
#51298=ORIENTED_EDGE('',*,*,#37606,.T.);
#51299=ORIENTED_EDGE('',*,*,#37607,.T.);
#51300=ORIENTED_EDGE('',*,*,#37608,.F.);
#51301=ORIENTED_EDGE('',*,*,#37607,.F.);
#51302=ORIENTED_EDGE('',*,*,#37605,.F.);
#51303=ORIENTED_EDGE('',*,*,#37609,.F.);
#51304=ORIENTED_EDGE('',*,*,#37610,.F.);
#51305=ORIENTED_EDGE('',*,*,#37314,.T.);
#51306=ORIENTED_EDGE('',*,*,#37611,.F.);
#51307=ORIENTED_EDGE('',*,*,#37612,.T.);
#51308=ORIENTED_EDGE('',*,*,#37613,.F.);
#51309=ORIENTED_EDGE('',*,*,#37315,.T.);
#51310=ORIENTED_EDGE('',*,*,#37613,.T.);
#51311=ORIENTED_EDGE('',*,*,#37614,.T.);
#51312=ORIENTED_EDGE('',*,*,#37615,.F.);
#51313=ORIENTED_EDGE('',*,*,#37614,.F.);
#51314=ORIENTED_EDGE('',*,*,#37612,.F.);
#51315=ORIENTED_EDGE('',*,*,#37616,.F.);
#51316=ORIENTED_EDGE('',*,*,#37617,.F.);
#51317=ORIENTED_EDGE('',*,*,#37317,.T.);
#51318=ORIENTED_EDGE('',*,*,#37618,.F.);
#51319=ORIENTED_EDGE('',*,*,#37619,.T.);
#51320=ORIENTED_EDGE('',*,*,#37620,.F.);
#51321=ORIENTED_EDGE('',*,*,#37318,.T.);
#51322=ORIENTED_EDGE('',*,*,#37620,.T.);
#51323=ORIENTED_EDGE('',*,*,#37621,.T.);
#51324=ORIENTED_EDGE('',*,*,#37622,.F.);
#51325=ORIENTED_EDGE('',*,*,#37621,.F.);
#51326=ORIENTED_EDGE('',*,*,#37619,.F.);
#51327=ORIENTED_EDGE('',*,*,#37623,.F.);
#51328=ORIENTED_EDGE('',*,*,#37624,.F.);
#51329=ORIENTED_EDGE('',*,*,#37320,.T.);
#51330=ORIENTED_EDGE('',*,*,#37625,.F.);
#51331=ORIENTED_EDGE('',*,*,#37626,.T.);
#51332=ORIENTED_EDGE('',*,*,#37627,.F.);
#51333=ORIENTED_EDGE('',*,*,#37321,.T.);
#51334=ORIENTED_EDGE('',*,*,#37627,.T.);
#51335=ORIENTED_EDGE('',*,*,#37628,.T.);
#51336=ORIENTED_EDGE('',*,*,#37629,.F.);
#51337=ORIENTED_EDGE('',*,*,#37628,.F.);
#51338=ORIENTED_EDGE('',*,*,#37626,.F.);
#51339=ORIENTED_EDGE('',*,*,#37630,.F.);
#51340=ORIENTED_EDGE('',*,*,#37631,.F.);
#51341=ORIENTED_EDGE('',*,*,#37323,.T.);
#51342=ORIENTED_EDGE('',*,*,#37632,.F.);
#51343=ORIENTED_EDGE('',*,*,#37633,.T.);
#51344=ORIENTED_EDGE('',*,*,#37634,.F.);
#51345=ORIENTED_EDGE('',*,*,#37324,.T.);
#51346=ORIENTED_EDGE('',*,*,#37634,.T.);
#51347=ORIENTED_EDGE('',*,*,#37635,.T.);
#51348=ORIENTED_EDGE('',*,*,#37636,.F.);
#51349=ORIENTED_EDGE('',*,*,#37635,.F.);
#51350=ORIENTED_EDGE('',*,*,#37633,.F.);
#51351=ORIENTED_EDGE('',*,*,#37637,.F.);
#51352=ORIENTED_EDGE('',*,*,#37638,.F.);
#51353=ORIENTED_EDGE('',*,*,#37326,.T.);
#51354=ORIENTED_EDGE('',*,*,#37639,.F.);
#51355=ORIENTED_EDGE('',*,*,#37640,.T.);
#51356=ORIENTED_EDGE('',*,*,#37641,.F.);
#51357=ORIENTED_EDGE('',*,*,#37327,.T.);
#51358=ORIENTED_EDGE('',*,*,#37641,.T.);
#51359=ORIENTED_EDGE('',*,*,#37642,.T.);
#51360=ORIENTED_EDGE('',*,*,#37643,.F.);
#51361=ORIENTED_EDGE('',*,*,#37642,.F.);
#51362=ORIENTED_EDGE('',*,*,#37640,.F.);
#51363=ORIENTED_EDGE('',*,*,#37644,.F.);
#51364=ORIENTED_EDGE('',*,*,#37645,.F.);
#51365=ORIENTED_EDGE('',*,*,#37329,.T.);
#51366=ORIENTED_EDGE('',*,*,#37646,.F.);
#51367=ORIENTED_EDGE('',*,*,#37647,.T.);
#51368=ORIENTED_EDGE('',*,*,#37648,.F.);
#51369=ORIENTED_EDGE('',*,*,#37330,.T.);
#51370=ORIENTED_EDGE('',*,*,#37648,.T.);
#51371=ORIENTED_EDGE('',*,*,#37649,.T.);
#51372=ORIENTED_EDGE('',*,*,#37650,.F.);
#51373=ORIENTED_EDGE('',*,*,#37649,.F.);
#51374=ORIENTED_EDGE('',*,*,#37647,.F.);
#51375=ORIENTED_EDGE('',*,*,#37651,.F.);
#51376=ORIENTED_EDGE('',*,*,#37652,.F.);
#51377=ORIENTED_EDGE('',*,*,#37332,.T.);
#51378=ORIENTED_EDGE('',*,*,#37653,.F.);
#51379=ORIENTED_EDGE('',*,*,#37654,.T.);
#51380=ORIENTED_EDGE('',*,*,#37655,.F.);
#51381=ORIENTED_EDGE('',*,*,#37333,.T.);
#51382=ORIENTED_EDGE('',*,*,#37655,.T.);
#51383=ORIENTED_EDGE('',*,*,#37656,.T.);
#51384=ORIENTED_EDGE('',*,*,#37657,.F.);
#51385=ORIENTED_EDGE('',*,*,#37656,.F.);
#51386=ORIENTED_EDGE('',*,*,#37654,.F.);
#51387=ORIENTED_EDGE('',*,*,#37658,.F.);
#51388=ORIENTED_EDGE('',*,*,#37659,.F.);
#51389=ORIENTED_EDGE('',*,*,#37335,.T.);
#51390=ORIENTED_EDGE('',*,*,#37660,.F.);
#51391=ORIENTED_EDGE('',*,*,#37661,.T.);
#51392=ORIENTED_EDGE('',*,*,#37662,.F.);
#51393=ORIENTED_EDGE('',*,*,#37336,.T.);
#51394=ORIENTED_EDGE('',*,*,#37662,.T.);
#51395=ORIENTED_EDGE('',*,*,#37663,.T.);
#51396=ORIENTED_EDGE('',*,*,#37664,.F.);
#51397=ORIENTED_EDGE('',*,*,#37663,.F.);
#51398=ORIENTED_EDGE('',*,*,#37661,.F.);
#51399=ORIENTED_EDGE('',*,*,#37665,.F.);
#51400=ORIENTED_EDGE('',*,*,#37666,.F.);
#51401=ORIENTED_EDGE('',*,*,#37338,.T.);
#51402=ORIENTED_EDGE('',*,*,#37667,.F.);
#51403=ORIENTED_EDGE('',*,*,#37668,.T.);
#51404=ORIENTED_EDGE('',*,*,#37669,.F.);
#51405=ORIENTED_EDGE('',*,*,#37339,.T.);
#51406=ORIENTED_EDGE('',*,*,#37669,.T.);
#51407=ORIENTED_EDGE('',*,*,#37670,.T.);
#51408=ORIENTED_EDGE('',*,*,#37671,.F.);
#51409=ORIENTED_EDGE('',*,*,#37670,.F.);
#51410=ORIENTED_EDGE('',*,*,#37668,.F.);
#51411=ORIENTED_EDGE('',*,*,#37672,.F.);
#51412=ORIENTED_EDGE('',*,*,#37673,.F.);
#51413=ORIENTED_EDGE('',*,*,#37341,.T.);
#51414=ORIENTED_EDGE('',*,*,#37674,.F.);
#51415=ORIENTED_EDGE('',*,*,#37675,.T.);
#51416=ORIENTED_EDGE('',*,*,#37676,.F.);
#51417=ORIENTED_EDGE('',*,*,#37342,.T.);
#51418=ORIENTED_EDGE('',*,*,#37676,.T.);
#51419=ORIENTED_EDGE('',*,*,#37677,.T.);
#51420=ORIENTED_EDGE('',*,*,#37678,.F.);
#51421=ORIENTED_EDGE('',*,*,#37677,.F.);
#51422=ORIENTED_EDGE('',*,*,#37675,.F.);
#51423=ORIENTED_EDGE('',*,*,#37679,.F.);
#51424=ORIENTED_EDGE('',*,*,#37680,.F.);
#51425=ORIENTED_EDGE('',*,*,#37344,.T.);
#51426=ORIENTED_EDGE('',*,*,#37681,.F.);
#51427=ORIENTED_EDGE('',*,*,#37682,.T.);
#51428=ORIENTED_EDGE('',*,*,#37683,.F.);
#51429=ORIENTED_EDGE('',*,*,#37345,.T.);
#51430=ORIENTED_EDGE('',*,*,#37683,.T.);
#51431=ORIENTED_EDGE('',*,*,#37684,.T.);
#51432=ORIENTED_EDGE('',*,*,#37685,.F.);
#51433=ORIENTED_EDGE('',*,*,#37684,.F.);
#51434=ORIENTED_EDGE('',*,*,#37682,.F.);
#51435=ORIENTED_EDGE('',*,*,#37686,.F.);
#51436=ORIENTED_EDGE('',*,*,#37687,.F.);
#51437=ORIENTED_EDGE('',*,*,#37347,.T.);
#51438=ORIENTED_EDGE('',*,*,#37688,.F.);
#51439=ORIENTED_EDGE('',*,*,#37689,.T.);
#51440=ORIENTED_EDGE('',*,*,#37690,.F.);
#51441=ORIENTED_EDGE('',*,*,#37348,.T.);
#51442=ORIENTED_EDGE('',*,*,#37690,.T.);
#51443=ORIENTED_EDGE('',*,*,#37691,.T.);
#51444=ORIENTED_EDGE('',*,*,#37692,.F.);
#51445=ORIENTED_EDGE('',*,*,#37691,.F.);
#51446=ORIENTED_EDGE('',*,*,#37689,.F.);
#51447=ORIENTED_EDGE('',*,*,#37693,.F.);
#51448=ORIENTED_EDGE('',*,*,#37694,.F.);
#51449=ORIENTED_EDGE('',*,*,#37350,.T.);
#51450=ORIENTED_EDGE('',*,*,#37695,.F.);
#51451=ORIENTED_EDGE('',*,*,#37696,.T.);
#51452=ORIENTED_EDGE('',*,*,#37697,.F.);
#51453=ORIENTED_EDGE('',*,*,#37351,.T.);
#51454=ORIENTED_EDGE('',*,*,#37697,.T.);
#51455=ORIENTED_EDGE('',*,*,#37698,.T.);
#51456=ORIENTED_EDGE('',*,*,#37699,.F.);
#51457=ORIENTED_EDGE('',*,*,#37698,.F.);
#51458=ORIENTED_EDGE('',*,*,#37696,.F.);
#51459=ORIENTED_EDGE('',*,*,#37700,.F.);
#51460=ORIENTED_EDGE('',*,*,#37701,.F.);
#51461=ORIENTED_EDGE('',*,*,#37353,.T.);
#51462=ORIENTED_EDGE('',*,*,#37702,.F.);
#51463=ORIENTED_EDGE('',*,*,#37703,.T.);
#51464=ORIENTED_EDGE('',*,*,#37704,.F.);
#51465=ORIENTED_EDGE('',*,*,#37354,.T.);
#51466=ORIENTED_EDGE('',*,*,#37704,.T.);
#51467=ORIENTED_EDGE('',*,*,#37705,.T.);
#51468=ORIENTED_EDGE('',*,*,#37706,.F.);
#51469=ORIENTED_EDGE('',*,*,#37705,.F.);
#51470=ORIENTED_EDGE('',*,*,#37703,.F.);
#51471=ORIENTED_EDGE('',*,*,#37707,.F.);
#51472=ORIENTED_EDGE('',*,*,#37708,.F.);
#51473=ORIENTED_EDGE('',*,*,#37356,.T.);
#51474=ORIENTED_EDGE('',*,*,#37709,.F.);
#51475=ORIENTED_EDGE('',*,*,#37710,.T.);
#51476=ORIENTED_EDGE('',*,*,#37711,.F.);
#51477=ORIENTED_EDGE('',*,*,#37357,.T.);
#51478=ORIENTED_EDGE('',*,*,#37711,.T.);
#51479=ORIENTED_EDGE('',*,*,#37712,.T.);
#51480=ORIENTED_EDGE('',*,*,#37713,.F.);
#51481=ORIENTED_EDGE('',*,*,#37712,.F.);
#51482=ORIENTED_EDGE('',*,*,#37710,.F.);
#51483=ORIENTED_EDGE('',*,*,#37714,.F.);
#51484=ORIENTED_EDGE('',*,*,#37715,.F.);
#51485=ORIENTED_EDGE('',*,*,#37359,.T.);
#51486=ORIENTED_EDGE('',*,*,#37716,.F.);
#51487=ORIENTED_EDGE('',*,*,#37717,.T.);
#51488=ORIENTED_EDGE('',*,*,#37718,.F.);
#51489=ORIENTED_EDGE('',*,*,#37360,.T.);
#51490=ORIENTED_EDGE('',*,*,#37718,.T.);
#51491=ORIENTED_EDGE('',*,*,#37719,.T.);
#51492=ORIENTED_EDGE('',*,*,#37720,.F.);
#51493=ORIENTED_EDGE('',*,*,#37719,.F.);
#51494=ORIENTED_EDGE('',*,*,#37717,.F.);
#51495=ORIENTED_EDGE('',*,*,#37721,.F.);
#51496=ORIENTED_EDGE('',*,*,#37722,.F.);
#51497=ORIENTED_EDGE('',*,*,#37362,.T.);
#51498=ORIENTED_EDGE('',*,*,#37723,.F.);
#51499=ORIENTED_EDGE('',*,*,#37724,.T.);
#51500=ORIENTED_EDGE('',*,*,#37725,.F.);
#51501=ORIENTED_EDGE('',*,*,#37363,.T.);
#51502=ORIENTED_EDGE('',*,*,#37725,.T.);
#51503=ORIENTED_EDGE('',*,*,#37726,.T.);
#51504=ORIENTED_EDGE('',*,*,#37727,.F.);
#51505=ORIENTED_EDGE('',*,*,#37726,.F.);
#51506=ORIENTED_EDGE('',*,*,#37724,.F.);
#51507=ORIENTED_EDGE('',*,*,#37728,.F.);
#51508=ORIENTED_EDGE('',*,*,#37729,.F.);
#51509=ORIENTED_EDGE('',*,*,#37365,.T.);
#51510=ORIENTED_EDGE('',*,*,#37730,.F.);
#51511=ORIENTED_EDGE('',*,*,#37731,.T.);
#51512=ORIENTED_EDGE('',*,*,#37732,.F.);
#51513=ORIENTED_EDGE('',*,*,#37366,.T.);
#51514=ORIENTED_EDGE('',*,*,#37732,.T.);
#51515=ORIENTED_EDGE('',*,*,#37733,.T.);
#51516=ORIENTED_EDGE('',*,*,#37734,.F.);
#51517=ORIENTED_EDGE('',*,*,#37733,.F.);
#51518=ORIENTED_EDGE('',*,*,#37731,.F.);
#51519=ORIENTED_EDGE('',*,*,#37735,.F.);
#51520=ORIENTED_EDGE('',*,*,#37736,.F.);
#51521=ORIENTED_EDGE('',*,*,#37368,.T.);
#51522=ORIENTED_EDGE('',*,*,#37737,.F.);
#51523=ORIENTED_EDGE('',*,*,#34428,.T.);
#51524=ORIENTED_EDGE('',*,*,#37738,.F.);
#51525=ORIENTED_EDGE('',*,*,#37369,.T.);
#51526=ORIENTED_EDGE('',*,*,#37738,.T.);
#51527=ORIENTED_EDGE('',*,*,#34427,.T.);
#51528=ORIENTED_EDGE('',*,*,#37739,.F.);
#51529=ORIENTED_EDGE('',*,*,#37371,.T.);
#51530=ORIENTED_EDGE('',*,*,#37740,.F.);
#51531=ORIENTED_EDGE('',*,*,#37741,.T.);
#51532=ORIENTED_EDGE('',*,*,#37742,.F.);
#51533=ORIENTED_EDGE('',*,*,#37372,.T.);
#51534=ORIENTED_EDGE('',*,*,#37742,.T.);
#51535=ORIENTED_EDGE('',*,*,#37743,.T.);
#51536=ORIENTED_EDGE('',*,*,#37744,.F.);
#51537=ORIENTED_EDGE('',*,*,#37743,.F.);
#51538=ORIENTED_EDGE('',*,*,#37741,.F.);
#51539=ORIENTED_EDGE('',*,*,#37745,.F.);
#51540=ORIENTED_EDGE('',*,*,#37746,.F.);
#51541=ORIENTED_EDGE('',*,*,#37374,.T.);
#51542=ORIENTED_EDGE('',*,*,#37747,.F.);
#51543=ORIENTED_EDGE('',*,*,#37748,.T.);
#51544=ORIENTED_EDGE('',*,*,#37749,.F.);
#51545=ORIENTED_EDGE('',*,*,#37375,.T.);
#51546=ORIENTED_EDGE('',*,*,#37749,.T.);
#51547=ORIENTED_EDGE('',*,*,#37750,.T.);
#51548=ORIENTED_EDGE('',*,*,#37751,.F.);
#51549=ORIENTED_EDGE('',*,*,#37750,.F.);
#51550=ORIENTED_EDGE('',*,*,#37748,.F.);
#51551=ORIENTED_EDGE('',*,*,#37752,.F.);
#51552=ORIENTED_EDGE('',*,*,#37753,.F.);
#51553=ORIENTED_EDGE('',*,*,#37377,.T.);
#51554=ORIENTED_EDGE('',*,*,#37754,.F.);
#51555=ORIENTED_EDGE('',*,*,#37755,.T.);
#51556=ORIENTED_EDGE('',*,*,#37756,.F.);
#51557=ORIENTED_EDGE('',*,*,#37378,.T.);
#51558=ORIENTED_EDGE('',*,*,#37756,.T.);
#51559=ORIENTED_EDGE('',*,*,#37757,.T.);
#51560=ORIENTED_EDGE('',*,*,#37758,.F.);
#51561=ORIENTED_EDGE('',*,*,#37757,.F.);
#51562=ORIENTED_EDGE('',*,*,#37755,.F.);
#51563=ORIENTED_EDGE('',*,*,#37759,.F.);
#51564=ORIENTED_EDGE('',*,*,#37760,.F.);
#51565=ORIENTED_EDGE('',*,*,#37380,.T.);
#51566=ORIENTED_EDGE('',*,*,#37761,.F.);
#51567=ORIENTED_EDGE('',*,*,#37762,.T.);
#51568=ORIENTED_EDGE('',*,*,#37763,.F.);
#51569=ORIENTED_EDGE('',*,*,#37381,.T.);
#51570=ORIENTED_EDGE('',*,*,#37763,.T.);
#51571=ORIENTED_EDGE('',*,*,#37764,.T.);
#51572=ORIENTED_EDGE('',*,*,#37765,.F.);
#51573=ORIENTED_EDGE('',*,*,#37764,.F.);
#51574=ORIENTED_EDGE('',*,*,#37762,.F.);
#51575=ORIENTED_EDGE('',*,*,#37766,.F.);
#51576=ORIENTED_EDGE('',*,*,#37767,.F.);
#51577=ORIENTED_EDGE('',*,*,#37383,.T.);
#51578=ORIENTED_EDGE('',*,*,#37768,.F.);
#51579=ORIENTED_EDGE('',*,*,#37769,.T.);
#51580=ORIENTED_EDGE('',*,*,#37770,.F.);
#51581=ORIENTED_EDGE('',*,*,#37384,.T.);
#51582=ORIENTED_EDGE('',*,*,#37770,.T.);
#51583=ORIENTED_EDGE('',*,*,#37771,.T.);
#51584=ORIENTED_EDGE('',*,*,#37772,.F.);
#51585=ORIENTED_EDGE('',*,*,#37771,.F.);
#51586=ORIENTED_EDGE('',*,*,#37769,.F.);
#51587=ORIENTED_EDGE('',*,*,#37773,.F.);
#51588=ORIENTED_EDGE('',*,*,#37774,.F.);
#51589=ORIENTED_EDGE('',*,*,#37386,.T.);
#51590=ORIENTED_EDGE('',*,*,#37775,.F.);
#51591=ORIENTED_EDGE('',*,*,#37776,.T.);
#51592=ORIENTED_EDGE('',*,*,#37777,.F.);
#51593=ORIENTED_EDGE('',*,*,#37387,.T.);
#51594=ORIENTED_EDGE('',*,*,#37777,.T.);
#51595=ORIENTED_EDGE('',*,*,#37778,.T.);
#51596=ORIENTED_EDGE('',*,*,#37779,.F.);
#51597=ORIENTED_EDGE('',*,*,#37778,.F.);
#51598=ORIENTED_EDGE('',*,*,#37776,.F.);
#51599=ORIENTED_EDGE('',*,*,#37780,.F.);
#51600=ORIENTED_EDGE('',*,*,#37781,.F.);
#51601=ORIENTED_EDGE('',*,*,#37389,.T.);
#51602=ORIENTED_EDGE('',*,*,#37782,.F.);
#51603=ORIENTED_EDGE('',*,*,#37783,.T.);
#51604=ORIENTED_EDGE('',*,*,#37784,.F.);
#51605=ORIENTED_EDGE('',*,*,#37785,.T.);
#51606=ORIENTED_EDGE('',*,*,#37786,.F.);
#51607=ORIENTED_EDGE('',*,*,#37390,.T.);
#51608=ORIENTED_EDGE('',*,*,#37784,.T.);
#51609=ORIENTED_EDGE('',*,*,#37787,.F.);
#51610=ORIENTED_EDGE('',*,*,#37788,.F.);
#51611=ORIENTED_EDGE('',*,*,#37785,.F.);
#51612=ORIENTED_EDGE('',*,*,#37783,.F.);
#51613=ORIENTED_EDGE('',*,*,#37789,.F.);
#51614=ORIENTED_EDGE('',*,*,#37790,.F.);
#51615=ORIENTED_EDGE('',*,*,#37394,.T.);
#51616=ORIENTED_EDGE('',*,*,#37393,.T.);
#51617=ORIENTED_EDGE('',*,*,#37791,.F.);
#51618=ORIENTED_EDGE('',*,*,#37397,.T.);
#51619=ORIENTED_EDGE('',*,*,#37395,.T.);
#51620=ORIENTED_EDGE('',*,*,#37790,.T.);
#51621=ORIENTED_EDGE('',*,*,#37792,.F.);
#51622=ORIENTED_EDGE('',*,*,#37793,.F.);
#51623=ORIENTED_EDGE('',*,*,#37401,.T.);
#51624=ORIENTED_EDGE('',*,*,#37400,.T.);
#51625=ORIENTED_EDGE('',*,*,#37794,.F.);
#51626=ORIENTED_EDGE('',*,*,#37404,.T.);
#51627=ORIENTED_EDGE('',*,*,#37402,.T.);
#51628=ORIENTED_EDGE('',*,*,#37793,.T.);
#51629=ORIENTED_EDGE('',*,*,#37795,.F.);
#51630=ORIENTED_EDGE('',*,*,#37796,.F.);
#51631=ORIENTED_EDGE('',*,*,#37408,.T.);
#51632=ORIENTED_EDGE('',*,*,#37407,.T.);
#51633=ORIENTED_EDGE('',*,*,#37797,.F.);
#51634=ORIENTED_EDGE('',*,*,#37411,.T.);
#51635=ORIENTED_EDGE('',*,*,#37409,.T.);
#51636=ORIENTED_EDGE('',*,*,#37796,.T.);
#51637=ORIENTED_EDGE('',*,*,#37798,.F.);
#51638=ORIENTED_EDGE('',*,*,#37799,.F.);
#51639=ORIENTED_EDGE('',*,*,#37415,.T.);
#51640=ORIENTED_EDGE('',*,*,#37414,.T.);
#51641=ORIENTED_EDGE('',*,*,#37800,.F.);
#51642=ORIENTED_EDGE('',*,*,#37418,.T.);
#51643=ORIENTED_EDGE('',*,*,#37416,.T.);
#51644=ORIENTED_EDGE('',*,*,#37799,.T.);
#51645=ORIENTED_EDGE('',*,*,#37801,.F.);
#51646=ORIENTED_EDGE('',*,*,#37802,.F.);
#51647=ORIENTED_EDGE('',*,*,#37422,.T.);
#51648=ORIENTED_EDGE('',*,*,#37421,.T.);
#51649=ORIENTED_EDGE('',*,*,#37803,.F.);
#51650=ORIENTED_EDGE('',*,*,#37425,.T.);
#51651=ORIENTED_EDGE('',*,*,#37423,.T.);
#51652=ORIENTED_EDGE('',*,*,#37802,.T.);
#51653=ORIENTED_EDGE('',*,*,#37804,.F.);
#51654=ORIENTED_EDGE('',*,*,#37805,.F.);
#51655=ORIENTED_EDGE('',*,*,#37429,.T.);
#51656=ORIENTED_EDGE('',*,*,#37428,.T.);
#51657=ORIENTED_EDGE('',*,*,#37806,.F.);
#51658=ORIENTED_EDGE('',*,*,#37432,.T.);
#51659=ORIENTED_EDGE('',*,*,#37430,.T.);
#51660=ORIENTED_EDGE('',*,*,#37805,.T.);
#51661=ORIENTED_EDGE('',*,*,#37807,.F.);
#51662=ORIENTED_EDGE('',*,*,#37808,.F.);
#51663=ORIENTED_EDGE('',*,*,#37436,.T.);
#51664=ORIENTED_EDGE('',*,*,#37435,.T.);
#51665=ORIENTED_EDGE('',*,*,#37809,.F.);
#51666=ORIENTED_EDGE('',*,*,#37439,.T.);
#51667=ORIENTED_EDGE('',*,*,#37437,.T.);
#51668=ORIENTED_EDGE('',*,*,#37808,.T.);
#51669=ORIENTED_EDGE('',*,*,#37810,.F.);
#51670=ORIENTED_EDGE('',*,*,#37811,.F.);
#51671=ORIENTED_EDGE('',*,*,#37443,.T.);
#51672=ORIENTED_EDGE('',*,*,#37442,.T.);
#51673=ORIENTED_EDGE('',*,*,#37812,.F.);
#51674=ORIENTED_EDGE('',*,*,#37446,.T.);
#51675=ORIENTED_EDGE('',*,*,#37444,.T.);
#51676=ORIENTED_EDGE('',*,*,#37811,.T.);
#51677=ORIENTED_EDGE('',*,*,#37813,.F.);
#51678=ORIENTED_EDGE('',*,*,#37814,.F.);
#51679=ORIENTED_EDGE('',*,*,#37450,.T.);
#51680=ORIENTED_EDGE('',*,*,#37449,.T.);
#51681=ORIENTED_EDGE('',*,*,#37815,.F.);
#51682=ORIENTED_EDGE('',*,*,#37453,.T.);
#51683=ORIENTED_EDGE('',*,*,#37451,.T.);
#51684=ORIENTED_EDGE('',*,*,#37814,.T.);
#51685=ORIENTED_EDGE('',*,*,#37816,.F.);
#51686=ORIENTED_EDGE('',*,*,#37817,.F.);
#51687=ORIENTED_EDGE('',*,*,#37457,.T.);
#51688=ORIENTED_EDGE('',*,*,#37456,.T.);
#51689=ORIENTED_EDGE('',*,*,#37818,.F.);
#51690=ORIENTED_EDGE('',*,*,#37460,.T.);
#51691=ORIENTED_EDGE('',*,*,#37458,.T.);
#51692=ORIENTED_EDGE('',*,*,#37817,.T.);
#51693=ORIENTED_EDGE('',*,*,#37819,.F.);
#51694=ORIENTED_EDGE('',*,*,#37820,.F.);
#51695=ORIENTED_EDGE('',*,*,#37464,.T.);
#51696=ORIENTED_EDGE('',*,*,#37463,.T.);
#51697=ORIENTED_EDGE('',*,*,#37821,.F.);
#51698=ORIENTED_EDGE('',*,*,#37467,.T.);
#51699=ORIENTED_EDGE('',*,*,#37465,.T.);
#51700=ORIENTED_EDGE('',*,*,#37820,.T.);
#51701=ORIENTED_EDGE('',*,*,#37822,.F.);
#51702=ORIENTED_EDGE('',*,*,#37823,.F.);
#51703=ORIENTED_EDGE('',*,*,#37471,.T.);
#51704=ORIENTED_EDGE('',*,*,#37470,.T.);
#51705=ORIENTED_EDGE('',*,*,#37824,.F.);
#51706=ORIENTED_EDGE('',*,*,#37474,.T.);
#51707=ORIENTED_EDGE('',*,*,#37472,.T.);
#51708=ORIENTED_EDGE('',*,*,#37823,.T.);
#51709=ORIENTED_EDGE('',*,*,#37825,.F.);
#51710=ORIENTED_EDGE('',*,*,#37826,.F.);
#51711=ORIENTED_EDGE('',*,*,#37478,.T.);
#51712=ORIENTED_EDGE('',*,*,#37477,.T.);
#51713=ORIENTED_EDGE('',*,*,#37827,.F.);
#51714=ORIENTED_EDGE('',*,*,#37481,.T.);
#51715=ORIENTED_EDGE('',*,*,#37479,.T.);
#51716=ORIENTED_EDGE('',*,*,#37826,.T.);
#51717=ORIENTED_EDGE('',*,*,#37828,.F.);
#51718=ORIENTED_EDGE('',*,*,#37829,.F.);
#51719=ORIENTED_EDGE('',*,*,#37485,.T.);
#51720=ORIENTED_EDGE('',*,*,#37484,.T.);
#51721=ORIENTED_EDGE('',*,*,#37830,.F.);
#51722=ORIENTED_EDGE('',*,*,#37488,.T.);
#51723=ORIENTED_EDGE('',*,*,#37486,.T.);
#51724=ORIENTED_EDGE('',*,*,#37829,.T.);
#51725=ORIENTED_EDGE('',*,*,#37831,.F.);
#51726=ORIENTED_EDGE('',*,*,#37832,.F.);
#51727=ORIENTED_EDGE('',*,*,#34430,.T.);
#51728=ORIENTED_EDGE('',*,*,#37490,.T.);
#51729=ORIENTED_EDGE('',*,*,#37833,.F.);
#51730=ORIENTED_EDGE('',*,*,#37491,.T.);
#51731=ORIENTED_EDGE('',*,*,#34431,.T.);
#51732=ORIENTED_EDGE('',*,*,#37832,.T.);
#51733=ORIENTED_EDGE('',*,*,#37834,.F.);
#51734=ORIENTED_EDGE('',*,*,#37835,.F.);
#51735=ORIENTED_EDGE('',*,*,#37495,.T.);
#51736=ORIENTED_EDGE('',*,*,#37494,.T.);
#51737=ORIENTED_EDGE('',*,*,#37836,.F.);
#51738=ORIENTED_EDGE('',*,*,#37498,.T.);
#51739=ORIENTED_EDGE('',*,*,#37496,.T.);
#51740=ORIENTED_EDGE('',*,*,#37835,.T.);
#51741=ORIENTED_EDGE('',*,*,#37837,.F.);
#51742=ORIENTED_EDGE('',*,*,#37838,.F.);
#51743=ORIENTED_EDGE('',*,*,#37502,.T.);
#51744=ORIENTED_EDGE('',*,*,#37501,.T.);
#51745=ORIENTED_EDGE('',*,*,#37839,.F.);
#51746=ORIENTED_EDGE('',*,*,#37505,.T.);
#51747=ORIENTED_EDGE('',*,*,#37503,.T.);
#51748=ORIENTED_EDGE('',*,*,#37838,.T.);
#51749=ORIENTED_EDGE('',*,*,#37840,.F.);
#51750=ORIENTED_EDGE('',*,*,#37841,.F.);
#51751=ORIENTED_EDGE('',*,*,#37509,.T.);
#51752=ORIENTED_EDGE('',*,*,#37508,.T.);
#51753=ORIENTED_EDGE('',*,*,#37842,.F.);
#51754=ORIENTED_EDGE('',*,*,#37512,.T.);
#51755=ORIENTED_EDGE('',*,*,#37510,.T.);
#51756=ORIENTED_EDGE('',*,*,#37841,.T.);
#51757=ORIENTED_EDGE('',*,*,#37843,.F.);
#51758=ORIENTED_EDGE('',*,*,#37844,.F.);
#51759=ORIENTED_EDGE('',*,*,#37516,.T.);
#51760=ORIENTED_EDGE('',*,*,#37515,.T.);
#51761=ORIENTED_EDGE('',*,*,#37845,.F.);
#51762=ORIENTED_EDGE('',*,*,#37519,.T.);
#51763=ORIENTED_EDGE('',*,*,#37517,.T.);
#51764=ORIENTED_EDGE('',*,*,#37844,.T.);
#51765=ORIENTED_EDGE('',*,*,#37846,.F.);
#51766=ORIENTED_EDGE('',*,*,#37847,.F.);
#51767=ORIENTED_EDGE('',*,*,#37523,.T.);
#51768=ORIENTED_EDGE('',*,*,#37522,.T.);
#51769=ORIENTED_EDGE('',*,*,#37848,.F.);
#51770=ORIENTED_EDGE('',*,*,#37526,.T.);
#51771=ORIENTED_EDGE('',*,*,#37524,.T.);
#51772=ORIENTED_EDGE('',*,*,#37847,.T.);
#51773=ORIENTED_EDGE('',*,*,#37849,.F.);
#51774=ORIENTED_EDGE('',*,*,#37850,.F.);
#51775=ORIENTED_EDGE('',*,*,#37530,.T.);
#51776=ORIENTED_EDGE('',*,*,#37529,.T.);
#51777=ORIENTED_EDGE('',*,*,#37851,.F.);
#51778=ORIENTED_EDGE('',*,*,#37533,.T.);
#51779=ORIENTED_EDGE('',*,*,#37531,.T.);
#51780=ORIENTED_EDGE('',*,*,#37850,.T.);
#51781=ORIENTED_EDGE('',*,*,#37852,.F.);
#51782=ORIENTED_EDGE('',*,*,#37853,.F.);
#51783=ORIENTED_EDGE('',*,*,#37537,.T.);
#51784=ORIENTED_EDGE('',*,*,#37536,.T.);
#51785=ORIENTED_EDGE('',*,*,#37854,.F.);
#51786=ORIENTED_EDGE('',*,*,#37540,.T.);
#51787=ORIENTED_EDGE('',*,*,#37538,.T.);
#51788=ORIENTED_EDGE('',*,*,#37853,.T.);
#51789=ORIENTED_EDGE('',*,*,#37855,.F.);
#51790=ORIENTED_EDGE('',*,*,#37856,.F.);
#51791=ORIENTED_EDGE('',*,*,#37546,.T.);
#51792=ORIENTED_EDGE('',*,*,#37543,.T.);
#51793=ORIENTED_EDGE('',*,*,#37547,.T.);
#51794=ORIENTED_EDGE('',*,*,#37856,.T.);
#51795=ORIENTED_EDGE('',*,*,#37857,.F.);
#51796=ORIENTED_EDGE('',*,*,#37545,.T.);
#51797=ORIENTED_EDGE('',*,*,#37552,.T.);
#51798=ORIENTED_EDGE('',*,*,#37548,.T.);
#51799=ORIENTED_EDGE('',*,*,#37858,.F.);
#51800=ORIENTED_EDGE('',*,*,#37859,.F.);
#51801=ORIENTED_EDGE('',*,*,#37860,.F.);
#51802=ORIENTED_EDGE('',*,*,#37554,.T.);
#51803=ORIENTED_EDGE('',*,*,#37553,.T.);
#51804=ORIENTED_EDGE('',*,*,#37859,.T.);
#51805=ORIENTED_EDGE('',*,*,#37861,.F.);
#51806=ORIENTED_EDGE('',*,*,#37862,.F.);
#51807=ORIENTED_EDGE('',*,*,#37558,.T.);
#51808=ORIENTED_EDGE('',*,*,#37557,.T.);
#51809=ORIENTED_EDGE('',*,*,#37863,.F.);
#51810=ORIENTED_EDGE('',*,*,#37561,.T.);
#51811=ORIENTED_EDGE('',*,*,#37559,.T.);
#51812=ORIENTED_EDGE('',*,*,#37862,.T.);
#51813=ORIENTED_EDGE('',*,*,#37864,.F.);
#51814=ORIENTED_EDGE('',*,*,#37865,.F.);
#51815=ORIENTED_EDGE('',*,*,#37565,.T.);
#51816=ORIENTED_EDGE('',*,*,#37564,.T.);
#51817=ORIENTED_EDGE('',*,*,#37866,.F.);
#51818=ORIENTED_EDGE('',*,*,#37568,.T.);
#51819=ORIENTED_EDGE('',*,*,#37566,.T.);
#51820=ORIENTED_EDGE('',*,*,#37865,.T.);
#51821=ORIENTED_EDGE('',*,*,#37867,.F.);
#51822=ORIENTED_EDGE('',*,*,#37868,.F.);
#51823=ORIENTED_EDGE('',*,*,#37572,.T.);
#51824=ORIENTED_EDGE('',*,*,#37571,.T.);
#51825=ORIENTED_EDGE('',*,*,#37869,.F.);
#51826=ORIENTED_EDGE('',*,*,#37575,.T.);
#51827=ORIENTED_EDGE('',*,*,#37573,.T.);
#51828=ORIENTED_EDGE('',*,*,#37868,.T.);
#51829=ORIENTED_EDGE('',*,*,#37870,.F.);
#51830=ORIENTED_EDGE('',*,*,#37871,.F.);
#51831=ORIENTED_EDGE('',*,*,#37579,.T.);
#51832=ORIENTED_EDGE('',*,*,#37578,.T.);
#51833=ORIENTED_EDGE('',*,*,#37872,.F.);
#51834=ORIENTED_EDGE('',*,*,#37582,.T.);
#51835=ORIENTED_EDGE('',*,*,#37580,.T.);
#51836=ORIENTED_EDGE('',*,*,#37871,.T.);
#51837=ORIENTED_EDGE('',*,*,#37873,.F.);
#51838=ORIENTED_EDGE('',*,*,#37874,.F.);
#51839=ORIENTED_EDGE('',*,*,#37586,.T.);
#51840=ORIENTED_EDGE('',*,*,#37585,.T.);
#51841=ORIENTED_EDGE('',*,*,#37875,.F.);
#51842=ORIENTED_EDGE('',*,*,#37589,.T.);
#51843=ORIENTED_EDGE('',*,*,#37587,.T.);
#51844=ORIENTED_EDGE('',*,*,#37874,.T.);
#51845=ORIENTED_EDGE('',*,*,#37595,.T.);
#51846=ORIENTED_EDGE('',*,*,#37590,.T.);
#51847=ORIENTED_EDGE('',*,*,#37876,.F.);
#51848=ORIENTED_EDGE('',*,*,#37877,.F.);
#51849=ORIENTED_EDGE('',*,*,#37596,.T.);
#51850=ORIENTED_EDGE('',*,*,#37877,.T.);
#51851=ORIENTED_EDGE('',*,*,#37878,.F.);
#51852=ORIENTED_EDGE('',*,*,#37594,.T.);
#51853=ORIENTED_EDGE('',*,*,#37602,.T.);
#51854=ORIENTED_EDGE('',*,*,#37597,.T.);
#51855=ORIENTED_EDGE('',*,*,#37879,.F.);
#51856=ORIENTED_EDGE('',*,*,#37880,.F.);
#51857=ORIENTED_EDGE('',*,*,#37603,.T.);
#51858=ORIENTED_EDGE('',*,*,#37880,.T.);
#51859=ORIENTED_EDGE('',*,*,#37881,.F.);
#51860=ORIENTED_EDGE('',*,*,#37601,.T.);
#51861=ORIENTED_EDGE('',*,*,#37609,.T.);
#51862=ORIENTED_EDGE('',*,*,#37604,.T.);
#51863=ORIENTED_EDGE('',*,*,#37882,.F.);
#51864=ORIENTED_EDGE('',*,*,#37883,.F.);
#51865=ORIENTED_EDGE('',*,*,#37610,.T.);
#51866=ORIENTED_EDGE('',*,*,#37883,.T.);
#51867=ORIENTED_EDGE('',*,*,#37884,.F.);
#51868=ORIENTED_EDGE('',*,*,#37608,.T.);
#51869=ORIENTED_EDGE('',*,*,#37616,.T.);
#51870=ORIENTED_EDGE('',*,*,#37611,.T.);
#51871=ORIENTED_EDGE('',*,*,#37885,.F.);
#51872=ORIENTED_EDGE('',*,*,#37886,.F.);
#51873=ORIENTED_EDGE('',*,*,#37617,.T.);
#51874=ORIENTED_EDGE('',*,*,#37886,.T.);
#51875=ORIENTED_EDGE('',*,*,#37887,.F.);
#51876=ORIENTED_EDGE('',*,*,#37615,.T.);
#51877=ORIENTED_EDGE('',*,*,#37623,.T.);
#51878=ORIENTED_EDGE('',*,*,#37618,.T.);
#51879=ORIENTED_EDGE('',*,*,#37888,.F.);
#51880=ORIENTED_EDGE('',*,*,#37889,.F.);
#51881=ORIENTED_EDGE('',*,*,#37624,.T.);
#51882=ORIENTED_EDGE('',*,*,#37889,.T.);
#51883=ORIENTED_EDGE('',*,*,#37890,.F.);
#51884=ORIENTED_EDGE('',*,*,#37622,.T.);
#51885=ORIENTED_EDGE('',*,*,#37630,.T.);
#51886=ORIENTED_EDGE('',*,*,#37625,.T.);
#51887=ORIENTED_EDGE('',*,*,#37891,.F.);
#51888=ORIENTED_EDGE('',*,*,#37892,.F.);
#51889=ORIENTED_EDGE('',*,*,#37631,.T.);
#51890=ORIENTED_EDGE('',*,*,#37892,.T.);
#51891=ORIENTED_EDGE('',*,*,#37893,.F.);
#51892=ORIENTED_EDGE('',*,*,#37629,.T.);
#51893=ORIENTED_EDGE('',*,*,#37637,.T.);
#51894=ORIENTED_EDGE('',*,*,#37632,.T.);
#51895=ORIENTED_EDGE('',*,*,#37894,.F.);
#51896=ORIENTED_EDGE('',*,*,#37895,.F.);
#51897=ORIENTED_EDGE('',*,*,#37638,.T.);
#51898=ORIENTED_EDGE('',*,*,#37895,.T.);
#51899=ORIENTED_EDGE('',*,*,#37896,.F.);
#51900=ORIENTED_EDGE('',*,*,#37636,.T.);
#51901=ORIENTED_EDGE('',*,*,#37644,.T.);
#51902=ORIENTED_EDGE('',*,*,#37639,.T.);
#51903=ORIENTED_EDGE('',*,*,#37897,.F.);
#51904=ORIENTED_EDGE('',*,*,#37898,.F.);
#51905=ORIENTED_EDGE('',*,*,#37645,.T.);
#51906=ORIENTED_EDGE('',*,*,#37898,.T.);
#51907=ORIENTED_EDGE('',*,*,#37899,.F.);
#51908=ORIENTED_EDGE('',*,*,#37643,.T.);
#51909=ORIENTED_EDGE('',*,*,#37651,.T.);
#51910=ORIENTED_EDGE('',*,*,#37646,.T.);
#51911=ORIENTED_EDGE('',*,*,#37900,.F.);
#51912=ORIENTED_EDGE('',*,*,#37901,.F.);
#51913=ORIENTED_EDGE('',*,*,#37652,.T.);
#51914=ORIENTED_EDGE('',*,*,#37901,.T.);
#51915=ORIENTED_EDGE('',*,*,#37902,.F.);
#51916=ORIENTED_EDGE('',*,*,#37650,.T.);
#51917=ORIENTED_EDGE('',*,*,#37658,.T.);
#51918=ORIENTED_EDGE('',*,*,#37653,.T.);
#51919=ORIENTED_EDGE('',*,*,#37903,.F.);
#51920=ORIENTED_EDGE('',*,*,#37904,.F.);
#51921=ORIENTED_EDGE('',*,*,#37659,.T.);
#51922=ORIENTED_EDGE('',*,*,#37904,.T.);
#51923=ORIENTED_EDGE('',*,*,#37905,.F.);
#51924=ORIENTED_EDGE('',*,*,#37657,.T.);
#51925=ORIENTED_EDGE('',*,*,#37665,.T.);
#51926=ORIENTED_EDGE('',*,*,#37660,.T.);
#51927=ORIENTED_EDGE('',*,*,#37906,.F.);
#51928=ORIENTED_EDGE('',*,*,#37907,.F.);
#51929=ORIENTED_EDGE('',*,*,#37666,.T.);
#51930=ORIENTED_EDGE('',*,*,#37907,.T.);
#51931=ORIENTED_EDGE('',*,*,#37908,.F.);
#51932=ORIENTED_EDGE('',*,*,#37664,.T.);
#51933=ORIENTED_EDGE('',*,*,#37672,.T.);
#51934=ORIENTED_EDGE('',*,*,#37667,.T.);
#51935=ORIENTED_EDGE('',*,*,#37909,.F.);
#51936=ORIENTED_EDGE('',*,*,#37910,.F.);
#51937=ORIENTED_EDGE('',*,*,#37673,.T.);
#51938=ORIENTED_EDGE('',*,*,#37910,.T.);
#51939=ORIENTED_EDGE('',*,*,#37911,.F.);
#51940=ORIENTED_EDGE('',*,*,#37671,.T.);
#51941=ORIENTED_EDGE('',*,*,#37679,.T.);
#51942=ORIENTED_EDGE('',*,*,#37674,.T.);
#51943=ORIENTED_EDGE('',*,*,#37912,.F.);
#51944=ORIENTED_EDGE('',*,*,#37913,.F.);
#51945=ORIENTED_EDGE('',*,*,#37680,.T.);
#51946=ORIENTED_EDGE('',*,*,#37913,.T.);
#51947=ORIENTED_EDGE('',*,*,#37914,.F.);
#51948=ORIENTED_EDGE('',*,*,#37678,.T.);
#51949=ORIENTED_EDGE('',*,*,#37686,.T.);
#51950=ORIENTED_EDGE('',*,*,#37681,.T.);
#51951=ORIENTED_EDGE('',*,*,#37915,.F.);
#51952=ORIENTED_EDGE('',*,*,#37916,.F.);
#51953=ORIENTED_EDGE('',*,*,#37687,.T.);
#51954=ORIENTED_EDGE('',*,*,#37916,.T.);
#51955=ORIENTED_EDGE('',*,*,#37917,.F.);
#51956=ORIENTED_EDGE('',*,*,#37685,.T.);
#51957=ORIENTED_EDGE('',*,*,#37693,.T.);
#51958=ORIENTED_EDGE('',*,*,#37688,.T.);
#51959=ORIENTED_EDGE('',*,*,#37918,.F.);
#51960=ORIENTED_EDGE('',*,*,#37919,.F.);
#51961=ORIENTED_EDGE('',*,*,#37694,.T.);
#51962=ORIENTED_EDGE('',*,*,#37919,.T.);
#51963=ORIENTED_EDGE('',*,*,#37920,.F.);
#51964=ORIENTED_EDGE('',*,*,#37692,.T.);
#51965=ORIENTED_EDGE('',*,*,#37700,.T.);
#51966=ORIENTED_EDGE('',*,*,#37695,.T.);
#51967=ORIENTED_EDGE('',*,*,#37921,.F.);
#51968=ORIENTED_EDGE('',*,*,#37922,.F.);
#51969=ORIENTED_EDGE('',*,*,#37701,.T.);
#51970=ORIENTED_EDGE('',*,*,#37922,.T.);
#51971=ORIENTED_EDGE('',*,*,#37923,.F.);
#51972=ORIENTED_EDGE('',*,*,#37699,.T.);
#51973=ORIENTED_EDGE('',*,*,#37707,.T.);
#51974=ORIENTED_EDGE('',*,*,#37702,.T.);
#51975=ORIENTED_EDGE('',*,*,#37924,.F.);
#51976=ORIENTED_EDGE('',*,*,#37925,.F.);
#51977=ORIENTED_EDGE('',*,*,#37708,.T.);
#51978=ORIENTED_EDGE('',*,*,#37925,.T.);
#51979=ORIENTED_EDGE('',*,*,#37926,.F.);
#51980=ORIENTED_EDGE('',*,*,#37706,.T.);
#51981=ORIENTED_EDGE('',*,*,#37714,.T.);
#51982=ORIENTED_EDGE('',*,*,#37709,.T.);
#51983=ORIENTED_EDGE('',*,*,#37927,.F.);
#51984=ORIENTED_EDGE('',*,*,#37928,.F.);
#51985=ORIENTED_EDGE('',*,*,#37715,.T.);
#51986=ORIENTED_EDGE('',*,*,#37928,.T.);
#51987=ORIENTED_EDGE('',*,*,#37929,.F.);
#51988=ORIENTED_EDGE('',*,*,#37713,.T.);
#51989=ORIENTED_EDGE('',*,*,#37721,.T.);
#51990=ORIENTED_EDGE('',*,*,#37716,.T.);
#51991=ORIENTED_EDGE('',*,*,#37930,.F.);
#51992=ORIENTED_EDGE('',*,*,#37931,.F.);
#51993=ORIENTED_EDGE('',*,*,#37722,.T.);
#51994=ORIENTED_EDGE('',*,*,#37931,.T.);
#51995=ORIENTED_EDGE('',*,*,#37932,.F.);
#51996=ORIENTED_EDGE('',*,*,#37720,.T.);
#51997=ORIENTED_EDGE('',*,*,#37728,.T.);
#51998=ORIENTED_EDGE('',*,*,#37723,.T.);
#51999=ORIENTED_EDGE('',*,*,#37933,.F.);
#52000=ORIENTED_EDGE('',*,*,#37934,.F.);
#52001=ORIENTED_EDGE('',*,*,#37729,.T.);
#52002=ORIENTED_EDGE('',*,*,#37934,.T.);
#52003=ORIENTED_EDGE('',*,*,#37935,.F.);
#52004=ORIENTED_EDGE('',*,*,#37727,.T.);
#52005=ORIENTED_EDGE('',*,*,#37735,.T.);
#52006=ORIENTED_EDGE('',*,*,#37730,.T.);
#52007=ORIENTED_EDGE('',*,*,#37936,.F.);
#52008=ORIENTED_EDGE('',*,*,#37937,.F.);
#52009=ORIENTED_EDGE('',*,*,#37736,.T.);
#52010=ORIENTED_EDGE('',*,*,#37937,.T.);
#52011=ORIENTED_EDGE('',*,*,#37938,.F.);
#52012=ORIENTED_EDGE('',*,*,#37734,.T.);
#52013=ORIENTED_EDGE('',*,*,#34425,.T.);
#52014=ORIENTED_EDGE('',*,*,#37737,.T.);
#52015=ORIENTED_EDGE('',*,*,#37939,.F.);
#52016=ORIENTED_EDGE('',*,*,#37940,.F.);
#52017=ORIENTED_EDGE('',*,*,#34426,.T.);
#52018=ORIENTED_EDGE('',*,*,#37940,.T.);
#52019=ORIENTED_EDGE('',*,*,#37941,.F.);
#52020=ORIENTED_EDGE('',*,*,#37739,.T.);
#52021=ORIENTED_EDGE('',*,*,#37745,.T.);
#52022=ORIENTED_EDGE('',*,*,#37740,.T.);
#52023=ORIENTED_EDGE('',*,*,#37942,.F.);
#52024=ORIENTED_EDGE('',*,*,#37943,.F.);
#52025=ORIENTED_EDGE('',*,*,#37746,.T.);
#52026=ORIENTED_EDGE('',*,*,#37943,.T.);
#52027=ORIENTED_EDGE('',*,*,#37944,.F.);
#52028=ORIENTED_EDGE('',*,*,#37744,.T.);
#52029=ORIENTED_EDGE('',*,*,#37752,.T.);
#52030=ORIENTED_EDGE('',*,*,#37747,.T.);
#52031=ORIENTED_EDGE('',*,*,#37945,.F.);
#52032=ORIENTED_EDGE('',*,*,#37946,.F.);
#52033=ORIENTED_EDGE('',*,*,#37753,.T.);
#52034=ORIENTED_EDGE('',*,*,#37946,.T.);
#52035=ORIENTED_EDGE('',*,*,#37947,.F.);
#52036=ORIENTED_EDGE('',*,*,#37751,.T.);
#52037=ORIENTED_EDGE('',*,*,#37759,.T.);
#52038=ORIENTED_EDGE('',*,*,#37754,.T.);
#52039=ORIENTED_EDGE('',*,*,#37948,.F.);
#52040=ORIENTED_EDGE('',*,*,#37949,.F.);
#52041=ORIENTED_EDGE('',*,*,#37760,.T.);
#52042=ORIENTED_EDGE('',*,*,#37949,.T.);
#52043=ORIENTED_EDGE('',*,*,#37950,.F.);
#52044=ORIENTED_EDGE('',*,*,#37758,.T.);
#52045=ORIENTED_EDGE('',*,*,#37766,.T.);
#52046=ORIENTED_EDGE('',*,*,#37761,.T.);
#52047=ORIENTED_EDGE('',*,*,#37951,.F.);
#52048=ORIENTED_EDGE('',*,*,#37952,.F.);
#52049=ORIENTED_EDGE('',*,*,#37767,.T.);
#52050=ORIENTED_EDGE('',*,*,#37952,.T.);
#52051=ORIENTED_EDGE('',*,*,#37953,.F.);
#52052=ORIENTED_EDGE('',*,*,#37765,.T.);
#52053=ORIENTED_EDGE('',*,*,#37773,.T.);
#52054=ORIENTED_EDGE('',*,*,#37768,.T.);
#52055=ORIENTED_EDGE('',*,*,#37954,.F.);
#52056=ORIENTED_EDGE('',*,*,#37955,.F.);
#52057=ORIENTED_EDGE('',*,*,#37774,.T.);
#52058=ORIENTED_EDGE('',*,*,#37955,.T.);
#52059=ORIENTED_EDGE('',*,*,#37956,.F.);
#52060=ORIENTED_EDGE('',*,*,#37772,.T.);
#52061=ORIENTED_EDGE('',*,*,#37780,.T.);
#52062=ORIENTED_EDGE('',*,*,#37775,.T.);
#52063=ORIENTED_EDGE('',*,*,#37957,.F.);
#52064=ORIENTED_EDGE('',*,*,#37958,.F.);
#52065=ORIENTED_EDGE('',*,*,#37781,.T.);
#52066=ORIENTED_EDGE('',*,*,#37958,.T.);
#52067=ORIENTED_EDGE('',*,*,#37959,.F.);
#52068=ORIENTED_EDGE('',*,*,#37779,.T.);
#52069=ORIENTED_EDGE('',*,*,#37960,.F.);
#52070=ORIENTED_EDGE('',*,*,#37961,.F.);
#52071=ORIENTED_EDGE('',*,*,#37787,.T.);
#52072=ORIENTED_EDGE('',*,*,#37782,.T.);
#52073=ORIENTED_EDGE('',*,*,#37788,.T.);
#52074=ORIENTED_EDGE('',*,*,#37961,.T.);
#52075=ORIENTED_EDGE('',*,*,#37962,.F.);
#52076=ORIENTED_EDGE('',*,*,#37786,.T.);
#52077=ORIENTED_EDGE('',*,*,#37963,.T.);
#52078=ORIENTED_EDGE('',*,*,#37964,.F.);
#52079=ORIENTED_EDGE('',*,*,#37789,.T.);
#52080=ORIENTED_EDGE('',*,*,#37965,.F.);
#52081=ORIENTED_EDGE('',*,*,#37966,.T.);
#52082=ORIENTED_EDGE('',*,*,#37967,.F.);
#52083=ORIENTED_EDGE('',*,*,#37791,.T.);
#52084=ORIENTED_EDGE('',*,*,#37968,.F.);
#52085=ORIENTED_EDGE('',*,*,#37969,.F.);
#52086=ORIENTED_EDGE('',*,*,#37970,.F.);
#52087=ORIENTED_EDGE('',*,*,#37971,.F.);
#52088=ORIENTED_EDGE('',*,*,#37966,.F.);
#52089=ORIENTED_EDGE('',*,*,#37971,.T.);
#52090=ORIENTED_EDGE('',*,*,#37972,.F.);
#52091=ORIENTED_EDGE('',*,*,#37792,.T.);
#52092=ORIENTED_EDGE('',*,*,#37967,.T.);
#52093=ORIENTED_EDGE('',*,*,#37973,.T.);
#52094=ORIENTED_EDGE('',*,*,#37974,.F.);
#52095=ORIENTED_EDGE('',*,*,#37794,.T.);
#52096=ORIENTED_EDGE('',*,*,#37975,.F.);
#52097=ORIENTED_EDGE('',*,*,#37976,.F.);
#52098=ORIENTED_EDGE('',*,*,#37977,.F.);
#52099=ORIENTED_EDGE('',*,*,#37978,.F.);
#52100=ORIENTED_EDGE('',*,*,#37973,.F.);
#52101=ORIENTED_EDGE('',*,*,#37978,.T.);
#52102=ORIENTED_EDGE('',*,*,#37979,.F.);
#52103=ORIENTED_EDGE('',*,*,#37795,.T.);
#52104=ORIENTED_EDGE('',*,*,#37974,.T.);
#52105=ORIENTED_EDGE('',*,*,#37980,.T.);
#52106=ORIENTED_EDGE('',*,*,#37981,.F.);
#52107=ORIENTED_EDGE('',*,*,#37797,.T.);
#52108=ORIENTED_EDGE('',*,*,#37982,.F.);
#52109=ORIENTED_EDGE('',*,*,#37983,.F.);
#52110=ORIENTED_EDGE('',*,*,#37984,.F.);
#52111=ORIENTED_EDGE('',*,*,#37985,.F.);
#52112=ORIENTED_EDGE('',*,*,#37980,.F.);
#52113=ORIENTED_EDGE('',*,*,#37985,.T.);
#52114=ORIENTED_EDGE('',*,*,#37986,.F.);
#52115=ORIENTED_EDGE('',*,*,#37798,.T.);
#52116=ORIENTED_EDGE('',*,*,#37981,.T.);
#52117=ORIENTED_EDGE('',*,*,#37987,.T.);
#52118=ORIENTED_EDGE('',*,*,#37988,.F.);
#52119=ORIENTED_EDGE('',*,*,#37800,.T.);
#52120=ORIENTED_EDGE('',*,*,#37989,.F.);
#52121=ORIENTED_EDGE('',*,*,#37990,.F.);
#52122=ORIENTED_EDGE('',*,*,#37991,.F.);
#52123=ORIENTED_EDGE('',*,*,#37992,.F.);
#52124=ORIENTED_EDGE('',*,*,#37987,.F.);
#52125=ORIENTED_EDGE('',*,*,#37992,.T.);
#52126=ORIENTED_EDGE('',*,*,#37993,.F.);
#52127=ORIENTED_EDGE('',*,*,#37801,.T.);
#52128=ORIENTED_EDGE('',*,*,#37988,.T.);
#52129=ORIENTED_EDGE('',*,*,#37994,.T.);
#52130=ORIENTED_EDGE('',*,*,#37995,.F.);
#52131=ORIENTED_EDGE('',*,*,#37803,.T.);
#52132=ORIENTED_EDGE('',*,*,#37996,.F.);
#52133=ORIENTED_EDGE('',*,*,#37997,.F.);
#52134=ORIENTED_EDGE('',*,*,#37998,.F.);
#52135=ORIENTED_EDGE('',*,*,#37999,.F.);
#52136=ORIENTED_EDGE('',*,*,#37994,.F.);
#52137=ORIENTED_EDGE('',*,*,#37999,.T.);
#52138=ORIENTED_EDGE('',*,*,#38000,.F.);
#52139=ORIENTED_EDGE('',*,*,#37804,.T.);
#52140=ORIENTED_EDGE('',*,*,#37995,.T.);
#52141=ORIENTED_EDGE('',*,*,#38001,.T.);
#52142=ORIENTED_EDGE('',*,*,#38002,.F.);
#52143=ORIENTED_EDGE('',*,*,#37806,.T.);
#52144=ORIENTED_EDGE('',*,*,#38003,.F.);
#52145=ORIENTED_EDGE('',*,*,#38004,.F.);
#52146=ORIENTED_EDGE('',*,*,#38005,.F.);
#52147=ORIENTED_EDGE('',*,*,#38006,.F.);
#52148=ORIENTED_EDGE('',*,*,#38001,.F.);
#52149=ORIENTED_EDGE('',*,*,#38006,.T.);
#52150=ORIENTED_EDGE('',*,*,#38007,.F.);
#52151=ORIENTED_EDGE('',*,*,#37807,.T.);
#52152=ORIENTED_EDGE('',*,*,#38002,.T.);
#52153=ORIENTED_EDGE('',*,*,#34422,.T.);
#52154=ORIENTED_EDGE('',*,*,#38008,.F.);
#52155=ORIENTED_EDGE('',*,*,#37809,.T.);
#52156=ORIENTED_EDGE('',*,*,#38009,.F.);
#52157=ORIENTED_EDGE('',*,*,#34421,.T.);
#52158=ORIENTED_EDGE('',*,*,#38010,.F.);
#52159=ORIENTED_EDGE('',*,*,#37810,.T.);
#52160=ORIENTED_EDGE('',*,*,#38008,.T.);
#52161=ORIENTED_EDGE('',*,*,#38011,.T.);
#52162=ORIENTED_EDGE('',*,*,#38012,.F.);
#52163=ORIENTED_EDGE('',*,*,#37812,.T.);
#52164=ORIENTED_EDGE('',*,*,#38013,.F.);
#52165=ORIENTED_EDGE('',*,*,#38014,.F.);
#52166=ORIENTED_EDGE('',*,*,#38015,.F.);
#52167=ORIENTED_EDGE('',*,*,#38016,.F.);
#52168=ORIENTED_EDGE('',*,*,#38011,.F.);
#52169=ORIENTED_EDGE('',*,*,#38016,.T.);
#52170=ORIENTED_EDGE('',*,*,#38017,.F.);
#52171=ORIENTED_EDGE('',*,*,#37813,.T.);
#52172=ORIENTED_EDGE('',*,*,#38012,.T.);
#52173=ORIENTED_EDGE('',*,*,#38018,.T.);
#52174=ORIENTED_EDGE('',*,*,#38019,.F.);
#52175=ORIENTED_EDGE('',*,*,#37815,.T.);
#52176=ORIENTED_EDGE('',*,*,#38020,.F.);
#52177=ORIENTED_EDGE('',*,*,#38021,.F.);
#52178=ORIENTED_EDGE('',*,*,#38022,.F.);
#52179=ORIENTED_EDGE('',*,*,#38023,.F.);
#52180=ORIENTED_EDGE('',*,*,#38018,.F.);
#52181=ORIENTED_EDGE('',*,*,#38023,.T.);
#52182=ORIENTED_EDGE('',*,*,#38024,.F.);
#52183=ORIENTED_EDGE('',*,*,#37816,.T.);
#52184=ORIENTED_EDGE('',*,*,#38019,.T.);
#52185=ORIENTED_EDGE('',*,*,#38025,.T.);
#52186=ORIENTED_EDGE('',*,*,#38026,.F.);
#52187=ORIENTED_EDGE('',*,*,#37818,.T.);
#52188=ORIENTED_EDGE('',*,*,#38027,.F.);
#52189=ORIENTED_EDGE('',*,*,#38028,.F.);
#52190=ORIENTED_EDGE('',*,*,#38029,.F.);
#52191=ORIENTED_EDGE('',*,*,#38030,.F.);
#52192=ORIENTED_EDGE('',*,*,#38025,.F.);
#52193=ORIENTED_EDGE('',*,*,#38030,.T.);
#52194=ORIENTED_EDGE('',*,*,#38031,.F.);
#52195=ORIENTED_EDGE('',*,*,#37819,.T.);
#52196=ORIENTED_EDGE('',*,*,#38026,.T.);
#52197=ORIENTED_EDGE('',*,*,#38032,.T.);
#52198=ORIENTED_EDGE('',*,*,#38033,.F.);
#52199=ORIENTED_EDGE('',*,*,#37821,.T.);
#52200=ORIENTED_EDGE('',*,*,#38034,.F.);
#52201=ORIENTED_EDGE('',*,*,#38035,.F.);
#52202=ORIENTED_EDGE('',*,*,#38036,.F.);
#52203=ORIENTED_EDGE('',*,*,#38037,.F.);
#52204=ORIENTED_EDGE('',*,*,#38032,.F.);
#52205=ORIENTED_EDGE('',*,*,#38037,.T.);
#52206=ORIENTED_EDGE('',*,*,#38038,.F.);
#52207=ORIENTED_EDGE('',*,*,#37822,.T.);
#52208=ORIENTED_EDGE('',*,*,#38033,.T.);
#52209=ORIENTED_EDGE('',*,*,#38039,.T.);
#52210=ORIENTED_EDGE('',*,*,#38040,.F.);
#52211=ORIENTED_EDGE('',*,*,#37824,.T.);
#52212=ORIENTED_EDGE('',*,*,#38041,.F.);
#52213=ORIENTED_EDGE('',*,*,#38042,.F.);
#52214=ORIENTED_EDGE('',*,*,#38043,.F.);
#52215=ORIENTED_EDGE('',*,*,#38044,.F.);
#52216=ORIENTED_EDGE('',*,*,#38039,.F.);
#52217=ORIENTED_EDGE('',*,*,#38044,.T.);
#52218=ORIENTED_EDGE('',*,*,#38045,.F.);
#52219=ORIENTED_EDGE('',*,*,#37825,.T.);
#52220=ORIENTED_EDGE('',*,*,#38040,.T.);
#52221=ORIENTED_EDGE('',*,*,#38046,.T.);
#52222=ORIENTED_EDGE('',*,*,#38047,.F.);
#52223=ORIENTED_EDGE('',*,*,#37827,.T.);
#52224=ORIENTED_EDGE('',*,*,#38048,.F.);
#52225=ORIENTED_EDGE('',*,*,#38049,.F.);
#52226=ORIENTED_EDGE('',*,*,#38050,.F.);
#52227=ORIENTED_EDGE('',*,*,#38051,.F.);
#52228=ORIENTED_EDGE('',*,*,#38046,.F.);
#52229=ORIENTED_EDGE('',*,*,#38051,.T.);
#52230=ORIENTED_EDGE('',*,*,#38052,.F.);
#52231=ORIENTED_EDGE('',*,*,#37828,.T.);
#52232=ORIENTED_EDGE('',*,*,#38047,.T.);
#52233=ORIENTED_EDGE('',*,*,#38053,.T.);
#52234=ORIENTED_EDGE('',*,*,#38054,.F.);
#52235=ORIENTED_EDGE('',*,*,#37830,.T.);
#52236=ORIENTED_EDGE('',*,*,#38055,.F.);
#52237=ORIENTED_EDGE('',*,*,#38056,.F.);
#52238=ORIENTED_EDGE('',*,*,#38057,.F.);
#52239=ORIENTED_EDGE('',*,*,#38058,.F.);
#52240=ORIENTED_EDGE('',*,*,#38053,.F.);
#52241=ORIENTED_EDGE('',*,*,#38058,.T.);
#52242=ORIENTED_EDGE('',*,*,#38059,.F.);
#52243=ORIENTED_EDGE('',*,*,#37831,.T.);
#52244=ORIENTED_EDGE('',*,*,#38054,.T.);
#52245=ORIENTED_EDGE('',*,*,#38060,.T.);
#52246=ORIENTED_EDGE('',*,*,#38061,.F.);
#52247=ORIENTED_EDGE('',*,*,#37833,.T.);
#52248=ORIENTED_EDGE('',*,*,#38062,.F.);
#52249=ORIENTED_EDGE('',*,*,#38063,.F.);
#52250=ORIENTED_EDGE('',*,*,#38064,.F.);
#52251=ORIENTED_EDGE('',*,*,#38065,.F.);
#52252=ORIENTED_EDGE('',*,*,#38060,.F.);
#52253=ORIENTED_EDGE('',*,*,#38065,.T.);
#52254=ORIENTED_EDGE('',*,*,#38066,.F.);
#52255=ORIENTED_EDGE('',*,*,#37834,.T.);
#52256=ORIENTED_EDGE('',*,*,#38061,.T.);
#52257=ORIENTED_EDGE('',*,*,#38067,.T.);
#52258=ORIENTED_EDGE('',*,*,#38068,.F.);
#52259=ORIENTED_EDGE('',*,*,#37836,.T.);
#52260=ORIENTED_EDGE('',*,*,#38069,.F.);
#52261=ORIENTED_EDGE('',*,*,#38070,.F.);
#52262=ORIENTED_EDGE('',*,*,#38071,.F.);
#52263=ORIENTED_EDGE('',*,*,#38072,.F.);
#52264=ORIENTED_EDGE('',*,*,#38067,.F.);
#52265=ORIENTED_EDGE('',*,*,#38072,.T.);
#52266=ORIENTED_EDGE('',*,*,#38073,.F.);
#52267=ORIENTED_EDGE('',*,*,#37837,.T.);
#52268=ORIENTED_EDGE('',*,*,#38068,.T.);
#52269=ORIENTED_EDGE('',*,*,#38074,.T.);
#52270=ORIENTED_EDGE('',*,*,#38075,.F.);
#52271=ORIENTED_EDGE('',*,*,#37839,.T.);
#52272=ORIENTED_EDGE('',*,*,#38076,.F.);
#52273=ORIENTED_EDGE('',*,*,#38077,.F.);
#52274=ORIENTED_EDGE('',*,*,#38078,.F.);
#52275=ORIENTED_EDGE('',*,*,#38079,.F.);
#52276=ORIENTED_EDGE('',*,*,#38074,.F.);
#52277=ORIENTED_EDGE('',*,*,#38079,.T.);
#52278=ORIENTED_EDGE('',*,*,#38080,.F.);
#52279=ORIENTED_EDGE('',*,*,#37840,.T.);
#52280=ORIENTED_EDGE('',*,*,#38075,.T.);
#52281=ORIENTED_EDGE('',*,*,#38081,.T.);
#52282=ORIENTED_EDGE('',*,*,#38082,.F.);
#52283=ORIENTED_EDGE('',*,*,#37842,.T.);
#52284=ORIENTED_EDGE('',*,*,#38083,.F.);
#52285=ORIENTED_EDGE('',*,*,#38084,.F.);
#52286=ORIENTED_EDGE('',*,*,#38085,.F.);
#52287=ORIENTED_EDGE('',*,*,#38086,.F.);
#52288=ORIENTED_EDGE('',*,*,#38081,.F.);
#52289=ORIENTED_EDGE('',*,*,#38086,.T.);
#52290=ORIENTED_EDGE('',*,*,#38087,.F.);
#52291=ORIENTED_EDGE('',*,*,#37843,.T.);
#52292=ORIENTED_EDGE('',*,*,#38082,.T.);
#52293=ORIENTED_EDGE('',*,*,#38088,.T.);
#52294=ORIENTED_EDGE('',*,*,#38089,.F.);
#52295=ORIENTED_EDGE('',*,*,#37845,.T.);
#52296=ORIENTED_EDGE('',*,*,#38090,.F.);
#52297=ORIENTED_EDGE('',*,*,#38091,.F.);
#52298=ORIENTED_EDGE('',*,*,#38092,.F.);
#52299=ORIENTED_EDGE('',*,*,#38093,.F.);
#52300=ORIENTED_EDGE('',*,*,#38088,.F.);
#52301=ORIENTED_EDGE('',*,*,#38093,.T.);
#52302=ORIENTED_EDGE('',*,*,#38094,.F.);
#52303=ORIENTED_EDGE('',*,*,#37846,.T.);
#52304=ORIENTED_EDGE('',*,*,#38089,.T.);
#52305=ORIENTED_EDGE('',*,*,#38095,.T.);
#52306=ORIENTED_EDGE('',*,*,#38096,.F.);
#52307=ORIENTED_EDGE('',*,*,#37848,.T.);
#52308=ORIENTED_EDGE('',*,*,#38097,.F.);
#52309=ORIENTED_EDGE('',*,*,#38098,.F.);
#52310=ORIENTED_EDGE('',*,*,#38099,.F.);
#52311=ORIENTED_EDGE('',*,*,#38100,.F.);
#52312=ORIENTED_EDGE('',*,*,#38095,.F.);
#52313=ORIENTED_EDGE('',*,*,#38100,.T.);
#52314=ORIENTED_EDGE('',*,*,#38101,.F.);
#52315=ORIENTED_EDGE('',*,*,#37849,.T.);
#52316=ORIENTED_EDGE('',*,*,#38096,.T.);
#52317=ORIENTED_EDGE('',*,*,#38102,.T.);
#52318=ORIENTED_EDGE('',*,*,#38103,.F.);
#52319=ORIENTED_EDGE('',*,*,#37851,.T.);
#52320=ORIENTED_EDGE('',*,*,#38104,.F.);
#52321=ORIENTED_EDGE('',*,*,#38105,.F.);
#52322=ORIENTED_EDGE('',*,*,#38106,.F.);
#52323=ORIENTED_EDGE('',*,*,#38107,.F.);
#52324=ORIENTED_EDGE('',*,*,#38102,.F.);
#52325=ORIENTED_EDGE('',*,*,#38107,.T.);
#52326=ORIENTED_EDGE('',*,*,#38108,.F.);
#52327=ORIENTED_EDGE('',*,*,#37852,.T.);
#52328=ORIENTED_EDGE('',*,*,#38103,.T.);
#52329=ORIENTED_EDGE('',*,*,#38109,.T.);
#52330=ORIENTED_EDGE('',*,*,#38110,.F.);
#52331=ORIENTED_EDGE('',*,*,#37854,.T.);
#52332=ORIENTED_EDGE('',*,*,#38111,.F.);
#52333=ORIENTED_EDGE('',*,*,#38112,.T.);
#52334=ORIENTED_EDGE('',*,*,#38113,.F.);
#52335=ORIENTED_EDGE('',*,*,#37855,.T.);
#52336=ORIENTED_EDGE('',*,*,#38110,.T.);
#52337=ORIENTED_EDGE('',*,*,#38114,.F.);
#52338=ORIENTED_EDGE('',*,*,#38115,.F.);
#52339=ORIENTED_EDGE('',*,*,#38112,.F.);
#52340=ORIENTED_EDGE('',*,*,#38109,.F.);
#52341=ORIENTED_EDGE('',*,*,#37857,.T.);
#52342=ORIENTED_EDGE('',*,*,#38116,.F.);
#52343=ORIENTED_EDGE('',*,*,#38117,.T.);
#52344=ORIENTED_EDGE('',*,*,#38118,.F.);
#52345=ORIENTED_EDGE('',*,*,#38119,.F.);
#52346=ORIENTED_EDGE('',*,*,#38117,.F.);
#52347=ORIENTED_EDGE('',*,*,#38120,.F.);
#52348=ORIENTED_EDGE('',*,*,#38121,.F.);
#52349=ORIENTED_EDGE('',*,*,#37858,.T.);
#52350=ORIENTED_EDGE('',*,*,#38118,.T.);
#52351=ORIENTED_EDGE('',*,*,#38119,.T.);
#52352=ORIENTED_EDGE('',*,*,#38122,.F.);
#52353=ORIENTED_EDGE('',*,*,#38123,.T.);
#52354=ORIENTED_EDGE('',*,*,#38124,.F.);
#52355=ORIENTED_EDGE('',*,*,#37860,.T.);
#52356=ORIENTED_EDGE('',*,*,#38125,.F.);
#52357=ORIENTED_EDGE('',*,*,#38126,.F.);
#52358=ORIENTED_EDGE('',*,*,#38127,.F.);
#52359=ORIENTED_EDGE('',*,*,#38128,.F.);
#52360=ORIENTED_EDGE('',*,*,#38123,.F.);
#52361=ORIENTED_EDGE('',*,*,#38128,.T.);
#52362=ORIENTED_EDGE('',*,*,#38129,.F.);
#52363=ORIENTED_EDGE('',*,*,#37861,.T.);
#52364=ORIENTED_EDGE('',*,*,#38124,.T.);
#52365=ORIENTED_EDGE('',*,*,#38130,.T.);
#52366=ORIENTED_EDGE('',*,*,#38131,.F.);
#52367=ORIENTED_EDGE('',*,*,#37863,.T.);
#52368=ORIENTED_EDGE('',*,*,#38132,.F.);
#52369=ORIENTED_EDGE('',*,*,#38133,.F.);
#52370=ORIENTED_EDGE('',*,*,#38134,.F.);
#52371=ORIENTED_EDGE('',*,*,#38135,.F.);
#52372=ORIENTED_EDGE('',*,*,#38130,.F.);
#52373=ORIENTED_EDGE('',*,*,#38135,.T.);
#52374=ORIENTED_EDGE('',*,*,#38136,.F.);
#52375=ORIENTED_EDGE('',*,*,#37864,.T.);
#52376=ORIENTED_EDGE('',*,*,#38131,.T.);
#52377=ORIENTED_EDGE('',*,*,#38137,.T.);
#52378=ORIENTED_EDGE('',*,*,#38138,.F.);
#52379=ORIENTED_EDGE('',*,*,#37866,.T.);
#52380=ORIENTED_EDGE('',*,*,#38139,.F.);
#52381=ORIENTED_EDGE('',*,*,#38140,.F.);
#52382=ORIENTED_EDGE('',*,*,#38141,.F.);
#52383=ORIENTED_EDGE('',*,*,#38142,.F.);
#52384=ORIENTED_EDGE('',*,*,#38137,.F.);
#52385=ORIENTED_EDGE('',*,*,#38142,.T.);
#52386=ORIENTED_EDGE('',*,*,#38143,.F.);
#52387=ORIENTED_EDGE('',*,*,#37867,.T.);
#52388=ORIENTED_EDGE('',*,*,#38138,.T.);
#52389=ORIENTED_EDGE('',*,*,#38144,.T.);
#52390=ORIENTED_EDGE('',*,*,#38145,.F.);
#52391=ORIENTED_EDGE('',*,*,#37869,.T.);
#52392=ORIENTED_EDGE('',*,*,#38146,.F.);
#52393=ORIENTED_EDGE('',*,*,#38147,.F.);
#52394=ORIENTED_EDGE('',*,*,#38148,.F.);
#52395=ORIENTED_EDGE('',*,*,#38149,.F.);
#52396=ORIENTED_EDGE('',*,*,#38144,.F.);
#52397=ORIENTED_EDGE('',*,*,#38149,.T.);
#52398=ORIENTED_EDGE('',*,*,#38150,.F.);
#52399=ORIENTED_EDGE('',*,*,#37870,.T.);
#52400=ORIENTED_EDGE('',*,*,#38145,.T.);
#52401=ORIENTED_EDGE('',*,*,#38151,.T.);
#52402=ORIENTED_EDGE('',*,*,#38152,.F.);
#52403=ORIENTED_EDGE('',*,*,#37872,.T.);
#52404=ORIENTED_EDGE('',*,*,#38153,.F.);
#52405=ORIENTED_EDGE('',*,*,#38154,.F.);
#52406=ORIENTED_EDGE('',*,*,#38155,.F.);
#52407=ORIENTED_EDGE('',*,*,#38156,.F.);
#52408=ORIENTED_EDGE('',*,*,#38151,.F.);
#52409=ORIENTED_EDGE('',*,*,#38156,.T.);
#52410=ORIENTED_EDGE('',*,*,#38157,.F.);
#52411=ORIENTED_EDGE('',*,*,#37873,.T.);
#52412=ORIENTED_EDGE('',*,*,#38152,.T.);
#52413=ORIENTED_EDGE('',*,*,#38158,.F.);
#52414=ORIENTED_EDGE('',*,*,#38159,.F.);
#52415=ORIENTED_EDGE('',*,*,#37963,.F.);
#52416=ORIENTED_EDGE('',*,*,#38160,.F.);
#52417=ORIENTED_EDGE('',*,*,#38160,.T.);
#52418=ORIENTED_EDGE('',*,*,#37965,.T.);
#52419=ORIENTED_EDGE('',*,*,#37875,.T.);
#52420=ORIENTED_EDGE('',*,*,#38161,.F.);
#52421=ORIENTED_EDGE('',*,*,#37876,.T.);
#52422=ORIENTED_EDGE('',*,*,#38162,.F.);
#52423=ORIENTED_EDGE('',*,*,#38163,.T.);
#52424=ORIENTED_EDGE('',*,*,#38164,.F.);
#52425=ORIENTED_EDGE('',*,*,#37878,.T.);
#52426=ORIENTED_EDGE('',*,*,#38165,.F.);
#52427=ORIENTED_EDGE('',*,*,#38166,.T.);
#52428=ORIENTED_EDGE('',*,*,#38167,.F.);
#52429=ORIENTED_EDGE('',*,*,#37879,.T.);
#52430=ORIENTED_EDGE('',*,*,#38167,.T.);
#52431=ORIENTED_EDGE('',*,*,#38168,.T.);
#52432=ORIENTED_EDGE('',*,*,#38169,.F.);
#52433=ORIENTED_EDGE('',*,*,#38168,.F.);
#52434=ORIENTED_EDGE('',*,*,#38166,.F.);
#52435=ORIENTED_EDGE('',*,*,#38170,.F.);
#52436=ORIENTED_EDGE('',*,*,#38171,.F.);
#52437=ORIENTED_EDGE('',*,*,#37881,.T.);
#52438=ORIENTED_EDGE('',*,*,#38172,.F.);
#52439=ORIENTED_EDGE('',*,*,#38173,.T.);
#52440=ORIENTED_EDGE('',*,*,#38174,.F.);
#52441=ORIENTED_EDGE('',*,*,#37882,.T.);
#52442=ORIENTED_EDGE('',*,*,#38174,.T.);
#52443=ORIENTED_EDGE('',*,*,#38175,.T.);
#52444=ORIENTED_EDGE('',*,*,#38176,.F.);
#52445=ORIENTED_EDGE('',*,*,#38175,.F.);
#52446=ORIENTED_EDGE('',*,*,#38173,.F.);
#52447=ORIENTED_EDGE('',*,*,#38177,.F.);
#52448=ORIENTED_EDGE('',*,*,#38178,.F.);
#52449=ORIENTED_EDGE('',*,*,#37884,.T.);
#52450=ORIENTED_EDGE('',*,*,#38179,.F.);
#52451=ORIENTED_EDGE('',*,*,#38180,.T.);
#52452=ORIENTED_EDGE('',*,*,#38181,.F.);
#52453=ORIENTED_EDGE('',*,*,#37885,.T.);
#52454=ORIENTED_EDGE('',*,*,#38181,.T.);
#52455=ORIENTED_EDGE('',*,*,#38182,.T.);
#52456=ORIENTED_EDGE('',*,*,#38183,.F.);
#52457=ORIENTED_EDGE('',*,*,#38182,.F.);
#52458=ORIENTED_EDGE('',*,*,#38180,.F.);
#52459=ORIENTED_EDGE('',*,*,#38184,.F.);
#52460=ORIENTED_EDGE('',*,*,#38185,.F.);
#52461=ORIENTED_EDGE('',*,*,#37887,.T.);
#52462=ORIENTED_EDGE('',*,*,#38186,.F.);
#52463=ORIENTED_EDGE('',*,*,#38187,.T.);
#52464=ORIENTED_EDGE('',*,*,#38188,.F.);
#52465=ORIENTED_EDGE('',*,*,#37888,.T.);
#52466=ORIENTED_EDGE('',*,*,#38188,.T.);
#52467=ORIENTED_EDGE('',*,*,#38189,.T.);
#52468=ORIENTED_EDGE('',*,*,#38190,.F.);
#52469=ORIENTED_EDGE('',*,*,#38189,.F.);
#52470=ORIENTED_EDGE('',*,*,#38187,.F.);
#52471=ORIENTED_EDGE('',*,*,#38191,.F.);
#52472=ORIENTED_EDGE('',*,*,#38192,.F.);
#52473=ORIENTED_EDGE('',*,*,#37890,.T.);
#52474=ORIENTED_EDGE('',*,*,#38193,.F.);
#52475=ORIENTED_EDGE('',*,*,#38194,.T.);
#52476=ORIENTED_EDGE('',*,*,#38195,.F.);
#52477=ORIENTED_EDGE('',*,*,#37891,.T.);
#52478=ORIENTED_EDGE('',*,*,#38195,.T.);
#52479=ORIENTED_EDGE('',*,*,#38196,.T.);
#52480=ORIENTED_EDGE('',*,*,#38197,.F.);
#52481=ORIENTED_EDGE('',*,*,#38196,.F.);
#52482=ORIENTED_EDGE('',*,*,#38194,.F.);
#52483=ORIENTED_EDGE('',*,*,#38198,.F.);
#52484=ORIENTED_EDGE('',*,*,#38199,.F.);
#52485=ORIENTED_EDGE('',*,*,#37893,.T.);
#52486=ORIENTED_EDGE('',*,*,#38200,.F.);
#52487=ORIENTED_EDGE('',*,*,#38201,.T.);
#52488=ORIENTED_EDGE('',*,*,#38202,.F.);
#52489=ORIENTED_EDGE('',*,*,#37894,.T.);
#52490=ORIENTED_EDGE('',*,*,#38202,.T.);
#52491=ORIENTED_EDGE('',*,*,#38203,.T.);
#52492=ORIENTED_EDGE('',*,*,#38204,.F.);
#52493=ORIENTED_EDGE('',*,*,#38203,.F.);
#52494=ORIENTED_EDGE('',*,*,#38201,.F.);
#52495=ORIENTED_EDGE('',*,*,#38205,.F.);
#52496=ORIENTED_EDGE('',*,*,#38206,.F.);
#52497=ORIENTED_EDGE('',*,*,#37896,.T.);
#52498=ORIENTED_EDGE('',*,*,#38207,.F.);
#52499=ORIENTED_EDGE('',*,*,#38208,.T.);
#52500=ORIENTED_EDGE('',*,*,#38209,.F.);
#52501=ORIENTED_EDGE('',*,*,#37897,.T.);
#52502=ORIENTED_EDGE('',*,*,#38209,.T.);
#52503=ORIENTED_EDGE('',*,*,#38210,.T.);
#52504=ORIENTED_EDGE('',*,*,#38211,.F.);
#52505=ORIENTED_EDGE('',*,*,#38210,.F.);
#52506=ORIENTED_EDGE('',*,*,#38208,.F.);
#52507=ORIENTED_EDGE('',*,*,#38212,.F.);
#52508=ORIENTED_EDGE('',*,*,#38213,.F.);
#52509=ORIENTED_EDGE('',*,*,#37899,.T.);
#52510=ORIENTED_EDGE('',*,*,#38214,.F.);
#52511=ORIENTED_EDGE('',*,*,#38215,.T.);
#52512=ORIENTED_EDGE('',*,*,#38216,.F.);
#52513=ORIENTED_EDGE('',*,*,#37900,.T.);
#52514=ORIENTED_EDGE('',*,*,#38216,.T.);
#52515=ORIENTED_EDGE('',*,*,#38217,.T.);
#52516=ORIENTED_EDGE('',*,*,#38218,.F.);
#52517=ORIENTED_EDGE('',*,*,#38217,.F.);
#52518=ORIENTED_EDGE('',*,*,#38215,.F.);
#52519=ORIENTED_EDGE('',*,*,#38219,.F.);
#52520=ORIENTED_EDGE('',*,*,#38220,.F.);
#52521=ORIENTED_EDGE('',*,*,#37902,.T.);
#52522=ORIENTED_EDGE('',*,*,#38221,.F.);
#52523=ORIENTED_EDGE('',*,*,#38222,.T.);
#52524=ORIENTED_EDGE('',*,*,#38223,.F.);
#52525=ORIENTED_EDGE('',*,*,#37903,.T.);
#52526=ORIENTED_EDGE('',*,*,#38223,.T.);
#52527=ORIENTED_EDGE('',*,*,#38224,.T.);
#52528=ORIENTED_EDGE('',*,*,#38225,.F.);
#52529=ORIENTED_EDGE('',*,*,#38224,.F.);
#52530=ORIENTED_EDGE('',*,*,#38222,.F.);
#52531=ORIENTED_EDGE('',*,*,#38226,.F.);
#52532=ORIENTED_EDGE('',*,*,#38227,.F.);
#52533=ORIENTED_EDGE('',*,*,#37905,.T.);
#52534=ORIENTED_EDGE('',*,*,#38228,.F.);
#52535=ORIENTED_EDGE('',*,*,#38229,.T.);
#52536=ORIENTED_EDGE('',*,*,#38230,.F.);
#52537=ORIENTED_EDGE('',*,*,#37906,.T.);
#52538=ORIENTED_EDGE('',*,*,#38230,.T.);
#52539=ORIENTED_EDGE('',*,*,#38231,.T.);
#52540=ORIENTED_EDGE('',*,*,#38232,.F.);
#52541=ORIENTED_EDGE('',*,*,#38231,.F.);
#52542=ORIENTED_EDGE('',*,*,#38229,.F.);
#52543=ORIENTED_EDGE('',*,*,#38233,.F.);
#52544=ORIENTED_EDGE('',*,*,#38234,.F.);
#52545=ORIENTED_EDGE('',*,*,#37908,.T.);
#52546=ORIENTED_EDGE('',*,*,#38235,.F.);
#52547=ORIENTED_EDGE('',*,*,#38236,.T.);
#52548=ORIENTED_EDGE('',*,*,#38237,.F.);
#52549=ORIENTED_EDGE('',*,*,#37909,.T.);
#52550=ORIENTED_EDGE('',*,*,#38237,.T.);
#52551=ORIENTED_EDGE('',*,*,#38238,.T.);
#52552=ORIENTED_EDGE('',*,*,#38239,.F.);
#52553=ORIENTED_EDGE('',*,*,#38238,.F.);
#52554=ORIENTED_EDGE('',*,*,#38236,.F.);
#52555=ORIENTED_EDGE('',*,*,#38240,.F.);
#52556=ORIENTED_EDGE('',*,*,#38241,.F.);
#52557=ORIENTED_EDGE('',*,*,#37911,.T.);
#52558=ORIENTED_EDGE('',*,*,#38242,.F.);
#52559=ORIENTED_EDGE('',*,*,#38243,.T.);
#52560=ORIENTED_EDGE('',*,*,#38244,.F.);
#52561=ORIENTED_EDGE('',*,*,#37912,.T.);
#52562=ORIENTED_EDGE('',*,*,#38244,.T.);
#52563=ORIENTED_EDGE('',*,*,#38245,.T.);
#52564=ORIENTED_EDGE('',*,*,#38246,.F.);
#52565=ORIENTED_EDGE('',*,*,#38245,.F.);
#52566=ORIENTED_EDGE('',*,*,#38243,.F.);
#52567=ORIENTED_EDGE('',*,*,#38247,.F.);
#52568=ORIENTED_EDGE('',*,*,#38248,.F.);
#52569=ORIENTED_EDGE('',*,*,#37914,.T.);
#52570=ORIENTED_EDGE('',*,*,#38249,.F.);
#52571=ORIENTED_EDGE('',*,*,#38250,.T.);
#52572=ORIENTED_EDGE('',*,*,#38251,.F.);
#52573=ORIENTED_EDGE('',*,*,#37915,.T.);
#52574=ORIENTED_EDGE('',*,*,#38251,.T.);
#52575=ORIENTED_EDGE('',*,*,#38252,.T.);
#52576=ORIENTED_EDGE('',*,*,#38253,.F.);
#52577=ORIENTED_EDGE('',*,*,#38252,.F.);
#52578=ORIENTED_EDGE('',*,*,#38250,.F.);
#52579=ORIENTED_EDGE('',*,*,#38254,.F.);
#52580=ORIENTED_EDGE('',*,*,#38255,.F.);
#52581=ORIENTED_EDGE('',*,*,#37917,.T.);
#52582=ORIENTED_EDGE('',*,*,#38256,.F.);
#52583=ORIENTED_EDGE('',*,*,#34419,.T.);
#52584=ORIENTED_EDGE('',*,*,#38257,.F.);
#52585=ORIENTED_EDGE('',*,*,#37918,.T.);
#52586=ORIENTED_EDGE('',*,*,#38257,.T.);
#52587=ORIENTED_EDGE('',*,*,#34418,.T.);
#52588=ORIENTED_EDGE('',*,*,#38258,.F.);
#52589=ORIENTED_EDGE('',*,*,#37920,.T.);
#52590=ORIENTED_EDGE('',*,*,#38259,.F.);
#52591=ORIENTED_EDGE('',*,*,#38260,.T.);
#52592=ORIENTED_EDGE('',*,*,#38261,.F.);
#52593=ORIENTED_EDGE('',*,*,#37921,.T.);
#52594=ORIENTED_EDGE('',*,*,#38261,.T.);
#52595=ORIENTED_EDGE('',*,*,#38262,.T.);
#52596=ORIENTED_EDGE('',*,*,#38263,.F.);
#52597=ORIENTED_EDGE('',*,*,#38262,.F.);
#52598=ORIENTED_EDGE('',*,*,#38260,.F.);
#52599=ORIENTED_EDGE('',*,*,#38264,.F.);
#52600=ORIENTED_EDGE('',*,*,#38265,.F.);
#52601=ORIENTED_EDGE('',*,*,#37923,.T.);
#52602=ORIENTED_EDGE('',*,*,#38266,.F.);
#52603=ORIENTED_EDGE('',*,*,#38267,.T.);
#52604=ORIENTED_EDGE('',*,*,#38268,.F.);
#52605=ORIENTED_EDGE('',*,*,#37924,.T.);
#52606=ORIENTED_EDGE('',*,*,#38268,.T.);
#52607=ORIENTED_EDGE('',*,*,#38269,.T.);
#52608=ORIENTED_EDGE('',*,*,#38270,.F.);
#52609=ORIENTED_EDGE('',*,*,#38269,.F.);
#52610=ORIENTED_EDGE('',*,*,#38267,.F.);
#52611=ORIENTED_EDGE('',*,*,#38271,.F.);
#52612=ORIENTED_EDGE('',*,*,#38272,.F.);
#52613=ORIENTED_EDGE('',*,*,#37926,.T.);
#52614=ORIENTED_EDGE('',*,*,#38273,.F.);
#52615=ORIENTED_EDGE('',*,*,#38274,.T.);
#52616=ORIENTED_EDGE('',*,*,#38275,.F.);
#52617=ORIENTED_EDGE('',*,*,#37927,.T.);
#52618=ORIENTED_EDGE('',*,*,#38275,.T.);
#52619=ORIENTED_EDGE('',*,*,#38276,.T.);
#52620=ORIENTED_EDGE('',*,*,#38277,.F.);
#52621=ORIENTED_EDGE('',*,*,#38276,.F.);
#52622=ORIENTED_EDGE('',*,*,#38274,.F.);
#52623=ORIENTED_EDGE('',*,*,#38278,.F.);
#52624=ORIENTED_EDGE('',*,*,#38279,.F.);
#52625=ORIENTED_EDGE('',*,*,#37929,.T.);
#52626=ORIENTED_EDGE('',*,*,#38280,.F.);
#52627=ORIENTED_EDGE('',*,*,#38281,.T.);
#52628=ORIENTED_EDGE('',*,*,#38282,.F.);
#52629=ORIENTED_EDGE('',*,*,#37930,.T.);
#52630=ORIENTED_EDGE('',*,*,#38282,.T.);
#52631=ORIENTED_EDGE('',*,*,#38283,.T.);
#52632=ORIENTED_EDGE('',*,*,#38284,.F.);
#52633=ORIENTED_EDGE('',*,*,#38283,.F.);
#52634=ORIENTED_EDGE('',*,*,#38281,.F.);
#52635=ORIENTED_EDGE('',*,*,#38285,.F.);
#52636=ORIENTED_EDGE('',*,*,#38286,.F.);
#52637=ORIENTED_EDGE('',*,*,#37932,.T.);
#52638=ORIENTED_EDGE('',*,*,#38287,.F.);
#52639=ORIENTED_EDGE('',*,*,#38288,.T.);
#52640=ORIENTED_EDGE('',*,*,#38289,.F.);
#52641=ORIENTED_EDGE('',*,*,#37933,.T.);
#52642=ORIENTED_EDGE('',*,*,#38289,.T.);
#52643=ORIENTED_EDGE('',*,*,#38290,.T.);
#52644=ORIENTED_EDGE('',*,*,#38291,.F.);
#52645=ORIENTED_EDGE('',*,*,#38290,.F.);
#52646=ORIENTED_EDGE('',*,*,#38288,.F.);
#52647=ORIENTED_EDGE('',*,*,#38292,.F.);
#52648=ORIENTED_EDGE('',*,*,#38293,.F.);
#52649=ORIENTED_EDGE('',*,*,#37935,.T.);
#52650=ORIENTED_EDGE('',*,*,#38294,.F.);
#52651=ORIENTED_EDGE('',*,*,#38295,.T.);
#52652=ORIENTED_EDGE('',*,*,#38296,.F.);
#52653=ORIENTED_EDGE('',*,*,#37936,.T.);
#52654=ORIENTED_EDGE('',*,*,#38296,.T.);
#52655=ORIENTED_EDGE('',*,*,#38297,.T.);
#52656=ORIENTED_EDGE('',*,*,#38298,.F.);
#52657=ORIENTED_EDGE('',*,*,#38297,.F.);
#52658=ORIENTED_EDGE('',*,*,#38295,.F.);
#52659=ORIENTED_EDGE('',*,*,#38299,.F.);
#52660=ORIENTED_EDGE('',*,*,#38300,.F.);
#52661=ORIENTED_EDGE('',*,*,#37938,.T.);
#52662=ORIENTED_EDGE('',*,*,#38301,.F.);
#52663=ORIENTED_EDGE('',*,*,#38302,.T.);
#52664=ORIENTED_EDGE('',*,*,#38303,.F.);
#52665=ORIENTED_EDGE('',*,*,#37939,.T.);
#52666=ORIENTED_EDGE('',*,*,#38303,.T.);
#52667=ORIENTED_EDGE('',*,*,#38304,.T.);
#52668=ORIENTED_EDGE('',*,*,#38305,.F.);
#52669=ORIENTED_EDGE('',*,*,#38304,.F.);
#52670=ORIENTED_EDGE('',*,*,#38302,.F.);
#52671=ORIENTED_EDGE('',*,*,#38306,.F.);
#52672=ORIENTED_EDGE('',*,*,#38307,.F.);
#52673=ORIENTED_EDGE('',*,*,#37941,.T.);
#52674=ORIENTED_EDGE('',*,*,#38308,.F.);
#52675=ORIENTED_EDGE('',*,*,#38309,.T.);
#52676=ORIENTED_EDGE('',*,*,#38310,.F.);
#52677=ORIENTED_EDGE('',*,*,#37942,.T.);
#52678=ORIENTED_EDGE('',*,*,#38310,.T.);
#52679=ORIENTED_EDGE('',*,*,#38311,.T.);
#52680=ORIENTED_EDGE('',*,*,#38312,.F.);
#52681=ORIENTED_EDGE('',*,*,#38311,.F.);
#52682=ORIENTED_EDGE('',*,*,#38309,.F.);
#52683=ORIENTED_EDGE('',*,*,#38313,.F.);
#52684=ORIENTED_EDGE('',*,*,#38314,.F.);
#52685=ORIENTED_EDGE('',*,*,#37944,.T.);
#52686=ORIENTED_EDGE('',*,*,#38315,.F.);
#52687=ORIENTED_EDGE('',*,*,#38316,.T.);
#52688=ORIENTED_EDGE('',*,*,#38317,.F.);
#52689=ORIENTED_EDGE('',*,*,#37945,.T.);
#52690=ORIENTED_EDGE('',*,*,#38317,.T.);
#52691=ORIENTED_EDGE('',*,*,#38318,.T.);
#52692=ORIENTED_EDGE('',*,*,#38319,.F.);
#52693=ORIENTED_EDGE('',*,*,#38318,.F.);
#52694=ORIENTED_EDGE('',*,*,#38316,.F.);
#52695=ORIENTED_EDGE('',*,*,#38320,.F.);
#52696=ORIENTED_EDGE('',*,*,#38321,.F.);
#52697=ORIENTED_EDGE('',*,*,#37947,.T.);
#52698=ORIENTED_EDGE('',*,*,#38322,.F.);
#52699=ORIENTED_EDGE('',*,*,#38323,.T.);
#52700=ORIENTED_EDGE('',*,*,#38324,.F.);
#52701=ORIENTED_EDGE('',*,*,#37948,.T.);
#52702=ORIENTED_EDGE('',*,*,#38324,.T.);
#52703=ORIENTED_EDGE('',*,*,#38325,.T.);
#52704=ORIENTED_EDGE('',*,*,#38326,.F.);
#52705=ORIENTED_EDGE('',*,*,#38325,.F.);
#52706=ORIENTED_EDGE('',*,*,#38323,.F.);
#52707=ORIENTED_EDGE('',*,*,#38327,.F.);
#52708=ORIENTED_EDGE('',*,*,#38328,.F.);
#52709=ORIENTED_EDGE('',*,*,#37950,.T.);
#52710=ORIENTED_EDGE('',*,*,#38329,.F.);
#52711=ORIENTED_EDGE('',*,*,#38330,.T.);
#52712=ORIENTED_EDGE('',*,*,#38331,.F.);
#52713=ORIENTED_EDGE('',*,*,#37951,.T.);
#52714=ORIENTED_EDGE('',*,*,#38331,.T.);
#52715=ORIENTED_EDGE('',*,*,#38332,.T.);
#52716=ORIENTED_EDGE('',*,*,#38333,.F.);
#52717=ORIENTED_EDGE('',*,*,#38332,.F.);
#52718=ORIENTED_EDGE('',*,*,#38330,.F.);
#52719=ORIENTED_EDGE('',*,*,#38334,.F.);
#52720=ORIENTED_EDGE('',*,*,#38335,.F.);
#52721=ORIENTED_EDGE('',*,*,#37953,.T.);
#52722=ORIENTED_EDGE('',*,*,#38336,.F.);
#52723=ORIENTED_EDGE('',*,*,#38337,.T.);
#52724=ORIENTED_EDGE('',*,*,#38338,.F.);
#52725=ORIENTED_EDGE('',*,*,#37954,.T.);
#52726=ORIENTED_EDGE('',*,*,#38338,.T.);
#52727=ORIENTED_EDGE('',*,*,#38339,.T.);
#52728=ORIENTED_EDGE('',*,*,#38340,.F.);
#52729=ORIENTED_EDGE('',*,*,#38339,.F.);
#52730=ORIENTED_EDGE('',*,*,#38337,.F.);
#52731=ORIENTED_EDGE('',*,*,#38341,.F.);
#52732=ORIENTED_EDGE('',*,*,#38342,.F.);
#52733=ORIENTED_EDGE('',*,*,#37956,.T.);
#52734=ORIENTED_EDGE('',*,*,#38343,.F.);
#52735=ORIENTED_EDGE('',*,*,#38344,.T.);
#52736=ORIENTED_EDGE('',*,*,#38345,.F.);
#52737=ORIENTED_EDGE('',*,*,#37957,.T.);
#52738=ORIENTED_EDGE('',*,*,#38345,.T.);
#52739=ORIENTED_EDGE('',*,*,#38346,.T.);
#52740=ORIENTED_EDGE('',*,*,#38347,.F.);
#52741=ORIENTED_EDGE('',*,*,#38346,.F.);
#52742=ORIENTED_EDGE('',*,*,#38344,.F.);
#52743=ORIENTED_EDGE('',*,*,#38348,.F.);
#52744=ORIENTED_EDGE('',*,*,#38349,.F.);
#52745=ORIENTED_EDGE('',*,*,#37959,.T.);
#52746=ORIENTED_EDGE('',*,*,#38350,.F.);
#52747=ORIENTED_EDGE('',*,*,#38351,.T.);
#52748=ORIENTED_EDGE('',*,*,#38352,.F.);
#52749=ORIENTED_EDGE('',*,*,#38353,.T.);
#52750=ORIENTED_EDGE('',*,*,#38354,.F.);
#52751=ORIENTED_EDGE('',*,*,#37960,.T.);
#52752=ORIENTED_EDGE('',*,*,#38352,.T.);
#52753=ORIENTED_EDGE('',*,*,#38355,.F.);
#52754=ORIENTED_EDGE('',*,*,#38356,.F.);
#52755=ORIENTED_EDGE('',*,*,#38353,.F.);
#52756=ORIENTED_EDGE('',*,*,#38351,.F.);
#52757=ORIENTED_EDGE('',*,*,#38163,.F.);
#52758=ORIENTED_EDGE('',*,*,#38357,.F.);
#52759=ORIENTED_EDGE('',*,*,#38358,.F.);
#52760=ORIENTED_EDGE('',*,*,#38359,.F.);
#52761=ORIENTED_EDGE('',*,*,#37962,.T.);
#52762=ORIENTED_EDGE('',*,*,#38360,.F.);
#52763=ORIENTED_EDGE('',*,*,#38357,.T.);
#52764=ORIENTED_EDGE('',*,*,#38162,.T.);
#52765=ORIENTED_EDGE('',*,*,#38361,.F.);
#52766=ORIENTED_EDGE('',*,*,#37964,.T.);
#52767=ORIENTED_EDGE('',*,*,#38159,.T.);
#52768=ORIENTED_EDGE('',*,*,#38362,.F.);
#52769=ORIENTED_EDGE('',*,*,#38363,.F.);
#52770=ORIENTED_EDGE('',*,*,#38364,.F.);
#52771=ORIENTED_EDGE('',*,*,#37969,.T.);
#52772=ORIENTED_EDGE('',*,*,#37968,.T.);
#52773=ORIENTED_EDGE('',*,*,#38365,.F.);
#52774=ORIENTED_EDGE('',*,*,#37972,.T.);
#52775=ORIENTED_EDGE('',*,*,#37970,.T.);
#52776=ORIENTED_EDGE('',*,*,#38364,.T.);
#52777=ORIENTED_EDGE('',*,*,#38366,.F.);
#52778=ORIENTED_EDGE('',*,*,#38367,.F.);
#52779=ORIENTED_EDGE('',*,*,#37976,.T.);
#52780=ORIENTED_EDGE('',*,*,#37975,.T.);
#52781=ORIENTED_EDGE('',*,*,#38368,.F.);
#52782=ORIENTED_EDGE('',*,*,#37979,.T.);
#52783=ORIENTED_EDGE('',*,*,#37977,.T.);
#52784=ORIENTED_EDGE('',*,*,#38367,.T.);
#52785=ORIENTED_EDGE('',*,*,#38369,.F.);
#52786=ORIENTED_EDGE('',*,*,#38370,.F.);
#52787=ORIENTED_EDGE('',*,*,#37983,.T.);
#52788=ORIENTED_EDGE('',*,*,#37982,.T.);
#52789=ORIENTED_EDGE('',*,*,#38371,.F.);
#52790=ORIENTED_EDGE('',*,*,#37986,.T.);
#52791=ORIENTED_EDGE('',*,*,#37984,.T.);
#52792=ORIENTED_EDGE('',*,*,#38370,.T.);
#52793=ORIENTED_EDGE('',*,*,#38372,.F.);
#52794=ORIENTED_EDGE('',*,*,#38373,.F.);
#52795=ORIENTED_EDGE('',*,*,#37990,.T.);
#52796=ORIENTED_EDGE('',*,*,#37989,.T.);
#52797=ORIENTED_EDGE('',*,*,#38374,.F.);
#52798=ORIENTED_EDGE('',*,*,#37993,.T.);
#52799=ORIENTED_EDGE('',*,*,#37991,.T.);
#52800=ORIENTED_EDGE('',*,*,#38373,.T.);
#52801=ORIENTED_EDGE('',*,*,#38375,.F.);
#52802=ORIENTED_EDGE('',*,*,#38376,.F.);
#52803=ORIENTED_EDGE('',*,*,#37997,.T.);
#52804=ORIENTED_EDGE('',*,*,#37996,.T.);
#52805=ORIENTED_EDGE('',*,*,#38377,.F.);
#52806=ORIENTED_EDGE('',*,*,#38000,.T.);
#52807=ORIENTED_EDGE('',*,*,#37998,.T.);
#52808=ORIENTED_EDGE('',*,*,#38376,.T.);
#52809=ORIENTED_EDGE('',*,*,#38378,.F.);
#52810=ORIENTED_EDGE('',*,*,#38379,.F.);
#52811=ORIENTED_EDGE('',*,*,#38004,.T.);
#52812=ORIENTED_EDGE('',*,*,#38003,.T.);
#52813=ORIENTED_EDGE('',*,*,#38380,.F.);
#52814=ORIENTED_EDGE('',*,*,#38007,.T.);
#52815=ORIENTED_EDGE('',*,*,#38005,.T.);
#52816=ORIENTED_EDGE('',*,*,#38379,.T.);
#52817=ORIENTED_EDGE('',*,*,#38381,.F.);
#52818=ORIENTED_EDGE('',*,*,#38382,.F.);
#52819=ORIENTED_EDGE('',*,*,#34423,.T.);
#52820=ORIENTED_EDGE('',*,*,#38009,.T.);
#52821=ORIENTED_EDGE('',*,*,#38383,.F.);
#52822=ORIENTED_EDGE('',*,*,#38010,.T.);
#52823=ORIENTED_EDGE('',*,*,#34424,.T.);
#52824=ORIENTED_EDGE('',*,*,#38382,.T.);
#52825=ORIENTED_EDGE('',*,*,#38384,.F.);
#52826=ORIENTED_EDGE('',*,*,#38385,.F.);
#52827=ORIENTED_EDGE('',*,*,#38014,.T.);
#52828=ORIENTED_EDGE('',*,*,#38013,.T.);
#52829=ORIENTED_EDGE('',*,*,#38386,.F.);
#52830=ORIENTED_EDGE('',*,*,#38017,.T.);
#52831=ORIENTED_EDGE('',*,*,#38015,.T.);
#52832=ORIENTED_EDGE('',*,*,#38385,.T.);
#52833=ORIENTED_EDGE('',*,*,#38387,.F.);
#52834=ORIENTED_EDGE('',*,*,#38388,.F.);
#52835=ORIENTED_EDGE('',*,*,#38021,.T.);
#52836=ORIENTED_EDGE('',*,*,#38020,.T.);
#52837=ORIENTED_EDGE('',*,*,#38389,.F.);
#52838=ORIENTED_EDGE('',*,*,#38024,.T.);
#52839=ORIENTED_EDGE('',*,*,#38022,.T.);
#52840=ORIENTED_EDGE('',*,*,#38388,.T.);
#52841=ORIENTED_EDGE('',*,*,#38390,.F.);
#52842=ORIENTED_EDGE('',*,*,#38391,.F.);
#52843=ORIENTED_EDGE('',*,*,#38028,.T.);
#52844=ORIENTED_EDGE('',*,*,#38027,.T.);
#52845=ORIENTED_EDGE('',*,*,#38392,.F.);
#52846=ORIENTED_EDGE('',*,*,#38031,.T.);
#52847=ORIENTED_EDGE('',*,*,#38029,.T.);
#52848=ORIENTED_EDGE('',*,*,#38391,.T.);
#52849=ORIENTED_EDGE('',*,*,#38393,.F.);
#52850=ORIENTED_EDGE('',*,*,#38394,.F.);
#52851=ORIENTED_EDGE('',*,*,#38035,.T.);
#52852=ORIENTED_EDGE('',*,*,#38034,.T.);
#52853=ORIENTED_EDGE('',*,*,#38395,.F.);
#52854=ORIENTED_EDGE('',*,*,#38038,.T.);
#52855=ORIENTED_EDGE('',*,*,#38036,.T.);
#52856=ORIENTED_EDGE('',*,*,#38394,.T.);
#52857=ORIENTED_EDGE('',*,*,#38396,.F.);
#52858=ORIENTED_EDGE('',*,*,#38397,.F.);
#52859=ORIENTED_EDGE('',*,*,#38042,.T.);
#52860=ORIENTED_EDGE('',*,*,#38041,.T.);
#52861=ORIENTED_EDGE('',*,*,#38398,.F.);
#52862=ORIENTED_EDGE('',*,*,#38045,.T.);
#52863=ORIENTED_EDGE('',*,*,#38043,.T.);
#52864=ORIENTED_EDGE('',*,*,#38397,.T.);
#52865=ORIENTED_EDGE('',*,*,#38399,.F.);
#52866=ORIENTED_EDGE('',*,*,#38400,.F.);
#52867=ORIENTED_EDGE('',*,*,#38049,.T.);
#52868=ORIENTED_EDGE('',*,*,#38048,.T.);
#52869=ORIENTED_EDGE('',*,*,#38401,.F.);
#52870=ORIENTED_EDGE('',*,*,#38052,.T.);
#52871=ORIENTED_EDGE('',*,*,#38050,.T.);
#52872=ORIENTED_EDGE('',*,*,#38400,.T.);
#52873=ORIENTED_EDGE('',*,*,#38402,.F.);
#52874=ORIENTED_EDGE('',*,*,#38403,.F.);
#52875=ORIENTED_EDGE('',*,*,#38056,.T.);
#52876=ORIENTED_EDGE('',*,*,#38055,.T.);
#52877=ORIENTED_EDGE('',*,*,#38404,.F.);
#52878=ORIENTED_EDGE('',*,*,#38059,.T.);
#52879=ORIENTED_EDGE('',*,*,#38057,.T.);
#52880=ORIENTED_EDGE('',*,*,#38403,.T.);
#52881=ORIENTED_EDGE('',*,*,#38405,.F.);
#52882=ORIENTED_EDGE('',*,*,#38406,.F.);
#52883=ORIENTED_EDGE('',*,*,#38063,.T.);
#52884=ORIENTED_EDGE('',*,*,#38062,.T.);
#52885=ORIENTED_EDGE('',*,*,#38407,.F.);
#52886=ORIENTED_EDGE('',*,*,#38066,.T.);
#52887=ORIENTED_EDGE('',*,*,#38064,.T.);
#52888=ORIENTED_EDGE('',*,*,#38406,.T.);
#52889=ORIENTED_EDGE('',*,*,#38408,.F.);
#52890=ORIENTED_EDGE('',*,*,#38409,.F.);
#52891=ORIENTED_EDGE('',*,*,#38070,.T.);
#52892=ORIENTED_EDGE('',*,*,#38069,.T.);
#52893=ORIENTED_EDGE('',*,*,#38410,.F.);
#52894=ORIENTED_EDGE('',*,*,#38073,.T.);
#52895=ORIENTED_EDGE('',*,*,#38071,.T.);
#52896=ORIENTED_EDGE('',*,*,#38409,.T.);
#52897=ORIENTED_EDGE('',*,*,#38411,.F.);
#52898=ORIENTED_EDGE('',*,*,#38412,.F.);
#52899=ORIENTED_EDGE('',*,*,#38077,.T.);
#52900=ORIENTED_EDGE('',*,*,#38076,.T.);
#52901=ORIENTED_EDGE('',*,*,#38413,.F.);
#52902=ORIENTED_EDGE('',*,*,#38080,.T.);
#52903=ORIENTED_EDGE('',*,*,#38078,.T.);
#52904=ORIENTED_EDGE('',*,*,#38412,.T.);
#52905=ORIENTED_EDGE('',*,*,#38414,.F.);
#52906=ORIENTED_EDGE('',*,*,#38415,.F.);
#52907=ORIENTED_EDGE('',*,*,#38084,.T.);
#52908=ORIENTED_EDGE('',*,*,#38083,.T.);
#52909=ORIENTED_EDGE('',*,*,#38416,.F.);
#52910=ORIENTED_EDGE('',*,*,#38087,.T.);
#52911=ORIENTED_EDGE('',*,*,#38085,.T.);
#52912=ORIENTED_EDGE('',*,*,#38415,.T.);
#52913=ORIENTED_EDGE('',*,*,#38417,.F.);
#52914=ORIENTED_EDGE('',*,*,#38418,.F.);
#52915=ORIENTED_EDGE('',*,*,#38091,.T.);
#52916=ORIENTED_EDGE('',*,*,#38090,.T.);
#52917=ORIENTED_EDGE('',*,*,#38419,.F.);
#52918=ORIENTED_EDGE('',*,*,#38094,.T.);
#52919=ORIENTED_EDGE('',*,*,#38092,.T.);
#52920=ORIENTED_EDGE('',*,*,#38418,.T.);
#52921=ORIENTED_EDGE('',*,*,#38420,.F.);
#52922=ORIENTED_EDGE('',*,*,#38421,.F.);
#52923=ORIENTED_EDGE('',*,*,#38098,.T.);
#52924=ORIENTED_EDGE('',*,*,#38097,.T.);
#52925=ORIENTED_EDGE('',*,*,#38422,.F.);
#52926=ORIENTED_EDGE('',*,*,#38101,.T.);
#52927=ORIENTED_EDGE('',*,*,#38099,.T.);
#52928=ORIENTED_EDGE('',*,*,#38421,.T.);
#52929=ORIENTED_EDGE('',*,*,#38423,.F.);
#52930=ORIENTED_EDGE('',*,*,#38424,.F.);
#52931=ORIENTED_EDGE('',*,*,#38105,.T.);
#52932=ORIENTED_EDGE('',*,*,#38104,.T.);
#52933=ORIENTED_EDGE('',*,*,#38425,.F.);
#52934=ORIENTED_EDGE('',*,*,#38108,.T.);
#52935=ORIENTED_EDGE('',*,*,#38106,.T.);
#52936=ORIENTED_EDGE('',*,*,#38424,.T.);
#52937=ORIENTED_EDGE('',*,*,#38426,.F.);
#52938=ORIENTED_EDGE('',*,*,#38427,.F.);
#52939=ORIENTED_EDGE('',*,*,#38114,.T.);
#52940=ORIENTED_EDGE('',*,*,#38111,.T.);
#52941=ORIENTED_EDGE('',*,*,#38115,.T.);
#52942=ORIENTED_EDGE('',*,*,#38427,.T.);
#52943=ORIENTED_EDGE('',*,*,#38428,.F.);
#52944=ORIENTED_EDGE('',*,*,#38113,.T.);
#52945=ORIENTED_EDGE('',*,*,#38120,.T.);
#52946=ORIENTED_EDGE('',*,*,#38116,.T.);
#52947=ORIENTED_EDGE('',*,*,#38429,.F.);
#52948=ORIENTED_EDGE('',*,*,#38430,.F.);
#52949=ORIENTED_EDGE('',*,*,#38431,.F.);
#52950=ORIENTED_EDGE('',*,*,#38122,.T.);
#52951=ORIENTED_EDGE('',*,*,#38121,.T.);
#52952=ORIENTED_EDGE('',*,*,#38430,.T.);
#52953=ORIENTED_EDGE('',*,*,#38432,.F.);
#52954=ORIENTED_EDGE('',*,*,#38433,.F.);
#52955=ORIENTED_EDGE('',*,*,#38126,.T.);
#52956=ORIENTED_EDGE('',*,*,#38125,.T.);
#52957=ORIENTED_EDGE('',*,*,#38434,.F.);
#52958=ORIENTED_EDGE('',*,*,#38129,.T.);
#52959=ORIENTED_EDGE('',*,*,#38127,.T.);
#52960=ORIENTED_EDGE('',*,*,#38433,.T.);
#52961=ORIENTED_EDGE('',*,*,#38435,.F.);
#52962=ORIENTED_EDGE('',*,*,#38436,.F.);
#52963=ORIENTED_EDGE('',*,*,#38133,.T.);
#52964=ORIENTED_EDGE('',*,*,#38132,.T.);
#52965=ORIENTED_EDGE('',*,*,#38437,.F.);
#52966=ORIENTED_EDGE('',*,*,#38136,.T.);
#52967=ORIENTED_EDGE('',*,*,#38134,.T.);
#52968=ORIENTED_EDGE('',*,*,#38436,.T.);
#52969=ORIENTED_EDGE('',*,*,#38438,.F.);
#52970=ORIENTED_EDGE('',*,*,#38439,.F.);
#52971=ORIENTED_EDGE('',*,*,#38140,.T.);
#52972=ORIENTED_EDGE('',*,*,#38139,.T.);
#52973=ORIENTED_EDGE('',*,*,#38440,.F.);
#52974=ORIENTED_EDGE('',*,*,#38143,.T.);
#52975=ORIENTED_EDGE('',*,*,#38141,.T.);
#52976=ORIENTED_EDGE('',*,*,#38439,.T.);
#52977=ORIENTED_EDGE('',*,*,#38441,.F.);
#52978=ORIENTED_EDGE('',*,*,#38442,.F.);
#52979=ORIENTED_EDGE('',*,*,#38147,.T.);
#52980=ORIENTED_EDGE('',*,*,#38146,.T.);
#52981=ORIENTED_EDGE('',*,*,#38443,.F.);
#52982=ORIENTED_EDGE('',*,*,#38150,.T.);
#52983=ORIENTED_EDGE('',*,*,#38148,.T.);
#52984=ORIENTED_EDGE('',*,*,#38442,.T.);
#52985=ORIENTED_EDGE('',*,*,#38444,.F.);
#52986=ORIENTED_EDGE('',*,*,#38445,.F.);
#52987=ORIENTED_EDGE('',*,*,#38154,.T.);
#52988=ORIENTED_EDGE('',*,*,#38153,.T.);
#52989=ORIENTED_EDGE('',*,*,#38446,.F.);
#52990=ORIENTED_EDGE('',*,*,#38157,.T.);
#52991=ORIENTED_EDGE('',*,*,#38155,.T.);
#52992=ORIENTED_EDGE('',*,*,#38445,.T.);
#52993=ORIENTED_EDGE('',*,*,#38447,.F.);
#52994=ORIENTED_EDGE('',*,*,#38362,.T.);
#52995=ORIENTED_EDGE('',*,*,#38158,.T.);
#52996=ORIENTED_EDGE('',*,*,#38161,.T.);
#52997=ORIENTED_EDGE('',*,*,#38359,.T.);
#52998=ORIENTED_EDGE('',*,*,#38448,.F.);
#52999=ORIENTED_EDGE('',*,*,#38449,.F.);
#53000=ORIENTED_EDGE('',*,*,#38164,.T.);
#53001=ORIENTED_EDGE('',*,*,#38170,.T.);
#53002=ORIENTED_EDGE('',*,*,#38165,.T.);
#53003=ORIENTED_EDGE('',*,*,#38450,.F.);
#53004=ORIENTED_EDGE('',*,*,#38451,.F.);
#53005=ORIENTED_EDGE('',*,*,#38171,.T.);
#53006=ORIENTED_EDGE('',*,*,#38451,.T.);
#53007=ORIENTED_EDGE('',*,*,#38452,.F.);
#53008=ORIENTED_EDGE('',*,*,#38169,.T.);
#53009=ORIENTED_EDGE('',*,*,#38177,.T.);
#53010=ORIENTED_EDGE('',*,*,#38172,.T.);
#53011=ORIENTED_EDGE('',*,*,#38453,.F.);
#53012=ORIENTED_EDGE('',*,*,#38454,.F.);
#53013=ORIENTED_EDGE('',*,*,#38178,.T.);
#53014=ORIENTED_EDGE('',*,*,#38454,.T.);
#53015=ORIENTED_EDGE('',*,*,#38455,.F.);
#53016=ORIENTED_EDGE('',*,*,#38176,.T.);
#53017=ORIENTED_EDGE('',*,*,#38184,.T.);
#53018=ORIENTED_EDGE('',*,*,#38179,.T.);
#53019=ORIENTED_EDGE('',*,*,#38456,.F.);
#53020=ORIENTED_EDGE('',*,*,#38457,.F.);
#53021=ORIENTED_EDGE('',*,*,#38185,.T.);
#53022=ORIENTED_EDGE('',*,*,#38457,.T.);
#53023=ORIENTED_EDGE('',*,*,#38458,.F.);
#53024=ORIENTED_EDGE('',*,*,#38183,.T.);
#53025=ORIENTED_EDGE('',*,*,#38191,.T.);
#53026=ORIENTED_EDGE('',*,*,#38186,.T.);
#53027=ORIENTED_EDGE('',*,*,#38459,.F.);
#53028=ORIENTED_EDGE('',*,*,#38460,.F.);
#53029=ORIENTED_EDGE('',*,*,#38192,.T.);
#53030=ORIENTED_EDGE('',*,*,#38460,.T.);
#53031=ORIENTED_EDGE('',*,*,#38461,.F.);
#53032=ORIENTED_EDGE('',*,*,#38190,.T.);
#53033=ORIENTED_EDGE('',*,*,#38198,.T.);
#53034=ORIENTED_EDGE('',*,*,#38193,.T.);
#53035=ORIENTED_EDGE('',*,*,#38462,.F.);
#53036=ORIENTED_EDGE('',*,*,#38463,.F.);
#53037=ORIENTED_EDGE('',*,*,#38199,.T.);
#53038=ORIENTED_EDGE('',*,*,#38463,.T.);
#53039=ORIENTED_EDGE('',*,*,#38464,.F.);
#53040=ORIENTED_EDGE('',*,*,#38197,.T.);
#53041=ORIENTED_EDGE('',*,*,#38205,.T.);
#53042=ORIENTED_EDGE('',*,*,#38200,.T.);
#53043=ORIENTED_EDGE('',*,*,#38465,.F.);
#53044=ORIENTED_EDGE('',*,*,#38466,.F.);
#53045=ORIENTED_EDGE('',*,*,#38206,.T.);
#53046=ORIENTED_EDGE('',*,*,#38466,.T.);
#53047=ORIENTED_EDGE('',*,*,#38467,.F.);
#53048=ORIENTED_EDGE('',*,*,#38204,.T.);
#53049=ORIENTED_EDGE('',*,*,#38212,.T.);
#53050=ORIENTED_EDGE('',*,*,#38207,.T.);
#53051=ORIENTED_EDGE('',*,*,#38468,.F.);
#53052=ORIENTED_EDGE('',*,*,#38469,.F.);
#53053=ORIENTED_EDGE('',*,*,#38213,.T.);
#53054=ORIENTED_EDGE('',*,*,#38469,.T.);
#53055=ORIENTED_EDGE('',*,*,#38470,.F.);
#53056=ORIENTED_EDGE('',*,*,#38211,.T.);
#53057=ORIENTED_EDGE('',*,*,#38219,.T.);
#53058=ORIENTED_EDGE('',*,*,#38214,.T.);
#53059=ORIENTED_EDGE('',*,*,#38471,.F.);
#53060=ORIENTED_EDGE('',*,*,#38472,.F.);
#53061=ORIENTED_EDGE('',*,*,#38220,.T.);
#53062=ORIENTED_EDGE('',*,*,#38472,.T.);
#53063=ORIENTED_EDGE('',*,*,#38473,.F.);
#53064=ORIENTED_EDGE('',*,*,#38218,.T.);
#53065=ORIENTED_EDGE('',*,*,#38226,.T.);
#53066=ORIENTED_EDGE('',*,*,#38221,.T.);
#53067=ORIENTED_EDGE('',*,*,#38474,.F.);
#53068=ORIENTED_EDGE('',*,*,#38475,.F.);
#53069=ORIENTED_EDGE('',*,*,#38227,.T.);
#53070=ORIENTED_EDGE('',*,*,#38475,.T.);
#53071=ORIENTED_EDGE('',*,*,#38476,.F.);
#53072=ORIENTED_EDGE('',*,*,#38225,.T.);
#53073=ORIENTED_EDGE('',*,*,#38233,.T.);
#53074=ORIENTED_EDGE('',*,*,#38228,.T.);
#53075=ORIENTED_EDGE('',*,*,#38477,.F.);
#53076=ORIENTED_EDGE('',*,*,#38478,.F.);
#53077=ORIENTED_EDGE('',*,*,#38234,.T.);
#53078=ORIENTED_EDGE('',*,*,#38478,.T.);
#53079=ORIENTED_EDGE('',*,*,#38479,.F.);
#53080=ORIENTED_EDGE('',*,*,#38232,.T.);
#53081=ORIENTED_EDGE('',*,*,#38240,.T.);
#53082=ORIENTED_EDGE('',*,*,#38235,.T.);
#53083=ORIENTED_EDGE('',*,*,#38480,.F.);
#53084=ORIENTED_EDGE('',*,*,#38481,.F.);
#53085=ORIENTED_EDGE('',*,*,#38241,.T.);
#53086=ORIENTED_EDGE('',*,*,#38481,.T.);
#53087=ORIENTED_EDGE('',*,*,#38482,.F.);
#53088=ORIENTED_EDGE('',*,*,#38239,.T.);
#53089=ORIENTED_EDGE('',*,*,#38247,.T.);
#53090=ORIENTED_EDGE('',*,*,#38242,.T.);
#53091=ORIENTED_EDGE('',*,*,#38483,.F.);
#53092=ORIENTED_EDGE('',*,*,#38484,.F.);
#53093=ORIENTED_EDGE('',*,*,#38248,.T.);
#53094=ORIENTED_EDGE('',*,*,#38484,.T.);
#53095=ORIENTED_EDGE('',*,*,#38485,.F.);
#53096=ORIENTED_EDGE('',*,*,#38246,.T.);
#53097=ORIENTED_EDGE('',*,*,#38254,.T.);
#53098=ORIENTED_EDGE('',*,*,#38249,.T.);
#53099=ORIENTED_EDGE('',*,*,#38486,.F.);
#53100=ORIENTED_EDGE('',*,*,#38487,.F.);
#53101=ORIENTED_EDGE('',*,*,#38255,.T.);
#53102=ORIENTED_EDGE('',*,*,#38487,.T.);
#53103=ORIENTED_EDGE('',*,*,#38488,.F.);
#53104=ORIENTED_EDGE('',*,*,#38253,.T.);
#53105=ORIENTED_EDGE('',*,*,#34420,.T.);
#53106=ORIENTED_EDGE('',*,*,#38256,.T.);
#53107=ORIENTED_EDGE('',*,*,#38489,.F.);
#53108=ORIENTED_EDGE('',*,*,#38490,.F.);
#53109=ORIENTED_EDGE('',*,*,#34417,.T.);
#53110=ORIENTED_EDGE('',*,*,#38490,.T.);
#53111=ORIENTED_EDGE('',*,*,#38491,.F.);
#53112=ORIENTED_EDGE('',*,*,#38258,.T.);
#53113=ORIENTED_EDGE('',*,*,#38264,.T.);
#53114=ORIENTED_EDGE('',*,*,#38259,.T.);
#53115=ORIENTED_EDGE('',*,*,#38492,.F.);
#53116=ORIENTED_EDGE('',*,*,#38493,.F.);
#53117=ORIENTED_EDGE('',*,*,#38265,.T.);
#53118=ORIENTED_EDGE('',*,*,#38493,.T.);
#53119=ORIENTED_EDGE('',*,*,#38494,.F.);
#53120=ORIENTED_EDGE('',*,*,#38263,.T.);
#53121=ORIENTED_EDGE('',*,*,#38271,.T.);
#53122=ORIENTED_EDGE('',*,*,#38266,.T.);
#53123=ORIENTED_EDGE('',*,*,#38495,.F.);
#53124=ORIENTED_EDGE('',*,*,#38496,.F.);
#53125=ORIENTED_EDGE('',*,*,#38272,.T.);
#53126=ORIENTED_EDGE('',*,*,#38496,.T.);
#53127=ORIENTED_EDGE('',*,*,#38497,.F.);
#53128=ORIENTED_EDGE('',*,*,#38270,.T.);
#53129=ORIENTED_EDGE('',*,*,#38278,.T.);
#53130=ORIENTED_EDGE('',*,*,#38273,.T.);
#53131=ORIENTED_EDGE('',*,*,#38498,.F.);
#53132=ORIENTED_EDGE('',*,*,#38499,.F.);
#53133=ORIENTED_EDGE('',*,*,#38279,.T.);
#53134=ORIENTED_EDGE('',*,*,#38499,.T.);
#53135=ORIENTED_EDGE('',*,*,#38500,.F.);
#53136=ORIENTED_EDGE('',*,*,#38277,.T.);
#53137=ORIENTED_EDGE('',*,*,#38285,.T.);
#53138=ORIENTED_EDGE('',*,*,#38280,.T.);
#53139=ORIENTED_EDGE('',*,*,#38501,.F.);
#53140=ORIENTED_EDGE('',*,*,#38502,.F.);
#53141=ORIENTED_EDGE('',*,*,#38286,.T.);
#53142=ORIENTED_EDGE('',*,*,#38502,.T.);
#53143=ORIENTED_EDGE('',*,*,#38503,.F.);
#53144=ORIENTED_EDGE('',*,*,#38284,.T.);
#53145=ORIENTED_EDGE('',*,*,#38292,.T.);
#53146=ORIENTED_EDGE('',*,*,#38287,.T.);
#53147=ORIENTED_EDGE('',*,*,#38504,.F.);
#53148=ORIENTED_EDGE('',*,*,#38505,.F.);
#53149=ORIENTED_EDGE('',*,*,#38293,.T.);
#53150=ORIENTED_EDGE('',*,*,#38505,.T.);
#53151=ORIENTED_EDGE('',*,*,#38506,.F.);
#53152=ORIENTED_EDGE('',*,*,#38291,.T.);
#53153=ORIENTED_EDGE('',*,*,#38299,.T.);
#53154=ORIENTED_EDGE('',*,*,#38294,.T.);
#53155=ORIENTED_EDGE('',*,*,#38507,.F.);
#53156=ORIENTED_EDGE('',*,*,#38508,.F.);
#53157=ORIENTED_EDGE('',*,*,#38300,.T.);
#53158=ORIENTED_EDGE('',*,*,#38508,.T.);
#53159=ORIENTED_EDGE('',*,*,#38509,.F.);
#53160=ORIENTED_EDGE('',*,*,#38298,.T.);
#53161=ORIENTED_EDGE('',*,*,#38306,.T.);
#53162=ORIENTED_EDGE('',*,*,#38301,.T.);
#53163=ORIENTED_EDGE('',*,*,#38510,.F.);
#53164=ORIENTED_EDGE('',*,*,#38511,.F.);
#53165=ORIENTED_EDGE('',*,*,#38307,.T.);
#53166=ORIENTED_EDGE('',*,*,#38511,.T.);
#53167=ORIENTED_EDGE('',*,*,#38512,.F.);
#53168=ORIENTED_EDGE('',*,*,#38305,.T.);
#53169=ORIENTED_EDGE('',*,*,#38313,.T.);
#53170=ORIENTED_EDGE('',*,*,#38308,.T.);
#53171=ORIENTED_EDGE('',*,*,#38513,.F.);
#53172=ORIENTED_EDGE('',*,*,#38514,.F.);
#53173=ORIENTED_EDGE('',*,*,#38314,.T.);
#53174=ORIENTED_EDGE('',*,*,#38514,.T.);
#53175=ORIENTED_EDGE('',*,*,#38515,.F.);
#53176=ORIENTED_EDGE('',*,*,#38312,.T.);
#53177=ORIENTED_EDGE('',*,*,#38320,.T.);
#53178=ORIENTED_EDGE('',*,*,#38315,.T.);
#53179=ORIENTED_EDGE('',*,*,#38516,.F.);
#53180=ORIENTED_EDGE('',*,*,#38517,.F.);
#53181=ORIENTED_EDGE('',*,*,#38321,.T.);
#53182=ORIENTED_EDGE('',*,*,#38517,.T.);
#53183=ORIENTED_EDGE('',*,*,#38518,.F.);
#53184=ORIENTED_EDGE('',*,*,#38319,.T.);
#53185=ORIENTED_EDGE('',*,*,#38327,.T.);
#53186=ORIENTED_EDGE('',*,*,#38322,.T.);
#53187=ORIENTED_EDGE('',*,*,#38519,.F.);
#53188=ORIENTED_EDGE('',*,*,#38520,.F.);
#53189=ORIENTED_EDGE('',*,*,#38328,.T.);
#53190=ORIENTED_EDGE('',*,*,#38520,.T.);
#53191=ORIENTED_EDGE('',*,*,#38521,.F.);
#53192=ORIENTED_EDGE('',*,*,#38326,.T.);
#53193=ORIENTED_EDGE('',*,*,#38334,.T.);
#53194=ORIENTED_EDGE('',*,*,#38329,.T.);
#53195=ORIENTED_EDGE('',*,*,#38522,.F.);
#53196=ORIENTED_EDGE('',*,*,#38523,.F.);
#53197=ORIENTED_EDGE('',*,*,#38335,.T.);
#53198=ORIENTED_EDGE('',*,*,#38523,.T.);
#53199=ORIENTED_EDGE('',*,*,#38524,.F.);
#53200=ORIENTED_EDGE('',*,*,#38333,.T.);
#53201=ORIENTED_EDGE('',*,*,#38341,.T.);
#53202=ORIENTED_EDGE('',*,*,#38336,.T.);
#53203=ORIENTED_EDGE('',*,*,#38525,.F.);
#53204=ORIENTED_EDGE('',*,*,#38526,.F.);
#53205=ORIENTED_EDGE('',*,*,#38342,.T.);
#53206=ORIENTED_EDGE('',*,*,#38526,.T.);
#53207=ORIENTED_EDGE('',*,*,#38527,.F.);
#53208=ORIENTED_EDGE('',*,*,#38340,.T.);
#53209=ORIENTED_EDGE('',*,*,#38348,.T.);
#53210=ORIENTED_EDGE('',*,*,#38343,.T.);
#53211=ORIENTED_EDGE('',*,*,#38528,.F.);
#53212=ORIENTED_EDGE('',*,*,#38529,.F.);
#53213=ORIENTED_EDGE('',*,*,#38349,.T.);
#53214=ORIENTED_EDGE('',*,*,#38529,.T.);
#53215=ORIENTED_EDGE('',*,*,#38530,.F.);
#53216=ORIENTED_EDGE('',*,*,#38347,.T.);
#53217=ORIENTED_EDGE('',*,*,#38531,.F.);
#53218=ORIENTED_EDGE('',*,*,#38532,.F.);
#53219=ORIENTED_EDGE('',*,*,#38355,.T.);
#53220=ORIENTED_EDGE('',*,*,#38350,.T.);
#53221=ORIENTED_EDGE('',*,*,#38356,.T.);
#53222=ORIENTED_EDGE('',*,*,#38532,.T.);
#53223=ORIENTED_EDGE('',*,*,#38533,.F.);
#53224=ORIENTED_EDGE('',*,*,#38354,.T.);
#53225=ORIENTED_EDGE('',*,*,#38358,.T.);
#53226=ORIENTED_EDGE('',*,*,#38360,.T.);
#53227=ORIENTED_EDGE('',*,*,#38534,.F.);
#53228=ORIENTED_EDGE('',*,*,#38448,.T.);
#53229=ORIENTED_EDGE('',*,*,#38535,.T.);
#53230=ORIENTED_EDGE('',*,*,#38536,.F.);
#53231=ORIENTED_EDGE('',*,*,#38361,.T.);
#53232=ORIENTED_EDGE('',*,*,#38537,.F.);
#53233=ORIENTED_EDGE('',*,*,#38538,.F.);
#53234=ORIENTED_EDGE('',*,*,#38539,.F.);
#53235=ORIENTED_EDGE('',*,*,#38540,.F.);
#53236=ORIENTED_EDGE('',*,*,#38535,.F.);
#53237=ORIENTED_EDGE('',*,*,#38540,.T.);
#53238=ORIENTED_EDGE('',*,*,#38541,.F.);
#53239=ORIENTED_EDGE('',*,*,#38363,.T.);
#53240=ORIENTED_EDGE('',*,*,#38536,.T.);
#53241=ORIENTED_EDGE('',*,*,#38542,.T.);
#53242=ORIENTED_EDGE('',*,*,#38543,.F.);
#53243=ORIENTED_EDGE('',*,*,#38365,.T.);
#53244=ORIENTED_EDGE('',*,*,#38544,.F.);
#53245=ORIENTED_EDGE('',*,*,#38545,.F.);
#53246=ORIENTED_EDGE('',*,*,#38546,.F.);
#53247=ORIENTED_EDGE('',*,*,#38547,.F.);
#53248=ORIENTED_EDGE('',*,*,#38542,.F.);
#53249=ORIENTED_EDGE('',*,*,#38547,.T.);
#53250=ORIENTED_EDGE('',*,*,#38548,.F.);
#53251=ORIENTED_EDGE('',*,*,#38366,.T.);
#53252=ORIENTED_EDGE('',*,*,#38543,.T.);
#53253=ORIENTED_EDGE('',*,*,#38549,.T.);
#53254=ORIENTED_EDGE('',*,*,#38550,.F.);
#53255=ORIENTED_EDGE('',*,*,#38368,.T.);
#53256=ORIENTED_EDGE('',*,*,#38551,.F.);
#53257=ORIENTED_EDGE('',*,*,#38552,.F.);
#53258=ORIENTED_EDGE('',*,*,#38553,.F.);
#53259=ORIENTED_EDGE('',*,*,#38554,.F.);
#53260=ORIENTED_EDGE('',*,*,#38549,.F.);
#53261=ORIENTED_EDGE('',*,*,#38554,.T.);
#53262=ORIENTED_EDGE('',*,*,#38555,.F.);
#53263=ORIENTED_EDGE('',*,*,#38369,.T.);
#53264=ORIENTED_EDGE('',*,*,#38550,.T.);
#53265=ORIENTED_EDGE('',*,*,#38556,.T.);
#53266=ORIENTED_EDGE('',*,*,#38557,.F.);
#53267=ORIENTED_EDGE('',*,*,#38371,.T.);
#53268=ORIENTED_EDGE('',*,*,#38558,.F.);
#53269=ORIENTED_EDGE('',*,*,#38559,.F.);
#53270=ORIENTED_EDGE('',*,*,#38560,.F.);
#53271=ORIENTED_EDGE('',*,*,#38561,.F.);
#53272=ORIENTED_EDGE('',*,*,#38556,.F.);
#53273=ORIENTED_EDGE('',*,*,#38561,.T.);
#53274=ORIENTED_EDGE('',*,*,#38562,.F.);
#53275=ORIENTED_EDGE('',*,*,#38372,.T.);
#53276=ORIENTED_EDGE('',*,*,#38557,.T.);
#53277=ORIENTED_EDGE('',*,*,#38563,.T.);
#53278=ORIENTED_EDGE('',*,*,#38564,.F.);
#53279=ORIENTED_EDGE('',*,*,#38374,.T.);
#53280=ORIENTED_EDGE('',*,*,#38565,.F.);
#53281=ORIENTED_EDGE('',*,*,#38566,.F.);
#53282=ORIENTED_EDGE('',*,*,#38567,.F.);
#53283=ORIENTED_EDGE('',*,*,#38568,.F.);
#53284=ORIENTED_EDGE('',*,*,#38563,.F.);
#53285=ORIENTED_EDGE('',*,*,#38568,.T.);
#53286=ORIENTED_EDGE('',*,*,#38569,.F.);
#53287=ORIENTED_EDGE('',*,*,#38375,.T.);
#53288=ORIENTED_EDGE('',*,*,#38564,.T.);
#53289=ORIENTED_EDGE('',*,*,#38570,.T.);
#53290=ORIENTED_EDGE('',*,*,#38571,.F.);
#53291=ORIENTED_EDGE('',*,*,#38377,.T.);
#53292=ORIENTED_EDGE('',*,*,#38572,.F.);
#53293=ORIENTED_EDGE('',*,*,#38573,.F.);
#53294=ORIENTED_EDGE('',*,*,#38574,.F.);
#53295=ORIENTED_EDGE('',*,*,#38575,.F.);
#53296=ORIENTED_EDGE('',*,*,#38570,.F.);
#53297=ORIENTED_EDGE('',*,*,#38575,.T.);
#53298=ORIENTED_EDGE('',*,*,#38576,.F.);
#53299=ORIENTED_EDGE('',*,*,#38378,.T.);
#53300=ORIENTED_EDGE('',*,*,#38571,.T.);
#53301=ORIENTED_EDGE('',*,*,#38577,.T.);
#53302=ORIENTED_EDGE('',*,*,#38578,.F.);
#53303=ORIENTED_EDGE('',*,*,#38380,.T.);
#53304=ORIENTED_EDGE('',*,*,#38579,.F.);
#53305=ORIENTED_EDGE('',*,*,#38580,.F.);
#53306=ORIENTED_EDGE('',*,*,#38581,.F.);
#53307=ORIENTED_EDGE('',*,*,#38582,.F.);
#53308=ORIENTED_EDGE('',*,*,#38577,.F.);
#53309=ORIENTED_EDGE('',*,*,#38582,.T.);
#53310=ORIENTED_EDGE('',*,*,#38583,.F.);
#53311=ORIENTED_EDGE('',*,*,#38381,.T.);
#53312=ORIENTED_EDGE('',*,*,#38578,.T.);
#53313=ORIENTED_EDGE('',*,*,#38584,.T.);
#53314=ORIENTED_EDGE('',*,*,#38585,.F.);
#53315=ORIENTED_EDGE('',*,*,#38383,.T.);
#53316=ORIENTED_EDGE('',*,*,#38586,.F.);
#53317=ORIENTED_EDGE('',*,*,#38587,.F.);
#53318=ORIENTED_EDGE('',*,*,#38588,.F.);
#53319=ORIENTED_EDGE('',*,*,#38589,.F.);
#53320=ORIENTED_EDGE('',*,*,#38584,.F.);
#53321=ORIENTED_EDGE('',*,*,#38589,.T.);
#53322=ORIENTED_EDGE('',*,*,#38590,.F.);
#53323=ORIENTED_EDGE('',*,*,#38384,.T.);
#53324=ORIENTED_EDGE('',*,*,#38585,.T.);
#53325=ORIENTED_EDGE('',*,*,#38591,.T.);
#53326=ORIENTED_EDGE('',*,*,#38592,.F.);
#53327=ORIENTED_EDGE('',*,*,#38386,.T.);
#53328=ORIENTED_EDGE('',*,*,#38593,.F.);
#53329=ORIENTED_EDGE('',*,*,#38594,.F.);
#53330=ORIENTED_EDGE('',*,*,#38595,.F.);
#53331=ORIENTED_EDGE('',*,*,#38596,.F.);
#53332=ORIENTED_EDGE('',*,*,#38591,.F.);
#53333=ORIENTED_EDGE('',*,*,#38596,.T.);
#53334=ORIENTED_EDGE('',*,*,#38597,.F.);
#53335=ORIENTED_EDGE('',*,*,#38387,.T.);
#53336=ORIENTED_EDGE('',*,*,#38592,.T.);
#53337=ORIENTED_EDGE('',*,*,#38598,.T.);
#53338=ORIENTED_EDGE('',*,*,#38599,.F.);
#53339=ORIENTED_EDGE('',*,*,#38389,.T.);
#53340=ORIENTED_EDGE('',*,*,#38600,.F.);
#53341=ORIENTED_EDGE('',*,*,#38601,.F.);
#53342=ORIENTED_EDGE('',*,*,#38602,.F.);
#53343=ORIENTED_EDGE('',*,*,#38603,.F.);
#53344=ORIENTED_EDGE('',*,*,#38598,.F.);
#53345=ORIENTED_EDGE('',*,*,#38603,.T.);
#53346=ORIENTED_EDGE('',*,*,#38604,.F.);
#53347=ORIENTED_EDGE('',*,*,#38390,.T.);
#53348=ORIENTED_EDGE('',*,*,#38599,.T.);
#53349=ORIENTED_EDGE('',*,*,#38605,.T.);
#53350=ORIENTED_EDGE('',*,*,#38606,.F.);
#53351=ORIENTED_EDGE('',*,*,#38392,.T.);
#53352=ORIENTED_EDGE('',*,*,#38607,.F.);
#53353=ORIENTED_EDGE('',*,*,#38608,.F.);
#53354=ORIENTED_EDGE('',*,*,#38609,.F.);
#53355=ORIENTED_EDGE('',*,*,#38610,.F.);
#53356=ORIENTED_EDGE('',*,*,#38605,.F.);
#53357=ORIENTED_EDGE('',*,*,#38610,.T.);
#53358=ORIENTED_EDGE('',*,*,#38611,.F.);
#53359=ORIENTED_EDGE('',*,*,#38393,.T.);
#53360=ORIENTED_EDGE('',*,*,#38606,.T.);
#53361=ORIENTED_EDGE('',*,*,#38612,.T.);
#53362=ORIENTED_EDGE('',*,*,#38613,.F.);
#53363=ORIENTED_EDGE('',*,*,#38395,.T.);
#53364=ORIENTED_EDGE('',*,*,#38614,.F.);
#53365=ORIENTED_EDGE('',*,*,#38615,.F.);
#53366=ORIENTED_EDGE('',*,*,#38616,.F.);
#53367=ORIENTED_EDGE('',*,*,#38617,.F.);
#53368=ORIENTED_EDGE('',*,*,#38612,.F.);
#53369=ORIENTED_EDGE('',*,*,#38617,.T.);
#53370=ORIENTED_EDGE('',*,*,#38618,.F.);
#53371=ORIENTED_EDGE('',*,*,#38396,.T.);
#53372=ORIENTED_EDGE('',*,*,#38613,.T.);
#53373=ORIENTED_EDGE('',*,*,#38619,.T.);
#53374=ORIENTED_EDGE('',*,*,#38620,.F.);
#53375=ORIENTED_EDGE('',*,*,#38398,.T.);
#53376=ORIENTED_EDGE('',*,*,#38621,.F.);
#53377=ORIENTED_EDGE('',*,*,#38622,.F.);
#53378=ORIENTED_EDGE('',*,*,#38623,.F.);
#53379=ORIENTED_EDGE('',*,*,#38624,.F.);
#53380=ORIENTED_EDGE('',*,*,#38619,.F.);
#53381=ORIENTED_EDGE('',*,*,#38624,.T.);
#53382=ORIENTED_EDGE('',*,*,#38625,.F.);
#53383=ORIENTED_EDGE('',*,*,#38399,.T.);
#53384=ORIENTED_EDGE('',*,*,#38620,.T.);
#53385=ORIENTED_EDGE('',*,*,#38626,.T.);
#53386=ORIENTED_EDGE('',*,*,#38627,.F.);
#53387=ORIENTED_EDGE('',*,*,#38401,.T.);
#53388=ORIENTED_EDGE('',*,*,#38628,.F.);
#53389=ORIENTED_EDGE('',*,*,#38629,.F.);
#53390=ORIENTED_EDGE('',*,*,#38630,.F.);
#53391=ORIENTED_EDGE('',*,*,#38631,.F.);
#53392=ORIENTED_EDGE('',*,*,#38626,.F.);
#53393=ORIENTED_EDGE('',*,*,#38631,.T.);
#53394=ORIENTED_EDGE('',*,*,#38632,.F.);
#53395=ORIENTED_EDGE('',*,*,#38402,.T.);
#53396=ORIENTED_EDGE('',*,*,#38627,.T.);
#53397=ORIENTED_EDGE('',*,*,#34413,.T.);
#53398=ORIENTED_EDGE('',*,*,#38633,.F.);
#53399=ORIENTED_EDGE('',*,*,#38404,.T.);
#53400=ORIENTED_EDGE('',*,*,#38634,.F.);
#53401=ORIENTED_EDGE('',*,*,#34416,.T.);
#53402=ORIENTED_EDGE('',*,*,#38635,.F.);
#53403=ORIENTED_EDGE('',*,*,#38405,.T.);
#53404=ORIENTED_EDGE('',*,*,#38633,.T.);
#53405=ORIENTED_EDGE('',*,*,#38636,.T.);
#53406=ORIENTED_EDGE('',*,*,#38637,.F.);
#53407=ORIENTED_EDGE('',*,*,#38407,.T.);
#53408=ORIENTED_EDGE('',*,*,#38638,.F.);
#53409=ORIENTED_EDGE('',*,*,#38639,.F.);
#53410=ORIENTED_EDGE('',*,*,#38640,.F.);
#53411=ORIENTED_EDGE('',*,*,#38641,.F.);
#53412=ORIENTED_EDGE('',*,*,#38636,.F.);
#53413=ORIENTED_EDGE('',*,*,#38641,.T.);
#53414=ORIENTED_EDGE('',*,*,#38642,.F.);
#53415=ORIENTED_EDGE('',*,*,#38408,.T.);
#53416=ORIENTED_EDGE('',*,*,#38637,.T.);
#53417=ORIENTED_EDGE('',*,*,#38643,.T.);
#53418=ORIENTED_EDGE('',*,*,#38644,.F.);
#53419=ORIENTED_EDGE('',*,*,#38410,.T.);
#53420=ORIENTED_EDGE('',*,*,#38645,.F.);
#53421=ORIENTED_EDGE('',*,*,#38646,.F.);
#53422=ORIENTED_EDGE('',*,*,#38647,.F.);
#53423=ORIENTED_EDGE('',*,*,#38648,.F.);
#53424=ORIENTED_EDGE('',*,*,#38643,.F.);
#53425=ORIENTED_EDGE('',*,*,#38648,.T.);
#53426=ORIENTED_EDGE('',*,*,#38649,.F.);
#53427=ORIENTED_EDGE('',*,*,#38411,.T.);
#53428=ORIENTED_EDGE('',*,*,#38644,.T.);
#53429=ORIENTED_EDGE('',*,*,#38650,.T.);
#53430=ORIENTED_EDGE('',*,*,#38651,.F.);
#53431=ORIENTED_EDGE('',*,*,#38413,.T.);
#53432=ORIENTED_EDGE('',*,*,#38652,.F.);
#53433=ORIENTED_EDGE('',*,*,#38653,.F.);
#53434=ORIENTED_EDGE('',*,*,#38654,.F.);
#53435=ORIENTED_EDGE('',*,*,#38655,.F.);
#53436=ORIENTED_EDGE('',*,*,#38650,.F.);
#53437=ORIENTED_EDGE('',*,*,#38655,.T.);
#53438=ORIENTED_EDGE('',*,*,#38656,.F.);
#53439=ORIENTED_EDGE('',*,*,#38414,.T.);
#53440=ORIENTED_EDGE('',*,*,#38651,.T.);
#53441=ORIENTED_EDGE('',*,*,#38657,.T.);
#53442=ORIENTED_EDGE('',*,*,#38658,.F.);
#53443=ORIENTED_EDGE('',*,*,#38416,.T.);
#53444=ORIENTED_EDGE('',*,*,#38659,.F.);
#53445=ORIENTED_EDGE('',*,*,#38660,.F.);
#53446=ORIENTED_EDGE('',*,*,#38661,.F.);
#53447=ORIENTED_EDGE('',*,*,#38662,.F.);
#53448=ORIENTED_EDGE('',*,*,#38657,.F.);
#53449=ORIENTED_EDGE('',*,*,#38662,.T.);
#53450=ORIENTED_EDGE('',*,*,#38663,.F.);
#53451=ORIENTED_EDGE('',*,*,#38417,.T.);
#53452=ORIENTED_EDGE('',*,*,#38658,.T.);
#53453=ORIENTED_EDGE('',*,*,#38664,.T.);
#53454=ORIENTED_EDGE('',*,*,#38665,.F.);
#53455=ORIENTED_EDGE('',*,*,#38419,.T.);
#53456=ORIENTED_EDGE('',*,*,#38666,.F.);
#53457=ORIENTED_EDGE('',*,*,#38667,.F.);
#53458=ORIENTED_EDGE('',*,*,#38668,.F.);
#53459=ORIENTED_EDGE('',*,*,#38669,.F.);
#53460=ORIENTED_EDGE('',*,*,#38664,.F.);
#53461=ORIENTED_EDGE('',*,*,#38669,.T.);
#53462=ORIENTED_EDGE('',*,*,#38670,.F.);
#53463=ORIENTED_EDGE('',*,*,#38420,.T.);
#53464=ORIENTED_EDGE('',*,*,#38665,.T.);
#53465=ORIENTED_EDGE('',*,*,#38671,.T.);
#53466=ORIENTED_EDGE('',*,*,#38672,.F.);
#53467=ORIENTED_EDGE('',*,*,#38422,.T.);
#53468=ORIENTED_EDGE('',*,*,#38673,.F.);
#53469=ORIENTED_EDGE('',*,*,#38674,.F.);
#53470=ORIENTED_EDGE('',*,*,#38675,.F.);
#53471=ORIENTED_EDGE('',*,*,#38676,.F.);
#53472=ORIENTED_EDGE('',*,*,#38671,.F.);
#53473=ORIENTED_EDGE('',*,*,#38676,.T.);
#53474=ORIENTED_EDGE('',*,*,#38677,.F.);
#53475=ORIENTED_EDGE('',*,*,#38423,.T.);
#53476=ORIENTED_EDGE('',*,*,#38672,.T.);
#53477=ORIENTED_EDGE('',*,*,#38678,.T.);
#53478=ORIENTED_EDGE('',*,*,#38679,.F.);
#53479=ORIENTED_EDGE('',*,*,#38425,.T.);
#53480=ORIENTED_EDGE('',*,*,#38680,.F.);
#53481=ORIENTED_EDGE('',*,*,#38681,.T.);
#53482=ORIENTED_EDGE('',*,*,#38682,.F.);
#53483=ORIENTED_EDGE('',*,*,#38426,.T.);
#53484=ORIENTED_EDGE('',*,*,#38679,.T.);
#53485=ORIENTED_EDGE('',*,*,#38683,.F.);
#53486=ORIENTED_EDGE('',*,*,#38684,.F.);
#53487=ORIENTED_EDGE('',*,*,#38681,.F.);
#53488=ORIENTED_EDGE('',*,*,#38678,.F.);
#53489=ORIENTED_EDGE('',*,*,#38428,.T.);
#53490=ORIENTED_EDGE('',*,*,#38685,.F.);
#53491=ORIENTED_EDGE('',*,*,#38686,.T.);
#53492=ORIENTED_EDGE('',*,*,#38687,.F.);
#53493=ORIENTED_EDGE('',*,*,#38688,.F.);
#53494=ORIENTED_EDGE('',*,*,#38686,.F.);
#53495=ORIENTED_EDGE('',*,*,#38689,.F.);
#53496=ORIENTED_EDGE('',*,*,#38690,.F.);
#53497=ORIENTED_EDGE('',*,*,#38429,.T.);
#53498=ORIENTED_EDGE('',*,*,#38687,.T.);
#53499=ORIENTED_EDGE('',*,*,#38688,.T.);
#53500=ORIENTED_EDGE('',*,*,#38691,.F.);
#53501=ORIENTED_EDGE('',*,*,#38692,.T.);
#53502=ORIENTED_EDGE('',*,*,#38693,.F.);
#53503=ORIENTED_EDGE('',*,*,#38431,.T.);
#53504=ORIENTED_EDGE('',*,*,#38694,.F.);
#53505=ORIENTED_EDGE('',*,*,#38695,.F.);
#53506=ORIENTED_EDGE('',*,*,#38696,.F.);
#53507=ORIENTED_EDGE('',*,*,#38697,.F.);
#53508=ORIENTED_EDGE('',*,*,#38692,.F.);
#53509=ORIENTED_EDGE('',*,*,#38697,.T.);
#53510=ORIENTED_EDGE('',*,*,#38698,.F.);
#53511=ORIENTED_EDGE('',*,*,#38432,.T.);
#53512=ORIENTED_EDGE('',*,*,#38693,.T.);
#53513=ORIENTED_EDGE('',*,*,#38699,.T.);
#53514=ORIENTED_EDGE('',*,*,#38700,.F.);
#53515=ORIENTED_EDGE('',*,*,#38434,.T.);
#53516=ORIENTED_EDGE('',*,*,#38701,.F.);
#53517=ORIENTED_EDGE('',*,*,#38702,.F.);
#53518=ORIENTED_EDGE('',*,*,#38703,.F.);
#53519=ORIENTED_EDGE('',*,*,#38704,.F.);
#53520=ORIENTED_EDGE('',*,*,#38699,.F.);
#53521=ORIENTED_EDGE('',*,*,#38704,.T.);
#53522=ORIENTED_EDGE('',*,*,#38705,.F.);
#53523=ORIENTED_EDGE('',*,*,#38435,.T.);
#53524=ORIENTED_EDGE('',*,*,#38700,.T.);
#53525=ORIENTED_EDGE('',*,*,#38706,.T.);
#53526=ORIENTED_EDGE('',*,*,#38707,.F.);
#53527=ORIENTED_EDGE('',*,*,#38437,.T.);
#53528=ORIENTED_EDGE('',*,*,#38708,.F.);
#53529=ORIENTED_EDGE('',*,*,#38709,.F.);
#53530=ORIENTED_EDGE('',*,*,#38710,.F.);
#53531=ORIENTED_EDGE('',*,*,#38711,.F.);
#53532=ORIENTED_EDGE('',*,*,#38706,.F.);
#53533=ORIENTED_EDGE('',*,*,#38711,.T.);
#53534=ORIENTED_EDGE('',*,*,#38712,.F.);
#53535=ORIENTED_EDGE('',*,*,#38438,.T.);
#53536=ORIENTED_EDGE('',*,*,#38707,.T.);
#53537=ORIENTED_EDGE('',*,*,#38713,.T.);
#53538=ORIENTED_EDGE('',*,*,#38714,.F.);
#53539=ORIENTED_EDGE('',*,*,#38440,.T.);
#53540=ORIENTED_EDGE('',*,*,#38715,.F.);
#53541=ORIENTED_EDGE('',*,*,#38716,.F.);
#53542=ORIENTED_EDGE('',*,*,#38717,.F.);
#53543=ORIENTED_EDGE('',*,*,#38718,.F.);
#53544=ORIENTED_EDGE('',*,*,#38713,.F.);
#53545=ORIENTED_EDGE('',*,*,#38718,.T.);
#53546=ORIENTED_EDGE('',*,*,#38719,.F.);
#53547=ORIENTED_EDGE('',*,*,#38441,.T.);
#53548=ORIENTED_EDGE('',*,*,#38714,.T.);
#53549=ORIENTED_EDGE('',*,*,#38720,.T.);
#53550=ORIENTED_EDGE('',*,*,#38721,.F.);
#53551=ORIENTED_EDGE('',*,*,#38443,.T.);
#53552=ORIENTED_EDGE('',*,*,#38722,.F.);
#53553=ORIENTED_EDGE('',*,*,#38723,.F.);
#53554=ORIENTED_EDGE('',*,*,#38724,.F.);
#53555=ORIENTED_EDGE('',*,*,#38725,.F.);
#53556=ORIENTED_EDGE('',*,*,#38720,.F.);
#53557=ORIENTED_EDGE('',*,*,#38725,.T.);
#53558=ORIENTED_EDGE('',*,*,#38726,.F.);
#53559=ORIENTED_EDGE('',*,*,#38444,.T.);
#53560=ORIENTED_EDGE('',*,*,#38721,.T.);
#53561=ORIENTED_EDGE('',*,*,#38727,.T.);
#53562=ORIENTED_EDGE('',*,*,#38728,.F.);
#53563=ORIENTED_EDGE('',*,*,#38446,.T.);
#53564=ORIENTED_EDGE('',*,*,#38729,.F.);
#53565=ORIENTED_EDGE('',*,*,#38730,.F.);
#53566=ORIENTED_EDGE('',*,*,#38731,.F.);
#53567=ORIENTED_EDGE('',*,*,#38732,.F.);
#53568=ORIENTED_EDGE('',*,*,#38727,.F.);
#53569=ORIENTED_EDGE('',*,*,#38732,.T.);
#53570=ORIENTED_EDGE('',*,*,#38733,.F.);
#53571=ORIENTED_EDGE('',*,*,#38447,.T.);
#53572=ORIENTED_EDGE('',*,*,#38728,.T.);
#53573=ORIENTED_EDGE('',*,*,#38449,.T.);
#53574=ORIENTED_EDGE('',*,*,#38734,.F.);
#53575=ORIENTED_EDGE('',*,*,#38735,.T.);
#53576=ORIENTED_EDGE('',*,*,#38736,.F.);
#53577=ORIENTED_EDGE('',*,*,#38450,.T.);
#53578=ORIENTED_EDGE('',*,*,#38736,.T.);
#53579=ORIENTED_EDGE('',*,*,#38737,.T.);
#53580=ORIENTED_EDGE('',*,*,#38738,.F.);
#53581=ORIENTED_EDGE('',*,*,#38737,.F.);
#53582=ORIENTED_EDGE('',*,*,#38735,.F.);
#53583=ORIENTED_EDGE('',*,*,#38739,.F.);
#53584=ORIENTED_EDGE('',*,*,#38740,.F.);
#53585=ORIENTED_EDGE('',*,*,#38452,.T.);
#53586=ORIENTED_EDGE('',*,*,#38741,.F.);
#53587=ORIENTED_EDGE('',*,*,#38742,.T.);
#53588=ORIENTED_EDGE('',*,*,#38743,.F.);
#53589=ORIENTED_EDGE('',*,*,#38453,.T.);
#53590=ORIENTED_EDGE('',*,*,#38743,.T.);
#53591=ORIENTED_EDGE('',*,*,#38744,.T.);
#53592=ORIENTED_EDGE('',*,*,#38745,.F.);
#53593=ORIENTED_EDGE('',*,*,#38744,.F.);
#53594=ORIENTED_EDGE('',*,*,#38742,.F.);
#53595=ORIENTED_EDGE('',*,*,#38746,.F.);
#53596=ORIENTED_EDGE('',*,*,#38747,.F.);
#53597=ORIENTED_EDGE('',*,*,#38455,.T.);
#53598=ORIENTED_EDGE('',*,*,#38748,.F.);
#53599=ORIENTED_EDGE('',*,*,#38749,.T.);
#53600=ORIENTED_EDGE('',*,*,#38750,.F.);
#53601=ORIENTED_EDGE('',*,*,#38456,.T.);
#53602=ORIENTED_EDGE('',*,*,#38750,.T.);
#53603=ORIENTED_EDGE('',*,*,#38751,.T.);
#53604=ORIENTED_EDGE('',*,*,#38752,.F.);
#53605=ORIENTED_EDGE('',*,*,#38751,.F.);
#53606=ORIENTED_EDGE('',*,*,#38749,.F.);
#53607=ORIENTED_EDGE('',*,*,#38753,.F.);
#53608=ORIENTED_EDGE('',*,*,#38754,.F.);
#53609=ORIENTED_EDGE('',*,*,#38458,.T.);
#53610=ORIENTED_EDGE('',*,*,#38755,.F.);
#53611=ORIENTED_EDGE('',*,*,#38756,.T.);
#53612=ORIENTED_EDGE('',*,*,#38757,.F.);
#53613=ORIENTED_EDGE('',*,*,#38459,.T.);
#53614=ORIENTED_EDGE('',*,*,#38757,.T.);
#53615=ORIENTED_EDGE('',*,*,#38758,.T.);
#53616=ORIENTED_EDGE('',*,*,#38759,.F.);
#53617=ORIENTED_EDGE('',*,*,#38758,.F.);
#53618=ORIENTED_EDGE('',*,*,#38756,.F.);
#53619=ORIENTED_EDGE('',*,*,#38760,.F.);
#53620=ORIENTED_EDGE('',*,*,#38761,.F.);
#53621=ORIENTED_EDGE('',*,*,#38461,.T.);
#53622=ORIENTED_EDGE('',*,*,#38762,.F.);
#53623=ORIENTED_EDGE('',*,*,#38763,.T.);
#53624=ORIENTED_EDGE('',*,*,#38764,.F.);
#53625=ORIENTED_EDGE('',*,*,#38462,.T.);
#53626=ORIENTED_EDGE('',*,*,#38764,.T.);
#53627=ORIENTED_EDGE('',*,*,#38765,.T.);
#53628=ORIENTED_EDGE('',*,*,#38766,.F.);
#53629=ORIENTED_EDGE('',*,*,#38765,.F.);
#53630=ORIENTED_EDGE('',*,*,#38763,.F.);
#53631=ORIENTED_EDGE('',*,*,#38767,.F.);
#53632=ORIENTED_EDGE('',*,*,#38768,.F.);
#53633=ORIENTED_EDGE('',*,*,#38464,.T.);
#53634=ORIENTED_EDGE('',*,*,#38769,.F.);
#53635=ORIENTED_EDGE('',*,*,#38770,.T.);
#53636=ORIENTED_EDGE('',*,*,#38771,.F.);
#53637=ORIENTED_EDGE('',*,*,#38465,.T.);
#53638=ORIENTED_EDGE('',*,*,#38771,.T.);
#53639=ORIENTED_EDGE('',*,*,#38772,.T.);
#53640=ORIENTED_EDGE('',*,*,#38773,.F.);
#53641=ORIENTED_EDGE('',*,*,#38772,.F.);
#53642=ORIENTED_EDGE('',*,*,#38770,.F.);
#53643=ORIENTED_EDGE('',*,*,#38774,.F.);
#53644=ORIENTED_EDGE('',*,*,#38775,.F.);
#53645=ORIENTED_EDGE('',*,*,#38467,.T.);
#53646=ORIENTED_EDGE('',*,*,#38776,.F.);
#53647=ORIENTED_EDGE('',*,*,#38777,.T.);
#53648=ORIENTED_EDGE('',*,*,#38778,.F.);
#53649=ORIENTED_EDGE('',*,*,#38468,.T.);
#53650=ORIENTED_EDGE('',*,*,#38778,.T.);
#53651=ORIENTED_EDGE('',*,*,#38779,.T.);
#53652=ORIENTED_EDGE('',*,*,#38780,.F.);
#53653=ORIENTED_EDGE('',*,*,#38779,.F.);
#53654=ORIENTED_EDGE('',*,*,#38777,.F.);
#53655=ORIENTED_EDGE('',*,*,#38781,.F.);
#53656=ORIENTED_EDGE('',*,*,#38782,.F.);
#53657=ORIENTED_EDGE('',*,*,#38470,.T.);
#53658=ORIENTED_EDGE('',*,*,#38783,.F.);
#53659=ORIENTED_EDGE('',*,*,#38784,.T.);
#53660=ORIENTED_EDGE('',*,*,#38785,.F.);
#53661=ORIENTED_EDGE('',*,*,#38471,.T.);
#53662=ORIENTED_EDGE('',*,*,#38785,.T.);
#53663=ORIENTED_EDGE('',*,*,#38786,.T.);
#53664=ORIENTED_EDGE('',*,*,#38787,.F.);
#53665=ORIENTED_EDGE('',*,*,#38786,.F.);
#53666=ORIENTED_EDGE('',*,*,#38784,.F.);
#53667=ORIENTED_EDGE('',*,*,#38788,.F.);
#53668=ORIENTED_EDGE('',*,*,#38789,.F.);
#53669=ORIENTED_EDGE('',*,*,#38473,.T.);
#53670=ORIENTED_EDGE('',*,*,#38790,.F.);
#53671=ORIENTED_EDGE('',*,*,#38791,.T.);
#53672=ORIENTED_EDGE('',*,*,#38792,.F.);
#53673=ORIENTED_EDGE('',*,*,#38474,.T.);
#53674=ORIENTED_EDGE('',*,*,#38792,.T.);
#53675=ORIENTED_EDGE('',*,*,#38793,.T.);
#53676=ORIENTED_EDGE('',*,*,#38794,.F.);
#53677=ORIENTED_EDGE('',*,*,#38793,.F.);
#53678=ORIENTED_EDGE('',*,*,#38791,.F.);
#53679=ORIENTED_EDGE('',*,*,#38795,.F.);
#53680=ORIENTED_EDGE('',*,*,#38796,.F.);
#53681=ORIENTED_EDGE('',*,*,#38476,.T.);
#53682=ORIENTED_EDGE('',*,*,#38797,.F.);
#53683=ORIENTED_EDGE('',*,*,#38798,.T.);
#53684=ORIENTED_EDGE('',*,*,#38799,.F.);
#53685=ORIENTED_EDGE('',*,*,#38477,.T.);
#53686=ORIENTED_EDGE('',*,*,#38799,.T.);
#53687=ORIENTED_EDGE('',*,*,#38800,.T.);
#53688=ORIENTED_EDGE('',*,*,#38801,.F.);
#53689=ORIENTED_EDGE('',*,*,#38800,.F.);
#53690=ORIENTED_EDGE('',*,*,#38798,.F.);
#53691=ORIENTED_EDGE('',*,*,#38802,.F.);
#53692=ORIENTED_EDGE('',*,*,#38803,.F.);
#53693=ORIENTED_EDGE('',*,*,#38479,.T.);
#53694=ORIENTED_EDGE('',*,*,#38804,.F.);
#53695=ORIENTED_EDGE('',*,*,#38805,.T.);
#53696=ORIENTED_EDGE('',*,*,#38806,.F.);
#53697=ORIENTED_EDGE('',*,*,#38480,.T.);
#53698=ORIENTED_EDGE('',*,*,#38806,.T.);
#53699=ORIENTED_EDGE('',*,*,#38807,.T.);
#53700=ORIENTED_EDGE('',*,*,#38808,.F.);
#53701=ORIENTED_EDGE('',*,*,#38807,.F.);
#53702=ORIENTED_EDGE('',*,*,#38805,.F.);
#53703=ORIENTED_EDGE('',*,*,#38809,.F.);
#53704=ORIENTED_EDGE('',*,*,#38810,.F.);
#53705=ORIENTED_EDGE('',*,*,#38482,.T.);
#53706=ORIENTED_EDGE('',*,*,#38811,.F.);
#53707=ORIENTED_EDGE('',*,*,#38812,.T.);
#53708=ORIENTED_EDGE('',*,*,#38813,.F.);
#53709=ORIENTED_EDGE('',*,*,#38483,.T.);
#53710=ORIENTED_EDGE('',*,*,#38813,.T.);
#53711=ORIENTED_EDGE('',*,*,#38814,.T.);
#53712=ORIENTED_EDGE('',*,*,#38815,.F.);
#53713=ORIENTED_EDGE('',*,*,#38814,.F.);
#53714=ORIENTED_EDGE('',*,*,#38812,.F.);
#53715=ORIENTED_EDGE('',*,*,#38816,.F.);
#53716=ORIENTED_EDGE('',*,*,#38817,.F.);
#53717=ORIENTED_EDGE('',*,*,#38485,.T.);
#53718=ORIENTED_EDGE('',*,*,#38818,.F.);
#53719=ORIENTED_EDGE('',*,*,#38819,.T.);
#53720=ORIENTED_EDGE('',*,*,#38820,.F.);
#53721=ORIENTED_EDGE('',*,*,#38486,.T.);
#53722=ORIENTED_EDGE('',*,*,#38820,.T.);
#53723=ORIENTED_EDGE('',*,*,#38821,.T.);
#53724=ORIENTED_EDGE('',*,*,#38822,.F.);
#53725=ORIENTED_EDGE('',*,*,#38821,.F.);
#53726=ORIENTED_EDGE('',*,*,#38819,.F.);
#53727=ORIENTED_EDGE('',*,*,#38823,.F.);
#53728=ORIENTED_EDGE('',*,*,#38824,.F.);
#53729=ORIENTED_EDGE('',*,*,#38488,.T.);
#53730=ORIENTED_EDGE('',*,*,#38825,.F.);
#53731=ORIENTED_EDGE('',*,*,#38826,.T.);
#53732=ORIENTED_EDGE('',*,*,#38827,.F.);
#53733=ORIENTED_EDGE('',*,*,#38489,.T.);
#53734=ORIENTED_EDGE('',*,*,#38827,.T.);
#53735=ORIENTED_EDGE('',*,*,#38828,.T.);
#53736=ORIENTED_EDGE('',*,*,#38829,.F.);
#53737=ORIENTED_EDGE('',*,*,#38828,.F.);
#53738=ORIENTED_EDGE('',*,*,#38826,.F.);
#53739=ORIENTED_EDGE('',*,*,#38830,.F.);
#53740=ORIENTED_EDGE('',*,*,#38831,.F.);
#53741=ORIENTED_EDGE('',*,*,#38491,.T.);
#53742=ORIENTED_EDGE('',*,*,#38832,.F.);
#53743=ORIENTED_EDGE('',*,*,#38833,.T.);
#53744=ORIENTED_EDGE('',*,*,#38834,.F.);
#53745=ORIENTED_EDGE('',*,*,#38492,.T.);
#53746=ORIENTED_EDGE('',*,*,#38834,.T.);
#53747=ORIENTED_EDGE('',*,*,#38835,.T.);
#53748=ORIENTED_EDGE('',*,*,#38836,.F.);
#53749=ORIENTED_EDGE('',*,*,#38835,.F.);
#53750=ORIENTED_EDGE('',*,*,#38833,.F.);
#53751=ORIENTED_EDGE('',*,*,#38837,.F.);
#53752=ORIENTED_EDGE('',*,*,#38838,.F.);
#53753=ORIENTED_EDGE('',*,*,#38494,.T.);
#53754=ORIENTED_EDGE('',*,*,#38839,.F.);
#53755=ORIENTED_EDGE('',*,*,#38840,.T.);
#53756=ORIENTED_EDGE('',*,*,#38841,.F.);
#53757=ORIENTED_EDGE('',*,*,#38495,.T.);
#53758=ORIENTED_EDGE('',*,*,#38841,.T.);
#53759=ORIENTED_EDGE('',*,*,#38842,.T.);
#53760=ORIENTED_EDGE('',*,*,#38843,.F.);
#53761=ORIENTED_EDGE('',*,*,#38842,.F.);
#53762=ORIENTED_EDGE('',*,*,#38840,.F.);
#53763=ORIENTED_EDGE('',*,*,#38844,.F.);
#53764=ORIENTED_EDGE('',*,*,#38845,.F.);
#53765=ORIENTED_EDGE('',*,*,#38497,.T.);
#53766=ORIENTED_EDGE('',*,*,#38846,.F.);
#53767=ORIENTED_EDGE('',*,*,#38847,.T.);
#53768=ORIENTED_EDGE('',*,*,#38848,.F.);
#53769=ORIENTED_EDGE('',*,*,#38498,.T.);
#53770=ORIENTED_EDGE('',*,*,#38848,.T.);
#53771=ORIENTED_EDGE('',*,*,#38849,.T.);
#53772=ORIENTED_EDGE('',*,*,#38850,.F.);
#53773=ORIENTED_EDGE('',*,*,#38849,.F.);
#53774=ORIENTED_EDGE('',*,*,#38847,.F.);
#53775=ORIENTED_EDGE('',*,*,#38851,.F.);
#53776=ORIENTED_EDGE('',*,*,#38852,.F.);
#53777=ORIENTED_EDGE('',*,*,#38500,.T.);
#53778=ORIENTED_EDGE('',*,*,#38853,.F.);
#53779=ORIENTED_EDGE('',*,*,#38854,.T.);
#53780=ORIENTED_EDGE('',*,*,#38855,.F.);
#53781=ORIENTED_EDGE('',*,*,#38501,.T.);
#53782=ORIENTED_EDGE('',*,*,#38855,.T.);
#53783=ORIENTED_EDGE('',*,*,#38856,.T.);
#53784=ORIENTED_EDGE('',*,*,#38857,.F.);
#53785=ORIENTED_EDGE('',*,*,#38856,.F.);
#53786=ORIENTED_EDGE('',*,*,#38854,.F.);
#53787=ORIENTED_EDGE('',*,*,#38858,.F.);
#53788=ORIENTED_EDGE('',*,*,#38859,.F.);
#53789=ORIENTED_EDGE('',*,*,#38503,.T.);
#53790=ORIENTED_EDGE('',*,*,#38860,.F.);
#53791=ORIENTED_EDGE('',*,*,#38861,.T.);
#53792=ORIENTED_EDGE('',*,*,#38862,.F.);
#53793=ORIENTED_EDGE('',*,*,#38504,.T.);
#53794=ORIENTED_EDGE('',*,*,#38862,.T.);
#53795=ORIENTED_EDGE('',*,*,#38863,.T.);
#53796=ORIENTED_EDGE('',*,*,#38864,.F.);
#53797=ORIENTED_EDGE('',*,*,#38863,.F.);
#53798=ORIENTED_EDGE('',*,*,#38861,.F.);
#53799=ORIENTED_EDGE('',*,*,#38865,.F.);
#53800=ORIENTED_EDGE('',*,*,#38866,.F.);
#53801=ORIENTED_EDGE('',*,*,#38506,.T.);
#53802=ORIENTED_EDGE('',*,*,#38867,.F.);
#53803=ORIENTED_EDGE('',*,*,#38868,.T.);
#53804=ORIENTED_EDGE('',*,*,#38869,.F.);
#53805=ORIENTED_EDGE('',*,*,#38507,.T.);
#53806=ORIENTED_EDGE('',*,*,#38869,.T.);
#53807=ORIENTED_EDGE('',*,*,#38870,.T.);
#53808=ORIENTED_EDGE('',*,*,#38871,.F.);
#53809=ORIENTED_EDGE('',*,*,#38870,.F.);
#53810=ORIENTED_EDGE('',*,*,#38868,.F.);
#53811=ORIENTED_EDGE('',*,*,#38872,.F.);
#53812=ORIENTED_EDGE('',*,*,#38873,.F.);
#53813=ORIENTED_EDGE('',*,*,#38509,.T.);
#53814=ORIENTED_EDGE('',*,*,#38874,.F.);
#53815=ORIENTED_EDGE('',*,*,#38875,.T.);
#53816=ORIENTED_EDGE('',*,*,#38876,.F.);
#53817=ORIENTED_EDGE('',*,*,#38510,.T.);
#53818=ORIENTED_EDGE('',*,*,#38876,.T.);
#53819=ORIENTED_EDGE('',*,*,#38877,.T.);
#53820=ORIENTED_EDGE('',*,*,#38878,.F.);
#53821=ORIENTED_EDGE('',*,*,#38877,.F.);
#53822=ORIENTED_EDGE('',*,*,#38875,.F.);
#53823=ORIENTED_EDGE('',*,*,#38879,.F.);
#53824=ORIENTED_EDGE('',*,*,#38880,.F.);
#53825=ORIENTED_EDGE('',*,*,#38512,.T.);
#53826=ORIENTED_EDGE('',*,*,#38881,.F.);
#53827=ORIENTED_EDGE('',*,*,#34412,.T.);
#53828=ORIENTED_EDGE('',*,*,#38882,.F.);
#53829=ORIENTED_EDGE('',*,*,#38513,.T.);
#53830=ORIENTED_EDGE('',*,*,#38882,.T.);
#53831=ORIENTED_EDGE('',*,*,#34411,.T.);
#53832=ORIENTED_EDGE('',*,*,#38883,.F.);
#53833=ORIENTED_EDGE('',*,*,#38515,.T.);
#53834=ORIENTED_EDGE('',*,*,#38884,.F.);
#53835=ORIENTED_EDGE('',*,*,#38885,.T.);
#53836=ORIENTED_EDGE('',*,*,#38886,.F.);
#53837=ORIENTED_EDGE('',*,*,#38516,.T.);
#53838=ORIENTED_EDGE('',*,*,#38886,.T.);
#53839=ORIENTED_EDGE('',*,*,#38887,.T.);
#53840=ORIENTED_EDGE('',*,*,#38888,.F.);
#53841=ORIENTED_EDGE('',*,*,#38887,.F.);
#53842=ORIENTED_EDGE('',*,*,#38885,.F.);
#53843=ORIENTED_EDGE('',*,*,#38889,.F.);
#53844=ORIENTED_EDGE('',*,*,#38890,.F.);
#53845=ORIENTED_EDGE('',*,*,#38518,.T.);
#53846=ORIENTED_EDGE('',*,*,#38891,.F.);
#53847=ORIENTED_EDGE('',*,*,#38892,.T.);
#53848=ORIENTED_EDGE('',*,*,#38893,.F.);
#53849=ORIENTED_EDGE('',*,*,#38519,.T.);
#53850=ORIENTED_EDGE('',*,*,#38893,.T.);
#53851=ORIENTED_EDGE('',*,*,#38894,.T.);
#53852=ORIENTED_EDGE('',*,*,#38895,.F.);
#53853=ORIENTED_EDGE('',*,*,#38894,.F.);
#53854=ORIENTED_EDGE('',*,*,#38892,.F.);
#53855=ORIENTED_EDGE('',*,*,#38896,.F.);
#53856=ORIENTED_EDGE('',*,*,#38897,.F.);
#53857=ORIENTED_EDGE('',*,*,#38521,.T.);
#53858=ORIENTED_EDGE('',*,*,#38898,.F.);
#53859=ORIENTED_EDGE('',*,*,#38899,.T.);
#53860=ORIENTED_EDGE('',*,*,#38900,.F.);
#53861=ORIENTED_EDGE('',*,*,#38522,.T.);
#53862=ORIENTED_EDGE('',*,*,#38900,.T.);
#53863=ORIENTED_EDGE('',*,*,#38901,.T.);
#53864=ORIENTED_EDGE('',*,*,#38902,.F.);
#53865=ORIENTED_EDGE('',*,*,#38901,.F.);
#53866=ORIENTED_EDGE('',*,*,#38899,.F.);
#53867=ORIENTED_EDGE('',*,*,#38903,.F.);
#53868=ORIENTED_EDGE('',*,*,#38904,.F.);
#53869=ORIENTED_EDGE('',*,*,#38524,.T.);
#53870=ORIENTED_EDGE('',*,*,#38905,.F.);
#53871=ORIENTED_EDGE('',*,*,#38906,.T.);
#53872=ORIENTED_EDGE('',*,*,#38907,.F.);
#53873=ORIENTED_EDGE('',*,*,#38525,.T.);
#53874=ORIENTED_EDGE('',*,*,#38907,.T.);
#53875=ORIENTED_EDGE('',*,*,#38908,.T.);
#53876=ORIENTED_EDGE('',*,*,#38909,.F.);
#53877=ORIENTED_EDGE('',*,*,#38908,.F.);
#53878=ORIENTED_EDGE('',*,*,#38906,.F.);
#53879=ORIENTED_EDGE('',*,*,#38910,.F.);
#53880=ORIENTED_EDGE('',*,*,#38911,.F.);
#53881=ORIENTED_EDGE('',*,*,#38527,.T.);
#53882=ORIENTED_EDGE('',*,*,#38912,.F.);
#53883=ORIENTED_EDGE('',*,*,#38913,.T.);
#53884=ORIENTED_EDGE('',*,*,#38914,.F.);
#53885=ORIENTED_EDGE('',*,*,#38528,.T.);
#53886=ORIENTED_EDGE('',*,*,#38914,.T.);
#53887=ORIENTED_EDGE('',*,*,#38915,.T.);
#53888=ORIENTED_EDGE('',*,*,#38916,.F.);
#53889=ORIENTED_EDGE('',*,*,#38915,.F.);
#53890=ORIENTED_EDGE('',*,*,#38913,.F.);
#53891=ORIENTED_EDGE('',*,*,#38917,.F.);
#53892=ORIENTED_EDGE('',*,*,#38918,.F.);
#53893=ORIENTED_EDGE('',*,*,#38530,.T.);
#53894=ORIENTED_EDGE('',*,*,#38919,.F.);
#53895=ORIENTED_EDGE('',*,*,#38920,.T.);
#53896=ORIENTED_EDGE('',*,*,#38921,.F.);
#53897=ORIENTED_EDGE('',*,*,#38922,.T.);
#53898=ORIENTED_EDGE('',*,*,#38923,.F.);
#53899=ORIENTED_EDGE('',*,*,#38531,.T.);
#53900=ORIENTED_EDGE('',*,*,#38921,.T.);
#53901=ORIENTED_EDGE('',*,*,#38924,.F.);
#53902=ORIENTED_EDGE('',*,*,#38925,.F.);
#53903=ORIENTED_EDGE('',*,*,#38922,.F.);
#53904=ORIENTED_EDGE('',*,*,#38920,.F.);
#53905=ORIENTED_EDGE('',*,*,#38533,.T.);
#53906=ORIENTED_EDGE('',*,*,#38926,.F.);
#53907=ORIENTED_EDGE('',*,*,#38927,.T.);
#53908=ORIENTED_EDGE('',*,*,#38928,.F.);
#53909=ORIENTED_EDGE('',*,*,#38534,.T.);
#53910=ORIENTED_EDGE('',*,*,#38928,.T.);
#53911=ORIENTED_EDGE('',*,*,#38929,.T.);
#53912=ORIENTED_EDGE('',*,*,#38930,.F.);
#53913=ORIENTED_EDGE('',*,*,#38929,.F.);
#53914=ORIENTED_EDGE('',*,*,#38927,.F.);
#53915=ORIENTED_EDGE('',*,*,#38931,.F.);
#53916=ORIENTED_EDGE('',*,*,#38932,.F.);
#53917=ORIENTED_EDGE('',*,*,#38933,.F.);
#53918=ORIENTED_EDGE('',*,*,#38934,.F.);
#53919=ORIENTED_EDGE('',*,*,#38538,.T.);
#53920=ORIENTED_EDGE('',*,*,#38537,.T.);
#53921=ORIENTED_EDGE('',*,*,#38935,.F.);
#53922=ORIENTED_EDGE('',*,*,#38541,.T.);
#53923=ORIENTED_EDGE('',*,*,#38539,.T.);
#53924=ORIENTED_EDGE('',*,*,#38934,.T.);
#53925=ORIENTED_EDGE('',*,*,#38936,.F.);
#53926=ORIENTED_EDGE('',*,*,#38937,.F.);
#53927=ORIENTED_EDGE('',*,*,#38545,.T.);
#53928=ORIENTED_EDGE('',*,*,#38544,.T.);
#53929=ORIENTED_EDGE('',*,*,#38938,.F.);
#53930=ORIENTED_EDGE('',*,*,#38548,.T.);
#53931=ORIENTED_EDGE('',*,*,#38546,.T.);
#53932=ORIENTED_EDGE('',*,*,#38937,.T.);
#53933=ORIENTED_EDGE('',*,*,#38939,.F.);
#53934=ORIENTED_EDGE('',*,*,#38940,.F.);
#53935=ORIENTED_EDGE('',*,*,#38552,.T.);
#53936=ORIENTED_EDGE('',*,*,#38551,.T.);
#53937=ORIENTED_EDGE('',*,*,#38941,.F.);
#53938=ORIENTED_EDGE('',*,*,#38555,.T.);
#53939=ORIENTED_EDGE('',*,*,#38553,.T.);
#53940=ORIENTED_EDGE('',*,*,#38940,.T.);
#53941=ORIENTED_EDGE('',*,*,#38942,.F.);
#53942=ORIENTED_EDGE('',*,*,#38943,.F.);
#53943=ORIENTED_EDGE('',*,*,#38559,.T.);
#53944=ORIENTED_EDGE('',*,*,#38558,.T.);
#53945=ORIENTED_EDGE('',*,*,#38944,.F.);
#53946=ORIENTED_EDGE('',*,*,#38562,.T.);
#53947=ORIENTED_EDGE('',*,*,#38560,.T.);
#53948=ORIENTED_EDGE('',*,*,#38943,.T.);
#53949=ORIENTED_EDGE('',*,*,#38945,.F.);
#53950=ORIENTED_EDGE('',*,*,#38946,.F.);
#53951=ORIENTED_EDGE('',*,*,#38566,.T.);
#53952=ORIENTED_EDGE('',*,*,#38565,.T.);
#53953=ORIENTED_EDGE('',*,*,#38947,.F.);
#53954=ORIENTED_EDGE('',*,*,#38569,.T.);
#53955=ORIENTED_EDGE('',*,*,#38567,.T.);
#53956=ORIENTED_EDGE('',*,*,#38946,.T.);
#53957=ORIENTED_EDGE('',*,*,#38948,.F.);
#53958=ORIENTED_EDGE('',*,*,#38949,.F.);
#53959=ORIENTED_EDGE('',*,*,#38573,.T.);
#53960=ORIENTED_EDGE('',*,*,#38572,.T.);
#53961=ORIENTED_EDGE('',*,*,#38950,.F.);
#53962=ORIENTED_EDGE('',*,*,#38576,.T.);
#53963=ORIENTED_EDGE('',*,*,#38574,.T.);
#53964=ORIENTED_EDGE('',*,*,#38949,.T.);
#53965=ORIENTED_EDGE('',*,*,#38951,.F.);
#53966=ORIENTED_EDGE('',*,*,#38952,.F.);
#53967=ORIENTED_EDGE('',*,*,#38580,.T.);
#53968=ORIENTED_EDGE('',*,*,#38579,.T.);
#53969=ORIENTED_EDGE('',*,*,#38953,.F.);
#53970=ORIENTED_EDGE('',*,*,#38583,.T.);
#53971=ORIENTED_EDGE('',*,*,#38581,.T.);
#53972=ORIENTED_EDGE('',*,*,#38952,.T.);
#53973=ORIENTED_EDGE('',*,*,#38954,.F.);
#53974=ORIENTED_EDGE('',*,*,#38955,.F.);
#53975=ORIENTED_EDGE('',*,*,#38587,.T.);
#53976=ORIENTED_EDGE('',*,*,#38586,.T.);
#53977=ORIENTED_EDGE('',*,*,#38956,.F.);
#53978=ORIENTED_EDGE('',*,*,#38590,.T.);
#53979=ORIENTED_EDGE('',*,*,#38588,.T.);
#53980=ORIENTED_EDGE('',*,*,#38955,.T.);
#53981=ORIENTED_EDGE('',*,*,#38957,.F.);
#53982=ORIENTED_EDGE('',*,*,#38958,.F.);
#53983=ORIENTED_EDGE('',*,*,#38594,.T.);
#53984=ORIENTED_EDGE('',*,*,#38593,.T.);
#53985=ORIENTED_EDGE('',*,*,#38959,.F.);
#53986=ORIENTED_EDGE('',*,*,#38597,.T.);
#53987=ORIENTED_EDGE('',*,*,#38595,.T.);
#53988=ORIENTED_EDGE('',*,*,#38958,.T.);
#53989=ORIENTED_EDGE('',*,*,#38960,.F.);
#53990=ORIENTED_EDGE('',*,*,#38961,.F.);
#53991=ORIENTED_EDGE('',*,*,#38601,.T.);
#53992=ORIENTED_EDGE('',*,*,#38600,.T.);
#53993=ORIENTED_EDGE('',*,*,#38962,.F.);
#53994=ORIENTED_EDGE('',*,*,#38604,.T.);
#53995=ORIENTED_EDGE('',*,*,#38602,.T.);
#53996=ORIENTED_EDGE('',*,*,#38961,.T.);
#53997=ORIENTED_EDGE('',*,*,#38963,.F.);
#53998=ORIENTED_EDGE('',*,*,#38964,.F.);
#53999=ORIENTED_EDGE('',*,*,#38608,.T.);
#54000=ORIENTED_EDGE('',*,*,#38607,.T.);
#54001=ORIENTED_EDGE('',*,*,#38965,.F.);
#54002=ORIENTED_EDGE('',*,*,#38611,.T.);
#54003=ORIENTED_EDGE('',*,*,#38609,.T.);
#54004=ORIENTED_EDGE('',*,*,#38964,.T.);
#54005=ORIENTED_EDGE('',*,*,#38966,.F.);
#54006=ORIENTED_EDGE('',*,*,#38967,.F.);
#54007=ORIENTED_EDGE('',*,*,#38615,.T.);
#54008=ORIENTED_EDGE('',*,*,#38614,.T.);
#54009=ORIENTED_EDGE('',*,*,#38968,.F.);
#54010=ORIENTED_EDGE('',*,*,#38618,.T.);
#54011=ORIENTED_EDGE('',*,*,#38616,.T.);
#54012=ORIENTED_EDGE('',*,*,#38967,.T.);
#54013=ORIENTED_EDGE('',*,*,#38969,.F.);
#54014=ORIENTED_EDGE('',*,*,#38970,.F.);
#54015=ORIENTED_EDGE('',*,*,#38622,.T.);
#54016=ORIENTED_EDGE('',*,*,#38621,.T.);
#54017=ORIENTED_EDGE('',*,*,#38971,.F.);
#54018=ORIENTED_EDGE('',*,*,#38625,.T.);
#54019=ORIENTED_EDGE('',*,*,#38623,.T.);
#54020=ORIENTED_EDGE('',*,*,#38970,.T.);
#54021=ORIENTED_EDGE('',*,*,#38972,.F.);
#54022=ORIENTED_EDGE('',*,*,#38973,.F.);
#54023=ORIENTED_EDGE('',*,*,#38629,.T.);
#54024=ORIENTED_EDGE('',*,*,#38628,.T.);
#54025=ORIENTED_EDGE('',*,*,#38974,.F.);
#54026=ORIENTED_EDGE('',*,*,#38632,.T.);
#54027=ORIENTED_EDGE('',*,*,#38630,.T.);
#54028=ORIENTED_EDGE('',*,*,#38973,.T.);
#54029=ORIENTED_EDGE('',*,*,#38975,.F.);
#54030=ORIENTED_EDGE('',*,*,#38976,.F.);
#54031=ORIENTED_EDGE('',*,*,#34414,.T.);
#54032=ORIENTED_EDGE('',*,*,#38634,.T.);
#54033=ORIENTED_EDGE('',*,*,#38977,.F.);
#54034=ORIENTED_EDGE('',*,*,#38635,.T.);
#54035=ORIENTED_EDGE('',*,*,#34415,.T.);
#54036=ORIENTED_EDGE('',*,*,#38976,.T.);
#54037=ORIENTED_EDGE('',*,*,#38978,.F.);
#54038=ORIENTED_EDGE('',*,*,#38979,.F.);
#54039=ORIENTED_EDGE('',*,*,#38639,.T.);
#54040=ORIENTED_EDGE('',*,*,#38638,.T.);
#54041=ORIENTED_EDGE('',*,*,#38980,.F.);
#54042=ORIENTED_EDGE('',*,*,#38642,.T.);
#54043=ORIENTED_EDGE('',*,*,#38640,.T.);
#54044=ORIENTED_EDGE('',*,*,#38979,.T.);
#54045=ORIENTED_EDGE('',*,*,#38981,.F.);
#54046=ORIENTED_EDGE('',*,*,#38982,.F.);
#54047=ORIENTED_EDGE('',*,*,#38646,.T.);
#54048=ORIENTED_EDGE('',*,*,#38645,.T.);
#54049=ORIENTED_EDGE('',*,*,#38983,.F.);
#54050=ORIENTED_EDGE('',*,*,#38649,.T.);
#54051=ORIENTED_EDGE('',*,*,#38647,.T.);
#54052=ORIENTED_EDGE('',*,*,#38982,.T.);
#54053=ORIENTED_EDGE('',*,*,#38984,.F.);
#54054=ORIENTED_EDGE('',*,*,#38985,.F.);
#54055=ORIENTED_EDGE('',*,*,#38653,.T.);
#54056=ORIENTED_EDGE('',*,*,#38652,.T.);
#54057=ORIENTED_EDGE('',*,*,#38986,.F.);
#54058=ORIENTED_EDGE('',*,*,#38656,.T.);
#54059=ORIENTED_EDGE('',*,*,#38654,.T.);
#54060=ORIENTED_EDGE('',*,*,#38985,.T.);
#54061=ORIENTED_EDGE('',*,*,#38987,.F.);
#54062=ORIENTED_EDGE('',*,*,#38988,.F.);
#54063=ORIENTED_EDGE('',*,*,#38660,.T.);
#54064=ORIENTED_EDGE('',*,*,#38659,.T.);
#54065=ORIENTED_EDGE('',*,*,#38989,.F.);
#54066=ORIENTED_EDGE('',*,*,#38663,.T.);
#54067=ORIENTED_EDGE('',*,*,#38661,.T.);
#54068=ORIENTED_EDGE('',*,*,#38988,.T.);
#54069=ORIENTED_EDGE('',*,*,#38990,.F.);
#54070=ORIENTED_EDGE('',*,*,#38991,.F.);
#54071=ORIENTED_EDGE('',*,*,#38667,.T.);
#54072=ORIENTED_EDGE('',*,*,#38666,.T.);
#54073=ORIENTED_EDGE('',*,*,#38992,.F.);
#54074=ORIENTED_EDGE('',*,*,#38670,.T.);
#54075=ORIENTED_EDGE('',*,*,#38668,.T.);
#54076=ORIENTED_EDGE('',*,*,#38991,.T.);
#54077=ORIENTED_EDGE('',*,*,#38993,.F.);
#54078=ORIENTED_EDGE('',*,*,#38994,.F.);
#54079=ORIENTED_EDGE('',*,*,#38674,.T.);
#54080=ORIENTED_EDGE('',*,*,#38673,.T.);
#54081=ORIENTED_EDGE('',*,*,#38995,.F.);
#54082=ORIENTED_EDGE('',*,*,#38677,.T.);
#54083=ORIENTED_EDGE('',*,*,#38675,.T.);
#54084=ORIENTED_EDGE('',*,*,#38994,.T.);
#54085=ORIENTED_EDGE('',*,*,#38996,.F.);
#54086=ORIENTED_EDGE('',*,*,#38997,.F.);
#54087=ORIENTED_EDGE('',*,*,#38683,.T.);
#54088=ORIENTED_EDGE('',*,*,#38680,.T.);
#54089=ORIENTED_EDGE('',*,*,#38684,.T.);
#54090=ORIENTED_EDGE('',*,*,#38997,.T.);
#54091=ORIENTED_EDGE('',*,*,#38998,.F.);
#54092=ORIENTED_EDGE('',*,*,#38682,.T.);
#54093=ORIENTED_EDGE('',*,*,#38689,.T.);
#54094=ORIENTED_EDGE('',*,*,#38685,.T.);
#54095=ORIENTED_EDGE('',*,*,#38999,.F.);
#54096=ORIENTED_EDGE('',*,*,#39000,.F.);
#54097=ORIENTED_EDGE('',*,*,#39001,.F.);
#54098=ORIENTED_EDGE('',*,*,#38691,.T.);
#54099=ORIENTED_EDGE('',*,*,#38690,.T.);
#54100=ORIENTED_EDGE('',*,*,#39000,.T.);
#54101=ORIENTED_EDGE('',*,*,#39002,.F.);
#54102=ORIENTED_EDGE('',*,*,#39003,.F.);
#54103=ORIENTED_EDGE('',*,*,#38695,.T.);
#54104=ORIENTED_EDGE('',*,*,#38694,.T.);
#54105=ORIENTED_EDGE('',*,*,#39004,.F.);
#54106=ORIENTED_EDGE('',*,*,#38698,.T.);
#54107=ORIENTED_EDGE('',*,*,#38696,.T.);
#54108=ORIENTED_EDGE('',*,*,#39003,.T.);
#54109=ORIENTED_EDGE('',*,*,#39005,.F.);
#54110=ORIENTED_EDGE('',*,*,#39006,.F.);
#54111=ORIENTED_EDGE('',*,*,#38702,.T.);
#54112=ORIENTED_EDGE('',*,*,#38701,.T.);
#54113=ORIENTED_EDGE('',*,*,#39007,.F.);
#54114=ORIENTED_EDGE('',*,*,#38705,.T.);
#54115=ORIENTED_EDGE('',*,*,#38703,.T.);
#54116=ORIENTED_EDGE('',*,*,#39006,.T.);
#54117=ORIENTED_EDGE('',*,*,#39008,.F.);
#54118=ORIENTED_EDGE('',*,*,#39009,.F.);
#54119=ORIENTED_EDGE('',*,*,#38709,.T.);
#54120=ORIENTED_EDGE('',*,*,#38708,.T.);
#54121=ORIENTED_EDGE('',*,*,#39010,.F.);
#54122=ORIENTED_EDGE('',*,*,#38712,.T.);
#54123=ORIENTED_EDGE('',*,*,#38710,.T.);
#54124=ORIENTED_EDGE('',*,*,#39009,.T.);
#54125=ORIENTED_EDGE('',*,*,#39011,.F.);
#54126=ORIENTED_EDGE('',*,*,#39012,.F.);
#54127=ORIENTED_EDGE('',*,*,#38716,.T.);
#54128=ORIENTED_EDGE('',*,*,#38715,.T.);
#54129=ORIENTED_EDGE('',*,*,#39013,.F.);
#54130=ORIENTED_EDGE('',*,*,#38719,.T.);
#54131=ORIENTED_EDGE('',*,*,#38717,.T.);
#54132=ORIENTED_EDGE('',*,*,#39012,.T.);
#54133=ORIENTED_EDGE('',*,*,#39014,.F.);
#54134=ORIENTED_EDGE('',*,*,#39015,.F.);
#54135=ORIENTED_EDGE('',*,*,#38723,.T.);
#54136=ORIENTED_EDGE('',*,*,#38722,.T.);
#54137=ORIENTED_EDGE('',*,*,#39016,.F.);
#54138=ORIENTED_EDGE('',*,*,#38726,.T.);
#54139=ORIENTED_EDGE('',*,*,#38724,.T.);
#54140=ORIENTED_EDGE('',*,*,#39015,.T.);
#54141=ORIENTED_EDGE('',*,*,#39017,.F.);
#54142=ORIENTED_EDGE('',*,*,#39018,.F.);
#54143=ORIENTED_EDGE('',*,*,#38730,.T.);
#54144=ORIENTED_EDGE('',*,*,#38729,.T.);
#54145=ORIENTED_EDGE('',*,*,#39019,.F.);
#54146=ORIENTED_EDGE('',*,*,#38733,.T.);
#54147=ORIENTED_EDGE('',*,*,#38731,.T.);
#54148=ORIENTED_EDGE('',*,*,#39018,.T.);
#54149=ORIENTED_EDGE('',*,*,#38739,.T.);
#54150=ORIENTED_EDGE('',*,*,#38734,.T.);
#54151=ORIENTED_EDGE('',*,*,#39020,.F.);
#54152=ORIENTED_EDGE('',*,*,#39021,.F.);
#54153=ORIENTED_EDGE('',*,*,#38740,.T.);
#54154=ORIENTED_EDGE('',*,*,#39021,.T.);
#54155=ORIENTED_EDGE('',*,*,#39022,.F.);
#54156=ORIENTED_EDGE('',*,*,#38738,.T.);
#54157=ORIENTED_EDGE('',*,*,#38746,.T.);
#54158=ORIENTED_EDGE('',*,*,#38741,.T.);
#54159=ORIENTED_EDGE('',*,*,#39023,.F.);
#54160=ORIENTED_EDGE('',*,*,#39024,.F.);
#54161=ORIENTED_EDGE('',*,*,#38747,.T.);
#54162=ORIENTED_EDGE('',*,*,#39024,.T.);
#54163=ORIENTED_EDGE('',*,*,#39025,.F.);
#54164=ORIENTED_EDGE('',*,*,#38745,.T.);
#54165=ORIENTED_EDGE('',*,*,#38753,.T.);
#54166=ORIENTED_EDGE('',*,*,#38748,.T.);
#54167=ORIENTED_EDGE('',*,*,#39026,.F.);
#54168=ORIENTED_EDGE('',*,*,#39027,.F.);
#54169=ORIENTED_EDGE('',*,*,#38754,.T.);
#54170=ORIENTED_EDGE('',*,*,#39027,.T.);
#54171=ORIENTED_EDGE('',*,*,#39028,.F.);
#54172=ORIENTED_EDGE('',*,*,#38752,.T.);
#54173=ORIENTED_EDGE('',*,*,#38760,.T.);
#54174=ORIENTED_EDGE('',*,*,#38755,.T.);
#54175=ORIENTED_EDGE('',*,*,#39029,.F.);
#54176=ORIENTED_EDGE('',*,*,#39030,.F.);
#54177=ORIENTED_EDGE('',*,*,#38761,.T.);
#54178=ORIENTED_EDGE('',*,*,#39030,.T.);
#54179=ORIENTED_EDGE('',*,*,#39031,.F.);
#54180=ORIENTED_EDGE('',*,*,#38759,.T.);
#54181=ORIENTED_EDGE('',*,*,#38767,.T.);
#54182=ORIENTED_EDGE('',*,*,#38762,.T.);
#54183=ORIENTED_EDGE('',*,*,#39032,.F.);
#54184=ORIENTED_EDGE('',*,*,#39033,.F.);
#54185=ORIENTED_EDGE('',*,*,#38768,.T.);
#54186=ORIENTED_EDGE('',*,*,#39033,.T.);
#54187=ORIENTED_EDGE('',*,*,#39034,.F.);
#54188=ORIENTED_EDGE('',*,*,#38766,.T.);
#54189=ORIENTED_EDGE('',*,*,#38774,.T.);
#54190=ORIENTED_EDGE('',*,*,#38769,.T.);
#54191=ORIENTED_EDGE('',*,*,#39035,.F.);
#54192=ORIENTED_EDGE('',*,*,#39036,.F.);
#54193=ORIENTED_EDGE('',*,*,#38775,.T.);
#54194=ORIENTED_EDGE('',*,*,#39036,.T.);
#54195=ORIENTED_EDGE('',*,*,#39037,.F.);
#54196=ORIENTED_EDGE('',*,*,#38773,.T.);
#54197=ORIENTED_EDGE('',*,*,#38781,.T.);
#54198=ORIENTED_EDGE('',*,*,#38776,.T.);
#54199=ORIENTED_EDGE('',*,*,#39038,.F.);
#54200=ORIENTED_EDGE('',*,*,#39039,.F.);
#54201=ORIENTED_EDGE('',*,*,#38782,.T.);
#54202=ORIENTED_EDGE('',*,*,#39039,.T.);
#54203=ORIENTED_EDGE('',*,*,#39040,.F.);
#54204=ORIENTED_EDGE('',*,*,#38780,.T.);
#54205=ORIENTED_EDGE('',*,*,#38788,.T.);
#54206=ORIENTED_EDGE('',*,*,#38783,.T.);
#54207=ORIENTED_EDGE('',*,*,#39041,.F.);
#54208=ORIENTED_EDGE('',*,*,#39042,.F.);
#54209=ORIENTED_EDGE('',*,*,#38789,.T.);
#54210=ORIENTED_EDGE('',*,*,#39042,.T.);
#54211=ORIENTED_EDGE('',*,*,#39043,.F.);
#54212=ORIENTED_EDGE('',*,*,#38787,.T.);
#54213=ORIENTED_EDGE('',*,*,#38795,.T.);
#54214=ORIENTED_EDGE('',*,*,#38790,.T.);
#54215=ORIENTED_EDGE('',*,*,#39044,.F.);
#54216=ORIENTED_EDGE('',*,*,#39045,.F.);
#54217=ORIENTED_EDGE('',*,*,#38796,.T.);
#54218=ORIENTED_EDGE('',*,*,#39045,.T.);
#54219=ORIENTED_EDGE('',*,*,#39046,.F.);
#54220=ORIENTED_EDGE('',*,*,#38794,.T.);
#54221=ORIENTED_EDGE('',*,*,#38802,.T.);
#54222=ORIENTED_EDGE('',*,*,#38797,.T.);
#54223=ORIENTED_EDGE('',*,*,#39047,.F.);
#54224=ORIENTED_EDGE('',*,*,#39048,.F.);
#54225=ORIENTED_EDGE('',*,*,#38803,.T.);
#54226=ORIENTED_EDGE('',*,*,#39048,.T.);
#54227=ORIENTED_EDGE('',*,*,#39049,.F.);
#54228=ORIENTED_EDGE('',*,*,#38801,.T.);
#54229=ORIENTED_EDGE('',*,*,#38809,.T.);
#54230=ORIENTED_EDGE('',*,*,#38804,.T.);
#54231=ORIENTED_EDGE('',*,*,#39050,.F.);
#54232=ORIENTED_EDGE('',*,*,#39051,.F.);
#54233=ORIENTED_EDGE('',*,*,#38810,.T.);
#54234=ORIENTED_EDGE('',*,*,#39051,.T.);
#54235=ORIENTED_EDGE('',*,*,#39052,.F.);
#54236=ORIENTED_EDGE('',*,*,#38808,.T.);
#54237=ORIENTED_EDGE('',*,*,#38816,.T.);
#54238=ORIENTED_EDGE('',*,*,#38811,.T.);
#54239=ORIENTED_EDGE('',*,*,#39053,.F.);
#54240=ORIENTED_EDGE('',*,*,#39054,.F.);
#54241=ORIENTED_EDGE('',*,*,#38817,.T.);
#54242=ORIENTED_EDGE('',*,*,#39054,.T.);
#54243=ORIENTED_EDGE('',*,*,#39055,.F.);
#54244=ORIENTED_EDGE('',*,*,#38815,.T.);
#54245=ORIENTED_EDGE('',*,*,#38823,.T.);
#54246=ORIENTED_EDGE('',*,*,#38818,.T.);
#54247=ORIENTED_EDGE('',*,*,#39056,.F.);
#54248=ORIENTED_EDGE('',*,*,#39057,.F.);
#54249=ORIENTED_EDGE('',*,*,#38824,.T.);
#54250=ORIENTED_EDGE('',*,*,#39057,.T.);
#54251=ORIENTED_EDGE('',*,*,#39058,.F.);
#54252=ORIENTED_EDGE('',*,*,#38822,.T.);
#54253=ORIENTED_EDGE('',*,*,#38830,.T.);
#54254=ORIENTED_EDGE('',*,*,#38825,.T.);
#54255=ORIENTED_EDGE('',*,*,#39059,.F.);
#54256=ORIENTED_EDGE('',*,*,#39060,.F.);
#54257=ORIENTED_EDGE('',*,*,#38831,.T.);
#54258=ORIENTED_EDGE('',*,*,#39060,.T.);
#54259=ORIENTED_EDGE('',*,*,#39061,.F.);
#54260=ORIENTED_EDGE('',*,*,#38829,.T.);
#54261=ORIENTED_EDGE('',*,*,#38837,.T.);
#54262=ORIENTED_EDGE('',*,*,#38832,.T.);
#54263=ORIENTED_EDGE('',*,*,#39062,.F.);
#54264=ORIENTED_EDGE('',*,*,#39063,.F.);
#54265=ORIENTED_EDGE('',*,*,#38838,.T.);
#54266=ORIENTED_EDGE('',*,*,#39063,.T.);
#54267=ORIENTED_EDGE('',*,*,#39064,.F.);
#54268=ORIENTED_EDGE('',*,*,#38836,.T.);
#54269=ORIENTED_EDGE('',*,*,#38844,.T.);
#54270=ORIENTED_EDGE('',*,*,#38839,.T.);
#54271=ORIENTED_EDGE('',*,*,#39065,.F.);
#54272=ORIENTED_EDGE('',*,*,#39066,.F.);
#54273=ORIENTED_EDGE('',*,*,#38845,.T.);
#54274=ORIENTED_EDGE('',*,*,#39066,.T.);
#54275=ORIENTED_EDGE('',*,*,#39067,.F.);
#54276=ORIENTED_EDGE('',*,*,#38843,.T.);
#54277=ORIENTED_EDGE('',*,*,#38851,.T.);
#54278=ORIENTED_EDGE('',*,*,#38846,.T.);
#54279=ORIENTED_EDGE('',*,*,#39068,.F.);
#54280=ORIENTED_EDGE('',*,*,#39069,.F.);
#54281=ORIENTED_EDGE('',*,*,#38852,.T.);
#54282=ORIENTED_EDGE('',*,*,#39069,.T.);
#54283=ORIENTED_EDGE('',*,*,#39070,.F.);
#54284=ORIENTED_EDGE('',*,*,#38850,.T.);
#54285=ORIENTED_EDGE('',*,*,#38858,.T.);
#54286=ORIENTED_EDGE('',*,*,#38853,.T.);
#54287=ORIENTED_EDGE('',*,*,#39071,.F.);
#54288=ORIENTED_EDGE('',*,*,#39072,.F.);
#54289=ORIENTED_EDGE('',*,*,#38859,.T.);
#54290=ORIENTED_EDGE('',*,*,#39072,.T.);
#54291=ORIENTED_EDGE('',*,*,#39073,.F.);
#54292=ORIENTED_EDGE('',*,*,#38857,.T.);
#54293=ORIENTED_EDGE('',*,*,#38865,.T.);
#54294=ORIENTED_EDGE('',*,*,#38860,.T.);
#54295=ORIENTED_EDGE('',*,*,#39074,.F.);
#54296=ORIENTED_EDGE('',*,*,#39075,.F.);
#54297=ORIENTED_EDGE('',*,*,#38866,.T.);
#54298=ORIENTED_EDGE('',*,*,#39075,.T.);
#54299=ORIENTED_EDGE('',*,*,#39076,.F.);
#54300=ORIENTED_EDGE('',*,*,#38864,.T.);
#54301=ORIENTED_EDGE('',*,*,#38872,.T.);
#54302=ORIENTED_EDGE('',*,*,#38867,.T.);
#54303=ORIENTED_EDGE('',*,*,#39077,.F.);
#54304=ORIENTED_EDGE('',*,*,#39078,.F.);
#54305=ORIENTED_EDGE('',*,*,#38873,.T.);
#54306=ORIENTED_EDGE('',*,*,#39078,.T.);
#54307=ORIENTED_EDGE('',*,*,#39079,.F.);
#54308=ORIENTED_EDGE('',*,*,#38871,.T.);
#54309=ORIENTED_EDGE('',*,*,#38879,.T.);
#54310=ORIENTED_EDGE('',*,*,#38874,.T.);
#54311=ORIENTED_EDGE('',*,*,#39080,.F.);
#54312=ORIENTED_EDGE('',*,*,#39081,.F.);
#54313=ORIENTED_EDGE('',*,*,#38880,.T.);
#54314=ORIENTED_EDGE('',*,*,#39081,.T.);
#54315=ORIENTED_EDGE('',*,*,#39082,.F.);
#54316=ORIENTED_EDGE('',*,*,#38878,.T.);
#54317=ORIENTED_EDGE('',*,*,#34409,.T.);
#54318=ORIENTED_EDGE('',*,*,#38881,.T.);
#54319=ORIENTED_EDGE('',*,*,#39083,.F.);
#54320=ORIENTED_EDGE('',*,*,#39084,.F.);
#54321=ORIENTED_EDGE('',*,*,#34410,.T.);
#54322=ORIENTED_EDGE('',*,*,#39084,.T.);
#54323=ORIENTED_EDGE('',*,*,#39085,.F.);
#54324=ORIENTED_EDGE('',*,*,#38883,.T.);
#54325=ORIENTED_EDGE('',*,*,#38889,.T.);
#54326=ORIENTED_EDGE('',*,*,#38884,.T.);
#54327=ORIENTED_EDGE('',*,*,#39086,.F.);
#54328=ORIENTED_EDGE('',*,*,#39087,.F.);
#54329=ORIENTED_EDGE('',*,*,#38890,.T.);
#54330=ORIENTED_EDGE('',*,*,#39087,.T.);
#54331=ORIENTED_EDGE('',*,*,#39088,.F.);
#54332=ORIENTED_EDGE('',*,*,#38888,.T.);
#54333=ORIENTED_EDGE('',*,*,#38896,.T.);
#54334=ORIENTED_EDGE('',*,*,#38891,.T.);
#54335=ORIENTED_EDGE('',*,*,#39089,.F.);
#54336=ORIENTED_EDGE('',*,*,#39090,.F.);
#54337=ORIENTED_EDGE('',*,*,#38897,.T.);
#54338=ORIENTED_EDGE('',*,*,#39090,.T.);
#54339=ORIENTED_EDGE('',*,*,#39091,.F.);
#54340=ORIENTED_EDGE('',*,*,#38895,.T.);
#54341=ORIENTED_EDGE('',*,*,#38903,.T.);
#54342=ORIENTED_EDGE('',*,*,#38898,.T.);
#54343=ORIENTED_EDGE('',*,*,#39092,.F.);
#54344=ORIENTED_EDGE('',*,*,#39093,.F.);
#54345=ORIENTED_EDGE('',*,*,#38904,.T.);
#54346=ORIENTED_EDGE('',*,*,#39093,.T.);
#54347=ORIENTED_EDGE('',*,*,#39094,.F.);
#54348=ORIENTED_EDGE('',*,*,#38902,.T.);
#54349=ORIENTED_EDGE('',*,*,#38910,.T.);
#54350=ORIENTED_EDGE('',*,*,#38905,.T.);
#54351=ORIENTED_EDGE('',*,*,#39095,.F.);
#54352=ORIENTED_EDGE('',*,*,#39096,.F.);
#54353=ORIENTED_EDGE('',*,*,#38911,.T.);
#54354=ORIENTED_EDGE('',*,*,#39096,.T.);
#54355=ORIENTED_EDGE('',*,*,#39097,.F.);
#54356=ORIENTED_EDGE('',*,*,#38909,.T.);
#54357=ORIENTED_EDGE('',*,*,#38917,.T.);
#54358=ORIENTED_EDGE('',*,*,#38912,.T.);
#54359=ORIENTED_EDGE('',*,*,#39098,.F.);
#54360=ORIENTED_EDGE('',*,*,#39099,.F.);
#54361=ORIENTED_EDGE('',*,*,#38918,.T.);
#54362=ORIENTED_EDGE('',*,*,#39099,.T.);
#54363=ORIENTED_EDGE('',*,*,#39100,.F.);
#54364=ORIENTED_EDGE('',*,*,#38916,.T.);
#54365=ORIENTED_EDGE('',*,*,#39101,.F.);
#54366=ORIENTED_EDGE('',*,*,#39102,.F.);
#54367=ORIENTED_EDGE('',*,*,#38924,.T.);
#54368=ORIENTED_EDGE('',*,*,#38919,.T.);
#54369=ORIENTED_EDGE('',*,*,#38925,.T.);
#54370=ORIENTED_EDGE('',*,*,#39102,.T.);
#54371=ORIENTED_EDGE('',*,*,#39103,.F.);
#54372=ORIENTED_EDGE('',*,*,#38923,.T.);
#54373=ORIENTED_EDGE('',*,*,#38931,.T.);
#54374=ORIENTED_EDGE('',*,*,#38926,.T.);
#54375=ORIENTED_EDGE('',*,*,#39104,.F.);
#54376=ORIENTED_EDGE('',*,*,#39105,.F.);
#54377=ORIENTED_EDGE('',*,*,#38932,.T.);
#54378=ORIENTED_EDGE('',*,*,#39105,.T.);
#54379=ORIENTED_EDGE('',*,*,#39106,.F.);
#54380=ORIENTED_EDGE('',*,*,#38930,.T.);
#54381=ORIENTED_EDGE('',*,*,#39107,.T.);
#54382=ORIENTED_EDGE('',*,*,#39108,.F.);
#54383=ORIENTED_EDGE('',*,*,#38933,.T.);
#54384=ORIENTED_EDGE('',*,*,#39109,.F.);
#54385=ORIENTED_EDGE('',*,*,#39110,.T.);
#54386=ORIENTED_EDGE('',*,*,#39111,.F.);
#54387=ORIENTED_EDGE('',*,*,#38935,.T.);
#54388=ORIENTED_EDGE('',*,*,#39112,.F.);
#54389=ORIENTED_EDGE('',*,*,#39113,.F.);
#54390=ORIENTED_EDGE('',*,*,#39114,.F.);
#54391=ORIENTED_EDGE('',*,*,#39115,.F.);
#54392=ORIENTED_EDGE('',*,*,#39110,.F.);
#54393=ORIENTED_EDGE('',*,*,#39115,.T.);
#54394=ORIENTED_EDGE('',*,*,#39116,.F.);
#54395=ORIENTED_EDGE('',*,*,#38936,.T.);
#54396=ORIENTED_EDGE('',*,*,#39111,.T.);
#54397=ORIENTED_EDGE('',*,*,#39117,.T.);
#54398=ORIENTED_EDGE('',*,*,#39118,.F.);
#54399=ORIENTED_EDGE('',*,*,#38938,.T.);
#54400=ORIENTED_EDGE('',*,*,#39119,.F.);
#54401=ORIENTED_EDGE('',*,*,#39120,.F.);
#54402=ORIENTED_EDGE('',*,*,#39121,.F.);
#54403=ORIENTED_EDGE('',*,*,#39122,.F.);
#54404=ORIENTED_EDGE('',*,*,#39117,.F.);
#54405=ORIENTED_EDGE('',*,*,#39122,.T.);
#54406=ORIENTED_EDGE('',*,*,#39123,.F.);
#54407=ORIENTED_EDGE('',*,*,#38939,.T.);
#54408=ORIENTED_EDGE('',*,*,#39118,.T.);
#54409=ORIENTED_EDGE('',*,*,#39124,.T.);
#54410=ORIENTED_EDGE('',*,*,#39125,.F.);
#54411=ORIENTED_EDGE('',*,*,#38941,.T.);
#54412=ORIENTED_EDGE('',*,*,#39126,.F.);
#54413=ORIENTED_EDGE('',*,*,#39127,.F.);
#54414=ORIENTED_EDGE('',*,*,#39128,.F.);
#54415=ORIENTED_EDGE('',*,*,#39129,.F.);
#54416=ORIENTED_EDGE('',*,*,#39124,.F.);
#54417=ORIENTED_EDGE('',*,*,#39129,.T.);
#54418=ORIENTED_EDGE('',*,*,#39130,.F.);
#54419=ORIENTED_EDGE('',*,*,#38942,.T.);
#54420=ORIENTED_EDGE('',*,*,#39125,.T.);
#54421=ORIENTED_EDGE('',*,*,#39131,.T.);
#54422=ORIENTED_EDGE('',*,*,#39132,.F.);
#54423=ORIENTED_EDGE('',*,*,#38944,.T.);
#54424=ORIENTED_EDGE('',*,*,#39133,.F.);
#54425=ORIENTED_EDGE('',*,*,#39134,.F.);
#54426=ORIENTED_EDGE('',*,*,#39135,.F.);
#54427=ORIENTED_EDGE('',*,*,#39136,.F.);
#54428=ORIENTED_EDGE('',*,*,#39131,.F.);
#54429=ORIENTED_EDGE('',*,*,#39136,.T.);
#54430=ORIENTED_EDGE('',*,*,#39137,.F.);
#54431=ORIENTED_EDGE('',*,*,#38945,.T.);
#54432=ORIENTED_EDGE('',*,*,#39132,.T.);
#54433=ORIENTED_EDGE('',*,*,#39138,.T.);
#54434=ORIENTED_EDGE('',*,*,#39139,.F.);
#54435=ORIENTED_EDGE('',*,*,#38947,.T.);
#54436=ORIENTED_EDGE('',*,*,#39140,.F.);
#54437=ORIENTED_EDGE('',*,*,#39141,.F.);
#54438=ORIENTED_EDGE('',*,*,#39142,.F.);
#54439=ORIENTED_EDGE('',*,*,#39143,.F.);
#54440=ORIENTED_EDGE('',*,*,#39138,.F.);
#54441=ORIENTED_EDGE('',*,*,#39143,.T.);
#54442=ORIENTED_EDGE('',*,*,#39144,.F.);
#54443=ORIENTED_EDGE('',*,*,#38948,.T.);
#54444=ORIENTED_EDGE('',*,*,#39139,.T.);
#54445=ORIENTED_EDGE('',*,*,#39145,.T.);
#54446=ORIENTED_EDGE('',*,*,#39146,.F.);
#54447=ORIENTED_EDGE('',*,*,#38950,.T.);
#54448=ORIENTED_EDGE('',*,*,#39147,.F.);
#54449=ORIENTED_EDGE('',*,*,#39148,.F.);
#54450=ORIENTED_EDGE('',*,*,#39149,.F.);
#54451=ORIENTED_EDGE('',*,*,#39150,.F.);
#54452=ORIENTED_EDGE('',*,*,#39145,.F.);
#54453=ORIENTED_EDGE('',*,*,#39150,.T.);
#54454=ORIENTED_EDGE('',*,*,#39151,.F.);
#54455=ORIENTED_EDGE('',*,*,#38951,.T.);
#54456=ORIENTED_EDGE('',*,*,#39146,.T.);
#54457=ORIENTED_EDGE('',*,*,#34406,.T.);
#54458=ORIENTED_EDGE('',*,*,#39152,.F.);
#54459=ORIENTED_EDGE('',*,*,#38953,.T.);
#54460=ORIENTED_EDGE('',*,*,#39153,.F.);
#54461=ORIENTED_EDGE('',*,*,#34405,.T.);
#54462=ORIENTED_EDGE('',*,*,#39154,.F.);
#54463=ORIENTED_EDGE('',*,*,#38954,.T.);
#54464=ORIENTED_EDGE('',*,*,#39152,.T.);
#54465=ORIENTED_EDGE('',*,*,#39155,.T.);
#54466=ORIENTED_EDGE('',*,*,#39156,.F.);
#54467=ORIENTED_EDGE('',*,*,#38956,.T.);
#54468=ORIENTED_EDGE('',*,*,#39157,.F.);
#54469=ORIENTED_EDGE('',*,*,#39158,.F.);
#54470=ORIENTED_EDGE('',*,*,#39159,.F.);
#54471=ORIENTED_EDGE('',*,*,#39160,.F.);
#54472=ORIENTED_EDGE('',*,*,#39155,.F.);
#54473=ORIENTED_EDGE('',*,*,#39160,.T.);
#54474=ORIENTED_EDGE('',*,*,#39161,.F.);
#54475=ORIENTED_EDGE('',*,*,#38957,.T.);
#54476=ORIENTED_EDGE('',*,*,#39156,.T.);
#54477=ORIENTED_EDGE('',*,*,#39162,.T.);
#54478=ORIENTED_EDGE('',*,*,#39163,.F.);
#54479=ORIENTED_EDGE('',*,*,#38959,.T.);
#54480=ORIENTED_EDGE('',*,*,#39164,.F.);
#54481=ORIENTED_EDGE('',*,*,#39165,.F.);
#54482=ORIENTED_EDGE('',*,*,#39166,.F.);
#54483=ORIENTED_EDGE('',*,*,#39167,.F.);
#54484=ORIENTED_EDGE('',*,*,#39162,.F.);
#54485=ORIENTED_EDGE('',*,*,#39167,.T.);
#54486=ORIENTED_EDGE('',*,*,#39168,.F.);
#54487=ORIENTED_EDGE('',*,*,#38960,.T.);
#54488=ORIENTED_EDGE('',*,*,#39163,.T.);
#54489=ORIENTED_EDGE('',*,*,#39169,.T.);
#54490=ORIENTED_EDGE('',*,*,#39170,.F.);
#54491=ORIENTED_EDGE('',*,*,#38962,.T.);
#54492=ORIENTED_EDGE('',*,*,#39171,.F.);
#54493=ORIENTED_EDGE('',*,*,#39172,.F.);
#54494=ORIENTED_EDGE('',*,*,#39173,.F.);
#54495=ORIENTED_EDGE('',*,*,#39174,.F.);
#54496=ORIENTED_EDGE('',*,*,#39169,.F.);
#54497=ORIENTED_EDGE('',*,*,#39174,.T.);
#54498=ORIENTED_EDGE('',*,*,#39175,.F.);
#54499=ORIENTED_EDGE('',*,*,#38963,.T.);
#54500=ORIENTED_EDGE('',*,*,#39170,.T.);
#54501=ORIENTED_EDGE('',*,*,#39176,.T.);
#54502=ORIENTED_EDGE('',*,*,#39177,.F.);
#54503=ORIENTED_EDGE('',*,*,#38965,.T.);
#54504=ORIENTED_EDGE('',*,*,#39178,.F.);
#54505=ORIENTED_EDGE('',*,*,#39179,.F.);
#54506=ORIENTED_EDGE('',*,*,#39180,.F.);
#54507=ORIENTED_EDGE('',*,*,#39181,.F.);
#54508=ORIENTED_EDGE('',*,*,#39176,.F.);
#54509=ORIENTED_EDGE('',*,*,#39181,.T.);
#54510=ORIENTED_EDGE('',*,*,#39182,.F.);
#54511=ORIENTED_EDGE('',*,*,#38966,.T.);
#54512=ORIENTED_EDGE('',*,*,#39177,.T.);
#54513=ORIENTED_EDGE('',*,*,#39183,.T.);
#54514=ORIENTED_EDGE('',*,*,#39184,.F.);
#54515=ORIENTED_EDGE('',*,*,#38968,.T.);
#54516=ORIENTED_EDGE('',*,*,#39185,.F.);
#54517=ORIENTED_EDGE('',*,*,#39186,.F.);
#54518=ORIENTED_EDGE('',*,*,#39187,.F.);
#54519=ORIENTED_EDGE('',*,*,#39188,.F.);
#54520=ORIENTED_EDGE('',*,*,#39183,.F.);
#54521=ORIENTED_EDGE('',*,*,#39188,.T.);
#54522=ORIENTED_EDGE('',*,*,#39189,.F.);
#54523=ORIENTED_EDGE('',*,*,#38969,.T.);
#54524=ORIENTED_EDGE('',*,*,#39184,.T.);
#54525=ORIENTED_EDGE('',*,*,#39190,.T.);
#54526=ORIENTED_EDGE('',*,*,#39191,.F.);
#54527=ORIENTED_EDGE('',*,*,#38971,.T.);
#54528=ORIENTED_EDGE('',*,*,#39192,.F.);
#54529=ORIENTED_EDGE('',*,*,#39193,.F.);
#54530=ORIENTED_EDGE('',*,*,#39194,.F.);
#54531=ORIENTED_EDGE('',*,*,#39195,.F.);
#54532=ORIENTED_EDGE('',*,*,#39190,.F.);
#54533=ORIENTED_EDGE('',*,*,#39195,.T.);
#54534=ORIENTED_EDGE('',*,*,#39196,.F.);
#54535=ORIENTED_EDGE('',*,*,#38972,.T.);
#54536=ORIENTED_EDGE('',*,*,#39191,.T.);
#54537=ORIENTED_EDGE('',*,*,#39197,.T.);
#54538=ORIENTED_EDGE('',*,*,#39198,.F.);
#54539=ORIENTED_EDGE('',*,*,#38974,.T.);
#54540=ORIENTED_EDGE('',*,*,#39199,.F.);
#54541=ORIENTED_EDGE('',*,*,#39200,.F.);
#54542=ORIENTED_EDGE('',*,*,#39201,.F.);
#54543=ORIENTED_EDGE('',*,*,#39202,.F.);
#54544=ORIENTED_EDGE('',*,*,#39197,.F.);
#54545=ORIENTED_EDGE('',*,*,#39202,.T.);
#54546=ORIENTED_EDGE('',*,*,#39203,.F.);
#54547=ORIENTED_EDGE('',*,*,#38975,.T.);
#54548=ORIENTED_EDGE('',*,*,#39198,.T.);
#54549=ORIENTED_EDGE('',*,*,#39204,.T.);
#54550=ORIENTED_EDGE('',*,*,#39205,.F.);
#54551=ORIENTED_EDGE('',*,*,#38977,.T.);
#54552=ORIENTED_EDGE('',*,*,#39206,.F.);
#54553=ORIENTED_EDGE('',*,*,#39207,.F.);
#54554=ORIENTED_EDGE('',*,*,#39208,.F.);
#54555=ORIENTED_EDGE('',*,*,#39209,.F.);
#54556=ORIENTED_EDGE('',*,*,#39204,.F.);
#54557=ORIENTED_EDGE('',*,*,#39209,.T.);
#54558=ORIENTED_EDGE('',*,*,#39210,.F.);
#54559=ORIENTED_EDGE('',*,*,#38978,.T.);
#54560=ORIENTED_EDGE('',*,*,#39205,.T.);
#54561=ORIENTED_EDGE('',*,*,#39211,.T.);
#54562=ORIENTED_EDGE('',*,*,#39212,.F.);
#54563=ORIENTED_EDGE('',*,*,#38980,.T.);
#54564=ORIENTED_EDGE('',*,*,#39213,.F.);
#54565=ORIENTED_EDGE('',*,*,#39214,.F.);
#54566=ORIENTED_EDGE('',*,*,#39215,.F.);
#54567=ORIENTED_EDGE('',*,*,#39216,.F.);
#54568=ORIENTED_EDGE('',*,*,#39211,.F.);
#54569=ORIENTED_EDGE('',*,*,#39216,.T.);
#54570=ORIENTED_EDGE('',*,*,#39217,.F.);
#54571=ORIENTED_EDGE('',*,*,#38981,.T.);
#54572=ORIENTED_EDGE('',*,*,#39212,.T.);
#54573=ORIENTED_EDGE('',*,*,#39218,.T.);
#54574=ORIENTED_EDGE('',*,*,#39219,.F.);
#54575=ORIENTED_EDGE('',*,*,#38983,.T.);
#54576=ORIENTED_EDGE('',*,*,#39220,.F.);
#54577=ORIENTED_EDGE('',*,*,#39221,.F.);
#54578=ORIENTED_EDGE('',*,*,#39222,.F.);
#54579=ORIENTED_EDGE('',*,*,#39223,.F.);
#54580=ORIENTED_EDGE('',*,*,#39218,.F.);
#54581=ORIENTED_EDGE('',*,*,#39223,.T.);
#54582=ORIENTED_EDGE('',*,*,#39224,.F.);
#54583=ORIENTED_EDGE('',*,*,#38984,.T.);
#54584=ORIENTED_EDGE('',*,*,#39219,.T.);
#54585=ORIENTED_EDGE('',*,*,#39225,.T.);
#54586=ORIENTED_EDGE('',*,*,#39226,.F.);
#54587=ORIENTED_EDGE('',*,*,#38986,.T.);
#54588=ORIENTED_EDGE('',*,*,#39227,.F.);
#54589=ORIENTED_EDGE('',*,*,#39228,.F.);
#54590=ORIENTED_EDGE('',*,*,#39229,.F.);
#54591=ORIENTED_EDGE('',*,*,#39230,.F.);
#54592=ORIENTED_EDGE('',*,*,#39225,.F.);
#54593=ORIENTED_EDGE('',*,*,#39230,.T.);
#54594=ORIENTED_EDGE('',*,*,#39231,.F.);
#54595=ORIENTED_EDGE('',*,*,#38987,.T.);
#54596=ORIENTED_EDGE('',*,*,#39226,.T.);
#54597=ORIENTED_EDGE('',*,*,#39232,.T.);
#54598=ORIENTED_EDGE('',*,*,#39233,.F.);
#54599=ORIENTED_EDGE('',*,*,#38989,.T.);
#54600=ORIENTED_EDGE('',*,*,#39234,.F.);
#54601=ORIENTED_EDGE('',*,*,#39235,.F.);
#54602=ORIENTED_EDGE('',*,*,#39236,.F.);
#54603=ORIENTED_EDGE('',*,*,#39237,.F.);
#54604=ORIENTED_EDGE('',*,*,#39232,.F.);
#54605=ORIENTED_EDGE('',*,*,#39237,.T.);
#54606=ORIENTED_EDGE('',*,*,#39238,.F.);
#54607=ORIENTED_EDGE('',*,*,#38990,.T.);
#54608=ORIENTED_EDGE('',*,*,#39233,.T.);
#54609=ORIENTED_EDGE('',*,*,#39239,.T.);
#54610=ORIENTED_EDGE('',*,*,#39240,.F.);
#54611=ORIENTED_EDGE('',*,*,#38992,.T.);
#54612=ORIENTED_EDGE('',*,*,#39241,.F.);
#54613=ORIENTED_EDGE('',*,*,#39242,.F.);
#54614=ORIENTED_EDGE('',*,*,#39243,.F.);
#54615=ORIENTED_EDGE('',*,*,#39244,.F.);
#54616=ORIENTED_EDGE('',*,*,#39239,.F.);
#54617=ORIENTED_EDGE('',*,*,#39244,.T.);
#54618=ORIENTED_EDGE('',*,*,#39245,.F.);
#54619=ORIENTED_EDGE('',*,*,#38993,.T.);
#54620=ORIENTED_EDGE('',*,*,#39240,.T.);
#54621=ORIENTED_EDGE('',*,*,#39246,.T.);
#54622=ORIENTED_EDGE('',*,*,#39247,.F.);
#54623=ORIENTED_EDGE('',*,*,#38995,.T.);
#54624=ORIENTED_EDGE('',*,*,#39248,.F.);
#54625=ORIENTED_EDGE('',*,*,#39249,.T.);
#54626=ORIENTED_EDGE('',*,*,#39250,.F.);
#54627=ORIENTED_EDGE('',*,*,#38996,.T.);
#54628=ORIENTED_EDGE('',*,*,#39247,.T.);
#54629=ORIENTED_EDGE('',*,*,#39251,.F.);
#54630=ORIENTED_EDGE('',*,*,#39252,.F.);
#54631=ORIENTED_EDGE('',*,*,#39249,.F.);
#54632=ORIENTED_EDGE('',*,*,#39246,.F.);
#54633=ORIENTED_EDGE('',*,*,#38998,.T.);
#54634=ORIENTED_EDGE('',*,*,#39253,.F.);
#54635=ORIENTED_EDGE('',*,*,#39254,.T.);
#54636=ORIENTED_EDGE('',*,*,#39255,.F.);
#54637=ORIENTED_EDGE('',*,*,#39256,.F.);
#54638=ORIENTED_EDGE('',*,*,#39254,.F.);
#54639=ORIENTED_EDGE('',*,*,#39257,.F.);
#54640=ORIENTED_EDGE('',*,*,#39258,.F.);
#54641=ORIENTED_EDGE('',*,*,#38999,.T.);
#54642=ORIENTED_EDGE('',*,*,#39255,.T.);
#54643=ORIENTED_EDGE('',*,*,#39256,.T.);
#54644=ORIENTED_EDGE('',*,*,#39259,.F.);
#54645=ORIENTED_EDGE('',*,*,#39260,.T.);
#54646=ORIENTED_EDGE('',*,*,#39261,.F.);
#54647=ORIENTED_EDGE('',*,*,#39001,.T.);
#54648=ORIENTED_EDGE('',*,*,#39262,.F.);
#54649=ORIENTED_EDGE('',*,*,#39263,.F.);
#54650=ORIENTED_EDGE('',*,*,#39264,.F.);
#54651=ORIENTED_EDGE('',*,*,#39265,.F.);
#54652=ORIENTED_EDGE('',*,*,#39260,.F.);
#54653=ORIENTED_EDGE('',*,*,#39265,.T.);
#54654=ORIENTED_EDGE('',*,*,#39266,.F.);
#54655=ORIENTED_EDGE('',*,*,#39002,.T.);
#54656=ORIENTED_EDGE('',*,*,#39261,.T.);
#54657=ORIENTED_EDGE('',*,*,#39267,.T.);
#54658=ORIENTED_EDGE('',*,*,#39268,.F.);
#54659=ORIENTED_EDGE('',*,*,#39004,.T.);
#54660=ORIENTED_EDGE('',*,*,#39269,.F.);
#54661=ORIENTED_EDGE('',*,*,#39270,.F.);
#54662=ORIENTED_EDGE('',*,*,#39271,.F.);
#54663=ORIENTED_EDGE('',*,*,#39272,.F.);
#54664=ORIENTED_EDGE('',*,*,#39267,.F.);
#54665=ORIENTED_EDGE('',*,*,#39272,.T.);
#54666=ORIENTED_EDGE('',*,*,#39273,.F.);
#54667=ORIENTED_EDGE('',*,*,#39005,.T.);
#54668=ORIENTED_EDGE('',*,*,#39268,.T.);
#54669=ORIENTED_EDGE('',*,*,#39274,.T.);
#54670=ORIENTED_EDGE('',*,*,#39275,.F.);
#54671=ORIENTED_EDGE('',*,*,#39007,.T.);
#54672=ORIENTED_EDGE('',*,*,#39276,.F.);
#54673=ORIENTED_EDGE('',*,*,#39277,.F.);
#54674=ORIENTED_EDGE('',*,*,#39278,.F.);
#54675=ORIENTED_EDGE('',*,*,#39279,.F.);
#54676=ORIENTED_EDGE('',*,*,#39274,.F.);
#54677=ORIENTED_EDGE('',*,*,#39279,.T.);
#54678=ORIENTED_EDGE('',*,*,#39280,.F.);
#54679=ORIENTED_EDGE('',*,*,#39008,.T.);
#54680=ORIENTED_EDGE('',*,*,#39275,.T.);
#54681=ORIENTED_EDGE('',*,*,#39281,.T.);
#54682=ORIENTED_EDGE('',*,*,#39282,.F.);
#54683=ORIENTED_EDGE('',*,*,#39010,.T.);
#54684=ORIENTED_EDGE('',*,*,#39283,.F.);
#54685=ORIENTED_EDGE('',*,*,#39284,.F.);
#54686=ORIENTED_EDGE('',*,*,#39285,.F.);
#54687=ORIENTED_EDGE('',*,*,#39286,.F.);
#54688=ORIENTED_EDGE('',*,*,#39281,.F.);
#54689=ORIENTED_EDGE('',*,*,#39286,.T.);
#54690=ORIENTED_EDGE('',*,*,#39287,.F.);
#54691=ORIENTED_EDGE('',*,*,#39011,.T.);
#54692=ORIENTED_EDGE('',*,*,#39282,.T.);
#54693=ORIENTED_EDGE('',*,*,#39288,.T.);
#54694=ORIENTED_EDGE('',*,*,#39289,.F.);
#54695=ORIENTED_EDGE('',*,*,#39013,.T.);
#54696=ORIENTED_EDGE('',*,*,#39290,.F.);
#54697=ORIENTED_EDGE('',*,*,#39291,.F.);
#54698=ORIENTED_EDGE('',*,*,#39292,.F.);
#54699=ORIENTED_EDGE('',*,*,#39293,.F.);
#54700=ORIENTED_EDGE('',*,*,#39288,.F.);
#54701=ORIENTED_EDGE('',*,*,#39293,.T.);
#54702=ORIENTED_EDGE('',*,*,#39294,.F.);
#54703=ORIENTED_EDGE('',*,*,#39014,.T.);
#54704=ORIENTED_EDGE('',*,*,#39289,.T.);
#54705=ORIENTED_EDGE('',*,*,#39295,.T.);
#54706=ORIENTED_EDGE('',*,*,#39296,.F.);
#54707=ORIENTED_EDGE('',*,*,#39016,.T.);
#54708=ORIENTED_EDGE('',*,*,#39297,.F.);
#54709=ORIENTED_EDGE('',*,*,#39298,.F.);
#54710=ORIENTED_EDGE('',*,*,#39299,.F.);
#54711=ORIENTED_EDGE('',*,*,#39300,.F.);
#54712=ORIENTED_EDGE('',*,*,#39295,.F.);
#54713=ORIENTED_EDGE('',*,*,#39300,.T.);
#54714=ORIENTED_EDGE('',*,*,#39301,.F.);
#54715=ORIENTED_EDGE('',*,*,#39017,.T.);
#54716=ORIENTED_EDGE('',*,*,#39296,.T.);
#54717=ORIENTED_EDGE('',*,*,#39302,.F.);
#54718=ORIENTED_EDGE('',*,*,#39303,.F.);
#54719=ORIENTED_EDGE('',*,*,#39107,.F.);
#54720=ORIENTED_EDGE('',*,*,#39304,.F.);
#54721=ORIENTED_EDGE('',*,*,#39304,.T.);
#54722=ORIENTED_EDGE('',*,*,#39109,.T.);
#54723=ORIENTED_EDGE('',*,*,#39019,.T.);
#54724=ORIENTED_EDGE('',*,*,#39305,.F.);
#54725=ORIENTED_EDGE('',*,*,#39020,.T.);
#54726=ORIENTED_EDGE('',*,*,#39306,.F.);
#54727=ORIENTED_EDGE('',*,*,#39307,.T.);
#54728=ORIENTED_EDGE('',*,*,#39308,.F.);
#54729=ORIENTED_EDGE('',*,*,#39022,.T.);
#54730=ORIENTED_EDGE('',*,*,#39309,.F.);
#54731=ORIENTED_EDGE('',*,*,#39310,.T.);
#54732=ORIENTED_EDGE('',*,*,#39311,.F.);
#54733=ORIENTED_EDGE('',*,*,#39023,.T.);
#54734=ORIENTED_EDGE('',*,*,#39311,.T.);
#54735=ORIENTED_EDGE('',*,*,#39312,.T.);
#54736=ORIENTED_EDGE('',*,*,#39313,.F.);
#54737=ORIENTED_EDGE('',*,*,#39312,.F.);
#54738=ORIENTED_EDGE('',*,*,#39310,.F.);
#54739=ORIENTED_EDGE('',*,*,#39314,.F.);
#54740=ORIENTED_EDGE('',*,*,#39315,.F.);
#54741=ORIENTED_EDGE('',*,*,#39025,.T.);
#54742=ORIENTED_EDGE('',*,*,#39316,.F.);
#54743=ORIENTED_EDGE('',*,*,#39317,.T.);
#54744=ORIENTED_EDGE('',*,*,#39318,.F.);
#54745=ORIENTED_EDGE('',*,*,#39026,.T.);
#54746=ORIENTED_EDGE('',*,*,#39318,.T.);
#54747=ORIENTED_EDGE('',*,*,#39319,.T.);
#54748=ORIENTED_EDGE('',*,*,#39320,.F.);
#54749=ORIENTED_EDGE('',*,*,#39319,.F.);
#54750=ORIENTED_EDGE('',*,*,#39317,.F.);
#54751=ORIENTED_EDGE('',*,*,#39321,.F.);
#54752=ORIENTED_EDGE('',*,*,#39322,.F.);
#54753=ORIENTED_EDGE('',*,*,#39028,.T.);
#54754=ORIENTED_EDGE('',*,*,#39323,.F.);
#54755=ORIENTED_EDGE('',*,*,#39324,.T.);
#54756=ORIENTED_EDGE('',*,*,#39325,.F.);
#54757=ORIENTED_EDGE('',*,*,#39029,.T.);
#54758=ORIENTED_EDGE('',*,*,#39325,.T.);
#54759=ORIENTED_EDGE('',*,*,#39326,.T.);
#54760=ORIENTED_EDGE('',*,*,#39327,.F.);
#54761=ORIENTED_EDGE('',*,*,#39326,.F.);
#54762=ORIENTED_EDGE('',*,*,#39324,.F.);
#54763=ORIENTED_EDGE('',*,*,#39328,.F.);
#54764=ORIENTED_EDGE('',*,*,#39329,.F.);
#54765=ORIENTED_EDGE('',*,*,#39031,.T.);
#54766=ORIENTED_EDGE('',*,*,#39330,.F.);
#54767=ORIENTED_EDGE('',*,*,#39331,.T.);
#54768=ORIENTED_EDGE('',*,*,#39332,.F.);
#54769=ORIENTED_EDGE('',*,*,#39032,.T.);
#54770=ORIENTED_EDGE('',*,*,#39332,.T.);
#54771=ORIENTED_EDGE('',*,*,#39333,.T.);
#54772=ORIENTED_EDGE('',*,*,#39334,.F.);
#54773=ORIENTED_EDGE('',*,*,#39333,.F.);
#54774=ORIENTED_EDGE('',*,*,#39331,.F.);
#54775=ORIENTED_EDGE('',*,*,#39335,.F.);
#54776=ORIENTED_EDGE('',*,*,#39336,.F.);
#54777=ORIENTED_EDGE('',*,*,#39034,.T.);
#54778=ORIENTED_EDGE('',*,*,#39337,.F.);
#54779=ORIENTED_EDGE('',*,*,#39338,.T.);
#54780=ORIENTED_EDGE('',*,*,#39339,.F.);
#54781=ORIENTED_EDGE('',*,*,#39035,.T.);
#54782=ORIENTED_EDGE('',*,*,#39339,.T.);
#54783=ORIENTED_EDGE('',*,*,#39340,.T.);
#54784=ORIENTED_EDGE('',*,*,#39341,.F.);
#54785=ORIENTED_EDGE('',*,*,#39340,.F.);
#54786=ORIENTED_EDGE('',*,*,#39338,.F.);
#54787=ORIENTED_EDGE('',*,*,#39342,.F.);
#54788=ORIENTED_EDGE('',*,*,#39343,.F.);
#54789=ORIENTED_EDGE('',*,*,#39037,.T.);
#54790=ORIENTED_EDGE('',*,*,#39344,.F.);
#54791=ORIENTED_EDGE('',*,*,#39345,.T.);
#54792=ORIENTED_EDGE('',*,*,#39346,.F.);
#54793=ORIENTED_EDGE('',*,*,#39038,.T.);
#54794=ORIENTED_EDGE('',*,*,#39346,.T.);
#54795=ORIENTED_EDGE('',*,*,#39347,.T.);
#54796=ORIENTED_EDGE('',*,*,#39348,.F.);
#54797=ORIENTED_EDGE('',*,*,#39347,.F.);
#54798=ORIENTED_EDGE('',*,*,#39345,.F.);
#54799=ORIENTED_EDGE('',*,*,#39349,.F.);
#54800=ORIENTED_EDGE('',*,*,#39350,.F.);
#54801=ORIENTED_EDGE('',*,*,#39040,.T.);
#54802=ORIENTED_EDGE('',*,*,#39351,.F.);
#54803=ORIENTED_EDGE('',*,*,#39352,.T.);
#54804=ORIENTED_EDGE('',*,*,#39353,.F.);
#54805=ORIENTED_EDGE('',*,*,#39041,.T.);
#54806=ORIENTED_EDGE('',*,*,#39353,.T.);
#54807=ORIENTED_EDGE('',*,*,#39354,.T.);
#54808=ORIENTED_EDGE('',*,*,#39355,.F.);
#54809=ORIENTED_EDGE('',*,*,#39354,.F.);
#54810=ORIENTED_EDGE('',*,*,#39352,.F.);
#54811=ORIENTED_EDGE('',*,*,#39356,.F.);
#54812=ORIENTED_EDGE('',*,*,#39357,.F.);
#54813=ORIENTED_EDGE('',*,*,#39043,.T.);
#54814=ORIENTED_EDGE('',*,*,#39358,.F.);
#54815=ORIENTED_EDGE('',*,*,#39359,.T.);
#54816=ORIENTED_EDGE('',*,*,#39360,.F.);
#54817=ORIENTED_EDGE('',*,*,#39044,.T.);
#54818=ORIENTED_EDGE('',*,*,#39360,.T.);
#54819=ORIENTED_EDGE('',*,*,#39361,.T.);
#54820=ORIENTED_EDGE('',*,*,#39362,.F.);
#54821=ORIENTED_EDGE('',*,*,#39361,.F.);
#54822=ORIENTED_EDGE('',*,*,#39359,.F.);
#54823=ORIENTED_EDGE('',*,*,#39363,.F.);
#54824=ORIENTED_EDGE('',*,*,#39364,.F.);
#54825=ORIENTED_EDGE('',*,*,#39046,.T.);
#54826=ORIENTED_EDGE('',*,*,#39365,.F.);
#54827=ORIENTED_EDGE('',*,*,#39366,.T.);
#54828=ORIENTED_EDGE('',*,*,#39367,.F.);
#54829=ORIENTED_EDGE('',*,*,#39047,.T.);
#54830=ORIENTED_EDGE('',*,*,#39367,.T.);
#54831=ORIENTED_EDGE('',*,*,#39368,.T.);
#54832=ORIENTED_EDGE('',*,*,#39369,.F.);
#54833=ORIENTED_EDGE('',*,*,#39368,.F.);
#54834=ORIENTED_EDGE('',*,*,#39366,.F.);
#54835=ORIENTED_EDGE('',*,*,#39370,.F.);
#54836=ORIENTED_EDGE('',*,*,#39371,.F.);
#54837=ORIENTED_EDGE('',*,*,#39049,.T.);
#54838=ORIENTED_EDGE('',*,*,#39372,.F.);
#54839=ORIENTED_EDGE('',*,*,#39373,.T.);
#54840=ORIENTED_EDGE('',*,*,#39374,.F.);
#54841=ORIENTED_EDGE('',*,*,#39050,.T.);
#54842=ORIENTED_EDGE('',*,*,#39374,.T.);
#54843=ORIENTED_EDGE('',*,*,#39375,.T.);
#54844=ORIENTED_EDGE('',*,*,#39376,.F.);
#54845=ORIENTED_EDGE('',*,*,#39375,.F.);
#54846=ORIENTED_EDGE('',*,*,#39373,.F.);
#54847=ORIENTED_EDGE('',*,*,#39377,.F.);
#54848=ORIENTED_EDGE('',*,*,#39378,.F.);
#54849=ORIENTED_EDGE('',*,*,#39052,.T.);
#54850=ORIENTED_EDGE('',*,*,#39379,.F.);
#54851=ORIENTED_EDGE('',*,*,#39380,.T.);
#54852=ORIENTED_EDGE('',*,*,#39381,.F.);
#54853=ORIENTED_EDGE('',*,*,#39053,.T.);
#54854=ORIENTED_EDGE('',*,*,#39381,.T.);
#54855=ORIENTED_EDGE('',*,*,#39382,.T.);
#54856=ORIENTED_EDGE('',*,*,#39383,.F.);
#54857=ORIENTED_EDGE('',*,*,#39382,.F.);
#54858=ORIENTED_EDGE('',*,*,#39380,.F.);
#54859=ORIENTED_EDGE('',*,*,#39384,.F.);
#54860=ORIENTED_EDGE('',*,*,#39385,.F.);
#54861=ORIENTED_EDGE('',*,*,#39055,.T.);
#54862=ORIENTED_EDGE('',*,*,#39386,.F.);
#54863=ORIENTED_EDGE('',*,*,#39387,.T.);
#54864=ORIENTED_EDGE('',*,*,#39388,.F.);
#54865=ORIENTED_EDGE('',*,*,#39056,.T.);
#54866=ORIENTED_EDGE('',*,*,#39388,.T.);
#54867=ORIENTED_EDGE('',*,*,#39389,.T.);
#54868=ORIENTED_EDGE('',*,*,#39390,.F.);
#54869=ORIENTED_EDGE('',*,*,#39389,.F.);
#54870=ORIENTED_EDGE('',*,*,#39387,.F.);
#54871=ORIENTED_EDGE('',*,*,#39391,.F.);
#54872=ORIENTED_EDGE('',*,*,#39392,.F.);
#54873=ORIENTED_EDGE('',*,*,#39058,.T.);
#54874=ORIENTED_EDGE('',*,*,#39393,.F.);
#54875=ORIENTED_EDGE('',*,*,#39394,.T.);
#54876=ORIENTED_EDGE('',*,*,#39395,.F.);
#54877=ORIENTED_EDGE('',*,*,#39059,.T.);
#54878=ORIENTED_EDGE('',*,*,#39395,.T.);
#54879=ORIENTED_EDGE('',*,*,#39396,.T.);
#54880=ORIENTED_EDGE('',*,*,#39397,.F.);
#54881=ORIENTED_EDGE('',*,*,#39396,.F.);
#54882=ORIENTED_EDGE('',*,*,#39394,.F.);
#54883=ORIENTED_EDGE('',*,*,#39398,.F.);
#54884=ORIENTED_EDGE('',*,*,#39399,.F.);
#54885=ORIENTED_EDGE('',*,*,#39061,.T.);
#54886=ORIENTED_EDGE('',*,*,#39400,.F.);
#54887=ORIENTED_EDGE('',*,*,#34403,.T.);
#54888=ORIENTED_EDGE('',*,*,#39401,.F.);
#54889=ORIENTED_EDGE('',*,*,#39062,.T.);
#54890=ORIENTED_EDGE('',*,*,#39401,.T.);
#54891=ORIENTED_EDGE('',*,*,#34402,.T.);
#54892=ORIENTED_EDGE('',*,*,#39402,.F.);
#54893=ORIENTED_EDGE('',*,*,#39064,.T.);
#54894=ORIENTED_EDGE('',*,*,#39403,.F.);
#54895=ORIENTED_EDGE('',*,*,#39404,.T.);
#54896=ORIENTED_EDGE('',*,*,#39405,.F.);
#54897=ORIENTED_EDGE('',*,*,#39065,.T.);
#54898=ORIENTED_EDGE('',*,*,#39405,.T.);
#54899=ORIENTED_EDGE('',*,*,#39406,.T.);
#54900=ORIENTED_EDGE('',*,*,#39407,.F.);
#54901=ORIENTED_EDGE('',*,*,#39406,.F.);
#54902=ORIENTED_EDGE('',*,*,#39404,.F.);
#54903=ORIENTED_EDGE('',*,*,#39408,.F.);
#54904=ORIENTED_EDGE('',*,*,#39409,.F.);
#54905=ORIENTED_EDGE('',*,*,#39067,.T.);
#54906=ORIENTED_EDGE('',*,*,#39410,.F.);
#54907=ORIENTED_EDGE('',*,*,#39411,.T.);
#54908=ORIENTED_EDGE('',*,*,#39412,.F.);
#54909=ORIENTED_EDGE('',*,*,#39068,.T.);
#54910=ORIENTED_EDGE('',*,*,#39412,.T.);
#54911=ORIENTED_EDGE('',*,*,#39413,.T.);
#54912=ORIENTED_EDGE('',*,*,#39414,.F.);
#54913=ORIENTED_EDGE('',*,*,#39413,.F.);
#54914=ORIENTED_EDGE('',*,*,#39411,.F.);
#54915=ORIENTED_EDGE('',*,*,#39415,.F.);
#54916=ORIENTED_EDGE('',*,*,#39416,.F.);
#54917=ORIENTED_EDGE('',*,*,#39070,.T.);
#54918=ORIENTED_EDGE('',*,*,#39417,.F.);
#54919=ORIENTED_EDGE('',*,*,#39418,.T.);
#54920=ORIENTED_EDGE('',*,*,#39419,.F.);
#54921=ORIENTED_EDGE('',*,*,#39071,.T.);
#54922=ORIENTED_EDGE('',*,*,#39419,.T.);
#54923=ORIENTED_EDGE('',*,*,#39420,.T.);
#54924=ORIENTED_EDGE('',*,*,#39421,.F.);
#54925=ORIENTED_EDGE('',*,*,#39420,.F.);
#54926=ORIENTED_EDGE('',*,*,#39418,.F.);
#54927=ORIENTED_EDGE('',*,*,#39422,.F.);
#54928=ORIENTED_EDGE('',*,*,#39423,.F.);
#54929=ORIENTED_EDGE('',*,*,#39073,.T.);
#54930=ORIENTED_EDGE('',*,*,#39424,.F.);
#54931=ORIENTED_EDGE('',*,*,#39425,.T.);
#54932=ORIENTED_EDGE('',*,*,#39426,.F.);
#54933=ORIENTED_EDGE('',*,*,#39074,.T.);
#54934=ORIENTED_EDGE('',*,*,#39426,.T.);
#54935=ORIENTED_EDGE('',*,*,#39427,.T.);
#54936=ORIENTED_EDGE('',*,*,#39428,.F.);
#54937=ORIENTED_EDGE('',*,*,#39427,.F.);
#54938=ORIENTED_EDGE('',*,*,#39425,.F.);
#54939=ORIENTED_EDGE('',*,*,#39429,.F.);
#54940=ORIENTED_EDGE('',*,*,#39430,.F.);
#54941=ORIENTED_EDGE('',*,*,#39076,.T.);
#54942=ORIENTED_EDGE('',*,*,#39431,.F.);
#54943=ORIENTED_EDGE('',*,*,#39432,.T.);
#54944=ORIENTED_EDGE('',*,*,#39433,.F.);
#54945=ORIENTED_EDGE('',*,*,#39077,.T.);
#54946=ORIENTED_EDGE('',*,*,#39433,.T.);
#54947=ORIENTED_EDGE('',*,*,#39434,.T.);
#54948=ORIENTED_EDGE('',*,*,#39435,.F.);
#54949=ORIENTED_EDGE('',*,*,#39434,.F.);
#54950=ORIENTED_EDGE('',*,*,#39432,.F.);
#54951=ORIENTED_EDGE('',*,*,#39436,.F.);
#54952=ORIENTED_EDGE('',*,*,#39437,.F.);
#54953=ORIENTED_EDGE('',*,*,#39079,.T.);
#54954=ORIENTED_EDGE('',*,*,#39438,.F.);
#54955=ORIENTED_EDGE('',*,*,#39439,.T.);
#54956=ORIENTED_EDGE('',*,*,#39440,.F.);
#54957=ORIENTED_EDGE('',*,*,#39080,.T.);
#54958=ORIENTED_EDGE('',*,*,#39440,.T.);
#54959=ORIENTED_EDGE('',*,*,#39441,.T.);
#54960=ORIENTED_EDGE('',*,*,#39442,.F.);
#54961=ORIENTED_EDGE('',*,*,#39441,.F.);
#54962=ORIENTED_EDGE('',*,*,#39439,.F.);
#54963=ORIENTED_EDGE('',*,*,#39443,.F.);
#54964=ORIENTED_EDGE('',*,*,#39444,.F.);
#54965=ORIENTED_EDGE('',*,*,#39082,.T.);
#54966=ORIENTED_EDGE('',*,*,#39445,.F.);
#54967=ORIENTED_EDGE('',*,*,#39446,.T.);
#54968=ORIENTED_EDGE('',*,*,#39447,.F.);
#54969=ORIENTED_EDGE('',*,*,#39083,.T.);
#54970=ORIENTED_EDGE('',*,*,#39447,.T.);
#54971=ORIENTED_EDGE('',*,*,#39448,.T.);
#54972=ORIENTED_EDGE('',*,*,#39449,.F.);
#54973=ORIENTED_EDGE('',*,*,#39448,.F.);
#54974=ORIENTED_EDGE('',*,*,#39446,.F.);
#54975=ORIENTED_EDGE('',*,*,#39450,.F.);
#54976=ORIENTED_EDGE('',*,*,#39451,.F.);
#54977=ORIENTED_EDGE('',*,*,#39085,.T.);
#54978=ORIENTED_EDGE('',*,*,#39452,.F.);
#54979=ORIENTED_EDGE('',*,*,#39453,.T.);
#54980=ORIENTED_EDGE('',*,*,#39454,.F.);
#54981=ORIENTED_EDGE('',*,*,#39086,.T.);
#54982=ORIENTED_EDGE('',*,*,#39454,.T.);
#54983=ORIENTED_EDGE('',*,*,#39455,.T.);
#54984=ORIENTED_EDGE('',*,*,#39456,.F.);
#54985=ORIENTED_EDGE('',*,*,#39455,.F.);
#54986=ORIENTED_EDGE('',*,*,#39453,.F.);
#54987=ORIENTED_EDGE('',*,*,#39457,.F.);
#54988=ORIENTED_EDGE('',*,*,#39458,.F.);
#54989=ORIENTED_EDGE('',*,*,#39088,.T.);
#54990=ORIENTED_EDGE('',*,*,#39459,.F.);
#54991=ORIENTED_EDGE('',*,*,#39460,.T.);
#54992=ORIENTED_EDGE('',*,*,#39461,.F.);
#54993=ORIENTED_EDGE('',*,*,#39089,.T.);
#54994=ORIENTED_EDGE('',*,*,#39461,.T.);
#54995=ORIENTED_EDGE('',*,*,#39462,.T.);
#54996=ORIENTED_EDGE('',*,*,#39463,.F.);
#54997=ORIENTED_EDGE('',*,*,#39462,.F.);
#54998=ORIENTED_EDGE('',*,*,#39460,.F.);
#54999=ORIENTED_EDGE('',*,*,#39464,.F.);
#55000=ORIENTED_EDGE('',*,*,#39465,.F.);
#55001=ORIENTED_EDGE('',*,*,#39091,.T.);
#55002=ORIENTED_EDGE('',*,*,#39466,.F.);
#55003=ORIENTED_EDGE('',*,*,#39467,.T.);
#55004=ORIENTED_EDGE('',*,*,#39468,.F.);
#55005=ORIENTED_EDGE('',*,*,#39092,.T.);
#55006=ORIENTED_EDGE('',*,*,#39468,.T.);
#55007=ORIENTED_EDGE('',*,*,#39469,.T.);
#55008=ORIENTED_EDGE('',*,*,#39470,.F.);
#55009=ORIENTED_EDGE('',*,*,#39469,.F.);
#55010=ORIENTED_EDGE('',*,*,#39467,.F.);
#55011=ORIENTED_EDGE('',*,*,#39471,.F.);
#55012=ORIENTED_EDGE('',*,*,#39472,.F.);
#55013=ORIENTED_EDGE('',*,*,#39094,.T.);
#55014=ORIENTED_EDGE('',*,*,#39473,.F.);
#55015=ORIENTED_EDGE('',*,*,#39474,.T.);
#55016=ORIENTED_EDGE('',*,*,#39475,.F.);
#55017=ORIENTED_EDGE('',*,*,#39095,.T.);
#55018=ORIENTED_EDGE('',*,*,#39475,.T.);
#55019=ORIENTED_EDGE('',*,*,#39476,.T.);
#55020=ORIENTED_EDGE('',*,*,#39477,.F.);
#55021=ORIENTED_EDGE('',*,*,#39476,.F.);
#55022=ORIENTED_EDGE('',*,*,#39474,.F.);
#55023=ORIENTED_EDGE('',*,*,#39478,.F.);
#55024=ORIENTED_EDGE('',*,*,#39479,.F.);
#55025=ORIENTED_EDGE('',*,*,#39097,.T.);
#55026=ORIENTED_EDGE('',*,*,#39480,.F.);
#55027=ORIENTED_EDGE('',*,*,#39481,.T.);
#55028=ORIENTED_EDGE('',*,*,#39482,.F.);
#55029=ORIENTED_EDGE('',*,*,#39098,.T.);
#55030=ORIENTED_EDGE('',*,*,#39482,.T.);
#55031=ORIENTED_EDGE('',*,*,#39483,.T.);
#55032=ORIENTED_EDGE('',*,*,#39484,.F.);
#55033=ORIENTED_EDGE('',*,*,#39483,.F.);
#55034=ORIENTED_EDGE('',*,*,#39481,.F.);
#55035=ORIENTED_EDGE('',*,*,#39485,.F.);
#55036=ORIENTED_EDGE('',*,*,#39486,.F.);
#55037=ORIENTED_EDGE('',*,*,#39100,.T.);
#55038=ORIENTED_EDGE('',*,*,#39487,.F.);
#55039=ORIENTED_EDGE('',*,*,#39488,.T.);
#55040=ORIENTED_EDGE('',*,*,#39489,.F.);
#55041=ORIENTED_EDGE('',*,*,#39490,.T.);
#55042=ORIENTED_EDGE('',*,*,#39491,.F.);
#55043=ORIENTED_EDGE('',*,*,#39101,.T.);
#55044=ORIENTED_EDGE('',*,*,#39489,.T.);
#55045=ORIENTED_EDGE('',*,*,#39492,.F.);
#55046=ORIENTED_EDGE('',*,*,#39493,.F.);
#55047=ORIENTED_EDGE('',*,*,#39490,.F.);
#55048=ORIENTED_EDGE('',*,*,#39488,.F.);
#55049=ORIENTED_EDGE('',*,*,#39103,.T.);
#55050=ORIENTED_EDGE('',*,*,#39494,.F.);
#55051=ORIENTED_EDGE('',*,*,#39495,.T.);
#55052=ORIENTED_EDGE('',*,*,#39496,.F.);
#55053=ORIENTED_EDGE('',*,*,#39104,.T.);
#55054=ORIENTED_EDGE('',*,*,#39496,.T.);
#55055=ORIENTED_EDGE('',*,*,#39497,.T.);
#55056=ORIENTED_EDGE('',*,*,#39498,.F.);
#55057=ORIENTED_EDGE('',*,*,#39497,.F.);
#55058=ORIENTED_EDGE('',*,*,#39495,.F.);
#55059=ORIENTED_EDGE('',*,*,#39499,.F.);
#55060=ORIENTED_EDGE('',*,*,#39500,.F.);
#55061=ORIENTED_EDGE('',*,*,#39307,.F.);
#55062=ORIENTED_EDGE('',*,*,#39501,.F.);
#55063=ORIENTED_EDGE('',*,*,#39502,.F.);
#55064=ORIENTED_EDGE('',*,*,#39503,.F.);
#55065=ORIENTED_EDGE('',*,*,#39106,.T.);
#55066=ORIENTED_EDGE('',*,*,#39504,.F.);
#55067=ORIENTED_EDGE('',*,*,#39501,.T.);
#55068=ORIENTED_EDGE('',*,*,#39306,.T.);
#55069=ORIENTED_EDGE('',*,*,#39505,.F.);
#55070=ORIENTED_EDGE('',*,*,#39108,.T.);
#55071=ORIENTED_EDGE('',*,*,#39303,.T.);
#55072=ORIENTED_EDGE('',*,*,#39506,.F.);
#55073=ORIENTED_EDGE('',*,*,#39507,.F.);
#55074=ORIENTED_EDGE('',*,*,#39508,.F.);
#55075=ORIENTED_EDGE('',*,*,#39113,.T.);
#55076=ORIENTED_EDGE('',*,*,#39112,.T.);
#55077=ORIENTED_EDGE('',*,*,#39509,.F.);
#55078=ORIENTED_EDGE('',*,*,#39116,.T.);
#55079=ORIENTED_EDGE('',*,*,#39114,.T.);
#55080=ORIENTED_EDGE('',*,*,#39508,.T.);
#55081=ORIENTED_EDGE('',*,*,#39510,.F.);
#55082=ORIENTED_EDGE('',*,*,#39511,.F.);
#55083=ORIENTED_EDGE('',*,*,#39120,.T.);
#55084=ORIENTED_EDGE('',*,*,#39119,.T.);
#55085=ORIENTED_EDGE('',*,*,#39512,.F.);
#55086=ORIENTED_EDGE('',*,*,#39123,.T.);
#55087=ORIENTED_EDGE('',*,*,#39121,.T.);
#55088=ORIENTED_EDGE('',*,*,#39511,.T.);
#55089=ORIENTED_EDGE('',*,*,#39513,.F.);
#55090=ORIENTED_EDGE('',*,*,#39514,.F.);
#55091=ORIENTED_EDGE('',*,*,#39127,.T.);
#55092=ORIENTED_EDGE('',*,*,#39126,.T.);
#55093=ORIENTED_EDGE('',*,*,#39515,.F.);
#55094=ORIENTED_EDGE('',*,*,#39130,.T.);
#55095=ORIENTED_EDGE('',*,*,#39128,.T.);
#55096=ORIENTED_EDGE('',*,*,#39514,.T.);
#55097=ORIENTED_EDGE('',*,*,#39516,.F.);
#55098=ORIENTED_EDGE('',*,*,#39517,.F.);
#55099=ORIENTED_EDGE('',*,*,#39134,.T.);
#55100=ORIENTED_EDGE('',*,*,#39133,.T.);
#55101=ORIENTED_EDGE('',*,*,#39518,.F.);
#55102=ORIENTED_EDGE('',*,*,#39137,.T.);
#55103=ORIENTED_EDGE('',*,*,#39135,.T.);
#55104=ORIENTED_EDGE('',*,*,#39517,.T.);
#55105=ORIENTED_EDGE('',*,*,#39519,.F.);
#55106=ORIENTED_EDGE('',*,*,#39520,.F.);
#55107=ORIENTED_EDGE('',*,*,#39141,.T.);
#55108=ORIENTED_EDGE('',*,*,#39140,.T.);
#55109=ORIENTED_EDGE('',*,*,#39521,.F.);
#55110=ORIENTED_EDGE('',*,*,#39144,.T.);
#55111=ORIENTED_EDGE('',*,*,#39142,.T.);
#55112=ORIENTED_EDGE('',*,*,#39520,.T.);
#55113=ORIENTED_EDGE('',*,*,#39522,.F.);
#55114=ORIENTED_EDGE('',*,*,#39523,.F.);
#55115=ORIENTED_EDGE('',*,*,#39148,.T.);
#55116=ORIENTED_EDGE('',*,*,#39147,.T.);
#55117=ORIENTED_EDGE('',*,*,#39524,.F.);
#55118=ORIENTED_EDGE('',*,*,#39151,.T.);
#55119=ORIENTED_EDGE('',*,*,#39149,.T.);
#55120=ORIENTED_EDGE('',*,*,#39523,.T.);
#55121=ORIENTED_EDGE('',*,*,#39525,.F.);
#55122=ORIENTED_EDGE('',*,*,#39526,.F.);
#55123=ORIENTED_EDGE('',*,*,#34407,.T.);
#55124=ORIENTED_EDGE('',*,*,#39153,.T.);
#55125=ORIENTED_EDGE('',*,*,#39527,.F.);
#55126=ORIENTED_EDGE('',*,*,#39154,.T.);
#55127=ORIENTED_EDGE('',*,*,#34408,.T.);
#55128=ORIENTED_EDGE('',*,*,#39526,.T.);
#55129=ORIENTED_EDGE('',*,*,#39528,.F.);
#55130=ORIENTED_EDGE('',*,*,#39529,.F.);
#55131=ORIENTED_EDGE('',*,*,#39158,.T.);
#55132=ORIENTED_EDGE('',*,*,#39157,.T.);
#55133=ORIENTED_EDGE('',*,*,#39530,.F.);
#55134=ORIENTED_EDGE('',*,*,#39161,.T.);
#55135=ORIENTED_EDGE('',*,*,#39159,.T.);
#55136=ORIENTED_EDGE('',*,*,#39529,.T.);
#55137=ORIENTED_EDGE('',*,*,#39531,.F.);
#55138=ORIENTED_EDGE('',*,*,#39532,.F.);
#55139=ORIENTED_EDGE('',*,*,#39165,.T.);
#55140=ORIENTED_EDGE('',*,*,#39164,.T.);
#55141=ORIENTED_EDGE('',*,*,#39533,.F.);
#55142=ORIENTED_EDGE('',*,*,#39168,.T.);
#55143=ORIENTED_EDGE('',*,*,#39166,.T.);
#55144=ORIENTED_EDGE('',*,*,#39532,.T.);
#55145=ORIENTED_EDGE('',*,*,#39534,.F.);
#55146=ORIENTED_EDGE('',*,*,#39535,.F.);
#55147=ORIENTED_EDGE('',*,*,#39172,.T.);
#55148=ORIENTED_EDGE('',*,*,#39171,.T.);
#55149=ORIENTED_EDGE('',*,*,#39536,.F.);
#55150=ORIENTED_EDGE('',*,*,#39175,.T.);
#55151=ORIENTED_EDGE('',*,*,#39173,.T.);
#55152=ORIENTED_EDGE('',*,*,#39535,.T.);
#55153=ORIENTED_EDGE('',*,*,#39537,.F.);
#55154=ORIENTED_EDGE('',*,*,#39538,.F.);
#55155=ORIENTED_EDGE('',*,*,#39179,.T.);
#55156=ORIENTED_EDGE('',*,*,#39178,.T.);
#55157=ORIENTED_EDGE('',*,*,#39539,.F.);
#55158=ORIENTED_EDGE('',*,*,#39182,.T.);
#55159=ORIENTED_EDGE('',*,*,#39180,.T.);
#55160=ORIENTED_EDGE('',*,*,#39538,.T.);
#55161=ORIENTED_EDGE('',*,*,#39540,.F.);
#55162=ORIENTED_EDGE('',*,*,#39541,.F.);
#55163=ORIENTED_EDGE('',*,*,#39186,.T.);
#55164=ORIENTED_EDGE('',*,*,#39185,.T.);
#55165=ORIENTED_EDGE('',*,*,#39542,.F.);
#55166=ORIENTED_EDGE('',*,*,#39189,.T.);
#55167=ORIENTED_EDGE('',*,*,#39187,.T.);
#55168=ORIENTED_EDGE('',*,*,#39541,.T.);
#55169=ORIENTED_EDGE('',*,*,#39543,.F.);
#55170=ORIENTED_EDGE('',*,*,#39544,.F.);
#55171=ORIENTED_EDGE('',*,*,#39193,.T.);
#55172=ORIENTED_EDGE('',*,*,#39192,.T.);
#55173=ORIENTED_EDGE('',*,*,#39545,.F.);
#55174=ORIENTED_EDGE('',*,*,#39196,.T.);
#55175=ORIENTED_EDGE('',*,*,#39194,.T.);
#55176=ORIENTED_EDGE('',*,*,#39544,.T.);
#55177=ORIENTED_EDGE('',*,*,#39546,.F.);
#55178=ORIENTED_EDGE('',*,*,#39547,.F.);
#55179=ORIENTED_EDGE('',*,*,#39200,.T.);
#55180=ORIENTED_EDGE('',*,*,#39199,.T.);
#55181=ORIENTED_EDGE('',*,*,#39548,.F.);
#55182=ORIENTED_EDGE('',*,*,#39203,.T.);
#55183=ORIENTED_EDGE('',*,*,#39201,.T.);
#55184=ORIENTED_EDGE('',*,*,#39547,.T.);
#55185=ORIENTED_EDGE('',*,*,#39549,.F.);
#55186=ORIENTED_EDGE('',*,*,#39550,.F.);
#55187=ORIENTED_EDGE('',*,*,#39207,.T.);
#55188=ORIENTED_EDGE('',*,*,#39206,.T.);
#55189=ORIENTED_EDGE('',*,*,#39551,.F.);
#55190=ORIENTED_EDGE('',*,*,#39210,.T.);
#55191=ORIENTED_EDGE('',*,*,#39208,.T.);
#55192=ORIENTED_EDGE('',*,*,#39550,.T.);
#55193=ORIENTED_EDGE('',*,*,#39552,.F.);
#55194=ORIENTED_EDGE('',*,*,#39553,.F.);
#55195=ORIENTED_EDGE('',*,*,#39214,.T.);
#55196=ORIENTED_EDGE('',*,*,#39213,.T.);
#55197=ORIENTED_EDGE('',*,*,#39554,.F.);
#55198=ORIENTED_EDGE('',*,*,#39217,.T.);
#55199=ORIENTED_EDGE('',*,*,#39215,.T.);
#55200=ORIENTED_EDGE('',*,*,#39553,.T.);
#55201=ORIENTED_EDGE('',*,*,#39555,.F.);
#55202=ORIENTED_EDGE('',*,*,#39556,.F.);
#55203=ORIENTED_EDGE('',*,*,#39221,.T.);
#55204=ORIENTED_EDGE('',*,*,#39220,.T.);
#55205=ORIENTED_EDGE('',*,*,#39557,.F.);
#55206=ORIENTED_EDGE('',*,*,#39224,.T.);
#55207=ORIENTED_EDGE('',*,*,#39222,.T.);
#55208=ORIENTED_EDGE('',*,*,#39556,.T.);
#55209=ORIENTED_EDGE('',*,*,#39558,.F.);
#55210=ORIENTED_EDGE('',*,*,#39559,.F.);
#55211=ORIENTED_EDGE('',*,*,#39228,.T.);
#55212=ORIENTED_EDGE('',*,*,#39227,.T.);
#55213=ORIENTED_EDGE('',*,*,#39560,.F.);
#55214=ORIENTED_EDGE('',*,*,#39231,.T.);
#55215=ORIENTED_EDGE('',*,*,#39229,.T.);
#55216=ORIENTED_EDGE('',*,*,#39559,.T.);
#55217=ORIENTED_EDGE('',*,*,#39561,.F.);
#55218=ORIENTED_EDGE('',*,*,#39562,.F.);
#55219=ORIENTED_EDGE('',*,*,#39235,.T.);
#55220=ORIENTED_EDGE('',*,*,#39234,.T.);
#55221=ORIENTED_EDGE('',*,*,#39563,.F.);
#55222=ORIENTED_EDGE('',*,*,#39238,.T.);
#55223=ORIENTED_EDGE('',*,*,#39236,.T.);
#55224=ORIENTED_EDGE('',*,*,#39562,.T.);
#55225=ORIENTED_EDGE('',*,*,#39564,.F.);
#55226=ORIENTED_EDGE('',*,*,#39565,.F.);
#55227=ORIENTED_EDGE('',*,*,#39242,.T.);
#55228=ORIENTED_EDGE('',*,*,#39241,.T.);
#55229=ORIENTED_EDGE('',*,*,#39566,.F.);
#55230=ORIENTED_EDGE('',*,*,#39245,.T.);
#55231=ORIENTED_EDGE('',*,*,#39243,.T.);
#55232=ORIENTED_EDGE('',*,*,#39565,.T.);
#55233=ORIENTED_EDGE('',*,*,#39567,.F.);
#55234=ORIENTED_EDGE('',*,*,#39568,.F.);
#55235=ORIENTED_EDGE('',*,*,#39251,.T.);
#55236=ORIENTED_EDGE('',*,*,#39248,.T.);
#55237=ORIENTED_EDGE('',*,*,#39252,.T.);
#55238=ORIENTED_EDGE('',*,*,#39568,.T.);
#55239=ORIENTED_EDGE('',*,*,#39569,.F.);
#55240=ORIENTED_EDGE('',*,*,#39250,.T.);
#55241=ORIENTED_EDGE('',*,*,#39257,.T.);
#55242=ORIENTED_EDGE('',*,*,#39253,.T.);
#55243=ORIENTED_EDGE('',*,*,#39570,.F.);
#55244=ORIENTED_EDGE('',*,*,#39571,.F.);
#55245=ORIENTED_EDGE('',*,*,#39572,.F.);
#55246=ORIENTED_EDGE('',*,*,#39259,.T.);
#55247=ORIENTED_EDGE('',*,*,#39258,.T.);
#55248=ORIENTED_EDGE('',*,*,#39571,.T.);
#55249=ORIENTED_EDGE('',*,*,#39573,.F.);
#55250=ORIENTED_EDGE('',*,*,#39574,.F.);
#55251=ORIENTED_EDGE('',*,*,#39263,.T.);
#55252=ORIENTED_EDGE('',*,*,#39262,.T.);
#55253=ORIENTED_EDGE('',*,*,#39575,.F.);
#55254=ORIENTED_EDGE('',*,*,#39266,.T.);
#55255=ORIENTED_EDGE('',*,*,#39264,.T.);
#55256=ORIENTED_EDGE('',*,*,#39574,.T.);
#55257=ORIENTED_EDGE('',*,*,#39576,.F.);
#55258=ORIENTED_EDGE('',*,*,#39577,.F.);
#55259=ORIENTED_EDGE('',*,*,#39270,.T.);
#55260=ORIENTED_EDGE('',*,*,#39269,.T.);
#55261=ORIENTED_EDGE('',*,*,#39578,.F.);
#55262=ORIENTED_EDGE('',*,*,#39273,.T.);
#55263=ORIENTED_EDGE('',*,*,#39271,.T.);
#55264=ORIENTED_EDGE('',*,*,#39577,.T.);
#55265=ORIENTED_EDGE('',*,*,#39579,.F.);
#55266=ORIENTED_EDGE('',*,*,#39580,.F.);
#55267=ORIENTED_EDGE('',*,*,#39277,.T.);
#55268=ORIENTED_EDGE('',*,*,#39276,.T.);
#55269=ORIENTED_EDGE('',*,*,#39581,.F.);
#55270=ORIENTED_EDGE('',*,*,#39280,.T.);
#55271=ORIENTED_EDGE('',*,*,#39278,.T.);
#55272=ORIENTED_EDGE('',*,*,#39580,.T.);
#55273=ORIENTED_EDGE('',*,*,#39582,.F.);
#55274=ORIENTED_EDGE('',*,*,#39583,.F.);
#55275=ORIENTED_EDGE('',*,*,#39284,.T.);
#55276=ORIENTED_EDGE('',*,*,#39283,.T.);
#55277=ORIENTED_EDGE('',*,*,#39584,.F.);
#55278=ORIENTED_EDGE('',*,*,#39287,.T.);
#55279=ORIENTED_EDGE('',*,*,#39285,.T.);
#55280=ORIENTED_EDGE('',*,*,#39583,.T.);
#55281=ORIENTED_EDGE('',*,*,#39585,.F.);
#55282=ORIENTED_EDGE('',*,*,#39586,.F.);
#55283=ORIENTED_EDGE('',*,*,#39291,.T.);
#55284=ORIENTED_EDGE('',*,*,#39290,.T.);
#55285=ORIENTED_EDGE('',*,*,#39587,.F.);
#55286=ORIENTED_EDGE('',*,*,#39294,.T.);
#55287=ORIENTED_EDGE('',*,*,#39292,.T.);
#55288=ORIENTED_EDGE('',*,*,#39586,.T.);
#55289=ORIENTED_EDGE('',*,*,#39588,.F.);
#55290=ORIENTED_EDGE('',*,*,#39589,.F.);
#55291=ORIENTED_EDGE('',*,*,#39298,.T.);
#55292=ORIENTED_EDGE('',*,*,#39297,.T.);
#55293=ORIENTED_EDGE('',*,*,#39590,.F.);
#55294=ORIENTED_EDGE('',*,*,#39301,.T.);
#55295=ORIENTED_EDGE('',*,*,#39299,.T.);
#55296=ORIENTED_EDGE('',*,*,#39589,.T.);
#55297=ORIENTED_EDGE('',*,*,#39591,.F.);
#55298=ORIENTED_EDGE('',*,*,#39506,.T.);
#55299=ORIENTED_EDGE('',*,*,#39302,.T.);
#55300=ORIENTED_EDGE('',*,*,#39305,.T.);
#55301=ORIENTED_EDGE('',*,*,#39503,.T.);
#55302=ORIENTED_EDGE('',*,*,#39592,.F.);
#55303=ORIENTED_EDGE('',*,*,#39593,.F.);
#55304=ORIENTED_EDGE('',*,*,#39308,.T.);
#55305=ORIENTED_EDGE('',*,*,#39314,.T.);
#55306=ORIENTED_EDGE('',*,*,#39309,.T.);
#55307=ORIENTED_EDGE('',*,*,#39594,.F.);
#55308=ORIENTED_EDGE('',*,*,#39595,.F.);
#55309=ORIENTED_EDGE('',*,*,#39315,.T.);
#55310=ORIENTED_EDGE('',*,*,#39595,.T.);
#55311=ORIENTED_EDGE('',*,*,#39596,.F.);
#55312=ORIENTED_EDGE('',*,*,#39313,.T.);
#55313=ORIENTED_EDGE('',*,*,#39321,.T.);
#55314=ORIENTED_EDGE('',*,*,#39316,.T.);
#55315=ORIENTED_EDGE('',*,*,#39597,.F.);
#55316=ORIENTED_EDGE('',*,*,#39598,.F.);
#55317=ORIENTED_EDGE('',*,*,#39322,.T.);
#55318=ORIENTED_EDGE('',*,*,#39598,.T.);
#55319=ORIENTED_EDGE('',*,*,#39599,.F.);
#55320=ORIENTED_EDGE('',*,*,#39320,.T.);
#55321=ORIENTED_EDGE('',*,*,#39328,.T.);
#55322=ORIENTED_EDGE('',*,*,#39323,.T.);
#55323=ORIENTED_EDGE('',*,*,#39600,.F.);
#55324=ORIENTED_EDGE('',*,*,#39601,.F.);
#55325=ORIENTED_EDGE('',*,*,#39329,.T.);
#55326=ORIENTED_EDGE('',*,*,#39601,.T.);
#55327=ORIENTED_EDGE('',*,*,#39602,.F.);
#55328=ORIENTED_EDGE('',*,*,#39327,.T.);
#55329=ORIENTED_EDGE('',*,*,#39335,.T.);
#55330=ORIENTED_EDGE('',*,*,#39330,.T.);
#55331=ORIENTED_EDGE('',*,*,#39603,.F.);
#55332=ORIENTED_EDGE('',*,*,#39604,.F.);
#55333=ORIENTED_EDGE('',*,*,#39336,.T.);
#55334=ORIENTED_EDGE('',*,*,#39604,.T.);
#55335=ORIENTED_EDGE('',*,*,#39605,.F.);
#55336=ORIENTED_EDGE('',*,*,#39334,.T.);
#55337=ORIENTED_EDGE('',*,*,#39342,.T.);
#55338=ORIENTED_EDGE('',*,*,#39337,.T.);
#55339=ORIENTED_EDGE('',*,*,#39606,.F.);
#55340=ORIENTED_EDGE('',*,*,#39607,.F.);
#55341=ORIENTED_EDGE('',*,*,#39343,.T.);
#55342=ORIENTED_EDGE('',*,*,#39607,.T.);
#55343=ORIENTED_EDGE('',*,*,#39608,.F.);
#55344=ORIENTED_EDGE('',*,*,#39341,.T.);
#55345=ORIENTED_EDGE('',*,*,#39349,.T.);
#55346=ORIENTED_EDGE('',*,*,#39344,.T.);
#55347=ORIENTED_EDGE('',*,*,#39609,.F.);
#55348=ORIENTED_EDGE('',*,*,#39610,.F.);
#55349=ORIENTED_EDGE('',*,*,#39350,.T.);
#55350=ORIENTED_EDGE('',*,*,#39610,.T.);
#55351=ORIENTED_EDGE('',*,*,#39611,.F.);
#55352=ORIENTED_EDGE('',*,*,#39348,.T.);
#55353=ORIENTED_EDGE('',*,*,#39356,.T.);
#55354=ORIENTED_EDGE('',*,*,#39351,.T.);
#55355=ORIENTED_EDGE('',*,*,#39612,.F.);
#55356=ORIENTED_EDGE('',*,*,#39613,.F.);
#55357=ORIENTED_EDGE('',*,*,#39357,.T.);
#55358=ORIENTED_EDGE('',*,*,#39613,.T.);
#55359=ORIENTED_EDGE('',*,*,#39614,.F.);
#55360=ORIENTED_EDGE('',*,*,#39355,.T.);
#55361=ORIENTED_EDGE('',*,*,#39363,.T.);
#55362=ORIENTED_EDGE('',*,*,#39358,.T.);
#55363=ORIENTED_EDGE('',*,*,#39615,.F.);
#55364=ORIENTED_EDGE('',*,*,#39616,.F.);
#55365=ORIENTED_EDGE('',*,*,#39364,.T.);
#55366=ORIENTED_EDGE('',*,*,#39616,.T.);
#55367=ORIENTED_EDGE('',*,*,#39617,.F.);
#55368=ORIENTED_EDGE('',*,*,#39362,.T.);
#55369=ORIENTED_EDGE('',*,*,#39370,.T.);
#55370=ORIENTED_EDGE('',*,*,#39365,.T.);
#55371=ORIENTED_EDGE('',*,*,#39618,.F.);
#55372=ORIENTED_EDGE('',*,*,#39619,.F.);
#55373=ORIENTED_EDGE('',*,*,#39371,.T.);
#55374=ORIENTED_EDGE('',*,*,#39619,.T.);
#55375=ORIENTED_EDGE('',*,*,#39620,.F.);
#55376=ORIENTED_EDGE('',*,*,#39369,.T.);
#55377=ORIENTED_EDGE('',*,*,#39377,.T.);
#55378=ORIENTED_EDGE('',*,*,#39372,.T.);
#55379=ORIENTED_EDGE('',*,*,#39621,.F.);
#55380=ORIENTED_EDGE('',*,*,#39622,.F.);
#55381=ORIENTED_EDGE('',*,*,#39378,.T.);
#55382=ORIENTED_EDGE('',*,*,#39622,.T.);
#55383=ORIENTED_EDGE('',*,*,#39623,.F.);
#55384=ORIENTED_EDGE('',*,*,#39376,.T.);
#55385=ORIENTED_EDGE('',*,*,#39384,.T.);
#55386=ORIENTED_EDGE('',*,*,#39379,.T.);
#55387=ORIENTED_EDGE('',*,*,#39624,.F.);
#55388=ORIENTED_EDGE('',*,*,#39625,.F.);
#55389=ORIENTED_EDGE('',*,*,#39385,.T.);
#55390=ORIENTED_EDGE('',*,*,#39625,.T.);
#55391=ORIENTED_EDGE('',*,*,#39626,.F.);
#55392=ORIENTED_EDGE('',*,*,#39383,.T.);
#55393=ORIENTED_EDGE('',*,*,#39391,.T.);
#55394=ORIENTED_EDGE('',*,*,#39386,.T.);
#55395=ORIENTED_EDGE('',*,*,#39627,.F.);
#55396=ORIENTED_EDGE('',*,*,#39628,.F.);
#55397=ORIENTED_EDGE('',*,*,#39392,.T.);
#55398=ORIENTED_EDGE('',*,*,#39628,.T.);
#55399=ORIENTED_EDGE('',*,*,#39629,.F.);
#55400=ORIENTED_EDGE('',*,*,#39390,.T.);
#55401=ORIENTED_EDGE('',*,*,#39398,.T.);
#55402=ORIENTED_EDGE('',*,*,#39393,.T.);
#55403=ORIENTED_EDGE('',*,*,#39630,.F.);
#55404=ORIENTED_EDGE('',*,*,#39631,.F.);
#55405=ORIENTED_EDGE('',*,*,#39399,.T.);
#55406=ORIENTED_EDGE('',*,*,#39631,.T.);
#55407=ORIENTED_EDGE('',*,*,#39632,.F.);
#55408=ORIENTED_EDGE('',*,*,#39397,.T.);
#55409=ORIENTED_EDGE('',*,*,#34404,.T.);
#55410=ORIENTED_EDGE('',*,*,#39400,.T.);
#55411=ORIENTED_EDGE('',*,*,#39633,.F.);
#55412=ORIENTED_EDGE('',*,*,#39634,.F.);
#55413=ORIENTED_EDGE('',*,*,#34401,.T.);
#55414=ORIENTED_EDGE('',*,*,#39634,.T.);
#55415=ORIENTED_EDGE('',*,*,#39635,.F.);
#55416=ORIENTED_EDGE('',*,*,#39402,.T.);
#55417=ORIENTED_EDGE('',*,*,#39408,.T.);
#55418=ORIENTED_EDGE('',*,*,#39403,.T.);
#55419=ORIENTED_EDGE('',*,*,#39636,.F.);
#55420=ORIENTED_EDGE('',*,*,#39637,.F.);
#55421=ORIENTED_EDGE('',*,*,#39409,.T.);
#55422=ORIENTED_EDGE('',*,*,#39637,.T.);
#55423=ORIENTED_EDGE('',*,*,#39638,.F.);
#55424=ORIENTED_EDGE('',*,*,#39407,.T.);
#55425=ORIENTED_EDGE('',*,*,#39415,.T.);
#55426=ORIENTED_EDGE('',*,*,#39410,.T.);
#55427=ORIENTED_EDGE('',*,*,#39639,.F.);
#55428=ORIENTED_EDGE('',*,*,#39640,.F.);
#55429=ORIENTED_EDGE('',*,*,#39416,.T.);
#55430=ORIENTED_EDGE('',*,*,#39640,.T.);
#55431=ORIENTED_EDGE('',*,*,#39641,.F.);
#55432=ORIENTED_EDGE('',*,*,#39414,.T.);
#55433=ORIENTED_EDGE('',*,*,#39422,.T.);
#55434=ORIENTED_EDGE('',*,*,#39417,.T.);
#55435=ORIENTED_EDGE('',*,*,#39642,.F.);
#55436=ORIENTED_EDGE('',*,*,#39643,.F.);
#55437=ORIENTED_EDGE('',*,*,#39423,.T.);
#55438=ORIENTED_EDGE('',*,*,#39643,.T.);
#55439=ORIENTED_EDGE('',*,*,#39644,.F.);
#55440=ORIENTED_EDGE('',*,*,#39421,.T.);
#55441=ORIENTED_EDGE('',*,*,#39429,.T.);
#55442=ORIENTED_EDGE('',*,*,#39424,.T.);
#55443=ORIENTED_EDGE('',*,*,#39645,.F.);
#55444=ORIENTED_EDGE('',*,*,#39646,.F.);
#55445=ORIENTED_EDGE('',*,*,#39430,.T.);
#55446=ORIENTED_EDGE('',*,*,#39646,.T.);
#55447=ORIENTED_EDGE('',*,*,#39647,.F.);
#55448=ORIENTED_EDGE('',*,*,#39428,.T.);
#55449=ORIENTED_EDGE('',*,*,#39436,.T.);
#55450=ORIENTED_EDGE('',*,*,#39431,.T.);
#55451=ORIENTED_EDGE('',*,*,#39648,.F.);
#55452=ORIENTED_EDGE('',*,*,#39649,.F.);
#55453=ORIENTED_EDGE('',*,*,#39437,.T.);
#55454=ORIENTED_EDGE('',*,*,#39649,.T.);
#55455=ORIENTED_EDGE('',*,*,#39650,.F.);
#55456=ORIENTED_EDGE('',*,*,#39435,.T.);
#55457=ORIENTED_EDGE('',*,*,#39443,.T.);
#55458=ORIENTED_EDGE('',*,*,#39438,.T.);
#55459=ORIENTED_EDGE('',*,*,#39651,.F.);
#55460=ORIENTED_EDGE('',*,*,#39652,.F.);
#55461=ORIENTED_EDGE('',*,*,#39444,.T.);
#55462=ORIENTED_EDGE('',*,*,#39652,.T.);
#55463=ORIENTED_EDGE('',*,*,#39653,.F.);
#55464=ORIENTED_EDGE('',*,*,#39442,.T.);
#55465=ORIENTED_EDGE('',*,*,#39450,.T.);
#55466=ORIENTED_EDGE('',*,*,#39445,.T.);
#55467=ORIENTED_EDGE('',*,*,#39654,.F.);
#55468=ORIENTED_EDGE('',*,*,#39655,.F.);
#55469=ORIENTED_EDGE('',*,*,#39451,.T.);
#55470=ORIENTED_EDGE('',*,*,#39655,.T.);
#55471=ORIENTED_EDGE('',*,*,#39656,.F.);
#55472=ORIENTED_EDGE('',*,*,#39449,.T.);
#55473=ORIENTED_EDGE('',*,*,#39457,.T.);
#55474=ORIENTED_EDGE('',*,*,#39452,.T.);
#55475=ORIENTED_EDGE('',*,*,#39657,.F.);
#55476=ORIENTED_EDGE('',*,*,#39658,.F.);
#55477=ORIENTED_EDGE('',*,*,#39458,.T.);
#55478=ORIENTED_EDGE('',*,*,#39658,.T.);
#55479=ORIENTED_EDGE('',*,*,#39659,.F.);
#55480=ORIENTED_EDGE('',*,*,#39456,.T.);
#55481=ORIENTED_EDGE('',*,*,#39464,.T.);
#55482=ORIENTED_EDGE('',*,*,#39459,.T.);
#55483=ORIENTED_EDGE('',*,*,#39660,.F.);
#55484=ORIENTED_EDGE('',*,*,#39661,.F.);
#55485=ORIENTED_EDGE('',*,*,#39465,.T.);
#55486=ORIENTED_EDGE('',*,*,#39661,.T.);
#55487=ORIENTED_EDGE('',*,*,#39662,.F.);
#55488=ORIENTED_EDGE('',*,*,#39463,.T.);
#55489=ORIENTED_EDGE('',*,*,#39471,.T.);
#55490=ORIENTED_EDGE('',*,*,#39466,.T.);
#55491=ORIENTED_EDGE('',*,*,#39663,.F.);
#55492=ORIENTED_EDGE('',*,*,#39664,.F.);
#55493=ORIENTED_EDGE('',*,*,#39472,.T.);
#55494=ORIENTED_EDGE('',*,*,#39664,.T.);
#55495=ORIENTED_EDGE('',*,*,#39665,.F.);
#55496=ORIENTED_EDGE('',*,*,#39470,.T.);
#55497=ORIENTED_EDGE('',*,*,#39478,.T.);
#55498=ORIENTED_EDGE('',*,*,#39473,.T.);
#55499=ORIENTED_EDGE('',*,*,#39666,.F.);
#55500=ORIENTED_EDGE('',*,*,#39667,.F.);
#55501=ORIENTED_EDGE('',*,*,#39479,.T.);
#55502=ORIENTED_EDGE('',*,*,#39667,.T.);
#55503=ORIENTED_EDGE('',*,*,#39668,.F.);
#55504=ORIENTED_EDGE('',*,*,#39477,.T.);
#55505=ORIENTED_EDGE('',*,*,#39485,.T.);
#55506=ORIENTED_EDGE('',*,*,#39480,.T.);
#55507=ORIENTED_EDGE('',*,*,#39669,.F.);
#55508=ORIENTED_EDGE('',*,*,#39670,.F.);
#55509=ORIENTED_EDGE('',*,*,#39486,.T.);
#55510=ORIENTED_EDGE('',*,*,#39670,.T.);
#55511=ORIENTED_EDGE('',*,*,#39671,.F.);
#55512=ORIENTED_EDGE('',*,*,#39484,.T.);
#55513=ORIENTED_EDGE('',*,*,#39672,.F.);
#55514=ORIENTED_EDGE('',*,*,#39673,.F.);
#55515=ORIENTED_EDGE('',*,*,#39492,.T.);
#55516=ORIENTED_EDGE('',*,*,#39487,.T.);
#55517=ORIENTED_EDGE('',*,*,#39493,.T.);
#55518=ORIENTED_EDGE('',*,*,#39673,.T.);
#55519=ORIENTED_EDGE('',*,*,#39674,.F.);
#55520=ORIENTED_EDGE('',*,*,#39491,.T.);
#55521=ORIENTED_EDGE('',*,*,#39499,.T.);
#55522=ORIENTED_EDGE('',*,*,#39494,.T.);
#55523=ORIENTED_EDGE('',*,*,#39675,.F.);
#55524=ORIENTED_EDGE('',*,*,#39676,.F.);
#55525=ORIENTED_EDGE('',*,*,#39500,.T.);
#55526=ORIENTED_EDGE('',*,*,#39676,.T.);
#55527=ORIENTED_EDGE('',*,*,#39677,.F.);
#55528=ORIENTED_EDGE('',*,*,#39498,.T.);
#55529=ORIENTED_EDGE('',*,*,#39502,.T.);
#55530=ORIENTED_EDGE('',*,*,#39504,.T.);
#55531=ORIENTED_EDGE('',*,*,#39678,.F.);
#55532=ORIENTED_EDGE('',*,*,#39592,.T.);
#55533=ORIENTED_EDGE('',*,*,#39679,.T.);
#55534=ORIENTED_EDGE('',*,*,#39680,.F.);
#55535=ORIENTED_EDGE('',*,*,#39505,.T.);
#55536=ORIENTED_EDGE('',*,*,#39681,.F.);
#55537=ORIENTED_EDGE('',*,*,#39682,.F.);
#55538=ORIENTED_EDGE('',*,*,#39683,.F.);
#55539=ORIENTED_EDGE('',*,*,#39684,.F.);
#55540=ORIENTED_EDGE('',*,*,#39679,.F.);
#55541=ORIENTED_EDGE('',*,*,#39684,.T.);
#55542=ORIENTED_EDGE('',*,*,#39685,.F.);
#55543=ORIENTED_EDGE('',*,*,#39507,.T.);
#55544=ORIENTED_EDGE('',*,*,#39680,.T.);
#55545=ORIENTED_EDGE('',*,*,#39686,.T.);
#55546=ORIENTED_EDGE('',*,*,#39687,.F.);
#55547=ORIENTED_EDGE('',*,*,#39509,.T.);
#55548=ORIENTED_EDGE('',*,*,#39688,.F.);
#55549=ORIENTED_EDGE('',*,*,#39689,.F.);
#55550=ORIENTED_EDGE('',*,*,#39690,.F.);
#55551=ORIENTED_EDGE('',*,*,#39691,.F.);
#55552=ORIENTED_EDGE('',*,*,#39686,.F.);
#55553=ORIENTED_EDGE('',*,*,#39691,.T.);
#55554=ORIENTED_EDGE('',*,*,#39692,.F.);
#55555=ORIENTED_EDGE('',*,*,#39510,.T.);
#55556=ORIENTED_EDGE('',*,*,#39687,.T.);
#55557=ORIENTED_EDGE('',*,*,#39693,.T.);
#55558=ORIENTED_EDGE('',*,*,#39694,.F.);
#55559=ORIENTED_EDGE('',*,*,#39512,.T.);
#55560=ORIENTED_EDGE('',*,*,#39695,.F.);
#55561=ORIENTED_EDGE('',*,*,#39696,.F.);
#55562=ORIENTED_EDGE('',*,*,#39697,.F.);
#55563=ORIENTED_EDGE('',*,*,#39698,.F.);
#55564=ORIENTED_EDGE('',*,*,#39693,.F.);
#55565=ORIENTED_EDGE('',*,*,#39698,.T.);
#55566=ORIENTED_EDGE('',*,*,#39699,.F.);
#55567=ORIENTED_EDGE('',*,*,#39513,.T.);
#55568=ORIENTED_EDGE('',*,*,#39694,.T.);
#55569=ORIENTED_EDGE('',*,*,#39700,.T.);
#55570=ORIENTED_EDGE('',*,*,#39701,.F.);
#55571=ORIENTED_EDGE('',*,*,#39515,.T.);
#55572=ORIENTED_EDGE('',*,*,#39702,.F.);
#55573=ORIENTED_EDGE('',*,*,#39703,.F.);
#55574=ORIENTED_EDGE('',*,*,#39704,.F.);
#55575=ORIENTED_EDGE('',*,*,#39705,.F.);
#55576=ORIENTED_EDGE('',*,*,#39700,.F.);
#55577=ORIENTED_EDGE('',*,*,#39705,.T.);
#55578=ORIENTED_EDGE('',*,*,#39706,.F.);
#55579=ORIENTED_EDGE('',*,*,#39516,.T.);
#55580=ORIENTED_EDGE('',*,*,#39701,.T.);
#55581=ORIENTED_EDGE('',*,*,#39707,.T.);
#55582=ORIENTED_EDGE('',*,*,#39708,.F.);
#55583=ORIENTED_EDGE('',*,*,#39518,.T.);
#55584=ORIENTED_EDGE('',*,*,#39709,.F.);
#55585=ORIENTED_EDGE('',*,*,#39710,.F.);
#55586=ORIENTED_EDGE('',*,*,#39711,.F.);
#55587=ORIENTED_EDGE('',*,*,#39712,.F.);
#55588=ORIENTED_EDGE('',*,*,#39707,.F.);
#55589=ORIENTED_EDGE('',*,*,#39712,.T.);
#55590=ORIENTED_EDGE('',*,*,#39713,.F.);
#55591=ORIENTED_EDGE('',*,*,#39519,.T.);
#55592=ORIENTED_EDGE('',*,*,#39708,.T.);
#55593=ORIENTED_EDGE('',*,*,#39714,.T.);
#55594=ORIENTED_EDGE('',*,*,#39715,.F.);
#55595=ORIENTED_EDGE('',*,*,#39521,.T.);
#55596=ORIENTED_EDGE('',*,*,#39716,.F.);
#55597=ORIENTED_EDGE('',*,*,#39717,.F.);
#55598=ORIENTED_EDGE('',*,*,#39718,.F.);
#55599=ORIENTED_EDGE('',*,*,#39719,.F.);
#55600=ORIENTED_EDGE('',*,*,#39714,.F.);
#55601=ORIENTED_EDGE('',*,*,#39719,.T.);
#55602=ORIENTED_EDGE('',*,*,#39720,.F.);
#55603=ORIENTED_EDGE('',*,*,#39522,.T.);
#55604=ORIENTED_EDGE('',*,*,#39715,.T.);
#55605=ORIENTED_EDGE('',*,*,#39721,.T.);
#55606=ORIENTED_EDGE('',*,*,#39722,.F.);
#55607=ORIENTED_EDGE('',*,*,#39524,.T.);
#55608=ORIENTED_EDGE('',*,*,#39723,.F.);
#55609=ORIENTED_EDGE('',*,*,#39724,.F.);
#55610=ORIENTED_EDGE('',*,*,#39725,.F.);
#55611=ORIENTED_EDGE('',*,*,#39726,.F.);
#55612=ORIENTED_EDGE('',*,*,#39721,.F.);
#55613=ORIENTED_EDGE('',*,*,#39726,.T.);
#55614=ORIENTED_EDGE('',*,*,#39727,.F.);
#55615=ORIENTED_EDGE('',*,*,#39525,.T.);
#55616=ORIENTED_EDGE('',*,*,#39722,.T.);
#55617=ORIENTED_EDGE('',*,*,#39728,.T.);
#55618=ORIENTED_EDGE('',*,*,#39729,.F.);
#55619=ORIENTED_EDGE('',*,*,#39527,.T.);
#55620=ORIENTED_EDGE('',*,*,#39730,.F.);
#55621=ORIENTED_EDGE('',*,*,#39731,.F.);
#55622=ORIENTED_EDGE('',*,*,#39732,.F.);
#55623=ORIENTED_EDGE('',*,*,#39733,.F.);
#55624=ORIENTED_EDGE('',*,*,#39728,.F.);
#55625=ORIENTED_EDGE('',*,*,#39733,.T.);
#55626=ORIENTED_EDGE('',*,*,#39734,.F.);
#55627=ORIENTED_EDGE('',*,*,#39528,.T.);
#55628=ORIENTED_EDGE('',*,*,#39729,.T.);
#55629=ORIENTED_EDGE('',*,*,#39735,.T.);
#55630=ORIENTED_EDGE('',*,*,#39736,.F.);
#55631=ORIENTED_EDGE('',*,*,#39530,.T.);
#55632=ORIENTED_EDGE('',*,*,#39737,.F.);
#55633=ORIENTED_EDGE('',*,*,#39738,.F.);
#55634=ORIENTED_EDGE('',*,*,#39739,.F.);
#55635=ORIENTED_EDGE('',*,*,#39740,.F.);
#55636=ORIENTED_EDGE('',*,*,#39735,.F.);
#55637=ORIENTED_EDGE('',*,*,#39740,.T.);
#55638=ORIENTED_EDGE('',*,*,#39741,.F.);
#55639=ORIENTED_EDGE('',*,*,#39531,.T.);
#55640=ORIENTED_EDGE('',*,*,#39736,.T.);
#55641=ORIENTED_EDGE('',*,*,#39742,.T.);
#55642=ORIENTED_EDGE('',*,*,#39743,.F.);
#55643=ORIENTED_EDGE('',*,*,#39533,.T.);
#55644=ORIENTED_EDGE('',*,*,#39744,.F.);
#55645=ORIENTED_EDGE('',*,*,#39745,.F.);
#55646=ORIENTED_EDGE('',*,*,#39746,.F.);
#55647=ORIENTED_EDGE('',*,*,#39747,.F.);
#55648=ORIENTED_EDGE('',*,*,#39742,.F.);
#55649=ORIENTED_EDGE('',*,*,#39747,.T.);
#55650=ORIENTED_EDGE('',*,*,#39748,.F.);
#55651=ORIENTED_EDGE('',*,*,#39534,.T.);
#55652=ORIENTED_EDGE('',*,*,#39743,.T.);
#55653=ORIENTED_EDGE('',*,*,#39749,.T.);
#55654=ORIENTED_EDGE('',*,*,#39750,.F.);
#55655=ORIENTED_EDGE('',*,*,#39536,.T.);
#55656=ORIENTED_EDGE('',*,*,#39751,.F.);
#55657=ORIENTED_EDGE('',*,*,#39752,.F.);
#55658=ORIENTED_EDGE('',*,*,#39753,.F.);
#55659=ORIENTED_EDGE('',*,*,#39754,.F.);
#55660=ORIENTED_EDGE('',*,*,#39749,.F.);
#55661=ORIENTED_EDGE('',*,*,#39754,.T.);
#55662=ORIENTED_EDGE('',*,*,#39755,.F.);
#55663=ORIENTED_EDGE('',*,*,#39537,.T.);
#55664=ORIENTED_EDGE('',*,*,#39750,.T.);
#55665=ORIENTED_EDGE('',*,*,#39756,.T.);
#55666=ORIENTED_EDGE('',*,*,#39757,.F.);
#55667=ORIENTED_EDGE('',*,*,#39539,.T.);
#55668=ORIENTED_EDGE('',*,*,#39758,.F.);
#55669=ORIENTED_EDGE('',*,*,#39759,.F.);
#55670=ORIENTED_EDGE('',*,*,#39760,.F.);
#55671=ORIENTED_EDGE('',*,*,#39761,.F.);
#55672=ORIENTED_EDGE('',*,*,#39756,.F.);
#55673=ORIENTED_EDGE('',*,*,#39761,.T.);
#55674=ORIENTED_EDGE('',*,*,#39762,.F.);
#55675=ORIENTED_EDGE('',*,*,#39540,.T.);
#55676=ORIENTED_EDGE('',*,*,#39757,.T.);
#55677=ORIENTED_EDGE('',*,*,#39763,.T.);
#55678=ORIENTED_EDGE('',*,*,#39764,.F.);
#55679=ORIENTED_EDGE('',*,*,#39542,.T.);
#55680=ORIENTED_EDGE('',*,*,#39765,.F.);
#55681=ORIENTED_EDGE('',*,*,#39766,.F.);
#55682=ORIENTED_EDGE('',*,*,#39767,.F.);
#55683=ORIENTED_EDGE('',*,*,#39768,.F.);
#55684=ORIENTED_EDGE('',*,*,#39763,.F.);
#55685=ORIENTED_EDGE('',*,*,#39768,.T.);
#55686=ORIENTED_EDGE('',*,*,#39769,.F.);
#55687=ORIENTED_EDGE('',*,*,#39543,.T.);
#55688=ORIENTED_EDGE('',*,*,#39764,.T.);
#55689=ORIENTED_EDGE('',*,*,#39770,.T.);
#55690=ORIENTED_EDGE('',*,*,#39771,.F.);
#55691=ORIENTED_EDGE('',*,*,#39545,.T.);
#55692=ORIENTED_EDGE('',*,*,#39772,.F.);
#55693=ORIENTED_EDGE('',*,*,#39773,.F.);
#55694=ORIENTED_EDGE('',*,*,#39774,.F.);
#55695=ORIENTED_EDGE('',*,*,#39775,.F.);
#55696=ORIENTED_EDGE('',*,*,#39770,.F.);
#55697=ORIENTED_EDGE('',*,*,#39775,.T.);
#55698=ORIENTED_EDGE('',*,*,#39776,.F.);
#55699=ORIENTED_EDGE('',*,*,#39546,.T.);
#55700=ORIENTED_EDGE('',*,*,#39771,.T.);
#55701=ORIENTED_EDGE('',*,*,#34397,.T.);
#55702=ORIENTED_EDGE('',*,*,#39777,.F.);
#55703=ORIENTED_EDGE('',*,*,#39548,.T.);
#55704=ORIENTED_EDGE('',*,*,#39778,.F.);
#55705=ORIENTED_EDGE('',*,*,#34400,.T.);
#55706=ORIENTED_EDGE('',*,*,#39779,.F.);
#55707=ORIENTED_EDGE('',*,*,#39549,.T.);
#55708=ORIENTED_EDGE('',*,*,#39777,.T.);
#55709=ORIENTED_EDGE('',*,*,#39780,.T.);
#55710=ORIENTED_EDGE('',*,*,#39781,.F.);
#55711=ORIENTED_EDGE('',*,*,#39551,.T.);
#55712=ORIENTED_EDGE('',*,*,#39782,.F.);
#55713=ORIENTED_EDGE('',*,*,#39783,.F.);
#55714=ORIENTED_EDGE('',*,*,#39784,.F.);
#55715=ORIENTED_EDGE('',*,*,#39785,.F.);
#55716=ORIENTED_EDGE('',*,*,#39780,.F.);
#55717=ORIENTED_EDGE('',*,*,#39785,.T.);
#55718=ORIENTED_EDGE('',*,*,#39786,.F.);
#55719=ORIENTED_EDGE('',*,*,#39552,.T.);
#55720=ORIENTED_EDGE('',*,*,#39781,.T.);
#55721=ORIENTED_EDGE('',*,*,#39787,.T.);
#55722=ORIENTED_EDGE('',*,*,#39788,.F.);
#55723=ORIENTED_EDGE('',*,*,#39554,.T.);
#55724=ORIENTED_EDGE('',*,*,#39789,.F.);
#55725=ORIENTED_EDGE('',*,*,#39790,.F.);
#55726=ORIENTED_EDGE('',*,*,#39791,.F.);
#55727=ORIENTED_EDGE('',*,*,#39792,.F.);
#55728=ORIENTED_EDGE('',*,*,#39787,.F.);
#55729=ORIENTED_EDGE('',*,*,#39792,.T.);
#55730=ORIENTED_EDGE('',*,*,#39793,.F.);
#55731=ORIENTED_EDGE('',*,*,#39555,.T.);
#55732=ORIENTED_EDGE('',*,*,#39788,.T.);
#55733=ORIENTED_EDGE('',*,*,#39794,.T.);
#55734=ORIENTED_EDGE('',*,*,#39795,.F.);
#55735=ORIENTED_EDGE('',*,*,#39557,.T.);
#55736=ORIENTED_EDGE('',*,*,#39796,.F.);
#55737=ORIENTED_EDGE('',*,*,#39797,.F.);
#55738=ORIENTED_EDGE('',*,*,#39798,.F.);
#55739=ORIENTED_EDGE('',*,*,#39799,.F.);
#55740=ORIENTED_EDGE('',*,*,#39794,.F.);
#55741=ORIENTED_EDGE('',*,*,#39799,.T.);
#55742=ORIENTED_EDGE('',*,*,#39800,.F.);
#55743=ORIENTED_EDGE('',*,*,#39558,.T.);
#55744=ORIENTED_EDGE('',*,*,#39795,.T.);
#55745=ORIENTED_EDGE('',*,*,#39801,.T.);
#55746=ORIENTED_EDGE('',*,*,#39802,.F.);
#55747=ORIENTED_EDGE('',*,*,#39560,.T.);
#55748=ORIENTED_EDGE('',*,*,#39803,.F.);
#55749=ORIENTED_EDGE('',*,*,#39804,.F.);
#55750=ORIENTED_EDGE('',*,*,#39805,.F.);
#55751=ORIENTED_EDGE('',*,*,#39806,.F.);
#55752=ORIENTED_EDGE('',*,*,#39801,.F.);
#55753=ORIENTED_EDGE('',*,*,#39806,.T.);
#55754=ORIENTED_EDGE('',*,*,#39807,.F.);
#55755=ORIENTED_EDGE('',*,*,#39561,.T.);
#55756=ORIENTED_EDGE('',*,*,#39802,.T.);
#55757=ORIENTED_EDGE('',*,*,#39808,.T.);
#55758=ORIENTED_EDGE('',*,*,#39809,.F.);
#55759=ORIENTED_EDGE('',*,*,#39563,.T.);
#55760=ORIENTED_EDGE('',*,*,#39810,.F.);
#55761=ORIENTED_EDGE('',*,*,#39811,.F.);
#55762=ORIENTED_EDGE('',*,*,#39812,.F.);
#55763=ORIENTED_EDGE('',*,*,#39813,.F.);
#55764=ORIENTED_EDGE('',*,*,#39808,.F.);
#55765=ORIENTED_EDGE('',*,*,#39813,.T.);
#55766=ORIENTED_EDGE('',*,*,#39814,.F.);
#55767=ORIENTED_EDGE('',*,*,#39564,.T.);
#55768=ORIENTED_EDGE('',*,*,#39809,.T.);
#55769=ORIENTED_EDGE('',*,*,#39815,.T.);
#55770=ORIENTED_EDGE('',*,*,#39816,.F.);
#55771=ORIENTED_EDGE('',*,*,#39566,.T.);
#55772=ORIENTED_EDGE('',*,*,#39817,.F.);
#55773=ORIENTED_EDGE('',*,*,#39818,.T.);
#55774=ORIENTED_EDGE('',*,*,#39819,.F.);
#55775=ORIENTED_EDGE('',*,*,#39567,.T.);
#55776=ORIENTED_EDGE('',*,*,#39816,.T.);
#55777=ORIENTED_EDGE('',*,*,#39820,.F.);
#55778=ORIENTED_EDGE('',*,*,#39821,.F.);
#55779=ORIENTED_EDGE('',*,*,#39818,.F.);
#55780=ORIENTED_EDGE('',*,*,#39815,.F.);
#55781=ORIENTED_EDGE('',*,*,#39569,.T.);
#55782=ORIENTED_EDGE('',*,*,#39822,.F.);
#55783=ORIENTED_EDGE('',*,*,#39823,.T.);
#55784=ORIENTED_EDGE('',*,*,#39824,.F.);
#55785=ORIENTED_EDGE('',*,*,#39825,.F.);
#55786=ORIENTED_EDGE('',*,*,#39823,.F.);
#55787=ORIENTED_EDGE('',*,*,#39826,.F.);
#55788=ORIENTED_EDGE('',*,*,#39827,.F.);
#55789=ORIENTED_EDGE('',*,*,#39570,.T.);
#55790=ORIENTED_EDGE('',*,*,#39824,.T.);
#55791=ORIENTED_EDGE('',*,*,#39825,.T.);
#55792=ORIENTED_EDGE('',*,*,#39828,.F.);
#55793=ORIENTED_EDGE('',*,*,#39829,.T.);
#55794=ORIENTED_EDGE('',*,*,#39830,.F.);
#55795=ORIENTED_EDGE('',*,*,#39572,.T.);
#55796=ORIENTED_EDGE('',*,*,#39831,.F.);
#55797=ORIENTED_EDGE('',*,*,#39832,.F.);
#55798=ORIENTED_EDGE('',*,*,#39833,.F.);
#55799=ORIENTED_EDGE('',*,*,#39834,.F.);
#55800=ORIENTED_EDGE('',*,*,#39829,.F.);
#55801=ORIENTED_EDGE('',*,*,#39834,.T.);
#55802=ORIENTED_EDGE('',*,*,#39835,.F.);
#55803=ORIENTED_EDGE('',*,*,#39573,.T.);
#55804=ORIENTED_EDGE('',*,*,#39830,.T.);
#55805=ORIENTED_EDGE('',*,*,#39836,.T.);
#55806=ORIENTED_EDGE('',*,*,#39837,.F.);
#55807=ORIENTED_EDGE('',*,*,#39575,.T.);
#55808=ORIENTED_EDGE('',*,*,#39838,.F.);
#55809=ORIENTED_EDGE('',*,*,#39839,.F.);
#55810=ORIENTED_EDGE('',*,*,#39840,.F.);
#55811=ORIENTED_EDGE('',*,*,#39841,.F.);
#55812=ORIENTED_EDGE('',*,*,#39836,.F.);
#55813=ORIENTED_EDGE('',*,*,#39841,.T.);
#55814=ORIENTED_EDGE('',*,*,#39842,.F.);
#55815=ORIENTED_EDGE('',*,*,#39576,.T.);
#55816=ORIENTED_EDGE('',*,*,#39837,.T.);
#55817=ORIENTED_EDGE('',*,*,#39843,.T.);
#55818=ORIENTED_EDGE('',*,*,#39844,.F.);
#55819=ORIENTED_EDGE('',*,*,#39578,.T.);
#55820=ORIENTED_EDGE('',*,*,#39845,.F.);
#55821=ORIENTED_EDGE('',*,*,#39846,.F.);
#55822=ORIENTED_EDGE('',*,*,#39847,.F.);
#55823=ORIENTED_EDGE('',*,*,#39848,.F.);
#55824=ORIENTED_EDGE('',*,*,#39843,.F.);
#55825=ORIENTED_EDGE('',*,*,#39848,.T.);
#55826=ORIENTED_EDGE('',*,*,#39849,.F.);
#55827=ORIENTED_EDGE('',*,*,#39579,.T.);
#55828=ORIENTED_EDGE('',*,*,#39844,.T.);
#55829=ORIENTED_EDGE('',*,*,#39850,.T.);
#55830=ORIENTED_EDGE('',*,*,#39851,.F.);
#55831=ORIENTED_EDGE('',*,*,#39581,.T.);
#55832=ORIENTED_EDGE('',*,*,#39852,.F.);
#55833=ORIENTED_EDGE('',*,*,#39853,.F.);
#55834=ORIENTED_EDGE('',*,*,#39854,.F.);
#55835=ORIENTED_EDGE('',*,*,#39855,.F.);
#55836=ORIENTED_EDGE('',*,*,#39850,.F.);
#55837=ORIENTED_EDGE('',*,*,#39855,.T.);
#55838=ORIENTED_EDGE('',*,*,#39856,.F.);
#55839=ORIENTED_EDGE('',*,*,#39582,.T.);
#55840=ORIENTED_EDGE('',*,*,#39851,.T.);
#55841=ORIENTED_EDGE('',*,*,#39857,.T.);
#55842=ORIENTED_EDGE('',*,*,#39858,.F.);
#55843=ORIENTED_EDGE('',*,*,#39584,.T.);
#55844=ORIENTED_EDGE('',*,*,#39859,.F.);
#55845=ORIENTED_EDGE('',*,*,#39860,.F.);
#55846=ORIENTED_EDGE('',*,*,#39861,.F.);
#55847=ORIENTED_EDGE('',*,*,#39862,.F.);
#55848=ORIENTED_EDGE('',*,*,#39857,.F.);
#55849=ORIENTED_EDGE('',*,*,#39862,.T.);
#55850=ORIENTED_EDGE('',*,*,#39863,.F.);
#55851=ORIENTED_EDGE('',*,*,#39585,.T.);
#55852=ORIENTED_EDGE('',*,*,#39858,.T.);
#55853=ORIENTED_EDGE('',*,*,#39864,.T.);
#55854=ORIENTED_EDGE('',*,*,#39865,.F.);
#55855=ORIENTED_EDGE('',*,*,#39587,.T.);
#55856=ORIENTED_EDGE('',*,*,#39866,.F.);
#55857=ORIENTED_EDGE('',*,*,#39867,.F.);
#55858=ORIENTED_EDGE('',*,*,#39868,.F.);
#55859=ORIENTED_EDGE('',*,*,#39869,.F.);
#55860=ORIENTED_EDGE('',*,*,#39864,.F.);
#55861=ORIENTED_EDGE('',*,*,#39869,.T.);
#55862=ORIENTED_EDGE('',*,*,#39870,.F.);
#55863=ORIENTED_EDGE('',*,*,#39588,.T.);
#55864=ORIENTED_EDGE('',*,*,#39865,.T.);
#55865=ORIENTED_EDGE('',*,*,#39871,.T.);
#55866=ORIENTED_EDGE('',*,*,#39872,.F.);
#55867=ORIENTED_EDGE('',*,*,#39590,.T.);
#55868=ORIENTED_EDGE('',*,*,#39873,.F.);
#55869=ORIENTED_EDGE('',*,*,#39874,.F.);
#55870=ORIENTED_EDGE('',*,*,#39875,.F.);
#55871=ORIENTED_EDGE('',*,*,#39876,.F.);
#55872=ORIENTED_EDGE('',*,*,#39871,.F.);
#55873=ORIENTED_EDGE('',*,*,#39876,.T.);
#55874=ORIENTED_EDGE('',*,*,#39877,.F.);
#55875=ORIENTED_EDGE('',*,*,#39591,.T.);
#55876=ORIENTED_EDGE('',*,*,#39872,.T.);
#55877=ORIENTED_EDGE('',*,*,#39593,.T.);
#55878=ORIENTED_EDGE('',*,*,#39878,.F.);
#55879=ORIENTED_EDGE('',*,*,#39879,.T.);
#55880=ORIENTED_EDGE('',*,*,#39880,.F.);
#55881=ORIENTED_EDGE('',*,*,#39594,.T.);
#55882=ORIENTED_EDGE('',*,*,#39880,.T.);
#55883=ORIENTED_EDGE('',*,*,#39881,.T.);
#55884=ORIENTED_EDGE('',*,*,#39882,.F.);
#55885=ORIENTED_EDGE('',*,*,#39881,.F.);
#55886=ORIENTED_EDGE('',*,*,#39879,.F.);
#55887=ORIENTED_EDGE('',*,*,#39883,.F.);
#55888=ORIENTED_EDGE('',*,*,#39884,.F.);
#55889=ORIENTED_EDGE('',*,*,#39596,.T.);
#55890=ORIENTED_EDGE('',*,*,#39885,.F.);
#55891=ORIENTED_EDGE('',*,*,#39886,.T.);
#55892=ORIENTED_EDGE('',*,*,#39887,.F.);
#55893=ORIENTED_EDGE('',*,*,#39597,.T.);
#55894=ORIENTED_EDGE('',*,*,#39887,.T.);
#55895=ORIENTED_EDGE('',*,*,#39888,.T.);
#55896=ORIENTED_EDGE('',*,*,#39889,.F.);
#55897=ORIENTED_EDGE('',*,*,#39888,.F.);
#55898=ORIENTED_EDGE('',*,*,#39886,.F.);
#55899=ORIENTED_EDGE('',*,*,#39890,.F.);
#55900=ORIENTED_EDGE('',*,*,#39891,.F.);
#55901=ORIENTED_EDGE('',*,*,#39599,.T.);
#55902=ORIENTED_EDGE('',*,*,#39892,.F.);
#55903=ORIENTED_EDGE('',*,*,#39893,.T.);
#55904=ORIENTED_EDGE('',*,*,#39894,.F.);
#55905=ORIENTED_EDGE('',*,*,#39600,.T.);
#55906=ORIENTED_EDGE('',*,*,#39894,.T.);
#55907=ORIENTED_EDGE('',*,*,#39895,.T.);
#55908=ORIENTED_EDGE('',*,*,#39896,.F.);
#55909=ORIENTED_EDGE('',*,*,#39895,.F.);
#55910=ORIENTED_EDGE('',*,*,#39893,.F.);
#55911=ORIENTED_EDGE('',*,*,#39897,.F.);
#55912=ORIENTED_EDGE('',*,*,#39898,.F.);
#55913=ORIENTED_EDGE('',*,*,#39602,.T.);
#55914=ORIENTED_EDGE('',*,*,#39899,.F.);
#55915=ORIENTED_EDGE('',*,*,#39900,.T.);
#55916=ORIENTED_EDGE('',*,*,#39901,.F.);
#55917=ORIENTED_EDGE('',*,*,#39603,.T.);
#55918=ORIENTED_EDGE('',*,*,#39901,.T.);
#55919=ORIENTED_EDGE('',*,*,#39902,.T.);
#55920=ORIENTED_EDGE('',*,*,#39903,.F.);
#55921=ORIENTED_EDGE('',*,*,#39902,.F.);
#55922=ORIENTED_EDGE('',*,*,#39900,.F.);
#55923=ORIENTED_EDGE('',*,*,#39904,.F.);
#55924=ORIENTED_EDGE('',*,*,#39905,.F.);
#55925=ORIENTED_EDGE('',*,*,#39605,.T.);
#55926=ORIENTED_EDGE('',*,*,#39906,.F.);
#55927=ORIENTED_EDGE('',*,*,#39907,.T.);
#55928=ORIENTED_EDGE('',*,*,#39908,.F.);
#55929=ORIENTED_EDGE('',*,*,#39606,.T.);
#55930=ORIENTED_EDGE('',*,*,#39908,.T.);
#55931=ORIENTED_EDGE('',*,*,#39909,.T.);
#55932=ORIENTED_EDGE('',*,*,#39910,.F.);
#55933=ORIENTED_EDGE('',*,*,#39909,.F.);
#55934=ORIENTED_EDGE('',*,*,#39907,.F.);
#55935=ORIENTED_EDGE('',*,*,#39911,.F.);
#55936=ORIENTED_EDGE('',*,*,#39912,.F.);
#55937=ORIENTED_EDGE('',*,*,#39608,.T.);
#55938=ORIENTED_EDGE('',*,*,#39913,.F.);
#55939=ORIENTED_EDGE('',*,*,#39914,.T.);
#55940=ORIENTED_EDGE('',*,*,#39915,.F.);
#55941=ORIENTED_EDGE('',*,*,#39609,.T.);
#55942=ORIENTED_EDGE('',*,*,#39915,.T.);
#55943=ORIENTED_EDGE('',*,*,#39916,.T.);
#55944=ORIENTED_EDGE('',*,*,#39917,.F.);
#55945=ORIENTED_EDGE('',*,*,#39916,.F.);
#55946=ORIENTED_EDGE('',*,*,#39914,.F.);
#55947=ORIENTED_EDGE('',*,*,#39918,.F.);
#55948=ORIENTED_EDGE('',*,*,#39919,.F.);
#55949=ORIENTED_EDGE('',*,*,#39611,.T.);
#55950=ORIENTED_EDGE('',*,*,#39920,.F.);
#55951=ORIENTED_EDGE('',*,*,#39921,.T.);
#55952=ORIENTED_EDGE('',*,*,#39922,.F.);
#55953=ORIENTED_EDGE('',*,*,#39612,.T.);
#55954=ORIENTED_EDGE('',*,*,#39922,.T.);
#55955=ORIENTED_EDGE('',*,*,#39923,.T.);
#55956=ORIENTED_EDGE('',*,*,#39924,.F.);
#55957=ORIENTED_EDGE('',*,*,#39923,.F.);
#55958=ORIENTED_EDGE('',*,*,#39921,.F.);
#55959=ORIENTED_EDGE('',*,*,#39925,.F.);
#55960=ORIENTED_EDGE('',*,*,#39926,.F.);
#55961=ORIENTED_EDGE('',*,*,#39614,.T.);
#55962=ORIENTED_EDGE('',*,*,#39927,.F.);
#55963=ORIENTED_EDGE('',*,*,#39928,.T.);
#55964=ORIENTED_EDGE('',*,*,#39929,.F.);
#55965=ORIENTED_EDGE('',*,*,#39615,.T.);
#55966=ORIENTED_EDGE('',*,*,#39929,.T.);
#55967=ORIENTED_EDGE('',*,*,#39930,.T.);
#55968=ORIENTED_EDGE('',*,*,#39931,.F.);
#55969=ORIENTED_EDGE('',*,*,#39930,.F.);
#55970=ORIENTED_EDGE('',*,*,#39928,.F.);
#55971=ORIENTED_EDGE('',*,*,#39932,.F.);
#55972=ORIENTED_EDGE('',*,*,#39933,.F.);
#55973=ORIENTED_EDGE('',*,*,#39617,.T.);
#55974=ORIENTED_EDGE('',*,*,#39934,.F.);
#55975=ORIENTED_EDGE('',*,*,#39935,.T.);
#55976=ORIENTED_EDGE('',*,*,#39936,.F.);
#55977=ORIENTED_EDGE('',*,*,#39618,.T.);
#55978=ORIENTED_EDGE('',*,*,#39936,.T.);
#55979=ORIENTED_EDGE('',*,*,#39937,.T.);
#55980=ORIENTED_EDGE('',*,*,#39938,.F.);
#55981=ORIENTED_EDGE('',*,*,#39937,.F.);
#55982=ORIENTED_EDGE('',*,*,#39935,.F.);
#55983=ORIENTED_EDGE('',*,*,#39939,.F.);
#55984=ORIENTED_EDGE('',*,*,#39940,.F.);
#55985=ORIENTED_EDGE('',*,*,#39620,.T.);
#55986=ORIENTED_EDGE('',*,*,#39941,.F.);
#55987=ORIENTED_EDGE('',*,*,#39942,.T.);
#55988=ORIENTED_EDGE('',*,*,#39943,.F.);
#55989=ORIENTED_EDGE('',*,*,#39621,.T.);
#55990=ORIENTED_EDGE('',*,*,#39943,.T.);
#55991=ORIENTED_EDGE('',*,*,#39944,.T.);
#55992=ORIENTED_EDGE('',*,*,#39945,.F.);
#55993=ORIENTED_EDGE('',*,*,#39944,.F.);
#55994=ORIENTED_EDGE('',*,*,#39942,.F.);
#55995=ORIENTED_EDGE('',*,*,#39946,.F.);
#55996=ORIENTED_EDGE('',*,*,#39947,.F.);
#55997=ORIENTED_EDGE('',*,*,#39623,.T.);
#55998=ORIENTED_EDGE('',*,*,#39948,.F.);
#55999=ORIENTED_EDGE('',*,*,#39949,.T.);
#56000=ORIENTED_EDGE('',*,*,#39950,.F.);
#56001=ORIENTED_EDGE('',*,*,#39624,.T.);
#56002=ORIENTED_EDGE('',*,*,#39950,.T.);
#56003=ORIENTED_EDGE('',*,*,#39951,.T.);
#56004=ORIENTED_EDGE('',*,*,#39952,.F.);
#56005=ORIENTED_EDGE('',*,*,#39951,.F.);
#56006=ORIENTED_EDGE('',*,*,#39949,.F.);
#56007=ORIENTED_EDGE('',*,*,#39953,.F.);
#56008=ORIENTED_EDGE('',*,*,#39954,.F.);
#56009=ORIENTED_EDGE('',*,*,#39626,.T.);
#56010=ORIENTED_EDGE('',*,*,#39955,.F.);
#56011=ORIENTED_EDGE('',*,*,#39956,.T.);
#56012=ORIENTED_EDGE('',*,*,#39957,.F.);
#56013=ORIENTED_EDGE('',*,*,#39627,.T.);
#56014=ORIENTED_EDGE('',*,*,#39957,.T.);
#56015=ORIENTED_EDGE('',*,*,#39958,.T.);
#56016=ORIENTED_EDGE('',*,*,#39959,.F.);
#56017=ORIENTED_EDGE('',*,*,#39958,.F.);
#56018=ORIENTED_EDGE('',*,*,#39956,.F.);
#56019=ORIENTED_EDGE('',*,*,#39960,.F.);
#56020=ORIENTED_EDGE('',*,*,#39961,.F.);
#56021=ORIENTED_EDGE('',*,*,#39629,.T.);
#56022=ORIENTED_EDGE('',*,*,#39962,.F.);
#56023=ORIENTED_EDGE('',*,*,#39963,.T.);
#56024=ORIENTED_EDGE('',*,*,#39964,.F.);
#56025=ORIENTED_EDGE('',*,*,#39630,.T.);
#56026=ORIENTED_EDGE('',*,*,#39964,.T.);
#56027=ORIENTED_EDGE('',*,*,#39965,.T.);
#56028=ORIENTED_EDGE('',*,*,#39966,.F.);
#56029=ORIENTED_EDGE('',*,*,#39965,.F.);
#56030=ORIENTED_EDGE('',*,*,#39963,.F.);
#56031=ORIENTED_EDGE('',*,*,#39967,.F.);
#56032=ORIENTED_EDGE('',*,*,#39968,.F.);
#56033=ORIENTED_EDGE('',*,*,#39632,.T.);
#56034=ORIENTED_EDGE('',*,*,#39969,.F.);
#56035=ORIENTED_EDGE('',*,*,#39970,.T.);
#56036=ORIENTED_EDGE('',*,*,#39971,.F.);
#56037=ORIENTED_EDGE('',*,*,#39633,.T.);
#56038=ORIENTED_EDGE('',*,*,#39971,.T.);
#56039=ORIENTED_EDGE('',*,*,#39972,.T.);
#56040=ORIENTED_EDGE('',*,*,#39973,.F.);
#56041=ORIENTED_EDGE('',*,*,#39972,.F.);
#56042=ORIENTED_EDGE('',*,*,#39970,.F.);
#56043=ORIENTED_EDGE('',*,*,#39974,.F.);
#56044=ORIENTED_EDGE('',*,*,#39975,.F.);
#56045=ORIENTED_EDGE('',*,*,#39635,.T.);
#56046=ORIENTED_EDGE('',*,*,#39976,.F.);
#56047=ORIENTED_EDGE('',*,*,#39977,.T.);
#56048=ORIENTED_EDGE('',*,*,#39978,.F.);
#56049=ORIENTED_EDGE('',*,*,#39636,.T.);
#56050=ORIENTED_EDGE('',*,*,#39978,.T.);
#56051=ORIENTED_EDGE('',*,*,#39979,.T.);
#56052=ORIENTED_EDGE('',*,*,#39980,.F.);
#56053=ORIENTED_EDGE('',*,*,#39979,.F.);
#56054=ORIENTED_EDGE('',*,*,#39977,.F.);
#56055=ORIENTED_EDGE('',*,*,#39981,.F.);
#56056=ORIENTED_EDGE('',*,*,#39982,.F.);
#56057=ORIENTED_EDGE('',*,*,#39638,.T.);
#56058=ORIENTED_EDGE('',*,*,#39983,.F.);
#56059=ORIENTED_EDGE('',*,*,#39984,.T.);
#56060=ORIENTED_EDGE('',*,*,#39985,.F.);
#56061=ORIENTED_EDGE('',*,*,#39639,.T.);
#56062=ORIENTED_EDGE('',*,*,#39985,.T.);
#56063=ORIENTED_EDGE('',*,*,#39986,.T.);
#56064=ORIENTED_EDGE('',*,*,#39987,.F.);
#56065=ORIENTED_EDGE('',*,*,#39986,.F.);
#56066=ORIENTED_EDGE('',*,*,#39984,.F.);
#56067=ORIENTED_EDGE('',*,*,#39988,.F.);
#56068=ORIENTED_EDGE('',*,*,#39989,.F.);
#56069=ORIENTED_EDGE('',*,*,#39641,.T.);
#56070=ORIENTED_EDGE('',*,*,#39990,.F.);
#56071=ORIENTED_EDGE('',*,*,#39991,.T.);
#56072=ORIENTED_EDGE('',*,*,#39992,.F.);
#56073=ORIENTED_EDGE('',*,*,#39642,.T.);
#56074=ORIENTED_EDGE('',*,*,#39992,.T.);
#56075=ORIENTED_EDGE('',*,*,#39993,.T.);
#56076=ORIENTED_EDGE('',*,*,#39994,.F.);
#56077=ORIENTED_EDGE('',*,*,#39993,.F.);
#56078=ORIENTED_EDGE('',*,*,#39991,.F.);
#56079=ORIENTED_EDGE('',*,*,#39995,.F.);
#56080=ORIENTED_EDGE('',*,*,#39996,.F.);
#56081=ORIENTED_EDGE('',*,*,#39644,.T.);
#56082=ORIENTED_EDGE('',*,*,#39997,.F.);
#56083=ORIENTED_EDGE('',*,*,#39998,.T.);
#56084=ORIENTED_EDGE('',*,*,#39999,.F.);
#56085=ORIENTED_EDGE('',*,*,#39645,.T.);
#56086=ORIENTED_EDGE('',*,*,#39999,.T.);
#56087=ORIENTED_EDGE('',*,*,#40000,.T.);
#56088=ORIENTED_EDGE('',*,*,#40001,.F.);
#56089=ORIENTED_EDGE('',*,*,#40000,.F.);
#56090=ORIENTED_EDGE('',*,*,#39998,.F.);
#56091=ORIENTED_EDGE('',*,*,#40002,.F.);
#56092=ORIENTED_EDGE('',*,*,#40003,.F.);
#56093=ORIENTED_EDGE('',*,*,#39647,.T.);
#56094=ORIENTED_EDGE('',*,*,#40004,.F.);
#56095=ORIENTED_EDGE('',*,*,#40005,.T.);
#56096=ORIENTED_EDGE('',*,*,#40006,.F.);
#56097=ORIENTED_EDGE('',*,*,#39648,.T.);
#56098=ORIENTED_EDGE('',*,*,#40006,.T.);
#56099=ORIENTED_EDGE('',*,*,#40007,.T.);
#56100=ORIENTED_EDGE('',*,*,#40008,.F.);
#56101=ORIENTED_EDGE('',*,*,#40007,.F.);
#56102=ORIENTED_EDGE('',*,*,#40005,.F.);
#56103=ORIENTED_EDGE('',*,*,#40009,.F.);
#56104=ORIENTED_EDGE('',*,*,#40010,.F.);
#56105=ORIENTED_EDGE('',*,*,#39650,.T.);
#56106=ORIENTED_EDGE('',*,*,#40011,.F.);
#56107=ORIENTED_EDGE('',*,*,#40012,.T.);
#56108=ORIENTED_EDGE('',*,*,#40013,.F.);
#56109=ORIENTED_EDGE('',*,*,#39651,.T.);
#56110=ORIENTED_EDGE('',*,*,#40013,.T.);
#56111=ORIENTED_EDGE('',*,*,#40014,.T.);
#56112=ORIENTED_EDGE('',*,*,#40015,.F.);
#56113=ORIENTED_EDGE('',*,*,#40014,.F.);
#56114=ORIENTED_EDGE('',*,*,#40012,.F.);
#56115=ORIENTED_EDGE('',*,*,#40016,.F.);
#56116=ORIENTED_EDGE('',*,*,#40017,.F.);
#56117=ORIENTED_EDGE('',*,*,#39653,.T.);
#56118=ORIENTED_EDGE('',*,*,#40018,.F.);
#56119=ORIENTED_EDGE('',*,*,#40019,.T.);
#56120=ORIENTED_EDGE('',*,*,#40020,.F.);
#56121=ORIENTED_EDGE('',*,*,#39654,.T.);
#56122=ORIENTED_EDGE('',*,*,#40020,.T.);
#56123=ORIENTED_EDGE('',*,*,#40021,.T.);
#56124=ORIENTED_EDGE('',*,*,#40022,.F.);
#56125=ORIENTED_EDGE('',*,*,#40021,.F.);
#56126=ORIENTED_EDGE('',*,*,#40019,.F.);
#56127=ORIENTED_EDGE('',*,*,#40023,.F.);
#56128=ORIENTED_EDGE('',*,*,#40024,.F.);
#56129=ORIENTED_EDGE('',*,*,#39656,.T.);
#56130=ORIENTED_EDGE('',*,*,#40025,.F.);
#56131=ORIENTED_EDGE('',*,*,#40026,.T.);
#56132=ORIENTED_EDGE('',*,*,#40027,.F.);
#56133=ORIENTED_EDGE('',*,*,#39657,.T.);
#56134=ORIENTED_EDGE('',*,*,#40027,.T.);
#56135=ORIENTED_EDGE('',*,*,#40028,.T.);
#56136=ORIENTED_EDGE('',*,*,#40029,.F.);
#56137=ORIENTED_EDGE('',*,*,#40028,.F.);
#56138=ORIENTED_EDGE('',*,*,#40026,.F.);
#56139=ORIENTED_EDGE('',*,*,#40030,.F.);
#56140=ORIENTED_EDGE('',*,*,#40031,.F.);
#56141=ORIENTED_EDGE('',*,*,#39659,.T.);
#56142=ORIENTED_EDGE('',*,*,#40032,.F.);
#56143=ORIENTED_EDGE('',*,*,#40033,.T.);
#56144=ORIENTED_EDGE('',*,*,#40034,.F.);
#56145=ORIENTED_EDGE('',*,*,#39660,.T.);
#56146=ORIENTED_EDGE('',*,*,#40034,.T.);
#56147=ORIENTED_EDGE('',*,*,#40035,.T.);
#56148=ORIENTED_EDGE('',*,*,#40036,.F.);
#56149=ORIENTED_EDGE('',*,*,#40035,.F.);
#56150=ORIENTED_EDGE('',*,*,#40033,.F.);
#56151=ORIENTED_EDGE('',*,*,#40037,.F.);
#56152=ORIENTED_EDGE('',*,*,#40038,.F.);
#56153=ORIENTED_EDGE('',*,*,#39662,.T.);
#56154=ORIENTED_EDGE('',*,*,#40039,.F.);
#56155=ORIENTED_EDGE('',*,*,#40040,.T.);
#56156=ORIENTED_EDGE('',*,*,#40041,.F.);
#56157=ORIENTED_EDGE('',*,*,#39663,.T.);
#56158=ORIENTED_EDGE('',*,*,#40041,.T.);
#56159=ORIENTED_EDGE('',*,*,#40042,.T.);
#56160=ORIENTED_EDGE('',*,*,#40043,.F.);
#56161=ORIENTED_EDGE('',*,*,#40042,.F.);
#56162=ORIENTED_EDGE('',*,*,#40040,.F.);
#56163=ORIENTED_EDGE('',*,*,#40044,.F.);
#56164=ORIENTED_EDGE('',*,*,#40045,.F.);
#56165=ORIENTED_EDGE('',*,*,#39665,.T.);
#56166=ORIENTED_EDGE('',*,*,#40046,.F.);
#56167=ORIENTED_EDGE('',*,*,#40047,.T.);
#56168=ORIENTED_EDGE('',*,*,#40048,.F.);
#56169=ORIENTED_EDGE('',*,*,#39666,.T.);
#56170=ORIENTED_EDGE('',*,*,#40048,.T.);
#56171=ORIENTED_EDGE('',*,*,#40049,.T.);
#56172=ORIENTED_EDGE('',*,*,#40050,.F.);
#56173=ORIENTED_EDGE('',*,*,#40049,.F.);
#56174=ORIENTED_EDGE('',*,*,#40047,.F.);
#56175=ORIENTED_EDGE('',*,*,#40051,.F.);
#56176=ORIENTED_EDGE('',*,*,#40052,.F.);
#56177=ORIENTED_EDGE('',*,*,#39668,.T.);
#56178=ORIENTED_EDGE('',*,*,#40053,.F.);
#56179=ORIENTED_EDGE('',*,*,#40054,.T.);
#56180=ORIENTED_EDGE('',*,*,#40055,.F.);
#56181=ORIENTED_EDGE('',*,*,#39669,.T.);
#56182=ORIENTED_EDGE('',*,*,#40055,.T.);
#56183=ORIENTED_EDGE('',*,*,#40056,.T.);
#56184=ORIENTED_EDGE('',*,*,#40057,.F.);
#56185=ORIENTED_EDGE('',*,*,#40056,.F.);
#56186=ORIENTED_EDGE('',*,*,#40054,.F.);
#56187=ORIENTED_EDGE('',*,*,#40058,.F.);
#56188=ORIENTED_EDGE('',*,*,#40059,.F.);
#56189=ORIENTED_EDGE('',*,*,#39671,.T.);
#56190=ORIENTED_EDGE('',*,*,#40060,.F.);
#56191=ORIENTED_EDGE('',*,*,#40061,.T.);
#56192=ORIENTED_EDGE('',*,*,#40062,.F.);
#56193=ORIENTED_EDGE('',*,*,#40063,.T.);
#56194=ORIENTED_EDGE('',*,*,#40064,.F.);
#56195=ORIENTED_EDGE('',*,*,#39672,.T.);
#56196=ORIENTED_EDGE('',*,*,#40062,.T.);
#56197=ORIENTED_EDGE('',*,*,#40065,.F.);
#56198=ORIENTED_EDGE('',*,*,#40066,.F.);
#56199=ORIENTED_EDGE('',*,*,#40063,.F.);
#56200=ORIENTED_EDGE('',*,*,#40061,.F.);
#56201=ORIENTED_EDGE('',*,*,#39674,.T.);
#56202=ORIENTED_EDGE('',*,*,#40067,.F.);
#56203=ORIENTED_EDGE('',*,*,#40068,.T.);
#56204=ORIENTED_EDGE('',*,*,#40069,.F.);
#56205=ORIENTED_EDGE('',*,*,#39675,.T.);
#56206=ORIENTED_EDGE('',*,*,#40069,.T.);
#56207=ORIENTED_EDGE('',*,*,#40070,.T.);
#56208=ORIENTED_EDGE('',*,*,#40071,.F.);
#56209=ORIENTED_EDGE('',*,*,#40070,.F.);
#56210=ORIENTED_EDGE('',*,*,#40068,.F.);
#56211=ORIENTED_EDGE('',*,*,#40072,.F.);
#56212=ORIENTED_EDGE('',*,*,#40073,.F.);
#56213=ORIENTED_EDGE('',*,*,#39677,.T.);
#56214=ORIENTED_EDGE('',*,*,#40074,.F.);
#56215=ORIENTED_EDGE('',*,*,#40075,.T.);
#56216=ORIENTED_EDGE('',*,*,#40076,.F.);
#56217=ORIENTED_EDGE('',*,*,#39678,.T.);
#56218=ORIENTED_EDGE('',*,*,#40076,.T.);
#56219=ORIENTED_EDGE('',*,*,#40077,.T.);
#56220=ORIENTED_EDGE('',*,*,#40078,.F.);
#56221=ORIENTED_EDGE('',*,*,#40077,.F.);
#56222=ORIENTED_EDGE('',*,*,#40075,.F.);
#56223=ORIENTED_EDGE('',*,*,#40079,.F.);
#56224=ORIENTED_EDGE('',*,*,#40080,.F.);
#56225=ORIENTED_EDGE('',*,*,#40081,.F.);
#56226=ORIENTED_EDGE('',*,*,#40082,.F.);
#56227=ORIENTED_EDGE('',*,*,#39682,.T.);
#56228=ORIENTED_EDGE('',*,*,#39681,.T.);
#56229=ORIENTED_EDGE('',*,*,#40083,.F.);
#56230=ORIENTED_EDGE('',*,*,#39685,.T.);
#56231=ORIENTED_EDGE('',*,*,#39683,.T.);
#56232=ORIENTED_EDGE('',*,*,#40082,.T.);
#56233=ORIENTED_EDGE('',*,*,#40084,.F.);
#56234=ORIENTED_EDGE('',*,*,#40085,.F.);
#56235=ORIENTED_EDGE('',*,*,#39689,.T.);
#56236=ORIENTED_EDGE('',*,*,#39688,.T.);
#56237=ORIENTED_EDGE('',*,*,#40086,.F.);
#56238=ORIENTED_EDGE('',*,*,#39692,.T.);
#56239=ORIENTED_EDGE('',*,*,#39690,.T.);
#56240=ORIENTED_EDGE('',*,*,#40085,.T.);
#56241=ORIENTED_EDGE('',*,*,#40087,.F.);
#56242=ORIENTED_EDGE('',*,*,#40088,.F.);
#56243=ORIENTED_EDGE('',*,*,#39696,.T.);
#56244=ORIENTED_EDGE('',*,*,#39695,.T.);
#56245=ORIENTED_EDGE('',*,*,#40089,.F.);
#56246=ORIENTED_EDGE('',*,*,#39699,.T.);
#56247=ORIENTED_EDGE('',*,*,#39697,.T.);
#56248=ORIENTED_EDGE('',*,*,#40088,.T.);
#56249=ORIENTED_EDGE('',*,*,#40090,.F.);
#56250=ORIENTED_EDGE('',*,*,#40091,.F.);
#56251=ORIENTED_EDGE('',*,*,#39703,.T.);
#56252=ORIENTED_EDGE('',*,*,#39702,.T.);
#56253=ORIENTED_EDGE('',*,*,#40092,.F.);
#56254=ORIENTED_EDGE('',*,*,#39706,.T.);
#56255=ORIENTED_EDGE('',*,*,#39704,.T.);
#56256=ORIENTED_EDGE('',*,*,#40091,.T.);
#56257=ORIENTED_EDGE('',*,*,#40093,.F.);
#56258=ORIENTED_EDGE('',*,*,#40094,.F.);
#56259=ORIENTED_EDGE('',*,*,#39710,.T.);
#56260=ORIENTED_EDGE('',*,*,#39709,.T.);
#56261=ORIENTED_EDGE('',*,*,#40095,.F.);
#56262=ORIENTED_EDGE('',*,*,#39713,.T.);
#56263=ORIENTED_EDGE('',*,*,#39711,.T.);
#56264=ORIENTED_EDGE('',*,*,#40094,.T.);
#56265=ORIENTED_EDGE('',*,*,#40096,.F.);
#56266=ORIENTED_EDGE('',*,*,#40097,.F.);
#56267=ORIENTED_EDGE('',*,*,#39717,.T.);
#56268=ORIENTED_EDGE('',*,*,#39716,.T.);
#56269=ORIENTED_EDGE('',*,*,#40098,.F.);
#56270=ORIENTED_EDGE('',*,*,#39720,.T.);
#56271=ORIENTED_EDGE('',*,*,#39718,.T.);
#56272=ORIENTED_EDGE('',*,*,#40097,.T.);
#56273=ORIENTED_EDGE('',*,*,#40099,.F.);
#56274=ORIENTED_EDGE('',*,*,#40100,.F.);
#56275=ORIENTED_EDGE('',*,*,#39724,.T.);
#56276=ORIENTED_EDGE('',*,*,#39723,.T.);
#56277=ORIENTED_EDGE('',*,*,#40101,.F.);
#56278=ORIENTED_EDGE('',*,*,#39727,.T.);
#56279=ORIENTED_EDGE('',*,*,#39725,.T.);
#56280=ORIENTED_EDGE('',*,*,#40100,.T.);
#56281=ORIENTED_EDGE('',*,*,#40102,.F.);
#56282=ORIENTED_EDGE('',*,*,#40103,.F.);
#56283=ORIENTED_EDGE('',*,*,#39731,.T.);
#56284=ORIENTED_EDGE('',*,*,#39730,.T.);
#56285=ORIENTED_EDGE('',*,*,#40104,.F.);
#56286=ORIENTED_EDGE('',*,*,#39734,.T.);
#56287=ORIENTED_EDGE('',*,*,#39732,.T.);
#56288=ORIENTED_EDGE('',*,*,#40103,.T.);
#56289=ORIENTED_EDGE('',*,*,#40105,.F.);
#56290=ORIENTED_EDGE('',*,*,#40106,.F.);
#56291=ORIENTED_EDGE('',*,*,#39738,.T.);
#56292=ORIENTED_EDGE('',*,*,#39737,.T.);
#56293=ORIENTED_EDGE('',*,*,#40107,.F.);
#56294=ORIENTED_EDGE('',*,*,#39741,.T.);
#56295=ORIENTED_EDGE('',*,*,#39739,.T.);
#56296=ORIENTED_EDGE('',*,*,#40106,.T.);
#56297=ORIENTED_EDGE('',*,*,#40108,.F.);
#56298=ORIENTED_EDGE('',*,*,#40109,.F.);
#56299=ORIENTED_EDGE('',*,*,#39745,.T.);
#56300=ORIENTED_EDGE('',*,*,#39744,.T.);
#56301=ORIENTED_EDGE('',*,*,#40110,.F.);
#56302=ORIENTED_EDGE('',*,*,#39748,.T.);
#56303=ORIENTED_EDGE('',*,*,#39746,.T.);
#56304=ORIENTED_EDGE('',*,*,#40109,.T.);
#56305=ORIENTED_EDGE('',*,*,#40111,.F.);
#56306=ORIENTED_EDGE('',*,*,#40112,.F.);
#56307=ORIENTED_EDGE('',*,*,#39752,.T.);
#56308=ORIENTED_EDGE('',*,*,#39751,.T.);
#56309=ORIENTED_EDGE('',*,*,#40113,.F.);
#56310=ORIENTED_EDGE('',*,*,#39755,.T.);
#56311=ORIENTED_EDGE('',*,*,#39753,.T.);
#56312=ORIENTED_EDGE('',*,*,#40112,.T.);
#56313=ORIENTED_EDGE('',*,*,#40114,.F.);
#56314=ORIENTED_EDGE('',*,*,#40115,.F.);
#56315=ORIENTED_EDGE('',*,*,#39759,.T.);
#56316=ORIENTED_EDGE('',*,*,#39758,.T.);
#56317=ORIENTED_EDGE('',*,*,#40116,.F.);
#56318=ORIENTED_EDGE('',*,*,#39762,.T.);
#56319=ORIENTED_EDGE('',*,*,#39760,.T.);
#56320=ORIENTED_EDGE('',*,*,#40115,.T.);
#56321=ORIENTED_EDGE('',*,*,#40117,.F.);
#56322=ORIENTED_EDGE('',*,*,#40118,.F.);
#56323=ORIENTED_EDGE('',*,*,#39766,.T.);
#56324=ORIENTED_EDGE('',*,*,#39765,.T.);
#56325=ORIENTED_EDGE('',*,*,#40119,.F.);
#56326=ORIENTED_EDGE('',*,*,#39769,.T.);
#56327=ORIENTED_EDGE('',*,*,#39767,.T.);
#56328=ORIENTED_EDGE('',*,*,#40118,.T.);
#56329=ORIENTED_EDGE('',*,*,#40120,.F.);
#56330=ORIENTED_EDGE('',*,*,#40121,.F.);
#56331=ORIENTED_EDGE('',*,*,#39773,.T.);
#56332=ORIENTED_EDGE('',*,*,#39772,.T.);
#56333=ORIENTED_EDGE('',*,*,#40122,.F.);
#56334=ORIENTED_EDGE('',*,*,#39776,.T.);
#56335=ORIENTED_EDGE('',*,*,#39774,.T.);
#56336=ORIENTED_EDGE('',*,*,#40121,.T.);
#56337=ORIENTED_EDGE('',*,*,#40123,.F.);
#56338=ORIENTED_EDGE('',*,*,#40124,.F.);
#56339=ORIENTED_EDGE('',*,*,#34398,.T.);
#56340=ORIENTED_EDGE('',*,*,#39778,.T.);
#56341=ORIENTED_EDGE('',*,*,#40125,.F.);
#56342=ORIENTED_EDGE('',*,*,#39779,.T.);
#56343=ORIENTED_EDGE('',*,*,#34399,.T.);
#56344=ORIENTED_EDGE('',*,*,#40124,.T.);
#56345=ORIENTED_EDGE('',*,*,#40126,.F.);
#56346=ORIENTED_EDGE('',*,*,#40127,.F.);
#56347=ORIENTED_EDGE('',*,*,#39783,.T.);
#56348=ORIENTED_EDGE('',*,*,#39782,.T.);
#56349=ORIENTED_EDGE('',*,*,#40128,.F.);
#56350=ORIENTED_EDGE('',*,*,#39786,.T.);
#56351=ORIENTED_EDGE('',*,*,#39784,.T.);
#56352=ORIENTED_EDGE('',*,*,#40127,.T.);
#56353=ORIENTED_EDGE('',*,*,#40129,.F.);
#56354=ORIENTED_EDGE('',*,*,#40130,.F.);
#56355=ORIENTED_EDGE('',*,*,#39790,.T.);
#56356=ORIENTED_EDGE('',*,*,#39789,.T.);
#56357=ORIENTED_EDGE('',*,*,#40131,.F.);
#56358=ORIENTED_EDGE('',*,*,#39793,.T.);
#56359=ORIENTED_EDGE('',*,*,#39791,.T.);
#56360=ORIENTED_EDGE('',*,*,#40130,.T.);
#56361=ORIENTED_EDGE('',*,*,#40132,.F.);
#56362=ORIENTED_EDGE('',*,*,#40133,.F.);
#56363=ORIENTED_EDGE('',*,*,#39797,.T.);
#56364=ORIENTED_EDGE('',*,*,#39796,.T.);
#56365=ORIENTED_EDGE('',*,*,#40134,.F.);
#56366=ORIENTED_EDGE('',*,*,#39800,.T.);
#56367=ORIENTED_EDGE('',*,*,#39798,.T.);
#56368=ORIENTED_EDGE('',*,*,#40133,.T.);
#56369=ORIENTED_EDGE('',*,*,#40135,.F.);
#56370=ORIENTED_EDGE('',*,*,#40136,.F.);
#56371=ORIENTED_EDGE('',*,*,#39804,.T.);
#56372=ORIENTED_EDGE('',*,*,#39803,.T.);
#56373=ORIENTED_EDGE('',*,*,#40137,.F.);
#56374=ORIENTED_EDGE('',*,*,#39807,.T.);
#56375=ORIENTED_EDGE('',*,*,#39805,.T.);
#56376=ORIENTED_EDGE('',*,*,#40136,.T.);
#56377=ORIENTED_EDGE('',*,*,#40138,.F.);
#56378=ORIENTED_EDGE('',*,*,#40139,.F.);
#56379=ORIENTED_EDGE('',*,*,#39811,.T.);
#56380=ORIENTED_EDGE('',*,*,#39810,.T.);
#56381=ORIENTED_EDGE('',*,*,#40140,.F.);
#56382=ORIENTED_EDGE('',*,*,#39814,.T.);
#56383=ORIENTED_EDGE('',*,*,#39812,.T.);
#56384=ORIENTED_EDGE('',*,*,#40139,.T.);
#56385=ORIENTED_EDGE('',*,*,#40141,.F.);
#56386=ORIENTED_EDGE('',*,*,#40142,.F.);
#56387=ORIENTED_EDGE('',*,*,#39820,.T.);
#56388=ORIENTED_EDGE('',*,*,#39817,.T.);
#56389=ORIENTED_EDGE('',*,*,#39821,.T.);
#56390=ORIENTED_EDGE('',*,*,#40142,.T.);
#56391=ORIENTED_EDGE('',*,*,#40143,.F.);
#56392=ORIENTED_EDGE('',*,*,#39819,.T.);
#56393=ORIENTED_EDGE('',*,*,#39826,.T.);
#56394=ORIENTED_EDGE('',*,*,#39822,.T.);
#56395=ORIENTED_EDGE('',*,*,#40144,.F.);
#56396=ORIENTED_EDGE('',*,*,#40145,.F.);
#56397=ORIENTED_EDGE('',*,*,#40146,.F.);
#56398=ORIENTED_EDGE('',*,*,#39828,.T.);
#56399=ORIENTED_EDGE('',*,*,#39827,.T.);
#56400=ORIENTED_EDGE('',*,*,#40145,.T.);
#56401=ORIENTED_EDGE('',*,*,#40147,.F.);
#56402=ORIENTED_EDGE('',*,*,#40148,.F.);
#56403=ORIENTED_EDGE('',*,*,#39832,.T.);
#56404=ORIENTED_EDGE('',*,*,#39831,.T.);
#56405=ORIENTED_EDGE('',*,*,#40149,.F.);
#56406=ORIENTED_EDGE('',*,*,#39835,.T.);
#56407=ORIENTED_EDGE('',*,*,#39833,.T.);
#56408=ORIENTED_EDGE('',*,*,#40148,.T.);
#56409=ORIENTED_EDGE('',*,*,#40150,.F.);
#56410=ORIENTED_EDGE('',*,*,#40151,.F.);
#56411=ORIENTED_EDGE('',*,*,#39839,.T.);
#56412=ORIENTED_EDGE('',*,*,#39838,.T.);
#56413=ORIENTED_EDGE('',*,*,#40152,.F.);
#56414=ORIENTED_EDGE('',*,*,#39842,.T.);
#56415=ORIENTED_EDGE('',*,*,#39840,.T.);
#56416=ORIENTED_EDGE('',*,*,#40151,.T.);
#56417=ORIENTED_EDGE('',*,*,#40153,.F.);
#56418=ORIENTED_EDGE('',*,*,#40154,.F.);
#56419=ORIENTED_EDGE('',*,*,#39846,.T.);
#56420=ORIENTED_EDGE('',*,*,#39845,.T.);
#56421=ORIENTED_EDGE('',*,*,#40155,.F.);
#56422=ORIENTED_EDGE('',*,*,#39849,.T.);
#56423=ORIENTED_EDGE('',*,*,#39847,.T.);
#56424=ORIENTED_EDGE('',*,*,#40154,.T.);
#56425=ORIENTED_EDGE('',*,*,#40156,.F.);
#56426=ORIENTED_EDGE('',*,*,#40157,.F.);
#56427=ORIENTED_EDGE('',*,*,#39853,.T.);
#56428=ORIENTED_EDGE('',*,*,#39852,.T.);
#56429=ORIENTED_EDGE('',*,*,#40158,.F.);
#56430=ORIENTED_EDGE('',*,*,#39856,.T.);
#56431=ORIENTED_EDGE('',*,*,#39854,.T.);
#56432=ORIENTED_EDGE('',*,*,#40157,.T.);
#56433=ORIENTED_EDGE('',*,*,#40159,.F.);
#56434=ORIENTED_EDGE('',*,*,#40160,.F.);
#56435=ORIENTED_EDGE('',*,*,#39860,.T.);
#56436=ORIENTED_EDGE('',*,*,#39859,.T.);
#56437=ORIENTED_EDGE('',*,*,#40161,.F.);
#56438=ORIENTED_EDGE('',*,*,#39863,.T.);
#56439=ORIENTED_EDGE('',*,*,#39861,.T.);
#56440=ORIENTED_EDGE('',*,*,#40160,.T.);
#56441=ORIENTED_EDGE('',*,*,#40162,.F.);
#56442=ORIENTED_EDGE('',*,*,#40163,.F.);
#56443=ORIENTED_EDGE('',*,*,#39867,.T.);
#56444=ORIENTED_EDGE('',*,*,#39866,.T.);
#56445=ORIENTED_EDGE('',*,*,#40164,.F.);
#56446=ORIENTED_EDGE('',*,*,#39870,.T.);
#56447=ORIENTED_EDGE('',*,*,#39868,.T.);
#56448=ORIENTED_EDGE('',*,*,#40163,.T.);
#56449=ORIENTED_EDGE('',*,*,#40165,.F.);
#56450=ORIENTED_EDGE('',*,*,#40166,.F.);
#56451=ORIENTED_EDGE('',*,*,#39874,.T.);
#56452=ORIENTED_EDGE('',*,*,#39873,.T.);
#56453=ORIENTED_EDGE('',*,*,#40167,.F.);
#56454=ORIENTED_EDGE('',*,*,#39877,.T.);
#56455=ORIENTED_EDGE('',*,*,#39875,.T.);
#56456=ORIENTED_EDGE('',*,*,#40166,.T.);
#56457=ORIENTED_EDGE('',*,*,#39883,.T.);
#56458=ORIENTED_EDGE('',*,*,#39878,.T.);
#56459=ORIENTED_EDGE('',*,*,#40168,.F.);
#56460=ORIENTED_EDGE('',*,*,#40169,.F.);
#56461=ORIENTED_EDGE('',*,*,#39884,.T.);
#56462=ORIENTED_EDGE('',*,*,#40169,.T.);
#56463=ORIENTED_EDGE('',*,*,#40170,.F.);
#56464=ORIENTED_EDGE('',*,*,#39882,.T.);
#56465=ORIENTED_EDGE('',*,*,#39890,.T.);
#56466=ORIENTED_EDGE('',*,*,#39885,.T.);
#56467=ORIENTED_EDGE('',*,*,#40171,.F.);
#56468=ORIENTED_EDGE('',*,*,#40172,.F.);
#56469=ORIENTED_EDGE('',*,*,#39891,.T.);
#56470=ORIENTED_EDGE('',*,*,#40172,.T.);
#56471=ORIENTED_EDGE('',*,*,#40173,.F.);
#56472=ORIENTED_EDGE('',*,*,#39889,.T.);
#56473=ORIENTED_EDGE('',*,*,#39897,.T.);
#56474=ORIENTED_EDGE('',*,*,#39892,.T.);
#56475=ORIENTED_EDGE('',*,*,#40174,.F.);
#56476=ORIENTED_EDGE('',*,*,#40175,.F.);
#56477=ORIENTED_EDGE('',*,*,#39898,.T.);
#56478=ORIENTED_EDGE('',*,*,#40175,.T.);
#56479=ORIENTED_EDGE('',*,*,#40176,.F.);
#56480=ORIENTED_EDGE('',*,*,#39896,.T.);
#56481=ORIENTED_EDGE('',*,*,#39904,.T.);
#56482=ORIENTED_EDGE('',*,*,#39899,.T.);
#56483=ORIENTED_EDGE('',*,*,#40177,.F.);
#56484=ORIENTED_EDGE('',*,*,#40178,.F.);
#56485=ORIENTED_EDGE('',*,*,#39905,.T.);
#56486=ORIENTED_EDGE('',*,*,#40178,.T.);
#56487=ORIENTED_EDGE('',*,*,#40179,.F.);
#56488=ORIENTED_EDGE('',*,*,#39903,.T.);
#56489=ORIENTED_EDGE('',*,*,#39911,.T.);
#56490=ORIENTED_EDGE('',*,*,#39906,.T.);
#56491=ORIENTED_EDGE('',*,*,#40180,.F.);
#56492=ORIENTED_EDGE('',*,*,#40181,.F.);
#56493=ORIENTED_EDGE('',*,*,#39912,.T.);
#56494=ORIENTED_EDGE('',*,*,#40181,.T.);
#56495=ORIENTED_EDGE('',*,*,#40182,.F.);
#56496=ORIENTED_EDGE('',*,*,#39910,.T.);
#56497=ORIENTED_EDGE('',*,*,#39918,.T.);
#56498=ORIENTED_EDGE('',*,*,#39913,.T.);
#56499=ORIENTED_EDGE('',*,*,#40183,.F.);
#56500=ORIENTED_EDGE('',*,*,#40184,.F.);
#56501=ORIENTED_EDGE('',*,*,#39919,.T.);
#56502=ORIENTED_EDGE('',*,*,#40184,.T.);
#56503=ORIENTED_EDGE('',*,*,#40185,.F.);
#56504=ORIENTED_EDGE('',*,*,#39917,.T.);
#56505=ORIENTED_EDGE('',*,*,#39925,.T.);
#56506=ORIENTED_EDGE('',*,*,#39920,.T.);
#56507=ORIENTED_EDGE('',*,*,#40186,.F.);
#56508=ORIENTED_EDGE('',*,*,#40187,.F.);
#56509=ORIENTED_EDGE('',*,*,#39926,.T.);
#56510=ORIENTED_EDGE('',*,*,#40187,.T.);
#56511=ORIENTED_EDGE('',*,*,#40188,.F.);
#56512=ORIENTED_EDGE('',*,*,#39924,.T.);
#56513=ORIENTED_EDGE('',*,*,#39932,.T.);
#56514=ORIENTED_EDGE('',*,*,#39927,.T.);
#56515=ORIENTED_EDGE('',*,*,#40189,.F.);
#56516=ORIENTED_EDGE('',*,*,#40190,.F.);
#56517=ORIENTED_EDGE('',*,*,#39933,.T.);
#56518=ORIENTED_EDGE('',*,*,#40190,.T.);
#56519=ORIENTED_EDGE('',*,*,#40191,.F.);
#56520=ORIENTED_EDGE('',*,*,#39931,.T.);
#56521=ORIENTED_EDGE('',*,*,#39939,.T.);
#56522=ORIENTED_EDGE('',*,*,#39934,.T.);
#56523=ORIENTED_EDGE('',*,*,#40192,.F.);
#56524=ORIENTED_EDGE('',*,*,#40193,.F.);
#56525=ORIENTED_EDGE('',*,*,#39940,.T.);
#56526=ORIENTED_EDGE('',*,*,#40193,.T.);
#56527=ORIENTED_EDGE('',*,*,#40194,.F.);
#56528=ORIENTED_EDGE('',*,*,#39938,.T.);
#56529=ORIENTED_EDGE('',*,*,#39946,.T.);
#56530=ORIENTED_EDGE('',*,*,#39941,.T.);
#56531=ORIENTED_EDGE('',*,*,#40195,.F.);
#56532=ORIENTED_EDGE('',*,*,#40196,.F.);
#56533=ORIENTED_EDGE('',*,*,#39947,.T.);
#56534=ORIENTED_EDGE('',*,*,#40196,.T.);
#56535=ORIENTED_EDGE('',*,*,#40197,.F.);
#56536=ORIENTED_EDGE('',*,*,#39945,.T.);
#56537=ORIENTED_EDGE('',*,*,#39953,.T.);
#56538=ORIENTED_EDGE('',*,*,#39948,.T.);
#56539=ORIENTED_EDGE('',*,*,#40198,.F.);
#56540=ORIENTED_EDGE('',*,*,#40199,.F.);
#56541=ORIENTED_EDGE('',*,*,#39954,.T.);
#56542=ORIENTED_EDGE('',*,*,#40199,.T.);
#56543=ORIENTED_EDGE('',*,*,#40200,.F.);
#56544=ORIENTED_EDGE('',*,*,#39952,.T.);
#56545=ORIENTED_EDGE('',*,*,#39960,.T.);
#56546=ORIENTED_EDGE('',*,*,#39955,.T.);
#56547=ORIENTED_EDGE('',*,*,#40201,.F.);
#56548=ORIENTED_EDGE('',*,*,#40202,.F.);
#56549=ORIENTED_EDGE('',*,*,#39961,.T.);
#56550=ORIENTED_EDGE('',*,*,#40202,.T.);
#56551=ORIENTED_EDGE('',*,*,#40203,.F.);
#56552=ORIENTED_EDGE('',*,*,#39959,.T.);
#56553=ORIENTED_EDGE('',*,*,#39967,.T.);
#56554=ORIENTED_EDGE('',*,*,#39962,.T.);
#56555=ORIENTED_EDGE('',*,*,#40204,.F.);
#56556=ORIENTED_EDGE('',*,*,#40205,.F.);
#56557=ORIENTED_EDGE('',*,*,#39968,.T.);
#56558=ORIENTED_EDGE('',*,*,#40205,.T.);
#56559=ORIENTED_EDGE('',*,*,#40206,.F.);
#56560=ORIENTED_EDGE('',*,*,#39966,.T.);
#56561=ORIENTED_EDGE('',*,*,#39974,.T.);
#56562=ORIENTED_EDGE('',*,*,#39969,.T.);
#56563=ORIENTED_EDGE('',*,*,#40207,.F.);
#56564=ORIENTED_EDGE('',*,*,#40208,.F.);
#56565=ORIENTED_EDGE('',*,*,#39975,.T.);
#56566=ORIENTED_EDGE('',*,*,#40208,.T.);
#56567=ORIENTED_EDGE('',*,*,#40209,.F.);
#56568=ORIENTED_EDGE('',*,*,#39973,.T.);
#56569=ORIENTED_EDGE('',*,*,#39981,.T.);
#56570=ORIENTED_EDGE('',*,*,#39976,.T.);
#56571=ORIENTED_EDGE('',*,*,#40210,.F.);
#56572=ORIENTED_EDGE('',*,*,#40211,.F.);
#56573=ORIENTED_EDGE('',*,*,#39982,.T.);
#56574=ORIENTED_EDGE('',*,*,#40211,.T.);
#56575=ORIENTED_EDGE('',*,*,#40212,.F.);
#56576=ORIENTED_EDGE('',*,*,#39980,.T.);
#56577=ORIENTED_EDGE('',*,*,#39988,.T.);
#56578=ORIENTED_EDGE('',*,*,#39983,.T.);
#56579=ORIENTED_EDGE('',*,*,#40213,.F.);
#56580=ORIENTED_EDGE('',*,*,#40214,.F.);
#56581=ORIENTED_EDGE('',*,*,#39989,.T.);
#56582=ORIENTED_EDGE('',*,*,#40214,.T.);
#56583=ORIENTED_EDGE('',*,*,#40215,.F.);
#56584=ORIENTED_EDGE('',*,*,#39987,.T.);
#56585=ORIENTED_EDGE('',*,*,#39995,.T.);
#56586=ORIENTED_EDGE('',*,*,#39990,.T.);
#56587=ORIENTED_EDGE('',*,*,#40216,.F.);
#56588=ORIENTED_EDGE('',*,*,#40217,.F.);
#56589=ORIENTED_EDGE('',*,*,#39996,.T.);
#56590=ORIENTED_EDGE('',*,*,#40217,.T.);
#56591=ORIENTED_EDGE('',*,*,#40218,.F.);
#56592=ORIENTED_EDGE('',*,*,#39994,.T.);
#56593=ORIENTED_EDGE('',*,*,#40002,.T.);
#56594=ORIENTED_EDGE('',*,*,#39997,.T.);
#56595=ORIENTED_EDGE('',*,*,#40219,.F.);
#56596=ORIENTED_EDGE('',*,*,#40220,.F.);
#56597=ORIENTED_EDGE('',*,*,#40003,.T.);
#56598=ORIENTED_EDGE('',*,*,#40220,.T.);
#56599=ORIENTED_EDGE('',*,*,#40221,.F.);
#56600=ORIENTED_EDGE('',*,*,#40001,.T.);
#56601=ORIENTED_EDGE('',*,*,#40009,.T.);
#56602=ORIENTED_EDGE('',*,*,#40004,.T.);
#56603=ORIENTED_EDGE('',*,*,#40222,.F.);
#56604=ORIENTED_EDGE('',*,*,#40223,.F.);
#56605=ORIENTED_EDGE('',*,*,#40010,.T.);
#56606=ORIENTED_EDGE('',*,*,#40223,.T.);
#56607=ORIENTED_EDGE('',*,*,#40224,.F.);
#56608=ORIENTED_EDGE('',*,*,#40008,.T.);
#56609=ORIENTED_EDGE('',*,*,#40016,.T.);
#56610=ORIENTED_EDGE('',*,*,#40011,.T.);
#56611=ORIENTED_EDGE('',*,*,#40225,.F.);
#56612=ORIENTED_EDGE('',*,*,#40226,.F.);
#56613=ORIENTED_EDGE('',*,*,#40017,.T.);
#56614=ORIENTED_EDGE('',*,*,#40226,.T.);
#56615=ORIENTED_EDGE('',*,*,#40227,.F.);
#56616=ORIENTED_EDGE('',*,*,#40015,.T.);
#56617=ORIENTED_EDGE('',*,*,#40023,.T.);
#56618=ORIENTED_EDGE('',*,*,#40018,.T.);
#56619=ORIENTED_EDGE('',*,*,#40228,.F.);
#56620=ORIENTED_EDGE('',*,*,#40229,.F.);
#56621=ORIENTED_EDGE('',*,*,#40024,.T.);
#56622=ORIENTED_EDGE('',*,*,#40229,.T.);
#56623=ORIENTED_EDGE('',*,*,#40230,.F.);
#56624=ORIENTED_EDGE('',*,*,#40022,.T.);
#56625=ORIENTED_EDGE('',*,*,#40030,.T.);
#56626=ORIENTED_EDGE('',*,*,#40025,.T.);
#56627=ORIENTED_EDGE('',*,*,#40231,.F.);
#56628=ORIENTED_EDGE('',*,*,#40232,.F.);
#56629=ORIENTED_EDGE('',*,*,#40031,.T.);
#56630=ORIENTED_EDGE('',*,*,#40232,.T.);
#56631=ORIENTED_EDGE('',*,*,#40233,.F.);
#56632=ORIENTED_EDGE('',*,*,#40029,.T.);
#56633=ORIENTED_EDGE('',*,*,#40037,.T.);
#56634=ORIENTED_EDGE('',*,*,#40032,.T.);
#56635=ORIENTED_EDGE('',*,*,#40234,.F.);
#56636=ORIENTED_EDGE('',*,*,#40235,.F.);
#56637=ORIENTED_EDGE('',*,*,#40038,.T.);
#56638=ORIENTED_EDGE('',*,*,#40235,.T.);
#56639=ORIENTED_EDGE('',*,*,#40236,.F.);
#56640=ORIENTED_EDGE('',*,*,#40036,.T.);
#56641=ORIENTED_EDGE('',*,*,#40044,.T.);
#56642=ORIENTED_EDGE('',*,*,#40039,.T.);
#56643=ORIENTED_EDGE('',*,*,#40237,.F.);
#56644=ORIENTED_EDGE('',*,*,#40238,.F.);
#56645=ORIENTED_EDGE('',*,*,#40045,.T.);
#56646=ORIENTED_EDGE('',*,*,#40238,.T.);
#56647=ORIENTED_EDGE('',*,*,#40239,.F.);
#56648=ORIENTED_EDGE('',*,*,#40043,.T.);
#56649=ORIENTED_EDGE('',*,*,#40051,.T.);
#56650=ORIENTED_EDGE('',*,*,#40046,.T.);
#56651=ORIENTED_EDGE('',*,*,#40240,.F.);
#56652=ORIENTED_EDGE('',*,*,#40241,.F.);
#56653=ORIENTED_EDGE('',*,*,#40052,.T.);
#56654=ORIENTED_EDGE('',*,*,#40241,.T.);
#56655=ORIENTED_EDGE('',*,*,#40242,.F.);
#56656=ORIENTED_EDGE('',*,*,#40050,.T.);
#56657=ORIENTED_EDGE('',*,*,#40058,.T.);
#56658=ORIENTED_EDGE('',*,*,#40053,.T.);
#56659=ORIENTED_EDGE('',*,*,#40243,.F.);
#56660=ORIENTED_EDGE('',*,*,#40244,.F.);
#56661=ORIENTED_EDGE('',*,*,#40059,.T.);
#56662=ORIENTED_EDGE('',*,*,#40244,.T.);
#56663=ORIENTED_EDGE('',*,*,#40245,.F.);
#56664=ORIENTED_EDGE('',*,*,#40057,.T.);
#56665=ORIENTED_EDGE('',*,*,#40246,.F.);
#56666=ORIENTED_EDGE('',*,*,#40247,.F.);
#56667=ORIENTED_EDGE('',*,*,#40065,.T.);
#56668=ORIENTED_EDGE('',*,*,#40060,.T.);
#56669=ORIENTED_EDGE('',*,*,#40066,.T.);
#56670=ORIENTED_EDGE('',*,*,#40247,.T.);
#56671=ORIENTED_EDGE('',*,*,#40248,.F.);
#56672=ORIENTED_EDGE('',*,*,#40064,.T.);
#56673=ORIENTED_EDGE('',*,*,#40072,.T.);
#56674=ORIENTED_EDGE('',*,*,#40067,.T.);
#56675=ORIENTED_EDGE('',*,*,#40249,.F.);
#56676=ORIENTED_EDGE('',*,*,#40250,.F.);
#56677=ORIENTED_EDGE('',*,*,#40073,.T.);
#56678=ORIENTED_EDGE('',*,*,#40250,.T.);
#56679=ORIENTED_EDGE('',*,*,#40251,.F.);
#56680=ORIENTED_EDGE('',*,*,#40071,.T.);
#56681=ORIENTED_EDGE('',*,*,#40079,.T.);
#56682=ORIENTED_EDGE('',*,*,#40074,.T.);
#56683=ORIENTED_EDGE('',*,*,#40252,.F.);
#56684=ORIENTED_EDGE('',*,*,#40253,.F.);
#56685=ORIENTED_EDGE('',*,*,#40080,.T.);
#56686=ORIENTED_EDGE('',*,*,#40253,.T.);
#56687=ORIENTED_EDGE('',*,*,#40254,.F.);
#56688=ORIENTED_EDGE('',*,*,#40078,.T.);
#56689=ORIENTED_EDGE('',*,*,#40255,.T.);
#56690=ORIENTED_EDGE('',*,*,#40256,.F.);
#56691=ORIENTED_EDGE('',*,*,#40081,.T.);
#56692=ORIENTED_EDGE('',*,*,#40257,.F.);
#56693=ORIENTED_EDGE('',*,*,#40258,.T.);
#56694=ORIENTED_EDGE('',*,*,#40259,.F.);
#56695=ORIENTED_EDGE('',*,*,#40083,.T.);
#56696=ORIENTED_EDGE('',*,*,#40260,.F.);
#56697=ORIENTED_EDGE('',*,*,#40261,.F.);
#56698=ORIENTED_EDGE('',*,*,#40262,.F.);
#56699=ORIENTED_EDGE('',*,*,#40263,.F.);
#56700=ORIENTED_EDGE('',*,*,#40258,.F.);
#56701=ORIENTED_EDGE('',*,*,#40263,.T.);
#56702=ORIENTED_EDGE('',*,*,#40264,.F.);
#56703=ORIENTED_EDGE('',*,*,#40084,.T.);
#56704=ORIENTED_EDGE('',*,*,#40259,.T.);
#56705=ORIENTED_EDGE('',*,*,#40265,.T.);
#56706=ORIENTED_EDGE('',*,*,#40266,.F.);
#56707=ORIENTED_EDGE('',*,*,#40086,.T.);
#56708=ORIENTED_EDGE('',*,*,#40267,.F.);
#56709=ORIENTED_EDGE('',*,*,#40268,.F.);
#56710=ORIENTED_EDGE('',*,*,#40269,.F.);
#56711=ORIENTED_EDGE('',*,*,#40270,.F.);
#56712=ORIENTED_EDGE('',*,*,#40265,.F.);
#56713=ORIENTED_EDGE('',*,*,#40270,.T.);
#56714=ORIENTED_EDGE('',*,*,#40271,.F.);
#56715=ORIENTED_EDGE('',*,*,#40087,.T.);
#56716=ORIENTED_EDGE('',*,*,#40266,.T.);
#56717=ORIENTED_EDGE('',*,*,#40272,.T.);
#56718=ORIENTED_EDGE('',*,*,#40273,.F.);
#56719=ORIENTED_EDGE('',*,*,#40089,.T.);
#56720=ORIENTED_EDGE('',*,*,#40274,.F.);
#56721=ORIENTED_EDGE('',*,*,#40275,.F.);
#56722=ORIENTED_EDGE('',*,*,#40276,.F.);
#56723=ORIENTED_EDGE('',*,*,#40277,.F.);
#56724=ORIENTED_EDGE('',*,*,#40272,.F.);
#56725=ORIENTED_EDGE('',*,*,#40277,.T.);
#56726=ORIENTED_EDGE('',*,*,#40278,.F.);
#56727=ORIENTED_EDGE('',*,*,#40090,.T.);
#56728=ORIENTED_EDGE('',*,*,#40273,.T.);
#56729=ORIENTED_EDGE('',*,*,#40279,.T.);
#56730=ORIENTED_EDGE('',*,*,#40280,.F.);
#56731=ORIENTED_EDGE('',*,*,#40092,.T.);
#56732=ORIENTED_EDGE('',*,*,#40281,.F.);
#56733=ORIENTED_EDGE('',*,*,#40282,.F.);
#56734=ORIENTED_EDGE('',*,*,#40283,.F.);
#56735=ORIENTED_EDGE('',*,*,#40284,.F.);
#56736=ORIENTED_EDGE('',*,*,#40279,.F.);
#56737=ORIENTED_EDGE('',*,*,#40284,.T.);
#56738=ORIENTED_EDGE('',*,*,#40285,.F.);
#56739=ORIENTED_EDGE('',*,*,#40093,.T.);
#56740=ORIENTED_EDGE('',*,*,#40280,.T.);
#56741=ORIENTED_EDGE('',*,*,#40286,.T.);
#56742=ORIENTED_EDGE('',*,*,#40287,.F.);
#56743=ORIENTED_EDGE('',*,*,#40095,.T.);
#56744=ORIENTED_EDGE('',*,*,#40288,.F.);
#56745=ORIENTED_EDGE('',*,*,#40289,.F.);
#56746=ORIENTED_EDGE('',*,*,#40290,.F.);
#56747=ORIENTED_EDGE('',*,*,#40291,.F.);
#56748=ORIENTED_EDGE('',*,*,#40286,.F.);
#56749=ORIENTED_EDGE('',*,*,#40291,.T.);
#56750=ORIENTED_EDGE('',*,*,#40292,.F.);
#56751=ORIENTED_EDGE('',*,*,#40096,.T.);
#56752=ORIENTED_EDGE('',*,*,#40287,.T.);
#56753=ORIENTED_EDGE('',*,*,#40293,.T.);
#56754=ORIENTED_EDGE('',*,*,#40294,.F.);
#56755=ORIENTED_EDGE('',*,*,#40098,.T.);
#56756=ORIENTED_EDGE('',*,*,#40295,.F.);
#56757=ORIENTED_EDGE('',*,*,#40296,.F.);
#56758=ORIENTED_EDGE('',*,*,#40297,.F.);
#56759=ORIENTED_EDGE('',*,*,#40298,.F.);
#56760=ORIENTED_EDGE('',*,*,#40293,.F.);
#56761=ORIENTED_EDGE('',*,*,#40298,.T.);
#56762=ORIENTED_EDGE('',*,*,#40299,.F.);
#56763=ORIENTED_EDGE('',*,*,#40099,.T.);
#56764=ORIENTED_EDGE('',*,*,#40294,.T.);
#56765=ORIENTED_EDGE('',*,*,#34394,.T.);
#56766=ORIENTED_EDGE('',*,*,#40300,.F.);
#56767=ORIENTED_EDGE('',*,*,#40101,.T.);
#56768=ORIENTED_EDGE('',*,*,#40301,.F.);
#56769=ORIENTED_EDGE('',*,*,#34393,.T.);
#56770=ORIENTED_EDGE('',*,*,#40302,.F.);
#56771=ORIENTED_EDGE('',*,*,#40102,.T.);
#56772=ORIENTED_EDGE('',*,*,#40300,.T.);
#56773=ORIENTED_EDGE('',*,*,#40303,.T.);
#56774=ORIENTED_EDGE('',*,*,#40304,.F.);
#56775=ORIENTED_EDGE('',*,*,#40104,.T.);
#56776=ORIENTED_EDGE('',*,*,#40305,.F.);
#56777=ORIENTED_EDGE('',*,*,#40306,.F.);
#56778=ORIENTED_EDGE('',*,*,#40307,.F.);
#56779=ORIENTED_EDGE('',*,*,#40308,.F.);
#56780=ORIENTED_EDGE('',*,*,#40303,.F.);
#56781=ORIENTED_EDGE('',*,*,#40308,.T.);
#56782=ORIENTED_EDGE('',*,*,#40309,.F.);
#56783=ORIENTED_EDGE('',*,*,#40105,.T.);
#56784=ORIENTED_EDGE('',*,*,#40304,.T.);
#56785=ORIENTED_EDGE('',*,*,#40310,.T.);
#56786=ORIENTED_EDGE('',*,*,#40311,.F.);
#56787=ORIENTED_EDGE('',*,*,#40107,.T.);
#56788=ORIENTED_EDGE('',*,*,#40312,.F.);
#56789=ORIENTED_EDGE('',*,*,#40313,.F.);
#56790=ORIENTED_EDGE('',*,*,#40314,.F.);
#56791=ORIENTED_EDGE('',*,*,#40315,.F.);
#56792=ORIENTED_EDGE('',*,*,#40310,.F.);
#56793=ORIENTED_EDGE('',*,*,#40315,.T.);
#56794=ORIENTED_EDGE('',*,*,#40316,.F.);
#56795=ORIENTED_EDGE('',*,*,#40108,.T.);
#56796=ORIENTED_EDGE('',*,*,#40311,.T.);
#56797=ORIENTED_EDGE('',*,*,#40317,.T.);
#56798=ORIENTED_EDGE('',*,*,#40318,.F.);
#56799=ORIENTED_EDGE('',*,*,#40110,.T.);
#56800=ORIENTED_EDGE('',*,*,#40319,.F.);
#56801=ORIENTED_EDGE('',*,*,#40320,.F.);
#56802=ORIENTED_EDGE('',*,*,#40321,.F.);
#56803=ORIENTED_EDGE('',*,*,#40322,.F.);
#56804=ORIENTED_EDGE('',*,*,#40317,.F.);
#56805=ORIENTED_EDGE('',*,*,#40322,.T.);
#56806=ORIENTED_EDGE('',*,*,#40323,.F.);
#56807=ORIENTED_EDGE('',*,*,#40111,.T.);
#56808=ORIENTED_EDGE('',*,*,#40318,.T.);
#56809=ORIENTED_EDGE('',*,*,#40324,.T.);
#56810=ORIENTED_EDGE('',*,*,#40325,.F.);
#56811=ORIENTED_EDGE('',*,*,#40113,.T.);
#56812=ORIENTED_EDGE('',*,*,#40326,.F.);
#56813=ORIENTED_EDGE('',*,*,#40327,.F.);
#56814=ORIENTED_EDGE('',*,*,#40328,.F.);
#56815=ORIENTED_EDGE('',*,*,#40329,.F.);
#56816=ORIENTED_EDGE('',*,*,#40324,.F.);
#56817=ORIENTED_EDGE('',*,*,#40329,.T.);
#56818=ORIENTED_EDGE('',*,*,#40330,.F.);
#56819=ORIENTED_EDGE('',*,*,#40114,.T.);
#56820=ORIENTED_EDGE('',*,*,#40325,.T.);
#56821=ORIENTED_EDGE('',*,*,#40331,.T.);
#56822=ORIENTED_EDGE('',*,*,#40332,.F.);
#56823=ORIENTED_EDGE('',*,*,#40116,.T.);
#56824=ORIENTED_EDGE('',*,*,#40333,.F.);
#56825=ORIENTED_EDGE('',*,*,#40334,.F.);
#56826=ORIENTED_EDGE('',*,*,#40335,.F.);
#56827=ORIENTED_EDGE('',*,*,#40336,.F.);
#56828=ORIENTED_EDGE('',*,*,#40331,.F.);
#56829=ORIENTED_EDGE('',*,*,#40336,.T.);
#56830=ORIENTED_EDGE('',*,*,#40337,.F.);
#56831=ORIENTED_EDGE('',*,*,#40117,.T.);
#56832=ORIENTED_EDGE('',*,*,#40332,.T.);
#56833=ORIENTED_EDGE('',*,*,#40338,.T.);
#56834=ORIENTED_EDGE('',*,*,#40339,.F.);
#56835=ORIENTED_EDGE('',*,*,#40119,.T.);
#56836=ORIENTED_EDGE('',*,*,#40340,.F.);
#56837=ORIENTED_EDGE('',*,*,#40341,.F.);
#56838=ORIENTED_EDGE('',*,*,#40342,.F.);
#56839=ORIENTED_EDGE('',*,*,#40343,.F.);
#56840=ORIENTED_EDGE('',*,*,#40338,.F.);
#56841=ORIENTED_EDGE('',*,*,#40343,.T.);
#56842=ORIENTED_EDGE('',*,*,#40344,.F.);
#56843=ORIENTED_EDGE('',*,*,#40120,.T.);
#56844=ORIENTED_EDGE('',*,*,#40339,.T.);
#56845=ORIENTED_EDGE('',*,*,#40345,.T.);
#56846=ORIENTED_EDGE('',*,*,#40346,.F.);
#56847=ORIENTED_EDGE('',*,*,#40122,.T.);
#56848=ORIENTED_EDGE('',*,*,#40347,.F.);
#56849=ORIENTED_EDGE('',*,*,#40348,.F.);
#56850=ORIENTED_EDGE('',*,*,#40349,.F.);
#56851=ORIENTED_EDGE('',*,*,#40350,.F.);
#56852=ORIENTED_EDGE('',*,*,#40345,.F.);
#56853=ORIENTED_EDGE('',*,*,#40350,.T.);
#56854=ORIENTED_EDGE('',*,*,#40351,.F.);
#56855=ORIENTED_EDGE('',*,*,#40123,.T.);
#56856=ORIENTED_EDGE('',*,*,#40346,.T.);
#56857=ORIENTED_EDGE('',*,*,#40352,.T.);
#56858=ORIENTED_EDGE('',*,*,#40353,.F.);
#56859=ORIENTED_EDGE('',*,*,#40125,.T.);
#56860=ORIENTED_EDGE('',*,*,#40354,.F.);
#56861=ORIENTED_EDGE('',*,*,#40355,.F.);
#56862=ORIENTED_EDGE('',*,*,#40356,.F.);
#56863=ORIENTED_EDGE('',*,*,#40357,.F.);
#56864=ORIENTED_EDGE('',*,*,#40352,.F.);
#56865=ORIENTED_EDGE('',*,*,#40357,.T.);
#56866=ORIENTED_EDGE('',*,*,#40358,.F.);
#56867=ORIENTED_EDGE('',*,*,#40126,.T.);
#56868=ORIENTED_EDGE('',*,*,#40353,.T.);
#56869=ORIENTED_EDGE('',*,*,#40359,.T.);
#56870=ORIENTED_EDGE('',*,*,#40360,.F.);
#56871=ORIENTED_EDGE('',*,*,#40128,.T.);
#56872=ORIENTED_EDGE('',*,*,#40361,.F.);
#56873=ORIENTED_EDGE('',*,*,#40362,.F.);
#56874=ORIENTED_EDGE('',*,*,#40363,.F.);
#56875=ORIENTED_EDGE('',*,*,#40364,.F.);
#56876=ORIENTED_EDGE('',*,*,#40359,.F.);
#56877=ORIENTED_EDGE('',*,*,#40364,.T.);
#56878=ORIENTED_EDGE('',*,*,#40365,.F.);
#56879=ORIENTED_EDGE('',*,*,#40129,.T.);
#56880=ORIENTED_EDGE('',*,*,#40360,.T.);
#56881=ORIENTED_EDGE('',*,*,#40366,.T.);
#56882=ORIENTED_EDGE('',*,*,#40367,.F.);
#56883=ORIENTED_EDGE('',*,*,#40131,.T.);
#56884=ORIENTED_EDGE('',*,*,#40368,.F.);
#56885=ORIENTED_EDGE('',*,*,#40369,.F.);
#56886=ORIENTED_EDGE('',*,*,#40370,.F.);
#56887=ORIENTED_EDGE('',*,*,#40371,.F.);
#56888=ORIENTED_EDGE('',*,*,#40366,.F.);
#56889=ORIENTED_EDGE('',*,*,#40371,.T.);
#56890=ORIENTED_EDGE('',*,*,#40372,.F.);
#56891=ORIENTED_EDGE('',*,*,#40132,.T.);
#56892=ORIENTED_EDGE('',*,*,#40367,.T.);
#56893=ORIENTED_EDGE('',*,*,#40373,.T.);
#56894=ORIENTED_EDGE('',*,*,#40374,.F.);
#56895=ORIENTED_EDGE('',*,*,#40134,.T.);
#56896=ORIENTED_EDGE('',*,*,#40375,.F.);
#56897=ORIENTED_EDGE('',*,*,#40376,.F.);
#56898=ORIENTED_EDGE('',*,*,#40377,.F.);
#56899=ORIENTED_EDGE('',*,*,#40378,.F.);
#56900=ORIENTED_EDGE('',*,*,#40373,.F.);
#56901=ORIENTED_EDGE('',*,*,#40378,.T.);
#56902=ORIENTED_EDGE('',*,*,#40379,.F.);
#56903=ORIENTED_EDGE('',*,*,#40135,.T.);
#56904=ORIENTED_EDGE('',*,*,#40374,.T.);
#56905=ORIENTED_EDGE('',*,*,#40380,.T.);
#56906=ORIENTED_EDGE('',*,*,#40381,.F.);
#56907=ORIENTED_EDGE('',*,*,#40137,.T.);
#56908=ORIENTED_EDGE('',*,*,#40382,.F.);
#56909=ORIENTED_EDGE('',*,*,#40383,.F.);
#56910=ORIENTED_EDGE('',*,*,#40384,.F.);
#56911=ORIENTED_EDGE('',*,*,#40385,.F.);
#56912=ORIENTED_EDGE('',*,*,#40380,.F.);
#56913=ORIENTED_EDGE('',*,*,#40385,.T.);
#56914=ORIENTED_EDGE('',*,*,#40386,.F.);
#56915=ORIENTED_EDGE('',*,*,#40138,.T.);
#56916=ORIENTED_EDGE('',*,*,#40381,.T.);
#56917=ORIENTED_EDGE('',*,*,#40387,.T.);
#56918=ORIENTED_EDGE('',*,*,#40388,.F.);
#56919=ORIENTED_EDGE('',*,*,#40140,.T.);
#56920=ORIENTED_EDGE('',*,*,#40389,.F.);
#56921=ORIENTED_EDGE('',*,*,#40390,.T.);
#56922=ORIENTED_EDGE('',*,*,#40391,.F.);
#56923=ORIENTED_EDGE('',*,*,#40141,.T.);
#56924=ORIENTED_EDGE('',*,*,#40388,.T.);
#56925=ORIENTED_EDGE('',*,*,#40392,.F.);
#56926=ORIENTED_EDGE('',*,*,#40393,.F.);
#56927=ORIENTED_EDGE('',*,*,#40390,.F.);
#56928=ORIENTED_EDGE('',*,*,#40387,.F.);
#56929=ORIENTED_EDGE('',*,*,#40143,.T.);
#56930=ORIENTED_EDGE('',*,*,#40394,.F.);
#56931=ORIENTED_EDGE('',*,*,#40395,.T.);
#56932=ORIENTED_EDGE('',*,*,#40396,.F.);
#56933=ORIENTED_EDGE('',*,*,#40397,.F.);
#56934=ORIENTED_EDGE('',*,*,#40395,.F.);
#56935=ORIENTED_EDGE('',*,*,#40398,.F.);
#56936=ORIENTED_EDGE('',*,*,#40399,.F.);
#56937=ORIENTED_EDGE('',*,*,#40144,.T.);
#56938=ORIENTED_EDGE('',*,*,#40396,.T.);
#56939=ORIENTED_EDGE('',*,*,#40397,.T.);
#56940=ORIENTED_EDGE('',*,*,#40400,.F.);
#56941=ORIENTED_EDGE('',*,*,#40401,.T.);
#56942=ORIENTED_EDGE('',*,*,#40402,.F.);
#56943=ORIENTED_EDGE('',*,*,#40146,.T.);
#56944=ORIENTED_EDGE('',*,*,#40403,.F.);
#56945=ORIENTED_EDGE('',*,*,#40404,.F.);
#56946=ORIENTED_EDGE('',*,*,#40405,.F.);
#56947=ORIENTED_EDGE('',*,*,#40406,.F.);
#56948=ORIENTED_EDGE('',*,*,#40401,.F.);
#56949=ORIENTED_EDGE('',*,*,#40406,.T.);
#56950=ORIENTED_EDGE('',*,*,#40407,.F.);
#56951=ORIENTED_EDGE('',*,*,#40147,.T.);
#56952=ORIENTED_EDGE('',*,*,#40402,.T.);
#56953=ORIENTED_EDGE('',*,*,#40408,.T.);
#56954=ORIENTED_EDGE('',*,*,#40409,.F.);
#56955=ORIENTED_EDGE('',*,*,#40149,.T.);
#56956=ORIENTED_EDGE('',*,*,#40410,.F.);
#56957=ORIENTED_EDGE('',*,*,#40411,.F.);
#56958=ORIENTED_EDGE('',*,*,#40412,.F.);
#56959=ORIENTED_EDGE('',*,*,#40413,.F.);
#56960=ORIENTED_EDGE('',*,*,#40408,.F.);
#56961=ORIENTED_EDGE('',*,*,#40413,.T.);
#56962=ORIENTED_EDGE('',*,*,#40414,.F.);
#56963=ORIENTED_EDGE('',*,*,#40150,.T.);
#56964=ORIENTED_EDGE('',*,*,#40409,.T.);
#56965=ORIENTED_EDGE('',*,*,#40415,.T.);
#56966=ORIENTED_EDGE('',*,*,#40416,.F.);
#56967=ORIENTED_EDGE('',*,*,#40152,.T.);
#56968=ORIENTED_EDGE('',*,*,#40417,.F.);
#56969=ORIENTED_EDGE('',*,*,#40418,.F.);
#56970=ORIENTED_EDGE('',*,*,#40419,.F.);
#56971=ORIENTED_EDGE('',*,*,#40420,.F.);
#56972=ORIENTED_EDGE('',*,*,#40415,.F.);
#56973=ORIENTED_EDGE('',*,*,#40420,.T.);
#56974=ORIENTED_EDGE('',*,*,#40421,.F.);
#56975=ORIENTED_EDGE('',*,*,#40153,.T.);
#56976=ORIENTED_EDGE('',*,*,#40416,.T.);
#56977=ORIENTED_EDGE('',*,*,#40422,.T.);
#56978=ORIENTED_EDGE('',*,*,#40423,.F.);
#56979=ORIENTED_EDGE('',*,*,#40155,.T.);
#56980=ORIENTED_EDGE('',*,*,#40424,.F.);
#56981=ORIENTED_EDGE('',*,*,#40425,.F.);
#56982=ORIENTED_EDGE('',*,*,#40426,.F.);
#56983=ORIENTED_EDGE('',*,*,#40427,.F.);
#56984=ORIENTED_EDGE('',*,*,#40422,.F.);
#56985=ORIENTED_EDGE('',*,*,#40427,.T.);
#56986=ORIENTED_EDGE('',*,*,#40428,.F.);
#56987=ORIENTED_EDGE('',*,*,#40156,.T.);
#56988=ORIENTED_EDGE('',*,*,#40423,.T.);
#56989=ORIENTED_EDGE('',*,*,#40429,.T.);
#56990=ORIENTED_EDGE('',*,*,#40430,.F.);
#56991=ORIENTED_EDGE('',*,*,#40158,.T.);
#56992=ORIENTED_EDGE('',*,*,#40431,.F.);
#56993=ORIENTED_EDGE('',*,*,#40432,.F.);
#56994=ORIENTED_EDGE('',*,*,#40433,.F.);
#56995=ORIENTED_EDGE('',*,*,#40434,.F.);
#56996=ORIENTED_EDGE('',*,*,#40429,.F.);
#56997=ORIENTED_EDGE('',*,*,#40434,.T.);
#56998=ORIENTED_EDGE('',*,*,#40435,.F.);
#56999=ORIENTED_EDGE('',*,*,#40159,.T.);
#57000=ORIENTED_EDGE('',*,*,#40430,.T.);
#57001=ORIENTED_EDGE('',*,*,#40436,.T.);
#57002=ORIENTED_EDGE('',*,*,#40437,.F.);
#57003=ORIENTED_EDGE('',*,*,#40161,.T.);
#57004=ORIENTED_EDGE('',*,*,#40438,.F.);
#57005=ORIENTED_EDGE('',*,*,#40439,.F.);
#57006=ORIENTED_EDGE('',*,*,#40440,.F.);
#57007=ORIENTED_EDGE('',*,*,#40441,.F.);
#57008=ORIENTED_EDGE('',*,*,#40436,.F.);
#57009=ORIENTED_EDGE('',*,*,#40441,.T.);
#57010=ORIENTED_EDGE('',*,*,#40442,.F.);
#57011=ORIENTED_EDGE('',*,*,#40162,.T.);
#57012=ORIENTED_EDGE('',*,*,#40437,.T.);
#57013=ORIENTED_EDGE('',*,*,#40443,.T.);
#57014=ORIENTED_EDGE('',*,*,#40444,.F.);
#57015=ORIENTED_EDGE('',*,*,#40164,.T.);
#57016=ORIENTED_EDGE('',*,*,#40445,.F.);
#57017=ORIENTED_EDGE('',*,*,#40446,.F.);
#57018=ORIENTED_EDGE('',*,*,#40447,.F.);
#57019=ORIENTED_EDGE('',*,*,#40448,.F.);
#57020=ORIENTED_EDGE('',*,*,#40443,.F.);
#57021=ORIENTED_EDGE('',*,*,#40448,.T.);
#57022=ORIENTED_EDGE('',*,*,#40449,.F.);
#57023=ORIENTED_EDGE('',*,*,#40165,.T.);
#57024=ORIENTED_EDGE('',*,*,#40444,.T.);
#57025=ORIENTED_EDGE('',*,*,#40450,.F.);
#57026=ORIENTED_EDGE('',*,*,#40451,.F.);
#57027=ORIENTED_EDGE('',*,*,#40255,.F.);
#57028=ORIENTED_EDGE('',*,*,#40452,.F.);
#57029=ORIENTED_EDGE('',*,*,#40452,.T.);
#57030=ORIENTED_EDGE('',*,*,#40257,.T.);
#57031=ORIENTED_EDGE('',*,*,#40167,.T.);
#57032=ORIENTED_EDGE('',*,*,#40453,.F.);
#57033=ORIENTED_EDGE('',*,*,#40168,.T.);
#57034=ORIENTED_EDGE('',*,*,#40454,.F.);
#57035=ORIENTED_EDGE('',*,*,#40455,.T.);
#57036=ORIENTED_EDGE('',*,*,#40456,.F.);
#57037=ORIENTED_EDGE('',*,*,#40170,.T.);
#57038=ORIENTED_EDGE('',*,*,#40457,.F.);
#57039=ORIENTED_EDGE('',*,*,#40458,.T.);
#57040=ORIENTED_EDGE('',*,*,#40459,.F.);
#57041=ORIENTED_EDGE('',*,*,#40171,.T.);
#57042=ORIENTED_EDGE('',*,*,#40459,.T.);
#57043=ORIENTED_EDGE('',*,*,#40460,.T.);
#57044=ORIENTED_EDGE('',*,*,#40461,.F.);
#57045=ORIENTED_EDGE('',*,*,#40460,.F.);
#57046=ORIENTED_EDGE('',*,*,#40458,.F.);
#57047=ORIENTED_EDGE('',*,*,#40462,.F.);
#57048=ORIENTED_EDGE('',*,*,#40463,.F.);
#57049=ORIENTED_EDGE('',*,*,#40173,.T.);
#57050=ORIENTED_EDGE('',*,*,#40464,.F.);
#57051=ORIENTED_EDGE('',*,*,#40465,.T.);
#57052=ORIENTED_EDGE('',*,*,#40466,.F.);
#57053=ORIENTED_EDGE('',*,*,#40174,.T.);
#57054=ORIENTED_EDGE('',*,*,#40466,.T.);
#57055=ORIENTED_EDGE('',*,*,#40467,.T.);
#57056=ORIENTED_EDGE('',*,*,#40468,.F.);
#57057=ORIENTED_EDGE('',*,*,#40467,.F.);
#57058=ORIENTED_EDGE('',*,*,#40465,.F.);
#57059=ORIENTED_EDGE('',*,*,#40469,.F.);
#57060=ORIENTED_EDGE('',*,*,#40470,.F.);
#57061=ORIENTED_EDGE('',*,*,#40176,.T.);
#57062=ORIENTED_EDGE('',*,*,#40471,.F.);
#57063=ORIENTED_EDGE('',*,*,#40472,.T.);
#57064=ORIENTED_EDGE('',*,*,#40473,.F.);
#57065=ORIENTED_EDGE('',*,*,#40177,.T.);
#57066=ORIENTED_EDGE('',*,*,#40473,.T.);
#57067=ORIENTED_EDGE('',*,*,#40474,.T.);
#57068=ORIENTED_EDGE('',*,*,#40475,.F.);
#57069=ORIENTED_EDGE('',*,*,#40474,.F.);
#57070=ORIENTED_EDGE('',*,*,#40472,.F.);
#57071=ORIENTED_EDGE('',*,*,#40476,.F.);
#57072=ORIENTED_EDGE('',*,*,#40477,.F.);
#57073=ORIENTED_EDGE('',*,*,#40179,.T.);
#57074=ORIENTED_EDGE('',*,*,#40478,.F.);
#57075=ORIENTED_EDGE('',*,*,#40479,.T.);
#57076=ORIENTED_EDGE('',*,*,#40480,.F.);
#57077=ORIENTED_EDGE('',*,*,#40180,.T.);
#57078=ORIENTED_EDGE('',*,*,#40480,.T.);
#57079=ORIENTED_EDGE('',*,*,#40481,.T.);
#57080=ORIENTED_EDGE('',*,*,#40482,.F.);
#57081=ORIENTED_EDGE('',*,*,#40481,.F.);
#57082=ORIENTED_EDGE('',*,*,#40479,.F.);
#57083=ORIENTED_EDGE('',*,*,#40483,.F.);
#57084=ORIENTED_EDGE('',*,*,#40484,.F.);
#57085=ORIENTED_EDGE('',*,*,#40182,.T.);
#57086=ORIENTED_EDGE('',*,*,#40485,.F.);
#57087=ORIENTED_EDGE('',*,*,#40486,.T.);
#57088=ORIENTED_EDGE('',*,*,#40487,.F.);
#57089=ORIENTED_EDGE('',*,*,#40183,.T.);
#57090=ORIENTED_EDGE('',*,*,#40487,.T.);
#57091=ORIENTED_EDGE('',*,*,#40488,.T.);
#57092=ORIENTED_EDGE('',*,*,#40489,.F.);
#57093=ORIENTED_EDGE('',*,*,#40488,.F.);
#57094=ORIENTED_EDGE('',*,*,#40486,.F.);
#57095=ORIENTED_EDGE('',*,*,#40490,.F.);
#57096=ORIENTED_EDGE('',*,*,#40491,.F.);
#57097=ORIENTED_EDGE('',*,*,#40185,.T.);
#57098=ORIENTED_EDGE('',*,*,#40492,.F.);
#57099=ORIENTED_EDGE('',*,*,#40493,.T.);
#57100=ORIENTED_EDGE('',*,*,#40494,.F.);
#57101=ORIENTED_EDGE('',*,*,#40186,.T.);
#57102=ORIENTED_EDGE('',*,*,#40494,.T.);
#57103=ORIENTED_EDGE('',*,*,#40495,.T.);
#57104=ORIENTED_EDGE('',*,*,#40496,.F.);
#57105=ORIENTED_EDGE('',*,*,#40495,.F.);
#57106=ORIENTED_EDGE('',*,*,#40493,.F.);
#57107=ORIENTED_EDGE('',*,*,#40497,.F.);
#57108=ORIENTED_EDGE('',*,*,#40498,.F.);
#57109=ORIENTED_EDGE('',*,*,#40188,.T.);
#57110=ORIENTED_EDGE('',*,*,#40499,.F.);
#57111=ORIENTED_EDGE('',*,*,#40500,.T.);
#57112=ORIENTED_EDGE('',*,*,#40501,.F.);
#57113=ORIENTED_EDGE('',*,*,#40189,.T.);
#57114=ORIENTED_EDGE('',*,*,#40501,.T.);
#57115=ORIENTED_EDGE('',*,*,#40502,.T.);
#57116=ORIENTED_EDGE('',*,*,#40503,.F.);
#57117=ORIENTED_EDGE('',*,*,#40502,.F.);
#57118=ORIENTED_EDGE('',*,*,#40500,.F.);
#57119=ORIENTED_EDGE('',*,*,#40504,.F.);
#57120=ORIENTED_EDGE('',*,*,#40505,.F.);
#57121=ORIENTED_EDGE('',*,*,#40191,.T.);
#57122=ORIENTED_EDGE('',*,*,#40506,.F.);
#57123=ORIENTED_EDGE('',*,*,#40507,.T.);
#57124=ORIENTED_EDGE('',*,*,#40508,.F.);
#57125=ORIENTED_EDGE('',*,*,#40192,.T.);
#57126=ORIENTED_EDGE('',*,*,#40508,.T.);
#57127=ORIENTED_EDGE('',*,*,#40509,.T.);
#57128=ORIENTED_EDGE('',*,*,#40510,.F.);
#57129=ORIENTED_EDGE('',*,*,#40509,.F.);
#57130=ORIENTED_EDGE('',*,*,#40507,.F.);
#57131=ORIENTED_EDGE('',*,*,#40511,.F.);
#57132=ORIENTED_EDGE('',*,*,#40512,.F.);
#57133=ORIENTED_EDGE('',*,*,#40194,.T.);
#57134=ORIENTED_EDGE('',*,*,#40513,.F.);
#57135=ORIENTED_EDGE('',*,*,#40514,.T.);
#57136=ORIENTED_EDGE('',*,*,#40515,.F.);
#57137=ORIENTED_EDGE('',*,*,#40195,.T.);
#57138=ORIENTED_EDGE('',*,*,#40515,.T.);
#57139=ORIENTED_EDGE('',*,*,#40516,.T.);
#57140=ORIENTED_EDGE('',*,*,#40517,.F.);
#57141=ORIENTED_EDGE('',*,*,#40516,.F.);
#57142=ORIENTED_EDGE('',*,*,#40514,.F.);
#57143=ORIENTED_EDGE('',*,*,#40518,.F.);
#57144=ORIENTED_EDGE('',*,*,#40519,.F.);
#57145=ORIENTED_EDGE('',*,*,#40197,.T.);
#57146=ORIENTED_EDGE('',*,*,#40520,.F.);
#57147=ORIENTED_EDGE('',*,*,#40521,.T.);
#57148=ORIENTED_EDGE('',*,*,#40522,.F.);
#57149=ORIENTED_EDGE('',*,*,#40198,.T.);
#57150=ORIENTED_EDGE('',*,*,#40522,.T.);
#57151=ORIENTED_EDGE('',*,*,#40523,.T.);
#57152=ORIENTED_EDGE('',*,*,#40524,.F.);
#57153=ORIENTED_EDGE('',*,*,#40523,.F.);
#57154=ORIENTED_EDGE('',*,*,#40521,.F.);
#57155=ORIENTED_EDGE('',*,*,#40525,.F.);
#57156=ORIENTED_EDGE('',*,*,#40526,.F.);
#57157=ORIENTED_EDGE('',*,*,#40200,.T.);
#57158=ORIENTED_EDGE('',*,*,#40527,.F.);
#57159=ORIENTED_EDGE('',*,*,#40528,.T.);
#57160=ORIENTED_EDGE('',*,*,#40529,.F.);
#57161=ORIENTED_EDGE('',*,*,#40201,.T.);
#57162=ORIENTED_EDGE('',*,*,#40529,.T.);
#57163=ORIENTED_EDGE('',*,*,#40530,.T.);
#57164=ORIENTED_EDGE('',*,*,#40531,.F.);
#57165=ORIENTED_EDGE('',*,*,#40530,.F.);
#57166=ORIENTED_EDGE('',*,*,#40528,.F.);
#57167=ORIENTED_EDGE('',*,*,#40532,.F.);
#57168=ORIENTED_EDGE('',*,*,#40533,.F.);
#57169=ORIENTED_EDGE('',*,*,#40203,.T.);
#57170=ORIENTED_EDGE('',*,*,#40534,.F.);
#57171=ORIENTED_EDGE('',*,*,#40535,.T.);
#57172=ORIENTED_EDGE('',*,*,#40536,.F.);
#57173=ORIENTED_EDGE('',*,*,#40204,.T.);
#57174=ORIENTED_EDGE('',*,*,#40536,.T.);
#57175=ORIENTED_EDGE('',*,*,#40537,.T.);
#57176=ORIENTED_EDGE('',*,*,#40538,.F.);
#57177=ORIENTED_EDGE('',*,*,#40537,.F.);
#57178=ORIENTED_EDGE('',*,*,#40535,.F.);
#57179=ORIENTED_EDGE('',*,*,#40539,.F.);
#57180=ORIENTED_EDGE('',*,*,#40540,.F.);
#57181=ORIENTED_EDGE('',*,*,#40206,.T.);
#57182=ORIENTED_EDGE('',*,*,#40541,.F.);
#57183=ORIENTED_EDGE('',*,*,#40542,.T.);
#57184=ORIENTED_EDGE('',*,*,#40543,.F.);
#57185=ORIENTED_EDGE('',*,*,#40207,.T.);
#57186=ORIENTED_EDGE('',*,*,#40543,.T.);
#57187=ORIENTED_EDGE('',*,*,#40544,.T.);
#57188=ORIENTED_EDGE('',*,*,#40545,.F.);
#57189=ORIENTED_EDGE('',*,*,#40544,.F.);
#57190=ORIENTED_EDGE('',*,*,#40542,.F.);
#57191=ORIENTED_EDGE('',*,*,#40546,.F.);
#57192=ORIENTED_EDGE('',*,*,#40547,.F.);
#57193=ORIENTED_EDGE('',*,*,#40209,.T.);
#57194=ORIENTED_EDGE('',*,*,#40548,.F.);
#57195=ORIENTED_EDGE('',*,*,#34391,.T.);
#57196=ORIENTED_EDGE('',*,*,#40549,.F.);
#57197=ORIENTED_EDGE('',*,*,#40210,.T.);
#57198=ORIENTED_EDGE('',*,*,#40549,.T.);
#57199=ORIENTED_EDGE('',*,*,#34390,.T.);
#57200=ORIENTED_EDGE('',*,*,#40550,.F.);
#57201=ORIENTED_EDGE('',*,*,#40212,.T.);
#57202=ORIENTED_EDGE('',*,*,#40551,.F.);
#57203=ORIENTED_EDGE('',*,*,#40552,.T.);
#57204=ORIENTED_EDGE('',*,*,#40553,.F.);
#57205=ORIENTED_EDGE('',*,*,#40213,.T.);
#57206=ORIENTED_EDGE('',*,*,#40553,.T.);
#57207=ORIENTED_EDGE('',*,*,#40554,.T.);
#57208=ORIENTED_EDGE('',*,*,#40555,.F.);
#57209=ORIENTED_EDGE('',*,*,#40554,.F.);
#57210=ORIENTED_EDGE('',*,*,#40552,.F.);
#57211=ORIENTED_EDGE('',*,*,#40556,.F.);
#57212=ORIENTED_EDGE('',*,*,#40557,.F.);
#57213=ORIENTED_EDGE('',*,*,#40215,.T.);
#57214=ORIENTED_EDGE('',*,*,#40558,.F.);
#57215=ORIENTED_EDGE('',*,*,#40559,.T.);
#57216=ORIENTED_EDGE('',*,*,#40560,.F.);
#57217=ORIENTED_EDGE('',*,*,#40216,.T.);
#57218=ORIENTED_EDGE('',*,*,#40560,.T.);
#57219=ORIENTED_EDGE('',*,*,#40561,.T.);
#57220=ORIENTED_EDGE('',*,*,#40562,.F.);
#57221=ORIENTED_EDGE('',*,*,#40561,.F.);
#57222=ORIENTED_EDGE('',*,*,#40559,.F.);
#57223=ORIENTED_EDGE('',*,*,#40563,.F.);
#57224=ORIENTED_EDGE('',*,*,#40564,.F.);
#57225=ORIENTED_EDGE('',*,*,#40218,.T.);
#57226=ORIENTED_EDGE('',*,*,#40565,.F.);
#57227=ORIENTED_EDGE('',*,*,#40566,.T.);
#57228=ORIENTED_EDGE('',*,*,#40567,.F.);
#57229=ORIENTED_EDGE('',*,*,#40219,.T.);
#57230=ORIENTED_EDGE('',*,*,#40567,.T.);
#57231=ORIENTED_EDGE('',*,*,#40568,.T.);
#57232=ORIENTED_EDGE('',*,*,#40569,.F.);
#57233=ORIENTED_EDGE('',*,*,#40568,.F.);
#57234=ORIENTED_EDGE('',*,*,#40566,.F.);
#57235=ORIENTED_EDGE('',*,*,#40570,.F.);
#57236=ORIENTED_EDGE('',*,*,#40571,.F.);
#57237=ORIENTED_EDGE('',*,*,#40221,.T.);
#57238=ORIENTED_EDGE('',*,*,#40572,.F.);
#57239=ORIENTED_EDGE('',*,*,#40573,.T.);
#57240=ORIENTED_EDGE('',*,*,#40574,.F.);
#57241=ORIENTED_EDGE('',*,*,#40222,.T.);
#57242=ORIENTED_EDGE('',*,*,#40574,.T.);
#57243=ORIENTED_EDGE('',*,*,#40575,.T.);
#57244=ORIENTED_EDGE('',*,*,#40576,.F.);
#57245=ORIENTED_EDGE('',*,*,#40575,.F.);
#57246=ORIENTED_EDGE('',*,*,#40573,.F.);
#57247=ORIENTED_EDGE('',*,*,#40577,.F.);
#57248=ORIENTED_EDGE('',*,*,#40578,.F.);
#57249=ORIENTED_EDGE('',*,*,#40224,.T.);
#57250=ORIENTED_EDGE('',*,*,#40579,.F.);
#57251=ORIENTED_EDGE('',*,*,#40580,.T.);
#57252=ORIENTED_EDGE('',*,*,#40581,.F.);
#57253=ORIENTED_EDGE('',*,*,#40225,.T.);
#57254=ORIENTED_EDGE('',*,*,#40581,.T.);
#57255=ORIENTED_EDGE('',*,*,#40582,.T.);
#57256=ORIENTED_EDGE('',*,*,#40583,.F.);
#57257=ORIENTED_EDGE('',*,*,#40582,.F.);
#57258=ORIENTED_EDGE('',*,*,#40580,.F.);
#57259=ORIENTED_EDGE('',*,*,#40584,.F.);
#57260=ORIENTED_EDGE('',*,*,#40585,.F.);
#57261=ORIENTED_EDGE('',*,*,#40227,.T.);
#57262=ORIENTED_EDGE('',*,*,#40586,.F.);
#57263=ORIENTED_EDGE('',*,*,#40587,.T.);
#57264=ORIENTED_EDGE('',*,*,#40588,.F.);
#57265=ORIENTED_EDGE('',*,*,#40228,.T.);
#57266=ORIENTED_EDGE('',*,*,#40588,.T.);
#57267=ORIENTED_EDGE('',*,*,#40589,.T.);
#57268=ORIENTED_EDGE('',*,*,#40590,.F.);
#57269=ORIENTED_EDGE('',*,*,#40589,.F.);
#57270=ORIENTED_EDGE('',*,*,#40587,.F.);
#57271=ORIENTED_EDGE('',*,*,#40591,.F.);
#57272=ORIENTED_EDGE('',*,*,#40592,.F.);
#57273=ORIENTED_EDGE('',*,*,#40230,.T.);
#57274=ORIENTED_EDGE('',*,*,#40593,.F.);
#57275=ORIENTED_EDGE('',*,*,#40594,.T.);
#57276=ORIENTED_EDGE('',*,*,#40595,.F.);
#57277=ORIENTED_EDGE('',*,*,#40231,.T.);
#57278=ORIENTED_EDGE('',*,*,#40595,.T.);
#57279=ORIENTED_EDGE('',*,*,#40596,.T.);
#57280=ORIENTED_EDGE('',*,*,#40597,.F.);
#57281=ORIENTED_EDGE('',*,*,#40596,.F.);
#57282=ORIENTED_EDGE('',*,*,#40594,.F.);
#57283=ORIENTED_EDGE('',*,*,#40598,.F.);
#57284=ORIENTED_EDGE('',*,*,#40599,.F.);
#57285=ORIENTED_EDGE('',*,*,#40233,.T.);
#57286=ORIENTED_EDGE('',*,*,#40600,.F.);
#57287=ORIENTED_EDGE('',*,*,#40601,.T.);
#57288=ORIENTED_EDGE('',*,*,#40602,.F.);
#57289=ORIENTED_EDGE('',*,*,#40234,.T.);
#57290=ORIENTED_EDGE('',*,*,#40602,.T.);
#57291=ORIENTED_EDGE('',*,*,#40603,.T.);
#57292=ORIENTED_EDGE('',*,*,#40604,.F.);
#57293=ORIENTED_EDGE('',*,*,#40603,.F.);
#57294=ORIENTED_EDGE('',*,*,#40601,.F.);
#57295=ORIENTED_EDGE('',*,*,#40605,.F.);
#57296=ORIENTED_EDGE('',*,*,#40606,.F.);
#57297=ORIENTED_EDGE('',*,*,#40236,.T.);
#57298=ORIENTED_EDGE('',*,*,#40607,.F.);
#57299=ORIENTED_EDGE('',*,*,#40608,.T.);
#57300=ORIENTED_EDGE('',*,*,#40609,.F.);
#57301=ORIENTED_EDGE('',*,*,#40237,.T.);
#57302=ORIENTED_EDGE('',*,*,#40609,.T.);
#57303=ORIENTED_EDGE('',*,*,#40610,.T.);
#57304=ORIENTED_EDGE('',*,*,#40611,.F.);
#57305=ORIENTED_EDGE('',*,*,#40610,.F.);
#57306=ORIENTED_EDGE('',*,*,#40608,.F.);
#57307=ORIENTED_EDGE('',*,*,#40612,.F.);
#57308=ORIENTED_EDGE('',*,*,#40613,.F.);
#57309=ORIENTED_EDGE('',*,*,#40239,.T.);
#57310=ORIENTED_EDGE('',*,*,#40614,.F.);
#57311=ORIENTED_EDGE('',*,*,#40615,.T.);
#57312=ORIENTED_EDGE('',*,*,#40616,.F.);
#57313=ORIENTED_EDGE('',*,*,#40240,.T.);
#57314=ORIENTED_EDGE('',*,*,#40616,.T.);
#57315=ORIENTED_EDGE('',*,*,#40617,.T.);
#57316=ORIENTED_EDGE('',*,*,#40618,.F.);
#57317=ORIENTED_EDGE('',*,*,#40617,.F.);
#57318=ORIENTED_EDGE('',*,*,#40615,.F.);
#57319=ORIENTED_EDGE('',*,*,#40619,.F.);
#57320=ORIENTED_EDGE('',*,*,#40620,.F.);
#57321=ORIENTED_EDGE('',*,*,#40242,.T.);
#57322=ORIENTED_EDGE('',*,*,#40621,.F.);
#57323=ORIENTED_EDGE('',*,*,#40622,.T.);
#57324=ORIENTED_EDGE('',*,*,#40623,.F.);
#57325=ORIENTED_EDGE('',*,*,#40243,.T.);
#57326=ORIENTED_EDGE('',*,*,#40623,.T.);
#57327=ORIENTED_EDGE('',*,*,#40624,.T.);
#57328=ORIENTED_EDGE('',*,*,#40625,.F.);
#57329=ORIENTED_EDGE('',*,*,#40624,.F.);
#57330=ORIENTED_EDGE('',*,*,#40622,.F.);
#57331=ORIENTED_EDGE('',*,*,#40626,.F.);
#57332=ORIENTED_EDGE('',*,*,#40627,.F.);
#57333=ORIENTED_EDGE('',*,*,#40245,.T.);
#57334=ORIENTED_EDGE('',*,*,#40628,.F.);
#57335=ORIENTED_EDGE('',*,*,#40629,.T.);
#57336=ORIENTED_EDGE('',*,*,#40630,.F.);
#57337=ORIENTED_EDGE('',*,*,#40631,.T.);
#57338=ORIENTED_EDGE('',*,*,#40632,.F.);
#57339=ORIENTED_EDGE('',*,*,#40246,.T.);
#57340=ORIENTED_EDGE('',*,*,#40630,.T.);
#57341=ORIENTED_EDGE('',*,*,#40633,.F.);
#57342=ORIENTED_EDGE('',*,*,#40634,.F.);
#57343=ORIENTED_EDGE('',*,*,#40631,.F.);
#57344=ORIENTED_EDGE('',*,*,#40629,.F.);
#57345=ORIENTED_EDGE('',*,*,#40248,.T.);
#57346=ORIENTED_EDGE('',*,*,#40635,.F.);
#57347=ORIENTED_EDGE('',*,*,#40636,.T.);
#57348=ORIENTED_EDGE('',*,*,#40637,.F.);
#57349=ORIENTED_EDGE('',*,*,#40249,.T.);
#57350=ORIENTED_EDGE('',*,*,#40637,.T.);
#57351=ORIENTED_EDGE('',*,*,#40638,.T.);
#57352=ORIENTED_EDGE('',*,*,#40639,.F.);
#57353=ORIENTED_EDGE('',*,*,#40638,.F.);
#57354=ORIENTED_EDGE('',*,*,#40636,.F.);
#57355=ORIENTED_EDGE('',*,*,#40640,.F.);
#57356=ORIENTED_EDGE('',*,*,#40641,.F.);
#57357=ORIENTED_EDGE('',*,*,#40251,.T.);
#57358=ORIENTED_EDGE('',*,*,#40642,.F.);
#57359=ORIENTED_EDGE('',*,*,#40643,.T.);
#57360=ORIENTED_EDGE('',*,*,#40644,.F.);
#57361=ORIENTED_EDGE('',*,*,#40252,.T.);
#57362=ORIENTED_EDGE('',*,*,#40644,.T.);
#57363=ORIENTED_EDGE('',*,*,#40645,.T.);
#57364=ORIENTED_EDGE('',*,*,#40646,.F.);
#57365=ORIENTED_EDGE('',*,*,#40645,.F.);
#57366=ORIENTED_EDGE('',*,*,#40643,.F.);
#57367=ORIENTED_EDGE('',*,*,#40647,.F.);
#57368=ORIENTED_EDGE('',*,*,#40648,.F.);
#57369=ORIENTED_EDGE('',*,*,#40455,.F.);
#57370=ORIENTED_EDGE('',*,*,#40649,.F.);
#57371=ORIENTED_EDGE('',*,*,#40650,.F.);
#57372=ORIENTED_EDGE('',*,*,#40651,.F.);
#57373=ORIENTED_EDGE('',*,*,#40254,.T.);
#57374=ORIENTED_EDGE('',*,*,#40652,.F.);
#57375=ORIENTED_EDGE('',*,*,#40649,.T.);
#57376=ORIENTED_EDGE('',*,*,#40454,.T.);
#57377=ORIENTED_EDGE('',*,*,#40653,.F.);
#57378=ORIENTED_EDGE('',*,*,#40256,.T.);
#57379=ORIENTED_EDGE('',*,*,#40451,.T.);
#57380=ORIENTED_EDGE('',*,*,#40654,.F.);
#57381=ORIENTED_EDGE('',*,*,#40655,.F.);
#57382=ORIENTED_EDGE('',*,*,#40656,.F.);
#57383=ORIENTED_EDGE('',*,*,#40261,.T.);
#57384=ORIENTED_EDGE('',*,*,#40260,.T.);
#57385=ORIENTED_EDGE('',*,*,#40657,.F.);
#57386=ORIENTED_EDGE('',*,*,#40264,.T.);
#57387=ORIENTED_EDGE('',*,*,#40262,.T.);
#57388=ORIENTED_EDGE('',*,*,#40656,.T.);
#57389=ORIENTED_EDGE('',*,*,#40658,.F.);
#57390=ORIENTED_EDGE('',*,*,#40659,.F.);
#57391=ORIENTED_EDGE('',*,*,#40268,.T.);
#57392=ORIENTED_EDGE('',*,*,#40267,.T.);
#57393=ORIENTED_EDGE('',*,*,#40660,.F.);
#57394=ORIENTED_EDGE('',*,*,#40271,.T.);
#57395=ORIENTED_EDGE('',*,*,#40269,.T.);
#57396=ORIENTED_EDGE('',*,*,#40659,.T.);
#57397=ORIENTED_EDGE('',*,*,#40661,.F.);
#57398=ORIENTED_EDGE('',*,*,#40662,.F.);
#57399=ORIENTED_EDGE('',*,*,#40275,.T.);
#57400=ORIENTED_EDGE('',*,*,#40274,.T.);
#57401=ORIENTED_EDGE('',*,*,#40663,.F.);
#57402=ORIENTED_EDGE('',*,*,#40278,.T.);
#57403=ORIENTED_EDGE('',*,*,#40276,.T.);
#57404=ORIENTED_EDGE('',*,*,#40662,.T.);
#57405=ORIENTED_EDGE('',*,*,#40664,.F.);
#57406=ORIENTED_EDGE('',*,*,#40665,.F.);
#57407=ORIENTED_EDGE('',*,*,#40282,.T.);
#57408=ORIENTED_EDGE('',*,*,#40281,.T.);
#57409=ORIENTED_EDGE('',*,*,#40666,.F.);
#57410=ORIENTED_EDGE('',*,*,#40285,.T.);
#57411=ORIENTED_EDGE('',*,*,#40283,.T.);
#57412=ORIENTED_EDGE('',*,*,#40665,.T.);
#57413=ORIENTED_EDGE('',*,*,#40667,.F.);
#57414=ORIENTED_EDGE('',*,*,#40668,.F.);
#57415=ORIENTED_EDGE('',*,*,#40289,.T.);
#57416=ORIENTED_EDGE('',*,*,#40288,.T.);
#57417=ORIENTED_EDGE('',*,*,#40669,.F.);
#57418=ORIENTED_EDGE('',*,*,#40292,.T.);
#57419=ORIENTED_EDGE('',*,*,#40290,.T.);
#57420=ORIENTED_EDGE('',*,*,#40668,.T.);
#57421=ORIENTED_EDGE('',*,*,#40670,.F.);
#57422=ORIENTED_EDGE('',*,*,#40671,.F.);
#57423=ORIENTED_EDGE('',*,*,#40296,.T.);
#57424=ORIENTED_EDGE('',*,*,#40295,.T.);
#57425=ORIENTED_EDGE('',*,*,#40672,.F.);
#57426=ORIENTED_EDGE('',*,*,#40299,.T.);
#57427=ORIENTED_EDGE('',*,*,#40297,.T.);
#57428=ORIENTED_EDGE('',*,*,#40671,.T.);
#57429=ORIENTED_EDGE('',*,*,#40673,.F.);
#57430=ORIENTED_EDGE('',*,*,#40674,.F.);
#57431=ORIENTED_EDGE('',*,*,#34395,.T.);
#57432=ORIENTED_EDGE('',*,*,#40301,.T.);
#57433=ORIENTED_EDGE('',*,*,#40675,.F.);
#57434=ORIENTED_EDGE('',*,*,#40302,.T.);
#57435=ORIENTED_EDGE('',*,*,#34396,.T.);
#57436=ORIENTED_EDGE('',*,*,#40674,.T.);
#57437=ORIENTED_EDGE('',*,*,#40676,.F.);
#57438=ORIENTED_EDGE('',*,*,#40677,.F.);
#57439=ORIENTED_EDGE('',*,*,#40306,.T.);
#57440=ORIENTED_EDGE('',*,*,#40305,.T.);
#57441=ORIENTED_EDGE('',*,*,#40678,.F.);
#57442=ORIENTED_EDGE('',*,*,#40309,.T.);
#57443=ORIENTED_EDGE('',*,*,#40307,.T.);
#57444=ORIENTED_EDGE('',*,*,#40677,.T.);
#57445=ORIENTED_EDGE('',*,*,#40679,.F.);
#57446=ORIENTED_EDGE('',*,*,#40680,.F.);
#57447=ORIENTED_EDGE('',*,*,#40313,.T.);
#57448=ORIENTED_EDGE('',*,*,#40312,.T.);
#57449=ORIENTED_EDGE('',*,*,#40681,.F.);
#57450=ORIENTED_EDGE('',*,*,#40316,.T.);
#57451=ORIENTED_EDGE('',*,*,#40314,.T.);
#57452=ORIENTED_EDGE('',*,*,#40680,.T.);
#57453=ORIENTED_EDGE('',*,*,#40682,.F.);
#57454=ORIENTED_EDGE('',*,*,#40683,.F.);
#57455=ORIENTED_EDGE('',*,*,#40320,.T.);
#57456=ORIENTED_EDGE('',*,*,#40319,.T.);
#57457=ORIENTED_EDGE('',*,*,#40684,.F.);
#57458=ORIENTED_EDGE('',*,*,#40323,.T.);
#57459=ORIENTED_EDGE('',*,*,#40321,.T.);
#57460=ORIENTED_EDGE('',*,*,#40683,.T.);
#57461=ORIENTED_EDGE('',*,*,#40685,.F.);
#57462=ORIENTED_EDGE('',*,*,#40686,.F.);
#57463=ORIENTED_EDGE('',*,*,#40327,.T.);
#57464=ORIENTED_EDGE('',*,*,#40326,.T.);
#57465=ORIENTED_EDGE('',*,*,#40687,.F.);
#57466=ORIENTED_EDGE('',*,*,#40330,.T.);
#57467=ORIENTED_EDGE('',*,*,#40328,.T.);
#57468=ORIENTED_EDGE('',*,*,#40686,.T.);
#57469=ORIENTED_EDGE('',*,*,#40688,.F.);
#57470=ORIENTED_EDGE('',*,*,#40689,.F.);
#57471=ORIENTED_EDGE('',*,*,#40334,.T.);
#57472=ORIENTED_EDGE('',*,*,#40333,.T.);
#57473=ORIENTED_EDGE('',*,*,#40690,.F.);
#57474=ORIENTED_EDGE('',*,*,#40337,.T.);
#57475=ORIENTED_EDGE('',*,*,#40335,.T.);
#57476=ORIENTED_EDGE('',*,*,#40689,.T.);
#57477=ORIENTED_EDGE('',*,*,#40691,.F.);
#57478=ORIENTED_EDGE('',*,*,#40692,.F.);
#57479=ORIENTED_EDGE('',*,*,#40341,.T.);
#57480=ORIENTED_EDGE('',*,*,#40340,.T.);
#57481=ORIENTED_EDGE('',*,*,#40693,.F.);
#57482=ORIENTED_EDGE('',*,*,#40344,.T.);
#57483=ORIENTED_EDGE('',*,*,#40342,.T.);
#57484=ORIENTED_EDGE('',*,*,#40692,.T.);
#57485=ORIENTED_EDGE('',*,*,#40694,.F.);
#57486=ORIENTED_EDGE('',*,*,#40695,.F.);
#57487=ORIENTED_EDGE('',*,*,#40348,.T.);
#57488=ORIENTED_EDGE('',*,*,#40347,.T.);
#57489=ORIENTED_EDGE('',*,*,#40696,.F.);
#57490=ORIENTED_EDGE('',*,*,#40351,.T.);
#57491=ORIENTED_EDGE('',*,*,#40349,.T.);
#57492=ORIENTED_EDGE('',*,*,#40695,.T.);
#57493=ORIENTED_EDGE('',*,*,#40697,.F.);
#57494=ORIENTED_EDGE('',*,*,#40698,.F.);
#57495=ORIENTED_EDGE('',*,*,#40355,.T.);
#57496=ORIENTED_EDGE('',*,*,#40354,.T.);
#57497=ORIENTED_EDGE('',*,*,#40699,.F.);
#57498=ORIENTED_EDGE('',*,*,#40358,.T.);
#57499=ORIENTED_EDGE('',*,*,#40356,.T.);
#57500=ORIENTED_EDGE('',*,*,#40698,.T.);
#57501=ORIENTED_EDGE('',*,*,#40700,.F.);
#57502=ORIENTED_EDGE('',*,*,#40701,.F.);
#57503=ORIENTED_EDGE('',*,*,#40362,.T.);
#57504=ORIENTED_EDGE('',*,*,#40361,.T.);
#57505=ORIENTED_EDGE('',*,*,#40702,.F.);
#57506=ORIENTED_EDGE('',*,*,#40365,.T.);
#57507=ORIENTED_EDGE('',*,*,#40363,.T.);
#57508=ORIENTED_EDGE('',*,*,#40701,.T.);
#57509=ORIENTED_EDGE('',*,*,#40703,.F.);
#57510=ORIENTED_EDGE('',*,*,#40704,.F.);
#57511=ORIENTED_EDGE('',*,*,#40369,.T.);
#57512=ORIENTED_EDGE('',*,*,#40368,.T.);
#57513=ORIENTED_EDGE('',*,*,#40705,.F.);
#57514=ORIENTED_EDGE('',*,*,#40372,.T.);
#57515=ORIENTED_EDGE('',*,*,#40370,.T.);
#57516=ORIENTED_EDGE('',*,*,#40704,.T.);
#57517=ORIENTED_EDGE('',*,*,#40706,.F.);
#57518=ORIENTED_EDGE('',*,*,#40707,.F.);
#57519=ORIENTED_EDGE('',*,*,#40376,.T.);
#57520=ORIENTED_EDGE('',*,*,#40375,.T.);
#57521=ORIENTED_EDGE('',*,*,#40708,.F.);
#57522=ORIENTED_EDGE('',*,*,#40379,.T.);
#57523=ORIENTED_EDGE('',*,*,#40377,.T.);
#57524=ORIENTED_EDGE('',*,*,#40707,.T.);
#57525=ORIENTED_EDGE('',*,*,#40709,.F.);
#57526=ORIENTED_EDGE('',*,*,#40710,.F.);
#57527=ORIENTED_EDGE('',*,*,#40383,.T.);
#57528=ORIENTED_EDGE('',*,*,#40382,.T.);
#57529=ORIENTED_EDGE('',*,*,#40711,.F.);
#57530=ORIENTED_EDGE('',*,*,#40386,.T.);
#57531=ORIENTED_EDGE('',*,*,#40384,.T.);
#57532=ORIENTED_EDGE('',*,*,#40710,.T.);
#57533=ORIENTED_EDGE('',*,*,#40712,.F.);
#57534=ORIENTED_EDGE('',*,*,#40713,.F.);
#57535=ORIENTED_EDGE('',*,*,#40392,.T.);
#57536=ORIENTED_EDGE('',*,*,#40389,.T.);
#57537=ORIENTED_EDGE('',*,*,#40393,.T.);
#57538=ORIENTED_EDGE('',*,*,#40713,.T.);
#57539=ORIENTED_EDGE('',*,*,#40714,.F.);
#57540=ORIENTED_EDGE('',*,*,#40391,.T.);
#57541=ORIENTED_EDGE('',*,*,#40398,.T.);
#57542=ORIENTED_EDGE('',*,*,#40394,.T.);
#57543=ORIENTED_EDGE('',*,*,#40715,.F.);
#57544=ORIENTED_EDGE('',*,*,#40716,.F.);
#57545=ORIENTED_EDGE('',*,*,#40717,.F.);
#57546=ORIENTED_EDGE('',*,*,#40400,.T.);
#57547=ORIENTED_EDGE('',*,*,#40399,.T.);
#57548=ORIENTED_EDGE('',*,*,#40716,.T.);
#57549=ORIENTED_EDGE('',*,*,#40718,.F.);
#57550=ORIENTED_EDGE('',*,*,#40719,.F.);
#57551=ORIENTED_EDGE('',*,*,#40404,.T.);
#57552=ORIENTED_EDGE('',*,*,#40403,.T.);
#57553=ORIENTED_EDGE('',*,*,#40720,.F.);
#57554=ORIENTED_EDGE('',*,*,#40407,.T.);
#57555=ORIENTED_EDGE('',*,*,#40405,.T.);
#57556=ORIENTED_EDGE('',*,*,#40719,.T.);
#57557=ORIENTED_EDGE('',*,*,#40721,.F.);
#57558=ORIENTED_EDGE('',*,*,#40722,.F.);
#57559=ORIENTED_EDGE('',*,*,#40411,.T.);
#57560=ORIENTED_EDGE('',*,*,#40410,.T.);
#57561=ORIENTED_EDGE('',*,*,#40723,.F.);
#57562=ORIENTED_EDGE('',*,*,#40414,.T.);
#57563=ORIENTED_EDGE('',*,*,#40412,.T.);
#57564=ORIENTED_EDGE('',*,*,#40722,.T.);
#57565=ORIENTED_EDGE('',*,*,#40724,.F.);
#57566=ORIENTED_EDGE('',*,*,#40725,.F.);
#57567=ORIENTED_EDGE('',*,*,#40418,.T.);
#57568=ORIENTED_EDGE('',*,*,#40417,.T.);
#57569=ORIENTED_EDGE('',*,*,#40726,.F.);
#57570=ORIENTED_EDGE('',*,*,#40421,.T.);
#57571=ORIENTED_EDGE('',*,*,#40419,.T.);
#57572=ORIENTED_EDGE('',*,*,#40725,.T.);
#57573=ORIENTED_EDGE('',*,*,#40727,.F.);
#57574=ORIENTED_EDGE('',*,*,#40728,.F.);
#57575=ORIENTED_EDGE('',*,*,#40425,.T.);
#57576=ORIENTED_EDGE('',*,*,#40424,.T.);
#57577=ORIENTED_EDGE('',*,*,#40729,.F.);
#57578=ORIENTED_EDGE('',*,*,#40428,.T.);
#57579=ORIENTED_EDGE('',*,*,#40426,.T.);
#57580=ORIENTED_EDGE('',*,*,#40728,.T.);
#57581=ORIENTED_EDGE('',*,*,#40730,.F.);
#57582=ORIENTED_EDGE('',*,*,#40731,.F.);
#57583=ORIENTED_EDGE('',*,*,#40432,.T.);
#57584=ORIENTED_EDGE('',*,*,#40431,.T.);
#57585=ORIENTED_EDGE('',*,*,#40732,.F.);
#57586=ORIENTED_EDGE('',*,*,#40435,.T.);
#57587=ORIENTED_EDGE('',*,*,#40433,.T.);
#57588=ORIENTED_EDGE('',*,*,#40731,.T.);
#57589=ORIENTED_EDGE('',*,*,#40733,.F.);
#57590=ORIENTED_EDGE('',*,*,#40734,.F.);
#57591=ORIENTED_EDGE('',*,*,#40439,.T.);
#57592=ORIENTED_EDGE('',*,*,#40438,.T.);
#57593=ORIENTED_EDGE('',*,*,#40735,.F.);
#57594=ORIENTED_EDGE('',*,*,#40442,.T.);
#57595=ORIENTED_EDGE('',*,*,#40440,.T.);
#57596=ORIENTED_EDGE('',*,*,#40734,.T.);
#57597=ORIENTED_EDGE('',*,*,#40736,.F.);
#57598=ORIENTED_EDGE('',*,*,#40737,.F.);
#57599=ORIENTED_EDGE('',*,*,#40446,.T.);
#57600=ORIENTED_EDGE('',*,*,#40445,.T.);
#57601=ORIENTED_EDGE('',*,*,#40738,.F.);
#57602=ORIENTED_EDGE('',*,*,#40449,.T.);
#57603=ORIENTED_EDGE('',*,*,#40447,.T.);
#57604=ORIENTED_EDGE('',*,*,#40737,.T.);
#57605=ORIENTED_EDGE('',*,*,#40739,.F.);
#57606=ORIENTED_EDGE('',*,*,#40654,.T.);
#57607=ORIENTED_EDGE('',*,*,#40450,.T.);
#57608=ORIENTED_EDGE('',*,*,#40453,.T.);
#57609=ORIENTED_EDGE('',*,*,#40651,.T.);
#57610=ORIENTED_EDGE('',*,*,#40740,.F.);
#57611=ORIENTED_EDGE('',*,*,#40741,.F.);
#57612=ORIENTED_EDGE('',*,*,#40456,.T.);
#57613=ORIENTED_EDGE('',*,*,#40462,.T.);
#57614=ORIENTED_EDGE('',*,*,#40457,.T.);
#57615=ORIENTED_EDGE('',*,*,#40742,.F.);
#57616=ORIENTED_EDGE('',*,*,#40743,.F.);
#57617=ORIENTED_EDGE('',*,*,#40463,.T.);
#57618=ORIENTED_EDGE('',*,*,#40743,.T.);
#57619=ORIENTED_EDGE('',*,*,#40744,.F.);
#57620=ORIENTED_EDGE('',*,*,#40461,.T.);
#57621=ORIENTED_EDGE('',*,*,#40469,.T.);
#57622=ORIENTED_EDGE('',*,*,#40464,.T.);
#57623=ORIENTED_EDGE('',*,*,#40745,.F.);
#57624=ORIENTED_EDGE('',*,*,#40746,.F.);
#57625=ORIENTED_EDGE('',*,*,#40470,.T.);
#57626=ORIENTED_EDGE('',*,*,#40746,.T.);
#57627=ORIENTED_EDGE('',*,*,#40747,.F.);
#57628=ORIENTED_EDGE('',*,*,#40468,.T.);
#57629=ORIENTED_EDGE('',*,*,#40476,.T.);
#57630=ORIENTED_EDGE('',*,*,#40471,.T.);
#57631=ORIENTED_EDGE('',*,*,#40748,.F.);
#57632=ORIENTED_EDGE('',*,*,#40749,.F.);
#57633=ORIENTED_EDGE('',*,*,#40477,.T.);
#57634=ORIENTED_EDGE('',*,*,#40749,.T.);
#57635=ORIENTED_EDGE('',*,*,#40750,.F.);
#57636=ORIENTED_EDGE('',*,*,#40475,.T.);
#57637=ORIENTED_EDGE('',*,*,#40483,.T.);
#57638=ORIENTED_EDGE('',*,*,#40478,.T.);
#57639=ORIENTED_EDGE('',*,*,#40751,.F.);
#57640=ORIENTED_EDGE('',*,*,#40752,.F.);
#57641=ORIENTED_EDGE('',*,*,#40484,.T.);
#57642=ORIENTED_EDGE('',*,*,#40752,.T.);
#57643=ORIENTED_EDGE('',*,*,#40753,.F.);
#57644=ORIENTED_EDGE('',*,*,#40482,.T.);
#57645=ORIENTED_EDGE('',*,*,#40490,.T.);
#57646=ORIENTED_EDGE('',*,*,#40485,.T.);
#57647=ORIENTED_EDGE('',*,*,#40754,.F.);
#57648=ORIENTED_EDGE('',*,*,#40755,.F.);
#57649=ORIENTED_EDGE('',*,*,#40491,.T.);
#57650=ORIENTED_EDGE('',*,*,#40755,.T.);
#57651=ORIENTED_EDGE('',*,*,#40756,.F.);
#57652=ORIENTED_EDGE('',*,*,#40489,.T.);
#57653=ORIENTED_EDGE('',*,*,#40497,.T.);
#57654=ORIENTED_EDGE('',*,*,#40492,.T.);
#57655=ORIENTED_EDGE('',*,*,#40757,.F.);
#57656=ORIENTED_EDGE('',*,*,#40758,.F.);
#57657=ORIENTED_EDGE('',*,*,#40498,.T.);
#57658=ORIENTED_EDGE('',*,*,#40758,.T.);
#57659=ORIENTED_EDGE('',*,*,#40759,.F.);
#57660=ORIENTED_EDGE('',*,*,#40496,.T.);
#57661=ORIENTED_EDGE('',*,*,#40504,.T.);
#57662=ORIENTED_EDGE('',*,*,#40499,.T.);
#57663=ORIENTED_EDGE('',*,*,#40760,.F.);
#57664=ORIENTED_EDGE('',*,*,#40761,.F.);
#57665=ORIENTED_EDGE('',*,*,#40505,.T.);
#57666=ORIENTED_EDGE('',*,*,#40761,.T.);
#57667=ORIENTED_EDGE('',*,*,#40762,.F.);
#57668=ORIENTED_EDGE('',*,*,#40503,.T.);
#57669=ORIENTED_EDGE('',*,*,#40511,.T.);
#57670=ORIENTED_EDGE('',*,*,#40506,.T.);
#57671=ORIENTED_EDGE('',*,*,#40763,.F.);
#57672=ORIENTED_EDGE('',*,*,#40764,.F.);
#57673=ORIENTED_EDGE('',*,*,#40512,.T.);
#57674=ORIENTED_EDGE('',*,*,#40764,.T.);
#57675=ORIENTED_EDGE('',*,*,#40765,.F.);
#57676=ORIENTED_EDGE('',*,*,#40510,.T.);
#57677=ORIENTED_EDGE('',*,*,#40518,.T.);
#57678=ORIENTED_EDGE('',*,*,#40513,.T.);
#57679=ORIENTED_EDGE('',*,*,#40766,.F.);
#57680=ORIENTED_EDGE('',*,*,#40767,.F.);
#57681=ORIENTED_EDGE('',*,*,#40519,.T.);
#57682=ORIENTED_EDGE('',*,*,#40767,.T.);
#57683=ORIENTED_EDGE('',*,*,#40768,.F.);
#57684=ORIENTED_EDGE('',*,*,#40517,.T.);
#57685=ORIENTED_EDGE('',*,*,#40525,.T.);
#57686=ORIENTED_EDGE('',*,*,#40520,.T.);
#57687=ORIENTED_EDGE('',*,*,#40769,.F.);
#57688=ORIENTED_EDGE('',*,*,#40770,.F.);
#57689=ORIENTED_EDGE('',*,*,#40526,.T.);
#57690=ORIENTED_EDGE('',*,*,#40770,.T.);
#57691=ORIENTED_EDGE('',*,*,#40771,.F.);
#57692=ORIENTED_EDGE('',*,*,#40524,.T.);
#57693=ORIENTED_EDGE('',*,*,#40532,.T.);
#57694=ORIENTED_EDGE('',*,*,#40527,.T.);
#57695=ORIENTED_EDGE('',*,*,#40772,.F.);
#57696=ORIENTED_EDGE('',*,*,#40773,.F.);
#57697=ORIENTED_EDGE('',*,*,#40533,.T.);
#57698=ORIENTED_EDGE('',*,*,#40773,.T.);
#57699=ORIENTED_EDGE('',*,*,#40774,.F.);
#57700=ORIENTED_EDGE('',*,*,#40531,.T.);
#57701=ORIENTED_EDGE('',*,*,#40539,.T.);
#57702=ORIENTED_EDGE('',*,*,#40534,.T.);
#57703=ORIENTED_EDGE('',*,*,#40775,.F.);
#57704=ORIENTED_EDGE('',*,*,#40776,.F.);
#57705=ORIENTED_EDGE('',*,*,#40540,.T.);
#57706=ORIENTED_EDGE('',*,*,#40776,.T.);
#57707=ORIENTED_EDGE('',*,*,#40777,.F.);
#57708=ORIENTED_EDGE('',*,*,#40538,.T.);
#57709=ORIENTED_EDGE('',*,*,#40546,.T.);
#57710=ORIENTED_EDGE('',*,*,#40541,.T.);
#57711=ORIENTED_EDGE('',*,*,#40778,.F.);
#57712=ORIENTED_EDGE('',*,*,#40779,.F.);
#57713=ORIENTED_EDGE('',*,*,#40547,.T.);
#57714=ORIENTED_EDGE('',*,*,#40779,.T.);
#57715=ORIENTED_EDGE('',*,*,#40780,.F.);
#57716=ORIENTED_EDGE('',*,*,#40545,.T.);
#57717=ORIENTED_EDGE('',*,*,#34392,.T.);
#57718=ORIENTED_EDGE('',*,*,#40548,.T.);
#57719=ORIENTED_EDGE('',*,*,#40781,.F.);
#57720=ORIENTED_EDGE('',*,*,#40782,.F.);
#57721=ORIENTED_EDGE('',*,*,#34389,.T.);
#57722=ORIENTED_EDGE('',*,*,#40782,.T.);
#57723=ORIENTED_EDGE('',*,*,#40783,.F.);
#57724=ORIENTED_EDGE('',*,*,#40550,.T.);
#57725=ORIENTED_EDGE('',*,*,#40556,.T.);
#57726=ORIENTED_EDGE('',*,*,#40551,.T.);
#57727=ORIENTED_EDGE('',*,*,#40784,.F.);
#57728=ORIENTED_EDGE('',*,*,#40785,.F.);
#57729=ORIENTED_EDGE('',*,*,#40557,.T.);
#57730=ORIENTED_EDGE('',*,*,#40785,.T.);
#57731=ORIENTED_EDGE('',*,*,#40786,.F.);
#57732=ORIENTED_EDGE('',*,*,#40555,.T.);
#57733=ORIENTED_EDGE('',*,*,#40563,.T.);
#57734=ORIENTED_EDGE('',*,*,#40558,.T.);
#57735=ORIENTED_EDGE('',*,*,#40787,.F.);
#57736=ORIENTED_EDGE('',*,*,#40788,.F.);
#57737=ORIENTED_EDGE('',*,*,#40564,.T.);
#57738=ORIENTED_EDGE('',*,*,#40788,.T.);
#57739=ORIENTED_EDGE('',*,*,#40789,.F.);
#57740=ORIENTED_EDGE('',*,*,#40562,.T.);
#57741=ORIENTED_EDGE('',*,*,#40570,.T.);
#57742=ORIENTED_EDGE('',*,*,#40565,.T.);
#57743=ORIENTED_EDGE('',*,*,#40790,.F.);
#57744=ORIENTED_EDGE('',*,*,#40791,.F.);
#57745=ORIENTED_EDGE('',*,*,#40571,.T.);
#57746=ORIENTED_EDGE('',*,*,#40791,.T.);
#57747=ORIENTED_EDGE('',*,*,#40792,.F.);
#57748=ORIENTED_EDGE('',*,*,#40569,.T.);
#57749=ORIENTED_EDGE('',*,*,#40577,.T.);
#57750=ORIENTED_EDGE('',*,*,#40572,.T.);
#57751=ORIENTED_EDGE('',*,*,#40793,.F.);
#57752=ORIENTED_EDGE('',*,*,#40794,.F.);
#57753=ORIENTED_EDGE('',*,*,#40578,.T.);
#57754=ORIENTED_EDGE('',*,*,#40794,.T.);
#57755=ORIENTED_EDGE('',*,*,#40795,.F.);
#57756=ORIENTED_EDGE('',*,*,#40576,.T.);
#57757=ORIENTED_EDGE('',*,*,#40584,.T.);
#57758=ORIENTED_EDGE('',*,*,#40579,.T.);
#57759=ORIENTED_EDGE('',*,*,#40796,.F.);
#57760=ORIENTED_EDGE('',*,*,#40797,.F.);
#57761=ORIENTED_EDGE('',*,*,#40585,.T.);
#57762=ORIENTED_EDGE('',*,*,#40797,.T.);
#57763=ORIENTED_EDGE('',*,*,#40798,.F.);
#57764=ORIENTED_EDGE('',*,*,#40583,.T.);
#57765=ORIENTED_EDGE('',*,*,#40591,.T.);
#57766=ORIENTED_EDGE('',*,*,#40586,.T.);
#57767=ORIENTED_EDGE('',*,*,#40799,.F.);
#57768=ORIENTED_EDGE('',*,*,#40800,.F.);
#57769=ORIENTED_EDGE('',*,*,#40592,.T.);
#57770=ORIENTED_EDGE('',*,*,#40800,.T.);
#57771=ORIENTED_EDGE('',*,*,#40801,.F.);
#57772=ORIENTED_EDGE('',*,*,#40590,.T.);
#57773=ORIENTED_EDGE('',*,*,#40598,.T.);
#57774=ORIENTED_EDGE('',*,*,#40593,.T.);
#57775=ORIENTED_EDGE('',*,*,#40802,.F.);
#57776=ORIENTED_EDGE('',*,*,#40803,.F.);
#57777=ORIENTED_EDGE('',*,*,#40599,.T.);
#57778=ORIENTED_EDGE('',*,*,#40803,.T.);
#57779=ORIENTED_EDGE('',*,*,#40804,.F.);
#57780=ORIENTED_EDGE('',*,*,#40597,.T.);
#57781=ORIENTED_EDGE('',*,*,#40605,.T.);
#57782=ORIENTED_EDGE('',*,*,#40600,.T.);
#57783=ORIENTED_EDGE('',*,*,#40805,.F.);
#57784=ORIENTED_EDGE('',*,*,#40806,.F.);
#57785=ORIENTED_EDGE('',*,*,#40606,.T.);
#57786=ORIENTED_EDGE('',*,*,#40806,.T.);
#57787=ORIENTED_EDGE('',*,*,#40807,.F.);
#57788=ORIENTED_EDGE('',*,*,#40604,.T.);
#57789=ORIENTED_EDGE('',*,*,#40612,.T.);
#57790=ORIENTED_EDGE('',*,*,#40607,.T.);
#57791=ORIENTED_EDGE('',*,*,#40808,.F.);
#57792=ORIENTED_EDGE('',*,*,#40809,.F.);
#57793=ORIENTED_EDGE('',*,*,#40613,.T.);
#57794=ORIENTED_EDGE('',*,*,#40809,.T.);
#57795=ORIENTED_EDGE('',*,*,#40810,.F.);
#57796=ORIENTED_EDGE('',*,*,#40611,.T.);
#57797=ORIENTED_EDGE('',*,*,#40619,.T.);
#57798=ORIENTED_EDGE('',*,*,#40614,.T.);
#57799=ORIENTED_EDGE('',*,*,#40811,.F.);
#57800=ORIENTED_EDGE('',*,*,#40812,.F.);
#57801=ORIENTED_EDGE('',*,*,#40620,.T.);
#57802=ORIENTED_EDGE('',*,*,#40812,.T.);
#57803=ORIENTED_EDGE('',*,*,#40813,.F.);
#57804=ORIENTED_EDGE('',*,*,#40618,.T.);
#57805=ORIENTED_EDGE('',*,*,#40626,.T.);
#57806=ORIENTED_EDGE('',*,*,#40621,.T.);
#57807=ORIENTED_EDGE('',*,*,#40814,.F.);
#57808=ORIENTED_EDGE('',*,*,#40815,.F.);
#57809=ORIENTED_EDGE('',*,*,#40627,.T.);
#57810=ORIENTED_EDGE('',*,*,#40815,.T.);
#57811=ORIENTED_EDGE('',*,*,#40816,.F.);
#57812=ORIENTED_EDGE('',*,*,#40625,.T.);
#57813=ORIENTED_EDGE('',*,*,#40817,.F.);
#57814=ORIENTED_EDGE('',*,*,#40818,.F.);
#57815=ORIENTED_EDGE('',*,*,#40633,.T.);
#57816=ORIENTED_EDGE('',*,*,#40628,.T.);
#57817=ORIENTED_EDGE('',*,*,#40634,.T.);
#57818=ORIENTED_EDGE('',*,*,#40818,.T.);
#57819=ORIENTED_EDGE('',*,*,#40819,.F.);
#57820=ORIENTED_EDGE('',*,*,#40632,.T.);
#57821=ORIENTED_EDGE('',*,*,#40640,.T.);
#57822=ORIENTED_EDGE('',*,*,#40635,.T.);
#57823=ORIENTED_EDGE('',*,*,#40820,.F.);
#57824=ORIENTED_EDGE('',*,*,#40821,.F.);
#57825=ORIENTED_EDGE('',*,*,#40641,.T.);
#57826=ORIENTED_EDGE('',*,*,#40821,.T.);
#57827=ORIENTED_EDGE('',*,*,#40822,.F.);
#57828=ORIENTED_EDGE('',*,*,#40639,.T.);
#57829=ORIENTED_EDGE('',*,*,#40647,.T.);
#57830=ORIENTED_EDGE('',*,*,#40642,.T.);
#57831=ORIENTED_EDGE('',*,*,#40823,.F.);
#57832=ORIENTED_EDGE('',*,*,#40824,.F.);
#57833=ORIENTED_EDGE('',*,*,#40648,.T.);
#57834=ORIENTED_EDGE('',*,*,#40824,.T.);
#57835=ORIENTED_EDGE('',*,*,#40825,.F.);
#57836=ORIENTED_EDGE('',*,*,#40646,.T.);
#57837=ORIENTED_EDGE('',*,*,#40650,.T.);
#57838=ORIENTED_EDGE('',*,*,#40652,.T.);
#57839=ORIENTED_EDGE('',*,*,#40826,.F.);
#57840=ORIENTED_EDGE('',*,*,#40740,.T.);
#57841=ORIENTED_EDGE('',*,*,#40827,.T.);
#57842=ORIENTED_EDGE('',*,*,#40828,.F.);
#57843=ORIENTED_EDGE('',*,*,#40653,.T.);
#57844=ORIENTED_EDGE('',*,*,#40829,.F.);
#57845=ORIENTED_EDGE('',*,*,#40830,.F.);
#57846=ORIENTED_EDGE('',*,*,#40831,.F.);
#57847=ORIENTED_EDGE('',*,*,#40832,.F.);
#57848=ORIENTED_EDGE('',*,*,#40827,.F.);
#57849=ORIENTED_EDGE('',*,*,#40832,.T.);
#57850=ORIENTED_EDGE('',*,*,#40833,.F.);
#57851=ORIENTED_EDGE('',*,*,#40655,.T.);
#57852=ORIENTED_EDGE('',*,*,#40828,.T.);
#57853=ORIENTED_EDGE('',*,*,#40834,.T.);
#57854=ORIENTED_EDGE('',*,*,#40835,.F.);
#57855=ORIENTED_EDGE('',*,*,#40657,.T.);
#57856=ORIENTED_EDGE('',*,*,#40836,.F.);
#57857=ORIENTED_EDGE('',*,*,#40837,.F.);
#57858=ORIENTED_EDGE('',*,*,#40838,.F.);
#57859=ORIENTED_EDGE('',*,*,#40839,.F.);
#57860=ORIENTED_EDGE('',*,*,#40834,.F.);
#57861=ORIENTED_EDGE('',*,*,#40839,.T.);
#57862=ORIENTED_EDGE('',*,*,#40840,.F.);
#57863=ORIENTED_EDGE('',*,*,#40658,.T.);
#57864=ORIENTED_EDGE('',*,*,#40835,.T.);
#57865=ORIENTED_EDGE('',*,*,#40841,.T.);
#57866=ORIENTED_EDGE('',*,*,#40842,.F.);
#57867=ORIENTED_EDGE('',*,*,#40660,.T.);
#57868=ORIENTED_EDGE('',*,*,#40843,.F.);
#57869=ORIENTED_EDGE('',*,*,#40844,.F.);
#57870=ORIENTED_EDGE('',*,*,#40845,.F.);
#57871=ORIENTED_EDGE('',*,*,#40846,.F.);
#57872=ORIENTED_EDGE('',*,*,#40841,.F.);
#57873=ORIENTED_EDGE('',*,*,#40846,.T.);
#57874=ORIENTED_EDGE('',*,*,#40847,.F.);
#57875=ORIENTED_EDGE('',*,*,#40661,.T.);
#57876=ORIENTED_EDGE('',*,*,#40842,.T.);
#57877=ORIENTED_EDGE('',*,*,#40848,.T.);
#57878=ORIENTED_EDGE('',*,*,#40849,.F.);
#57879=ORIENTED_EDGE('',*,*,#40663,.T.);
#57880=ORIENTED_EDGE('',*,*,#40850,.F.);
#57881=ORIENTED_EDGE('',*,*,#40851,.F.);
#57882=ORIENTED_EDGE('',*,*,#40852,.F.);
#57883=ORIENTED_EDGE('',*,*,#40853,.F.);
#57884=ORIENTED_EDGE('',*,*,#40848,.F.);
#57885=ORIENTED_EDGE('',*,*,#40853,.T.);
#57886=ORIENTED_EDGE('',*,*,#40854,.F.);
#57887=ORIENTED_EDGE('',*,*,#40664,.T.);
#57888=ORIENTED_EDGE('',*,*,#40849,.T.);
#57889=ORIENTED_EDGE('',*,*,#40855,.T.);
#57890=ORIENTED_EDGE('',*,*,#40856,.F.);
#57891=ORIENTED_EDGE('',*,*,#40666,.T.);
#57892=ORIENTED_EDGE('',*,*,#40857,.F.);
#57893=ORIENTED_EDGE('',*,*,#40858,.F.);
#57894=ORIENTED_EDGE('',*,*,#40859,.F.);
#57895=ORIENTED_EDGE('',*,*,#40860,.F.);
#57896=ORIENTED_EDGE('',*,*,#40855,.F.);
#57897=ORIENTED_EDGE('',*,*,#40860,.T.);
#57898=ORIENTED_EDGE('',*,*,#40861,.F.);
#57899=ORIENTED_EDGE('',*,*,#40667,.T.);
#57900=ORIENTED_EDGE('',*,*,#40856,.T.);
#57901=ORIENTED_EDGE('',*,*,#40862,.T.);
#57902=ORIENTED_EDGE('',*,*,#40863,.F.);
#57903=ORIENTED_EDGE('',*,*,#40669,.T.);
#57904=ORIENTED_EDGE('',*,*,#40864,.F.);
#57905=ORIENTED_EDGE('',*,*,#40865,.F.);
#57906=ORIENTED_EDGE('',*,*,#40866,.F.);
#57907=ORIENTED_EDGE('',*,*,#40867,.F.);
#57908=ORIENTED_EDGE('',*,*,#40862,.F.);
#57909=ORIENTED_EDGE('',*,*,#40867,.T.);
#57910=ORIENTED_EDGE('',*,*,#40868,.F.);
#57911=ORIENTED_EDGE('',*,*,#40670,.T.);
#57912=ORIENTED_EDGE('',*,*,#40863,.T.);
#57913=ORIENTED_EDGE('',*,*,#40869,.T.);
#57914=ORIENTED_EDGE('',*,*,#40870,.F.);
#57915=ORIENTED_EDGE('',*,*,#40672,.T.);
#57916=ORIENTED_EDGE('',*,*,#40871,.F.);
#57917=ORIENTED_EDGE('',*,*,#40872,.F.);
#57918=ORIENTED_EDGE('',*,*,#40873,.F.);
#57919=ORIENTED_EDGE('',*,*,#40874,.F.);
#57920=ORIENTED_EDGE('',*,*,#40869,.F.);
#57921=ORIENTED_EDGE('',*,*,#40874,.T.);
#57922=ORIENTED_EDGE('',*,*,#40875,.F.);
#57923=ORIENTED_EDGE('',*,*,#40673,.T.);
#57924=ORIENTED_EDGE('',*,*,#40870,.T.);
#57925=ORIENTED_EDGE('',*,*,#40876,.T.);
#57926=ORIENTED_EDGE('',*,*,#40877,.F.);
#57927=ORIENTED_EDGE('',*,*,#40675,.T.);
#57928=ORIENTED_EDGE('',*,*,#40878,.F.);
#57929=ORIENTED_EDGE('',*,*,#40879,.F.);
#57930=ORIENTED_EDGE('',*,*,#40880,.F.);
#57931=ORIENTED_EDGE('',*,*,#40881,.F.);
#57932=ORIENTED_EDGE('',*,*,#40876,.F.);
#57933=ORIENTED_EDGE('',*,*,#40881,.T.);
#57934=ORIENTED_EDGE('',*,*,#40882,.F.);
#57935=ORIENTED_EDGE('',*,*,#40676,.T.);
#57936=ORIENTED_EDGE('',*,*,#40877,.T.);
#57937=ORIENTED_EDGE('',*,*,#40883,.T.);
#57938=ORIENTED_EDGE('',*,*,#40884,.F.);
#57939=ORIENTED_EDGE('',*,*,#40678,.T.);
#57940=ORIENTED_EDGE('',*,*,#40885,.F.);
#57941=ORIENTED_EDGE('',*,*,#40886,.F.);
#57942=ORIENTED_EDGE('',*,*,#40887,.F.);
#57943=ORIENTED_EDGE('',*,*,#40888,.F.);
#57944=ORIENTED_EDGE('',*,*,#40883,.F.);
#57945=ORIENTED_EDGE('',*,*,#40888,.T.);
#57946=ORIENTED_EDGE('',*,*,#40889,.F.);
#57947=ORIENTED_EDGE('',*,*,#40679,.T.);
#57948=ORIENTED_EDGE('',*,*,#40884,.T.);
#57949=ORIENTED_EDGE('',*,*,#40890,.T.);
#57950=ORIENTED_EDGE('',*,*,#40891,.F.);
#57951=ORIENTED_EDGE('',*,*,#40681,.T.);
#57952=ORIENTED_EDGE('',*,*,#40892,.F.);
#57953=ORIENTED_EDGE('',*,*,#40893,.F.);
#57954=ORIENTED_EDGE('',*,*,#40894,.F.);
#57955=ORIENTED_EDGE('',*,*,#40895,.F.);
#57956=ORIENTED_EDGE('',*,*,#40890,.F.);
#57957=ORIENTED_EDGE('',*,*,#40895,.T.);
#57958=ORIENTED_EDGE('',*,*,#40896,.F.);
#57959=ORIENTED_EDGE('',*,*,#40682,.T.);
#57960=ORIENTED_EDGE('',*,*,#40891,.T.);
#57961=ORIENTED_EDGE('',*,*,#40897,.T.);
#57962=ORIENTED_EDGE('',*,*,#40898,.F.);
#57963=ORIENTED_EDGE('',*,*,#40684,.T.);
#57964=ORIENTED_EDGE('',*,*,#40899,.F.);
#57965=ORIENTED_EDGE('',*,*,#40900,.F.);
#57966=ORIENTED_EDGE('',*,*,#40901,.F.);
#57967=ORIENTED_EDGE('',*,*,#40902,.F.);
#57968=ORIENTED_EDGE('',*,*,#40897,.F.);
#57969=ORIENTED_EDGE('',*,*,#40902,.T.);
#57970=ORIENTED_EDGE('',*,*,#40903,.F.);
#57971=ORIENTED_EDGE('',*,*,#40685,.T.);
#57972=ORIENTED_EDGE('',*,*,#40898,.T.);
#57973=ORIENTED_EDGE('',*,*,#40904,.T.);
#57974=ORIENTED_EDGE('',*,*,#40905,.F.);
#57975=ORIENTED_EDGE('',*,*,#40687,.T.);
#57976=ORIENTED_EDGE('',*,*,#40906,.F.);
#57977=ORIENTED_EDGE('',*,*,#40907,.F.);
#57978=ORIENTED_EDGE('',*,*,#40908,.F.);
#57979=ORIENTED_EDGE('',*,*,#40909,.F.);
#57980=ORIENTED_EDGE('',*,*,#40904,.F.);
#57981=ORIENTED_EDGE('',*,*,#40909,.T.);
#57982=ORIENTED_EDGE('',*,*,#40910,.F.);
#57983=ORIENTED_EDGE('',*,*,#40688,.T.);
#57984=ORIENTED_EDGE('',*,*,#40905,.T.);
#57985=ORIENTED_EDGE('',*,*,#40911,.T.);
#57986=ORIENTED_EDGE('',*,*,#40912,.F.);
#57987=ORIENTED_EDGE('',*,*,#40690,.T.);
#57988=ORIENTED_EDGE('',*,*,#40913,.F.);
#57989=ORIENTED_EDGE('',*,*,#40914,.F.);
#57990=ORIENTED_EDGE('',*,*,#40915,.F.);
#57991=ORIENTED_EDGE('',*,*,#40916,.F.);
#57992=ORIENTED_EDGE('',*,*,#40911,.F.);
#57993=ORIENTED_EDGE('',*,*,#40916,.T.);
#57994=ORIENTED_EDGE('',*,*,#40917,.F.);
#57995=ORIENTED_EDGE('',*,*,#40691,.T.);
#57996=ORIENTED_EDGE('',*,*,#40912,.T.);
#57997=ORIENTED_EDGE('',*,*,#40918,.T.);
#57998=ORIENTED_EDGE('',*,*,#40919,.F.);
#57999=ORIENTED_EDGE('',*,*,#40693,.T.);
#58000=ORIENTED_EDGE('',*,*,#40920,.F.);
#58001=ORIENTED_EDGE('',*,*,#40921,.F.);
#58002=ORIENTED_EDGE('',*,*,#40922,.F.);
#58003=ORIENTED_EDGE('',*,*,#40923,.F.);
#58004=ORIENTED_EDGE('',*,*,#40918,.F.);
#58005=ORIENTED_EDGE('',*,*,#40923,.T.);
#58006=ORIENTED_EDGE('',*,*,#40924,.F.);
#58007=ORIENTED_EDGE('',*,*,#40694,.T.);
#58008=ORIENTED_EDGE('',*,*,#40919,.T.);
#58009=ORIENTED_EDGE('',*,*,#34385,.T.);
#58010=ORIENTED_EDGE('',*,*,#40925,.F.);
#58011=ORIENTED_EDGE('',*,*,#40696,.T.);
#58012=ORIENTED_EDGE('',*,*,#40926,.F.);
#58013=ORIENTED_EDGE('',*,*,#34388,.T.);
#58014=ORIENTED_EDGE('',*,*,#40927,.F.);
#58015=ORIENTED_EDGE('',*,*,#40697,.T.);
#58016=ORIENTED_EDGE('',*,*,#40925,.T.);
#58017=ORIENTED_EDGE('',*,*,#40928,.T.);
#58018=ORIENTED_EDGE('',*,*,#40929,.F.);
#58019=ORIENTED_EDGE('',*,*,#40699,.T.);
#58020=ORIENTED_EDGE('',*,*,#40930,.F.);
#58021=ORIENTED_EDGE('',*,*,#40931,.F.);
#58022=ORIENTED_EDGE('',*,*,#40932,.F.);
#58023=ORIENTED_EDGE('',*,*,#40933,.F.);
#58024=ORIENTED_EDGE('',*,*,#40928,.F.);
#58025=ORIENTED_EDGE('',*,*,#40933,.T.);
#58026=ORIENTED_EDGE('',*,*,#40934,.F.);
#58027=ORIENTED_EDGE('',*,*,#40700,.T.);
#58028=ORIENTED_EDGE('',*,*,#40929,.T.);
#58029=ORIENTED_EDGE('',*,*,#40935,.T.);
#58030=ORIENTED_EDGE('',*,*,#40936,.F.);
#58031=ORIENTED_EDGE('',*,*,#40702,.T.);
#58032=ORIENTED_EDGE('',*,*,#40937,.F.);
#58033=ORIENTED_EDGE('',*,*,#40938,.F.);
#58034=ORIENTED_EDGE('',*,*,#40939,.F.);
#58035=ORIENTED_EDGE('',*,*,#40940,.F.);
#58036=ORIENTED_EDGE('',*,*,#40935,.F.);
#58037=ORIENTED_EDGE('',*,*,#40940,.T.);
#58038=ORIENTED_EDGE('',*,*,#40941,.F.);
#58039=ORIENTED_EDGE('',*,*,#40703,.T.);
#58040=ORIENTED_EDGE('',*,*,#40936,.T.);
#58041=ORIENTED_EDGE('',*,*,#40942,.T.);
#58042=ORIENTED_EDGE('',*,*,#40943,.F.);
#58043=ORIENTED_EDGE('',*,*,#40705,.T.);
#58044=ORIENTED_EDGE('',*,*,#40944,.F.);
#58045=ORIENTED_EDGE('',*,*,#40945,.F.);
#58046=ORIENTED_EDGE('',*,*,#40946,.F.);
#58047=ORIENTED_EDGE('',*,*,#40947,.F.);
#58048=ORIENTED_EDGE('',*,*,#40942,.F.);
#58049=ORIENTED_EDGE('',*,*,#40947,.T.);
#58050=ORIENTED_EDGE('',*,*,#40948,.F.);
#58051=ORIENTED_EDGE('',*,*,#40706,.T.);
#58052=ORIENTED_EDGE('',*,*,#40943,.T.);
#58053=ORIENTED_EDGE('',*,*,#40949,.T.);
#58054=ORIENTED_EDGE('',*,*,#40950,.F.);
#58055=ORIENTED_EDGE('',*,*,#40708,.T.);
#58056=ORIENTED_EDGE('',*,*,#40951,.F.);
#58057=ORIENTED_EDGE('',*,*,#40952,.F.);
#58058=ORIENTED_EDGE('',*,*,#40953,.F.);
#58059=ORIENTED_EDGE('',*,*,#40954,.F.);
#58060=ORIENTED_EDGE('',*,*,#40949,.F.);
#58061=ORIENTED_EDGE('',*,*,#40954,.T.);
#58062=ORIENTED_EDGE('',*,*,#40955,.F.);
#58063=ORIENTED_EDGE('',*,*,#40709,.T.);
#58064=ORIENTED_EDGE('',*,*,#40950,.T.);
#58065=ORIENTED_EDGE('',*,*,#40956,.T.);
#58066=ORIENTED_EDGE('',*,*,#40957,.F.);
#58067=ORIENTED_EDGE('',*,*,#40711,.T.);
#58068=ORIENTED_EDGE('',*,*,#40958,.F.);
#58069=ORIENTED_EDGE('',*,*,#40959,.T.);
#58070=ORIENTED_EDGE('',*,*,#40960,.F.);
#58071=ORIENTED_EDGE('',*,*,#40712,.T.);
#58072=ORIENTED_EDGE('',*,*,#40957,.T.);
#58073=ORIENTED_EDGE('',*,*,#40961,.F.);
#58074=ORIENTED_EDGE('',*,*,#40962,.F.);
#58075=ORIENTED_EDGE('',*,*,#40959,.F.);
#58076=ORIENTED_EDGE('',*,*,#40956,.F.);
#58077=ORIENTED_EDGE('',*,*,#40714,.T.);
#58078=ORIENTED_EDGE('',*,*,#40963,.F.);
#58079=ORIENTED_EDGE('',*,*,#40964,.T.);
#58080=ORIENTED_EDGE('',*,*,#40965,.F.);
#58081=ORIENTED_EDGE('',*,*,#40966,.F.);
#58082=ORIENTED_EDGE('',*,*,#40964,.F.);
#58083=ORIENTED_EDGE('',*,*,#40967,.F.);
#58084=ORIENTED_EDGE('',*,*,#40968,.F.);
#58085=ORIENTED_EDGE('',*,*,#40715,.T.);
#58086=ORIENTED_EDGE('',*,*,#40965,.T.);
#58087=ORIENTED_EDGE('',*,*,#40966,.T.);
#58088=ORIENTED_EDGE('',*,*,#40969,.F.);
#58089=ORIENTED_EDGE('',*,*,#40970,.T.);
#58090=ORIENTED_EDGE('',*,*,#40971,.F.);
#58091=ORIENTED_EDGE('',*,*,#40717,.T.);
#58092=ORIENTED_EDGE('',*,*,#40972,.F.);
#58093=ORIENTED_EDGE('',*,*,#40973,.F.);
#58094=ORIENTED_EDGE('',*,*,#40974,.F.);
#58095=ORIENTED_EDGE('',*,*,#40975,.F.);
#58096=ORIENTED_EDGE('',*,*,#40970,.F.);
#58097=ORIENTED_EDGE('',*,*,#40975,.T.);
#58098=ORIENTED_EDGE('',*,*,#40976,.F.);
#58099=ORIENTED_EDGE('',*,*,#40718,.T.);
#58100=ORIENTED_EDGE('',*,*,#40971,.T.);
#58101=ORIENTED_EDGE('',*,*,#40977,.T.);
#58102=ORIENTED_EDGE('',*,*,#40978,.F.);
#58103=ORIENTED_EDGE('',*,*,#40720,.T.);
#58104=ORIENTED_EDGE('',*,*,#40979,.F.);
#58105=ORIENTED_EDGE('',*,*,#40980,.F.);
#58106=ORIENTED_EDGE('',*,*,#40981,.F.);
#58107=ORIENTED_EDGE('',*,*,#40982,.F.);
#58108=ORIENTED_EDGE('',*,*,#40977,.F.);
#58109=ORIENTED_EDGE('',*,*,#40982,.T.);
#58110=ORIENTED_EDGE('',*,*,#40983,.F.);
#58111=ORIENTED_EDGE('',*,*,#40721,.T.);
#58112=ORIENTED_EDGE('',*,*,#40978,.T.);
#58113=ORIENTED_EDGE('',*,*,#40984,.T.);
#58114=ORIENTED_EDGE('',*,*,#40985,.F.);
#58115=ORIENTED_EDGE('',*,*,#40723,.T.);
#58116=ORIENTED_EDGE('',*,*,#40986,.F.);
#58117=ORIENTED_EDGE('',*,*,#40987,.F.);
#58118=ORIENTED_EDGE('',*,*,#40988,.F.);
#58119=ORIENTED_EDGE('',*,*,#40989,.F.);
#58120=ORIENTED_EDGE('',*,*,#40984,.F.);
#58121=ORIENTED_EDGE('',*,*,#40989,.T.);
#58122=ORIENTED_EDGE('',*,*,#40990,.F.);
#58123=ORIENTED_EDGE('',*,*,#40724,.T.);
#58124=ORIENTED_EDGE('',*,*,#40985,.T.);
#58125=ORIENTED_EDGE('',*,*,#40991,.T.);
#58126=ORIENTED_EDGE('',*,*,#40992,.F.);
#58127=ORIENTED_EDGE('',*,*,#40726,.T.);
#58128=ORIENTED_EDGE('',*,*,#40993,.F.);
#58129=ORIENTED_EDGE('',*,*,#40994,.F.);
#58130=ORIENTED_EDGE('',*,*,#40995,.F.);
#58131=ORIENTED_EDGE('',*,*,#40996,.F.);
#58132=ORIENTED_EDGE('',*,*,#40991,.F.);
#58133=ORIENTED_EDGE('',*,*,#40996,.T.);
#58134=ORIENTED_EDGE('',*,*,#40997,.F.);
#58135=ORIENTED_EDGE('',*,*,#40727,.T.);
#58136=ORIENTED_EDGE('',*,*,#40992,.T.);
#58137=ORIENTED_EDGE('',*,*,#40998,.T.);
#58138=ORIENTED_EDGE('',*,*,#40999,.F.);
#58139=ORIENTED_EDGE('',*,*,#40729,.T.);
#58140=ORIENTED_EDGE('',*,*,#41000,.F.);
#58141=ORIENTED_EDGE('',*,*,#41001,.F.);
#58142=ORIENTED_EDGE('',*,*,#41002,.F.);
#58143=ORIENTED_EDGE('',*,*,#41003,.F.);
#58144=ORIENTED_EDGE('',*,*,#40998,.F.);
#58145=ORIENTED_EDGE('',*,*,#41003,.T.);
#58146=ORIENTED_EDGE('',*,*,#41004,.F.);
#58147=ORIENTED_EDGE('',*,*,#40730,.T.);
#58148=ORIENTED_EDGE('',*,*,#40999,.T.);
#58149=ORIENTED_EDGE('',*,*,#41005,.T.);
#58150=ORIENTED_EDGE('',*,*,#41006,.F.);
#58151=ORIENTED_EDGE('',*,*,#40732,.T.);
#58152=ORIENTED_EDGE('',*,*,#41007,.F.);
#58153=ORIENTED_EDGE('',*,*,#41008,.F.);
#58154=ORIENTED_EDGE('',*,*,#41009,.F.);
#58155=ORIENTED_EDGE('',*,*,#41010,.F.);
#58156=ORIENTED_EDGE('',*,*,#41005,.F.);
#58157=ORIENTED_EDGE('',*,*,#41010,.T.);
#58158=ORIENTED_EDGE('',*,*,#41011,.F.);
#58159=ORIENTED_EDGE('',*,*,#40733,.T.);
#58160=ORIENTED_EDGE('',*,*,#41006,.T.);
#58161=ORIENTED_EDGE('',*,*,#41012,.T.);
#58162=ORIENTED_EDGE('',*,*,#41013,.F.);
#58163=ORIENTED_EDGE('',*,*,#40735,.T.);
#58164=ORIENTED_EDGE('',*,*,#41014,.F.);
#58165=ORIENTED_EDGE('',*,*,#41015,.F.);
#58166=ORIENTED_EDGE('',*,*,#41016,.F.);
#58167=ORIENTED_EDGE('',*,*,#41017,.F.);
#58168=ORIENTED_EDGE('',*,*,#41012,.F.);
#58169=ORIENTED_EDGE('',*,*,#41017,.T.);
#58170=ORIENTED_EDGE('',*,*,#41018,.F.);
#58171=ORIENTED_EDGE('',*,*,#40736,.T.);
#58172=ORIENTED_EDGE('',*,*,#41013,.T.);
#58173=ORIENTED_EDGE('',*,*,#41019,.T.);
#58174=ORIENTED_EDGE('',*,*,#41020,.F.);
#58175=ORIENTED_EDGE('',*,*,#40738,.T.);
#58176=ORIENTED_EDGE('',*,*,#41021,.F.);
#58177=ORIENTED_EDGE('',*,*,#41022,.F.);
#58178=ORIENTED_EDGE('',*,*,#41023,.F.);
#58179=ORIENTED_EDGE('',*,*,#41024,.F.);
#58180=ORIENTED_EDGE('',*,*,#41019,.F.);
#58181=ORIENTED_EDGE('',*,*,#41024,.T.);
#58182=ORIENTED_EDGE('',*,*,#41025,.F.);
#58183=ORIENTED_EDGE('',*,*,#40739,.T.);
#58184=ORIENTED_EDGE('',*,*,#41020,.T.);
#58185=ORIENTED_EDGE('',*,*,#40741,.T.);
#58186=ORIENTED_EDGE('',*,*,#41026,.F.);
#58187=ORIENTED_EDGE('',*,*,#41027,.T.);
#58188=ORIENTED_EDGE('',*,*,#41028,.F.);
#58189=ORIENTED_EDGE('',*,*,#40742,.T.);
#58190=ORIENTED_EDGE('',*,*,#41028,.T.);
#58191=ORIENTED_EDGE('',*,*,#41029,.T.);
#58192=ORIENTED_EDGE('',*,*,#41030,.F.);
#58193=ORIENTED_EDGE('',*,*,#41029,.F.);
#58194=ORIENTED_EDGE('',*,*,#41027,.F.);
#58195=ORIENTED_EDGE('',*,*,#41031,.F.);
#58196=ORIENTED_EDGE('',*,*,#41032,.F.);
#58197=ORIENTED_EDGE('',*,*,#40744,.T.);
#58198=ORIENTED_EDGE('',*,*,#41033,.F.);
#58199=ORIENTED_EDGE('',*,*,#41034,.T.);
#58200=ORIENTED_EDGE('',*,*,#41035,.F.);
#58201=ORIENTED_EDGE('',*,*,#40745,.T.);
#58202=ORIENTED_EDGE('',*,*,#41035,.T.);
#58203=ORIENTED_EDGE('',*,*,#41036,.T.);
#58204=ORIENTED_EDGE('',*,*,#41037,.F.);
#58205=ORIENTED_EDGE('',*,*,#41036,.F.);
#58206=ORIENTED_EDGE('',*,*,#41034,.F.);
#58207=ORIENTED_EDGE('',*,*,#41038,.F.);
#58208=ORIENTED_EDGE('',*,*,#41039,.F.);
#58209=ORIENTED_EDGE('',*,*,#40747,.T.);
#58210=ORIENTED_EDGE('',*,*,#41040,.F.);
#58211=ORIENTED_EDGE('',*,*,#41041,.T.);
#58212=ORIENTED_EDGE('',*,*,#41042,.F.);
#58213=ORIENTED_EDGE('',*,*,#40748,.T.);
#58214=ORIENTED_EDGE('',*,*,#41042,.T.);
#58215=ORIENTED_EDGE('',*,*,#41043,.T.);
#58216=ORIENTED_EDGE('',*,*,#41044,.F.);
#58217=ORIENTED_EDGE('',*,*,#41043,.F.);
#58218=ORIENTED_EDGE('',*,*,#41041,.F.);
#58219=ORIENTED_EDGE('',*,*,#41045,.F.);
#58220=ORIENTED_EDGE('',*,*,#41046,.F.);
#58221=ORIENTED_EDGE('',*,*,#40750,.T.);
#58222=ORIENTED_EDGE('',*,*,#41047,.F.);
#58223=ORIENTED_EDGE('',*,*,#41048,.T.);
#58224=ORIENTED_EDGE('',*,*,#41049,.F.);
#58225=ORIENTED_EDGE('',*,*,#40751,.T.);
#58226=ORIENTED_EDGE('',*,*,#41049,.T.);
#58227=ORIENTED_EDGE('',*,*,#41050,.T.);
#58228=ORIENTED_EDGE('',*,*,#41051,.F.);
#58229=ORIENTED_EDGE('',*,*,#41050,.F.);
#58230=ORIENTED_EDGE('',*,*,#41048,.F.);
#58231=ORIENTED_EDGE('',*,*,#41052,.F.);
#58232=ORIENTED_EDGE('',*,*,#41053,.F.);
#58233=ORIENTED_EDGE('',*,*,#40753,.T.);
#58234=ORIENTED_EDGE('',*,*,#41054,.F.);
#58235=ORIENTED_EDGE('',*,*,#41055,.T.);
#58236=ORIENTED_EDGE('',*,*,#41056,.F.);
#58237=ORIENTED_EDGE('',*,*,#40754,.T.);
#58238=ORIENTED_EDGE('',*,*,#41056,.T.);
#58239=ORIENTED_EDGE('',*,*,#41057,.T.);
#58240=ORIENTED_EDGE('',*,*,#41058,.F.);
#58241=ORIENTED_EDGE('',*,*,#41057,.F.);
#58242=ORIENTED_EDGE('',*,*,#41055,.F.);
#58243=ORIENTED_EDGE('',*,*,#41059,.F.);
#58244=ORIENTED_EDGE('',*,*,#41060,.F.);
#58245=ORIENTED_EDGE('',*,*,#40756,.T.);
#58246=ORIENTED_EDGE('',*,*,#41061,.F.);
#58247=ORIENTED_EDGE('',*,*,#41062,.T.);
#58248=ORIENTED_EDGE('',*,*,#41063,.F.);
#58249=ORIENTED_EDGE('',*,*,#40757,.T.);
#58250=ORIENTED_EDGE('',*,*,#41063,.T.);
#58251=ORIENTED_EDGE('',*,*,#41064,.T.);
#58252=ORIENTED_EDGE('',*,*,#41065,.F.);
#58253=ORIENTED_EDGE('',*,*,#41064,.F.);
#58254=ORIENTED_EDGE('',*,*,#41062,.F.);
#58255=ORIENTED_EDGE('',*,*,#41066,.F.);
#58256=ORIENTED_EDGE('',*,*,#41067,.F.);
#58257=ORIENTED_EDGE('',*,*,#40759,.T.);
#58258=ORIENTED_EDGE('',*,*,#41068,.F.);
#58259=ORIENTED_EDGE('',*,*,#41069,.T.);
#58260=ORIENTED_EDGE('',*,*,#41070,.F.);
#58261=ORIENTED_EDGE('',*,*,#40760,.T.);
#58262=ORIENTED_EDGE('',*,*,#41070,.T.);
#58263=ORIENTED_EDGE('',*,*,#41071,.T.);
#58264=ORIENTED_EDGE('',*,*,#41072,.F.);
#58265=ORIENTED_EDGE('',*,*,#41071,.F.);
#58266=ORIENTED_EDGE('',*,*,#41069,.F.);
#58267=ORIENTED_EDGE('',*,*,#41073,.F.);
#58268=ORIENTED_EDGE('',*,*,#41074,.F.);
#58269=ORIENTED_EDGE('',*,*,#40762,.T.);
#58270=ORIENTED_EDGE('',*,*,#41075,.F.);
#58271=ORIENTED_EDGE('',*,*,#41076,.T.);
#58272=ORIENTED_EDGE('',*,*,#41077,.F.);
#58273=ORIENTED_EDGE('',*,*,#40763,.T.);
#58274=ORIENTED_EDGE('',*,*,#41077,.T.);
#58275=ORIENTED_EDGE('',*,*,#41078,.T.);
#58276=ORIENTED_EDGE('',*,*,#41079,.F.);
#58277=ORIENTED_EDGE('',*,*,#41078,.F.);
#58278=ORIENTED_EDGE('',*,*,#41076,.F.);
#58279=ORIENTED_EDGE('',*,*,#41080,.F.);
#58280=ORIENTED_EDGE('',*,*,#41081,.F.);
#58281=ORIENTED_EDGE('',*,*,#40765,.T.);
#58282=ORIENTED_EDGE('',*,*,#41082,.F.);
#58283=ORIENTED_EDGE('',*,*,#41083,.T.);
#58284=ORIENTED_EDGE('',*,*,#41084,.F.);
#58285=ORIENTED_EDGE('',*,*,#40766,.T.);
#58286=ORIENTED_EDGE('',*,*,#41084,.T.);
#58287=ORIENTED_EDGE('',*,*,#41085,.T.);
#58288=ORIENTED_EDGE('',*,*,#41086,.F.);
#58289=ORIENTED_EDGE('',*,*,#41085,.F.);
#58290=ORIENTED_EDGE('',*,*,#41083,.F.);
#58291=ORIENTED_EDGE('',*,*,#41087,.F.);
#58292=ORIENTED_EDGE('',*,*,#41088,.F.);
#58293=ORIENTED_EDGE('',*,*,#40768,.T.);
#58294=ORIENTED_EDGE('',*,*,#41089,.F.);
#58295=ORIENTED_EDGE('',*,*,#41090,.T.);
#58296=ORIENTED_EDGE('',*,*,#41091,.F.);
#58297=ORIENTED_EDGE('',*,*,#40769,.T.);
#58298=ORIENTED_EDGE('',*,*,#41091,.T.);
#58299=ORIENTED_EDGE('',*,*,#41092,.T.);
#58300=ORIENTED_EDGE('',*,*,#41093,.F.);
#58301=ORIENTED_EDGE('',*,*,#41092,.F.);
#58302=ORIENTED_EDGE('',*,*,#41090,.F.);
#58303=ORIENTED_EDGE('',*,*,#41094,.F.);
#58304=ORIENTED_EDGE('',*,*,#41095,.F.);
#58305=ORIENTED_EDGE('',*,*,#40771,.T.);
#58306=ORIENTED_EDGE('',*,*,#41096,.F.);
#58307=ORIENTED_EDGE('',*,*,#41097,.T.);
#58308=ORIENTED_EDGE('',*,*,#41098,.F.);
#58309=ORIENTED_EDGE('',*,*,#40772,.T.);
#58310=ORIENTED_EDGE('',*,*,#41098,.T.);
#58311=ORIENTED_EDGE('',*,*,#41099,.T.);
#58312=ORIENTED_EDGE('',*,*,#41100,.F.);
#58313=ORIENTED_EDGE('',*,*,#41099,.F.);
#58314=ORIENTED_EDGE('',*,*,#41097,.F.);
#58315=ORIENTED_EDGE('',*,*,#41101,.F.);
#58316=ORIENTED_EDGE('',*,*,#41102,.F.);
#58317=ORIENTED_EDGE('',*,*,#40774,.T.);
#58318=ORIENTED_EDGE('',*,*,#41103,.F.);
#58319=ORIENTED_EDGE('',*,*,#41104,.T.);
#58320=ORIENTED_EDGE('',*,*,#41105,.F.);
#58321=ORIENTED_EDGE('',*,*,#40775,.T.);
#58322=ORIENTED_EDGE('',*,*,#41105,.T.);
#58323=ORIENTED_EDGE('',*,*,#41106,.T.);
#58324=ORIENTED_EDGE('',*,*,#41107,.F.);
#58325=ORIENTED_EDGE('',*,*,#41106,.F.);
#58326=ORIENTED_EDGE('',*,*,#41104,.F.);
#58327=ORIENTED_EDGE('',*,*,#41108,.F.);
#58328=ORIENTED_EDGE('',*,*,#41109,.F.);
#58329=ORIENTED_EDGE('',*,*,#40777,.T.);
#58330=ORIENTED_EDGE('',*,*,#41110,.F.);
#58331=ORIENTED_EDGE('',*,*,#41111,.T.);
#58332=ORIENTED_EDGE('',*,*,#41112,.F.);
#58333=ORIENTED_EDGE('',*,*,#40778,.T.);
#58334=ORIENTED_EDGE('',*,*,#41112,.T.);
#58335=ORIENTED_EDGE('',*,*,#41113,.T.);
#58336=ORIENTED_EDGE('',*,*,#41114,.F.);
#58337=ORIENTED_EDGE('',*,*,#41113,.F.);
#58338=ORIENTED_EDGE('',*,*,#41111,.F.);
#58339=ORIENTED_EDGE('',*,*,#41115,.F.);
#58340=ORIENTED_EDGE('',*,*,#41116,.F.);
#58341=ORIENTED_EDGE('',*,*,#40780,.T.);
#58342=ORIENTED_EDGE('',*,*,#41117,.F.);
#58343=ORIENTED_EDGE('',*,*,#41118,.T.);
#58344=ORIENTED_EDGE('',*,*,#41119,.F.);
#58345=ORIENTED_EDGE('',*,*,#40781,.T.);
#58346=ORIENTED_EDGE('',*,*,#41119,.T.);
#58347=ORIENTED_EDGE('',*,*,#41120,.T.);
#58348=ORIENTED_EDGE('',*,*,#41121,.F.);
#58349=ORIENTED_EDGE('',*,*,#41120,.F.);
#58350=ORIENTED_EDGE('',*,*,#41118,.F.);
#58351=ORIENTED_EDGE('',*,*,#41122,.F.);
#58352=ORIENTED_EDGE('',*,*,#41123,.F.);
#58353=ORIENTED_EDGE('',*,*,#40783,.T.);
#58354=ORIENTED_EDGE('',*,*,#41124,.F.);
#58355=ORIENTED_EDGE('',*,*,#41125,.T.);
#58356=ORIENTED_EDGE('',*,*,#41126,.F.);
#58357=ORIENTED_EDGE('',*,*,#40784,.T.);
#58358=ORIENTED_EDGE('',*,*,#41126,.T.);
#58359=ORIENTED_EDGE('',*,*,#41127,.T.);
#58360=ORIENTED_EDGE('',*,*,#41128,.F.);
#58361=ORIENTED_EDGE('',*,*,#41127,.F.);
#58362=ORIENTED_EDGE('',*,*,#41125,.F.);
#58363=ORIENTED_EDGE('',*,*,#41129,.F.);
#58364=ORIENTED_EDGE('',*,*,#41130,.F.);
#58365=ORIENTED_EDGE('',*,*,#40786,.T.);
#58366=ORIENTED_EDGE('',*,*,#41131,.F.);
#58367=ORIENTED_EDGE('',*,*,#41132,.T.);
#58368=ORIENTED_EDGE('',*,*,#41133,.F.);
#58369=ORIENTED_EDGE('',*,*,#40787,.T.);
#58370=ORIENTED_EDGE('',*,*,#41133,.T.);
#58371=ORIENTED_EDGE('',*,*,#41134,.T.);
#58372=ORIENTED_EDGE('',*,*,#41135,.F.);
#58373=ORIENTED_EDGE('',*,*,#41134,.F.);
#58374=ORIENTED_EDGE('',*,*,#41132,.F.);
#58375=ORIENTED_EDGE('',*,*,#41136,.F.);
#58376=ORIENTED_EDGE('',*,*,#41137,.F.);
#58377=ORIENTED_EDGE('',*,*,#40789,.T.);
#58378=ORIENTED_EDGE('',*,*,#41138,.F.);
#58379=ORIENTED_EDGE('',*,*,#41139,.T.);
#58380=ORIENTED_EDGE('',*,*,#41140,.F.);
#58381=ORIENTED_EDGE('',*,*,#40790,.T.);
#58382=ORIENTED_EDGE('',*,*,#41140,.T.);
#58383=ORIENTED_EDGE('',*,*,#41141,.T.);
#58384=ORIENTED_EDGE('',*,*,#41142,.F.);
#58385=ORIENTED_EDGE('',*,*,#41141,.F.);
#58386=ORIENTED_EDGE('',*,*,#41139,.F.);
#58387=ORIENTED_EDGE('',*,*,#41143,.F.);
#58388=ORIENTED_EDGE('',*,*,#41144,.F.);
#58389=ORIENTED_EDGE('',*,*,#40792,.T.);
#58390=ORIENTED_EDGE('',*,*,#41145,.F.);
#58391=ORIENTED_EDGE('',*,*,#41146,.T.);
#58392=ORIENTED_EDGE('',*,*,#41147,.F.);
#58393=ORIENTED_EDGE('',*,*,#40793,.T.);
#58394=ORIENTED_EDGE('',*,*,#41147,.T.);
#58395=ORIENTED_EDGE('',*,*,#41148,.T.);
#58396=ORIENTED_EDGE('',*,*,#41149,.F.);
#58397=ORIENTED_EDGE('',*,*,#41148,.F.);
#58398=ORIENTED_EDGE('',*,*,#41146,.F.);
#58399=ORIENTED_EDGE('',*,*,#41150,.F.);
#58400=ORIENTED_EDGE('',*,*,#41151,.F.);
#58401=ORIENTED_EDGE('',*,*,#40795,.T.);
#58402=ORIENTED_EDGE('',*,*,#41152,.F.);
#58403=ORIENTED_EDGE('',*,*,#41153,.T.);
#58404=ORIENTED_EDGE('',*,*,#41154,.F.);
#58405=ORIENTED_EDGE('',*,*,#40796,.T.);
#58406=ORIENTED_EDGE('',*,*,#41154,.T.);
#58407=ORIENTED_EDGE('',*,*,#41155,.T.);
#58408=ORIENTED_EDGE('',*,*,#41156,.F.);
#58409=ORIENTED_EDGE('',*,*,#41155,.F.);
#58410=ORIENTED_EDGE('',*,*,#41153,.F.);
#58411=ORIENTED_EDGE('',*,*,#41157,.F.);
#58412=ORIENTED_EDGE('',*,*,#41158,.F.);
#58413=ORIENTED_EDGE('',*,*,#40798,.T.);
#58414=ORIENTED_EDGE('',*,*,#41159,.F.);
#58415=ORIENTED_EDGE('',*,*,#41160,.T.);
#58416=ORIENTED_EDGE('',*,*,#41161,.F.);
#58417=ORIENTED_EDGE('',*,*,#40799,.T.);
#58418=ORIENTED_EDGE('',*,*,#41161,.T.);
#58419=ORIENTED_EDGE('',*,*,#41162,.T.);
#58420=ORIENTED_EDGE('',*,*,#41163,.F.);
#58421=ORIENTED_EDGE('',*,*,#41162,.F.);
#58422=ORIENTED_EDGE('',*,*,#41160,.F.);
#58423=ORIENTED_EDGE('',*,*,#41164,.F.);
#58424=ORIENTED_EDGE('',*,*,#41165,.F.);
#58425=ORIENTED_EDGE('',*,*,#40801,.T.);
#58426=ORIENTED_EDGE('',*,*,#41166,.F.);
#58427=ORIENTED_EDGE('',*,*,#41167,.T.);
#58428=ORIENTED_EDGE('',*,*,#41168,.F.);
#58429=ORIENTED_EDGE('',*,*,#40802,.T.);
#58430=ORIENTED_EDGE('',*,*,#41168,.T.);
#58431=ORIENTED_EDGE('',*,*,#41169,.T.);
#58432=ORIENTED_EDGE('',*,*,#41170,.F.);
#58433=ORIENTED_EDGE('',*,*,#41169,.F.);
#58434=ORIENTED_EDGE('',*,*,#41167,.F.);
#58435=ORIENTED_EDGE('',*,*,#41171,.F.);
#58436=ORIENTED_EDGE('',*,*,#41172,.F.);
#58437=ORIENTED_EDGE('',*,*,#40804,.T.);
#58438=ORIENTED_EDGE('',*,*,#41173,.F.);
#58439=ORIENTED_EDGE('',*,*,#34384,.T.);
#58440=ORIENTED_EDGE('',*,*,#41174,.F.);
#58441=ORIENTED_EDGE('',*,*,#40805,.T.);
#58442=ORIENTED_EDGE('',*,*,#41174,.T.);
#58443=ORIENTED_EDGE('',*,*,#34383,.T.);
#58444=ORIENTED_EDGE('',*,*,#41175,.F.);
#58445=ORIENTED_EDGE('',*,*,#40807,.T.);
#58446=ORIENTED_EDGE('',*,*,#41176,.F.);
#58447=ORIENTED_EDGE('',*,*,#41177,.T.);
#58448=ORIENTED_EDGE('',*,*,#41178,.F.);
#58449=ORIENTED_EDGE('',*,*,#40808,.T.);
#58450=ORIENTED_EDGE('',*,*,#41178,.T.);
#58451=ORIENTED_EDGE('',*,*,#41179,.T.);
#58452=ORIENTED_EDGE('',*,*,#41180,.F.);
#58453=ORIENTED_EDGE('',*,*,#41179,.F.);
#58454=ORIENTED_EDGE('',*,*,#41177,.F.);
#58455=ORIENTED_EDGE('',*,*,#41181,.F.);
#58456=ORIENTED_EDGE('',*,*,#41182,.F.);
#58457=ORIENTED_EDGE('',*,*,#40810,.T.);
#58458=ORIENTED_EDGE('',*,*,#41183,.F.);
#58459=ORIENTED_EDGE('',*,*,#41184,.T.);
#58460=ORIENTED_EDGE('',*,*,#41185,.F.);
#58461=ORIENTED_EDGE('',*,*,#40811,.T.);
#58462=ORIENTED_EDGE('',*,*,#41185,.T.);
#58463=ORIENTED_EDGE('',*,*,#41186,.T.);
#58464=ORIENTED_EDGE('',*,*,#41187,.F.);
#58465=ORIENTED_EDGE('',*,*,#41186,.F.);
#58466=ORIENTED_EDGE('',*,*,#41184,.F.);
#58467=ORIENTED_EDGE('',*,*,#41188,.F.);
#58468=ORIENTED_EDGE('',*,*,#41189,.F.);
#58469=ORIENTED_EDGE('',*,*,#40813,.T.);
#58470=ORIENTED_EDGE('',*,*,#41190,.F.);
#58471=ORIENTED_EDGE('',*,*,#41191,.T.);
#58472=ORIENTED_EDGE('',*,*,#41192,.F.);
#58473=ORIENTED_EDGE('',*,*,#40814,.T.);
#58474=ORIENTED_EDGE('',*,*,#41192,.T.);
#58475=ORIENTED_EDGE('',*,*,#41193,.T.);
#58476=ORIENTED_EDGE('',*,*,#41194,.F.);
#58477=ORIENTED_EDGE('',*,*,#41193,.F.);
#58478=ORIENTED_EDGE('',*,*,#41191,.F.);
#58479=ORIENTED_EDGE('',*,*,#41195,.F.);
#58480=ORIENTED_EDGE('',*,*,#41196,.F.);
#58481=ORIENTED_EDGE('',*,*,#40816,.T.);
#58482=ORIENTED_EDGE('',*,*,#41197,.F.);
#58483=ORIENTED_EDGE('',*,*,#41198,.T.);
#58484=ORIENTED_EDGE('',*,*,#41199,.F.);
#58485=ORIENTED_EDGE('',*,*,#41200,.T.);
#58486=ORIENTED_EDGE('',*,*,#41201,.F.);
#58487=ORIENTED_EDGE('',*,*,#40817,.T.);
#58488=ORIENTED_EDGE('',*,*,#41199,.T.);
#58489=ORIENTED_EDGE('',*,*,#41202,.F.);
#58490=ORIENTED_EDGE('',*,*,#41203,.F.);
#58491=ORIENTED_EDGE('',*,*,#41200,.F.);
#58492=ORIENTED_EDGE('',*,*,#41198,.F.);
#58493=ORIENTED_EDGE('',*,*,#40819,.T.);
#58494=ORIENTED_EDGE('',*,*,#41204,.F.);
#58495=ORIENTED_EDGE('',*,*,#41205,.T.);
#58496=ORIENTED_EDGE('',*,*,#41206,.F.);
#58497=ORIENTED_EDGE('',*,*,#40820,.T.);
#58498=ORIENTED_EDGE('',*,*,#41206,.T.);
#58499=ORIENTED_EDGE('',*,*,#41207,.T.);
#58500=ORIENTED_EDGE('',*,*,#41208,.F.);
#58501=ORIENTED_EDGE('',*,*,#41207,.F.);
#58502=ORIENTED_EDGE('',*,*,#41205,.F.);
#58503=ORIENTED_EDGE('',*,*,#41209,.F.);
#58504=ORIENTED_EDGE('',*,*,#41210,.F.);
#58505=ORIENTED_EDGE('',*,*,#40822,.T.);
#58506=ORIENTED_EDGE('',*,*,#41211,.F.);
#58507=ORIENTED_EDGE('',*,*,#41212,.T.);
#58508=ORIENTED_EDGE('',*,*,#41213,.F.);
#58509=ORIENTED_EDGE('',*,*,#40823,.T.);
#58510=ORIENTED_EDGE('',*,*,#41213,.T.);
#58511=ORIENTED_EDGE('',*,*,#41214,.T.);
#58512=ORIENTED_EDGE('',*,*,#41215,.F.);
#58513=ORIENTED_EDGE('',*,*,#41214,.F.);
#58514=ORIENTED_EDGE('',*,*,#41212,.F.);
#58515=ORIENTED_EDGE('',*,*,#41216,.F.);
#58516=ORIENTED_EDGE('',*,*,#41217,.F.);
#58517=ORIENTED_EDGE('',*,*,#40825,.T.);
#58518=ORIENTED_EDGE('',*,*,#41218,.F.);
#58519=ORIENTED_EDGE('',*,*,#41219,.T.);
#58520=ORIENTED_EDGE('',*,*,#41220,.F.);
#58521=ORIENTED_EDGE('',*,*,#40826,.T.);
#58522=ORIENTED_EDGE('',*,*,#41220,.T.);
#58523=ORIENTED_EDGE('',*,*,#41221,.T.);
#58524=ORIENTED_EDGE('',*,*,#41222,.F.);
#58525=ORIENTED_EDGE('',*,*,#41221,.F.);
#58526=ORIENTED_EDGE('',*,*,#41219,.F.);
#58527=ORIENTED_EDGE('',*,*,#41223,.F.);
#58528=ORIENTED_EDGE('',*,*,#41224,.F.);
#58529=ORIENTED_EDGE('',*,*,#41225,.F.);
#58530=ORIENTED_EDGE('',*,*,#41226,.F.);
#58531=ORIENTED_EDGE('',*,*,#40830,.T.);
#58532=ORIENTED_EDGE('',*,*,#40829,.T.);
#58533=ORIENTED_EDGE('',*,*,#41227,.F.);
#58534=ORIENTED_EDGE('',*,*,#40833,.T.);
#58535=ORIENTED_EDGE('',*,*,#40831,.T.);
#58536=ORIENTED_EDGE('',*,*,#41226,.T.);
#58537=ORIENTED_EDGE('',*,*,#41228,.F.);
#58538=ORIENTED_EDGE('',*,*,#41229,.F.);
#58539=ORIENTED_EDGE('',*,*,#40837,.T.);
#58540=ORIENTED_EDGE('',*,*,#40836,.T.);
#58541=ORIENTED_EDGE('',*,*,#41230,.F.);
#58542=ORIENTED_EDGE('',*,*,#40840,.T.);
#58543=ORIENTED_EDGE('',*,*,#40838,.T.);
#58544=ORIENTED_EDGE('',*,*,#41229,.T.);
#58545=ORIENTED_EDGE('',*,*,#41231,.F.);
#58546=ORIENTED_EDGE('',*,*,#41232,.F.);
#58547=ORIENTED_EDGE('',*,*,#40844,.T.);
#58548=ORIENTED_EDGE('',*,*,#40843,.T.);
#58549=ORIENTED_EDGE('',*,*,#41233,.F.);
#58550=ORIENTED_EDGE('',*,*,#40847,.T.);
#58551=ORIENTED_EDGE('',*,*,#40845,.T.);
#58552=ORIENTED_EDGE('',*,*,#41232,.T.);
#58553=ORIENTED_EDGE('',*,*,#41234,.F.);
#58554=ORIENTED_EDGE('',*,*,#41235,.F.);
#58555=ORIENTED_EDGE('',*,*,#40851,.T.);
#58556=ORIENTED_EDGE('',*,*,#40850,.T.);
#58557=ORIENTED_EDGE('',*,*,#41236,.F.);
#58558=ORIENTED_EDGE('',*,*,#40854,.T.);
#58559=ORIENTED_EDGE('',*,*,#40852,.T.);
#58560=ORIENTED_EDGE('',*,*,#41235,.T.);
#58561=ORIENTED_EDGE('',*,*,#41237,.F.);
#58562=ORIENTED_EDGE('',*,*,#41238,.F.);
#58563=ORIENTED_EDGE('',*,*,#40858,.T.);
#58564=ORIENTED_EDGE('',*,*,#40857,.T.);
#58565=ORIENTED_EDGE('',*,*,#41239,.F.);
#58566=ORIENTED_EDGE('',*,*,#40861,.T.);
#58567=ORIENTED_EDGE('',*,*,#40859,.T.);
#58568=ORIENTED_EDGE('',*,*,#41238,.T.);
#58569=ORIENTED_EDGE('',*,*,#41240,.F.);
#58570=ORIENTED_EDGE('',*,*,#41241,.F.);
#58571=ORIENTED_EDGE('',*,*,#40865,.T.);
#58572=ORIENTED_EDGE('',*,*,#40864,.T.);
#58573=ORIENTED_EDGE('',*,*,#41242,.F.);
#58574=ORIENTED_EDGE('',*,*,#40868,.T.);
#58575=ORIENTED_EDGE('',*,*,#40866,.T.);
#58576=ORIENTED_EDGE('',*,*,#41241,.T.);
#58577=ORIENTED_EDGE('',*,*,#41243,.F.);
#58578=ORIENTED_EDGE('',*,*,#41244,.F.);
#58579=ORIENTED_EDGE('',*,*,#40872,.T.);
#58580=ORIENTED_EDGE('',*,*,#40871,.T.);
#58581=ORIENTED_EDGE('',*,*,#41245,.F.);
#58582=ORIENTED_EDGE('',*,*,#40875,.T.);
#58583=ORIENTED_EDGE('',*,*,#40873,.T.);
#58584=ORIENTED_EDGE('',*,*,#41244,.T.);
#58585=ORIENTED_EDGE('',*,*,#41246,.F.);
#58586=ORIENTED_EDGE('',*,*,#41247,.F.);
#58587=ORIENTED_EDGE('',*,*,#40879,.T.);
#58588=ORIENTED_EDGE('',*,*,#40878,.T.);
#58589=ORIENTED_EDGE('',*,*,#41248,.F.);
#58590=ORIENTED_EDGE('',*,*,#40882,.T.);
#58591=ORIENTED_EDGE('',*,*,#40880,.T.);
#58592=ORIENTED_EDGE('',*,*,#41247,.T.);
#58593=ORIENTED_EDGE('',*,*,#41249,.F.);
#58594=ORIENTED_EDGE('',*,*,#41250,.F.);
#58595=ORIENTED_EDGE('',*,*,#40886,.T.);
#58596=ORIENTED_EDGE('',*,*,#40885,.T.);
#58597=ORIENTED_EDGE('',*,*,#41251,.F.);
#58598=ORIENTED_EDGE('',*,*,#40889,.T.);
#58599=ORIENTED_EDGE('',*,*,#40887,.T.);
#58600=ORIENTED_EDGE('',*,*,#41250,.T.);
#58601=ORIENTED_EDGE('',*,*,#41252,.F.);
#58602=ORIENTED_EDGE('',*,*,#41253,.F.);
#58603=ORIENTED_EDGE('',*,*,#40893,.T.);
#58604=ORIENTED_EDGE('',*,*,#40892,.T.);
#58605=ORIENTED_EDGE('',*,*,#41254,.F.);
#58606=ORIENTED_EDGE('',*,*,#40896,.T.);
#58607=ORIENTED_EDGE('',*,*,#40894,.T.);
#58608=ORIENTED_EDGE('',*,*,#41253,.T.);
#58609=ORIENTED_EDGE('',*,*,#41255,.F.);
#58610=ORIENTED_EDGE('',*,*,#41256,.F.);
#58611=ORIENTED_EDGE('',*,*,#40900,.T.);
#58612=ORIENTED_EDGE('',*,*,#40899,.T.);
#58613=ORIENTED_EDGE('',*,*,#41257,.F.);
#58614=ORIENTED_EDGE('',*,*,#40903,.T.);
#58615=ORIENTED_EDGE('',*,*,#40901,.T.);
#58616=ORIENTED_EDGE('',*,*,#41256,.T.);
#58617=ORIENTED_EDGE('',*,*,#41258,.F.);
#58618=ORIENTED_EDGE('',*,*,#41259,.F.);
#58619=ORIENTED_EDGE('',*,*,#40907,.T.);
#58620=ORIENTED_EDGE('',*,*,#40906,.T.);
#58621=ORIENTED_EDGE('',*,*,#41260,.F.);
#58622=ORIENTED_EDGE('',*,*,#40910,.T.);
#58623=ORIENTED_EDGE('',*,*,#40908,.T.);
#58624=ORIENTED_EDGE('',*,*,#41259,.T.);
#58625=ORIENTED_EDGE('',*,*,#41261,.F.);
#58626=ORIENTED_EDGE('',*,*,#41262,.F.);
#58627=ORIENTED_EDGE('',*,*,#40914,.T.);
#58628=ORIENTED_EDGE('',*,*,#40913,.T.);
#58629=ORIENTED_EDGE('',*,*,#41263,.F.);
#58630=ORIENTED_EDGE('',*,*,#40917,.T.);
#58631=ORIENTED_EDGE('',*,*,#40915,.T.);
#58632=ORIENTED_EDGE('',*,*,#41262,.T.);
#58633=ORIENTED_EDGE('',*,*,#41264,.F.);
#58634=ORIENTED_EDGE('',*,*,#41265,.F.);
#58635=ORIENTED_EDGE('',*,*,#40921,.T.);
#58636=ORIENTED_EDGE('',*,*,#40920,.T.);
#58637=ORIENTED_EDGE('',*,*,#41266,.F.);
#58638=ORIENTED_EDGE('',*,*,#40924,.T.);
#58639=ORIENTED_EDGE('',*,*,#40922,.T.);
#58640=ORIENTED_EDGE('',*,*,#41265,.T.);
#58641=ORIENTED_EDGE('',*,*,#41267,.F.);
#58642=ORIENTED_EDGE('',*,*,#41268,.F.);
#58643=ORIENTED_EDGE('',*,*,#34386,.T.);
#58644=ORIENTED_EDGE('',*,*,#40926,.T.);
#58645=ORIENTED_EDGE('',*,*,#41269,.F.);
#58646=ORIENTED_EDGE('',*,*,#40927,.T.);
#58647=ORIENTED_EDGE('',*,*,#34387,.T.);
#58648=ORIENTED_EDGE('',*,*,#41268,.T.);
#58649=ORIENTED_EDGE('',*,*,#41270,.F.);
#58650=ORIENTED_EDGE('',*,*,#41271,.F.);
#58651=ORIENTED_EDGE('',*,*,#40931,.T.);
#58652=ORIENTED_EDGE('',*,*,#40930,.T.);
#58653=ORIENTED_EDGE('',*,*,#41272,.F.);
#58654=ORIENTED_EDGE('',*,*,#40934,.T.);
#58655=ORIENTED_EDGE('',*,*,#40932,.T.);
#58656=ORIENTED_EDGE('',*,*,#41271,.T.);
#58657=ORIENTED_EDGE('',*,*,#41273,.F.);
#58658=ORIENTED_EDGE('',*,*,#41274,.F.);
#58659=ORIENTED_EDGE('',*,*,#40938,.T.);
#58660=ORIENTED_EDGE('',*,*,#40937,.T.);
#58661=ORIENTED_EDGE('',*,*,#41275,.F.);
#58662=ORIENTED_EDGE('',*,*,#40941,.T.);
#58663=ORIENTED_EDGE('',*,*,#40939,.T.);
#58664=ORIENTED_EDGE('',*,*,#41274,.T.);
#58665=ORIENTED_EDGE('',*,*,#41276,.F.);
#58666=ORIENTED_EDGE('',*,*,#41277,.F.);
#58667=ORIENTED_EDGE('',*,*,#40945,.T.);
#58668=ORIENTED_EDGE('',*,*,#40944,.T.);
#58669=ORIENTED_EDGE('',*,*,#41278,.F.);
#58670=ORIENTED_EDGE('',*,*,#40948,.T.);
#58671=ORIENTED_EDGE('',*,*,#40946,.T.);
#58672=ORIENTED_EDGE('',*,*,#41277,.T.);
#58673=ORIENTED_EDGE('',*,*,#41279,.F.);
#58674=ORIENTED_EDGE('',*,*,#41280,.F.);
#58675=ORIENTED_EDGE('',*,*,#40952,.T.);
#58676=ORIENTED_EDGE('',*,*,#40951,.T.);
#58677=ORIENTED_EDGE('',*,*,#41281,.F.);
#58678=ORIENTED_EDGE('',*,*,#40955,.T.);
#58679=ORIENTED_EDGE('',*,*,#40953,.T.);
#58680=ORIENTED_EDGE('',*,*,#41280,.T.);
#58681=ORIENTED_EDGE('',*,*,#41282,.F.);
#58682=ORIENTED_EDGE('',*,*,#41283,.F.);
#58683=ORIENTED_EDGE('',*,*,#40961,.T.);
#58684=ORIENTED_EDGE('',*,*,#40958,.T.);
#58685=ORIENTED_EDGE('',*,*,#40962,.T.);
#58686=ORIENTED_EDGE('',*,*,#41283,.T.);
#58687=ORIENTED_EDGE('',*,*,#41284,.F.);
#58688=ORIENTED_EDGE('',*,*,#40960,.T.);
#58689=ORIENTED_EDGE('',*,*,#40967,.T.);
#58690=ORIENTED_EDGE('',*,*,#40963,.T.);
#58691=ORIENTED_EDGE('',*,*,#41285,.F.);
#58692=ORIENTED_EDGE('',*,*,#41286,.F.);
#58693=ORIENTED_EDGE('',*,*,#41287,.F.);
#58694=ORIENTED_EDGE('',*,*,#40969,.T.);
#58695=ORIENTED_EDGE('',*,*,#40968,.T.);
#58696=ORIENTED_EDGE('',*,*,#41286,.T.);
#58697=ORIENTED_EDGE('',*,*,#41288,.F.);
#58698=ORIENTED_EDGE('',*,*,#41289,.F.);
#58699=ORIENTED_EDGE('',*,*,#40973,.T.);
#58700=ORIENTED_EDGE('',*,*,#40972,.T.);
#58701=ORIENTED_EDGE('',*,*,#41290,.F.);
#58702=ORIENTED_EDGE('',*,*,#40976,.T.);
#58703=ORIENTED_EDGE('',*,*,#40974,.T.);
#58704=ORIENTED_EDGE('',*,*,#41289,.T.);
#58705=ORIENTED_EDGE('',*,*,#41291,.F.);
#58706=ORIENTED_EDGE('',*,*,#41292,.F.);
#58707=ORIENTED_EDGE('',*,*,#40980,.T.);
#58708=ORIENTED_EDGE('',*,*,#40979,.T.);
#58709=ORIENTED_EDGE('',*,*,#41293,.F.);
#58710=ORIENTED_EDGE('',*,*,#40983,.T.);
#58711=ORIENTED_EDGE('',*,*,#40981,.T.);
#58712=ORIENTED_EDGE('',*,*,#41292,.T.);
#58713=ORIENTED_EDGE('',*,*,#41294,.F.);
#58714=ORIENTED_EDGE('',*,*,#41295,.F.);
#58715=ORIENTED_EDGE('',*,*,#40987,.T.);
#58716=ORIENTED_EDGE('',*,*,#40986,.T.);
#58717=ORIENTED_EDGE('',*,*,#41296,.F.);
#58718=ORIENTED_EDGE('',*,*,#40990,.T.);
#58719=ORIENTED_EDGE('',*,*,#40988,.T.);
#58720=ORIENTED_EDGE('',*,*,#41295,.T.);
#58721=ORIENTED_EDGE('',*,*,#41297,.F.);
#58722=ORIENTED_EDGE('',*,*,#41298,.F.);
#58723=ORIENTED_EDGE('',*,*,#40994,.T.);
#58724=ORIENTED_EDGE('',*,*,#40993,.T.);
#58725=ORIENTED_EDGE('',*,*,#41299,.F.);
#58726=ORIENTED_EDGE('',*,*,#40997,.T.);
#58727=ORIENTED_EDGE('',*,*,#40995,.T.);
#58728=ORIENTED_EDGE('',*,*,#41298,.T.);
#58729=ORIENTED_EDGE('',*,*,#41300,.F.);
#58730=ORIENTED_EDGE('',*,*,#41301,.F.);
#58731=ORIENTED_EDGE('',*,*,#41001,.T.);
#58732=ORIENTED_EDGE('',*,*,#41000,.T.);
#58733=ORIENTED_EDGE('',*,*,#41302,.F.);
#58734=ORIENTED_EDGE('',*,*,#41004,.T.);
#58735=ORIENTED_EDGE('',*,*,#41002,.T.);
#58736=ORIENTED_EDGE('',*,*,#41301,.T.);
#58737=ORIENTED_EDGE('',*,*,#41303,.F.);
#58738=ORIENTED_EDGE('',*,*,#41304,.F.);
#58739=ORIENTED_EDGE('',*,*,#41008,.T.);
#58740=ORIENTED_EDGE('',*,*,#41007,.T.);
#58741=ORIENTED_EDGE('',*,*,#41305,.F.);
#58742=ORIENTED_EDGE('',*,*,#41011,.T.);
#58743=ORIENTED_EDGE('',*,*,#41009,.T.);
#58744=ORIENTED_EDGE('',*,*,#41304,.T.);
#58745=ORIENTED_EDGE('',*,*,#41306,.F.);
#58746=ORIENTED_EDGE('',*,*,#41307,.F.);
#58747=ORIENTED_EDGE('',*,*,#41015,.T.);
#58748=ORIENTED_EDGE('',*,*,#41014,.T.);
#58749=ORIENTED_EDGE('',*,*,#41308,.F.);
#58750=ORIENTED_EDGE('',*,*,#41018,.T.);
#58751=ORIENTED_EDGE('',*,*,#41016,.T.);
#58752=ORIENTED_EDGE('',*,*,#41307,.T.);
#58753=ORIENTED_EDGE('',*,*,#41309,.F.);
#58754=ORIENTED_EDGE('',*,*,#41310,.F.);
#58755=ORIENTED_EDGE('',*,*,#41022,.T.);
#58756=ORIENTED_EDGE('',*,*,#41021,.T.);
#58757=ORIENTED_EDGE('',*,*,#41311,.F.);
#58758=ORIENTED_EDGE('',*,*,#41025,.T.);
#58759=ORIENTED_EDGE('',*,*,#41023,.T.);
#58760=ORIENTED_EDGE('',*,*,#41310,.T.);
#58761=ORIENTED_EDGE('',*,*,#41031,.T.);
#58762=ORIENTED_EDGE('',*,*,#41026,.T.);
#58763=ORIENTED_EDGE('',*,*,#41312,.F.);
#58764=ORIENTED_EDGE('',*,*,#41313,.F.);
#58765=ORIENTED_EDGE('',*,*,#41032,.T.);
#58766=ORIENTED_EDGE('',*,*,#41313,.T.);
#58767=ORIENTED_EDGE('',*,*,#41314,.F.);
#58768=ORIENTED_EDGE('',*,*,#41030,.T.);
#58769=ORIENTED_EDGE('',*,*,#41038,.T.);
#58770=ORIENTED_EDGE('',*,*,#41033,.T.);
#58771=ORIENTED_EDGE('',*,*,#41315,.F.);
#58772=ORIENTED_EDGE('',*,*,#41316,.F.);
#58773=ORIENTED_EDGE('',*,*,#41039,.T.);
#58774=ORIENTED_EDGE('',*,*,#41316,.T.);
#58775=ORIENTED_EDGE('',*,*,#41317,.F.);
#58776=ORIENTED_EDGE('',*,*,#41037,.T.);
#58777=ORIENTED_EDGE('',*,*,#41045,.T.);
#58778=ORIENTED_EDGE('',*,*,#41040,.T.);
#58779=ORIENTED_EDGE('',*,*,#41318,.F.);
#58780=ORIENTED_EDGE('',*,*,#41319,.F.);
#58781=ORIENTED_EDGE('',*,*,#41046,.T.);
#58782=ORIENTED_EDGE('',*,*,#41319,.T.);
#58783=ORIENTED_EDGE('',*,*,#41320,.F.);
#58784=ORIENTED_EDGE('',*,*,#41044,.T.);
#58785=ORIENTED_EDGE('',*,*,#41052,.T.);
#58786=ORIENTED_EDGE('',*,*,#41047,.T.);
#58787=ORIENTED_EDGE('',*,*,#41321,.F.);
#58788=ORIENTED_EDGE('',*,*,#41322,.F.);
#58789=ORIENTED_EDGE('',*,*,#41053,.T.);
#58790=ORIENTED_EDGE('',*,*,#41322,.T.);
#58791=ORIENTED_EDGE('',*,*,#41323,.F.);
#58792=ORIENTED_EDGE('',*,*,#41051,.T.);
#58793=ORIENTED_EDGE('',*,*,#41059,.T.);
#58794=ORIENTED_EDGE('',*,*,#41054,.T.);
#58795=ORIENTED_EDGE('',*,*,#41324,.F.);
#58796=ORIENTED_EDGE('',*,*,#41325,.F.);
#58797=ORIENTED_EDGE('',*,*,#41060,.T.);
#58798=ORIENTED_EDGE('',*,*,#41325,.T.);
#58799=ORIENTED_EDGE('',*,*,#41326,.F.);
#58800=ORIENTED_EDGE('',*,*,#41058,.T.);
#58801=ORIENTED_EDGE('',*,*,#41066,.T.);
#58802=ORIENTED_EDGE('',*,*,#41061,.T.);
#58803=ORIENTED_EDGE('',*,*,#41327,.F.);
#58804=ORIENTED_EDGE('',*,*,#41328,.F.);
#58805=ORIENTED_EDGE('',*,*,#41067,.T.);
#58806=ORIENTED_EDGE('',*,*,#41328,.T.);
#58807=ORIENTED_EDGE('',*,*,#41329,.F.);
#58808=ORIENTED_EDGE('',*,*,#41065,.T.);
#58809=ORIENTED_EDGE('',*,*,#41073,.T.);
#58810=ORIENTED_EDGE('',*,*,#41068,.T.);
#58811=ORIENTED_EDGE('',*,*,#41330,.F.);
#58812=ORIENTED_EDGE('',*,*,#41331,.F.);
#58813=ORIENTED_EDGE('',*,*,#41074,.T.);
#58814=ORIENTED_EDGE('',*,*,#41331,.T.);
#58815=ORIENTED_EDGE('',*,*,#41332,.F.);
#58816=ORIENTED_EDGE('',*,*,#41072,.T.);
#58817=ORIENTED_EDGE('',*,*,#41080,.T.);
#58818=ORIENTED_EDGE('',*,*,#41075,.T.);
#58819=ORIENTED_EDGE('',*,*,#41333,.F.);
#58820=ORIENTED_EDGE('',*,*,#41334,.F.);
#58821=ORIENTED_EDGE('',*,*,#41081,.T.);
#58822=ORIENTED_EDGE('',*,*,#41334,.T.);
#58823=ORIENTED_EDGE('',*,*,#41335,.F.);
#58824=ORIENTED_EDGE('',*,*,#41079,.T.);
#58825=ORIENTED_EDGE('',*,*,#41087,.T.);
#58826=ORIENTED_EDGE('',*,*,#41082,.T.);
#58827=ORIENTED_EDGE('',*,*,#41336,.F.);
#58828=ORIENTED_EDGE('',*,*,#41337,.F.);
#58829=ORIENTED_EDGE('',*,*,#41088,.T.);
#58830=ORIENTED_EDGE('',*,*,#41337,.T.);
#58831=ORIENTED_EDGE('',*,*,#41338,.F.);
#58832=ORIENTED_EDGE('',*,*,#41086,.T.);
#58833=ORIENTED_EDGE('',*,*,#41094,.T.);
#58834=ORIENTED_EDGE('',*,*,#41089,.T.);
#58835=ORIENTED_EDGE('',*,*,#41339,.F.);
#58836=ORIENTED_EDGE('',*,*,#41340,.F.);
#58837=ORIENTED_EDGE('',*,*,#41095,.T.);
#58838=ORIENTED_EDGE('',*,*,#41340,.T.);
#58839=ORIENTED_EDGE('',*,*,#41341,.F.);
#58840=ORIENTED_EDGE('',*,*,#41093,.T.);
#58841=ORIENTED_EDGE('',*,*,#41101,.T.);
#58842=ORIENTED_EDGE('',*,*,#41096,.T.);
#58843=ORIENTED_EDGE('',*,*,#41342,.F.);
#58844=ORIENTED_EDGE('',*,*,#41343,.F.);
#58845=ORIENTED_EDGE('',*,*,#41102,.T.);
#58846=ORIENTED_EDGE('',*,*,#41343,.T.);
#58847=ORIENTED_EDGE('',*,*,#41344,.F.);
#58848=ORIENTED_EDGE('',*,*,#41100,.T.);
#58849=ORIENTED_EDGE('',*,*,#41108,.T.);
#58850=ORIENTED_EDGE('',*,*,#41103,.T.);
#58851=ORIENTED_EDGE('',*,*,#41345,.F.);
#58852=ORIENTED_EDGE('',*,*,#41346,.F.);
#58853=ORIENTED_EDGE('',*,*,#41109,.T.);
#58854=ORIENTED_EDGE('',*,*,#41346,.T.);
#58855=ORIENTED_EDGE('',*,*,#41347,.F.);
#58856=ORIENTED_EDGE('',*,*,#41107,.T.);
#58857=ORIENTED_EDGE('',*,*,#41115,.T.);
#58858=ORIENTED_EDGE('',*,*,#41110,.T.);
#58859=ORIENTED_EDGE('',*,*,#41348,.F.);
#58860=ORIENTED_EDGE('',*,*,#41349,.F.);
#58861=ORIENTED_EDGE('',*,*,#41116,.T.);
#58862=ORIENTED_EDGE('',*,*,#41349,.T.);
#58863=ORIENTED_EDGE('',*,*,#41350,.F.);
#58864=ORIENTED_EDGE('',*,*,#41114,.T.);
#58865=ORIENTED_EDGE('',*,*,#41122,.T.);
#58866=ORIENTED_EDGE('',*,*,#41117,.T.);
#58867=ORIENTED_EDGE('',*,*,#41351,.F.);
#58868=ORIENTED_EDGE('',*,*,#41352,.F.);
#58869=ORIENTED_EDGE('',*,*,#41123,.T.);
#58870=ORIENTED_EDGE('',*,*,#41352,.T.);
#58871=ORIENTED_EDGE('',*,*,#41353,.F.);
#58872=ORIENTED_EDGE('',*,*,#41121,.T.);
#58873=ORIENTED_EDGE('',*,*,#41129,.T.);
#58874=ORIENTED_EDGE('',*,*,#41124,.T.);
#58875=ORIENTED_EDGE('',*,*,#41354,.F.);
#58876=ORIENTED_EDGE('',*,*,#41355,.F.);
#58877=ORIENTED_EDGE('',*,*,#41130,.T.);
#58878=ORIENTED_EDGE('',*,*,#41355,.T.);
#58879=ORIENTED_EDGE('',*,*,#41356,.F.);
#58880=ORIENTED_EDGE('',*,*,#41128,.T.);
#58881=ORIENTED_EDGE('',*,*,#41136,.T.);
#58882=ORIENTED_EDGE('',*,*,#41131,.T.);
#58883=ORIENTED_EDGE('',*,*,#41357,.F.);
#58884=ORIENTED_EDGE('',*,*,#41358,.F.);
#58885=ORIENTED_EDGE('',*,*,#41137,.T.);
#58886=ORIENTED_EDGE('',*,*,#41358,.T.);
#58887=ORIENTED_EDGE('',*,*,#41359,.F.);
#58888=ORIENTED_EDGE('',*,*,#41135,.T.);
#58889=ORIENTED_EDGE('',*,*,#41143,.T.);
#58890=ORIENTED_EDGE('',*,*,#41138,.T.);
#58891=ORIENTED_EDGE('',*,*,#41360,.F.);
#58892=ORIENTED_EDGE('',*,*,#41361,.F.);
#58893=ORIENTED_EDGE('',*,*,#41144,.T.);
#58894=ORIENTED_EDGE('',*,*,#41361,.T.);
#58895=ORIENTED_EDGE('',*,*,#41362,.F.);
#58896=ORIENTED_EDGE('',*,*,#41142,.T.);
#58897=ORIENTED_EDGE('',*,*,#41150,.T.);
#58898=ORIENTED_EDGE('',*,*,#41145,.T.);
#58899=ORIENTED_EDGE('',*,*,#41363,.F.);
#58900=ORIENTED_EDGE('',*,*,#41364,.F.);
#58901=ORIENTED_EDGE('',*,*,#41151,.T.);
#58902=ORIENTED_EDGE('',*,*,#41364,.T.);
#58903=ORIENTED_EDGE('',*,*,#41365,.F.);
#58904=ORIENTED_EDGE('',*,*,#41149,.T.);
#58905=ORIENTED_EDGE('',*,*,#41157,.T.);
#58906=ORIENTED_EDGE('',*,*,#41152,.T.);
#58907=ORIENTED_EDGE('',*,*,#41366,.F.);
#58908=ORIENTED_EDGE('',*,*,#41367,.F.);
#58909=ORIENTED_EDGE('',*,*,#41158,.T.);
#58910=ORIENTED_EDGE('',*,*,#41367,.T.);
#58911=ORIENTED_EDGE('',*,*,#41368,.F.);
#58912=ORIENTED_EDGE('',*,*,#41156,.T.);
#58913=ORIENTED_EDGE('',*,*,#41164,.T.);
#58914=ORIENTED_EDGE('',*,*,#41159,.T.);
#58915=ORIENTED_EDGE('',*,*,#41369,.F.);
#58916=ORIENTED_EDGE('',*,*,#41370,.F.);
#58917=ORIENTED_EDGE('',*,*,#41165,.T.);
#58918=ORIENTED_EDGE('',*,*,#41370,.T.);
#58919=ORIENTED_EDGE('',*,*,#41371,.F.);
#58920=ORIENTED_EDGE('',*,*,#41163,.T.);
#58921=ORIENTED_EDGE('',*,*,#41171,.T.);
#58922=ORIENTED_EDGE('',*,*,#41166,.T.);
#58923=ORIENTED_EDGE('',*,*,#41372,.F.);
#58924=ORIENTED_EDGE('',*,*,#41373,.F.);
#58925=ORIENTED_EDGE('',*,*,#41172,.T.);
#58926=ORIENTED_EDGE('',*,*,#41373,.T.);
#58927=ORIENTED_EDGE('',*,*,#41374,.F.);
#58928=ORIENTED_EDGE('',*,*,#41170,.T.);
#58929=ORIENTED_EDGE('',*,*,#34381,.T.);
#58930=ORIENTED_EDGE('',*,*,#41173,.T.);
#58931=ORIENTED_EDGE('',*,*,#41375,.F.);
#58932=ORIENTED_EDGE('',*,*,#41376,.F.);
#58933=ORIENTED_EDGE('',*,*,#34382,.T.);
#58934=ORIENTED_EDGE('',*,*,#41376,.T.);
#58935=ORIENTED_EDGE('',*,*,#41377,.F.);
#58936=ORIENTED_EDGE('',*,*,#41175,.T.);
#58937=ORIENTED_EDGE('',*,*,#41181,.T.);
#58938=ORIENTED_EDGE('',*,*,#41176,.T.);
#58939=ORIENTED_EDGE('',*,*,#41378,.F.);
#58940=ORIENTED_EDGE('',*,*,#41379,.F.);
#58941=ORIENTED_EDGE('',*,*,#41182,.T.);
#58942=ORIENTED_EDGE('',*,*,#41379,.T.);
#58943=ORIENTED_EDGE('',*,*,#41380,.F.);
#58944=ORIENTED_EDGE('',*,*,#41180,.T.);
#58945=ORIENTED_EDGE('',*,*,#41188,.T.);
#58946=ORIENTED_EDGE('',*,*,#41183,.T.);
#58947=ORIENTED_EDGE('',*,*,#41381,.F.);
#58948=ORIENTED_EDGE('',*,*,#41382,.F.);
#58949=ORIENTED_EDGE('',*,*,#41189,.T.);
#58950=ORIENTED_EDGE('',*,*,#41382,.T.);
#58951=ORIENTED_EDGE('',*,*,#41383,.F.);
#58952=ORIENTED_EDGE('',*,*,#41187,.T.);
#58953=ORIENTED_EDGE('',*,*,#41195,.T.);
#58954=ORIENTED_EDGE('',*,*,#41190,.T.);
#58955=ORIENTED_EDGE('',*,*,#41384,.F.);
#58956=ORIENTED_EDGE('',*,*,#41385,.F.);
#58957=ORIENTED_EDGE('',*,*,#41196,.T.);
#58958=ORIENTED_EDGE('',*,*,#41385,.T.);
#58959=ORIENTED_EDGE('',*,*,#41386,.F.);
#58960=ORIENTED_EDGE('',*,*,#41194,.T.);
#58961=ORIENTED_EDGE('',*,*,#41387,.F.);
#58962=ORIENTED_EDGE('',*,*,#41388,.F.);
#58963=ORIENTED_EDGE('',*,*,#41202,.T.);
#58964=ORIENTED_EDGE('',*,*,#41197,.T.);
#58965=ORIENTED_EDGE('',*,*,#41203,.T.);
#58966=ORIENTED_EDGE('',*,*,#41388,.T.);
#58967=ORIENTED_EDGE('',*,*,#41389,.F.);
#58968=ORIENTED_EDGE('',*,*,#41201,.T.);
#58969=ORIENTED_EDGE('',*,*,#41209,.T.);
#58970=ORIENTED_EDGE('',*,*,#41204,.T.);
#58971=ORIENTED_EDGE('',*,*,#41390,.F.);
#58972=ORIENTED_EDGE('',*,*,#41391,.F.);
#58973=ORIENTED_EDGE('',*,*,#41210,.T.);
#58974=ORIENTED_EDGE('',*,*,#41391,.T.);
#58975=ORIENTED_EDGE('',*,*,#41392,.F.);
#58976=ORIENTED_EDGE('',*,*,#41208,.T.);
#58977=ORIENTED_EDGE('',*,*,#41216,.T.);
#58978=ORIENTED_EDGE('',*,*,#41211,.T.);
#58979=ORIENTED_EDGE('',*,*,#41393,.F.);
#58980=ORIENTED_EDGE('',*,*,#41394,.F.);
#58981=ORIENTED_EDGE('',*,*,#41217,.T.);
#58982=ORIENTED_EDGE('',*,*,#41394,.T.);
#58983=ORIENTED_EDGE('',*,*,#41395,.F.);
#58984=ORIENTED_EDGE('',*,*,#41215,.T.);
#58985=ORIENTED_EDGE('',*,*,#41223,.T.);
#58986=ORIENTED_EDGE('',*,*,#41218,.T.);
#58987=ORIENTED_EDGE('',*,*,#41396,.F.);
#58988=ORIENTED_EDGE('',*,*,#41397,.F.);
#58989=ORIENTED_EDGE('',*,*,#41224,.T.);
#58990=ORIENTED_EDGE('',*,*,#41397,.T.);
#58991=ORIENTED_EDGE('',*,*,#41398,.F.);
#58992=ORIENTED_EDGE('',*,*,#41222,.T.);
#58993=ORIENTED_EDGE('',*,*,#41399,.T.);
#58994=ORIENTED_EDGE('',*,*,#41400,.F.);
#58995=ORIENTED_EDGE('',*,*,#41225,.T.);
#58996=ORIENTED_EDGE('',*,*,#41401,.F.);
#58997=ORIENTED_EDGE('',*,*,#41402,.T.);
#58998=ORIENTED_EDGE('',*,*,#41403,.F.);
#58999=ORIENTED_EDGE('',*,*,#41227,.T.);
#59000=ORIENTED_EDGE('',*,*,#41404,.F.);
#59001=ORIENTED_EDGE('',*,*,#41405,.F.);
#59002=ORIENTED_EDGE('',*,*,#41406,.F.);
#59003=ORIENTED_EDGE('',*,*,#41407,.F.);
#59004=ORIENTED_EDGE('',*,*,#41402,.F.);
#59005=ORIENTED_EDGE('',*,*,#41407,.T.);
#59006=ORIENTED_EDGE('',*,*,#41408,.F.);
#59007=ORIENTED_EDGE('',*,*,#41228,.T.);
#59008=ORIENTED_EDGE('',*,*,#41403,.T.);
#59009=ORIENTED_EDGE('',*,*,#41409,.T.);
#59010=ORIENTED_EDGE('',*,*,#41410,.F.);
#59011=ORIENTED_EDGE('',*,*,#41230,.T.);
#59012=ORIENTED_EDGE('',*,*,#41411,.F.);
#59013=ORIENTED_EDGE('',*,*,#41412,.F.);
#59014=ORIENTED_EDGE('',*,*,#41413,.F.);
#59015=ORIENTED_EDGE('',*,*,#41414,.F.);
#59016=ORIENTED_EDGE('',*,*,#41409,.F.);
#59017=ORIENTED_EDGE('',*,*,#41414,.T.);
#59018=ORIENTED_EDGE('',*,*,#41415,.F.);
#59019=ORIENTED_EDGE('',*,*,#41231,.T.);
#59020=ORIENTED_EDGE('',*,*,#41410,.T.);
#59021=ORIENTED_EDGE('',*,*,#41416,.T.);
#59022=ORIENTED_EDGE('',*,*,#41417,.F.);
#59023=ORIENTED_EDGE('',*,*,#41233,.T.);
#59024=ORIENTED_EDGE('',*,*,#41418,.F.);
#59025=ORIENTED_EDGE('',*,*,#41419,.F.);
#59026=ORIENTED_EDGE('',*,*,#41420,.F.);
#59027=ORIENTED_EDGE('',*,*,#41421,.F.);
#59028=ORIENTED_EDGE('',*,*,#41416,.F.);
#59029=ORIENTED_EDGE('',*,*,#41421,.T.);
#59030=ORIENTED_EDGE('',*,*,#41422,.F.);
#59031=ORIENTED_EDGE('',*,*,#41234,.T.);
#59032=ORIENTED_EDGE('',*,*,#41417,.T.);
#59033=ORIENTED_EDGE('',*,*,#41423,.T.);
#59034=ORIENTED_EDGE('',*,*,#41424,.F.);
#59035=ORIENTED_EDGE('',*,*,#41236,.T.);
#59036=ORIENTED_EDGE('',*,*,#41425,.F.);
#59037=ORIENTED_EDGE('',*,*,#41426,.F.);
#59038=ORIENTED_EDGE('',*,*,#41427,.F.);
#59039=ORIENTED_EDGE('',*,*,#41428,.F.);
#59040=ORIENTED_EDGE('',*,*,#41423,.F.);
#59041=ORIENTED_EDGE('',*,*,#41428,.T.);
#59042=ORIENTED_EDGE('',*,*,#41429,.F.);
#59043=ORIENTED_EDGE('',*,*,#41237,.T.);
#59044=ORIENTED_EDGE('',*,*,#41424,.T.);
#59045=ORIENTED_EDGE('',*,*,#41430,.T.);
#59046=ORIENTED_EDGE('',*,*,#41431,.F.);
#59047=ORIENTED_EDGE('',*,*,#41239,.T.);
#59048=ORIENTED_EDGE('',*,*,#41432,.F.);
#59049=ORIENTED_EDGE('',*,*,#41433,.F.);
#59050=ORIENTED_EDGE('',*,*,#41434,.F.);
#59051=ORIENTED_EDGE('',*,*,#41435,.F.);
#59052=ORIENTED_EDGE('',*,*,#41430,.F.);
#59053=ORIENTED_EDGE('',*,*,#41435,.T.);
#59054=ORIENTED_EDGE('',*,*,#41436,.F.);
#59055=ORIENTED_EDGE('',*,*,#41240,.T.);
#59056=ORIENTED_EDGE('',*,*,#41431,.T.);
#59057=ORIENTED_EDGE('',*,*,#41437,.T.);
#59058=ORIENTED_EDGE('',*,*,#41438,.F.);
#59059=ORIENTED_EDGE('',*,*,#41242,.T.);
#59060=ORIENTED_EDGE('',*,*,#41439,.F.);
#59061=ORIENTED_EDGE('',*,*,#41440,.F.);
#59062=ORIENTED_EDGE('',*,*,#41441,.F.);
#59063=ORIENTED_EDGE('',*,*,#41442,.F.);
#59064=ORIENTED_EDGE('',*,*,#41437,.F.);
#59065=ORIENTED_EDGE('',*,*,#41442,.T.);
#59066=ORIENTED_EDGE('',*,*,#41443,.F.);
#59067=ORIENTED_EDGE('',*,*,#41243,.T.);
#59068=ORIENTED_EDGE('',*,*,#41438,.T.);
#59069=ORIENTED_EDGE('',*,*,#34378,.T.);
#59070=ORIENTED_EDGE('',*,*,#41444,.F.);
#59071=ORIENTED_EDGE('',*,*,#41245,.T.);
#59072=ORIENTED_EDGE('',*,*,#41445,.F.);
#59073=ORIENTED_EDGE('',*,*,#34377,.T.);
#59074=ORIENTED_EDGE('',*,*,#41446,.F.);
#59075=ORIENTED_EDGE('',*,*,#41246,.T.);
#59076=ORIENTED_EDGE('',*,*,#41444,.T.);
#59077=ORIENTED_EDGE('',*,*,#41447,.T.);
#59078=ORIENTED_EDGE('',*,*,#41448,.F.);
#59079=ORIENTED_EDGE('',*,*,#41248,.T.);
#59080=ORIENTED_EDGE('',*,*,#41449,.F.);
#59081=ORIENTED_EDGE('',*,*,#41450,.F.);
#59082=ORIENTED_EDGE('',*,*,#41451,.F.);
#59083=ORIENTED_EDGE('',*,*,#41452,.F.);
#59084=ORIENTED_EDGE('',*,*,#41447,.F.);
#59085=ORIENTED_EDGE('',*,*,#41452,.T.);
#59086=ORIENTED_EDGE('',*,*,#41453,.F.);
#59087=ORIENTED_EDGE('',*,*,#41249,.T.);
#59088=ORIENTED_EDGE('',*,*,#41448,.T.);
#59089=ORIENTED_EDGE('',*,*,#41454,.T.);
#59090=ORIENTED_EDGE('',*,*,#41455,.F.);
#59091=ORIENTED_EDGE('',*,*,#41251,.T.);
#59092=ORIENTED_EDGE('',*,*,#41456,.F.);
#59093=ORIENTED_EDGE('',*,*,#41457,.F.);
#59094=ORIENTED_EDGE('',*,*,#41458,.F.);
#59095=ORIENTED_EDGE('',*,*,#41459,.F.);
#59096=ORIENTED_EDGE('',*,*,#41454,.F.);
#59097=ORIENTED_EDGE('',*,*,#41459,.T.);
#59098=ORIENTED_EDGE('',*,*,#41460,.F.);
#59099=ORIENTED_EDGE('',*,*,#41252,.T.);
#59100=ORIENTED_EDGE('',*,*,#41455,.T.);
#59101=ORIENTED_EDGE('',*,*,#41461,.T.);
#59102=ORIENTED_EDGE('',*,*,#41462,.F.);
#59103=ORIENTED_EDGE('',*,*,#41254,.T.);
#59104=ORIENTED_EDGE('',*,*,#41463,.F.);
#59105=ORIENTED_EDGE('',*,*,#41464,.F.);
#59106=ORIENTED_EDGE('',*,*,#41465,.F.);
#59107=ORIENTED_EDGE('',*,*,#41466,.F.);
#59108=ORIENTED_EDGE('',*,*,#41461,.F.);
#59109=ORIENTED_EDGE('',*,*,#41466,.T.);
#59110=ORIENTED_EDGE('',*,*,#41467,.F.);
#59111=ORIENTED_EDGE('',*,*,#41255,.T.);
#59112=ORIENTED_EDGE('',*,*,#41462,.T.);
#59113=ORIENTED_EDGE('',*,*,#41468,.T.);
#59114=ORIENTED_EDGE('',*,*,#41469,.F.);
#59115=ORIENTED_EDGE('',*,*,#41257,.T.);
#59116=ORIENTED_EDGE('',*,*,#41470,.F.);
#59117=ORIENTED_EDGE('',*,*,#41471,.F.);
#59118=ORIENTED_EDGE('',*,*,#41472,.F.);
#59119=ORIENTED_EDGE('',*,*,#41473,.F.);
#59120=ORIENTED_EDGE('',*,*,#41468,.F.);
#59121=ORIENTED_EDGE('',*,*,#41473,.T.);
#59122=ORIENTED_EDGE('',*,*,#41474,.F.);
#59123=ORIENTED_EDGE('',*,*,#41258,.T.);
#59124=ORIENTED_EDGE('',*,*,#41469,.T.);
#59125=ORIENTED_EDGE('',*,*,#41475,.T.);
#59126=ORIENTED_EDGE('',*,*,#41476,.F.);
#59127=ORIENTED_EDGE('',*,*,#41260,.T.);
#59128=ORIENTED_EDGE('',*,*,#41477,.F.);
#59129=ORIENTED_EDGE('',*,*,#41478,.F.);
#59130=ORIENTED_EDGE('',*,*,#41479,.F.);
#59131=ORIENTED_EDGE('',*,*,#41480,.F.);
#59132=ORIENTED_EDGE('',*,*,#41475,.F.);
#59133=ORIENTED_EDGE('',*,*,#41480,.T.);
#59134=ORIENTED_EDGE('',*,*,#41481,.F.);
#59135=ORIENTED_EDGE('',*,*,#41261,.T.);
#59136=ORIENTED_EDGE('',*,*,#41476,.T.);
#59137=ORIENTED_EDGE('',*,*,#41482,.T.);
#59138=ORIENTED_EDGE('',*,*,#41483,.F.);
#59139=ORIENTED_EDGE('',*,*,#41263,.T.);
#59140=ORIENTED_EDGE('',*,*,#41484,.F.);
#59141=ORIENTED_EDGE('',*,*,#41485,.F.);
#59142=ORIENTED_EDGE('',*,*,#41486,.F.);
#59143=ORIENTED_EDGE('',*,*,#41487,.F.);
#59144=ORIENTED_EDGE('',*,*,#41482,.F.);
#59145=ORIENTED_EDGE('',*,*,#41487,.T.);
#59146=ORIENTED_EDGE('',*,*,#41488,.F.);
#59147=ORIENTED_EDGE('',*,*,#41264,.T.);
#59148=ORIENTED_EDGE('',*,*,#41483,.T.);
#59149=ORIENTED_EDGE('',*,*,#41489,.T.);
#59150=ORIENTED_EDGE('',*,*,#41490,.F.);
#59151=ORIENTED_EDGE('',*,*,#41266,.T.);
#59152=ORIENTED_EDGE('',*,*,#41491,.F.);
#59153=ORIENTED_EDGE('',*,*,#41492,.F.);
#59154=ORIENTED_EDGE('',*,*,#41493,.F.);
#59155=ORIENTED_EDGE('',*,*,#41494,.F.);
#59156=ORIENTED_EDGE('',*,*,#41489,.F.);
#59157=ORIENTED_EDGE('',*,*,#41494,.T.);
#59158=ORIENTED_EDGE('',*,*,#41495,.F.);
#59159=ORIENTED_EDGE('',*,*,#41267,.T.);
#59160=ORIENTED_EDGE('',*,*,#41490,.T.);
#59161=ORIENTED_EDGE('',*,*,#41496,.T.);
#59162=ORIENTED_EDGE('',*,*,#41497,.F.);
#59163=ORIENTED_EDGE('',*,*,#41269,.T.);
#59164=ORIENTED_EDGE('',*,*,#41498,.F.);
#59165=ORIENTED_EDGE('',*,*,#41499,.F.);
#59166=ORIENTED_EDGE('',*,*,#41500,.F.);
#59167=ORIENTED_EDGE('',*,*,#41501,.F.);
#59168=ORIENTED_EDGE('',*,*,#41496,.F.);
#59169=ORIENTED_EDGE('',*,*,#41501,.T.);
#59170=ORIENTED_EDGE('',*,*,#41502,.F.);
#59171=ORIENTED_EDGE('',*,*,#41270,.T.);
#59172=ORIENTED_EDGE('',*,*,#41497,.T.);
#59173=ORIENTED_EDGE('',*,*,#41503,.T.);
#59174=ORIENTED_EDGE('',*,*,#41504,.F.);
#59175=ORIENTED_EDGE('',*,*,#41272,.T.);
#59176=ORIENTED_EDGE('',*,*,#41505,.F.);
#59177=ORIENTED_EDGE('',*,*,#41506,.F.);
#59178=ORIENTED_EDGE('',*,*,#41507,.F.);
#59179=ORIENTED_EDGE('',*,*,#41508,.F.);
#59180=ORIENTED_EDGE('',*,*,#41503,.F.);
#59181=ORIENTED_EDGE('',*,*,#41508,.T.);
#59182=ORIENTED_EDGE('',*,*,#41509,.F.);
#59183=ORIENTED_EDGE('',*,*,#41273,.T.);
#59184=ORIENTED_EDGE('',*,*,#41504,.T.);
#59185=ORIENTED_EDGE('',*,*,#41510,.T.);
#59186=ORIENTED_EDGE('',*,*,#41511,.F.);
#59187=ORIENTED_EDGE('',*,*,#41275,.T.);
#59188=ORIENTED_EDGE('',*,*,#41512,.F.);
#59189=ORIENTED_EDGE('',*,*,#41513,.F.);
#59190=ORIENTED_EDGE('',*,*,#41514,.F.);
#59191=ORIENTED_EDGE('',*,*,#41515,.F.);
#59192=ORIENTED_EDGE('',*,*,#41510,.F.);
#59193=ORIENTED_EDGE('',*,*,#41515,.T.);
#59194=ORIENTED_EDGE('',*,*,#41516,.F.);
#59195=ORIENTED_EDGE('',*,*,#41276,.T.);
#59196=ORIENTED_EDGE('',*,*,#41511,.T.);
#59197=ORIENTED_EDGE('',*,*,#41517,.T.);
#59198=ORIENTED_EDGE('',*,*,#41518,.F.);
#59199=ORIENTED_EDGE('',*,*,#41278,.T.);
#59200=ORIENTED_EDGE('',*,*,#41519,.F.);
#59201=ORIENTED_EDGE('',*,*,#41520,.F.);
#59202=ORIENTED_EDGE('',*,*,#41521,.F.);
#59203=ORIENTED_EDGE('',*,*,#41522,.F.);
#59204=ORIENTED_EDGE('',*,*,#41517,.F.);
#59205=ORIENTED_EDGE('',*,*,#41522,.T.);
#59206=ORIENTED_EDGE('',*,*,#41523,.F.);
#59207=ORIENTED_EDGE('',*,*,#41279,.T.);
#59208=ORIENTED_EDGE('',*,*,#41518,.T.);
#59209=ORIENTED_EDGE('',*,*,#41524,.T.);
#59210=ORIENTED_EDGE('',*,*,#41525,.F.);
#59211=ORIENTED_EDGE('',*,*,#41281,.T.);
#59212=ORIENTED_EDGE('',*,*,#41526,.F.);
#59213=ORIENTED_EDGE('',*,*,#41527,.T.);
#59214=ORIENTED_EDGE('',*,*,#41528,.F.);
#59215=ORIENTED_EDGE('',*,*,#41282,.T.);
#59216=ORIENTED_EDGE('',*,*,#41525,.T.);
#59217=ORIENTED_EDGE('',*,*,#41529,.F.);
#59218=ORIENTED_EDGE('',*,*,#41530,.F.);
#59219=ORIENTED_EDGE('',*,*,#41527,.F.);
#59220=ORIENTED_EDGE('',*,*,#41524,.F.);
#59221=ORIENTED_EDGE('',*,*,#41284,.T.);
#59222=ORIENTED_EDGE('',*,*,#41531,.F.);
#59223=ORIENTED_EDGE('',*,*,#41532,.T.);
#59224=ORIENTED_EDGE('',*,*,#41533,.F.);
#59225=ORIENTED_EDGE('',*,*,#41534,.F.);
#59226=ORIENTED_EDGE('',*,*,#41532,.F.);
#59227=ORIENTED_EDGE('',*,*,#41535,.F.);
#59228=ORIENTED_EDGE('',*,*,#41536,.F.);
#59229=ORIENTED_EDGE('',*,*,#41285,.T.);
#59230=ORIENTED_EDGE('',*,*,#41533,.T.);
#59231=ORIENTED_EDGE('',*,*,#41534,.T.);
#59232=ORIENTED_EDGE('',*,*,#41537,.F.);
#59233=ORIENTED_EDGE('',*,*,#41538,.T.);
#59234=ORIENTED_EDGE('',*,*,#41539,.F.);
#59235=ORIENTED_EDGE('',*,*,#41287,.T.);
#59236=ORIENTED_EDGE('',*,*,#41540,.F.);
#59237=ORIENTED_EDGE('',*,*,#41541,.F.);
#59238=ORIENTED_EDGE('',*,*,#41542,.F.);
#59239=ORIENTED_EDGE('',*,*,#41543,.F.);
#59240=ORIENTED_EDGE('',*,*,#41538,.F.);
#59241=ORIENTED_EDGE('',*,*,#41543,.T.);
#59242=ORIENTED_EDGE('',*,*,#41544,.F.);
#59243=ORIENTED_EDGE('',*,*,#41288,.T.);
#59244=ORIENTED_EDGE('',*,*,#41539,.T.);
#59245=ORIENTED_EDGE('',*,*,#41545,.T.);
#59246=ORIENTED_EDGE('',*,*,#41546,.F.);
#59247=ORIENTED_EDGE('',*,*,#41290,.T.);
#59248=ORIENTED_EDGE('',*,*,#41547,.F.);
#59249=ORIENTED_EDGE('',*,*,#41548,.F.);
#59250=ORIENTED_EDGE('',*,*,#41549,.F.);
#59251=ORIENTED_EDGE('',*,*,#41550,.F.);
#59252=ORIENTED_EDGE('',*,*,#41545,.F.);
#59253=ORIENTED_EDGE('',*,*,#41550,.T.);
#59254=ORIENTED_EDGE('',*,*,#41551,.F.);
#59255=ORIENTED_EDGE('',*,*,#41291,.T.);
#59256=ORIENTED_EDGE('',*,*,#41546,.T.);
#59257=ORIENTED_EDGE('',*,*,#41552,.T.);
#59258=ORIENTED_EDGE('',*,*,#41553,.F.);
#59259=ORIENTED_EDGE('',*,*,#41293,.T.);
#59260=ORIENTED_EDGE('',*,*,#41554,.F.);
#59261=ORIENTED_EDGE('',*,*,#41555,.F.);
#59262=ORIENTED_EDGE('',*,*,#41556,.F.);
#59263=ORIENTED_EDGE('',*,*,#41557,.F.);
#59264=ORIENTED_EDGE('',*,*,#41552,.F.);
#59265=ORIENTED_EDGE('',*,*,#41557,.T.);
#59266=ORIENTED_EDGE('',*,*,#41558,.F.);
#59267=ORIENTED_EDGE('',*,*,#41294,.T.);
#59268=ORIENTED_EDGE('',*,*,#41553,.T.);
#59269=ORIENTED_EDGE('',*,*,#41559,.T.);
#59270=ORIENTED_EDGE('',*,*,#41560,.F.);
#59271=ORIENTED_EDGE('',*,*,#41296,.T.);
#59272=ORIENTED_EDGE('',*,*,#41561,.F.);
#59273=ORIENTED_EDGE('',*,*,#41562,.F.);
#59274=ORIENTED_EDGE('',*,*,#41563,.F.);
#59275=ORIENTED_EDGE('',*,*,#41564,.F.);
#59276=ORIENTED_EDGE('',*,*,#41559,.F.);
#59277=ORIENTED_EDGE('',*,*,#41564,.T.);
#59278=ORIENTED_EDGE('',*,*,#41565,.F.);
#59279=ORIENTED_EDGE('',*,*,#41297,.T.);
#59280=ORIENTED_EDGE('',*,*,#41560,.T.);
#59281=ORIENTED_EDGE('',*,*,#41566,.T.);
#59282=ORIENTED_EDGE('',*,*,#41567,.F.);
#59283=ORIENTED_EDGE('',*,*,#41299,.T.);
#59284=ORIENTED_EDGE('',*,*,#41568,.F.);
#59285=ORIENTED_EDGE('',*,*,#41569,.F.);
#59286=ORIENTED_EDGE('',*,*,#41570,.F.);
#59287=ORIENTED_EDGE('',*,*,#41571,.F.);
#59288=ORIENTED_EDGE('',*,*,#41566,.F.);
#59289=ORIENTED_EDGE('',*,*,#41571,.T.);
#59290=ORIENTED_EDGE('',*,*,#41572,.F.);
#59291=ORIENTED_EDGE('',*,*,#41300,.T.);
#59292=ORIENTED_EDGE('',*,*,#41567,.T.);
#59293=ORIENTED_EDGE('',*,*,#41573,.T.);
#59294=ORIENTED_EDGE('',*,*,#41574,.F.);
#59295=ORIENTED_EDGE('',*,*,#41302,.T.);
#59296=ORIENTED_EDGE('',*,*,#41575,.F.);
#59297=ORIENTED_EDGE('',*,*,#41576,.F.);
#59298=ORIENTED_EDGE('',*,*,#41577,.F.);
#59299=ORIENTED_EDGE('',*,*,#41578,.F.);
#59300=ORIENTED_EDGE('',*,*,#41573,.F.);
#59301=ORIENTED_EDGE('',*,*,#41578,.T.);
#59302=ORIENTED_EDGE('',*,*,#41579,.F.);
#59303=ORIENTED_EDGE('',*,*,#41303,.T.);
#59304=ORIENTED_EDGE('',*,*,#41574,.T.);
#59305=ORIENTED_EDGE('',*,*,#41580,.T.);
#59306=ORIENTED_EDGE('',*,*,#41581,.F.);
#59307=ORIENTED_EDGE('',*,*,#41305,.T.);
#59308=ORIENTED_EDGE('',*,*,#41582,.F.);
#59309=ORIENTED_EDGE('',*,*,#41583,.F.);
#59310=ORIENTED_EDGE('',*,*,#41584,.F.);
#59311=ORIENTED_EDGE('',*,*,#41585,.F.);
#59312=ORIENTED_EDGE('',*,*,#41580,.F.);
#59313=ORIENTED_EDGE('',*,*,#41585,.T.);
#59314=ORIENTED_EDGE('',*,*,#41586,.F.);
#59315=ORIENTED_EDGE('',*,*,#41306,.T.);
#59316=ORIENTED_EDGE('',*,*,#41581,.T.);
#59317=ORIENTED_EDGE('',*,*,#41587,.T.);
#59318=ORIENTED_EDGE('',*,*,#41588,.F.);
#59319=ORIENTED_EDGE('',*,*,#41308,.T.);
#59320=ORIENTED_EDGE('',*,*,#41589,.F.);
#59321=ORIENTED_EDGE('',*,*,#41590,.F.);
#59322=ORIENTED_EDGE('',*,*,#41591,.F.);
#59323=ORIENTED_EDGE('',*,*,#41592,.F.);
#59324=ORIENTED_EDGE('',*,*,#41587,.F.);
#59325=ORIENTED_EDGE('',*,*,#41592,.T.);
#59326=ORIENTED_EDGE('',*,*,#41593,.F.);
#59327=ORIENTED_EDGE('',*,*,#41309,.T.);
#59328=ORIENTED_EDGE('',*,*,#41588,.T.);
#59329=ORIENTED_EDGE('',*,*,#41594,.F.);
#59330=ORIENTED_EDGE('',*,*,#41595,.F.);
#59331=ORIENTED_EDGE('',*,*,#41399,.F.);
#59332=ORIENTED_EDGE('',*,*,#41596,.F.);
#59333=ORIENTED_EDGE('',*,*,#41596,.T.);
#59334=ORIENTED_EDGE('',*,*,#41401,.T.);
#59335=ORIENTED_EDGE('',*,*,#41311,.T.);
#59336=ORIENTED_EDGE('',*,*,#41597,.F.);
#59337=ORIENTED_EDGE('',*,*,#41312,.T.);
#59338=ORIENTED_EDGE('',*,*,#41598,.F.);
#59339=ORIENTED_EDGE('',*,*,#41599,.T.);
#59340=ORIENTED_EDGE('',*,*,#41600,.F.);
#59341=ORIENTED_EDGE('',*,*,#41314,.T.);
#59342=ORIENTED_EDGE('',*,*,#41601,.F.);
#59343=ORIENTED_EDGE('',*,*,#41602,.T.);
#59344=ORIENTED_EDGE('',*,*,#41603,.F.);
#59345=ORIENTED_EDGE('',*,*,#41315,.T.);
#59346=ORIENTED_EDGE('',*,*,#41603,.T.);
#59347=ORIENTED_EDGE('',*,*,#41604,.T.);
#59348=ORIENTED_EDGE('',*,*,#41605,.F.);
#59349=ORIENTED_EDGE('',*,*,#41604,.F.);
#59350=ORIENTED_EDGE('',*,*,#41602,.F.);
#59351=ORIENTED_EDGE('',*,*,#41606,.F.);
#59352=ORIENTED_EDGE('',*,*,#41607,.F.);
#59353=ORIENTED_EDGE('',*,*,#41317,.T.);
#59354=ORIENTED_EDGE('',*,*,#41608,.F.);
#59355=ORIENTED_EDGE('',*,*,#41609,.T.);
#59356=ORIENTED_EDGE('',*,*,#41610,.F.);
#59357=ORIENTED_EDGE('',*,*,#41318,.T.);
#59358=ORIENTED_EDGE('',*,*,#41610,.T.);
#59359=ORIENTED_EDGE('',*,*,#41611,.T.);
#59360=ORIENTED_EDGE('',*,*,#41612,.F.);
#59361=ORIENTED_EDGE('',*,*,#41611,.F.);
#59362=ORIENTED_EDGE('',*,*,#41609,.F.);
#59363=ORIENTED_EDGE('',*,*,#41613,.F.);
#59364=ORIENTED_EDGE('',*,*,#41614,.F.);
#59365=ORIENTED_EDGE('',*,*,#41320,.T.);
#59366=ORIENTED_EDGE('',*,*,#41615,.F.);
#59367=ORIENTED_EDGE('',*,*,#41616,.T.);
#59368=ORIENTED_EDGE('',*,*,#41617,.F.);
#59369=ORIENTED_EDGE('',*,*,#41321,.T.);
#59370=ORIENTED_EDGE('',*,*,#41617,.T.);
#59371=ORIENTED_EDGE('',*,*,#41618,.T.);
#59372=ORIENTED_EDGE('',*,*,#41619,.F.);
#59373=ORIENTED_EDGE('',*,*,#41618,.F.);
#59374=ORIENTED_EDGE('',*,*,#41616,.F.);
#59375=ORIENTED_EDGE('',*,*,#41620,.F.);
#59376=ORIENTED_EDGE('',*,*,#41621,.F.);
#59377=ORIENTED_EDGE('',*,*,#41323,.T.);
#59378=ORIENTED_EDGE('',*,*,#41622,.F.);
#59379=ORIENTED_EDGE('',*,*,#41623,.T.);
#59380=ORIENTED_EDGE('',*,*,#41624,.F.);
#59381=ORIENTED_EDGE('',*,*,#41324,.T.);
#59382=ORIENTED_EDGE('',*,*,#41624,.T.);
#59383=ORIENTED_EDGE('',*,*,#41625,.T.);
#59384=ORIENTED_EDGE('',*,*,#41626,.F.);
#59385=ORIENTED_EDGE('',*,*,#41625,.F.);
#59386=ORIENTED_EDGE('',*,*,#41623,.F.);
#59387=ORIENTED_EDGE('',*,*,#41627,.F.);
#59388=ORIENTED_EDGE('',*,*,#41628,.F.);
#59389=ORIENTED_EDGE('',*,*,#41326,.T.);
#59390=ORIENTED_EDGE('',*,*,#41629,.F.);
#59391=ORIENTED_EDGE('',*,*,#41630,.T.);
#59392=ORIENTED_EDGE('',*,*,#41631,.F.);
#59393=ORIENTED_EDGE('',*,*,#41327,.T.);
#59394=ORIENTED_EDGE('',*,*,#41631,.T.);
#59395=ORIENTED_EDGE('',*,*,#41632,.T.);
#59396=ORIENTED_EDGE('',*,*,#41633,.F.);
#59397=ORIENTED_EDGE('',*,*,#41632,.F.);
#59398=ORIENTED_EDGE('',*,*,#41630,.F.);
#59399=ORIENTED_EDGE('',*,*,#41634,.F.);
#59400=ORIENTED_EDGE('',*,*,#41635,.F.);
#59401=ORIENTED_EDGE('',*,*,#41329,.T.);
#59402=ORIENTED_EDGE('',*,*,#41636,.F.);
#59403=ORIENTED_EDGE('',*,*,#41637,.T.);
#59404=ORIENTED_EDGE('',*,*,#41638,.F.);
#59405=ORIENTED_EDGE('',*,*,#41330,.T.);
#59406=ORIENTED_EDGE('',*,*,#41638,.T.);
#59407=ORIENTED_EDGE('',*,*,#41639,.T.);
#59408=ORIENTED_EDGE('',*,*,#41640,.F.);
#59409=ORIENTED_EDGE('',*,*,#41639,.F.);
#59410=ORIENTED_EDGE('',*,*,#41637,.F.);
#59411=ORIENTED_EDGE('',*,*,#41641,.F.);
#59412=ORIENTED_EDGE('',*,*,#41642,.F.);
#59413=ORIENTED_EDGE('',*,*,#41332,.T.);
#59414=ORIENTED_EDGE('',*,*,#41643,.F.);
#59415=ORIENTED_EDGE('',*,*,#41644,.T.);
#59416=ORIENTED_EDGE('',*,*,#41645,.F.);
#59417=ORIENTED_EDGE('',*,*,#41333,.T.);
#59418=ORIENTED_EDGE('',*,*,#41645,.T.);
#59419=ORIENTED_EDGE('',*,*,#41646,.T.);
#59420=ORIENTED_EDGE('',*,*,#41647,.F.);
#59421=ORIENTED_EDGE('',*,*,#41646,.F.);
#59422=ORIENTED_EDGE('',*,*,#41644,.F.);
#59423=ORIENTED_EDGE('',*,*,#41648,.F.);
#59424=ORIENTED_EDGE('',*,*,#41649,.F.);
#59425=ORIENTED_EDGE('',*,*,#41335,.T.);
#59426=ORIENTED_EDGE('',*,*,#41650,.F.);
#59427=ORIENTED_EDGE('',*,*,#41651,.T.);
#59428=ORIENTED_EDGE('',*,*,#41652,.F.);
#59429=ORIENTED_EDGE('',*,*,#41336,.T.);
#59430=ORIENTED_EDGE('',*,*,#41652,.T.);
#59431=ORIENTED_EDGE('',*,*,#41653,.T.);
#59432=ORIENTED_EDGE('',*,*,#41654,.F.);
#59433=ORIENTED_EDGE('',*,*,#41653,.F.);
#59434=ORIENTED_EDGE('',*,*,#41651,.F.);
#59435=ORIENTED_EDGE('',*,*,#41655,.F.);
#59436=ORIENTED_EDGE('',*,*,#41656,.F.);
#59437=ORIENTED_EDGE('',*,*,#41338,.T.);
#59438=ORIENTED_EDGE('',*,*,#41657,.F.);
#59439=ORIENTED_EDGE('',*,*,#41658,.T.);
#59440=ORIENTED_EDGE('',*,*,#41659,.F.);
#59441=ORIENTED_EDGE('',*,*,#41339,.T.);
#59442=ORIENTED_EDGE('',*,*,#41659,.T.);
#59443=ORIENTED_EDGE('',*,*,#41660,.T.);
#59444=ORIENTED_EDGE('',*,*,#41661,.F.);
#59445=ORIENTED_EDGE('',*,*,#41660,.F.);
#59446=ORIENTED_EDGE('',*,*,#41658,.F.);
#59447=ORIENTED_EDGE('',*,*,#41662,.F.);
#59448=ORIENTED_EDGE('',*,*,#41663,.F.);
#59449=ORIENTED_EDGE('',*,*,#41341,.T.);
#59450=ORIENTED_EDGE('',*,*,#41664,.F.);
#59451=ORIENTED_EDGE('',*,*,#41665,.T.);
#59452=ORIENTED_EDGE('',*,*,#41666,.F.);
#59453=ORIENTED_EDGE('',*,*,#41342,.T.);
#59454=ORIENTED_EDGE('',*,*,#41666,.T.);
#59455=ORIENTED_EDGE('',*,*,#41667,.T.);
#59456=ORIENTED_EDGE('',*,*,#41668,.F.);
#59457=ORIENTED_EDGE('',*,*,#41667,.F.);
#59458=ORIENTED_EDGE('',*,*,#41665,.F.);
#59459=ORIENTED_EDGE('',*,*,#41669,.F.);
#59460=ORIENTED_EDGE('',*,*,#41670,.F.);
#59461=ORIENTED_EDGE('',*,*,#41344,.T.);
#59462=ORIENTED_EDGE('',*,*,#41671,.F.);
#59463=ORIENTED_EDGE('',*,*,#41672,.T.);
#59464=ORIENTED_EDGE('',*,*,#41673,.F.);
#59465=ORIENTED_EDGE('',*,*,#41345,.T.);
#59466=ORIENTED_EDGE('',*,*,#41673,.T.);
#59467=ORIENTED_EDGE('',*,*,#41674,.T.);
#59468=ORIENTED_EDGE('',*,*,#41675,.F.);
#59469=ORIENTED_EDGE('',*,*,#41674,.F.);
#59470=ORIENTED_EDGE('',*,*,#41672,.F.);
#59471=ORIENTED_EDGE('',*,*,#41676,.F.);
#59472=ORIENTED_EDGE('',*,*,#41677,.F.);
#59473=ORIENTED_EDGE('',*,*,#41347,.T.);
#59474=ORIENTED_EDGE('',*,*,#41678,.F.);
#59475=ORIENTED_EDGE('',*,*,#41679,.T.);
#59476=ORIENTED_EDGE('',*,*,#41680,.F.);
#59477=ORIENTED_EDGE('',*,*,#41348,.T.);
#59478=ORIENTED_EDGE('',*,*,#41680,.T.);
#59479=ORIENTED_EDGE('',*,*,#41681,.T.);
#59480=ORIENTED_EDGE('',*,*,#41682,.F.);
#59481=ORIENTED_EDGE('',*,*,#41681,.F.);
#59482=ORIENTED_EDGE('',*,*,#41679,.F.);
#59483=ORIENTED_EDGE('',*,*,#41683,.F.);
#59484=ORIENTED_EDGE('',*,*,#41684,.F.);
#59485=ORIENTED_EDGE('',*,*,#41350,.T.);
#59486=ORIENTED_EDGE('',*,*,#41685,.F.);
#59487=ORIENTED_EDGE('',*,*,#41686,.T.);
#59488=ORIENTED_EDGE('',*,*,#41687,.F.);
#59489=ORIENTED_EDGE('',*,*,#41351,.T.);
#59490=ORIENTED_EDGE('',*,*,#41687,.T.);
#59491=ORIENTED_EDGE('',*,*,#41688,.T.);
#59492=ORIENTED_EDGE('',*,*,#41689,.F.);
#59493=ORIENTED_EDGE('',*,*,#41688,.F.);
#59494=ORIENTED_EDGE('',*,*,#41686,.F.);
#59495=ORIENTED_EDGE('',*,*,#41690,.F.);
#59496=ORIENTED_EDGE('',*,*,#41691,.F.);
#59497=ORIENTED_EDGE('',*,*,#41353,.T.);
#59498=ORIENTED_EDGE('',*,*,#41692,.F.);
#59499=ORIENTED_EDGE('',*,*,#34375,.T.);
#59500=ORIENTED_EDGE('',*,*,#41693,.F.);
#59501=ORIENTED_EDGE('',*,*,#41354,.T.);
#59502=ORIENTED_EDGE('',*,*,#41693,.T.);
#59503=ORIENTED_EDGE('',*,*,#34374,.T.);
#59504=ORIENTED_EDGE('',*,*,#41694,.F.);
#59505=ORIENTED_EDGE('',*,*,#41356,.T.);
#59506=ORIENTED_EDGE('',*,*,#41695,.F.);
#59507=ORIENTED_EDGE('',*,*,#41696,.T.);
#59508=ORIENTED_EDGE('',*,*,#41697,.F.);
#59509=ORIENTED_EDGE('',*,*,#41357,.T.);
#59510=ORIENTED_EDGE('',*,*,#41697,.T.);
#59511=ORIENTED_EDGE('',*,*,#41698,.T.);
#59512=ORIENTED_EDGE('',*,*,#41699,.F.);
#59513=ORIENTED_EDGE('',*,*,#41698,.F.);
#59514=ORIENTED_EDGE('',*,*,#41696,.F.);
#59515=ORIENTED_EDGE('',*,*,#41700,.F.);
#59516=ORIENTED_EDGE('',*,*,#41701,.F.);
#59517=ORIENTED_EDGE('',*,*,#41359,.T.);
#59518=ORIENTED_EDGE('',*,*,#41702,.F.);
#59519=ORIENTED_EDGE('',*,*,#41703,.T.);
#59520=ORIENTED_EDGE('',*,*,#41704,.F.);
#59521=ORIENTED_EDGE('',*,*,#41360,.T.);
#59522=ORIENTED_EDGE('',*,*,#41704,.T.);
#59523=ORIENTED_EDGE('',*,*,#41705,.T.);
#59524=ORIENTED_EDGE('',*,*,#41706,.F.);
#59525=ORIENTED_EDGE('',*,*,#41705,.F.);
#59526=ORIENTED_EDGE('',*,*,#41703,.F.);
#59527=ORIENTED_EDGE('',*,*,#41707,.F.);
#59528=ORIENTED_EDGE('',*,*,#41708,.F.);
#59529=ORIENTED_EDGE('',*,*,#41362,.T.);
#59530=ORIENTED_EDGE('',*,*,#41709,.F.);
#59531=ORIENTED_EDGE('',*,*,#41710,.T.);
#59532=ORIENTED_EDGE('',*,*,#41711,.F.);
#59533=ORIENTED_EDGE('',*,*,#41363,.T.);
#59534=ORIENTED_EDGE('',*,*,#41711,.T.);
#59535=ORIENTED_EDGE('',*,*,#41712,.T.);
#59536=ORIENTED_EDGE('',*,*,#41713,.F.);
#59537=ORIENTED_EDGE('',*,*,#41712,.F.);
#59538=ORIENTED_EDGE('',*,*,#41710,.F.);
#59539=ORIENTED_EDGE('',*,*,#41714,.F.);
#59540=ORIENTED_EDGE('',*,*,#41715,.F.);
#59541=ORIENTED_EDGE('',*,*,#41365,.T.);
#59542=ORIENTED_EDGE('',*,*,#41716,.F.);
#59543=ORIENTED_EDGE('',*,*,#41717,.T.);
#59544=ORIENTED_EDGE('',*,*,#41718,.F.);
#59545=ORIENTED_EDGE('',*,*,#41366,.T.);
#59546=ORIENTED_EDGE('',*,*,#41718,.T.);
#59547=ORIENTED_EDGE('',*,*,#41719,.T.);
#59548=ORIENTED_EDGE('',*,*,#41720,.F.);
#59549=ORIENTED_EDGE('',*,*,#41719,.F.);
#59550=ORIENTED_EDGE('',*,*,#41717,.F.);
#59551=ORIENTED_EDGE('',*,*,#41721,.F.);
#59552=ORIENTED_EDGE('',*,*,#41722,.F.);
#59553=ORIENTED_EDGE('',*,*,#41368,.T.);
#59554=ORIENTED_EDGE('',*,*,#41723,.F.);
#59555=ORIENTED_EDGE('',*,*,#41724,.T.);
#59556=ORIENTED_EDGE('',*,*,#41725,.F.);
#59557=ORIENTED_EDGE('',*,*,#41369,.T.);
#59558=ORIENTED_EDGE('',*,*,#41725,.T.);
#59559=ORIENTED_EDGE('',*,*,#41726,.T.);
#59560=ORIENTED_EDGE('',*,*,#41727,.F.);
#59561=ORIENTED_EDGE('',*,*,#41726,.F.);
#59562=ORIENTED_EDGE('',*,*,#41724,.F.);
#59563=ORIENTED_EDGE('',*,*,#41728,.F.);
#59564=ORIENTED_EDGE('',*,*,#41729,.F.);
#59565=ORIENTED_EDGE('',*,*,#41371,.T.);
#59566=ORIENTED_EDGE('',*,*,#41730,.F.);
#59567=ORIENTED_EDGE('',*,*,#41731,.T.);
#59568=ORIENTED_EDGE('',*,*,#41732,.F.);
#59569=ORIENTED_EDGE('',*,*,#41372,.T.);
#59570=ORIENTED_EDGE('',*,*,#41732,.T.);
#59571=ORIENTED_EDGE('',*,*,#41733,.T.);
#59572=ORIENTED_EDGE('',*,*,#41734,.F.);
#59573=ORIENTED_EDGE('',*,*,#41733,.F.);
#59574=ORIENTED_EDGE('',*,*,#41731,.F.);
#59575=ORIENTED_EDGE('',*,*,#41735,.F.);
#59576=ORIENTED_EDGE('',*,*,#41736,.F.);
#59577=ORIENTED_EDGE('',*,*,#41374,.T.);
#59578=ORIENTED_EDGE('',*,*,#41737,.F.);
#59579=ORIENTED_EDGE('',*,*,#41738,.T.);
#59580=ORIENTED_EDGE('',*,*,#41739,.F.);
#59581=ORIENTED_EDGE('',*,*,#41375,.T.);
#59582=ORIENTED_EDGE('',*,*,#41739,.T.);
#59583=ORIENTED_EDGE('',*,*,#41740,.T.);
#59584=ORIENTED_EDGE('',*,*,#41741,.F.);
#59585=ORIENTED_EDGE('',*,*,#41740,.F.);
#59586=ORIENTED_EDGE('',*,*,#41738,.F.);
#59587=ORIENTED_EDGE('',*,*,#41742,.F.);
#59588=ORIENTED_EDGE('',*,*,#41743,.F.);
#59589=ORIENTED_EDGE('',*,*,#41377,.T.);
#59590=ORIENTED_EDGE('',*,*,#41744,.F.);
#59591=ORIENTED_EDGE('',*,*,#41745,.T.);
#59592=ORIENTED_EDGE('',*,*,#41746,.F.);
#59593=ORIENTED_EDGE('',*,*,#41378,.T.);
#59594=ORIENTED_EDGE('',*,*,#41746,.T.);
#59595=ORIENTED_EDGE('',*,*,#41747,.T.);
#59596=ORIENTED_EDGE('',*,*,#41748,.F.);
#59597=ORIENTED_EDGE('',*,*,#41747,.F.);
#59598=ORIENTED_EDGE('',*,*,#41745,.F.);
#59599=ORIENTED_EDGE('',*,*,#41749,.F.);
#59600=ORIENTED_EDGE('',*,*,#41750,.F.);
#59601=ORIENTED_EDGE('',*,*,#41380,.T.);
#59602=ORIENTED_EDGE('',*,*,#41751,.F.);
#59603=ORIENTED_EDGE('',*,*,#41752,.T.);
#59604=ORIENTED_EDGE('',*,*,#41753,.F.);
#59605=ORIENTED_EDGE('',*,*,#41381,.T.);
#59606=ORIENTED_EDGE('',*,*,#41753,.T.);
#59607=ORIENTED_EDGE('',*,*,#41754,.T.);
#59608=ORIENTED_EDGE('',*,*,#41755,.F.);
#59609=ORIENTED_EDGE('',*,*,#41754,.F.);
#59610=ORIENTED_EDGE('',*,*,#41752,.F.);
#59611=ORIENTED_EDGE('',*,*,#41756,.F.);
#59612=ORIENTED_EDGE('',*,*,#41757,.F.);
#59613=ORIENTED_EDGE('',*,*,#41383,.T.);
#59614=ORIENTED_EDGE('',*,*,#41758,.F.);
#59615=ORIENTED_EDGE('',*,*,#41759,.T.);
#59616=ORIENTED_EDGE('',*,*,#41760,.F.);
#59617=ORIENTED_EDGE('',*,*,#41384,.T.);
#59618=ORIENTED_EDGE('',*,*,#41760,.T.);
#59619=ORIENTED_EDGE('',*,*,#41761,.T.);
#59620=ORIENTED_EDGE('',*,*,#41762,.F.);
#59621=ORIENTED_EDGE('',*,*,#41761,.F.);
#59622=ORIENTED_EDGE('',*,*,#41759,.F.);
#59623=ORIENTED_EDGE('',*,*,#41763,.F.);
#59624=ORIENTED_EDGE('',*,*,#41764,.F.);
#59625=ORIENTED_EDGE('',*,*,#41386,.T.);
#59626=ORIENTED_EDGE('',*,*,#41765,.F.);
#59627=ORIENTED_EDGE('',*,*,#41766,.T.);
#59628=ORIENTED_EDGE('',*,*,#41767,.F.);
#59629=ORIENTED_EDGE('',*,*,#41768,.T.);
#59630=ORIENTED_EDGE('',*,*,#41769,.F.);
#59631=ORIENTED_EDGE('',*,*,#41387,.T.);
#59632=ORIENTED_EDGE('',*,*,#41767,.T.);
#59633=ORIENTED_EDGE('',*,*,#41770,.F.);
#59634=ORIENTED_EDGE('',*,*,#41771,.F.);
#59635=ORIENTED_EDGE('',*,*,#41768,.F.);
#59636=ORIENTED_EDGE('',*,*,#41766,.F.);
#59637=ORIENTED_EDGE('',*,*,#41389,.T.);
#59638=ORIENTED_EDGE('',*,*,#41772,.F.);
#59639=ORIENTED_EDGE('',*,*,#41773,.T.);
#59640=ORIENTED_EDGE('',*,*,#41774,.F.);
#59641=ORIENTED_EDGE('',*,*,#41390,.T.);
#59642=ORIENTED_EDGE('',*,*,#41774,.T.);
#59643=ORIENTED_EDGE('',*,*,#41775,.T.);
#59644=ORIENTED_EDGE('',*,*,#41776,.F.);
#59645=ORIENTED_EDGE('',*,*,#41775,.F.);
#59646=ORIENTED_EDGE('',*,*,#41773,.F.);
#59647=ORIENTED_EDGE('',*,*,#41777,.F.);
#59648=ORIENTED_EDGE('',*,*,#41778,.F.);
#59649=ORIENTED_EDGE('',*,*,#41392,.T.);
#59650=ORIENTED_EDGE('',*,*,#41779,.F.);
#59651=ORIENTED_EDGE('',*,*,#41780,.T.);
#59652=ORIENTED_EDGE('',*,*,#41781,.F.);
#59653=ORIENTED_EDGE('',*,*,#41393,.T.);
#59654=ORIENTED_EDGE('',*,*,#41781,.T.);
#59655=ORIENTED_EDGE('',*,*,#41782,.T.);
#59656=ORIENTED_EDGE('',*,*,#41783,.F.);
#59657=ORIENTED_EDGE('',*,*,#41782,.F.);
#59658=ORIENTED_EDGE('',*,*,#41780,.F.);
#59659=ORIENTED_EDGE('',*,*,#41784,.F.);
#59660=ORIENTED_EDGE('',*,*,#41785,.F.);
#59661=ORIENTED_EDGE('',*,*,#41395,.T.);
#59662=ORIENTED_EDGE('',*,*,#41786,.F.);
#59663=ORIENTED_EDGE('',*,*,#41787,.T.);
#59664=ORIENTED_EDGE('',*,*,#41788,.F.);
#59665=ORIENTED_EDGE('',*,*,#41396,.T.);
#59666=ORIENTED_EDGE('',*,*,#41788,.T.);
#59667=ORIENTED_EDGE('',*,*,#41789,.T.);
#59668=ORIENTED_EDGE('',*,*,#41790,.F.);
#59669=ORIENTED_EDGE('',*,*,#41789,.F.);
#59670=ORIENTED_EDGE('',*,*,#41787,.F.);
#59671=ORIENTED_EDGE('',*,*,#41791,.F.);
#59672=ORIENTED_EDGE('',*,*,#41792,.F.);
#59673=ORIENTED_EDGE('',*,*,#41599,.F.);
#59674=ORIENTED_EDGE('',*,*,#41793,.F.);
#59675=ORIENTED_EDGE('',*,*,#41794,.F.);
#59676=ORIENTED_EDGE('',*,*,#41795,.F.);
#59677=ORIENTED_EDGE('',*,*,#41398,.T.);
#59678=ORIENTED_EDGE('',*,*,#41796,.F.);
#59679=ORIENTED_EDGE('',*,*,#41793,.T.);
#59680=ORIENTED_EDGE('',*,*,#41598,.T.);
#59681=ORIENTED_EDGE('',*,*,#41797,.F.);
#59682=ORIENTED_EDGE('',*,*,#41400,.T.);
#59683=ORIENTED_EDGE('',*,*,#41595,.T.);
#59684=ORIENTED_EDGE('',*,*,#41798,.F.);
#59685=ORIENTED_EDGE('',*,*,#41799,.F.);
#59686=ORIENTED_EDGE('',*,*,#41800,.F.);
#59687=ORIENTED_EDGE('',*,*,#41405,.T.);
#59688=ORIENTED_EDGE('',*,*,#41404,.T.);
#59689=ORIENTED_EDGE('',*,*,#41801,.F.);
#59690=ORIENTED_EDGE('',*,*,#41408,.T.);
#59691=ORIENTED_EDGE('',*,*,#41406,.T.);
#59692=ORIENTED_EDGE('',*,*,#41800,.T.);
#59693=ORIENTED_EDGE('',*,*,#41802,.F.);
#59694=ORIENTED_EDGE('',*,*,#41803,.F.);
#59695=ORIENTED_EDGE('',*,*,#41412,.T.);
#59696=ORIENTED_EDGE('',*,*,#41411,.T.);
#59697=ORIENTED_EDGE('',*,*,#41804,.F.);
#59698=ORIENTED_EDGE('',*,*,#41415,.T.);
#59699=ORIENTED_EDGE('',*,*,#41413,.T.);
#59700=ORIENTED_EDGE('',*,*,#41803,.T.);
#59701=ORIENTED_EDGE('',*,*,#41805,.F.);
#59702=ORIENTED_EDGE('',*,*,#41806,.F.);
#59703=ORIENTED_EDGE('',*,*,#41419,.T.);
#59704=ORIENTED_EDGE('',*,*,#41418,.T.);
#59705=ORIENTED_EDGE('',*,*,#41807,.F.);
#59706=ORIENTED_EDGE('',*,*,#41422,.T.);
#59707=ORIENTED_EDGE('',*,*,#41420,.T.);
#59708=ORIENTED_EDGE('',*,*,#41806,.T.);
#59709=ORIENTED_EDGE('',*,*,#41808,.F.);
#59710=ORIENTED_EDGE('',*,*,#41809,.F.);
#59711=ORIENTED_EDGE('',*,*,#41426,.T.);
#59712=ORIENTED_EDGE('',*,*,#41425,.T.);
#59713=ORIENTED_EDGE('',*,*,#41810,.F.);
#59714=ORIENTED_EDGE('',*,*,#41429,.T.);
#59715=ORIENTED_EDGE('',*,*,#41427,.T.);
#59716=ORIENTED_EDGE('',*,*,#41809,.T.);
#59717=ORIENTED_EDGE('',*,*,#41811,.F.);
#59718=ORIENTED_EDGE('',*,*,#41812,.F.);
#59719=ORIENTED_EDGE('',*,*,#41433,.T.);
#59720=ORIENTED_EDGE('',*,*,#41432,.T.);
#59721=ORIENTED_EDGE('',*,*,#41813,.F.);
#59722=ORIENTED_EDGE('',*,*,#41436,.T.);
#59723=ORIENTED_EDGE('',*,*,#41434,.T.);
#59724=ORIENTED_EDGE('',*,*,#41812,.T.);
#59725=ORIENTED_EDGE('',*,*,#41814,.F.);
#59726=ORIENTED_EDGE('',*,*,#41815,.F.);
#59727=ORIENTED_EDGE('',*,*,#41440,.T.);
#59728=ORIENTED_EDGE('',*,*,#41439,.T.);
#59729=ORIENTED_EDGE('',*,*,#41816,.F.);
#59730=ORIENTED_EDGE('',*,*,#41443,.T.);
#59731=ORIENTED_EDGE('',*,*,#41441,.T.);
#59732=ORIENTED_EDGE('',*,*,#41815,.T.);
#59733=ORIENTED_EDGE('',*,*,#41817,.F.);
#59734=ORIENTED_EDGE('',*,*,#41818,.F.);
#59735=ORIENTED_EDGE('',*,*,#34379,.T.);
#59736=ORIENTED_EDGE('',*,*,#41445,.T.);
#59737=ORIENTED_EDGE('',*,*,#41819,.F.);
#59738=ORIENTED_EDGE('',*,*,#41446,.T.);
#59739=ORIENTED_EDGE('',*,*,#34380,.T.);
#59740=ORIENTED_EDGE('',*,*,#41818,.T.);
#59741=ORIENTED_EDGE('',*,*,#41820,.F.);
#59742=ORIENTED_EDGE('',*,*,#41821,.F.);
#59743=ORIENTED_EDGE('',*,*,#41450,.T.);
#59744=ORIENTED_EDGE('',*,*,#41449,.T.);
#59745=ORIENTED_EDGE('',*,*,#41822,.F.);
#59746=ORIENTED_EDGE('',*,*,#41453,.T.);
#59747=ORIENTED_EDGE('',*,*,#41451,.T.);
#59748=ORIENTED_EDGE('',*,*,#41821,.T.);
#59749=ORIENTED_EDGE('',*,*,#41823,.F.);
#59750=ORIENTED_EDGE('',*,*,#41824,.F.);
#59751=ORIENTED_EDGE('',*,*,#41457,.T.);
#59752=ORIENTED_EDGE('',*,*,#41456,.T.);
#59753=ORIENTED_EDGE('',*,*,#41825,.F.);
#59754=ORIENTED_EDGE('',*,*,#41460,.T.);
#59755=ORIENTED_EDGE('',*,*,#41458,.T.);
#59756=ORIENTED_EDGE('',*,*,#41824,.T.);
#59757=ORIENTED_EDGE('',*,*,#41826,.F.);
#59758=ORIENTED_EDGE('',*,*,#41827,.F.);
#59759=ORIENTED_EDGE('',*,*,#41464,.T.);
#59760=ORIENTED_EDGE('',*,*,#41463,.T.);
#59761=ORIENTED_EDGE('',*,*,#41828,.F.);
#59762=ORIENTED_EDGE('',*,*,#41467,.T.);
#59763=ORIENTED_EDGE('',*,*,#41465,.T.);
#59764=ORIENTED_EDGE('',*,*,#41827,.T.);
#59765=ORIENTED_EDGE('',*,*,#41829,.F.);
#59766=ORIENTED_EDGE('',*,*,#41830,.F.);
#59767=ORIENTED_EDGE('',*,*,#41471,.T.);
#59768=ORIENTED_EDGE('',*,*,#41470,.T.);
#59769=ORIENTED_EDGE('',*,*,#41831,.F.);
#59770=ORIENTED_EDGE('',*,*,#41474,.T.);
#59771=ORIENTED_EDGE('',*,*,#41472,.T.);
#59772=ORIENTED_EDGE('',*,*,#41830,.T.);
#59773=ORIENTED_EDGE('',*,*,#41832,.F.);
#59774=ORIENTED_EDGE('',*,*,#41833,.F.);
#59775=ORIENTED_EDGE('',*,*,#41478,.T.);
#59776=ORIENTED_EDGE('',*,*,#41477,.T.);
#59777=ORIENTED_EDGE('',*,*,#41834,.F.);
#59778=ORIENTED_EDGE('',*,*,#41481,.T.);
#59779=ORIENTED_EDGE('',*,*,#41479,.T.);
#59780=ORIENTED_EDGE('',*,*,#41833,.T.);
#59781=ORIENTED_EDGE('',*,*,#41835,.F.);
#59782=ORIENTED_EDGE('',*,*,#41836,.F.);
#59783=ORIENTED_EDGE('',*,*,#41485,.T.);
#59784=ORIENTED_EDGE('',*,*,#41484,.T.);
#59785=ORIENTED_EDGE('',*,*,#41837,.F.);
#59786=ORIENTED_EDGE('',*,*,#41488,.T.);
#59787=ORIENTED_EDGE('',*,*,#41486,.T.);
#59788=ORIENTED_EDGE('',*,*,#41836,.T.);
#59789=ORIENTED_EDGE('',*,*,#41838,.F.);
#59790=ORIENTED_EDGE('',*,*,#41839,.F.);
#59791=ORIENTED_EDGE('',*,*,#41492,.T.);
#59792=ORIENTED_EDGE('',*,*,#41491,.T.);
#59793=ORIENTED_EDGE('',*,*,#41840,.F.);
#59794=ORIENTED_EDGE('',*,*,#41495,.T.);
#59795=ORIENTED_EDGE('',*,*,#41493,.T.);
#59796=ORIENTED_EDGE('',*,*,#41839,.T.);
#59797=ORIENTED_EDGE('',*,*,#41841,.F.);
#59798=ORIENTED_EDGE('',*,*,#41842,.F.);
#59799=ORIENTED_EDGE('',*,*,#41499,.T.);
#59800=ORIENTED_EDGE('',*,*,#41498,.T.);
#59801=ORIENTED_EDGE('',*,*,#41843,.F.);
#59802=ORIENTED_EDGE('',*,*,#41502,.T.);
#59803=ORIENTED_EDGE('',*,*,#41500,.T.);
#59804=ORIENTED_EDGE('',*,*,#41842,.T.);
#59805=ORIENTED_EDGE('',*,*,#41844,.F.);
#59806=ORIENTED_EDGE('',*,*,#41845,.F.);
#59807=ORIENTED_EDGE('',*,*,#41506,.T.);
#59808=ORIENTED_EDGE('',*,*,#41505,.T.);
#59809=ORIENTED_EDGE('',*,*,#41846,.F.);
#59810=ORIENTED_EDGE('',*,*,#41509,.T.);
#59811=ORIENTED_EDGE('',*,*,#41507,.T.);
#59812=ORIENTED_EDGE('',*,*,#41845,.T.);
#59813=ORIENTED_EDGE('',*,*,#41847,.F.);
#59814=ORIENTED_EDGE('',*,*,#41848,.F.);
#59815=ORIENTED_EDGE('',*,*,#41513,.T.);
#59816=ORIENTED_EDGE('',*,*,#41512,.T.);
#59817=ORIENTED_EDGE('',*,*,#41849,.F.);
#59818=ORIENTED_EDGE('',*,*,#41516,.T.);
#59819=ORIENTED_EDGE('',*,*,#41514,.T.);
#59820=ORIENTED_EDGE('',*,*,#41848,.T.);
#59821=ORIENTED_EDGE('',*,*,#41850,.F.);
#59822=ORIENTED_EDGE('',*,*,#41851,.F.);
#59823=ORIENTED_EDGE('',*,*,#41520,.T.);
#59824=ORIENTED_EDGE('',*,*,#41519,.T.);
#59825=ORIENTED_EDGE('',*,*,#41852,.F.);
#59826=ORIENTED_EDGE('',*,*,#41523,.T.);
#59827=ORIENTED_EDGE('',*,*,#41521,.T.);
#59828=ORIENTED_EDGE('',*,*,#41851,.T.);
#59829=ORIENTED_EDGE('',*,*,#41853,.F.);
#59830=ORIENTED_EDGE('',*,*,#41854,.F.);
#59831=ORIENTED_EDGE('',*,*,#41529,.T.);
#59832=ORIENTED_EDGE('',*,*,#41526,.T.);
#59833=ORIENTED_EDGE('',*,*,#41530,.T.);
#59834=ORIENTED_EDGE('',*,*,#41854,.T.);
#59835=ORIENTED_EDGE('',*,*,#41855,.F.);
#59836=ORIENTED_EDGE('',*,*,#41528,.T.);
#59837=ORIENTED_EDGE('',*,*,#41535,.T.);
#59838=ORIENTED_EDGE('',*,*,#41531,.T.);
#59839=ORIENTED_EDGE('',*,*,#41856,.F.);
#59840=ORIENTED_EDGE('',*,*,#41857,.F.);
#59841=ORIENTED_EDGE('',*,*,#41858,.F.);
#59842=ORIENTED_EDGE('',*,*,#41537,.T.);
#59843=ORIENTED_EDGE('',*,*,#41536,.T.);
#59844=ORIENTED_EDGE('',*,*,#41857,.T.);
#59845=ORIENTED_EDGE('',*,*,#41859,.F.);
#59846=ORIENTED_EDGE('',*,*,#41860,.F.);
#59847=ORIENTED_EDGE('',*,*,#41541,.T.);
#59848=ORIENTED_EDGE('',*,*,#41540,.T.);
#59849=ORIENTED_EDGE('',*,*,#41861,.F.);
#59850=ORIENTED_EDGE('',*,*,#41544,.T.);
#59851=ORIENTED_EDGE('',*,*,#41542,.T.);
#59852=ORIENTED_EDGE('',*,*,#41860,.T.);
#59853=ORIENTED_EDGE('',*,*,#41862,.F.);
#59854=ORIENTED_EDGE('',*,*,#41863,.F.);
#59855=ORIENTED_EDGE('',*,*,#41548,.T.);
#59856=ORIENTED_EDGE('',*,*,#41547,.T.);
#59857=ORIENTED_EDGE('',*,*,#41864,.F.);
#59858=ORIENTED_EDGE('',*,*,#41551,.T.);
#59859=ORIENTED_EDGE('',*,*,#41549,.T.);
#59860=ORIENTED_EDGE('',*,*,#41863,.T.);
#59861=ORIENTED_EDGE('',*,*,#41865,.F.);
#59862=ORIENTED_EDGE('',*,*,#41866,.F.);
#59863=ORIENTED_EDGE('',*,*,#41555,.T.);
#59864=ORIENTED_EDGE('',*,*,#41554,.T.);
#59865=ORIENTED_EDGE('',*,*,#41867,.F.);
#59866=ORIENTED_EDGE('',*,*,#41558,.T.);
#59867=ORIENTED_EDGE('',*,*,#41556,.T.);
#59868=ORIENTED_EDGE('',*,*,#41866,.T.);
#59869=ORIENTED_EDGE('',*,*,#41868,.F.);
#59870=ORIENTED_EDGE('',*,*,#41869,.F.);
#59871=ORIENTED_EDGE('',*,*,#41562,.T.);
#59872=ORIENTED_EDGE('',*,*,#41561,.T.);
#59873=ORIENTED_EDGE('',*,*,#41870,.F.);
#59874=ORIENTED_EDGE('',*,*,#41565,.T.);
#59875=ORIENTED_EDGE('',*,*,#41563,.T.);
#59876=ORIENTED_EDGE('',*,*,#41869,.T.);
#59877=ORIENTED_EDGE('',*,*,#41871,.F.);
#59878=ORIENTED_EDGE('',*,*,#41872,.F.);
#59879=ORIENTED_EDGE('',*,*,#41569,.T.);
#59880=ORIENTED_EDGE('',*,*,#41568,.T.);
#59881=ORIENTED_EDGE('',*,*,#41873,.F.);
#59882=ORIENTED_EDGE('',*,*,#41572,.T.);
#59883=ORIENTED_EDGE('',*,*,#41570,.T.);
#59884=ORIENTED_EDGE('',*,*,#41872,.T.);
#59885=ORIENTED_EDGE('',*,*,#41874,.F.);
#59886=ORIENTED_EDGE('',*,*,#41875,.F.);
#59887=ORIENTED_EDGE('',*,*,#41576,.T.);
#59888=ORIENTED_EDGE('',*,*,#41575,.T.);
#59889=ORIENTED_EDGE('',*,*,#41876,.F.);
#59890=ORIENTED_EDGE('',*,*,#41579,.T.);
#59891=ORIENTED_EDGE('',*,*,#41577,.T.);
#59892=ORIENTED_EDGE('',*,*,#41875,.T.);
#59893=ORIENTED_EDGE('',*,*,#41877,.F.);
#59894=ORIENTED_EDGE('',*,*,#41878,.F.);
#59895=ORIENTED_EDGE('',*,*,#41583,.T.);
#59896=ORIENTED_EDGE('',*,*,#41582,.T.);
#59897=ORIENTED_EDGE('',*,*,#41879,.F.);
#59898=ORIENTED_EDGE('',*,*,#41586,.T.);
#59899=ORIENTED_EDGE('',*,*,#41584,.T.);
#59900=ORIENTED_EDGE('',*,*,#41878,.T.);
#59901=ORIENTED_EDGE('',*,*,#41880,.F.);
#59902=ORIENTED_EDGE('',*,*,#41881,.F.);
#59903=ORIENTED_EDGE('',*,*,#41590,.T.);
#59904=ORIENTED_EDGE('',*,*,#41589,.T.);
#59905=ORIENTED_EDGE('',*,*,#41882,.F.);
#59906=ORIENTED_EDGE('',*,*,#41593,.T.);
#59907=ORIENTED_EDGE('',*,*,#41591,.T.);
#59908=ORIENTED_EDGE('',*,*,#41881,.T.);
#59909=ORIENTED_EDGE('',*,*,#41883,.F.);
#59910=ORIENTED_EDGE('',*,*,#41798,.T.);
#59911=ORIENTED_EDGE('',*,*,#41594,.T.);
#59912=ORIENTED_EDGE('',*,*,#41597,.T.);
#59913=ORIENTED_EDGE('',*,*,#41795,.T.);
#59914=ORIENTED_EDGE('',*,*,#41884,.F.);
#59915=ORIENTED_EDGE('',*,*,#41885,.F.);
#59916=ORIENTED_EDGE('',*,*,#41600,.T.);
#59917=ORIENTED_EDGE('',*,*,#41606,.T.);
#59918=ORIENTED_EDGE('',*,*,#41601,.T.);
#59919=ORIENTED_EDGE('',*,*,#41886,.F.);
#59920=ORIENTED_EDGE('',*,*,#41887,.F.);
#59921=ORIENTED_EDGE('',*,*,#41607,.T.);
#59922=ORIENTED_EDGE('',*,*,#41887,.T.);
#59923=ORIENTED_EDGE('',*,*,#41888,.F.);
#59924=ORIENTED_EDGE('',*,*,#41605,.T.);
#59925=ORIENTED_EDGE('',*,*,#41613,.T.);
#59926=ORIENTED_EDGE('',*,*,#41608,.T.);
#59927=ORIENTED_EDGE('',*,*,#41889,.F.);
#59928=ORIENTED_EDGE('',*,*,#41890,.F.);
#59929=ORIENTED_EDGE('',*,*,#41614,.T.);
#59930=ORIENTED_EDGE('',*,*,#41890,.T.);
#59931=ORIENTED_EDGE('',*,*,#41891,.F.);
#59932=ORIENTED_EDGE('',*,*,#41612,.T.);
#59933=ORIENTED_EDGE('',*,*,#41620,.T.);
#59934=ORIENTED_EDGE('',*,*,#41615,.T.);
#59935=ORIENTED_EDGE('',*,*,#41892,.F.);
#59936=ORIENTED_EDGE('',*,*,#41893,.F.);
#59937=ORIENTED_EDGE('',*,*,#41621,.T.);
#59938=ORIENTED_EDGE('',*,*,#41893,.T.);
#59939=ORIENTED_EDGE('',*,*,#41894,.F.);
#59940=ORIENTED_EDGE('',*,*,#41619,.T.);
#59941=ORIENTED_EDGE('',*,*,#41627,.T.);
#59942=ORIENTED_EDGE('',*,*,#41622,.T.);
#59943=ORIENTED_EDGE('',*,*,#41895,.F.);
#59944=ORIENTED_EDGE('',*,*,#41896,.F.);
#59945=ORIENTED_EDGE('',*,*,#41628,.T.);
#59946=ORIENTED_EDGE('',*,*,#41896,.T.);
#59947=ORIENTED_EDGE('',*,*,#41897,.F.);
#59948=ORIENTED_EDGE('',*,*,#41626,.T.);
#59949=ORIENTED_EDGE('',*,*,#41634,.T.);
#59950=ORIENTED_EDGE('',*,*,#41629,.T.);
#59951=ORIENTED_EDGE('',*,*,#41898,.F.);
#59952=ORIENTED_EDGE('',*,*,#41899,.F.);
#59953=ORIENTED_EDGE('',*,*,#41635,.T.);
#59954=ORIENTED_EDGE('',*,*,#41899,.T.);
#59955=ORIENTED_EDGE('',*,*,#41900,.F.);
#59956=ORIENTED_EDGE('',*,*,#41633,.T.);
#59957=ORIENTED_EDGE('',*,*,#41641,.T.);
#59958=ORIENTED_EDGE('',*,*,#41636,.T.);
#59959=ORIENTED_EDGE('',*,*,#41901,.F.);
#59960=ORIENTED_EDGE('',*,*,#41902,.F.);
#59961=ORIENTED_EDGE('',*,*,#41642,.T.);
#59962=ORIENTED_EDGE('',*,*,#41902,.T.);
#59963=ORIENTED_EDGE('',*,*,#41903,.F.);
#59964=ORIENTED_EDGE('',*,*,#41640,.T.);
#59965=ORIENTED_EDGE('',*,*,#41648,.T.);
#59966=ORIENTED_EDGE('',*,*,#41643,.T.);
#59967=ORIENTED_EDGE('',*,*,#41904,.F.);
#59968=ORIENTED_EDGE('',*,*,#41905,.F.);
#59969=ORIENTED_EDGE('',*,*,#41649,.T.);
#59970=ORIENTED_EDGE('',*,*,#41905,.T.);
#59971=ORIENTED_EDGE('',*,*,#41906,.F.);
#59972=ORIENTED_EDGE('',*,*,#41647,.T.);
#59973=ORIENTED_EDGE('',*,*,#41655,.T.);
#59974=ORIENTED_EDGE('',*,*,#41650,.T.);
#59975=ORIENTED_EDGE('',*,*,#41907,.F.);
#59976=ORIENTED_EDGE('',*,*,#41908,.F.);
#59977=ORIENTED_EDGE('',*,*,#41656,.T.);
#59978=ORIENTED_EDGE('',*,*,#41908,.T.);
#59979=ORIENTED_EDGE('',*,*,#41909,.F.);
#59980=ORIENTED_EDGE('',*,*,#41654,.T.);
#59981=ORIENTED_EDGE('',*,*,#41662,.T.);
#59982=ORIENTED_EDGE('',*,*,#41657,.T.);
#59983=ORIENTED_EDGE('',*,*,#41910,.F.);
#59984=ORIENTED_EDGE('',*,*,#41911,.F.);
#59985=ORIENTED_EDGE('',*,*,#41663,.T.);
#59986=ORIENTED_EDGE('',*,*,#41911,.T.);
#59987=ORIENTED_EDGE('',*,*,#41912,.F.);
#59988=ORIENTED_EDGE('',*,*,#41661,.T.);
#59989=ORIENTED_EDGE('',*,*,#41669,.T.);
#59990=ORIENTED_EDGE('',*,*,#41664,.T.);
#59991=ORIENTED_EDGE('',*,*,#41913,.F.);
#59992=ORIENTED_EDGE('',*,*,#41914,.F.);
#59993=ORIENTED_EDGE('',*,*,#41670,.T.);
#59994=ORIENTED_EDGE('',*,*,#41914,.T.);
#59995=ORIENTED_EDGE('',*,*,#41915,.F.);
#59996=ORIENTED_EDGE('',*,*,#41668,.T.);
#59997=ORIENTED_EDGE('',*,*,#41676,.T.);
#59998=ORIENTED_EDGE('',*,*,#41671,.T.);
#59999=ORIENTED_EDGE('',*,*,#41916,.F.);
#60000=ORIENTED_EDGE('',*,*,#41917,.F.);
#60001=ORIENTED_EDGE('',*,*,#41677,.T.);
#60002=ORIENTED_EDGE('',*,*,#41917,.T.);
#60003=ORIENTED_EDGE('',*,*,#41918,.F.);
#60004=ORIENTED_EDGE('',*,*,#41675,.T.);
#60005=ORIENTED_EDGE('',*,*,#41683,.T.);
#60006=ORIENTED_EDGE('',*,*,#41678,.T.);
#60007=ORIENTED_EDGE('',*,*,#41919,.F.);
#60008=ORIENTED_EDGE('',*,*,#41920,.F.);
#60009=ORIENTED_EDGE('',*,*,#41684,.T.);
#60010=ORIENTED_EDGE('',*,*,#41920,.T.);
#60011=ORIENTED_EDGE('',*,*,#41921,.F.);
#60012=ORIENTED_EDGE('',*,*,#41682,.T.);
#60013=ORIENTED_EDGE('',*,*,#41690,.T.);
#60014=ORIENTED_EDGE('',*,*,#41685,.T.);
#60015=ORIENTED_EDGE('',*,*,#41922,.F.);
#60016=ORIENTED_EDGE('',*,*,#41923,.F.);
#60017=ORIENTED_EDGE('',*,*,#41691,.T.);
#60018=ORIENTED_EDGE('',*,*,#41923,.T.);
#60019=ORIENTED_EDGE('',*,*,#41924,.F.);
#60020=ORIENTED_EDGE('',*,*,#41689,.T.);
#60021=ORIENTED_EDGE('',*,*,#34376,.T.);
#60022=ORIENTED_EDGE('',*,*,#41692,.T.);
#60023=ORIENTED_EDGE('',*,*,#41925,.F.);
#60024=ORIENTED_EDGE('',*,*,#41926,.F.);
#60025=ORIENTED_EDGE('',*,*,#34373,.T.);
#60026=ORIENTED_EDGE('',*,*,#41926,.T.);
#60027=ORIENTED_EDGE('',*,*,#41927,.F.);
#60028=ORIENTED_EDGE('',*,*,#41694,.T.);
#60029=ORIENTED_EDGE('',*,*,#41700,.T.);
#60030=ORIENTED_EDGE('',*,*,#41695,.T.);
#60031=ORIENTED_EDGE('',*,*,#41928,.F.);
#60032=ORIENTED_EDGE('',*,*,#41929,.F.);
#60033=ORIENTED_EDGE('',*,*,#41701,.T.);
#60034=ORIENTED_EDGE('',*,*,#41929,.T.);
#60035=ORIENTED_EDGE('',*,*,#41930,.F.);
#60036=ORIENTED_EDGE('',*,*,#41699,.T.);
#60037=ORIENTED_EDGE('',*,*,#41707,.T.);
#60038=ORIENTED_EDGE('',*,*,#41702,.T.);
#60039=ORIENTED_EDGE('',*,*,#41931,.F.);
#60040=ORIENTED_EDGE('',*,*,#41932,.F.);
#60041=ORIENTED_EDGE('',*,*,#41708,.T.);
#60042=ORIENTED_EDGE('',*,*,#41932,.T.);
#60043=ORIENTED_EDGE('',*,*,#41933,.F.);
#60044=ORIENTED_EDGE('',*,*,#41706,.T.);
#60045=ORIENTED_EDGE('',*,*,#41714,.T.);
#60046=ORIENTED_EDGE('',*,*,#41709,.T.);
#60047=ORIENTED_EDGE('',*,*,#41934,.F.);
#60048=ORIENTED_EDGE('',*,*,#41935,.F.);
#60049=ORIENTED_EDGE('',*,*,#41715,.T.);
#60050=ORIENTED_EDGE('',*,*,#41935,.T.);
#60051=ORIENTED_EDGE('',*,*,#41936,.F.);
#60052=ORIENTED_EDGE('',*,*,#41713,.T.);
#60053=ORIENTED_EDGE('',*,*,#41721,.T.);
#60054=ORIENTED_EDGE('',*,*,#41716,.T.);
#60055=ORIENTED_EDGE('',*,*,#41937,.F.);
#60056=ORIENTED_EDGE('',*,*,#41938,.F.);
#60057=ORIENTED_EDGE('',*,*,#41722,.T.);
#60058=ORIENTED_EDGE('',*,*,#41938,.T.);
#60059=ORIENTED_EDGE('',*,*,#41939,.F.);
#60060=ORIENTED_EDGE('',*,*,#41720,.T.);
#60061=ORIENTED_EDGE('',*,*,#41728,.T.);
#60062=ORIENTED_EDGE('',*,*,#41723,.T.);
#60063=ORIENTED_EDGE('',*,*,#41940,.F.);
#60064=ORIENTED_EDGE('',*,*,#41941,.F.);
#60065=ORIENTED_EDGE('',*,*,#41729,.T.);
#60066=ORIENTED_EDGE('',*,*,#41941,.T.);
#60067=ORIENTED_EDGE('',*,*,#41942,.F.);
#60068=ORIENTED_EDGE('',*,*,#41727,.T.);
#60069=ORIENTED_EDGE('',*,*,#41735,.T.);
#60070=ORIENTED_EDGE('',*,*,#41730,.T.);
#60071=ORIENTED_EDGE('',*,*,#41943,.F.);
#60072=ORIENTED_EDGE('',*,*,#41944,.F.);
#60073=ORIENTED_EDGE('',*,*,#41736,.T.);
#60074=ORIENTED_EDGE('',*,*,#41944,.T.);
#60075=ORIENTED_EDGE('',*,*,#41945,.F.);
#60076=ORIENTED_EDGE('',*,*,#41734,.T.);
#60077=ORIENTED_EDGE('',*,*,#41742,.T.);
#60078=ORIENTED_EDGE('',*,*,#41737,.T.);
#60079=ORIENTED_EDGE('',*,*,#41946,.F.);
#60080=ORIENTED_EDGE('',*,*,#41947,.F.);
#60081=ORIENTED_EDGE('',*,*,#41743,.T.);
#60082=ORIENTED_EDGE('',*,*,#41947,.T.);
#60083=ORIENTED_EDGE('',*,*,#41948,.F.);
#60084=ORIENTED_EDGE('',*,*,#41741,.T.);
#60085=ORIENTED_EDGE('',*,*,#41749,.T.);
#60086=ORIENTED_EDGE('',*,*,#41744,.T.);
#60087=ORIENTED_EDGE('',*,*,#41949,.F.);
#60088=ORIENTED_EDGE('',*,*,#41950,.F.);
#60089=ORIENTED_EDGE('',*,*,#41750,.T.);
#60090=ORIENTED_EDGE('',*,*,#41950,.T.);
#60091=ORIENTED_EDGE('',*,*,#41951,.F.);
#60092=ORIENTED_EDGE('',*,*,#41748,.T.);
#60093=ORIENTED_EDGE('',*,*,#41756,.T.);
#60094=ORIENTED_EDGE('',*,*,#41751,.T.);
#60095=ORIENTED_EDGE('',*,*,#41952,.F.);
#60096=ORIENTED_EDGE('',*,*,#41953,.F.);
#60097=ORIENTED_EDGE('',*,*,#41757,.T.);
#60098=ORIENTED_EDGE('',*,*,#41953,.T.);
#60099=ORIENTED_EDGE('',*,*,#41954,.F.);
#60100=ORIENTED_EDGE('',*,*,#41755,.T.);
#60101=ORIENTED_EDGE('',*,*,#41763,.T.);
#60102=ORIENTED_EDGE('',*,*,#41758,.T.);
#60103=ORIENTED_EDGE('',*,*,#41955,.F.);
#60104=ORIENTED_EDGE('',*,*,#41956,.F.);
#60105=ORIENTED_EDGE('',*,*,#41764,.T.);
#60106=ORIENTED_EDGE('',*,*,#41956,.T.);
#60107=ORIENTED_EDGE('',*,*,#41957,.F.);
#60108=ORIENTED_EDGE('',*,*,#41762,.T.);
#60109=ORIENTED_EDGE('',*,*,#41958,.F.);
#60110=ORIENTED_EDGE('',*,*,#41959,.F.);
#60111=ORIENTED_EDGE('',*,*,#41770,.T.);
#60112=ORIENTED_EDGE('',*,*,#41765,.T.);
#60113=ORIENTED_EDGE('',*,*,#41771,.T.);
#60114=ORIENTED_EDGE('',*,*,#41959,.T.);
#60115=ORIENTED_EDGE('',*,*,#41960,.F.);
#60116=ORIENTED_EDGE('',*,*,#41769,.T.);
#60117=ORIENTED_EDGE('',*,*,#41777,.T.);
#60118=ORIENTED_EDGE('',*,*,#41772,.T.);
#60119=ORIENTED_EDGE('',*,*,#41961,.F.);
#60120=ORIENTED_EDGE('',*,*,#41962,.F.);
#60121=ORIENTED_EDGE('',*,*,#41778,.T.);
#60122=ORIENTED_EDGE('',*,*,#41962,.T.);
#60123=ORIENTED_EDGE('',*,*,#41963,.F.);
#60124=ORIENTED_EDGE('',*,*,#41776,.T.);
#60125=ORIENTED_EDGE('',*,*,#41784,.T.);
#60126=ORIENTED_EDGE('',*,*,#41779,.T.);
#60127=ORIENTED_EDGE('',*,*,#41964,.F.);
#60128=ORIENTED_EDGE('',*,*,#41965,.F.);
#60129=ORIENTED_EDGE('',*,*,#41785,.T.);
#60130=ORIENTED_EDGE('',*,*,#41965,.T.);
#60131=ORIENTED_EDGE('',*,*,#41966,.F.);
#60132=ORIENTED_EDGE('',*,*,#41783,.T.);
#60133=ORIENTED_EDGE('',*,*,#41791,.T.);
#60134=ORIENTED_EDGE('',*,*,#41786,.T.);
#60135=ORIENTED_EDGE('',*,*,#41967,.F.);
#60136=ORIENTED_EDGE('',*,*,#41968,.F.);
#60137=ORIENTED_EDGE('',*,*,#41792,.T.);
#60138=ORIENTED_EDGE('',*,*,#41968,.T.);
#60139=ORIENTED_EDGE('',*,*,#41969,.F.);
#60140=ORIENTED_EDGE('',*,*,#41790,.T.);
#60141=ORIENTED_EDGE('',*,*,#41794,.T.);
#60142=ORIENTED_EDGE('',*,*,#41796,.T.);
#60143=ORIENTED_EDGE('',*,*,#41970,.F.);
#60144=ORIENTED_EDGE('',*,*,#41884,.T.);
#60145=ORIENTED_EDGE('',*,*,#41971,.T.);
#60146=ORIENTED_EDGE('',*,*,#41972,.F.);
#60147=ORIENTED_EDGE('',*,*,#41797,.T.);
#60148=ORIENTED_EDGE('',*,*,#41973,.F.);
#60149=ORIENTED_EDGE('',*,*,#41974,.F.);
#60150=ORIENTED_EDGE('',*,*,#41975,.F.);
#60151=ORIENTED_EDGE('',*,*,#41976,.F.);
#60152=ORIENTED_EDGE('',*,*,#41971,.F.);
#60153=ORIENTED_EDGE('',*,*,#41976,.T.);
#60154=ORIENTED_EDGE('',*,*,#41977,.F.);
#60155=ORIENTED_EDGE('',*,*,#41799,.T.);
#60156=ORIENTED_EDGE('',*,*,#41972,.T.);
#60157=ORIENTED_EDGE('',*,*,#41978,.T.);
#60158=ORIENTED_EDGE('',*,*,#41979,.F.);
#60159=ORIENTED_EDGE('',*,*,#41801,.T.);
#60160=ORIENTED_EDGE('',*,*,#41980,.F.);
#60161=ORIENTED_EDGE('',*,*,#41981,.F.);
#60162=ORIENTED_EDGE('',*,*,#41982,.F.);
#60163=ORIENTED_EDGE('',*,*,#41983,.F.);
#60164=ORIENTED_EDGE('',*,*,#41978,.F.);
#60165=ORIENTED_EDGE('',*,*,#41983,.T.);
#60166=ORIENTED_EDGE('',*,*,#41984,.F.);
#60167=ORIENTED_EDGE('',*,*,#41802,.T.);
#60168=ORIENTED_EDGE('',*,*,#41979,.T.);
#60169=ORIENTED_EDGE('',*,*,#41985,.T.);
#60170=ORIENTED_EDGE('',*,*,#41986,.F.);
#60171=ORIENTED_EDGE('',*,*,#41804,.T.);
#60172=ORIENTED_EDGE('',*,*,#41987,.F.);
#60173=ORIENTED_EDGE('',*,*,#41988,.F.);
#60174=ORIENTED_EDGE('',*,*,#41989,.F.);
#60175=ORIENTED_EDGE('',*,*,#41990,.F.);
#60176=ORIENTED_EDGE('',*,*,#41985,.F.);
#60177=ORIENTED_EDGE('',*,*,#41990,.T.);
#60178=ORIENTED_EDGE('',*,*,#41991,.F.);
#60179=ORIENTED_EDGE('',*,*,#41805,.T.);
#60180=ORIENTED_EDGE('',*,*,#41986,.T.);
#60181=ORIENTED_EDGE('',*,*,#41992,.T.);
#60182=ORIENTED_EDGE('',*,*,#41993,.F.);
#60183=ORIENTED_EDGE('',*,*,#41807,.T.);
#60184=ORIENTED_EDGE('',*,*,#41994,.F.);
#60185=ORIENTED_EDGE('',*,*,#41995,.F.);
#60186=ORIENTED_EDGE('',*,*,#41996,.F.);
#60187=ORIENTED_EDGE('',*,*,#41997,.F.);
#60188=ORIENTED_EDGE('',*,*,#41992,.F.);
#60189=ORIENTED_EDGE('',*,*,#41997,.T.);
#60190=ORIENTED_EDGE('',*,*,#41998,.F.);
#60191=ORIENTED_EDGE('',*,*,#41808,.T.);
#60192=ORIENTED_EDGE('',*,*,#41993,.T.);
#60193=ORIENTED_EDGE('',*,*,#41999,.T.);
#60194=ORIENTED_EDGE('',*,*,#42000,.F.);
#60195=ORIENTED_EDGE('',*,*,#41810,.T.);
#60196=ORIENTED_EDGE('',*,*,#42001,.F.);
#60197=ORIENTED_EDGE('',*,*,#42002,.F.);
#60198=ORIENTED_EDGE('',*,*,#42003,.F.);
#60199=ORIENTED_EDGE('',*,*,#42004,.F.);
#60200=ORIENTED_EDGE('',*,*,#41999,.F.);
#60201=ORIENTED_EDGE('',*,*,#42004,.T.);
#60202=ORIENTED_EDGE('',*,*,#42005,.F.);
#60203=ORIENTED_EDGE('',*,*,#41811,.T.);
#60204=ORIENTED_EDGE('',*,*,#42000,.T.);
#60205=ORIENTED_EDGE('',*,*,#42006,.T.);
#60206=ORIENTED_EDGE('',*,*,#42007,.F.);
#60207=ORIENTED_EDGE('',*,*,#41813,.T.);
#60208=ORIENTED_EDGE('',*,*,#42008,.F.);
#60209=ORIENTED_EDGE('',*,*,#42009,.F.);
#60210=ORIENTED_EDGE('',*,*,#42010,.F.);
#60211=ORIENTED_EDGE('',*,*,#42011,.F.);
#60212=ORIENTED_EDGE('',*,*,#42006,.F.);
#60213=ORIENTED_EDGE('',*,*,#42011,.T.);
#60214=ORIENTED_EDGE('',*,*,#42012,.F.);
#60215=ORIENTED_EDGE('',*,*,#41814,.T.);
#60216=ORIENTED_EDGE('',*,*,#42007,.T.);
#60217=ORIENTED_EDGE('',*,*,#42013,.T.);
#60218=ORIENTED_EDGE('',*,*,#42014,.F.);
#60219=ORIENTED_EDGE('',*,*,#41816,.T.);
#60220=ORIENTED_EDGE('',*,*,#42015,.F.);
#60221=ORIENTED_EDGE('',*,*,#42016,.F.);
#60222=ORIENTED_EDGE('',*,*,#42017,.F.);
#60223=ORIENTED_EDGE('',*,*,#42018,.F.);
#60224=ORIENTED_EDGE('',*,*,#42013,.F.);
#60225=ORIENTED_EDGE('',*,*,#42018,.T.);
#60226=ORIENTED_EDGE('',*,*,#42019,.F.);
#60227=ORIENTED_EDGE('',*,*,#41817,.T.);
#60228=ORIENTED_EDGE('',*,*,#42014,.T.);
#60229=ORIENTED_EDGE('',*,*,#42020,.T.);
#60230=ORIENTED_EDGE('',*,*,#42021,.F.);
#60231=ORIENTED_EDGE('',*,*,#41819,.T.);
#60232=ORIENTED_EDGE('',*,*,#42022,.F.);
#60233=ORIENTED_EDGE('',*,*,#42023,.F.);
#60234=ORIENTED_EDGE('',*,*,#42024,.F.);
#60235=ORIENTED_EDGE('',*,*,#42025,.F.);
#60236=ORIENTED_EDGE('',*,*,#42020,.F.);
#60237=ORIENTED_EDGE('',*,*,#42025,.T.);
#60238=ORIENTED_EDGE('',*,*,#42026,.F.);
#60239=ORIENTED_EDGE('',*,*,#41820,.T.);
#60240=ORIENTED_EDGE('',*,*,#42021,.T.);
#60241=ORIENTED_EDGE('',*,*,#42027,.T.);
#60242=ORIENTED_EDGE('',*,*,#42028,.F.);
#60243=ORIENTED_EDGE('',*,*,#41822,.T.);
#60244=ORIENTED_EDGE('',*,*,#42029,.F.);
#60245=ORIENTED_EDGE('',*,*,#42030,.F.);
#60246=ORIENTED_EDGE('',*,*,#42031,.F.);
#60247=ORIENTED_EDGE('',*,*,#42032,.F.);
#60248=ORIENTED_EDGE('',*,*,#42027,.F.);
#60249=ORIENTED_EDGE('',*,*,#42032,.T.);
#60250=ORIENTED_EDGE('',*,*,#42033,.F.);
#60251=ORIENTED_EDGE('',*,*,#41823,.T.);
#60252=ORIENTED_EDGE('',*,*,#42028,.T.);
#60253=ORIENTED_EDGE('',*,*,#42034,.T.);
#60254=ORIENTED_EDGE('',*,*,#42035,.F.);
#60255=ORIENTED_EDGE('',*,*,#41825,.T.);
#60256=ORIENTED_EDGE('',*,*,#42036,.F.);
#60257=ORIENTED_EDGE('',*,*,#42037,.F.);
#60258=ORIENTED_EDGE('',*,*,#42038,.F.);
#60259=ORIENTED_EDGE('',*,*,#42039,.F.);
#60260=ORIENTED_EDGE('',*,*,#42034,.F.);
#60261=ORIENTED_EDGE('',*,*,#42039,.T.);
#60262=ORIENTED_EDGE('',*,*,#42040,.F.);
#60263=ORIENTED_EDGE('',*,*,#41826,.T.);
#60264=ORIENTED_EDGE('',*,*,#42035,.T.);
#60265=ORIENTED_EDGE('',*,*,#42041,.T.);
#60266=ORIENTED_EDGE('',*,*,#42042,.F.);
#60267=ORIENTED_EDGE('',*,*,#41828,.T.);
#60268=ORIENTED_EDGE('',*,*,#42043,.F.);
#60269=ORIENTED_EDGE('',*,*,#42044,.F.);
#60270=ORIENTED_EDGE('',*,*,#42045,.F.);
#60271=ORIENTED_EDGE('',*,*,#42046,.F.);
#60272=ORIENTED_EDGE('',*,*,#42041,.F.);
#60273=ORIENTED_EDGE('',*,*,#42046,.T.);
#60274=ORIENTED_EDGE('',*,*,#42047,.F.);
#60275=ORIENTED_EDGE('',*,*,#41829,.T.);
#60276=ORIENTED_EDGE('',*,*,#42042,.T.);
#60277=ORIENTED_EDGE('',*,*,#42048,.T.);
#60278=ORIENTED_EDGE('',*,*,#42049,.F.);
#60279=ORIENTED_EDGE('',*,*,#41831,.T.);
#60280=ORIENTED_EDGE('',*,*,#42050,.F.);
#60281=ORIENTED_EDGE('',*,*,#42051,.F.);
#60282=ORIENTED_EDGE('',*,*,#42052,.F.);
#60283=ORIENTED_EDGE('',*,*,#42053,.F.);
#60284=ORIENTED_EDGE('',*,*,#42048,.F.);
#60285=ORIENTED_EDGE('',*,*,#42053,.T.);
#60286=ORIENTED_EDGE('',*,*,#42054,.F.);
#60287=ORIENTED_EDGE('',*,*,#41832,.T.);
#60288=ORIENTED_EDGE('',*,*,#42049,.T.);
#60289=ORIENTED_EDGE('',*,*,#42055,.T.);
#60290=ORIENTED_EDGE('',*,*,#42056,.F.);
#60291=ORIENTED_EDGE('',*,*,#41834,.T.);
#60292=ORIENTED_EDGE('',*,*,#42057,.F.);
#60293=ORIENTED_EDGE('',*,*,#42058,.F.);
#60294=ORIENTED_EDGE('',*,*,#42059,.F.);
#60295=ORIENTED_EDGE('',*,*,#42060,.F.);
#60296=ORIENTED_EDGE('',*,*,#42055,.F.);
#60297=ORIENTED_EDGE('',*,*,#42060,.T.);
#60298=ORIENTED_EDGE('',*,*,#42061,.F.);
#60299=ORIENTED_EDGE('',*,*,#41835,.T.);
#60300=ORIENTED_EDGE('',*,*,#42056,.T.);
#60301=ORIENTED_EDGE('',*,*,#42062,.T.);
#60302=ORIENTED_EDGE('',*,*,#42063,.F.);
#60303=ORIENTED_EDGE('',*,*,#41837,.T.);
#60304=ORIENTED_EDGE('',*,*,#42064,.F.);
#60305=ORIENTED_EDGE('',*,*,#42065,.F.);
#60306=ORIENTED_EDGE('',*,*,#42066,.F.);
#60307=ORIENTED_EDGE('',*,*,#42067,.F.);
#60308=ORIENTED_EDGE('',*,*,#42062,.F.);
#60309=ORIENTED_EDGE('',*,*,#42067,.T.);
#60310=ORIENTED_EDGE('',*,*,#42068,.F.);
#60311=ORIENTED_EDGE('',*,*,#41838,.T.);
#60312=ORIENTED_EDGE('',*,*,#42063,.T.);
#60313=ORIENTED_EDGE('',*,*,#34369,.T.);
#60314=ORIENTED_EDGE('',*,*,#42069,.F.);
#60315=ORIENTED_EDGE('',*,*,#41840,.T.);
#60316=ORIENTED_EDGE('',*,*,#42070,.F.);
#60317=ORIENTED_EDGE('',*,*,#34372,.T.);
#60318=ORIENTED_EDGE('',*,*,#42071,.F.);
#60319=ORIENTED_EDGE('',*,*,#41841,.T.);
#60320=ORIENTED_EDGE('',*,*,#42069,.T.);
#60321=ORIENTED_EDGE('',*,*,#42072,.T.);
#60322=ORIENTED_EDGE('',*,*,#42073,.F.);
#60323=ORIENTED_EDGE('',*,*,#41843,.T.);
#60324=ORIENTED_EDGE('',*,*,#42074,.F.);
#60325=ORIENTED_EDGE('',*,*,#42075,.F.);
#60326=ORIENTED_EDGE('',*,*,#42076,.F.);
#60327=ORIENTED_EDGE('',*,*,#42077,.F.);
#60328=ORIENTED_EDGE('',*,*,#42072,.F.);
#60329=ORIENTED_EDGE('',*,*,#42077,.T.);
#60330=ORIENTED_EDGE('',*,*,#42078,.F.);
#60331=ORIENTED_EDGE('',*,*,#41844,.T.);
#60332=ORIENTED_EDGE('',*,*,#42073,.T.);
#60333=ORIENTED_EDGE('',*,*,#42079,.T.);
#60334=ORIENTED_EDGE('',*,*,#42080,.F.);
#60335=ORIENTED_EDGE('',*,*,#41846,.T.);
#60336=ORIENTED_EDGE('',*,*,#42081,.F.);
#60337=ORIENTED_EDGE('',*,*,#42082,.F.);
#60338=ORIENTED_EDGE('',*,*,#42083,.F.);
#60339=ORIENTED_EDGE('',*,*,#42084,.F.);
#60340=ORIENTED_EDGE('',*,*,#42079,.F.);
#60341=ORIENTED_EDGE('',*,*,#42084,.T.);
#60342=ORIENTED_EDGE('',*,*,#42085,.F.);
#60343=ORIENTED_EDGE('',*,*,#41847,.T.);
#60344=ORIENTED_EDGE('',*,*,#42080,.T.);
#60345=ORIENTED_EDGE('',*,*,#42086,.T.);
#60346=ORIENTED_EDGE('',*,*,#42087,.F.);
#60347=ORIENTED_EDGE('',*,*,#41849,.T.);
#60348=ORIENTED_EDGE('',*,*,#42088,.F.);
#60349=ORIENTED_EDGE('',*,*,#42089,.F.);
#60350=ORIENTED_EDGE('',*,*,#42090,.F.);
#60351=ORIENTED_EDGE('',*,*,#42091,.F.);
#60352=ORIENTED_EDGE('',*,*,#42086,.F.);
#60353=ORIENTED_EDGE('',*,*,#42091,.T.);
#60354=ORIENTED_EDGE('',*,*,#42092,.F.);
#60355=ORIENTED_EDGE('',*,*,#41850,.T.);
#60356=ORIENTED_EDGE('',*,*,#42087,.T.);
#60357=ORIENTED_EDGE('',*,*,#42093,.T.);
#60358=ORIENTED_EDGE('',*,*,#42094,.F.);
#60359=ORIENTED_EDGE('',*,*,#41852,.T.);
#60360=ORIENTED_EDGE('',*,*,#42095,.F.);
#60361=ORIENTED_EDGE('',*,*,#42096,.T.);
#60362=ORIENTED_EDGE('',*,*,#42097,.F.);
#60363=ORIENTED_EDGE('',*,*,#41853,.T.);
#60364=ORIENTED_EDGE('',*,*,#42094,.T.);
#60365=ORIENTED_EDGE('',*,*,#42098,.F.);
#60366=ORIENTED_EDGE('',*,*,#42099,.F.);
#60367=ORIENTED_EDGE('',*,*,#42096,.F.);
#60368=ORIENTED_EDGE('',*,*,#42093,.F.);
#60369=ORIENTED_EDGE('',*,*,#41855,.T.);
#60370=ORIENTED_EDGE('',*,*,#42100,.F.);
#60371=ORIENTED_EDGE('',*,*,#42101,.T.);
#60372=ORIENTED_EDGE('',*,*,#42102,.F.);
#60373=ORIENTED_EDGE('',*,*,#42103,.F.);
#60374=ORIENTED_EDGE('',*,*,#42101,.F.);
#60375=ORIENTED_EDGE('',*,*,#42104,.F.);
#60376=ORIENTED_EDGE('',*,*,#42105,.F.);
#60377=ORIENTED_EDGE('',*,*,#41856,.T.);
#60378=ORIENTED_EDGE('',*,*,#42102,.T.);
#60379=ORIENTED_EDGE('',*,*,#42103,.T.);
#60380=ORIENTED_EDGE('',*,*,#42106,.F.);
#60381=ORIENTED_EDGE('',*,*,#42107,.T.);
#60382=ORIENTED_EDGE('',*,*,#42108,.F.);
#60383=ORIENTED_EDGE('',*,*,#41858,.T.);
#60384=ORIENTED_EDGE('',*,*,#42109,.F.);
#60385=ORIENTED_EDGE('',*,*,#42110,.F.);
#60386=ORIENTED_EDGE('',*,*,#42111,.F.);
#60387=ORIENTED_EDGE('',*,*,#42112,.F.);
#60388=ORIENTED_EDGE('',*,*,#42107,.F.);
#60389=ORIENTED_EDGE('',*,*,#42112,.T.);
#60390=ORIENTED_EDGE('',*,*,#42113,.F.);
#60391=ORIENTED_EDGE('',*,*,#41859,.T.);
#60392=ORIENTED_EDGE('',*,*,#42108,.T.);
#60393=ORIENTED_EDGE('',*,*,#42114,.T.);
#60394=ORIENTED_EDGE('',*,*,#42115,.F.);
#60395=ORIENTED_EDGE('',*,*,#41861,.T.);
#60396=ORIENTED_EDGE('',*,*,#42116,.F.);
#60397=ORIENTED_EDGE('',*,*,#42117,.F.);
#60398=ORIENTED_EDGE('',*,*,#42118,.F.);
#60399=ORIENTED_EDGE('',*,*,#42119,.F.);
#60400=ORIENTED_EDGE('',*,*,#42114,.F.);
#60401=ORIENTED_EDGE('',*,*,#42119,.T.);
#60402=ORIENTED_EDGE('',*,*,#42120,.F.);
#60403=ORIENTED_EDGE('',*,*,#41862,.T.);
#60404=ORIENTED_EDGE('',*,*,#42115,.T.);
#60405=ORIENTED_EDGE('',*,*,#42121,.T.);
#60406=ORIENTED_EDGE('',*,*,#42122,.F.);
#60407=ORIENTED_EDGE('',*,*,#41864,.T.);
#60408=ORIENTED_EDGE('',*,*,#42123,.F.);
#60409=ORIENTED_EDGE('',*,*,#42124,.F.);
#60410=ORIENTED_EDGE('',*,*,#42125,.F.);
#60411=ORIENTED_EDGE('',*,*,#42126,.F.);
#60412=ORIENTED_EDGE('',*,*,#42121,.F.);
#60413=ORIENTED_EDGE('',*,*,#42126,.T.);
#60414=ORIENTED_EDGE('',*,*,#42127,.F.);
#60415=ORIENTED_EDGE('',*,*,#41865,.T.);
#60416=ORIENTED_EDGE('',*,*,#42122,.T.);
#60417=ORIENTED_EDGE('',*,*,#42128,.T.);
#60418=ORIENTED_EDGE('',*,*,#42129,.F.);
#60419=ORIENTED_EDGE('',*,*,#41867,.T.);
#60420=ORIENTED_EDGE('',*,*,#42130,.F.);
#60421=ORIENTED_EDGE('',*,*,#42131,.F.);
#60422=ORIENTED_EDGE('',*,*,#42132,.F.);
#60423=ORIENTED_EDGE('',*,*,#42133,.F.);
#60424=ORIENTED_EDGE('',*,*,#42128,.F.);
#60425=ORIENTED_EDGE('',*,*,#42133,.T.);
#60426=ORIENTED_EDGE('',*,*,#42134,.F.);
#60427=ORIENTED_EDGE('',*,*,#41868,.T.);
#60428=ORIENTED_EDGE('',*,*,#42129,.T.);
#60429=ORIENTED_EDGE('',*,*,#42135,.T.);
#60430=ORIENTED_EDGE('',*,*,#42136,.F.);
#60431=ORIENTED_EDGE('',*,*,#41870,.T.);
#60432=ORIENTED_EDGE('',*,*,#42137,.F.);
#60433=ORIENTED_EDGE('',*,*,#42138,.F.);
#60434=ORIENTED_EDGE('',*,*,#42139,.F.);
#60435=ORIENTED_EDGE('',*,*,#42140,.F.);
#60436=ORIENTED_EDGE('',*,*,#42135,.F.);
#60437=ORIENTED_EDGE('',*,*,#42140,.T.);
#60438=ORIENTED_EDGE('',*,*,#42141,.F.);
#60439=ORIENTED_EDGE('',*,*,#41871,.T.);
#60440=ORIENTED_EDGE('',*,*,#42136,.T.);
#60441=ORIENTED_EDGE('',*,*,#42142,.T.);
#60442=ORIENTED_EDGE('',*,*,#42143,.F.);
#60443=ORIENTED_EDGE('',*,*,#41873,.T.);
#60444=ORIENTED_EDGE('',*,*,#42144,.F.);
#60445=ORIENTED_EDGE('',*,*,#42145,.F.);
#60446=ORIENTED_EDGE('',*,*,#42146,.F.);
#60447=ORIENTED_EDGE('',*,*,#42147,.F.);
#60448=ORIENTED_EDGE('',*,*,#42142,.F.);
#60449=ORIENTED_EDGE('',*,*,#42147,.T.);
#60450=ORIENTED_EDGE('',*,*,#42148,.F.);
#60451=ORIENTED_EDGE('',*,*,#41874,.T.);
#60452=ORIENTED_EDGE('',*,*,#42143,.T.);
#60453=ORIENTED_EDGE('',*,*,#42149,.T.);
#60454=ORIENTED_EDGE('',*,*,#42150,.F.);
#60455=ORIENTED_EDGE('',*,*,#41876,.T.);
#60456=ORIENTED_EDGE('',*,*,#42151,.F.);
#60457=ORIENTED_EDGE('',*,*,#42152,.F.);
#60458=ORIENTED_EDGE('',*,*,#42153,.F.);
#60459=ORIENTED_EDGE('',*,*,#42154,.F.);
#60460=ORIENTED_EDGE('',*,*,#42149,.F.);
#60461=ORIENTED_EDGE('',*,*,#42154,.T.);
#60462=ORIENTED_EDGE('',*,*,#42155,.F.);
#60463=ORIENTED_EDGE('',*,*,#41877,.T.);
#60464=ORIENTED_EDGE('',*,*,#42150,.T.);
#60465=ORIENTED_EDGE('',*,*,#42156,.T.);
#60466=ORIENTED_EDGE('',*,*,#42157,.F.);
#60467=ORIENTED_EDGE('',*,*,#41879,.T.);
#60468=ORIENTED_EDGE('',*,*,#42158,.F.);
#60469=ORIENTED_EDGE('',*,*,#42159,.F.);
#60470=ORIENTED_EDGE('',*,*,#42160,.F.);
#60471=ORIENTED_EDGE('',*,*,#42161,.F.);
#60472=ORIENTED_EDGE('',*,*,#42156,.F.);
#60473=ORIENTED_EDGE('',*,*,#42161,.T.);
#60474=ORIENTED_EDGE('',*,*,#42162,.F.);
#60475=ORIENTED_EDGE('',*,*,#41880,.T.);
#60476=ORIENTED_EDGE('',*,*,#42157,.T.);
#60477=ORIENTED_EDGE('',*,*,#42163,.T.);
#60478=ORIENTED_EDGE('',*,*,#42164,.F.);
#60479=ORIENTED_EDGE('',*,*,#41882,.T.);
#60480=ORIENTED_EDGE('',*,*,#42165,.F.);
#60481=ORIENTED_EDGE('',*,*,#42166,.F.);
#60482=ORIENTED_EDGE('',*,*,#42167,.F.);
#60483=ORIENTED_EDGE('',*,*,#42168,.F.);
#60484=ORIENTED_EDGE('',*,*,#42163,.F.);
#60485=ORIENTED_EDGE('',*,*,#42168,.T.);
#60486=ORIENTED_EDGE('',*,*,#42169,.F.);
#60487=ORIENTED_EDGE('',*,*,#41883,.T.);
#60488=ORIENTED_EDGE('',*,*,#42164,.T.);
#60489=ORIENTED_EDGE('',*,*,#41885,.T.);
#60490=ORIENTED_EDGE('',*,*,#42170,.F.);
#60491=ORIENTED_EDGE('',*,*,#42171,.T.);
#60492=ORIENTED_EDGE('',*,*,#42172,.F.);
#60493=ORIENTED_EDGE('',*,*,#42173,.F.);
#60494=ORIENTED_EDGE('',*,*,#42174,.T.);
#60495=ORIENTED_EDGE('',*,*,#42175,.F.);
#60496=ORIENTED_EDGE('',*,*,#41886,.T.);
#60497=ORIENTED_EDGE('',*,*,#42172,.T.);
#60498=ORIENTED_EDGE('',*,*,#42176,.T.);
#60499=ORIENTED_EDGE('',*,*,#42177,.F.);
#60500=ORIENTED_EDGE('',*,*,#42178,.F.);
#60501=ORIENTED_EDGE('',*,*,#42176,.F.);
#60502=ORIENTED_EDGE('',*,*,#42171,.F.);
#60503=ORIENTED_EDGE('',*,*,#42179,.F.);
#60504=ORIENTED_EDGE('',*,*,#42174,.F.);
#60505=ORIENTED_EDGE('',*,*,#41888,.T.);
#60506=ORIENTED_EDGE('',*,*,#42180,.F.);
#60507=ORIENTED_EDGE('',*,*,#42181,.T.);
#60508=ORIENTED_EDGE('',*,*,#42182,.F.);
#60509=ORIENTED_EDGE('',*,*,#42183,.F.);
#60510=ORIENTED_EDGE('',*,*,#42184,.T.);
#60511=ORIENTED_EDGE('',*,*,#42185,.F.);
#60512=ORIENTED_EDGE('',*,*,#41889,.T.);
#60513=ORIENTED_EDGE('',*,*,#42182,.T.);
#60514=ORIENTED_EDGE('',*,*,#42186,.T.);
#60515=ORIENTED_EDGE('',*,*,#42187,.F.);
#60516=ORIENTED_EDGE('',*,*,#42188,.F.);
#60517=ORIENTED_EDGE('',*,*,#42186,.F.);
#60518=ORIENTED_EDGE('',*,*,#42181,.F.);
#60519=ORIENTED_EDGE('',*,*,#42189,.F.);
#60520=ORIENTED_EDGE('',*,*,#42184,.F.);
#60521=ORIENTED_EDGE('',*,*,#41891,.T.);
#60522=ORIENTED_EDGE('',*,*,#42190,.F.);
#60523=ORIENTED_EDGE('',*,*,#42191,.T.);
#60524=ORIENTED_EDGE('',*,*,#42192,.F.);
#60525=ORIENTED_EDGE('',*,*,#42193,.F.);
#60526=ORIENTED_EDGE('',*,*,#42194,.T.);
#60527=ORIENTED_EDGE('',*,*,#42195,.F.);
#60528=ORIENTED_EDGE('',*,*,#41892,.T.);
#60529=ORIENTED_EDGE('',*,*,#42192,.T.);
#60530=ORIENTED_EDGE('',*,*,#42196,.T.);
#60531=ORIENTED_EDGE('',*,*,#42197,.F.);
#60532=ORIENTED_EDGE('',*,*,#42198,.F.);
#60533=ORIENTED_EDGE('',*,*,#42196,.F.);
#60534=ORIENTED_EDGE('',*,*,#42191,.F.);
#60535=ORIENTED_EDGE('',*,*,#42199,.F.);
#60536=ORIENTED_EDGE('',*,*,#42194,.F.);
#60537=ORIENTED_EDGE('',*,*,#41894,.T.);
#60538=ORIENTED_EDGE('',*,*,#42200,.F.);
#60539=ORIENTED_EDGE('',*,*,#42201,.T.);
#60540=ORIENTED_EDGE('',*,*,#42202,.F.);
#60541=ORIENTED_EDGE('',*,*,#42203,.F.);
#60542=ORIENTED_EDGE('',*,*,#42204,.T.);
#60543=ORIENTED_EDGE('',*,*,#42205,.F.);
#60544=ORIENTED_EDGE('',*,*,#41895,.T.);
#60545=ORIENTED_EDGE('',*,*,#42202,.T.);
#60546=ORIENTED_EDGE('',*,*,#42206,.T.);
#60547=ORIENTED_EDGE('',*,*,#42207,.F.);
#60548=ORIENTED_EDGE('',*,*,#42208,.F.);
#60549=ORIENTED_EDGE('',*,*,#42206,.F.);
#60550=ORIENTED_EDGE('',*,*,#42201,.F.);
#60551=ORIENTED_EDGE('',*,*,#42209,.F.);
#60552=ORIENTED_EDGE('',*,*,#42204,.F.);
#60553=ORIENTED_EDGE('',*,*,#41897,.T.);
#60554=ORIENTED_EDGE('',*,*,#42210,.F.);
#60555=ORIENTED_EDGE('',*,*,#42211,.T.);
#60556=ORIENTED_EDGE('',*,*,#42212,.F.);
#60557=ORIENTED_EDGE('',*,*,#42213,.F.);
#60558=ORIENTED_EDGE('',*,*,#42214,.T.);
#60559=ORIENTED_EDGE('',*,*,#42215,.F.);
#60560=ORIENTED_EDGE('',*,*,#41898,.T.);
#60561=ORIENTED_EDGE('',*,*,#42212,.T.);
#60562=ORIENTED_EDGE('',*,*,#42216,.T.);
#60563=ORIENTED_EDGE('',*,*,#42217,.F.);
#60564=ORIENTED_EDGE('',*,*,#42218,.F.);
#60565=ORIENTED_EDGE('',*,*,#42216,.F.);
#60566=ORIENTED_EDGE('',*,*,#42211,.F.);
#60567=ORIENTED_EDGE('',*,*,#42219,.F.);
#60568=ORIENTED_EDGE('',*,*,#42214,.F.);
#60569=ORIENTED_EDGE('',*,*,#41900,.T.);
#60570=ORIENTED_EDGE('',*,*,#42220,.F.);
#60571=ORIENTED_EDGE('',*,*,#42221,.T.);
#60572=ORIENTED_EDGE('',*,*,#42222,.F.);
#60573=ORIENTED_EDGE('',*,*,#42223,.F.);
#60574=ORIENTED_EDGE('',*,*,#42224,.T.);
#60575=ORIENTED_EDGE('',*,*,#42225,.F.);
#60576=ORIENTED_EDGE('',*,*,#41901,.T.);
#60577=ORIENTED_EDGE('',*,*,#42222,.T.);
#60578=ORIENTED_EDGE('',*,*,#42226,.T.);
#60579=ORIENTED_EDGE('',*,*,#42227,.F.);
#60580=ORIENTED_EDGE('',*,*,#42228,.F.);
#60581=ORIENTED_EDGE('',*,*,#42226,.F.);
#60582=ORIENTED_EDGE('',*,*,#42221,.F.);
#60583=ORIENTED_EDGE('',*,*,#42229,.F.);
#60584=ORIENTED_EDGE('',*,*,#42224,.F.);
#60585=ORIENTED_EDGE('',*,*,#41903,.T.);
#60586=ORIENTED_EDGE('',*,*,#42230,.F.);
#60587=ORIENTED_EDGE('',*,*,#42231,.T.);
#60588=ORIENTED_EDGE('',*,*,#42232,.F.);
#60589=ORIENTED_EDGE('',*,*,#42233,.F.);
#60590=ORIENTED_EDGE('',*,*,#42234,.T.);
#60591=ORIENTED_EDGE('',*,*,#42235,.F.);
#60592=ORIENTED_EDGE('',*,*,#41904,.T.);
#60593=ORIENTED_EDGE('',*,*,#42232,.T.);
#60594=ORIENTED_EDGE('',*,*,#42236,.T.);
#60595=ORIENTED_EDGE('',*,*,#42237,.F.);
#60596=ORIENTED_EDGE('',*,*,#42238,.F.);
#60597=ORIENTED_EDGE('',*,*,#42236,.F.);
#60598=ORIENTED_EDGE('',*,*,#42231,.F.);
#60599=ORIENTED_EDGE('',*,*,#42239,.F.);
#60600=ORIENTED_EDGE('',*,*,#42234,.F.);
#60601=ORIENTED_EDGE('',*,*,#41906,.T.);
#60602=ORIENTED_EDGE('',*,*,#42240,.F.);
#60603=ORIENTED_EDGE('',*,*,#42241,.T.);
#60604=ORIENTED_EDGE('',*,*,#42242,.F.);
#60605=ORIENTED_EDGE('',*,*,#42243,.F.);
#60606=ORIENTED_EDGE('',*,*,#42244,.T.);
#60607=ORIENTED_EDGE('',*,*,#42245,.F.);
#60608=ORIENTED_EDGE('',*,*,#41907,.T.);
#60609=ORIENTED_EDGE('',*,*,#42242,.T.);
#60610=ORIENTED_EDGE('',*,*,#42246,.T.);
#60611=ORIENTED_EDGE('',*,*,#42247,.F.);
#60612=ORIENTED_EDGE('',*,*,#42248,.F.);
#60613=ORIENTED_EDGE('',*,*,#42246,.F.);
#60614=ORIENTED_EDGE('',*,*,#42241,.F.);
#60615=ORIENTED_EDGE('',*,*,#42249,.F.);
#60616=ORIENTED_EDGE('',*,*,#42244,.F.);
#60617=ORIENTED_EDGE('',*,*,#41909,.T.);
#60618=ORIENTED_EDGE('',*,*,#42250,.F.);
#60619=ORIENTED_EDGE('',*,*,#42251,.T.);
#60620=ORIENTED_EDGE('',*,*,#42252,.F.);
#60621=ORIENTED_EDGE('',*,*,#42253,.F.);
#60622=ORIENTED_EDGE('',*,*,#42254,.T.);
#60623=ORIENTED_EDGE('',*,*,#42255,.F.);
#60624=ORIENTED_EDGE('',*,*,#41910,.T.);
#60625=ORIENTED_EDGE('',*,*,#42252,.T.);
#60626=ORIENTED_EDGE('',*,*,#42256,.T.);
#60627=ORIENTED_EDGE('',*,*,#42257,.F.);
#60628=ORIENTED_EDGE('',*,*,#42258,.F.);
#60629=ORIENTED_EDGE('',*,*,#42256,.F.);
#60630=ORIENTED_EDGE('',*,*,#42251,.F.);
#60631=ORIENTED_EDGE('',*,*,#42259,.F.);
#60632=ORIENTED_EDGE('',*,*,#42254,.F.);
#60633=ORIENTED_EDGE('',*,*,#41912,.T.);
#60634=ORIENTED_EDGE('',*,*,#42260,.F.);
#60635=ORIENTED_EDGE('',*,*,#42261,.T.);
#60636=ORIENTED_EDGE('',*,*,#42262,.F.);
#60637=ORIENTED_EDGE('',*,*,#42263,.F.);
#60638=ORIENTED_EDGE('',*,*,#42264,.T.);
#60639=ORIENTED_EDGE('',*,*,#42265,.F.);
#60640=ORIENTED_EDGE('',*,*,#41913,.T.);
#60641=ORIENTED_EDGE('',*,*,#42262,.T.);
#60642=ORIENTED_EDGE('',*,*,#42266,.T.);
#60643=ORIENTED_EDGE('',*,*,#42267,.F.);
#60644=ORIENTED_EDGE('',*,*,#42268,.F.);
#60645=ORIENTED_EDGE('',*,*,#42266,.F.);
#60646=ORIENTED_EDGE('',*,*,#42261,.F.);
#60647=ORIENTED_EDGE('',*,*,#42269,.F.);
#60648=ORIENTED_EDGE('',*,*,#42264,.F.);
#60649=ORIENTED_EDGE('',*,*,#41915,.T.);
#60650=ORIENTED_EDGE('',*,*,#42270,.F.);
#60651=ORIENTED_EDGE('',*,*,#42271,.T.);
#60652=ORIENTED_EDGE('',*,*,#42272,.F.);
#60653=ORIENTED_EDGE('',*,*,#42273,.F.);
#60654=ORIENTED_EDGE('',*,*,#42274,.T.);
#60655=ORIENTED_EDGE('',*,*,#42275,.F.);
#60656=ORIENTED_EDGE('',*,*,#41916,.T.);
#60657=ORIENTED_EDGE('',*,*,#42272,.T.);
#60658=ORIENTED_EDGE('',*,*,#42276,.T.);
#60659=ORIENTED_EDGE('',*,*,#42277,.F.);
#60660=ORIENTED_EDGE('',*,*,#42278,.F.);
#60661=ORIENTED_EDGE('',*,*,#42276,.F.);
#60662=ORIENTED_EDGE('',*,*,#42271,.F.);
#60663=ORIENTED_EDGE('',*,*,#42279,.F.);
#60664=ORIENTED_EDGE('',*,*,#42274,.F.);
#60665=ORIENTED_EDGE('',*,*,#41918,.T.);
#60666=ORIENTED_EDGE('',*,*,#42280,.F.);
#60667=ORIENTED_EDGE('',*,*,#42281,.T.);
#60668=ORIENTED_EDGE('',*,*,#42282,.F.);
#60669=ORIENTED_EDGE('',*,*,#42283,.F.);
#60670=ORIENTED_EDGE('',*,*,#42284,.T.);
#60671=ORIENTED_EDGE('',*,*,#42285,.F.);
#60672=ORIENTED_EDGE('',*,*,#41919,.T.);
#60673=ORIENTED_EDGE('',*,*,#42282,.T.);
#60674=ORIENTED_EDGE('',*,*,#42286,.T.);
#60675=ORIENTED_EDGE('',*,*,#42287,.F.);
#60676=ORIENTED_EDGE('',*,*,#42288,.F.);
#60677=ORIENTED_EDGE('',*,*,#42286,.F.);
#60678=ORIENTED_EDGE('',*,*,#42281,.F.);
#60679=ORIENTED_EDGE('',*,*,#42289,.F.);
#60680=ORIENTED_EDGE('',*,*,#42284,.F.);
#60681=ORIENTED_EDGE('',*,*,#41921,.T.);
#60682=ORIENTED_EDGE('',*,*,#42290,.F.);
#60683=ORIENTED_EDGE('',*,*,#42291,.T.);
#60684=ORIENTED_EDGE('',*,*,#42292,.F.);
#60685=ORIENTED_EDGE('',*,*,#42293,.F.);
#60686=ORIENTED_EDGE('',*,*,#42294,.T.);
#60687=ORIENTED_EDGE('',*,*,#42295,.F.);
#60688=ORIENTED_EDGE('',*,*,#41922,.T.);
#60689=ORIENTED_EDGE('',*,*,#42292,.T.);
#60690=ORIENTED_EDGE('',*,*,#42296,.T.);
#60691=ORIENTED_EDGE('',*,*,#42297,.F.);
#60692=ORIENTED_EDGE('',*,*,#42298,.F.);
#60693=ORIENTED_EDGE('',*,*,#42296,.F.);
#60694=ORIENTED_EDGE('',*,*,#42291,.F.);
#60695=ORIENTED_EDGE('',*,*,#42299,.F.);
#60696=ORIENTED_EDGE('',*,*,#42294,.F.);
#60697=ORIENTED_EDGE('',*,*,#41924,.T.);
#60698=ORIENTED_EDGE('',*,*,#42300,.F.);
#60699=ORIENTED_EDGE('',*,*,#42301,.T.);
#60700=ORIENTED_EDGE('',*,*,#42302,.F.);
#60701=ORIENTED_EDGE('',*,*,#42303,.F.);
#60702=ORIENTED_EDGE('',*,*,#42304,.T.);
#60703=ORIENTED_EDGE('',*,*,#42305,.F.);
#60704=ORIENTED_EDGE('',*,*,#41925,.T.);
#60705=ORIENTED_EDGE('',*,*,#42302,.T.);
#60706=ORIENTED_EDGE('',*,*,#42306,.T.);
#60707=ORIENTED_EDGE('',*,*,#42307,.F.);
#60708=ORIENTED_EDGE('',*,*,#42308,.F.);
#60709=ORIENTED_EDGE('',*,*,#42306,.F.);
#60710=ORIENTED_EDGE('',*,*,#42301,.F.);
#60711=ORIENTED_EDGE('',*,*,#42309,.F.);
#60712=ORIENTED_EDGE('',*,*,#42304,.F.);
#60713=ORIENTED_EDGE('',*,*,#41927,.T.);
#60714=ORIENTED_EDGE('',*,*,#42310,.F.);
#60715=ORIENTED_EDGE('',*,*,#42311,.T.);
#60716=ORIENTED_EDGE('',*,*,#42312,.F.);
#60717=ORIENTED_EDGE('',*,*,#42313,.F.);
#60718=ORIENTED_EDGE('',*,*,#42314,.T.);
#60719=ORIENTED_EDGE('',*,*,#42315,.F.);
#60720=ORIENTED_EDGE('',*,*,#41928,.T.);
#60721=ORIENTED_EDGE('',*,*,#42312,.T.);
#60722=ORIENTED_EDGE('',*,*,#42316,.T.);
#60723=ORIENTED_EDGE('',*,*,#42317,.F.);
#60724=ORIENTED_EDGE('',*,*,#42318,.F.);
#60725=ORIENTED_EDGE('',*,*,#42316,.F.);
#60726=ORIENTED_EDGE('',*,*,#42311,.F.);
#60727=ORIENTED_EDGE('',*,*,#42319,.F.);
#60728=ORIENTED_EDGE('',*,*,#42314,.F.);
#60729=ORIENTED_EDGE('',*,*,#41930,.T.);
#60730=ORIENTED_EDGE('',*,*,#42320,.F.);
#60731=ORIENTED_EDGE('',*,*,#42321,.T.);
#60732=ORIENTED_EDGE('',*,*,#42322,.F.);
#60733=ORIENTED_EDGE('',*,*,#42323,.F.);
#60734=ORIENTED_EDGE('',*,*,#42324,.T.);
#60735=ORIENTED_EDGE('',*,*,#42325,.F.);
#60736=ORIENTED_EDGE('',*,*,#41931,.T.);
#60737=ORIENTED_EDGE('',*,*,#42322,.T.);
#60738=ORIENTED_EDGE('',*,*,#42326,.T.);
#60739=ORIENTED_EDGE('',*,*,#42327,.F.);
#60740=ORIENTED_EDGE('',*,*,#42328,.F.);
#60741=ORIENTED_EDGE('',*,*,#42326,.F.);
#60742=ORIENTED_EDGE('',*,*,#42321,.F.);
#60743=ORIENTED_EDGE('',*,*,#42329,.F.);
#60744=ORIENTED_EDGE('',*,*,#42324,.F.);
#60745=ORIENTED_EDGE('',*,*,#41933,.T.);
#60746=ORIENTED_EDGE('',*,*,#42330,.F.);
#60747=ORIENTED_EDGE('',*,*,#42331,.T.);
#60748=ORIENTED_EDGE('',*,*,#42332,.F.);
#60749=ORIENTED_EDGE('',*,*,#42333,.F.);
#60750=ORIENTED_EDGE('',*,*,#42334,.T.);
#60751=ORIENTED_EDGE('',*,*,#42335,.F.);
#60752=ORIENTED_EDGE('',*,*,#41934,.T.);
#60753=ORIENTED_EDGE('',*,*,#42332,.T.);
#60754=ORIENTED_EDGE('',*,*,#42336,.T.);
#60755=ORIENTED_EDGE('',*,*,#42337,.F.);
#60756=ORIENTED_EDGE('',*,*,#42338,.F.);
#60757=ORIENTED_EDGE('',*,*,#42336,.F.);
#60758=ORIENTED_EDGE('',*,*,#42331,.F.);
#60759=ORIENTED_EDGE('',*,*,#42339,.F.);
#60760=ORIENTED_EDGE('',*,*,#42334,.F.);
#60761=ORIENTED_EDGE('',*,*,#41936,.T.);
#60762=ORIENTED_EDGE('',*,*,#42340,.F.);
#60763=ORIENTED_EDGE('',*,*,#42341,.T.);
#60764=ORIENTED_EDGE('',*,*,#42342,.F.);
#60765=ORIENTED_EDGE('',*,*,#42343,.F.);
#60766=ORIENTED_EDGE('',*,*,#42344,.T.);
#60767=ORIENTED_EDGE('',*,*,#42345,.F.);
#60768=ORIENTED_EDGE('',*,*,#41937,.T.);
#60769=ORIENTED_EDGE('',*,*,#42342,.T.);
#60770=ORIENTED_EDGE('',*,*,#42346,.T.);
#60771=ORIENTED_EDGE('',*,*,#42347,.F.);
#60772=ORIENTED_EDGE('',*,*,#42348,.F.);
#60773=ORIENTED_EDGE('',*,*,#42346,.F.);
#60774=ORIENTED_EDGE('',*,*,#42341,.F.);
#60775=ORIENTED_EDGE('',*,*,#42349,.F.);
#60776=ORIENTED_EDGE('',*,*,#42344,.F.);
#60777=ORIENTED_EDGE('',*,*,#41939,.T.);
#60778=ORIENTED_EDGE('',*,*,#42350,.F.);
#60779=ORIENTED_EDGE('',*,*,#42351,.T.);
#60780=ORIENTED_EDGE('',*,*,#42352,.F.);
#60781=ORIENTED_EDGE('',*,*,#42353,.F.);
#60782=ORIENTED_EDGE('',*,*,#42354,.T.);
#60783=ORIENTED_EDGE('',*,*,#42355,.F.);
#60784=ORIENTED_EDGE('',*,*,#41940,.T.);
#60785=ORIENTED_EDGE('',*,*,#42352,.T.);
#60786=ORIENTED_EDGE('',*,*,#42356,.T.);
#60787=ORIENTED_EDGE('',*,*,#42357,.F.);
#60788=ORIENTED_EDGE('',*,*,#42358,.F.);
#60789=ORIENTED_EDGE('',*,*,#42356,.F.);
#60790=ORIENTED_EDGE('',*,*,#42351,.F.);
#60791=ORIENTED_EDGE('',*,*,#42359,.F.);
#60792=ORIENTED_EDGE('',*,*,#42354,.F.);
#60793=ORIENTED_EDGE('',*,*,#41942,.T.);
#60794=ORIENTED_EDGE('',*,*,#42360,.F.);
#60795=ORIENTED_EDGE('',*,*,#42361,.T.);
#60796=ORIENTED_EDGE('',*,*,#42362,.F.);
#60797=ORIENTED_EDGE('',*,*,#42363,.F.);
#60798=ORIENTED_EDGE('',*,*,#42364,.T.);
#60799=ORIENTED_EDGE('',*,*,#42365,.F.);
#60800=ORIENTED_EDGE('',*,*,#41943,.T.);
#60801=ORIENTED_EDGE('',*,*,#42362,.T.);
#60802=ORIENTED_EDGE('',*,*,#42366,.T.);
#60803=ORIENTED_EDGE('',*,*,#42367,.F.);
#60804=ORIENTED_EDGE('',*,*,#42368,.F.);
#60805=ORIENTED_EDGE('',*,*,#42366,.F.);
#60806=ORIENTED_EDGE('',*,*,#42361,.F.);
#60807=ORIENTED_EDGE('',*,*,#42369,.F.);
#60808=ORIENTED_EDGE('',*,*,#42364,.F.);
#60809=ORIENTED_EDGE('',*,*,#41945,.T.);
#60810=ORIENTED_EDGE('',*,*,#42370,.F.);
#60811=ORIENTED_EDGE('',*,*,#42371,.T.);
#60812=ORIENTED_EDGE('',*,*,#42372,.F.);
#60813=ORIENTED_EDGE('',*,*,#42373,.F.);
#60814=ORIENTED_EDGE('',*,*,#42374,.T.);
#60815=ORIENTED_EDGE('',*,*,#42375,.F.);
#60816=ORIENTED_EDGE('',*,*,#41946,.T.);
#60817=ORIENTED_EDGE('',*,*,#42372,.T.);
#60818=ORIENTED_EDGE('',*,*,#42376,.T.);
#60819=ORIENTED_EDGE('',*,*,#42377,.F.);
#60820=ORIENTED_EDGE('',*,*,#42378,.F.);
#60821=ORIENTED_EDGE('',*,*,#42376,.F.);
#60822=ORIENTED_EDGE('',*,*,#42371,.F.);
#60823=ORIENTED_EDGE('',*,*,#42379,.F.);
#60824=ORIENTED_EDGE('',*,*,#42374,.F.);
#60825=ORIENTED_EDGE('',*,*,#41948,.T.);
#60826=ORIENTED_EDGE('',*,*,#42380,.F.);
#60827=ORIENTED_EDGE('',*,*,#34365,.T.);
#60828=ORIENTED_EDGE('',*,*,#42381,.F.);
#60829=ORIENTED_EDGE('',*,*,#41949,.T.);
#60830=ORIENTED_EDGE('',*,*,#42381,.T.);
#60831=ORIENTED_EDGE('',*,*,#34364,.T.);
#60832=ORIENTED_EDGE('',*,*,#42382,.F.);
#60833=ORIENTED_EDGE('',*,*,#41951,.T.);
#60834=ORIENTED_EDGE('',*,*,#42383,.F.);
#60835=ORIENTED_EDGE('',*,*,#42384,.T.);
#60836=ORIENTED_EDGE('',*,*,#42385,.F.);
#60837=ORIENTED_EDGE('',*,*,#42386,.F.);
#60838=ORIENTED_EDGE('',*,*,#42387,.T.);
#60839=ORIENTED_EDGE('',*,*,#42388,.F.);
#60840=ORIENTED_EDGE('',*,*,#41952,.T.);
#60841=ORIENTED_EDGE('',*,*,#42385,.T.);
#60842=ORIENTED_EDGE('',*,*,#42389,.T.);
#60843=ORIENTED_EDGE('',*,*,#42390,.F.);
#60844=ORIENTED_EDGE('',*,*,#42391,.F.);
#60845=ORIENTED_EDGE('',*,*,#42389,.F.);
#60846=ORIENTED_EDGE('',*,*,#42384,.F.);
#60847=ORIENTED_EDGE('',*,*,#42392,.F.);
#60848=ORIENTED_EDGE('',*,*,#42387,.F.);
#60849=ORIENTED_EDGE('',*,*,#41954,.T.);
#60850=ORIENTED_EDGE('',*,*,#42393,.F.);
#60851=ORIENTED_EDGE('',*,*,#42394,.T.);
#60852=ORIENTED_EDGE('',*,*,#42395,.F.);
#60853=ORIENTED_EDGE('',*,*,#42396,.F.);
#60854=ORIENTED_EDGE('',*,*,#42397,.T.);
#60855=ORIENTED_EDGE('',*,*,#42398,.F.);
#60856=ORIENTED_EDGE('',*,*,#41955,.T.);
#60857=ORIENTED_EDGE('',*,*,#42395,.T.);
#60858=ORIENTED_EDGE('',*,*,#42399,.T.);
#60859=ORIENTED_EDGE('',*,*,#42400,.F.);
#60860=ORIENTED_EDGE('',*,*,#42401,.F.);
#60861=ORIENTED_EDGE('',*,*,#42399,.F.);
#60862=ORIENTED_EDGE('',*,*,#42394,.F.);
#60863=ORIENTED_EDGE('',*,*,#42402,.F.);
#60864=ORIENTED_EDGE('',*,*,#42397,.F.);
#60865=ORIENTED_EDGE('',*,*,#41957,.T.);
#60866=ORIENTED_EDGE('',*,*,#42403,.F.);
#60867=ORIENTED_EDGE('',*,*,#42404,.T.);
#60868=ORIENTED_EDGE('',*,*,#42405,.F.);
#60869=ORIENTED_EDGE('',*,*,#42406,.F.);
#60870=ORIENTED_EDGE('',*,*,#42407,.F.);
#60871=ORIENTED_EDGE('',*,*,#42408,.T.);
#60872=ORIENTED_EDGE('',*,*,#42409,.T.);
#60873=ORIENTED_EDGE('',*,*,#42410,.F.);
#60874=ORIENTED_EDGE('',*,*,#41958,.T.);
#60875=ORIENTED_EDGE('',*,*,#42405,.T.);
#60876=ORIENTED_EDGE('',*,*,#42411,.F.);
#60877=ORIENTED_EDGE('',*,*,#42409,.F.);
#60878=ORIENTED_EDGE('',*,*,#42404,.F.);
#60879=ORIENTED_EDGE('',*,*,#42412,.F.);
#60880=ORIENTED_EDGE('',*,*,#42408,.F.);
#60881=ORIENTED_EDGE('',*,*,#41960,.T.);
#60882=ORIENTED_EDGE('',*,*,#42413,.F.);
#60883=ORIENTED_EDGE('',*,*,#42414,.T.);
#60884=ORIENTED_EDGE('',*,*,#42415,.F.);
#60885=ORIENTED_EDGE('',*,*,#42416,.F.);
#60886=ORIENTED_EDGE('',*,*,#42417,.T.);
#60887=ORIENTED_EDGE('',*,*,#42418,.F.);
#60888=ORIENTED_EDGE('',*,*,#41961,.T.);
#60889=ORIENTED_EDGE('',*,*,#42415,.T.);
#60890=ORIENTED_EDGE('',*,*,#42419,.T.);
#60891=ORIENTED_EDGE('',*,*,#42420,.F.);
#60892=ORIENTED_EDGE('',*,*,#42421,.F.);
#60893=ORIENTED_EDGE('',*,*,#42419,.F.);
#60894=ORIENTED_EDGE('',*,*,#42414,.F.);
#60895=ORIENTED_EDGE('',*,*,#42422,.F.);
#60896=ORIENTED_EDGE('',*,*,#42417,.F.);
#60897=ORIENTED_EDGE('',*,*,#41963,.T.);
#60898=ORIENTED_EDGE('',*,*,#42423,.F.);
#60899=ORIENTED_EDGE('',*,*,#42424,.T.);
#60900=ORIENTED_EDGE('',*,*,#42425,.F.);
#60901=ORIENTED_EDGE('',*,*,#42426,.F.);
#60902=ORIENTED_EDGE('',*,*,#42427,.T.);
#60903=ORIENTED_EDGE('',*,*,#42428,.F.);
#60904=ORIENTED_EDGE('',*,*,#41964,.T.);
#60905=ORIENTED_EDGE('',*,*,#42425,.T.);
#60906=ORIENTED_EDGE('',*,*,#42429,.T.);
#60907=ORIENTED_EDGE('',*,*,#42430,.F.);
#60908=ORIENTED_EDGE('',*,*,#42431,.F.);
#60909=ORIENTED_EDGE('',*,*,#42429,.F.);
#60910=ORIENTED_EDGE('',*,*,#42424,.F.);
#60911=ORIENTED_EDGE('',*,*,#42432,.F.);
#60912=ORIENTED_EDGE('',*,*,#42427,.F.);
#60913=ORIENTED_EDGE('',*,*,#41966,.T.);
#60914=ORIENTED_EDGE('',*,*,#42433,.F.);
#60915=ORIENTED_EDGE('',*,*,#42434,.T.);
#60916=ORIENTED_EDGE('',*,*,#42435,.F.);
#60917=ORIENTED_EDGE('',*,*,#42436,.F.);
#60918=ORIENTED_EDGE('',*,*,#42437,.T.);
#60919=ORIENTED_EDGE('',*,*,#42438,.F.);
#60920=ORIENTED_EDGE('',*,*,#41967,.T.);
#60921=ORIENTED_EDGE('',*,*,#42435,.T.);
#60922=ORIENTED_EDGE('',*,*,#42439,.T.);
#60923=ORIENTED_EDGE('',*,*,#42440,.F.);
#60924=ORIENTED_EDGE('',*,*,#42441,.F.);
#60925=ORIENTED_EDGE('',*,*,#42439,.F.);
#60926=ORIENTED_EDGE('',*,*,#42434,.F.);
#60927=ORIENTED_EDGE('',*,*,#42442,.F.);
#60928=ORIENTED_EDGE('',*,*,#42437,.F.);
#60929=ORIENTED_EDGE('',*,*,#41969,.T.);
#60930=ORIENTED_EDGE('',*,*,#42443,.F.);
#60931=ORIENTED_EDGE('',*,*,#42444,.T.);
#60932=ORIENTED_EDGE('',*,*,#42445,.F.);
#60933=ORIENTED_EDGE('',*,*,#42446,.F.);
#60934=ORIENTED_EDGE('',*,*,#42447,.T.);
#60935=ORIENTED_EDGE('',*,*,#42448,.F.);
#60936=ORIENTED_EDGE('',*,*,#41970,.T.);
#60937=ORIENTED_EDGE('',*,*,#42445,.T.);
#60938=ORIENTED_EDGE('',*,*,#42449,.T.);
#60939=ORIENTED_EDGE('',*,*,#42450,.F.);
#60940=ORIENTED_EDGE('',*,*,#42451,.F.);
#60941=ORIENTED_EDGE('',*,*,#42449,.F.);
#60942=ORIENTED_EDGE('',*,*,#42444,.F.);
#60943=ORIENTED_EDGE('',*,*,#42452,.F.);
#60944=ORIENTED_EDGE('',*,*,#42447,.F.);
#60945=ORIENTED_EDGE('',*,*,#42453,.F.);
#60946=ORIENTED_EDGE('',*,*,#42454,.F.);
#60947=ORIENTED_EDGE('',*,*,#41974,.T.);
#60948=ORIENTED_EDGE('',*,*,#41973,.T.);
#60949=ORIENTED_EDGE('',*,*,#42455,.F.);
#60950=ORIENTED_EDGE('',*,*,#41977,.T.);
#60951=ORIENTED_EDGE('',*,*,#41975,.T.);
#60952=ORIENTED_EDGE('',*,*,#42454,.T.);
#60953=ORIENTED_EDGE('',*,*,#42456,.F.);
#60954=ORIENTED_EDGE('',*,*,#42457,.F.);
#60955=ORIENTED_EDGE('',*,*,#41981,.T.);
#60956=ORIENTED_EDGE('',*,*,#41980,.T.);
#60957=ORIENTED_EDGE('',*,*,#42458,.F.);
#60958=ORIENTED_EDGE('',*,*,#41984,.T.);
#60959=ORIENTED_EDGE('',*,*,#41982,.T.);
#60960=ORIENTED_EDGE('',*,*,#42457,.T.);
#60961=ORIENTED_EDGE('',*,*,#42459,.F.);
#60962=ORIENTED_EDGE('',*,*,#42460,.F.);
#60963=ORIENTED_EDGE('',*,*,#41988,.T.);
#60964=ORIENTED_EDGE('',*,*,#41987,.T.);
#60965=ORIENTED_EDGE('',*,*,#42461,.F.);
#60966=ORIENTED_EDGE('',*,*,#41991,.T.);
#60967=ORIENTED_EDGE('',*,*,#41989,.T.);
#60968=ORIENTED_EDGE('',*,*,#42460,.T.);
#60969=ORIENTED_EDGE('',*,*,#42462,.F.);
#60970=ORIENTED_EDGE('',*,*,#42463,.F.);
#60971=ORIENTED_EDGE('',*,*,#41995,.T.);
#60972=ORIENTED_EDGE('',*,*,#41994,.T.);
#60973=ORIENTED_EDGE('',*,*,#42464,.F.);
#60974=ORIENTED_EDGE('',*,*,#41998,.T.);
#60975=ORIENTED_EDGE('',*,*,#41996,.T.);
#60976=ORIENTED_EDGE('',*,*,#42463,.T.);
#60977=ORIENTED_EDGE('',*,*,#42465,.F.);
#60978=ORIENTED_EDGE('',*,*,#42466,.F.);
#60979=ORIENTED_EDGE('',*,*,#42002,.T.);
#60980=ORIENTED_EDGE('',*,*,#42001,.T.);
#60981=ORIENTED_EDGE('',*,*,#42467,.F.);
#60982=ORIENTED_EDGE('',*,*,#42005,.T.);
#60983=ORIENTED_EDGE('',*,*,#42003,.T.);
#60984=ORIENTED_EDGE('',*,*,#42466,.T.);
#60985=ORIENTED_EDGE('',*,*,#42468,.F.);
#60986=ORIENTED_EDGE('',*,*,#42469,.F.);
#60987=ORIENTED_EDGE('',*,*,#42009,.T.);
#60988=ORIENTED_EDGE('',*,*,#42008,.T.);
#60989=ORIENTED_EDGE('',*,*,#42470,.F.);
#60990=ORIENTED_EDGE('',*,*,#42012,.T.);
#60991=ORIENTED_EDGE('',*,*,#42010,.T.);
#60992=ORIENTED_EDGE('',*,*,#42469,.T.);
#60993=ORIENTED_EDGE('',*,*,#42471,.F.);
#60994=ORIENTED_EDGE('',*,*,#42472,.F.);
#60995=ORIENTED_EDGE('',*,*,#42016,.T.);
#60996=ORIENTED_EDGE('',*,*,#42015,.T.);
#60997=ORIENTED_EDGE('',*,*,#42473,.F.);
#60998=ORIENTED_EDGE('',*,*,#42019,.T.);
#60999=ORIENTED_EDGE('',*,*,#42017,.T.);
#61000=ORIENTED_EDGE('',*,*,#42472,.T.);
#61001=ORIENTED_EDGE('',*,*,#42474,.F.);
#61002=ORIENTED_EDGE('',*,*,#42475,.F.);
#61003=ORIENTED_EDGE('',*,*,#42023,.T.);
#61004=ORIENTED_EDGE('',*,*,#42022,.T.);
#61005=ORIENTED_EDGE('',*,*,#42476,.F.);
#61006=ORIENTED_EDGE('',*,*,#42026,.T.);
#61007=ORIENTED_EDGE('',*,*,#42024,.T.);
#61008=ORIENTED_EDGE('',*,*,#42475,.T.);
#61009=ORIENTED_EDGE('',*,*,#42477,.F.);
#61010=ORIENTED_EDGE('',*,*,#42478,.F.);
#61011=ORIENTED_EDGE('',*,*,#42030,.T.);
#61012=ORIENTED_EDGE('',*,*,#42029,.T.);
#61013=ORIENTED_EDGE('',*,*,#42479,.F.);
#61014=ORIENTED_EDGE('',*,*,#42033,.T.);
#61015=ORIENTED_EDGE('',*,*,#42031,.T.);
#61016=ORIENTED_EDGE('',*,*,#42478,.T.);
#61017=ORIENTED_EDGE('',*,*,#42480,.F.);
#61018=ORIENTED_EDGE('',*,*,#42481,.F.);
#61019=ORIENTED_EDGE('',*,*,#42037,.T.);
#61020=ORIENTED_EDGE('',*,*,#42036,.T.);
#61021=ORIENTED_EDGE('',*,*,#42482,.F.);
#61022=ORIENTED_EDGE('',*,*,#42040,.T.);
#61023=ORIENTED_EDGE('',*,*,#42038,.T.);
#61024=ORIENTED_EDGE('',*,*,#42481,.T.);
#61025=ORIENTED_EDGE('',*,*,#42483,.F.);
#61026=ORIENTED_EDGE('',*,*,#42484,.F.);
#61027=ORIENTED_EDGE('',*,*,#42044,.T.);
#61028=ORIENTED_EDGE('',*,*,#42043,.T.);
#61029=ORIENTED_EDGE('',*,*,#42485,.F.);
#61030=ORIENTED_EDGE('',*,*,#42047,.T.);
#61031=ORIENTED_EDGE('',*,*,#42045,.T.);
#61032=ORIENTED_EDGE('',*,*,#42484,.T.);
#61033=ORIENTED_EDGE('',*,*,#42486,.F.);
#61034=ORIENTED_EDGE('',*,*,#42487,.F.);
#61035=ORIENTED_EDGE('',*,*,#42051,.T.);
#61036=ORIENTED_EDGE('',*,*,#42050,.T.);
#61037=ORIENTED_EDGE('',*,*,#42488,.F.);
#61038=ORIENTED_EDGE('',*,*,#42054,.T.);
#61039=ORIENTED_EDGE('',*,*,#42052,.T.);
#61040=ORIENTED_EDGE('',*,*,#42487,.T.);
#61041=ORIENTED_EDGE('',*,*,#42489,.F.);
#61042=ORIENTED_EDGE('',*,*,#42490,.F.);
#61043=ORIENTED_EDGE('',*,*,#42058,.T.);
#61044=ORIENTED_EDGE('',*,*,#42057,.T.);
#61045=ORIENTED_EDGE('',*,*,#42491,.F.);
#61046=ORIENTED_EDGE('',*,*,#42061,.T.);
#61047=ORIENTED_EDGE('',*,*,#42059,.T.);
#61048=ORIENTED_EDGE('',*,*,#42490,.T.);
#61049=ORIENTED_EDGE('',*,*,#42492,.F.);
#61050=ORIENTED_EDGE('',*,*,#42493,.F.);
#61051=ORIENTED_EDGE('',*,*,#42065,.T.);
#61052=ORIENTED_EDGE('',*,*,#42064,.T.);
#61053=ORIENTED_EDGE('',*,*,#42494,.F.);
#61054=ORIENTED_EDGE('',*,*,#42068,.T.);
#61055=ORIENTED_EDGE('',*,*,#42066,.T.);
#61056=ORIENTED_EDGE('',*,*,#42493,.T.);
#61057=ORIENTED_EDGE('',*,*,#42495,.F.);
#61058=ORIENTED_EDGE('',*,*,#42496,.F.);
#61059=ORIENTED_EDGE('',*,*,#34370,.T.);
#61060=ORIENTED_EDGE('',*,*,#42070,.T.);
#61061=ORIENTED_EDGE('',*,*,#42497,.F.);
#61062=ORIENTED_EDGE('',*,*,#42071,.T.);
#61063=ORIENTED_EDGE('',*,*,#34371,.T.);
#61064=ORIENTED_EDGE('',*,*,#42496,.T.);
#61065=ORIENTED_EDGE('',*,*,#42498,.F.);
#61066=ORIENTED_EDGE('',*,*,#42499,.F.);
#61067=ORIENTED_EDGE('',*,*,#42075,.T.);
#61068=ORIENTED_EDGE('',*,*,#42074,.T.);
#61069=ORIENTED_EDGE('',*,*,#42500,.F.);
#61070=ORIENTED_EDGE('',*,*,#42078,.T.);
#61071=ORIENTED_EDGE('',*,*,#42076,.T.);
#61072=ORIENTED_EDGE('',*,*,#42499,.T.);
#61073=ORIENTED_EDGE('',*,*,#42501,.F.);
#61074=ORIENTED_EDGE('',*,*,#42502,.F.);
#61075=ORIENTED_EDGE('',*,*,#42082,.T.);
#61076=ORIENTED_EDGE('',*,*,#42081,.T.);
#61077=ORIENTED_EDGE('',*,*,#42503,.F.);
#61078=ORIENTED_EDGE('',*,*,#42085,.T.);
#61079=ORIENTED_EDGE('',*,*,#42083,.T.);
#61080=ORIENTED_EDGE('',*,*,#42502,.T.);
#61081=ORIENTED_EDGE('',*,*,#42504,.F.);
#61082=ORIENTED_EDGE('',*,*,#42505,.F.);
#61083=ORIENTED_EDGE('',*,*,#42089,.T.);
#61084=ORIENTED_EDGE('',*,*,#42088,.T.);
#61085=ORIENTED_EDGE('',*,*,#42506,.F.);
#61086=ORIENTED_EDGE('',*,*,#42092,.T.);
#61087=ORIENTED_EDGE('',*,*,#42090,.T.);
#61088=ORIENTED_EDGE('',*,*,#42505,.T.);
#61089=ORIENTED_EDGE('',*,*,#42507,.F.);
#61090=ORIENTED_EDGE('',*,*,#42508,.F.);
#61091=ORIENTED_EDGE('',*,*,#42098,.T.);
#61092=ORIENTED_EDGE('',*,*,#42095,.T.);
#61093=ORIENTED_EDGE('',*,*,#42099,.T.);
#61094=ORIENTED_EDGE('',*,*,#42508,.T.);
#61095=ORIENTED_EDGE('',*,*,#42509,.F.);
#61096=ORIENTED_EDGE('',*,*,#42097,.T.);
#61097=ORIENTED_EDGE('',*,*,#42104,.T.);
#61098=ORIENTED_EDGE('',*,*,#42100,.T.);
#61099=ORIENTED_EDGE('',*,*,#42510,.F.);
#61100=ORIENTED_EDGE('',*,*,#42511,.F.);
#61101=ORIENTED_EDGE('',*,*,#42512,.F.);
#61102=ORIENTED_EDGE('',*,*,#42106,.T.);
#61103=ORIENTED_EDGE('',*,*,#42105,.T.);
#61104=ORIENTED_EDGE('',*,*,#42511,.T.);
#61105=ORIENTED_EDGE('',*,*,#42513,.F.);
#61106=ORIENTED_EDGE('',*,*,#42514,.F.);
#61107=ORIENTED_EDGE('',*,*,#42110,.T.);
#61108=ORIENTED_EDGE('',*,*,#42109,.T.);
#61109=ORIENTED_EDGE('',*,*,#42515,.F.);
#61110=ORIENTED_EDGE('',*,*,#42113,.T.);
#61111=ORIENTED_EDGE('',*,*,#42111,.T.);
#61112=ORIENTED_EDGE('',*,*,#42514,.T.);
#61113=ORIENTED_EDGE('',*,*,#42516,.F.);
#61114=ORIENTED_EDGE('',*,*,#42517,.F.);
#61115=ORIENTED_EDGE('',*,*,#42117,.T.);
#61116=ORIENTED_EDGE('',*,*,#42116,.T.);
#61117=ORIENTED_EDGE('',*,*,#42518,.F.);
#61118=ORIENTED_EDGE('',*,*,#42120,.T.);
#61119=ORIENTED_EDGE('',*,*,#42118,.T.);
#61120=ORIENTED_EDGE('',*,*,#42517,.T.);
#61121=ORIENTED_EDGE('',*,*,#42519,.F.);
#61122=ORIENTED_EDGE('',*,*,#42520,.F.);
#61123=ORIENTED_EDGE('',*,*,#42124,.T.);
#61124=ORIENTED_EDGE('',*,*,#42123,.T.);
#61125=ORIENTED_EDGE('',*,*,#42521,.F.);
#61126=ORIENTED_EDGE('',*,*,#42127,.T.);
#61127=ORIENTED_EDGE('',*,*,#42125,.T.);
#61128=ORIENTED_EDGE('',*,*,#42520,.T.);
#61129=ORIENTED_EDGE('',*,*,#42522,.F.);
#61130=ORIENTED_EDGE('',*,*,#42523,.F.);
#61131=ORIENTED_EDGE('',*,*,#42131,.T.);
#61132=ORIENTED_EDGE('',*,*,#42130,.T.);
#61133=ORIENTED_EDGE('',*,*,#42524,.F.);
#61134=ORIENTED_EDGE('',*,*,#42134,.T.);
#61135=ORIENTED_EDGE('',*,*,#42132,.T.);
#61136=ORIENTED_EDGE('',*,*,#42523,.T.);
#61137=ORIENTED_EDGE('',*,*,#42525,.F.);
#61138=ORIENTED_EDGE('',*,*,#42526,.F.);
#61139=ORIENTED_EDGE('',*,*,#42138,.T.);
#61140=ORIENTED_EDGE('',*,*,#42137,.T.);
#61141=ORIENTED_EDGE('',*,*,#42527,.F.);
#61142=ORIENTED_EDGE('',*,*,#42141,.T.);
#61143=ORIENTED_EDGE('',*,*,#42139,.T.);
#61144=ORIENTED_EDGE('',*,*,#42526,.T.);
#61145=ORIENTED_EDGE('',*,*,#42528,.F.);
#61146=ORIENTED_EDGE('',*,*,#42529,.F.);
#61147=ORIENTED_EDGE('',*,*,#42145,.T.);
#61148=ORIENTED_EDGE('',*,*,#42144,.T.);
#61149=ORIENTED_EDGE('',*,*,#42530,.F.);
#61150=ORIENTED_EDGE('',*,*,#42148,.T.);
#61151=ORIENTED_EDGE('',*,*,#42146,.T.);
#61152=ORIENTED_EDGE('',*,*,#42529,.T.);
#61153=ORIENTED_EDGE('',*,*,#42531,.F.);
#61154=ORIENTED_EDGE('',*,*,#42532,.F.);
#61155=ORIENTED_EDGE('',*,*,#42152,.T.);
#61156=ORIENTED_EDGE('',*,*,#42151,.T.);
#61157=ORIENTED_EDGE('',*,*,#42533,.F.);
#61158=ORIENTED_EDGE('',*,*,#42155,.T.);
#61159=ORIENTED_EDGE('',*,*,#42153,.T.);
#61160=ORIENTED_EDGE('',*,*,#42532,.T.);
#61161=ORIENTED_EDGE('',*,*,#42534,.F.);
#61162=ORIENTED_EDGE('',*,*,#42535,.F.);
#61163=ORIENTED_EDGE('',*,*,#42159,.T.);
#61164=ORIENTED_EDGE('',*,*,#42158,.T.);
#61165=ORIENTED_EDGE('',*,*,#42536,.F.);
#61166=ORIENTED_EDGE('',*,*,#42162,.T.);
#61167=ORIENTED_EDGE('',*,*,#42160,.T.);
#61168=ORIENTED_EDGE('',*,*,#42535,.T.);
#61169=ORIENTED_EDGE('',*,*,#42537,.F.);
#61170=ORIENTED_EDGE('',*,*,#42538,.F.);
#61171=ORIENTED_EDGE('',*,*,#42166,.T.);
#61172=ORIENTED_EDGE('',*,*,#42165,.T.);
#61173=ORIENTED_EDGE('',*,*,#42539,.F.);
#61174=ORIENTED_EDGE('',*,*,#42169,.T.);
#61175=ORIENTED_EDGE('',*,*,#42167,.T.);
#61176=ORIENTED_EDGE('',*,*,#42538,.T.);
#61177=ORIENTED_EDGE('',*,*,#42540,.F.);
#61178=ORIENTED_EDGE('',*,*,#42541,.F.);
#61179=ORIENTED_EDGE('',*,*,#42175,.T.);
#61180=ORIENTED_EDGE('',*,*,#42179,.T.);
#61181=ORIENTED_EDGE('',*,*,#42170,.T.);
#61182=ORIENTED_EDGE('',*,*,#42177,.T.);
#61183=ORIENTED_EDGE('',*,*,#42178,.T.);
#61184=ORIENTED_EDGE('',*,*,#42173,.T.);
#61185=ORIENTED_EDGE('',*,*,#42541,.T.);
#61186=ORIENTED_EDGE('',*,*,#42542,.F.);
#61187=ORIENTED_EDGE('',*,*,#42543,.F.);
#61188=ORIENTED_EDGE('',*,*,#42544,.F.);
#61189=ORIENTED_EDGE('',*,*,#42185,.T.);
#61190=ORIENTED_EDGE('',*,*,#42189,.T.);
#61191=ORIENTED_EDGE('',*,*,#42180,.T.);
#61192=ORIENTED_EDGE('',*,*,#42187,.T.);
#61193=ORIENTED_EDGE('',*,*,#42188,.T.);
#61194=ORIENTED_EDGE('',*,*,#42183,.T.);
#61195=ORIENTED_EDGE('',*,*,#42544,.T.);
#61196=ORIENTED_EDGE('',*,*,#42545,.F.);
#61197=ORIENTED_EDGE('',*,*,#42546,.F.);
#61198=ORIENTED_EDGE('',*,*,#42547,.F.);
#61199=ORIENTED_EDGE('',*,*,#42195,.T.);
#61200=ORIENTED_EDGE('',*,*,#42199,.T.);
#61201=ORIENTED_EDGE('',*,*,#42190,.T.);
#61202=ORIENTED_EDGE('',*,*,#42197,.T.);
#61203=ORIENTED_EDGE('',*,*,#42198,.T.);
#61204=ORIENTED_EDGE('',*,*,#42193,.T.);
#61205=ORIENTED_EDGE('',*,*,#42547,.T.);
#61206=ORIENTED_EDGE('',*,*,#42548,.F.);
#61207=ORIENTED_EDGE('',*,*,#42549,.F.);
#61208=ORIENTED_EDGE('',*,*,#42550,.F.);
#61209=ORIENTED_EDGE('',*,*,#42205,.T.);
#61210=ORIENTED_EDGE('',*,*,#42209,.T.);
#61211=ORIENTED_EDGE('',*,*,#42200,.T.);
#61212=ORIENTED_EDGE('',*,*,#42207,.T.);
#61213=ORIENTED_EDGE('',*,*,#42208,.T.);
#61214=ORIENTED_EDGE('',*,*,#42203,.T.);
#61215=ORIENTED_EDGE('',*,*,#42550,.T.);
#61216=ORIENTED_EDGE('',*,*,#42551,.F.);
#61217=ORIENTED_EDGE('',*,*,#42552,.F.);
#61218=ORIENTED_EDGE('',*,*,#42553,.F.);
#61219=ORIENTED_EDGE('',*,*,#42215,.T.);
#61220=ORIENTED_EDGE('',*,*,#42219,.T.);
#61221=ORIENTED_EDGE('',*,*,#42210,.T.);
#61222=ORIENTED_EDGE('',*,*,#42217,.T.);
#61223=ORIENTED_EDGE('',*,*,#42218,.T.);
#61224=ORIENTED_EDGE('',*,*,#42213,.T.);
#61225=ORIENTED_EDGE('',*,*,#42553,.T.);
#61226=ORIENTED_EDGE('',*,*,#42554,.F.);
#61227=ORIENTED_EDGE('',*,*,#42555,.F.);
#61228=ORIENTED_EDGE('',*,*,#42556,.F.);
#61229=ORIENTED_EDGE('',*,*,#42225,.T.);
#61230=ORIENTED_EDGE('',*,*,#42229,.T.);
#61231=ORIENTED_EDGE('',*,*,#42220,.T.);
#61232=ORIENTED_EDGE('',*,*,#42227,.T.);
#61233=ORIENTED_EDGE('',*,*,#42228,.T.);
#61234=ORIENTED_EDGE('',*,*,#42223,.T.);
#61235=ORIENTED_EDGE('',*,*,#42556,.T.);
#61236=ORIENTED_EDGE('',*,*,#42557,.F.);
#61237=ORIENTED_EDGE('',*,*,#42558,.F.);
#61238=ORIENTED_EDGE('',*,*,#42559,.F.);
#61239=ORIENTED_EDGE('',*,*,#42235,.T.);
#61240=ORIENTED_EDGE('',*,*,#42239,.T.);
#61241=ORIENTED_EDGE('',*,*,#42230,.T.);
#61242=ORIENTED_EDGE('',*,*,#42237,.T.);
#61243=ORIENTED_EDGE('',*,*,#42238,.T.);
#61244=ORIENTED_EDGE('',*,*,#42233,.T.);
#61245=ORIENTED_EDGE('',*,*,#42559,.T.);
#61246=ORIENTED_EDGE('',*,*,#42560,.F.);
#61247=ORIENTED_EDGE('',*,*,#42561,.F.);
#61248=ORIENTED_EDGE('',*,*,#42562,.F.);
#61249=ORIENTED_EDGE('',*,*,#42245,.T.);
#61250=ORIENTED_EDGE('',*,*,#42249,.T.);
#61251=ORIENTED_EDGE('',*,*,#42240,.T.);
#61252=ORIENTED_EDGE('',*,*,#42247,.T.);
#61253=ORIENTED_EDGE('',*,*,#42248,.T.);
#61254=ORIENTED_EDGE('',*,*,#42243,.T.);
#61255=ORIENTED_EDGE('',*,*,#42562,.T.);
#61256=ORIENTED_EDGE('',*,*,#42563,.F.);
#61257=ORIENTED_EDGE('',*,*,#42564,.F.);
#61258=ORIENTED_EDGE('',*,*,#42565,.F.);
#61259=ORIENTED_EDGE('',*,*,#42255,.T.);
#61260=ORIENTED_EDGE('',*,*,#42259,.T.);
#61261=ORIENTED_EDGE('',*,*,#42250,.T.);
#61262=ORIENTED_EDGE('',*,*,#42257,.T.);
#61263=ORIENTED_EDGE('',*,*,#42258,.T.);
#61264=ORIENTED_EDGE('',*,*,#42253,.T.);
#61265=ORIENTED_EDGE('',*,*,#42565,.T.);
#61266=ORIENTED_EDGE('',*,*,#42566,.F.);
#61267=ORIENTED_EDGE('',*,*,#42567,.F.);
#61268=ORIENTED_EDGE('',*,*,#42568,.F.);
#61269=ORIENTED_EDGE('',*,*,#42265,.T.);
#61270=ORIENTED_EDGE('',*,*,#42269,.T.);
#61271=ORIENTED_EDGE('',*,*,#42260,.T.);
#61272=ORIENTED_EDGE('',*,*,#42267,.T.);
#61273=ORIENTED_EDGE('',*,*,#42268,.T.);
#61274=ORIENTED_EDGE('',*,*,#42263,.T.);
#61275=ORIENTED_EDGE('',*,*,#42568,.T.);
#61276=ORIENTED_EDGE('',*,*,#42569,.F.);
#61277=ORIENTED_EDGE('',*,*,#42570,.F.);
#61278=ORIENTED_EDGE('',*,*,#42571,.F.);
#61279=ORIENTED_EDGE('',*,*,#42275,.T.);
#61280=ORIENTED_EDGE('',*,*,#42279,.T.);
#61281=ORIENTED_EDGE('',*,*,#42270,.T.);
#61282=ORIENTED_EDGE('',*,*,#42277,.T.);
#61283=ORIENTED_EDGE('',*,*,#42278,.T.);
#61284=ORIENTED_EDGE('',*,*,#42273,.T.);
#61285=ORIENTED_EDGE('',*,*,#42571,.T.);
#61286=ORIENTED_EDGE('',*,*,#42572,.F.);
#61287=ORIENTED_EDGE('',*,*,#42573,.F.);
#61288=ORIENTED_EDGE('',*,*,#42574,.F.);
#61289=ORIENTED_EDGE('',*,*,#42285,.T.);
#61290=ORIENTED_EDGE('',*,*,#42289,.T.);
#61291=ORIENTED_EDGE('',*,*,#42280,.T.);
#61292=ORIENTED_EDGE('',*,*,#42287,.T.);
#61293=ORIENTED_EDGE('',*,*,#42288,.T.);
#61294=ORIENTED_EDGE('',*,*,#42283,.T.);
#61295=ORIENTED_EDGE('',*,*,#42574,.T.);
#61296=ORIENTED_EDGE('',*,*,#42575,.F.);
#61297=ORIENTED_EDGE('',*,*,#42576,.F.);
#61298=ORIENTED_EDGE('',*,*,#42577,.F.);
#61299=ORIENTED_EDGE('',*,*,#42295,.T.);
#61300=ORIENTED_EDGE('',*,*,#42299,.T.);
#61301=ORIENTED_EDGE('',*,*,#42290,.T.);
#61302=ORIENTED_EDGE('',*,*,#42297,.T.);
#61303=ORIENTED_EDGE('',*,*,#42298,.T.);
#61304=ORIENTED_EDGE('',*,*,#42293,.T.);
#61305=ORIENTED_EDGE('',*,*,#42577,.T.);
#61306=ORIENTED_EDGE('',*,*,#42578,.F.);
#61307=ORIENTED_EDGE('',*,*,#42579,.F.);
#61308=ORIENTED_EDGE('',*,*,#42580,.F.);
#61309=ORIENTED_EDGE('',*,*,#42305,.T.);
#61310=ORIENTED_EDGE('',*,*,#42309,.T.);
#61311=ORIENTED_EDGE('',*,*,#42300,.T.);
#61312=ORIENTED_EDGE('',*,*,#42307,.T.);
#61313=ORIENTED_EDGE('',*,*,#42308,.T.);
#61314=ORIENTED_EDGE('',*,*,#42303,.T.);
#61315=ORIENTED_EDGE('',*,*,#42580,.T.);
#61316=ORIENTED_EDGE('',*,*,#42581,.F.);
#61317=ORIENTED_EDGE('',*,*,#42582,.F.);
#61318=ORIENTED_EDGE('',*,*,#42583,.F.);
#61319=ORIENTED_EDGE('',*,*,#42315,.T.);
#61320=ORIENTED_EDGE('',*,*,#42319,.T.);
#61321=ORIENTED_EDGE('',*,*,#42310,.T.);
#61322=ORIENTED_EDGE('',*,*,#42317,.T.);
#61323=ORIENTED_EDGE('',*,*,#42318,.T.);
#61324=ORIENTED_EDGE('',*,*,#42313,.T.);
#61325=ORIENTED_EDGE('',*,*,#42583,.T.);
#61326=ORIENTED_EDGE('',*,*,#42584,.F.);
#61327=ORIENTED_EDGE('',*,*,#42585,.F.);
#61328=ORIENTED_EDGE('',*,*,#42586,.F.);
#61329=ORIENTED_EDGE('',*,*,#42325,.T.);
#61330=ORIENTED_EDGE('',*,*,#42329,.T.);
#61331=ORIENTED_EDGE('',*,*,#42320,.T.);
#61332=ORIENTED_EDGE('',*,*,#42327,.T.);
#61333=ORIENTED_EDGE('',*,*,#42328,.T.);
#61334=ORIENTED_EDGE('',*,*,#42323,.T.);
#61335=ORIENTED_EDGE('',*,*,#42586,.T.);
#61336=ORIENTED_EDGE('',*,*,#42587,.F.);
#61337=ORIENTED_EDGE('',*,*,#42588,.F.);
#61338=ORIENTED_EDGE('',*,*,#42589,.F.);
#61339=ORIENTED_EDGE('',*,*,#42335,.T.);
#61340=ORIENTED_EDGE('',*,*,#42339,.T.);
#61341=ORIENTED_EDGE('',*,*,#42330,.T.);
#61342=ORIENTED_EDGE('',*,*,#42337,.T.);
#61343=ORIENTED_EDGE('',*,*,#42338,.T.);
#61344=ORIENTED_EDGE('',*,*,#42333,.T.);
#61345=ORIENTED_EDGE('',*,*,#42589,.T.);
#61346=ORIENTED_EDGE('',*,*,#42590,.F.);
#61347=ORIENTED_EDGE('',*,*,#42591,.F.);
#61348=ORIENTED_EDGE('',*,*,#42592,.F.);
#61349=ORIENTED_EDGE('',*,*,#42345,.T.);
#61350=ORIENTED_EDGE('',*,*,#42349,.T.);
#61351=ORIENTED_EDGE('',*,*,#42340,.T.);
#61352=ORIENTED_EDGE('',*,*,#42347,.T.);
#61353=ORIENTED_EDGE('',*,*,#42348,.T.);
#61354=ORIENTED_EDGE('',*,*,#42343,.T.);
#61355=ORIENTED_EDGE('',*,*,#42592,.T.);
#61356=ORIENTED_EDGE('',*,*,#42593,.F.);
#61357=ORIENTED_EDGE('',*,*,#42594,.F.);
#61358=ORIENTED_EDGE('',*,*,#42595,.F.);
#61359=ORIENTED_EDGE('',*,*,#42355,.T.);
#61360=ORIENTED_EDGE('',*,*,#42359,.T.);
#61361=ORIENTED_EDGE('',*,*,#42350,.T.);
#61362=ORIENTED_EDGE('',*,*,#42357,.T.);
#61363=ORIENTED_EDGE('',*,*,#42358,.T.);
#61364=ORIENTED_EDGE('',*,*,#42353,.T.);
#61365=ORIENTED_EDGE('',*,*,#42595,.T.);
#61366=ORIENTED_EDGE('',*,*,#42596,.F.);
#61367=ORIENTED_EDGE('',*,*,#42597,.F.);
#61368=ORIENTED_EDGE('',*,*,#42598,.F.);
#61369=ORIENTED_EDGE('',*,*,#42365,.T.);
#61370=ORIENTED_EDGE('',*,*,#42369,.T.);
#61371=ORIENTED_EDGE('',*,*,#42360,.T.);
#61372=ORIENTED_EDGE('',*,*,#42367,.T.);
#61373=ORIENTED_EDGE('',*,*,#42368,.T.);
#61374=ORIENTED_EDGE('',*,*,#42363,.T.);
#61375=ORIENTED_EDGE('',*,*,#42598,.T.);
#61376=ORIENTED_EDGE('',*,*,#42599,.F.);
#61377=ORIENTED_EDGE('',*,*,#42600,.F.);
#61378=ORIENTED_EDGE('',*,*,#42601,.F.);
#61379=ORIENTED_EDGE('',*,*,#42375,.T.);
#61380=ORIENTED_EDGE('',*,*,#42379,.T.);
#61381=ORIENTED_EDGE('',*,*,#42370,.T.);
#61382=ORIENTED_EDGE('',*,*,#42377,.T.);
#61383=ORIENTED_EDGE('',*,*,#42378,.T.);
#61384=ORIENTED_EDGE('',*,*,#42373,.T.);
#61385=ORIENTED_EDGE('',*,*,#42601,.T.);
#61386=ORIENTED_EDGE('',*,*,#42602,.F.);
#61387=ORIENTED_EDGE('',*,*,#42603,.F.);
#61388=ORIENTED_EDGE('',*,*,#42604,.F.);
#61389=ORIENTED_EDGE('',*,*,#34367,.T.);
#61390=ORIENTED_EDGE('',*,*,#34366,.T.);
#61391=ORIENTED_EDGE('',*,*,#42380,.T.);
#61392=ORIENTED_EDGE('',*,*,#42382,.T.);
#61393=ORIENTED_EDGE('',*,*,#34363,.T.);
#61394=ORIENTED_EDGE('',*,*,#34368,.T.);
#61395=ORIENTED_EDGE('',*,*,#42604,.T.);
#61396=ORIENTED_EDGE('',*,*,#42605,.F.);
#61397=ORIENTED_EDGE('',*,*,#42606,.F.);
#61398=ORIENTED_EDGE('',*,*,#42607,.F.);
#61399=ORIENTED_EDGE('',*,*,#42388,.T.);
#61400=ORIENTED_EDGE('',*,*,#42392,.T.);
#61401=ORIENTED_EDGE('',*,*,#42383,.T.);
#61402=ORIENTED_EDGE('',*,*,#42390,.T.);
#61403=ORIENTED_EDGE('',*,*,#42391,.T.);
#61404=ORIENTED_EDGE('',*,*,#42386,.T.);
#61405=ORIENTED_EDGE('',*,*,#42607,.T.);
#61406=ORIENTED_EDGE('',*,*,#42608,.F.);
#61407=ORIENTED_EDGE('',*,*,#42609,.F.);
#61408=ORIENTED_EDGE('',*,*,#42610,.F.);
#61409=ORIENTED_EDGE('',*,*,#42398,.T.);
#61410=ORIENTED_EDGE('',*,*,#42402,.T.);
#61411=ORIENTED_EDGE('',*,*,#42393,.T.);
#61412=ORIENTED_EDGE('',*,*,#42400,.T.);
#61413=ORIENTED_EDGE('',*,*,#42401,.T.);
#61414=ORIENTED_EDGE('',*,*,#42396,.T.);
#61415=ORIENTED_EDGE('',*,*,#42610,.T.);
#61416=ORIENTED_EDGE('',*,*,#42611,.F.);
#61417=ORIENTED_EDGE('',*,*,#42612,.F.);
#61418=ORIENTED_EDGE('',*,*,#42613,.F.);
#61419=ORIENTED_EDGE('',*,*,#42406,.T.);
#61420=ORIENTED_EDGE('',*,*,#42412,.T.);
#61421=ORIENTED_EDGE('',*,*,#42403,.T.);
#61422=ORIENTED_EDGE('',*,*,#42410,.T.);
#61423=ORIENTED_EDGE('',*,*,#42411,.T.);
#61424=ORIENTED_EDGE('',*,*,#42407,.T.);
#61425=ORIENTED_EDGE('',*,*,#42613,.T.);
#61426=ORIENTED_EDGE('',*,*,#42614,.F.);
#61427=ORIENTED_EDGE('',*,*,#42615,.F.);
#61428=ORIENTED_EDGE('',*,*,#42616,.F.);
#61429=ORIENTED_EDGE('',*,*,#42418,.T.);
#61430=ORIENTED_EDGE('',*,*,#42422,.T.);
#61431=ORIENTED_EDGE('',*,*,#42413,.T.);
#61432=ORIENTED_EDGE('',*,*,#42420,.T.);
#61433=ORIENTED_EDGE('',*,*,#42421,.T.);
#61434=ORIENTED_EDGE('',*,*,#42416,.T.);
#61435=ORIENTED_EDGE('',*,*,#42616,.T.);
#61436=ORIENTED_EDGE('',*,*,#42617,.F.);
#61437=ORIENTED_EDGE('',*,*,#42618,.F.);
#61438=ORIENTED_EDGE('',*,*,#42619,.F.);
#61439=ORIENTED_EDGE('',*,*,#42428,.T.);
#61440=ORIENTED_EDGE('',*,*,#42432,.T.);
#61441=ORIENTED_EDGE('',*,*,#42423,.T.);
#61442=ORIENTED_EDGE('',*,*,#42430,.T.);
#61443=ORIENTED_EDGE('',*,*,#42431,.T.);
#61444=ORIENTED_EDGE('',*,*,#42426,.T.);
#61445=ORIENTED_EDGE('',*,*,#42619,.T.);
#61446=ORIENTED_EDGE('',*,*,#42620,.F.);
#61447=ORIENTED_EDGE('',*,*,#42621,.F.);
#61448=ORIENTED_EDGE('',*,*,#42622,.F.);
#61449=ORIENTED_EDGE('',*,*,#42438,.T.);
#61450=ORIENTED_EDGE('',*,*,#42442,.T.);
#61451=ORIENTED_EDGE('',*,*,#42433,.T.);
#61452=ORIENTED_EDGE('',*,*,#42440,.T.);
#61453=ORIENTED_EDGE('',*,*,#42441,.T.);
#61454=ORIENTED_EDGE('',*,*,#42436,.T.);
#61455=ORIENTED_EDGE('',*,*,#42622,.T.);
#61456=ORIENTED_EDGE('',*,*,#42623,.F.);
#61457=ORIENTED_EDGE('',*,*,#42624,.F.);
#61458=ORIENTED_EDGE('',*,*,#42625,.F.);
#61459=ORIENTED_EDGE('',*,*,#42448,.T.);
#61460=ORIENTED_EDGE('',*,*,#42452,.T.);
#61461=ORIENTED_EDGE('',*,*,#42443,.T.);
#61462=ORIENTED_EDGE('',*,*,#42450,.T.);
#61463=ORIENTED_EDGE('',*,*,#42451,.T.);
#61464=ORIENTED_EDGE('',*,*,#42446,.T.);
#61465=ORIENTED_EDGE('',*,*,#42625,.T.);
#61466=ORIENTED_EDGE('',*,*,#42626,.F.);
#61467=ORIENTED_EDGE('',*,*,#42627,.T.);
#61468=ORIENTED_EDGE('',*,*,#42628,.F.);
#61469=ORIENTED_EDGE('',*,*,#42453,.T.);
#61470=ORIENTED_EDGE('',*,*,#42629,.F.);
#61471=ORIENTED_EDGE('',*,*,#42630,.T.);
#61472=ORIENTED_EDGE('',*,*,#42631,.F.);
#61473=ORIENTED_EDGE('',*,*,#42455,.T.);
#61474=ORIENTED_EDGE('',*,*,#42632,.F.);
#61475=ORIENTED_EDGE('',*,*,#42633,.F.);
#61476=ORIENTED_EDGE('',*,*,#42634,.F.);
#61477=ORIENTED_EDGE('',*,*,#42635,.F.);
#61478=ORIENTED_EDGE('',*,*,#42630,.F.);
#61479=ORIENTED_EDGE('',*,*,#42635,.T.);
#61480=ORIENTED_EDGE('',*,*,#42636,.F.);
#61481=ORIENTED_EDGE('',*,*,#42456,.T.);
#61482=ORIENTED_EDGE('',*,*,#42631,.T.);
#61483=ORIENTED_EDGE('',*,*,#42637,.T.);
#61484=ORIENTED_EDGE('',*,*,#42638,.F.);
#61485=ORIENTED_EDGE('',*,*,#42458,.T.);
#61486=ORIENTED_EDGE('',*,*,#42639,.F.);
#61487=ORIENTED_EDGE('',*,*,#42640,.F.);
#61488=ORIENTED_EDGE('',*,*,#42641,.F.);
#61489=ORIENTED_EDGE('',*,*,#42642,.F.);
#61490=ORIENTED_EDGE('',*,*,#42637,.F.);
#61491=ORIENTED_EDGE('',*,*,#42642,.T.);
#61492=ORIENTED_EDGE('',*,*,#42643,.F.);
#61493=ORIENTED_EDGE('',*,*,#42459,.T.);
#61494=ORIENTED_EDGE('',*,*,#42638,.T.);
#61495=ORIENTED_EDGE('',*,*,#42644,.T.);
#61496=ORIENTED_EDGE('',*,*,#42645,.F.);
#61497=ORIENTED_EDGE('',*,*,#42461,.T.);
#61498=ORIENTED_EDGE('',*,*,#42646,.F.);
#61499=ORIENTED_EDGE('',*,*,#42647,.F.);
#61500=ORIENTED_EDGE('',*,*,#42648,.F.);
#61501=ORIENTED_EDGE('',*,*,#42649,.F.);
#61502=ORIENTED_EDGE('',*,*,#42644,.F.);
#61503=ORIENTED_EDGE('',*,*,#42649,.T.);
#61504=ORIENTED_EDGE('',*,*,#42650,.F.);
#61505=ORIENTED_EDGE('',*,*,#42462,.T.);
#61506=ORIENTED_EDGE('',*,*,#42645,.T.);
#61507=ORIENTED_EDGE('',*,*,#42651,.T.);
#61508=ORIENTED_EDGE('',*,*,#42652,.F.);
#61509=ORIENTED_EDGE('',*,*,#42464,.T.);
#61510=ORIENTED_EDGE('',*,*,#42653,.F.);
#61511=ORIENTED_EDGE('',*,*,#42654,.F.);
#61512=ORIENTED_EDGE('',*,*,#42655,.F.);
#61513=ORIENTED_EDGE('',*,*,#42656,.F.);
#61514=ORIENTED_EDGE('',*,*,#42651,.F.);
#61515=ORIENTED_EDGE('',*,*,#42656,.T.);
#61516=ORIENTED_EDGE('',*,*,#42657,.F.);
#61517=ORIENTED_EDGE('',*,*,#42465,.T.);
#61518=ORIENTED_EDGE('',*,*,#42652,.T.);
#61519=ORIENTED_EDGE('',*,*,#42658,.T.);
#61520=ORIENTED_EDGE('',*,*,#42659,.F.);
#61521=ORIENTED_EDGE('',*,*,#42467,.T.);
#61522=ORIENTED_EDGE('',*,*,#42660,.F.);
#61523=ORIENTED_EDGE('',*,*,#42661,.F.);
#61524=ORIENTED_EDGE('',*,*,#42662,.F.);
#61525=ORIENTED_EDGE('',*,*,#42663,.F.);
#61526=ORIENTED_EDGE('',*,*,#42658,.F.);
#61527=ORIENTED_EDGE('',*,*,#42663,.T.);
#61528=ORIENTED_EDGE('',*,*,#42664,.F.);
#61529=ORIENTED_EDGE('',*,*,#42468,.T.);
#61530=ORIENTED_EDGE('',*,*,#42659,.T.);
#61531=ORIENTED_EDGE('',*,*,#42665,.T.);
#61532=ORIENTED_EDGE('',*,*,#42666,.F.);
#61533=ORIENTED_EDGE('',*,*,#42470,.T.);
#61534=ORIENTED_EDGE('',*,*,#42667,.F.);
#61535=ORIENTED_EDGE('',*,*,#42668,.F.);
#61536=ORIENTED_EDGE('',*,*,#42669,.F.);
#61537=ORIENTED_EDGE('',*,*,#42670,.F.);
#61538=ORIENTED_EDGE('',*,*,#42665,.F.);
#61539=ORIENTED_EDGE('',*,*,#42670,.T.);
#61540=ORIENTED_EDGE('',*,*,#42671,.F.);
#61541=ORIENTED_EDGE('',*,*,#42471,.T.);
#61542=ORIENTED_EDGE('',*,*,#42666,.T.);
#61543=ORIENTED_EDGE('',*,*,#34359,.T.);
#61544=ORIENTED_EDGE('',*,*,#42672,.F.);
#61545=ORIENTED_EDGE('',*,*,#42473,.T.);
#61546=ORIENTED_EDGE('',*,*,#42673,.F.);
#61547=ORIENTED_EDGE('',*,*,#34358,.T.);
#61548=ORIENTED_EDGE('',*,*,#42674,.F.);
#61549=ORIENTED_EDGE('',*,*,#42474,.T.);
#61550=ORIENTED_EDGE('',*,*,#42672,.T.);
#61551=ORIENTED_EDGE('',*,*,#42675,.T.);
#61552=ORIENTED_EDGE('',*,*,#42676,.F.);
#61553=ORIENTED_EDGE('',*,*,#42476,.T.);
#61554=ORIENTED_EDGE('',*,*,#42677,.F.);
#61555=ORIENTED_EDGE('',*,*,#42678,.F.);
#61556=ORIENTED_EDGE('',*,*,#42679,.F.);
#61557=ORIENTED_EDGE('',*,*,#42680,.F.);
#61558=ORIENTED_EDGE('',*,*,#42675,.F.);
#61559=ORIENTED_EDGE('',*,*,#42680,.T.);
#61560=ORIENTED_EDGE('',*,*,#42681,.F.);
#61561=ORIENTED_EDGE('',*,*,#42477,.T.);
#61562=ORIENTED_EDGE('',*,*,#42676,.T.);
#61563=ORIENTED_EDGE('',*,*,#42682,.T.);
#61564=ORIENTED_EDGE('',*,*,#42683,.F.);
#61565=ORIENTED_EDGE('',*,*,#42479,.T.);
#61566=ORIENTED_EDGE('',*,*,#42684,.F.);
#61567=ORIENTED_EDGE('',*,*,#42685,.F.);
#61568=ORIENTED_EDGE('',*,*,#42686,.F.);
#61569=ORIENTED_EDGE('',*,*,#42687,.F.);
#61570=ORIENTED_EDGE('',*,*,#42682,.F.);
#61571=ORIENTED_EDGE('',*,*,#42687,.T.);
#61572=ORIENTED_EDGE('',*,*,#42688,.F.);
#61573=ORIENTED_EDGE('',*,*,#42480,.T.);
#61574=ORIENTED_EDGE('',*,*,#42683,.T.);
#61575=ORIENTED_EDGE('',*,*,#42689,.T.);
#61576=ORIENTED_EDGE('',*,*,#42690,.F.);
#61577=ORIENTED_EDGE('',*,*,#42482,.T.);
#61578=ORIENTED_EDGE('',*,*,#42691,.F.);
#61579=ORIENTED_EDGE('',*,*,#42692,.F.);
#61580=ORIENTED_EDGE('',*,*,#42693,.F.);
#61581=ORIENTED_EDGE('',*,*,#42694,.F.);
#61582=ORIENTED_EDGE('',*,*,#42689,.F.);
#61583=ORIENTED_EDGE('',*,*,#42694,.T.);
#61584=ORIENTED_EDGE('',*,*,#42695,.F.);
#61585=ORIENTED_EDGE('',*,*,#42483,.T.);
#61586=ORIENTED_EDGE('',*,*,#42690,.T.);
#61587=ORIENTED_EDGE('',*,*,#42696,.T.);
#61588=ORIENTED_EDGE('',*,*,#42697,.F.);
#61589=ORIENTED_EDGE('',*,*,#42485,.T.);
#61590=ORIENTED_EDGE('',*,*,#42698,.F.);
#61591=ORIENTED_EDGE('',*,*,#42699,.F.);
#61592=ORIENTED_EDGE('',*,*,#42700,.F.);
#61593=ORIENTED_EDGE('',*,*,#42701,.F.);
#61594=ORIENTED_EDGE('',*,*,#42696,.F.);
#61595=ORIENTED_EDGE('',*,*,#42701,.T.);
#61596=ORIENTED_EDGE('',*,*,#42702,.F.);
#61597=ORIENTED_EDGE('',*,*,#42486,.T.);
#61598=ORIENTED_EDGE('',*,*,#42697,.T.);
#61599=ORIENTED_EDGE('',*,*,#42703,.T.);
#61600=ORIENTED_EDGE('',*,*,#42704,.F.);
#61601=ORIENTED_EDGE('',*,*,#42488,.T.);
#61602=ORIENTED_EDGE('',*,*,#42705,.F.);
#61603=ORIENTED_EDGE('',*,*,#42706,.F.);
#61604=ORIENTED_EDGE('',*,*,#42707,.F.);
#61605=ORIENTED_EDGE('',*,*,#42708,.F.);
#61606=ORIENTED_EDGE('',*,*,#42703,.F.);
#61607=ORIENTED_EDGE('',*,*,#42708,.T.);
#61608=ORIENTED_EDGE('',*,*,#42709,.F.);
#61609=ORIENTED_EDGE('',*,*,#42489,.T.);
#61610=ORIENTED_EDGE('',*,*,#42704,.T.);
#61611=ORIENTED_EDGE('',*,*,#42710,.T.);
#61612=ORIENTED_EDGE('',*,*,#42711,.F.);
#61613=ORIENTED_EDGE('',*,*,#42491,.T.);
#61614=ORIENTED_EDGE('',*,*,#42712,.F.);
#61615=ORIENTED_EDGE('',*,*,#42713,.F.);
#61616=ORIENTED_EDGE('',*,*,#42714,.F.);
#61617=ORIENTED_EDGE('',*,*,#42715,.F.);
#61618=ORIENTED_EDGE('',*,*,#42710,.F.);
#61619=ORIENTED_EDGE('',*,*,#42715,.T.);
#61620=ORIENTED_EDGE('',*,*,#42716,.F.);
#61621=ORIENTED_EDGE('',*,*,#42492,.T.);
#61622=ORIENTED_EDGE('',*,*,#42711,.T.);
#61623=ORIENTED_EDGE('',*,*,#42717,.T.);
#61624=ORIENTED_EDGE('',*,*,#42718,.F.);
#61625=ORIENTED_EDGE('',*,*,#42494,.T.);
#61626=ORIENTED_EDGE('',*,*,#42719,.F.);
#61627=ORIENTED_EDGE('',*,*,#42720,.F.);
#61628=ORIENTED_EDGE('',*,*,#42721,.F.);
#61629=ORIENTED_EDGE('',*,*,#42722,.F.);
#61630=ORIENTED_EDGE('',*,*,#42717,.F.);
#61631=ORIENTED_EDGE('',*,*,#42722,.T.);
#61632=ORIENTED_EDGE('',*,*,#42723,.F.);
#61633=ORIENTED_EDGE('',*,*,#42495,.T.);
#61634=ORIENTED_EDGE('',*,*,#42718,.T.);
#61635=ORIENTED_EDGE('',*,*,#42724,.T.);
#61636=ORIENTED_EDGE('',*,*,#42725,.F.);
#61637=ORIENTED_EDGE('',*,*,#42497,.T.);
#61638=ORIENTED_EDGE('',*,*,#42726,.F.);
#61639=ORIENTED_EDGE('',*,*,#42727,.F.);
#61640=ORIENTED_EDGE('',*,*,#42728,.F.);
#61641=ORIENTED_EDGE('',*,*,#42729,.F.);
#61642=ORIENTED_EDGE('',*,*,#42724,.F.);
#61643=ORIENTED_EDGE('',*,*,#42729,.T.);
#61644=ORIENTED_EDGE('',*,*,#42730,.F.);
#61645=ORIENTED_EDGE('',*,*,#42498,.T.);
#61646=ORIENTED_EDGE('',*,*,#42725,.T.);
#61647=ORIENTED_EDGE('',*,*,#42731,.T.);
#61648=ORIENTED_EDGE('',*,*,#42732,.F.);
#61649=ORIENTED_EDGE('',*,*,#42500,.T.);
#61650=ORIENTED_EDGE('',*,*,#42733,.F.);
#61651=ORIENTED_EDGE('',*,*,#42734,.F.);
#61652=ORIENTED_EDGE('',*,*,#42735,.F.);
#61653=ORIENTED_EDGE('',*,*,#42736,.F.);
#61654=ORIENTED_EDGE('',*,*,#42731,.F.);
#61655=ORIENTED_EDGE('',*,*,#42736,.T.);
#61656=ORIENTED_EDGE('',*,*,#42737,.F.);
#61657=ORIENTED_EDGE('',*,*,#42501,.T.);
#61658=ORIENTED_EDGE('',*,*,#42732,.T.);
#61659=ORIENTED_EDGE('',*,*,#42738,.T.);
#61660=ORIENTED_EDGE('',*,*,#42739,.F.);
#61661=ORIENTED_EDGE('',*,*,#42503,.T.);
#61662=ORIENTED_EDGE('',*,*,#42740,.F.);
#61663=ORIENTED_EDGE('',*,*,#42741,.F.);
#61664=ORIENTED_EDGE('',*,*,#42742,.F.);
#61665=ORIENTED_EDGE('',*,*,#42743,.F.);
#61666=ORIENTED_EDGE('',*,*,#42738,.F.);
#61667=ORIENTED_EDGE('',*,*,#42743,.T.);
#61668=ORIENTED_EDGE('',*,*,#42744,.F.);
#61669=ORIENTED_EDGE('',*,*,#42504,.T.);
#61670=ORIENTED_EDGE('',*,*,#42739,.T.);
#61671=ORIENTED_EDGE('',*,*,#42745,.T.);
#61672=ORIENTED_EDGE('',*,*,#42746,.F.);
#61673=ORIENTED_EDGE('',*,*,#42506,.T.);
#61674=ORIENTED_EDGE('',*,*,#42747,.F.);
#61675=ORIENTED_EDGE('',*,*,#42748,.T.);
#61676=ORIENTED_EDGE('',*,*,#42749,.F.);
#61677=ORIENTED_EDGE('',*,*,#42507,.T.);
#61678=ORIENTED_EDGE('',*,*,#42746,.T.);
#61679=ORIENTED_EDGE('',*,*,#42750,.F.);
#61680=ORIENTED_EDGE('',*,*,#42751,.F.);
#61681=ORIENTED_EDGE('',*,*,#42748,.F.);
#61682=ORIENTED_EDGE('',*,*,#42745,.F.);
#61683=ORIENTED_EDGE('',*,*,#42509,.T.);
#61684=ORIENTED_EDGE('',*,*,#42752,.F.);
#61685=ORIENTED_EDGE('',*,*,#42753,.T.);
#61686=ORIENTED_EDGE('',*,*,#42754,.F.);
#61687=ORIENTED_EDGE('',*,*,#42755,.F.);
#61688=ORIENTED_EDGE('',*,*,#42753,.F.);
#61689=ORIENTED_EDGE('',*,*,#42756,.F.);
#61690=ORIENTED_EDGE('',*,*,#42757,.F.);
#61691=ORIENTED_EDGE('',*,*,#42510,.T.);
#61692=ORIENTED_EDGE('',*,*,#42754,.T.);
#61693=ORIENTED_EDGE('',*,*,#42755,.T.);
#61694=ORIENTED_EDGE('',*,*,#42758,.F.);
#61695=ORIENTED_EDGE('',*,*,#42759,.T.);
#61696=ORIENTED_EDGE('',*,*,#42760,.F.);
#61697=ORIENTED_EDGE('',*,*,#42512,.T.);
#61698=ORIENTED_EDGE('',*,*,#42761,.F.);
#61699=ORIENTED_EDGE('',*,*,#42762,.F.);
#61700=ORIENTED_EDGE('',*,*,#42763,.F.);
#61701=ORIENTED_EDGE('',*,*,#42764,.F.);
#61702=ORIENTED_EDGE('',*,*,#42759,.F.);
#61703=ORIENTED_EDGE('',*,*,#42764,.T.);
#61704=ORIENTED_EDGE('',*,*,#42765,.F.);
#61705=ORIENTED_EDGE('',*,*,#42513,.T.);
#61706=ORIENTED_EDGE('',*,*,#42760,.T.);
#61707=ORIENTED_EDGE('',*,*,#42766,.T.);
#61708=ORIENTED_EDGE('',*,*,#42767,.F.);
#61709=ORIENTED_EDGE('',*,*,#42515,.T.);
#61710=ORIENTED_EDGE('',*,*,#42768,.F.);
#61711=ORIENTED_EDGE('',*,*,#42769,.F.);
#61712=ORIENTED_EDGE('',*,*,#42770,.F.);
#61713=ORIENTED_EDGE('',*,*,#42771,.F.);
#61714=ORIENTED_EDGE('',*,*,#42766,.F.);
#61715=ORIENTED_EDGE('',*,*,#42771,.T.);
#61716=ORIENTED_EDGE('',*,*,#42772,.F.);
#61717=ORIENTED_EDGE('',*,*,#42516,.T.);
#61718=ORIENTED_EDGE('',*,*,#42767,.T.);
#61719=ORIENTED_EDGE('',*,*,#42773,.T.);
#61720=ORIENTED_EDGE('',*,*,#42774,.F.);
#61721=ORIENTED_EDGE('',*,*,#42518,.T.);
#61722=ORIENTED_EDGE('',*,*,#42775,.F.);
#61723=ORIENTED_EDGE('',*,*,#42776,.F.);
#61724=ORIENTED_EDGE('',*,*,#42777,.F.);
#61725=ORIENTED_EDGE('',*,*,#42778,.F.);
#61726=ORIENTED_EDGE('',*,*,#42773,.F.);
#61727=ORIENTED_EDGE('',*,*,#42778,.T.);
#61728=ORIENTED_EDGE('',*,*,#42779,.F.);
#61729=ORIENTED_EDGE('',*,*,#42519,.T.);
#61730=ORIENTED_EDGE('',*,*,#42774,.T.);
#61731=ORIENTED_EDGE('',*,*,#42780,.T.);
#61732=ORIENTED_EDGE('',*,*,#42781,.F.);
#61733=ORIENTED_EDGE('',*,*,#42521,.T.);
#61734=ORIENTED_EDGE('',*,*,#42782,.F.);
#61735=ORIENTED_EDGE('',*,*,#42783,.F.);
#61736=ORIENTED_EDGE('',*,*,#42784,.F.);
#61737=ORIENTED_EDGE('',*,*,#42785,.F.);
#61738=ORIENTED_EDGE('',*,*,#42780,.F.);
#61739=ORIENTED_EDGE('',*,*,#42785,.T.);
#61740=ORIENTED_EDGE('',*,*,#42786,.F.);
#61741=ORIENTED_EDGE('',*,*,#42522,.T.);
#61742=ORIENTED_EDGE('',*,*,#42781,.T.);
#61743=ORIENTED_EDGE('',*,*,#42787,.T.);
#61744=ORIENTED_EDGE('',*,*,#42788,.F.);
#61745=ORIENTED_EDGE('',*,*,#42524,.T.);
#61746=ORIENTED_EDGE('',*,*,#42789,.F.);
#61747=ORIENTED_EDGE('',*,*,#42790,.F.);
#61748=ORIENTED_EDGE('',*,*,#42791,.F.);
#61749=ORIENTED_EDGE('',*,*,#42792,.F.);
#61750=ORIENTED_EDGE('',*,*,#42787,.F.);
#61751=ORIENTED_EDGE('',*,*,#42792,.T.);
#61752=ORIENTED_EDGE('',*,*,#42793,.F.);
#61753=ORIENTED_EDGE('',*,*,#42525,.T.);
#61754=ORIENTED_EDGE('',*,*,#42788,.T.);
#61755=ORIENTED_EDGE('',*,*,#42794,.T.);
#61756=ORIENTED_EDGE('',*,*,#42795,.F.);
#61757=ORIENTED_EDGE('',*,*,#42527,.T.);
#61758=ORIENTED_EDGE('',*,*,#42796,.F.);
#61759=ORIENTED_EDGE('',*,*,#42797,.F.);
#61760=ORIENTED_EDGE('',*,*,#42798,.F.);
#61761=ORIENTED_EDGE('',*,*,#42799,.F.);
#61762=ORIENTED_EDGE('',*,*,#42794,.F.);
#61763=ORIENTED_EDGE('',*,*,#42799,.T.);
#61764=ORIENTED_EDGE('',*,*,#42800,.F.);
#61765=ORIENTED_EDGE('',*,*,#42528,.T.);
#61766=ORIENTED_EDGE('',*,*,#42795,.T.);
#61767=ORIENTED_EDGE('',*,*,#42801,.T.);
#61768=ORIENTED_EDGE('',*,*,#42802,.F.);
#61769=ORIENTED_EDGE('',*,*,#42530,.T.);
#61770=ORIENTED_EDGE('',*,*,#42803,.F.);
#61771=ORIENTED_EDGE('',*,*,#42804,.F.);
#61772=ORIENTED_EDGE('',*,*,#42805,.F.);
#61773=ORIENTED_EDGE('',*,*,#42806,.F.);
#61774=ORIENTED_EDGE('',*,*,#42801,.F.);
#61775=ORIENTED_EDGE('',*,*,#42806,.T.);
#61776=ORIENTED_EDGE('',*,*,#42807,.F.);
#61777=ORIENTED_EDGE('',*,*,#42531,.T.);
#61778=ORIENTED_EDGE('',*,*,#42802,.T.);
#61779=ORIENTED_EDGE('',*,*,#42808,.T.);
#61780=ORIENTED_EDGE('',*,*,#42809,.F.);
#61781=ORIENTED_EDGE('',*,*,#42533,.T.);
#61782=ORIENTED_EDGE('',*,*,#42810,.F.);
#61783=ORIENTED_EDGE('',*,*,#42811,.F.);
#61784=ORIENTED_EDGE('',*,*,#42812,.F.);
#61785=ORIENTED_EDGE('',*,*,#42813,.F.);
#61786=ORIENTED_EDGE('',*,*,#42808,.F.);
#61787=ORIENTED_EDGE('',*,*,#42813,.T.);
#61788=ORIENTED_EDGE('',*,*,#42814,.F.);
#61789=ORIENTED_EDGE('',*,*,#42534,.T.);
#61790=ORIENTED_EDGE('',*,*,#42809,.T.);
#61791=ORIENTED_EDGE('',*,*,#42815,.T.);
#61792=ORIENTED_EDGE('',*,*,#42816,.F.);
#61793=ORIENTED_EDGE('',*,*,#42536,.T.);
#61794=ORIENTED_EDGE('',*,*,#42817,.F.);
#61795=ORIENTED_EDGE('',*,*,#42818,.F.);
#61796=ORIENTED_EDGE('',*,*,#42819,.F.);
#61797=ORIENTED_EDGE('',*,*,#42820,.F.);
#61798=ORIENTED_EDGE('',*,*,#42815,.F.);
#61799=ORIENTED_EDGE('',*,*,#42820,.T.);
#61800=ORIENTED_EDGE('',*,*,#42821,.F.);
#61801=ORIENTED_EDGE('',*,*,#42537,.T.);
#61802=ORIENTED_EDGE('',*,*,#42816,.T.);
#61803=ORIENTED_EDGE('',*,*,#42822,.F.);
#61804=ORIENTED_EDGE('',*,*,#42823,.F.);
#61805=ORIENTED_EDGE('',*,*,#42627,.F.);
#61806=ORIENTED_EDGE('',*,*,#42824,.F.);
#61807=ORIENTED_EDGE('',*,*,#42824,.T.);
#61808=ORIENTED_EDGE('',*,*,#42629,.T.);
#61809=ORIENTED_EDGE('',*,*,#42539,.T.);
#61810=ORIENTED_EDGE('',*,*,#42825,.F.);
#61811=ORIENTED_EDGE('',*,*,#42826,.F.);
#61812=ORIENTED_EDGE('',*,*,#42827,.T.);
#61813=ORIENTED_EDGE('',*,*,#42828,.F.);
#61814=ORIENTED_EDGE('',*,*,#42540,.T.);
#61815=ORIENTED_EDGE('',*,*,#42542,.T.);
#61816=ORIENTED_EDGE('',*,*,#42829,.F.);
#61817=ORIENTED_EDGE('',*,*,#42830,.T.);
#61818=ORIENTED_EDGE('',*,*,#42831,.F.);
#61819=ORIENTED_EDGE('',*,*,#42830,.F.);
#61820=ORIENTED_EDGE('',*,*,#42832,.F.);
#61821=ORIENTED_EDGE('',*,*,#42833,.F.);
#61822=ORIENTED_EDGE('',*,*,#42834,.F.);
#61823=ORIENTED_EDGE('',*,*,#42831,.T.);
#61824=ORIENTED_EDGE('',*,*,#42834,.T.);
#61825=ORIENTED_EDGE('',*,*,#42835,.F.);
#61826=ORIENTED_EDGE('',*,*,#42543,.T.);
#61827=ORIENTED_EDGE('',*,*,#42545,.T.);
#61828=ORIENTED_EDGE('',*,*,#42836,.F.);
#61829=ORIENTED_EDGE('',*,*,#42837,.T.);
#61830=ORIENTED_EDGE('',*,*,#42838,.F.);
#61831=ORIENTED_EDGE('',*,*,#42837,.F.);
#61832=ORIENTED_EDGE('',*,*,#42839,.F.);
#61833=ORIENTED_EDGE('',*,*,#42840,.F.);
#61834=ORIENTED_EDGE('',*,*,#42841,.F.);
#61835=ORIENTED_EDGE('',*,*,#42838,.T.);
#61836=ORIENTED_EDGE('',*,*,#42841,.T.);
#61837=ORIENTED_EDGE('',*,*,#42842,.F.);
#61838=ORIENTED_EDGE('',*,*,#42546,.T.);
#61839=ORIENTED_EDGE('',*,*,#42548,.T.);
#61840=ORIENTED_EDGE('',*,*,#42843,.F.);
#61841=ORIENTED_EDGE('',*,*,#42844,.T.);
#61842=ORIENTED_EDGE('',*,*,#42845,.F.);
#61843=ORIENTED_EDGE('',*,*,#42844,.F.);
#61844=ORIENTED_EDGE('',*,*,#42846,.F.);
#61845=ORIENTED_EDGE('',*,*,#42847,.F.);
#61846=ORIENTED_EDGE('',*,*,#42848,.F.);
#61847=ORIENTED_EDGE('',*,*,#42845,.T.);
#61848=ORIENTED_EDGE('',*,*,#42848,.T.);
#61849=ORIENTED_EDGE('',*,*,#42849,.F.);
#61850=ORIENTED_EDGE('',*,*,#42549,.T.);
#61851=ORIENTED_EDGE('',*,*,#42551,.T.);
#61852=ORIENTED_EDGE('',*,*,#42850,.F.);
#61853=ORIENTED_EDGE('',*,*,#42851,.T.);
#61854=ORIENTED_EDGE('',*,*,#42852,.F.);
#61855=ORIENTED_EDGE('',*,*,#42851,.F.);
#61856=ORIENTED_EDGE('',*,*,#42853,.F.);
#61857=ORIENTED_EDGE('',*,*,#42854,.F.);
#61858=ORIENTED_EDGE('',*,*,#42855,.F.);
#61859=ORIENTED_EDGE('',*,*,#42852,.T.);
#61860=ORIENTED_EDGE('',*,*,#42855,.T.);
#61861=ORIENTED_EDGE('',*,*,#42856,.F.);
#61862=ORIENTED_EDGE('',*,*,#42552,.T.);
#61863=ORIENTED_EDGE('',*,*,#42554,.T.);
#61864=ORIENTED_EDGE('',*,*,#42857,.F.);
#61865=ORIENTED_EDGE('',*,*,#42858,.T.);
#61866=ORIENTED_EDGE('',*,*,#42859,.F.);
#61867=ORIENTED_EDGE('',*,*,#42858,.F.);
#61868=ORIENTED_EDGE('',*,*,#42860,.F.);
#61869=ORIENTED_EDGE('',*,*,#42861,.F.);
#61870=ORIENTED_EDGE('',*,*,#42862,.F.);
#61871=ORIENTED_EDGE('',*,*,#42859,.T.);
#61872=ORIENTED_EDGE('',*,*,#42862,.T.);
#61873=ORIENTED_EDGE('',*,*,#42863,.F.);
#61874=ORIENTED_EDGE('',*,*,#42555,.T.);
#61875=ORIENTED_EDGE('',*,*,#42557,.T.);
#61876=ORIENTED_EDGE('',*,*,#42864,.F.);
#61877=ORIENTED_EDGE('',*,*,#42865,.T.);
#61878=ORIENTED_EDGE('',*,*,#42866,.F.);
#61879=ORIENTED_EDGE('',*,*,#42865,.F.);
#61880=ORIENTED_EDGE('',*,*,#42867,.F.);
#61881=ORIENTED_EDGE('',*,*,#42868,.F.);
#61882=ORIENTED_EDGE('',*,*,#42869,.F.);
#61883=ORIENTED_EDGE('',*,*,#42866,.T.);
#61884=ORIENTED_EDGE('',*,*,#42869,.T.);
#61885=ORIENTED_EDGE('',*,*,#42870,.F.);
#61886=ORIENTED_EDGE('',*,*,#42558,.T.);
#61887=ORIENTED_EDGE('',*,*,#42560,.T.);
#61888=ORIENTED_EDGE('',*,*,#42871,.F.);
#61889=ORIENTED_EDGE('',*,*,#42872,.T.);
#61890=ORIENTED_EDGE('',*,*,#42873,.F.);
#61891=ORIENTED_EDGE('',*,*,#42872,.F.);
#61892=ORIENTED_EDGE('',*,*,#42874,.F.);
#61893=ORIENTED_EDGE('',*,*,#42875,.F.);
#61894=ORIENTED_EDGE('',*,*,#42876,.F.);
#61895=ORIENTED_EDGE('',*,*,#42873,.T.);
#61896=ORIENTED_EDGE('',*,*,#42876,.T.);
#61897=ORIENTED_EDGE('',*,*,#42877,.F.);
#61898=ORIENTED_EDGE('',*,*,#42561,.T.);
#61899=ORIENTED_EDGE('',*,*,#42563,.T.);
#61900=ORIENTED_EDGE('',*,*,#42878,.F.);
#61901=ORIENTED_EDGE('',*,*,#42879,.T.);
#61902=ORIENTED_EDGE('',*,*,#42880,.F.);
#61903=ORIENTED_EDGE('',*,*,#42879,.F.);
#61904=ORIENTED_EDGE('',*,*,#42881,.F.);
#61905=ORIENTED_EDGE('',*,*,#42882,.F.);
#61906=ORIENTED_EDGE('',*,*,#42883,.F.);
#61907=ORIENTED_EDGE('',*,*,#42880,.T.);
#61908=ORIENTED_EDGE('',*,*,#42883,.T.);
#61909=ORIENTED_EDGE('',*,*,#42884,.F.);
#61910=ORIENTED_EDGE('',*,*,#42564,.T.);
#61911=ORIENTED_EDGE('',*,*,#42566,.T.);
#61912=ORIENTED_EDGE('',*,*,#42885,.F.);
#61913=ORIENTED_EDGE('',*,*,#42886,.T.);
#61914=ORIENTED_EDGE('',*,*,#42887,.F.);
#61915=ORIENTED_EDGE('',*,*,#42886,.F.);
#61916=ORIENTED_EDGE('',*,*,#42888,.F.);
#61917=ORIENTED_EDGE('',*,*,#42889,.F.);
#61918=ORIENTED_EDGE('',*,*,#42890,.F.);
#61919=ORIENTED_EDGE('',*,*,#42887,.T.);
#61920=ORIENTED_EDGE('',*,*,#42890,.T.);
#61921=ORIENTED_EDGE('',*,*,#42891,.F.);
#61922=ORIENTED_EDGE('',*,*,#42567,.T.);
#61923=ORIENTED_EDGE('',*,*,#42569,.T.);
#61924=ORIENTED_EDGE('',*,*,#42892,.F.);
#61925=ORIENTED_EDGE('',*,*,#42893,.T.);
#61926=ORIENTED_EDGE('',*,*,#42894,.F.);
#61927=ORIENTED_EDGE('',*,*,#42893,.F.);
#61928=ORIENTED_EDGE('',*,*,#42895,.F.);
#61929=ORIENTED_EDGE('',*,*,#42896,.F.);
#61930=ORIENTED_EDGE('',*,*,#42897,.F.);
#61931=ORIENTED_EDGE('',*,*,#42894,.T.);
#61932=ORIENTED_EDGE('',*,*,#42897,.T.);
#61933=ORIENTED_EDGE('',*,*,#42898,.F.);
#61934=ORIENTED_EDGE('',*,*,#42570,.T.);
#61935=ORIENTED_EDGE('',*,*,#42572,.T.);
#61936=ORIENTED_EDGE('',*,*,#42899,.F.);
#61937=ORIENTED_EDGE('',*,*,#42900,.T.);
#61938=ORIENTED_EDGE('',*,*,#42901,.F.);
#61939=ORIENTED_EDGE('',*,*,#42900,.F.);
#61940=ORIENTED_EDGE('',*,*,#42902,.F.);
#61941=ORIENTED_EDGE('',*,*,#42903,.F.);
#61942=ORIENTED_EDGE('',*,*,#42904,.F.);
#61943=ORIENTED_EDGE('',*,*,#42901,.T.);
#61944=ORIENTED_EDGE('',*,*,#42904,.T.);
#61945=ORIENTED_EDGE('',*,*,#42905,.F.);
#61946=ORIENTED_EDGE('',*,*,#42573,.T.);
#61947=ORIENTED_EDGE('',*,*,#42575,.T.);
#61948=ORIENTED_EDGE('',*,*,#42906,.F.);
#61949=ORIENTED_EDGE('',*,*,#42907,.T.);
#61950=ORIENTED_EDGE('',*,*,#42908,.F.);
#61951=ORIENTED_EDGE('',*,*,#42907,.F.);
#61952=ORIENTED_EDGE('',*,*,#42909,.F.);
#61953=ORIENTED_EDGE('',*,*,#42910,.F.);
#61954=ORIENTED_EDGE('',*,*,#42911,.F.);
#61955=ORIENTED_EDGE('',*,*,#42908,.T.);
#61956=ORIENTED_EDGE('',*,*,#42911,.T.);
#61957=ORIENTED_EDGE('',*,*,#42912,.F.);
#61958=ORIENTED_EDGE('',*,*,#42576,.T.);
#61959=ORIENTED_EDGE('',*,*,#42578,.T.);
#61960=ORIENTED_EDGE('',*,*,#42913,.F.);
#61961=ORIENTED_EDGE('',*,*,#42914,.T.);
#61962=ORIENTED_EDGE('',*,*,#42915,.F.);
#61963=ORIENTED_EDGE('',*,*,#42914,.F.);
#61964=ORIENTED_EDGE('',*,*,#42916,.F.);
#61965=ORIENTED_EDGE('',*,*,#42917,.F.);
#61966=ORIENTED_EDGE('',*,*,#42918,.F.);
#61967=ORIENTED_EDGE('',*,*,#42915,.T.);
#61968=ORIENTED_EDGE('',*,*,#42918,.T.);
#61969=ORIENTED_EDGE('',*,*,#42919,.F.);
#61970=ORIENTED_EDGE('',*,*,#42579,.T.);
#61971=ORIENTED_EDGE('',*,*,#42581,.T.);
#61972=ORIENTED_EDGE('',*,*,#42920,.F.);
#61973=ORIENTED_EDGE('',*,*,#34356,.T.);
#61974=ORIENTED_EDGE('',*,*,#42921,.F.);
#61975=ORIENTED_EDGE('',*,*,#34355,.T.);
#61976=ORIENTED_EDGE('',*,*,#42922,.F.);
#61977=ORIENTED_EDGE('',*,*,#42582,.T.);
#61978=ORIENTED_EDGE('',*,*,#42921,.T.);
#61979=ORIENTED_EDGE('',*,*,#42584,.T.);
#61980=ORIENTED_EDGE('',*,*,#42923,.F.);
#61981=ORIENTED_EDGE('',*,*,#42924,.T.);
#61982=ORIENTED_EDGE('',*,*,#42925,.F.);
#61983=ORIENTED_EDGE('',*,*,#42924,.F.);
#61984=ORIENTED_EDGE('',*,*,#42926,.F.);
#61985=ORIENTED_EDGE('',*,*,#42927,.F.);
#61986=ORIENTED_EDGE('',*,*,#42928,.F.);
#61987=ORIENTED_EDGE('',*,*,#42925,.T.);
#61988=ORIENTED_EDGE('',*,*,#42928,.T.);
#61989=ORIENTED_EDGE('',*,*,#42929,.F.);
#61990=ORIENTED_EDGE('',*,*,#42585,.T.);
#61991=ORIENTED_EDGE('',*,*,#42587,.T.);
#61992=ORIENTED_EDGE('',*,*,#42930,.F.);
#61993=ORIENTED_EDGE('',*,*,#42931,.T.);
#61994=ORIENTED_EDGE('',*,*,#42932,.F.);
#61995=ORIENTED_EDGE('',*,*,#42931,.F.);
#61996=ORIENTED_EDGE('',*,*,#42933,.F.);
#61997=ORIENTED_EDGE('',*,*,#42934,.F.);
#61998=ORIENTED_EDGE('',*,*,#42935,.F.);
#61999=ORIENTED_EDGE('',*,*,#42932,.T.);
#62000=ORIENTED_EDGE('',*,*,#42935,.T.);
#62001=ORIENTED_EDGE('',*,*,#42936,.F.);
#62002=ORIENTED_EDGE('',*,*,#42588,.T.);
#62003=ORIENTED_EDGE('',*,*,#42590,.T.);
#62004=ORIENTED_EDGE('',*,*,#42937,.F.);
#62005=ORIENTED_EDGE('',*,*,#42938,.T.);
#62006=ORIENTED_EDGE('',*,*,#42939,.F.);
#62007=ORIENTED_EDGE('',*,*,#42938,.F.);
#62008=ORIENTED_EDGE('',*,*,#42940,.F.);
#62009=ORIENTED_EDGE('',*,*,#42941,.F.);
#62010=ORIENTED_EDGE('',*,*,#42942,.F.);
#62011=ORIENTED_EDGE('',*,*,#42939,.T.);
#62012=ORIENTED_EDGE('',*,*,#42942,.T.);
#62013=ORIENTED_EDGE('',*,*,#42943,.F.);
#62014=ORIENTED_EDGE('',*,*,#42591,.T.);
#62015=ORIENTED_EDGE('',*,*,#42593,.T.);
#62016=ORIENTED_EDGE('',*,*,#42944,.F.);
#62017=ORIENTED_EDGE('',*,*,#42945,.T.);
#62018=ORIENTED_EDGE('',*,*,#42946,.F.);
#62019=ORIENTED_EDGE('',*,*,#42945,.F.);
#62020=ORIENTED_EDGE('',*,*,#42947,.F.);
#62021=ORIENTED_EDGE('',*,*,#42948,.F.);
#62022=ORIENTED_EDGE('',*,*,#42949,.F.);
#62023=ORIENTED_EDGE('',*,*,#42946,.T.);
#62024=ORIENTED_EDGE('',*,*,#42949,.T.);
#62025=ORIENTED_EDGE('',*,*,#42950,.F.);
#62026=ORIENTED_EDGE('',*,*,#42594,.T.);
#62027=ORIENTED_EDGE('',*,*,#42596,.T.);
#62028=ORIENTED_EDGE('',*,*,#42951,.F.);
#62029=ORIENTED_EDGE('',*,*,#42952,.T.);
#62030=ORIENTED_EDGE('',*,*,#42953,.F.);
#62031=ORIENTED_EDGE('',*,*,#42952,.F.);
#62032=ORIENTED_EDGE('',*,*,#42954,.F.);
#62033=ORIENTED_EDGE('',*,*,#42955,.F.);
#62034=ORIENTED_EDGE('',*,*,#42956,.F.);
#62035=ORIENTED_EDGE('',*,*,#42953,.T.);
#62036=ORIENTED_EDGE('',*,*,#42956,.T.);
#62037=ORIENTED_EDGE('',*,*,#42957,.F.);
#62038=ORIENTED_EDGE('',*,*,#42597,.T.);
#62039=ORIENTED_EDGE('',*,*,#42599,.T.);
#62040=ORIENTED_EDGE('',*,*,#42958,.F.);
#62041=ORIENTED_EDGE('',*,*,#42959,.T.);
#62042=ORIENTED_EDGE('',*,*,#42960,.F.);
#62043=ORIENTED_EDGE('',*,*,#42959,.F.);
#62044=ORIENTED_EDGE('',*,*,#42961,.F.);
#62045=ORIENTED_EDGE('',*,*,#42962,.F.);
#62046=ORIENTED_EDGE('',*,*,#42963,.F.);
#62047=ORIENTED_EDGE('',*,*,#42960,.T.);
#62048=ORIENTED_EDGE('',*,*,#42963,.T.);
#62049=ORIENTED_EDGE('',*,*,#42964,.F.);
#62050=ORIENTED_EDGE('',*,*,#42600,.T.);
#62051=ORIENTED_EDGE('',*,*,#42602,.T.);
#62052=ORIENTED_EDGE('',*,*,#42965,.F.);
#62053=ORIENTED_EDGE('',*,*,#34352,.T.);
#62054=ORIENTED_EDGE('',*,*,#42966,.F.);
#62055=ORIENTED_EDGE('',*,*,#42966,.T.);
#62056=ORIENTED_EDGE('',*,*,#34351,.T.);
#62057=ORIENTED_EDGE('',*,*,#42967,.F.);
#62058=ORIENTED_EDGE('',*,*,#42603,.T.);
#62059=ORIENTED_EDGE('',*,*,#42605,.T.);
#62060=ORIENTED_EDGE('',*,*,#42968,.F.);
#62061=ORIENTED_EDGE('',*,*,#42969,.T.);
#62062=ORIENTED_EDGE('',*,*,#42970,.F.);
#62063=ORIENTED_EDGE('',*,*,#42969,.F.);
#62064=ORIENTED_EDGE('',*,*,#42971,.F.);
#62065=ORIENTED_EDGE('',*,*,#42972,.F.);
#62066=ORIENTED_EDGE('',*,*,#42973,.F.);
#62067=ORIENTED_EDGE('',*,*,#42970,.T.);
#62068=ORIENTED_EDGE('',*,*,#42973,.T.);
#62069=ORIENTED_EDGE('',*,*,#42974,.F.);
#62070=ORIENTED_EDGE('',*,*,#42606,.T.);
#62071=ORIENTED_EDGE('',*,*,#42608,.T.);
#62072=ORIENTED_EDGE('',*,*,#42975,.F.);
#62073=ORIENTED_EDGE('',*,*,#42976,.T.);
#62074=ORIENTED_EDGE('',*,*,#42977,.F.);
#62075=ORIENTED_EDGE('',*,*,#42976,.F.);
#62076=ORIENTED_EDGE('',*,*,#42978,.F.);
#62077=ORIENTED_EDGE('',*,*,#42979,.F.);
#62078=ORIENTED_EDGE('',*,*,#42980,.F.);
#62079=ORIENTED_EDGE('',*,*,#42977,.T.);
#62080=ORIENTED_EDGE('',*,*,#42980,.T.);
#62081=ORIENTED_EDGE('',*,*,#42981,.F.);
#62082=ORIENTED_EDGE('',*,*,#42609,.T.);
#62083=ORIENTED_EDGE('',*,*,#42611,.T.);
#62084=ORIENTED_EDGE('',*,*,#42982,.F.);
#62085=ORIENTED_EDGE('',*,*,#42983,.T.);
#62086=ORIENTED_EDGE('',*,*,#42984,.F.);
#62087=ORIENTED_EDGE('',*,*,#42983,.F.);
#62088=ORIENTED_EDGE('',*,*,#42985,.F.);
#62089=ORIENTED_EDGE('',*,*,#42986,.F.);
#62090=ORIENTED_EDGE('',*,*,#42987,.F.);
#62091=ORIENTED_EDGE('',*,*,#42984,.T.);
#62092=ORIENTED_EDGE('',*,*,#42987,.T.);
#62093=ORIENTED_EDGE('',*,*,#42988,.F.);
#62094=ORIENTED_EDGE('',*,*,#42612,.T.);
#62095=ORIENTED_EDGE('',*,*,#42614,.T.);
#62096=ORIENTED_EDGE('',*,*,#42989,.F.);
#62097=ORIENTED_EDGE('',*,*,#42990,.T.);
#62098=ORIENTED_EDGE('',*,*,#42991,.F.);
#62099=ORIENTED_EDGE('',*,*,#42990,.F.);
#62100=ORIENTED_EDGE('',*,*,#42992,.F.);
#62101=ORIENTED_EDGE('',*,*,#42993,.F.);
#62102=ORIENTED_EDGE('',*,*,#42994,.F.);
#62103=ORIENTED_EDGE('',*,*,#42991,.T.);
#62104=ORIENTED_EDGE('',*,*,#42994,.T.);
#62105=ORIENTED_EDGE('',*,*,#42995,.F.);
#62106=ORIENTED_EDGE('',*,*,#42615,.T.);
#62107=ORIENTED_EDGE('',*,*,#42617,.T.);
#62108=ORIENTED_EDGE('',*,*,#42996,.F.);
#62109=ORIENTED_EDGE('',*,*,#42997,.T.);
#62110=ORIENTED_EDGE('',*,*,#42998,.F.);
#62111=ORIENTED_EDGE('',*,*,#42997,.F.);
#62112=ORIENTED_EDGE('',*,*,#42999,.F.);
#62113=ORIENTED_EDGE('',*,*,#43000,.F.);
#62114=ORIENTED_EDGE('',*,*,#43001,.F.);
#62115=ORIENTED_EDGE('',*,*,#42998,.T.);
#62116=ORIENTED_EDGE('',*,*,#43001,.T.);
#62117=ORIENTED_EDGE('',*,*,#43002,.F.);
#62118=ORIENTED_EDGE('',*,*,#42618,.T.);
#62119=ORIENTED_EDGE('',*,*,#42620,.T.);
#62120=ORIENTED_EDGE('',*,*,#43003,.F.);
#62121=ORIENTED_EDGE('',*,*,#43004,.T.);
#62122=ORIENTED_EDGE('',*,*,#43005,.F.);
#62123=ORIENTED_EDGE('',*,*,#43004,.F.);
#62124=ORIENTED_EDGE('',*,*,#43006,.F.);
#62125=ORIENTED_EDGE('',*,*,#43007,.F.);
#62126=ORIENTED_EDGE('',*,*,#43008,.F.);
#62127=ORIENTED_EDGE('',*,*,#43005,.T.);
#62128=ORIENTED_EDGE('',*,*,#43008,.T.);
#62129=ORIENTED_EDGE('',*,*,#43009,.F.);
#62130=ORIENTED_EDGE('',*,*,#42621,.T.);
#62131=ORIENTED_EDGE('',*,*,#42623,.T.);
#62132=ORIENTED_EDGE('',*,*,#43010,.F.);
#62133=ORIENTED_EDGE('',*,*,#43011,.T.);
#62134=ORIENTED_EDGE('',*,*,#43012,.F.);
#62135=ORIENTED_EDGE('',*,*,#43011,.F.);
#62136=ORIENTED_EDGE('',*,*,#43013,.F.);
#62137=ORIENTED_EDGE('',*,*,#43014,.F.);
#62138=ORIENTED_EDGE('',*,*,#43015,.F.);
#62139=ORIENTED_EDGE('',*,*,#43012,.T.);
#62140=ORIENTED_EDGE('',*,*,#43015,.T.);
#62141=ORIENTED_EDGE('',*,*,#43016,.F.);
#62142=ORIENTED_EDGE('',*,*,#42624,.T.);
#62143=ORIENTED_EDGE('',*,*,#43017,.F.);
#62144=ORIENTED_EDGE('',*,*,#43018,.F.);
#62145=ORIENTED_EDGE('',*,*,#43019,.F.);
#62146=ORIENTED_EDGE('',*,*,#42827,.F.);
#62147=ORIENTED_EDGE('',*,*,#42626,.T.);
#62148=ORIENTED_EDGE('',*,*,#43020,.F.);
#62149=ORIENTED_EDGE('',*,*,#43017,.T.);
#62150=ORIENTED_EDGE('',*,*,#42826,.T.);
#62151=ORIENTED_EDGE('',*,*,#43021,.F.);
#62152=ORIENTED_EDGE('',*,*,#42628,.T.);
#62153=ORIENTED_EDGE('',*,*,#42823,.T.);
#62154=ORIENTED_EDGE('',*,*,#43022,.F.);
#62155=ORIENTED_EDGE('',*,*,#43023,.F.);
#62156=ORIENTED_EDGE('',*,*,#43024,.F.);
#62157=ORIENTED_EDGE('',*,*,#42633,.T.);
#62158=ORIENTED_EDGE('',*,*,#42632,.T.);
#62159=ORIENTED_EDGE('',*,*,#43025,.F.);
#62160=ORIENTED_EDGE('',*,*,#42636,.T.);
#62161=ORIENTED_EDGE('',*,*,#42634,.T.);
#62162=ORIENTED_EDGE('',*,*,#43024,.T.);
#62163=ORIENTED_EDGE('',*,*,#43026,.F.);
#62164=ORIENTED_EDGE('',*,*,#43027,.F.);
#62165=ORIENTED_EDGE('',*,*,#42640,.T.);
#62166=ORIENTED_EDGE('',*,*,#42639,.T.);
#62167=ORIENTED_EDGE('',*,*,#43028,.F.);
#62168=ORIENTED_EDGE('',*,*,#42643,.T.);
#62169=ORIENTED_EDGE('',*,*,#42641,.T.);
#62170=ORIENTED_EDGE('',*,*,#43027,.T.);
#62171=ORIENTED_EDGE('',*,*,#43029,.F.);
#62172=ORIENTED_EDGE('',*,*,#43030,.F.);
#62173=ORIENTED_EDGE('',*,*,#42647,.T.);
#62174=ORIENTED_EDGE('',*,*,#42646,.T.);
#62175=ORIENTED_EDGE('',*,*,#43031,.F.);
#62176=ORIENTED_EDGE('',*,*,#42650,.T.);
#62177=ORIENTED_EDGE('',*,*,#42648,.T.);
#62178=ORIENTED_EDGE('',*,*,#43030,.T.);
#62179=ORIENTED_EDGE('',*,*,#43032,.F.);
#62180=ORIENTED_EDGE('',*,*,#43033,.F.);
#62181=ORIENTED_EDGE('',*,*,#42654,.T.);
#62182=ORIENTED_EDGE('',*,*,#42653,.T.);
#62183=ORIENTED_EDGE('',*,*,#43034,.F.);
#62184=ORIENTED_EDGE('',*,*,#42657,.T.);
#62185=ORIENTED_EDGE('',*,*,#42655,.T.);
#62186=ORIENTED_EDGE('',*,*,#43033,.T.);
#62187=ORIENTED_EDGE('',*,*,#43035,.F.);
#62188=ORIENTED_EDGE('',*,*,#43036,.F.);
#62189=ORIENTED_EDGE('',*,*,#42661,.T.);
#62190=ORIENTED_EDGE('',*,*,#42660,.T.);
#62191=ORIENTED_EDGE('',*,*,#43037,.F.);
#62192=ORIENTED_EDGE('',*,*,#42664,.T.);
#62193=ORIENTED_EDGE('',*,*,#42662,.T.);
#62194=ORIENTED_EDGE('',*,*,#43036,.T.);
#62195=ORIENTED_EDGE('',*,*,#43038,.F.);
#62196=ORIENTED_EDGE('',*,*,#43039,.F.);
#62197=ORIENTED_EDGE('',*,*,#42668,.T.);
#62198=ORIENTED_EDGE('',*,*,#42667,.T.);
#62199=ORIENTED_EDGE('',*,*,#43040,.F.);
#62200=ORIENTED_EDGE('',*,*,#42671,.T.);
#62201=ORIENTED_EDGE('',*,*,#42669,.T.);
#62202=ORIENTED_EDGE('',*,*,#43039,.T.);
#62203=ORIENTED_EDGE('',*,*,#43041,.F.);
#62204=ORIENTED_EDGE('',*,*,#43042,.F.);
#62205=ORIENTED_EDGE('',*,*,#34360,.T.);
#62206=ORIENTED_EDGE('',*,*,#42673,.T.);
#62207=ORIENTED_EDGE('',*,*,#43043,.F.);
#62208=ORIENTED_EDGE('',*,*,#42674,.T.);
#62209=ORIENTED_EDGE('',*,*,#34361,.T.);
#62210=ORIENTED_EDGE('',*,*,#43042,.T.);
#62211=ORIENTED_EDGE('',*,*,#43044,.F.);
#62212=ORIENTED_EDGE('',*,*,#43045,.F.);
#62213=ORIENTED_EDGE('',*,*,#42678,.T.);
#62214=ORIENTED_EDGE('',*,*,#42677,.T.);
#62215=ORIENTED_EDGE('',*,*,#43046,.F.);
#62216=ORIENTED_EDGE('',*,*,#42681,.T.);
#62217=ORIENTED_EDGE('',*,*,#42679,.T.);
#62218=ORIENTED_EDGE('',*,*,#43045,.T.);
#62219=ORIENTED_EDGE('',*,*,#43047,.F.);
#62220=ORIENTED_EDGE('',*,*,#43048,.F.);
#62221=ORIENTED_EDGE('',*,*,#42685,.T.);
#62222=ORIENTED_EDGE('',*,*,#42684,.T.);
#62223=ORIENTED_EDGE('',*,*,#43049,.F.);
#62224=ORIENTED_EDGE('',*,*,#42688,.T.);
#62225=ORIENTED_EDGE('',*,*,#42686,.T.);
#62226=ORIENTED_EDGE('',*,*,#43048,.T.);
#62227=ORIENTED_EDGE('',*,*,#43050,.F.);
#62228=ORIENTED_EDGE('',*,*,#43051,.F.);
#62229=ORIENTED_EDGE('',*,*,#42692,.T.);
#62230=ORIENTED_EDGE('',*,*,#42691,.T.);
#62231=ORIENTED_EDGE('',*,*,#43052,.F.);
#62232=ORIENTED_EDGE('',*,*,#42695,.T.);
#62233=ORIENTED_EDGE('',*,*,#42693,.T.);
#62234=ORIENTED_EDGE('',*,*,#43051,.T.);
#62235=ORIENTED_EDGE('',*,*,#43053,.F.);
#62236=ORIENTED_EDGE('',*,*,#43054,.F.);
#62237=ORIENTED_EDGE('',*,*,#42699,.T.);
#62238=ORIENTED_EDGE('',*,*,#42698,.T.);
#62239=ORIENTED_EDGE('',*,*,#43055,.F.);
#62240=ORIENTED_EDGE('',*,*,#42702,.T.);
#62241=ORIENTED_EDGE('',*,*,#42700,.T.);
#62242=ORIENTED_EDGE('',*,*,#43054,.T.);
#62243=ORIENTED_EDGE('',*,*,#43056,.F.);
#62244=ORIENTED_EDGE('',*,*,#43057,.F.);
#62245=ORIENTED_EDGE('',*,*,#42706,.T.);
#62246=ORIENTED_EDGE('',*,*,#42705,.T.);
#62247=ORIENTED_EDGE('',*,*,#43058,.F.);
#62248=ORIENTED_EDGE('',*,*,#42709,.T.);
#62249=ORIENTED_EDGE('',*,*,#42707,.T.);
#62250=ORIENTED_EDGE('',*,*,#43057,.T.);
#62251=ORIENTED_EDGE('',*,*,#43059,.F.);
#62252=ORIENTED_EDGE('',*,*,#43060,.F.);
#62253=ORIENTED_EDGE('',*,*,#42713,.T.);
#62254=ORIENTED_EDGE('',*,*,#42712,.T.);
#62255=ORIENTED_EDGE('',*,*,#43061,.F.);
#62256=ORIENTED_EDGE('',*,*,#42716,.T.);
#62257=ORIENTED_EDGE('',*,*,#42714,.T.);
#62258=ORIENTED_EDGE('',*,*,#43060,.T.);
#62259=ORIENTED_EDGE('',*,*,#43062,.F.);
#62260=ORIENTED_EDGE('',*,*,#43063,.F.);
#62261=ORIENTED_EDGE('',*,*,#42720,.T.);
#62262=ORIENTED_EDGE('',*,*,#42719,.T.);
#62263=ORIENTED_EDGE('',*,*,#43064,.F.);
#62264=ORIENTED_EDGE('',*,*,#42723,.T.);
#62265=ORIENTED_EDGE('',*,*,#42721,.T.);
#62266=ORIENTED_EDGE('',*,*,#43063,.T.);
#62267=ORIENTED_EDGE('',*,*,#43065,.F.);
#62268=ORIENTED_EDGE('',*,*,#43066,.F.);
#62269=ORIENTED_EDGE('',*,*,#42727,.T.);
#62270=ORIENTED_EDGE('',*,*,#42726,.T.);
#62271=ORIENTED_EDGE('',*,*,#43067,.F.);
#62272=ORIENTED_EDGE('',*,*,#42730,.T.);
#62273=ORIENTED_EDGE('',*,*,#42728,.T.);
#62274=ORIENTED_EDGE('',*,*,#43066,.T.);
#62275=ORIENTED_EDGE('',*,*,#43068,.F.);
#62276=ORIENTED_EDGE('',*,*,#43069,.F.);
#62277=ORIENTED_EDGE('',*,*,#42734,.T.);
#62278=ORIENTED_EDGE('',*,*,#42733,.T.);
#62279=ORIENTED_EDGE('',*,*,#43070,.F.);
#62280=ORIENTED_EDGE('',*,*,#42737,.T.);
#62281=ORIENTED_EDGE('',*,*,#42735,.T.);
#62282=ORIENTED_EDGE('',*,*,#43069,.T.);
#62283=ORIENTED_EDGE('',*,*,#43071,.F.);
#62284=ORIENTED_EDGE('',*,*,#43072,.F.);
#62285=ORIENTED_EDGE('',*,*,#42741,.T.);
#62286=ORIENTED_EDGE('',*,*,#42740,.T.);
#62287=ORIENTED_EDGE('',*,*,#43073,.F.);
#62288=ORIENTED_EDGE('',*,*,#42744,.T.);
#62289=ORIENTED_EDGE('',*,*,#42742,.T.);
#62290=ORIENTED_EDGE('',*,*,#43072,.T.);
#62291=ORIENTED_EDGE('',*,*,#43074,.F.);
#62292=ORIENTED_EDGE('',*,*,#43075,.F.);
#62293=ORIENTED_EDGE('',*,*,#42750,.T.);
#62294=ORIENTED_EDGE('',*,*,#42747,.T.);
#62295=ORIENTED_EDGE('',*,*,#42751,.T.);
#62296=ORIENTED_EDGE('',*,*,#43075,.T.);
#62297=ORIENTED_EDGE('',*,*,#43076,.F.);
#62298=ORIENTED_EDGE('',*,*,#42749,.T.);
#62299=ORIENTED_EDGE('',*,*,#42756,.T.);
#62300=ORIENTED_EDGE('',*,*,#42752,.T.);
#62301=ORIENTED_EDGE('',*,*,#43077,.F.);
#62302=ORIENTED_EDGE('',*,*,#43078,.F.);
#62303=ORIENTED_EDGE('',*,*,#43079,.F.);
#62304=ORIENTED_EDGE('',*,*,#42758,.T.);
#62305=ORIENTED_EDGE('',*,*,#42757,.T.);
#62306=ORIENTED_EDGE('',*,*,#43078,.T.);
#62307=ORIENTED_EDGE('',*,*,#43080,.F.);
#62308=ORIENTED_EDGE('',*,*,#43081,.F.);
#62309=ORIENTED_EDGE('',*,*,#42762,.T.);
#62310=ORIENTED_EDGE('',*,*,#42761,.T.);
#62311=ORIENTED_EDGE('',*,*,#43082,.F.);
#62312=ORIENTED_EDGE('',*,*,#42765,.T.);
#62313=ORIENTED_EDGE('',*,*,#42763,.T.);
#62314=ORIENTED_EDGE('',*,*,#43081,.T.);
#62315=ORIENTED_EDGE('',*,*,#43083,.F.);
#62316=ORIENTED_EDGE('',*,*,#43084,.F.);
#62317=ORIENTED_EDGE('',*,*,#42769,.T.);
#62318=ORIENTED_EDGE('',*,*,#42768,.T.);
#62319=ORIENTED_EDGE('',*,*,#43085,.F.);
#62320=ORIENTED_EDGE('',*,*,#42772,.T.);
#62321=ORIENTED_EDGE('',*,*,#42770,.T.);
#62322=ORIENTED_EDGE('',*,*,#43084,.T.);
#62323=ORIENTED_EDGE('',*,*,#43086,.F.);
#62324=ORIENTED_EDGE('',*,*,#43087,.F.);
#62325=ORIENTED_EDGE('',*,*,#42776,.T.);
#62326=ORIENTED_EDGE('',*,*,#42775,.T.);
#62327=ORIENTED_EDGE('',*,*,#43088,.F.);
#62328=ORIENTED_EDGE('',*,*,#42779,.T.);
#62329=ORIENTED_EDGE('',*,*,#42777,.T.);
#62330=ORIENTED_EDGE('',*,*,#43087,.T.);
#62331=ORIENTED_EDGE('',*,*,#43089,.F.);
#62332=ORIENTED_EDGE('',*,*,#43090,.F.);
#62333=ORIENTED_EDGE('',*,*,#42783,.T.);
#62334=ORIENTED_EDGE('',*,*,#42782,.T.);
#62335=ORIENTED_EDGE('',*,*,#43091,.F.);
#62336=ORIENTED_EDGE('',*,*,#42786,.T.);
#62337=ORIENTED_EDGE('',*,*,#42784,.T.);
#62338=ORIENTED_EDGE('',*,*,#43090,.T.);
#62339=ORIENTED_EDGE('',*,*,#43092,.F.);
#62340=ORIENTED_EDGE('',*,*,#43093,.F.);
#62341=ORIENTED_EDGE('',*,*,#42790,.T.);
#62342=ORIENTED_EDGE('',*,*,#42789,.T.);
#62343=ORIENTED_EDGE('',*,*,#43094,.F.);
#62344=ORIENTED_EDGE('',*,*,#42793,.T.);
#62345=ORIENTED_EDGE('',*,*,#42791,.T.);
#62346=ORIENTED_EDGE('',*,*,#43093,.T.);
#62347=ORIENTED_EDGE('',*,*,#43095,.F.);
#62348=ORIENTED_EDGE('',*,*,#43096,.F.);
#62349=ORIENTED_EDGE('',*,*,#42797,.T.);
#62350=ORIENTED_EDGE('',*,*,#42796,.T.);
#62351=ORIENTED_EDGE('',*,*,#43097,.F.);
#62352=ORIENTED_EDGE('',*,*,#42800,.T.);
#62353=ORIENTED_EDGE('',*,*,#42798,.T.);
#62354=ORIENTED_EDGE('',*,*,#43096,.T.);
#62355=ORIENTED_EDGE('',*,*,#43098,.F.);
#62356=ORIENTED_EDGE('',*,*,#43099,.F.);
#62357=ORIENTED_EDGE('',*,*,#42804,.T.);
#62358=ORIENTED_EDGE('',*,*,#42803,.T.);
#62359=ORIENTED_EDGE('',*,*,#43100,.F.);
#62360=ORIENTED_EDGE('',*,*,#42807,.T.);
#62361=ORIENTED_EDGE('',*,*,#42805,.T.);
#62362=ORIENTED_EDGE('',*,*,#43099,.T.);
#62363=ORIENTED_EDGE('',*,*,#43101,.F.);
#62364=ORIENTED_EDGE('',*,*,#43102,.F.);
#62365=ORIENTED_EDGE('',*,*,#42811,.T.);
#62366=ORIENTED_EDGE('',*,*,#42810,.T.);
#62367=ORIENTED_EDGE('',*,*,#43103,.F.);
#62368=ORIENTED_EDGE('',*,*,#42814,.T.);
#62369=ORIENTED_EDGE('',*,*,#42812,.T.);
#62370=ORIENTED_EDGE('',*,*,#43102,.T.);
#62371=ORIENTED_EDGE('',*,*,#43104,.F.);
#62372=ORIENTED_EDGE('',*,*,#43105,.F.);
#62373=ORIENTED_EDGE('',*,*,#42818,.T.);
#62374=ORIENTED_EDGE('',*,*,#42817,.T.);
#62375=ORIENTED_EDGE('',*,*,#43106,.F.);
#62376=ORIENTED_EDGE('',*,*,#42821,.T.);
#62377=ORIENTED_EDGE('',*,*,#42819,.T.);
#62378=ORIENTED_EDGE('',*,*,#43105,.T.);
#62379=ORIENTED_EDGE('',*,*,#43107,.F.);
#62380=ORIENTED_EDGE('',*,*,#43022,.T.);
#62381=ORIENTED_EDGE('',*,*,#42822,.T.);
#62382=ORIENTED_EDGE('',*,*,#42825,.T.);
#62383=ORIENTED_EDGE('',*,*,#43108,.F.);
#62384=ORIENTED_EDGE('',*,*,#42828,.T.);
#62385=ORIENTED_EDGE('',*,*,#43019,.T.);
#62386=ORIENTED_EDGE('',*,*,#43109,.F.);
#62387=ORIENTED_EDGE('',*,*,#43110,.F.);
#62388=ORIENTED_EDGE('',*,*,#43111,.F.);
#62389=ORIENTED_EDGE('',*,*,#42832,.T.);
#62390=ORIENTED_EDGE('',*,*,#42829,.T.);
#62391=ORIENTED_EDGE('',*,*,#43112,.F.);
#62392=ORIENTED_EDGE('',*,*,#42835,.T.);
#62393=ORIENTED_EDGE('',*,*,#42833,.T.);
#62394=ORIENTED_EDGE('',*,*,#43111,.T.);
#62395=ORIENTED_EDGE('',*,*,#43113,.F.);
#62396=ORIENTED_EDGE('',*,*,#43114,.F.);
#62397=ORIENTED_EDGE('',*,*,#42839,.T.);
#62398=ORIENTED_EDGE('',*,*,#42836,.T.);
#62399=ORIENTED_EDGE('',*,*,#43115,.F.);
#62400=ORIENTED_EDGE('',*,*,#42842,.T.);
#62401=ORIENTED_EDGE('',*,*,#42840,.T.);
#62402=ORIENTED_EDGE('',*,*,#43114,.T.);
#62403=ORIENTED_EDGE('',*,*,#43116,.F.);
#62404=ORIENTED_EDGE('',*,*,#43117,.F.);
#62405=ORIENTED_EDGE('',*,*,#42846,.T.);
#62406=ORIENTED_EDGE('',*,*,#42843,.T.);
#62407=ORIENTED_EDGE('',*,*,#43118,.F.);
#62408=ORIENTED_EDGE('',*,*,#42849,.T.);
#62409=ORIENTED_EDGE('',*,*,#42847,.T.);
#62410=ORIENTED_EDGE('',*,*,#43117,.T.);
#62411=ORIENTED_EDGE('',*,*,#43119,.F.);
#62412=ORIENTED_EDGE('',*,*,#43120,.F.);
#62413=ORIENTED_EDGE('',*,*,#42853,.T.);
#62414=ORIENTED_EDGE('',*,*,#42850,.T.);
#62415=ORIENTED_EDGE('',*,*,#43121,.F.);
#62416=ORIENTED_EDGE('',*,*,#42856,.T.);
#62417=ORIENTED_EDGE('',*,*,#42854,.T.);
#62418=ORIENTED_EDGE('',*,*,#43120,.T.);
#62419=ORIENTED_EDGE('',*,*,#43122,.F.);
#62420=ORIENTED_EDGE('',*,*,#43123,.F.);
#62421=ORIENTED_EDGE('',*,*,#42860,.T.);
#62422=ORIENTED_EDGE('',*,*,#42857,.T.);
#62423=ORIENTED_EDGE('',*,*,#43124,.F.);
#62424=ORIENTED_EDGE('',*,*,#42863,.T.);
#62425=ORIENTED_EDGE('',*,*,#42861,.T.);
#62426=ORIENTED_EDGE('',*,*,#43123,.T.);
#62427=ORIENTED_EDGE('',*,*,#43125,.F.);
#62428=ORIENTED_EDGE('',*,*,#43126,.F.);
#62429=ORIENTED_EDGE('',*,*,#42867,.T.);
#62430=ORIENTED_EDGE('',*,*,#42864,.T.);
#62431=ORIENTED_EDGE('',*,*,#43127,.F.);
#62432=ORIENTED_EDGE('',*,*,#42870,.T.);
#62433=ORIENTED_EDGE('',*,*,#42868,.T.);
#62434=ORIENTED_EDGE('',*,*,#43126,.T.);
#62435=ORIENTED_EDGE('',*,*,#43128,.F.);
#62436=ORIENTED_EDGE('',*,*,#43129,.F.);
#62437=ORIENTED_EDGE('',*,*,#42874,.T.);
#62438=ORIENTED_EDGE('',*,*,#42871,.T.);
#62439=ORIENTED_EDGE('',*,*,#43130,.F.);
#62440=ORIENTED_EDGE('',*,*,#42877,.T.);
#62441=ORIENTED_EDGE('',*,*,#42875,.T.);
#62442=ORIENTED_EDGE('',*,*,#43129,.T.);
#62443=ORIENTED_EDGE('',*,*,#43131,.F.);
#62444=ORIENTED_EDGE('',*,*,#43132,.F.);
#62445=ORIENTED_EDGE('',*,*,#42881,.T.);
#62446=ORIENTED_EDGE('',*,*,#42878,.T.);
#62447=ORIENTED_EDGE('',*,*,#43133,.F.);
#62448=ORIENTED_EDGE('',*,*,#42884,.T.);
#62449=ORIENTED_EDGE('',*,*,#42882,.T.);
#62450=ORIENTED_EDGE('',*,*,#43132,.T.);
#62451=ORIENTED_EDGE('',*,*,#43134,.F.);
#62452=ORIENTED_EDGE('',*,*,#43135,.F.);
#62453=ORIENTED_EDGE('',*,*,#42888,.T.);
#62454=ORIENTED_EDGE('',*,*,#42885,.T.);
#62455=ORIENTED_EDGE('',*,*,#43136,.F.);
#62456=ORIENTED_EDGE('',*,*,#42891,.T.);
#62457=ORIENTED_EDGE('',*,*,#42889,.T.);
#62458=ORIENTED_EDGE('',*,*,#43135,.T.);
#62459=ORIENTED_EDGE('',*,*,#43137,.F.);
#62460=ORIENTED_EDGE('',*,*,#43138,.F.);
#62461=ORIENTED_EDGE('',*,*,#42895,.T.);
#62462=ORIENTED_EDGE('',*,*,#42892,.T.);
#62463=ORIENTED_EDGE('',*,*,#43139,.F.);
#62464=ORIENTED_EDGE('',*,*,#42898,.T.);
#62465=ORIENTED_EDGE('',*,*,#42896,.T.);
#62466=ORIENTED_EDGE('',*,*,#43138,.T.);
#62467=ORIENTED_EDGE('',*,*,#43140,.F.);
#62468=ORIENTED_EDGE('',*,*,#43141,.F.);
#62469=ORIENTED_EDGE('',*,*,#42902,.T.);
#62470=ORIENTED_EDGE('',*,*,#42899,.T.);
#62471=ORIENTED_EDGE('',*,*,#43142,.F.);
#62472=ORIENTED_EDGE('',*,*,#42905,.T.);
#62473=ORIENTED_EDGE('',*,*,#42903,.T.);
#62474=ORIENTED_EDGE('',*,*,#43141,.T.);
#62475=ORIENTED_EDGE('',*,*,#43143,.F.);
#62476=ORIENTED_EDGE('',*,*,#43144,.F.);
#62477=ORIENTED_EDGE('',*,*,#42909,.T.);
#62478=ORIENTED_EDGE('',*,*,#42906,.T.);
#62479=ORIENTED_EDGE('',*,*,#43145,.F.);
#62480=ORIENTED_EDGE('',*,*,#42912,.T.);
#62481=ORIENTED_EDGE('',*,*,#42910,.T.);
#62482=ORIENTED_EDGE('',*,*,#43144,.T.);
#62483=ORIENTED_EDGE('',*,*,#43146,.F.);
#62484=ORIENTED_EDGE('',*,*,#43147,.F.);
#62485=ORIENTED_EDGE('',*,*,#42916,.T.);
#62486=ORIENTED_EDGE('',*,*,#42913,.T.);
#62487=ORIENTED_EDGE('',*,*,#43148,.F.);
#62488=ORIENTED_EDGE('',*,*,#42919,.T.);
#62489=ORIENTED_EDGE('',*,*,#42917,.T.);
#62490=ORIENTED_EDGE('',*,*,#43147,.T.);
#62491=ORIENTED_EDGE('',*,*,#43149,.F.);
#62492=ORIENTED_EDGE('',*,*,#43150,.F.);
#62493=ORIENTED_EDGE('',*,*,#34357,.T.);
#62494=ORIENTED_EDGE('',*,*,#42920,.T.);
#62495=ORIENTED_EDGE('',*,*,#42922,.T.);
#62496=ORIENTED_EDGE('',*,*,#34354,.T.);
#62497=ORIENTED_EDGE('',*,*,#43150,.T.);
#62498=ORIENTED_EDGE('',*,*,#43151,.F.);
#62499=ORIENTED_EDGE('',*,*,#43152,.F.);
#62500=ORIENTED_EDGE('',*,*,#43153,.F.);
#62501=ORIENTED_EDGE('',*,*,#42926,.T.);
#62502=ORIENTED_EDGE('',*,*,#42923,.T.);
#62503=ORIENTED_EDGE('',*,*,#43154,.F.);
#62504=ORIENTED_EDGE('',*,*,#42929,.T.);
#62505=ORIENTED_EDGE('',*,*,#42927,.T.);
#62506=ORIENTED_EDGE('',*,*,#43153,.T.);
#62507=ORIENTED_EDGE('',*,*,#43155,.F.);
#62508=ORIENTED_EDGE('',*,*,#43156,.F.);
#62509=ORIENTED_EDGE('',*,*,#42933,.T.);
#62510=ORIENTED_EDGE('',*,*,#42930,.T.);
#62511=ORIENTED_EDGE('',*,*,#43157,.F.);
#62512=ORIENTED_EDGE('',*,*,#42936,.T.);
#62513=ORIENTED_EDGE('',*,*,#42934,.T.);
#62514=ORIENTED_EDGE('',*,*,#43156,.T.);
#62515=ORIENTED_EDGE('',*,*,#43158,.F.);
#62516=ORIENTED_EDGE('',*,*,#43159,.F.);
#62517=ORIENTED_EDGE('',*,*,#42940,.T.);
#62518=ORIENTED_EDGE('',*,*,#42937,.T.);
#62519=ORIENTED_EDGE('',*,*,#43160,.F.);
#62520=ORIENTED_EDGE('',*,*,#42943,.T.);
#62521=ORIENTED_EDGE('',*,*,#42941,.T.);
#62522=ORIENTED_EDGE('',*,*,#43159,.T.);
#62523=ORIENTED_EDGE('',*,*,#43161,.F.);
#62524=ORIENTED_EDGE('',*,*,#43162,.F.);
#62525=ORIENTED_EDGE('',*,*,#42947,.T.);
#62526=ORIENTED_EDGE('',*,*,#42944,.T.);
#62527=ORIENTED_EDGE('',*,*,#43163,.F.);
#62528=ORIENTED_EDGE('',*,*,#42950,.T.);
#62529=ORIENTED_EDGE('',*,*,#42948,.T.);
#62530=ORIENTED_EDGE('',*,*,#43162,.T.);
#62531=ORIENTED_EDGE('',*,*,#43164,.F.);
#62532=ORIENTED_EDGE('',*,*,#43165,.F.);
#62533=ORIENTED_EDGE('',*,*,#42954,.T.);
#62534=ORIENTED_EDGE('',*,*,#42951,.T.);
#62535=ORIENTED_EDGE('',*,*,#43166,.F.);
#62536=ORIENTED_EDGE('',*,*,#42957,.T.);
#62537=ORIENTED_EDGE('',*,*,#42955,.T.);
#62538=ORIENTED_EDGE('',*,*,#43165,.T.);
#62539=ORIENTED_EDGE('',*,*,#43167,.F.);
#62540=ORIENTED_EDGE('',*,*,#43168,.F.);
#62541=ORIENTED_EDGE('',*,*,#42961,.T.);
#62542=ORIENTED_EDGE('',*,*,#42958,.T.);
#62543=ORIENTED_EDGE('',*,*,#43169,.F.);
#62544=ORIENTED_EDGE('',*,*,#42964,.T.);
#62545=ORIENTED_EDGE('',*,*,#42962,.T.);
#62546=ORIENTED_EDGE('',*,*,#43168,.T.);
#62547=ORIENTED_EDGE('',*,*,#43170,.F.);
#62548=ORIENTED_EDGE('',*,*,#43171,.F.);
#62549=ORIENTED_EDGE('',*,*,#34353,.T.);
#62550=ORIENTED_EDGE('',*,*,#42965,.T.);
#62551=ORIENTED_EDGE('',*,*,#43172,.F.);
#62552=ORIENTED_EDGE('',*,*,#42967,.T.);
#62553=ORIENTED_EDGE('',*,*,#34350,.T.);
#62554=ORIENTED_EDGE('',*,*,#43171,.T.);
#62555=ORIENTED_EDGE('',*,*,#43173,.F.);
#62556=ORIENTED_EDGE('',*,*,#43174,.F.);
#62557=ORIENTED_EDGE('',*,*,#42971,.T.);
#62558=ORIENTED_EDGE('',*,*,#42968,.T.);
#62559=ORIENTED_EDGE('',*,*,#43175,.F.);
#62560=ORIENTED_EDGE('',*,*,#42974,.T.);
#62561=ORIENTED_EDGE('',*,*,#42972,.T.);
#62562=ORIENTED_EDGE('',*,*,#43174,.T.);
#62563=ORIENTED_EDGE('',*,*,#43176,.F.);
#62564=ORIENTED_EDGE('',*,*,#43177,.F.);
#62565=ORIENTED_EDGE('',*,*,#42978,.T.);
#62566=ORIENTED_EDGE('',*,*,#42975,.T.);
#62567=ORIENTED_EDGE('',*,*,#43178,.F.);
#62568=ORIENTED_EDGE('',*,*,#42981,.T.);
#62569=ORIENTED_EDGE('',*,*,#42979,.T.);
#62570=ORIENTED_EDGE('',*,*,#43177,.T.);
#62571=ORIENTED_EDGE('',*,*,#43179,.F.);
#62572=ORIENTED_EDGE('',*,*,#43180,.F.);
#62573=ORIENTED_EDGE('',*,*,#42985,.T.);
#62574=ORIENTED_EDGE('',*,*,#42982,.T.);
#62575=ORIENTED_EDGE('',*,*,#43181,.F.);
#62576=ORIENTED_EDGE('',*,*,#42988,.T.);
#62577=ORIENTED_EDGE('',*,*,#42986,.T.);
#62578=ORIENTED_EDGE('',*,*,#43180,.T.);
#62579=ORIENTED_EDGE('',*,*,#43182,.F.);
#62580=ORIENTED_EDGE('',*,*,#43183,.F.);
#62581=ORIENTED_EDGE('',*,*,#42992,.T.);
#62582=ORIENTED_EDGE('',*,*,#42989,.T.);
#62583=ORIENTED_EDGE('',*,*,#43184,.F.);
#62584=ORIENTED_EDGE('',*,*,#42995,.T.);
#62585=ORIENTED_EDGE('',*,*,#42993,.T.);
#62586=ORIENTED_EDGE('',*,*,#43183,.T.);
#62587=ORIENTED_EDGE('',*,*,#43185,.F.);
#62588=ORIENTED_EDGE('',*,*,#43186,.F.);
#62589=ORIENTED_EDGE('',*,*,#42999,.T.);
#62590=ORIENTED_EDGE('',*,*,#42996,.T.);
#62591=ORIENTED_EDGE('',*,*,#43187,.F.);
#62592=ORIENTED_EDGE('',*,*,#43002,.T.);
#62593=ORIENTED_EDGE('',*,*,#43000,.T.);
#62594=ORIENTED_EDGE('',*,*,#43186,.T.);
#62595=ORIENTED_EDGE('',*,*,#43188,.F.);
#62596=ORIENTED_EDGE('',*,*,#43189,.F.);
#62597=ORIENTED_EDGE('',*,*,#43006,.T.);
#62598=ORIENTED_EDGE('',*,*,#43003,.T.);
#62599=ORIENTED_EDGE('',*,*,#43190,.F.);
#62600=ORIENTED_EDGE('',*,*,#43009,.T.);
#62601=ORIENTED_EDGE('',*,*,#43007,.T.);
#62602=ORIENTED_EDGE('',*,*,#43189,.T.);
#62603=ORIENTED_EDGE('',*,*,#43191,.F.);
#62604=ORIENTED_EDGE('',*,*,#43192,.F.);
#62605=ORIENTED_EDGE('',*,*,#43013,.T.);
#62606=ORIENTED_EDGE('',*,*,#43010,.T.);
#62607=ORIENTED_EDGE('',*,*,#43193,.F.);
#62608=ORIENTED_EDGE('',*,*,#43016,.T.);
#62609=ORIENTED_EDGE('',*,*,#43014,.T.);
#62610=ORIENTED_EDGE('',*,*,#43192,.T.);
#62611=ORIENTED_EDGE('',*,*,#43194,.F.);
#62612=ORIENTED_EDGE('',*,*,#43109,.T.);
#62613=ORIENTED_EDGE('',*,*,#43018,.T.);
#62614=ORIENTED_EDGE('',*,*,#43020,.T.);
#62615=ORIENTED_EDGE('',*,*,#43195,.T.);
#62616=ORIENTED_EDGE('',*,*,#43196,.F.);
#62617=ORIENTED_EDGE('',*,*,#43021,.T.);
#62618=ORIENTED_EDGE('',*,*,#43197,.F.);
#62619=ORIENTED_EDGE('',*,*,#43198,.F.);
#62620=ORIENTED_EDGE('',*,*,#43199,.F.);
#62621=ORIENTED_EDGE('',*,*,#43200,.F.);
#62622=ORIENTED_EDGE('',*,*,#43195,.F.);
#62623=ORIENTED_EDGE('',*,*,#43200,.T.);
#62624=ORIENTED_EDGE('',*,*,#43201,.F.);
#62625=ORIENTED_EDGE('',*,*,#43023,.T.);
#62626=ORIENTED_EDGE('',*,*,#43196,.T.);
#62627=ORIENTED_EDGE('',*,*,#43202,.T.);
#62628=ORIENTED_EDGE('',*,*,#43203,.F.);
#62629=ORIENTED_EDGE('',*,*,#43025,.T.);
#62630=ORIENTED_EDGE('',*,*,#43204,.F.);
#62631=ORIENTED_EDGE('',*,*,#43205,.F.);
#62632=ORIENTED_EDGE('',*,*,#43206,.F.);
#62633=ORIENTED_EDGE('',*,*,#43207,.F.);
#62634=ORIENTED_EDGE('',*,*,#43202,.F.);
#62635=ORIENTED_EDGE('',*,*,#43207,.T.);
#62636=ORIENTED_EDGE('',*,*,#43208,.F.);
#62637=ORIENTED_EDGE('',*,*,#43026,.T.);
#62638=ORIENTED_EDGE('',*,*,#43203,.T.);
#62639=ORIENTED_EDGE('',*,*,#43209,.T.);
#62640=ORIENTED_EDGE('',*,*,#43210,.F.);
#62641=ORIENTED_EDGE('',*,*,#43028,.T.);
#62642=ORIENTED_EDGE('',*,*,#43211,.F.);
#62643=ORIENTED_EDGE('',*,*,#43212,.F.);
#62644=ORIENTED_EDGE('',*,*,#43213,.F.);
#62645=ORIENTED_EDGE('',*,*,#43214,.F.);
#62646=ORIENTED_EDGE('',*,*,#43209,.F.);
#62647=ORIENTED_EDGE('',*,*,#43214,.T.);
#62648=ORIENTED_EDGE('',*,*,#43215,.F.);
#62649=ORIENTED_EDGE('',*,*,#43029,.T.);
#62650=ORIENTED_EDGE('',*,*,#43210,.T.);
#62651=ORIENTED_EDGE('',*,*,#43216,.T.);
#62652=ORIENTED_EDGE('',*,*,#43217,.F.);
#62653=ORIENTED_EDGE('',*,*,#43031,.T.);
#62654=ORIENTED_EDGE('',*,*,#43218,.F.);
#62655=ORIENTED_EDGE('',*,*,#43219,.F.);
#62656=ORIENTED_EDGE('',*,*,#43220,.F.);
#62657=ORIENTED_EDGE('',*,*,#43221,.F.);
#62658=ORIENTED_EDGE('',*,*,#43216,.F.);
#62659=ORIENTED_EDGE('',*,*,#43221,.T.);
#62660=ORIENTED_EDGE('',*,*,#43222,.F.);
#62661=ORIENTED_EDGE('',*,*,#43032,.T.);
#62662=ORIENTED_EDGE('',*,*,#43217,.T.);
#62663=ORIENTED_EDGE('',*,*,#43223,.T.);
#62664=ORIENTED_EDGE('',*,*,#43224,.F.);
#62665=ORIENTED_EDGE('',*,*,#43034,.T.);
#62666=ORIENTED_EDGE('',*,*,#43225,.F.);
#62667=ORIENTED_EDGE('',*,*,#43226,.F.);
#62668=ORIENTED_EDGE('',*,*,#43227,.F.);
#62669=ORIENTED_EDGE('',*,*,#43228,.F.);
#62670=ORIENTED_EDGE('',*,*,#43223,.F.);
#62671=ORIENTED_EDGE('',*,*,#43228,.T.);
#62672=ORIENTED_EDGE('',*,*,#43229,.F.);
#62673=ORIENTED_EDGE('',*,*,#43035,.T.);
#62674=ORIENTED_EDGE('',*,*,#43224,.T.);
#62675=ORIENTED_EDGE('',*,*,#43230,.T.);
#62676=ORIENTED_EDGE('',*,*,#43231,.F.);
#62677=ORIENTED_EDGE('',*,*,#43037,.T.);
#62678=ORIENTED_EDGE('',*,*,#43232,.F.);
#62679=ORIENTED_EDGE('',*,*,#43233,.F.);
#62680=ORIENTED_EDGE('',*,*,#43234,.F.);
#62681=ORIENTED_EDGE('',*,*,#43235,.F.);
#62682=ORIENTED_EDGE('',*,*,#43230,.F.);
#62683=ORIENTED_EDGE('',*,*,#43235,.T.);
#62684=ORIENTED_EDGE('',*,*,#43236,.F.);
#62685=ORIENTED_EDGE('',*,*,#43038,.T.);
#62686=ORIENTED_EDGE('',*,*,#43231,.T.);
#62687=ORIENTED_EDGE('',*,*,#43237,.T.);
#62688=ORIENTED_EDGE('',*,*,#43238,.F.);
#62689=ORIENTED_EDGE('',*,*,#43040,.T.);
#62690=ORIENTED_EDGE('',*,*,#43239,.F.);
#62691=ORIENTED_EDGE('',*,*,#43240,.F.);
#62692=ORIENTED_EDGE('',*,*,#43241,.F.);
#62693=ORIENTED_EDGE('',*,*,#43242,.F.);
#62694=ORIENTED_EDGE('',*,*,#43237,.F.);
#62695=ORIENTED_EDGE('',*,*,#43242,.T.);
#62696=ORIENTED_EDGE('',*,*,#43243,.F.);
#62697=ORIENTED_EDGE('',*,*,#43041,.T.);
#62698=ORIENTED_EDGE('',*,*,#43238,.T.);
#62699=ORIENTED_EDGE('',*,*,#43244,.T.);
#62700=ORIENTED_EDGE('',*,*,#43245,.F.);
#62701=ORIENTED_EDGE('',*,*,#43043,.T.);
#62702=ORIENTED_EDGE('',*,*,#43246,.F.);
#62703=ORIENTED_EDGE('',*,*,#43247,.F.);
#62704=ORIENTED_EDGE('',*,*,#43248,.F.);
#62705=ORIENTED_EDGE('',*,*,#43249,.F.);
#62706=ORIENTED_EDGE('',*,*,#43244,.F.);
#62707=ORIENTED_EDGE('',*,*,#43249,.T.);
#62708=ORIENTED_EDGE('',*,*,#43250,.F.);
#62709=ORIENTED_EDGE('',*,*,#43044,.T.);
#62710=ORIENTED_EDGE('',*,*,#43245,.T.);
#62711=ORIENTED_EDGE('',*,*,#43251,.T.);
#62712=ORIENTED_EDGE('',*,*,#43252,.F.);
#62713=ORIENTED_EDGE('',*,*,#43046,.T.);
#62714=ORIENTED_EDGE('',*,*,#43253,.F.);
#62715=ORIENTED_EDGE('',*,*,#43254,.F.);
#62716=ORIENTED_EDGE('',*,*,#43255,.F.);
#62717=ORIENTED_EDGE('',*,*,#43256,.F.);
#62718=ORIENTED_EDGE('',*,*,#43251,.F.);
#62719=ORIENTED_EDGE('',*,*,#43256,.T.);
#62720=ORIENTED_EDGE('',*,*,#43257,.F.);
#62721=ORIENTED_EDGE('',*,*,#43047,.T.);
#62722=ORIENTED_EDGE('',*,*,#43252,.T.);
#62723=ORIENTED_EDGE('',*,*,#43258,.T.);
#62724=ORIENTED_EDGE('',*,*,#43259,.F.);
#62725=ORIENTED_EDGE('',*,*,#43049,.T.);
#62726=ORIENTED_EDGE('',*,*,#43260,.F.);
#62727=ORIENTED_EDGE('',*,*,#43261,.F.);
#62728=ORIENTED_EDGE('',*,*,#43262,.F.);
#62729=ORIENTED_EDGE('',*,*,#43263,.F.);
#62730=ORIENTED_EDGE('',*,*,#43258,.F.);
#62731=ORIENTED_EDGE('',*,*,#43263,.T.);
#62732=ORIENTED_EDGE('',*,*,#43264,.F.);
#62733=ORIENTED_EDGE('',*,*,#43050,.T.);
#62734=ORIENTED_EDGE('',*,*,#43259,.T.);
#62735=ORIENTED_EDGE('',*,*,#43265,.T.);
#62736=ORIENTED_EDGE('',*,*,#43266,.F.);
#62737=ORIENTED_EDGE('',*,*,#43052,.T.);
#62738=ORIENTED_EDGE('',*,*,#43267,.F.);
#62739=ORIENTED_EDGE('',*,*,#43268,.F.);
#62740=ORIENTED_EDGE('',*,*,#43269,.F.);
#62741=ORIENTED_EDGE('',*,*,#43270,.F.);
#62742=ORIENTED_EDGE('',*,*,#43265,.F.);
#62743=ORIENTED_EDGE('',*,*,#43270,.T.);
#62744=ORIENTED_EDGE('',*,*,#43271,.F.);
#62745=ORIENTED_EDGE('',*,*,#43053,.T.);
#62746=ORIENTED_EDGE('',*,*,#43266,.T.);
#62747=ORIENTED_EDGE('',*,*,#43272,.T.);
#62748=ORIENTED_EDGE('',*,*,#43273,.F.);
#62749=ORIENTED_EDGE('',*,*,#43055,.T.);
#62750=ORIENTED_EDGE('',*,*,#43274,.F.);
#62751=ORIENTED_EDGE('',*,*,#43275,.F.);
#62752=ORIENTED_EDGE('',*,*,#43276,.F.);
#62753=ORIENTED_EDGE('',*,*,#43277,.F.);
#62754=ORIENTED_EDGE('',*,*,#43272,.F.);
#62755=ORIENTED_EDGE('',*,*,#43277,.T.);
#62756=ORIENTED_EDGE('',*,*,#43278,.F.);
#62757=ORIENTED_EDGE('',*,*,#43056,.T.);
#62758=ORIENTED_EDGE('',*,*,#43273,.T.);
#62759=ORIENTED_EDGE('',*,*,#43279,.T.);
#62760=ORIENTED_EDGE('',*,*,#43280,.F.);
#62761=ORIENTED_EDGE('',*,*,#43058,.T.);
#62762=ORIENTED_EDGE('',*,*,#43281,.F.);
#62763=ORIENTED_EDGE('',*,*,#43282,.F.);
#62764=ORIENTED_EDGE('',*,*,#43283,.F.);
#62765=ORIENTED_EDGE('',*,*,#43284,.F.);
#62766=ORIENTED_EDGE('',*,*,#43279,.F.);
#62767=ORIENTED_EDGE('',*,*,#43284,.T.);
#62768=ORIENTED_EDGE('',*,*,#43285,.F.);
#62769=ORIENTED_EDGE('',*,*,#43059,.T.);
#62770=ORIENTED_EDGE('',*,*,#43280,.T.);
#62771=ORIENTED_EDGE('',*,*,#43286,.T.);
#62772=ORIENTED_EDGE('',*,*,#43287,.F.);
#62773=ORIENTED_EDGE('',*,*,#43061,.T.);
#62774=ORIENTED_EDGE('',*,*,#43288,.F.);
#62775=ORIENTED_EDGE('',*,*,#43289,.F.);
#62776=ORIENTED_EDGE('',*,*,#43290,.F.);
#62777=ORIENTED_EDGE('',*,*,#43291,.F.);
#62778=ORIENTED_EDGE('',*,*,#43286,.F.);
#62779=ORIENTED_EDGE('',*,*,#43291,.T.);
#62780=ORIENTED_EDGE('',*,*,#43292,.F.);
#62781=ORIENTED_EDGE('',*,*,#43062,.T.);
#62782=ORIENTED_EDGE('',*,*,#43287,.T.);
#62783=ORIENTED_EDGE('',*,*,#34346,.T.);
#62784=ORIENTED_EDGE('',*,*,#43293,.F.);
#62785=ORIENTED_EDGE('',*,*,#43064,.T.);
#62786=ORIENTED_EDGE('',*,*,#43294,.F.);
#62787=ORIENTED_EDGE('',*,*,#34349,.T.);
#62788=ORIENTED_EDGE('',*,*,#43295,.F.);
#62789=ORIENTED_EDGE('',*,*,#43065,.T.);
#62790=ORIENTED_EDGE('',*,*,#43293,.T.);
#62791=ORIENTED_EDGE('',*,*,#43296,.T.);
#62792=ORIENTED_EDGE('',*,*,#43297,.F.);
#62793=ORIENTED_EDGE('',*,*,#43067,.T.);
#62794=ORIENTED_EDGE('',*,*,#43298,.F.);
#62795=ORIENTED_EDGE('',*,*,#43299,.F.);
#62796=ORIENTED_EDGE('',*,*,#43300,.F.);
#62797=ORIENTED_EDGE('',*,*,#43301,.F.);
#62798=ORIENTED_EDGE('',*,*,#43296,.F.);
#62799=ORIENTED_EDGE('',*,*,#43301,.T.);
#62800=ORIENTED_EDGE('',*,*,#43302,.F.);
#62801=ORIENTED_EDGE('',*,*,#43068,.T.);
#62802=ORIENTED_EDGE('',*,*,#43297,.T.);
#62803=ORIENTED_EDGE('',*,*,#43303,.T.);
#62804=ORIENTED_EDGE('',*,*,#43304,.F.);
#62805=ORIENTED_EDGE('',*,*,#43070,.T.);
#62806=ORIENTED_EDGE('',*,*,#43305,.F.);
#62807=ORIENTED_EDGE('',*,*,#43306,.F.);
#62808=ORIENTED_EDGE('',*,*,#43307,.F.);
#62809=ORIENTED_EDGE('',*,*,#43308,.F.);
#62810=ORIENTED_EDGE('',*,*,#43303,.F.);
#62811=ORIENTED_EDGE('',*,*,#43308,.T.);
#62812=ORIENTED_EDGE('',*,*,#43309,.F.);
#62813=ORIENTED_EDGE('',*,*,#43071,.T.);
#62814=ORIENTED_EDGE('',*,*,#43304,.T.);
#62815=ORIENTED_EDGE('',*,*,#43310,.T.);
#62816=ORIENTED_EDGE('',*,*,#43311,.F.);
#62817=ORIENTED_EDGE('',*,*,#43073,.T.);
#62818=ORIENTED_EDGE('',*,*,#43312,.F.);
#62819=ORIENTED_EDGE('',*,*,#43313,.T.);
#62820=ORIENTED_EDGE('',*,*,#43314,.F.);
#62821=ORIENTED_EDGE('',*,*,#43074,.T.);
#62822=ORIENTED_EDGE('',*,*,#43311,.T.);
#62823=ORIENTED_EDGE('',*,*,#43315,.F.);
#62824=ORIENTED_EDGE('',*,*,#43316,.F.);
#62825=ORIENTED_EDGE('',*,*,#43313,.F.);
#62826=ORIENTED_EDGE('',*,*,#43310,.F.);
#62827=ORIENTED_EDGE('',*,*,#43076,.T.);
#62828=ORIENTED_EDGE('',*,*,#43317,.F.);
#62829=ORIENTED_EDGE('',*,*,#43318,.T.);
#62830=ORIENTED_EDGE('',*,*,#43319,.F.);
#62831=ORIENTED_EDGE('',*,*,#43320,.F.);
#62832=ORIENTED_EDGE('',*,*,#43318,.F.);
#62833=ORIENTED_EDGE('',*,*,#43321,.F.);
#62834=ORIENTED_EDGE('',*,*,#43322,.F.);
#62835=ORIENTED_EDGE('',*,*,#43077,.T.);
#62836=ORIENTED_EDGE('',*,*,#43319,.T.);
#62837=ORIENTED_EDGE('',*,*,#43320,.T.);
#62838=ORIENTED_EDGE('',*,*,#43323,.F.);
#62839=ORIENTED_EDGE('',*,*,#43324,.T.);
#62840=ORIENTED_EDGE('',*,*,#43325,.F.);
#62841=ORIENTED_EDGE('',*,*,#43079,.T.);
#62842=ORIENTED_EDGE('',*,*,#43326,.F.);
#62843=ORIENTED_EDGE('',*,*,#43327,.F.);
#62844=ORIENTED_EDGE('',*,*,#43328,.F.);
#62845=ORIENTED_EDGE('',*,*,#43329,.F.);
#62846=ORIENTED_EDGE('',*,*,#43324,.F.);
#62847=ORIENTED_EDGE('',*,*,#43329,.T.);
#62848=ORIENTED_EDGE('',*,*,#43330,.F.);
#62849=ORIENTED_EDGE('',*,*,#43080,.T.);
#62850=ORIENTED_EDGE('',*,*,#43325,.T.);
#62851=ORIENTED_EDGE('',*,*,#43331,.T.);
#62852=ORIENTED_EDGE('',*,*,#43332,.F.);
#62853=ORIENTED_EDGE('',*,*,#43082,.T.);
#62854=ORIENTED_EDGE('',*,*,#43333,.F.);
#62855=ORIENTED_EDGE('',*,*,#43334,.F.);
#62856=ORIENTED_EDGE('',*,*,#43335,.F.);
#62857=ORIENTED_EDGE('',*,*,#43336,.F.);
#62858=ORIENTED_EDGE('',*,*,#43331,.F.);
#62859=ORIENTED_EDGE('',*,*,#43336,.T.);
#62860=ORIENTED_EDGE('',*,*,#43337,.F.);
#62861=ORIENTED_EDGE('',*,*,#43083,.T.);
#62862=ORIENTED_EDGE('',*,*,#43332,.T.);
#62863=ORIENTED_EDGE('',*,*,#43338,.T.);
#62864=ORIENTED_EDGE('',*,*,#43339,.F.);
#62865=ORIENTED_EDGE('',*,*,#43085,.T.);
#62866=ORIENTED_EDGE('',*,*,#43340,.F.);
#62867=ORIENTED_EDGE('',*,*,#43341,.F.);
#62868=ORIENTED_EDGE('',*,*,#43342,.F.);
#62869=ORIENTED_EDGE('',*,*,#43343,.F.);
#62870=ORIENTED_EDGE('',*,*,#43338,.F.);
#62871=ORIENTED_EDGE('',*,*,#43343,.T.);
#62872=ORIENTED_EDGE('',*,*,#43344,.F.);
#62873=ORIENTED_EDGE('',*,*,#43086,.T.);
#62874=ORIENTED_EDGE('',*,*,#43339,.T.);
#62875=ORIENTED_EDGE('',*,*,#43345,.T.);
#62876=ORIENTED_EDGE('',*,*,#43346,.F.);
#62877=ORIENTED_EDGE('',*,*,#43088,.T.);
#62878=ORIENTED_EDGE('',*,*,#43347,.F.);
#62879=ORIENTED_EDGE('',*,*,#43348,.F.);
#62880=ORIENTED_EDGE('',*,*,#43349,.F.);
#62881=ORIENTED_EDGE('',*,*,#43350,.F.);
#62882=ORIENTED_EDGE('',*,*,#43345,.F.);
#62883=ORIENTED_EDGE('',*,*,#43350,.T.);
#62884=ORIENTED_EDGE('',*,*,#43351,.F.);
#62885=ORIENTED_EDGE('',*,*,#43089,.T.);
#62886=ORIENTED_EDGE('',*,*,#43346,.T.);
#62887=ORIENTED_EDGE('',*,*,#43352,.T.);
#62888=ORIENTED_EDGE('',*,*,#43353,.F.);
#62889=ORIENTED_EDGE('',*,*,#43091,.T.);
#62890=ORIENTED_EDGE('',*,*,#43354,.F.);
#62891=ORIENTED_EDGE('',*,*,#43355,.F.);
#62892=ORIENTED_EDGE('',*,*,#43356,.F.);
#62893=ORIENTED_EDGE('',*,*,#43357,.F.);
#62894=ORIENTED_EDGE('',*,*,#43352,.F.);
#62895=ORIENTED_EDGE('',*,*,#43357,.T.);
#62896=ORIENTED_EDGE('',*,*,#43358,.F.);
#62897=ORIENTED_EDGE('',*,*,#43092,.T.);
#62898=ORIENTED_EDGE('',*,*,#43353,.T.);
#62899=ORIENTED_EDGE('',*,*,#43359,.T.);
#62900=ORIENTED_EDGE('',*,*,#43360,.F.);
#62901=ORIENTED_EDGE('',*,*,#43094,.T.);
#62902=ORIENTED_EDGE('',*,*,#43361,.F.);
#62903=ORIENTED_EDGE('',*,*,#43362,.F.);
#62904=ORIENTED_EDGE('',*,*,#43363,.F.);
#62905=ORIENTED_EDGE('',*,*,#43364,.F.);
#62906=ORIENTED_EDGE('',*,*,#43359,.F.);
#62907=ORIENTED_EDGE('',*,*,#43364,.T.);
#62908=ORIENTED_EDGE('',*,*,#43365,.F.);
#62909=ORIENTED_EDGE('',*,*,#43095,.T.);
#62910=ORIENTED_EDGE('',*,*,#43360,.T.);
#62911=ORIENTED_EDGE('',*,*,#43366,.T.);
#62912=ORIENTED_EDGE('',*,*,#43367,.F.);
#62913=ORIENTED_EDGE('',*,*,#43097,.T.);
#62914=ORIENTED_EDGE('',*,*,#43368,.F.);
#62915=ORIENTED_EDGE('',*,*,#43369,.F.);
#62916=ORIENTED_EDGE('',*,*,#43370,.F.);
#62917=ORIENTED_EDGE('',*,*,#43371,.F.);
#62918=ORIENTED_EDGE('',*,*,#43366,.F.);
#62919=ORIENTED_EDGE('',*,*,#43371,.T.);
#62920=ORIENTED_EDGE('',*,*,#43372,.F.);
#62921=ORIENTED_EDGE('',*,*,#43098,.T.);
#62922=ORIENTED_EDGE('',*,*,#43367,.T.);
#62923=ORIENTED_EDGE('',*,*,#43373,.T.);
#62924=ORIENTED_EDGE('',*,*,#43374,.F.);
#62925=ORIENTED_EDGE('',*,*,#43100,.T.);
#62926=ORIENTED_EDGE('',*,*,#43375,.F.);
#62927=ORIENTED_EDGE('',*,*,#43376,.F.);
#62928=ORIENTED_EDGE('',*,*,#43377,.F.);
#62929=ORIENTED_EDGE('',*,*,#43378,.F.);
#62930=ORIENTED_EDGE('',*,*,#43373,.F.);
#62931=ORIENTED_EDGE('',*,*,#43378,.T.);
#62932=ORIENTED_EDGE('',*,*,#43379,.F.);
#62933=ORIENTED_EDGE('',*,*,#43101,.T.);
#62934=ORIENTED_EDGE('',*,*,#43374,.T.);
#62935=ORIENTED_EDGE('',*,*,#43380,.T.);
#62936=ORIENTED_EDGE('',*,*,#43381,.F.);
#62937=ORIENTED_EDGE('',*,*,#43103,.T.);
#62938=ORIENTED_EDGE('',*,*,#43382,.F.);
#62939=ORIENTED_EDGE('',*,*,#43383,.F.);
#62940=ORIENTED_EDGE('',*,*,#43384,.F.);
#62941=ORIENTED_EDGE('',*,*,#43385,.F.);
#62942=ORIENTED_EDGE('',*,*,#43380,.F.);
#62943=ORIENTED_EDGE('',*,*,#43385,.T.);
#62944=ORIENTED_EDGE('',*,*,#43386,.F.);
#62945=ORIENTED_EDGE('',*,*,#43104,.T.);
#62946=ORIENTED_EDGE('',*,*,#43381,.T.);
#62947=ORIENTED_EDGE('',*,*,#43387,.T.);
#62948=ORIENTED_EDGE('',*,*,#43388,.F.);
#62949=ORIENTED_EDGE('',*,*,#43106,.T.);
#62950=ORIENTED_EDGE('',*,*,#43389,.F.);
#62951=ORIENTED_EDGE('',*,*,#43390,.F.);
#62952=ORIENTED_EDGE('',*,*,#43391,.F.);
#62953=ORIENTED_EDGE('',*,*,#43392,.F.);
#62954=ORIENTED_EDGE('',*,*,#43387,.F.);
#62955=ORIENTED_EDGE('',*,*,#43392,.T.);
#62956=ORIENTED_EDGE('',*,*,#43393,.F.);
#62957=ORIENTED_EDGE('',*,*,#43107,.T.);
#62958=ORIENTED_EDGE('',*,*,#43388,.T.);
#62959=ORIENTED_EDGE('',*,*,#43394,.F.);
#62960=ORIENTED_EDGE('',*,*,#43395,.F.);
#62961=ORIENTED_EDGE('',*,*,#34242,.T.);
#62962=ORIENTED_EDGE('',*,*,#43396,.F.);
#62963=ORIENTED_EDGE('',*,*,#43394,.T.);
#62964=ORIENTED_EDGE('',*,*,#34241,.T.);
#62965=ORIENTED_EDGE('',*,*,#43397,.F.);
#62966=ORIENTED_EDGE('',*,*,#43396,.T.);
#62967=ORIENTED_EDGE('',*,*,#34240,.T.);
#62968=ORIENTED_EDGE('',*,*,#43398,.F.);
#62969=ORIENTED_EDGE('',*,*,#43397,.T.);
#62970=ORIENTED_EDGE('',*,*,#34239,.T.);
#62971=ORIENTED_EDGE('',*,*,#43108,.T.);
#62972=ORIENTED_EDGE('',*,*,#43398,.T.);
#62973=ORIENTED_EDGE('',*,*,#34238,.T.);
#62974=ORIENTED_EDGE('',*,*,#43399,.F.);
#62975=ORIENTED_EDGE('',*,*,#43110,.T.);
#62976=ORIENTED_EDGE('',*,*,#43399,.T.);
#62977=ORIENTED_EDGE('',*,*,#34237,.T.);
#62978=ORIENTED_EDGE('',*,*,#43400,.F.);
#62979=ORIENTED_EDGE('',*,*,#43401,.F.);
#62980=ORIENTED_EDGE('',*,*,#43400,.T.);
#62981=ORIENTED_EDGE('',*,*,#34236,.T.);
#62982=ORIENTED_EDGE('',*,*,#43402,.F.);
#62983=ORIENTED_EDGE('',*,*,#43401,.T.);
#62984=ORIENTED_EDGE('',*,*,#34235,.T.);
#62985=ORIENTED_EDGE('',*,*,#43403,.F.);
#62986=ORIENTED_EDGE('',*,*,#43402,.T.);
#62987=ORIENTED_EDGE('',*,*,#34234,.T.);
#62988=ORIENTED_EDGE('',*,*,#43404,.F.);
#62989=ORIENTED_EDGE('',*,*,#43403,.T.);
#62990=ORIENTED_EDGE('',*,*,#34233,.T.);
#62991=ORIENTED_EDGE('',*,*,#43112,.T.);
#62992=ORIENTED_EDGE('',*,*,#43404,.T.);
#62993=ORIENTED_EDGE('',*,*,#34232,.T.);
#62994=ORIENTED_EDGE('',*,*,#43405,.F.);
#62995=ORIENTED_EDGE('',*,*,#43113,.T.);
#62996=ORIENTED_EDGE('',*,*,#43405,.T.);
#62997=ORIENTED_EDGE('',*,*,#34231,.T.);
#62998=ORIENTED_EDGE('',*,*,#43406,.F.);
#62999=ORIENTED_EDGE('',*,*,#43407,.F.);
#63000=ORIENTED_EDGE('',*,*,#43406,.T.);
#63001=ORIENTED_EDGE('',*,*,#34230,.T.);
#63002=ORIENTED_EDGE('',*,*,#43408,.F.);
#63003=ORIENTED_EDGE('',*,*,#43407,.T.);
#63004=ORIENTED_EDGE('',*,*,#34229,.T.);
#63005=ORIENTED_EDGE('',*,*,#43409,.F.);
#63006=ORIENTED_EDGE('',*,*,#43408,.T.);
#63007=ORIENTED_EDGE('',*,*,#34228,.T.);
#63008=ORIENTED_EDGE('',*,*,#43410,.F.);
#63009=ORIENTED_EDGE('',*,*,#43409,.T.);
#63010=ORIENTED_EDGE('',*,*,#34227,.T.);
#63011=ORIENTED_EDGE('',*,*,#43115,.T.);
#63012=ORIENTED_EDGE('',*,*,#43410,.T.);
#63013=ORIENTED_EDGE('',*,*,#34226,.T.);
#63014=ORIENTED_EDGE('',*,*,#43411,.F.);
#63015=ORIENTED_EDGE('',*,*,#43116,.T.);
#63016=ORIENTED_EDGE('',*,*,#43411,.T.);
#63017=ORIENTED_EDGE('',*,*,#34225,.T.);
#63018=ORIENTED_EDGE('',*,*,#43412,.F.);
#63019=ORIENTED_EDGE('',*,*,#43413,.F.);
#63020=ORIENTED_EDGE('',*,*,#43412,.T.);
#63021=ORIENTED_EDGE('',*,*,#34224,.T.);
#63022=ORIENTED_EDGE('',*,*,#43414,.F.);
#63023=ORIENTED_EDGE('',*,*,#43413,.T.);
#63024=ORIENTED_EDGE('',*,*,#34223,.T.);
#63025=ORIENTED_EDGE('',*,*,#43415,.F.);
#63026=ORIENTED_EDGE('',*,*,#43414,.T.);
#63027=ORIENTED_EDGE('',*,*,#34222,.T.);
#63028=ORIENTED_EDGE('',*,*,#43416,.F.);
#63029=ORIENTED_EDGE('',*,*,#43415,.T.);
#63030=ORIENTED_EDGE('',*,*,#34221,.T.);
#63031=ORIENTED_EDGE('',*,*,#43118,.T.);
#63032=ORIENTED_EDGE('',*,*,#43416,.T.);
#63033=ORIENTED_EDGE('',*,*,#34220,.T.);
#63034=ORIENTED_EDGE('',*,*,#43417,.F.);
#63035=ORIENTED_EDGE('',*,*,#43119,.T.);
#63036=ORIENTED_EDGE('',*,*,#43417,.T.);
#63037=ORIENTED_EDGE('',*,*,#34219,.T.);
#63038=ORIENTED_EDGE('',*,*,#43418,.F.);
#63039=ORIENTED_EDGE('',*,*,#43419,.F.);
#63040=ORIENTED_EDGE('',*,*,#43418,.T.);
#63041=ORIENTED_EDGE('',*,*,#34218,.T.);
#63042=ORIENTED_EDGE('',*,*,#43420,.F.);
#63043=ORIENTED_EDGE('',*,*,#43419,.T.);
#63044=ORIENTED_EDGE('',*,*,#34217,.T.);
#63045=ORIENTED_EDGE('',*,*,#43421,.F.);
#63046=ORIENTED_EDGE('',*,*,#43420,.T.);
#63047=ORIENTED_EDGE('',*,*,#34216,.T.);
#63048=ORIENTED_EDGE('',*,*,#43422,.F.);
#63049=ORIENTED_EDGE('',*,*,#43421,.T.);
#63050=ORIENTED_EDGE('',*,*,#34215,.T.);
#63051=ORIENTED_EDGE('',*,*,#43121,.T.);
#63052=ORIENTED_EDGE('',*,*,#43422,.T.);
#63053=ORIENTED_EDGE('',*,*,#34214,.T.);
#63054=ORIENTED_EDGE('',*,*,#43423,.F.);
#63055=ORIENTED_EDGE('',*,*,#43122,.T.);
#63056=ORIENTED_EDGE('',*,*,#43423,.T.);
#63057=ORIENTED_EDGE('',*,*,#34213,.T.);
#63058=ORIENTED_EDGE('',*,*,#43424,.F.);
#63059=ORIENTED_EDGE('',*,*,#43425,.F.);
#63060=ORIENTED_EDGE('',*,*,#43424,.T.);
#63061=ORIENTED_EDGE('',*,*,#34212,.T.);
#63062=ORIENTED_EDGE('',*,*,#43426,.F.);
#63063=ORIENTED_EDGE('',*,*,#43425,.T.);
#63064=ORIENTED_EDGE('',*,*,#34211,.T.);
#63065=ORIENTED_EDGE('',*,*,#43427,.F.);
#63066=ORIENTED_EDGE('',*,*,#43426,.T.);
#63067=ORIENTED_EDGE('',*,*,#34210,.T.);
#63068=ORIENTED_EDGE('',*,*,#43428,.F.);
#63069=ORIENTED_EDGE('',*,*,#43427,.T.);
#63070=ORIENTED_EDGE('',*,*,#34209,.T.);
#63071=ORIENTED_EDGE('',*,*,#43124,.T.);
#63072=ORIENTED_EDGE('',*,*,#43428,.T.);
#63073=ORIENTED_EDGE('',*,*,#34208,.T.);
#63074=ORIENTED_EDGE('',*,*,#43429,.F.);
#63075=ORIENTED_EDGE('',*,*,#43125,.T.);
#63076=ORIENTED_EDGE('',*,*,#43429,.T.);
#63077=ORIENTED_EDGE('',*,*,#34207,.T.);
#63078=ORIENTED_EDGE('',*,*,#43430,.F.);
#63079=ORIENTED_EDGE('',*,*,#43431,.F.);
#63080=ORIENTED_EDGE('',*,*,#43430,.T.);
#63081=ORIENTED_EDGE('',*,*,#34206,.T.);
#63082=ORIENTED_EDGE('',*,*,#43432,.F.);
#63083=ORIENTED_EDGE('',*,*,#43431,.T.);
#63084=ORIENTED_EDGE('',*,*,#34205,.T.);
#63085=ORIENTED_EDGE('',*,*,#43433,.F.);
#63086=ORIENTED_EDGE('',*,*,#43432,.T.);
#63087=ORIENTED_EDGE('',*,*,#34204,.T.);
#63088=ORIENTED_EDGE('',*,*,#43434,.F.);
#63089=ORIENTED_EDGE('',*,*,#43433,.T.);
#63090=ORIENTED_EDGE('',*,*,#34203,.T.);
#63091=ORIENTED_EDGE('',*,*,#43127,.T.);
#63092=ORIENTED_EDGE('',*,*,#43434,.T.);
#63093=ORIENTED_EDGE('',*,*,#34202,.T.);
#63094=ORIENTED_EDGE('',*,*,#43435,.F.);
#63095=ORIENTED_EDGE('',*,*,#43128,.T.);
#63096=ORIENTED_EDGE('',*,*,#43435,.T.);
#63097=ORIENTED_EDGE('',*,*,#34201,.T.);
#63098=ORIENTED_EDGE('',*,*,#43436,.F.);
#63099=ORIENTED_EDGE('',*,*,#43437,.F.);
#63100=ORIENTED_EDGE('',*,*,#43436,.T.);
#63101=ORIENTED_EDGE('',*,*,#34200,.T.);
#63102=ORIENTED_EDGE('',*,*,#43438,.F.);
#63103=ORIENTED_EDGE('',*,*,#43437,.T.);
#63104=ORIENTED_EDGE('',*,*,#34199,.T.);
#63105=ORIENTED_EDGE('',*,*,#43439,.F.);
#63106=ORIENTED_EDGE('',*,*,#43438,.T.);
#63107=ORIENTED_EDGE('',*,*,#34198,.T.);
#63108=ORIENTED_EDGE('',*,*,#43440,.F.);
#63109=ORIENTED_EDGE('',*,*,#43439,.T.);
#63110=ORIENTED_EDGE('',*,*,#34197,.T.);
#63111=ORIENTED_EDGE('',*,*,#43130,.T.);
#63112=ORIENTED_EDGE('',*,*,#43440,.T.);
#63113=ORIENTED_EDGE('',*,*,#34196,.T.);
#63114=ORIENTED_EDGE('',*,*,#43441,.F.);
#63115=ORIENTED_EDGE('',*,*,#43131,.T.);
#63116=ORIENTED_EDGE('',*,*,#43441,.T.);
#63117=ORIENTED_EDGE('',*,*,#34195,.T.);
#63118=ORIENTED_EDGE('',*,*,#43442,.F.);
#63119=ORIENTED_EDGE('',*,*,#43443,.F.);
#63120=ORIENTED_EDGE('',*,*,#43442,.T.);
#63121=ORIENTED_EDGE('',*,*,#34194,.T.);
#63122=ORIENTED_EDGE('',*,*,#43444,.F.);
#63123=ORIENTED_EDGE('',*,*,#43443,.T.);
#63124=ORIENTED_EDGE('',*,*,#34193,.T.);
#63125=ORIENTED_EDGE('',*,*,#43445,.F.);
#63126=ORIENTED_EDGE('',*,*,#43444,.T.);
#63127=ORIENTED_EDGE('',*,*,#34192,.T.);
#63128=ORIENTED_EDGE('',*,*,#43446,.F.);
#63129=ORIENTED_EDGE('',*,*,#43445,.T.);
#63130=ORIENTED_EDGE('',*,*,#34191,.T.);
#63131=ORIENTED_EDGE('',*,*,#43133,.T.);
#63132=ORIENTED_EDGE('',*,*,#43446,.T.);
#63133=ORIENTED_EDGE('',*,*,#34190,.T.);
#63134=ORIENTED_EDGE('',*,*,#43447,.F.);
#63135=ORIENTED_EDGE('',*,*,#43134,.T.);
#63136=ORIENTED_EDGE('',*,*,#43447,.T.);
#63137=ORIENTED_EDGE('',*,*,#34189,.T.);
#63138=ORIENTED_EDGE('',*,*,#43448,.F.);
#63139=ORIENTED_EDGE('',*,*,#43449,.F.);
#63140=ORIENTED_EDGE('',*,*,#43448,.T.);
#63141=ORIENTED_EDGE('',*,*,#34188,.T.);
#63142=ORIENTED_EDGE('',*,*,#43450,.F.);
#63143=ORIENTED_EDGE('',*,*,#43449,.T.);
#63144=ORIENTED_EDGE('',*,*,#34187,.T.);
#63145=ORIENTED_EDGE('',*,*,#43451,.F.);
#63146=ORIENTED_EDGE('',*,*,#43450,.T.);
#63147=ORIENTED_EDGE('',*,*,#34186,.T.);
#63148=ORIENTED_EDGE('',*,*,#43452,.F.);
#63149=ORIENTED_EDGE('',*,*,#43451,.T.);
#63150=ORIENTED_EDGE('',*,*,#34185,.T.);
#63151=ORIENTED_EDGE('',*,*,#43136,.T.);
#63152=ORIENTED_EDGE('',*,*,#43452,.T.);
#63153=ORIENTED_EDGE('',*,*,#34184,.T.);
#63154=ORIENTED_EDGE('',*,*,#43453,.F.);
#63155=ORIENTED_EDGE('',*,*,#43137,.T.);
#63156=ORIENTED_EDGE('',*,*,#43453,.T.);
#63157=ORIENTED_EDGE('',*,*,#34183,.T.);
#63158=ORIENTED_EDGE('',*,*,#43454,.F.);
#63159=ORIENTED_EDGE('',*,*,#43455,.F.);
#63160=ORIENTED_EDGE('',*,*,#43454,.T.);
#63161=ORIENTED_EDGE('',*,*,#34182,.T.);
#63162=ORIENTED_EDGE('',*,*,#43456,.F.);
#63163=ORIENTED_EDGE('',*,*,#43455,.T.);
#63164=ORIENTED_EDGE('',*,*,#34181,.T.);
#63165=ORIENTED_EDGE('',*,*,#43457,.F.);
#63166=ORIENTED_EDGE('',*,*,#43456,.T.);
#63167=ORIENTED_EDGE('',*,*,#34180,.T.);
#63168=ORIENTED_EDGE('',*,*,#43458,.F.);
#63169=ORIENTED_EDGE('',*,*,#43457,.T.);
#63170=ORIENTED_EDGE('',*,*,#34179,.T.);
#63171=ORIENTED_EDGE('',*,*,#43139,.T.);
#63172=ORIENTED_EDGE('',*,*,#43458,.T.);
#63173=ORIENTED_EDGE('',*,*,#34178,.T.);
#63174=ORIENTED_EDGE('',*,*,#43459,.F.);
#63175=ORIENTED_EDGE('',*,*,#43140,.T.);
#63176=ORIENTED_EDGE('',*,*,#43459,.T.);
#63177=ORIENTED_EDGE('',*,*,#34177,.T.);
#63178=ORIENTED_EDGE('',*,*,#43460,.F.);
#63179=ORIENTED_EDGE('',*,*,#43461,.F.);
#63180=ORIENTED_EDGE('',*,*,#43460,.T.);
#63181=ORIENTED_EDGE('',*,*,#34176,.T.);
#63182=ORIENTED_EDGE('',*,*,#43462,.F.);
#63183=ORIENTED_EDGE('',*,*,#43461,.T.);
#63184=ORIENTED_EDGE('',*,*,#34175,.T.);
#63185=ORIENTED_EDGE('',*,*,#43463,.F.);
#63186=ORIENTED_EDGE('',*,*,#43462,.T.);
#63187=ORIENTED_EDGE('',*,*,#34174,.T.);
#63188=ORIENTED_EDGE('',*,*,#43464,.F.);
#63189=ORIENTED_EDGE('',*,*,#43463,.T.);
#63190=ORIENTED_EDGE('',*,*,#34173,.T.);
#63191=ORIENTED_EDGE('',*,*,#43142,.T.);
#63192=ORIENTED_EDGE('',*,*,#43464,.T.);
#63193=ORIENTED_EDGE('',*,*,#34172,.T.);
#63194=ORIENTED_EDGE('',*,*,#43465,.F.);
#63195=ORIENTED_EDGE('',*,*,#43143,.T.);
#63196=ORIENTED_EDGE('',*,*,#43465,.T.);
#63197=ORIENTED_EDGE('',*,*,#34171,.T.);
#63198=ORIENTED_EDGE('',*,*,#43466,.F.);
#63199=ORIENTED_EDGE('',*,*,#43467,.F.);
#63200=ORIENTED_EDGE('',*,*,#43466,.T.);
#63201=ORIENTED_EDGE('',*,*,#34170,.T.);
#63202=ORIENTED_EDGE('',*,*,#43468,.F.);
#63203=ORIENTED_EDGE('',*,*,#43467,.T.);
#63204=ORIENTED_EDGE('',*,*,#34169,.T.);
#63205=ORIENTED_EDGE('',*,*,#43469,.F.);
#63206=ORIENTED_EDGE('',*,*,#43468,.T.);
#63207=ORIENTED_EDGE('',*,*,#34168,.T.);
#63208=ORIENTED_EDGE('',*,*,#43470,.F.);
#63209=ORIENTED_EDGE('',*,*,#43469,.T.);
#63210=ORIENTED_EDGE('',*,*,#34167,.T.);
#63211=ORIENTED_EDGE('',*,*,#43145,.T.);
#63212=ORIENTED_EDGE('',*,*,#43470,.T.);
#63213=ORIENTED_EDGE('',*,*,#34166,.T.);
#63214=ORIENTED_EDGE('',*,*,#43471,.F.);
#63215=ORIENTED_EDGE('',*,*,#43146,.T.);
#63216=ORIENTED_EDGE('',*,*,#43471,.T.);
#63217=ORIENTED_EDGE('',*,*,#34165,.T.);
#63218=ORIENTED_EDGE('',*,*,#43472,.F.);
#63219=ORIENTED_EDGE('',*,*,#43473,.F.);
#63220=ORIENTED_EDGE('',*,*,#43472,.T.);
#63221=ORIENTED_EDGE('',*,*,#34164,.T.);
#63222=ORIENTED_EDGE('',*,*,#43474,.F.);
#63223=ORIENTED_EDGE('',*,*,#43473,.T.);
#63224=ORIENTED_EDGE('',*,*,#34163,.T.);
#63225=ORIENTED_EDGE('',*,*,#43475,.F.);
#63226=ORIENTED_EDGE('',*,*,#43474,.T.);
#63227=ORIENTED_EDGE('',*,*,#34162,.T.);
#63228=ORIENTED_EDGE('',*,*,#43476,.F.);
#63229=ORIENTED_EDGE('',*,*,#43475,.T.);
#63230=ORIENTED_EDGE('',*,*,#34161,.T.);
#63231=ORIENTED_EDGE('',*,*,#43148,.T.);
#63232=ORIENTED_EDGE('',*,*,#43476,.T.);
#63233=ORIENTED_EDGE('',*,*,#34160,.T.);
#63234=ORIENTED_EDGE('',*,*,#43477,.F.);
#63235=ORIENTED_EDGE('',*,*,#43149,.T.);
#63236=ORIENTED_EDGE('',*,*,#43477,.T.);
#63237=ORIENTED_EDGE('',*,*,#34159,.T.);
#63238=ORIENTED_EDGE('',*,*,#43478,.F.);
#63239=ORIENTED_EDGE('',*,*,#43479,.F.);
#63240=ORIENTED_EDGE('',*,*,#43478,.T.);
#63241=ORIENTED_EDGE('',*,*,#34158,.T.);
#63242=ORIENTED_EDGE('',*,*,#43480,.F.);
#63243=ORIENTED_EDGE('',*,*,#43479,.T.);
#63244=ORIENTED_EDGE('',*,*,#34157,.T.);
#63245=ORIENTED_EDGE('',*,*,#43480,.T.);
#63246=ORIENTED_EDGE('',*,*,#34156,.T.);
#63247=ORIENTED_EDGE('',*,*,#43481,.F.);
#63248=ORIENTED_EDGE('',*,*,#43481,.T.);
#63249=ORIENTED_EDGE('',*,*,#34332,.T.);
#63250=ORIENTED_EDGE('',*,*,#43482,.F.);
#63251=ORIENTED_EDGE('',*,*,#43482,.T.);
#63252=ORIENTED_EDGE('',*,*,#34331,.T.);
#63253=ORIENTED_EDGE('',*,*,#43483,.F.);
#63254=ORIENTED_EDGE('',*,*,#43151,.T.);
#63255=ORIENTED_EDGE('',*,*,#43152,.T.);
#63256=ORIENTED_EDGE('',*,*,#43483,.T.);
#63257=ORIENTED_EDGE('',*,*,#34330,.T.);
#63258=ORIENTED_EDGE('',*,*,#43484,.F.);
#63259=ORIENTED_EDGE('',*,*,#43485,.F.);
#63260=ORIENTED_EDGE('',*,*,#43484,.T.);
#63261=ORIENTED_EDGE('',*,*,#34329,.T.);
#63262=ORIENTED_EDGE('',*,*,#43486,.F.);
#63263=ORIENTED_EDGE('',*,*,#43485,.T.);
#63264=ORIENTED_EDGE('',*,*,#34328,.T.);
#63265=ORIENTED_EDGE('',*,*,#43487,.F.);
#63266=ORIENTED_EDGE('',*,*,#43486,.T.);
#63267=ORIENTED_EDGE('',*,*,#34327,.T.);
#63268=ORIENTED_EDGE('',*,*,#43488,.F.);
#63269=ORIENTED_EDGE('',*,*,#43487,.T.);
#63270=ORIENTED_EDGE('',*,*,#34326,.T.);
#63271=ORIENTED_EDGE('',*,*,#43154,.T.);
#63272=ORIENTED_EDGE('',*,*,#43488,.T.);
#63273=ORIENTED_EDGE('',*,*,#34325,.T.);
#63274=ORIENTED_EDGE('',*,*,#43489,.F.);
#63275=ORIENTED_EDGE('',*,*,#43155,.T.);
#63276=ORIENTED_EDGE('',*,*,#43489,.T.);
#63277=ORIENTED_EDGE('',*,*,#34324,.T.);
#63278=ORIENTED_EDGE('',*,*,#43490,.F.);
#63279=ORIENTED_EDGE('',*,*,#43491,.F.);
#63280=ORIENTED_EDGE('',*,*,#43490,.T.);
#63281=ORIENTED_EDGE('',*,*,#34323,.T.);
#63282=ORIENTED_EDGE('',*,*,#43492,.F.);
#63283=ORIENTED_EDGE('',*,*,#43491,.T.);
#63284=ORIENTED_EDGE('',*,*,#34322,.T.);
#63285=ORIENTED_EDGE('',*,*,#43493,.F.);
#63286=ORIENTED_EDGE('',*,*,#43492,.T.);
#63287=ORIENTED_EDGE('',*,*,#34321,.T.);
#63288=ORIENTED_EDGE('',*,*,#43494,.F.);
#63289=ORIENTED_EDGE('',*,*,#43493,.T.);
#63290=ORIENTED_EDGE('',*,*,#34320,.T.);
#63291=ORIENTED_EDGE('',*,*,#43157,.T.);
#63292=ORIENTED_EDGE('',*,*,#43494,.T.);
#63293=ORIENTED_EDGE('',*,*,#34319,.T.);
#63294=ORIENTED_EDGE('',*,*,#43495,.F.);
#63295=ORIENTED_EDGE('',*,*,#43158,.T.);
#63296=ORIENTED_EDGE('',*,*,#43495,.T.);
#63297=ORIENTED_EDGE('',*,*,#34318,.T.);
#63298=ORIENTED_EDGE('',*,*,#43496,.F.);
#63299=ORIENTED_EDGE('',*,*,#43497,.F.);
#63300=ORIENTED_EDGE('',*,*,#43496,.T.);
#63301=ORIENTED_EDGE('',*,*,#34317,.T.);
#63302=ORIENTED_EDGE('',*,*,#43498,.F.);
#63303=ORIENTED_EDGE('',*,*,#43497,.T.);
#63304=ORIENTED_EDGE('',*,*,#34316,.T.);
#63305=ORIENTED_EDGE('',*,*,#43499,.F.);
#63306=ORIENTED_EDGE('',*,*,#43498,.T.);
#63307=ORIENTED_EDGE('',*,*,#34315,.T.);
#63308=ORIENTED_EDGE('',*,*,#43500,.F.);
#63309=ORIENTED_EDGE('',*,*,#43499,.T.);
#63310=ORIENTED_EDGE('',*,*,#34314,.T.);
#63311=ORIENTED_EDGE('',*,*,#43160,.T.);
#63312=ORIENTED_EDGE('',*,*,#43500,.T.);
#63313=ORIENTED_EDGE('',*,*,#34313,.T.);
#63314=ORIENTED_EDGE('',*,*,#43501,.F.);
#63315=ORIENTED_EDGE('',*,*,#43161,.T.);
#63316=ORIENTED_EDGE('',*,*,#43501,.T.);
#63317=ORIENTED_EDGE('',*,*,#34312,.T.);
#63318=ORIENTED_EDGE('',*,*,#43502,.F.);
#63319=ORIENTED_EDGE('',*,*,#43503,.F.);
#63320=ORIENTED_EDGE('',*,*,#43502,.T.);
#63321=ORIENTED_EDGE('',*,*,#34311,.T.);
#63322=ORIENTED_EDGE('',*,*,#43504,.F.);
#63323=ORIENTED_EDGE('',*,*,#43503,.T.);
#63324=ORIENTED_EDGE('',*,*,#34310,.T.);
#63325=ORIENTED_EDGE('',*,*,#43505,.F.);
#63326=ORIENTED_EDGE('',*,*,#43504,.T.);
#63327=ORIENTED_EDGE('',*,*,#34309,.T.);
#63328=ORIENTED_EDGE('',*,*,#43506,.F.);
#63329=ORIENTED_EDGE('',*,*,#43505,.T.);
#63330=ORIENTED_EDGE('',*,*,#34308,.T.);
#63331=ORIENTED_EDGE('',*,*,#43163,.T.);
#63332=ORIENTED_EDGE('',*,*,#43506,.T.);
#63333=ORIENTED_EDGE('',*,*,#34307,.T.);
#63334=ORIENTED_EDGE('',*,*,#43507,.F.);
#63335=ORIENTED_EDGE('',*,*,#43164,.T.);
#63336=ORIENTED_EDGE('',*,*,#43507,.T.);
#63337=ORIENTED_EDGE('',*,*,#34306,.T.);
#63338=ORIENTED_EDGE('',*,*,#43508,.F.);
#63339=ORIENTED_EDGE('',*,*,#43509,.F.);
#63340=ORIENTED_EDGE('',*,*,#43508,.T.);
#63341=ORIENTED_EDGE('',*,*,#34305,.T.);
#63342=ORIENTED_EDGE('',*,*,#43510,.F.);
#63343=ORIENTED_EDGE('',*,*,#43509,.T.);
#63344=ORIENTED_EDGE('',*,*,#34304,.T.);
#63345=ORIENTED_EDGE('',*,*,#43511,.F.);
#63346=ORIENTED_EDGE('',*,*,#43510,.T.);
#63347=ORIENTED_EDGE('',*,*,#34303,.T.);
#63348=ORIENTED_EDGE('',*,*,#43512,.F.);
#63349=ORIENTED_EDGE('',*,*,#43511,.T.);
#63350=ORIENTED_EDGE('',*,*,#34302,.T.);
#63351=ORIENTED_EDGE('',*,*,#43166,.T.);
#63352=ORIENTED_EDGE('',*,*,#43512,.T.);
#63353=ORIENTED_EDGE('',*,*,#34301,.T.);
#63354=ORIENTED_EDGE('',*,*,#43513,.F.);
#63355=ORIENTED_EDGE('',*,*,#43167,.T.);
#63356=ORIENTED_EDGE('',*,*,#43513,.T.);
#63357=ORIENTED_EDGE('',*,*,#34300,.T.);
#63358=ORIENTED_EDGE('',*,*,#43514,.F.);
#63359=ORIENTED_EDGE('',*,*,#43515,.F.);
#63360=ORIENTED_EDGE('',*,*,#43514,.T.);
#63361=ORIENTED_EDGE('',*,*,#34299,.T.);
#63362=ORIENTED_EDGE('',*,*,#43516,.F.);
#63363=ORIENTED_EDGE('',*,*,#43515,.T.);
#63364=ORIENTED_EDGE('',*,*,#34298,.T.);
#63365=ORIENTED_EDGE('',*,*,#43517,.F.);
#63366=ORIENTED_EDGE('',*,*,#43516,.T.);
#63367=ORIENTED_EDGE('',*,*,#34297,.T.);
#63368=ORIENTED_EDGE('',*,*,#43518,.F.);
#63369=ORIENTED_EDGE('',*,*,#43517,.T.);
#63370=ORIENTED_EDGE('',*,*,#34296,.T.);
#63371=ORIENTED_EDGE('',*,*,#43169,.T.);
#63372=ORIENTED_EDGE('',*,*,#43518,.T.);
#63373=ORIENTED_EDGE('',*,*,#34295,.T.);
#63374=ORIENTED_EDGE('',*,*,#43519,.F.);
#63375=ORIENTED_EDGE('',*,*,#43170,.T.);
#63376=ORIENTED_EDGE('',*,*,#43519,.T.);
#63377=ORIENTED_EDGE('',*,*,#34294,.T.);
#63378=ORIENTED_EDGE('',*,*,#43520,.F.);
#63379=ORIENTED_EDGE('',*,*,#43521,.F.);
#63380=ORIENTED_EDGE('',*,*,#43520,.T.);
#63381=ORIENTED_EDGE('',*,*,#34293,.T.);
#63382=ORIENTED_EDGE('',*,*,#43522,.F.);
#63383=ORIENTED_EDGE('',*,*,#43521,.T.);
#63384=ORIENTED_EDGE('',*,*,#34292,.T.);
#63385=ORIENTED_EDGE('',*,*,#43523,.F.);
#63386=ORIENTED_EDGE('',*,*,#43522,.T.);
#63387=ORIENTED_EDGE('',*,*,#34291,.T.);
#63388=ORIENTED_EDGE('',*,*,#43524,.F.);
#63389=ORIENTED_EDGE('',*,*,#43523,.T.);
#63390=ORIENTED_EDGE('',*,*,#34290,.T.);
#63391=ORIENTED_EDGE('',*,*,#43172,.T.);
#63392=ORIENTED_EDGE('',*,*,#43524,.T.);
#63393=ORIENTED_EDGE('',*,*,#34289,.T.);
#63394=ORIENTED_EDGE('',*,*,#43525,.F.);
#63395=ORIENTED_EDGE('',*,*,#43173,.T.);
#63396=ORIENTED_EDGE('',*,*,#43525,.T.);
#63397=ORIENTED_EDGE('',*,*,#34288,.T.);
#63398=ORIENTED_EDGE('',*,*,#43526,.F.);
#63399=ORIENTED_EDGE('',*,*,#43527,.F.);
#63400=ORIENTED_EDGE('',*,*,#43526,.T.);
#63401=ORIENTED_EDGE('',*,*,#34287,.T.);
#63402=ORIENTED_EDGE('',*,*,#43528,.F.);
#63403=ORIENTED_EDGE('',*,*,#43527,.T.);
#63404=ORIENTED_EDGE('',*,*,#34286,.T.);
#63405=ORIENTED_EDGE('',*,*,#43529,.F.);
#63406=ORIENTED_EDGE('',*,*,#43528,.T.);
#63407=ORIENTED_EDGE('',*,*,#34285,.T.);
#63408=ORIENTED_EDGE('',*,*,#43530,.F.);
#63409=ORIENTED_EDGE('',*,*,#43529,.T.);
#63410=ORIENTED_EDGE('',*,*,#34284,.T.);
#63411=ORIENTED_EDGE('',*,*,#43175,.T.);
#63412=ORIENTED_EDGE('',*,*,#43530,.T.);
#63413=ORIENTED_EDGE('',*,*,#34283,.T.);
#63414=ORIENTED_EDGE('',*,*,#43531,.F.);
#63415=ORIENTED_EDGE('',*,*,#43176,.T.);
#63416=ORIENTED_EDGE('',*,*,#43531,.T.);
#63417=ORIENTED_EDGE('',*,*,#34282,.T.);
#63418=ORIENTED_EDGE('',*,*,#43532,.F.);
#63419=ORIENTED_EDGE('',*,*,#43533,.F.);
#63420=ORIENTED_EDGE('',*,*,#43532,.T.);
#63421=ORIENTED_EDGE('',*,*,#34281,.T.);
#63422=ORIENTED_EDGE('',*,*,#43534,.F.);
#63423=ORIENTED_EDGE('',*,*,#43533,.T.);
#63424=ORIENTED_EDGE('',*,*,#34280,.T.);
#63425=ORIENTED_EDGE('',*,*,#43535,.F.);
#63426=ORIENTED_EDGE('',*,*,#43534,.T.);
#63427=ORIENTED_EDGE('',*,*,#34279,.T.);
#63428=ORIENTED_EDGE('',*,*,#43536,.F.);
#63429=ORIENTED_EDGE('',*,*,#43535,.T.);
#63430=ORIENTED_EDGE('',*,*,#34278,.T.);
#63431=ORIENTED_EDGE('',*,*,#43178,.T.);
#63432=ORIENTED_EDGE('',*,*,#43536,.T.);
#63433=ORIENTED_EDGE('',*,*,#34277,.T.);
#63434=ORIENTED_EDGE('',*,*,#43537,.F.);
#63435=ORIENTED_EDGE('',*,*,#43179,.T.);
#63436=ORIENTED_EDGE('',*,*,#43537,.T.);
#63437=ORIENTED_EDGE('',*,*,#34276,.T.);
#63438=ORIENTED_EDGE('',*,*,#43538,.F.);
#63439=ORIENTED_EDGE('',*,*,#43539,.F.);
#63440=ORIENTED_EDGE('',*,*,#43538,.T.);
#63441=ORIENTED_EDGE('',*,*,#34275,.T.);
#63442=ORIENTED_EDGE('',*,*,#43540,.F.);
#63443=ORIENTED_EDGE('',*,*,#43539,.T.);
#63444=ORIENTED_EDGE('',*,*,#34274,.T.);
#63445=ORIENTED_EDGE('',*,*,#43541,.F.);
#63446=ORIENTED_EDGE('',*,*,#43540,.T.);
#63447=ORIENTED_EDGE('',*,*,#34273,.T.);
#63448=ORIENTED_EDGE('',*,*,#43542,.F.);
#63449=ORIENTED_EDGE('',*,*,#43541,.T.);
#63450=ORIENTED_EDGE('',*,*,#34272,.T.);
#63451=ORIENTED_EDGE('',*,*,#43181,.T.);
#63452=ORIENTED_EDGE('',*,*,#43542,.T.);
#63453=ORIENTED_EDGE('',*,*,#34271,.T.);
#63454=ORIENTED_EDGE('',*,*,#43543,.F.);
#63455=ORIENTED_EDGE('',*,*,#43182,.T.);
#63456=ORIENTED_EDGE('',*,*,#43543,.T.);
#63457=ORIENTED_EDGE('',*,*,#34270,.T.);
#63458=ORIENTED_EDGE('',*,*,#43544,.F.);
#63459=ORIENTED_EDGE('',*,*,#43545,.F.);
#63460=ORIENTED_EDGE('',*,*,#43544,.T.);
#63461=ORIENTED_EDGE('',*,*,#34269,.T.);
#63462=ORIENTED_EDGE('',*,*,#43546,.F.);
#63463=ORIENTED_EDGE('',*,*,#43545,.T.);
#63464=ORIENTED_EDGE('',*,*,#34268,.T.);
#63465=ORIENTED_EDGE('',*,*,#43547,.F.);
#63466=ORIENTED_EDGE('',*,*,#43546,.T.);
#63467=ORIENTED_EDGE('',*,*,#34267,.T.);
#63468=ORIENTED_EDGE('',*,*,#43548,.F.);
#63469=ORIENTED_EDGE('',*,*,#43547,.T.);
#63470=ORIENTED_EDGE('',*,*,#34266,.T.);
#63471=ORIENTED_EDGE('',*,*,#43184,.T.);
#63472=ORIENTED_EDGE('',*,*,#43548,.T.);
#63473=ORIENTED_EDGE('',*,*,#34265,.T.);
#63474=ORIENTED_EDGE('',*,*,#43549,.F.);
#63475=ORIENTED_EDGE('',*,*,#43185,.T.);
#63476=ORIENTED_EDGE('',*,*,#43549,.T.);
#63477=ORIENTED_EDGE('',*,*,#34264,.T.);
#63478=ORIENTED_EDGE('',*,*,#43550,.F.);
#63479=ORIENTED_EDGE('',*,*,#43551,.F.);
#63480=ORIENTED_EDGE('',*,*,#43550,.T.);
#63481=ORIENTED_EDGE('',*,*,#34263,.T.);
#63482=ORIENTED_EDGE('',*,*,#43552,.F.);
#63483=ORIENTED_EDGE('',*,*,#43551,.T.);
#63484=ORIENTED_EDGE('',*,*,#34262,.T.);
#63485=ORIENTED_EDGE('',*,*,#43553,.F.);
#63486=ORIENTED_EDGE('',*,*,#43552,.T.);
#63487=ORIENTED_EDGE('',*,*,#34261,.T.);
#63488=ORIENTED_EDGE('',*,*,#43554,.F.);
#63489=ORIENTED_EDGE('',*,*,#43553,.T.);
#63490=ORIENTED_EDGE('',*,*,#34260,.T.);
#63491=ORIENTED_EDGE('',*,*,#43187,.T.);
#63492=ORIENTED_EDGE('',*,*,#43554,.T.);
#63493=ORIENTED_EDGE('',*,*,#34259,.T.);
#63494=ORIENTED_EDGE('',*,*,#43555,.F.);
#63495=ORIENTED_EDGE('',*,*,#43188,.T.);
#63496=ORIENTED_EDGE('',*,*,#43555,.T.);
#63497=ORIENTED_EDGE('',*,*,#34258,.T.);
#63498=ORIENTED_EDGE('',*,*,#43556,.F.);
#63499=ORIENTED_EDGE('',*,*,#43557,.F.);
#63500=ORIENTED_EDGE('',*,*,#43556,.T.);
#63501=ORIENTED_EDGE('',*,*,#34257,.T.);
#63502=ORIENTED_EDGE('',*,*,#43558,.F.);
#63503=ORIENTED_EDGE('',*,*,#43557,.T.);
#63504=ORIENTED_EDGE('',*,*,#34256,.T.);
#63505=ORIENTED_EDGE('',*,*,#43559,.F.);
#63506=ORIENTED_EDGE('',*,*,#43558,.T.);
#63507=ORIENTED_EDGE('',*,*,#34255,.T.);
#63508=ORIENTED_EDGE('',*,*,#43560,.F.);
#63509=ORIENTED_EDGE('',*,*,#43559,.T.);
#63510=ORIENTED_EDGE('',*,*,#34254,.T.);
#63511=ORIENTED_EDGE('',*,*,#43190,.T.);
#63512=ORIENTED_EDGE('',*,*,#43560,.T.);
#63513=ORIENTED_EDGE('',*,*,#34253,.T.);
#63514=ORIENTED_EDGE('',*,*,#43561,.F.);
#63515=ORIENTED_EDGE('',*,*,#43191,.T.);
#63516=ORIENTED_EDGE('',*,*,#43561,.T.);
#63517=ORIENTED_EDGE('',*,*,#34252,.T.);
#63518=ORIENTED_EDGE('',*,*,#43562,.F.);
#63519=ORIENTED_EDGE('',*,*,#43563,.F.);
#63520=ORIENTED_EDGE('',*,*,#43562,.T.);
#63521=ORIENTED_EDGE('',*,*,#34251,.T.);
#63522=ORIENTED_EDGE('',*,*,#43564,.F.);
#63523=ORIENTED_EDGE('',*,*,#43563,.T.);
#63524=ORIENTED_EDGE('',*,*,#34250,.T.);
#63525=ORIENTED_EDGE('',*,*,#43565,.F.);
#63526=ORIENTED_EDGE('',*,*,#43564,.T.);
#63527=ORIENTED_EDGE('',*,*,#34249,.T.);
#63528=ORIENTED_EDGE('',*,*,#43566,.F.);
#63529=ORIENTED_EDGE('',*,*,#43565,.T.);
#63530=ORIENTED_EDGE('',*,*,#34248,.T.);
#63531=ORIENTED_EDGE('',*,*,#43193,.T.);
#63532=ORIENTED_EDGE('',*,*,#43566,.T.);
#63533=ORIENTED_EDGE('',*,*,#34247,.T.);
#63534=ORIENTED_EDGE('',*,*,#43567,.F.);
#63535=ORIENTED_EDGE('',*,*,#43567,.T.);
#63536=ORIENTED_EDGE('',*,*,#34246,.T.);
#63537=ORIENTED_EDGE('',*,*,#34243,.T.);
#63538=ORIENTED_EDGE('',*,*,#43395,.T.);
#63539=ORIENTED_EDGE('',*,*,#43194,.T.);
#63540=ORIENTED_EDGE('',*,*,#43568,.F.);
#63541=ORIENTED_EDGE('',*,*,#43569,.F.);
#63542=ORIENTED_EDGE('',*,*,#43198,.T.);
#63543=ORIENTED_EDGE('',*,*,#43197,.T.);
#63544=ORIENTED_EDGE('',*,*,#43570,.F.);
#63545=ORIENTED_EDGE('',*,*,#43201,.T.);
#63546=ORIENTED_EDGE('',*,*,#43199,.T.);
#63547=ORIENTED_EDGE('',*,*,#43569,.T.);
#63548=ORIENTED_EDGE('',*,*,#43571,.F.);
#63549=ORIENTED_EDGE('',*,*,#43572,.F.);
#63550=ORIENTED_EDGE('',*,*,#43205,.T.);
#63551=ORIENTED_EDGE('',*,*,#43204,.T.);
#63552=ORIENTED_EDGE('',*,*,#43573,.F.);
#63553=ORIENTED_EDGE('',*,*,#43208,.T.);
#63554=ORIENTED_EDGE('',*,*,#43206,.T.);
#63555=ORIENTED_EDGE('',*,*,#43572,.T.);
#63556=ORIENTED_EDGE('',*,*,#43574,.F.);
#63557=ORIENTED_EDGE('',*,*,#43575,.F.);
#63558=ORIENTED_EDGE('',*,*,#43212,.T.);
#63559=ORIENTED_EDGE('',*,*,#43211,.T.);
#63560=ORIENTED_EDGE('',*,*,#43576,.F.);
#63561=ORIENTED_EDGE('',*,*,#43215,.T.);
#63562=ORIENTED_EDGE('',*,*,#43213,.T.);
#63563=ORIENTED_EDGE('',*,*,#43575,.T.);
#63564=ORIENTED_EDGE('',*,*,#43577,.F.);
#63565=ORIENTED_EDGE('',*,*,#43578,.F.);
#63566=ORIENTED_EDGE('',*,*,#43219,.T.);
#63567=ORIENTED_EDGE('',*,*,#43218,.T.);
#63568=ORIENTED_EDGE('',*,*,#43579,.F.);
#63569=ORIENTED_EDGE('',*,*,#43222,.T.);
#63570=ORIENTED_EDGE('',*,*,#43220,.T.);
#63571=ORIENTED_EDGE('',*,*,#43578,.T.);
#63572=ORIENTED_EDGE('',*,*,#43580,.F.);
#63573=ORIENTED_EDGE('',*,*,#43581,.F.);
#63574=ORIENTED_EDGE('',*,*,#43226,.T.);
#63575=ORIENTED_EDGE('',*,*,#43225,.T.);
#63576=ORIENTED_EDGE('',*,*,#43582,.F.);
#63577=ORIENTED_EDGE('',*,*,#43229,.T.);
#63578=ORIENTED_EDGE('',*,*,#43227,.T.);
#63579=ORIENTED_EDGE('',*,*,#43581,.T.);
#63580=ORIENTED_EDGE('',*,*,#43583,.F.);
#63581=ORIENTED_EDGE('',*,*,#43584,.F.);
#63582=ORIENTED_EDGE('',*,*,#43233,.T.);
#63583=ORIENTED_EDGE('',*,*,#43232,.T.);
#63584=ORIENTED_EDGE('',*,*,#43585,.F.);
#63585=ORIENTED_EDGE('',*,*,#43236,.T.);
#63586=ORIENTED_EDGE('',*,*,#43234,.T.);
#63587=ORIENTED_EDGE('',*,*,#43584,.T.);
#63588=ORIENTED_EDGE('',*,*,#43586,.F.);
#63589=ORIENTED_EDGE('',*,*,#43587,.F.);
#63590=ORIENTED_EDGE('',*,*,#43240,.T.);
#63591=ORIENTED_EDGE('',*,*,#43239,.T.);
#63592=ORIENTED_EDGE('',*,*,#43588,.F.);
#63593=ORIENTED_EDGE('',*,*,#43243,.T.);
#63594=ORIENTED_EDGE('',*,*,#43241,.T.);
#63595=ORIENTED_EDGE('',*,*,#43587,.T.);
#63596=ORIENTED_EDGE('',*,*,#43589,.F.);
#63597=ORIENTED_EDGE('',*,*,#43590,.F.);
#63598=ORIENTED_EDGE('',*,*,#43247,.T.);
#63599=ORIENTED_EDGE('',*,*,#43246,.T.);
#63600=ORIENTED_EDGE('',*,*,#43591,.F.);
#63601=ORIENTED_EDGE('',*,*,#43250,.T.);
#63602=ORIENTED_EDGE('',*,*,#43248,.T.);
#63603=ORIENTED_EDGE('',*,*,#43590,.T.);
#63604=ORIENTED_EDGE('',*,*,#43592,.F.);
#63605=ORIENTED_EDGE('',*,*,#43593,.F.);
#63606=ORIENTED_EDGE('',*,*,#43254,.T.);
#63607=ORIENTED_EDGE('',*,*,#43253,.T.);
#63608=ORIENTED_EDGE('',*,*,#43594,.F.);
#63609=ORIENTED_EDGE('',*,*,#43257,.T.);
#63610=ORIENTED_EDGE('',*,*,#43255,.T.);
#63611=ORIENTED_EDGE('',*,*,#43593,.T.);
#63612=ORIENTED_EDGE('',*,*,#43595,.F.);
#63613=ORIENTED_EDGE('',*,*,#43596,.F.);
#63614=ORIENTED_EDGE('',*,*,#43261,.T.);
#63615=ORIENTED_EDGE('',*,*,#43260,.T.);
#63616=ORIENTED_EDGE('',*,*,#43597,.F.);
#63617=ORIENTED_EDGE('',*,*,#43264,.T.);
#63618=ORIENTED_EDGE('',*,*,#43262,.T.);
#63619=ORIENTED_EDGE('',*,*,#43596,.T.);
#63620=ORIENTED_EDGE('',*,*,#43598,.F.);
#63621=ORIENTED_EDGE('',*,*,#43599,.F.);
#63622=ORIENTED_EDGE('',*,*,#43268,.T.);
#63623=ORIENTED_EDGE('',*,*,#43267,.T.);
#63624=ORIENTED_EDGE('',*,*,#43600,.F.);
#63625=ORIENTED_EDGE('',*,*,#43271,.T.);
#63626=ORIENTED_EDGE('',*,*,#43269,.T.);
#63627=ORIENTED_EDGE('',*,*,#43599,.T.);
#63628=ORIENTED_EDGE('',*,*,#43601,.F.);
#63629=ORIENTED_EDGE('',*,*,#43602,.F.);
#63630=ORIENTED_EDGE('',*,*,#43275,.T.);
#63631=ORIENTED_EDGE('',*,*,#43274,.T.);
#63632=ORIENTED_EDGE('',*,*,#43603,.F.);
#63633=ORIENTED_EDGE('',*,*,#43278,.T.);
#63634=ORIENTED_EDGE('',*,*,#43276,.T.);
#63635=ORIENTED_EDGE('',*,*,#43602,.T.);
#63636=ORIENTED_EDGE('',*,*,#43604,.F.);
#63637=ORIENTED_EDGE('',*,*,#43605,.F.);
#63638=ORIENTED_EDGE('',*,*,#43282,.T.);
#63639=ORIENTED_EDGE('',*,*,#43281,.T.);
#63640=ORIENTED_EDGE('',*,*,#43606,.F.);
#63641=ORIENTED_EDGE('',*,*,#43285,.T.);
#63642=ORIENTED_EDGE('',*,*,#43283,.T.);
#63643=ORIENTED_EDGE('',*,*,#43605,.T.);
#63644=ORIENTED_EDGE('',*,*,#43607,.F.);
#63645=ORIENTED_EDGE('',*,*,#43608,.F.);
#63646=ORIENTED_EDGE('',*,*,#43289,.T.);
#63647=ORIENTED_EDGE('',*,*,#43288,.T.);
#63648=ORIENTED_EDGE('',*,*,#43609,.F.);
#63649=ORIENTED_EDGE('',*,*,#43292,.T.);
#63650=ORIENTED_EDGE('',*,*,#43290,.T.);
#63651=ORIENTED_EDGE('',*,*,#43608,.T.);
#63652=ORIENTED_EDGE('',*,*,#43610,.F.);
#63653=ORIENTED_EDGE('',*,*,#43611,.F.);
#63654=ORIENTED_EDGE('',*,*,#34347,.T.);
#63655=ORIENTED_EDGE('',*,*,#43294,.T.);
#63656=ORIENTED_EDGE('',*,*,#43612,.F.);
#63657=ORIENTED_EDGE('',*,*,#43295,.T.);
#63658=ORIENTED_EDGE('',*,*,#34348,.T.);
#63659=ORIENTED_EDGE('',*,*,#43611,.T.);
#63660=ORIENTED_EDGE('',*,*,#43613,.F.);
#63661=ORIENTED_EDGE('',*,*,#43614,.F.);
#63662=ORIENTED_EDGE('',*,*,#43299,.T.);
#63663=ORIENTED_EDGE('',*,*,#43298,.T.);
#63664=ORIENTED_EDGE('',*,*,#43615,.F.);
#63665=ORIENTED_EDGE('',*,*,#43302,.T.);
#63666=ORIENTED_EDGE('',*,*,#43300,.T.);
#63667=ORIENTED_EDGE('',*,*,#43614,.T.);
#63668=ORIENTED_EDGE('',*,*,#43616,.F.);
#63669=ORIENTED_EDGE('',*,*,#43617,.F.);
#63670=ORIENTED_EDGE('',*,*,#43306,.T.);
#63671=ORIENTED_EDGE('',*,*,#43305,.T.);
#63672=ORIENTED_EDGE('',*,*,#43618,.F.);
#63673=ORIENTED_EDGE('',*,*,#43309,.T.);
#63674=ORIENTED_EDGE('',*,*,#43307,.T.);
#63675=ORIENTED_EDGE('',*,*,#43617,.T.);
#63676=ORIENTED_EDGE('',*,*,#43619,.F.);
#63677=ORIENTED_EDGE('',*,*,#43620,.F.);
#63678=ORIENTED_EDGE('',*,*,#43315,.T.);
#63679=ORIENTED_EDGE('',*,*,#43312,.T.);
#63680=ORIENTED_EDGE('',*,*,#43316,.T.);
#63681=ORIENTED_EDGE('',*,*,#43620,.T.);
#63682=ORIENTED_EDGE('',*,*,#43621,.F.);
#63683=ORIENTED_EDGE('',*,*,#43314,.T.);
#63684=ORIENTED_EDGE('',*,*,#43321,.T.);
#63685=ORIENTED_EDGE('',*,*,#43317,.T.);
#63686=ORIENTED_EDGE('',*,*,#43622,.F.);
#63687=ORIENTED_EDGE('',*,*,#43623,.F.);
#63688=ORIENTED_EDGE('',*,*,#43624,.F.);
#63689=ORIENTED_EDGE('',*,*,#43323,.T.);
#63690=ORIENTED_EDGE('',*,*,#43322,.T.);
#63691=ORIENTED_EDGE('',*,*,#43623,.T.);
#63692=ORIENTED_EDGE('',*,*,#43625,.F.);
#63693=ORIENTED_EDGE('',*,*,#43626,.F.);
#63694=ORIENTED_EDGE('',*,*,#43327,.T.);
#63695=ORIENTED_EDGE('',*,*,#43326,.T.);
#63696=ORIENTED_EDGE('',*,*,#43627,.F.);
#63697=ORIENTED_EDGE('',*,*,#43330,.T.);
#63698=ORIENTED_EDGE('',*,*,#43328,.T.);
#63699=ORIENTED_EDGE('',*,*,#43626,.T.);
#63700=ORIENTED_EDGE('',*,*,#43628,.F.);
#63701=ORIENTED_EDGE('',*,*,#43629,.F.);
#63702=ORIENTED_EDGE('',*,*,#43334,.T.);
#63703=ORIENTED_EDGE('',*,*,#43333,.T.);
#63704=ORIENTED_EDGE('',*,*,#43630,.F.);
#63705=ORIENTED_EDGE('',*,*,#43337,.T.);
#63706=ORIENTED_EDGE('',*,*,#43335,.T.);
#63707=ORIENTED_EDGE('',*,*,#43629,.T.);
#63708=ORIENTED_EDGE('',*,*,#43631,.F.);
#63709=ORIENTED_EDGE('',*,*,#43632,.F.);
#63710=ORIENTED_EDGE('',*,*,#43341,.T.);
#63711=ORIENTED_EDGE('',*,*,#43340,.T.);
#63712=ORIENTED_EDGE('',*,*,#43633,.F.);
#63713=ORIENTED_EDGE('',*,*,#43344,.T.);
#63714=ORIENTED_EDGE('',*,*,#43342,.T.);
#63715=ORIENTED_EDGE('',*,*,#43632,.T.);
#63716=ORIENTED_EDGE('',*,*,#43634,.F.);
#63717=ORIENTED_EDGE('',*,*,#43635,.F.);
#63718=ORIENTED_EDGE('',*,*,#43348,.T.);
#63719=ORIENTED_EDGE('',*,*,#43347,.T.);
#63720=ORIENTED_EDGE('',*,*,#43636,.F.);
#63721=ORIENTED_EDGE('',*,*,#43351,.T.);
#63722=ORIENTED_EDGE('',*,*,#43349,.T.);
#63723=ORIENTED_EDGE('',*,*,#43635,.T.);
#63724=ORIENTED_EDGE('',*,*,#43637,.F.);
#63725=ORIENTED_EDGE('',*,*,#43638,.F.);
#63726=ORIENTED_EDGE('',*,*,#43355,.T.);
#63727=ORIENTED_EDGE('',*,*,#43354,.T.);
#63728=ORIENTED_EDGE('',*,*,#43639,.F.);
#63729=ORIENTED_EDGE('',*,*,#43358,.T.);
#63730=ORIENTED_EDGE('',*,*,#43356,.T.);
#63731=ORIENTED_EDGE('',*,*,#43638,.T.);
#63732=ORIENTED_EDGE('',*,*,#43640,.F.);
#63733=ORIENTED_EDGE('',*,*,#43641,.F.);
#63734=ORIENTED_EDGE('',*,*,#43362,.T.);
#63735=ORIENTED_EDGE('',*,*,#43361,.T.);
#63736=ORIENTED_EDGE('',*,*,#43642,.F.);
#63737=ORIENTED_EDGE('',*,*,#43365,.T.);
#63738=ORIENTED_EDGE('',*,*,#43363,.T.);
#63739=ORIENTED_EDGE('',*,*,#43641,.T.);
#63740=ORIENTED_EDGE('',*,*,#43643,.F.);
#63741=ORIENTED_EDGE('',*,*,#43644,.F.);
#63742=ORIENTED_EDGE('',*,*,#43369,.T.);
#63743=ORIENTED_EDGE('',*,*,#43368,.T.);
#63744=ORIENTED_EDGE('',*,*,#43645,.F.);
#63745=ORIENTED_EDGE('',*,*,#43372,.T.);
#63746=ORIENTED_EDGE('',*,*,#43370,.T.);
#63747=ORIENTED_EDGE('',*,*,#43644,.T.);
#63748=ORIENTED_EDGE('',*,*,#43646,.F.);
#63749=ORIENTED_EDGE('',*,*,#43647,.F.);
#63750=ORIENTED_EDGE('',*,*,#43376,.T.);
#63751=ORIENTED_EDGE('',*,*,#43375,.T.);
#63752=ORIENTED_EDGE('',*,*,#43648,.F.);
#63753=ORIENTED_EDGE('',*,*,#43379,.T.);
#63754=ORIENTED_EDGE('',*,*,#43377,.T.);
#63755=ORIENTED_EDGE('',*,*,#43647,.T.);
#63756=ORIENTED_EDGE('',*,*,#43649,.F.);
#63757=ORIENTED_EDGE('',*,*,#43650,.F.);
#63758=ORIENTED_EDGE('',*,*,#43383,.T.);
#63759=ORIENTED_EDGE('',*,*,#43382,.T.);
#63760=ORIENTED_EDGE('',*,*,#43651,.F.);
#63761=ORIENTED_EDGE('',*,*,#43386,.T.);
#63762=ORIENTED_EDGE('',*,*,#43384,.T.);
#63763=ORIENTED_EDGE('',*,*,#43650,.T.);
#63764=ORIENTED_EDGE('',*,*,#43652,.F.);
#63765=ORIENTED_EDGE('',*,*,#43653,.F.);
#63766=ORIENTED_EDGE('',*,*,#43390,.T.);
#63767=ORIENTED_EDGE('',*,*,#43389,.T.);
#63768=ORIENTED_EDGE('',*,*,#43654,.F.);
#63769=ORIENTED_EDGE('',*,*,#43393,.T.);
#63770=ORIENTED_EDGE('',*,*,#43391,.T.);
#63771=ORIENTED_EDGE('',*,*,#43653,.T.);
#63772=ORIENTED_EDGE('',*,*,#43655,.T.);
#63773=ORIENTED_EDGE('',*,*,#43656,.F.);
#63774=ORIENTED_EDGE('',*,*,#43568,.T.);
#63775=ORIENTED_EDGE('',*,*,#43657,.F.);
#63776=ORIENTED_EDGE('',*,*,#43658,.T.);
#63777=ORIENTED_EDGE('',*,*,#43659,.F.);
#63778=ORIENTED_EDGE('',*,*,#43570,.T.);
#63779=ORIENTED_EDGE('',*,*,#43660,.F.);
#63780=ORIENTED_EDGE('',*,*,#43661,.F.);
#63781=ORIENTED_EDGE('',*,*,#43662,.T.);
#63782=ORIENTED_EDGE('',*,*,#43663,.F.);
#63783=ORIENTED_EDGE('',*,*,#43664,.T.);
#63784=ORIENTED_EDGE('',*,*,#43665,.F.);
#63785=ORIENTED_EDGE('',*,*,#43571,.T.);
#63786=ORIENTED_EDGE('',*,*,#43659,.T.);
#63787=ORIENTED_EDGE('',*,*,#43666,.F.);
#63788=ORIENTED_EDGE('',*,*,#43664,.F.);
#63789=ORIENTED_EDGE('',*,*,#43658,.F.);
#63790=ORIENTED_EDGE('',*,*,#43667,.F.);
#63791=ORIENTED_EDGE('',*,*,#43662,.F.);
#63792=ORIENTED_EDGE('',*,*,#43668,.T.);
#63793=ORIENTED_EDGE('',*,*,#43669,.F.);
#63794=ORIENTED_EDGE('',*,*,#43573,.T.);
#63795=ORIENTED_EDGE('',*,*,#43670,.F.);
#63796=ORIENTED_EDGE('',*,*,#43671,.F.);
#63797=ORIENTED_EDGE('',*,*,#43672,.T.);
#63798=ORIENTED_EDGE('',*,*,#43673,.F.);
#63799=ORIENTED_EDGE('',*,*,#43674,.T.);
#63800=ORIENTED_EDGE('',*,*,#43675,.F.);
#63801=ORIENTED_EDGE('',*,*,#43574,.T.);
#63802=ORIENTED_EDGE('',*,*,#43669,.T.);
#63803=ORIENTED_EDGE('',*,*,#43676,.F.);
#63804=ORIENTED_EDGE('',*,*,#43674,.F.);
#63805=ORIENTED_EDGE('',*,*,#43668,.F.);
#63806=ORIENTED_EDGE('',*,*,#43677,.F.);
#63807=ORIENTED_EDGE('',*,*,#43672,.F.);
#63808=ORIENTED_EDGE('',*,*,#43678,.T.);
#63809=ORIENTED_EDGE('',*,*,#43679,.F.);
#63810=ORIENTED_EDGE('',*,*,#43576,.T.);
#63811=ORIENTED_EDGE('',*,*,#43680,.F.);
#63812=ORIENTED_EDGE('',*,*,#43681,.F.);
#63813=ORIENTED_EDGE('',*,*,#43682,.T.);
#63814=ORIENTED_EDGE('',*,*,#43683,.F.);
#63815=ORIENTED_EDGE('',*,*,#43684,.T.);
#63816=ORIENTED_EDGE('',*,*,#43685,.F.);
#63817=ORIENTED_EDGE('',*,*,#43577,.T.);
#63818=ORIENTED_EDGE('',*,*,#43679,.T.);
#63819=ORIENTED_EDGE('',*,*,#43686,.F.);
#63820=ORIENTED_EDGE('',*,*,#43684,.F.);
#63821=ORIENTED_EDGE('',*,*,#43678,.F.);
#63822=ORIENTED_EDGE('',*,*,#43687,.F.);
#63823=ORIENTED_EDGE('',*,*,#43682,.F.);
#63824=ORIENTED_EDGE('',*,*,#43688,.T.);
#63825=ORIENTED_EDGE('',*,*,#43689,.F.);
#63826=ORIENTED_EDGE('',*,*,#43579,.T.);
#63827=ORIENTED_EDGE('',*,*,#43690,.F.);
#63828=ORIENTED_EDGE('',*,*,#43691,.F.);
#63829=ORIENTED_EDGE('',*,*,#43692,.T.);
#63830=ORIENTED_EDGE('',*,*,#43693,.F.);
#63831=ORIENTED_EDGE('',*,*,#43694,.T.);
#63832=ORIENTED_EDGE('',*,*,#43695,.F.);
#63833=ORIENTED_EDGE('',*,*,#43580,.T.);
#63834=ORIENTED_EDGE('',*,*,#43689,.T.);
#63835=ORIENTED_EDGE('',*,*,#43696,.F.);
#63836=ORIENTED_EDGE('',*,*,#43694,.F.);
#63837=ORIENTED_EDGE('',*,*,#43688,.F.);
#63838=ORIENTED_EDGE('',*,*,#43697,.F.);
#63839=ORIENTED_EDGE('',*,*,#43692,.F.);
#63840=ORIENTED_EDGE('',*,*,#43698,.T.);
#63841=ORIENTED_EDGE('',*,*,#43699,.F.);
#63842=ORIENTED_EDGE('',*,*,#43582,.T.);
#63843=ORIENTED_EDGE('',*,*,#43700,.F.);
#63844=ORIENTED_EDGE('',*,*,#43701,.F.);
#63845=ORIENTED_EDGE('',*,*,#43702,.T.);
#63846=ORIENTED_EDGE('',*,*,#43703,.F.);
#63847=ORIENTED_EDGE('',*,*,#43704,.T.);
#63848=ORIENTED_EDGE('',*,*,#43705,.F.);
#63849=ORIENTED_EDGE('',*,*,#43583,.T.);
#63850=ORIENTED_EDGE('',*,*,#43699,.T.);
#63851=ORIENTED_EDGE('',*,*,#43706,.F.);
#63852=ORIENTED_EDGE('',*,*,#43704,.F.);
#63853=ORIENTED_EDGE('',*,*,#43698,.F.);
#63854=ORIENTED_EDGE('',*,*,#43707,.F.);
#63855=ORIENTED_EDGE('',*,*,#43702,.F.);
#63856=ORIENTED_EDGE('',*,*,#43708,.T.);
#63857=ORIENTED_EDGE('',*,*,#43709,.F.);
#63858=ORIENTED_EDGE('',*,*,#43585,.T.);
#63859=ORIENTED_EDGE('',*,*,#43710,.F.);
#63860=ORIENTED_EDGE('',*,*,#43711,.F.);
#63861=ORIENTED_EDGE('',*,*,#43712,.T.);
#63862=ORIENTED_EDGE('',*,*,#43713,.F.);
#63863=ORIENTED_EDGE('',*,*,#43714,.T.);
#63864=ORIENTED_EDGE('',*,*,#43715,.F.);
#63865=ORIENTED_EDGE('',*,*,#43586,.T.);
#63866=ORIENTED_EDGE('',*,*,#43709,.T.);
#63867=ORIENTED_EDGE('',*,*,#43716,.F.);
#63868=ORIENTED_EDGE('',*,*,#43714,.F.);
#63869=ORIENTED_EDGE('',*,*,#43708,.F.);
#63870=ORIENTED_EDGE('',*,*,#43717,.F.);
#63871=ORIENTED_EDGE('',*,*,#43712,.F.);
#63872=ORIENTED_EDGE('',*,*,#34342,.T.);
#63873=ORIENTED_EDGE('',*,*,#43718,.F.);
#63874=ORIENTED_EDGE('',*,*,#43588,.T.);
#63875=ORIENTED_EDGE('',*,*,#43719,.F.);
#63876=ORIENTED_EDGE('',*,*,#43720,.F.);
#63877=ORIENTED_EDGE('',*,*,#34344,.T.);
#63878=ORIENTED_EDGE('',*,*,#43721,.F.);
#63879=ORIENTED_EDGE('',*,*,#34341,.T.);
#63880=ORIENTED_EDGE('',*,*,#43722,.F.);
#63881=ORIENTED_EDGE('',*,*,#43589,.T.);
#63882=ORIENTED_EDGE('',*,*,#43718,.T.);
#63883=ORIENTED_EDGE('',*,*,#43723,.T.);
#63884=ORIENTED_EDGE('',*,*,#43724,.F.);
#63885=ORIENTED_EDGE('',*,*,#43591,.T.);
#63886=ORIENTED_EDGE('',*,*,#43725,.F.);
#63887=ORIENTED_EDGE('',*,*,#43726,.F.);
#63888=ORIENTED_EDGE('',*,*,#43727,.T.);
#63889=ORIENTED_EDGE('',*,*,#43728,.F.);
#63890=ORIENTED_EDGE('',*,*,#43729,.T.);
#63891=ORIENTED_EDGE('',*,*,#43730,.F.);
#63892=ORIENTED_EDGE('',*,*,#43592,.T.);
#63893=ORIENTED_EDGE('',*,*,#43724,.T.);
#63894=ORIENTED_EDGE('',*,*,#43731,.F.);
#63895=ORIENTED_EDGE('',*,*,#43729,.F.);
#63896=ORIENTED_EDGE('',*,*,#43723,.F.);
#63897=ORIENTED_EDGE('',*,*,#43732,.F.);
#63898=ORIENTED_EDGE('',*,*,#43727,.F.);
#63899=ORIENTED_EDGE('',*,*,#43733,.T.);
#63900=ORIENTED_EDGE('',*,*,#43734,.F.);
#63901=ORIENTED_EDGE('',*,*,#43594,.T.);
#63902=ORIENTED_EDGE('',*,*,#43735,.F.);
#63903=ORIENTED_EDGE('',*,*,#43736,.F.);
#63904=ORIENTED_EDGE('',*,*,#43737,.T.);
#63905=ORIENTED_EDGE('',*,*,#43738,.F.);
#63906=ORIENTED_EDGE('',*,*,#43739,.T.);
#63907=ORIENTED_EDGE('',*,*,#43740,.F.);
#63908=ORIENTED_EDGE('',*,*,#43595,.T.);
#63909=ORIENTED_EDGE('',*,*,#43734,.T.);
#63910=ORIENTED_EDGE('',*,*,#43741,.F.);
#63911=ORIENTED_EDGE('',*,*,#43739,.F.);
#63912=ORIENTED_EDGE('',*,*,#43733,.F.);
#63913=ORIENTED_EDGE('',*,*,#43742,.F.);
#63914=ORIENTED_EDGE('',*,*,#43737,.F.);
#63915=ORIENTED_EDGE('',*,*,#43743,.T.);
#63916=ORIENTED_EDGE('',*,*,#43744,.F.);
#63917=ORIENTED_EDGE('',*,*,#43597,.T.);
#63918=ORIENTED_EDGE('',*,*,#43745,.F.);
#63919=ORIENTED_EDGE('',*,*,#43746,.F.);
#63920=ORIENTED_EDGE('',*,*,#43747,.T.);
#63921=ORIENTED_EDGE('',*,*,#43748,.F.);
#63922=ORIENTED_EDGE('',*,*,#43749,.T.);
#63923=ORIENTED_EDGE('',*,*,#43750,.F.);
#63924=ORIENTED_EDGE('',*,*,#43598,.T.);
#63925=ORIENTED_EDGE('',*,*,#43744,.T.);
#63926=ORIENTED_EDGE('',*,*,#43751,.F.);
#63927=ORIENTED_EDGE('',*,*,#43749,.F.);
#63928=ORIENTED_EDGE('',*,*,#43743,.F.);
#63929=ORIENTED_EDGE('',*,*,#43752,.F.);
#63930=ORIENTED_EDGE('',*,*,#43747,.F.);
#63931=ORIENTED_EDGE('',*,*,#43753,.T.);
#63932=ORIENTED_EDGE('',*,*,#43754,.F.);
#63933=ORIENTED_EDGE('',*,*,#43600,.T.);
#63934=ORIENTED_EDGE('',*,*,#43755,.F.);
#63935=ORIENTED_EDGE('',*,*,#43756,.F.);
#63936=ORIENTED_EDGE('',*,*,#43757,.T.);
#63937=ORIENTED_EDGE('',*,*,#43758,.F.);
#63938=ORIENTED_EDGE('',*,*,#43759,.T.);
#63939=ORIENTED_EDGE('',*,*,#43760,.F.);
#63940=ORIENTED_EDGE('',*,*,#43601,.T.);
#63941=ORIENTED_EDGE('',*,*,#43754,.T.);
#63942=ORIENTED_EDGE('',*,*,#43761,.F.);
#63943=ORIENTED_EDGE('',*,*,#43759,.F.);
#63944=ORIENTED_EDGE('',*,*,#43753,.F.);
#63945=ORIENTED_EDGE('',*,*,#43762,.F.);
#63946=ORIENTED_EDGE('',*,*,#43757,.F.);
#63947=ORIENTED_EDGE('',*,*,#43763,.T.);
#63948=ORIENTED_EDGE('',*,*,#43764,.F.);
#63949=ORIENTED_EDGE('',*,*,#43603,.T.);
#63950=ORIENTED_EDGE('',*,*,#43765,.F.);
#63951=ORIENTED_EDGE('',*,*,#43766,.F.);
#63952=ORIENTED_EDGE('',*,*,#43767,.T.);
#63953=ORIENTED_EDGE('',*,*,#43768,.F.);
#63954=ORIENTED_EDGE('',*,*,#43769,.T.);
#63955=ORIENTED_EDGE('',*,*,#43770,.F.);
#63956=ORIENTED_EDGE('',*,*,#43604,.T.);
#63957=ORIENTED_EDGE('',*,*,#43764,.T.);
#63958=ORIENTED_EDGE('',*,*,#43771,.F.);
#63959=ORIENTED_EDGE('',*,*,#43769,.F.);
#63960=ORIENTED_EDGE('',*,*,#43763,.F.);
#63961=ORIENTED_EDGE('',*,*,#43772,.F.);
#63962=ORIENTED_EDGE('',*,*,#43767,.F.);
#63963=ORIENTED_EDGE('',*,*,#43773,.T.);
#63964=ORIENTED_EDGE('',*,*,#43774,.F.);
#63965=ORIENTED_EDGE('',*,*,#43606,.T.);
#63966=ORIENTED_EDGE('',*,*,#43775,.F.);
#63967=ORIENTED_EDGE('',*,*,#43776,.F.);
#63968=ORIENTED_EDGE('',*,*,#43777,.T.);
#63969=ORIENTED_EDGE('',*,*,#43778,.F.);
#63970=ORIENTED_EDGE('',*,*,#43779,.T.);
#63971=ORIENTED_EDGE('',*,*,#43780,.F.);
#63972=ORIENTED_EDGE('',*,*,#43607,.T.);
#63973=ORIENTED_EDGE('',*,*,#43774,.T.);
#63974=ORIENTED_EDGE('',*,*,#43781,.F.);
#63975=ORIENTED_EDGE('',*,*,#43779,.F.);
#63976=ORIENTED_EDGE('',*,*,#43773,.F.);
#63977=ORIENTED_EDGE('',*,*,#43782,.F.);
#63978=ORIENTED_EDGE('',*,*,#43777,.F.);
#63979=ORIENTED_EDGE('',*,*,#43783,.T.);
#63980=ORIENTED_EDGE('',*,*,#43784,.F.);
#63981=ORIENTED_EDGE('',*,*,#43609,.T.);
#63982=ORIENTED_EDGE('',*,*,#43785,.F.);
#63983=ORIENTED_EDGE('',*,*,#43786,.F.);
#63984=ORIENTED_EDGE('',*,*,#43787,.T.);
#63985=ORIENTED_EDGE('',*,*,#43788,.F.);
#63986=ORIENTED_EDGE('',*,*,#43789,.T.);
#63987=ORIENTED_EDGE('',*,*,#43790,.F.);
#63988=ORIENTED_EDGE('',*,*,#43610,.T.);
#63989=ORIENTED_EDGE('',*,*,#43784,.T.);
#63990=ORIENTED_EDGE('',*,*,#43791,.F.);
#63991=ORIENTED_EDGE('',*,*,#43789,.F.);
#63992=ORIENTED_EDGE('',*,*,#43783,.F.);
#63993=ORIENTED_EDGE('',*,*,#43792,.F.);
#63994=ORIENTED_EDGE('',*,*,#43787,.F.);
#63995=ORIENTED_EDGE('',*,*,#43793,.T.);
#63996=ORIENTED_EDGE('',*,*,#43794,.F.);
#63997=ORIENTED_EDGE('',*,*,#43612,.T.);
#63998=ORIENTED_EDGE('',*,*,#43795,.F.);
#63999=ORIENTED_EDGE('',*,*,#43796,.F.);
#64000=ORIENTED_EDGE('',*,*,#43797,.T.);
#64001=ORIENTED_EDGE('',*,*,#43798,.F.);
#64002=ORIENTED_EDGE('',*,*,#43799,.T.);
#64003=ORIENTED_EDGE('',*,*,#43800,.F.);
#64004=ORIENTED_EDGE('',*,*,#43613,.T.);
#64005=ORIENTED_EDGE('',*,*,#43794,.T.);
#64006=ORIENTED_EDGE('',*,*,#43801,.F.);
#64007=ORIENTED_EDGE('',*,*,#43799,.F.);
#64008=ORIENTED_EDGE('',*,*,#43793,.F.);
#64009=ORIENTED_EDGE('',*,*,#43802,.F.);
#64010=ORIENTED_EDGE('',*,*,#43797,.F.);
#64011=ORIENTED_EDGE('',*,*,#43803,.T.);
#64012=ORIENTED_EDGE('',*,*,#43804,.F.);
#64013=ORIENTED_EDGE('',*,*,#43615,.T.);
#64014=ORIENTED_EDGE('',*,*,#43805,.F.);
#64015=ORIENTED_EDGE('',*,*,#43806,.F.);
#64016=ORIENTED_EDGE('',*,*,#43807,.T.);
#64017=ORIENTED_EDGE('',*,*,#43808,.F.);
#64018=ORIENTED_EDGE('',*,*,#43809,.T.);
#64019=ORIENTED_EDGE('',*,*,#43810,.F.);
#64020=ORIENTED_EDGE('',*,*,#43616,.T.);
#64021=ORIENTED_EDGE('',*,*,#43804,.T.);
#64022=ORIENTED_EDGE('',*,*,#43811,.F.);
#64023=ORIENTED_EDGE('',*,*,#43809,.F.);
#64024=ORIENTED_EDGE('',*,*,#43803,.F.);
#64025=ORIENTED_EDGE('',*,*,#43812,.F.);
#64026=ORIENTED_EDGE('',*,*,#43807,.F.);
#64027=ORIENTED_EDGE('',*,*,#43813,.T.);
#64028=ORIENTED_EDGE('',*,*,#43814,.F.);
#64029=ORIENTED_EDGE('',*,*,#43618,.T.);
#64030=ORIENTED_EDGE('',*,*,#43815,.F.);
#64031=ORIENTED_EDGE('',*,*,#43816,.F.);
#64032=ORIENTED_EDGE('',*,*,#43817,.T.);
#64033=ORIENTED_EDGE('',*,*,#43818,.F.);
#64034=ORIENTED_EDGE('',*,*,#43819,.T.);
#64035=ORIENTED_EDGE('',*,*,#43820,.F.);
#64036=ORIENTED_EDGE('',*,*,#43619,.T.);
#64037=ORIENTED_EDGE('',*,*,#43814,.T.);
#64038=ORIENTED_EDGE('',*,*,#43821,.F.);
#64039=ORIENTED_EDGE('',*,*,#43819,.F.);
#64040=ORIENTED_EDGE('',*,*,#43813,.F.);
#64041=ORIENTED_EDGE('',*,*,#43822,.F.);
#64042=ORIENTED_EDGE('',*,*,#43817,.F.);
#64043=ORIENTED_EDGE('',*,*,#43621,.T.);
#64044=ORIENTED_EDGE('',*,*,#43823,.F.);
#64045=ORIENTED_EDGE('',*,*,#43824,.T.);
#64046=ORIENTED_EDGE('',*,*,#43825,.F.);
#64047=ORIENTED_EDGE('',*,*,#43826,.F.);
#64048=ORIENTED_EDGE('',*,*,#43827,.T.);
#64049=ORIENTED_EDGE('',*,*,#43828,.F.);
#64050=ORIENTED_EDGE('',*,*,#43622,.T.);
#64051=ORIENTED_EDGE('',*,*,#43825,.T.);
#64052=ORIENTED_EDGE('',*,*,#43829,.T.);
#64053=ORIENTED_EDGE('',*,*,#43830,.F.);
#64054=ORIENTED_EDGE('',*,*,#43831,.F.);
#64055=ORIENTED_EDGE('',*,*,#43829,.F.);
#64056=ORIENTED_EDGE('',*,*,#43824,.F.);
#64057=ORIENTED_EDGE('',*,*,#43832,.F.);
#64058=ORIENTED_EDGE('',*,*,#43827,.F.);
#64059=ORIENTED_EDGE('',*,*,#43833,.T.);
#64060=ORIENTED_EDGE('',*,*,#43834,.F.);
#64061=ORIENTED_EDGE('',*,*,#43624,.T.);
#64062=ORIENTED_EDGE('',*,*,#43835,.F.);
#64063=ORIENTED_EDGE('',*,*,#43836,.F.);
#64064=ORIENTED_EDGE('',*,*,#43837,.T.);
#64065=ORIENTED_EDGE('',*,*,#43838,.F.);
#64066=ORIENTED_EDGE('',*,*,#43839,.T.);
#64067=ORIENTED_EDGE('',*,*,#43840,.F.);
#64068=ORIENTED_EDGE('',*,*,#43625,.T.);
#64069=ORIENTED_EDGE('',*,*,#43834,.T.);
#64070=ORIENTED_EDGE('',*,*,#43841,.F.);
#64071=ORIENTED_EDGE('',*,*,#43839,.F.);
#64072=ORIENTED_EDGE('',*,*,#43833,.F.);
#64073=ORIENTED_EDGE('',*,*,#43842,.F.);
#64074=ORIENTED_EDGE('',*,*,#43837,.F.);
#64075=ORIENTED_EDGE('',*,*,#43843,.T.);
#64076=ORIENTED_EDGE('',*,*,#43844,.F.);
#64077=ORIENTED_EDGE('',*,*,#43627,.T.);
#64078=ORIENTED_EDGE('',*,*,#43845,.F.);
#64079=ORIENTED_EDGE('',*,*,#43846,.F.);
#64080=ORIENTED_EDGE('',*,*,#43847,.T.);
#64081=ORIENTED_EDGE('',*,*,#43848,.F.);
#64082=ORIENTED_EDGE('',*,*,#43849,.T.);
#64083=ORIENTED_EDGE('',*,*,#43850,.F.);
#64084=ORIENTED_EDGE('',*,*,#43628,.T.);
#64085=ORIENTED_EDGE('',*,*,#43844,.T.);
#64086=ORIENTED_EDGE('',*,*,#43851,.F.);
#64087=ORIENTED_EDGE('',*,*,#43849,.F.);
#64088=ORIENTED_EDGE('',*,*,#43843,.F.);
#64089=ORIENTED_EDGE('',*,*,#43852,.F.);
#64090=ORIENTED_EDGE('',*,*,#43847,.F.);
#64091=ORIENTED_EDGE('',*,*,#43853,.T.);
#64092=ORIENTED_EDGE('',*,*,#43854,.F.);
#64093=ORIENTED_EDGE('',*,*,#43630,.T.);
#64094=ORIENTED_EDGE('',*,*,#43855,.F.);
#64095=ORIENTED_EDGE('',*,*,#43856,.F.);
#64096=ORIENTED_EDGE('',*,*,#43857,.T.);
#64097=ORIENTED_EDGE('',*,*,#43858,.F.);
#64098=ORIENTED_EDGE('',*,*,#43859,.T.);
#64099=ORIENTED_EDGE('',*,*,#43860,.F.);
#64100=ORIENTED_EDGE('',*,*,#43631,.T.);
#64101=ORIENTED_EDGE('',*,*,#43854,.T.);
#64102=ORIENTED_EDGE('',*,*,#43861,.F.);
#64103=ORIENTED_EDGE('',*,*,#43859,.F.);
#64104=ORIENTED_EDGE('',*,*,#43853,.F.);
#64105=ORIENTED_EDGE('',*,*,#43862,.F.);
#64106=ORIENTED_EDGE('',*,*,#43857,.F.);
#64107=ORIENTED_EDGE('',*,*,#43863,.T.);
#64108=ORIENTED_EDGE('',*,*,#43864,.F.);
#64109=ORIENTED_EDGE('',*,*,#43633,.T.);
#64110=ORIENTED_EDGE('',*,*,#43865,.F.);
#64111=ORIENTED_EDGE('',*,*,#43866,.F.);
#64112=ORIENTED_EDGE('',*,*,#43867,.T.);
#64113=ORIENTED_EDGE('',*,*,#43868,.F.);
#64114=ORIENTED_EDGE('',*,*,#43869,.T.);
#64115=ORIENTED_EDGE('',*,*,#43870,.F.);
#64116=ORIENTED_EDGE('',*,*,#43634,.T.);
#64117=ORIENTED_EDGE('',*,*,#43864,.T.);
#64118=ORIENTED_EDGE('',*,*,#43871,.F.);
#64119=ORIENTED_EDGE('',*,*,#43869,.F.);
#64120=ORIENTED_EDGE('',*,*,#43863,.F.);
#64121=ORIENTED_EDGE('',*,*,#43872,.F.);
#64122=ORIENTED_EDGE('',*,*,#43867,.F.);
#64123=ORIENTED_EDGE('',*,*,#43873,.T.);
#64124=ORIENTED_EDGE('',*,*,#43874,.F.);
#64125=ORIENTED_EDGE('',*,*,#43636,.T.);
#64126=ORIENTED_EDGE('',*,*,#43875,.F.);
#64127=ORIENTED_EDGE('',*,*,#43876,.F.);
#64128=ORIENTED_EDGE('',*,*,#43877,.T.);
#64129=ORIENTED_EDGE('',*,*,#43878,.F.);
#64130=ORIENTED_EDGE('',*,*,#43879,.T.);
#64131=ORIENTED_EDGE('',*,*,#43880,.F.);
#64132=ORIENTED_EDGE('',*,*,#43637,.T.);
#64133=ORIENTED_EDGE('',*,*,#43874,.T.);
#64134=ORIENTED_EDGE('',*,*,#43881,.F.);
#64135=ORIENTED_EDGE('',*,*,#43879,.F.);
#64136=ORIENTED_EDGE('',*,*,#43873,.F.);
#64137=ORIENTED_EDGE('',*,*,#43882,.F.);
#64138=ORIENTED_EDGE('',*,*,#43877,.F.);
#64139=ORIENTED_EDGE('',*,*,#43883,.T.);
#64140=ORIENTED_EDGE('',*,*,#43884,.F.);
#64141=ORIENTED_EDGE('',*,*,#43639,.T.);
#64142=ORIENTED_EDGE('',*,*,#43885,.F.);
#64143=ORIENTED_EDGE('',*,*,#43886,.F.);
#64144=ORIENTED_EDGE('',*,*,#43887,.T.);
#64145=ORIENTED_EDGE('',*,*,#43888,.F.);
#64146=ORIENTED_EDGE('',*,*,#43889,.T.);
#64147=ORIENTED_EDGE('',*,*,#43890,.F.);
#64148=ORIENTED_EDGE('',*,*,#43640,.T.);
#64149=ORIENTED_EDGE('',*,*,#43884,.T.);
#64150=ORIENTED_EDGE('',*,*,#43891,.F.);
#64151=ORIENTED_EDGE('',*,*,#43889,.F.);
#64152=ORIENTED_EDGE('',*,*,#43883,.F.);
#64153=ORIENTED_EDGE('',*,*,#43892,.F.);
#64154=ORIENTED_EDGE('',*,*,#43887,.F.);
#64155=ORIENTED_EDGE('',*,*,#43893,.T.);
#64156=ORIENTED_EDGE('',*,*,#43894,.F.);
#64157=ORIENTED_EDGE('',*,*,#43642,.T.);
#64158=ORIENTED_EDGE('',*,*,#43895,.F.);
#64159=ORIENTED_EDGE('',*,*,#43896,.F.);
#64160=ORIENTED_EDGE('',*,*,#43897,.T.);
#64161=ORIENTED_EDGE('',*,*,#43898,.F.);
#64162=ORIENTED_EDGE('',*,*,#43899,.T.);
#64163=ORIENTED_EDGE('',*,*,#43900,.F.);
#64164=ORIENTED_EDGE('',*,*,#43643,.T.);
#64165=ORIENTED_EDGE('',*,*,#43894,.T.);
#64166=ORIENTED_EDGE('',*,*,#43901,.F.);
#64167=ORIENTED_EDGE('',*,*,#43899,.F.);
#64168=ORIENTED_EDGE('',*,*,#43893,.F.);
#64169=ORIENTED_EDGE('',*,*,#43902,.F.);
#64170=ORIENTED_EDGE('',*,*,#43897,.F.);
#64171=ORIENTED_EDGE('',*,*,#43903,.T.);
#64172=ORIENTED_EDGE('',*,*,#43904,.F.);
#64173=ORIENTED_EDGE('',*,*,#43645,.T.);
#64174=ORIENTED_EDGE('',*,*,#43905,.F.);
#64175=ORIENTED_EDGE('',*,*,#43906,.F.);
#64176=ORIENTED_EDGE('',*,*,#43907,.T.);
#64177=ORIENTED_EDGE('',*,*,#43908,.F.);
#64178=ORIENTED_EDGE('',*,*,#43909,.T.);
#64179=ORIENTED_EDGE('',*,*,#43910,.F.);
#64180=ORIENTED_EDGE('',*,*,#43646,.T.);
#64181=ORIENTED_EDGE('',*,*,#43904,.T.);
#64182=ORIENTED_EDGE('',*,*,#43911,.F.);
#64183=ORIENTED_EDGE('',*,*,#43909,.F.);
#64184=ORIENTED_EDGE('',*,*,#43903,.F.);
#64185=ORIENTED_EDGE('',*,*,#43912,.F.);
#64186=ORIENTED_EDGE('',*,*,#43907,.F.);
#64187=ORIENTED_EDGE('',*,*,#43913,.T.);
#64188=ORIENTED_EDGE('',*,*,#43914,.F.);
#64189=ORIENTED_EDGE('',*,*,#43648,.T.);
#64190=ORIENTED_EDGE('',*,*,#43915,.F.);
#64191=ORIENTED_EDGE('',*,*,#43916,.F.);
#64192=ORIENTED_EDGE('',*,*,#43917,.T.);
#64193=ORIENTED_EDGE('',*,*,#43918,.F.);
#64194=ORIENTED_EDGE('',*,*,#43919,.T.);
#64195=ORIENTED_EDGE('',*,*,#43920,.F.);
#64196=ORIENTED_EDGE('',*,*,#43649,.T.);
#64197=ORIENTED_EDGE('',*,*,#43914,.T.);
#64198=ORIENTED_EDGE('',*,*,#43921,.F.);
#64199=ORIENTED_EDGE('',*,*,#43919,.F.);
#64200=ORIENTED_EDGE('',*,*,#43913,.F.);
#64201=ORIENTED_EDGE('',*,*,#43922,.F.);
#64202=ORIENTED_EDGE('',*,*,#43917,.F.);
#64203=ORIENTED_EDGE('',*,*,#43923,.T.);
#64204=ORIENTED_EDGE('',*,*,#43924,.F.);
#64205=ORIENTED_EDGE('',*,*,#43651,.T.);
#64206=ORIENTED_EDGE('',*,*,#43925,.F.);
#64207=ORIENTED_EDGE('',*,*,#43926,.F.);
#64208=ORIENTED_EDGE('',*,*,#43927,.T.);
#64209=ORIENTED_EDGE('',*,*,#43928,.F.);
#64210=ORIENTED_EDGE('',*,*,#43929,.T.);
#64211=ORIENTED_EDGE('',*,*,#43930,.F.);
#64212=ORIENTED_EDGE('',*,*,#43652,.T.);
#64213=ORIENTED_EDGE('',*,*,#43924,.T.);
#64214=ORIENTED_EDGE('',*,*,#43931,.F.);
#64215=ORIENTED_EDGE('',*,*,#43929,.F.);
#64216=ORIENTED_EDGE('',*,*,#43923,.F.);
#64217=ORIENTED_EDGE('',*,*,#43932,.F.);
#64218=ORIENTED_EDGE('',*,*,#43927,.F.);
#64219=ORIENTED_EDGE('',*,*,#43933,.F.);
#64220=ORIENTED_EDGE('',*,*,#43934,.T.);
#64221=ORIENTED_EDGE('',*,*,#43935,.F.);
#64222=ORIENTED_EDGE('',*,*,#43936,.F.);
#64223=ORIENTED_EDGE('',*,*,#43655,.F.);
#64224=ORIENTED_EDGE('',*,*,#43937,.F.);
#64225=ORIENTED_EDGE('',*,*,#43938,.F.);
#64226=ORIENTED_EDGE('',*,*,#43934,.F.);
#64227=ORIENTED_EDGE('',*,*,#43937,.T.);
#64228=ORIENTED_EDGE('',*,*,#43657,.T.);
#64229=ORIENTED_EDGE('',*,*,#43654,.T.);
#64230=ORIENTED_EDGE('',*,*,#43939,.F.);
#64231=ORIENTED_EDGE('',*,*,#34245,.T.);
#64232=ORIENTED_EDGE('',*,*,#34155,.F.);
#64233=ORIENTED_EDGE('',*,*,#43656,.T.);
#64234=ORIENTED_EDGE('',*,*,#43936,.T.);
#64235=ORIENTED_EDGE('',*,*,#43933,.T.);
#64236=ORIENTED_EDGE('',*,*,#43940,.F.);
#64237=ORIENTED_EDGE('',*,*,#43941,.F.);
#64238=ORIENTED_EDGE('',*,*,#43942,.F.);
#64239=ORIENTED_EDGE('',*,*,#43943,.F.);
#64240=ORIENTED_EDGE('',*,*,#43663,.T.);
#64241=ORIENTED_EDGE('',*,*,#43667,.T.);
#64242=ORIENTED_EDGE('',*,*,#43660,.T.);
#64243=ORIENTED_EDGE('',*,*,#43665,.T.);
#64244=ORIENTED_EDGE('',*,*,#43666,.T.);
#64245=ORIENTED_EDGE('',*,*,#43661,.T.);
#64246=ORIENTED_EDGE('',*,*,#43943,.T.);
#64247=ORIENTED_EDGE('',*,*,#43944,.F.);
#64248=ORIENTED_EDGE('',*,*,#43945,.F.);
#64249=ORIENTED_EDGE('',*,*,#43946,.F.);
#64250=ORIENTED_EDGE('',*,*,#43673,.T.);
#64251=ORIENTED_EDGE('',*,*,#43677,.T.);
#64252=ORIENTED_EDGE('',*,*,#43670,.T.);
#64253=ORIENTED_EDGE('',*,*,#43675,.T.);
#64254=ORIENTED_EDGE('',*,*,#43676,.T.);
#64255=ORIENTED_EDGE('',*,*,#43671,.T.);
#64256=ORIENTED_EDGE('',*,*,#43946,.T.);
#64257=ORIENTED_EDGE('',*,*,#43947,.F.);
#64258=ORIENTED_EDGE('',*,*,#43948,.F.);
#64259=ORIENTED_EDGE('',*,*,#43949,.F.);
#64260=ORIENTED_EDGE('',*,*,#43683,.T.);
#64261=ORIENTED_EDGE('',*,*,#43687,.T.);
#64262=ORIENTED_EDGE('',*,*,#43680,.T.);
#64263=ORIENTED_EDGE('',*,*,#43685,.T.);
#64264=ORIENTED_EDGE('',*,*,#43686,.T.);
#64265=ORIENTED_EDGE('',*,*,#43681,.T.);
#64266=ORIENTED_EDGE('',*,*,#43949,.T.);
#64267=ORIENTED_EDGE('',*,*,#43950,.F.);
#64268=ORIENTED_EDGE('',*,*,#43951,.F.);
#64269=ORIENTED_EDGE('',*,*,#43952,.F.);
#64270=ORIENTED_EDGE('',*,*,#43693,.T.);
#64271=ORIENTED_EDGE('',*,*,#43697,.T.);
#64272=ORIENTED_EDGE('',*,*,#43690,.T.);
#64273=ORIENTED_EDGE('',*,*,#43695,.T.);
#64274=ORIENTED_EDGE('',*,*,#43696,.T.);
#64275=ORIENTED_EDGE('',*,*,#43691,.T.);
#64276=ORIENTED_EDGE('',*,*,#43952,.T.);
#64277=ORIENTED_EDGE('',*,*,#43953,.F.);
#64278=ORIENTED_EDGE('',*,*,#43954,.F.);
#64279=ORIENTED_EDGE('',*,*,#43955,.F.);
#64280=ORIENTED_EDGE('',*,*,#43703,.T.);
#64281=ORIENTED_EDGE('',*,*,#43707,.T.);
#64282=ORIENTED_EDGE('',*,*,#43700,.T.);
#64283=ORIENTED_EDGE('',*,*,#43705,.T.);
#64284=ORIENTED_EDGE('',*,*,#43706,.T.);
#64285=ORIENTED_EDGE('',*,*,#43701,.T.);
#64286=ORIENTED_EDGE('',*,*,#43955,.T.);
#64287=ORIENTED_EDGE('',*,*,#43956,.F.);
#64288=ORIENTED_EDGE('',*,*,#43957,.F.);
#64289=ORIENTED_EDGE('',*,*,#43958,.F.);
#64290=ORIENTED_EDGE('',*,*,#43713,.T.);
#64291=ORIENTED_EDGE('',*,*,#43717,.T.);
#64292=ORIENTED_EDGE('',*,*,#43710,.T.);
#64293=ORIENTED_EDGE('',*,*,#43715,.T.);
#64294=ORIENTED_EDGE('',*,*,#43716,.T.);
#64295=ORIENTED_EDGE('',*,*,#43711,.T.);
#64296=ORIENTED_EDGE('',*,*,#43958,.T.);
#64297=ORIENTED_EDGE('',*,*,#43959,.F.);
#64298=ORIENTED_EDGE('',*,*,#43960,.F.);
#64299=ORIENTED_EDGE('',*,*,#43961,.F.);
#64300=ORIENTED_EDGE('',*,*,#43721,.T.);
#64301=ORIENTED_EDGE('',*,*,#34343,.T.);
#64302=ORIENTED_EDGE('',*,*,#43719,.T.);
#64303=ORIENTED_EDGE('',*,*,#43722,.T.);
#64304=ORIENTED_EDGE('',*,*,#34345,.T.);
#64305=ORIENTED_EDGE('',*,*,#43720,.T.);
#64306=ORIENTED_EDGE('',*,*,#43961,.T.);
#64307=ORIENTED_EDGE('',*,*,#43962,.F.);
#64308=ORIENTED_EDGE('',*,*,#43963,.F.);
#64309=ORIENTED_EDGE('',*,*,#43964,.F.);
#64310=ORIENTED_EDGE('',*,*,#43728,.T.);
#64311=ORIENTED_EDGE('',*,*,#43732,.T.);
#64312=ORIENTED_EDGE('',*,*,#43725,.T.);
#64313=ORIENTED_EDGE('',*,*,#43730,.T.);
#64314=ORIENTED_EDGE('',*,*,#43731,.T.);
#64315=ORIENTED_EDGE('',*,*,#43726,.T.);
#64316=ORIENTED_EDGE('',*,*,#43964,.T.);
#64317=ORIENTED_EDGE('',*,*,#43965,.F.);
#64318=ORIENTED_EDGE('',*,*,#43966,.F.);
#64319=ORIENTED_EDGE('',*,*,#43967,.F.);
#64320=ORIENTED_EDGE('',*,*,#43738,.T.);
#64321=ORIENTED_EDGE('',*,*,#43742,.T.);
#64322=ORIENTED_EDGE('',*,*,#43735,.T.);
#64323=ORIENTED_EDGE('',*,*,#43740,.T.);
#64324=ORIENTED_EDGE('',*,*,#43741,.T.);
#64325=ORIENTED_EDGE('',*,*,#43736,.T.);
#64326=ORIENTED_EDGE('',*,*,#43967,.T.);
#64327=ORIENTED_EDGE('',*,*,#43968,.F.);
#64328=ORIENTED_EDGE('',*,*,#43969,.F.);
#64329=ORIENTED_EDGE('',*,*,#43970,.F.);
#64330=ORIENTED_EDGE('',*,*,#43748,.T.);
#64331=ORIENTED_EDGE('',*,*,#43752,.T.);
#64332=ORIENTED_EDGE('',*,*,#43745,.T.);
#64333=ORIENTED_EDGE('',*,*,#43750,.T.);
#64334=ORIENTED_EDGE('',*,*,#43751,.T.);
#64335=ORIENTED_EDGE('',*,*,#43746,.T.);
#64336=ORIENTED_EDGE('',*,*,#43970,.T.);
#64337=ORIENTED_EDGE('',*,*,#43971,.F.);
#64338=ORIENTED_EDGE('',*,*,#43972,.F.);
#64339=ORIENTED_EDGE('',*,*,#43973,.F.);
#64340=ORIENTED_EDGE('',*,*,#43758,.T.);
#64341=ORIENTED_EDGE('',*,*,#43762,.T.);
#64342=ORIENTED_EDGE('',*,*,#43755,.T.);
#64343=ORIENTED_EDGE('',*,*,#43760,.T.);
#64344=ORIENTED_EDGE('',*,*,#43761,.T.);
#64345=ORIENTED_EDGE('',*,*,#43756,.T.);
#64346=ORIENTED_EDGE('',*,*,#43973,.T.);
#64347=ORIENTED_EDGE('',*,*,#43974,.F.);
#64348=ORIENTED_EDGE('',*,*,#43975,.F.);
#64349=ORIENTED_EDGE('',*,*,#43976,.F.);
#64350=ORIENTED_EDGE('',*,*,#43768,.T.);
#64351=ORIENTED_EDGE('',*,*,#43772,.T.);
#64352=ORIENTED_EDGE('',*,*,#43765,.T.);
#64353=ORIENTED_EDGE('',*,*,#43770,.T.);
#64354=ORIENTED_EDGE('',*,*,#43771,.T.);
#64355=ORIENTED_EDGE('',*,*,#43766,.T.);
#64356=ORIENTED_EDGE('',*,*,#43976,.T.);
#64357=ORIENTED_EDGE('',*,*,#43977,.F.);
#64358=ORIENTED_EDGE('',*,*,#43978,.F.);
#64359=ORIENTED_EDGE('',*,*,#43979,.F.);
#64360=ORIENTED_EDGE('',*,*,#43778,.T.);
#64361=ORIENTED_EDGE('',*,*,#43782,.T.);
#64362=ORIENTED_EDGE('',*,*,#43775,.T.);
#64363=ORIENTED_EDGE('',*,*,#43780,.T.);
#64364=ORIENTED_EDGE('',*,*,#43781,.T.);
#64365=ORIENTED_EDGE('',*,*,#43776,.T.);
#64366=ORIENTED_EDGE('',*,*,#43979,.T.);
#64367=ORIENTED_EDGE('',*,*,#43980,.F.);
#64368=ORIENTED_EDGE('',*,*,#43981,.F.);
#64369=ORIENTED_EDGE('',*,*,#43982,.F.);
#64370=ORIENTED_EDGE('',*,*,#43788,.T.);
#64371=ORIENTED_EDGE('',*,*,#43792,.T.);
#64372=ORIENTED_EDGE('',*,*,#43785,.T.);
#64373=ORIENTED_EDGE('',*,*,#43790,.T.);
#64374=ORIENTED_EDGE('',*,*,#43791,.T.);
#64375=ORIENTED_EDGE('',*,*,#43786,.T.);
#64376=ORIENTED_EDGE('',*,*,#43982,.T.);
#64377=ORIENTED_EDGE('',*,*,#43983,.F.);
#64378=ORIENTED_EDGE('',*,*,#43984,.F.);
#64379=ORIENTED_EDGE('',*,*,#43985,.F.);
#64380=ORIENTED_EDGE('',*,*,#43798,.T.);
#64381=ORIENTED_EDGE('',*,*,#43802,.T.);
#64382=ORIENTED_EDGE('',*,*,#43795,.T.);
#64383=ORIENTED_EDGE('',*,*,#43800,.T.);
#64384=ORIENTED_EDGE('',*,*,#43801,.T.);
#64385=ORIENTED_EDGE('',*,*,#43796,.T.);
#64386=ORIENTED_EDGE('',*,*,#43985,.T.);
#64387=ORIENTED_EDGE('',*,*,#43986,.F.);
#64388=ORIENTED_EDGE('',*,*,#43987,.F.);
#64389=ORIENTED_EDGE('',*,*,#43988,.F.);
#64390=ORIENTED_EDGE('',*,*,#43808,.T.);
#64391=ORIENTED_EDGE('',*,*,#43812,.T.);
#64392=ORIENTED_EDGE('',*,*,#43805,.T.);
#64393=ORIENTED_EDGE('',*,*,#43810,.T.);
#64394=ORIENTED_EDGE('',*,*,#43811,.T.);
#64395=ORIENTED_EDGE('',*,*,#43806,.T.);
#64396=ORIENTED_EDGE('',*,*,#43988,.T.);
#64397=ORIENTED_EDGE('',*,*,#43989,.F.);
#64398=ORIENTED_EDGE('',*,*,#43990,.F.);
#64399=ORIENTED_EDGE('',*,*,#43991,.F.);
#64400=ORIENTED_EDGE('',*,*,#43818,.T.);
#64401=ORIENTED_EDGE('',*,*,#43822,.T.);
#64402=ORIENTED_EDGE('',*,*,#43815,.T.);
#64403=ORIENTED_EDGE('',*,*,#43820,.T.);
#64404=ORIENTED_EDGE('',*,*,#43821,.T.);
#64405=ORIENTED_EDGE('',*,*,#43816,.T.);
#64406=ORIENTED_EDGE('',*,*,#43991,.T.);
#64407=ORIENTED_EDGE('',*,*,#43992,.F.);
#64408=ORIENTED_EDGE('',*,*,#43993,.F.);
#64409=ORIENTED_EDGE('',*,*,#43994,.F.);
#64410=ORIENTED_EDGE('',*,*,#43828,.T.);
#64411=ORIENTED_EDGE('',*,*,#43832,.T.);
#64412=ORIENTED_EDGE('',*,*,#43823,.T.);
#64413=ORIENTED_EDGE('',*,*,#43830,.T.);
#64414=ORIENTED_EDGE('',*,*,#43831,.T.);
#64415=ORIENTED_EDGE('',*,*,#43826,.T.);
#64416=ORIENTED_EDGE('',*,*,#43994,.T.);
#64417=ORIENTED_EDGE('',*,*,#43995,.F.);
#64418=ORIENTED_EDGE('',*,*,#43996,.F.);
#64419=ORIENTED_EDGE('',*,*,#43997,.F.);
#64420=ORIENTED_EDGE('',*,*,#43838,.T.);
#64421=ORIENTED_EDGE('',*,*,#43842,.T.);
#64422=ORIENTED_EDGE('',*,*,#43835,.T.);
#64423=ORIENTED_EDGE('',*,*,#43840,.T.);
#64424=ORIENTED_EDGE('',*,*,#43841,.T.);
#64425=ORIENTED_EDGE('',*,*,#43836,.T.);
#64426=ORIENTED_EDGE('',*,*,#43997,.T.);
#64427=ORIENTED_EDGE('',*,*,#43998,.F.);
#64428=ORIENTED_EDGE('',*,*,#43999,.F.);
#64429=ORIENTED_EDGE('',*,*,#44000,.F.);
#64430=ORIENTED_EDGE('',*,*,#43848,.T.);
#64431=ORIENTED_EDGE('',*,*,#43852,.T.);
#64432=ORIENTED_EDGE('',*,*,#43845,.T.);
#64433=ORIENTED_EDGE('',*,*,#43850,.T.);
#64434=ORIENTED_EDGE('',*,*,#43851,.T.);
#64435=ORIENTED_EDGE('',*,*,#43846,.T.);
#64436=ORIENTED_EDGE('',*,*,#44000,.T.);
#64437=ORIENTED_EDGE('',*,*,#44001,.F.);
#64438=ORIENTED_EDGE('',*,*,#44002,.F.);
#64439=ORIENTED_EDGE('',*,*,#44003,.F.);
#64440=ORIENTED_EDGE('',*,*,#43858,.T.);
#64441=ORIENTED_EDGE('',*,*,#43862,.T.);
#64442=ORIENTED_EDGE('',*,*,#43855,.T.);
#64443=ORIENTED_EDGE('',*,*,#43860,.T.);
#64444=ORIENTED_EDGE('',*,*,#43861,.T.);
#64445=ORIENTED_EDGE('',*,*,#43856,.T.);
#64446=ORIENTED_EDGE('',*,*,#44003,.T.);
#64447=ORIENTED_EDGE('',*,*,#44004,.F.);
#64448=ORIENTED_EDGE('',*,*,#44005,.F.);
#64449=ORIENTED_EDGE('',*,*,#44006,.F.);
#64450=ORIENTED_EDGE('',*,*,#43868,.T.);
#64451=ORIENTED_EDGE('',*,*,#43872,.T.);
#64452=ORIENTED_EDGE('',*,*,#43865,.T.);
#64453=ORIENTED_EDGE('',*,*,#43870,.T.);
#64454=ORIENTED_EDGE('',*,*,#43871,.T.);
#64455=ORIENTED_EDGE('',*,*,#43866,.T.);
#64456=ORIENTED_EDGE('',*,*,#44006,.T.);
#64457=ORIENTED_EDGE('',*,*,#44007,.F.);
#64458=ORIENTED_EDGE('',*,*,#44008,.F.);
#64459=ORIENTED_EDGE('',*,*,#44009,.F.);
#64460=ORIENTED_EDGE('',*,*,#43878,.T.);
#64461=ORIENTED_EDGE('',*,*,#43882,.T.);
#64462=ORIENTED_EDGE('',*,*,#43875,.T.);
#64463=ORIENTED_EDGE('',*,*,#43880,.T.);
#64464=ORIENTED_EDGE('',*,*,#43881,.T.);
#64465=ORIENTED_EDGE('',*,*,#43876,.T.);
#64466=ORIENTED_EDGE('',*,*,#44009,.T.);
#64467=ORIENTED_EDGE('',*,*,#44010,.F.);
#64468=ORIENTED_EDGE('',*,*,#44011,.F.);
#64469=ORIENTED_EDGE('',*,*,#44012,.F.);
#64470=ORIENTED_EDGE('',*,*,#43888,.T.);
#64471=ORIENTED_EDGE('',*,*,#43892,.T.);
#64472=ORIENTED_EDGE('',*,*,#43885,.T.);
#64473=ORIENTED_EDGE('',*,*,#43890,.T.);
#64474=ORIENTED_EDGE('',*,*,#43891,.T.);
#64475=ORIENTED_EDGE('',*,*,#43886,.T.);
#64476=ORIENTED_EDGE('',*,*,#44012,.T.);
#64477=ORIENTED_EDGE('',*,*,#44013,.F.);
#64478=ORIENTED_EDGE('',*,*,#44014,.F.);
#64479=ORIENTED_EDGE('',*,*,#44015,.F.);
#64480=ORIENTED_EDGE('',*,*,#43898,.T.);
#64481=ORIENTED_EDGE('',*,*,#43902,.T.);
#64482=ORIENTED_EDGE('',*,*,#43895,.T.);
#64483=ORIENTED_EDGE('',*,*,#43900,.T.);
#64484=ORIENTED_EDGE('',*,*,#43901,.T.);
#64485=ORIENTED_EDGE('',*,*,#43896,.T.);
#64486=ORIENTED_EDGE('',*,*,#44015,.T.);
#64487=ORIENTED_EDGE('',*,*,#44016,.F.);
#64488=ORIENTED_EDGE('',*,*,#44017,.F.);
#64489=ORIENTED_EDGE('',*,*,#44018,.F.);
#64490=ORIENTED_EDGE('',*,*,#43908,.T.);
#64491=ORIENTED_EDGE('',*,*,#43912,.T.);
#64492=ORIENTED_EDGE('',*,*,#43905,.T.);
#64493=ORIENTED_EDGE('',*,*,#43910,.T.);
#64494=ORIENTED_EDGE('',*,*,#43911,.T.);
#64495=ORIENTED_EDGE('',*,*,#43906,.T.);
#64496=ORIENTED_EDGE('',*,*,#44018,.T.);
#64497=ORIENTED_EDGE('',*,*,#44019,.F.);
#64498=ORIENTED_EDGE('',*,*,#44020,.F.);
#64499=ORIENTED_EDGE('',*,*,#44021,.F.);
#64500=ORIENTED_EDGE('',*,*,#43918,.T.);
#64501=ORIENTED_EDGE('',*,*,#43922,.T.);
#64502=ORIENTED_EDGE('',*,*,#43915,.T.);
#64503=ORIENTED_EDGE('',*,*,#43920,.T.);
#64504=ORIENTED_EDGE('',*,*,#43921,.T.);
#64505=ORIENTED_EDGE('',*,*,#43916,.T.);
#64506=ORIENTED_EDGE('',*,*,#44021,.T.);
#64507=ORIENTED_EDGE('',*,*,#44022,.F.);
#64508=ORIENTED_EDGE('',*,*,#44023,.F.);
#64509=ORIENTED_EDGE('',*,*,#44024,.F.);
#64510=ORIENTED_EDGE('',*,*,#43928,.T.);
#64511=ORIENTED_EDGE('',*,*,#43932,.T.);
#64512=ORIENTED_EDGE('',*,*,#43925,.T.);
#64513=ORIENTED_EDGE('',*,*,#43930,.T.);
#64514=ORIENTED_EDGE('',*,*,#43931,.T.);
#64515=ORIENTED_EDGE('',*,*,#43926,.T.);
#64516=ORIENTED_EDGE('',*,*,#44024,.T.);
#64517=ORIENTED_EDGE('',*,*,#44025,.F.);
#64518=ORIENTED_EDGE('',*,*,#44026,.F.);
#64519=ORIENTED_EDGE('',*,*,#43940,.T.);
#64520=ORIENTED_EDGE('',*,*,#43935,.T.);
#64521=ORIENTED_EDGE('',*,*,#43938,.T.);
#64522=ORIENTED_EDGE('',*,*,#43939,.T.);
#64523=ORIENTED_EDGE('',*,*,#43941,.T.);
#64524=ORIENTED_EDGE('',*,*,#44027,.F.);
#64525=ORIENTED_EDGE('',*,*,#44028,.T.);
#64526=ORIENTED_EDGE('',*,*,#44029,.F.);
#64527=ORIENTED_EDGE('',*,*,#44030,.F.);
#64528=ORIENTED_EDGE('',*,*,#44031,.F.);
#64529=ORIENTED_EDGE('',*,*,#44028,.F.);
#64530=ORIENTED_EDGE('',*,*,#44032,.F.);
#64531=ORIENTED_EDGE('',*,*,#44029,.T.);
#64532=ORIENTED_EDGE('',*,*,#44031,.T.);
#64533=ORIENTED_EDGE('',*,*,#44033,.F.);
#64534=ORIENTED_EDGE('',*,*,#43942,.T.);
#64535=ORIENTED_EDGE('',*,*,#43944,.T.);
#64536=ORIENTED_EDGE('',*,*,#44034,.F.);
#64537=ORIENTED_EDGE('',*,*,#44035,.T.);
#64538=ORIENTED_EDGE('',*,*,#44036,.F.);
#64539=ORIENTED_EDGE('',*,*,#44037,.F.);
#64540=ORIENTED_EDGE('',*,*,#44038,.F.);
#64541=ORIENTED_EDGE('',*,*,#44035,.F.);
#64542=ORIENTED_EDGE('',*,*,#44039,.F.);
#64543=ORIENTED_EDGE('',*,*,#44036,.T.);
#64544=ORIENTED_EDGE('',*,*,#44038,.T.);
#64545=ORIENTED_EDGE('',*,*,#44040,.F.);
#64546=ORIENTED_EDGE('',*,*,#43945,.T.);
#64547=ORIENTED_EDGE('',*,*,#43947,.T.);
#64548=ORIENTED_EDGE('',*,*,#44041,.F.);
#64549=ORIENTED_EDGE('',*,*,#44042,.T.);
#64550=ORIENTED_EDGE('',*,*,#44043,.F.);
#64551=ORIENTED_EDGE('',*,*,#44044,.F.);
#64552=ORIENTED_EDGE('',*,*,#44045,.F.);
#64553=ORIENTED_EDGE('',*,*,#44042,.F.);
#64554=ORIENTED_EDGE('',*,*,#44046,.F.);
#64555=ORIENTED_EDGE('',*,*,#44043,.T.);
#64556=ORIENTED_EDGE('',*,*,#44045,.T.);
#64557=ORIENTED_EDGE('',*,*,#44047,.F.);
#64558=ORIENTED_EDGE('',*,*,#43948,.T.);
#64559=ORIENTED_EDGE('',*,*,#43950,.T.);
#64560=ORIENTED_EDGE('',*,*,#44048,.F.);
#64561=ORIENTED_EDGE('',*,*,#44049,.T.);
#64562=ORIENTED_EDGE('',*,*,#44050,.F.);
#64563=ORIENTED_EDGE('',*,*,#44051,.F.);
#64564=ORIENTED_EDGE('',*,*,#44052,.F.);
#64565=ORIENTED_EDGE('',*,*,#44049,.F.);
#64566=ORIENTED_EDGE('',*,*,#44053,.F.);
#64567=ORIENTED_EDGE('',*,*,#44050,.T.);
#64568=ORIENTED_EDGE('',*,*,#44052,.T.);
#64569=ORIENTED_EDGE('',*,*,#44054,.F.);
#64570=ORIENTED_EDGE('',*,*,#43951,.T.);
#64571=ORIENTED_EDGE('',*,*,#43953,.T.);
#64572=ORIENTED_EDGE('',*,*,#44055,.F.);
#64573=ORIENTED_EDGE('',*,*,#44056,.T.);
#64574=ORIENTED_EDGE('',*,*,#44057,.F.);
#64575=ORIENTED_EDGE('',*,*,#44058,.F.);
#64576=ORIENTED_EDGE('',*,*,#44059,.F.);
#64577=ORIENTED_EDGE('',*,*,#44056,.F.);
#64578=ORIENTED_EDGE('',*,*,#44060,.F.);
#64579=ORIENTED_EDGE('',*,*,#44057,.T.);
#64580=ORIENTED_EDGE('',*,*,#44059,.T.);
#64581=ORIENTED_EDGE('',*,*,#44061,.F.);
#64582=ORIENTED_EDGE('',*,*,#43954,.T.);
#64583=ORIENTED_EDGE('',*,*,#43956,.T.);
#64584=ORIENTED_EDGE('',*,*,#44062,.F.);
#64585=ORIENTED_EDGE('',*,*,#44063,.T.);
#64586=ORIENTED_EDGE('',*,*,#44064,.F.);
#64587=ORIENTED_EDGE('',*,*,#44065,.F.);
#64588=ORIENTED_EDGE('',*,*,#44066,.F.);
#64589=ORIENTED_EDGE('',*,*,#44063,.F.);
#64590=ORIENTED_EDGE('',*,*,#44067,.F.);
#64591=ORIENTED_EDGE('',*,*,#44064,.T.);
#64592=ORIENTED_EDGE('',*,*,#44066,.T.);
#64593=ORIENTED_EDGE('',*,*,#44068,.F.);
#64594=ORIENTED_EDGE('',*,*,#43957,.T.);
#64595=ORIENTED_EDGE('',*,*,#43959,.T.);
#64596=ORIENTED_EDGE('',*,*,#44069,.F.);
#64597=ORIENTED_EDGE('',*,*,#44070,.T.);
#64598=ORIENTED_EDGE('',*,*,#44071,.F.);
#64599=ORIENTED_EDGE('',*,*,#44072,.F.);
#64600=ORIENTED_EDGE('',*,*,#44073,.F.);
#64601=ORIENTED_EDGE('',*,*,#44070,.F.);
#64602=ORIENTED_EDGE('',*,*,#44074,.F.);
#64603=ORIENTED_EDGE('',*,*,#44071,.T.);
#64604=ORIENTED_EDGE('',*,*,#44073,.T.);
#64605=ORIENTED_EDGE('',*,*,#44075,.F.);
#64606=ORIENTED_EDGE('',*,*,#43960,.T.);
#64607=ORIENTED_EDGE('',*,*,#43962,.T.);
#64608=ORIENTED_EDGE('',*,*,#44076,.F.);
#64609=ORIENTED_EDGE('',*,*,#44077,.T.);
#64610=ORIENTED_EDGE('',*,*,#44078,.F.);
#64611=ORIENTED_EDGE('',*,*,#44079,.F.);
#64612=ORIENTED_EDGE('',*,*,#44080,.F.);
#64613=ORIENTED_EDGE('',*,*,#44077,.F.);
#64614=ORIENTED_EDGE('',*,*,#44081,.F.);
#64615=ORIENTED_EDGE('',*,*,#44078,.T.);
#64616=ORIENTED_EDGE('',*,*,#44080,.T.);
#64617=ORIENTED_EDGE('',*,*,#44082,.F.);
#64618=ORIENTED_EDGE('',*,*,#43963,.T.);
#64619=ORIENTED_EDGE('',*,*,#43965,.T.);
#64620=ORIENTED_EDGE('',*,*,#44083,.F.);
#64621=ORIENTED_EDGE('',*,*,#44084,.T.);
#64622=ORIENTED_EDGE('',*,*,#44085,.F.);
#64623=ORIENTED_EDGE('',*,*,#44086,.F.);
#64624=ORIENTED_EDGE('',*,*,#44087,.F.);
#64625=ORIENTED_EDGE('',*,*,#44084,.F.);
#64626=ORIENTED_EDGE('',*,*,#44088,.F.);
#64627=ORIENTED_EDGE('',*,*,#44085,.T.);
#64628=ORIENTED_EDGE('',*,*,#44087,.T.);
#64629=ORIENTED_EDGE('',*,*,#44089,.F.);
#64630=ORIENTED_EDGE('',*,*,#43966,.T.);
#64631=ORIENTED_EDGE('',*,*,#43968,.T.);
#64632=ORIENTED_EDGE('',*,*,#44090,.F.);
#64633=ORIENTED_EDGE('',*,*,#44091,.T.);
#64634=ORIENTED_EDGE('',*,*,#44092,.F.);
#64635=ORIENTED_EDGE('',*,*,#44093,.F.);
#64636=ORIENTED_EDGE('',*,*,#44094,.F.);
#64637=ORIENTED_EDGE('',*,*,#44091,.F.);
#64638=ORIENTED_EDGE('',*,*,#44095,.F.);
#64639=ORIENTED_EDGE('',*,*,#44092,.T.);
#64640=ORIENTED_EDGE('',*,*,#44094,.T.);
#64641=ORIENTED_EDGE('',*,*,#44096,.F.);
#64642=ORIENTED_EDGE('',*,*,#43969,.T.);
#64643=ORIENTED_EDGE('',*,*,#43971,.T.);
#64644=ORIENTED_EDGE('',*,*,#44097,.F.);
#64645=ORIENTED_EDGE('',*,*,#44098,.T.);
#64646=ORIENTED_EDGE('',*,*,#44099,.F.);
#64647=ORIENTED_EDGE('',*,*,#44100,.F.);
#64648=ORIENTED_EDGE('',*,*,#44101,.F.);
#64649=ORIENTED_EDGE('',*,*,#44098,.F.);
#64650=ORIENTED_EDGE('',*,*,#44102,.F.);
#64651=ORIENTED_EDGE('',*,*,#44099,.T.);
#64652=ORIENTED_EDGE('',*,*,#44101,.T.);
#64653=ORIENTED_EDGE('',*,*,#44103,.F.);
#64654=ORIENTED_EDGE('',*,*,#43972,.T.);
#64655=ORIENTED_EDGE('',*,*,#43974,.T.);
#64656=ORIENTED_EDGE('',*,*,#44104,.F.);
#64657=ORIENTED_EDGE('',*,*,#44105,.T.);
#64658=ORIENTED_EDGE('',*,*,#44106,.F.);
#64659=ORIENTED_EDGE('',*,*,#44107,.F.);
#64660=ORIENTED_EDGE('',*,*,#44108,.F.);
#64661=ORIENTED_EDGE('',*,*,#44105,.F.);
#64662=ORIENTED_EDGE('',*,*,#44109,.F.);
#64663=ORIENTED_EDGE('',*,*,#44106,.T.);
#64664=ORIENTED_EDGE('',*,*,#44108,.T.);
#64665=ORIENTED_EDGE('',*,*,#44110,.F.);
#64666=ORIENTED_EDGE('',*,*,#43975,.T.);
#64667=ORIENTED_EDGE('',*,*,#43977,.T.);
#64668=ORIENTED_EDGE('',*,*,#44111,.F.);
#64669=ORIENTED_EDGE('',*,*,#44112,.T.);
#64670=ORIENTED_EDGE('',*,*,#44113,.F.);
#64671=ORIENTED_EDGE('',*,*,#44114,.F.);
#64672=ORIENTED_EDGE('',*,*,#44115,.F.);
#64673=ORIENTED_EDGE('',*,*,#44112,.F.);
#64674=ORIENTED_EDGE('',*,*,#44116,.F.);
#64675=ORIENTED_EDGE('',*,*,#44113,.T.);
#64676=ORIENTED_EDGE('',*,*,#44115,.T.);
#64677=ORIENTED_EDGE('',*,*,#44117,.F.);
#64678=ORIENTED_EDGE('',*,*,#43978,.T.);
#64679=ORIENTED_EDGE('',*,*,#43980,.T.);
#64680=ORIENTED_EDGE('',*,*,#44118,.F.);
#64681=ORIENTED_EDGE('',*,*,#44119,.T.);
#64682=ORIENTED_EDGE('',*,*,#44120,.F.);
#64683=ORIENTED_EDGE('',*,*,#44121,.F.);
#64684=ORIENTED_EDGE('',*,*,#44122,.F.);
#64685=ORIENTED_EDGE('',*,*,#44119,.F.);
#64686=ORIENTED_EDGE('',*,*,#44123,.F.);
#64687=ORIENTED_EDGE('',*,*,#44120,.T.);
#64688=ORIENTED_EDGE('',*,*,#44122,.T.);
#64689=ORIENTED_EDGE('',*,*,#44124,.F.);
#64690=ORIENTED_EDGE('',*,*,#43981,.T.);
#64691=ORIENTED_EDGE('',*,*,#43983,.T.);
#64692=ORIENTED_EDGE('',*,*,#44125,.F.);
#64693=ORIENTED_EDGE('',*,*,#44126,.T.);
#64694=ORIENTED_EDGE('',*,*,#44127,.F.);
#64695=ORIENTED_EDGE('',*,*,#44128,.F.);
#64696=ORIENTED_EDGE('',*,*,#44129,.F.);
#64697=ORIENTED_EDGE('',*,*,#44126,.F.);
#64698=ORIENTED_EDGE('',*,*,#44130,.F.);
#64699=ORIENTED_EDGE('',*,*,#44127,.T.);
#64700=ORIENTED_EDGE('',*,*,#44129,.T.);
#64701=ORIENTED_EDGE('',*,*,#44131,.F.);
#64702=ORIENTED_EDGE('',*,*,#43984,.T.);
#64703=ORIENTED_EDGE('',*,*,#43986,.T.);
#64704=ORIENTED_EDGE('',*,*,#44132,.F.);
#64705=ORIENTED_EDGE('',*,*,#44133,.T.);
#64706=ORIENTED_EDGE('',*,*,#44134,.F.);
#64707=ORIENTED_EDGE('',*,*,#44135,.F.);
#64708=ORIENTED_EDGE('',*,*,#44136,.F.);
#64709=ORIENTED_EDGE('',*,*,#44133,.F.);
#64710=ORIENTED_EDGE('',*,*,#44137,.F.);
#64711=ORIENTED_EDGE('',*,*,#44134,.T.);
#64712=ORIENTED_EDGE('',*,*,#44136,.T.);
#64713=ORIENTED_EDGE('',*,*,#44138,.F.);
#64714=ORIENTED_EDGE('',*,*,#43987,.T.);
#64715=ORIENTED_EDGE('',*,*,#43989,.T.);
#64716=ORIENTED_EDGE('',*,*,#44139,.F.);
#64717=ORIENTED_EDGE('',*,*,#44140,.T.);
#64718=ORIENTED_EDGE('',*,*,#44141,.F.);
#64719=ORIENTED_EDGE('',*,*,#44142,.F.);
#64720=ORIENTED_EDGE('',*,*,#44143,.F.);
#64721=ORIENTED_EDGE('',*,*,#44140,.F.);
#64722=ORIENTED_EDGE('',*,*,#44144,.F.);
#64723=ORIENTED_EDGE('',*,*,#44141,.T.);
#64724=ORIENTED_EDGE('',*,*,#44143,.T.);
#64725=ORIENTED_EDGE('',*,*,#44145,.F.);
#64726=ORIENTED_EDGE('',*,*,#43990,.T.);
#64727=ORIENTED_EDGE('',*,*,#43992,.T.);
#64728=ORIENTED_EDGE('',*,*,#44146,.F.);
#64729=ORIENTED_EDGE('',*,*,#44147,.T.);
#64730=ORIENTED_EDGE('',*,*,#44148,.F.);
#64731=ORIENTED_EDGE('',*,*,#44147,.F.);
#64732=ORIENTED_EDGE('',*,*,#44149,.F.);
#64733=ORIENTED_EDGE('',*,*,#44150,.F.);
#64734=ORIENTED_EDGE('',*,*,#44151,.F.);
#64735=ORIENTED_EDGE('',*,*,#44148,.T.);
#64736=ORIENTED_EDGE('',*,*,#44151,.T.);
#64737=ORIENTED_EDGE('',*,*,#44152,.F.);
#64738=ORIENTED_EDGE('',*,*,#43993,.T.);
#64739=ORIENTED_EDGE('',*,*,#43995,.T.);
#64740=ORIENTED_EDGE('',*,*,#44153,.F.);
#64741=ORIENTED_EDGE('',*,*,#44154,.T.);
#64742=ORIENTED_EDGE('',*,*,#44155,.F.);
#64743=ORIENTED_EDGE('',*,*,#44156,.F.);
#64744=ORIENTED_EDGE('',*,*,#44157,.F.);
#64745=ORIENTED_EDGE('',*,*,#44154,.F.);
#64746=ORIENTED_EDGE('',*,*,#44158,.F.);
#64747=ORIENTED_EDGE('',*,*,#44155,.T.);
#64748=ORIENTED_EDGE('',*,*,#44157,.T.);
#64749=ORIENTED_EDGE('',*,*,#44159,.F.);
#64750=ORIENTED_EDGE('',*,*,#43996,.T.);
#64751=ORIENTED_EDGE('',*,*,#43998,.T.);
#64752=ORIENTED_EDGE('',*,*,#44160,.F.);
#64753=ORIENTED_EDGE('',*,*,#44161,.T.);
#64754=ORIENTED_EDGE('',*,*,#44162,.F.);
#64755=ORIENTED_EDGE('',*,*,#44163,.F.);
#64756=ORIENTED_EDGE('',*,*,#44164,.F.);
#64757=ORIENTED_EDGE('',*,*,#44161,.F.);
#64758=ORIENTED_EDGE('',*,*,#44165,.F.);
#64759=ORIENTED_EDGE('',*,*,#44162,.T.);
#64760=ORIENTED_EDGE('',*,*,#44164,.T.);
#64761=ORIENTED_EDGE('',*,*,#44166,.F.);
#64762=ORIENTED_EDGE('',*,*,#43999,.T.);
#64763=ORIENTED_EDGE('',*,*,#44001,.T.);
#64764=ORIENTED_EDGE('',*,*,#44167,.F.);
#64765=ORIENTED_EDGE('',*,*,#44168,.T.);
#64766=ORIENTED_EDGE('',*,*,#44169,.F.);
#64767=ORIENTED_EDGE('',*,*,#44170,.F.);
#64768=ORIENTED_EDGE('',*,*,#44171,.F.);
#64769=ORIENTED_EDGE('',*,*,#44168,.F.);
#64770=ORIENTED_EDGE('',*,*,#44172,.F.);
#64771=ORIENTED_EDGE('',*,*,#44169,.T.);
#64772=ORIENTED_EDGE('',*,*,#44171,.T.);
#64773=ORIENTED_EDGE('',*,*,#44173,.F.);
#64774=ORIENTED_EDGE('',*,*,#44002,.T.);
#64775=ORIENTED_EDGE('',*,*,#44004,.T.);
#64776=ORIENTED_EDGE('',*,*,#44174,.F.);
#64777=ORIENTED_EDGE('',*,*,#34339,.T.);
#64778=ORIENTED_EDGE('',*,*,#44175,.F.);
#64779=ORIENTED_EDGE('',*,*,#44175,.T.);
#64780=ORIENTED_EDGE('',*,*,#34338,.T.);
#64781=ORIENTED_EDGE('',*,*,#44176,.F.);
#64782=ORIENTED_EDGE('',*,*,#44005,.T.);
#64783=ORIENTED_EDGE('',*,*,#44007,.T.);
#64784=ORIENTED_EDGE('',*,*,#44177,.F.);
#64785=ORIENTED_EDGE('',*,*,#44178,.T.);
#64786=ORIENTED_EDGE('',*,*,#44179,.F.);
#64787=ORIENTED_EDGE('',*,*,#44180,.F.);
#64788=ORIENTED_EDGE('',*,*,#44181,.F.);
#64789=ORIENTED_EDGE('',*,*,#44178,.F.);
#64790=ORIENTED_EDGE('',*,*,#44182,.F.);
#64791=ORIENTED_EDGE('',*,*,#44179,.T.);
#64792=ORIENTED_EDGE('',*,*,#44181,.T.);
#64793=ORIENTED_EDGE('',*,*,#44183,.F.);
#64794=ORIENTED_EDGE('',*,*,#44008,.T.);
#64795=ORIENTED_EDGE('',*,*,#44010,.T.);
#64796=ORIENTED_EDGE('',*,*,#44184,.F.);
#64797=ORIENTED_EDGE('',*,*,#44185,.T.);
#64798=ORIENTED_EDGE('',*,*,#44186,.F.);
#64799=ORIENTED_EDGE('',*,*,#44187,.F.);
#64800=ORIENTED_EDGE('',*,*,#44188,.F.);
#64801=ORIENTED_EDGE('',*,*,#44185,.F.);
#64802=ORIENTED_EDGE('',*,*,#44189,.F.);
#64803=ORIENTED_EDGE('',*,*,#44186,.T.);
#64804=ORIENTED_EDGE('',*,*,#44188,.T.);
#64805=ORIENTED_EDGE('',*,*,#44190,.F.);
#64806=ORIENTED_EDGE('',*,*,#44011,.T.);
#64807=ORIENTED_EDGE('',*,*,#44013,.T.);
#64808=ORIENTED_EDGE('',*,*,#44191,.F.);
#64809=ORIENTED_EDGE('',*,*,#44192,.T.);
#64810=ORIENTED_EDGE('',*,*,#44193,.F.);
#64811=ORIENTED_EDGE('',*,*,#44194,.F.);
#64812=ORIENTED_EDGE('',*,*,#44195,.F.);
#64813=ORIENTED_EDGE('',*,*,#44192,.F.);
#64814=ORIENTED_EDGE('',*,*,#44196,.F.);
#64815=ORIENTED_EDGE('',*,*,#44193,.T.);
#64816=ORIENTED_EDGE('',*,*,#44195,.T.);
#64817=ORIENTED_EDGE('',*,*,#44197,.F.);
#64818=ORIENTED_EDGE('',*,*,#44014,.T.);
#64819=ORIENTED_EDGE('',*,*,#44016,.T.);
#64820=ORIENTED_EDGE('',*,*,#44198,.F.);
#64821=ORIENTED_EDGE('',*,*,#44199,.T.);
#64822=ORIENTED_EDGE('',*,*,#44200,.F.);
#64823=ORIENTED_EDGE('',*,*,#44201,.F.);
#64824=ORIENTED_EDGE('',*,*,#44202,.F.);
#64825=ORIENTED_EDGE('',*,*,#44199,.F.);
#64826=ORIENTED_EDGE('',*,*,#44203,.F.);
#64827=ORIENTED_EDGE('',*,*,#44200,.T.);
#64828=ORIENTED_EDGE('',*,*,#44202,.T.);
#64829=ORIENTED_EDGE('',*,*,#44204,.F.);
#64830=ORIENTED_EDGE('',*,*,#44017,.T.);
#64831=ORIENTED_EDGE('',*,*,#44019,.T.);
#64832=ORIENTED_EDGE('',*,*,#44205,.F.);
#64833=ORIENTED_EDGE('',*,*,#44206,.T.);
#64834=ORIENTED_EDGE('',*,*,#44207,.F.);
#64835=ORIENTED_EDGE('',*,*,#44208,.F.);
#64836=ORIENTED_EDGE('',*,*,#44209,.F.);
#64837=ORIENTED_EDGE('',*,*,#44206,.F.);
#64838=ORIENTED_EDGE('',*,*,#44210,.F.);
#64839=ORIENTED_EDGE('',*,*,#44207,.T.);
#64840=ORIENTED_EDGE('',*,*,#44209,.T.);
#64841=ORIENTED_EDGE('',*,*,#44211,.F.);
#64842=ORIENTED_EDGE('',*,*,#44020,.T.);
#64843=ORIENTED_EDGE('',*,*,#44022,.T.);
#64844=ORIENTED_EDGE('',*,*,#44212,.F.);
#64845=ORIENTED_EDGE('',*,*,#44213,.T.);
#64846=ORIENTED_EDGE('',*,*,#44214,.F.);
#64847=ORIENTED_EDGE('',*,*,#44215,.F.);
#64848=ORIENTED_EDGE('',*,*,#44216,.F.);
#64849=ORIENTED_EDGE('',*,*,#44213,.F.);
#64850=ORIENTED_EDGE('',*,*,#44217,.F.);
#64851=ORIENTED_EDGE('',*,*,#44214,.T.);
#64852=ORIENTED_EDGE('',*,*,#44216,.T.);
#64853=ORIENTED_EDGE('',*,*,#44218,.F.);
#64854=ORIENTED_EDGE('',*,*,#44023,.T.);
#64855=ORIENTED_EDGE('',*,*,#44025,.T.);
#64856=ORIENTED_EDGE('',*,*,#44219,.F.);
#64857=ORIENTED_EDGE('',*,*,#34335,.T.);
#64858=ORIENTED_EDGE('',*,*,#44220,.F.);
#64859=ORIENTED_EDGE('',*,*,#44220,.T.);
#64860=ORIENTED_EDGE('',*,*,#34334,.T.);
#64861=ORIENTED_EDGE('',*,*,#44221,.F.);
#64862=ORIENTED_EDGE('',*,*,#44026,.T.);
#64863=ORIENTED_EDGE('',*,*,#44222,.F.);
#64864=ORIENTED_EDGE('',*,*,#44223,.F.);
#64865=ORIENTED_EDGE('',*,*,#44032,.T.);
#64866=ORIENTED_EDGE('',*,*,#44027,.T.);
#64867=ORIENTED_EDGE('',*,*,#44224,.F.);
#64868=ORIENTED_EDGE('',*,*,#44033,.T.);
#64869=ORIENTED_EDGE('',*,*,#44030,.T.);
#64870=ORIENTED_EDGE('',*,*,#44223,.T.);
#64871=ORIENTED_EDGE('',*,*,#44225,.F.);
#64872=ORIENTED_EDGE('',*,*,#44226,.F.);
#64873=ORIENTED_EDGE('',*,*,#44039,.T.);
#64874=ORIENTED_EDGE('',*,*,#44034,.T.);
#64875=ORIENTED_EDGE('',*,*,#44227,.F.);
#64876=ORIENTED_EDGE('',*,*,#44040,.T.);
#64877=ORIENTED_EDGE('',*,*,#44037,.T.);
#64878=ORIENTED_EDGE('',*,*,#44226,.T.);
#64879=ORIENTED_EDGE('',*,*,#44228,.F.);
#64880=ORIENTED_EDGE('',*,*,#44229,.F.);
#64881=ORIENTED_EDGE('',*,*,#44046,.T.);
#64882=ORIENTED_EDGE('',*,*,#44041,.T.);
#64883=ORIENTED_EDGE('',*,*,#44230,.F.);
#64884=ORIENTED_EDGE('',*,*,#44047,.T.);
#64885=ORIENTED_EDGE('',*,*,#44044,.T.);
#64886=ORIENTED_EDGE('',*,*,#44229,.T.);
#64887=ORIENTED_EDGE('',*,*,#44231,.F.);
#64888=ORIENTED_EDGE('',*,*,#44232,.F.);
#64889=ORIENTED_EDGE('',*,*,#44053,.T.);
#64890=ORIENTED_EDGE('',*,*,#44048,.T.);
#64891=ORIENTED_EDGE('',*,*,#44233,.F.);
#64892=ORIENTED_EDGE('',*,*,#44054,.T.);
#64893=ORIENTED_EDGE('',*,*,#44051,.T.);
#64894=ORIENTED_EDGE('',*,*,#44232,.T.);
#64895=ORIENTED_EDGE('',*,*,#44234,.F.);
#64896=ORIENTED_EDGE('',*,*,#44235,.F.);
#64897=ORIENTED_EDGE('',*,*,#44060,.T.);
#64898=ORIENTED_EDGE('',*,*,#44055,.T.);
#64899=ORIENTED_EDGE('',*,*,#44236,.F.);
#64900=ORIENTED_EDGE('',*,*,#44061,.T.);
#64901=ORIENTED_EDGE('',*,*,#44058,.T.);
#64902=ORIENTED_EDGE('',*,*,#44235,.T.);
#64903=ORIENTED_EDGE('',*,*,#44237,.F.);
#64904=ORIENTED_EDGE('',*,*,#44238,.F.);
#64905=ORIENTED_EDGE('',*,*,#44067,.T.);
#64906=ORIENTED_EDGE('',*,*,#44062,.T.);
#64907=ORIENTED_EDGE('',*,*,#44239,.F.);
#64908=ORIENTED_EDGE('',*,*,#44068,.T.);
#64909=ORIENTED_EDGE('',*,*,#44065,.T.);
#64910=ORIENTED_EDGE('',*,*,#44238,.T.);
#64911=ORIENTED_EDGE('',*,*,#44240,.F.);
#64912=ORIENTED_EDGE('',*,*,#44241,.F.);
#64913=ORIENTED_EDGE('',*,*,#44074,.T.);
#64914=ORIENTED_EDGE('',*,*,#44069,.T.);
#64915=ORIENTED_EDGE('',*,*,#44242,.F.);
#64916=ORIENTED_EDGE('',*,*,#44075,.T.);
#64917=ORIENTED_EDGE('',*,*,#44072,.T.);
#64918=ORIENTED_EDGE('',*,*,#44241,.T.);
#64919=ORIENTED_EDGE('',*,*,#44243,.F.);
#64920=ORIENTED_EDGE('',*,*,#44244,.F.);
#64921=ORIENTED_EDGE('',*,*,#44081,.T.);
#64922=ORIENTED_EDGE('',*,*,#44076,.T.);
#64923=ORIENTED_EDGE('',*,*,#44245,.F.);
#64924=ORIENTED_EDGE('',*,*,#44082,.T.);
#64925=ORIENTED_EDGE('',*,*,#44079,.T.);
#64926=ORIENTED_EDGE('',*,*,#44244,.T.);
#64927=ORIENTED_EDGE('',*,*,#44246,.F.);
#64928=ORIENTED_EDGE('',*,*,#44247,.F.);
#64929=ORIENTED_EDGE('',*,*,#44088,.T.);
#64930=ORIENTED_EDGE('',*,*,#44083,.T.);
#64931=ORIENTED_EDGE('',*,*,#44248,.F.);
#64932=ORIENTED_EDGE('',*,*,#44089,.T.);
#64933=ORIENTED_EDGE('',*,*,#44086,.T.);
#64934=ORIENTED_EDGE('',*,*,#44247,.T.);
#64935=ORIENTED_EDGE('',*,*,#44249,.F.);
#64936=ORIENTED_EDGE('',*,*,#44250,.F.);
#64937=ORIENTED_EDGE('',*,*,#44095,.T.);
#64938=ORIENTED_EDGE('',*,*,#44090,.T.);
#64939=ORIENTED_EDGE('',*,*,#44251,.F.);
#64940=ORIENTED_EDGE('',*,*,#44096,.T.);
#64941=ORIENTED_EDGE('',*,*,#44093,.T.);
#64942=ORIENTED_EDGE('',*,*,#44250,.T.);
#64943=ORIENTED_EDGE('',*,*,#44252,.F.);
#64944=ORIENTED_EDGE('',*,*,#44253,.F.);
#64945=ORIENTED_EDGE('',*,*,#44102,.T.);
#64946=ORIENTED_EDGE('',*,*,#44097,.T.);
#64947=ORIENTED_EDGE('',*,*,#44254,.F.);
#64948=ORIENTED_EDGE('',*,*,#44103,.T.);
#64949=ORIENTED_EDGE('',*,*,#44100,.T.);
#64950=ORIENTED_EDGE('',*,*,#44253,.T.);
#64951=ORIENTED_EDGE('',*,*,#44255,.F.);
#64952=ORIENTED_EDGE('',*,*,#44256,.F.);
#64953=ORIENTED_EDGE('',*,*,#44109,.T.);
#64954=ORIENTED_EDGE('',*,*,#44104,.T.);
#64955=ORIENTED_EDGE('',*,*,#44257,.F.);
#64956=ORIENTED_EDGE('',*,*,#44110,.T.);
#64957=ORIENTED_EDGE('',*,*,#44107,.T.);
#64958=ORIENTED_EDGE('',*,*,#44256,.T.);
#64959=ORIENTED_EDGE('',*,*,#44258,.F.);
#64960=ORIENTED_EDGE('',*,*,#44259,.F.);
#64961=ORIENTED_EDGE('',*,*,#44116,.T.);
#64962=ORIENTED_EDGE('',*,*,#44111,.T.);
#64963=ORIENTED_EDGE('',*,*,#44260,.F.);
#64964=ORIENTED_EDGE('',*,*,#44117,.T.);
#64965=ORIENTED_EDGE('',*,*,#44114,.T.);
#64966=ORIENTED_EDGE('',*,*,#44259,.T.);
#64967=ORIENTED_EDGE('',*,*,#44261,.F.);
#64968=ORIENTED_EDGE('',*,*,#44262,.F.);
#64969=ORIENTED_EDGE('',*,*,#44123,.T.);
#64970=ORIENTED_EDGE('',*,*,#44118,.T.);
#64971=ORIENTED_EDGE('',*,*,#44263,.F.);
#64972=ORIENTED_EDGE('',*,*,#44124,.T.);
#64973=ORIENTED_EDGE('',*,*,#44121,.T.);
#64974=ORIENTED_EDGE('',*,*,#44262,.T.);
#64975=ORIENTED_EDGE('',*,*,#44264,.F.);
#64976=ORIENTED_EDGE('',*,*,#44265,.F.);
#64977=ORIENTED_EDGE('',*,*,#44130,.T.);
#64978=ORIENTED_EDGE('',*,*,#44125,.T.);
#64979=ORIENTED_EDGE('',*,*,#44266,.F.);
#64980=ORIENTED_EDGE('',*,*,#44131,.T.);
#64981=ORIENTED_EDGE('',*,*,#44128,.T.);
#64982=ORIENTED_EDGE('',*,*,#44265,.T.);
#64983=ORIENTED_EDGE('',*,*,#44267,.F.);
#64984=ORIENTED_EDGE('',*,*,#44268,.F.);
#64985=ORIENTED_EDGE('',*,*,#44137,.T.);
#64986=ORIENTED_EDGE('',*,*,#44132,.T.);
#64987=ORIENTED_EDGE('',*,*,#44269,.F.);
#64988=ORIENTED_EDGE('',*,*,#44138,.T.);
#64989=ORIENTED_EDGE('',*,*,#44135,.T.);
#64990=ORIENTED_EDGE('',*,*,#44268,.T.);
#64991=ORIENTED_EDGE('',*,*,#44270,.F.);
#64992=ORIENTED_EDGE('',*,*,#44271,.F.);
#64993=ORIENTED_EDGE('',*,*,#44144,.T.);
#64994=ORIENTED_EDGE('',*,*,#44139,.T.);
#64995=ORIENTED_EDGE('',*,*,#44272,.F.);
#64996=ORIENTED_EDGE('',*,*,#44145,.T.);
#64997=ORIENTED_EDGE('',*,*,#44142,.T.);
#64998=ORIENTED_EDGE('',*,*,#44271,.T.);
#64999=ORIENTED_EDGE('',*,*,#44273,.F.);
#65000=ORIENTED_EDGE('',*,*,#44274,.F.);
#65001=ORIENTED_EDGE('',*,*,#44149,.T.);
#65002=ORIENTED_EDGE('',*,*,#44146,.T.);
#65003=ORIENTED_EDGE('',*,*,#44275,.F.);
#65004=ORIENTED_EDGE('',*,*,#44152,.T.);
#65005=ORIENTED_EDGE('',*,*,#44150,.T.);
#65006=ORIENTED_EDGE('',*,*,#44274,.T.);
#65007=ORIENTED_EDGE('',*,*,#44276,.F.);
#65008=ORIENTED_EDGE('',*,*,#44277,.F.);
#65009=ORIENTED_EDGE('',*,*,#44158,.T.);
#65010=ORIENTED_EDGE('',*,*,#44153,.T.);
#65011=ORIENTED_EDGE('',*,*,#44278,.F.);
#65012=ORIENTED_EDGE('',*,*,#44159,.T.);
#65013=ORIENTED_EDGE('',*,*,#44156,.T.);
#65014=ORIENTED_EDGE('',*,*,#44277,.T.);
#65015=ORIENTED_EDGE('',*,*,#44279,.F.);
#65016=ORIENTED_EDGE('',*,*,#44280,.F.);
#65017=ORIENTED_EDGE('',*,*,#44165,.T.);
#65018=ORIENTED_EDGE('',*,*,#44160,.T.);
#65019=ORIENTED_EDGE('',*,*,#44281,.F.);
#65020=ORIENTED_EDGE('',*,*,#44166,.T.);
#65021=ORIENTED_EDGE('',*,*,#44163,.T.);
#65022=ORIENTED_EDGE('',*,*,#44280,.T.);
#65023=ORIENTED_EDGE('',*,*,#44282,.F.);
#65024=ORIENTED_EDGE('',*,*,#44283,.F.);
#65025=ORIENTED_EDGE('',*,*,#44172,.T.);
#65026=ORIENTED_EDGE('',*,*,#44167,.T.);
#65027=ORIENTED_EDGE('',*,*,#44284,.F.);
#65028=ORIENTED_EDGE('',*,*,#44173,.T.);
#65029=ORIENTED_EDGE('',*,*,#44170,.T.);
#65030=ORIENTED_EDGE('',*,*,#44283,.T.);
#65031=ORIENTED_EDGE('',*,*,#44285,.F.);
#65032=ORIENTED_EDGE('',*,*,#44286,.F.);
#65033=ORIENTED_EDGE('',*,*,#34340,.T.);
#65034=ORIENTED_EDGE('',*,*,#44174,.T.);
#65035=ORIENTED_EDGE('',*,*,#44287,.F.);
#65036=ORIENTED_EDGE('',*,*,#44176,.T.);
#65037=ORIENTED_EDGE('',*,*,#34337,.T.);
#65038=ORIENTED_EDGE('',*,*,#44286,.T.);
#65039=ORIENTED_EDGE('',*,*,#44288,.F.);
#65040=ORIENTED_EDGE('',*,*,#44289,.F.);
#65041=ORIENTED_EDGE('',*,*,#44182,.T.);
#65042=ORIENTED_EDGE('',*,*,#44177,.T.);
#65043=ORIENTED_EDGE('',*,*,#44290,.F.);
#65044=ORIENTED_EDGE('',*,*,#44183,.T.);
#65045=ORIENTED_EDGE('',*,*,#44180,.T.);
#65046=ORIENTED_EDGE('',*,*,#44289,.T.);
#65047=ORIENTED_EDGE('',*,*,#44291,.F.);
#65048=ORIENTED_EDGE('',*,*,#44292,.F.);
#65049=ORIENTED_EDGE('',*,*,#44189,.T.);
#65050=ORIENTED_EDGE('',*,*,#44184,.T.);
#65051=ORIENTED_EDGE('',*,*,#44293,.F.);
#65052=ORIENTED_EDGE('',*,*,#44190,.T.);
#65053=ORIENTED_EDGE('',*,*,#44187,.T.);
#65054=ORIENTED_EDGE('',*,*,#44292,.T.);
#65055=ORIENTED_EDGE('',*,*,#44294,.F.);
#65056=ORIENTED_EDGE('',*,*,#44295,.F.);
#65057=ORIENTED_EDGE('',*,*,#44196,.T.);
#65058=ORIENTED_EDGE('',*,*,#44191,.T.);
#65059=ORIENTED_EDGE('',*,*,#44296,.F.);
#65060=ORIENTED_EDGE('',*,*,#44197,.T.);
#65061=ORIENTED_EDGE('',*,*,#44194,.T.);
#65062=ORIENTED_EDGE('',*,*,#44295,.T.);
#65063=ORIENTED_EDGE('',*,*,#44297,.F.);
#65064=ORIENTED_EDGE('',*,*,#44298,.F.);
#65065=ORIENTED_EDGE('',*,*,#44203,.T.);
#65066=ORIENTED_EDGE('',*,*,#44198,.T.);
#65067=ORIENTED_EDGE('',*,*,#44299,.F.);
#65068=ORIENTED_EDGE('',*,*,#44204,.T.);
#65069=ORIENTED_EDGE('',*,*,#44201,.T.);
#65070=ORIENTED_EDGE('',*,*,#44298,.T.);
#65071=ORIENTED_EDGE('',*,*,#44300,.F.);
#65072=ORIENTED_EDGE('',*,*,#44301,.F.);
#65073=ORIENTED_EDGE('',*,*,#44210,.T.);
#65074=ORIENTED_EDGE('',*,*,#44205,.T.);
#65075=ORIENTED_EDGE('',*,*,#44302,.F.);
#65076=ORIENTED_EDGE('',*,*,#44211,.T.);
#65077=ORIENTED_EDGE('',*,*,#44208,.T.);
#65078=ORIENTED_EDGE('',*,*,#44301,.T.);
#65079=ORIENTED_EDGE('',*,*,#44303,.F.);
#65080=ORIENTED_EDGE('',*,*,#44304,.F.);
#65081=ORIENTED_EDGE('',*,*,#44217,.T.);
#65082=ORIENTED_EDGE('',*,*,#44212,.T.);
#65083=ORIENTED_EDGE('',*,*,#44305,.F.);
#65084=ORIENTED_EDGE('',*,*,#44218,.T.);
#65085=ORIENTED_EDGE('',*,*,#44215,.T.);
#65086=ORIENTED_EDGE('',*,*,#44304,.T.);
#65087=ORIENTED_EDGE('',*,*,#44306,.F.);
#65088=ORIENTED_EDGE('',*,*,#44307,.F.);
#65089=ORIENTED_EDGE('',*,*,#34336,.T.);
#65090=ORIENTED_EDGE('',*,*,#44219,.T.);
#65091=ORIENTED_EDGE('',*,*,#44221,.T.);
#65092=ORIENTED_EDGE('',*,*,#34333,.T.);
#65093=ORIENTED_EDGE('',*,*,#44307,.T.);
#65094=ORIENTED_EDGE('',*,*,#44308,.F.);
#65095=ORIENTED_EDGE('',*,*,#34147,.F.);
#65096=ORIENTED_EDGE('',*,*,#34152,.T.);
#65097=ORIENTED_EDGE('',*,*,#44222,.T.);
#65098=ORIENTED_EDGE('',*,*,#44309,.F.);
#65099=ORIENTED_EDGE('',*,*,#34049,.T.);
#65100=ORIENTED_EDGE('',*,*,#44310,.F.);
#65101=ORIENTED_EDGE('',*,*,#44311,.F.);
#65102=ORIENTED_EDGE('',*,*,#44310,.T.);
#65103=ORIENTED_EDGE('',*,*,#34048,.T.);
#65104=ORIENTED_EDGE('',*,*,#44312,.F.);
#65105=ORIENTED_EDGE('',*,*,#44311,.T.);
#65106=ORIENTED_EDGE('',*,*,#34047,.T.);
#65107=ORIENTED_EDGE('',*,*,#44313,.F.);
#65108=ORIENTED_EDGE('',*,*,#44312,.T.);
#65109=ORIENTED_EDGE('',*,*,#34046,.T.);
#65110=ORIENTED_EDGE('',*,*,#44314,.F.);
#65111=ORIENTED_EDGE('',*,*,#44313,.T.);
#65112=ORIENTED_EDGE('',*,*,#34045,.T.);
#65113=ORIENTED_EDGE('',*,*,#44224,.T.);
#65114=ORIENTED_EDGE('',*,*,#44314,.T.);
#65115=ORIENTED_EDGE('',*,*,#34044,.T.);
#65116=ORIENTED_EDGE('',*,*,#44315,.F.);
#65117=ORIENTED_EDGE('',*,*,#44225,.T.);
#65118=ORIENTED_EDGE('',*,*,#44315,.T.);
#65119=ORIENTED_EDGE('',*,*,#34043,.T.);
#65120=ORIENTED_EDGE('',*,*,#44316,.F.);
#65121=ORIENTED_EDGE('',*,*,#44317,.F.);
#65122=ORIENTED_EDGE('',*,*,#44316,.T.);
#65123=ORIENTED_EDGE('',*,*,#34042,.T.);
#65124=ORIENTED_EDGE('',*,*,#44318,.F.);
#65125=ORIENTED_EDGE('',*,*,#44317,.T.);
#65126=ORIENTED_EDGE('',*,*,#34041,.T.);
#65127=ORIENTED_EDGE('',*,*,#44319,.F.);
#65128=ORIENTED_EDGE('',*,*,#44318,.T.);
#65129=ORIENTED_EDGE('',*,*,#34040,.T.);
#65130=ORIENTED_EDGE('',*,*,#44320,.F.);
#65131=ORIENTED_EDGE('',*,*,#44319,.T.);
#65132=ORIENTED_EDGE('',*,*,#34039,.T.);
#65133=ORIENTED_EDGE('',*,*,#44227,.T.);
#65134=ORIENTED_EDGE('',*,*,#44320,.T.);
#65135=ORIENTED_EDGE('',*,*,#34038,.T.);
#65136=ORIENTED_EDGE('',*,*,#44321,.F.);
#65137=ORIENTED_EDGE('',*,*,#44228,.T.);
#65138=ORIENTED_EDGE('',*,*,#44321,.T.);
#65139=ORIENTED_EDGE('',*,*,#34037,.T.);
#65140=ORIENTED_EDGE('',*,*,#44322,.F.);
#65141=ORIENTED_EDGE('',*,*,#44323,.F.);
#65142=ORIENTED_EDGE('',*,*,#44322,.T.);
#65143=ORIENTED_EDGE('',*,*,#34036,.T.);
#65144=ORIENTED_EDGE('',*,*,#44324,.F.);
#65145=ORIENTED_EDGE('',*,*,#44323,.T.);
#65146=ORIENTED_EDGE('',*,*,#34035,.T.);
#65147=ORIENTED_EDGE('',*,*,#44325,.F.);
#65148=ORIENTED_EDGE('',*,*,#44324,.T.);
#65149=ORIENTED_EDGE('',*,*,#34034,.T.);
#65150=ORIENTED_EDGE('',*,*,#44326,.F.);
#65151=ORIENTED_EDGE('',*,*,#44325,.T.);
#65152=ORIENTED_EDGE('',*,*,#34033,.T.);
#65153=ORIENTED_EDGE('',*,*,#44230,.T.);
#65154=ORIENTED_EDGE('',*,*,#44326,.T.);
#65155=ORIENTED_EDGE('',*,*,#34032,.T.);
#65156=ORIENTED_EDGE('',*,*,#44327,.F.);
#65157=ORIENTED_EDGE('',*,*,#44231,.T.);
#65158=ORIENTED_EDGE('',*,*,#44327,.T.);
#65159=ORIENTED_EDGE('',*,*,#34031,.T.);
#65160=ORIENTED_EDGE('',*,*,#44328,.F.);
#65161=ORIENTED_EDGE('',*,*,#44329,.F.);
#65162=ORIENTED_EDGE('',*,*,#44328,.T.);
#65163=ORIENTED_EDGE('',*,*,#34030,.T.);
#65164=ORIENTED_EDGE('',*,*,#44330,.F.);
#65165=ORIENTED_EDGE('',*,*,#44329,.T.);
#65166=ORIENTED_EDGE('',*,*,#34029,.T.);
#65167=ORIENTED_EDGE('',*,*,#44331,.F.);
#65168=ORIENTED_EDGE('',*,*,#44330,.T.);
#65169=ORIENTED_EDGE('',*,*,#34028,.T.);
#65170=ORIENTED_EDGE('',*,*,#44332,.F.);
#65171=ORIENTED_EDGE('',*,*,#44331,.T.);
#65172=ORIENTED_EDGE('',*,*,#34027,.T.);
#65173=ORIENTED_EDGE('',*,*,#44233,.T.);
#65174=ORIENTED_EDGE('',*,*,#44332,.T.);
#65175=ORIENTED_EDGE('',*,*,#34026,.T.);
#65176=ORIENTED_EDGE('',*,*,#44333,.F.);
#65177=ORIENTED_EDGE('',*,*,#44234,.T.);
#65178=ORIENTED_EDGE('',*,*,#44333,.T.);
#65179=ORIENTED_EDGE('',*,*,#34025,.T.);
#65180=ORIENTED_EDGE('',*,*,#44334,.F.);
#65181=ORIENTED_EDGE('',*,*,#44335,.F.);
#65182=ORIENTED_EDGE('',*,*,#44334,.T.);
#65183=ORIENTED_EDGE('',*,*,#34024,.T.);
#65184=ORIENTED_EDGE('',*,*,#44336,.F.);
#65185=ORIENTED_EDGE('',*,*,#44335,.T.);
#65186=ORIENTED_EDGE('',*,*,#34023,.T.);
#65187=ORIENTED_EDGE('',*,*,#44337,.F.);
#65188=ORIENTED_EDGE('',*,*,#44336,.T.);
#65189=ORIENTED_EDGE('',*,*,#34022,.T.);
#65190=ORIENTED_EDGE('',*,*,#44338,.F.);
#65191=ORIENTED_EDGE('',*,*,#44337,.T.);
#65192=ORIENTED_EDGE('',*,*,#34021,.T.);
#65193=ORIENTED_EDGE('',*,*,#44236,.T.);
#65194=ORIENTED_EDGE('',*,*,#44338,.T.);
#65195=ORIENTED_EDGE('',*,*,#34020,.T.);
#65196=ORIENTED_EDGE('',*,*,#44339,.F.);
#65197=ORIENTED_EDGE('',*,*,#44237,.T.);
#65198=ORIENTED_EDGE('',*,*,#44339,.T.);
#65199=ORIENTED_EDGE('',*,*,#34019,.T.);
#65200=ORIENTED_EDGE('',*,*,#44340,.F.);
#65201=ORIENTED_EDGE('',*,*,#44341,.F.);
#65202=ORIENTED_EDGE('',*,*,#44340,.T.);
#65203=ORIENTED_EDGE('',*,*,#34018,.T.);
#65204=ORIENTED_EDGE('',*,*,#44342,.F.);
#65205=ORIENTED_EDGE('',*,*,#44341,.T.);
#65206=ORIENTED_EDGE('',*,*,#34017,.T.);
#65207=ORIENTED_EDGE('',*,*,#44343,.F.);
#65208=ORIENTED_EDGE('',*,*,#44342,.T.);
#65209=ORIENTED_EDGE('',*,*,#34016,.T.);
#65210=ORIENTED_EDGE('',*,*,#44344,.F.);
#65211=ORIENTED_EDGE('',*,*,#44343,.T.);
#65212=ORIENTED_EDGE('',*,*,#34015,.T.);
#65213=ORIENTED_EDGE('',*,*,#44239,.T.);
#65214=ORIENTED_EDGE('',*,*,#44344,.T.);
#65215=ORIENTED_EDGE('',*,*,#34014,.T.);
#65216=ORIENTED_EDGE('',*,*,#44345,.F.);
#65217=ORIENTED_EDGE('',*,*,#44240,.T.);
#65218=ORIENTED_EDGE('',*,*,#44345,.T.);
#65219=ORIENTED_EDGE('',*,*,#34013,.T.);
#65220=ORIENTED_EDGE('',*,*,#44346,.F.);
#65221=ORIENTED_EDGE('',*,*,#44347,.F.);
#65222=ORIENTED_EDGE('',*,*,#44346,.T.);
#65223=ORIENTED_EDGE('',*,*,#34012,.T.);
#65224=ORIENTED_EDGE('',*,*,#44348,.F.);
#65225=ORIENTED_EDGE('',*,*,#44347,.T.);
#65226=ORIENTED_EDGE('',*,*,#34011,.T.);
#65227=ORIENTED_EDGE('',*,*,#44349,.F.);
#65228=ORIENTED_EDGE('',*,*,#44348,.T.);
#65229=ORIENTED_EDGE('',*,*,#34010,.T.);
#65230=ORIENTED_EDGE('',*,*,#44350,.F.);
#65231=ORIENTED_EDGE('',*,*,#44349,.T.);
#65232=ORIENTED_EDGE('',*,*,#34009,.T.);
#65233=ORIENTED_EDGE('',*,*,#44242,.T.);
#65234=ORIENTED_EDGE('',*,*,#44350,.T.);
#65235=ORIENTED_EDGE('',*,*,#34008,.T.);
#65236=ORIENTED_EDGE('',*,*,#44351,.F.);
#65237=ORIENTED_EDGE('',*,*,#44243,.T.);
#65238=ORIENTED_EDGE('',*,*,#44351,.T.);
#65239=ORIENTED_EDGE('',*,*,#34007,.T.);
#65240=ORIENTED_EDGE('',*,*,#44352,.F.);
#65241=ORIENTED_EDGE('',*,*,#44353,.F.);
#65242=ORIENTED_EDGE('',*,*,#44352,.T.);
#65243=ORIENTED_EDGE('',*,*,#34006,.T.);
#65244=ORIENTED_EDGE('',*,*,#44354,.F.);
#65245=ORIENTED_EDGE('',*,*,#44353,.T.);
#65246=ORIENTED_EDGE('',*,*,#34005,.T.);
#65247=ORIENTED_EDGE('',*,*,#44355,.F.);
#65248=ORIENTED_EDGE('',*,*,#44354,.T.);
#65249=ORIENTED_EDGE('',*,*,#34004,.T.);
#65250=ORIENTED_EDGE('',*,*,#44356,.F.);
#65251=ORIENTED_EDGE('',*,*,#44355,.T.);
#65252=ORIENTED_EDGE('',*,*,#34003,.T.);
#65253=ORIENTED_EDGE('',*,*,#44245,.T.);
#65254=ORIENTED_EDGE('',*,*,#44356,.T.);
#65255=ORIENTED_EDGE('',*,*,#34002,.T.);
#65256=ORIENTED_EDGE('',*,*,#44357,.F.);
#65257=ORIENTED_EDGE('',*,*,#44246,.T.);
#65258=ORIENTED_EDGE('',*,*,#44357,.T.);
#65259=ORIENTED_EDGE('',*,*,#34001,.T.);
#65260=ORIENTED_EDGE('',*,*,#44358,.F.);
#65261=ORIENTED_EDGE('',*,*,#44359,.F.);
#65262=ORIENTED_EDGE('',*,*,#44358,.T.);
#65263=ORIENTED_EDGE('',*,*,#34000,.T.);
#65264=ORIENTED_EDGE('',*,*,#44360,.F.);
#65265=ORIENTED_EDGE('',*,*,#44359,.T.);
#65266=ORIENTED_EDGE('',*,*,#33999,.T.);
#65267=ORIENTED_EDGE('',*,*,#44361,.F.);
#65268=ORIENTED_EDGE('',*,*,#44360,.T.);
#65269=ORIENTED_EDGE('',*,*,#33998,.T.);
#65270=ORIENTED_EDGE('',*,*,#44362,.F.);
#65271=ORIENTED_EDGE('',*,*,#44361,.T.);
#65272=ORIENTED_EDGE('',*,*,#33997,.T.);
#65273=ORIENTED_EDGE('',*,*,#44248,.T.);
#65274=ORIENTED_EDGE('',*,*,#44362,.T.);
#65275=ORIENTED_EDGE('',*,*,#33996,.T.);
#65276=ORIENTED_EDGE('',*,*,#44363,.F.);
#65277=ORIENTED_EDGE('',*,*,#44249,.T.);
#65278=ORIENTED_EDGE('',*,*,#44363,.T.);
#65279=ORIENTED_EDGE('',*,*,#33995,.T.);
#65280=ORIENTED_EDGE('',*,*,#44364,.F.);
#65281=ORIENTED_EDGE('',*,*,#44365,.F.);
#65282=ORIENTED_EDGE('',*,*,#44364,.T.);
#65283=ORIENTED_EDGE('',*,*,#33994,.T.);
#65284=ORIENTED_EDGE('',*,*,#44366,.F.);
#65285=ORIENTED_EDGE('',*,*,#44365,.T.);
#65286=ORIENTED_EDGE('',*,*,#33993,.T.);
#65287=ORIENTED_EDGE('',*,*,#44367,.F.);
#65288=ORIENTED_EDGE('',*,*,#44366,.T.);
#65289=ORIENTED_EDGE('',*,*,#33992,.T.);
#65290=ORIENTED_EDGE('',*,*,#44368,.F.);
#65291=ORIENTED_EDGE('',*,*,#44367,.T.);
#65292=ORIENTED_EDGE('',*,*,#33991,.T.);
#65293=ORIENTED_EDGE('',*,*,#44251,.T.);
#65294=ORIENTED_EDGE('',*,*,#44368,.T.);
#65295=ORIENTED_EDGE('',*,*,#33990,.T.);
#65296=ORIENTED_EDGE('',*,*,#44369,.F.);
#65297=ORIENTED_EDGE('',*,*,#44252,.T.);
#65298=ORIENTED_EDGE('',*,*,#44369,.T.);
#65299=ORIENTED_EDGE('',*,*,#33989,.T.);
#65300=ORIENTED_EDGE('',*,*,#44370,.F.);
#65301=ORIENTED_EDGE('',*,*,#44371,.F.);
#65302=ORIENTED_EDGE('',*,*,#44370,.T.);
#65303=ORIENTED_EDGE('',*,*,#33988,.T.);
#65304=ORIENTED_EDGE('',*,*,#44372,.F.);
#65305=ORIENTED_EDGE('',*,*,#44371,.T.);
#65306=ORIENTED_EDGE('',*,*,#33987,.T.);
#65307=ORIENTED_EDGE('',*,*,#44373,.F.);
#65308=ORIENTED_EDGE('',*,*,#44372,.T.);
#65309=ORIENTED_EDGE('',*,*,#33986,.T.);
#65310=ORIENTED_EDGE('',*,*,#44374,.F.);
#65311=ORIENTED_EDGE('',*,*,#44373,.T.);
#65312=ORIENTED_EDGE('',*,*,#33985,.T.);
#65313=ORIENTED_EDGE('',*,*,#44254,.T.);
#65314=ORIENTED_EDGE('',*,*,#44374,.T.);
#65315=ORIENTED_EDGE('',*,*,#33984,.T.);
#65316=ORIENTED_EDGE('',*,*,#44375,.F.);
#65317=ORIENTED_EDGE('',*,*,#44255,.T.);
#65318=ORIENTED_EDGE('',*,*,#44375,.T.);
#65319=ORIENTED_EDGE('',*,*,#33983,.T.);
#65320=ORIENTED_EDGE('',*,*,#44376,.F.);
#65321=ORIENTED_EDGE('',*,*,#44377,.F.);
#65322=ORIENTED_EDGE('',*,*,#44376,.T.);
#65323=ORIENTED_EDGE('',*,*,#33982,.T.);
#65324=ORIENTED_EDGE('',*,*,#44378,.F.);
#65325=ORIENTED_EDGE('',*,*,#44377,.T.);
#65326=ORIENTED_EDGE('',*,*,#33981,.T.);
#65327=ORIENTED_EDGE('',*,*,#44379,.F.);
#65328=ORIENTED_EDGE('',*,*,#44378,.T.);
#65329=ORIENTED_EDGE('',*,*,#33980,.T.);
#65330=ORIENTED_EDGE('',*,*,#44380,.F.);
#65331=ORIENTED_EDGE('',*,*,#44379,.T.);
#65332=ORIENTED_EDGE('',*,*,#33979,.T.);
#65333=ORIENTED_EDGE('',*,*,#44257,.T.);
#65334=ORIENTED_EDGE('',*,*,#44380,.T.);
#65335=ORIENTED_EDGE('',*,*,#33978,.T.);
#65336=ORIENTED_EDGE('',*,*,#44381,.F.);
#65337=ORIENTED_EDGE('',*,*,#44258,.T.);
#65338=ORIENTED_EDGE('',*,*,#44381,.T.);
#65339=ORIENTED_EDGE('',*,*,#33977,.T.);
#65340=ORIENTED_EDGE('',*,*,#44382,.F.);
#65341=ORIENTED_EDGE('',*,*,#44383,.F.);
#65342=ORIENTED_EDGE('',*,*,#44382,.T.);
#65343=ORIENTED_EDGE('',*,*,#33976,.T.);
#65344=ORIENTED_EDGE('',*,*,#44384,.F.);
#65345=ORIENTED_EDGE('',*,*,#44383,.T.);
#65346=ORIENTED_EDGE('',*,*,#33975,.T.);
#65347=ORIENTED_EDGE('',*,*,#44385,.F.);
#65348=ORIENTED_EDGE('',*,*,#44384,.T.);
#65349=ORIENTED_EDGE('',*,*,#33974,.T.);
#65350=ORIENTED_EDGE('',*,*,#44386,.F.);
#65351=ORIENTED_EDGE('',*,*,#44385,.T.);
#65352=ORIENTED_EDGE('',*,*,#33973,.T.);
#65353=ORIENTED_EDGE('',*,*,#44260,.T.);
#65354=ORIENTED_EDGE('',*,*,#44386,.T.);
#65355=ORIENTED_EDGE('',*,*,#33972,.T.);
#65356=ORIENTED_EDGE('',*,*,#44387,.F.);
#65357=ORIENTED_EDGE('',*,*,#44261,.T.);
#65358=ORIENTED_EDGE('',*,*,#44387,.T.);
#65359=ORIENTED_EDGE('',*,*,#33971,.T.);
#65360=ORIENTED_EDGE('',*,*,#44388,.F.);
#65361=ORIENTED_EDGE('',*,*,#44389,.F.);
#65362=ORIENTED_EDGE('',*,*,#44388,.T.);
#65363=ORIENTED_EDGE('',*,*,#33970,.T.);
#65364=ORIENTED_EDGE('',*,*,#44390,.F.);
#65365=ORIENTED_EDGE('',*,*,#44389,.T.);
#65366=ORIENTED_EDGE('',*,*,#33969,.T.);
#65367=ORIENTED_EDGE('',*,*,#44391,.F.);
#65368=ORIENTED_EDGE('',*,*,#44390,.T.);
#65369=ORIENTED_EDGE('',*,*,#33968,.T.);
#65370=ORIENTED_EDGE('',*,*,#44392,.F.);
#65371=ORIENTED_EDGE('',*,*,#44391,.T.);
#65372=ORIENTED_EDGE('',*,*,#33967,.T.);
#65373=ORIENTED_EDGE('',*,*,#44263,.T.);
#65374=ORIENTED_EDGE('',*,*,#44392,.T.);
#65375=ORIENTED_EDGE('',*,*,#33966,.T.);
#65376=ORIENTED_EDGE('',*,*,#44393,.F.);
#65377=ORIENTED_EDGE('',*,*,#44393,.T.);
#65378=ORIENTED_EDGE('',*,*,#33965,.T.);
#65379=ORIENTED_EDGE('',*,*,#34146,.T.);
#65380=ORIENTED_EDGE('',*,*,#44394,.F.);
#65381=ORIENTED_EDGE('',*,*,#44264,.T.);
#65382=ORIENTED_EDGE('',*,*,#44394,.T.);
#65383=ORIENTED_EDGE('',*,*,#34145,.T.);
#65384=ORIENTED_EDGE('',*,*,#34141,.T.);
#65385=ORIENTED_EDGE('',*,*,#44395,.F.);
#65386=ORIENTED_EDGE('',*,*,#44395,.T.);
#65387=ORIENTED_EDGE('',*,*,#34140,.T.);
#65388=ORIENTED_EDGE('',*,*,#34137,.T.);
#65389=ORIENTED_EDGE('',*,*,#44396,.F.);
#65390=ORIENTED_EDGE('',*,*,#44397,.F.);
#65391=ORIENTED_EDGE('',*,*,#44396,.T.);
#65392=ORIENTED_EDGE('',*,*,#34136,.T.);
#65393=ORIENTED_EDGE('',*,*,#44398,.F.);
#65394=ORIENTED_EDGE('',*,*,#44397,.T.);
#65395=ORIENTED_EDGE('',*,*,#34135,.T.);
#65396=ORIENTED_EDGE('',*,*,#44266,.T.);
#65397=ORIENTED_EDGE('',*,*,#44398,.T.);
#65398=ORIENTED_EDGE('',*,*,#34134,.T.);
#65399=ORIENTED_EDGE('',*,*,#44399,.F.);
#65400=ORIENTED_EDGE('',*,*,#44267,.T.);
#65401=ORIENTED_EDGE('',*,*,#44399,.T.);
#65402=ORIENTED_EDGE('',*,*,#34133,.T.);
#65403=ORIENTED_EDGE('',*,*,#44400,.F.);
#65404=ORIENTED_EDGE('',*,*,#44401,.F.);
#65405=ORIENTED_EDGE('',*,*,#44400,.T.);
#65406=ORIENTED_EDGE('',*,*,#34132,.T.);
#65407=ORIENTED_EDGE('',*,*,#44402,.F.);
#65408=ORIENTED_EDGE('',*,*,#44401,.T.);
#65409=ORIENTED_EDGE('',*,*,#34131,.T.);
#65410=ORIENTED_EDGE('',*,*,#44403,.F.);
#65411=ORIENTED_EDGE('',*,*,#44402,.T.);
#65412=ORIENTED_EDGE('',*,*,#34130,.T.);
#65413=ORIENTED_EDGE('',*,*,#44404,.F.);
#65414=ORIENTED_EDGE('',*,*,#44403,.T.);
#65415=ORIENTED_EDGE('',*,*,#34129,.T.);
#65416=ORIENTED_EDGE('',*,*,#44269,.T.);
#65417=ORIENTED_EDGE('',*,*,#44404,.T.);
#65418=ORIENTED_EDGE('',*,*,#34128,.T.);
#65419=ORIENTED_EDGE('',*,*,#44405,.F.);
#65420=ORIENTED_EDGE('',*,*,#44270,.T.);
#65421=ORIENTED_EDGE('',*,*,#44405,.T.);
#65422=ORIENTED_EDGE('',*,*,#34127,.T.);
#65423=ORIENTED_EDGE('',*,*,#44406,.F.);
#65424=ORIENTED_EDGE('',*,*,#44407,.F.);
#65425=ORIENTED_EDGE('',*,*,#44406,.T.);
#65426=ORIENTED_EDGE('',*,*,#34126,.T.);
#65427=ORIENTED_EDGE('',*,*,#44408,.F.);
#65428=ORIENTED_EDGE('',*,*,#44407,.T.);
#65429=ORIENTED_EDGE('',*,*,#34125,.T.);
#65430=ORIENTED_EDGE('',*,*,#44409,.F.);
#65431=ORIENTED_EDGE('',*,*,#44408,.T.);
#65432=ORIENTED_EDGE('',*,*,#34124,.T.);
#65433=ORIENTED_EDGE('',*,*,#44410,.F.);
#65434=ORIENTED_EDGE('',*,*,#44409,.T.);
#65435=ORIENTED_EDGE('',*,*,#34123,.T.);
#65436=ORIENTED_EDGE('',*,*,#44272,.T.);
#65437=ORIENTED_EDGE('',*,*,#44410,.T.);
#65438=ORIENTED_EDGE('',*,*,#34122,.T.);
#65439=ORIENTED_EDGE('',*,*,#44411,.F.);
#65440=ORIENTED_EDGE('',*,*,#44273,.T.);
#65441=ORIENTED_EDGE('',*,*,#44411,.T.);
#65442=ORIENTED_EDGE('',*,*,#34121,.T.);
#65443=ORIENTED_EDGE('',*,*,#44412,.F.);
#65444=ORIENTED_EDGE('',*,*,#44413,.F.);
#65445=ORIENTED_EDGE('',*,*,#44412,.T.);
#65446=ORIENTED_EDGE('',*,*,#34120,.T.);
#65447=ORIENTED_EDGE('',*,*,#44414,.F.);
#65448=ORIENTED_EDGE('',*,*,#44413,.T.);
#65449=ORIENTED_EDGE('',*,*,#34119,.T.);
#65450=ORIENTED_EDGE('',*,*,#44415,.F.);
#65451=ORIENTED_EDGE('',*,*,#44414,.T.);
#65452=ORIENTED_EDGE('',*,*,#34118,.T.);
#65453=ORIENTED_EDGE('',*,*,#44416,.F.);
#65454=ORIENTED_EDGE('',*,*,#44415,.T.);
#65455=ORIENTED_EDGE('',*,*,#34117,.T.);
#65456=ORIENTED_EDGE('',*,*,#44275,.T.);
#65457=ORIENTED_EDGE('',*,*,#44416,.T.);
#65458=ORIENTED_EDGE('',*,*,#34116,.T.);
#65459=ORIENTED_EDGE('',*,*,#44417,.F.);
#65460=ORIENTED_EDGE('',*,*,#44276,.T.);
#65461=ORIENTED_EDGE('',*,*,#44417,.T.);
#65462=ORIENTED_EDGE('',*,*,#34115,.T.);
#65463=ORIENTED_EDGE('',*,*,#44418,.F.);
#65464=ORIENTED_EDGE('',*,*,#44419,.F.);
#65465=ORIENTED_EDGE('',*,*,#44418,.T.);
#65466=ORIENTED_EDGE('',*,*,#34114,.T.);
#65467=ORIENTED_EDGE('',*,*,#44420,.F.);
#65468=ORIENTED_EDGE('',*,*,#44419,.T.);
#65469=ORIENTED_EDGE('',*,*,#34113,.T.);
#65470=ORIENTED_EDGE('',*,*,#44421,.F.);
#65471=ORIENTED_EDGE('',*,*,#44420,.T.);
#65472=ORIENTED_EDGE('',*,*,#34112,.T.);
#65473=ORIENTED_EDGE('',*,*,#44422,.F.);
#65474=ORIENTED_EDGE('',*,*,#44421,.T.);
#65475=ORIENTED_EDGE('',*,*,#34111,.T.);
#65476=ORIENTED_EDGE('',*,*,#44278,.T.);
#65477=ORIENTED_EDGE('',*,*,#44422,.T.);
#65478=ORIENTED_EDGE('',*,*,#34110,.T.);
#65479=ORIENTED_EDGE('',*,*,#44423,.F.);
#65480=ORIENTED_EDGE('',*,*,#44279,.T.);
#65481=ORIENTED_EDGE('',*,*,#44423,.T.);
#65482=ORIENTED_EDGE('',*,*,#34109,.T.);
#65483=ORIENTED_EDGE('',*,*,#44424,.F.);
#65484=ORIENTED_EDGE('',*,*,#44425,.F.);
#65485=ORIENTED_EDGE('',*,*,#44424,.T.);
#65486=ORIENTED_EDGE('',*,*,#34108,.T.);
#65487=ORIENTED_EDGE('',*,*,#44426,.F.);
#65488=ORIENTED_EDGE('',*,*,#44425,.T.);
#65489=ORIENTED_EDGE('',*,*,#34107,.T.);
#65490=ORIENTED_EDGE('',*,*,#44427,.F.);
#65491=ORIENTED_EDGE('',*,*,#44426,.T.);
#65492=ORIENTED_EDGE('',*,*,#34106,.T.);
#65493=ORIENTED_EDGE('',*,*,#44428,.F.);
#65494=ORIENTED_EDGE('',*,*,#44427,.T.);
#65495=ORIENTED_EDGE('',*,*,#34105,.T.);
#65496=ORIENTED_EDGE('',*,*,#44281,.T.);
#65497=ORIENTED_EDGE('',*,*,#44428,.T.);
#65498=ORIENTED_EDGE('',*,*,#34104,.T.);
#65499=ORIENTED_EDGE('',*,*,#44429,.F.);
#65500=ORIENTED_EDGE('',*,*,#44282,.T.);
#65501=ORIENTED_EDGE('',*,*,#44429,.T.);
#65502=ORIENTED_EDGE('',*,*,#34103,.T.);
#65503=ORIENTED_EDGE('',*,*,#44430,.F.);
#65504=ORIENTED_EDGE('',*,*,#44431,.F.);
#65505=ORIENTED_EDGE('',*,*,#44430,.T.);
#65506=ORIENTED_EDGE('',*,*,#34102,.T.);
#65507=ORIENTED_EDGE('',*,*,#44432,.F.);
#65508=ORIENTED_EDGE('',*,*,#44431,.T.);
#65509=ORIENTED_EDGE('',*,*,#34101,.T.);
#65510=ORIENTED_EDGE('',*,*,#44433,.F.);
#65511=ORIENTED_EDGE('',*,*,#44432,.T.);
#65512=ORIENTED_EDGE('',*,*,#34100,.T.);
#65513=ORIENTED_EDGE('',*,*,#44434,.F.);
#65514=ORIENTED_EDGE('',*,*,#44433,.T.);
#65515=ORIENTED_EDGE('',*,*,#34099,.T.);
#65516=ORIENTED_EDGE('',*,*,#44284,.T.);
#65517=ORIENTED_EDGE('',*,*,#44434,.T.);
#65518=ORIENTED_EDGE('',*,*,#34098,.T.);
#65519=ORIENTED_EDGE('',*,*,#44435,.F.);
#65520=ORIENTED_EDGE('',*,*,#44285,.T.);
#65521=ORIENTED_EDGE('',*,*,#44435,.T.);
#65522=ORIENTED_EDGE('',*,*,#34097,.T.);
#65523=ORIENTED_EDGE('',*,*,#44436,.F.);
#65524=ORIENTED_EDGE('',*,*,#44437,.F.);
#65525=ORIENTED_EDGE('',*,*,#44436,.T.);
#65526=ORIENTED_EDGE('',*,*,#34096,.T.);
#65527=ORIENTED_EDGE('',*,*,#44438,.F.);
#65528=ORIENTED_EDGE('',*,*,#44437,.T.);
#65529=ORIENTED_EDGE('',*,*,#34095,.T.);
#65530=ORIENTED_EDGE('',*,*,#44439,.F.);
#65531=ORIENTED_EDGE('',*,*,#44438,.T.);
#65532=ORIENTED_EDGE('',*,*,#34094,.T.);
#65533=ORIENTED_EDGE('',*,*,#44440,.F.);
#65534=ORIENTED_EDGE('',*,*,#44439,.T.);
#65535=ORIENTED_EDGE('',*,*,#34093,.T.);
#65536=ORIENTED_EDGE('',*,*,#44287,.T.);
#65537=ORIENTED_EDGE('',*,*,#44440,.T.);
#65538=ORIENTED_EDGE('',*,*,#34092,.T.);
#65539=ORIENTED_EDGE('',*,*,#44441,.F.);
#65540=ORIENTED_EDGE('',*,*,#44288,.T.);
#65541=ORIENTED_EDGE('',*,*,#44441,.T.);
#65542=ORIENTED_EDGE('',*,*,#34091,.T.);
#65543=ORIENTED_EDGE('',*,*,#44442,.F.);
#65544=ORIENTED_EDGE('',*,*,#44443,.F.);
#65545=ORIENTED_EDGE('',*,*,#44442,.T.);
#65546=ORIENTED_EDGE('',*,*,#34090,.T.);
#65547=ORIENTED_EDGE('',*,*,#44444,.F.);
#65548=ORIENTED_EDGE('',*,*,#44443,.T.);
#65549=ORIENTED_EDGE('',*,*,#34089,.T.);
#65550=ORIENTED_EDGE('',*,*,#44445,.F.);
#65551=ORIENTED_EDGE('',*,*,#44444,.T.);
#65552=ORIENTED_EDGE('',*,*,#34088,.T.);
#65553=ORIENTED_EDGE('',*,*,#44446,.F.);
#65554=ORIENTED_EDGE('',*,*,#44445,.T.);
#65555=ORIENTED_EDGE('',*,*,#34087,.T.);
#65556=ORIENTED_EDGE('',*,*,#44290,.T.);
#65557=ORIENTED_EDGE('',*,*,#44446,.T.);
#65558=ORIENTED_EDGE('',*,*,#34086,.T.);
#65559=ORIENTED_EDGE('',*,*,#44447,.F.);
#65560=ORIENTED_EDGE('',*,*,#44291,.T.);
#65561=ORIENTED_EDGE('',*,*,#44447,.T.);
#65562=ORIENTED_EDGE('',*,*,#34085,.T.);
#65563=ORIENTED_EDGE('',*,*,#44448,.F.);
#65564=ORIENTED_EDGE('',*,*,#44449,.F.);
#65565=ORIENTED_EDGE('',*,*,#44448,.T.);
#65566=ORIENTED_EDGE('',*,*,#34084,.T.);
#65567=ORIENTED_EDGE('',*,*,#44450,.F.);
#65568=ORIENTED_EDGE('',*,*,#44449,.T.);
#65569=ORIENTED_EDGE('',*,*,#34083,.T.);
#65570=ORIENTED_EDGE('',*,*,#44451,.F.);
#65571=ORIENTED_EDGE('',*,*,#44450,.T.);
#65572=ORIENTED_EDGE('',*,*,#34082,.T.);
#65573=ORIENTED_EDGE('',*,*,#44452,.F.);
#65574=ORIENTED_EDGE('',*,*,#44451,.T.);
#65575=ORIENTED_EDGE('',*,*,#34081,.T.);
#65576=ORIENTED_EDGE('',*,*,#44293,.T.);
#65577=ORIENTED_EDGE('',*,*,#44452,.T.);
#65578=ORIENTED_EDGE('',*,*,#34080,.T.);
#65579=ORIENTED_EDGE('',*,*,#44453,.F.);
#65580=ORIENTED_EDGE('',*,*,#44294,.T.);
#65581=ORIENTED_EDGE('',*,*,#44453,.T.);
#65582=ORIENTED_EDGE('',*,*,#34079,.T.);
#65583=ORIENTED_EDGE('',*,*,#44454,.F.);
#65584=ORIENTED_EDGE('',*,*,#44455,.F.);
#65585=ORIENTED_EDGE('',*,*,#44454,.T.);
#65586=ORIENTED_EDGE('',*,*,#34078,.T.);
#65587=ORIENTED_EDGE('',*,*,#44456,.F.);
#65588=ORIENTED_EDGE('',*,*,#44455,.T.);
#65589=ORIENTED_EDGE('',*,*,#34077,.T.);
#65590=ORIENTED_EDGE('',*,*,#44457,.F.);
#65591=ORIENTED_EDGE('',*,*,#44456,.T.);
#65592=ORIENTED_EDGE('',*,*,#34076,.T.);
#65593=ORIENTED_EDGE('',*,*,#44458,.F.);
#65594=ORIENTED_EDGE('',*,*,#44457,.T.);
#65595=ORIENTED_EDGE('',*,*,#34075,.T.);
#65596=ORIENTED_EDGE('',*,*,#44296,.T.);
#65597=ORIENTED_EDGE('',*,*,#44458,.T.);
#65598=ORIENTED_EDGE('',*,*,#34074,.T.);
#65599=ORIENTED_EDGE('',*,*,#44459,.F.);
#65600=ORIENTED_EDGE('',*,*,#44297,.T.);
#65601=ORIENTED_EDGE('',*,*,#44459,.T.);
#65602=ORIENTED_EDGE('',*,*,#34073,.T.);
#65603=ORIENTED_EDGE('',*,*,#44460,.F.);
#65604=ORIENTED_EDGE('',*,*,#44461,.F.);
#65605=ORIENTED_EDGE('',*,*,#44460,.T.);
#65606=ORIENTED_EDGE('',*,*,#34072,.T.);
#65607=ORIENTED_EDGE('',*,*,#44462,.F.);
#65608=ORIENTED_EDGE('',*,*,#44461,.T.);
#65609=ORIENTED_EDGE('',*,*,#34071,.T.);
#65610=ORIENTED_EDGE('',*,*,#44463,.F.);
#65611=ORIENTED_EDGE('',*,*,#44462,.T.);
#65612=ORIENTED_EDGE('',*,*,#34070,.T.);
#65613=ORIENTED_EDGE('',*,*,#44464,.F.);
#65614=ORIENTED_EDGE('',*,*,#44463,.T.);
#65615=ORIENTED_EDGE('',*,*,#34069,.T.);
#65616=ORIENTED_EDGE('',*,*,#44299,.T.);
#65617=ORIENTED_EDGE('',*,*,#44464,.T.);
#65618=ORIENTED_EDGE('',*,*,#34068,.T.);
#65619=ORIENTED_EDGE('',*,*,#44465,.F.);
#65620=ORIENTED_EDGE('',*,*,#44300,.T.);
#65621=ORIENTED_EDGE('',*,*,#44465,.T.);
#65622=ORIENTED_EDGE('',*,*,#34067,.T.);
#65623=ORIENTED_EDGE('',*,*,#44466,.F.);
#65624=ORIENTED_EDGE('',*,*,#44467,.F.);
#65625=ORIENTED_EDGE('',*,*,#44466,.T.);
#65626=ORIENTED_EDGE('',*,*,#34066,.T.);
#65627=ORIENTED_EDGE('',*,*,#44468,.F.);
#65628=ORIENTED_EDGE('',*,*,#44467,.T.);
#65629=ORIENTED_EDGE('',*,*,#34065,.T.);
#65630=ORIENTED_EDGE('',*,*,#44469,.F.);
#65631=ORIENTED_EDGE('',*,*,#44468,.T.);
#65632=ORIENTED_EDGE('',*,*,#34064,.T.);
#65633=ORIENTED_EDGE('',*,*,#44470,.F.);
#65634=ORIENTED_EDGE('',*,*,#44469,.T.);
#65635=ORIENTED_EDGE('',*,*,#34063,.T.);
#65636=ORIENTED_EDGE('',*,*,#44302,.T.);
#65637=ORIENTED_EDGE('',*,*,#44470,.T.);
#65638=ORIENTED_EDGE('',*,*,#34062,.T.);
#65639=ORIENTED_EDGE('',*,*,#44471,.F.);
#65640=ORIENTED_EDGE('',*,*,#44303,.T.);
#65641=ORIENTED_EDGE('',*,*,#44471,.T.);
#65642=ORIENTED_EDGE('',*,*,#34061,.T.);
#65643=ORIENTED_EDGE('',*,*,#44472,.F.);
#65644=ORIENTED_EDGE('',*,*,#44473,.F.);
#65645=ORIENTED_EDGE('',*,*,#44472,.T.);
#65646=ORIENTED_EDGE('',*,*,#34060,.T.);
#65647=ORIENTED_EDGE('',*,*,#44474,.F.);
#65648=ORIENTED_EDGE('',*,*,#44473,.T.);
#65649=ORIENTED_EDGE('',*,*,#34059,.T.);
#65650=ORIENTED_EDGE('',*,*,#44475,.F.);
#65651=ORIENTED_EDGE('',*,*,#44474,.T.);
#65652=ORIENTED_EDGE('',*,*,#34058,.T.);
#65653=ORIENTED_EDGE('',*,*,#44476,.F.);
#65654=ORIENTED_EDGE('',*,*,#44475,.T.);
#65655=ORIENTED_EDGE('',*,*,#34057,.T.);
#65656=ORIENTED_EDGE('',*,*,#44305,.T.);
#65657=ORIENTED_EDGE('',*,*,#44476,.T.);
#65658=ORIENTED_EDGE('',*,*,#34056,.T.);
#65659=ORIENTED_EDGE('',*,*,#44477,.F.);
#65660=ORIENTED_EDGE('',*,*,#44306,.T.);
#65661=ORIENTED_EDGE('',*,*,#44477,.T.);
#65662=ORIENTED_EDGE('',*,*,#34055,.T.);
#65663=ORIENTED_EDGE('',*,*,#44478,.F.);
#65664=ORIENTED_EDGE('',*,*,#44479,.F.);
#65665=ORIENTED_EDGE('',*,*,#44478,.T.);
#65666=ORIENTED_EDGE('',*,*,#34054,.T.);
#65667=ORIENTED_EDGE('',*,*,#44480,.F.);
#65668=ORIENTED_EDGE('',*,*,#44479,.T.);
#65669=ORIENTED_EDGE('',*,*,#34053,.T.);
#65670=ORIENTED_EDGE('',*,*,#44481,.F.);
#65671=ORIENTED_EDGE('',*,*,#44480,.T.);
#65672=ORIENTED_EDGE('',*,*,#34052,.T.);
#65673=ORIENTED_EDGE('',*,*,#44482,.F.);
#65674=ORIENTED_EDGE('',*,*,#44481,.T.);
#65675=ORIENTED_EDGE('',*,*,#34051,.T.);
#65676=ORIENTED_EDGE('',*,*,#44482,.T.);
#65677=ORIENTED_EDGE('',*,*,#34050,.T.);
#65678=ORIENTED_EDGE('',*,*,#44309,.T.);
#65679=ORIENTED_EDGE('',*,*,#44308,.T.);
#65680=ORIENTED_EDGE('',*,*,#34149,.T.);
#65681=ORIENTED_EDGE('',*,*,#34142,.F.);
#65682=ORIENTED_EDGE('',*,*,#34139,.T.);
#65683=ORIENTED_EDGE('',*,*,#34144,.F.);
#66004=CONICAL_SURFACE('',#71473,6.75,0.785398163397449);
#66005=CONICAL_SURFACE('',#71536,6.75,0.785398163397449);
#66006=CONICAL_SURFACE('',#71544,6.125,0.785398163397448);
#66007=CONICAL_SURFACE('',#71546,6.75,0.785398163397449);
#66008=CONICAL_SURFACE('',#71606,7.31092570000179,0.78539816339742);
#66009=CONICAL_SURFACE('',#71609,7.3109256999998,0.785398163397457);
#66010=CONICAL_SURFACE('',#71619,7.31092569999943,0.785398163397357);
#66011=CONICAL_SURFACE('',#71621,7.3529052680094,0.785398163397219);
#66012=CONICAL_SURFACE('',#71631,7.46402854799594,0.785398163398244);
#66013=CONICAL_SURFACE('',#76253,7.46402854800012,0.785398163397918);
#66014=CONICAL_SURFACE('',#76262,7.46402854799495,0.785398163396894);
#66015=CONICAL_SURFACE('',#76271,7.46402854801104,0.785398163397641);
#66016=CONICAL_SURFACE('',#76280,7.46402854800908,0.785398163396339);
#66017=CONICAL_SURFACE('',#76289,7.46402854799712,0.78539816339951);
#66018=CONICAL_SURFACE('',#76298,7.46402854799119,0.785398163398774);
#66019=CONICAL_SURFACE('',#76307,7.46402854800175,0.785398163396942);
#66020=CONICAL_SURFACE('',#76316,7.46402854798451,0.78539816339517);
#66021=CONICAL_SURFACE('',#76325,7.46402854799257,0.785398163397629);
#66022=CONICAL_SURFACE('',#76334,7.46402854800718,0.785398163399594);
#66023=CONICAL_SURFACE('',#76343,7.46402854800848,0.785398163399028);
#66024=CONICAL_SURFACE('',#76352,7.46402854798724,0.785398163396677);
#66025=CONICAL_SURFACE('',#76361,7.46402854800366,0.785398163396978);
#66026=CONICAL_SURFACE('',#76370,7.46402854801209,0.78539816339822);
#66027=CONICAL_SURFACE('',#76379,7.46402854800802,0.785398163399305);
#66028=CONICAL_SURFACE('',#76388,7.46402854799688,0.785398163397931);
#66029=CONICAL_SURFACE('',#76397,7.46402854799781,0.785398163396628);
#66030=CONICAL_SURFACE('',#76406,7.46402854800837,0.785398163398763);
#66031=CONICAL_SURFACE('',#76415,7.46402854800493,0.785398163399257);
#66032=CONICAL_SURFACE('',#76424,7.46402854799559,0.785398163397219);
#66033=CONICAL_SURFACE('',#76433,7.46402854800237,0.785398163397388);
#66034=CONICAL_SURFACE('',#76442,7.46402854799716,0.785398163397943);
#66035=CONICAL_SURFACE('',#76451,7.46402854800031,0.785398163398955);
#66036=CONICAL_SURFACE('',#76460,7.46402854800001,0.785398163396978);
#66037=CONICAL_SURFACE('',#76469,7.46402854801467,0.785398163399221);
#66038=CONICAL_SURFACE('',#76478,7.46402854801943,0.785398163397738);
#66039=CONICAL_SURFACE('',#76487,7.46402854798882,0.785398163396134);
#66040=CONICAL_SURFACE('',#76496,7.46402854799016,0.785398163396424);
#66041=CONICAL_SURFACE('',#76789,7.31092570000081,0.785398163397382);
#66042=CONICAL_SURFACE('',#76790,7.31092569999921,0.785398163397411);
#66043=CONICAL_SURFACE('',#76791,7.31092569999958,0.785398163397313);
#66044=CONICAL_SURFACE('',#76792,7.3109257000012,0.785398163397469);
#66045=CONICAL_SURFACE('',#76793,7.31092570000094,0.785398163397484);
#66046=CONICAL_SURFACE('',#76794,7.31092569999998,0.78539816339753);
#66047=CONICAL_SURFACE('',#76795,7.31092570000055,0.785398163397313);
#66048=CONICAL_SURFACE('',#76796,7.31092569999908,0.785398163397528);
#66049=CONICAL_SURFACE('',#76797,7.31092570000038,0.785398163397484);
#66050=CONICAL_SURFACE('',#76798,7.31092570000067,0.785398163397379);
#66051=CONICAL_SURFACE('',#76799,7.31092569999975,0.785398163397275);
#66052=CONICAL_SURFACE('',#76800,7.3109257,0.785398163397532);
#66053=CONICAL_SURFACE('',#76801,7.31092570000065,0.785398163397496);
#66054=CONICAL_SURFACE('',#76802,7.31092569999959,0.785398163397267);
#66055=CONICAL_SURFACE('',#76803,7.31092569999963,0.785398163397375);
#66056=CONICAL_SURFACE('',#76804,7.31092569999986,0.785398163397386);
#66057=CONICAL_SURFACE('',#76805,7.31092569999971,0.785398163397473);
#66058=CONICAL_SURFACE('',#76806,7.31092569999938,0.785398163397394);
#66059=CONICAL_SURFACE('',#76807,7.31092569999932,0.785398163397628);
#66060=CONICAL_SURFACE('',#76808,7.31092569999901,0.78539816339744);
#66061=CONICAL_SURFACE('',#76809,7.31092569999891,0.785398163397488);
#66062=CONICAL_SURFACE('',#76810,7.31092569999985,0.785398163397619);
#66063=CONICAL_SURFACE('',#76811,7.31092570000066,0.785398163397634);
#66064=CONICAL_SURFACE('',#76812,7.3109256999997,0.785398163397488);
#66065=CONICAL_SURFACE('',#76813,7.31092569999926,0.785398163397338);
#66066=CONICAL_SURFACE('',#76814,7.31092570000021,0.7853981633974);
#66067=CONICAL_SURFACE('',#76815,7.31092569999984,0.785398163397532);
#66068=CONICAL_SURFACE('',#77161,7.46402854799838,0.785398163397463);
#66069=CONICAL_SURFACE('',#77170,7.46402854800787,0.785398163397463);
#66070=CONICAL_SURFACE('',#77179,7.46402854801097,0.785398163397423);
#66071=CONICAL_SURFACE('',#77188,7.46402854799594,0.785398163397718);
#66072=CONICAL_SURFACE('',#77197,7.46402854800662,0.785398163397451);
#66073=CONICAL_SURFACE('',#77206,7.46402854799811,0.785398163397486);
#66074=CONICAL_SURFACE('',#77214,7.46402854799591,0.785398163397632);
#66075=CONICAL_SURFACE('',#77218,7.46402854799987,0.785398163397621);
#66076=CONICAL_SURFACE('',#77227,7.46402854798396,0.785398163397703);
#66077=CONICAL_SURFACE('',#77236,7.46402854798974,0.785398163397734);
#66078=CONICAL_SURFACE('',#77245,7.46402854799754,0.785398163397156);
#66079=CONICAL_SURFACE('',#77254,7.46402854799756,0.785398163397393);
#66080=CONICAL_SURFACE('',#77263,7.46402854798607,0.785398163397496);
#66081=CONICAL_SURFACE('',#77272,7.46402854798888,0.7853981633974);
#66082=CONICAL_SURFACE('',#77281,7.46402854799924,0.785398163397339);
#66083=CONICAL_SURFACE('',#77290,7.46402854800191,0.785398163397406);
#66084=CONICAL_SURFACE('',#77299,7.46402854799075,0.785398163397348);
#66085=CONICAL_SURFACE('',#77308,7.46402854800954,0.785398163397388);
#66086=CONICAL_SURFACE('',#77317,7.46402854799126,0.785398163397592);
#66087=CONICAL_SURFACE('',#77326,7.46402854799435,0.785398163397487);
#66088=CONICAL_SURFACE('',#77335,7.46402854800158,0.785398163397697);
#66089=CONICAL_SURFACE('',#77344,7.4640285480086,0.785398163397334);
#66090=CONICAL_SURFACE('',#77353,7.46402854800634,0.785398163397451);
#66091=CONICAL_SURFACE('',#77362,7.4640285480148,0.785398163397331);
#66092=CONICAL_SURFACE('',#77371,7.46402854800437,0.785398163397692);
#66093=CONICAL_SURFACE('',#77380,7.46402854799968,0.785398163397385);
#66094=CONICAL_SURFACE('',#77389,7.46402854800945,0.785398163397409);
#66095=CONICAL_SURFACE('',#77398,7.46402854799185,0.785398163397598);
#66096=CONICAL_SURFACE('',#77406,7.46402854799058,0.785398163397741);
#66097=CONICAL_SURFACE('',#77502,7.31092570000008,0.785398163397451);
#66098=CONICAL_SURFACE('',#77503,7.31092570000018,0.785398163397452);
#66099=CONICAL_SURFACE('',#77504,7.31092570000096,0.785398163397458);
#66100=CONICAL_SURFACE('',#77505,7.31092569999937,0.785398163397437);
#66101=CONICAL_SURFACE('',#77506,7.31092569999996,0.785398163397438);
#66102=CONICAL_SURFACE('',#77507,7.31092569999865,0.785398163397447);
#66103=CONICAL_SURFACE('',#77508,7.31092570000104,0.785398163397416);
#66104=CONICAL_SURFACE('',#77509,7.31092569999903,0.785398163397454);
#66105=CONICAL_SURFACE('',#77510,7.31092569999917,0.785398163397461);
#66106=CONICAL_SURFACE('',#77511,7.31092569999884,0.785398163397461);
#66107=CONICAL_SURFACE('',#77512,7.31092570000051,0.78539816339743);
#66108=CONICAL_SURFACE('',#77513,7.31092569999899,0.78539816339745);
#66109=CONICAL_SURFACE('',#77514,7.31092570000054,0.785398163397441);
#66110=CONICAL_SURFACE('',#77515,7.31092569999955,0.785398163397439);
#66111=CONICAL_SURFACE('',#77516,7.31092570000009,0.785398163397455);
#66112=CONICAL_SURFACE('',#77517,7.31092569999947,0.785398163397443);
#66113=CONICAL_SURFACE('',#77518,7.31092570000149,0.785398163397419);
#66114=CONICAL_SURFACE('',#77519,7.31092570000005,0.785398163397435);
#66115=CONICAL_SURFACE('',#77520,7.31092570000153,0.785398163397446);
#66116=CONICAL_SURFACE('',#77521,7.3109256999999,0.785398163397472);
#66117=CONICAL_SURFACE('',#77522,7.31092569999987,0.785398163397457);
#66118=CONICAL_SURFACE('',#77523,7.31092569999961,0.785398163397432);
#66119=CONICAL_SURFACE('',#77524,7.31092570000154,0.785398163397434);
#66120=CONICAL_SURFACE('',#77525,7.31092569999873,0.785398163397455);
#66121=CONICAL_SURFACE('',#77526,7.31092569999843,0.785398163397445);
#66122=CONICAL_SURFACE('',#77527,7.3109256999992,0.785398163397447);
#66123=CONICAL_SURFACE('',#77528,7.31092569999984,0.785398163397452);
#66133=ADVANCED_FACE('',(#5383),#66004,.T.);
#66134=ADVANCED_FACE('',(#5384),#4459,.F.);
#66135=ADVANCED_FACE('',(#5385),#66005,.T.);
#66136=ADVANCED_FACE('',(#5386),#4460,.F.);
#66137=ADVANCED_FACE('',(#5387),#4461,.F.);
#66138=ADVANCED_FACE('',(#5388),#66006,.F.);
#66139=ADVANCED_FACE('',(#5389),#66007,.T.);
#66140=ADVANCED_FACE('',(#5390),#66008,.T.);
#66141=ADVANCED_FACE('',(#5391),#66009,.T.);
#66142=ADVANCED_FACE('',(#5392),#4462,.T.);
#66143=ADVANCED_FACE('',(#5393),#4463,.T.);
#66144=ADVANCED_FACE('',(#5394),#66010,.T.);
#66145=ADVANCED_FACE('',(#5395),#66011,.T.);
#66146=ADVANCED_FACE('',(#5396),#4464,.T.);
#66147=ADVANCED_FACE('',(#5397),#4465,.T.);
#66148=ADVANCED_FACE('',(#5398),#66012,.T.);
#66149=ADVANCED_FACE('',(#5399),#4466,.T.);
#66150=ADVANCED_FACE('',(#5400),#4467,.T.);
#66151=ADVANCED_FACE('',(#5401),#4468,.T.);
#66152=ADVANCED_FACE('',(#5402),#4469,.T.);
#66153=ADVANCED_FACE('',(#5403),#4470,.T.);
#66154=ADVANCED_FACE('',(#5404),#4471,.T.);
#66155=ADVANCED_FACE('',(#5405),#4472,.T.);
#66156=ADVANCED_FACE('',(#5406),#4473,.T.);
#66157=ADVANCED_FACE('',(#5407),#4474,.T.);
#66158=ADVANCED_FACE('',(#5408),#4475,.T.);
#66159=ADVANCED_FACE('',(#5409),#4476,.T.);
#66160=ADVANCED_FACE('',(#5410),#4477,.T.);
#66161=ADVANCED_FACE('',(#5411),#4478,.T.);
#66162=ADVANCED_FACE('',(#5412),#4479,.T.);
#66163=ADVANCED_FACE('',(#5413),#4480,.T.);
#66164=ADVANCED_FACE('',(#5414),#4481,.T.);
#66165=ADVANCED_FACE('',(#5415),#4482,.T.);
#66166=ADVANCED_FACE('',(#5416),#4483,.T.);
#66167=ADVANCED_FACE('',(#5417),#4484,.T.);
#66168=ADVANCED_FACE('',(#5418),#4485,.T.);
#66169=ADVANCED_FACE('',(#5419),#4486,.T.);
#66170=ADVANCED_FACE('',(#5420),#4487,.T.);
#66171=ADVANCED_FACE('',(#5421),#4488,.T.);
#66172=ADVANCED_FACE('',(#5422),#4489,.T.);
#66173=ADVANCED_FACE('',(#5423),#4490,.T.);
#66174=ADVANCED_FACE('',(#5424),#194,.T.);
#66175=ADVANCED_FACE('',(#5425),#195,.T.);
#66176=ADVANCED_FACE('',(#5426),#4491,.T.);
#66177=ADVANCED_FACE('',(#5427),#196,.T.);
#66178=ADVANCED_FACE('',(#5428),#197,.T.);
#66179=ADVANCED_FACE('',(#5429),#4492,.T.);
#66180=ADVANCED_FACE('',(#5430),#198,.T.);
#66181=ADVANCED_FACE('',(#5431),#199,.T.);
#66182=ADVANCED_FACE('',(#5432),#4493,.T.);
#66183=ADVANCED_FACE('',(#5433),#200,.T.);
#66184=ADVANCED_FACE('',(#5434),#201,.T.);
#66185=ADVANCED_FACE('',(#5435),#4494,.T.);
#66186=ADVANCED_FACE('',(#5436),#202,.T.);
#66187=ADVANCED_FACE('',(#5437),#203,.T.);
#66188=ADVANCED_FACE('',(#5438),#4495,.T.);
#66189=ADVANCED_FACE('',(#5439),#204,.T.);
#66190=ADVANCED_FACE('',(#5440),#205,.T.);
#66191=ADVANCED_FACE('',(#5441),#4496,.T.);
#66192=ADVANCED_FACE('',(#5442),#206,.T.);
#66193=ADVANCED_FACE('',(#5443),#207,.T.);
#66194=ADVANCED_FACE('',(#5444),#208,.T.);
#66195=ADVANCED_FACE('',(#5445),#209,.T.);
#66196=ADVANCED_FACE('',(#5446),#4497,.T.);
#66197=ADVANCED_FACE('',(#5447),#210,.T.);
#66198=ADVANCED_FACE('',(#5448),#211,.T.);
#66199=ADVANCED_FACE('',(#5449),#4498,.T.);
#66200=ADVANCED_FACE('',(#5450),#212,.T.);
#66201=ADVANCED_FACE('',(#5451),#213,.T.);
#66202=ADVANCED_FACE('',(#5452),#4499,.T.);
#66203=ADVANCED_FACE('',(#5453),#214,.T.);
#66204=ADVANCED_FACE('',(#5454),#215,.T.);
#66205=ADVANCED_FACE('',(#5455),#4500,.T.);
#66206=ADVANCED_FACE('',(#5456),#216,.T.);
#66207=ADVANCED_FACE('',(#5457),#217,.T.);
#66208=ADVANCED_FACE('',(#5458),#4501,.T.);
#66209=ADVANCED_FACE('',(#5459),#218,.T.);
#66210=ADVANCED_FACE('',(#5460),#219,.T.);
#66211=ADVANCED_FACE('',(#5461),#4502,.T.);
#66212=ADVANCED_FACE('',(#5462),#220,.T.);
#66213=ADVANCED_FACE('',(#5463),#221,.T.);
#66214=ADVANCED_FACE('',(#5464),#4503,.T.);
#66215=ADVANCED_FACE('',(#5465),#222,.T.);
#66216=ADVANCED_FACE('',(#5466),#223,.T.);
#66217=ADVANCED_FACE('',(#5467),#4504,.T.);
#66218=ADVANCED_FACE('',(#5468),#224,.T.);
#66219=ADVANCED_FACE('',(#5469),#225,.T.);
#66220=ADVANCED_FACE('',(#5470),#4505,.T.);
#66221=ADVANCED_FACE('',(#5471),#226,.T.);
#66222=ADVANCED_FACE('',(#5472),#227,.T.);
#66223=ADVANCED_FACE('',(#5473),#4506,.T.);
#66224=ADVANCED_FACE('',(#5474),#228,.T.);
#66225=ADVANCED_FACE('',(#5475),#229,.T.);
#66226=ADVANCED_FACE('',(#5476),#4507,.T.);
#66227=ADVANCED_FACE('',(#5477),#230,.T.);
#66228=ADVANCED_FACE('',(#5478),#231,.T.);
#66229=ADVANCED_FACE('',(#5479),#4508,.T.);
#66230=ADVANCED_FACE('',(#5480),#232,.T.);
#66231=ADVANCED_FACE('',(#5481),#233,.T.);
#66232=ADVANCED_FACE('',(#5482),#4509,.T.);
#66233=ADVANCED_FACE('',(#5483),#234,.T.);
#66234=ADVANCED_FACE('',(#5484),#235,.T.);
#66235=ADVANCED_FACE('',(#5485),#4510,.T.);
#66236=ADVANCED_FACE('',(#5486),#236,.T.);
#66237=ADVANCED_FACE('',(#5487),#237,.T.);
#66238=ADVANCED_FACE('',(#5488),#4511,.T.);
#66239=ADVANCED_FACE('',(#5489),#238,.T.);
#66240=ADVANCED_FACE('',(#5490),#239,.T.);
#66241=ADVANCED_FACE('',(#5491),#4512,.T.);
#66242=ADVANCED_FACE('',(#5492),#240,.T.);
#66243=ADVANCED_FACE('',(#5493),#241,.T.);
#66244=ADVANCED_FACE('',(#5494),#4513,.T.);
#66245=ADVANCED_FACE('',(#5495),#242,.T.);
#66246=ADVANCED_FACE('',(#5496),#243,.T.);
#66247=ADVANCED_FACE('',(#5497),#244,.T.);
#66248=ADVANCED_FACE('',(#5498),#4514,.T.);
#66249=ADVANCED_FACE('',(#5499),#245,.T.);
#66250=ADVANCED_FACE('',(#5500),#4515,.T.);
#66251=ADVANCED_FACE('',(#5501),#246,.T.);
#66252=ADVANCED_FACE('',(#5502),#247,.T.);
#66253=ADVANCED_FACE('',(#5503),#4516,.T.);
#66254=ADVANCED_FACE('',(#5504),#248,.T.);
#66255=ADVANCED_FACE('',(#5505),#249,.T.);
#66256=ADVANCED_FACE('',(#5506),#4517,.T.);
#66257=ADVANCED_FACE('',(#5507),#250,.T.);
#66258=ADVANCED_FACE('',(#5508),#4518,.T.);
#66259=ADVANCED_FACE('',(#5509),#251,.T.);
#66260=ADVANCED_FACE('',(#5510),#252,.T.);
#66261=ADVANCED_FACE('',(#5511),#253,.T.);
#66262=ADVANCED_FACE('',(#5512),#254,.T.);
#66263=ADVANCED_FACE('',(#5513),#4519,.T.);
#66264=ADVANCED_FACE('',(#5514),#255,.T.);
#66265=ADVANCED_FACE('',(#5515),#256,.T.);
#66266=ADVANCED_FACE('',(#5516),#4520,.T.);
#66267=ADVANCED_FACE('',(#5517),#257,.T.);
#66268=ADVANCED_FACE('',(#5518),#258,.T.);
#66269=ADVANCED_FACE('',(#5519),#4521,.T.);
#66270=ADVANCED_FACE('',(#5520),#259,.T.);
#66271=ADVANCED_FACE('',(#5521),#260,.T.);
#66272=ADVANCED_FACE('',(#5522),#4522,.T.);
#66273=ADVANCED_FACE('',(#5523),#261,.T.);
#66274=ADVANCED_FACE('',(#5524),#262,.T.);
#66275=ADVANCED_FACE('',(#5525),#4523,.T.);
#66276=ADVANCED_FACE('',(#5526),#263,.T.);
#66277=ADVANCED_FACE('',(#5527),#264,.T.);
#66278=ADVANCED_FACE('',(#5528),#4524,.T.);
#66279=ADVANCED_FACE('',(#5529),#265,.T.);
#66280=ADVANCED_FACE('',(#5530),#266,.T.);
#66281=ADVANCED_FACE('',(#5531),#4525,.T.);
#66282=ADVANCED_FACE('',(#5532),#267,.T.);
#66283=ADVANCED_FACE('',(#5533),#268,.T.);
#66284=ADVANCED_FACE('',(#5534),#4526,.T.);
#66285=ADVANCED_FACE('',(#5535),#269,.T.);
#66286=ADVANCED_FACE('',(#5536),#270,.T.);
#66287=ADVANCED_FACE('',(#5537),#4527,.T.);
#66288=ADVANCED_FACE('',(#5538),#271,.T.);
#66289=ADVANCED_FACE('',(#5539),#272,.T.);
#66290=ADVANCED_FACE('',(#5540),#4528,.T.);
#66291=ADVANCED_FACE('',(#5541),#273,.T.);
#66292=ADVANCED_FACE('',(#5542),#274,.T.);
#66293=ADVANCED_FACE('',(#5543),#4529,.T.);
#66294=ADVANCED_FACE('',(#5544),#275,.T.);
#66295=ADVANCED_FACE('',(#5545),#276,.T.);
#66296=ADVANCED_FACE('',(#5546),#4530,.T.);
#66297=ADVANCED_FACE('',(#5547),#277,.T.);
#66298=ADVANCED_FACE('',(#5548),#278,.T.);
#66299=ADVANCED_FACE('',(#5549),#4531,.T.);
#66300=ADVANCED_FACE('',(#5550),#279,.T.);
#66301=ADVANCED_FACE('',(#5551),#280,.T.);
#66302=ADVANCED_FACE('',(#5552),#281,.T.);
#66303=ADVANCED_FACE('',(#5553),#282,.T.);
#66304=ADVANCED_FACE('',(#5554),#4532,.T.);
#66305=ADVANCED_FACE('',(#5555),#283,.T.);
#66306=ADVANCED_FACE('',(#5556),#284,.T.);
#66307=ADVANCED_FACE('',(#5557),#4533,.T.);
#66308=ADVANCED_FACE('',(#5558),#285,.T.);
#66309=ADVANCED_FACE('',(#5559),#286,.T.);
#66310=ADVANCED_FACE('',(#5560),#4534,.T.);
#66311=ADVANCED_FACE('',(#5561),#287,.T.);
#66312=ADVANCED_FACE('',(#5562),#288,.T.);
#66313=ADVANCED_FACE('',(#5563),#4535,.T.);
#66314=ADVANCED_FACE('',(#5564),#289,.T.);
#66315=ADVANCED_FACE('',(#5565),#290,.T.);
#66316=ADVANCED_FACE('',(#5566),#4536,.T.);
#66317=ADVANCED_FACE('',(#5567),#291,.T.);
#66318=ADVANCED_FACE('',(#5568),#292,.T.);
#66319=ADVANCED_FACE('',(#5569),#4537,.T.);
#66320=ADVANCED_FACE('',(#5570),#293,.T.);
#66321=ADVANCED_FACE('',(#5571),#294,.T.);
#66322=ADVANCED_FACE('',(#5572),#4538,.T.);
#66323=ADVANCED_FACE('',(#5573),#295,.T.);
#66324=ADVANCED_FACE('',(#5574),#296,.T.);
#66325=ADVANCED_FACE('',(#5575),#4539,.T.);
#66326=ADVANCED_FACE('',(#5576),#297,.T.);
#66327=ADVANCED_FACE('',(#5577),#298,.T.);
#66328=ADVANCED_FACE('',(#5578),#4540,.T.);
#66329=ADVANCED_FACE('',(#5579),#299,.T.);
#66330=ADVANCED_FACE('',(#5580),#300,.T.);
#66331=ADVANCED_FACE('',(#5581),#4541,.T.);
#66332=ADVANCED_FACE('',(#5582),#301,.T.);
#66333=ADVANCED_FACE('',(#5583),#302,.T.);
#66334=ADVANCED_FACE('',(#5584),#4542,.T.);
#66335=ADVANCED_FACE('',(#5585),#303,.T.);
#66336=ADVANCED_FACE('',(#5586),#304,.T.);
#66337=ADVANCED_FACE('',(#5587),#4543,.T.);
#66338=ADVANCED_FACE('',(#5588),#305,.T.);
#66339=ADVANCED_FACE('',(#5589),#306,.T.);
#66340=ADVANCED_FACE('',(#5590),#4544,.T.);
#66341=ADVANCED_FACE('',(#5591),#307,.T.);
#66342=ADVANCED_FACE('',(#5592),#308,.T.);
#66343=ADVANCED_FACE('',(#5593),#4545,.T.);
#66344=ADVANCED_FACE('',(#5594),#4546,.T.);
#66345=ADVANCED_FACE('',(#5595),#309,.T.);
#66346=ADVANCED_FACE('',(#5596),#310,.T.);
#66347=ADVANCED_FACE('',(#5597),#311,.T.);
#66348=ADVANCED_FACE('',(#5598),#312,.T.);
#66349=ADVANCED_FACE('',(#5599),#313,.T.);
#66350=ADVANCED_FACE('',(#5600),#314,.T.);
#66351=ADVANCED_FACE('',(#5601),#315,.T.);
#66352=ADVANCED_FACE('',(#5602),#316,.T.);
#66353=ADVANCED_FACE('',(#5603),#317,.T.);
#66354=ADVANCED_FACE('',(#5604),#318,.T.);
#66355=ADVANCED_FACE('',(#5605),#319,.T.);
#66356=ADVANCED_FACE('',(#5606),#320,.T.);
#66357=ADVANCED_FACE('',(#5607),#321,.T.);
#66358=ADVANCED_FACE('',(#5608),#322,.T.);
#66359=ADVANCED_FACE('',(#5609),#323,.T.);
#66360=ADVANCED_FACE('',(#5610),#324,.T.);
#66361=ADVANCED_FACE('',(#5611),#325,.T.);
#66362=ADVANCED_FACE('',(#5612),#326,.T.);
#66363=ADVANCED_FACE('',(#5613),#327,.T.);
#66364=ADVANCED_FACE('',(#5614),#328,.T.);
#66365=ADVANCED_FACE('',(#5615),#329,.T.);
#66366=ADVANCED_FACE('',(#5616),#330,.T.);
#66367=ADVANCED_FACE('',(#5617),#331,.T.);
#66368=ADVANCED_FACE('',(#5618),#332,.T.);
#66369=ADVANCED_FACE('',(#5619),#333,.T.);
#66370=ADVANCED_FACE('',(#5620),#334,.T.);
#66371=ADVANCED_FACE('',(#5621),#335,.T.);
#66372=ADVANCED_FACE('',(#5622),#336,.T.);
#66373=ADVANCED_FACE('',(#5623),#337,.T.);
#66374=ADVANCED_FACE('',(#5624),#338,.T.);
#66375=ADVANCED_FACE('',(#5625),#339,.T.);
#66376=ADVANCED_FACE('',(#5626),#340,.T.);
#66377=ADVANCED_FACE('',(#5627),#341,.T.);
#66378=ADVANCED_FACE('',(#5628),#342,.T.);
#66379=ADVANCED_FACE('',(#5629),#343,.T.);
#66380=ADVANCED_FACE('',(#5630),#344,.T.);
#66381=ADVANCED_FACE('',(#5631),#345,.T.);
#66382=ADVANCED_FACE('',(#5632),#346,.T.);
#66383=ADVANCED_FACE('',(#5633),#347,.T.);
#66384=ADVANCED_FACE('',(#5634),#348,.T.);
#66385=ADVANCED_FACE('',(#5635),#349,.T.);
#66386=ADVANCED_FACE('',(#5636),#350,.T.);
#66387=ADVANCED_FACE('',(#5637),#351,.T.);
#66388=ADVANCED_FACE('',(#5638),#352,.T.);
#66389=ADVANCED_FACE('',(#5639),#353,.T.);
#66390=ADVANCED_FACE('',(#5640),#354,.T.);
#66391=ADVANCED_FACE('',(#5641),#355,.T.);
#66392=ADVANCED_FACE('',(#5642),#356,.T.);
#66393=ADVANCED_FACE('',(#5643),#357,.T.);
#66394=ADVANCED_FACE('',(#5644),#358,.T.);
#66395=ADVANCED_FACE('',(#5645),#359,.T.);
#66396=ADVANCED_FACE('',(#5646),#360,.T.);
#66397=ADVANCED_FACE('',(#5647),#361,.T.);
#66398=ADVANCED_FACE('',(#5648),#362,.T.);
#66399=ADVANCED_FACE('',(#5649),#363,.T.);
#66400=ADVANCED_FACE('',(#5650),#364,.T.);
#66401=ADVANCED_FACE('',(#5651),#365,.T.);
#66402=ADVANCED_FACE('',(#5652),#366,.T.);
#66403=ADVANCED_FACE('',(#5653),#367,.T.);
#66404=ADVANCED_FACE('',(#5654),#368,.T.);
#66405=ADVANCED_FACE('',(#5655),#369,.T.);
#66406=ADVANCED_FACE('',(#5656),#370,.T.);
#66407=ADVANCED_FACE('',(#5657),#371,.T.);
#66408=ADVANCED_FACE('',(#5658),#372,.T.);
#66409=ADVANCED_FACE('',(#5659),#373,.T.);
#66410=ADVANCED_FACE('',(#5660),#374,.T.);
#66411=ADVANCED_FACE('',(#5661),#375,.T.);
#66412=ADVANCED_FACE('',(#5662),#376,.T.);
#66413=ADVANCED_FACE('',(#5663),#377,.T.);
#66414=ADVANCED_FACE('',(#5664),#378,.T.);
#66415=ADVANCED_FACE('',(#5665),#379,.T.);
#66416=ADVANCED_FACE('',(#5666),#380,.T.);
#66417=ADVANCED_FACE('',(#5667),#381,.T.);
#66418=ADVANCED_FACE('',(#5668),#382,.T.);
#66419=ADVANCED_FACE('',(#5669),#383,.T.);
#66420=ADVANCED_FACE('',(#5670),#384,.T.);
#66421=ADVANCED_FACE('',(#5671),#385,.T.);
#66422=ADVANCED_FACE('',(#5672),#386,.T.);
#66423=ADVANCED_FACE('',(#5673),#387,.T.);
#66424=ADVANCED_FACE('',(#5674),#388,.T.);
#66425=ADVANCED_FACE('',(#5675),#389,.T.);
#66426=ADVANCED_FACE('',(#5676),#390,.T.);
#66427=ADVANCED_FACE('',(#5677),#391,.T.);
#66428=ADVANCED_FACE('',(#5678),#392,.T.);
#66429=ADVANCED_FACE('',(#5679),#393,.T.);
#66430=ADVANCED_FACE('',(#5680),#394,.T.);
#66431=ADVANCED_FACE('',(#5681),#395,.T.);
#66432=ADVANCED_FACE('',(#5682),#396,.T.);
#66433=ADVANCED_FACE('',(#5683),#397,.T.);
#66434=ADVANCED_FACE('',(#5684),#398,.T.);
#66435=ADVANCED_FACE('',(#5685),#399,.T.);
#66436=ADVANCED_FACE('',(#5686),#400,.T.);
#66437=ADVANCED_FACE('',(#5687),#401,.T.);
#66438=ADVANCED_FACE('',(#5688),#402,.T.);
#66439=ADVANCED_FACE('',(#5689),#403,.T.);
#66440=ADVANCED_FACE('',(#5690),#404,.T.);
#66441=ADVANCED_FACE('',(#5691),#405,.T.);
#66442=ADVANCED_FACE('',(#5692),#406,.T.);
#66443=ADVANCED_FACE('',(#5693),#407,.T.);
#66444=ADVANCED_FACE('',(#5694),#408,.T.);
#66445=ADVANCED_FACE('',(#5695),#409,.T.);
#66446=ADVANCED_FACE('',(#5696),#410,.T.);
#66447=ADVANCED_FACE('',(#5697),#411,.T.);
#66448=ADVANCED_FACE('',(#5698),#412,.T.);
#66449=ADVANCED_FACE('',(#5699),#413,.T.);
#66450=ADVANCED_FACE('',(#5700),#414,.T.);
#66451=ADVANCED_FACE('',(#5701),#415,.T.);
#66452=ADVANCED_FACE('',(#5702),#416,.T.);
#66453=ADVANCED_FACE('',(#5703),#417,.T.);
#66454=ADVANCED_FACE('',(#5704),#418,.T.);
#66455=ADVANCED_FACE('',(#5705),#419,.T.);
#66456=ADVANCED_FACE('',(#5706),#420,.T.);
#66457=ADVANCED_FACE('',(#5707),#421,.T.);
#66458=ADVANCED_FACE('',(#5708),#422,.T.);
#66459=ADVANCED_FACE('',(#5709),#423,.T.);
#66460=ADVANCED_FACE('',(#5710),#424,.T.);
#66461=ADVANCED_FACE('',(#5711),#425,.T.);
#66462=ADVANCED_FACE('',(#5712),#426,.T.);
#66463=ADVANCED_FACE('',(#5713),#4547,.T.);
#66464=ADVANCED_FACE('',(#5714),#427,.T.);
#66465=ADVANCED_FACE('',(#5715),#428,.T.);
#66466=ADVANCED_FACE('',(#5716),#4548,.T.);
#66467=ADVANCED_FACE('',(#5717),#429,.T.);
#66468=ADVANCED_FACE('',(#5718),#430,.T.);
#66469=ADVANCED_FACE('',(#5719),#4549,.T.);
#66470=ADVANCED_FACE('',(#5720),#431,.T.);
#66471=ADVANCED_FACE('',(#5721),#432,.T.);
#66472=ADVANCED_FACE('',(#5722),#4550,.T.);
#66473=ADVANCED_FACE('',(#5723),#433,.T.);
#66474=ADVANCED_FACE('',(#5724),#434,.T.);
#66475=ADVANCED_FACE('',(#5725),#4551,.T.);
#66476=ADVANCED_FACE('',(#5726),#435,.T.);
#66477=ADVANCED_FACE('',(#5727),#436,.T.);
#66478=ADVANCED_FACE('',(#5728),#4552,.T.);
#66479=ADVANCED_FACE('',(#5729),#437,.T.);
#66480=ADVANCED_FACE('',(#5730),#438,.T.);
#66481=ADVANCED_FACE('',(#5731),#4553,.T.);
#66482=ADVANCED_FACE('',(#5732),#439,.T.);
#66483=ADVANCED_FACE('',(#5733),#440,.T.);
#66484=ADVANCED_FACE('',(#5734),#4554,.T.);
#66485=ADVANCED_FACE('',(#5735),#441,.T.);
#66486=ADVANCED_FACE('',(#5736),#442,.T.);
#66487=ADVANCED_FACE('',(#5737),#4555,.T.);
#66488=ADVANCED_FACE('',(#5738),#443,.T.);
#66489=ADVANCED_FACE('',(#5739),#444,.T.);
#66490=ADVANCED_FACE('',(#5740),#4556,.T.);
#66491=ADVANCED_FACE('',(#5741),#445,.T.);
#66492=ADVANCED_FACE('',(#5742),#446,.T.);
#66493=ADVANCED_FACE('',(#5743),#4557,.T.);
#66494=ADVANCED_FACE('',(#5744),#447,.T.);
#66495=ADVANCED_FACE('',(#5745),#448,.T.);
#66496=ADVANCED_FACE('',(#5746),#4558,.T.);
#66497=ADVANCED_FACE('',(#5747),#449,.T.);
#66498=ADVANCED_FACE('',(#5748),#450,.T.);
#66499=ADVANCED_FACE('',(#5749),#4559,.T.);
#66500=ADVANCED_FACE('',(#5750),#451,.T.);
#66501=ADVANCED_FACE('',(#5751),#452,.T.);
#66502=ADVANCED_FACE('',(#5752),#4560,.T.);
#66503=ADVANCED_FACE('',(#5753),#453,.T.);
#66504=ADVANCED_FACE('',(#5754),#454,.T.);
#66505=ADVANCED_FACE('',(#5755),#455,.T.);
#66506=ADVANCED_FACE('',(#5756),#456,.T.);
#66507=ADVANCED_FACE('',(#5757),#4561,.T.);
#66508=ADVANCED_FACE('',(#5758),#457,.T.);
#66509=ADVANCED_FACE('',(#5759),#458,.T.);
#66510=ADVANCED_FACE('',(#5760),#4562,.T.);
#66511=ADVANCED_FACE('',(#5761),#459,.T.);
#66512=ADVANCED_FACE('',(#5762),#460,.T.);
#66513=ADVANCED_FACE('',(#5763),#4563,.T.);
#66514=ADVANCED_FACE('',(#5764),#461,.T.);
#66515=ADVANCED_FACE('',(#5765),#462,.T.);
#66516=ADVANCED_FACE('',(#5766),#4564,.T.);
#66517=ADVANCED_FACE('',(#5767),#463,.T.);
#66518=ADVANCED_FACE('',(#5768),#464,.T.);
#66519=ADVANCED_FACE('',(#5769),#4565,.T.);
#66520=ADVANCED_FACE('',(#5770),#465,.T.);
#66521=ADVANCED_FACE('',(#5771),#466,.T.);
#66522=ADVANCED_FACE('',(#5772),#4566,.T.);
#66523=ADVANCED_FACE('',(#5773),#467,.T.);
#66524=ADVANCED_FACE('',(#5774),#468,.T.);
#66525=ADVANCED_FACE('',(#5775),#4567,.T.);
#66526=ADVANCED_FACE('',(#5776),#469,.T.);
#66527=ADVANCED_FACE('',(#5777),#470,.T.);
#66528=ADVANCED_FACE('',(#5778),#4568,.T.);
#66529=ADVANCED_FACE('',(#5779),#471,.T.);
#66530=ADVANCED_FACE('',(#5780),#472,.T.);
#66531=ADVANCED_FACE('',(#5781),#4569,.T.);
#66532=ADVANCED_FACE('',(#5782),#473,.T.);
#66533=ADVANCED_FACE('',(#5783),#474,.T.);
#66534=ADVANCED_FACE('',(#5784),#475,.T.);
#66535=ADVANCED_FACE('',(#5785),#4570,.T.);
#66536=ADVANCED_FACE('',(#5786),#476,.T.);
#66537=ADVANCED_FACE('',(#5787),#4571,.T.);
#66538=ADVANCED_FACE('',(#5788),#477,.T.);
#66539=ADVANCED_FACE('',(#5789),#478,.T.);
#66540=ADVANCED_FACE('',(#5790),#4572,.T.);
#66541=ADVANCED_FACE('',(#5791),#479,.T.);
#66542=ADVANCED_FACE('',(#5792),#480,.T.);
#66543=ADVANCED_FACE('',(#5793),#4573,.T.);
#66544=ADVANCED_FACE('',(#5794),#481,.T.);
#66545=ADVANCED_FACE('',(#5795),#482,.T.);
#66546=ADVANCED_FACE('',(#5796),#4574,.T.);
#66547=ADVANCED_FACE('',(#5797),#483,.T.);
#66548=ADVANCED_FACE('',(#5798),#484,.T.);
#66549=ADVANCED_FACE('',(#5799),#485,.T.);
#66550=ADVANCED_FACE('',(#5800),#4575,.T.);
#66551=ADVANCED_FACE('',(#5801),#486,.T.);
#66552=ADVANCED_FACE('',(#5802),#487,.T.);
#66553=ADVANCED_FACE('',(#5803),#4576,.T.);
#66554=ADVANCED_FACE('',(#5804),#488,.T.);
#66555=ADVANCED_FACE('',(#5805),#489,.T.);
#66556=ADVANCED_FACE('',(#5806),#4577,.T.);
#66557=ADVANCED_FACE('',(#5807),#490,.T.);
#66558=ADVANCED_FACE('',(#5808),#491,.T.);
#66559=ADVANCED_FACE('',(#5809),#4578,.T.);
#66560=ADVANCED_FACE('',(#5810),#492,.T.);
#66561=ADVANCED_FACE('',(#5811),#493,.T.);
#66562=ADVANCED_FACE('',(#5812),#4579,.T.);
#66563=ADVANCED_FACE('',(#5813),#494,.T.);
#66564=ADVANCED_FACE('',(#5814),#495,.T.);
#66565=ADVANCED_FACE('',(#5815),#4580,.T.);
#66566=ADVANCED_FACE('',(#5816),#496,.T.);
#66567=ADVANCED_FACE('',(#5817),#497,.T.);
#66568=ADVANCED_FACE('',(#5818),#4581,.T.);
#66569=ADVANCED_FACE('',(#5819),#498,.T.);
#66570=ADVANCED_FACE('',(#5820),#499,.T.);
#66571=ADVANCED_FACE('',(#5821),#4582,.T.);
#66572=ADVANCED_FACE('',(#5822),#500,.T.);
#66573=ADVANCED_FACE('',(#5823),#501,.T.);
#66574=ADVANCED_FACE('',(#5824),#4583,.T.);
#66575=ADVANCED_FACE('',(#5825),#502,.T.);
#66576=ADVANCED_FACE('',(#5826),#503,.T.);
#66577=ADVANCED_FACE('',(#5827),#4584,.T.);
#66578=ADVANCED_FACE('',(#5828),#504,.T.);
#66579=ADVANCED_FACE('',(#5829),#505,.T.);
#66580=ADVANCED_FACE('',(#5830),#4585,.T.);
#66581=ADVANCED_FACE('',(#5831),#506,.T.);
#66582=ADVANCED_FACE('',(#5832),#507,.T.);
#66583=ADVANCED_FACE('',(#5833),#4586,.T.);
#66584=ADVANCED_FACE('',(#5834),#508,.T.);
#66585=ADVANCED_FACE('',(#5835),#509,.T.);
#66586=ADVANCED_FACE('',(#5836),#4587,.T.);
#66587=ADVANCED_FACE('',(#5837),#510,.T.);
#66588=ADVANCED_FACE('',(#5838),#511,.T.);
#66589=ADVANCED_FACE('',(#5839),#4588,.T.);
#66590=ADVANCED_FACE('',(#5840),#512,.T.);
#66591=ADVANCED_FACE('',(#5841),#513,.T.);
#66592=ADVANCED_FACE('',(#5842),#4589,.T.);
#66593=ADVANCED_FACE('',(#5843),#514,.T.);
#66594=ADVANCED_FACE('',(#5844),#515,.T.);
#66595=ADVANCED_FACE('',(#5845),#4590,.T.);
#66596=ADVANCED_FACE('',(#5846),#516,.T.);
#66597=ADVANCED_FACE('',(#5847),#517,.T.);
#66598=ADVANCED_FACE('',(#5848),#4591,.T.);
#66599=ADVANCED_FACE('',(#5849),#518,.T.);
#66600=ADVANCED_FACE('',(#5850),#519,.T.);
#66601=ADVANCED_FACE('',(#5851),#4592,.T.);
#66602=ADVANCED_FACE('',(#5852),#520,.T.);
#66603=ADVANCED_FACE('',(#5853),#521,.T.);
#66604=ADVANCED_FACE('',(#5854),#4593,.T.);
#66605=ADVANCED_FACE('',(#5855),#522,.T.);
#66606=ADVANCED_FACE('',(#5856),#523,.T.);
#66607=ADVANCED_FACE('',(#5857),#4594,.T.);
#66608=ADVANCED_FACE('',(#5858),#524,.T.);
#66609=ADVANCED_FACE('',(#5859),#525,.T.);
#66610=ADVANCED_FACE('',(#5860),#4595,.T.);
#66611=ADVANCED_FACE('',(#5861),#526,.T.);
#66612=ADVANCED_FACE('',(#5862),#527,.T.);
#66613=ADVANCED_FACE('',(#5863),#528,.T.);
#66614=ADVANCED_FACE('',(#5864),#529,.T.);
#66615=ADVANCED_FACE('',(#5865),#4596,.T.);
#66616=ADVANCED_FACE('',(#5866),#530,.T.);
#66617=ADVANCED_FACE('',(#5867),#531,.T.);
#66618=ADVANCED_FACE('',(#5868),#4597,.T.);
#66619=ADVANCED_FACE('',(#5869),#532,.T.);
#66620=ADVANCED_FACE('',(#5870),#533,.T.);
#66621=ADVANCED_FACE('',(#5871),#4598,.T.);
#66622=ADVANCED_FACE('',(#5872),#534,.T.);
#66623=ADVANCED_FACE('',(#5873),#535,.T.);
#66624=ADVANCED_FACE('',(#5874),#4599,.T.);
#66625=ADVANCED_FACE('',(#5875),#536,.T.);
#66626=ADVANCED_FACE('',(#5876),#537,.T.);
#66627=ADVANCED_FACE('',(#5877),#4600,.T.);
#66628=ADVANCED_FACE('',(#5878),#538,.T.);
#66629=ADVANCED_FACE('',(#5879),#539,.T.);
#66630=ADVANCED_FACE('',(#5880),#4601,.T.);
#66631=ADVANCED_FACE('',(#5881),#540,.T.);
#66632=ADVANCED_FACE('',(#5882),#541,.T.);
#66633=ADVANCED_FACE('',(#5883),#4602,.T.);
#66634=ADVANCED_FACE('',(#5884),#542,.T.);
#66635=ADVANCED_FACE('',(#5885),#543,.T.);
#66636=ADVANCED_FACE('',(#5886),#544,.T.);
#66637=ADVANCED_FACE('',(#5887),#545,.T.);
#66638=ADVANCED_FACE('',(#5888),#546,.T.);
#66639=ADVANCED_FACE('',(#5889),#547,.T.);
#66640=ADVANCED_FACE('',(#5890),#548,.T.);
#66641=ADVANCED_FACE('',(#5891),#549,.T.);
#66642=ADVANCED_FACE('',(#5892),#550,.T.);
#66643=ADVANCED_FACE('',(#5893),#551,.T.);
#66644=ADVANCED_FACE('',(#5894),#552,.T.);
#66645=ADVANCED_FACE('',(#5895),#553,.T.);
#66646=ADVANCED_FACE('',(#5896),#554,.T.);
#66647=ADVANCED_FACE('',(#5897),#555,.T.);
#66648=ADVANCED_FACE('',(#5898),#556,.T.);
#66649=ADVANCED_FACE('',(#5899),#557,.T.);
#66650=ADVANCED_FACE('',(#5900),#558,.T.);
#66651=ADVANCED_FACE('',(#5901),#559,.T.);
#66652=ADVANCED_FACE('',(#5902),#560,.T.);
#66653=ADVANCED_FACE('',(#5903),#561,.T.);
#66654=ADVANCED_FACE('',(#5904),#562,.T.);
#66655=ADVANCED_FACE('',(#5905),#563,.T.);
#66656=ADVANCED_FACE('',(#5906),#564,.T.);
#66657=ADVANCED_FACE('',(#5907),#565,.T.);
#66658=ADVANCED_FACE('',(#5908),#566,.T.);
#66659=ADVANCED_FACE('',(#5909),#567,.T.);
#66660=ADVANCED_FACE('',(#5910),#568,.T.);
#66661=ADVANCED_FACE('',(#5911),#569,.T.);
#66662=ADVANCED_FACE('',(#5912),#570,.T.);
#66663=ADVANCED_FACE('',(#5913),#571,.T.);
#66664=ADVANCED_FACE('',(#5914),#572,.T.);
#66665=ADVANCED_FACE('',(#5915),#573,.T.);
#66666=ADVANCED_FACE('',(#5916),#574,.T.);
#66667=ADVANCED_FACE('',(#5917),#575,.T.);
#66668=ADVANCED_FACE('',(#5918),#576,.T.);
#66669=ADVANCED_FACE('',(#5919),#577,.T.);
#66670=ADVANCED_FACE('',(#5920),#578,.T.);
#66671=ADVANCED_FACE('',(#5921),#579,.T.);
#66672=ADVANCED_FACE('',(#5922),#580,.T.);
#66673=ADVANCED_FACE('',(#5923),#581,.T.);
#66674=ADVANCED_FACE('',(#5924),#582,.T.);
#66675=ADVANCED_FACE('',(#5925),#583,.T.);
#66676=ADVANCED_FACE('',(#5926),#584,.T.);
#66677=ADVANCED_FACE('',(#5927),#585,.T.);
#66678=ADVANCED_FACE('',(#5928),#586,.T.);
#66679=ADVANCED_FACE('',(#5929),#587,.T.);
#66680=ADVANCED_FACE('',(#5930),#588,.T.);
#66681=ADVANCED_FACE('',(#5931),#589,.T.);
#66682=ADVANCED_FACE('',(#5932),#590,.T.);
#66683=ADVANCED_FACE('',(#5933),#591,.T.);
#66684=ADVANCED_FACE('',(#5934),#592,.T.);
#66685=ADVANCED_FACE('',(#5935),#593,.T.);
#66686=ADVANCED_FACE('',(#5936),#594,.T.);
#66687=ADVANCED_FACE('',(#5937),#595,.T.);
#66688=ADVANCED_FACE('',(#5938),#596,.T.);
#66689=ADVANCED_FACE('',(#5939),#597,.T.);
#66690=ADVANCED_FACE('',(#5940),#598,.T.);
#66691=ADVANCED_FACE('',(#5941),#599,.T.);
#66692=ADVANCED_FACE('',(#5942),#600,.T.);
#66693=ADVANCED_FACE('',(#5943),#601,.T.);
#66694=ADVANCED_FACE('',(#5944),#602,.T.);
#66695=ADVANCED_FACE('',(#5945),#603,.T.);
#66696=ADVANCED_FACE('',(#5946),#604,.T.);
#66697=ADVANCED_FACE('',(#5947),#605,.T.);
#66698=ADVANCED_FACE('',(#5948),#606,.T.);
#66699=ADVANCED_FACE('',(#5949),#607,.T.);
#66700=ADVANCED_FACE('',(#5950),#608,.T.);
#66701=ADVANCED_FACE('',(#5951),#609,.T.);
#66702=ADVANCED_FACE('',(#5952),#610,.T.);
#66703=ADVANCED_FACE('',(#5953),#611,.T.);
#66704=ADVANCED_FACE('',(#5954),#612,.T.);
#66705=ADVANCED_FACE('',(#5955),#613,.T.);
#66706=ADVANCED_FACE('',(#5956),#614,.T.);
#66707=ADVANCED_FACE('',(#5957),#615,.T.);
#66708=ADVANCED_FACE('',(#5958),#616,.T.);
#66709=ADVANCED_FACE('',(#5959),#617,.T.);
#66710=ADVANCED_FACE('',(#5960),#618,.T.);
#66711=ADVANCED_FACE('',(#5961),#619,.T.);
#66712=ADVANCED_FACE('',(#5962),#620,.T.);
#66713=ADVANCED_FACE('',(#5963),#621,.T.);
#66714=ADVANCED_FACE('',(#5964),#622,.T.);
#66715=ADVANCED_FACE('',(#5965),#623,.T.);
#66716=ADVANCED_FACE('',(#5966),#624,.T.);
#66717=ADVANCED_FACE('',(#5967),#625,.T.);
#66718=ADVANCED_FACE('',(#5968),#626,.T.);
#66719=ADVANCED_FACE('',(#5969),#627,.T.);
#66720=ADVANCED_FACE('',(#5970),#628,.T.);
#66721=ADVANCED_FACE('',(#5971),#629,.T.);
#66722=ADVANCED_FACE('',(#5972),#630,.T.);
#66723=ADVANCED_FACE('',(#5973),#631,.T.);
#66724=ADVANCED_FACE('',(#5974),#632,.T.);
#66725=ADVANCED_FACE('',(#5975),#633,.T.);
#66726=ADVANCED_FACE('',(#5976),#634,.T.);
#66727=ADVANCED_FACE('',(#5977),#635,.T.);
#66728=ADVANCED_FACE('',(#5978),#636,.T.);
#66729=ADVANCED_FACE('',(#5979),#637,.T.);
#66730=ADVANCED_FACE('',(#5980),#638,.T.);
#66731=ADVANCED_FACE('',(#5981),#639,.T.);
#66732=ADVANCED_FACE('',(#5982),#640,.T.);
#66733=ADVANCED_FACE('',(#5983),#641,.T.);
#66734=ADVANCED_FACE('',(#5984),#642,.T.);
#66735=ADVANCED_FACE('',(#5985),#643,.T.);
#66736=ADVANCED_FACE('',(#5986),#644,.T.);
#66737=ADVANCED_FACE('',(#5987),#645,.T.);
#66738=ADVANCED_FACE('',(#5988),#646,.T.);
#66739=ADVANCED_FACE('',(#5989),#647,.T.);
#66740=ADVANCED_FACE('',(#5990),#648,.T.);
#66741=ADVANCED_FACE('',(#5991),#649,.T.);
#66742=ADVANCED_FACE('',(#5992),#650,.T.);
#66743=ADVANCED_FACE('',(#5993),#651,.T.);
#66744=ADVANCED_FACE('',(#5994),#652,.T.);
#66745=ADVANCED_FACE('',(#5995),#653,.T.);
#66746=ADVANCED_FACE('',(#5996),#654,.T.);
#66747=ADVANCED_FACE('',(#5997),#655,.T.);
#66748=ADVANCED_FACE('',(#5998),#656,.T.);
#66749=ADVANCED_FACE('',(#5999),#657,.T.);
#66750=ADVANCED_FACE('',(#6000),#658,.T.);
#66751=ADVANCED_FACE('',(#6001),#659,.T.);
#66752=ADVANCED_FACE('',(#6002),#4603,.T.);
#66753=ADVANCED_FACE('',(#6003),#660,.T.);
#66754=ADVANCED_FACE('',(#6004),#661,.T.);
#66755=ADVANCED_FACE('',(#6005),#4604,.T.);
#66756=ADVANCED_FACE('',(#6006),#662,.T.);
#66757=ADVANCED_FACE('',(#6007),#663,.T.);
#66758=ADVANCED_FACE('',(#6008),#4605,.T.);
#66759=ADVANCED_FACE('',(#6009),#664,.T.);
#66760=ADVANCED_FACE('',(#6010),#665,.T.);
#66761=ADVANCED_FACE('',(#6011),#4606,.T.);
#66762=ADVANCED_FACE('',(#6012),#666,.T.);
#66763=ADVANCED_FACE('',(#6013),#667,.T.);
#66764=ADVANCED_FACE('',(#6014),#4607,.T.);
#66765=ADVANCED_FACE('',(#6015),#668,.T.);
#66766=ADVANCED_FACE('',(#6016),#669,.T.);
#66767=ADVANCED_FACE('',(#6017),#4608,.T.);
#66768=ADVANCED_FACE('',(#6018),#670,.T.);
#66769=ADVANCED_FACE('',(#6019),#671,.T.);
#66770=ADVANCED_FACE('',(#6020),#672,.T.);
#66771=ADVANCED_FACE('',(#6021),#673,.T.);
#66772=ADVANCED_FACE('',(#6022),#4609,.T.);
#66773=ADVANCED_FACE('',(#6023),#674,.T.);
#66774=ADVANCED_FACE('',(#6024),#675,.T.);
#66775=ADVANCED_FACE('',(#6025),#4610,.T.);
#66776=ADVANCED_FACE('',(#6026),#676,.T.);
#66777=ADVANCED_FACE('',(#6027),#677,.T.);
#66778=ADVANCED_FACE('',(#6028),#4611,.T.);
#66779=ADVANCED_FACE('',(#6029),#678,.T.);
#66780=ADVANCED_FACE('',(#6030),#679,.T.);
#66781=ADVANCED_FACE('',(#6031),#4612,.T.);
#66782=ADVANCED_FACE('',(#6032),#680,.T.);
#66783=ADVANCED_FACE('',(#6033),#681,.T.);
#66784=ADVANCED_FACE('',(#6034),#4613,.T.);
#66785=ADVANCED_FACE('',(#6035),#682,.T.);
#66786=ADVANCED_FACE('',(#6036),#683,.T.);
#66787=ADVANCED_FACE('',(#6037),#4614,.T.);
#66788=ADVANCED_FACE('',(#6038),#684,.T.);
#66789=ADVANCED_FACE('',(#6039),#685,.T.);
#66790=ADVANCED_FACE('',(#6040),#4615,.T.);
#66791=ADVANCED_FACE('',(#6041),#686,.T.);
#66792=ADVANCED_FACE('',(#6042),#687,.T.);
#66793=ADVANCED_FACE('',(#6043),#4616,.T.);
#66794=ADVANCED_FACE('',(#6044),#688,.T.);
#66795=ADVANCED_FACE('',(#6045),#689,.T.);
#66796=ADVANCED_FACE('',(#6046),#4617,.T.);
#66797=ADVANCED_FACE('',(#6047),#690,.T.);
#66798=ADVANCED_FACE('',(#6048),#691,.T.);
#66799=ADVANCED_FACE('',(#6049),#4618,.T.);
#66800=ADVANCED_FACE('',(#6050),#692,.T.);
#66801=ADVANCED_FACE('',(#6051),#693,.T.);
#66802=ADVANCED_FACE('',(#6052),#4619,.T.);
#66803=ADVANCED_FACE('',(#6053),#694,.T.);
#66804=ADVANCED_FACE('',(#6054),#695,.T.);
#66805=ADVANCED_FACE('',(#6055),#4620,.T.);
#66806=ADVANCED_FACE('',(#6056),#696,.T.);
#66807=ADVANCED_FACE('',(#6057),#697,.T.);
#66808=ADVANCED_FACE('',(#6058),#4621,.T.);
#66809=ADVANCED_FACE('',(#6059),#698,.T.);
#66810=ADVANCED_FACE('',(#6060),#699,.T.);
#66811=ADVANCED_FACE('',(#6061),#4622,.T.);
#66812=ADVANCED_FACE('',(#6062),#700,.T.);
#66813=ADVANCED_FACE('',(#6063),#701,.T.);
#66814=ADVANCED_FACE('',(#6064),#4623,.T.);
#66815=ADVANCED_FACE('',(#6065),#702,.T.);
#66816=ADVANCED_FACE('',(#6066),#703,.T.);
#66817=ADVANCED_FACE('',(#6067),#4624,.T.);
#66818=ADVANCED_FACE('',(#6068),#704,.T.);
#66819=ADVANCED_FACE('',(#6069),#705,.T.);
#66820=ADVANCED_FACE('',(#6070),#706,.T.);
#66821=ADVANCED_FACE('',(#6071),#4625,.T.);
#66822=ADVANCED_FACE('',(#6072),#707,.T.);
#66823=ADVANCED_FACE('',(#6073),#4626,.T.);
#66824=ADVANCED_FACE('',(#6074),#708,.T.);
#66825=ADVANCED_FACE('',(#6075),#709,.T.);
#66826=ADVANCED_FACE('',(#6076),#4627,.T.);
#66827=ADVANCED_FACE('',(#6077),#710,.T.);
#66828=ADVANCED_FACE('',(#6078),#711,.T.);
#66829=ADVANCED_FACE('',(#6079),#4628,.T.);
#66830=ADVANCED_FACE('',(#6080),#712,.T.);
#66831=ADVANCED_FACE('',(#6081),#713,.T.);
#66832=ADVANCED_FACE('',(#6082),#4629,.T.);
#66833=ADVANCED_FACE('',(#6083),#714,.T.);
#66834=ADVANCED_FACE('',(#6084),#4630,.T.);
#66835=ADVANCED_FACE('',(#6085),#715,.T.);
#66836=ADVANCED_FACE('',(#6086),#716,.T.);
#66837=ADVANCED_FACE('',(#6087),#717,.T.);
#66838=ADVANCED_FACE('',(#6088),#718,.T.);
#66839=ADVANCED_FACE('',(#6089),#4631,.T.);
#66840=ADVANCED_FACE('',(#6090),#719,.T.);
#66841=ADVANCED_FACE('',(#6091),#720,.T.);
#66842=ADVANCED_FACE('',(#6092),#4632,.T.);
#66843=ADVANCED_FACE('',(#6093),#721,.T.);
#66844=ADVANCED_FACE('',(#6094),#722,.T.);
#66845=ADVANCED_FACE('',(#6095),#4633,.T.);
#66846=ADVANCED_FACE('',(#6096),#723,.T.);
#66847=ADVANCED_FACE('',(#6097),#724,.T.);
#66848=ADVANCED_FACE('',(#6098),#4634,.T.);
#66849=ADVANCED_FACE('',(#6099),#725,.T.);
#66850=ADVANCED_FACE('',(#6100),#726,.T.);
#66851=ADVANCED_FACE('',(#6101),#4635,.T.);
#66852=ADVANCED_FACE('',(#6102),#727,.T.);
#66853=ADVANCED_FACE('',(#6103),#728,.T.);
#66854=ADVANCED_FACE('',(#6104),#4636,.T.);
#66855=ADVANCED_FACE('',(#6105),#729,.T.);
#66856=ADVANCED_FACE('',(#6106),#730,.T.);
#66857=ADVANCED_FACE('',(#6107),#4637,.T.);
#66858=ADVANCED_FACE('',(#6108),#731,.T.);
#66859=ADVANCED_FACE('',(#6109),#732,.T.);
#66860=ADVANCED_FACE('',(#6110),#4638,.T.);
#66861=ADVANCED_FACE('',(#6111),#733,.T.);
#66862=ADVANCED_FACE('',(#6112),#734,.T.);
#66863=ADVANCED_FACE('',(#6113),#4639,.T.);
#66864=ADVANCED_FACE('',(#6114),#735,.T.);
#66865=ADVANCED_FACE('',(#6115),#736,.T.);
#66866=ADVANCED_FACE('',(#6116),#4640,.T.);
#66867=ADVANCED_FACE('',(#6117),#737,.T.);
#66868=ADVANCED_FACE('',(#6118),#738,.T.);
#66869=ADVANCED_FACE('',(#6119),#4641,.T.);
#66870=ADVANCED_FACE('',(#6120),#739,.T.);
#66871=ADVANCED_FACE('',(#6121),#740,.T.);
#66872=ADVANCED_FACE('',(#6122),#4642,.T.);
#66873=ADVANCED_FACE('',(#6123),#741,.T.);
#66874=ADVANCED_FACE('',(#6124),#742,.T.);
#66875=ADVANCED_FACE('',(#6125),#4643,.T.);
#66876=ADVANCED_FACE('',(#6126),#743,.T.);
#66877=ADVANCED_FACE('',(#6127),#744,.T.);
#66878=ADVANCED_FACE('',(#6128),#745,.T.);
#66879=ADVANCED_FACE('',(#6129),#746,.T.);
#66880=ADVANCED_FACE('',(#6130),#4644,.T.);
#66881=ADVANCED_FACE('',(#6131),#747,.T.);
#66882=ADVANCED_FACE('',(#6132),#748,.T.);
#66883=ADVANCED_FACE('',(#6133),#4645,.T.);
#66884=ADVANCED_FACE('',(#6134),#749,.T.);
#66885=ADVANCED_FACE('',(#6135),#750,.T.);
#66886=ADVANCED_FACE('',(#6136),#4646,.T.);
#66887=ADVANCED_FACE('',(#6137),#751,.T.);
#66888=ADVANCED_FACE('',(#6138),#752,.T.);
#66889=ADVANCED_FACE('',(#6139),#4647,.T.);
#66890=ADVANCED_FACE('',(#6140),#753,.T.);
#66891=ADVANCED_FACE('',(#6141),#754,.T.);
#66892=ADVANCED_FACE('',(#6142),#4648,.T.);
#66893=ADVANCED_FACE('',(#6143),#755,.T.);
#66894=ADVANCED_FACE('',(#6144),#756,.T.);
#66895=ADVANCED_FACE('',(#6145),#4649,.T.);
#66896=ADVANCED_FACE('',(#6146),#757,.T.);
#66897=ADVANCED_FACE('',(#6147),#758,.T.);
#66898=ADVANCED_FACE('',(#6148),#4650,.T.);
#66899=ADVANCED_FACE('',(#6149),#759,.T.);
#66900=ADVANCED_FACE('',(#6150),#760,.T.);
#66901=ADVANCED_FACE('',(#6151),#4651,.T.);
#66902=ADVANCED_FACE('',(#6152),#761,.T.);
#66903=ADVANCED_FACE('',(#6153),#762,.T.);
#66904=ADVANCED_FACE('',(#6154),#4652,.T.);
#66905=ADVANCED_FACE('',(#6155),#763,.T.);
#66906=ADVANCED_FACE('',(#6156),#764,.T.);
#66907=ADVANCED_FACE('',(#6157),#4653,.T.);
#66908=ADVANCED_FACE('',(#6158),#765,.T.);
#66909=ADVANCED_FACE('',(#6159),#766,.T.);
#66910=ADVANCED_FACE('',(#6160),#4654,.T.);
#66911=ADVANCED_FACE('',(#6161),#767,.T.);
#66912=ADVANCED_FACE('',(#6162),#768,.T.);
#66913=ADVANCED_FACE('',(#6163),#4655,.T.);
#66914=ADVANCED_FACE('',(#6164),#769,.T.);
#66915=ADVANCED_FACE('',(#6165),#770,.T.);
#66916=ADVANCED_FACE('',(#6166),#4656,.T.);
#66917=ADVANCED_FACE('',(#6167),#771,.T.);
#66918=ADVANCED_FACE('',(#6168),#772,.T.);
#66919=ADVANCED_FACE('',(#6169),#4657,.T.);
#66920=ADVANCED_FACE('',(#6170),#4658,.T.);
#66921=ADVANCED_FACE('',(#6171),#773,.T.);
#66922=ADVANCED_FACE('',(#6172),#774,.T.);
#66923=ADVANCED_FACE('',(#6173),#775,.T.);
#66924=ADVANCED_FACE('',(#6174),#776,.T.);
#66925=ADVANCED_FACE('',(#6175),#777,.T.);
#66926=ADVANCED_FACE('',(#6176),#778,.T.);
#66927=ADVANCED_FACE('',(#6177),#779,.T.);
#66928=ADVANCED_FACE('',(#6178),#780,.T.);
#66929=ADVANCED_FACE('',(#6179),#781,.T.);
#66930=ADVANCED_FACE('',(#6180),#782,.T.);
#66931=ADVANCED_FACE('',(#6181),#783,.T.);
#66932=ADVANCED_FACE('',(#6182),#784,.T.);
#66933=ADVANCED_FACE('',(#6183),#785,.T.);
#66934=ADVANCED_FACE('',(#6184),#786,.T.);
#66935=ADVANCED_FACE('',(#6185),#787,.T.);
#66936=ADVANCED_FACE('',(#6186),#788,.T.);
#66937=ADVANCED_FACE('',(#6187),#789,.T.);
#66938=ADVANCED_FACE('',(#6188),#790,.T.);
#66939=ADVANCED_FACE('',(#6189),#791,.T.);
#66940=ADVANCED_FACE('',(#6190),#792,.T.);
#66941=ADVANCED_FACE('',(#6191),#793,.T.);
#66942=ADVANCED_FACE('',(#6192),#794,.T.);
#66943=ADVANCED_FACE('',(#6193),#795,.T.);
#66944=ADVANCED_FACE('',(#6194),#796,.T.);
#66945=ADVANCED_FACE('',(#6195),#797,.T.);
#66946=ADVANCED_FACE('',(#6196),#798,.T.);
#66947=ADVANCED_FACE('',(#6197),#799,.T.);
#66948=ADVANCED_FACE('',(#6198),#800,.T.);
#66949=ADVANCED_FACE('',(#6199),#801,.T.);
#66950=ADVANCED_FACE('',(#6200),#802,.T.);
#66951=ADVANCED_FACE('',(#6201),#803,.T.);
#66952=ADVANCED_FACE('',(#6202),#804,.T.);
#66953=ADVANCED_FACE('',(#6203),#805,.T.);
#66954=ADVANCED_FACE('',(#6204),#806,.T.);
#66955=ADVANCED_FACE('',(#6205),#807,.T.);
#66956=ADVANCED_FACE('',(#6206),#808,.T.);
#66957=ADVANCED_FACE('',(#6207),#809,.T.);
#66958=ADVANCED_FACE('',(#6208),#810,.T.);
#66959=ADVANCED_FACE('',(#6209),#811,.T.);
#66960=ADVANCED_FACE('',(#6210),#812,.T.);
#66961=ADVANCED_FACE('',(#6211),#813,.T.);
#66962=ADVANCED_FACE('',(#6212),#814,.T.);
#66963=ADVANCED_FACE('',(#6213),#815,.T.);
#66964=ADVANCED_FACE('',(#6214),#816,.T.);
#66965=ADVANCED_FACE('',(#6215),#817,.T.);
#66966=ADVANCED_FACE('',(#6216),#818,.T.);
#66967=ADVANCED_FACE('',(#6217),#819,.T.);
#66968=ADVANCED_FACE('',(#6218),#820,.T.);
#66969=ADVANCED_FACE('',(#6219),#821,.T.);
#66970=ADVANCED_FACE('',(#6220),#822,.T.);
#66971=ADVANCED_FACE('',(#6221),#823,.T.);
#66972=ADVANCED_FACE('',(#6222),#824,.T.);
#66973=ADVANCED_FACE('',(#6223),#825,.T.);
#66974=ADVANCED_FACE('',(#6224),#826,.T.);
#66975=ADVANCED_FACE('',(#6225),#827,.T.);
#66976=ADVANCED_FACE('',(#6226),#828,.T.);
#66977=ADVANCED_FACE('',(#6227),#829,.T.);
#66978=ADVANCED_FACE('',(#6228),#830,.T.);
#66979=ADVANCED_FACE('',(#6229),#831,.T.);
#66980=ADVANCED_FACE('',(#6230),#832,.T.);
#66981=ADVANCED_FACE('',(#6231),#833,.T.);
#66982=ADVANCED_FACE('',(#6232),#834,.T.);
#66983=ADVANCED_FACE('',(#6233),#835,.T.);
#66984=ADVANCED_FACE('',(#6234),#836,.T.);
#66985=ADVANCED_FACE('',(#6235),#837,.T.);
#66986=ADVANCED_FACE('',(#6236),#838,.T.);
#66987=ADVANCED_FACE('',(#6237),#839,.T.);
#66988=ADVANCED_FACE('',(#6238),#840,.T.);
#66989=ADVANCED_FACE('',(#6239),#841,.T.);
#66990=ADVANCED_FACE('',(#6240),#842,.T.);
#66991=ADVANCED_FACE('',(#6241),#843,.T.);
#66992=ADVANCED_FACE('',(#6242),#844,.T.);
#66993=ADVANCED_FACE('',(#6243),#845,.T.);
#66994=ADVANCED_FACE('',(#6244),#846,.T.);
#66995=ADVANCED_FACE('',(#6245),#847,.T.);
#66996=ADVANCED_FACE('',(#6246),#848,.T.);
#66997=ADVANCED_FACE('',(#6247),#849,.T.);
#66998=ADVANCED_FACE('',(#6248),#850,.T.);
#66999=ADVANCED_FACE('',(#6249),#851,.T.);
#67000=ADVANCED_FACE('',(#6250),#852,.T.);
#67001=ADVANCED_FACE('',(#6251),#853,.T.);
#67002=ADVANCED_FACE('',(#6252),#854,.T.);
#67003=ADVANCED_FACE('',(#6253),#855,.T.);
#67004=ADVANCED_FACE('',(#6254),#856,.T.);
#67005=ADVANCED_FACE('',(#6255),#857,.T.);
#67006=ADVANCED_FACE('',(#6256),#858,.T.);
#67007=ADVANCED_FACE('',(#6257),#859,.T.);
#67008=ADVANCED_FACE('',(#6258),#860,.T.);
#67009=ADVANCED_FACE('',(#6259),#861,.T.);
#67010=ADVANCED_FACE('',(#6260),#862,.T.);
#67011=ADVANCED_FACE('',(#6261),#863,.T.);
#67012=ADVANCED_FACE('',(#6262),#864,.T.);
#67013=ADVANCED_FACE('',(#6263),#865,.T.);
#67014=ADVANCED_FACE('',(#6264),#866,.T.);
#67015=ADVANCED_FACE('',(#6265),#867,.T.);
#67016=ADVANCED_FACE('',(#6266),#868,.T.);
#67017=ADVANCED_FACE('',(#6267),#869,.T.);
#67018=ADVANCED_FACE('',(#6268),#870,.T.);
#67019=ADVANCED_FACE('',(#6269),#871,.T.);
#67020=ADVANCED_FACE('',(#6270),#872,.T.);
#67021=ADVANCED_FACE('',(#6271),#873,.T.);
#67022=ADVANCED_FACE('',(#6272),#874,.T.);
#67023=ADVANCED_FACE('',(#6273),#875,.T.);
#67024=ADVANCED_FACE('',(#6274),#876,.T.);
#67025=ADVANCED_FACE('',(#6275),#877,.T.);
#67026=ADVANCED_FACE('',(#6276),#878,.T.);
#67027=ADVANCED_FACE('',(#6277),#879,.T.);
#67028=ADVANCED_FACE('',(#6278),#880,.T.);
#67029=ADVANCED_FACE('',(#6279),#881,.T.);
#67030=ADVANCED_FACE('',(#6280),#882,.T.);
#67031=ADVANCED_FACE('',(#6281),#883,.T.);
#67032=ADVANCED_FACE('',(#6282),#884,.T.);
#67033=ADVANCED_FACE('',(#6283),#885,.T.);
#67034=ADVANCED_FACE('',(#6284),#886,.T.);
#67035=ADVANCED_FACE('',(#6285),#887,.T.);
#67036=ADVANCED_FACE('',(#6286),#888,.T.);
#67037=ADVANCED_FACE('',(#6287),#889,.T.);
#67038=ADVANCED_FACE('',(#6288),#890,.T.);
#67039=ADVANCED_FACE('',(#6289),#4659,.T.);
#67040=ADVANCED_FACE('',(#6290),#891,.T.);
#67041=ADVANCED_FACE('',(#6291),#892,.T.);
#67042=ADVANCED_FACE('',(#6292),#4660,.T.);
#67043=ADVANCED_FACE('',(#6293),#893,.T.);
#67044=ADVANCED_FACE('',(#6294),#894,.T.);
#67045=ADVANCED_FACE('',(#6295),#4661,.T.);
#67046=ADVANCED_FACE('',(#6296),#895,.T.);
#67047=ADVANCED_FACE('',(#6297),#896,.T.);
#67048=ADVANCED_FACE('',(#6298),#4662,.T.);
#67049=ADVANCED_FACE('',(#6299),#897,.T.);
#67050=ADVANCED_FACE('',(#6300),#898,.T.);
#67051=ADVANCED_FACE('',(#6301),#4663,.T.);
#67052=ADVANCED_FACE('',(#6302),#899,.T.);
#67053=ADVANCED_FACE('',(#6303),#900,.T.);
#67054=ADVANCED_FACE('',(#6304),#4664,.T.);
#67055=ADVANCED_FACE('',(#6305),#901,.T.);
#67056=ADVANCED_FACE('',(#6306),#902,.T.);
#67057=ADVANCED_FACE('',(#6307),#4665,.T.);
#67058=ADVANCED_FACE('',(#6308),#903,.T.);
#67059=ADVANCED_FACE('',(#6309),#904,.T.);
#67060=ADVANCED_FACE('',(#6310),#4666,.T.);
#67061=ADVANCED_FACE('',(#6311),#905,.T.);
#67062=ADVANCED_FACE('',(#6312),#906,.T.);
#67063=ADVANCED_FACE('',(#6313),#4667,.T.);
#67064=ADVANCED_FACE('',(#6314),#907,.T.);
#67065=ADVANCED_FACE('',(#6315),#908,.T.);
#67066=ADVANCED_FACE('',(#6316),#4668,.T.);
#67067=ADVANCED_FACE('',(#6317),#909,.T.);
#67068=ADVANCED_FACE('',(#6318),#910,.T.);
#67069=ADVANCED_FACE('',(#6319),#4669,.T.);
#67070=ADVANCED_FACE('',(#6320),#911,.T.);
#67071=ADVANCED_FACE('',(#6321),#912,.T.);
#67072=ADVANCED_FACE('',(#6322),#4670,.T.);
#67073=ADVANCED_FACE('',(#6323),#913,.T.);
#67074=ADVANCED_FACE('',(#6324),#914,.T.);
#67075=ADVANCED_FACE('',(#6325),#4671,.T.);
#67076=ADVANCED_FACE('',(#6326),#915,.T.);
#67077=ADVANCED_FACE('',(#6327),#916,.T.);
#67078=ADVANCED_FACE('',(#6328),#4672,.T.);
#67079=ADVANCED_FACE('',(#6329),#917,.T.);
#67080=ADVANCED_FACE('',(#6330),#918,.T.);
#67081=ADVANCED_FACE('',(#6331),#919,.T.);
#67082=ADVANCED_FACE('',(#6332),#920,.T.);
#67083=ADVANCED_FACE('',(#6333),#4673,.T.);
#67084=ADVANCED_FACE('',(#6334),#921,.T.);
#67085=ADVANCED_FACE('',(#6335),#922,.T.);
#67086=ADVANCED_FACE('',(#6336),#4674,.T.);
#67087=ADVANCED_FACE('',(#6337),#923,.T.);
#67088=ADVANCED_FACE('',(#6338),#924,.T.);
#67089=ADVANCED_FACE('',(#6339),#4675,.T.);
#67090=ADVANCED_FACE('',(#6340),#925,.T.);
#67091=ADVANCED_FACE('',(#6341),#926,.T.);
#67092=ADVANCED_FACE('',(#6342),#4676,.T.);
#67093=ADVANCED_FACE('',(#6343),#927,.T.);
#67094=ADVANCED_FACE('',(#6344),#928,.T.);
#67095=ADVANCED_FACE('',(#6345),#4677,.T.);
#67096=ADVANCED_FACE('',(#6346),#929,.T.);
#67097=ADVANCED_FACE('',(#6347),#930,.T.);
#67098=ADVANCED_FACE('',(#6348),#4678,.T.);
#67099=ADVANCED_FACE('',(#6349),#931,.T.);
#67100=ADVANCED_FACE('',(#6350),#932,.T.);
#67101=ADVANCED_FACE('',(#6351),#4679,.T.);
#67102=ADVANCED_FACE('',(#6352),#933,.T.);
#67103=ADVANCED_FACE('',(#6353),#934,.T.);
#67104=ADVANCED_FACE('',(#6354),#4680,.T.);
#67105=ADVANCED_FACE('',(#6355),#935,.T.);
#67106=ADVANCED_FACE('',(#6356),#936,.T.);
#67107=ADVANCED_FACE('',(#6357),#937,.T.);
#67108=ADVANCED_FACE('',(#6358),#4681,.T.);
#67109=ADVANCED_FACE('',(#6359),#938,.T.);
#67110=ADVANCED_FACE('',(#6360),#4682,.T.);
#67111=ADVANCED_FACE('',(#6361),#939,.T.);
#67112=ADVANCED_FACE('',(#6362),#940,.T.);
#67113=ADVANCED_FACE('',(#6363),#4683,.T.);
#67114=ADVANCED_FACE('',(#6364),#941,.T.);
#67115=ADVANCED_FACE('',(#6365),#942,.T.);
#67116=ADVANCED_FACE('',(#6366),#4684,.T.);
#67117=ADVANCED_FACE('',(#6367),#943,.T.);
#67118=ADVANCED_FACE('',(#6368),#944,.T.);
#67119=ADVANCED_FACE('',(#6369),#4685,.T.);
#67120=ADVANCED_FACE('',(#6370),#945,.T.);
#67121=ADVANCED_FACE('',(#6371),#946,.T.);
#67122=ADVANCED_FACE('',(#6372),#4686,.T.);
#67123=ADVANCED_FACE('',(#6373),#947,.T.);
#67124=ADVANCED_FACE('',(#6374),#948,.T.);
#67125=ADVANCED_FACE('',(#6375),#949,.T.);
#67126=ADVANCED_FACE('',(#6376),#4687,.T.);
#67127=ADVANCED_FACE('',(#6377),#950,.T.);
#67128=ADVANCED_FACE('',(#6378),#951,.T.);
#67129=ADVANCED_FACE('',(#6379),#4688,.T.);
#67130=ADVANCED_FACE('',(#6380),#952,.T.);
#67131=ADVANCED_FACE('',(#6381),#953,.T.);
#67132=ADVANCED_FACE('',(#6382),#4689,.T.);
#67133=ADVANCED_FACE('',(#6383),#954,.T.);
#67134=ADVANCED_FACE('',(#6384),#955,.T.);
#67135=ADVANCED_FACE('',(#6385),#4690,.T.);
#67136=ADVANCED_FACE('',(#6386),#956,.T.);
#67137=ADVANCED_FACE('',(#6387),#957,.T.);
#67138=ADVANCED_FACE('',(#6388),#4691,.T.);
#67139=ADVANCED_FACE('',(#6389),#958,.T.);
#67140=ADVANCED_FACE('',(#6390),#959,.T.);
#67141=ADVANCED_FACE('',(#6391),#4692,.T.);
#67142=ADVANCED_FACE('',(#6392),#960,.T.);
#67143=ADVANCED_FACE('',(#6393),#961,.T.);
#67144=ADVANCED_FACE('',(#6394),#4693,.T.);
#67145=ADVANCED_FACE('',(#6395),#962,.T.);
#67146=ADVANCED_FACE('',(#6396),#963,.T.);
#67147=ADVANCED_FACE('',(#6397),#4694,.T.);
#67148=ADVANCED_FACE('',(#6398),#964,.T.);
#67149=ADVANCED_FACE('',(#6399),#965,.T.);
#67150=ADVANCED_FACE('',(#6400),#4695,.T.);
#67151=ADVANCED_FACE('',(#6401),#966,.T.);
#67152=ADVANCED_FACE('',(#6402),#967,.T.);
#67153=ADVANCED_FACE('',(#6403),#4696,.T.);
#67154=ADVANCED_FACE('',(#6404),#968,.T.);
#67155=ADVANCED_FACE('',(#6405),#969,.T.);
#67156=ADVANCED_FACE('',(#6406),#4697,.T.);
#67157=ADVANCED_FACE('',(#6407),#970,.T.);
#67158=ADVANCED_FACE('',(#6408),#971,.T.);
#67159=ADVANCED_FACE('',(#6409),#4698,.T.);
#67160=ADVANCED_FACE('',(#6410),#972,.T.);
#67161=ADVANCED_FACE('',(#6411),#973,.T.);
#67162=ADVANCED_FACE('',(#6412),#4699,.T.);
#67163=ADVANCED_FACE('',(#6413),#974,.T.);
#67164=ADVANCED_FACE('',(#6414),#975,.T.);
#67165=ADVANCED_FACE('',(#6415),#4700,.T.);
#67166=ADVANCED_FACE('',(#6416),#976,.T.);
#67167=ADVANCED_FACE('',(#6417),#977,.T.);
#67168=ADVANCED_FACE('',(#6418),#4701,.T.);
#67169=ADVANCED_FACE('',(#6419),#978,.T.);
#67170=ADVANCED_FACE('',(#6420),#979,.T.);
#67171=ADVANCED_FACE('',(#6421),#4702,.T.);
#67172=ADVANCED_FACE('',(#6422),#980,.T.);
#67173=ADVANCED_FACE('',(#6423),#981,.T.);
#67174=ADVANCED_FACE('',(#6424),#4703,.T.);
#67175=ADVANCED_FACE('',(#6425),#982,.T.);
#67176=ADVANCED_FACE('',(#6426),#983,.T.);
#67177=ADVANCED_FACE('',(#6427),#4704,.T.);
#67178=ADVANCED_FACE('',(#6428),#984,.T.);
#67179=ADVANCED_FACE('',(#6429),#985,.T.);
#67180=ADVANCED_FACE('',(#6430),#4705,.T.);
#67181=ADVANCED_FACE('',(#6431),#986,.T.);
#67182=ADVANCED_FACE('',(#6432),#987,.T.);
#67183=ADVANCED_FACE('',(#6433),#4706,.T.);
#67184=ADVANCED_FACE('',(#6434),#988,.T.);
#67185=ADVANCED_FACE('',(#6435),#989,.T.);
#67186=ADVANCED_FACE('',(#6436),#4707,.T.);
#67187=ADVANCED_FACE('',(#6437),#990,.T.);
#67188=ADVANCED_FACE('',(#6438),#991,.T.);
#67189=ADVANCED_FACE('',(#6439),#4708,.T.);
#67190=ADVANCED_FACE('',(#6440),#992,.T.);
#67191=ADVANCED_FACE('',(#6441),#993,.T.);
#67192=ADVANCED_FACE('',(#6442),#4709,.T.);
#67193=ADVANCED_FACE('',(#6443),#994,.T.);
#67194=ADVANCED_FACE('',(#6444),#995,.T.);
#67195=ADVANCED_FACE('',(#6445),#4710,.T.);
#67196=ADVANCED_FACE('',(#6446),#996,.T.);
#67197=ADVANCED_FACE('',(#6447),#997,.T.);
#67198=ADVANCED_FACE('',(#6448),#4711,.T.);
#67199=ADVANCED_FACE('',(#6449),#998,.T.);
#67200=ADVANCED_FACE('',(#6450),#999,.T.);
#67201=ADVANCED_FACE('',(#6451),#4712,.T.);
#67202=ADVANCED_FACE('',(#6452),#1000,.T.);
#67203=ADVANCED_FACE('',(#6453),#1001,.T.);
#67204=ADVANCED_FACE('',(#6454),#4713,.T.);
#67205=ADVANCED_FACE('',(#6455),#1002,.T.);
#67206=ADVANCED_FACE('',(#6456),#1003,.T.);
#67207=ADVANCED_FACE('',(#6457),#4714,.T.);
#67208=ADVANCED_FACE('',(#6458),#1004,.T.);
#67209=ADVANCED_FACE('',(#6459),#1005,.T.);
#67210=ADVANCED_FACE('',(#6460),#4715,.T.);
#67211=ADVANCED_FACE('',(#6461),#1006,.T.);
#67212=ADVANCED_FACE('',(#6462),#1007,.T.);
#67213=ADVANCED_FACE('',(#6463),#1008,.T.);
#67214=ADVANCED_FACE('',(#6464),#1009,.T.);
#67215=ADVANCED_FACE('',(#6465),#1010,.T.);
#67216=ADVANCED_FACE('',(#6466),#1011,.T.);
#67217=ADVANCED_FACE('',(#6467),#1012,.T.);
#67218=ADVANCED_FACE('',(#6468),#1013,.T.);
#67219=ADVANCED_FACE('',(#6469),#1014,.T.);
#67220=ADVANCED_FACE('',(#6470),#1015,.T.);
#67221=ADVANCED_FACE('',(#6471),#1016,.T.);
#67222=ADVANCED_FACE('',(#6472),#1017,.T.);
#67223=ADVANCED_FACE('',(#6473),#1018,.T.);
#67224=ADVANCED_FACE('',(#6474),#1019,.T.);
#67225=ADVANCED_FACE('',(#6475),#1020,.T.);
#67226=ADVANCED_FACE('',(#6476),#1021,.T.);
#67227=ADVANCED_FACE('',(#6477),#1022,.T.);
#67228=ADVANCED_FACE('',(#6478),#1023,.T.);
#67229=ADVANCED_FACE('',(#6479),#1024,.T.);
#67230=ADVANCED_FACE('',(#6480),#1025,.T.);
#67231=ADVANCED_FACE('',(#6481),#1026,.T.);
#67232=ADVANCED_FACE('',(#6482),#1027,.T.);
#67233=ADVANCED_FACE('',(#6483),#1028,.T.);
#67234=ADVANCED_FACE('',(#6484),#1029,.T.);
#67235=ADVANCED_FACE('',(#6485),#1030,.T.);
#67236=ADVANCED_FACE('',(#6486),#1031,.T.);
#67237=ADVANCED_FACE('',(#6487),#1032,.T.);
#67238=ADVANCED_FACE('',(#6488),#1033,.T.);
#67239=ADVANCED_FACE('',(#6489),#1034,.T.);
#67240=ADVANCED_FACE('',(#6490),#1035,.T.);
#67241=ADVANCED_FACE('',(#6491),#1036,.T.);
#67242=ADVANCED_FACE('',(#6492),#1037,.T.);
#67243=ADVANCED_FACE('',(#6493),#1038,.T.);
#67244=ADVANCED_FACE('',(#6494),#1039,.T.);
#67245=ADVANCED_FACE('',(#6495),#1040,.T.);
#67246=ADVANCED_FACE('',(#6496),#1041,.T.);
#67247=ADVANCED_FACE('',(#6497),#1042,.T.);
#67248=ADVANCED_FACE('',(#6498),#1043,.T.);
#67249=ADVANCED_FACE('',(#6499),#1044,.T.);
#67250=ADVANCED_FACE('',(#6500),#1045,.T.);
#67251=ADVANCED_FACE('',(#6501),#1046,.T.);
#67252=ADVANCED_FACE('',(#6502),#1047,.T.);
#67253=ADVANCED_FACE('',(#6503),#1048,.T.);
#67254=ADVANCED_FACE('',(#6504),#1049,.T.);
#67255=ADVANCED_FACE('',(#6505),#1050,.T.);
#67256=ADVANCED_FACE('',(#6506),#1051,.T.);
#67257=ADVANCED_FACE('',(#6507),#1052,.T.);
#67258=ADVANCED_FACE('',(#6508),#1053,.T.);
#67259=ADVANCED_FACE('',(#6509),#1054,.T.);
#67260=ADVANCED_FACE('',(#6510),#1055,.T.);
#67261=ADVANCED_FACE('',(#6511),#1056,.T.);
#67262=ADVANCED_FACE('',(#6512),#1057,.T.);
#67263=ADVANCED_FACE('',(#6513),#1058,.T.);
#67264=ADVANCED_FACE('',(#6514),#1059,.T.);
#67265=ADVANCED_FACE('',(#6515),#1060,.T.);
#67266=ADVANCED_FACE('',(#6516),#1061,.T.);
#67267=ADVANCED_FACE('',(#6517),#1062,.T.);
#67268=ADVANCED_FACE('',(#6518),#1063,.T.);
#67269=ADVANCED_FACE('',(#6519),#1064,.T.);
#67270=ADVANCED_FACE('',(#6520),#1065,.T.);
#67271=ADVANCED_FACE('',(#6521),#1066,.T.);
#67272=ADVANCED_FACE('',(#6522),#1067,.T.);
#67273=ADVANCED_FACE('',(#6523),#1068,.T.);
#67274=ADVANCED_FACE('',(#6524),#1069,.T.);
#67275=ADVANCED_FACE('',(#6525),#1070,.T.);
#67276=ADVANCED_FACE('',(#6526),#1071,.T.);
#67277=ADVANCED_FACE('',(#6527),#1072,.T.);
#67278=ADVANCED_FACE('',(#6528),#1073,.T.);
#67279=ADVANCED_FACE('',(#6529),#1074,.T.);
#67280=ADVANCED_FACE('',(#6530),#1075,.T.);
#67281=ADVANCED_FACE('',(#6531),#1076,.T.);
#67282=ADVANCED_FACE('',(#6532),#1077,.T.);
#67283=ADVANCED_FACE('',(#6533),#1078,.T.);
#67284=ADVANCED_FACE('',(#6534),#1079,.T.);
#67285=ADVANCED_FACE('',(#6535),#1080,.T.);
#67286=ADVANCED_FACE('',(#6536),#1081,.T.);
#67287=ADVANCED_FACE('',(#6537),#1082,.T.);
#67288=ADVANCED_FACE('',(#6538),#1083,.T.);
#67289=ADVANCED_FACE('',(#6539),#1084,.T.);
#67290=ADVANCED_FACE('',(#6540),#1085,.T.);
#67291=ADVANCED_FACE('',(#6541),#1086,.T.);
#67292=ADVANCED_FACE('',(#6542),#1087,.T.);
#67293=ADVANCED_FACE('',(#6543),#1088,.T.);
#67294=ADVANCED_FACE('',(#6544),#1089,.T.);
#67295=ADVANCED_FACE('',(#6545),#1090,.T.);
#67296=ADVANCED_FACE('',(#6546),#1091,.T.);
#67297=ADVANCED_FACE('',(#6547),#1092,.T.);
#67298=ADVANCED_FACE('',(#6548),#1093,.T.);
#67299=ADVANCED_FACE('',(#6549),#1094,.T.);
#67300=ADVANCED_FACE('',(#6550),#1095,.T.);
#67301=ADVANCED_FACE('',(#6551),#1096,.T.);
#67302=ADVANCED_FACE('',(#6552),#1097,.T.);
#67303=ADVANCED_FACE('',(#6553),#1098,.T.);
#67304=ADVANCED_FACE('',(#6554),#1099,.T.);
#67305=ADVANCED_FACE('',(#6555),#1100,.T.);
#67306=ADVANCED_FACE('',(#6556),#1101,.T.);
#67307=ADVANCED_FACE('',(#6557),#1102,.T.);
#67308=ADVANCED_FACE('',(#6558),#1103,.T.);
#67309=ADVANCED_FACE('',(#6559),#1104,.T.);
#67310=ADVANCED_FACE('',(#6560),#1105,.T.);
#67311=ADVANCED_FACE('',(#6561),#1106,.T.);
#67312=ADVANCED_FACE('',(#6562),#1107,.T.);
#67313=ADVANCED_FACE('',(#6563),#1108,.T.);
#67314=ADVANCED_FACE('',(#6564),#1109,.T.);
#67315=ADVANCED_FACE('',(#6565),#1110,.T.);
#67316=ADVANCED_FACE('',(#6566),#1111,.T.);
#67317=ADVANCED_FACE('',(#6567),#1112,.T.);
#67318=ADVANCED_FACE('',(#6568),#1113,.T.);
#67319=ADVANCED_FACE('',(#6569),#1114,.T.);
#67320=ADVANCED_FACE('',(#6570),#1115,.T.);
#67321=ADVANCED_FACE('',(#6571),#1116,.T.);
#67322=ADVANCED_FACE('',(#6572),#1117,.T.);
#67323=ADVANCED_FACE('',(#6573),#1118,.T.);
#67324=ADVANCED_FACE('',(#6574),#1119,.T.);
#67325=ADVANCED_FACE('',(#6575),#1120,.T.);
#67326=ADVANCED_FACE('',(#6576),#1121,.T.);
#67327=ADVANCED_FACE('',(#6577),#1122,.T.);
#67328=ADVANCED_FACE('',(#6578),#1123,.T.);
#67329=ADVANCED_FACE('',(#6579),#4716,.T.);
#67330=ADVANCED_FACE('',(#6580),#1124,.T.);
#67331=ADVANCED_FACE('',(#6581),#1125,.T.);
#67332=ADVANCED_FACE('',(#6582),#4717,.T.);
#67333=ADVANCED_FACE('',(#6583),#1126,.T.);
#67334=ADVANCED_FACE('',(#6584),#1127,.T.);
#67335=ADVANCED_FACE('',(#6585),#4718,.T.);
#67336=ADVANCED_FACE('',(#6586),#1128,.T.);
#67337=ADVANCED_FACE('',(#6587),#1129,.T.);
#67338=ADVANCED_FACE('',(#6588),#4719,.T.);
#67339=ADVANCED_FACE('',(#6589),#1130,.T.);
#67340=ADVANCED_FACE('',(#6590),#1131,.T.);
#67341=ADVANCED_FACE('',(#6591),#4720,.T.);
#67342=ADVANCED_FACE('',(#6592),#1132,.T.);
#67343=ADVANCED_FACE('',(#6593),#1133,.T.);
#67344=ADVANCED_FACE('',(#6594),#4721,.T.);
#67345=ADVANCED_FACE('',(#6595),#1134,.T.);
#67346=ADVANCED_FACE('',(#6596),#1135,.T.);
#67347=ADVANCED_FACE('',(#6597),#1136,.T.);
#67348=ADVANCED_FACE('',(#6598),#1137,.T.);
#67349=ADVANCED_FACE('',(#6599),#4722,.T.);
#67350=ADVANCED_FACE('',(#6600),#1138,.T.);
#67351=ADVANCED_FACE('',(#6601),#1139,.T.);
#67352=ADVANCED_FACE('',(#6602),#4723,.T.);
#67353=ADVANCED_FACE('',(#6603),#1140,.T.);
#67354=ADVANCED_FACE('',(#6604),#1141,.T.);
#67355=ADVANCED_FACE('',(#6605),#4724,.T.);
#67356=ADVANCED_FACE('',(#6606),#1142,.T.);
#67357=ADVANCED_FACE('',(#6607),#1143,.T.);
#67358=ADVANCED_FACE('',(#6608),#4725,.T.);
#67359=ADVANCED_FACE('',(#6609),#1144,.T.);
#67360=ADVANCED_FACE('',(#6610),#1145,.T.);
#67361=ADVANCED_FACE('',(#6611),#4726,.T.);
#67362=ADVANCED_FACE('',(#6612),#1146,.T.);
#67363=ADVANCED_FACE('',(#6613),#1147,.T.);
#67364=ADVANCED_FACE('',(#6614),#4727,.T.);
#67365=ADVANCED_FACE('',(#6615),#1148,.T.);
#67366=ADVANCED_FACE('',(#6616),#1149,.T.);
#67367=ADVANCED_FACE('',(#6617),#4728,.T.);
#67368=ADVANCED_FACE('',(#6618),#1150,.T.);
#67369=ADVANCED_FACE('',(#6619),#1151,.T.);
#67370=ADVANCED_FACE('',(#6620),#4729,.T.);
#67371=ADVANCED_FACE('',(#6621),#1152,.T.);
#67372=ADVANCED_FACE('',(#6622),#1153,.T.);
#67373=ADVANCED_FACE('',(#6623),#4730,.T.);
#67374=ADVANCED_FACE('',(#6624),#1154,.T.);
#67375=ADVANCED_FACE('',(#6625),#1155,.T.);
#67376=ADVANCED_FACE('',(#6626),#4731,.T.);
#67377=ADVANCED_FACE('',(#6627),#1156,.T.);
#67378=ADVANCED_FACE('',(#6628),#1157,.T.);
#67379=ADVANCED_FACE('',(#6629),#4732,.T.);
#67380=ADVANCED_FACE('',(#6630),#1158,.T.);
#67381=ADVANCED_FACE('',(#6631),#1159,.T.);
#67382=ADVANCED_FACE('',(#6632),#4733,.T.);
#67383=ADVANCED_FACE('',(#6633),#1160,.T.);
#67384=ADVANCED_FACE('',(#6634),#1161,.T.);
#67385=ADVANCED_FACE('',(#6635),#4734,.T.);
#67386=ADVANCED_FACE('',(#6636),#1162,.T.);
#67387=ADVANCED_FACE('',(#6637),#1163,.T.);
#67388=ADVANCED_FACE('',(#6638),#4735,.T.);
#67389=ADVANCED_FACE('',(#6639),#1164,.T.);
#67390=ADVANCED_FACE('',(#6640),#1165,.T.);
#67391=ADVANCED_FACE('',(#6641),#4736,.T.);
#67392=ADVANCED_FACE('',(#6642),#1166,.T.);
#67393=ADVANCED_FACE('',(#6643),#1167,.T.);
#67394=ADVANCED_FACE('',(#6644),#1168,.T.);
#67395=ADVANCED_FACE('',(#6645),#4737,.T.);
#67396=ADVANCED_FACE('',(#6646),#1169,.T.);
#67397=ADVANCED_FACE('',(#6647),#4738,.T.);
#67398=ADVANCED_FACE('',(#6648),#1170,.T.);
#67399=ADVANCED_FACE('',(#6649),#1171,.T.);
#67400=ADVANCED_FACE('',(#6650),#4739,.T.);
#67401=ADVANCED_FACE('',(#6651),#1172,.T.);
#67402=ADVANCED_FACE('',(#6652),#1173,.T.);
#67403=ADVANCED_FACE('',(#6653),#4740,.T.);
#67404=ADVANCED_FACE('',(#6654),#1174,.T.);
#67405=ADVANCED_FACE('',(#6655),#1175,.T.);
#67406=ADVANCED_FACE('',(#6656),#4741,.T.);
#67407=ADVANCED_FACE('',(#6657),#1176,.T.);
#67408=ADVANCED_FACE('',(#6658),#1177,.T.);
#67409=ADVANCED_FACE('',(#6659),#4742,.T.);
#67410=ADVANCED_FACE('',(#6660),#1178,.T.);
#67411=ADVANCED_FACE('',(#6661),#4743,.T.);
#67412=ADVANCED_FACE('',(#6662),#1179,.T.);
#67413=ADVANCED_FACE('',(#6663),#1180,.T.);
#67414=ADVANCED_FACE('',(#6664),#1181,.T.);
#67415=ADVANCED_FACE('',(#6665),#1182,.T.);
#67416=ADVANCED_FACE('',(#6666),#4744,.T.);
#67417=ADVANCED_FACE('',(#6667),#1183,.T.);
#67418=ADVANCED_FACE('',(#6668),#1184,.T.);
#67419=ADVANCED_FACE('',(#6669),#4745,.T.);
#67420=ADVANCED_FACE('',(#6670),#1185,.T.);
#67421=ADVANCED_FACE('',(#6671),#1186,.T.);
#67422=ADVANCED_FACE('',(#6672),#4746,.T.);
#67423=ADVANCED_FACE('',(#6673),#1187,.T.);
#67424=ADVANCED_FACE('',(#6674),#1188,.T.);
#67425=ADVANCED_FACE('',(#6675),#4747,.T.);
#67426=ADVANCED_FACE('',(#6676),#1189,.T.);
#67427=ADVANCED_FACE('',(#6677),#1190,.T.);
#67428=ADVANCED_FACE('',(#6678),#4748,.T.);
#67429=ADVANCED_FACE('',(#6679),#1191,.T.);
#67430=ADVANCED_FACE('',(#6680),#1192,.T.);
#67431=ADVANCED_FACE('',(#6681),#4749,.T.);
#67432=ADVANCED_FACE('',(#6682),#1193,.T.);
#67433=ADVANCED_FACE('',(#6683),#1194,.T.);
#67434=ADVANCED_FACE('',(#6684),#4750,.T.);
#67435=ADVANCED_FACE('',(#6685),#1195,.T.);
#67436=ADVANCED_FACE('',(#6686),#1196,.T.);
#67437=ADVANCED_FACE('',(#6687),#4751,.T.);
#67438=ADVANCED_FACE('',(#6688),#1197,.T.);
#67439=ADVANCED_FACE('',(#6689),#1198,.T.);
#67440=ADVANCED_FACE('',(#6690),#4752,.T.);
#67441=ADVANCED_FACE('',(#6691),#1199,.T.);
#67442=ADVANCED_FACE('',(#6692),#1200,.T.);
#67443=ADVANCED_FACE('',(#6693),#4753,.T.);
#67444=ADVANCED_FACE('',(#6694),#1201,.T.);
#67445=ADVANCED_FACE('',(#6695),#1202,.T.);
#67446=ADVANCED_FACE('',(#6696),#4754,.T.);
#67447=ADVANCED_FACE('',(#6697),#1203,.T.);
#67448=ADVANCED_FACE('',(#6698),#1204,.T.);
#67449=ADVANCED_FACE('',(#6699),#4755,.T.);
#67450=ADVANCED_FACE('',(#6700),#1205,.T.);
#67451=ADVANCED_FACE('',(#6701),#1206,.T.);
#67452=ADVANCED_FACE('',(#6702),#4756,.T.);
#67453=ADVANCED_FACE('',(#6703),#1207,.T.);
#67454=ADVANCED_FACE('',(#6704),#1208,.T.);
#67455=ADVANCED_FACE('',(#6705),#1209,.T.);
#67456=ADVANCED_FACE('',(#6706),#1210,.T.);
#67457=ADVANCED_FACE('',(#6707),#4757,.T.);
#67458=ADVANCED_FACE('',(#6708),#1211,.T.);
#67459=ADVANCED_FACE('',(#6709),#1212,.T.);
#67460=ADVANCED_FACE('',(#6710),#4758,.T.);
#67461=ADVANCED_FACE('',(#6711),#1213,.T.);
#67462=ADVANCED_FACE('',(#6712),#1214,.T.);
#67463=ADVANCED_FACE('',(#6713),#4759,.T.);
#67464=ADVANCED_FACE('',(#6714),#1215,.T.);
#67465=ADVANCED_FACE('',(#6715),#1216,.T.);
#67466=ADVANCED_FACE('',(#6716),#4760,.T.);
#67467=ADVANCED_FACE('',(#6717),#1217,.T.);
#67468=ADVANCED_FACE('',(#6718),#1218,.T.);
#67469=ADVANCED_FACE('',(#6719),#4761,.T.);
#67470=ADVANCED_FACE('',(#6720),#1219,.T.);
#67471=ADVANCED_FACE('',(#6721),#1220,.T.);
#67472=ADVANCED_FACE('',(#6722),#4762,.T.);
#67473=ADVANCED_FACE('',(#6723),#1221,.T.);
#67474=ADVANCED_FACE('',(#6724),#1222,.T.);
#67475=ADVANCED_FACE('',(#6725),#4763,.T.);
#67476=ADVANCED_FACE('',(#6726),#1223,.T.);
#67477=ADVANCED_FACE('',(#6727),#1224,.T.);
#67478=ADVANCED_FACE('',(#6728),#4764,.T.);
#67479=ADVANCED_FACE('',(#6729),#1225,.T.);
#67480=ADVANCED_FACE('',(#6730),#1226,.T.);
#67481=ADVANCED_FACE('',(#6731),#4765,.T.);
#67482=ADVANCED_FACE('',(#6732),#1227,.T.);
#67483=ADVANCED_FACE('',(#6733),#1228,.T.);
#67484=ADVANCED_FACE('',(#6734),#4766,.T.);
#67485=ADVANCED_FACE('',(#6735),#1229,.T.);
#67486=ADVANCED_FACE('',(#6736),#1230,.T.);
#67487=ADVANCED_FACE('',(#6737),#4767,.T.);
#67488=ADVANCED_FACE('',(#6738),#1231,.T.);
#67489=ADVANCED_FACE('',(#6739),#1232,.T.);
#67490=ADVANCED_FACE('',(#6740),#4768,.T.);
#67491=ADVANCED_FACE('',(#6741),#1233,.T.);
#67492=ADVANCED_FACE('',(#6742),#1234,.T.);
#67493=ADVANCED_FACE('',(#6743),#4769,.T.);
#67494=ADVANCED_FACE('',(#6744),#1235,.T.);
#67495=ADVANCED_FACE('',(#6745),#1236,.T.);
#67496=ADVANCED_FACE('',(#6746),#4770,.T.);
#67497=ADVANCED_FACE('',(#6747),#4771,.T.);
#67498=ADVANCED_FACE('',(#6748),#1237,.T.);
#67499=ADVANCED_FACE('',(#6749),#1238,.T.);
#67500=ADVANCED_FACE('',(#6750),#1239,.T.);
#67501=ADVANCED_FACE('',(#6751),#1240,.T.);
#67502=ADVANCED_FACE('',(#6752),#1241,.T.);
#67503=ADVANCED_FACE('',(#6753),#1242,.T.);
#67504=ADVANCED_FACE('',(#6754),#1243,.T.);
#67505=ADVANCED_FACE('',(#6755),#1244,.T.);
#67506=ADVANCED_FACE('',(#6756),#1245,.T.);
#67507=ADVANCED_FACE('',(#6757),#1246,.T.);
#67508=ADVANCED_FACE('',(#6758),#1247,.T.);
#67509=ADVANCED_FACE('',(#6759),#1248,.T.);
#67510=ADVANCED_FACE('',(#6760),#1249,.T.);
#67511=ADVANCED_FACE('',(#6761),#1250,.T.);
#67512=ADVANCED_FACE('',(#6762),#1251,.T.);
#67513=ADVANCED_FACE('',(#6763),#1252,.T.);
#67514=ADVANCED_FACE('',(#6764),#1253,.T.);
#67515=ADVANCED_FACE('',(#6765),#1254,.T.);
#67516=ADVANCED_FACE('',(#6766),#1255,.T.);
#67517=ADVANCED_FACE('',(#6767),#1256,.T.);
#67518=ADVANCED_FACE('',(#6768),#1257,.T.);
#67519=ADVANCED_FACE('',(#6769),#1258,.T.);
#67520=ADVANCED_FACE('',(#6770),#1259,.T.);
#67521=ADVANCED_FACE('',(#6771),#1260,.T.);
#67522=ADVANCED_FACE('',(#6772),#1261,.T.);
#67523=ADVANCED_FACE('',(#6773),#1262,.T.);
#67524=ADVANCED_FACE('',(#6774),#1263,.T.);
#67525=ADVANCED_FACE('',(#6775),#1264,.T.);
#67526=ADVANCED_FACE('',(#6776),#1265,.T.);
#67527=ADVANCED_FACE('',(#6777),#1266,.T.);
#67528=ADVANCED_FACE('',(#6778),#1267,.T.);
#67529=ADVANCED_FACE('',(#6779),#1268,.T.);
#67530=ADVANCED_FACE('',(#6780),#1269,.T.);
#67531=ADVANCED_FACE('',(#6781),#1270,.T.);
#67532=ADVANCED_FACE('',(#6782),#1271,.T.);
#67533=ADVANCED_FACE('',(#6783),#1272,.T.);
#67534=ADVANCED_FACE('',(#6784),#1273,.T.);
#67535=ADVANCED_FACE('',(#6785),#1274,.T.);
#67536=ADVANCED_FACE('',(#6786),#1275,.T.);
#67537=ADVANCED_FACE('',(#6787),#1276,.T.);
#67538=ADVANCED_FACE('',(#6788),#1277,.T.);
#67539=ADVANCED_FACE('',(#6789),#1278,.T.);
#67540=ADVANCED_FACE('',(#6790),#1279,.T.);
#67541=ADVANCED_FACE('',(#6791),#1280,.T.);
#67542=ADVANCED_FACE('',(#6792),#1281,.T.);
#67543=ADVANCED_FACE('',(#6793),#1282,.T.);
#67544=ADVANCED_FACE('',(#6794),#1283,.T.);
#67545=ADVANCED_FACE('',(#6795),#1284,.T.);
#67546=ADVANCED_FACE('',(#6796),#1285,.T.);
#67547=ADVANCED_FACE('',(#6797),#1286,.T.);
#67548=ADVANCED_FACE('',(#6798),#1287,.T.);
#67549=ADVANCED_FACE('',(#6799),#1288,.T.);
#67550=ADVANCED_FACE('',(#6800),#1289,.T.);
#67551=ADVANCED_FACE('',(#6801),#1290,.T.);
#67552=ADVANCED_FACE('',(#6802),#1291,.T.);
#67553=ADVANCED_FACE('',(#6803),#1292,.T.);
#67554=ADVANCED_FACE('',(#6804),#1293,.T.);
#67555=ADVANCED_FACE('',(#6805),#1294,.T.);
#67556=ADVANCED_FACE('',(#6806),#1295,.T.);
#67557=ADVANCED_FACE('',(#6807),#1296,.T.);
#67558=ADVANCED_FACE('',(#6808),#1297,.T.);
#67559=ADVANCED_FACE('',(#6809),#1298,.T.);
#67560=ADVANCED_FACE('',(#6810),#1299,.T.);
#67561=ADVANCED_FACE('',(#6811),#1300,.T.);
#67562=ADVANCED_FACE('',(#6812),#1301,.T.);
#67563=ADVANCED_FACE('',(#6813),#1302,.T.);
#67564=ADVANCED_FACE('',(#6814),#1303,.T.);
#67565=ADVANCED_FACE('',(#6815),#1304,.T.);
#67566=ADVANCED_FACE('',(#6816),#1305,.T.);
#67567=ADVANCED_FACE('',(#6817),#1306,.T.);
#67568=ADVANCED_FACE('',(#6818),#1307,.T.);
#67569=ADVANCED_FACE('',(#6819),#1308,.T.);
#67570=ADVANCED_FACE('',(#6820),#1309,.T.);
#67571=ADVANCED_FACE('',(#6821),#1310,.T.);
#67572=ADVANCED_FACE('',(#6822),#1311,.T.);
#67573=ADVANCED_FACE('',(#6823),#1312,.T.);
#67574=ADVANCED_FACE('',(#6824),#1313,.T.);
#67575=ADVANCED_FACE('',(#6825),#1314,.T.);
#67576=ADVANCED_FACE('',(#6826),#1315,.T.);
#67577=ADVANCED_FACE('',(#6827),#1316,.T.);
#67578=ADVANCED_FACE('',(#6828),#1317,.T.);
#67579=ADVANCED_FACE('',(#6829),#1318,.T.);
#67580=ADVANCED_FACE('',(#6830),#1319,.T.);
#67581=ADVANCED_FACE('',(#6831),#1320,.T.);
#67582=ADVANCED_FACE('',(#6832),#1321,.T.);
#67583=ADVANCED_FACE('',(#6833),#1322,.T.);
#67584=ADVANCED_FACE('',(#6834),#1323,.T.);
#67585=ADVANCED_FACE('',(#6835),#1324,.T.);
#67586=ADVANCED_FACE('',(#6836),#1325,.T.);
#67587=ADVANCED_FACE('',(#6837),#1326,.T.);
#67588=ADVANCED_FACE('',(#6838),#1327,.T.);
#67589=ADVANCED_FACE('',(#6839),#1328,.T.);
#67590=ADVANCED_FACE('',(#6840),#1329,.T.);
#67591=ADVANCED_FACE('',(#6841),#1330,.T.);
#67592=ADVANCED_FACE('',(#6842),#1331,.T.);
#67593=ADVANCED_FACE('',(#6843),#1332,.T.);
#67594=ADVANCED_FACE('',(#6844),#1333,.T.);
#67595=ADVANCED_FACE('',(#6845),#1334,.T.);
#67596=ADVANCED_FACE('',(#6846),#1335,.T.);
#67597=ADVANCED_FACE('',(#6847),#1336,.T.);
#67598=ADVANCED_FACE('',(#6848),#1337,.T.);
#67599=ADVANCED_FACE('',(#6849),#1338,.T.);
#67600=ADVANCED_FACE('',(#6850),#1339,.T.);
#67601=ADVANCED_FACE('',(#6851),#1340,.T.);
#67602=ADVANCED_FACE('',(#6852),#1341,.T.);
#67603=ADVANCED_FACE('',(#6853),#1342,.T.);
#67604=ADVANCED_FACE('',(#6854),#1343,.T.);
#67605=ADVANCED_FACE('',(#6855),#1344,.T.);
#67606=ADVANCED_FACE('',(#6856),#1345,.T.);
#67607=ADVANCED_FACE('',(#6857),#1346,.T.);
#67608=ADVANCED_FACE('',(#6858),#1347,.T.);
#67609=ADVANCED_FACE('',(#6859),#1348,.T.);
#67610=ADVANCED_FACE('',(#6860),#1349,.T.);
#67611=ADVANCED_FACE('',(#6861),#1350,.T.);
#67612=ADVANCED_FACE('',(#6862),#1351,.T.);
#67613=ADVANCED_FACE('',(#6863),#1352,.T.);
#67614=ADVANCED_FACE('',(#6864),#1353,.T.);
#67615=ADVANCED_FACE('',(#6865),#1354,.T.);
#67616=ADVANCED_FACE('',(#6866),#4772,.T.);
#67617=ADVANCED_FACE('',(#6867),#1355,.T.);
#67618=ADVANCED_FACE('',(#6868),#1356,.T.);
#67619=ADVANCED_FACE('',(#6869),#4773,.T.);
#67620=ADVANCED_FACE('',(#6870),#1357,.T.);
#67621=ADVANCED_FACE('',(#6871),#1358,.T.);
#67622=ADVANCED_FACE('',(#6872),#4774,.T.);
#67623=ADVANCED_FACE('',(#6873),#1359,.T.);
#67624=ADVANCED_FACE('',(#6874),#1360,.T.);
#67625=ADVANCED_FACE('',(#6875),#4775,.T.);
#67626=ADVANCED_FACE('',(#6876),#1361,.T.);
#67627=ADVANCED_FACE('',(#6877),#1362,.T.);
#67628=ADVANCED_FACE('',(#6878),#4776,.T.);
#67629=ADVANCED_FACE('',(#6879),#1363,.T.);
#67630=ADVANCED_FACE('',(#6880),#1364,.T.);
#67631=ADVANCED_FACE('',(#6881),#4777,.T.);
#67632=ADVANCED_FACE('',(#6882),#1365,.T.);
#67633=ADVANCED_FACE('',(#6883),#1366,.T.);
#67634=ADVANCED_FACE('',(#6884),#4778,.T.);
#67635=ADVANCED_FACE('',(#6885),#1367,.T.);
#67636=ADVANCED_FACE('',(#6886),#1368,.T.);
#67637=ADVANCED_FACE('',(#6887),#4779,.T.);
#67638=ADVANCED_FACE('',(#6888),#1369,.T.);
#67639=ADVANCED_FACE('',(#6889),#1370,.T.);
#67640=ADVANCED_FACE('',(#6890),#4780,.T.);
#67641=ADVANCED_FACE('',(#6891),#1371,.T.);
#67642=ADVANCED_FACE('',(#6892),#1372,.T.);
#67643=ADVANCED_FACE('',(#6893),#4781,.T.);
#67644=ADVANCED_FACE('',(#6894),#1373,.T.);
#67645=ADVANCED_FACE('',(#6895),#1374,.T.);
#67646=ADVANCED_FACE('',(#6896),#4782,.T.);
#67647=ADVANCED_FACE('',(#6897),#1375,.T.);
#67648=ADVANCED_FACE('',(#6898),#1376,.T.);
#67649=ADVANCED_FACE('',(#6899),#4783,.T.);
#67650=ADVANCED_FACE('',(#6900),#1377,.T.);
#67651=ADVANCED_FACE('',(#6901),#1378,.T.);
#67652=ADVANCED_FACE('',(#6902),#4784,.T.);
#67653=ADVANCED_FACE('',(#6903),#1379,.T.);
#67654=ADVANCED_FACE('',(#6904),#1380,.T.);
#67655=ADVANCED_FACE('',(#6905),#4785,.T.);
#67656=ADVANCED_FACE('',(#6906),#1381,.T.);
#67657=ADVANCED_FACE('',(#6907),#1382,.T.);
#67658=ADVANCED_FACE('',(#6908),#1383,.T.);
#67659=ADVANCED_FACE('',(#6909),#1384,.T.);
#67660=ADVANCED_FACE('',(#6910),#4786,.T.);
#67661=ADVANCED_FACE('',(#6911),#1385,.T.);
#67662=ADVANCED_FACE('',(#6912),#1386,.T.);
#67663=ADVANCED_FACE('',(#6913),#4787,.T.);
#67664=ADVANCED_FACE('',(#6914),#1387,.T.);
#67665=ADVANCED_FACE('',(#6915),#1388,.T.);
#67666=ADVANCED_FACE('',(#6916),#4788,.T.);
#67667=ADVANCED_FACE('',(#6917),#1389,.T.);
#67668=ADVANCED_FACE('',(#6918),#1390,.T.);
#67669=ADVANCED_FACE('',(#6919),#4789,.T.);
#67670=ADVANCED_FACE('',(#6920),#1391,.T.);
#67671=ADVANCED_FACE('',(#6921),#1392,.T.);
#67672=ADVANCED_FACE('',(#6922),#4790,.T.);
#67673=ADVANCED_FACE('',(#6923),#1393,.T.);
#67674=ADVANCED_FACE('',(#6924),#1394,.T.);
#67675=ADVANCED_FACE('',(#6925),#4791,.T.);
#67676=ADVANCED_FACE('',(#6926),#1395,.T.);
#67677=ADVANCED_FACE('',(#6927),#1396,.T.);
#67678=ADVANCED_FACE('',(#6928),#4792,.T.);
#67679=ADVANCED_FACE('',(#6929),#1397,.T.);
#67680=ADVANCED_FACE('',(#6930),#1398,.T.);
#67681=ADVANCED_FACE('',(#6931),#1399,.T.);
#67682=ADVANCED_FACE('',(#6932),#4793,.T.);
#67683=ADVANCED_FACE('',(#6933),#1400,.T.);
#67684=ADVANCED_FACE('',(#6934),#4794,.T.);
#67685=ADVANCED_FACE('',(#6935),#1401,.T.);
#67686=ADVANCED_FACE('',(#6936),#1402,.T.);
#67687=ADVANCED_FACE('',(#6937),#4795,.T.);
#67688=ADVANCED_FACE('',(#6938),#1403,.T.);
#67689=ADVANCED_FACE('',(#6939),#1404,.T.);
#67690=ADVANCED_FACE('',(#6940),#4796,.T.);
#67691=ADVANCED_FACE('',(#6941),#1405,.T.);
#67692=ADVANCED_FACE('',(#6942),#1406,.T.);
#67693=ADVANCED_FACE('',(#6943),#4797,.T.);
#67694=ADVANCED_FACE('',(#6944),#1407,.T.);
#67695=ADVANCED_FACE('',(#6945),#1408,.T.);
#67696=ADVANCED_FACE('',(#6946),#4798,.T.);
#67697=ADVANCED_FACE('',(#6947),#1409,.T.);
#67698=ADVANCED_FACE('',(#6948),#1410,.T.);
#67699=ADVANCED_FACE('',(#6949),#4799,.T.);
#67700=ADVANCED_FACE('',(#6950),#1411,.T.);
#67701=ADVANCED_FACE('',(#6951),#1412,.T.);
#67702=ADVANCED_FACE('',(#6952),#1413,.T.);
#67703=ADVANCED_FACE('',(#6953),#4800,.T.);
#67704=ADVANCED_FACE('',(#6954),#1414,.T.);
#67705=ADVANCED_FACE('',(#6955),#1415,.T.);
#67706=ADVANCED_FACE('',(#6956),#4801,.T.);
#67707=ADVANCED_FACE('',(#6957),#1416,.T.);
#67708=ADVANCED_FACE('',(#6958),#1417,.T.);
#67709=ADVANCED_FACE('',(#6959),#4802,.T.);
#67710=ADVANCED_FACE('',(#6960),#1418,.T.);
#67711=ADVANCED_FACE('',(#6961),#1419,.T.);
#67712=ADVANCED_FACE('',(#6962),#4803,.T.);
#67713=ADVANCED_FACE('',(#6963),#1420,.T.);
#67714=ADVANCED_FACE('',(#6964),#1421,.T.);
#67715=ADVANCED_FACE('',(#6965),#4804,.T.);
#67716=ADVANCED_FACE('',(#6966),#1422,.T.);
#67717=ADVANCED_FACE('',(#6967),#1423,.T.);
#67718=ADVANCED_FACE('',(#6968),#4805,.T.);
#67719=ADVANCED_FACE('',(#6969),#1424,.T.);
#67720=ADVANCED_FACE('',(#6970),#1425,.T.);
#67721=ADVANCED_FACE('',(#6971),#4806,.T.);
#67722=ADVANCED_FACE('',(#6972),#1426,.T.);
#67723=ADVANCED_FACE('',(#6973),#1427,.T.);
#67724=ADVANCED_FACE('',(#6974),#4807,.T.);
#67725=ADVANCED_FACE('',(#6975),#1428,.T.);
#67726=ADVANCED_FACE('',(#6976),#1429,.T.);
#67727=ADVANCED_FACE('',(#6977),#4808,.T.);
#67728=ADVANCED_FACE('',(#6978),#1430,.T.);
#67729=ADVANCED_FACE('',(#6979),#1431,.T.);
#67730=ADVANCED_FACE('',(#6980),#4809,.T.);
#67731=ADVANCED_FACE('',(#6981),#1432,.T.);
#67732=ADVANCED_FACE('',(#6982),#1433,.T.);
#67733=ADVANCED_FACE('',(#6983),#4810,.T.);
#67734=ADVANCED_FACE('',(#6984),#1434,.T.);
#67735=ADVANCED_FACE('',(#6985),#1435,.T.);
#67736=ADVANCED_FACE('',(#6986),#4811,.T.);
#67737=ADVANCED_FACE('',(#6987),#1436,.T.);
#67738=ADVANCED_FACE('',(#6988),#1437,.T.);
#67739=ADVANCED_FACE('',(#6989),#4812,.T.);
#67740=ADVANCED_FACE('',(#6990),#1438,.T.);
#67741=ADVANCED_FACE('',(#6991),#1439,.T.);
#67742=ADVANCED_FACE('',(#6992),#4813,.T.);
#67743=ADVANCED_FACE('',(#6993),#1440,.T.);
#67744=ADVANCED_FACE('',(#6994),#1441,.T.);
#67745=ADVANCED_FACE('',(#6995),#4814,.T.);
#67746=ADVANCED_FACE('',(#6996),#1442,.T.);
#67747=ADVANCED_FACE('',(#6997),#1443,.T.);
#67748=ADVANCED_FACE('',(#6998),#4815,.T.);
#67749=ADVANCED_FACE('',(#6999),#1444,.T.);
#67750=ADVANCED_FACE('',(#7000),#1445,.T.);
#67751=ADVANCED_FACE('',(#7001),#4816,.T.);
#67752=ADVANCED_FACE('',(#7002),#1446,.T.);
#67753=ADVANCED_FACE('',(#7003),#1447,.T.);
#67754=ADVANCED_FACE('',(#7004),#4817,.T.);
#67755=ADVANCED_FACE('',(#7005),#1448,.T.);
#67756=ADVANCED_FACE('',(#7006),#1449,.T.);
#67757=ADVANCED_FACE('',(#7007),#4818,.T.);
#67758=ADVANCED_FACE('',(#7008),#1450,.T.);
#67759=ADVANCED_FACE('',(#7009),#1451,.T.);
#67760=ADVANCED_FACE('',(#7010),#4819,.T.);
#67761=ADVANCED_FACE('',(#7011),#1452,.T.);
#67762=ADVANCED_FACE('',(#7012),#1453,.T.);
#67763=ADVANCED_FACE('',(#7013),#4820,.T.);
#67764=ADVANCED_FACE('',(#7014),#1454,.T.);
#67765=ADVANCED_FACE('',(#7015),#1455,.T.);
#67766=ADVANCED_FACE('',(#7016),#1456,.T.);
#67767=ADVANCED_FACE('',(#7017),#1457,.T.);
#67768=ADVANCED_FACE('',(#7018),#4821,.T.);
#67769=ADVANCED_FACE('',(#7019),#1458,.T.);
#67770=ADVANCED_FACE('',(#7020),#1459,.T.);
#67771=ADVANCED_FACE('',(#7021),#4822,.T.);
#67772=ADVANCED_FACE('',(#7022),#1460,.T.);
#67773=ADVANCED_FACE('',(#7023),#1461,.T.);
#67774=ADVANCED_FACE('',(#7024),#4823,.T.);
#67775=ADVANCED_FACE('',(#7025),#1462,.T.);
#67776=ADVANCED_FACE('',(#7026),#1463,.T.);
#67777=ADVANCED_FACE('',(#7027),#4824,.T.);
#67778=ADVANCED_FACE('',(#7028),#1464,.T.);
#67779=ADVANCED_FACE('',(#7029),#1465,.T.);
#67780=ADVANCED_FACE('',(#7030),#4825,.T.);
#67781=ADVANCED_FACE('',(#7031),#1466,.T.);
#67782=ADVANCED_FACE('',(#7032),#1467,.T.);
#67783=ADVANCED_FACE('',(#7033),#4826,.T.);
#67784=ADVANCED_FACE('',(#7034),#1468,.T.);
#67785=ADVANCED_FACE('',(#7035),#1469,.T.);
#67786=ADVANCED_FACE('',(#7036),#4827,.T.);
#67787=ADVANCED_FACE('',(#7037),#1470,.T.);
#67788=ADVANCED_FACE('',(#7038),#1471,.T.);
#67789=ADVANCED_FACE('',(#7039),#1472,.T.);
#67790=ADVANCED_FACE('',(#7040),#1473,.T.);
#67791=ADVANCED_FACE('',(#7041),#1474,.T.);
#67792=ADVANCED_FACE('',(#7042),#1475,.T.);
#67793=ADVANCED_FACE('',(#7043),#1476,.T.);
#67794=ADVANCED_FACE('',(#7044),#1477,.T.);
#67795=ADVANCED_FACE('',(#7045),#1478,.T.);
#67796=ADVANCED_FACE('',(#7046),#1479,.T.);
#67797=ADVANCED_FACE('',(#7047),#1480,.T.);
#67798=ADVANCED_FACE('',(#7048),#1481,.T.);
#67799=ADVANCED_FACE('',(#7049),#1482,.T.);
#67800=ADVANCED_FACE('',(#7050),#1483,.T.);
#67801=ADVANCED_FACE('',(#7051),#1484,.T.);
#67802=ADVANCED_FACE('',(#7052),#1485,.T.);
#67803=ADVANCED_FACE('',(#7053),#1486,.T.);
#67804=ADVANCED_FACE('',(#7054),#1487,.T.);
#67805=ADVANCED_FACE('',(#7055),#1488,.T.);
#67806=ADVANCED_FACE('',(#7056),#1489,.T.);
#67807=ADVANCED_FACE('',(#7057),#1490,.T.);
#67808=ADVANCED_FACE('',(#7058),#1491,.T.);
#67809=ADVANCED_FACE('',(#7059),#1492,.T.);
#67810=ADVANCED_FACE('',(#7060),#1493,.T.);
#67811=ADVANCED_FACE('',(#7061),#1494,.T.);
#67812=ADVANCED_FACE('',(#7062),#1495,.T.);
#67813=ADVANCED_FACE('',(#7063),#1496,.T.);
#67814=ADVANCED_FACE('',(#7064),#1497,.T.);
#67815=ADVANCED_FACE('',(#7065),#1498,.T.);
#67816=ADVANCED_FACE('',(#7066),#1499,.T.);
#67817=ADVANCED_FACE('',(#7067),#1500,.T.);
#67818=ADVANCED_FACE('',(#7068),#1501,.T.);
#67819=ADVANCED_FACE('',(#7069),#1502,.T.);
#67820=ADVANCED_FACE('',(#7070),#1503,.T.);
#67821=ADVANCED_FACE('',(#7071),#1504,.T.);
#67822=ADVANCED_FACE('',(#7072),#1505,.T.);
#67823=ADVANCED_FACE('',(#7073),#1506,.T.);
#67824=ADVANCED_FACE('',(#7074),#1507,.T.);
#67825=ADVANCED_FACE('',(#7075),#1508,.T.);
#67826=ADVANCED_FACE('',(#7076),#1509,.T.);
#67827=ADVANCED_FACE('',(#7077),#1510,.T.);
#67828=ADVANCED_FACE('',(#7078),#1511,.T.);
#67829=ADVANCED_FACE('',(#7079),#1512,.T.);
#67830=ADVANCED_FACE('',(#7080),#1513,.T.);
#67831=ADVANCED_FACE('',(#7081),#1514,.T.);
#67832=ADVANCED_FACE('',(#7082),#1515,.T.);
#67833=ADVANCED_FACE('',(#7083),#1516,.T.);
#67834=ADVANCED_FACE('',(#7084),#1517,.T.);
#67835=ADVANCED_FACE('',(#7085),#1518,.T.);
#67836=ADVANCED_FACE('',(#7086),#1519,.T.);
#67837=ADVANCED_FACE('',(#7087),#1520,.T.);
#67838=ADVANCED_FACE('',(#7088),#1521,.T.);
#67839=ADVANCED_FACE('',(#7089),#1522,.T.);
#67840=ADVANCED_FACE('',(#7090),#1523,.T.);
#67841=ADVANCED_FACE('',(#7091),#1524,.T.);
#67842=ADVANCED_FACE('',(#7092),#1525,.T.);
#67843=ADVANCED_FACE('',(#7093),#1526,.T.);
#67844=ADVANCED_FACE('',(#7094),#1527,.T.);
#67845=ADVANCED_FACE('',(#7095),#1528,.T.);
#67846=ADVANCED_FACE('',(#7096),#1529,.T.);
#67847=ADVANCED_FACE('',(#7097),#1530,.T.);
#67848=ADVANCED_FACE('',(#7098),#1531,.T.);
#67849=ADVANCED_FACE('',(#7099),#1532,.T.);
#67850=ADVANCED_FACE('',(#7100),#1533,.T.);
#67851=ADVANCED_FACE('',(#7101),#1534,.T.);
#67852=ADVANCED_FACE('',(#7102),#1535,.T.);
#67853=ADVANCED_FACE('',(#7103),#1536,.T.);
#67854=ADVANCED_FACE('',(#7104),#1537,.T.);
#67855=ADVANCED_FACE('',(#7105),#1538,.T.);
#67856=ADVANCED_FACE('',(#7106),#1539,.T.);
#67857=ADVANCED_FACE('',(#7107),#1540,.T.);
#67858=ADVANCED_FACE('',(#7108),#1541,.T.);
#67859=ADVANCED_FACE('',(#7109),#1542,.T.);
#67860=ADVANCED_FACE('',(#7110),#1543,.T.);
#67861=ADVANCED_FACE('',(#7111),#1544,.T.);
#67862=ADVANCED_FACE('',(#7112),#1545,.T.);
#67863=ADVANCED_FACE('',(#7113),#1546,.T.);
#67864=ADVANCED_FACE('',(#7114),#1547,.T.);
#67865=ADVANCED_FACE('',(#7115),#1548,.T.);
#67866=ADVANCED_FACE('',(#7116),#1549,.T.);
#67867=ADVANCED_FACE('',(#7117),#1550,.T.);
#67868=ADVANCED_FACE('',(#7118),#1551,.T.);
#67869=ADVANCED_FACE('',(#7119),#1552,.T.);
#67870=ADVANCED_FACE('',(#7120),#1553,.T.);
#67871=ADVANCED_FACE('',(#7121),#1554,.T.);
#67872=ADVANCED_FACE('',(#7122),#1555,.T.);
#67873=ADVANCED_FACE('',(#7123),#1556,.T.);
#67874=ADVANCED_FACE('',(#7124),#1557,.T.);
#67875=ADVANCED_FACE('',(#7125),#1558,.T.);
#67876=ADVANCED_FACE('',(#7126),#1559,.T.);
#67877=ADVANCED_FACE('',(#7127),#1560,.T.);
#67878=ADVANCED_FACE('',(#7128),#1561,.T.);
#67879=ADVANCED_FACE('',(#7129),#1562,.T.);
#67880=ADVANCED_FACE('',(#7130),#1563,.T.);
#67881=ADVANCED_FACE('',(#7131),#1564,.T.);
#67882=ADVANCED_FACE('',(#7132),#1565,.T.);
#67883=ADVANCED_FACE('',(#7133),#1566,.T.);
#67884=ADVANCED_FACE('',(#7134),#1567,.T.);
#67885=ADVANCED_FACE('',(#7135),#1568,.T.);
#67886=ADVANCED_FACE('',(#7136),#1569,.T.);
#67887=ADVANCED_FACE('',(#7137),#1570,.T.);
#67888=ADVANCED_FACE('',(#7138),#1571,.T.);
#67889=ADVANCED_FACE('',(#7139),#1572,.T.);
#67890=ADVANCED_FACE('',(#7140),#1573,.T.);
#67891=ADVANCED_FACE('',(#7141),#1574,.T.);
#67892=ADVANCED_FACE('',(#7142),#1575,.T.);
#67893=ADVANCED_FACE('',(#7143),#1576,.T.);
#67894=ADVANCED_FACE('',(#7144),#1577,.T.);
#67895=ADVANCED_FACE('',(#7145),#1578,.T.);
#67896=ADVANCED_FACE('',(#7146),#1579,.T.);
#67897=ADVANCED_FACE('',(#7147),#1580,.T.);
#67898=ADVANCED_FACE('',(#7148),#1581,.T.);
#67899=ADVANCED_FACE('',(#7149),#1582,.T.);
#67900=ADVANCED_FACE('',(#7150),#1583,.T.);
#67901=ADVANCED_FACE('',(#7151),#1584,.T.);
#67902=ADVANCED_FACE('',(#7152),#1585,.T.);
#67903=ADVANCED_FACE('',(#7153),#1586,.T.);
#67904=ADVANCED_FACE('',(#7154),#1587,.T.);
#67905=ADVANCED_FACE('',(#7155),#4828,.T.);
#67906=ADVANCED_FACE('',(#7156),#1588,.T.);
#67907=ADVANCED_FACE('',(#7157),#1589,.T.);
#67908=ADVANCED_FACE('',(#7158),#4829,.T.);
#67909=ADVANCED_FACE('',(#7159),#1590,.T.);
#67910=ADVANCED_FACE('',(#7160),#1591,.T.);
#67911=ADVANCED_FACE('',(#7161),#4830,.T.);
#67912=ADVANCED_FACE('',(#7162),#1592,.T.);
#67913=ADVANCED_FACE('',(#7163),#1593,.T.);
#67914=ADVANCED_FACE('',(#7164),#4831,.T.);
#67915=ADVANCED_FACE('',(#7165),#1594,.T.);
#67916=ADVANCED_FACE('',(#7166),#1595,.T.);
#67917=ADVANCED_FACE('',(#7167),#4832,.T.);
#67918=ADVANCED_FACE('',(#7168),#1596,.T.);
#67919=ADVANCED_FACE('',(#7169),#1597,.T.);
#67920=ADVANCED_FACE('',(#7170),#4833,.T.);
#67921=ADVANCED_FACE('',(#7171),#1598,.T.);
#67922=ADVANCED_FACE('',(#7172),#1599,.T.);
#67923=ADVANCED_FACE('',(#7173),#1600,.T.);
#67924=ADVANCED_FACE('',(#7174),#1601,.T.);
#67925=ADVANCED_FACE('',(#7175),#4834,.T.);
#67926=ADVANCED_FACE('',(#7176),#1602,.T.);
#67927=ADVANCED_FACE('',(#7177),#1603,.T.);
#67928=ADVANCED_FACE('',(#7178),#4835,.T.);
#67929=ADVANCED_FACE('',(#7179),#1604,.T.);
#67930=ADVANCED_FACE('',(#7180),#1605,.T.);
#67931=ADVANCED_FACE('',(#7181),#4836,.T.);
#67932=ADVANCED_FACE('',(#7182),#1606,.T.);
#67933=ADVANCED_FACE('',(#7183),#1607,.T.);
#67934=ADVANCED_FACE('',(#7184),#4837,.T.);
#67935=ADVANCED_FACE('',(#7185),#1608,.T.);
#67936=ADVANCED_FACE('',(#7186),#1609,.T.);
#67937=ADVANCED_FACE('',(#7187),#4838,.T.);
#67938=ADVANCED_FACE('',(#7188),#1610,.T.);
#67939=ADVANCED_FACE('',(#7189),#1611,.T.);
#67940=ADVANCED_FACE('',(#7190),#4839,.T.);
#67941=ADVANCED_FACE('',(#7191),#1612,.T.);
#67942=ADVANCED_FACE('',(#7192),#1613,.T.);
#67943=ADVANCED_FACE('',(#7193),#4840,.T.);
#67944=ADVANCED_FACE('',(#7194),#1614,.T.);
#67945=ADVANCED_FACE('',(#7195),#1615,.T.);
#67946=ADVANCED_FACE('',(#7196),#4841,.T.);
#67947=ADVANCED_FACE('',(#7197),#1616,.T.);
#67948=ADVANCED_FACE('',(#7198),#1617,.T.);
#67949=ADVANCED_FACE('',(#7199),#4842,.T.);
#67950=ADVANCED_FACE('',(#7200),#1618,.T.);
#67951=ADVANCED_FACE('',(#7201),#1619,.T.);
#67952=ADVANCED_FACE('',(#7202),#4843,.T.);
#67953=ADVANCED_FACE('',(#7203),#1620,.T.);
#67954=ADVANCED_FACE('',(#7204),#1621,.T.);
#67955=ADVANCED_FACE('',(#7205),#4844,.T.);
#67956=ADVANCED_FACE('',(#7206),#1622,.T.);
#67957=ADVANCED_FACE('',(#7207),#1623,.T.);
#67958=ADVANCED_FACE('',(#7208),#4845,.T.);
#67959=ADVANCED_FACE('',(#7209),#1624,.T.);
#67960=ADVANCED_FACE('',(#7210),#1625,.T.);
#67961=ADVANCED_FACE('',(#7211),#4846,.T.);
#67962=ADVANCED_FACE('',(#7212),#1626,.T.);
#67963=ADVANCED_FACE('',(#7213),#1627,.T.);
#67964=ADVANCED_FACE('',(#7214),#4847,.T.);
#67965=ADVANCED_FACE('',(#7215),#1628,.T.);
#67966=ADVANCED_FACE('',(#7216),#1629,.T.);
#67967=ADVANCED_FACE('',(#7217),#1630,.T.);
#67968=ADVANCED_FACE('',(#7218),#4848,.T.);
#67969=ADVANCED_FACE('',(#7219),#1631,.T.);
#67970=ADVANCED_FACE('',(#7220),#4849,.T.);
#67971=ADVANCED_FACE('',(#7221),#1632,.T.);
#67972=ADVANCED_FACE('',(#7222),#1633,.T.);
#67973=ADVANCED_FACE('',(#7223),#4850,.T.);
#67974=ADVANCED_FACE('',(#7224),#1634,.T.);
#67975=ADVANCED_FACE('',(#7225),#1635,.T.);
#67976=ADVANCED_FACE('',(#7226),#4851,.T.);
#67977=ADVANCED_FACE('',(#7227),#1636,.T.);
#67978=ADVANCED_FACE('',(#7228),#1637,.T.);
#67979=ADVANCED_FACE('',(#7229),#4852,.T.);
#67980=ADVANCED_FACE('',(#7230),#1638,.T.);
#67981=ADVANCED_FACE('',(#7231),#1639,.T.);
#67982=ADVANCED_FACE('',(#7232),#4853,.T.);
#67983=ADVANCED_FACE('',(#7233),#1640,.T.);
#67984=ADVANCED_FACE('',(#7234),#1641,.T.);
#67985=ADVANCED_FACE('',(#7235),#4854,.T.);
#67986=ADVANCED_FACE('',(#7236),#1642,.T.);
#67987=ADVANCED_FACE('',(#7237),#4855,.T.);
#67988=ADVANCED_FACE('',(#7238),#1643,.T.);
#67989=ADVANCED_FACE('',(#7239),#1644,.T.);
#67990=ADVANCED_FACE('',(#7240),#1645,.T.);
#67991=ADVANCED_FACE('',(#7241),#1646,.T.);
#67992=ADVANCED_FACE('',(#7242),#4856,.T.);
#67993=ADVANCED_FACE('',(#7243),#1647,.T.);
#67994=ADVANCED_FACE('',(#7244),#1648,.T.);
#67995=ADVANCED_FACE('',(#7245),#4857,.T.);
#67996=ADVANCED_FACE('',(#7246),#1649,.T.);
#67997=ADVANCED_FACE('',(#7247),#1650,.T.);
#67998=ADVANCED_FACE('',(#7248),#4858,.T.);
#67999=ADVANCED_FACE('',(#7249),#1651,.T.);
#68000=ADVANCED_FACE('',(#7250),#1652,.T.);
#68001=ADVANCED_FACE('',(#7251),#4859,.T.);
#68002=ADVANCED_FACE('',(#7252),#1653,.T.);
#68003=ADVANCED_FACE('',(#7253),#1654,.T.);
#68004=ADVANCED_FACE('',(#7254),#4860,.T.);
#68005=ADVANCED_FACE('',(#7255),#1655,.T.);
#68006=ADVANCED_FACE('',(#7256),#1656,.T.);
#68007=ADVANCED_FACE('',(#7257),#4861,.T.);
#68008=ADVANCED_FACE('',(#7258),#1657,.T.);
#68009=ADVANCED_FACE('',(#7259),#1658,.T.);
#68010=ADVANCED_FACE('',(#7260),#4862,.T.);
#68011=ADVANCED_FACE('',(#7261),#1659,.T.);
#68012=ADVANCED_FACE('',(#7262),#1660,.T.);
#68013=ADVANCED_FACE('',(#7263),#4863,.T.);
#68014=ADVANCED_FACE('',(#7264),#1661,.T.);
#68015=ADVANCED_FACE('',(#7265),#1662,.T.);
#68016=ADVANCED_FACE('',(#7266),#4864,.T.);
#68017=ADVANCED_FACE('',(#7267),#1663,.T.);
#68018=ADVANCED_FACE('',(#7268),#1664,.T.);
#68019=ADVANCED_FACE('',(#7269),#4865,.T.);
#68020=ADVANCED_FACE('',(#7270),#1665,.T.);
#68021=ADVANCED_FACE('',(#7271),#1666,.T.);
#68022=ADVANCED_FACE('',(#7272),#4866,.T.);
#68023=ADVANCED_FACE('',(#7273),#1667,.T.);
#68024=ADVANCED_FACE('',(#7274),#1668,.T.);
#68025=ADVANCED_FACE('',(#7275),#4867,.T.);
#68026=ADVANCED_FACE('',(#7276),#1669,.T.);
#68027=ADVANCED_FACE('',(#7277),#1670,.T.);
#68028=ADVANCED_FACE('',(#7278),#4868,.T.);
#68029=ADVANCED_FACE('',(#7279),#1671,.T.);
#68030=ADVANCED_FACE('',(#7280),#1672,.T.);
#68031=ADVANCED_FACE('',(#7281),#1673,.T.);
#68032=ADVANCED_FACE('',(#7282),#1674,.T.);
#68033=ADVANCED_FACE('',(#7283),#4869,.T.);
#68034=ADVANCED_FACE('',(#7284),#1675,.T.);
#68035=ADVANCED_FACE('',(#7285),#1676,.T.);
#68036=ADVANCED_FACE('',(#7286),#4870,.T.);
#68037=ADVANCED_FACE('',(#7287),#1677,.T.);
#68038=ADVANCED_FACE('',(#7288),#1678,.T.);
#68039=ADVANCED_FACE('',(#7289),#4871,.T.);
#68040=ADVANCED_FACE('',(#7290),#1679,.T.);
#68041=ADVANCED_FACE('',(#7291),#1680,.T.);
#68042=ADVANCED_FACE('',(#7292),#4872,.T.);
#68043=ADVANCED_FACE('',(#7293),#1681,.T.);
#68044=ADVANCED_FACE('',(#7294),#1682,.T.);
#68045=ADVANCED_FACE('',(#7295),#4873,.T.);
#68046=ADVANCED_FACE('',(#7296),#1683,.T.);
#68047=ADVANCED_FACE('',(#7297),#1684,.T.);
#68048=ADVANCED_FACE('',(#7298),#4874,.T.);
#68049=ADVANCED_FACE('',(#7299),#1685,.T.);
#68050=ADVANCED_FACE('',(#7300),#1686,.T.);
#68051=ADVANCED_FACE('',(#7301),#4875,.T.);
#68052=ADVANCED_FACE('',(#7302),#1687,.T.);
#68053=ADVANCED_FACE('',(#7303),#1688,.T.);
#68054=ADVANCED_FACE('',(#7304),#4876,.T.);
#68055=ADVANCED_FACE('',(#7305),#1689,.T.);
#68056=ADVANCED_FACE('',(#7306),#1690,.T.);
#68057=ADVANCED_FACE('',(#7307),#4877,.T.);
#68058=ADVANCED_FACE('',(#7308),#1691,.T.);
#68059=ADVANCED_FACE('',(#7309),#1692,.T.);
#68060=ADVANCED_FACE('',(#7310),#4878,.T.);
#68061=ADVANCED_FACE('',(#7311),#1693,.T.);
#68062=ADVANCED_FACE('',(#7312),#1694,.T.);
#68063=ADVANCED_FACE('',(#7313),#4879,.T.);
#68064=ADVANCED_FACE('',(#7314),#1695,.T.);
#68065=ADVANCED_FACE('',(#7315),#1696,.T.);
#68066=ADVANCED_FACE('',(#7316),#4880,.T.);
#68067=ADVANCED_FACE('',(#7317),#1697,.T.);
#68068=ADVANCED_FACE('',(#7318),#1698,.T.);
#68069=ADVANCED_FACE('',(#7319),#4881,.T.);
#68070=ADVANCED_FACE('',(#7320),#1699,.T.);
#68071=ADVANCED_FACE('',(#7321),#1700,.T.);
#68072=ADVANCED_FACE('',(#7322),#4882,.T.);
#68073=ADVANCED_FACE('',(#7323),#4883,.T.);
#68074=ADVANCED_FACE('',(#7324),#1701,.T.);
#68075=ADVANCED_FACE('',(#7325),#1702,.T.);
#68076=ADVANCED_FACE('',(#7326),#1703,.T.);
#68077=ADVANCED_FACE('',(#7327),#1704,.T.);
#68078=ADVANCED_FACE('',(#7328),#1705,.T.);
#68079=ADVANCED_FACE('',(#7329),#1706,.T.);
#68080=ADVANCED_FACE('',(#7330),#1707,.T.);
#68081=ADVANCED_FACE('',(#7331),#1708,.T.);
#68082=ADVANCED_FACE('',(#7332),#1709,.T.);
#68083=ADVANCED_FACE('',(#7333),#1710,.T.);
#68084=ADVANCED_FACE('',(#7334),#1711,.T.);
#68085=ADVANCED_FACE('',(#7335),#1712,.T.);
#68086=ADVANCED_FACE('',(#7336),#1713,.T.);
#68087=ADVANCED_FACE('',(#7337),#1714,.T.);
#68088=ADVANCED_FACE('',(#7338),#1715,.T.);
#68089=ADVANCED_FACE('',(#7339),#1716,.T.);
#68090=ADVANCED_FACE('',(#7340),#1717,.T.);
#68091=ADVANCED_FACE('',(#7341),#1718,.T.);
#68092=ADVANCED_FACE('',(#7342),#1719,.T.);
#68093=ADVANCED_FACE('',(#7343),#1720,.T.);
#68094=ADVANCED_FACE('',(#7344),#1721,.T.);
#68095=ADVANCED_FACE('',(#7345),#1722,.T.);
#68096=ADVANCED_FACE('',(#7346),#1723,.T.);
#68097=ADVANCED_FACE('',(#7347),#1724,.T.);
#68098=ADVANCED_FACE('',(#7348),#1725,.T.);
#68099=ADVANCED_FACE('',(#7349),#1726,.T.);
#68100=ADVANCED_FACE('',(#7350),#1727,.T.);
#68101=ADVANCED_FACE('',(#7351),#1728,.T.);
#68102=ADVANCED_FACE('',(#7352),#1729,.T.);
#68103=ADVANCED_FACE('',(#7353),#1730,.T.);
#68104=ADVANCED_FACE('',(#7354),#1731,.T.);
#68105=ADVANCED_FACE('',(#7355),#1732,.T.);
#68106=ADVANCED_FACE('',(#7356),#1733,.T.);
#68107=ADVANCED_FACE('',(#7357),#1734,.T.);
#68108=ADVANCED_FACE('',(#7358),#1735,.T.);
#68109=ADVANCED_FACE('',(#7359),#1736,.T.);
#68110=ADVANCED_FACE('',(#7360),#1737,.T.);
#68111=ADVANCED_FACE('',(#7361),#1738,.T.);
#68112=ADVANCED_FACE('',(#7362),#1739,.T.);
#68113=ADVANCED_FACE('',(#7363),#1740,.T.);
#68114=ADVANCED_FACE('',(#7364),#1741,.T.);
#68115=ADVANCED_FACE('',(#7365),#1742,.T.);
#68116=ADVANCED_FACE('',(#7366),#1743,.T.);
#68117=ADVANCED_FACE('',(#7367),#1744,.T.);
#68118=ADVANCED_FACE('',(#7368),#1745,.T.);
#68119=ADVANCED_FACE('',(#7369),#1746,.T.);
#68120=ADVANCED_FACE('',(#7370),#1747,.T.);
#68121=ADVANCED_FACE('',(#7371),#1748,.T.);
#68122=ADVANCED_FACE('',(#7372),#1749,.T.);
#68123=ADVANCED_FACE('',(#7373),#1750,.T.);
#68124=ADVANCED_FACE('',(#7374),#1751,.T.);
#68125=ADVANCED_FACE('',(#7375),#1752,.T.);
#68126=ADVANCED_FACE('',(#7376),#1753,.T.);
#68127=ADVANCED_FACE('',(#7377),#1754,.T.);
#68128=ADVANCED_FACE('',(#7378),#1755,.T.);
#68129=ADVANCED_FACE('',(#7379),#1756,.T.);
#68130=ADVANCED_FACE('',(#7380),#1757,.T.);
#68131=ADVANCED_FACE('',(#7381),#1758,.T.);
#68132=ADVANCED_FACE('',(#7382),#1759,.T.);
#68133=ADVANCED_FACE('',(#7383),#1760,.T.);
#68134=ADVANCED_FACE('',(#7384),#1761,.T.);
#68135=ADVANCED_FACE('',(#7385),#1762,.T.);
#68136=ADVANCED_FACE('',(#7386),#1763,.T.);
#68137=ADVANCED_FACE('',(#7387),#1764,.T.);
#68138=ADVANCED_FACE('',(#7388),#1765,.T.);
#68139=ADVANCED_FACE('',(#7389),#1766,.T.);
#68140=ADVANCED_FACE('',(#7390),#1767,.T.);
#68141=ADVANCED_FACE('',(#7391),#1768,.T.);
#68142=ADVANCED_FACE('',(#7392),#1769,.T.);
#68143=ADVANCED_FACE('',(#7393),#1770,.T.);
#68144=ADVANCED_FACE('',(#7394),#1771,.T.);
#68145=ADVANCED_FACE('',(#7395),#1772,.T.);
#68146=ADVANCED_FACE('',(#7396),#1773,.T.);
#68147=ADVANCED_FACE('',(#7397),#1774,.T.);
#68148=ADVANCED_FACE('',(#7398),#1775,.T.);
#68149=ADVANCED_FACE('',(#7399),#1776,.T.);
#68150=ADVANCED_FACE('',(#7400),#1777,.T.);
#68151=ADVANCED_FACE('',(#7401),#1778,.T.);
#68152=ADVANCED_FACE('',(#7402),#1779,.T.);
#68153=ADVANCED_FACE('',(#7403),#1780,.T.);
#68154=ADVANCED_FACE('',(#7404),#1781,.T.);
#68155=ADVANCED_FACE('',(#7405),#1782,.T.);
#68156=ADVANCED_FACE('',(#7406),#1783,.T.);
#68157=ADVANCED_FACE('',(#7407),#1784,.T.);
#68158=ADVANCED_FACE('',(#7408),#1785,.T.);
#68159=ADVANCED_FACE('',(#7409),#1786,.T.);
#68160=ADVANCED_FACE('',(#7410),#1787,.T.);
#68161=ADVANCED_FACE('',(#7411),#1788,.T.);
#68162=ADVANCED_FACE('',(#7412),#1789,.T.);
#68163=ADVANCED_FACE('',(#7413),#1790,.T.);
#68164=ADVANCED_FACE('',(#7414),#1791,.T.);
#68165=ADVANCED_FACE('',(#7415),#1792,.T.);
#68166=ADVANCED_FACE('',(#7416),#1793,.T.);
#68167=ADVANCED_FACE('',(#7417),#1794,.T.);
#68168=ADVANCED_FACE('',(#7418),#1795,.T.);
#68169=ADVANCED_FACE('',(#7419),#1796,.T.);
#68170=ADVANCED_FACE('',(#7420),#1797,.T.);
#68171=ADVANCED_FACE('',(#7421),#1798,.T.);
#68172=ADVANCED_FACE('',(#7422),#1799,.T.);
#68173=ADVANCED_FACE('',(#7423),#1800,.T.);
#68174=ADVANCED_FACE('',(#7424),#1801,.T.);
#68175=ADVANCED_FACE('',(#7425),#1802,.T.);
#68176=ADVANCED_FACE('',(#7426),#1803,.T.);
#68177=ADVANCED_FACE('',(#7427),#1804,.T.);
#68178=ADVANCED_FACE('',(#7428),#1805,.T.);
#68179=ADVANCED_FACE('',(#7429),#1806,.T.);
#68180=ADVANCED_FACE('',(#7430),#1807,.T.);
#68181=ADVANCED_FACE('',(#7431),#1808,.T.);
#68182=ADVANCED_FACE('',(#7432),#1809,.T.);
#68183=ADVANCED_FACE('',(#7433),#1810,.T.);
#68184=ADVANCED_FACE('',(#7434),#1811,.T.);
#68185=ADVANCED_FACE('',(#7435),#1812,.T.);
#68186=ADVANCED_FACE('',(#7436),#1813,.T.);
#68187=ADVANCED_FACE('',(#7437),#1814,.T.);
#68188=ADVANCED_FACE('',(#7438),#1815,.T.);
#68189=ADVANCED_FACE('',(#7439),#1816,.T.);
#68190=ADVANCED_FACE('',(#7440),#1817,.T.);
#68191=ADVANCED_FACE('',(#7441),#1818,.T.);
#68192=ADVANCED_FACE('',(#7442),#4884,.T.);
#68193=ADVANCED_FACE('',(#7443),#1819,.T.);
#68194=ADVANCED_FACE('',(#7444),#1820,.T.);
#68195=ADVANCED_FACE('',(#7445),#4885,.T.);
#68196=ADVANCED_FACE('',(#7446),#1821,.T.);
#68197=ADVANCED_FACE('',(#7447),#1822,.T.);
#68198=ADVANCED_FACE('',(#7448),#4886,.T.);
#68199=ADVANCED_FACE('',(#7449),#1823,.T.);
#68200=ADVANCED_FACE('',(#7450),#1824,.T.);
#68201=ADVANCED_FACE('',(#7451),#4887,.T.);
#68202=ADVANCED_FACE('',(#7452),#1825,.T.);
#68203=ADVANCED_FACE('',(#7453),#1826,.T.);
#68204=ADVANCED_FACE('',(#7454),#4888,.T.);
#68205=ADVANCED_FACE('',(#7455),#1827,.T.);
#68206=ADVANCED_FACE('',(#7456),#1828,.T.);
#68207=ADVANCED_FACE('',(#7457),#4889,.T.);
#68208=ADVANCED_FACE('',(#7458),#1829,.T.);
#68209=ADVANCED_FACE('',(#7459),#1830,.T.);
#68210=ADVANCED_FACE('',(#7460),#4890,.T.);
#68211=ADVANCED_FACE('',(#7461),#1831,.T.);
#68212=ADVANCED_FACE('',(#7462),#1832,.T.);
#68213=ADVANCED_FACE('',(#7463),#4891,.T.);
#68214=ADVANCED_FACE('',(#7464),#1833,.T.);
#68215=ADVANCED_FACE('',(#7465),#1834,.T.);
#68216=ADVANCED_FACE('',(#7466),#4892,.T.);
#68217=ADVANCED_FACE('',(#7467),#1835,.T.);
#68218=ADVANCED_FACE('',(#7468),#1836,.T.);
#68219=ADVANCED_FACE('',(#7469),#4893,.T.);
#68220=ADVANCED_FACE('',(#7470),#1837,.T.);
#68221=ADVANCED_FACE('',(#7471),#1838,.T.);
#68222=ADVANCED_FACE('',(#7472),#4894,.T.);
#68223=ADVANCED_FACE('',(#7473),#1839,.T.);
#68224=ADVANCED_FACE('',(#7474),#1840,.T.);
#68225=ADVANCED_FACE('',(#7475),#4895,.T.);
#68226=ADVANCED_FACE('',(#7476),#1841,.T.);
#68227=ADVANCED_FACE('',(#7477),#1842,.T.);
#68228=ADVANCED_FACE('',(#7478),#4896,.T.);
#68229=ADVANCED_FACE('',(#7479),#1843,.T.);
#68230=ADVANCED_FACE('',(#7480),#1844,.T.);
#68231=ADVANCED_FACE('',(#7481),#4897,.T.);
#68232=ADVANCED_FACE('',(#7482),#1845,.T.);
#68233=ADVANCED_FACE('',(#7483),#1846,.T.);
#68234=ADVANCED_FACE('',(#7484),#1847,.T.);
#68235=ADVANCED_FACE('',(#7485),#1848,.T.);
#68236=ADVANCED_FACE('',(#7486),#4898,.T.);
#68237=ADVANCED_FACE('',(#7487),#1849,.T.);
#68238=ADVANCED_FACE('',(#7488),#1850,.T.);
#68239=ADVANCED_FACE('',(#7489),#4899,.T.);
#68240=ADVANCED_FACE('',(#7490),#1851,.T.);
#68241=ADVANCED_FACE('',(#7491),#1852,.T.);
#68242=ADVANCED_FACE('',(#7492),#4900,.T.);
#68243=ADVANCED_FACE('',(#7493),#1853,.T.);
#68244=ADVANCED_FACE('',(#7494),#1854,.T.);
#68245=ADVANCED_FACE('',(#7495),#4901,.T.);
#68246=ADVANCED_FACE('',(#7496),#1855,.T.);
#68247=ADVANCED_FACE('',(#7497),#1856,.T.);
#68248=ADVANCED_FACE('',(#7498),#4902,.T.);
#68249=ADVANCED_FACE('',(#7499),#1857,.T.);
#68250=ADVANCED_FACE('',(#7500),#1858,.T.);
#68251=ADVANCED_FACE('',(#7501),#4903,.T.);
#68252=ADVANCED_FACE('',(#7502),#1859,.T.);
#68253=ADVANCED_FACE('',(#7503),#1860,.T.);
#68254=ADVANCED_FACE('',(#7504),#1861,.T.);
#68255=ADVANCED_FACE('',(#7505),#4904,.T.);
#68256=ADVANCED_FACE('',(#7506),#1862,.T.);
#68257=ADVANCED_FACE('',(#7507),#4905,.T.);
#68258=ADVANCED_FACE('',(#7508),#1863,.T.);
#68259=ADVANCED_FACE('',(#7509),#1864,.T.);
#68260=ADVANCED_FACE('',(#7510),#4906,.T.);
#68261=ADVANCED_FACE('',(#7511),#1865,.T.);
#68262=ADVANCED_FACE('',(#7512),#1866,.T.);
#68263=ADVANCED_FACE('',(#7513),#4907,.T.);
#68264=ADVANCED_FACE('',(#7514),#1867,.T.);
#68265=ADVANCED_FACE('',(#7515),#1868,.T.);
#68266=ADVANCED_FACE('',(#7516),#4908,.T.);
#68267=ADVANCED_FACE('',(#7517),#1869,.T.);
#68268=ADVANCED_FACE('',(#7518),#1870,.T.);
#68269=ADVANCED_FACE('',(#7519),#4909,.T.);
#68270=ADVANCED_FACE('',(#7520),#1871,.T.);
#68271=ADVANCED_FACE('',(#7521),#1872,.T.);
#68272=ADVANCED_FACE('',(#7522),#4910,.T.);
#68273=ADVANCED_FACE('',(#7523),#1873,.T.);
#68274=ADVANCED_FACE('',(#7524),#1874,.T.);
#68275=ADVANCED_FACE('',(#7525),#4911,.T.);
#68276=ADVANCED_FACE('',(#7526),#1875,.T.);
#68277=ADVANCED_FACE('',(#7527),#1876,.T.);
#68278=ADVANCED_FACE('',(#7528),#1877,.T.);
#68279=ADVANCED_FACE('',(#7529),#4912,.T.);
#68280=ADVANCED_FACE('',(#7530),#1878,.T.);
#68281=ADVANCED_FACE('',(#7531),#1879,.T.);
#68282=ADVANCED_FACE('',(#7532),#4913,.T.);
#68283=ADVANCED_FACE('',(#7533),#1880,.T.);
#68284=ADVANCED_FACE('',(#7534),#1881,.T.);
#68285=ADVANCED_FACE('',(#7535),#4914,.T.);
#68286=ADVANCED_FACE('',(#7536),#1882,.T.);
#68287=ADVANCED_FACE('',(#7537),#1883,.T.);
#68288=ADVANCED_FACE('',(#7538),#4915,.T.);
#68289=ADVANCED_FACE('',(#7539),#1884,.T.);
#68290=ADVANCED_FACE('',(#7540),#1885,.T.);
#68291=ADVANCED_FACE('',(#7541),#4916,.T.);
#68292=ADVANCED_FACE('',(#7542),#1886,.T.);
#68293=ADVANCED_FACE('',(#7543),#1887,.T.);
#68294=ADVANCED_FACE('',(#7544),#4917,.T.);
#68295=ADVANCED_FACE('',(#7545),#1888,.T.);
#68296=ADVANCED_FACE('',(#7546),#1889,.T.);
#68297=ADVANCED_FACE('',(#7547),#4918,.T.);
#68298=ADVANCED_FACE('',(#7548),#1890,.T.);
#68299=ADVANCED_FACE('',(#7549),#1891,.T.);
#68300=ADVANCED_FACE('',(#7550),#4919,.T.);
#68301=ADVANCED_FACE('',(#7551),#1892,.T.);
#68302=ADVANCED_FACE('',(#7552),#1893,.T.);
#68303=ADVANCED_FACE('',(#7553),#4920,.T.);
#68304=ADVANCED_FACE('',(#7554),#1894,.T.);
#68305=ADVANCED_FACE('',(#7555),#1895,.T.);
#68306=ADVANCED_FACE('',(#7556),#4921,.T.);
#68307=ADVANCED_FACE('',(#7557),#1896,.T.);
#68308=ADVANCED_FACE('',(#7558),#1897,.T.);
#68309=ADVANCED_FACE('',(#7559),#4922,.T.);
#68310=ADVANCED_FACE('',(#7560),#1898,.T.);
#68311=ADVANCED_FACE('',(#7561),#1899,.T.);
#68312=ADVANCED_FACE('',(#7562),#4923,.T.);
#68313=ADVANCED_FACE('',(#7563),#1900,.T.);
#68314=ADVANCED_FACE('',(#7564),#1901,.T.);
#68315=ADVANCED_FACE('',(#7565),#4924,.T.);
#68316=ADVANCED_FACE('',(#7566),#1902,.T.);
#68317=ADVANCED_FACE('',(#7567),#1903,.T.);
#68318=ADVANCED_FACE('',(#7568),#4925,.T.);
#68319=ADVANCED_FACE('',(#7569),#1904,.T.);
#68320=ADVANCED_FACE('',(#7570),#1905,.T.);
#68321=ADVANCED_FACE('',(#7571),#4926,.T.);
#68322=ADVANCED_FACE('',(#7572),#1906,.T.);
#68323=ADVANCED_FACE('',(#7573),#1907,.T.);
#68324=ADVANCED_FACE('',(#7574),#4927,.T.);
#68325=ADVANCED_FACE('',(#7575),#1908,.T.);
#68326=ADVANCED_FACE('',(#7576),#1909,.T.);
#68327=ADVANCED_FACE('',(#7577),#4928,.T.);
#68328=ADVANCED_FACE('',(#7578),#1910,.T.);
#68329=ADVANCED_FACE('',(#7579),#1911,.T.);
#68330=ADVANCED_FACE('',(#7580),#4929,.T.);
#68331=ADVANCED_FACE('',(#7581),#1912,.T.);
#68332=ADVANCED_FACE('',(#7582),#1913,.T.);
#68333=ADVANCED_FACE('',(#7583),#4930,.T.);
#68334=ADVANCED_FACE('',(#7584),#1914,.T.);
#68335=ADVANCED_FACE('',(#7585),#1915,.T.);
#68336=ADVANCED_FACE('',(#7586),#4931,.T.);
#68337=ADVANCED_FACE('',(#7587),#1916,.T.);
#68338=ADVANCED_FACE('',(#7588),#1917,.T.);
#68339=ADVANCED_FACE('',(#7589),#4932,.T.);
#68340=ADVANCED_FACE('',(#7590),#1918,.T.);
#68341=ADVANCED_FACE('',(#7591),#1919,.T.);
#68342=ADVANCED_FACE('',(#7592),#1920,.T.);
#68343=ADVANCED_FACE('',(#7593),#1921,.T.);
#68344=ADVANCED_FACE('',(#7594),#4933,.T.);
#68345=ADVANCED_FACE('',(#7595),#1922,.T.);
#68346=ADVANCED_FACE('',(#7596),#1923,.T.);
#68347=ADVANCED_FACE('',(#7597),#4934,.T.);
#68348=ADVANCED_FACE('',(#7598),#1924,.T.);
#68349=ADVANCED_FACE('',(#7599),#1925,.T.);
#68350=ADVANCED_FACE('',(#7600),#4935,.T.);
#68351=ADVANCED_FACE('',(#7601),#1926,.T.);
#68352=ADVANCED_FACE('',(#7602),#1927,.T.);
#68353=ADVANCED_FACE('',(#7603),#4936,.T.);
#68354=ADVANCED_FACE('',(#7604),#1928,.T.);
#68355=ADVANCED_FACE('',(#7605),#1929,.T.);
#68356=ADVANCED_FACE('',(#7606),#4937,.T.);
#68357=ADVANCED_FACE('',(#7607),#1930,.T.);
#68358=ADVANCED_FACE('',(#7608),#1931,.T.);
#68359=ADVANCED_FACE('',(#7609),#4938,.T.);
#68360=ADVANCED_FACE('',(#7610),#1932,.T.);
#68361=ADVANCED_FACE('',(#7611),#1933,.T.);
#68362=ADVANCED_FACE('',(#7612),#4939,.T.);
#68363=ADVANCED_FACE('',(#7613),#1934,.T.);
#68364=ADVANCED_FACE('',(#7614),#1935,.T.);
#68365=ADVANCED_FACE('',(#7615),#1936,.T.);
#68366=ADVANCED_FACE('',(#7616),#1937,.T.);
#68367=ADVANCED_FACE('',(#7617),#1938,.T.);
#68368=ADVANCED_FACE('',(#7618),#1939,.T.);
#68369=ADVANCED_FACE('',(#7619),#1940,.T.);
#68370=ADVANCED_FACE('',(#7620),#1941,.T.);
#68371=ADVANCED_FACE('',(#7621),#1942,.T.);
#68372=ADVANCED_FACE('',(#7622),#1943,.T.);
#68373=ADVANCED_FACE('',(#7623),#1944,.T.);
#68374=ADVANCED_FACE('',(#7624),#1945,.T.);
#68375=ADVANCED_FACE('',(#7625),#1946,.T.);
#68376=ADVANCED_FACE('',(#7626),#1947,.T.);
#68377=ADVANCED_FACE('',(#7627),#1948,.T.);
#68378=ADVANCED_FACE('',(#7628),#1949,.T.);
#68379=ADVANCED_FACE('',(#7629),#1950,.T.);
#68380=ADVANCED_FACE('',(#7630),#1951,.T.);
#68381=ADVANCED_FACE('',(#7631),#1952,.T.);
#68382=ADVANCED_FACE('',(#7632),#1953,.T.);
#68383=ADVANCED_FACE('',(#7633),#1954,.T.);
#68384=ADVANCED_FACE('',(#7634),#1955,.T.);
#68385=ADVANCED_FACE('',(#7635),#1956,.T.);
#68386=ADVANCED_FACE('',(#7636),#1957,.T.);
#68387=ADVANCED_FACE('',(#7637),#1958,.T.);
#68388=ADVANCED_FACE('',(#7638),#1959,.T.);
#68389=ADVANCED_FACE('',(#7639),#1960,.T.);
#68390=ADVANCED_FACE('',(#7640),#1961,.T.);
#68391=ADVANCED_FACE('',(#7641),#1962,.T.);
#68392=ADVANCED_FACE('',(#7642),#1963,.T.);
#68393=ADVANCED_FACE('',(#7643),#1964,.T.);
#68394=ADVANCED_FACE('',(#7644),#1965,.T.);
#68395=ADVANCED_FACE('',(#7645),#1966,.T.);
#68396=ADVANCED_FACE('',(#7646),#1967,.T.);
#68397=ADVANCED_FACE('',(#7647),#1968,.T.);
#68398=ADVANCED_FACE('',(#7648),#1969,.T.);
#68399=ADVANCED_FACE('',(#7649),#1970,.T.);
#68400=ADVANCED_FACE('',(#7650),#1971,.T.);
#68401=ADVANCED_FACE('',(#7651),#1972,.T.);
#68402=ADVANCED_FACE('',(#7652),#1973,.T.);
#68403=ADVANCED_FACE('',(#7653),#1974,.T.);
#68404=ADVANCED_FACE('',(#7654),#1975,.T.);
#68405=ADVANCED_FACE('',(#7655),#1976,.T.);
#68406=ADVANCED_FACE('',(#7656),#1977,.T.);
#68407=ADVANCED_FACE('',(#7657),#1978,.T.);
#68408=ADVANCED_FACE('',(#7658),#1979,.T.);
#68409=ADVANCED_FACE('',(#7659),#1980,.T.);
#68410=ADVANCED_FACE('',(#7660),#1981,.T.);
#68411=ADVANCED_FACE('',(#7661),#1982,.T.);
#68412=ADVANCED_FACE('',(#7662),#1983,.T.);
#68413=ADVANCED_FACE('',(#7663),#1984,.T.);
#68414=ADVANCED_FACE('',(#7664),#1985,.T.);
#68415=ADVANCED_FACE('',(#7665),#1986,.T.);
#68416=ADVANCED_FACE('',(#7666),#1987,.T.);
#68417=ADVANCED_FACE('',(#7667),#1988,.T.);
#68418=ADVANCED_FACE('',(#7668),#1989,.T.);
#68419=ADVANCED_FACE('',(#7669),#1990,.T.);
#68420=ADVANCED_FACE('',(#7670),#1991,.T.);
#68421=ADVANCED_FACE('',(#7671),#1992,.T.);
#68422=ADVANCED_FACE('',(#7672),#1993,.T.);
#68423=ADVANCED_FACE('',(#7673),#1994,.T.);
#68424=ADVANCED_FACE('',(#7674),#1995,.T.);
#68425=ADVANCED_FACE('',(#7675),#1996,.T.);
#68426=ADVANCED_FACE('',(#7676),#1997,.T.);
#68427=ADVANCED_FACE('',(#7677),#1998,.T.);
#68428=ADVANCED_FACE('',(#7678),#1999,.T.);
#68429=ADVANCED_FACE('',(#7679),#2000,.T.);
#68430=ADVANCED_FACE('',(#7680),#2001,.T.);
#68431=ADVANCED_FACE('',(#7681),#2002,.T.);
#68432=ADVANCED_FACE('',(#7682),#2003,.T.);
#68433=ADVANCED_FACE('',(#7683),#2004,.T.);
#68434=ADVANCED_FACE('',(#7684),#2005,.T.);
#68435=ADVANCED_FACE('',(#7685),#2006,.T.);
#68436=ADVANCED_FACE('',(#7686),#2007,.T.);
#68437=ADVANCED_FACE('',(#7687),#2008,.T.);
#68438=ADVANCED_FACE('',(#7688),#2009,.T.);
#68439=ADVANCED_FACE('',(#7689),#2010,.T.);
#68440=ADVANCED_FACE('',(#7690),#2011,.T.);
#68441=ADVANCED_FACE('',(#7691),#2012,.T.);
#68442=ADVANCED_FACE('',(#7692),#2013,.T.);
#68443=ADVANCED_FACE('',(#7693),#2014,.T.);
#68444=ADVANCED_FACE('',(#7694),#2015,.T.);
#68445=ADVANCED_FACE('',(#7695),#2016,.T.);
#68446=ADVANCED_FACE('',(#7696),#2017,.T.);
#68447=ADVANCED_FACE('',(#7697),#2018,.T.);
#68448=ADVANCED_FACE('',(#7698),#2019,.T.);
#68449=ADVANCED_FACE('',(#7699),#2020,.T.);
#68450=ADVANCED_FACE('',(#7700),#2021,.T.);
#68451=ADVANCED_FACE('',(#7701),#2022,.T.);
#68452=ADVANCED_FACE('',(#7702),#2023,.T.);
#68453=ADVANCED_FACE('',(#7703),#2024,.T.);
#68454=ADVANCED_FACE('',(#7704),#2025,.T.);
#68455=ADVANCED_FACE('',(#7705),#2026,.T.);
#68456=ADVANCED_FACE('',(#7706),#2027,.T.);
#68457=ADVANCED_FACE('',(#7707),#2028,.T.);
#68458=ADVANCED_FACE('',(#7708),#2029,.T.);
#68459=ADVANCED_FACE('',(#7709),#2030,.T.);
#68460=ADVANCED_FACE('',(#7710),#2031,.T.);
#68461=ADVANCED_FACE('',(#7711),#2032,.T.);
#68462=ADVANCED_FACE('',(#7712),#2033,.T.);
#68463=ADVANCED_FACE('',(#7713),#2034,.T.);
#68464=ADVANCED_FACE('',(#7714),#2035,.T.);
#68465=ADVANCED_FACE('',(#7715),#2036,.T.);
#68466=ADVANCED_FACE('',(#7716),#2037,.T.);
#68467=ADVANCED_FACE('',(#7717),#2038,.T.);
#68468=ADVANCED_FACE('',(#7718),#2039,.T.);
#68469=ADVANCED_FACE('',(#7719),#2040,.T.);
#68470=ADVANCED_FACE('',(#7720),#2041,.T.);
#68471=ADVANCED_FACE('',(#7721),#2042,.T.);
#68472=ADVANCED_FACE('',(#7722),#2043,.T.);
#68473=ADVANCED_FACE('',(#7723),#2044,.T.);
#68474=ADVANCED_FACE('',(#7724),#2045,.T.);
#68475=ADVANCED_FACE('',(#7725),#2046,.T.);
#68476=ADVANCED_FACE('',(#7726),#2047,.T.);
#68477=ADVANCED_FACE('',(#7727),#2048,.T.);
#68478=ADVANCED_FACE('',(#7728),#2049,.T.);
#68479=ADVANCED_FACE('',(#7729),#2050,.T.);
#68480=ADVANCED_FACE('',(#7730),#2051,.T.);
#68481=ADVANCED_FACE('',(#7731),#4940,.T.);
#68482=ADVANCED_FACE('',(#7732),#2052,.T.);
#68483=ADVANCED_FACE('',(#7733),#2053,.T.);
#68484=ADVANCED_FACE('',(#7734),#4941,.T.);
#68485=ADVANCED_FACE('',(#7735),#2054,.T.);
#68486=ADVANCED_FACE('',(#7736),#2055,.T.);
#68487=ADVANCED_FACE('',(#7737),#4942,.T.);
#68488=ADVANCED_FACE('',(#7738),#2056,.T.);
#68489=ADVANCED_FACE('',(#7739),#2057,.T.);
#68490=ADVANCED_FACE('',(#7740),#4943,.T.);
#68491=ADVANCED_FACE('',(#7741),#2058,.T.);
#68492=ADVANCED_FACE('',(#7742),#2059,.T.);
#68493=ADVANCED_FACE('',(#7743),#4944,.T.);
#68494=ADVANCED_FACE('',(#7744),#2060,.T.);
#68495=ADVANCED_FACE('',(#7745),#2061,.T.);
#68496=ADVANCED_FACE('',(#7746),#4945,.T.);
#68497=ADVANCED_FACE('',(#7747),#2062,.T.);
#68498=ADVANCED_FACE('',(#7748),#2063,.T.);
#68499=ADVANCED_FACE('',(#7749),#2064,.T.);
#68500=ADVANCED_FACE('',(#7750),#2065,.T.);
#68501=ADVANCED_FACE('',(#7751),#4946,.T.);
#68502=ADVANCED_FACE('',(#7752),#2066,.T.);
#68503=ADVANCED_FACE('',(#7753),#2067,.T.);
#68504=ADVANCED_FACE('',(#7754),#4947,.T.);
#68505=ADVANCED_FACE('',(#7755),#2068,.T.);
#68506=ADVANCED_FACE('',(#7756),#2069,.T.);
#68507=ADVANCED_FACE('',(#7757),#4948,.T.);
#68508=ADVANCED_FACE('',(#7758),#2070,.T.);
#68509=ADVANCED_FACE('',(#7759),#2071,.T.);
#68510=ADVANCED_FACE('',(#7760),#4949,.T.);
#68511=ADVANCED_FACE('',(#7761),#2072,.T.);
#68512=ADVANCED_FACE('',(#7762),#2073,.T.);
#68513=ADVANCED_FACE('',(#7763),#4950,.T.);
#68514=ADVANCED_FACE('',(#7764),#2074,.T.);
#68515=ADVANCED_FACE('',(#7765),#2075,.T.);
#68516=ADVANCED_FACE('',(#7766),#4951,.T.);
#68517=ADVANCED_FACE('',(#7767),#2076,.T.);
#68518=ADVANCED_FACE('',(#7768),#2077,.T.);
#68519=ADVANCED_FACE('',(#7769),#4952,.T.);
#68520=ADVANCED_FACE('',(#7770),#2078,.T.);
#68521=ADVANCED_FACE('',(#7771),#2079,.T.);
#68522=ADVANCED_FACE('',(#7772),#4953,.T.);
#68523=ADVANCED_FACE('',(#7773),#2080,.T.);
#68524=ADVANCED_FACE('',(#7774),#2081,.T.);
#68525=ADVANCED_FACE('',(#7775),#4954,.T.);
#68526=ADVANCED_FACE('',(#7776),#2082,.T.);
#68527=ADVANCED_FACE('',(#7777),#2083,.T.);
#68528=ADVANCED_FACE('',(#7778),#4955,.T.);
#68529=ADVANCED_FACE('',(#7779),#2084,.T.);
#68530=ADVANCED_FACE('',(#7780),#2085,.T.);
#68531=ADVANCED_FACE('',(#7781),#4956,.T.);
#68532=ADVANCED_FACE('',(#7782),#2086,.T.);
#68533=ADVANCED_FACE('',(#7783),#2087,.T.);
#68534=ADVANCED_FACE('',(#7784),#4957,.T.);
#68535=ADVANCED_FACE('',(#7785),#2088,.T.);
#68536=ADVANCED_FACE('',(#7786),#2089,.T.);
#68537=ADVANCED_FACE('',(#7787),#4958,.T.);
#68538=ADVANCED_FACE('',(#7788),#2090,.T.);
#68539=ADVANCED_FACE('',(#7789),#2091,.T.);
#68540=ADVANCED_FACE('',(#7790),#2092,.T.);
#68541=ADVANCED_FACE('',(#7791),#4959,.T.);
#68542=ADVANCED_FACE('',(#7792),#2093,.T.);
#68543=ADVANCED_FACE('',(#7793),#4960,.T.);
#68544=ADVANCED_FACE('',(#7794),#2094,.T.);
#68545=ADVANCED_FACE('',(#7795),#2095,.T.);
#68546=ADVANCED_FACE('',(#7796),#4961,.T.);
#68547=ADVANCED_FACE('',(#7797),#2096,.T.);
#68548=ADVANCED_FACE('',(#7798),#2097,.T.);
#68549=ADVANCED_FACE('',(#7799),#4962,.T.);
#68550=ADVANCED_FACE('',(#7800),#2098,.T.);
#68551=ADVANCED_FACE('',(#7801),#2099,.T.);
#68552=ADVANCED_FACE('',(#7802),#4963,.T.);
#68553=ADVANCED_FACE('',(#7803),#2100,.T.);
#68554=ADVANCED_FACE('',(#7804),#2101,.T.);
#68555=ADVANCED_FACE('',(#7805),#4964,.T.);
#68556=ADVANCED_FACE('',(#7806),#2102,.T.);
#68557=ADVANCED_FACE('',(#7807),#2103,.T.);
#68558=ADVANCED_FACE('',(#7808),#4965,.T.);
#68559=ADVANCED_FACE('',(#7809),#2104,.T.);
#68560=ADVANCED_FACE('',(#7810),#2105,.T.);
#68561=ADVANCED_FACE('',(#7811),#4966,.T.);
#68562=ADVANCED_FACE('',(#7812),#2106,.T.);
#68563=ADVANCED_FACE('',(#7813),#4967,.T.);
#68564=ADVANCED_FACE('',(#7814),#2107,.T.);
#68565=ADVANCED_FACE('',(#7815),#2108,.T.);
#68566=ADVANCED_FACE('',(#7816),#2109,.T.);
#68567=ADVANCED_FACE('',(#7817),#2110,.T.);
#68568=ADVANCED_FACE('',(#7818),#4968,.T.);
#68569=ADVANCED_FACE('',(#7819),#2111,.T.);
#68570=ADVANCED_FACE('',(#7820),#2112,.T.);
#68571=ADVANCED_FACE('',(#7821),#4969,.T.);
#68572=ADVANCED_FACE('',(#7822),#2113,.T.);
#68573=ADVANCED_FACE('',(#7823),#2114,.T.);
#68574=ADVANCED_FACE('',(#7824),#4970,.T.);
#68575=ADVANCED_FACE('',(#7825),#2115,.T.);
#68576=ADVANCED_FACE('',(#7826),#2116,.T.);
#68577=ADVANCED_FACE('',(#7827),#4971,.T.);
#68578=ADVANCED_FACE('',(#7828),#2117,.T.);
#68579=ADVANCED_FACE('',(#7829),#2118,.T.);
#68580=ADVANCED_FACE('',(#7830),#4972,.T.);
#68581=ADVANCED_FACE('',(#7831),#2119,.T.);
#68582=ADVANCED_FACE('',(#7832),#2120,.T.);
#68583=ADVANCED_FACE('',(#7833),#4973,.T.);
#68584=ADVANCED_FACE('',(#7834),#2121,.T.);
#68585=ADVANCED_FACE('',(#7835),#2122,.T.);
#68586=ADVANCED_FACE('',(#7836),#4974,.T.);
#68587=ADVANCED_FACE('',(#7837),#2123,.T.);
#68588=ADVANCED_FACE('',(#7838),#2124,.T.);
#68589=ADVANCED_FACE('',(#7839),#4975,.T.);
#68590=ADVANCED_FACE('',(#7840),#2125,.T.);
#68591=ADVANCED_FACE('',(#7841),#2126,.T.);
#68592=ADVANCED_FACE('',(#7842),#4976,.T.);
#68593=ADVANCED_FACE('',(#7843),#2127,.T.);
#68594=ADVANCED_FACE('',(#7844),#2128,.T.);
#68595=ADVANCED_FACE('',(#7845),#4977,.T.);
#68596=ADVANCED_FACE('',(#7846),#2129,.T.);
#68597=ADVANCED_FACE('',(#7847),#2130,.T.);
#68598=ADVANCED_FACE('',(#7848),#4978,.T.);
#68599=ADVANCED_FACE('',(#7849),#2131,.T.);
#68600=ADVANCED_FACE('',(#7850),#2132,.T.);
#68601=ADVANCED_FACE('',(#7851),#4979,.T.);
#68602=ADVANCED_FACE('',(#7852),#2133,.T.);
#68603=ADVANCED_FACE('',(#7853),#2134,.T.);
#68604=ADVANCED_FACE('',(#7854),#4980,.T.);
#68605=ADVANCED_FACE('',(#7855),#2135,.T.);
#68606=ADVANCED_FACE('',(#7856),#2136,.T.);
#68607=ADVANCED_FACE('',(#7857),#2137,.T.);
#68608=ADVANCED_FACE('',(#7858),#2138,.T.);
#68609=ADVANCED_FACE('',(#7859),#4981,.T.);
#68610=ADVANCED_FACE('',(#7860),#2139,.T.);
#68611=ADVANCED_FACE('',(#7861),#2140,.T.);
#68612=ADVANCED_FACE('',(#7862),#4982,.T.);
#68613=ADVANCED_FACE('',(#7863),#2141,.T.);
#68614=ADVANCED_FACE('',(#7864),#2142,.T.);
#68615=ADVANCED_FACE('',(#7865),#4983,.T.);
#68616=ADVANCED_FACE('',(#7866),#2143,.T.);
#68617=ADVANCED_FACE('',(#7867),#2144,.T.);
#68618=ADVANCED_FACE('',(#7868),#4984,.T.);
#68619=ADVANCED_FACE('',(#7869),#2145,.T.);
#68620=ADVANCED_FACE('',(#7870),#2146,.T.);
#68621=ADVANCED_FACE('',(#7871),#4985,.T.);
#68622=ADVANCED_FACE('',(#7872),#2147,.T.);
#68623=ADVANCED_FACE('',(#7873),#2148,.T.);
#68624=ADVANCED_FACE('',(#7874),#4986,.T.);
#68625=ADVANCED_FACE('',(#7875),#2149,.T.);
#68626=ADVANCED_FACE('',(#7876),#2150,.T.);
#68627=ADVANCED_FACE('',(#7877),#4987,.T.);
#68628=ADVANCED_FACE('',(#7878),#2151,.T.);
#68629=ADVANCED_FACE('',(#7879),#2152,.T.);
#68630=ADVANCED_FACE('',(#7880),#4988,.T.);
#68631=ADVANCED_FACE('',(#7881),#2153,.T.);
#68632=ADVANCED_FACE('',(#7882),#2154,.T.);
#68633=ADVANCED_FACE('',(#7883),#4989,.T.);
#68634=ADVANCED_FACE('',(#7884),#2155,.T.);
#68635=ADVANCED_FACE('',(#7885),#2156,.T.);
#68636=ADVANCED_FACE('',(#7886),#4990,.T.);
#68637=ADVANCED_FACE('',(#7887),#2157,.T.);
#68638=ADVANCED_FACE('',(#7888),#2158,.T.);
#68639=ADVANCED_FACE('',(#7889),#4991,.T.);
#68640=ADVANCED_FACE('',(#7890),#2159,.T.);
#68641=ADVANCED_FACE('',(#7891),#2160,.T.);
#68642=ADVANCED_FACE('',(#7892),#4992,.T.);
#68643=ADVANCED_FACE('',(#7893),#2161,.T.);
#68644=ADVANCED_FACE('',(#7894),#2162,.T.);
#68645=ADVANCED_FACE('',(#7895),#4993,.T.);
#68646=ADVANCED_FACE('',(#7896),#2163,.T.);
#68647=ADVANCED_FACE('',(#7897),#2164,.T.);
#68648=ADVANCED_FACE('',(#7898),#4994,.T.);
#68649=ADVANCED_FACE('',(#7899),#4995,.T.);
#68650=ADVANCED_FACE('',(#7900),#2165,.T.);
#68651=ADVANCED_FACE('',(#7901),#2166,.T.);
#68652=ADVANCED_FACE('',(#7902),#2167,.T.);
#68653=ADVANCED_FACE('',(#7903),#2168,.T.);
#68654=ADVANCED_FACE('',(#7904),#2169,.T.);
#68655=ADVANCED_FACE('',(#7905),#2170,.T.);
#68656=ADVANCED_FACE('',(#7906),#2171,.T.);
#68657=ADVANCED_FACE('',(#7907),#2172,.T.);
#68658=ADVANCED_FACE('',(#7908),#2173,.T.);
#68659=ADVANCED_FACE('',(#7909),#2174,.T.);
#68660=ADVANCED_FACE('',(#7910),#2175,.T.);
#68661=ADVANCED_FACE('',(#7911),#2176,.T.);
#68662=ADVANCED_FACE('',(#7912),#2177,.T.);
#68663=ADVANCED_FACE('',(#7913),#2178,.T.);
#68664=ADVANCED_FACE('',(#7914),#2179,.T.);
#68665=ADVANCED_FACE('',(#7915),#2180,.T.);
#68666=ADVANCED_FACE('',(#7916),#2181,.T.);
#68667=ADVANCED_FACE('',(#7917),#2182,.T.);
#68668=ADVANCED_FACE('',(#7918),#2183,.T.);
#68669=ADVANCED_FACE('',(#7919),#2184,.T.);
#68670=ADVANCED_FACE('',(#7920),#2185,.T.);
#68671=ADVANCED_FACE('',(#7921),#2186,.T.);
#68672=ADVANCED_FACE('',(#7922),#2187,.T.);
#68673=ADVANCED_FACE('',(#7923),#2188,.T.);
#68674=ADVANCED_FACE('',(#7924),#2189,.T.);
#68675=ADVANCED_FACE('',(#7925),#2190,.T.);
#68676=ADVANCED_FACE('',(#7926),#2191,.T.);
#68677=ADVANCED_FACE('',(#7927),#2192,.T.);
#68678=ADVANCED_FACE('',(#7928),#2193,.T.);
#68679=ADVANCED_FACE('',(#7929),#2194,.T.);
#68680=ADVANCED_FACE('',(#7930),#2195,.T.);
#68681=ADVANCED_FACE('',(#7931),#2196,.T.);
#68682=ADVANCED_FACE('',(#7932),#2197,.T.);
#68683=ADVANCED_FACE('',(#7933),#2198,.T.);
#68684=ADVANCED_FACE('',(#7934),#2199,.T.);
#68685=ADVANCED_FACE('',(#7935),#2200,.T.);
#68686=ADVANCED_FACE('',(#7936),#2201,.T.);
#68687=ADVANCED_FACE('',(#7937),#2202,.T.);
#68688=ADVANCED_FACE('',(#7938),#2203,.T.);
#68689=ADVANCED_FACE('',(#7939),#2204,.T.);
#68690=ADVANCED_FACE('',(#7940),#2205,.T.);
#68691=ADVANCED_FACE('',(#7941),#2206,.T.);
#68692=ADVANCED_FACE('',(#7942),#2207,.T.);
#68693=ADVANCED_FACE('',(#7943),#2208,.T.);
#68694=ADVANCED_FACE('',(#7944),#2209,.T.);
#68695=ADVANCED_FACE('',(#7945),#2210,.T.);
#68696=ADVANCED_FACE('',(#7946),#2211,.T.);
#68697=ADVANCED_FACE('',(#7947),#2212,.T.);
#68698=ADVANCED_FACE('',(#7948),#2213,.T.);
#68699=ADVANCED_FACE('',(#7949),#2214,.T.);
#68700=ADVANCED_FACE('',(#7950),#2215,.T.);
#68701=ADVANCED_FACE('',(#7951),#2216,.T.);
#68702=ADVANCED_FACE('',(#7952),#2217,.T.);
#68703=ADVANCED_FACE('',(#7953),#2218,.T.);
#68704=ADVANCED_FACE('',(#7954),#2219,.T.);
#68705=ADVANCED_FACE('',(#7955),#2220,.T.);
#68706=ADVANCED_FACE('',(#7956),#2221,.T.);
#68707=ADVANCED_FACE('',(#7957),#2222,.T.);
#68708=ADVANCED_FACE('',(#7958),#2223,.T.);
#68709=ADVANCED_FACE('',(#7959),#2224,.T.);
#68710=ADVANCED_FACE('',(#7960),#2225,.T.);
#68711=ADVANCED_FACE('',(#7961),#2226,.T.);
#68712=ADVANCED_FACE('',(#7962),#2227,.T.);
#68713=ADVANCED_FACE('',(#7963),#2228,.T.);
#68714=ADVANCED_FACE('',(#7964),#2229,.T.);
#68715=ADVANCED_FACE('',(#7965),#2230,.T.);
#68716=ADVANCED_FACE('',(#7966),#2231,.T.);
#68717=ADVANCED_FACE('',(#7967),#2232,.T.);
#68718=ADVANCED_FACE('',(#7968),#2233,.T.);
#68719=ADVANCED_FACE('',(#7969),#2234,.T.);
#68720=ADVANCED_FACE('',(#7970),#2235,.T.);
#68721=ADVANCED_FACE('',(#7971),#2236,.T.);
#68722=ADVANCED_FACE('',(#7972),#2237,.T.);
#68723=ADVANCED_FACE('',(#7973),#2238,.T.);
#68724=ADVANCED_FACE('',(#7974),#2239,.T.);
#68725=ADVANCED_FACE('',(#7975),#2240,.T.);
#68726=ADVANCED_FACE('',(#7976),#2241,.T.);
#68727=ADVANCED_FACE('',(#7977),#2242,.T.);
#68728=ADVANCED_FACE('',(#7978),#2243,.T.);
#68729=ADVANCED_FACE('',(#7979),#2244,.T.);
#68730=ADVANCED_FACE('',(#7980),#2245,.T.);
#68731=ADVANCED_FACE('',(#7981),#2246,.T.);
#68732=ADVANCED_FACE('',(#7982),#2247,.T.);
#68733=ADVANCED_FACE('',(#7983),#2248,.T.);
#68734=ADVANCED_FACE('',(#7984),#2249,.T.);
#68735=ADVANCED_FACE('',(#7985),#2250,.T.);
#68736=ADVANCED_FACE('',(#7986),#2251,.T.);
#68737=ADVANCED_FACE('',(#7987),#2252,.T.);
#68738=ADVANCED_FACE('',(#7988),#2253,.T.);
#68739=ADVANCED_FACE('',(#7989),#2254,.T.);
#68740=ADVANCED_FACE('',(#7990),#2255,.T.);
#68741=ADVANCED_FACE('',(#7991),#2256,.T.);
#68742=ADVANCED_FACE('',(#7992),#2257,.T.);
#68743=ADVANCED_FACE('',(#7993),#2258,.T.);
#68744=ADVANCED_FACE('',(#7994),#2259,.T.);
#68745=ADVANCED_FACE('',(#7995),#2260,.T.);
#68746=ADVANCED_FACE('',(#7996),#2261,.T.);
#68747=ADVANCED_FACE('',(#7997),#2262,.T.);
#68748=ADVANCED_FACE('',(#7998),#2263,.T.);
#68749=ADVANCED_FACE('',(#7999),#2264,.T.);
#68750=ADVANCED_FACE('',(#8000),#2265,.T.);
#68751=ADVANCED_FACE('',(#8001),#2266,.T.);
#68752=ADVANCED_FACE('',(#8002),#2267,.T.);
#68753=ADVANCED_FACE('',(#8003),#2268,.T.);
#68754=ADVANCED_FACE('',(#8004),#2269,.T.);
#68755=ADVANCED_FACE('',(#8005),#2270,.T.);
#68756=ADVANCED_FACE('',(#8006),#2271,.T.);
#68757=ADVANCED_FACE('',(#8007),#2272,.T.);
#68758=ADVANCED_FACE('',(#8008),#2273,.T.);
#68759=ADVANCED_FACE('',(#8009),#2274,.T.);
#68760=ADVANCED_FACE('',(#8010),#2275,.T.);
#68761=ADVANCED_FACE('',(#8011),#2276,.T.);
#68762=ADVANCED_FACE('',(#8012),#2277,.T.);
#68763=ADVANCED_FACE('',(#8013),#2278,.T.);
#68764=ADVANCED_FACE('',(#8014),#2279,.T.);
#68765=ADVANCED_FACE('',(#8015),#2280,.T.);
#68766=ADVANCED_FACE('',(#8016),#2281,.T.);
#68767=ADVANCED_FACE('',(#8017),#2282,.T.);
#68768=ADVANCED_FACE('',(#8018),#4996,.T.);
#68769=ADVANCED_FACE('',(#8019),#2283,.T.);
#68770=ADVANCED_FACE('',(#8020),#2284,.T.);
#68771=ADVANCED_FACE('',(#8021),#4997,.T.);
#68772=ADVANCED_FACE('',(#8022),#2285,.T.);
#68773=ADVANCED_FACE('',(#8023),#2286,.T.);
#68774=ADVANCED_FACE('',(#8024),#4998,.T.);
#68775=ADVANCED_FACE('',(#8025),#2287,.T.);
#68776=ADVANCED_FACE('',(#8026),#2288,.T.);
#68777=ADVANCED_FACE('',(#8027),#4999,.T.);
#68778=ADVANCED_FACE('',(#8028),#2289,.T.);
#68779=ADVANCED_FACE('',(#8029),#2290,.T.);
#68780=ADVANCED_FACE('',(#8030),#5000,.T.);
#68781=ADVANCED_FACE('',(#8031),#2291,.T.);
#68782=ADVANCED_FACE('',(#8032),#2292,.T.);
#68783=ADVANCED_FACE('',(#8033),#5001,.T.);
#68784=ADVANCED_FACE('',(#8034),#2293,.T.);
#68785=ADVANCED_FACE('',(#8035),#2294,.T.);
#68786=ADVANCED_FACE('',(#8036),#5002,.T.);
#68787=ADVANCED_FACE('',(#8037),#2295,.T.);
#68788=ADVANCED_FACE('',(#8038),#2296,.T.);
#68789=ADVANCED_FACE('',(#8039),#5003,.T.);
#68790=ADVANCED_FACE('',(#8040),#2297,.T.);
#68791=ADVANCED_FACE('',(#8041),#2298,.T.);
#68792=ADVANCED_FACE('',(#8042),#5004,.T.);
#68793=ADVANCED_FACE('',(#8043),#2299,.T.);
#68794=ADVANCED_FACE('',(#8044),#2300,.T.);
#68795=ADVANCED_FACE('',(#8045),#5005,.T.);
#68796=ADVANCED_FACE('',(#8046),#2301,.T.);
#68797=ADVANCED_FACE('',(#8047),#2302,.T.);
#68798=ADVANCED_FACE('',(#8048),#5006,.T.);
#68799=ADVANCED_FACE('',(#8049),#2303,.T.);
#68800=ADVANCED_FACE('',(#8050),#2304,.T.);
#68801=ADVANCED_FACE('',(#8051),#5007,.T.);
#68802=ADVANCED_FACE('',(#8052),#2305,.T.);
#68803=ADVANCED_FACE('',(#8053),#2306,.T.);
#68804=ADVANCED_FACE('',(#8054),#5008,.T.);
#68805=ADVANCED_FACE('',(#8055),#2307,.T.);
#68806=ADVANCED_FACE('',(#8056),#2308,.T.);
#68807=ADVANCED_FACE('',(#8057),#5009,.T.);
#68808=ADVANCED_FACE('',(#8058),#2309,.T.);
#68809=ADVANCED_FACE('',(#8059),#2310,.T.);
#68810=ADVANCED_FACE('',(#8060),#2311,.T.);
#68811=ADVANCED_FACE('',(#8061),#2312,.T.);
#68812=ADVANCED_FACE('',(#8062),#5010,.T.);
#68813=ADVANCED_FACE('',(#8063),#2313,.T.);
#68814=ADVANCED_FACE('',(#8064),#2314,.T.);
#68815=ADVANCED_FACE('',(#8065),#5011,.T.);
#68816=ADVANCED_FACE('',(#8066),#2315,.T.);
#68817=ADVANCED_FACE('',(#8067),#2316,.T.);
#68818=ADVANCED_FACE('',(#8068),#5012,.T.);
#68819=ADVANCED_FACE('',(#8069),#2317,.T.);
#68820=ADVANCED_FACE('',(#8070),#2318,.T.);
#68821=ADVANCED_FACE('',(#8071),#5013,.T.);
#68822=ADVANCED_FACE('',(#8072),#2319,.T.);
#68823=ADVANCED_FACE('',(#8073),#2320,.T.);
#68824=ADVANCED_FACE('',(#8074),#5014,.T.);
#68825=ADVANCED_FACE('',(#8075),#2321,.T.);
#68826=ADVANCED_FACE('',(#8076),#2322,.T.);
#68827=ADVANCED_FACE('',(#8077),#2323,.T.);
#68828=ADVANCED_FACE('',(#8078),#5015,.T.);
#68829=ADVANCED_FACE('',(#8079),#2324,.T.);
#68830=ADVANCED_FACE('',(#8080),#5016,.T.);
#68831=ADVANCED_FACE('',(#8081),#2325,.T.);
#68832=ADVANCED_FACE('',(#8082),#2326,.T.);
#68833=ADVANCED_FACE('',(#8083),#5017,.T.);
#68834=ADVANCED_FACE('',(#8084),#2327,.T.);
#68835=ADVANCED_FACE('',(#8085),#2328,.T.);
#68836=ADVANCED_FACE('',(#8086),#5018,.T.);
#68837=ADVANCED_FACE('',(#8087),#2329,.T.);
#68838=ADVANCED_FACE('',(#8088),#2330,.T.);
#68839=ADVANCED_FACE('',(#8089),#5019,.T.);
#68840=ADVANCED_FACE('',(#8090),#2331,.T.);
#68841=ADVANCED_FACE('',(#8091),#2332,.T.);
#68842=ADVANCED_FACE('',(#8092),#5020,.T.);
#68843=ADVANCED_FACE('',(#8093),#2333,.T.);
#68844=ADVANCED_FACE('',(#8094),#2334,.T.);
#68845=ADVANCED_FACE('',(#8095),#5021,.T.);
#68846=ADVANCED_FACE('',(#8096),#2335,.T.);
#68847=ADVANCED_FACE('',(#8097),#2336,.T.);
#68848=ADVANCED_FACE('',(#8098),#5022,.T.);
#68849=ADVANCED_FACE('',(#8099),#2337,.T.);
#68850=ADVANCED_FACE('',(#8100),#2338,.T.);
#68851=ADVANCED_FACE('',(#8101),#5023,.T.);
#68852=ADVANCED_FACE('',(#8102),#2339,.T.);
#68853=ADVANCED_FACE('',(#8103),#2340,.T.);
#68854=ADVANCED_FACE('',(#8104),#2341,.T.);
#68855=ADVANCED_FACE('',(#8105),#5024,.T.);
#68856=ADVANCED_FACE('',(#8106),#2342,.T.);
#68857=ADVANCED_FACE('',(#8107),#2343,.T.);
#68858=ADVANCED_FACE('',(#8108),#5025,.T.);
#68859=ADVANCED_FACE('',(#8109),#2344,.T.);
#68860=ADVANCED_FACE('',(#8110),#2345,.T.);
#68861=ADVANCED_FACE('',(#8111),#5026,.T.);
#68862=ADVANCED_FACE('',(#8112),#2346,.T.);
#68863=ADVANCED_FACE('',(#8113),#2347,.T.);
#68864=ADVANCED_FACE('',(#8114),#5027,.T.);
#68865=ADVANCED_FACE('',(#8115),#2348,.T.);
#68866=ADVANCED_FACE('',(#8116),#2349,.T.);
#68867=ADVANCED_FACE('',(#8117),#5028,.T.);
#68868=ADVANCED_FACE('',(#8118),#2350,.T.);
#68869=ADVANCED_FACE('',(#8119),#2351,.T.);
#68870=ADVANCED_FACE('',(#8120),#5029,.T.);
#68871=ADVANCED_FACE('',(#8121),#2352,.T.);
#68872=ADVANCED_FACE('',(#8122),#2353,.T.);
#68873=ADVANCED_FACE('',(#8123),#5030,.T.);
#68874=ADVANCED_FACE('',(#8124),#2354,.T.);
#68875=ADVANCED_FACE('',(#8125),#2355,.T.);
#68876=ADVANCED_FACE('',(#8126),#5031,.T.);
#68877=ADVANCED_FACE('',(#8127),#2356,.T.);
#68878=ADVANCED_FACE('',(#8128),#2357,.T.);
#68879=ADVANCED_FACE('',(#8129),#5032,.T.);
#68880=ADVANCED_FACE('',(#8130),#2358,.T.);
#68881=ADVANCED_FACE('',(#8131),#2359,.T.);
#68882=ADVANCED_FACE('',(#8132),#5033,.T.);
#68883=ADVANCED_FACE('',(#8133),#2360,.T.);
#68884=ADVANCED_FACE('',(#8134),#2361,.T.);
#68885=ADVANCED_FACE('',(#8135),#5034,.T.);
#68886=ADVANCED_FACE('',(#8136),#2362,.T.);
#68887=ADVANCED_FACE('',(#8137),#2363,.T.);
#68888=ADVANCED_FACE('',(#8138),#5035,.T.);
#68889=ADVANCED_FACE('',(#8139),#2364,.T.);
#68890=ADVANCED_FACE('',(#8140),#2365,.T.);
#68891=ADVANCED_FACE('',(#8141),#5036,.T.);
#68892=ADVANCED_FACE('',(#8142),#2366,.T.);
#68893=ADVANCED_FACE('',(#8143),#2367,.T.);
#68894=ADVANCED_FACE('',(#8144),#5037,.T.);
#68895=ADVANCED_FACE('',(#8145),#2368,.T.);
#68896=ADVANCED_FACE('',(#8146),#2369,.T.);
#68897=ADVANCED_FACE('',(#8147),#5038,.T.);
#68898=ADVANCED_FACE('',(#8148),#2370,.T.);
#68899=ADVANCED_FACE('',(#8149),#2371,.T.);
#68900=ADVANCED_FACE('',(#8150),#5039,.T.);
#68901=ADVANCED_FACE('',(#8151),#2372,.T.);
#68902=ADVANCED_FACE('',(#8152),#2373,.T.);
#68903=ADVANCED_FACE('',(#8153),#5040,.T.);
#68904=ADVANCED_FACE('',(#8154),#2374,.T.);
#68905=ADVANCED_FACE('',(#8155),#2375,.T.);
#68906=ADVANCED_FACE('',(#8156),#5041,.T.);
#68907=ADVANCED_FACE('',(#8157),#2376,.T.);
#68908=ADVANCED_FACE('',(#8158),#2377,.T.);
#68909=ADVANCED_FACE('',(#8159),#5042,.T.);
#68910=ADVANCED_FACE('',(#8160),#2378,.T.);
#68911=ADVANCED_FACE('',(#8161),#2379,.T.);
#68912=ADVANCED_FACE('',(#8162),#5043,.T.);
#68913=ADVANCED_FACE('',(#8163),#2380,.T.);
#68914=ADVANCED_FACE('',(#8164),#2381,.T.);
#68915=ADVANCED_FACE('',(#8165),#5044,.T.);
#68916=ADVANCED_FACE('',(#8166),#2382,.T.);
#68917=ADVANCED_FACE('',(#8167),#2383,.T.);
#68918=ADVANCED_FACE('',(#8168),#5045,.T.);
#68919=ADVANCED_FACE('',(#8169),#2384,.T.);
#68920=ADVANCED_FACE('',(#8170),#2385,.T.);
#68921=ADVANCED_FACE('',(#8171),#5046,.T.);
#68922=ADVANCED_FACE('',(#8172),#2386,.T.);
#68923=ADVANCED_FACE('',(#8173),#2387,.T.);
#68924=ADVANCED_FACE('',(#8174),#5047,.T.);
#68925=ADVANCED_FACE('',(#8175),#2388,.T.);
#68926=ADVANCED_FACE('',(#8176),#2389,.T.);
#68927=ADVANCED_FACE('',(#8177),#5048,.T.);
#68928=ADVANCED_FACE('',(#8178),#2390,.T.);
#68929=ADVANCED_FACE('',(#8179),#2391,.T.);
#68930=ADVANCED_FACE('',(#8180),#5049,.T.);
#68931=ADVANCED_FACE('',(#8181),#2392,.T.);
#68932=ADVANCED_FACE('',(#8182),#2393,.T.);
#68933=ADVANCED_FACE('',(#8183),#5050,.T.);
#68934=ADVANCED_FACE('',(#8184),#2394,.T.);
#68935=ADVANCED_FACE('',(#8185),#2395,.T.);
#68936=ADVANCED_FACE('',(#8186),#5051,.T.);
#68937=ADVANCED_FACE('',(#8187),#2396,.T.);
#68938=ADVANCED_FACE('',(#8188),#2397,.T.);
#68939=ADVANCED_FACE('',(#8189),#5052,.T.);
#68940=ADVANCED_FACE('',(#8190),#2398,.T.);
#68941=ADVANCED_FACE('',(#8191),#2399,.T.);
#68942=ADVANCED_FACE('',(#8192),#2400,.T.);
#68943=ADVANCED_FACE('',(#8193),#2401,.T.);
#68944=ADVANCED_FACE('',(#8194),#2402,.T.);
#68945=ADVANCED_FACE('',(#8195),#2403,.T.);
#68946=ADVANCED_FACE('',(#8196),#2404,.T.);
#68947=ADVANCED_FACE('',(#8197),#2405,.T.);
#68948=ADVANCED_FACE('',(#8198),#2406,.T.);
#68949=ADVANCED_FACE('',(#8199),#2407,.T.);
#68950=ADVANCED_FACE('',(#8200),#2408,.T.);
#68951=ADVANCED_FACE('',(#8201),#2409,.T.);
#68952=ADVANCED_FACE('',(#8202),#2410,.T.);
#68953=ADVANCED_FACE('',(#8203),#2411,.T.);
#68954=ADVANCED_FACE('',(#8204),#2412,.T.);
#68955=ADVANCED_FACE('',(#8205),#2413,.T.);
#68956=ADVANCED_FACE('',(#8206),#2414,.T.);
#68957=ADVANCED_FACE('',(#8207),#2415,.T.);
#68958=ADVANCED_FACE('',(#8208),#2416,.T.);
#68959=ADVANCED_FACE('',(#8209),#2417,.T.);
#68960=ADVANCED_FACE('',(#8210),#2418,.T.);
#68961=ADVANCED_FACE('',(#8211),#2419,.T.);
#68962=ADVANCED_FACE('',(#8212),#2420,.T.);
#68963=ADVANCED_FACE('',(#8213),#2421,.T.);
#68964=ADVANCED_FACE('',(#8214),#2422,.T.);
#68965=ADVANCED_FACE('',(#8215),#2423,.T.);
#68966=ADVANCED_FACE('',(#8216),#2424,.T.);
#68967=ADVANCED_FACE('',(#8217),#2425,.T.);
#68968=ADVANCED_FACE('',(#8218),#2426,.T.);
#68969=ADVANCED_FACE('',(#8219),#2427,.T.);
#68970=ADVANCED_FACE('',(#8220),#2428,.T.);
#68971=ADVANCED_FACE('',(#8221),#2429,.T.);
#68972=ADVANCED_FACE('',(#8222),#2430,.T.);
#68973=ADVANCED_FACE('',(#8223),#2431,.T.);
#68974=ADVANCED_FACE('',(#8224),#2432,.T.);
#68975=ADVANCED_FACE('',(#8225),#2433,.T.);
#68976=ADVANCED_FACE('',(#8226),#2434,.T.);
#68977=ADVANCED_FACE('',(#8227),#2435,.T.);
#68978=ADVANCED_FACE('',(#8228),#2436,.T.);
#68979=ADVANCED_FACE('',(#8229),#2437,.T.);
#68980=ADVANCED_FACE('',(#8230),#2438,.T.);
#68981=ADVANCED_FACE('',(#8231),#2439,.T.);
#68982=ADVANCED_FACE('',(#8232),#2440,.T.);
#68983=ADVANCED_FACE('',(#8233),#2441,.T.);
#68984=ADVANCED_FACE('',(#8234),#2442,.T.);
#68985=ADVANCED_FACE('',(#8235),#2443,.T.);
#68986=ADVANCED_FACE('',(#8236),#2444,.T.);
#68987=ADVANCED_FACE('',(#8237),#2445,.T.);
#68988=ADVANCED_FACE('',(#8238),#2446,.T.);
#68989=ADVANCED_FACE('',(#8239),#2447,.T.);
#68990=ADVANCED_FACE('',(#8240),#2448,.T.);
#68991=ADVANCED_FACE('',(#8241),#2449,.T.);
#68992=ADVANCED_FACE('',(#8242),#2450,.T.);
#68993=ADVANCED_FACE('',(#8243),#2451,.T.);
#68994=ADVANCED_FACE('',(#8244),#2452,.T.);
#68995=ADVANCED_FACE('',(#8245),#2453,.T.);
#68996=ADVANCED_FACE('',(#8246),#2454,.T.);
#68997=ADVANCED_FACE('',(#8247),#2455,.T.);
#68998=ADVANCED_FACE('',(#8248),#2456,.T.);
#68999=ADVANCED_FACE('',(#8249),#2457,.T.);
#69000=ADVANCED_FACE('',(#8250),#2458,.T.);
#69001=ADVANCED_FACE('',(#8251),#2459,.T.);
#69002=ADVANCED_FACE('',(#8252),#2460,.T.);
#69003=ADVANCED_FACE('',(#8253),#2461,.T.);
#69004=ADVANCED_FACE('',(#8254),#2462,.T.);
#69005=ADVANCED_FACE('',(#8255),#2463,.T.);
#69006=ADVANCED_FACE('',(#8256),#2464,.T.);
#69007=ADVANCED_FACE('',(#8257),#2465,.T.);
#69008=ADVANCED_FACE('',(#8258),#2466,.T.);
#69009=ADVANCED_FACE('',(#8259),#2467,.T.);
#69010=ADVANCED_FACE('',(#8260),#2468,.T.);
#69011=ADVANCED_FACE('',(#8261),#2469,.T.);
#69012=ADVANCED_FACE('',(#8262),#2470,.T.);
#69013=ADVANCED_FACE('',(#8263),#2471,.T.);
#69014=ADVANCED_FACE('',(#8264),#2472,.T.);
#69015=ADVANCED_FACE('',(#8265),#2473,.T.);
#69016=ADVANCED_FACE('',(#8266),#2474,.T.);
#69017=ADVANCED_FACE('',(#8267),#2475,.T.);
#69018=ADVANCED_FACE('',(#8268),#2476,.T.);
#69019=ADVANCED_FACE('',(#8269),#2477,.T.);
#69020=ADVANCED_FACE('',(#8270),#2478,.T.);
#69021=ADVANCED_FACE('',(#8271),#2479,.T.);
#69022=ADVANCED_FACE('',(#8272),#2480,.T.);
#69023=ADVANCED_FACE('',(#8273),#2481,.T.);
#69024=ADVANCED_FACE('',(#8274),#2482,.T.);
#69025=ADVANCED_FACE('',(#8275),#2483,.T.);
#69026=ADVANCED_FACE('',(#8276),#2484,.T.);
#69027=ADVANCED_FACE('',(#8277),#2485,.T.);
#69028=ADVANCED_FACE('',(#8278),#2486,.T.);
#69029=ADVANCED_FACE('',(#8279),#2487,.T.);
#69030=ADVANCED_FACE('',(#8280),#2488,.T.);
#69031=ADVANCED_FACE('',(#8281),#2489,.T.);
#69032=ADVANCED_FACE('',(#8282),#2490,.T.);
#69033=ADVANCED_FACE('',(#8283),#2491,.T.);
#69034=ADVANCED_FACE('',(#8284),#2492,.T.);
#69035=ADVANCED_FACE('',(#8285),#2493,.T.);
#69036=ADVANCED_FACE('',(#8286),#2494,.T.);
#69037=ADVANCED_FACE('',(#8287),#2495,.T.);
#69038=ADVANCED_FACE('',(#8288),#2496,.T.);
#69039=ADVANCED_FACE('',(#8289),#2497,.T.);
#69040=ADVANCED_FACE('',(#8290),#2498,.T.);
#69041=ADVANCED_FACE('',(#8291),#2499,.T.);
#69042=ADVANCED_FACE('',(#8292),#2500,.T.);
#69043=ADVANCED_FACE('',(#8293),#2501,.T.);
#69044=ADVANCED_FACE('',(#8294),#2502,.T.);
#69045=ADVANCED_FACE('',(#8295),#2503,.T.);
#69046=ADVANCED_FACE('',(#8296),#2504,.T.);
#69047=ADVANCED_FACE('',(#8297),#2505,.T.);
#69048=ADVANCED_FACE('',(#8298),#2506,.T.);
#69049=ADVANCED_FACE('',(#8299),#2507,.T.);
#69050=ADVANCED_FACE('',(#8300),#2508,.T.);
#69051=ADVANCED_FACE('',(#8301),#2509,.T.);
#69052=ADVANCED_FACE('',(#8302),#2510,.T.);
#69053=ADVANCED_FACE('',(#8303),#2511,.T.);
#69054=ADVANCED_FACE('',(#8304),#2512,.T.);
#69055=ADVANCED_FACE('',(#8305),#2513,.T.);
#69056=ADVANCED_FACE('',(#8306),#2514,.T.);
#69057=ADVANCED_FACE('',(#8307),#2515,.T.);
#69058=ADVANCED_FACE('',(#8308),#5053,.T.);
#69059=ADVANCED_FACE('',(#8309),#2516,.T.);
#69060=ADVANCED_FACE('',(#8310),#2517,.T.);
#69061=ADVANCED_FACE('',(#8311),#5054,.T.);
#69062=ADVANCED_FACE('',(#8312),#2518,.T.);
#69063=ADVANCED_FACE('',(#8313),#2519,.T.);
#69064=ADVANCED_FACE('',(#8314),#5055,.T.);
#69065=ADVANCED_FACE('',(#8315),#2520,.T.);
#69066=ADVANCED_FACE('',(#8316),#2521,.T.);
#69067=ADVANCED_FACE('',(#8317),#5056,.T.);
#69068=ADVANCED_FACE('',(#8318),#2522,.T.);
#69069=ADVANCED_FACE('',(#8319),#2523,.T.);
#69070=ADVANCED_FACE('',(#8320),#5057,.T.);
#69071=ADVANCED_FACE('',(#8321),#2524,.T.);
#69072=ADVANCED_FACE('',(#8322),#2525,.T.);
#69073=ADVANCED_FACE('',(#8323),#5058,.T.);
#69074=ADVANCED_FACE('',(#8324),#2526,.T.);
#69075=ADVANCED_FACE('',(#8325),#2527,.T.);
#69076=ADVANCED_FACE('',(#8326),#2528,.T.);
#69077=ADVANCED_FACE('',(#8327),#2529,.T.);
#69078=ADVANCED_FACE('',(#8328),#5059,.T.);
#69079=ADVANCED_FACE('',(#8329),#2530,.T.);
#69080=ADVANCED_FACE('',(#8330),#2531,.T.);
#69081=ADVANCED_FACE('',(#8331),#5060,.T.);
#69082=ADVANCED_FACE('',(#8332),#2532,.T.);
#69083=ADVANCED_FACE('',(#8333),#2533,.T.);
#69084=ADVANCED_FACE('',(#8334),#5061,.T.);
#69085=ADVANCED_FACE('',(#8335),#2534,.T.);
#69086=ADVANCED_FACE('',(#8336),#2535,.T.);
#69087=ADVANCED_FACE('',(#8337),#5062,.T.);
#69088=ADVANCED_FACE('',(#8338),#2536,.T.);
#69089=ADVANCED_FACE('',(#8339),#2537,.T.);
#69090=ADVANCED_FACE('',(#8340),#5063,.T.);
#69091=ADVANCED_FACE('',(#8341),#2538,.T.);
#69092=ADVANCED_FACE('',(#8342),#2539,.T.);
#69093=ADVANCED_FACE('',(#8343),#5064,.T.);
#69094=ADVANCED_FACE('',(#8344),#2540,.T.);
#69095=ADVANCED_FACE('',(#8345),#2541,.T.);
#69096=ADVANCED_FACE('',(#8346),#5065,.T.);
#69097=ADVANCED_FACE('',(#8347),#2542,.T.);
#69098=ADVANCED_FACE('',(#8348),#2543,.T.);
#69099=ADVANCED_FACE('',(#8349),#5066,.T.);
#69100=ADVANCED_FACE('',(#8350),#2544,.T.);
#69101=ADVANCED_FACE('',(#8351),#2545,.T.);
#69102=ADVANCED_FACE('',(#8352),#5067,.T.);
#69103=ADVANCED_FACE('',(#8353),#2546,.T.);
#69104=ADVANCED_FACE('',(#8354),#2547,.T.);
#69105=ADVANCED_FACE('',(#8355),#5068,.T.);
#69106=ADVANCED_FACE('',(#8356),#2548,.T.);
#69107=ADVANCED_FACE('',(#8357),#2549,.T.);
#69108=ADVANCED_FACE('',(#8358),#5069,.T.);
#69109=ADVANCED_FACE('',(#8359),#2550,.T.);
#69110=ADVANCED_FACE('',(#8360),#2551,.T.);
#69111=ADVANCED_FACE('',(#8361),#5070,.T.);
#69112=ADVANCED_FACE('',(#8362),#2552,.T.);
#69113=ADVANCED_FACE('',(#8363),#2553,.T.);
#69114=ADVANCED_FACE('',(#8364),#2554,.T.);
#69115=ADVANCED_FACE('',(#8365),#5071,.T.);
#69116=ADVANCED_FACE('',(#8366),#2555,.T.);
#69117=ADVANCED_FACE('',(#8367),#5072,.T.);
#69118=ADVANCED_FACE('',(#8368),#2556,.T.);
#69119=ADVANCED_FACE('',(#8369),#2557,.T.);
#69120=ADVANCED_FACE('',(#8370),#5073,.T.);
#69121=ADVANCED_FACE('',(#8371),#2558,.T.);
#69122=ADVANCED_FACE('',(#8372),#2559,.T.);
#69123=ADVANCED_FACE('',(#8373),#5074,.T.);
#69124=ADVANCED_FACE('',(#8374),#2560,.T.);
#69125=ADVANCED_FACE('',(#8375),#2561,.T.);
#69126=ADVANCED_FACE('',(#8376),#5075,.T.);
#69127=ADVANCED_FACE('',(#8377),#2562,.T.);
#69128=ADVANCED_FACE('',(#8378),#2563,.T.);
#69129=ADVANCED_FACE('',(#8379),#5076,.T.);
#69130=ADVANCED_FACE('',(#8380),#2564,.T.);
#69131=ADVANCED_FACE('',(#8381),#2565,.T.);
#69132=ADVANCED_FACE('',(#8382),#5077,.T.);
#69133=ADVANCED_FACE('',(#8383),#2566,.T.);
#69134=ADVANCED_FACE('',(#8384),#2567,.T.);
#69135=ADVANCED_FACE('',(#8385),#5078,.T.);
#69136=ADVANCED_FACE('',(#8386),#2568,.T.);
#69137=ADVANCED_FACE('',(#8387),#2569,.T.);
#69138=ADVANCED_FACE('',(#8388),#5079,.T.);
#69139=ADVANCED_FACE('',(#8389),#2570,.T.);
#69140=ADVANCED_FACE('',(#8390),#5080,.T.);
#69141=ADVANCED_FACE('',(#8391),#2571,.T.);
#69142=ADVANCED_FACE('',(#8392),#2572,.T.);
#69143=ADVANCED_FACE('',(#8393),#2573,.T.);
#69144=ADVANCED_FACE('',(#8394),#2574,.T.);
#69145=ADVANCED_FACE('',(#8395),#5081,.T.);
#69146=ADVANCED_FACE('',(#8396),#2575,.T.);
#69147=ADVANCED_FACE('',(#8397),#2576,.T.);
#69148=ADVANCED_FACE('',(#8398),#5082,.T.);
#69149=ADVANCED_FACE('',(#8399),#2577,.T.);
#69150=ADVANCED_FACE('',(#8400),#2578,.T.);
#69151=ADVANCED_FACE('',(#8401),#5083,.T.);
#69152=ADVANCED_FACE('',(#8402),#2579,.T.);
#69153=ADVANCED_FACE('',(#8403),#2580,.T.);
#69154=ADVANCED_FACE('',(#8404),#5084,.T.);
#69155=ADVANCED_FACE('',(#8405),#2581,.T.);
#69156=ADVANCED_FACE('',(#8406),#2582,.T.);
#69157=ADVANCED_FACE('',(#8407),#5085,.T.);
#69158=ADVANCED_FACE('',(#8408),#2583,.T.);
#69159=ADVANCED_FACE('',(#8409),#2584,.T.);
#69160=ADVANCED_FACE('',(#8410),#5086,.T.);
#69161=ADVANCED_FACE('',(#8411),#2585,.T.);
#69162=ADVANCED_FACE('',(#8412),#2586,.T.);
#69163=ADVANCED_FACE('',(#8413),#5087,.T.);
#69164=ADVANCED_FACE('',(#8414),#2587,.T.);
#69165=ADVANCED_FACE('',(#8415),#2588,.T.);
#69166=ADVANCED_FACE('',(#8416),#5088,.T.);
#69167=ADVANCED_FACE('',(#8417),#2589,.T.);
#69168=ADVANCED_FACE('',(#8418),#2590,.T.);
#69169=ADVANCED_FACE('',(#8419),#5089,.T.);
#69170=ADVANCED_FACE('',(#8420),#2591,.T.);
#69171=ADVANCED_FACE('',(#8421),#2592,.T.);
#69172=ADVANCED_FACE('',(#8422),#5090,.T.);
#69173=ADVANCED_FACE('',(#8423),#2593,.T.);
#69174=ADVANCED_FACE('',(#8424),#2594,.T.);
#69175=ADVANCED_FACE('',(#8425),#5091,.T.);
#69176=ADVANCED_FACE('',(#8426),#2595,.T.);
#69177=ADVANCED_FACE('',(#8427),#2596,.T.);
#69178=ADVANCED_FACE('',(#8428),#5092,.T.);
#69179=ADVANCED_FACE('',(#8429),#2597,.T.);
#69180=ADVANCED_FACE('',(#8430),#2598,.T.);
#69181=ADVANCED_FACE('',(#8431),#5093,.T.);
#69182=ADVANCED_FACE('',(#8432),#2599,.T.);
#69183=ADVANCED_FACE('',(#8433),#2600,.T.);
#69184=ADVANCED_FACE('',(#8434),#2601,.T.);
#69185=ADVANCED_FACE('',(#8435),#2602,.T.);
#69186=ADVANCED_FACE('',(#8436),#5094,.T.);
#69187=ADVANCED_FACE('',(#8437),#2603,.T.);
#69188=ADVANCED_FACE('',(#8438),#2604,.T.);
#69189=ADVANCED_FACE('',(#8439),#5095,.T.);
#69190=ADVANCED_FACE('',(#8440),#2605,.T.);
#69191=ADVANCED_FACE('',(#8441),#2606,.T.);
#69192=ADVANCED_FACE('',(#8442),#5096,.T.);
#69193=ADVANCED_FACE('',(#8443),#2607,.T.);
#69194=ADVANCED_FACE('',(#8444),#2608,.T.);
#69195=ADVANCED_FACE('',(#8445),#5097,.T.);
#69196=ADVANCED_FACE('',(#8446),#2609,.T.);
#69197=ADVANCED_FACE('',(#8447),#2610,.T.);
#69198=ADVANCED_FACE('',(#8448),#5098,.T.);
#69199=ADVANCED_FACE('',(#8449),#2611,.T.);
#69200=ADVANCED_FACE('',(#8450),#2612,.T.);
#69201=ADVANCED_FACE('',(#8451),#5099,.T.);
#69202=ADVANCED_FACE('',(#8452),#2613,.T.);
#69203=ADVANCED_FACE('',(#8453),#2614,.T.);
#69204=ADVANCED_FACE('',(#8454),#5100,.T.);
#69205=ADVANCED_FACE('',(#8455),#2615,.T.);
#69206=ADVANCED_FACE('',(#8456),#2616,.T.);
#69207=ADVANCED_FACE('',(#8457),#5101,.T.);
#69208=ADVANCED_FACE('',(#8458),#2617,.T.);
#69209=ADVANCED_FACE('',(#8459),#2618,.T.);
#69210=ADVANCED_FACE('',(#8460),#5102,.T.);
#69211=ADVANCED_FACE('',(#8461),#2619,.T.);
#69212=ADVANCED_FACE('',(#8462),#2620,.T.);
#69213=ADVANCED_FACE('',(#8463),#5103,.T.);
#69214=ADVANCED_FACE('',(#8464),#2621,.T.);
#69215=ADVANCED_FACE('',(#8465),#2622,.T.);
#69216=ADVANCED_FACE('',(#8466),#5104,.T.);
#69217=ADVANCED_FACE('',(#8467),#2623,.T.);
#69218=ADVANCED_FACE('',(#8468),#2624,.T.);
#69219=ADVANCED_FACE('',(#8469),#5105,.T.);
#69220=ADVANCED_FACE('',(#8470),#2625,.T.);
#69221=ADVANCED_FACE('',(#8471),#2626,.T.);
#69222=ADVANCED_FACE('',(#8472),#5106,.T.);
#69223=ADVANCED_FACE('',(#8473),#2627,.T.);
#69224=ADVANCED_FACE('',(#8474),#2628,.T.);
#69225=ADVANCED_FACE('',(#8475),#5107,.T.);
#69226=ADVANCED_FACE('',(#8476),#5108,.T.);
#69227=ADVANCED_FACE('',(#8477),#2629,.T.);
#69228=ADVANCED_FACE('',(#8478),#2630,.T.);
#69229=ADVANCED_FACE('',(#8479),#2631,.T.);
#69230=ADVANCED_FACE('',(#8480),#2632,.T.);
#69231=ADVANCED_FACE('',(#8481),#2633,.T.);
#69232=ADVANCED_FACE('',(#8482),#2634,.T.);
#69233=ADVANCED_FACE('',(#8483),#2635,.T.);
#69234=ADVANCED_FACE('',(#8484),#2636,.T.);
#69235=ADVANCED_FACE('',(#8485),#2637,.T.);
#69236=ADVANCED_FACE('',(#8486),#2638,.T.);
#69237=ADVANCED_FACE('',(#8487),#2639,.T.);
#69238=ADVANCED_FACE('',(#8488),#2640,.T.);
#69239=ADVANCED_FACE('',(#8489),#2641,.T.);
#69240=ADVANCED_FACE('',(#8490),#2642,.T.);
#69241=ADVANCED_FACE('',(#8491),#2643,.T.);
#69242=ADVANCED_FACE('',(#8492),#2644,.T.);
#69243=ADVANCED_FACE('',(#8493),#2645,.T.);
#69244=ADVANCED_FACE('',(#8494),#2646,.T.);
#69245=ADVANCED_FACE('',(#8495),#2647,.T.);
#69246=ADVANCED_FACE('',(#8496),#2648,.T.);
#69247=ADVANCED_FACE('',(#8497),#2649,.T.);
#69248=ADVANCED_FACE('',(#8498),#2650,.T.);
#69249=ADVANCED_FACE('',(#8499),#2651,.T.);
#69250=ADVANCED_FACE('',(#8500),#2652,.T.);
#69251=ADVANCED_FACE('',(#8501),#2653,.T.);
#69252=ADVANCED_FACE('',(#8502),#2654,.T.);
#69253=ADVANCED_FACE('',(#8503),#2655,.T.);
#69254=ADVANCED_FACE('',(#8504),#2656,.T.);
#69255=ADVANCED_FACE('',(#8505),#2657,.T.);
#69256=ADVANCED_FACE('',(#8506),#2658,.T.);
#69257=ADVANCED_FACE('',(#8507),#2659,.T.);
#69258=ADVANCED_FACE('',(#8508),#2660,.T.);
#69259=ADVANCED_FACE('',(#8509),#2661,.T.);
#69260=ADVANCED_FACE('',(#8510),#2662,.T.);
#69261=ADVANCED_FACE('',(#8511),#2663,.T.);
#69262=ADVANCED_FACE('',(#8512),#2664,.T.);
#69263=ADVANCED_FACE('',(#8513),#2665,.T.);
#69264=ADVANCED_FACE('',(#8514),#2666,.T.);
#69265=ADVANCED_FACE('',(#8515),#2667,.T.);
#69266=ADVANCED_FACE('',(#8516),#2668,.T.);
#69267=ADVANCED_FACE('',(#8517),#2669,.T.);
#69268=ADVANCED_FACE('',(#8518),#2670,.T.);
#69269=ADVANCED_FACE('',(#8519),#2671,.T.);
#69270=ADVANCED_FACE('',(#8520),#2672,.T.);
#69271=ADVANCED_FACE('',(#8521),#2673,.T.);
#69272=ADVANCED_FACE('',(#8522),#2674,.T.);
#69273=ADVANCED_FACE('',(#8523),#2675,.T.);
#69274=ADVANCED_FACE('',(#8524),#2676,.T.);
#69275=ADVANCED_FACE('',(#8525),#2677,.T.);
#69276=ADVANCED_FACE('',(#8526),#2678,.T.);
#69277=ADVANCED_FACE('',(#8527),#2679,.T.);
#69278=ADVANCED_FACE('',(#8528),#2680,.T.);
#69279=ADVANCED_FACE('',(#8529),#2681,.T.);
#69280=ADVANCED_FACE('',(#8530),#2682,.T.);
#69281=ADVANCED_FACE('',(#8531),#2683,.T.);
#69282=ADVANCED_FACE('',(#8532),#2684,.T.);
#69283=ADVANCED_FACE('',(#8533),#2685,.T.);
#69284=ADVANCED_FACE('',(#8534),#2686,.T.);
#69285=ADVANCED_FACE('',(#8535),#2687,.T.);
#69286=ADVANCED_FACE('',(#8536),#2688,.T.);
#69287=ADVANCED_FACE('',(#8537),#2689,.T.);
#69288=ADVANCED_FACE('',(#8538),#2690,.T.);
#69289=ADVANCED_FACE('',(#8539),#2691,.T.);
#69290=ADVANCED_FACE('',(#8540),#2692,.T.);
#69291=ADVANCED_FACE('',(#8541),#2693,.T.);
#69292=ADVANCED_FACE('',(#8542),#2694,.T.);
#69293=ADVANCED_FACE('',(#8543),#2695,.T.);
#69294=ADVANCED_FACE('',(#8544),#2696,.T.);
#69295=ADVANCED_FACE('',(#8545),#2697,.T.);
#69296=ADVANCED_FACE('',(#8546),#2698,.T.);
#69297=ADVANCED_FACE('',(#8547),#2699,.T.);
#69298=ADVANCED_FACE('',(#8548),#2700,.T.);
#69299=ADVANCED_FACE('',(#8549),#2701,.T.);
#69300=ADVANCED_FACE('',(#8550),#2702,.T.);
#69301=ADVANCED_FACE('',(#8551),#2703,.T.);
#69302=ADVANCED_FACE('',(#8552),#2704,.T.);
#69303=ADVANCED_FACE('',(#8553),#2705,.T.);
#69304=ADVANCED_FACE('',(#8554),#2706,.T.);
#69305=ADVANCED_FACE('',(#8555),#2707,.T.);
#69306=ADVANCED_FACE('',(#8556),#2708,.T.);
#69307=ADVANCED_FACE('',(#8557),#2709,.T.);
#69308=ADVANCED_FACE('',(#8558),#2710,.T.);
#69309=ADVANCED_FACE('',(#8559),#2711,.T.);
#69310=ADVANCED_FACE('',(#8560),#2712,.T.);
#69311=ADVANCED_FACE('',(#8561),#2713,.T.);
#69312=ADVANCED_FACE('',(#8562),#2714,.T.);
#69313=ADVANCED_FACE('',(#8563),#2715,.T.);
#69314=ADVANCED_FACE('',(#8564),#2716,.T.);
#69315=ADVANCED_FACE('',(#8565),#2717,.T.);
#69316=ADVANCED_FACE('',(#8566),#2718,.T.);
#69317=ADVANCED_FACE('',(#8567),#2719,.T.);
#69318=ADVANCED_FACE('',(#8568),#2720,.T.);
#69319=ADVANCED_FACE('',(#8569),#2721,.T.);
#69320=ADVANCED_FACE('',(#8570),#2722,.T.);
#69321=ADVANCED_FACE('',(#8571),#2723,.T.);
#69322=ADVANCED_FACE('',(#8572),#2724,.T.);
#69323=ADVANCED_FACE('',(#8573),#2725,.T.);
#69324=ADVANCED_FACE('',(#8574),#2726,.T.);
#69325=ADVANCED_FACE('',(#8575),#2727,.T.);
#69326=ADVANCED_FACE('',(#8576),#2728,.T.);
#69327=ADVANCED_FACE('',(#8577),#2729,.T.);
#69328=ADVANCED_FACE('',(#8578),#2730,.T.);
#69329=ADVANCED_FACE('',(#8579),#2731,.T.);
#69330=ADVANCED_FACE('',(#8580),#2732,.T.);
#69331=ADVANCED_FACE('',(#8581),#2733,.T.);
#69332=ADVANCED_FACE('',(#8582),#2734,.T.);
#69333=ADVANCED_FACE('',(#8583),#2735,.T.);
#69334=ADVANCED_FACE('',(#8584),#2736,.T.);
#69335=ADVANCED_FACE('',(#8585),#2737,.T.);
#69336=ADVANCED_FACE('',(#8586),#2738,.T.);
#69337=ADVANCED_FACE('',(#8587),#2739,.T.);
#69338=ADVANCED_FACE('',(#8588),#2740,.T.);
#69339=ADVANCED_FACE('',(#8589),#2741,.T.);
#69340=ADVANCED_FACE('',(#8590),#2742,.T.);
#69341=ADVANCED_FACE('',(#8591),#2743,.T.);
#69342=ADVANCED_FACE('',(#8592),#2744,.T.);
#69343=ADVANCED_FACE('',(#8593),#2745,.T.);
#69344=ADVANCED_FACE('',(#8594),#2746,.T.);
#69345=ADVANCED_FACE('',(#8595),#5109,.T.);
#69346=ADVANCED_FACE('',(#8596),#2747,.T.);
#69347=ADVANCED_FACE('',(#8597),#2748,.T.);
#69348=ADVANCED_FACE('',(#8598),#5110,.T.);
#69349=ADVANCED_FACE('',(#8599),#2749,.T.);
#69350=ADVANCED_FACE('',(#8600),#2750,.T.);
#69351=ADVANCED_FACE('',(#8601),#5111,.T.);
#69352=ADVANCED_FACE('',(#8602),#2751,.T.);
#69353=ADVANCED_FACE('',(#8603),#2752,.T.);
#69354=ADVANCED_FACE('',(#8604),#5112,.T.);
#69355=ADVANCED_FACE('',(#8605),#2753,.T.);
#69356=ADVANCED_FACE('',(#8606),#2754,.T.);
#69357=ADVANCED_FACE('',(#8607),#5113,.T.);
#69358=ADVANCED_FACE('',(#8608),#2755,.T.);
#69359=ADVANCED_FACE('',(#8609),#2756,.T.);
#69360=ADVANCED_FACE('',(#8610),#5114,.T.);
#69361=ADVANCED_FACE('',(#8611),#2757,.T.);
#69362=ADVANCED_FACE('',(#8612),#2758,.T.);
#69363=ADVANCED_FACE('',(#8613),#5115,.T.);
#69364=ADVANCED_FACE('',(#8614),#2759,.T.);
#69365=ADVANCED_FACE('',(#8615),#2760,.T.);
#69366=ADVANCED_FACE('',(#8616),#5116,.T.);
#69367=ADVANCED_FACE('',(#8617),#2761,.T.);
#69368=ADVANCED_FACE('',(#8618),#2762,.T.);
#69369=ADVANCED_FACE('',(#8619),#5117,.T.);
#69370=ADVANCED_FACE('',(#8620),#2763,.T.);
#69371=ADVANCED_FACE('',(#8621),#2764,.T.);
#69372=ADVANCED_FACE('',(#8622),#5118,.T.);
#69373=ADVANCED_FACE('',(#8623),#2765,.T.);
#69374=ADVANCED_FACE('',(#8624),#2766,.T.);
#69375=ADVANCED_FACE('',(#8625),#5119,.T.);
#69376=ADVANCED_FACE('',(#8626),#2767,.T.);
#69377=ADVANCED_FACE('',(#8627),#2768,.T.);
#69378=ADVANCED_FACE('',(#8628),#5120,.T.);
#69379=ADVANCED_FACE('',(#8629),#2769,.T.);
#69380=ADVANCED_FACE('',(#8630),#2770,.T.);
#69381=ADVANCED_FACE('',(#8631),#5121,.T.);
#69382=ADVANCED_FACE('',(#8632),#2771,.T.);
#69383=ADVANCED_FACE('',(#8633),#2772,.T.);
#69384=ADVANCED_FACE('',(#8634),#5122,.T.);
#69385=ADVANCED_FACE('',(#8635),#2773,.T.);
#69386=ADVANCED_FACE('',(#8636),#2774,.T.);
#69387=ADVANCED_FACE('',(#8637),#2775,.T.);
#69388=ADVANCED_FACE('',(#8638),#2776,.T.);
#69389=ADVANCED_FACE('',(#8639),#5123,.T.);
#69390=ADVANCED_FACE('',(#8640),#2777,.T.);
#69391=ADVANCED_FACE('',(#8641),#2778,.T.);
#69392=ADVANCED_FACE('',(#8642),#5124,.T.);
#69393=ADVANCED_FACE('',(#8643),#2779,.T.);
#69394=ADVANCED_FACE('',(#8644),#2780,.T.);
#69395=ADVANCED_FACE('',(#8645),#5125,.T.);
#69396=ADVANCED_FACE('',(#8646),#2781,.T.);
#69397=ADVANCED_FACE('',(#8647),#2782,.T.);
#69398=ADVANCED_FACE('',(#8648),#5126,.T.);
#69399=ADVANCED_FACE('',(#8649),#2783,.T.);
#69400=ADVANCED_FACE('',(#8650),#2784,.T.);
#69401=ADVANCED_FACE('',(#8651),#2785,.T.);
#69402=ADVANCED_FACE('',(#8652),#5127,.T.);
#69403=ADVANCED_FACE('',(#8653),#2786,.T.);
#69404=ADVANCED_FACE('',(#8654),#5128,.T.);
#69405=ADVANCED_FACE('',(#8655),#2787,.T.);
#69406=ADVANCED_FACE('',(#8656),#2788,.T.);
#69407=ADVANCED_FACE('',(#8657),#5129,.T.);
#69408=ADVANCED_FACE('',(#8658),#2789,.T.);
#69409=ADVANCED_FACE('',(#8659),#2790,.T.);
#69410=ADVANCED_FACE('',(#8660),#5130,.T.);
#69411=ADVANCED_FACE('',(#8661),#2791,.T.);
#69412=ADVANCED_FACE('',(#8662),#2792,.T.);
#69413=ADVANCED_FACE('',(#8663),#5131,.T.);
#69414=ADVANCED_FACE('',(#8664),#2793,.T.);
#69415=ADVANCED_FACE('',(#8665),#2794,.T.);
#69416=ADVANCED_FACE('',(#8666),#5132,.T.);
#69417=ADVANCED_FACE('',(#8667),#2795,.T.);
#69418=ADVANCED_FACE('',(#8668),#2796,.T.);
#69419=ADVANCED_FACE('',(#8669),#5133,.T.);
#69420=ADVANCED_FACE('',(#8670),#2797,.T.);
#69421=ADVANCED_FACE('',(#8671),#2798,.T.);
#69422=ADVANCED_FACE('',(#8672),#5134,.T.);
#69423=ADVANCED_FACE('',(#8673),#2799,.T.);
#69424=ADVANCED_FACE('',(#8674),#2800,.T.);
#69425=ADVANCED_FACE('',(#8675),#5135,.T.);
#69426=ADVANCED_FACE('',(#8676),#2801,.T.);
#69427=ADVANCED_FACE('',(#8677),#2802,.T.);
#69428=ADVANCED_FACE('',(#8678),#5136,.T.);
#69429=ADVANCED_FACE('',(#8679),#2803,.T.);
#69430=ADVANCED_FACE('',(#8680),#2804,.T.);
#69431=ADVANCED_FACE('',(#8681),#2805,.T.);
#69432=ADVANCED_FACE('',(#8682),#5137,.T.);
#69433=ADVANCED_FACE('',(#8683),#2806,.T.);
#69434=ADVANCED_FACE('',(#8684),#2807,.T.);
#69435=ADVANCED_FACE('',(#8685),#5138,.T.);
#69436=ADVANCED_FACE('',(#8686),#2808,.T.);
#69437=ADVANCED_FACE('',(#8687),#2809,.T.);
#69438=ADVANCED_FACE('',(#8688),#5139,.T.);
#69439=ADVANCED_FACE('',(#8689),#2810,.T.);
#69440=ADVANCED_FACE('',(#8690),#2811,.T.);
#69441=ADVANCED_FACE('',(#8691),#5140,.T.);
#69442=ADVANCED_FACE('',(#8692),#2812,.T.);
#69443=ADVANCED_FACE('',(#8693),#2813,.T.);
#69444=ADVANCED_FACE('',(#8694),#5141,.T.);
#69445=ADVANCED_FACE('',(#8695),#2814,.T.);
#69446=ADVANCED_FACE('',(#8696),#2815,.T.);
#69447=ADVANCED_FACE('',(#8697),#5142,.T.);
#69448=ADVANCED_FACE('',(#8698),#2816,.T.);
#69449=ADVANCED_FACE('',(#8699),#2817,.T.);
#69450=ADVANCED_FACE('',(#8700),#5143,.T.);
#69451=ADVANCED_FACE('',(#8701),#2818,.T.);
#69452=ADVANCED_FACE('',(#8702),#2819,.T.);
#69453=ADVANCED_FACE('',(#8703),#5144,.T.);
#69454=ADVANCED_FACE('',(#8704),#2820,.T.);
#69455=ADVANCED_FACE('',(#8705),#2821,.T.);
#69456=ADVANCED_FACE('',(#8706),#5145,.T.);
#69457=ADVANCED_FACE('',(#8707),#2822,.T.);
#69458=ADVANCED_FACE('',(#8708),#2823,.T.);
#69459=ADVANCED_FACE('',(#8709),#5146,.T.);
#69460=ADVANCED_FACE('',(#8710),#2824,.T.);
#69461=ADVANCED_FACE('',(#8711),#2825,.T.);
#69462=ADVANCED_FACE('',(#8712),#5147,.T.);
#69463=ADVANCED_FACE('',(#8713),#2826,.T.);
#69464=ADVANCED_FACE('',(#8714),#2827,.T.);
#69465=ADVANCED_FACE('',(#8715),#5148,.T.);
#69466=ADVANCED_FACE('',(#8716),#2828,.T.);
#69467=ADVANCED_FACE('',(#8717),#2829,.T.);
#69468=ADVANCED_FACE('',(#8718),#5149,.T.);
#69469=ADVANCED_FACE('',(#8719),#2830,.T.);
#69470=ADVANCED_FACE('',(#8720),#2831,.T.);
#69471=ADVANCED_FACE('',(#8721),#5150,.T.);
#69472=ADVANCED_FACE('',(#8722),#2832,.T.);
#69473=ADVANCED_FACE('',(#8723),#2833,.T.);
#69474=ADVANCED_FACE('',(#8724),#5151,.T.);
#69475=ADVANCED_FACE('',(#8725),#2834,.T.);
#69476=ADVANCED_FACE('',(#8726),#2835,.T.);
#69477=ADVANCED_FACE('',(#8727),#5152,.T.);
#69478=ADVANCED_FACE('',(#8728),#2836,.T.);
#69479=ADVANCED_FACE('',(#8729),#2837,.T.);
#69480=ADVANCED_FACE('',(#8730),#5153,.T.);
#69481=ADVANCED_FACE('',(#8731),#2838,.T.);
#69482=ADVANCED_FACE('',(#8732),#2839,.T.);
#69483=ADVANCED_FACE('',(#8733),#5154,.T.);
#69484=ADVANCED_FACE('',(#8734),#2840,.T.);
#69485=ADVANCED_FACE('',(#8735),#2841,.T.);
#69486=ADVANCED_FACE('',(#8736),#5155,.T.);
#69487=ADVANCED_FACE('',(#8737),#2842,.T.);
#69488=ADVANCED_FACE('',(#8738),#2843,.T.);
#69489=ADVANCED_FACE('',(#8739),#5156,.T.);
#69490=ADVANCED_FACE('',(#8740),#2844,.T.);
#69491=ADVANCED_FACE('',(#8741),#2845,.T.);
#69492=ADVANCED_FACE('',(#8742),#5157,.T.);
#69493=ADVANCED_FACE('',(#8743),#2846,.T.);
#69494=ADVANCED_FACE('',(#8744),#2847,.T.);
#69495=ADVANCED_FACE('',(#8745),#2848,.T.);
#69496=ADVANCED_FACE('',(#8746),#2849,.T.);
#69497=ADVANCED_FACE('',(#8747),#5158,.T.);
#69498=ADVANCED_FACE('',(#8748),#2850,.T.);
#69499=ADVANCED_FACE('',(#8749),#2851,.T.);
#69500=ADVANCED_FACE('',(#8750),#5159,.T.);
#69501=ADVANCED_FACE('',(#8751),#2852,.T.);
#69502=ADVANCED_FACE('',(#8752),#2853,.T.);
#69503=ADVANCED_FACE('',(#8753),#5160,.T.);
#69504=ADVANCED_FACE('',(#8754),#2854,.T.);
#69505=ADVANCED_FACE('',(#8755),#2855,.T.);
#69506=ADVANCED_FACE('',(#8756),#5161,.T.);
#69507=ADVANCED_FACE('',(#8757),#2856,.T.);
#69508=ADVANCED_FACE('',(#8758),#2857,.T.);
#69509=ADVANCED_FACE('',(#8759),#5162,.T.);
#69510=ADVANCED_FACE('',(#8760),#2858,.T.);
#69511=ADVANCED_FACE('',(#8761),#2859,.T.);
#69512=ADVANCED_FACE('',(#8762),#5163,.T.);
#69513=ADVANCED_FACE('',(#8763),#2860,.T.);
#69514=ADVANCED_FACE('',(#8764),#2861,.T.);
#69515=ADVANCED_FACE('',(#8765),#5164,.T.);
#69516=ADVANCED_FACE('',(#8766),#2862,.T.);
#69517=ADVANCED_FACE('',(#8767),#2863,.T.);
#69518=ADVANCED_FACE('',(#8768),#2864,.T.);
#69519=ADVANCED_FACE('',(#8769),#2865,.T.);
#69520=ADVANCED_FACE('',(#8770),#2866,.T.);
#69521=ADVANCED_FACE('',(#8771),#2867,.T.);
#69522=ADVANCED_FACE('',(#8772),#2868,.T.);
#69523=ADVANCED_FACE('',(#8773),#2869,.T.);
#69524=ADVANCED_FACE('',(#8774),#2870,.T.);
#69525=ADVANCED_FACE('',(#8775),#2871,.T.);
#69526=ADVANCED_FACE('',(#8776),#2872,.T.);
#69527=ADVANCED_FACE('',(#8777),#2873,.T.);
#69528=ADVANCED_FACE('',(#8778),#2874,.T.);
#69529=ADVANCED_FACE('',(#8779),#2875,.T.);
#69530=ADVANCED_FACE('',(#8780),#2876,.T.);
#69531=ADVANCED_FACE('',(#8781),#2877,.T.);
#69532=ADVANCED_FACE('',(#8782),#2878,.T.);
#69533=ADVANCED_FACE('',(#8783),#2879,.T.);
#69534=ADVANCED_FACE('',(#8784),#2880,.T.);
#69535=ADVANCED_FACE('',(#8785),#2881,.T.);
#69536=ADVANCED_FACE('',(#8786),#2882,.T.);
#69537=ADVANCED_FACE('',(#8787),#2883,.T.);
#69538=ADVANCED_FACE('',(#8788),#2884,.T.);
#69539=ADVANCED_FACE('',(#8789),#2885,.T.);
#69540=ADVANCED_FACE('',(#8790),#2886,.T.);
#69541=ADVANCED_FACE('',(#8791),#2887,.T.);
#69542=ADVANCED_FACE('',(#8792),#2888,.T.);
#69543=ADVANCED_FACE('',(#8793),#2889,.T.);
#69544=ADVANCED_FACE('',(#8794),#2890,.T.);
#69545=ADVANCED_FACE('',(#8795),#2891,.T.);
#69546=ADVANCED_FACE('',(#8796),#2892,.T.);
#69547=ADVANCED_FACE('',(#8797),#2893,.T.);
#69548=ADVANCED_FACE('',(#8798),#2894,.T.);
#69549=ADVANCED_FACE('',(#8799),#2895,.T.);
#69550=ADVANCED_FACE('',(#8800),#2896,.T.);
#69551=ADVANCED_FACE('',(#8801),#2897,.T.);
#69552=ADVANCED_FACE('',(#8802),#2898,.T.);
#69553=ADVANCED_FACE('',(#8803),#2899,.T.);
#69554=ADVANCED_FACE('',(#8804),#2900,.T.);
#69555=ADVANCED_FACE('',(#8805),#2901,.T.);
#69556=ADVANCED_FACE('',(#8806),#2902,.T.);
#69557=ADVANCED_FACE('',(#8807),#2903,.T.);
#69558=ADVANCED_FACE('',(#8808),#2904,.T.);
#69559=ADVANCED_FACE('',(#8809),#2905,.T.);
#69560=ADVANCED_FACE('',(#8810),#2906,.T.);
#69561=ADVANCED_FACE('',(#8811),#2907,.T.);
#69562=ADVANCED_FACE('',(#8812),#2908,.T.);
#69563=ADVANCED_FACE('',(#8813),#2909,.T.);
#69564=ADVANCED_FACE('',(#8814),#2910,.T.);
#69565=ADVANCED_FACE('',(#8815),#2911,.T.);
#69566=ADVANCED_FACE('',(#8816),#2912,.T.);
#69567=ADVANCED_FACE('',(#8817),#2913,.T.);
#69568=ADVANCED_FACE('',(#8818),#2914,.T.);
#69569=ADVANCED_FACE('',(#8819),#2915,.T.);
#69570=ADVANCED_FACE('',(#8820),#2916,.T.);
#69571=ADVANCED_FACE('',(#8821),#2917,.T.);
#69572=ADVANCED_FACE('',(#8822),#2918,.T.);
#69573=ADVANCED_FACE('',(#8823),#2919,.T.);
#69574=ADVANCED_FACE('',(#8824),#2920,.T.);
#69575=ADVANCED_FACE('',(#8825),#2921,.T.);
#69576=ADVANCED_FACE('',(#8826),#2922,.T.);
#69577=ADVANCED_FACE('',(#8827),#2923,.T.);
#69578=ADVANCED_FACE('',(#8828),#2924,.T.);
#69579=ADVANCED_FACE('',(#8829),#2925,.T.);
#69580=ADVANCED_FACE('',(#8830),#2926,.T.);
#69581=ADVANCED_FACE('',(#8831),#2927,.T.);
#69582=ADVANCED_FACE('',(#8832),#2928,.T.);
#69583=ADVANCED_FACE('',(#8833),#2929,.T.);
#69584=ADVANCED_FACE('',(#8834),#2930,.T.);
#69585=ADVANCED_FACE('',(#8835),#2931,.T.);
#69586=ADVANCED_FACE('',(#8836),#2932,.T.);
#69587=ADVANCED_FACE('',(#8837),#2933,.T.);
#69588=ADVANCED_FACE('',(#8838),#2934,.T.);
#69589=ADVANCED_FACE('',(#8839),#2935,.T.);
#69590=ADVANCED_FACE('',(#8840),#2936,.T.);
#69591=ADVANCED_FACE('',(#8841),#2937,.T.);
#69592=ADVANCED_FACE('',(#8842),#2938,.T.);
#69593=ADVANCED_FACE('',(#8843),#2939,.T.);
#69594=ADVANCED_FACE('',(#8844),#2940,.T.);
#69595=ADVANCED_FACE('',(#8845),#2941,.T.);
#69596=ADVANCED_FACE('',(#8846),#2942,.T.);
#69597=ADVANCED_FACE('',(#8847),#2943,.T.);
#69598=ADVANCED_FACE('',(#8848),#2944,.T.);
#69599=ADVANCED_FACE('',(#8849),#2945,.T.);
#69600=ADVANCED_FACE('',(#8850),#2946,.T.);
#69601=ADVANCED_FACE('',(#8851),#2947,.T.);
#69602=ADVANCED_FACE('',(#8852),#2948,.T.);
#69603=ADVANCED_FACE('',(#8853),#2949,.T.);
#69604=ADVANCED_FACE('',(#8854),#2950,.T.);
#69605=ADVANCED_FACE('',(#8855),#2951,.T.);
#69606=ADVANCED_FACE('',(#8856),#2952,.T.);
#69607=ADVANCED_FACE('',(#8857),#2953,.T.);
#69608=ADVANCED_FACE('',(#8858),#2954,.T.);
#69609=ADVANCED_FACE('',(#8859),#2955,.T.);
#69610=ADVANCED_FACE('',(#8860),#2956,.T.);
#69611=ADVANCED_FACE('',(#8861),#2957,.T.);
#69612=ADVANCED_FACE('',(#8862),#2958,.T.);
#69613=ADVANCED_FACE('',(#8863),#2959,.T.);
#69614=ADVANCED_FACE('',(#8864),#2960,.T.);
#69615=ADVANCED_FACE('',(#8865),#2961,.T.);
#69616=ADVANCED_FACE('',(#8866),#2962,.T.);
#69617=ADVANCED_FACE('',(#8867),#2963,.T.);
#69618=ADVANCED_FACE('',(#8868),#2964,.T.);
#69619=ADVANCED_FACE('',(#8869),#2965,.T.);
#69620=ADVANCED_FACE('',(#8870),#2966,.T.);
#69621=ADVANCED_FACE('',(#8871),#2967,.T.);
#69622=ADVANCED_FACE('',(#8872),#2968,.T.);
#69623=ADVANCED_FACE('',(#8873),#2969,.T.);
#69624=ADVANCED_FACE('',(#8874),#2970,.T.);
#69625=ADVANCED_FACE('',(#8875),#2971,.T.);
#69626=ADVANCED_FACE('',(#8876),#2972,.T.);
#69627=ADVANCED_FACE('',(#8877),#2973,.T.);
#69628=ADVANCED_FACE('',(#8878),#2974,.T.);
#69629=ADVANCED_FACE('',(#8879),#2975,.T.);
#69630=ADVANCED_FACE('',(#8880),#2976,.T.);
#69631=ADVANCED_FACE('',(#8881),#2977,.T.);
#69632=ADVANCED_FACE('',(#8882),#2978,.T.);
#69633=ADVANCED_FACE('',(#8883),#2979,.T.);
#69634=ADVANCED_FACE('',(#8884),#5165,.T.);
#69635=ADVANCED_FACE('',(#8885),#2980,.T.);
#69636=ADVANCED_FACE('',(#8886),#2981,.T.);
#69637=ADVANCED_FACE('',(#8887),#5166,.T.);
#69638=ADVANCED_FACE('',(#8888),#2982,.T.);
#69639=ADVANCED_FACE('',(#8889),#2983,.T.);
#69640=ADVANCED_FACE('',(#8890),#5167,.T.);
#69641=ADVANCED_FACE('',(#8891),#2984,.T.);
#69642=ADVANCED_FACE('',(#8892),#2985,.T.);
#69643=ADVANCED_FACE('',(#8893),#5168,.T.);
#69644=ADVANCED_FACE('',(#8894),#2986,.T.);
#69645=ADVANCED_FACE('',(#8895),#2987,.T.);
#69646=ADVANCED_FACE('',(#8896),#5169,.T.);
#69647=ADVANCED_FACE('',(#8897),#2988,.T.);
#69648=ADVANCED_FACE('',(#8898),#2989,.T.);
#69649=ADVANCED_FACE('',(#8899),#5170,.T.);
#69650=ADVANCED_FACE('',(#8900),#2990,.T.);
#69651=ADVANCED_FACE('',(#8901),#2991,.T.);
#69652=ADVANCED_FACE('',(#8902),#2992,.T.);
#69653=ADVANCED_FACE('',(#8903),#2993,.T.);
#69654=ADVANCED_FACE('',(#8904),#5171,.T.);
#69655=ADVANCED_FACE('',(#8905),#2994,.T.);
#69656=ADVANCED_FACE('',(#8906),#2995,.T.);
#69657=ADVANCED_FACE('',(#8907),#5172,.T.);
#69658=ADVANCED_FACE('',(#8908),#2996,.T.);
#69659=ADVANCED_FACE('',(#8909),#2997,.T.);
#69660=ADVANCED_FACE('',(#8910),#5173,.T.);
#69661=ADVANCED_FACE('',(#8911),#2998,.T.);
#69662=ADVANCED_FACE('',(#8912),#2999,.T.);
#69663=ADVANCED_FACE('',(#8913),#5174,.T.);
#69664=ADVANCED_FACE('',(#8914),#3000,.T.);
#69665=ADVANCED_FACE('',(#8915),#3001,.T.);
#69666=ADVANCED_FACE('',(#8916),#5175,.T.);
#69667=ADVANCED_FACE('',(#8917),#3002,.T.);
#69668=ADVANCED_FACE('',(#8918),#3003,.T.);
#69669=ADVANCED_FACE('',(#8919),#5176,.T.);
#69670=ADVANCED_FACE('',(#8920),#3004,.T.);
#69671=ADVANCED_FACE('',(#8921),#3005,.T.);
#69672=ADVANCED_FACE('',(#8922),#5177,.T.);
#69673=ADVANCED_FACE('',(#8923),#3006,.T.);
#69674=ADVANCED_FACE('',(#8924),#3007,.T.);
#69675=ADVANCED_FACE('',(#8925),#5178,.T.);
#69676=ADVANCED_FACE('',(#8926),#3008,.T.);
#69677=ADVANCED_FACE('',(#8927),#3009,.T.);
#69678=ADVANCED_FACE('',(#8928),#5179,.T.);
#69679=ADVANCED_FACE('',(#8929),#3010,.T.);
#69680=ADVANCED_FACE('',(#8930),#3011,.T.);
#69681=ADVANCED_FACE('',(#8931),#5180,.T.);
#69682=ADVANCED_FACE('',(#8932),#3012,.T.);
#69683=ADVANCED_FACE('',(#8933),#3013,.T.);
#69684=ADVANCED_FACE('',(#8934),#5181,.T.);
#69685=ADVANCED_FACE('',(#8935),#3014,.T.);
#69686=ADVANCED_FACE('',(#8936),#3015,.T.);
#69687=ADVANCED_FACE('',(#8937),#3016,.T.);
#69688=ADVANCED_FACE('',(#8938),#5182,.T.);
#69689=ADVANCED_FACE('',(#8939),#3017,.T.);
#69690=ADVANCED_FACE('',(#8940),#5183,.T.);
#69691=ADVANCED_FACE('',(#8941),#3018,.T.);
#69692=ADVANCED_FACE('',(#8942),#3019,.T.);
#69693=ADVANCED_FACE('',(#8943),#5184,.T.);
#69694=ADVANCED_FACE('',(#8944),#3020,.T.);
#69695=ADVANCED_FACE('',(#8945),#3021,.T.);
#69696=ADVANCED_FACE('',(#8946),#5185,.T.);
#69697=ADVANCED_FACE('',(#8947),#3022,.T.);
#69698=ADVANCED_FACE('',(#8948),#3023,.T.);
#69699=ADVANCED_FACE('',(#8949),#5186,.T.);
#69700=ADVANCED_FACE('',(#8950),#3024,.T.);
#69701=ADVANCED_FACE('',(#8951),#3025,.T.);
#69702=ADVANCED_FACE('',(#8952),#5187,.T.);
#69703=ADVANCED_FACE('',(#8953),#3026,.T.);
#69704=ADVANCED_FACE('',(#8954),#3027,.T.);
#69705=ADVANCED_FACE('',(#8955),#5188,.T.);
#69706=ADVANCED_FACE('',(#8956),#3028,.T.);
#69707=ADVANCED_FACE('',(#8957),#3029,.T.);
#69708=ADVANCED_FACE('',(#8958),#5189,.T.);
#69709=ADVANCED_FACE('',(#8959),#3030,.T.);
#69710=ADVANCED_FACE('',(#8960),#3031,.T.);
#69711=ADVANCED_FACE('',(#8961),#5190,.T.);
#69712=ADVANCED_FACE('',(#8962),#3032,.T.);
#69713=ADVANCED_FACE('',(#8963),#3033,.T.);
#69714=ADVANCED_FACE('',(#8964),#5191,.T.);
#69715=ADVANCED_FACE('',(#8965),#3034,.T.);
#69716=ADVANCED_FACE('',(#8966),#5192,.T.);
#69717=ADVANCED_FACE('',(#8967),#3035,.T.);
#69718=ADVANCED_FACE('',(#8968),#3036,.T.);
#69719=ADVANCED_FACE('',(#8969),#3037,.T.);
#69720=ADVANCED_FACE('',(#8970),#3038,.T.);
#69721=ADVANCED_FACE('',(#8971),#5193,.T.);
#69722=ADVANCED_FACE('',(#8972),#3039,.T.);
#69723=ADVANCED_FACE('',(#8973),#3040,.T.);
#69724=ADVANCED_FACE('',(#8974),#5194,.T.);
#69725=ADVANCED_FACE('',(#8975),#3041,.T.);
#69726=ADVANCED_FACE('',(#8976),#3042,.T.);
#69727=ADVANCED_FACE('',(#8977),#5195,.T.);
#69728=ADVANCED_FACE('',(#8978),#3043,.T.);
#69729=ADVANCED_FACE('',(#8979),#3044,.T.);
#69730=ADVANCED_FACE('',(#8980),#5196,.T.);
#69731=ADVANCED_FACE('',(#8981),#3045,.T.);
#69732=ADVANCED_FACE('',(#8982),#3046,.T.);
#69733=ADVANCED_FACE('',(#8983),#5197,.T.);
#69734=ADVANCED_FACE('',(#8984),#3047,.T.);
#69735=ADVANCED_FACE('',(#8985),#3048,.T.);
#69736=ADVANCED_FACE('',(#8986),#5198,.T.);
#69737=ADVANCED_FACE('',(#8987),#3049,.T.);
#69738=ADVANCED_FACE('',(#8988),#3050,.T.);
#69739=ADVANCED_FACE('',(#8989),#5199,.T.);
#69740=ADVANCED_FACE('',(#8990),#3051,.T.);
#69741=ADVANCED_FACE('',(#8991),#3052,.T.);
#69742=ADVANCED_FACE('',(#8992),#5200,.T.);
#69743=ADVANCED_FACE('',(#8993),#3053,.T.);
#69744=ADVANCED_FACE('',(#8994),#3054,.T.);
#69745=ADVANCED_FACE('',(#8995),#5201,.T.);
#69746=ADVANCED_FACE('',(#8996),#3055,.T.);
#69747=ADVANCED_FACE('',(#8997),#3056,.T.);
#69748=ADVANCED_FACE('',(#8998),#5202,.T.);
#69749=ADVANCED_FACE('',(#8999),#3057,.T.);
#69750=ADVANCED_FACE('',(#9000),#3058,.T.);
#69751=ADVANCED_FACE('',(#9001),#5203,.T.);
#69752=ADVANCED_FACE('',(#9002),#3059,.T.);
#69753=ADVANCED_FACE('',(#9003),#3060,.T.);
#69754=ADVANCED_FACE('',(#9004),#5204,.T.);
#69755=ADVANCED_FACE('',(#9005),#3061,.T.);
#69756=ADVANCED_FACE('',(#9006),#3062,.T.);
#69757=ADVANCED_FACE('',(#9007),#5205,.T.);
#69758=ADVANCED_FACE('',(#9008),#3063,.T.);
#69759=ADVANCED_FACE('',(#9009),#3064,.T.);
#69760=ADVANCED_FACE('',(#9010),#3065,.T.);
#69761=ADVANCED_FACE('',(#9011),#3066,.T.);
#69762=ADVANCED_FACE('',(#9012),#5206,.T.);
#69763=ADVANCED_FACE('',(#9013),#3067,.T.);
#69764=ADVANCED_FACE('',(#9014),#3068,.T.);
#69765=ADVANCED_FACE('',(#9015),#5207,.T.);
#69766=ADVANCED_FACE('',(#9016),#3069,.T.);
#69767=ADVANCED_FACE('',(#9017),#3070,.T.);
#69768=ADVANCED_FACE('',(#9018),#5208,.T.);
#69769=ADVANCED_FACE('',(#9019),#3071,.T.);
#69770=ADVANCED_FACE('',(#9020),#3072,.T.);
#69771=ADVANCED_FACE('',(#9021),#5209,.T.);
#69772=ADVANCED_FACE('',(#9022),#3073,.T.);
#69773=ADVANCED_FACE('',(#9023),#3074,.T.);
#69774=ADVANCED_FACE('',(#9024),#5210,.T.);
#69775=ADVANCED_FACE('',(#9025),#3075,.T.);
#69776=ADVANCED_FACE('',(#9026),#3076,.T.);
#69777=ADVANCED_FACE('',(#9027),#5211,.T.);
#69778=ADVANCED_FACE('',(#9028),#3077,.T.);
#69779=ADVANCED_FACE('',(#9029),#3078,.T.);
#69780=ADVANCED_FACE('',(#9030),#5212,.T.);
#69781=ADVANCED_FACE('',(#9031),#3079,.T.);
#69782=ADVANCED_FACE('',(#9032),#3080,.T.);
#69783=ADVANCED_FACE('',(#9033),#5213,.T.);
#69784=ADVANCED_FACE('',(#9034),#3081,.T.);
#69785=ADVANCED_FACE('',(#9035),#3082,.T.);
#69786=ADVANCED_FACE('',(#9036),#5214,.T.);
#69787=ADVANCED_FACE('',(#9037),#3083,.T.);
#69788=ADVANCED_FACE('',(#9038),#3084,.T.);
#69789=ADVANCED_FACE('',(#9039),#5215,.T.);
#69790=ADVANCED_FACE('',(#9040),#3085,.T.);
#69791=ADVANCED_FACE('',(#9041),#3086,.T.);
#69792=ADVANCED_FACE('',(#9042),#5216,.T.);
#69793=ADVANCED_FACE('',(#9043),#3087,.T.);
#69794=ADVANCED_FACE('',(#9044),#3088,.T.);
#69795=ADVANCED_FACE('',(#9045),#5217,.T.);
#69796=ADVANCED_FACE('',(#9046),#3089,.T.);
#69797=ADVANCED_FACE('',(#9047),#3090,.T.);
#69798=ADVANCED_FACE('',(#9048),#5218,.T.);
#69799=ADVANCED_FACE('',(#9049),#3091,.T.);
#69800=ADVANCED_FACE('',(#9050),#3092,.T.);
#69801=ADVANCED_FACE('',(#9051),#5219,.T.);
#69802=ADVANCED_FACE('',(#9052),#5220,.T.);
#69803=ADVANCED_FACE('',(#9053),#3093,.T.);
#69804=ADVANCED_FACE('',(#9054),#3094,.T.);
#69805=ADVANCED_FACE('',(#9055),#3095,.T.);
#69806=ADVANCED_FACE('',(#9056),#3096,.T.);
#69807=ADVANCED_FACE('',(#9057),#3097,.T.);
#69808=ADVANCED_FACE('',(#9058),#3098,.T.);
#69809=ADVANCED_FACE('',(#9059),#3099,.T.);
#69810=ADVANCED_FACE('',(#9060),#3100,.T.);
#69811=ADVANCED_FACE('',(#9061),#3101,.T.);
#69812=ADVANCED_FACE('',(#9062),#3102,.T.);
#69813=ADVANCED_FACE('',(#9063),#3103,.T.);
#69814=ADVANCED_FACE('',(#9064),#3104,.T.);
#69815=ADVANCED_FACE('',(#9065),#3105,.T.);
#69816=ADVANCED_FACE('',(#9066),#3106,.T.);
#69817=ADVANCED_FACE('',(#9067),#3107,.T.);
#69818=ADVANCED_FACE('',(#9068),#3108,.T.);
#69819=ADVANCED_FACE('',(#9069),#3109,.T.);
#69820=ADVANCED_FACE('',(#9070),#3110,.T.);
#69821=ADVANCED_FACE('',(#9071),#3111,.T.);
#69822=ADVANCED_FACE('',(#9072),#3112,.T.);
#69823=ADVANCED_FACE('',(#9073),#3113,.T.);
#69824=ADVANCED_FACE('',(#9074),#3114,.T.);
#69825=ADVANCED_FACE('',(#9075),#3115,.T.);
#69826=ADVANCED_FACE('',(#9076),#3116,.T.);
#69827=ADVANCED_FACE('',(#9077),#3117,.T.);
#69828=ADVANCED_FACE('',(#9078),#3118,.T.);
#69829=ADVANCED_FACE('',(#9079),#3119,.T.);
#69830=ADVANCED_FACE('',(#9080),#3120,.T.);
#69831=ADVANCED_FACE('',(#9081),#3121,.T.);
#69832=ADVANCED_FACE('',(#9082),#3122,.T.);
#69833=ADVANCED_FACE('',(#9083),#3123,.T.);
#69834=ADVANCED_FACE('',(#9084),#3124,.T.);
#69835=ADVANCED_FACE('',(#9085),#3125,.T.);
#69836=ADVANCED_FACE('',(#9086),#3126,.T.);
#69837=ADVANCED_FACE('',(#9087),#3127,.T.);
#69838=ADVANCED_FACE('',(#9088),#3128,.T.);
#69839=ADVANCED_FACE('',(#9089),#3129,.T.);
#69840=ADVANCED_FACE('',(#9090),#3130,.T.);
#69841=ADVANCED_FACE('',(#9091),#3131,.T.);
#69842=ADVANCED_FACE('',(#9092),#3132,.T.);
#69843=ADVANCED_FACE('',(#9093),#3133,.T.);
#69844=ADVANCED_FACE('',(#9094),#3134,.T.);
#69845=ADVANCED_FACE('',(#9095),#3135,.T.);
#69846=ADVANCED_FACE('',(#9096),#3136,.T.);
#69847=ADVANCED_FACE('',(#9097),#3137,.T.);
#69848=ADVANCED_FACE('',(#9098),#3138,.T.);
#69849=ADVANCED_FACE('',(#9099),#3139,.T.);
#69850=ADVANCED_FACE('',(#9100),#3140,.T.);
#69851=ADVANCED_FACE('',(#9101),#3141,.T.);
#69852=ADVANCED_FACE('',(#9102),#3142,.T.);
#69853=ADVANCED_FACE('',(#9103),#3143,.T.);
#69854=ADVANCED_FACE('',(#9104),#3144,.T.);
#69855=ADVANCED_FACE('',(#9105),#3145,.T.);
#69856=ADVANCED_FACE('',(#9106),#3146,.T.);
#69857=ADVANCED_FACE('',(#9107),#3147,.T.);
#69858=ADVANCED_FACE('',(#9108),#3148,.T.);
#69859=ADVANCED_FACE('',(#9109),#3149,.T.);
#69860=ADVANCED_FACE('',(#9110),#3150,.T.);
#69861=ADVANCED_FACE('',(#9111),#3151,.T.);
#69862=ADVANCED_FACE('',(#9112),#3152,.T.);
#69863=ADVANCED_FACE('',(#9113),#3153,.T.);
#69864=ADVANCED_FACE('',(#9114),#3154,.T.);
#69865=ADVANCED_FACE('',(#9115),#3155,.T.);
#69866=ADVANCED_FACE('',(#9116),#3156,.T.);
#69867=ADVANCED_FACE('',(#9117),#3157,.T.);
#69868=ADVANCED_FACE('',(#9118),#3158,.T.);
#69869=ADVANCED_FACE('',(#9119),#3159,.T.);
#69870=ADVANCED_FACE('',(#9120),#3160,.T.);
#69871=ADVANCED_FACE('',(#9121),#3161,.T.);
#69872=ADVANCED_FACE('',(#9122),#3162,.T.);
#69873=ADVANCED_FACE('',(#9123),#3163,.T.);
#69874=ADVANCED_FACE('',(#9124),#3164,.T.);
#69875=ADVANCED_FACE('',(#9125),#3165,.T.);
#69876=ADVANCED_FACE('',(#9126),#3166,.T.);
#69877=ADVANCED_FACE('',(#9127),#3167,.T.);
#69878=ADVANCED_FACE('',(#9128),#3168,.T.);
#69879=ADVANCED_FACE('',(#9129),#3169,.T.);
#69880=ADVANCED_FACE('',(#9130),#3170,.T.);
#69881=ADVANCED_FACE('',(#9131),#3171,.T.);
#69882=ADVANCED_FACE('',(#9132),#3172,.T.);
#69883=ADVANCED_FACE('',(#9133),#3173,.T.);
#69884=ADVANCED_FACE('',(#9134),#3174,.T.);
#69885=ADVANCED_FACE('',(#9135),#3175,.T.);
#69886=ADVANCED_FACE('',(#9136),#3176,.T.);
#69887=ADVANCED_FACE('',(#9137),#3177,.T.);
#69888=ADVANCED_FACE('',(#9138),#3178,.T.);
#69889=ADVANCED_FACE('',(#9139),#3179,.T.);
#69890=ADVANCED_FACE('',(#9140),#3180,.T.);
#69891=ADVANCED_FACE('',(#9141),#3181,.T.);
#69892=ADVANCED_FACE('',(#9142),#3182,.T.);
#69893=ADVANCED_FACE('',(#9143),#3183,.T.);
#69894=ADVANCED_FACE('',(#9144),#3184,.T.);
#69895=ADVANCED_FACE('',(#9145),#3185,.T.);
#69896=ADVANCED_FACE('',(#9146),#3186,.T.);
#69897=ADVANCED_FACE('',(#9147),#3187,.T.);
#69898=ADVANCED_FACE('',(#9148),#3188,.T.);
#69899=ADVANCED_FACE('',(#9149),#3189,.T.);
#69900=ADVANCED_FACE('',(#9150),#3190,.T.);
#69901=ADVANCED_FACE('',(#9151),#3191,.T.);
#69902=ADVANCED_FACE('',(#9152),#3192,.T.);
#69903=ADVANCED_FACE('',(#9153),#3193,.T.);
#69904=ADVANCED_FACE('',(#9154),#3194,.T.);
#69905=ADVANCED_FACE('',(#9155),#3195,.T.);
#69906=ADVANCED_FACE('',(#9156),#3196,.T.);
#69907=ADVANCED_FACE('',(#9157),#3197,.T.);
#69908=ADVANCED_FACE('',(#9158),#3198,.T.);
#69909=ADVANCED_FACE('',(#9159),#3199,.T.);
#69910=ADVANCED_FACE('',(#9160),#3200,.T.);
#69911=ADVANCED_FACE('',(#9161),#3201,.T.);
#69912=ADVANCED_FACE('',(#9162),#3202,.T.);
#69913=ADVANCED_FACE('',(#9163),#3203,.T.);
#69914=ADVANCED_FACE('',(#9164),#3204,.T.);
#69915=ADVANCED_FACE('',(#9165),#3205,.T.);
#69916=ADVANCED_FACE('',(#9166),#3206,.T.);
#69917=ADVANCED_FACE('',(#9167),#3207,.T.);
#69918=ADVANCED_FACE('',(#9168),#3208,.T.);
#69919=ADVANCED_FACE('',(#9169),#3209,.T.);
#69920=ADVANCED_FACE('',(#9170),#3210,.T.);
#69921=ADVANCED_FACE('',(#9171),#5221,.T.);
#69922=ADVANCED_FACE('',(#9172),#3211,.T.);
#69923=ADVANCED_FACE('',(#9173),#3212,.T.);
#69924=ADVANCED_FACE('',(#9174),#5222,.T.);
#69925=ADVANCED_FACE('',(#9175),#3213,.T.);
#69926=ADVANCED_FACE('',(#9176),#3214,.T.);
#69927=ADVANCED_FACE('',(#9177),#5223,.T.);
#69928=ADVANCED_FACE('',(#9178),#3215,.T.);
#69929=ADVANCED_FACE('',(#9179),#3216,.T.);
#69930=ADVANCED_FACE('',(#9180),#5224,.T.);
#69931=ADVANCED_FACE('',(#9181),#3217,.T.);
#69932=ADVANCED_FACE('',(#9182),#3218,.T.);
#69933=ADVANCED_FACE('',(#9183),#5225,.T.);
#69934=ADVANCED_FACE('',(#9184),#3219,.T.);
#69935=ADVANCED_FACE('',(#9185),#3220,.T.);
#69936=ADVANCED_FACE('',(#9186),#5226,.T.);
#69937=ADVANCED_FACE('',(#9187),#3221,.T.);
#69938=ADVANCED_FACE('',(#9188),#3222,.T.);
#69939=ADVANCED_FACE('',(#9189),#5227,.T.);
#69940=ADVANCED_FACE('',(#9190),#3223,.T.);
#69941=ADVANCED_FACE('',(#9191),#3224,.T.);
#69942=ADVANCED_FACE('',(#9192),#5228,.T.);
#69943=ADVANCED_FACE('',(#9193),#3225,.T.);
#69944=ADVANCED_FACE('',(#9194),#3226,.T.);
#69945=ADVANCED_FACE('',(#9195),#5229,.T.);
#69946=ADVANCED_FACE('',(#9196),#3227,.T.);
#69947=ADVANCED_FACE('',(#9197),#3228,.T.);
#69948=ADVANCED_FACE('',(#9198),#5230,.T.);
#69949=ADVANCED_FACE('',(#9199),#3229,.T.);
#69950=ADVANCED_FACE('',(#9200),#3230,.T.);
#69951=ADVANCED_FACE('',(#9201),#5231,.T.);
#69952=ADVANCED_FACE('',(#9202),#3231,.T.);
#69953=ADVANCED_FACE('',(#9203),#3232,.T.);
#69954=ADVANCED_FACE('',(#9204),#5232,.T.);
#69955=ADVANCED_FACE('',(#9205),#3233,.T.);
#69956=ADVANCED_FACE('',(#9206),#3234,.T.);
#69957=ADVANCED_FACE('',(#9207),#5233,.T.);
#69958=ADVANCED_FACE('',(#9208),#3235,.T.);
#69959=ADVANCED_FACE('',(#9209),#3236,.T.);
#69960=ADVANCED_FACE('',(#9210),#5234,.T.);
#69961=ADVANCED_FACE('',(#9211),#3237,.T.);
#69962=ADVANCED_FACE('',(#9212),#3238,.T.);
#69963=ADVANCED_FACE('',(#9213),#3239,.T.);
#69964=ADVANCED_FACE('',(#9214),#3240,.T.);
#69965=ADVANCED_FACE('',(#9215),#5235,.T.);
#69966=ADVANCED_FACE('',(#9216),#3241,.T.);
#69967=ADVANCED_FACE('',(#9217),#3242,.T.);
#69968=ADVANCED_FACE('',(#9218),#5236,.T.);
#69969=ADVANCED_FACE('',(#9219),#3243,.T.);
#69970=ADVANCED_FACE('',(#9220),#3244,.T.);
#69971=ADVANCED_FACE('',(#9221),#5237,.T.);
#69972=ADVANCED_FACE('',(#9222),#3245,.T.);
#69973=ADVANCED_FACE('',(#9223),#3246,.T.);
#69974=ADVANCED_FACE('',(#9224),#3247,.T.);
#69975=ADVANCED_FACE('',(#9225),#5238,.T.);
#69976=ADVANCED_FACE('',(#9226),#3248,.T.);
#69977=ADVANCED_FACE('',(#9227),#5239,.T.);
#69978=ADVANCED_FACE('',(#9228),#3249,.T.);
#69979=ADVANCED_FACE('',(#9229),#3250,.T.);
#69980=ADVANCED_FACE('',(#9230),#5240,.T.);
#69981=ADVANCED_FACE('',(#9231),#3251,.T.);
#69982=ADVANCED_FACE('',(#9232),#3252,.T.);
#69983=ADVANCED_FACE('',(#9233),#5241,.T.);
#69984=ADVANCED_FACE('',(#9234),#3253,.T.);
#69985=ADVANCED_FACE('',(#9235),#3254,.T.);
#69986=ADVANCED_FACE('',(#9236),#5242,.T.);
#69987=ADVANCED_FACE('',(#9237),#3255,.T.);
#69988=ADVANCED_FACE('',(#9238),#3256,.T.);
#69989=ADVANCED_FACE('',(#9239),#5243,.T.);
#69990=ADVANCED_FACE('',(#9240),#3257,.T.);
#69991=ADVANCED_FACE('',(#9241),#3258,.T.);
#69992=ADVANCED_FACE('',(#9242),#5244,.T.);
#69993=ADVANCED_FACE('',(#9243),#3259,.T.);
#69994=ADVANCED_FACE('',(#9244),#3260,.T.);
#69995=ADVANCED_FACE('',(#9245),#5245,.T.);
#69996=ADVANCED_FACE('',(#9246),#3261,.T.);
#69997=ADVANCED_FACE('',(#9247),#3262,.T.);
#69998=ADVANCED_FACE('',(#9248),#5246,.T.);
#69999=ADVANCED_FACE('',(#9249),#3263,.T.);
#70000=ADVANCED_FACE('',(#9250),#3264,.T.);
#70001=ADVANCED_FACE('',(#9251),#5247,.T.);
#70002=ADVANCED_FACE('',(#9252),#3265,.T.);
#70003=ADVANCED_FACE('',(#9253),#3266,.T.);
#70004=ADVANCED_FACE('',(#9254),#5248,.T.);
#70005=ADVANCED_FACE('',(#9255),#3267,.T.);
#70006=ADVANCED_FACE('',(#9256),#3268,.T.);
#70007=ADVANCED_FACE('',(#9257),#66013,.T.);
#70008=ADVANCED_FACE('',(#9258),#3269,.T.);
#70009=ADVANCED_FACE('',(#9259),#5249,.T.);
#70010=ADVANCED_FACE('',(#9260),#3270,.T.);
#70011=ADVANCED_FACE('',(#9261),#66014,.T.);
#70012=ADVANCED_FACE('',(#9262),#3271,.T.);
#70013=ADVANCED_FACE('',(#9263),#5250,.T.);
#70014=ADVANCED_FACE('',(#9264),#3272,.T.);
#70015=ADVANCED_FACE('',(#9265),#66015,.T.);
#70016=ADVANCED_FACE('',(#9266),#3273,.T.);
#70017=ADVANCED_FACE('',(#9267),#5251,.T.);
#70018=ADVANCED_FACE('',(#9268),#3274,.T.);
#70019=ADVANCED_FACE('',(#9269),#66016,.T.);
#70020=ADVANCED_FACE('',(#9270),#3275,.T.);
#70021=ADVANCED_FACE('',(#9271),#5252,.T.);
#70022=ADVANCED_FACE('',(#9272),#3276,.T.);
#70023=ADVANCED_FACE('',(#9273),#66017,.T.);
#70024=ADVANCED_FACE('',(#9274),#3277,.T.);
#70025=ADVANCED_FACE('',(#9275),#5253,.T.);
#70026=ADVANCED_FACE('',(#9276),#3278,.T.);
#70027=ADVANCED_FACE('',(#9277),#66018,.T.);
#70028=ADVANCED_FACE('',(#9278),#3279,.T.);
#70029=ADVANCED_FACE('',(#9279),#5254,.T.);
#70030=ADVANCED_FACE('',(#9280),#3280,.T.);
#70031=ADVANCED_FACE('',(#9281),#66019,.T.);
#70032=ADVANCED_FACE('',(#9282),#3281,.T.);
#70033=ADVANCED_FACE('',(#9283),#5255,.T.);
#70034=ADVANCED_FACE('',(#9284),#3282,.T.);
#70035=ADVANCED_FACE('',(#9285),#66020,.T.);
#70036=ADVANCED_FACE('',(#9286),#3283,.T.);
#70037=ADVANCED_FACE('',(#9287),#5256,.T.);
#70038=ADVANCED_FACE('',(#9288),#3284,.T.);
#70039=ADVANCED_FACE('',(#9289),#66021,.T.);
#70040=ADVANCED_FACE('',(#9290),#3285,.T.);
#70041=ADVANCED_FACE('',(#9291),#5257,.T.);
#70042=ADVANCED_FACE('',(#9292),#3286,.T.);
#70043=ADVANCED_FACE('',(#9293),#66022,.T.);
#70044=ADVANCED_FACE('',(#9294),#3287,.T.);
#70045=ADVANCED_FACE('',(#9295),#5258,.T.);
#70046=ADVANCED_FACE('',(#9296),#3288,.T.);
#70047=ADVANCED_FACE('',(#9297),#66023,.T.);
#70048=ADVANCED_FACE('',(#9298),#3289,.T.);
#70049=ADVANCED_FACE('',(#9299),#5259,.T.);
#70050=ADVANCED_FACE('',(#9300),#3290,.T.);
#70051=ADVANCED_FACE('',(#9301),#66024,.T.);
#70052=ADVANCED_FACE('',(#9302),#3291,.T.);
#70053=ADVANCED_FACE('',(#9303),#5260,.T.);
#70054=ADVANCED_FACE('',(#9304),#3292,.T.);
#70055=ADVANCED_FACE('',(#9305),#66025,.T.);
#70056=ADVANCED_FACE('',(#9306),#3293,.T.);
#70057=ADVANCED_FACE('',(#9307),#5261,.T.);
#70058=ADVANCED_FACE('',(#9308),#3294,.T.);
#70059=ADVANCED_FACE('',(#9309),#66026,.T.);
#70060=ADVANCED_FACE('',(#9310),#3295,.T.);
#70061=ADVANCED_FACE('',(#9311),#5262,.T.);
#70062=ADVANCED_FACE('',(#9312),#3296,.T.);
#70063=ADVANCED_FACE('',(#9313),#66027,.T.);
#70064=ADVANCED_FACE('',(#9314),#3297,.T.);
#70065=ADVANCED_FACE('',(#9315),#5263,.T.);
#70066=ADVANCED_FACE('',(#9316),#3298,.T.);
#70067=ADVANCED_FACE('',(#9317),#66028,.T.);
#70068=ADVANCED_FACE('',(#9318),#3299,.T.);
#70069=ADVANCED_FACE('',(#9319),#5264,.T.);
#70070=ADVANCED_FACE('',(#9320),#3300,.T.);
#70071=ADVANCED_FACE('',(#9321),#66029,.T.);
#70072=ADVANCED_FACE('',(#9322),#3301,.T.);
#70073=ADVANCED_FACE('',(#9323),#5265,.T.);
#70074=ADVANCED_FACE('',(#9324),#3302,.T.);
#70075=ADVANCED_FACE('',(#9325),#66030,.T.);
#70076=ADVANCED_FACE('',(#9326),#3303,.T.);
#70077=ADVANCED_FACE('',(#9327),#5266,.T.);
#70078=ADVANCED_FACE('',(#9328),#3304,.T.);
#70079=ADVANCED_FACE('',(#9329),#66031,.T.);
#70080=ADVANCED_FACE('',(#9330),#3305,.T.);
#70081=ADVANCED_FACE('',(#9331),#5267,.T.);
#70082=ADVANCED_FACE('',(#9332),#3306,.T.);
#70083=ADVANCED_FACE('',(#9333),#66032,.T.);
#70084=ADVANCED_FACE('',(#9334),#3307,.T.);
#70085=ADVANCED_FACE('',(#9335),#5268,.T.);
#70086=ADVANCED_FACE('',(#9336),#3308,.T.);
#70087=ADVANCED_FACE('',(#9337),#66033,.T.);
#70088=ADVANCED_FACE('',(#9338),#3309,.T.);
#70089=ADVANCED_FACE('',(#9339),#5269,.T.);
#70090=ADVANCED_FACE('',(#9340),#3310,.T.);
#70091=ADVANCED_FACE('',(#9341),#3311,.T.);
#70092=ADVANCED_FACE('',(#9342),#3312,.T.);
#70093=ADVANCED_FACE('',(#9343),#66034,.T.);
#70094=ADVANCED_FACE('',(#9344),#3313,.T.);
#70095=ADVANCED_FACE('',(#9345),#5270,.T.);
#70096=ADVANCED_FACE('',(#9346),#3314,.T.);
#70097=ADVANCED_FACE('',(#9347),#66035,.T.);
#70098=ADVANCED_FACE('',(#9348),#3315,.T.);
#70099=ADVANCED_FACE('',(#9349),#5271,.T.);
#70100=ADVANCED_FACE('',(#9350),#3316,.T.);
#70101=ADVANCED_FACE('',(#9351),#66036,.T.);
#70102=ADVANCED_FACE('',(#9352),#3317,.T.);
#70103=ADVANCED_FACE('',(#9353),#5272,.T.);
#70104=ADVANCED_FACE('',(#9354),#3318,.T.);
#70105=ADVANCED_FACE('',(#9355),#66037,.T.);
#70106=ADVANCED_FACE('',(#9356),#3319,.T.);
#70107=ADVANCED_FACE('',(#9357),#5273,.T.);
#70108=ADVANCED_FACE('',(#9358),#3320,.T.);
#70109=ADVANCED_FACE('',(#9359),#66038,.T.);
#70110=ADVANCED_FACE('',(#9360),#3321,.T.);
#70111=ADVANCED_FACE('',(#9361),#5274,.T.);
#70112=ADVANCED_FACE('',(#9362),#3322,.T.);
#70113=ADVANCED_FACE('',(#9363),#66039,.T.);
#70114=ADVANCED_FACE('',(#9364),#3323,.T.);
#70115=ADVANCED_FACE('',(#9365),#5275,.T.);
#70116=ADVANCED_FACE('',(#9366),#3324,.T.);
#70117=ADVANCED_FACE('',(#9367),#66040,.T.);
#70118=ADVANCED_FACE('',(#9368),#3325,.T.);
#70119=ADVANCED_FACE('',(#9369),#5276,.T.);
#70120=ADVANCED_FACE('',(#9370),#3326,.T.);
#70121=ADVANCED_FACE('',(#9371),#3327,.T.);
#70122=ADVANCED_FACE('',(#9372),#3328,.T.);
#70123=ADVANCED_FACE('',(#9373),#3329,.T.);
#70124=ADVANCED_FACE('',(#9374),#3330,.T.);
#70125=ADVANCED_FACE('',(#9375),#3331,.T.);
#70126=ADVANCED_FACE('',(#9376),#3332,.T.);
#70127=ADVANCED_FACE('',(#9377),#3333,.T.);
#70128=ADVANCED_FACE('',(#9378),#3334,.T.);
#70129=ADVANCED_FACE('',(#9379),#3335,.T.);
#70130=ADVANCED_FACE('',(#9380),#3336,.T.);
#70131=ADVANCED_FACE('',(#9381),#3337,.T.);
#70132=ADVANCED_FACE('',(#9382),#3338,.T.);
#70133=ADVANCED_FACE('',(#9383),#3339,.T.);
#70134=ADVANCED_FACE('',(#9384),#3340,.T.);
#70135=ADVANCED_FACE('',(#9385),#3341,.T.);
#70136=ADVANCED_FACE('',(#9386),#3342,.T.);
#70137=ADVANCED_FACE('',(#9387),#3343,.T.);
#70138=ADVANCED_FACE('',(#9388),#3344,.T.);
#70139=ADVANCED_FACE('',(#9389),#3345,.T.);
#70140=ADVANCED_FACE('',(#9390),#3346,.T.);
#70141=ADVANCED_FACE('',(#9391),#3347,.T.);
#70142=ADVANCED_FACE('',(#9392),#3348,.T.);
#70143=ADVANCED_FACE('',(#9393),#3349,.T.);
#70144=ADVANCED_FACE('',(#9394),#3350,.T.);
#70145=ADVANCED_FACE('',(#9395),#3351,.T.);
#70146=ADVANCED_FACE('',(#9396),#3352,.T.);
#70147=ADVANCED_FACE('',(#9397),#3353,.T.);
#70148=ADVANCED_FACE('',(#9398),#3354,.T.);
#70149=ADVANCED_FACE('',(#9399),#3355,.T.);
#70150=ADVANCED_FACE('',(#9400),#3356,.T.);
#70151=ADVANCED_FACE('',(#9401),#3357,.T.);
#70152=ADVANCED_FACE('',(#9402),#3358,.T.);
#70153=ADVANCED_FACE('',(#9403),#3359,.T.);
#70154=ADVANCED_FACE('',(#9404),#3360,.T.);
#70155=ADVANCED_FACE('',(#9405),#3361,.T.);
#70156=ADVANCED_FACE('',(#9406),#3362,.T.);
#70157=ADVANCED_FACE('',(#9407),#3363,.T.);
#70158=ADVANCED_FACE('',(#9408),#3364,.T.);
#70159=ADVANCED_FACE('',(#9409),#3365,.T.);
#70160=ADVANCED_FACE('',(#9410),#3366,.T.);
#70161=ADVANCED_FACE('',(#9411),#3367,.T.);
#70162=ADVANCED_FACE('',(#9412),#3368,.T.);
#70163=ADVANCED_FACE('',(#9413),#3369,.T.);
#70164=ADVANCED_FACE('',(#9414),#3370,.T.);
#70165=ADVANCED_FACE('',(#9415),#3371,.T.);
#70166=ADVANCED_FACE('',(#9416),#3372,.T.);
#70167=ADVANCED_FACE('',(#9417),#3373,.T.);
#70168=ADVANCED_FACE('',(#9418),#3374,.T.);
#70169=ADVANCED_FACE('',(#9419),#3375,.T.);
#70170=ADVANCED_FACE('',(#9420),#3376,.T.);
#70171=ADVANCED_FACE('',(#9421),#3377,.T.);
#70172=ADVANCED_FACE('',(#9422),#3378,.T.);
#70173=ADVANCED_FACE('',(#9423),#3379,.T.);
#70174=ADVANCED_FACE('',(#9424),#3380,.T.);
#70175=ADVANCED_FACE('',(#9425),#3381,.T.);
#70176=ADVANCED_FACE('',(#9426),#3382,.T.);
#70177=ADVANCED_FACE('',(#9427),#3383,.T.);
#70178=ADVANCED_FACE('',(#9428),#3384,.T.);
#70179=ADVANCED_FACE('',(#9429),#3385,.T.);
#70180=ADVANCED_FACE('',(#9430),#3386,.T.);
#70181=ADVANCED_FACE('',(#9431),#3387,.T.);
#70182=ADVANCED_FACE('',(#9432),#3388,.T.);
#70183=ADVANCED_FACE('',(#9433),#3389,.T.);
#70184=ADVANCED_FACE('',(#9434),#3390,.T.);
#70185=ADVANCED_FACE('',(#9435),#3391,.T.);
#70186=ADVANCED_FACE('',(#9436),#3392,.T.);
#70187=ADVANCED_FACE('',(#9437),#3393,.T.);
#70188=ADVANCED_FACE('',(#9438),#3394,.T.);
#70189=ADVANCED_FACE('',(#9439),#3395,.T.);
#70190=ADVANCED_FACE('',(#9440),#3396,.T.);
#70191=ADVANCED_FACE('',(#9441),#3397,.T.);
#70192=ADVANCED_FACE('',(#9442),#3398,.T.);
#70193=ADVANCED_FACE('',(#9443),#3399,.T.);
#70194=ADVANCED_FACE('',(#9444),#3400,.T.);
#70195=ADVANCED_FACE('',(#9445),#3401,.T.);
#70196=ADVANCED_FACE('',(#9446),#3402,.T.);
#70197=ADVANCED_FACE('',(#9447),#3403,.T.);
#70198=ADVANCED_FACE('',(#9448),#3404,.T.);
#70199=ADVANCED_FACE('',(#9449),#3405,.T.);
#70200=ADVANCED_FACE('',(#9450),#3406,.T.);
#70201=ADVANCED_FACE('',(#9451),#3407,.T.);
#70202=ADVANCED_FACE('',(#9452),#3408,.T.);
#70203=ADVANCED_FACE('',(#9453),#3409,.T.);
#70204=ADVANCED_FACE('',(#9454),#3410,.T.);
#70205=ADVANCED_FACE('',(#9455),#3411,.T.);
#70206=ADVANCED_FACE('',(#9456),#3412,.T.);
#70207=ADVANCED_FACE('',(#9457),#3413,.T.);
#70208=ADVANCED_FACE('',(#9458),#3414,.T.);
#70209=ADVANCED_FACE('',(#9459),#3415,.T.);
#70210=ADVANCED_FACE('',(#9460),#3416,.T.);
#70211=ADVANCED_FACE('',(#9461),#3417,.T.);
#70212=ADVANCED_FACE('',(#9462),#3418,.T.);
#70213=ADVANCED_FACE('',(#9463),#3419,.T.);
#70214=ADVANCED_FACE('',(#9464),#3420,.T.);
#70215=ADVANCED_FACE('',(#9465),#3421,.T.);
#70216=ADVANCED_FACE('',(#9466),#3422,.T.);
#70217=ADVANCED_FACE('',(#9467),#3423,.T.);
#70218=ADVANCED_FACE('',(#9468),#3424,.T.);
#70219=ADVANCED_FACE('',(#9469),#3425,.T.);
#70220=ADVANCED_FACE('',(#9470),#3426,.T.);
#70221=ADVANCED_FACE('',(#9471),#3427,.T.);
#70222=ADVANCED_FACE('',(#9472),#3428,.T.);
#70223=ADVANCED_FACE('',(#9473),#3429,.T.);
#70224=ADVANCED_FACE('',(#9474),#3430,.T.);
#70225=ADVANCED_FACE('',(#9475),#3431,.T.);
#70226=ADVANCED_FACE('',(#9476),#3432,.T.);
#70227=ADVANCED_FACE('',(#9477),#3433,.T.);
#70228=ADVANCED_FACE('',(#9478),#3434,.T.);
#70229=ADVANCED_FACE('',(#9479),#3435,.T.);
#70230=ADVANCED_FACE('',(#9480),#3436,.T.);
#70231=ADVANCED_FACE('',(#9481),#3437,.T.);
#70232=ADVANCED_FACE('',(#9482),#3438,.T.);
#70233=ADVANCED_FACE('',(#9483),#3439,.T.);
#70234=ADVANCED_FACE('',(#9484),#3440,.T.);
#70235=ADVANCED_FACE('',(#9485),#3441,.T.);
#70236=ADVANCED_FACE('',(#9486),#3442,.T.);
#70237=ADVANCED_FACE('',(#9487),#3443,.T.);
#70238=ADVANCED_FACE('',(#9488),#5277,.T.);
#70239=ADVANCED_FACE('',(#9489),#3444,.T.);
#70240=ADVANCED_FACE('',(#9490),#3445,.T.);
#70241=ADVANCED_FACE('',(#9491),#5278,.T.);
#70242=ADVANCED_FACE('',(#9492),#3446,.T.);
#70243=ADVANCED_FACE('',(#9493),#3447,.T.);
#70244=ADVANCED_FACE('',(#9494),#5279,.T.);
#70245=ADVANCED_FACE('',(#9495),#3448,.T.);
#70246=ADVANCED_FACE('',(#9496),#3449,.T.);
#70247=ADVANCED_FACE('',(#9497),#5280,.T.);
#70248=ADVANCED_FACE('',(#9498),#3450,.T.);
#70249=ADVANCED_FACE('',(#9499),#3451,.T.);
#70250=ADVANCED_FACE('',(#9500),#5281,.T.);
#70251=ADVANCED_FACE('',(#9501),#3452,.T.);
#70252=ADVANCED_FACE('',(#9502),#3453,.T.);
#70253=ADVANCED_FACE('',(#9503),#5282,.T.);
#70254=ADVANCED_FACE('',(#9504),#3454,.T.);
#70255=ADVANCED_FACE('',(#9505),#3455,.T.);
#70256=ADVANCED_FACE('',(#9506),#3456,.T.);
#70257=ADVANCED_FACE('',(#9507),#3457,.T.);
#70258=ADVANCED_FACE('',(#9508),#5283,.T.);
#70259=ADVANCED_FACE('',(#9509),#3458,.T.);
#70260=ADVANCED_FACE('',(#9510),#3459,.T.);
#70261=ADVANCED_FACE('',(#9511),#5284,.T.);
#70262=ADVANCED_FACE('',(#9512),#3460,.T.);
#70263=ADVANCED_FACE('',(#9513),#3461,.T.);
#70264=ADVANCED_FACE('',(#9514),#5285,.T.);
#70265=ADVANCED_FACE('',(#9515),#3462,.T.);
#70266=ADVANCED_FACE('',(#9516),#3463,.T.);
#70267=ADVANCED_FACE('',(#9517),#5286,.T.);
#70268=ADVANCED_FACE('',(#9518),#3464,.T.);
#70269=ADVANCED_FACE('',(#9519),#3465,.T.);
#70270=ADVANCED_FACE('',(#9520),#5287,.T.);
#70271=ADVANCED_FACE('',(#9521),#3466,.T.);
#70272=ADVANCED_FACE('',(#9522),#3467,.T.);
#70273=ADVANCED_FACE('',(#9523),#5288,.T.);
#70274=ADVANCED_FACE('',(#9524),#3468,.T.);
#70275=ADVANCED_FACE('',(#9525),#3469,.T.);
#70276=ADVANCED_FACE('',(#9526),#5289,.T.);
#70277=ADVANCED_FACE('',(#9527),#3470,.T.);
#70278=ADVANCED_FACE('',(#9528),#3471,.T.);
#70279=ADVANCED_FACE('',(#9529),#5290,.T.);
#70280=ADVANCED_FACE('',(#9530),#3472,.T.);
#70281=ADVANCED_FACE('',(#9531),#3473,.T.);
#70282=ADVANCED_FACE('',(#9532),#5291,.T.);
#70283=ADVANCED_FACE('',(#9533),#3474,.T.);
#70284=ADVANCED_FACE('',(#9534),#3475,.T.);
#70285=ADVANCED_FACE('',(#9535),#5292,.T.);
#70286=ADVANCED_FACE('',(#9536),#3476,.T.);
#70287=ADVANCED_FACE('',(#9537),#3477,.T.);
#70288=ADVANCED_FACE('',(#9538),#3478,.T.);
#70289=ADVANCED_FACE('',(#9539),#5293,.T.);
#70290=ADVANCED_FACE('',(#9540),#3479,.T.);
#70291=ADVANCED_FACE('',(#9541),#5294,.T.);
#70292=ADVANCED_FACE('',(#9542),#3480,.T.);
#70293=ADVANCED_FACE('',(#9543),#3481,.T.);
#70294=ADVANCED_FACE('',(#9544),#5295,.T.);
#70295=ADVANCED_FACE('',(#9545),#3482,.T.);
#70296=ADVANCED_FACE('',(#9546),#3483,.T.);
#70297=ADVANCED_FACE('',(#9547),#5296,.T.);
#70298=ADVANCED_FACE('',(#9548),#3484,.T.);
#70299=ADVANCED_FACE('',(#9549),#3485,.T.);
#70300=ADVANCED_FACE('',(#9550),#5297,.T.);
#70301=ADVANCED_FACE('',(#9551),#3486,.T.);
#70302=ADVANCED_FACE('',(#9552),#3487,.T.);
#70303=ADVANCED_FACE('',(#9553),#5298,.T.);
#70304=ADVANCED_FACE('',(#9554),#3488,.T.);
#70305=ADVANCED_FACE('',(#9555),#3489,.T.);
#70306=ADVANCED_FACE('',(#9556),#5299,.T.);
#70307=ADVANCED_FACE('',(#9557),#3490,.T.);
#70308=ADVANCED_FACE('',(#9558),#3491,.T.);
#70309=ADVANCED_FACE('',(#9559),#5300,.T.);
#70310=ADVANCED_FACE('',(#9560),#3492,.T.);
#70311=ADVANCED_FACE('',(#9561),#3493,.T.);
#70312=ADVANCED_FACE('',(#9562),#5301,.T.);
#70313=ADVANCED_FACE('',(#9563),#3494,.T.);
#70314=ADVANCED_FACE('',(#9564),#3495,.T.);
#70315=ADVANCED_FACE('',(#9565),#5302,.T.);
#70316=ADVANCED_FACE('',(#9566),#3496,.T.);
#70317=ADVANCED_FACE('',(#9567),#3497,.T.);
#70318=ADVANCED_FACE('',(#9568),#5303,.T.);
#70319=ADVANCED_FACE('',(#9569),#3498,.T.);
#70320=ADVANCED_FACE('',(#9570),#5304,.T.);
#70321=ADVANCED_FACE('',(#9571),#3499,.T.);
#70322=ADVANCED_FACE('',(#9572),#3500,.T.);
#70323=ADVANCED_FACE('',(#9573),#3501,.T.);
#70324=ADVANCED_FACE('',(#9574),#66041,.T.);
#70325=ADVANCED_FACE('',(#9575),#3502,.T.);
#70326=ADVANCED_FACE('',(#9576),#3503,.T.);
#70327=ADVANCED_FACE('',(#9577),#66042,.T.);
#70328=ADVANCED_FACE('',(#9578),#3504,.T.);
#70329=ADVANCED_FACE('',(#9579),#3505,.T.);
#70330=ADVANCED_FACE('',(#9580),#66043,.T.);
#70331=ADVANCED_FACE('',(#9581),#3506,.T.);
#70332=ADVANCED_FACE('',(#9582),#3507,.T.);
#70333=ADVANCED_FACE('',(#9583),#66044,.T.);
#70334=ADVANCED_FACE('',(#9584),#3508,.T.);
#70335=ADVANCED_FACE('',(#9585),#3509,.T.);
#70336=ADVANCED_FACE('',(#9586),#66045,.T.);
#70337=ADVANCED_FACE('',(#9587),#3510,.T.);
#70338=ADVANCED_FACE('',(#9588),#3511,.T.);
#70339=ADVANCED_FACE('',(#9589),#66046,.T.);
#70340=ADVANCED_FACE('',(#9590),#3512,.T.);
#70341=ADVANCED_FACE('',(#9591),#3513,.T.);
#70342=ADVANCED_FACE('',(#9592),#66047,.T.);
#70343=ADVANCED_FACE('',(#9593),#3514,.T.);
#70344=ADVANCED_FACE('',(#9594),#3515,.T.);
#70345=ADVANCED_FACE('',(#9595),#66048,.T.);
#70346=ADVANCED_FACE('',(#9596),#3516,.T.);
#70347=ADVANCED_FACE('',(#9597),#3517,.T.);
#70348=ADVANCED_FACE('',(#9598),#66049,.T.);
#70349=ADVANCED_FACE('',(#9599),#3518,.T.);
#70350=ADVANCED_FACE('',(#9600),#3519,.T.);
#70351=ADVANCED_FACE('',(#9601),#66050,.T.);
#70352=ADVANCED_FACE('',(#9602),#3520,.T.);
#70353=ADVANCED_FACE('',(#9603),#3521,.T.);
#70354=ADVANCED_FACE('',(#9604),#66051,.T.);
#70355=ADVANCED_FACE('',(#9605),#3522,.T.);
#70356=ADVANCED_FACE('',(#9606),#3523,.T.);
#70357=ADVANCED_FACE('',(#9607),#66052,.T.);
#70358=ADVANCED_FACE('',(#9608),#3524,.T.);
#70359=ADVANCED_FACE('',(#9609),#3525,.T.);
#70360=ADVANCED_FACE('',(#9610),#66053,.T.);
#70361=ADVANCED_FACE('',(#9611),#3526,.T.);
#70362=ADVANCED_FACE('',(#9612),#3527,.T.);
#70363=ADVANCED_FACE('',(#9613),#3528,.T.);
#70364=ADVANCED_FACE('',(#9614),#3529,.T.);
#70365=ADVANCED_FACE('',(#9615),#66054,.T.);
#70366=ADVANCED_FACE('',(#9616),#3530,.T.);
#70367=ADVANCED_FACE('',(#9617),#3531,.T.);
#70368=ADVANCED_FACE('',(#9618),#66055,.T.);
#70369=ADVANCED_FACE('',(#9619),#3532,.T.);
#70370=ADVANCED_FACE('',(#9620),#3533,.T.);
#70371=ADVANCED_FACE('',(#9621),#66056,.T.);
#70372=ADVANCED_FACE('',(#9622),#3534,.T.);
#70373=ADVANCED_FACE('',(#9623),#3535,.T.);
#70374=ADVANCED_FACE('',(#9624),#66057,.T.);
#70375=ADVANCED_FACE('',(#9625),#3536,.T.);
#70376=ADVANCED_FACE('',(#9626),#3537,.T.);
#70377=ADVANCED_FACE('',(#9627),#66058,.T.);
#70378=ADVANCED_FACE('',(#9628),#3538,.T.);
#70379=ADVANCED_FACE('',(#9629),#3539,.T.);
#70380=ADVANCED_FACE('',(#9630),#66059,.T.);
#70381=ADVANCED_FACE('',(#9631),#3540,.T.);
#70382=ADVANCED_FACE('',(#9632),#3541,.T.);
#70383=ADVANCED_FACE('',(#9633),#3542,.T.);
#70384=ADVANCED_FACE('',(#9634),#3543,.T.);
#70385=ADVANCED_FACE('',(#9635),#66060,.T.);
#70386=ADVANCED_FACE('',(#9636),#3544,.T.);
#70387=ADVANCED_FACE('',(#9637),#3545,.T.);
#70388=ADVANCED_FACE('',(#9638),#66061,.T.);
#70389=ADVANCED_FACE('',(#9639),#3546,.T.);
#70390=ADVANCED_FACE('',(#9640),#3547,.T.);
#70391=ADVANCED_FACE('',(#9641),#66062,.T.);
#70392=ADVANCED_FACE('',(#9642),#3548,.T.);
#70393=ADVANCED_FACE('',(#9643),#3549,.T.);
#70394=ADVANCED_FACE('',(#9644),#66063,.T.);
#70395=ADVANCED_FACE('',(#9645),#3550,.T.);
#70396=ADVANCED_FACE('',(#9646),#3551,.T.);
#70397=ADVANCED_FACE('',(#9647),#66064,.T.);
#70398=ADVANCED_FACE('',(#9648),#3552,.T.);
#70399=ADVANCED_FACE('',(#9649),#3553,.T.);
#70400=ADVANCED_FACE('',(#9650),#66065,.T.);
#70401=ADVANCED_FACE('',(#9651),#3554,.T.);
#70402=ADVANCED_FACE('',(#9652),#3555,.T.);
#70403=ADVANCED_FACE('',(#9653),#66066,.T.);
#70404=ADVANCED_FACE('',(#9654),#3556,.T.);
#70405=ADVANCED_FACE('',(#9655),#66067,.T.);
#70406=ADVANCED_FACE('',(#9656),#3557,.T.);
#70407=ADVANCED_FACE('',(#9657),#3558,.T.);
#70408=ADVANCED_FACE('',(#9658),#3559,.T.);
#70409=ADVANCED_FACE('',(#9659),#3560,.T.);
#70410=ADVANCED_FACE('',(#9660),#3561,.T.);
#70411=ADVANCED_FACE('',(#9661),#3562,.T.);
#70412=ADVANCED_FACE('',(#9662),#3563,.T.);
#70413=ADVANCED_FACE('',(#9663),#3564,.T.);
#70414=ADVANCED_FACE('',(#9664),#3565,.T.);
#70415=ADVANCED_FACE('',(#9665),#3566,.T.);
#70416=ADVANCED_FACE('',(#9666),#3567,.T.);
#70417=ADVANCED_FACE('',(#9667),#3568,.T.);
#70418=ADVANCED_FACE('',(#9668),#3569,.T.);
#70419=ADVANCED_FACE('',(#9669),#3570,.T.);
#70420=ADVANCED_FACE('',(#9670),#3571,.T.);
#70421=ADVANCED_FACE('',(#9671),#3572,.T.);
#70422=ADVANCED_FACE('',(#9672),#3573,.T.);
#70423=ADVANCED_FACE('',(#9673),#3574,.T.);
#70424=ADVANCED_FACE('',(#9674),#3575,.T.);
#70425=ADVANCED_FACE('',(#9675),#3576,.T.);
#70426=ADVANCED_FACE('',(#9676),#3577,.T.);
#70427=ADVANCED_FACE('',(#9677),#3578,.T.);
#70428=ADVANCED_FACE('',(#9678),#3579,.T.);
#70429=ADVANCED_FACE('',(#9679),#3580,.T.);
#70430=ADVANCED_FACE('',(#9680),#3581,.T.);
#70431=ADVANCED_FACE('',(#9681),#3582,.T.);
#70432=ADVANCED_FACE('',(#9682),#3583,.T.);
#70433=ADVANCED_FACE('',(#9683),#3584,.T.);
#70434=ADVANCED_FACE('',(#9684),#3585,.T.);
#70435=ADVANCED_FACE('',(#9685),#3586,.T.);
#70436=ADVANCED_FACE('',(#9686),#3587,.T.);
#70437=ADVANCED_FACE('',(#9687),#3588,.T.);
#70438=ADVANCED_FACE('',(#9688),#3589,.T.);
#70439=ADVANCED_FACE('',(#9689),#3590,.T.);
#70440=ADVANCED_FACE('',(#9690),#3591,.T.);
#70441=ADVANCED_FACE('',(#9691),#3592,.T.);
#70442=ADVANCED_FACE('',(#9692),#3593,.T.);
#70443=ADVANCED_FACE('',(#9693),#3594,.T.);
#70444=ADVANCED_FACE('',(#9694),#3595,.T.);
#70445=ADVANCED_FACE('',(#9695),#3596,.T.);
#70446=ADVANCED_FACE('',(#9696),#3597,.T.);
#70447=ADVANCED_FACE('',(#9697),#3598,.T.);
#70448=ADVANCED_FACE('',(#9698),#3599,.T.);
#70449=ADVANCED_FACE('',(#9699),#3600,.T.);
#70450=ADVANCED_FACE('',(#9700),#3601,.T.);
#70451=ADVANCED_FACE('',(#9701),#3602,.T.);
#70452=ADVANCED_FACE('',(#9702),#3603,.T.);
#70453=ADVANCED_FACE('',(#9703),#3604,.T.);
#70454=ADVANCED_FACE('',(#9704),#3605,.T.);
#70455=ADVANCED_FACE('',(#9705),#3606,.T.);
#70456=ADVANCED_FACE('',(#9706),#3607,.T.);
#70457=ADVANCED_FACE('',(#9707),#3608,.T.);
#70458=ADVANCED_FACE('',(#9708),#3609,.T.);
#70459=ADVANCED_FACE('',(#9709),#3610,.T.);
#70460=ADVANCED_FACE('',(#9710),#3611,.T.);
#70461=ADVANCED_FACE('',(#9711),#3612,.T.);
#70462=ADVANCED_FACE('',(#9712),#3613,.T.);
#70463=ADVANCED_FACE('',(#9713),#3614,.T.);
#70464=ADVANCED_FACE('',(#9714),#3615,.T.);
#70465=ADVANCED_FACE('',(#9715),#3616,.T.);
#70466=ADVANCED_FACE('',(#9716),#3617,.T.);
#70467=ADVANCED_FACE('',(#9717),#3618,.T.);
#70468=ADVANCED_FACE('',(#9718),#3619,.T.);
#70469=ADVANCED_FACE('',(#9719),#3620,.T.);
#70470=ADVANCED_FACE('',(#9720),#3621,.T.);
#70471=ADVANCED_FACE('',(#9721),#3622,.T.);
#70472=ADVANCED_FACE('',(#9722),#3623,.T.);
#70473=ADVANCED_FACE('',(#9723),#3624,.T.);
#70474=ADVANCED_FACE('',(#9724),#3625,.T.);
#70475=ADVANCED_FACE('',(#9725),#3626,.T.);
#70476=ADVANCED_FACE('',(#9726),#3627,.T.);
#70477=ADVANCED_FACE('',(#9727),#3628,.T.);
#70478=ADVANCED_FACE('',(#9728),#3629,.T.);
#70479=ADVANCED_FACE('',(#9729),#3630,.T.);
#70480=ADVANCED_FACE('',(#9730),#3631,.T.);
#70481=ADVANCED_FACE('',(#9731),#3632,.T.);
#70482=ADVANCED_FACE('',(#9732),#3633,.T.);
#70483=ADVANCED_FACE('',(#9733),#3634,.T.);
#70484=ADVANCED_FACE('',(#9734),#3635,.T.);
#70485=ADVANCED_FACE('',(#9735),#3636,.T.);
#70486=ADVANCED_FACE('',(#9736),#3637,.T.);
#70487=ADVANCED_FACE('',(#9737),#3638,.T.);
#70488=ADVANCED_FACE('',(#9738),#3639,.T.);
#70489=ADVANCED_FACE('',(#9739),#3640,.T.);
#70490=ADVANCED_FACE('',(#9740),#3641,.T.);
#70491=ADVANCED_FACE('',(#9741),#3642,.T.);
#70492=ADVANCED_FACE('',(#9742),#3643,.T.);
#70493=ADVANCED_FACE('',(#9743),#3644,.T.);
#70494=ADVANCED_FACE('',(#9744),#3645,.T.);
#70495=ADVANCED_FACE('',(#9745),#3646,.T.);
#70496=ADVANCED_FACE('',(#9746),#3647,.T.);
#70497=ADVANCED_FACE('',(#9747),#3648,.T.);
#70498=ADVANCED_FACE('',(#9748),#3649,.T.);
#70499=ADVANCED_FACE('',(#9749),#3650,.T.);
#70500=ADVANCED_FACE('',(#9750),#3651,.T.);
#70501=ADVANCED_FACE('',(#9751),#3652,.T.);
#70502=ADVANCED_FACE('',(#9752),#3653,.T.);
#70503=ADVANCED_FACE('',(#9753),#3654,.T.);
#70504=ADVANCED_FACE('',(#9754),#3655,.T.);
#70505=ADVANCED_FACE('',(#9755),#3656,.T.);
#70506=ADVANCED_FACE('',(#9756),#3657,.T.);
#70507=ADVANCED_FACE('',(#9757),#3658,.T.);
#70508=ADVANCED_FACE('',(#9758),#3659,.T.);
#70509=ADVANCED_FACE('',(#9759),#3660,.T.);
#70510=ADVANCED_FACE('',(#9760),#3661,.T.);
#70511=ADVANCED_FACE('',(#9761),#3662,.T.);
#70512=ADVANCED_FACE('',(#9762),#3663,.T.);
#70513=ADVANCED_FACE('',(#9763),#3664,.T.);
#70514=ADVANCED_FACE('',(#9764),#3665,.T.);
#70515=ADVANCED_FACE('',(#9765),#3666,.T.);
#70516=ADVANCED_FACE('',(#9766),#3667,.T.);
#70517=ADVANCED_FACE('',(#9767),#3668,.T.);
#70518=ADVANCED_FACE('',(#9768),#3669,.T.);
#70519=ADVANCED_FACE('',(#9769),#3670,.T.);
#70520=ADVANCED_FACE('',(#9770),#3671,.T.);
#70521=ADVANCED_FACE('',(#9771),#3672,.T.);
#70522=ADVANCED_FACE('',(#9772),#3673,.T.);
#70523=ADVANCED_FACE('',(#9773),#3674,.T.);
#70524=ADVANCED_FACE('',(#9774),#5305,.T.);
#70525=ADVANCED_FACE('',(#9775),#3675,.T.);
#70526=ADVANCED_FACE('',(#9776),#3676,.T.);
#70527=ADVANCED_FACE('',(#9777),#5306,.T.);
#70528=ADVANCED_FACE('',(#9778),#3677,.T.);
#70529=ADVANCED_FACE('',(#9779),#3678,.T.);
#70530=ADVANCED_FACE('',(#9780),#5307,.T.);
#70531=ADVANCED_FACE('',(#9781),#3679,.T.);
#70532=ADVANCED_FACE('',(#9782),#3680,.T.);
#70533=ADVANCED_FACE('',(#9783),#5308,.T.);
#70534=ADVANCED_FACE('',(#9784),#3681,.T.);
#70535=ADVANCED_FACE('',(#9785),#3682,.T.);
#70536=ADVANCED_FACE('',(#9786),#5309,.T.);
#70537=ADVANCED_FACE('',(#9787),#3683,.T.);
#70538=ADVANCED_FACE('',(#9788),#3684,.T.);
#70539=ADVANCED_FACE('',(#9789),#5310,.T.);
#70540=ADVANCED_FACE('',(#9790),#3685,.T.);
#70541=ADVANCED_FACE('',(#9791),#3686,.T.);
#70542=ADVANCED_FACE('',(#9792),#5311,.T.);
#70543=ADVANCED_FACE('',(#9793),#3687,.T.);
#70544=ADVANCED_FACE('',(#9794),#3688,.T.);
#70545=ADVANCED_FACE('',(#9795),#5312,.T.);
#70546=ADVANCED_FACE('',(#9796),#3689,.T.);
#70547=ADVANCED_FACE('',(#9797),#3690,.T.);
#70548=ADVANCED_FACE('',(#9798),#5313,.T.);
#70549=ADVANCED_FACE('',(#9799),#3691,.T.);
#70550=ADVANCED_FACE('',(#9800),#3692,.T.);
#70551=ADVANCED_FACE('',(#9801),#5314,.T.);
#70552=ADVANCED_FACE('',(#9802),#3693,.T.);
#70553=ADVANCED_FACE('',(#9803),#3694,.T.);
#70554=ADVANCED_FACE('',(#9804),#5315,.T.);
#70555=ADVANCED_FACE('',(#9805),#3695,.T.);
#70556=ADVANCED_FACE('',(#9806),#3696,.T.);
#70557=ADVANCED_FACE('',(#9807),#5316,.T.);
#70558=ADVANCED_FACE('',(#9808),#3697,.T.);
#70559=ADVANCED_FACE('',(#9809),#3698,.T.);
#70560=ADVANCED_FACE('',(#9810),#5317,.T.);
#70561=ADVANCED_FACE('',(#9811),#3699,.T.);
#70562=ADVANCED_FACE('',(#9812),#3700,.T.);
#70563=ADVANCED_FACE('',(#9813),#5318,.T.);
#70564=ADVANCED_FACE('',(#9814),#3701,.T.);
#70565=ADVANCED_FACE('',(#9815),#3702,.T.);
#70566=ADVANCED_FACE('',(#9816),#3703,.T.);
#70567=ADVANCED_FACE('',(#9817),#3704,.T.);
#70568=ADVANCED_FACE('',(#9818),#5319,.T.);
#70569=ADVANCED_FACE('',(#9819),#3705,.T.);
#70570=ADVANCED_FACE('',(#9820),#3706,.T.);
#70571=ADVANCED_FACE('',(#9821),#5320,.T.);
#70572=ADVANCED_FACE('',(#9822),#3707,.T.);
#70573=ADVANCED_FACE('',(#9823),#3708,.T.);
#70574=ADVANCED_FACE('',(#9824),#3709,.T.);
#70575=ADVANCED_FACE('',(#9825),#5321,.T.);
#70576=ADVANCED_FACE('',(#9826),#3710,.T.);
#70577=ADVANCED_FACE('',(#9827),#5322,.T.);
#70578=ADVANCED_FACE('',(#9828),#3711,.T.);
#70579=ADVANCED_FACE('',(#9829),#3712,.T.);
#70580=ADVANCED_FACE('',(#9830),#5323,.T.);
#70581=ADVANCED_FACE('',(#9831),#3713,.T.);
#70582=ADVANCED_FACE('',(#9832),#3714,.T.);
#70583=ADVANCED_FACE('',(#9833),#5324,.T.);
#70584=ADVANCED_FACE('',(#9834),#3715,.T.);
#70585=ADVANCED_FACE('',(#9835),#3716,.T.);
#70586=ADVANCED_FACE('',(#9836),#5325,.T.);
#70587=ADVANCED_FACE('',(#9837),#3717,.T.);
#70588=ADVANCED_FACE('',(#9838),#3718,.T.);
#70589=ADVANCED_FACE('',(#9839),#5326,.T.);
#70590=ADVANCED_FACE('',(#9840),#3719,.T.);
#70591=ADVANCED_FACE('',(#9841),#3720,.T.);
#70592=ADVANCED_FACE('',(#9842),#5327,.T.);
#70593=ADVANCED_FACE('',(#9843),#3721,.T.);
#70594=ADVANCED_FACE('',(#9844),#3722,.T.);
#70595=ADVANCED_FACE('',(#9845),#5328,.T.);
#70596=ADVANCED_FACE('',(#9846),#3723,.T.);
#70597=ADVANCED_FACE('',(#9847),#3724,.T.);
#70598=ADVANCED_FACE('',(#9848),#5329,.T.);
#70599=ADVANCED_FACE('',(#9849),#3725,.T.);
#70600=ADVANCED_FACE('',(#9850),#3726,.T.);
#70601=ADVANCED_FACE('',(#9851),#5330,.T.);
#70602=ADVANCED_FACE('',(#9852),#3727,.T.);
#70603=ADVANCED_FACE('',(#9853),#3728,.T.);
#70604=ADVANCED_FACE('',(#9854),#5331,.T.);
#70605=ADVANCED_FACE('',(#9855),#3729,.T.);
#70606=ADVANCED_FACE('',(#9856),#3730,.T.);
#70607=ADVANCED_FACE('',(#9857),#5332,.T.);
#70608=ADVANCED_FACE('',(#9858),#3731,.T.);
#70609=ADVANCED_FACE('',(#9859),#3732,.T.);
#70610=ADVANCED_FACE('',(#9860),#3733,.T.);
#70611=ADVANCED_FACE('',(#9861),#3734,.T.);
#70612=ADVANCED_FACE('',(#9862),#3735,.T.);
#70613=ADVANCED_FACE('',(#9863),#3736,.T.);
#70614=ADVANCED_FACE('',(#9864),#3737,.T.);
#70615=ADVANCED_FACE('',(#9865),#3738,.T.);
#70616=ADVANCED_FACE('',(#9866),#3739,.T.);
#70617=ADVANCED_FACE('',(#9867),#3740,.T.);
#70618=ADVANCED_FACE('',(#9868),#3741,.T.);
#70619=ADVANCED_FACE('',(#9869),#3742,.T.);
#70620=ADVANCED_FACE('',(#9870),#3743,.T.);
#70621=ADVANCED_FACE('',(#9871),#3744,.T.);
#70622=ADVANCED_FACE('',(#9872),#3745,.T.);
#70623=ADVANCED_FACE('',(#9873),#3746,.T.);
#70624=ADVANCED_FACE('',(#9874),#3747,.T.);
#70625=ADVANCED_FACE('',(#9875),#3748,.T.);
#70626=ADVANCED_FACE('',(#9876),#3749,.T.);
#70627=ADVANCED_FACE('',(#9877),#3750,.T.);
#70628=ADVANCED_FACE('',(#9878),#3751,.T.);
#70629=ADVANCED_FACE('',(#9879),#3752,.T.);
#70630=ADVANCED_FACE('',(#9880),#3753,.T.);
#70631=ADVANCED_FACE('',(#9881),#3754,.T.);
#70632=ADVANCED_FACE('',(#9882),#3755,.T.);
#70633=ADVANCED_FACE('',(#9883),#3756,.T.);
#70634=ADVANCED_FACE('',(#9884),#3757,.T.);
#70635=ADVANCED_FACE('',(#9885),#3758,.T.);
#70636=ADVANCED_FACE('',(#9886),#3759,.T.);
#70637=ADVANCED_FACE('',(#9887),#3760,.T.);
#70638=ADVANCED_FACE('',(#9888),#3761,.T.);
#70639=ADVANCED_FACE('',(#9889),#3762,.T.);
#70640=ADVANCED_FACE('',(#9890),#3763,.T.);
#70641=ADVANCED_FACE('',(#9891),#3764,.T.);
#70642=ADVANCED_FACE('',(#9892),#3765,.T.);
#70643=ADVANCED_FACE('',(#9893),#3766,.T.);
#70644=ADVANCED_FACE('',(#9894),#3767,.T.);
#70645=ADVANCED_FACE('',(#9895),#3768,.T.);
#70646=ADVANCED_FACE('',(#9896),#3769,.T.);
#70647=ADVANCED_FACE('',(#9897),#3770,.T.);
#70648=ADVANCED_FACE('',(#9898),#3771,.T.);
#70649=ADVANCED_FACE('',(#9899),#3772,.T.);
#70650=ADVANCED_FACE('',(#9900),#3773,.T.);
#70651=ADVANCED_FACE('',(#9901),#3774,.T.);
#70652=ADVANCED_FACE('',(#9902),#3775,.T.);
#70653=ADVANCED_FACE('',(#9903),#3776,.T.);
#70654=ADVANCED_FACE('',(#9904),#3777,.T.);
#70655=ADVANCED_FACE('',(#9905),#3778,.T.);
#70656=ADVANCED_FACE('',(#9906),#3779,.T.);
#70657=ADVANCED_FACE('',(#9907),#3780,.T.);
#70658=ADVANCED_FACE('',(#9908),#3781,.T.);
#70659=ADVANCED_FACE('',(#9909),#3782,.T.);
#70660=ADVANCED_FACE('',(#9910),#3783,.T.);
#70661=ADVANCED_FACE('',(#9911),#3784,.T.);
#70662=ADVANCED_FACE('',(#9912),#3785,.T.);
#70663=ADVANCED_FACE('',(#9913),#3786,.T.);
#70664=ADVANCED_FACE('',(#9914),#3787,.T.);
#70665=ADVANCED_FACE('',(#9915),#3788,.T.);
#70666=ADVANCED_FACE('',(#9916),#3789,.T.);
#70667=ADVANCED_FACE('',(#9917),#3790,.T.);
#70668=ADVANCED_FACE('',(#9918),#3791,.T.);
#70669=ADVANCED_FACE('',(#9919),#3792,.T.);
#70670=ADVANCED_FACE('',(#9920),#3793,.T.);
#70671=ADVANCED_FACE('',(#9921),#3794,.T.);
#70672=ADVANCED_FACE('',(#9922),#3795,.T.);
#70673=ADVANCED_FACE('',(#9923),#3796,.T.);
#70674=ADVANCED_FACE('',(#9924),#3797,.T.);
#70675=ADVANCED_FACE('',(#9925),#3798,.T.);
#70676=ADVANCED_FACE('',(#9926),#3799,.T.);
#70677=ADVANCED_FACE('',(#9927),#3800,.T.);
#70678=ADVANCED_FACE('',(#9928),#3801,.T.);
#70679=ADVANCED_FACE('',(#9929),#3802,.T.);
#70680=ADVANCED_FACE('',(#9930),#3803,.T.);
#70681=ADVANCED_FACE('',(#9931),#3804,.T.);
#70682=ADVANCED_FACE('',(#9932),#3805,.T.);
#70683=ADVANCED_FACE('',(#9933),#3806,.T.);
#70684=ADVANCED_FACE('',(#9934),#3807,.T.);
#70685=ADVANCED_FACE('',(#9935),#3808,.T.);
#70686=ADVANCED_FACE('',(#9936),#3809,.T.);
#70687=ADVANCED_FACE('',(#9937),#3810,.T.);
#70688=ADVANCED_FACE('',(#9938),#3811,.T.);
#70689=ADVANCED_FACE('',(#9939),#3812,.T.);
#70690=ADVANCED_FACE('',(#9940),#3813,.T.);
#70691=ADVANCED_FACE('',(#9941),#3814,.T.);
#70692=ADVANCED_FACE('',(#9942),#3815,.T.);
#70693=ADVANCED_FACE('',(#9943),#3816,.T.);
#70694=ADVANCED_FACE('',(#9944),#3817,.T.);
#70695=ADVANCED_FACE('',(#9945),#3818,.T.);
#70696=ADVANCED_FACE('',(#9946),#3819,.T.);
#70697=ADVANCED_FACE('',(#9947),#3820,.T.);
#70698=ADVANCED_FACE('',(#9948),#3821,.T.);
#70699=ADVANCED_FACE('',(#9949),#3822,.T.);
#70700=ADVANCED_FACE('',(#9950),#3823,.T.);
#70701=ADVANCED_FACE('',(#9951),#3824,.T.);
#70702=ADVANCED_FACE('',(#9952),#3825,.T.);
#70703=ADVANCED_FACE('',(#9953),#3826,.T.);
#70704=ADVANCED_FACE('',(#9954),#3827,.T.);
#70705=ADVANCED_FACE('',(#9955),#3828,.T.);
#70706=ADVANCED_FACE('',(#9956),#3829,.T.);
#70707=ADVANCED_FACE('',(#9957),#3830,.T.);
#70708=ADVANCED_FACE('',(#9958),#3831,.T.);
#70709=ADVANCED_FACE('',(#9959),#3832,.T.);
#70710=ADVANCED_FACE('',(#9960),#3833,.T.);
#70711=ADVANCED_FACE('',(#9961),#3834,.T.);
#70712=ADVANCED_FACE('',(#9962),#3835,.T.);
#70713=ADVANCED_FACE('',(#9963),#3836,.T.);
#70714=ADVANCED_FACE('',(#9964),#3837,.T.);
#70715=ADVANCED_FACE('',(#9965),#3838,.T.);
#70716=ADVANCED_FACE('',(#9966),#3839,.T.);
#70717=ADVANCED_FACE('',(#9967),#3840,.T.);
#70718=ADVANCED_FACE('',(#9968),#3841,.T.);
#70719=ADVANCED_FACE('',(#9969),#3842,.T.);
#70720=ADVANCED_FACE('',(#9970),#3843,.T.);
#70721=ADVANCED_FACE('',(#9971),#3844,.T.);
#70722=ADVANCED_FACE('',(#9972),#3845,.T.);
#70723=ADVANCED_FACE('',(#9973),#3846,.T.);
#70724=ADVANCED_FACE('',(#9974),#3847,.T.);
#70725=ADVANCED_FACE('',(#9975),#3848,.T.);
#70726=ADVANCED_FACE('',(#9976),#3849,.T.);
#70727=ADVANCED_FACE('',(#9977),#3850,.T.);
#70728=ADVANCED_FACE('',(#9978),#3851,.T.);
#70729=ADVANCED_FACE('',(#9979),#3852,.T.);
#70730=ADVANCED_FACE('',(#9980),#3853,.T.);
#70731=ADVANCED_FACE('',(#9981),#3854,.T.);
#70732=ADVANCED_FACE('',(#9982),#3855,.T.);
#70733=ADVANCED_FACE('',(#9983),#3856,.T.);
#70734=ADVANCED_FACE('',(#9984),#3857,.T.);
#70735=ADVANCED_FACE('',(#9985),#3858,.T.);
#70736=ADVANCED_FACE('',(#9986),#3859,.T.);
#70737=ADVANCED_FACE('',(#9987),#3860,.T.);
#70738=ADVANCED_FACE('',(#9988),#3861,.T.);
#70739=ADVANCED_FACE('',(#9989),#3862,.T.);
#70740=ADVANCED_FACE('',(#9990),#3863,.T.);
#70741=ADVANCED_FACE('',(#9991),#3864,.T.);
#70742=ADVANCED_FACE('',(#9992),#3865,.T.);
#70743=ADVANCED_FACE('',(#9993),#3866,.T.);
#70744=ADVANCED_FACE('',(#9994),#3867,.T.);
#70745=ADVANCED_FACE('',(#9995),#3868,.T.);
#70746=ADVANCED_FACE('',(#9996),#3869,.T.);
#70747=ADVANCED_FACE('',(#9997),#3870,.T.);
#70748=ADVANCED_FACE('',(#9998),#3871,.T.);
#70749=ADVANCED_FACE('',(#9999),#3872,.T.);
#70750=ADVANCED_FACE('',(#10000),#3873,.T.);
#70751=ADVANCED_FACE('',(#10001),#3874,.T.);
#70752=ADVANCED_FACE('',(#10002),#3875,.T.);
#70753=ADVANCED_FACE('',(#10003),#3876,.T.);
#70754=ADVANCED_FACE('',(#10004),#3877,.T.);
#70755=ADVANCED_FACE('',(#10005),#3878,.T.);
#70756=ADVANCED_FACE('',(#10006),#3879,.T.);
#70757=ADVANCED_FACE('',(#10007),#3880,.T.);
#70758=ADVANCED_FACE('',(#10008),#3881,.T.);
#70759=ADVANCED_FACE('',(#10009),#3882,.T.);
#70760=ADVANCED_FACE('',(#10010),#3883,.T.);
#70761=ADVANCED_FACE('',(#10011),#3884,.T.);
#70762=ADVANCED_FACE('',(#10012),#3885,.T.);
#70763=ADVANCED_FACE('',(#10013),#3886,.T.);
#70764=ADVANCED_FACE('',(#10014),#3887,.T.);
#70765=ADVANCED_FACE('',(#10015),#3888,.T.);
#70766=ADVANCED_FACE('',(#10016),#3889,.T.);
#70767=ADVANCED_FACE('',(#10017),#3890,.T.);
#70768=ADVANCED_FACE('',(#10018),#3891,.T.);
#70769=ADVANCED_FACE('',(#10019),#3892,.T.);
#70770=ADVANCED_FACE('',(#10020),#3893,.T.);
#70771=ADVANCED_FACE('',(#10021),#3894,.T.);
#70772=ADVANCED_FACE('',(#10022),#3895,.T.);
#70773=ADVANCED_FACE('',(#10023),#3896,.T.);
#70774=ADVANCED_FACE('',(#10024),#3897,.T.);
#70775=ADVANCED_FACE('',(#10025),#3898,.T.);
#70776=ADVANCED_FACE('',(#10026),#3899,.T.);
#70777=ADVANCED_FACE('',(#10027),#3900,.T.);
#70778=ADVANCED_FACE('',(#10028),#3901,.T.);
#70779=ADVANCED_FACE('',(#10029),#3902,.T.);
#70780=ADVANCED_FACE('',(#10030),#3903,.T.);
#70781=ADVANCED_FACE('',(#10031),#3904,.T.);
#70782=ADVANCED_FACE('',(#10032),#3905,.T.);
#70783=ADVANCED_FACE('',(#10033),#3906,.T.);
#70784=ADVANCED_FACE('',(#10034),#3907,.T.);
#70785=ADVANCED_FACE('',(#10035),#3908,.T.);
#70786=ADVANCED_FACE('',(#10036),#3909,.T.);
#70787=ADVANCED_FACE('',(#10037),#3910,.T.);
#70788=ADVANCED_FACE('',(#10038),#3911,.T.);
#70789=ADVANCED_FACE('',(#10039),#3912,.T.);
#70790=ADVANCED_FACE('',(#10040),#3913,.T.);
#70791=ADVANCED_FACE('',(#10041),#3914,.T.);
#70792=ADVANCED_FACE('',(#10042),#3915,.T.);
#70793=ADVANCED_FACE('',(#10043),#3916,.T.);
#70794=ADVANCED_FACE('',(#10044),#3917,.T.);
#70795=ADVANCED_FACE('',(#10045),#3918,.T.);
#70796=ADVANCED_FACE('',(#10046),#3919,.T.);
#70797=ADVANCED_FACE('',(#10047),#3920,.T.);
#70798=ADVANCED_FACE('',(#10048),#3921,.T.);
#70799=ADVANCED_FACE('',(#10049),#3922,.T.);
#70800=ADVANCED_FACE('',(#10050),#3923,.T.);
#70801=ADVANCED_FACE('',(#10051),#3924,.T.);
#70802=ADVANCED_FACE('',(#10052),#3925,.T.);
#70803=ADVANCED_FACE('',(#10053),#3926,.T.);
#70804=ADVANCED_FACE('',(#10054),#3927,.T.);
#70805=ADVANCED_FACE('',(#10055),#3928,.T.);
#70806=ADVANCED_FACE('',(#10056),#3929,.T.);
#70807=ADVANCED_FACE('',(#10057),#3930,.T.);
#70808=ADVANCED_FACE('',(#10058),#3931,.T.);
#70809=ADVANCED_FACE('',(#10059),#3932,.T.);
#70810=ADVANCED_FACE('',(#10060),#3933,.T.);
#70811=ADVANCED_FACE('',(#10061),#3934,.T.);
#70812=ADVANCED_FACE('',(#10062),#3935,.T.);
#70813=ADVANCED_FACE('',(#10063),#3936,.T.);
#70814=ADVANCED_FACE('',(#10064),#3937,.T.);
#70815=ADVANCED_FACE('',(#10065),#3938,.T.);
#70816=ADVANCED_FACE('',(#10066),#3939,.T.);
#70817=ADVANCED_FACE('',(#10067),#3940,.T.);
#70818=ADVANCED_FACE('',(#10068),#3941,.T.);
#70819=ADVANCED_FACE('',(#10069),#3942,.T.);
#70820=ADVANCED_FACE('',(#10070),#3943,.T.);
#70821=ADVANCED_FACE('',(#10071),#3944,.T.);
#70822=ADVANCED_FACE('',(#10072),#3945,.T.);
#70823=ADVANCED_FACE('',(#10073),#3946,.T.);
#70824=ADVANCED_FACE('',(#10074),#3947,.T.);
#70825=ADVANCED_FACE('',(#10075),#3948,.T.);
#70826=ADVANCED_FACE('',(#10076),#3949,.T.);
#70827=ADVANCED_FACE('',(#10077),#3950,.T.);
#70828=ADVANCED_FACE('',(#10078),#3951,.T.);
#70829=ADVANCED_FACE('',(#10079),#3952,.T.);
#70830=ADVANCED_FACE('',(#10080),#3953,.T.);
#70831=ADVANCED_FACE('',(#10081),#3954,.T.);
#70832=ADVANCED_FACE('',(#10082),#3955,.T.);
#70833=ADVANCED_FACE('',(#10083),#3956,.T.);
#70834=ADVANCED_FACE('',(#10084),#3957,.T.);
#70835=ADVANCED_FACE('',(#10085),#3958,.T.);
#70836=ADVANCED_FACE('',(#10086),#3959,.T.);
#70837=ADVANCED_FACE('',(#10087),#3960,.T.);
#70838=ADVANCED_FACE('',(#10088),#3961,.T.);
#70839=ADVANCED_FACE('',(#10089),#3962,.T.);
#70840=ADVANCED_FACE('',(#10090),#3963,.T.);
#70841=ADVANCED_FACE('',(#10091),#3964,.T.);
#70842=ADVANCED_FACE('',(#10092),#3965,.T.);
#70843=ADVANCED_FACE('',(#10093),#66068,.T.);
#70844=ADVANCED_FACE('',(#10094),#3966,.T.);
#70845=ADVANCED_FACE('',(#10095),#5333,.T.);
#70846=ADVANCED_FACE('',(#10096),#3967,.T.);
#70847=ADVANCED_FACE('',(#10097),#66069,.T.);
#70848=ADVANCED_FACE('',(#10098),#3968,.T.);
#70849=ADVANCED_FACE('',(#10099),#5334,.T.);
#70850=ADVANCED_FACE('',(#10100),#3969,.T.);
#70851=ADVANCED_FACE('',(#10101),#66070,.T.);
#70852=ADVANCED_FACE('',(#10102),#3970,.T.);
#70853=ADVANCED_FACE('',(#10103),#5335,.T.);
#70854=ADVANCED_FACE('',(#10104),#3971,.T.);
#70855=ADVANCED_FACE('',(#10105),#66071,.T.);
#70856=ADVANCED_FACE('',(#10106),#3972,.T.);
#70857=ADVANCED_FACE('',(#10107),#5336,.T.);
#70858=ADVANCED_FACE('',(#10108),#3973,.T.);
#70859=ADVANCED_FACE('',(#10109),#66072,.T.);
#70860=ADVANCED_FACE('',(#10110),#3974,.T.);
#70861=ADVANCED_FACE('',(#10111),#5337,.T.);
#70862=ADVANCED_FACE('',(#10112),#3975,.T.);
#70863=ADVANCED_FACE('',(#10113),#66073,.T.);
#70864=ADVANCED_FACE('',(#10114),#3976,.T.);
#70865=ADVANCED_FACE('',(#10115),#5338,.T.);
#70866=ADVANCED_FACE('',(#10116),#3977,.T.);
#70867=ADVANCED_FACE('',(#10117),#66074,.T.);
#70868=ADVANCED_FACE('',(#10118),#3978,.T.);
#70869=ADVANCED_FACE('',(#10119),#3979,.T.);
#70870=ADVANCED_FACE('',(#10120),#66075,.T.);
#70871=ADVANCED_FACE('',(#10121),#3980,.T.);
#70872=ADVANCED_FACE('',(#10122),#5339,.T.);
#70873=ADVANCED_FACE('',(#10123),#3981,.T.);
#70874=ADVANCED_FACE('',(#10124),#66076,.T.);
#70875=ADVANCED_FACE('',(#10125),#3982,.T.);
#70876=ADVANCED_FACE('',(#10126),#5340,.T.);
#70877=ADVANCED_FACE('',(#10127),#3983,.T.);
#70878=ADVANCED_FACE('',(#10128),#66077,.T.);
#70879=ADVANCED_FACE('',(#10129),#3984,.T.);
#70880=ADVANCED_FACE('',(#10130),#5341,.T.);
#70881=ADVANCED_FACE('',(#10131),#3985,.T.);
#70882=ADVANCED_FACE('',(#10132),#66078,.T.);
#70883=ADVANCED_FACE('',(#10133),#3986,.T.);
#70884=ADVANCED_FACE('',(#10134),#5342,.T.);
#70885=ADVANCED_FACE('',(#10135),#3987,.T.);
#70886=ADVANCED_FACE('',(#10136),#66079,.T.);
#70887=ADVANCED_FACE('',(#10137),#3988,.T.);
#70888=ADVANCED_FACE('',(#10138),#5343,.T.);
#70889=ADVANCED_FACE('',(#10139),#3989,.T.);
#70890=ADVANCED_FACE('',(#10140),#66080,.T.);
#70891=ADVANCED_FACE('',(#10141),#3990,.T.);
#70892=ADVANCED_FACE('',(#10142),#5344,.T.);
#70893=ADVANCED_FACE('',(#10143),#3991,.T.);
#70894=ADVANCED_FACE('',(#10144),#66081,.T.);
#70895=ADVANCED_FACE('',(#10145),#3992,.T.);
#70896=ADVANCED_FACE('',(#10146),#5345,.T.);
#70897=ADVANCED_FACE('',(#10147),#3993,.T.);
#70898=ADVANCED_FACE('',(#10148),#66082,.T.);
#70899=ADVANCED_FACE('',(#10149),#3994,.T.);
#70900=ADVANCED_FACE('',(#10150),#5346,.T.);
#70901=ADVANCED_FACE('',(#10151),#3995,.T.);
#70902=ADVANCED_FACE('',(#10152),#66083,.T.);
#70903=ADVANCED_FACE('',(#10153),#3996,.T.);
#70904=ADVANCED_FACE('',(#10154),#5347,.T.);
#70905=ADVANCED_FACE('',(#10155),#3997,.T.);
#70906=ADVANCED_FACE('',(#10156),#66084,.T.);
#70907=ADVANCED_FACE('',(#10157),#3998,.T.);
#70908=ADVANCED_FACE('',(#10158),#5348,.T.);
#70909=ADVANCED_FACE('',(#10159),#3999,.T.);
#70910=ADVANCED_FACE('',(#10160),#66085,.T.);
#70911=ADVANCED_FACE('',(#10161),#4000,.T.);
#70912=ADVANCED_FACE('',(#10162),#5349,.T.);
#70913=ADVANCED_FACE('',(#10163),#4001,.T.);
#70914=ADVANCED_FACE('',(#10164),#66086,.T.);
#70915=ADVANCED_FACE('',(#10165),#4002,.T.);
#70916=ADVANCED_FACE('',(#10166),#5350,.T.);
#70917=ADVANCED_FACE('',(#10167),#4003,.T.);
#70918=ADVANCED_FACE('',(#10168),#66087,.T.);
#70919=ADVANCED_FACE('',(#10169),#4004,.T.);
#70920=ADVANCED_FACE('',(#10170),#5351,.T.);
#70921=ADVANCED_FACE('',(#10171),#4005,.T.);
#70922=ADVANCED_FACE('',(#10172),#66088,.T.);
#70923=ADVANCED_FACE('',(#10173),#4006,.T.);
#70924=ADVANCED_FACE('',(#10174),#5352,.T.);
#70925=ADVANCED_FACE('',(#10175),#4007,.T.);
#70926=ADVANCED_FACE('',(#10176),#66089,.T.);
#70927=ADVANCED_FACE('',(#10177),#4008,.T.);
#70928=ADVANCED_FACE('',(#10178),#5353,.T.);
#70929=ADVANCED_FACE('',(#10179),#4009,.T.);
#70930=ADVANCED_FACE('',(#10180),#66090,.T.);
#70931=ADVANCED_FACE('',(#10181),#4010,.T.);
#70932=ADVANCED_FACE('',(#10182),#5354,.T.);
#70933=ADVANCED_FACE('',(#10183),#4011,.T.);
#70934=ADVANCED_FACE('',(#10184),#66091,.T.);
#70935=ADVANCED_FACE('',(#10185),#4012,.T.);
#70936=ADVANCED_FACE('',(#10186),#5355,.T.);
#70937=ADVANCED_FACE('',(#10187),#4013,.T.);
#70938=ADVANCED_FACE('',(#10188),#66092,.T.);
#70939=ADVANCED_FACE('',(#10189),#4014,.T.);
#70940=ADVANCED_FACE('',(#10190),#5356,.T.);
#70941=ADVANCED_FACE('',(#10191),#4015,.T.);
#70942=ADVANCED_FACE('',(#10192),#66093,.T.);
#70943=ADVANCED_FACE('',(#10193),#4016,.T.);
#70944=ADVANCED_FACE('',(#10194),#5357,.T.);
#70945=ADVANCED_FACE('',(#10195),#4017,.T.);
#70946=ADVANCED_FACE('',(#10196),#66094,.T.);
#70947=ADVANCED_FACE('',(#10197),#4018,.T.);
#70948=ADVANCED_FACE('',(#10198),#5358,.T.);
#70949=ADVANCED_FACE('',(#10199),#4019,.T.);
#70950=ADVANCED_FACE('',(#10200),#66095,.T.);
#70951=ADVANCED_FACE('',(#10201),#4020,.T.);
#70952=ADVANCED_FACE('',(#10202),#5359,.T.);
#70953=ADVANCED_FACE('',(#10203),#66096,.T.);
#70954=ADVANCED_FACE('',(#10204),#5360,.T.);
#70955=ADVANCED_FACE('',(#10205),#4021,.T.);
#70956=ADVANCED_FACE('',(#10206,#70),#86,.T.);
#70957=ADVANCED_FACE('',(#10207),#4022,.T.);
#70958=ADVANCED_FACE('',(#10208),#4023,.T.);
#70959=ADVANCED_FACE('',(#10209),#4024,.T.);
#70960=ADVANCED_FACE('',(#10210),#4025,.T.);
#70961=ADVANCED_FACE('',(#10211),#4026,.T.);
#70962=ADVANCED_FACE('',(#10212),#4027,.T.);
#70963=ADVANCED_FACE('',(#10213),#4028,.T.);
#70964=ADVANCED_FACE('',(#10214),#4029,.T.);
#70965=ADVANCED_FACE('',(#10215),#4030,.T.);
#70966=ADVANCED_FACE('',(#10216),#4031,.T.);
#70967=ADVANCED_FACE('',(#10217),#4032,.T.);
#70968=ADVANCED_FACE('',(#10218),#4033,.T.);
#70969=ADVANCED_FACE('',(#10219),#4034,.T.);
#70970=ADVANCED_FACE('',(#10220),#4035,.T.);
#70971=ADVANCED_FACE('',(#10221),#4036,.T.);
#70972=ADVANCED_FACE('',(#10222),#4037,.T.);
#70973=ADVANCED_FACE('',(#10223),#4038,.T.);
#70974=ADVANCED_FACE('',(#10224),#4039,.T.);
#70975=ADVANCED_FACE('',(#10225),#4040,.T.);
#70976=ADVANCED_FACE('',(#10226),#4041,.T.);
#70977=ADVANCED_FACE('',(#10227),#4042,.T.);
#70978=ADVANCED_FACE('',(#10228),#4043,.T.);
#70979=ADVANCED_FACE('',(#10229),#4044,.T.);
#70980=ADVANCED_FACE('',(#10230),#4045,.T.);
#70981=ADVANCED_FACE('',(#10231),#4046,.T.);
#70982=ADVANCED_FACE('',(#10232),#4047,.T.);
#70983=ADVANCED_FACE('',(#10233),#4048,.T.);
#70984=ADVANCED_FACE('',(#10234),#4049,.T.);
#70985=ADVANCED_FACE('',(#10235),#4050,.T.);
#70986=ADVANCED_FACE('',(#10236),#4051,.T.);
#70987=ADVANCED_FACE('',(#10237),#4052,.T.);
#70988=ADVANCED_FACE('',(#10238),#4053,.T.);
#70989=ADVANCED_FACE('',(#10239),#4054,.T.);
#70990=ADVANCED_FACE('',(#10240),#4055,.T.);
#70991=ADVANCED_FACE('',(#10241),#4056,.T.);
#70992=ADVANCED_FACE('',(#10242),#4057,.T.);
#70993=ADVANCED_FACE('',(#10243),#4058,.T.);
#70994=ADVANCED_FACE('',(#10244),#4059,.T.);
#70995=ADVANCED_FACE('',(#10245),#4060,.T.);
#70996=ADVANCED_FACE('',(#10246),#4061,.T.);
#70997=ADVANCED_FACE('',(#10247),#4062,.T.);
#70998=ADVANCED_FACE('',(#10248),#4063,.T.);
#70999=ADVANCED_FACE('',(#10249),#4064,.T.);
#71000=ADVANCED_FACE('',(#10250),#4065,.T.);
#71001=ADVANCED_FACE('',(#10251),#4066,.T.);
#71002=ADVANCED_FACE('',(#10252),#4067,.T.);
#71003=ADVANCED_FACE('',(#10253),#4068,.T.);
#71004=ADVANCED_FACE('',(#10254),#4069,.T.);
#71005=ADVANCED_FACE('',(#10255),#4070,.T.);
#71006=ADVANCED_FACE('',(#10256),#4071,.T.);
#71007=ADVANCED_FACE('',(#10257),#4072,.T.);
#71008=ADVANCED_FACE('',(#10258),#4073,.T.);
#71009=ADVANCED_FACE('',(#10259),#4074,.T.);
#71010=ADVANCED_FACE('',(#10260),#4075,.T.);
#71011=ADVANCED_FACE('',(#10261),#4076,.T.);
#71012=ADVANCED_FACE('',(#10262),#4077,.T.);
#71013=ADVANCED_FACE('',(#10263),#4078,.T.);
#71014=ADVANCED_FACE('',(#10264),#4079,.T.);
#71015=ADVANCED_FACE('',(#10265),#4080,.T.);
#71016=ADVANCED_FACE('',(#10266),#66097,.T.);
#71017=ADVANCED_FACE('',(#10267),#4081,.T.);
#71018=ADVANCED_FACE('',(#10268),#4082,.T.);
#71019=ADVANCED_FACE('',(#10269),#66098,.T.);
#71020=ADVANCED_FACE('',(#10270),#4083,.T.);
#71021=ADVANCED_FACE('',(#10271),#4084,.T.);
#71022=ADVANCED_FACE('',(#10272),#66099,.T.);
#71023=ADVANCED_FACE('',(#10273),#4085,.T.);
#71024=ADVANCED_FACE('',(#10274),#4086,.T.);
#71025=ADVANCED_FACE('',(#10275),#66100,.T.);
#71026=ADVANCED_FACE('',(#10276),#4087,.T.);
#71027=ADVANCED_FACE('',(#10277),#4088,.T.);
#71028=ADVANCED_FACE('',(#10278),#66101,.T.);
#71029=ADVANCED_FACE('',(#10279),#4089,.T.);
#71030=ADVANCED_FACE('',(#10280),#4090,.T.);
#71031=ADVANCED_FACE('',(#10281),#66102,.T.);
#71032=ADVANCED_FACE('',(#10282),#4091,.T.);
#71033=ADVANCED_FACE('',(#10283),#4092,.T.);
#71034=ADVANCED_FACE('',(#10284),#66103,.T.);
#71035=ADVANCED_FACE('',(#10285),#4093,.T.);
#71036=ADVANCED_FACE('',(#10286),#4094,.T.);
#71037=ADVANCED_FACE('',(#10287),#66104,.T.);
#71038=ADVANCED_FACE('',(#10288),#4095,.T.);
#71039=ADVANCED_FACE('',(#10289),#4096,.T.);
#71040=ADVANCED_FACE('',(#10290),#66105,.T.);
#71041=ADVANCED_FACE('',(#10291),#4097,.T.);
#71042=ADVANCED_FACE('',(#10292),#4098,.T.);
#71043=ADVANCED_FACE('',(#10293),#66106,.T.);
#71044=ADVANCED_FACE('',(#10294),#4099,.T.);
#71045=ADVANCED_FACE('',(#10295),#4100,.T.);
#71046=ADVANCED_FACE('',(#10296),#66107,.T.);
#71047=ADVANCED_FACE('',(#10297),#4101,.T.);
#71048=ADVANCED_FACE('',(#10298),#4102,.T.);
#71049=ADVANCED_FACE('',(#10299),#66108,.T.);
#71050=ADVANCED_FACE('',(#10300),#4103,.T.);
#71051=ADVANCED_FACE('',(#10301),#4104,.T.);
#71052=ADVANCED_FACE('',(#10302),#66109,.T.);
#71053=ADVANCED_FACE('',(#10303),#4105,.T.);
#71054=ADVANCED_FACE('',(#10304),#4106,.T.);
#71055=ADVANCED_FACE('',(#10305),#66110,.T.);
#71056=ADVANCED_FACE('',(#10306),#4107,.T.);
#71057=ADVANCED_FACE('',(#10307),#4108,.T.);
#71058=ADVANCED_FACE('',(#10308),#66111,.T.);
#71059=ADVANCED_FACE('',(#10309),#4109,.T.);
#71060=ADVANCED_FACE('',(#10310),#4110,.T.);
#71061=ADVANCED_FACE('',(#10311),#66112,.T.);
#71062=ADVANCED_FACE('',(#10312),#4111,.T.);
#71063=ADVANCED_FACE('',(#10313),#4112,.T.);
#71064=ADVANCED_FACE('',(#10314),#66113,.T.);
#71065=ADVANCED_FACE('',(#10315),#4113,.T.);
#71066=ADVANCED_FACE('',(#10316),#4114,.T.);
#71067=ADVANCED_FACE('',(#10317),#66114,.T.);
#71068=ADVANCED_FACE('',(#10318),#4115,.T.);
#71069=ADVANCED_FACE('',(#10319),#4116,.T.);
#71070=ADVANCED_FACE('',(#10320),#66115,.T.);
#71071=ADVANCED_FACE('',(#10321),#4117,.T.);
#71072=ADVANCED_FACE('',(#10322),#4118,.T.);
#71073=ADVANCED_FACE('',(#10323),#66116,.T.);
#71074=ADVANCED_FACE('',(#10324),#4119,.T.);
#71075=ADVANCED_FACE('',(#10325),#4120,.T.);
#71076=ADVANCED_FACE('',(#10326),#66117,.T.);
#71077=ADVANCED_FACE('',(#10327),#4121,.T.);
#71078=ADVANCED_FACE('',(#10328),#4122,.T.);
#71079=ADVANCED_FACE('',(#10329),#4123,.T.);
#71080=ADVANCED_FACE('',(#10330),#4124,.T.);
#71081=ADVANCED_FACE('',(#10331),#66118,.T.);
#71082=ADVANCED_FACE('',(#10332),#4125,.T.);
#71083=ADVANCED_FACE('',(#10333),#4126,.T.);
#71084=ADVANCED_FACE('',(#10334),#66119,.T.);
#71085=ADVANCED_FACE('',(#10335),#4127,.T.);
#71086=ADVANCED_FACE('',(#10336),#4128,.T.);
#71087=ADVANCED_FACE('',(#10337),#66120,.T.);
#71088=ADVANCED_FACE('',(#10338),#4129,.T.);
#71089=ADVANCED_FACE('',(#10339),#4130,.T.);
#71090=ADVANCED_FACE('',(#10340),#66121,.T.);
#71091=ADVANCED_FACE('',(#10341),#4131,.T.);
#71092=ADVANCED_FACE('',(#10342),#4132,.T.);
#71093=ADVANCED_FACE('',(#10343),#66122,.T.);
#71094=ADVANCED_FACE('',(#10344),#4133,.T.);
#71095=ADVANCED_FACE('',(#10345),#4134,.T.);
#71096=ADVANCED_FACE('',(#10346),#66123,.T.);
#71097=ADVANCED_FACE('',(#10347),#4135,.T.);
#71098=ADVANCED_FACE('',(#10348),#4136,.T.);
#71099=ADVANCED_FACE('',(#10349),#4137,.T.);
#71100=ADVANCED_FACE('',(#10350),#4138,.T.);
#71101=ADVANCED_FACE('',(#10351),#4139,.T.);
#71102=ADVANCED_FACE('',(#10352),#4140,.T.);
#71103=ADVANCED_FACE('',(#10353),#4141,.T.);
#71104=ADVANCED_FACE('',(#10354),#4142,.T.);
#71105=ADVANCED_FACE('',(#10355),#4143,.T.);
#71106=ADVANCED_FACE('',(#10356),#4144,.T.);
#71107=ADVANCED_FACE('',(#10357),#4145,.T.);
#71108=ADVANCED_FACE('',(#10358),#4146,.T.);
#71109=ADVANCED_FACE('',(#10359),#4147,.T.);
#71110=ADVANCED_FACE('',(#10360),#4148,.T.);
#71111=ADVANCED_FACE('',(#10361),#4149,.T.);
#71112=ADVANCED_FACE('',(#10362),#4150,.T.);
#71113=ADVANCED_FACE('',(#10363),#4151,.T.);
#71114=ADVANCED_FACE('',(#10364),#4152,.T.);
#71115=ADVANCED_FACE('',(#10365),#4153,.T.);
#71116=ADVANCED_FACE('',(#10366),#4154,.T.);
#71117=ADVANCED_FACE('',(#10367),#4155,.T.);
#71118=ADVANCED_FACE('',(#10368),#4156,.T.);
#71119=ADVANCED_FACE('',(#10369),#4157,.T.);
#71120=ADVANCED_FACE('',(#10370),#4158,.T.);
#71121=ADVANCED_FACE('',(#10371),#4159,.T.);
#71122=ADVANCED_FACE('',(#10372),#4160,.T.);
#71123=ADVANCED_FACE('',(#10373),#4161,.T.);
#71124=ADVANCED_FACE('',(#10374),#4162,.T.);
#71125=ADVANCED_FACE('',(#10375),#4163,.T.);
#71126=ADVANCED_FACE('',(#10376),#4164,.T.);
#71127=ADVANCED_FACE('',(#10377),#4165,.T.);
#71128=ADVANCED_FACE('',(#10378),#4166,.T.);
#71129=ADVANCED_FACE('',(#10379),#4167,.T.);
#71130=ADVANCED_FACE('',(#10380),#4168,.T.);
#71131=ADVANCED_FACE('',(#10381),#4169,.T.);
#71132=ADVANCED_FACE('',(#10382),#4170,.T.);
#71133=ADVANCED_FACE('',(#10383),#4171,.T.);
#71134=ADVANCED_FACE('',(#10384),#4172,.T.);
#71135=ADVANCED_FACE('',(#10385),#4173,.T.);
#71136=ADVANCED_FACE('',(#10386),#4174,.T.);
#71137=ADVANCED_FACE('',(#10387),#4175,.T.);
#71138=ADVANCED_FACE('',(#10388),#4176,.T.);
#71139=ADVANCED_FACE('',(#10389),#4177,.T.);
#71140=ADVANCED_FACE('',(#10390),#4178,.T.);
#71141=ADVANCED_FACE('',(#10391),#4179,.T.);
#71142=ADVANCED_FACE('',(#10392),#4180,.T.);
#71143=ADVANCED_FACE('',(#10393),#4181,.T.);
#71144=ADVANCED_FACE('',(#10394),#4182,.T.);
#71145=ADVANCED_FACE('',(#10395),#4183,.T.);
#71146=ADVANCED_FACE('',(#10396),#4184,.T.);
#71147=ADVANCED_FACE('',(#10397),#4185,.T.);
#71148=ADVANCED_FACE('',(#10398),#4186,.T.);
#71149=ADVANCED_FACE('',(#10399),#4187,.T.);
#71150=ADVANCED_FACE('',(#10400),#4188,.T.);
#71151=ADVANCED_FACE('',(#10401),#4189,.T.);
#71152=ADVANCED_FACE('',(#10402),#4190,.T.);
#71153=ADVANCED_FACE('',(#10403),#4191,.T.);
#71154=ADVANCED_FACE('',(#10404),#4192,.T.);
#71155=ADVANCED_FACE('',(#10405),#4193,.T.);
#71156=ADVANCED_FACE('',(#10406),#4194,.T.);
#71157=ADVANCED_FACE('',(#10407),#4195,.T.);
#71158=ADVANCED_FACE('',(#10408,#71),#87,.T.);
#71159=ADVANCED_FACE('',(#10409),#4196,.T.);
#71160=ADVANCED_FACE('',(#10410),#4197,.T.);
#71161=ADVANCED_FACE('',(#10411),#4198,.T.);
#71162=ADVANCED_FACE('',(#10412),#4199,.T.);
#71163=ADVANCED_FACE('',(#10413),#4200,.T.);
#71164=ADVANCED_FACE('',(#10414),#4201,.T.);
#71165=ADVANCED_FACE('',(#10415),#4202,.T.);
#71166=ADVANCED_FACE('',(#10416),#4203,.T.);
#71167=ADVANCED_FACE('',(#10417),#4204,.T.);
#71168=ADVANCED_FACE('',(#10418),#4205,.T.);
#71169=ADVANCED_FACE('',(#10419),#4206,.T.);
#71170=ADVANCED_FACE('',(#10420),#4207,.T.);
#71171=ADVANCED_FACE('',(#10421),#4208,.T.);
#71172=ADVANCED_FACE('',(#10422),#4209,.T.);
#71173=ADVANCED_FACE('',(#10423),#4210,.T.);
#71174=ADVANCED_FACE('',(#10424),#4211,.T.);
#71175=ADVANCED_FACE('',(#10425),#4212,.T.);
#71176=ADVANCED_FACE('',(#10426),#4213,.T.);
#71177=ADVANCED_FACE('',(#10427),#4214,.T.);
#71178=ADVANCED_FACE('',(#10428),#4215,.T.);
#71179=ADVANCED_FACE('',(#10429),#4216,.T.);
#71180=ADVANCED_FACE('',(#10430),#4217,.T.);
#71181=ADVANCED_FACE('',(#10431),#4218,.T.);
#71182=ADVANCED_FACE('',(#10432),#4219,.T.);
#71183=ADVANCED_FACE('',(#10433),#4220,.T.);
#71184=ADVANCED_FACE('',(#10434),#4221,.T.);
#71185=ADVANCED_FACE('',(#10435),#4222,.T.);
#71186=ADVANCED_FACE('',(#10436),#4223,.T.);
#71187=ADVANCED_FACE('',(#10437),#4224,.T.);
#71188=ADVANCED_FACE('',(#10438),#4225,.T.);
#71189=ADVANCED_FACE('',(#10439),#4226,.T.);
#71190=ADVANCED_FACE('',(#10440),#4227,.T.);
#71191=ADVANCED_FACE('',(#10441),#4228,.T.);
#71192=ADVANCED_FACE('',(#10442),#4229,.T.);
#71193=ADVANCED_FACE('',(#10443),#4230,.T.);
#71194=ADVANCED_FACE('',(#10444),#4231,.T.);
#71195=ADVANCED_FACE('',(#10445),#4232,.T.);
#71196=ADVANCED_FACE('',(#10446),#4233,.T.);
#71197=ADVANCED_FACE('',(#10447),#4234,.T.);
#71198=ADVANCED_FACE('',(#10448),#4235,.T.);
#71199=ADVANCED_FACE('',(#10449),#4236,.T.);
#71200=ADVANCED_FACE('',(#10450),#4237,.T.);
#71201=ADVANCED_FACE('',(#10451),#4238,.T.);
#71202=ADVANCED_FACE('',(#10452),#4239,.T.);
#71203=ADVANCED_FACE('',(#10453),#4240,.T.);
#71204=ADVANCED_FACE('',(#10454),#4241,.T.);
#71205=ADVANCED_FACE('',(#10455),#4242,.T.);
#71206=ADVANCED_FACE('',(#10456),#4243,.T.);
#71207=ADVANCED_FACE('',(#10457),#4244,.T.);
#71208=ADVANCED_FACE('',(#10458),#4245,.T.);
#71209=ADVANCED_FACE('',(#10459),#4246,.T.);
#71210=ADVANCED_FACE('',(#10460),#4247,.T.);
#71211=ADVANCED_FACE('',(#10461),#4248,.T.);
#71212=ADVANCED_FACE('',(#10462),#4249,.T.);
#71213=ADVANCED_FACE('',(#10463),#4250,.T.);
#71214=ADVANCED_FACE('',(#10464),#4251,.T.);
#71215=ADVANCED_FACE('',(#10465),#4252,.T.);
#71216=ADVANCED_FACE('',(#10466),#4253,.T.);
#71217=ADVANCED_FACE('',(#10467),#4254,.T.);
#71218=ADVANCED_FACE('',(#10468),#4255,.T.);
#71219=ADVANCED_FACE('',(#10469),#4256,.T.);
#71220=ADVANCED_FACE('',(#10470),#4257,.T.);
#71221=ADVANCED_FACE('',(#10471),#4258,.T.);
#71222=ADVANCED_FACE('',(#10472),#4259,.T.);
#71223=ADVANCED_FACE('',(#10473),#4260,.T.);
#71224=ADVANCED_FACE('',(#10474),#4261,.T.);
#71225=ADVANCED_FACE('',(#10475),#4262,.T.);
#71226=ADVANCED_FACE('',(#10476),#4263,.T.);
#71227=ADVANCED_FACE('',(#10477),#4264,.T.);
#71228=ADVANCED_FACE('',(#10478),#4265,.T.);
#71229=ADVANCED_FACE('',(#10479),#4266,.T.);
#71230=ADVANCED_FACE('',(#10480),#4267,.T.);
#71231=ADVANCED_FACE('',(#10481),#4268,.T.);
#71232=ADVANCED_FACE('',(#10482),#4269,.T.);
#71233=ADVANCED_FACE('',(#10483),#4270,.T.);
#71234=ADVANCED_FACE('',(#10484),#4271,.T.);
#71235=ADVANCED_FACE('',(#10485),#4272,.T.);
#71236=ADVANCED_FACE('',(#10486),#4273,.T.);
#71237=ADVANCED_FACE('',(#10487),#4274,.T.);
#71238=ADVANCED_FACE('',(#10488),#4275,.T.);
#71239=ADVANCED_FACE('',(#10489),#4276,.T.);
#71240=ADVANCED_FACE('',(#10490),#4277,.T.);
#71241=ADVANCED_FACE('',(#10491),#4278,.T.);
#71242=ADVANCED_FACE('',(#10492),#4279,.T.);
#71243=ADVANCED_FACE('',(#10493),#4280,.T.);
#71244=ADVANCED_FACE('',(#10494),#4281,.T.);
#71245=ADVANCED_FACE('',(#10495),#4282,.T.);
#71246=ADVANCED_FACE('',(#10496),#4283,.T.);
#71247=ADVANCED_FACE('',(#10497),#4284,.T.);
#71248=ADVANCED_FACE('',(#10498),#4285,.T.);
#71249=ADVANCED_FACE('',(#10499),#4286,.T.);
#71250=ADVANCED_FACE('',(#10500),#4287,.T.);
#71251=ADVANCED_FACE('',(#10501),#4288,.T.);
#71252=ADVANCED_FACE('',(#10502),#4289,.T.);
#71253=ADVANCED_FACE('',(#10503),#4290,.T.);
#71254=ADVANCED_FACE('',(#10504),#4291,.T.);
#71255=ADVANCED_FACE('',(#10505),#4292,.T.);
#71256=ADVANCED_FACE('',(#10506),#4293,.T.);
#71257=ADVANCED_FACE('',(#10507),#4294,.T.);
#71258=ADVANCED_FACE('',(#10508),#4295,.T.);
#71259=ADVANCED_FACE('',(#10509),#4296,.T.);
#71260=ADVANCED_FACE('',(#10510),#4297,.T.);
#71261=ADVANCED_FACE('',(#10511),#4298,.T.);
#71262=ADVANCED_FACE('',(#10512),#4299,.T.);
#71263=ADVANCED_FACE('',(#10513),#4300,.T.);
#71264=ADVANCED_FACE('',(#10514),#4301,.T.);
#71265=ADVANCED_FACE('',(#10515),#4302,.T.);
#71266=ADVANCED_FACE('',(#10516),#4303,.T.);
#71267=ADVANCED_FACE('',(#10517),#4304,.T.);
#71268=ADVANCED_FACE('',(#10518),#4305,.T.);
#71269=ADVANCED_FACE('',(#10519),#4306,.T.);
#71270=ADVANCED_FACE('',(#10520),#4307,.T.);
#71271=ADVANCED_FACE('',(#10521),#4308,.T.);
#71272=ADVANCED_FACE('',(#10522),#4309,.T.);
#71273=ADVANCED_FACE('',(#10523),#4310,.T.);
#71274=ADVANCED_FACE('',(#10524),#4311,.T.);
#71275=ADVANCED_FACE('',(#10525),#4312,.T.);
#71276=ADVANCED_FACE('',(#10526),#4313,.T.);
#71277=ADVANCED_FACE('',(#10527),#4314,.T.);
#71278=ADVANCED_FACE('',(#10528),#4315,.T.);
#71279=ADVANCED_FACE('',(#10529),#4316,.T.);
#71280=ADVANCED_FACE('',(#10530),#4317,.T.);
#71281=ADVANCED_FACE('',(#10531),#4318,.T.);
#71282=ADVANCED_FACE('',(#10532),#4319,.T.);
#71283=ADVANCED_FACE('',(#10533),#4320,.T.);
#71284=ADVANCED_FACE('',(#10534),#4321,.T.);
#71285=ADVANCED_FACE('',(#10535),#4322,.T.);
#71286=ADVANCED_FACE('',(#10536),#4323,.T.);
#71287=ADVANCED_FACE('',(#10537),#4324,.T.);
#71288=ADVANCED_FACE('',(#10538),#4325,.T.);
#71289=ADVANCED_FACE('',(#10539),#4326,.T.);
#71290=ADVANCED_FACE('',(#10540),#4327,.T.);
#71291=ADVANCED_FACE('',(#10541),#4328,.T.);
#71292=ADVANCED_FACE('',(#10542),#4329,.T.);
#71293=ADVANCED_FACE('',(#10543),#4330,.T.);
#71294=ADVANCED_FACE('',(#10544),#4331,.T.);
#71295=ADVANCED_FACE('',(#10545),#4332,.T.);
#71296=ADVANCED_FACE('',(#10546),#4333,.T.);
#71297=ADVANCED_FACE('',(#10547),#4334,.T.);
#71298=ADVANCED_FACE('',(#10548),#4335,.T.);
#71299=ADVANCED_FACE('',(#10549),#4336,.T.);
#71300=ADVANCED_FACE('',(#10550),#4337,.T.);
#71301=ADVANCED_FACE('',(#10551),#4338,.T.);
#71302=ADVANCED_FACE('',(#10552),#4339,.T.);
#71303=ADVANCED_FACE('',(#10553),#4340,.T.);
#71304=ADVANCED_FACE('',(#10554),#4341,.T.);
#71305=ADVANCED_FACE('',(#10555),#4342,.T.);
#71306=ADVANCED_FACE('',(#10556),#4343,.T.);
#71307=ADVANCED_FACE('',(#10557),#4344,.T.);
#71308=ADVANCED_FACE('',(#10558),#4345,.T.);
#71309=ADVANCED_FACE('',(#10559),#4346,.T.);
#71310=ADVANCED_FACE('',(#10560),#4347,.T.);
#71311=ADVANCED_FACE('',(#10561),#4348,.T.);
#71312=ADVANCED_FACE('',(#10562),#4349,.T.);
#71313=ADVANCED_FACE('',(#10563),#4350,.T.);
#71314=ADVANCED_FACE('',(#10564),#4351,.T.);
#71315=ADVANCED_FACE('',(#10565),#4352,.T.);
#71316=ADVANCED_FACE('',(#10566),#4353,.T.);
#71317=ADVANCED_FACE('',(#10567),#4354,.T.);
#71318=ADVANCED_FACE('',(#10568),#4355,.T.);
#71319=ADVANCED_FACE('',(#10569),#4356,.T.);
#71320=ADVANCED_FACE('',(#10570),#4357,.T.);
#71321=ADVANCED_FACE('',(#10571),#4358,.T.);
#71322=ADVANCED_FACE('',(#10572),#4359,.T.);
#71323=ADVANCED_FACE('',(#10573),#4360,.T.);
#71324=ADVANCED_FACE('',(#10574),#4361,.T.);
#71325=ADVANCED_FACE('',(#10575),#4362,.T.);
#71326=ADVANCED_FACE('',(#10576),#4363,.T.);
#71327=ADVANCED_FACE('',(#10577),#4364,.T.);
#71328=ADVANCED_FACE('',(#10578),#4365,.T.);
#71329=ADVANCED_FACE('',(#10579),#4366,.T.);
#71330=ADVANCED_FACE('',(#10580),#4367,.T.);
#71331=ADVANCED_FACE('',(#10581),#4368,.T.);
#71332=ADVANCED_FACE('',(#10582),#4369,.T.);
#71333=ADVANCED_FACE('',(#10583,#72),#88,.T.);
#71334=ADVANCED_FACE('',(#10584,#73),#89,.T.);
#71398=CLOSED_SHELL('',(#66133,#66134,#66135,#66136,#66137,#66138,#66139,
#66140,#66141,#66142,#66143,#66144,#66145,#66146,#66147,#66148,#66149,#66150,
#66151,#66152,#66153,#66154,#66155,#66156,#66157,#66158,#66159,#66160,#66161,
#66162,#66163,#66164,#66165,#66166,#66167,#66168,#66169,#66170,#66171,#66172,
#66173,#66174,#66175,#66176,#66177,#66178,#66179,#66180,#66181,#66182,#66183,
#66184,#66185,#66186,#66187,#66188,#66189,#66190,#66191,#66192,#66193,#66194,
#66195,#66196,#66197,#66198,#66199,#66200,#66201,#66202,#66203,#66204,#66205,
#66206,#66207,#66208,#66209,#66210,#66211,#66212,#66213,#66214,#66215,#66216,
#66217,#66218,#66219,#66220,#66221,#66222,#66223,#66224,#66225,#66226,#66227,
#66228,#66229,#66230,#66231,#66232,#66233,#66234,#66235,#66236,#66237,#66238,
#66239,#66240,#66241,#66242,#66243,#66244,#66245,#66246,#66247,#66248,#66249,
#66250,#66251,#66252,#66253,#66254,#66255,#66256,#66257,#66258,#66259,#66260,
#66261,#66262,#66263,#66264,#66265,#66266,#66267,#66268,#66269,#66270,#66271,
#66272,#66273,#66274,#66275,#66276,#66277,#66278,#66279,#66280,#66281,#66282,
#66283,#66284,#66285,#66286,#66287,#66288,#66289,#66290,#66291,#66292,#66293,
#66294,#66295,#66296,#66297,#66298,#66299,#66300,#66301,#66302,#66303,#66304,
#66305,#66306,#66307,#66308,#66309,#66310,#66311,#66312,#66313,#66314,#66315,
#66316,#66317,#66318,#66319,#66320,#66321,#66322,#66323,#66324,#66325,#66326,
#66327,#66328,#66329,#66330,#66331,#66332,#66333,#66334,#66335,#66336,#66337,
#66338,#66339,#66340,#66341,#66342,#66343,#66344,#66345,#66346,#66347,#66348,
#66349,#66350,#66351,#66352,#66353,#66354,#66355,#66356,#66357,#66358,#66359,
#66360,#66361,#66362,#66363,#66364,#66365,#66366,#66367,#66368,#66369,#66370,
#66371,#66372,#66373,#66374,#66375,#66376,#66377,#66378,#66379,#66380,#66381,
#66382,#66383,#66384,#66385,#66386,#66387,#66388,#66389,#66390,#66391,#66392,
#66393,#66394,#66395,#66396,#66397,#66398,#66399,#66400,#66401,#66402,#66403,
#66404,#66405,#66406,#66407,#66408,#66409,#66410,#66411,#66412,#66413,#66414,
#66415,#66416,#66417,#66418,#66419,#66420,#66421,#66422,#66423,#66424,#66425,
#66426,#66427,#66428,#66429,#66430,#66431,#66432,#66433,#66434,#66435,#66436,
#66437,#66438,#66439,#66440,#66441,#66442,#66443,#66444,#66445,#66446,#66447,
#66448,#66449,#66450,#66451,#66452,#66453,#66454,#66455,#66456,#66457,#66458,
#66459,#66460,#66461,#66462,#66463,#66464,#66465,#66466,#66467,#66468,#66469,
#66470,#66471,#66472,#66473,#66474,#66475,#66476,#66477,#66478,#66479,#66480,
#66481,#66482,#66483,#66484,#66485,#66486,#66487,#66488,#66489,#66490,#66491,
#66492,#66493,#66494,#66495,#66496,#66497,#66498,#66499,#66500,#66501,#66502,
#66503,#66504,#66505,#66506,#66507,#66508,#66509,#66510,#66511,#66512,#66513,
#66514,#66515,#66516,#66517,#66518,#66519,#66520,#66521,#66522,#66523,#66524,
#66525,#66526,#66527,#66528,#66529,#66530,#66531,#66532,#66533,#66534,#66535,
#66536,#66537,#66538,#66539,#66540,#66541,#66542,#66543,#66544,#66545,#66546,
#66547,#66548,#66549,#66550,#66551,#66552,#66553,#66554,#66555,#66556,#66557,
#66558,#66559,#66560,#66561,#66562,#66563,#66564,#66565,#66566,#66567,#66568,
#66569,#66570,#66571,#66572,#66573,#66574,#66575,#66576,#66577,#66578,#66579,
#66580,#66581,#66582,#66583,#66584,#66585,#66586,#66587,#66588,#66589,#66590,
#66591,#66592,#66593,#66594,#66595,#66596,#66597,#66598,#66599,#66600,#66601,
#66602,#66603,#66604,#66605,#66606,#66607,#66608,#66609,#66610,#66611,#66612,
#66613,#66614,#66615,#66616,#66617,#66618,#66619,#66620,#66621,#66622,#66623,
#66624,#66625,#66626,#66627,#66628,#66629,#66630,#66631,#66632,#66633,#66634,
#66635,#66636,#66637,#66638,#66639,#66640,#66641,#66642,#66643,#66644,#66645,
#66646,#66647,#66648,#66649,#66650,#66651,#66652,#66653,#66654,#66655,#66656,
#66657,#66658,#66659,#66660,#66661,#66662,#66663,#66664,#66665,#66666,#66667,
#66668,#66669,#66670,#66671,#66672,#66673,#66674,#66675,#66676,#66677,#66678,
#66679,#66680,#66681,#66682,#66683,#66684,#66685,#66686,#66687,#66688,#66689,
#66690,#66691,#66692,#66693,#66694,#66695,#66696,#66697,#66698,#66699,#66700,
#66701,#66702,#66703,#66704,#66705,#66706,#66707,#66708,#66709,#66710,#66711,
#66712,#66713,#66714,#66715,#66716,#66717,#66718,#66719,#66720,#66721,#66722,
#66723,#66724,#66725,#66726,#66727,#66728,#66729,#66730,#66731,#66732,#66733,
#66734,#66735,#66736,#66737,#66738,#66739,#66740,#66741,#66742,#66743,#66744,
#66745,#66746,#66747,#66748,#66749,#66750,#66751,#66752,#66753,#66754,#66755,
#66756,#66757,#66758,#66759,#66760,#66761,#66762,#66763,#66764,#66765,#66766,
#66767,#66768,#66769,#66770,#66771,#66772,#66773,#66774,#66775,#66776,#66777,
#66778,#66779,#66780,#66781,#66782,#66783,#66784,#66785,#66786,#66787,#66788,
#66789,#66790,#66791,#66792,#66793,#66794,#66795,#66796,#66797,#66798,#66799,
#66800,#66801,#66802,#66803,#66804,#66805,#66806,#66807,#66808,#66809,#66810,
#66811,#66812,#66813,#66814,#66815,#66816,#66817,#66818,#66819,#66820,#66821,
#66822,#66823,#66824,#66825,#66826,#66827,#66828,#66829,#66830,#66831,#66832,
#66833,#66834,#66835,#66836,#66837,#66838,#66839,#66840,#66841,#66842,#66843,
#66844,#66845,#66846,#66847,#66848,#66849,#66850,#66851,#66852,#66853,#66854,
#66855,#66856,#66857,#66858,#66859,#66860,#66861,#66862,#66863,#66864,#66865,
#66866,#66867,#66868,#66869,#66870,#66871,#66872,#66873,#66874,#66875,#66876,
#66877,#66878,#66879,#66880,#66881,#66882,#66883,#66884,#66885,#66886,#66887,
#66888,#66889,#66890,#66891,#66892,#66893,#66894,#66895,#66896,#66897,#66898,
#66899,#66900,#66901,#66902,#66903,#66904,#66905,#66906,#66907,#66908,#66909,
#66910,#66911,#66912,#66913,#66914,#66915,#66916,#66917,#66918,#66919,#66920,
#66921,#66922,#66923,#66924,#66925,#66926,#66927,#66928,#66929,#66930,#66931,
#66932,#66933,#66934,#66935,#66936,#66937,#66938,#66939,#66940,#66941,#66942,
#66943,#66944,#66945,#66946,#66947,#66948,#66949,#66950,#66951,#66952,#66953,
#66954,#66955,#66956,#66957,#66958,#66959,#66960,#66961,#66962,#66963,#66964,
#66965,#66966,#66967,#66968,#66969,#66970,#66971,#66972,#66973,#66974,#66975,
#66976,#66977,#66978,#66979,#66980,#66981,#66982,#66983,#66984,#66985,#66986,
#66987,#66988,#66989,#66990,#66991,#66992,#66993,#66994,#66995,#66996,#66997,
#66998,#66999,#67000,#67001,#67002,#67003,#67004,#67005,#67006,#67007,#67008,
#67009,#67010,#67011,#67012,#67013,#67014,#67015,#67016,#67017,#67018,#67019,
#67020,#67021,#67022,#67023,#67024,#67025,#67026,#67027,#67028,#67029,#67030,
#67031,#67032,#67033,#67034,#67035,#67036,#67037,#67038,#67039,#67040,#67041,
#67042,#67043,#67044,#67045,#67046,#67047,#67048,#67049,#67050,#67051,#67052,
#67053,#67054,#67055,#67056,#67057,#67058,#67059,#67060,#67061,#67062,#67063,
#67064,#67065,#67066,#67067,#67068,#67069,#67070,#67071,#67072,#67073,#67074,
#67075,#67076,#67077,#67078,#67079,#67080,#67081,#67082,#67083,#67084,#67085,
#67086,#67087,#67088,#67089,#67090,#67091,#67092,#67093,#67094,#67095,#67096,
#67097,#67098,#67099,#67100,#67101,#67102,#67103,#67104,#67105,#67106,#67107,
#67108,#67109,#67110,#67111,#67112,#67113,#67114,#67115,#67116,#67117,#67118,
#67119,#67120,#67121,#67122,#67123,#67124,#67125,#67126,#67127,#67128,#67129,
#67130,#67131,#67132,#67133,#67134,#67135,#67136,#67137,#67138,#67139,#67140,
#67141,#67142,#67143,#67144,#67145,#67146,#67147,#67148,#67149,#67150,#67151,
#67152,#67153,#67154,#67155,#67156,#67157,#67158,#67159,#67160,#67161,#67162,
#67163,#67164,#67165,#67166,#67167,#67168,#67169,#67170,#67171,#67172,#67173,
#67174,#67175,#67176,#67177,#67178,#67179,#67180,#67181,#67182,#67183,#67184,
#67185,#67186,#67187,#67188,#67189,#67190,#67191,#67192,#67193,#67194,#67195,
#67196,#67197,#67198,#67199,#67200,#67201,#67202,#67203,#67204,#67205,#67206,
#67207,#67208,#67209,#67210,#67211,#67212,#67213,#67214,#67215,#67216,#67217,
#67218,#67219,#67220,#67221,#67222,#67223,#67224,#67225,#67226,#67227,#67228,
#67229,#67230,#67231,#67232,#67233,#67234,#67235,#67236,#67237,#67238,#67239,
#67240,#67241,#67242,#67243,#67244,#67245,#67246,#67247,#67248,#67249,#67250,
#67251,#67252,#67253,#67254,#67255,#67256,#67257,#67258,#67259,#67260,#67261,
#67262,#67263,#67264,#67265,#67266,#67267,#67268,#67269,#67270,#67271,#67272,
#67273,#67274,#67275,#67276,#67277,#67278,#67279,#67280,#67281,#67282,#67283,
#67284,#67285,#67286,#67287,#67288,#67289,#67290,#67291,#67292,#67293,#67294,
#67295,#67296,#67297,#67298,#67299,#67300,#67301,#67302,#67303,#67304,#67305,
#67306,#67307,#67308,#67309,#67310,#67311,#67312,#67313,#67314,#67315,#67316,
#67317,#67318,#67319,#67320,#67321,#67322,#67323,#67324,#67325,#67326,#67327,
#67328,#67329,#67330,#67331,#67332,#67333,#67334,#67335,#67336,#67337,#67338,
#67339,#67340,#67341,#67342,#67343,#67344,#67345,#67346,#67347,#67348,#67349,
#67350,#67351,#67352,#67353,#67354,#67355,#67356,#67357,#67358,#67359,#67360,
#67361,#67362,#67363,#67364,#67365,#67366,#67367,#67368,#67369,#67370,#67371,
#67372,#67373,#67374,#67375,#67376,#67377,#67378,#67379,#67380,#67381,#67382,
#67383,#67384,#67385,#67386,#67387,#67388,#67389,#67390,#67391,#67392,#67393,
#67394,#67395,#67396,#67397,#67398,#67399,#67400,#67401,#67402,#67403,#67404,
#67405,#67406,#67407,#67408,#67409,#67410,#67411,#67412,#67413,#67414,#67415,
#67416,#67417,#67418,#67419,#67420,#67421,#67422,#67423,#67424,#67425,#67426,
#67427,#67428,#67429,#67430,#67431,#67432,#67433,#67434,#67435,#67436,#67437,
#67438,#67439,#67440,#67441,#67442,#67443,#67444,#67445,#67446,#67447,#67448,
#67449,#67450,#67451,#67452,#67453,#67454,#67455,#67456,#67457,#67458,#67459,
#67460,#67461,#67462,#67463,#67464,#67465,#67466,#67467,#67468,#67469,#67470,
#67471,#67472,#67473,#67474,#67475,#67476,#67477,#67478,#67479,#67480,#67481,
#67482,#67483,#67484,#67485,#67486,#67487,#67488,#67489,#67490,#67491,#67492,
#67493,#67494,#67495,#67496,#67497,#67498,#67499,#67500,#67501,#67502,#67503,
#67504,#67505,#67506,#67507,#67508,#67509,#67510,#67511,#67512,#67513,#67514,
#67515,#67516,#67517,#67518,#67519,#67520,#67521,#67522,#67523,#67524,#67525,
#67526,#67527,#67528,#67529,#67530,#67531,#67532,#67533,#67534,#67535,#67536,
#67537,#67538,#67539,#67540,#67541,#67542,#67543,#67544,#67545,#67546,#67547,
#67548,#67549,#67550,#67551,#67552,#67553,#67554,#67555,#67556,#67557,#67558,
#67559,#67560,#67561,#67562,#67563,#67564,#67565,#67566,#67567,#67568,#67569,
#67570,#67571,#67572,#67573,#67574,#67575,#67576,#67577,#67578,#67579,#67580,
#67581,#67582,#67583,#67584,#67585,#67586,#67587,#67588,#67589,#67590,#67591,
#67592,#67593,#67594,#67595,#67596,#67597,#67598,#67599,#67600,#67601,#67602,
#67603,#67604,#67605,#67606,#67607,#67608,#67609,#67610,#67611,#67612,#67613,
#67614,#67615,#67616,#67617,#67618,#67619,#67620,#67621,#67622,#67623,#67624,
#67625,#67626,#67627,#67628,#67629,#67630,#67631,#67632,#67633,#67634,#67635,
#67636,#67637,#67638,#67639,#67640,#67641,#67642,#67643,#67644,#67645,#67646,
#67647,#67648,#67649,#67650,#67651,#67652,#67653,#67654,#67655,#67656,#67657,
#67658,#67659,#67660,#67661,#67662,#67663,#67664,#67665,#67666,#67667,#67668,
#67669,#67670,#67671,#67672,#67673,#67674,#67675,#67676,#67677,#67678,#67679,
#67680,#67681,#67682,#67683,#67684,#67685,#67686,#67687,#67688,#67689,#67690,
#67691,#67692,#67693,#67694,#67695,#67696,#67697,#67698,#67699,#67700,#67701,
#67702,#67703,#67704,#67705,#67706,#67707,#67708,#67709,#67710,#67711,#67712,
#67713,#67714,#67715,#67716,#67717,#67718,#67719,#67720,#67721,#67722,#67723,
#67724,#67725,#67726,#67727,#67728,#67729,#67730,#67731,#67732,#67733,#67734,
#67735,#67736,#67737,#67738,#67739,#67740,#67741,#67742,#67743,#67744,#67745,
#67746,#67747,#67748,#67749,#67750,#67751,#67752,#67753,#67754,#67755,#67756,
#67757,#67758,#67759,#67760,#67761,#67762,#67763,#67764,#67765,#67766,#67767,
#67768,#67769,#67770,#67771,#67772,#67773,#67774,#67775,#67776,#67777,#67778,
#67779,#67780,#67781,#67782,#67783,#67784,#67785,#67786,#67787,#67788,#67789,
#67790,#67791,#67792,#67793,#67794,#67795,#67796,#67797,#67798,#67799,#67800,
#67801,#67802,#67803,#67804,#67805,#67806,#67807,#67808,#67809,#67810,#67811,
#67812,#67813,#67814,#67815,#67816,#67817,#67818,#67819,#67820,#67821,#67822,
#67823,#67824,#67825,#67826,#67827,#67828,#67829,#67830,#67831,#67832,#67833,
#67834,#67835,#67836,#67837,#67838,#67839,#67840,#67841,#67842,#67843,#67844,
#67845,#67846,#67847,#67848,#67849,#67850,#67851,#67852,#67853,#67854,#67855,
#67856,#67857,#67858,#67859,#67860,#67861,#67862,#67863,#67864,#67865,#67866,
#67867,#67868,#67869,#67870,#67871,#67872,#67873,#67874,#67875,#67876,#67877,
#67878,#67879,#67880,#67881,#67882,#67883,#67884,#67885,#67886,#67887,#67888,
#67889,#67890,#67891,#67892,#67893,#67894,#67895,#67896,#67897,#67898,#67899,
#67900,#67901,#67902,#67903,#67904,#67905,#67906,#67907,#67908,#67909,#67910,
#67911,#67912,#67913,#67914,#67915,#67916,#67917,#67918,#67919,#67920,#67921,
#67922,#67923,#67924,#67925,#67926,#67927,#67928,#67929,#67930,#67931,#67932,
#67933,#67934,#67935,#67936,#67937,#67938,#67939,#67940,#67941,#67942,#67943,
#67944,#67945,#67946,#67947,#67948,#67949,#67950,#67951,#67952,#67953,#67954,
#67955,#67956,#67957,#67958,#67959,#67960,#67961,#67962,#67963,#67964,#67965,
#67966,#67967,#67968,#67969,#67970,#67971,#67972,#67973,#67974,#67975,#67976,
#67977,#67978,#67979,#67980,#67981,#67982,#67983,#67984,#67985,#67986,#67987,
#67988,#67989,#67990,#67991,#67992,#67993,#67994,#67995,#67996,#67997,#67998,
#67999,#68000,#68001,#68002,#68003,#68004,#68005,#68006,#68007,#68008,#68009,
#68010,#68011,#68012,#68013,#68014,#68015,#68016,#68017,#68018,#68019,#68020,
#68021,#68022,#68023,#68024,#68025,#68026,#68027,#68028,#68029,#68030,#68031,
#68032,#68033,#68034,#68035,#68036,#68037,#68038,#68039,#68040,#68041,#68042,
#68043,#68044,#68045,#68046,#68047,#68048,#68049,#68050,#68051,#68052,#68053,
#68054,#68055,#68056,#68057,#68058,#68059,#68060,#68061,#68062,#68063,#68064,
#68065,#68066,#68067,#68068,#68069,#68070,#68071,#68072,#68073,#68074,#68075,
#68076,#68077,#68078,#68079,#68080,#68081,#68082,#68083,#68084,#68085,#68086,
#68087,#68088,#68089,#68090,#68091,#68092,#68093,#68094,#68095,#68096,#68097,
#68098,#68099,#68100,#68101,#68102,#68103,#68104,#68105,#68106,#68107,#68108,
#68109,#68110,#68111,#68112,#68113,#68114,#68115,#68116,#68117,#68118,#68119,
#68120,#68121,#68122,#68123,#68124,#68125,#68126,#68127,#68128,#68129,#68130,
#68131,#68132,#68133,#68134,#68135,#68136,#68137,#68138,#68139,#68140,#68141,
#68142,#68143,#68144,#68145,#68146,#68147,#68148,#68149,#68150,#68151,#68152,
#68153,#68154,#68155,#68156,#68157,#68158,#68159,#68160,#68161,#68162,#68163,
#68164,#68165,#68166,#68167,#68168,#68169,#68170,#68171,#68172,#68173,#68174,
#68175,#68176,#68177,#68178,#68179,#68180,#68181,#68182,#68183,#68184,#68185,
#68186,#68187,#68188,#68189,#68190,#68191,#68192,#68193,#68194,#68195,#68196,
#68197,#68198,#68199,#68200,#68201,#68202,#68203,#68204,#68205,#68206,#68207,
#68208,#68209,#68210,#68211,#68212,#68213,#68214,#68215,#68216,#68217,#68218,
#68219,#68220,#68221,#68222,#68223,#68224,#68225,#68226,#68227,#68228,#68229,
#68230,#68231,#68232,#68233,#68234,#68235,#68236,#68237,#68238,#68239,#68240,
#68241,#68242,#68243,#68244,#68245,#68246,#68247,#68248,#68249,#68250,#68251,
#68252,#68253,#68254,#68255,#68256,#68257,#68258,#68259,#68260,#68261,#68262,
#68263,#68264,#68265,#68266,#68267,#68268,#68269,#68270,#68271,#68272,#68273,
#68274,#68275,#68276,#68277,#68278,#68279,#68280,#68281,#68282,#68283,#68284,
#68285,#68286,#68287,#68288,#68289,#68290,#68291,#68292,#68293,#68294,#68295,
#68296,#68297,#68298,#68299,#68300,#68301,#68302,#68303,#68304,#68305,#68306,
#68307,#68308,#68309,#68310,#68311,#68312,#68313,#68314,#68315,#68316,#68317,
#68318,#68319,#68320,#68321,#68322,#68323,#68324,#68325,#68326,#68327,#68328,
#68329,#68330,#68331,#68332,#68333,#68334,#68335,#68336,#68337,#68338,#68339,
#68340,#68341,#68342,#68343,#68344,#68345,#68346,#68347,#68348,#68349,#68350,
#68351,#68352,#68353,#68354,#68355,#68356,#68357,#68358,#68359,#68360,#68361,
#68362,#68363,#68364,#68365,#68366,#68367,#68368,#68369,#68370,#68371,#68372,
#68373,#68374,#68375,#68376,#68377,#68378,#68379,#68380,#68381,#68382,#68383,
#68384,#68385,#68386,#68387,#68388,#68389,#68390,#68391,#68392,#68393,#68394,
#68395,#68396,#68397,#68398,#68399,#68400,#68401,#68402,#68403,#68404,#68405,
#68406,#68407,#68408,#68409,#68410,#68411,#68412,#68413,#68414,#68415,#68416,
#68417,#68418,#68419,#68420,#68421,#68422,#68423,#68424,#68425,#68426,#68427,
#68428,#68429,#68430,#68431,#68432,#68433,#68434,#68435,#68436,#68437,#68438,
#68439,#68440,#68441,#68442,#68443,#68444,#68445,#68446,#68447,#68448,#68449,
#68450,#68451,#68452,#68453,#68454,#68455,#68456,#68457,#68458,#68459,#68460,
#68461,#68462,#68463,#68464,#68465,#68466,#68467,#68468,#68469,#68470,#68471,
#68472,#68473,#68474,#68475,#68476,#68477,#68478,#68479,#68480,#68481,#68482,
#68483,#68484,#68485,#68486,#68487,#68488,#68489,#68490,#68491,#68492,#68493,
#68494,#68495,#68496,#68497,#68498,#68499,#68500,#68501,#68502,#68503,#68504,
#68505,#68506,#68507,#68508,#68509,#68510,#68511,#68512,#68513,#68514,#68515,
#68516,#68517,#68518,#68519,#68520,#68521,#68522,#68523,#68524,#68525,#68526,
#68527,#68528,#68529,#68530,#68531,#68532,#68533,#68534,#68535,#68536,#68537,
#68538,#68539,#68540,#68541,#68542,#68543,#68544,#68545,#68546,#68547,#68548,
#68549,#68550,#68551,#68552,#68553,#68554,#68555,#68556,#68557,#68558,#68559,
#68560,#68561,#68562,#68563,#68564,#68565,#68566,#68567,#68568,#68569,#68570,
#68571,#68572,#68573,#68574,#68575,#68576,#68577,#68578,#68579,#68580,#68581,
#68582,#68583,#68584,#68585,#68586,#68587,#68588,#68589,#68590,#68591,#68592,
#68593,#68594,#68595,#68596,#68597,#68598,#68599,#68600,#68601,#68602,#68603,
#68604,#68605,#68606,#68607,#68608,#68609,#68610,#68611,#68612,#68613,#68614,
#68615,#68616,#68617,#68618,#68619,#68620,#68621,#68622,#68623,#68624,#68625,
#68626,#68627,#68628,#68629,#68630,#68631,#68632,#68633,#68634,#68635,#68636,
#68637,#68638,#68639,#68640,#68641,#68642,#68643,#68644,#68645,#68646,#68647,
#68648,#68649,#68650,#68651,#68652,#68653,#68654,#68655,#68656,#68657,#68658,
#68659,#68660,#68661,#68662,#68663,#68664,#68665,#68666,#68667,#68668,#68669,
#68670,#68671,#68672,#68673,#68674,#68675,#68676,#68677,#68678,#68679,#68680,
#68681,#68682,#68683,#68684,#68685,#68686,#68687,#68688,#68689,#68690,#68691,
#68692,#68693,#68694,#68695,#68696,#68697,#68698,#68699,#68700,#68701,#68702,
#68703,#68704,#68705,#68706,#68707,#68708,#68709,#68710,#68711,#68712,#68713,
#68714,#68715,#68716,#68717,#68718,#68719,#68720,#68721,#68722,#68723,#68724,
#68725,#68726,#68727,#68728,#68729,#68730,#68731,#68732,#68733,#68734,#68735,
#68736,#68737,#68738,#68739,#68740,#68741,#68742,#68743,#68744,#68745,#68746,
#68747,#68748,#68749,#68750,#68751,#68752,#68753,#68754,#68755,#68756,#68757,
#68758,#68759,#68760,#68761,#68762,#68763,#68764,#68765,#68766,#68767,#68768,
#68769,#68770,#68771,#68772,#68773,#68774,#68775,#68776,#68777,#68778,#68779,
#68780,#68781,#68782,#68783,#68784,#68785,#68786,#68787,#68788,#68789,#68790,
#68791,#68792,#68793,#68794,#68795,#68796,#68797,#68798,#68799,#68800,#68801,
#68802,#68803,#68804,#68805,#68806,#68807,#68808,#68809,#68810,#68811,#68812,
#68813,#68814,#68815,#68816,#68817,#68818,#68819,#68820,#68821,#68822,#68823,
#68824,#68825,#68826,#68827,#68828,#68829,#68830,#68831,#68832,#68833,#68834,
#68835,#68836,#68837,#68838,#68839,#68840,#68841,#68842,#68843,#68844,#68845,
#68846,#68847,#68848,#68849,#68850,#68851,#68852,#68853,#68854,#68855,#68856,
#68857,#68858,#68859,#68860,#68861,#68862,#68863,#68864,#68865,#68866,#68867,
#68868,#68869,#68870,#68871,#68872,#68873,#68874,#68875,#68876,#68877,#68878,
#68879,#68880,#68881,#68882,#68883,#68884,#68885,#68886,#68887,#68888,#68889,
#68890,#68891,#68892,#68893,#68894,#68895,#68896,#68897,#68898,#68899,#68900,
#68901,#68902,#68903,#68904,#68905,#68906,#68907,#68908,#68909,#68910,#68911,
#68912,#68913,#68914,#68915,#68916,#68917,#68918,#68919,#68920,#68921,#68922,
#68923,#68924,#68925,#68926,#68927,#68928,#68929,#68930,#68931,#68932,#68933,
#68934,#68935,#68936,#68937,#68938,#68939,#68940,#68941,#68942,#68943,#68944,
#68945,#68946,#68947,#68948,#68949,#68950,#68951,#68952,#68953,#68954,#68955,
#68956,#68957,#68958,#68959,#68960,#68961,#68962,#68963,#68964,#68965,#68966,
#68967,#68968,#68969,#68970,#68971,#68972,#68973,#68974,#68975,#68976,#68977,
#68978,#68979,#68980,#68981,#68982,#68983,#68984,#68985,#68986,#68987,#68988,
#68989,#68990,#68991,#68992,#68993,#68994,#68995,#68996,#68997,#68998,#68999,
#69000,#69001,#69002,#69003,#69004,#69005,#69006,#69007,#69008,#69009,#69010,
#69011,#69012,#69013,#69014,#69015,#69016,#69017,#69018,#69019,#69020,#69021,
#69022,#69023,#69024,#69025,#69026,#69027,#69028,#69029,#69030,#69031,#69032,
#69033,#69034,#69035,#69036,#69037,#69038,#69039,#69040,#69041,#69042,#69043,
#69044,#69045,#69046,#69047,#69048,#69049,#69050,#69051,#69052,#69053,#69054,
#69055,#69056,#69057,#69058,#69059,#69060,#69061,#69062,#69063,#69064,#69065,
#69066,#69067,#69068,#69069,#69070,#69071,#69072,#69073,#69074,#69075,#69076,
#69077,#69078,#69079,#69080,#69081,#69082,#69083,#69084,#69085,#69086,#69087,
#69088,#69089,#69090,#69091,#69092,#69093,#69094,#69095,#69096,#69097,#69098,
#69099,#69100,#69101,#69102,#69103,#69104,#69105,#69106,#69107,#69108,#69109,
#69110,#69111,#69112,#69113,#69114,#69115,#69116,#69117,#69118,#69119,#69120,
#69121,#69122,#69123,#69124,#69125,#69126,#69127,#69128,#69129,#69130,#69131,
#69132,#69133,#69134,#69135,#69136,#69137,#69138,#69139,#69140,#69141,#69142,
#69143,#69144,#69145,#69146,#69147,#69148,#69149,#69150,#69151,#69152,#69153,
#69154,#69155,#69156,#69157,#69158,#69159,#69160,#69161,#69162,#69163,#69164,
#69165,#69166,#69167,#69168,#69169,#69170,#69171,#69172,#69173,#69174,#69175,
#69176,#69177,#69178,#69179,#69180,#69181,#69182,#69183,#69184,#69185,#69186,
#69187,#69188,#69189,#69190,#69191,#69192,#69193,#69194,#69195,#69196,#69197,
#69198,#69199,#69200,#69201,#69202,#69203,#69204,#69205,#69206,#69207,#69208,
#69209,#69210,#69211,#69212,#69213,#69214,#69215,#69216,#69217,#69218,#69219,
#69220,#69221,#69222,#69223,#69224,#69225,#69226,#69227,#69228,#69229,#69230,
#69231,#69232,#69233,#69234,#69235,#69236,#69237,#69238,#69239,#69240,#69241,
#69242,#69243,#69244,#69245,#69246,#69247,#69248,#69249,#69250,#69251,#69252,
#69253,#69254,#69255,#69256,#69257,#69258,#69259,#69260,#69261,#69262,#69263,
#69264,#69265,#69266,#69267,#69268,#69269,#69270,#69271,#69272,#69273,#69274,
#69275,#69276,#69277,#69278,#69279,#69280,#69281,#69282,#69283,#69284,#69285,
#69286,#69287,#69288,#69289,#69290,#69291,#69292,#69293,#69294,#69295,#69296,
#69297,#69298,#69299,#69300,#69301,#69302,#69303,#69304,#69305,#69306,#69307,
#69308,#69309,#69310,#69311,#69312,#69313,#69314,#69315,#69316,#69317,#69318,
#69319,#69320,#69321,#69322,#69323,#69324,#69325,#69326,#69327,#69328,#69329,
#69330,#69331,#69332,#69333,#69334,#69335,#69336,#69337,#69338,#69339,#69340,
#69341,#69342,#69343,#69344,#69345,#69346,#69347,#69348,#69349,#69350,#69351,
#69352,#69353,#69354,#69355,#69356,#69357,#69358,#69359,#69360,#69361,#69362,
#69363,#69364,#69365,#69366,#69367,#69368,#69369,#69370,#69371,#69372,#69373,
#69374,#69375,#69376,#69377,#69378,#69379,#69380,#69381,#69382,#69383,#69384,
#69385,#69386,#69387,#69388,#69389,#69390,#69391,#69392,#69393,#69394,#69395,
#69396,#69397,#69398,#69399,#69400,#69401,#69402,#69403,#69404,#69405,#69406,
#69407,#69408,#69409,#69410,#69411,#69412,#69413,#69414,#69415,#69416,#69417,
#69418,#69419,#69420,#69421,#69422,#69423,#69424,#69425,#69426,#69427,#69428,
#69429,#69430,#69431,#69432,#69433,#69434,#69435,#69436,#69437,#69438,#69439,
#69440,#69441,#69442,#69443,#69444,#69445,#69446,#69447,#69448,#69449,#69450,
#69451,#69452,#69453,#69454,#69455,#69456,#69457,#69458,#69459,#69460,#69461,
#69462,#69463,#69464,#69465,#69466,#69467,#69468,#69469,#69470,#69471,#69472,
#69473,#69474,#69475,#69476,#69477,#69478,#69479,#69480,#69481,#69482,#69483,
#69484,#69485,#69486,#69487,#69488,#69489,#69490,#69491,#69492,#69493,#69494,
#69495,#69496,#69497,#69498,#69499,#69500,#69501,#69502,#69503,#69504,#69505,
#69506,#69507,#69508,#69509,#69510,#69511,#69512,#69513,#69514,#69515,#69516,
#69517,#69518,#69519,#69520,#69521,#69522,#69523,#69524,#69525,#69526,#69527,
#69528,#69529,#69530,#69531,#69532,#69533,#69534,#69535,#69536,#69537,#69538,
#69539,#69540,#69541,#69542,#69543,#69544,#69545,#69546,#69547,#69548,#69549,
#69550,#69551,#69552,#69553,#69554,#69555,#69556,#69557,#69558,#69559,#69560,
#69561,#69562,#69563,#69564,#69565,#69566,#69567,#69568,#69569,#69570,#69571,
#69572,#69573,#69574,#69575,#69576,#69577,#69578,#69579,#69580,#69581,#69582,
#69583,#69584,#69585,#69586,#69587,#69588,#69589,#69590,#69591,#69592,#69593,
#69594,#69595,#69596,#69597,#69598,#69599,#69600,#69601,#69602,#69603,#69604,
#69605,#69606,#69607,#69608,#69609,#69610,#69611,#69612,#69613,#69614,#69615,
#69616,#69617,#69618,#69619,#69620,#69621,#69622,#69623,#69624,#69625,#69626,
#69627,#69628,#69629,#69630,#69631,#69632,#69633,#69634,#69635,#69636,#69637,
#69638,#69639,#69640,#69641,#69642,#69643,#69644,#69645,#69646,#69647,#69648,
#69649,#69650,#69651,#69652,#69653,#69654,#69655,#69656,#69657,#69658,#69659,
#69660,#69661,#69662,#69663,#69664,#69665,#69666,#69667,#69668,#69669,#69670,
#69671,#69672,#69673,#69674,#69675,#69676,#69677,#69678,#69679,#69680,#69681,
#69682,#69683,#69684,#69685,#69686,#69687,#69688,#69689,#69690,#69691,#69692,
#69693,#69694,#69695,#69696,#69697,#69698,#69699,#69700,#69701,#69702,#69703,
#69704,#69705,#69706,#69707,#69708,#69709,#69710,#69711,#69712,#69713,#69714,
#69715,#69716,#69717,#69718,#69719,#69720,#69721,#69722,#69723,#69724,#69725,
#69726,#69727,#69728,#69729,#69730,#69731,#69732,#69733,#69734,#69735,#69736,
#69737,#69738,#69739,#69740,#69741,#69742,#69743,#69744,#69745,#69746,#69747,
#69748,#69749,#69750,#69751,#69752,#69753,#69754,#69755,#69756,#69757,#69758,
#69759,#69760,#69761,#69762,#69763,#69764,#69765,#69766,#69767,#69768,#69769,
#69770,#69771,#69772,#69773,#69774,#69775,#69776,#69777,#69778,#69779,#69780,
#69781,#69782,#69783,#69784,#69785,#69786,#69787,#69788,#69789,#69790,#69791,
#69792,#69793,#69794,#69795,#69796,#69797,#69798,#69799,#69800,#69801,#69802,
#69803,#69804,#69805,#69806,#69807,#69808,#69809,#69810,#69811,#69812,#69813,
#69814,#69815,#69816,#69817,#69818,#69819,#69820,#69821,#69822,#69823,#69824,
#69825,#69826,#69827,#69828,#69829,#69830,#69831,#69832,#69833,#69834,#69835,
#69836,#69837,#69838,#69839,#69840,#69841,#69842,#69843,#69844,#69845,#69846,
#69847,#69848,#69849,#69850,#69851,#69852,#69853,#69854,#69855,#69856,#69857,
#69858,#69859,#69860,#69861,#69862,#69863,#69864,#69865,#69866,#69867,#69868,
#69869,#69870,#69871,#69872,#69873,#69874,#69875,#69876,#69877,#69878,#69879,
#69880,#69881,#69882,#69883,#69884,#69885,#69886,#69887,#69888,#69889,#69890,
#69891,#69892,#69893,#69894,#69895,#69896,#69897,#69898,#69899,#69900,#69901,
#69902,#69903,#69904,#69905,#69906,#69907,#69908,#69909,#69910,#69911,#69912,
#69913,#69914,#69915,#69916,#69917,#69918,#69919,#69920,#69921,#69922,#69923,
#69924,#69925,#69926,#69927,#69928,#69929,#69930,#69931,#69932,#69933,#69934,
#69935,#69936,#69937,#69938,#69939,#69940,#69941,#69942,#69943,#69944,#69945,
#69946,#69947,#69948,#69949,#69950,#69951,#69952,#69953,#69954,#69955,#69956,
#69957,#69958,#69959,#69960,#69961,#69962,#69963,#69964,#69965,#69966,#69967,
#69968,#69969,#69970,#69971,#69972,#69973,#69974,#69975,#69976,#69977,#69978,
#69979,#69980,#69981,#69982,#69983,#69984,#69985,#69986,#69987,#69988,#69989,
#69990,#69991,#69992,#69993,#69994,#69995,#69996,#69997,#69998,#69999,#70000,
#70001,#70002,#70003,#70004,#70005,#70006,#70007,#70008,#70009,#70010,#70011,
#70012,#70013,#70014,#70015,#70016,#70017,#70018,#70019,#70020,#70021,#70022,
#70023,#70024,#70025,#70026,#70027,#70028,#70029,#70030,#70031,#70032,#70033,
#70034,#70035,#70036,#70037,#70038,#70039,#70040,#70041,#70042,#70043,#70044,
#70045,#70046,#70047,#70048,#70049,#70050,#70051,#70052,#70053,#70054,#70055,
#70056,#70057,#70058,#70059,#70060,#70061,#70062,#70063,#70064,#70065,#70066,
#70067,#70068,#70069,#70070,#70071,#70072,#70073,#70074,#70075,#70076,#70077,
#70078,#70079,#70080,#70081,#70082,#70083,#70084,#70085,#70086,#70087,#70088,
#70089,#70090,#70091,#70092,#70093,#70094,#70095,#70096,#70097,#70098,#70099,
#70100,#70101,#70102,#70103,#70104,#70105,#70106,#70107,#70108,#70109,#70110,
#70111,#70112,#70113,#70114,#70115,#70116,#70117,#70118,#70119,#70120,#70121,
#70122,#70123,#70124,#70125,#70126,#70127,#70128,#70129,#70130,#70131,#70132,
#70133,#70134,#70135,#70136,#70137,#70138,#70139,#70140,#70141,#70142,#70143,
#70144,#70145,#70146,#70147,#70148,#70149,#70150,#70151,#70152,#70153,#70154,
#70155,#70156,#70157,#70158,#70159,#70160,#70161,#70162,#70163,#70164,#70165,
#70166,#70167,#70168,#70169,#70170,#70171,#70172,#70173,#70174,#70175,#70176,
#70177,#70178,#70179,#70180,#70181,#70182,#70183,#70184,#70185,#70186,#70187,
#70188,#70189,#70190,#70191,#70192,#70193,#70194,#70195,#70196,#70197,#70198,
#70199,#70200,#70201,#70202,#70203,#70204,#70205,#70206,#70207,#70208,#70209,
#70210,#70211,#70212,#70213,#70214,#70215,#70216,#70217,#70218,#70219,#70220,
#70221,#70222,#70223,#70224,#70225,#70226,#70227,#70228,#70229,#70230,#70231,
#70232,#70233,#70234,#70235,#70236,#70237,#70238,#70239,#70240,#70241,#70242,
#70243,#70244,#70245,#70246,#70247,#70248,#70249,#70250,#70251,#70252,#70253,
#70254,#70255,#70256,#70257,#70258,#70259,#70260,#70261,#70262,#70263,#70264,
#70265,#70266,#70267,#70268,#70269,#70270,#70271,#70272,#70273,#70274,#70275,
#70276,#70277,#70278,#70279,#70280,#70281,#70282,#70283,#70284,#70285,#70286,
#70287,#70288,#70289,#70290,#70291,#70292,#70293,#70294,#70295,#70296,#70297,
#70298,#70299,#70300,#70301,#70302,#70303,#70304,#70305,#70306,#70307,#70308,
#70309,#70310,#70311,#70312,#70313,#70314,#70315,#70316,#70317,#70318,#70319,
#70320,#70321,#70322,#70323,#70324,#70325,#70326,#70327,#70328,#70329,#70330,
#70331,#70332,#70333,#70334,#70335,#70336,#70337,#70338,#70339,#70340,#70341,
#70342,#70343,#70344,#70345,#70346,#70347,#70348,#70349,#70350,#70351,#70352,
#70353,#70354,#70355,#70356,#70357,#70358,#70359,#70360,#70361,#70362,#70363,
#70364,#70365,#70366,#70367,#70368,#70369,#70370,#70371,#70372,#70373,#70374,
#70375,#70376,#70377,#70378,#70379,#70380,#70381,#70382,#70383,#70384,#70385,
#70386,#70387,#70388,#70389,#70390,#70391,#70392,#70393,#70394,#70395,#70396,
#70397,#70398,#70399,#70400,#70401,#70402,#70403,#70404,#70405,#70406,#70407,
#70408,#70409,#70410,#70411,#70412,#70413,#70414,#70415,#70416,#70417,#70418,
#70419,#70420,#70421,#70422,#70423,#70424,#70425,#70426,#70427,#70428,#70429,
#70430,#70431,#70432,#70433,#70434,#70435,#70436,#70437,#70438,#70439,#70440,
#70441,#70442,#70443,#70444,#70445,#70446,#70447,#70448,#70449,#70450,#70451,
#70452,#70453,#70454,#70455,#70456,#70457,#70458,#70459,#70460,#70461,#70462,
#70463,#70464,#70465,#70466,#70467,#70468,#70469,#70470,#70471,#70472,#70473,
#70474,#70475,#70476,#70477,#70478,#70479,#70480,#70481,#70482,#70483,#70484,
#70485,#70486,#70487,#70488,#70489,#70490,#70491,#70492,#70493,#70494,#70495,
#70496,#70497,#70498,#70499,#70500,#70501,#70502,#70503,#70504,#70505,#70506,
#70507,#70508,#70509,#70510,#70511,#70512,#70513,#70514,#70515,#70516,#70517,
#70518,#70519,#70520,#70521,#70522,#70523,#70524,#70525,#70526,#70527,#70528,
#70529,#70530,#70531,#70532,#70533,#70534,#70535,#70536,#70537,#70538,#70539,
#70540,#70541,#70542,#70543,#70544,#70545,#70546,#70547,#70548,#70549,#70550,
#70551,#70552,#70553,#70554,#70555,#70556,#70557,#70558,#70559,#70560,#70561,
#70562,#70563,#70564,#70565,#70566,#70567,#70568,#70569,#70570,#70571,#70572,
#70573,#70574,#70575,#70576,#70577,#70578,#70579,#70580,#70581,#70582,#70583,
#70584,#70585,#70586,#70587,#70588,#70589,#70590,#70591,#70592,#70593,#70594,
#70595,#70596,#70597,#70598,#70599,#70600,#70601,#70602,#70603,#70604,#70605,
#70606,#70607,#70608,#70609,#70610,#70611,#70612,#70613,#70614,#70615,#70616,
#70617,#70618,#70619,#70620,#70621,#70622,#70623,#70624,#70625,#70626,#70627,
#70628,#70629,#70630,#70631,#70632,#70633,#70634,#70635,#70636,#70637,#70638,
#70639,#70640,#70641,#70642,#70643,#70644,#70645,#70646,#70647,#70648,#70649,
#70650,#70651,#70652,#70653,#70654,#70655,#70656,#70657,#70658,#70659,#70660,
#70661,#70662,#70663,#70664,#70665,#70666,#70667,#70668,#70669,#70670,#70671,
#70672,#70673,#70674,#70675,#70676,#70677,#70678,#70679,#70680,#70681,#70682,
#70683,#70684,#70685,#70686,#70687,#70688,#70689,#70690,#70691,#70692,#70693,
#70694,#70695,#70696,#70697,#70698,#70699,#70700,#70701,#70702,#70703,#70704,
#70705,#70706,#70707,#70708,#70709,#70710,#70711,#70712,#70713,#70714,#70715,
#70716,#70717,#70718,#70719,#70720,#70721,#70722,#70723,#70724,#70725,#70726,
#70727,#70728,#70729,#70730,#70731,#70732,#70733,#70734,#70735,#70736,#70737,
#70738,#70739,#70740,#70741,#70742,#70743,#70744,#70745,#70746,#70747,#70748,
#70749,#70750,#70751,#70752,#70753,#70754,#70755,#70756,#70757,#70758,#70759,
#70760,#70761,#70762,#70763,#70764,#70765,#70766,#70767,#70768,#70769,#70770,
#70771,#70772,#70773,#70774,#70775,#70776,#70777,#70778,#70779,#70780,#70781,
#70782,#70783,#70784,#70785,#70786,#70787,#70788,#70789,#70790,#70791,#70792,
#70793,#70794,#70795,#70796,#70797,#70798,#70799,#70800,#70801,#70802,#70803,
#70804,#70805,#70806,#70807,#70808,#70809,#70810,#70811,#70812,#70813,#70814,
#70815,#70816,#70817,#70818,#70819,#70820,#70821,#70822,#70823,#70824,#70825,
#70826,#70827,#70828,#70829,#70830,#70831,#70832,#70833,#70834,#70835,#70836,
#70837,#70838,#70839,#70840,#70841,#70842,#70843,#70844,#70845,#70846,#70847,
#70848,#70849,#70850,#70851,#70852,#70853,#70854,#70855,#70856,#70857,#70858,
#70859,#70860,#70861,#70862,#70863,#70864,#70865,#70866,#70867,#70868,#70869,
#70870,#70871,#70872,#70873,#70874,#70875,#70876,#70877,#70878,#70879,#70880,
#70881,#70882,#70883,#70884,#70885,#70886,#70887,#70888,#70889,#70890,#70891,
#70892,#70893,#70894,#70895,#70896,#70897,#70898,#70899,#70900,#70901,#70902,
#70903,#70904,#70905,#70906,#70907,#70908,#70909,#70910,#70911,#70912,#70913,
#70914,#70915,#70916,#70917,#70918,#70919,#70920,#70921,#70922,#70923,#70924,
#70925,#70926,#70927,#70928,#70929,#70930,#70931,#70932,#70933,#70934,#70935,
#70936,#70937,#70938,#70939,#70940,#70941,#70942,#70943,#70944,#70945,#70946,
#70947,#70948,#70949,#70950,#70951,#70952,#70953,#70954,#70955,#70956,#70957,
#70958,#70959,#70960,#70961,#70962,#70963,#70964,#70965,#70966,#70967,#70968,
#70969,#70970,#70971,#70972,#70973,#70974,#70975,#70976,#70977,#70978,#70979,
#70980,#70981,#70982,#70983,#70984,#70985,#70986,#70987,#70988,#70989,#70990,
#70991,#70992,#70993,#70994,#70995,#70996,#70997,#70998,#70999,#71000,#71001,
#71002,#71003,#71004,#71005,#71006,#71007,#71008,#71009,#71010,#71011,#71012,
#71013,#71014,#71015,#71016,#71017,#71018,#71019,#71020,#71021,#71022,#71023,
#71024,#71025,#71026,#71027,#71028,#71029,#71030,#71031,#71032,#71033,#71034,
#71035,#71036,#71037,#71038,#71039,#71040,#71041,#71042,#71043,#71044,#71045,
#71046,#71047,#71048,#71049,#71050,#71051,#71052,#71053,#71054,#71055,#71056,
#71057,#71058,#71059,#71060,#71061,#71062,#71063,#71064,#71065,#71066,#71067,
#71068,#71069,#71070,#71071,#71072,#71073,#71074,#71075,#71076,#71077,#71078,
#71079,#71080,#71081,#71082,#71083,#71084,#71085,#71086,#71087,#71088,#71089,
#71090,#71091,#71092,#71093,#71094,#71095,#71096,#71097,#71098,#71099,#71100,
#71101,#71102,#71103,#71104,#71105,#71106,#71107,#71108,#71109,#71110,#71111,
#71112,#71113,#71114,#71115,#71116,#71117,#71118,#71119,#71120,#71121,#71122,
#71123,#71124,#71125,#71126,#71127,#71128,#71129,#71130,#71131,#71132,#71133,
#71134,#71135,#71136,#71137,#71138,#71139,#71140,#71141,#71142,#71143,#71144,
#71145,#71146,#71147,#71148,#71149,#71150,#71151,#71152,#71153,#71154,#71155,
#71156,#71157,#71158,#71159,#71160,#71161,#71162,#71163,#71164,#71165,#71166,
#71167,#71168,#71169,#71170,#71171,#71172,#71173,#71174,#71175,#71176,#71177,
#71178,#71179,#71180,#71181,#71182,#71183,#71184,#71185,#71186,#71187,#71188,
#71189,#71190,#71191,#71192,#71193,#71194,#71195,#71196,#71197,#71198,#71199,
#71200,#71201,#71202,#71203,#71204,#71205,#71206,#71207,#71208,#71209,#71210,
#71211,#71212,#71213,#71214,#71215,#71216,#71217,#71218,#71219,#71220,#71221,
#71222,#71223,#71224,#71225,#71226,#71227,#71228,#71229,#71230,#71231,#71232,
#71233,#71234,#71235,#71236,#71237,#71238,#71239,#71240,#71241,#71242,#71243,
#71244,#71245,#71246,#71247,#71248,#71249,#71250,#71251,#71252,#71253,#71254,
#71255,#71256,#71257,#71258,#71259,#71260,#71261,#71262,#71263,#71264,#71265,
#71266,#71267,#71268,#71269,#71270,#71271,#71272,#71273,#71274,#71275,#71276,
#71277,#71278,#71279,#71280,#71281,#71282,#71283,#71284,#71285,#71286,#71287,
#71288,#71289,#71290,#71291,#71292,#71293,#71294,#71295,#71296,#71297,#71298,
#71299,#71300,#71301,#71302,#71303,#71304,#71305,#71306,#71307,#71308,#71309,
#71310,#71311,#71312,#71313,#71314,#71315,#71316,#71317,#71318,#71319,#71320,
#71321,#71322,#71323,#71324,#71325,#71326,#71327,#71328,#71329,#71330,#71331,
#71332,#71333,#71334));
#71472=AXIS2_PLACEMENT_3D('',#92436,#77765,#77766);
#71473=AXIS2_PLACEMENT_3D('',#92437,#77767,#77768);
#71474=AXIS2_PLACEMENT_3D('',#92460,#77770,#77771);
#71475=AXIS2_PLACEMENT_3D('',#92462,#77772,#77773);
#71476=AXIS2_PLACEMENT_3D('',#92500,#77774,#77775);
#71477=AXIS2_PLACEMENT_3D('',#92502,#77776,#77777);
#71478=AXIS2_PLACEMENT_3D('',#92540,#77778,#77779);
#71479=AXIS2_PLACEMENT_3D('',#92542,#77780,#77781);
#71480=AXIS2_PLACEMENT_3D('',#92580,#77782,#77783);
#71481=AXIS2_PLACEMENT_3D('',#92582,#77784,#77785);
#71482=AXIS2_PLACEMENT_3D('',#92620,#77786,#77787);
#71483=AXIS2_PLACEMENT_3D('',#92622,#77788,#77789);
#71484=AXIS2_PLACEMENT_3D('',#92660,#77790,#77791);
#71485=AXIS2_PLACEMENT_3D('',#92662,#77792,#77793);
#71486=AXIS2_PLACEMENT_3D('',#92700,#77794,#77795);
#71487=AXIS2_PLACEMENT_3D('',#92702,#77796,#77797);
#71488=AXIS2_PLACEMENT_3D('',#92740,#77798,#77799);
#71489=AXIS2_PLACEMENT_3D('',#92742,#77800,#77801);
#71490=AXIS2_PLACEMENT_3D('',#92780,#77802,#77803);
#71491=AXIS2_PLACEMENT_3D('',#92782,#77804,#77805);
#71492=AXIS2_PLACEMENT_3D('',#92820,#77806,#77807);
#71493=AXIS2_PLACEMENT_3D('',#92822,#77808,#77809);
#71494=AXIS2_PLACEMENT_3D('',#92860,#77810,#77811);
#71495=AXIS2_PLACEMENT_3D('',#92862,#77812,#77813);
#71496=AXIS2_PLACEMENT_3D('',#92900,#77814,#77815);
#71497=AXIS2_PLACEMENT_3D('',#92902,#77816,#77817);
#71498=AXIS2_PLACEMENT_3D('',#92940,#77818,#77819);
#71499=AXIS2_PLACEMENT_3D('',#92942,#77820,#77821);
#71500=AXIS2_PLACEMENT_3D('',#92980,#77822,#77823);
#71501=AXIS2_PLACEMENT_3D('',#92982,#77824,#77825);
#71502=AXIS2_PLACEMENT_3D('',#93020,#77826,#77827);
#71503=AXIS2_PLACEMENT_3D('',#93022,#77828,#77829);
#71504=AXIS2_PLACEMENT_3D('',#93060,#77830,#77831);
#71505=AXIS2_PLACEMENT_3D('',#93062,#77832,#77833);
#71506=AXIS2_PLACEMENT_3D('',#93100,#77834,#77835);
#71507=AXIS2_PLACEMENT_3D('',#93102,#77836,#77837);
#71508=AXIS2_PLACEMENT_3D('',#93140,#77838,#77839);
#71509=AXIS2_PLACEMENT_3D('',#93142,#77840,#77841);
#71510=AXIS2_PLACEMENT_3D('',#93180,#77842,#77843);
#71511=AXIS2_PLACEMENT_3D('',#93182,#77844,#77845);
#71512=AXIS2_PLACEMENT_3D('',#93220,#77846,#77847);
#71513=AXIS2_PLACEMENT_3D('',#93222,#77848,#77849);
#71514=AXIS2_PLACEMENT_3D('',#93260,#77850,#77851);
#71515=AXIS2_PLACEMENT_3D('',#93262,#77852,#77853);
#71516=AXIS2_PLACEMENT_3D('',#93300,#77854,#77855);
#71517=AXIS2_PLACEMENT_3D('',#93302,#77856,#77857);
#71518=AXIS2_PLACEMENT_3D('',#93340,#77858,#77859);
#71519=AXIS2_PLACEMENT_3D('',#93342,#77860,#77861);
#71520=AXIS2_PLACEMENT_3D('',#93380,#77862,#77863);
#71521=AXIS2_PLACEMENT_3D('',#93382,#77864,#77865);
#71522=AXIS2_PLACEMENT_3D('',#93420,#77866,#77867);
#71523=AXIS2_PLACEMENT_3D('',#93422,#77868,#77869);
#71524=AXIS2_PLACEMENT_3D('',#93460,#77870,#77871);
#71525=AXIS2_PLACEMENT_3D('',#93462,#77872,#77873);
#71526=AXIS2_PLACEMENT_3D('',#93500,#77874,#77875);
#71527=AXIS2_PLACEMENT_3D('',#93502,#77876,#77877);
#71528=AXIS2_PLACEMENT_3D('',#93540,#77878,#77879);
#71529=AXIS2_PLACEMENT_3D('',#93542,#77880,#77881);
#71530=AXIS2_PLACEMENT_3D('',#93580,#77882,#77883);
#71531=AXIS2_PLACEMENT_3D('',#93582,#77884,#77885);
#71532=AXIS2_PLACEMENT_3D('',#93592,#77887,#77888);
#71533=AXIS2_PLACEMENT_3D('',#93604,#77889,#77890);
#71534=AXIS2_PLACEMENT_3D('',#93606,#77891,#77892);
#71535=AXIS2_PLACEMENT_3D('',#93609,#77894,#77895);
#71536=AXIS2_PLACEMENT_3D('',#93610,#77896,#77897);
#71537=AXIS2_PLACEMENT_3D('',#93622,#77898,#77899);
#71538=AXIS2_PLACEMENT_3D('',#93624,#77900,#77901);
#71539=AXIS2_PLACEMENT_3D('',#93627,#77903,#77904);
#71540=AXIS2_PLACEMENT_3D('',#93628,#77905,#77906);
#71541=AXIS2_PLACEMENT_3D('',#93631,#77907,#77908);
#71542=AXIS2_PLACEMENT_3D('',#93634,#77910,#77911);
#71543=AXIS2_PLACEMENT_3D('',#93635,#77912,#77913);
#71544=AXIS2_PLACEMENT_3D('',#93636,#77914,#77915);
#71545=AXIS2_PLACEMENT_3D('',#93639,#77917,#77918);
#71546=AXIS2_PLACEMENT_3D('',#93640,#77919,#77920);
#71547=AXIS2_PLACEMENT_3D('',#93650,#77921,#77922);
#71548=AXIS2_PLACEMENT_3D('',#93652,#77923,#77924);
#71549=AXIS2_PLACEMENT_3D('',#93686,#77925,#77926);
#71550=AXIS2_PLACEMENT_3D('',#93688,#77927,#77928);
#71551=AXIS2_PLACEMENT_3D('',#93722,#77929,#77930);
#71552=AXIS2_PLACEMENT_3D('',#93724,#77931,#77932);
#71553=AXIS2_PLACEMENT_3D('',#93758,#77933,#77934);
#71554=AXIS2_PLACEMENT_3D('',#93760,#77935,#77936);
#71555=AXIS2_PLACEMENT_3D('',#93794,#77937,#77938);
#71556=AXIS2_PLACEMENT_3D('',#93796,#77939,#77940);
#71557=AXIS2_PLACEMENT_3D('',#93830,#77941,#77942);
#71558=AXIS2_PLACEMENT_3D('',#93832,#77943,#77944);
#71559=AXIS2_PLACEMENT_3D('',#93866,#77945,#77946);
#71560=AXIS2_PLACEMENT_3D('',#93868,#77947,#77948);
#71561=AXIS2_PLACEMENT_3D('',#93902,#77949,#77950);
#71562=AXIS2_PLACEMENT_3D('',#93904,#77951,#77952);
#71563=AXIS2_PLACEMENT_3D('',#93938,#77953,#77954);
#71564=AXIS2_PLACEMENT_3D('',#93940,#77955,#77956);
#71565=AXIS2_PLACEMENT_3D('',#93974,#77957,#77958);
#71566=AXIS2_PLACEMENT_3D('',#93976,#77959,#77960);
#71567=AXIS2_PLACEMENT_3D('',#94010,#77961,#77962);
#71568=AXIS2_PLACEMENT_3D('',#94012,#77963,#77964);
#71569=AXIS2_PLACEMENT_3D('',#94046,#77965,#77966);
#71570=AXIS2_PLACEMENT_3D('',#94048,#77967,#77968);
#71571=AXIS2_PLACEMENT_3D('',#94082,#77969,#77970);
#71572=AXIS2_PLACEMENT_3D('',#94084,#77971,#77972);
#71573=AXIS2_PLACEMENT_3D('',#94118,#77973,#77974);
#71574=AXIS2_PLACEMENT_3D('',#94120,#77975,#77976);
#71575=AXIS2_PLACEMENT_3D('',#94154,#77977,#77978);
#71576=AXIS2_PLACEMENT_3D('',#94156,#77979,#77980);
#71577=AXIS2_PLACEMENT_3D('',#94170,#77982,#77983);
#71578=AXIS2_PLACEMENT_3D('',#94198,#77984,#77985);
#71579=AXIS2_PLACEMENT_3D('',#94200,#77986,#77987);
#71580=AXIS2_PLACEMENT_3D('',#94234,#77988,#77989);
#71581=AXIS2_PLACEMENT_3D('',#94236,#77990,#77991);
#71582=AXIS2_PLACEMENT_3D('',#94270,#77992,#77993);
#71583=AXIS2_PLACEMENT_3D('',#94272,#77994,#77995);
#71584=AXIS2_PLACEMENT_3D('',#94306,#77996,#77997);
#71585=AXIS2_PLACEMENT_3D('',#94308,#77998,#77999);
#71586=AXIS2_PLACEMENT_3D('',#94342,#78000,#78001);
#71587=AXIS2_PLACEMENT_3D('',#94344,#78002,#78003);
#71588=AXIS2_PLACEMENT_3D('',#94378,#78004,#78005);
#71589=AXIS2_PLACEMENT_3D('',#94380,#78006,#78007);
#71590=AXIS2_PLACEMENT_3D('',#94414,#78008,#78009);
#71591=AXIS2_PLACEMENT_3D('',#94416,#78010,#78011);
#71592=AXIS2_PLACEMENT_3D('',#94450,#78012,#78013);
#71593=AXIS2_PLACEMENT_3D('',#94452,#78014,#78015);
#71594=AXIS2_PLACEMENT_3D('',#94486,#78016,#78017);
#71595=AXIS2_PLACEMENT_3D('',#94488,#78018,#78019);
#71596=AXIS2_PLACEMENT_3D('',#94522,#78020,#78021);
#71597=AXIS2_PLACEMENT_3D('',#94524,#78022,#78023);
#71598=AXIS2_PLACEMENT_3D('',#94558,#78024,#78025);
#71599=AXIS2_PLACEMENT_3D('',#94560,#78026,#78027);
#71600=AXIS2_PLACEMENT_3D('',#94594,#78028,#78029);
#71601=AXIS2_PLACEMENT_3D('',#94596,#78030,#78031);
#71602=AXIS2_PLACEMENT_3D('',#94630,#78032,#78033);
#71603=AXIS2_PLACEMENT_3D('',#94632,#78034,#78035);
#71604=AXIS2_PLACEMENT_3D('',#94666,#78036,#78037);
#71605=AXIS2_PLACEMENT_3D('',#94668,#78038,#78039);
#71606=AXIS2_PLACEMENT_3D('',#94693,#78040,#78041);
#71607=AXIS2_PLACEMENT_3D('',#94696,#78042,#78043);
#71608=AXIS2_PLACEMENT_3D('',#94698,#78044,#78045);
#71609=AXIS2_PLACEMENT_3D('',#94714,#78046,#78047);
#71610=AXIS2_PLACEMENT_3D('',#94726,#78048,#78049);
#71611=AXIS2_PLACEMENT_3D('',#94742,#78050,#78051);
#71612=AXIS2_PLACEMENT_3D('',#94758,#78052,#78053);
#71613=AXIS2_PLACEMENT_3D('',#94760,#78054,#78055);
#71614=AXIS2_PLACEMENT_3D('',#94762,#78056,#78057);
#71615=AXIS2_PLACEMENT_3D('',#94763,#78058,#78059);
#71616=AXIS2_PLACEMENT_3D('',#94764,#78060,#78061);
#71617=AXIS2_PLACEMENT_3D('',#94781,#78062,#78063);
#71618=AXIS2_PLACEMENT_3D('',#94782,#78064,#78065);
#71619=AXIS2_PLACEMENT_3D('',#94783,#78066,#78067);
#71620=AXIS2_PLACEMENT_3D('',#94795,#78068,#78069);
#71621=AXIS2_PLACEMENT_3D('',#94811,#78070,#78071);
#71622=AXIS2_PLACEMENT_3D('',#94823,#78072,#78073);
#71623=AXIS2_PLACEMENT_3D('',#94839,#78074,#78075);
#71624=AXIS2_PLACEMENT_3D('',#94849,#78076,#78077);
#71625=AXIS2_PLACEMENT_3D('',#94851,#78078,#78079);
#71626=AXIS2_PLACEMENT_3D('',#94858,#78080,#78081);
#71627=AXIS2_PLACEMENT_3D('',#94861,#78082,#78083);
#71628=AXIS2_PLACEMENT_3D('',#94863,#78084,#78085);
#71629=AXIS2_PLACEMENT_3D('',#94865,#78086,#78087);
#71630=AXIS2_PLACEMENT_3D('',#94879,#78088,#78089);
#71631=AXIS2_PLACEMENT_3D('',#94880,#78090,#78091);
#71632=AXIS2_PLACEMENT_3D('',#94888,#78092,#78093);
#71633=AXIS2_PLACEMENT_3D('',#94889,#78094,#78095);
#71634=AXIS2_PLACEMENT_3D('',#94918,#78096,#78097);
#71635=AXIS2_PLACEMENT_3D('',#94926,#78098,#78099);
#71636=AXIS2_PLACEMENT_3D('',#94943,#78100,#78101);
#71637=AXIS2_PLACEMENT_3D('',#94944,#78102,#78103);
#71638=AXIS2_PLACEMENT_3D('',#94945,#78104,#78105);
#71639=AXIS2_PLACEMENT_3D('',#94955,#78106,#78107);
#71640=AXIS2_PLACEMENT_3D('',#94957,#78108,#78109);
#71641=AXIS2_PLACEMENT_3D('',#94970,#78110,#78111);
#71642=AXIS2_PLACEMENT_3D('',#94980,#78112,#78113);
#71643=AXIS2_PLACEMENT_3D('',#94982,#78114,#78115);
#71644=AXIS2_PLACEMENT_3D('',#94989,#78116,#78117);
#71645=AXIS2_PLACEMENT_3D('',#95006,#78118,#78119);
#71646=AXIS2_PLACEMENT_3D('',#95007,#78120,#78121);
#71647=AXIS2_PLACEMENT_3D('',#95008,#78122,#78123);
#71648=AXIS2_PLACEMENT_3D('',#95032,#78124,#78125);
#71649=AXIS2_PLACEMENT_3D('',#95033,#78126,#78127);
#71650=AXIS2_PLACEMENT_3D('',#95057,#78128,#78129);
#71651=AXIS2_PLACEMENT_3D('',#95070,#78130,#78131);
#71652=AXIS2_PLACEMENT_3D('',#95087,#78132,#78133);
#71653=AXIS2_PLACEMENT_3D('',#95095,#78134,#78135);
#71654=AXIS2_PLACEMENT_3D('',#95112,#78136,#78137);
#71655=AXIS2_PLACEMENT_3D('',#95113,#78138,#78139);
#71656=AXIS2_PLACEMENT_3D('',#95114,#78140,#78141);
#71657=AXIS2_PLACEMENT_3D('',#95130,#78142,#78143);
#71658=AXIS2_PLACEMENT_3D('',#95132,#78144,#78145);
#71659=AXIS2_PLACEMENT_3D('',#95139,#78146,#78147);
#71660=AXIS2_PLACEMENT_3D('',#95155,#78148,#78149);
#71661=AXIS2_PLACEMENT_3D('',#95176,#78150,#78151);
#71662=AXIS2_PLACEMENT_3D('',#95205,#78152,#78153);
#71663=AXIS2_PLACEMENT_3D('',#95206,#78154,#78155);
#71664=AXIS2_PLACEMENT_3D('',#95207,#78156,#78157);
#71665=AXIS2_PLACEMENT_3D('',#95231,#78158,#78159);
#71666=AXIS2_PLACEMENT_3D('',#95232,#78160,#78161);
#71667=AXIS2_PLACEMENT_3D('',#95250,#78162,#78163);
#71668=AXIS2_PLACEMENT_3D('',#95257,#78164,#78165);
#71669=AXIS2_PLACEMENT_3D('',#95267,#78166,#78167);
#71670=AXIS2_PLACEMENT_3D('',#95269,#78168,#78169);
#71671=AXIS2_PLACEMENT_3D('',#95282,#78170,#78171);
#71672=AXIS2_PLACEMENT_3D('',#95305,#78172,#78173);
#71673=AXIS2_PLACEMENT_3D('',#95313,#78174,#78175);
#71674=AXIS2_PLACEMENT_3D('',#95342,#78176,#78177);
#71675=AXIS2_PLACEMENT_3D('',#95343,#78178,#78179);
#71676=AXIS2_PLACEMENT_3D('',#95344,#78180,#78181);
#71677=AXIS2_PLACEMENT_3D('',#95360,#78182,#78183);
#71678=AXIS2_PLACEMENT_3D('',#95378,#78184,#78185);
#71679=AXIS2_PLACEMENT_3D('',#95407,#78186,#78187);
#71680=AXIS2_PLACEMENT_3D('',#95408,#78188,#78189);
#71681=AXIS2_PLACEMENT_3D('',#95409,#78190,#78191);
#71682=AXIS2_PLACEMENT_3D('',#95439,#78192,#78193);
#71683=AXIS2_PLACEMENT_3D('',#95440,#78194,#78195);
#71684=AXIS2_PLACEMENT_3D('',#95458,#78196,#78197);
#71685=AXIS2_PLACEMENT_3D('',#95465,#78198,#78199);
#71686=AXIS2_PLACEMENT_3D('',#95481,#78200,#78201);
#71687=AXIS2_PLACEMENT_3D('',#95494,#78202,#78203);
#71688=AXIS2_PLACEMENT_3D('',#95525,#78204,#78205);
#71689=AXIS2_PLACEMENT_3D('',#95554,#78206,#78207);
#71690=AXIS2_PLACEMENT_3D('',#95555,#78208,#78209);
#71691=AXIS2_PLACEMENT_3D('',#95556,#78210,#78211);
#71692=AXIS2_PLACEMENT_3D('',#95566,#78212,#78213);
#71693=AXIS2_PLACEMENT_3D('',#95589,#78214,#78215);
#71694=AXIS2_PLACEMENT_3D('',#95593,#78217,#78218);
#71695=AXIS2_PLACEMENT_3D('',#95617,#78219,#78220);
#71696=AXIS2_PLACEMENT_3D('',#95625,#78221,#78222);
#71697=AXIS2_PLACEMENT_3D('',#95627,#78224,#78225);
#71698=AXIS2_PLACEMENT_3D('',#95637,#78226,#78227);
#71699=AXIS2_PLACEMENT_3D('',#95638,#78228,#78229);
#71700=AXIS2_PLACEMENT_3D('',#95647,#78231,#78232);
#71701=AXIS2_PLACEMENT_3D('',#95665,#78233,#78234);
#71702=AXIS2_PLACEMENT_3D('',#95673,#78235,#78236);
#71703=AXIS2_PLACEMENT_3D('',#95675,#78238,#78239);
#71704=AXIS2_PLACEMENT_3D('',#95685,#78240,#78241);
#71705=AXIS2_PLACEMENT_3D('',#95686,#78242,#78243);
#71706=AXIS2_PLACEMENT_3D('',#95695,#78245,#78246);
#71707=AXIS2_PLACEMENT_3D('',#95713,#78247,#78248);
#71708=AXIS2_PLACEMENT_3D('',#95721,#78249,#78250);
#71709=AXIS2_PLACEMENT_3D('',#95723,#78252,#78253);
#71710=AXIS2_PLACEMENT_3D('',#95733,#78254,#78255);
#71711=AXIS2_PLACEMENT_3D('',#95734,#78256,#78257);
#71712=AXIS2_PLACEMENT_3D('',#95743,#78259,#78260);
#71713=AXIS2_PLACEMENT_3D('',#95761,#78261,#78262);
#71714=AXIS2_PLACEMENT_3D('',#95769,#78263,#78264);
#71715=AXIS2_PLACEMENT_3D('',#95771,#78266,#78267);
#71716=AXIS2_PLACEMENT_3D('',#95781,#78268,#78269);
#71717=AXIS2_PLACEMENT_3D('',#95782,#78270,#78271);
#71718=AXIS2_PLACEMENT_3D('',#95791,#78273,#78274);
#71719=AXIS2_PLACEMENT_3D('',#95809,#78275,#78276);
#71720=AXIS2_PLACEMENT_3D('',#95817,#78277,#78278);
#71721=AXIS2_PLACEMENT_3D('',#95819,#78280,#78281);
#71722=AXIS2_PLACEMENT_3D('',#95829,#78282,#78283);
#71723=AXIS2_PLACEMENT_3D('',#95830,#78284,#78285);
#71724=AXIS2_PLACEMENT_3D('',#95839,#78287,#78288);
#71725=AXIS2_PLACEMENT_3D('',#95857,#78289,#78290);
#71726=AXIS2_PLACEMENT_3D('',#95865,#78291,#78292);
#71727=AXIS2_PLACEMENT_3D('',#95867,#78294,#78295);
#71728=AXIS2_PLACEMENT_3D('',#95877,#78296,#78297);
#71729=AXIS2_PLACEMENT_3D('',#95878,#78298,#78299);
#71730=AXIS2_PLACEMENT_3D('',#95887,#78301,#78302);
#71731=AXIS2_PLACEMENT_3D('',#95910,#78303,#78304);
#71732=AXIS2_PLACEMENT_3D('',#95920,#78307,#78308);
#71733=AXIS2_PLACEMENT_3D('',#95938,#78309,#78310);
#71734=AXIS2_PLACEMENT_3D('',#95946,#78311,#78312);
#71735=AXIS2_PLACEMENT_3D('',#95948,#78314,#78315);
#71736=AXIS2_PLACEMENT_3D('',#95958,#78316,#78317);
#71737=AXIS2_PLACEMENT_3D('',#95959,#78318,#78319);
#71738=AXIS2_PLACEMENT_3D('',#95968,#78321,#78322);
#71739=AXIS2_PLACEMENT_3D('',#95986,#78323,#78324);
#71740=AXIS2_PLACEMENT_3D('',#95994,#78325,#78326);
#71741=AXIS2_PLACEMENT_3D('',#95996,#78328,#78329);
#71742=AXIS2_PLACEMENT_3D('',#96006,#78330,#78331);
#71743=AXIS2_PLACEMENT_3D('',#96007,#78332,#78333);
#71744=AXIS2_PLACEMENT_3D('',#96016,#78335,#78336);
#71745=AXIS2_PLACEMENT_3D('',#96034,#78337,#78338);
#71746=AXIS2_PLACEMENT_3D('',#96042,#78339,#78340);
#71747=AXIS2_PLACEMENT_3D('',#96044,#78342,#78343);
#71748=AXIS2_PLACEMENT_3D('',#96054,#78344,#78345);
#71749=AXIS2_PLACEMENT_3D('',#96055,#78346,#78347);
#71750=AXIS2_PLACEMENT_3D('',#96064,#78349,#78350);
#71751=AXIS2_PLACEMENT_3D('',#96082,#78351,#78352);
#71752=AXIS2_PLACEMENT_3D('',#96090,#78353,#78354);
#71753=AXIS2_PLACEMENT_3D('',#96092,#78356,#78357);
#71754=AXIS2_PLACEMENT_3D('',#96102,#78358,#78359);
#71755=AXIS2_PLACEMENT_3D('',#96103,#78360,#78361);
#71756=AXIS2_PLACEMENT_3D('',#96112,#78363,#78364);
#71757=AXIS2_PLACEMENT_3D('',#96130,#78365,#78366);
#71758=AXIS2_PLACEMENT_3D('',#96138,#78367,#78368);
#71759=AXIS2_PLACEMENT_3D('',#96140,#78370,#78371);
#71760=AXIS2_PLACEMENT_3D('',#96150,#78372,#78373);
#71761=AXIS2_PLACEMENT_3D('',#96151,#78374,#78375);
#71762=AXIS2_PLACEMENT_3D('',#96160,#78377,#78378);
#71763=AXIS2_PLACEMENT_3D('',#96178,#78379,#78380);
#71764=AXIS2_PLACEMENT_3D('',#96186,#78381,#78382);
#71765=AXIS2_PLACEMENT_3D('',#96188,#78384,#78385);
#71766=AXIS2_PLACEMENT_3D('',#96198,#78386,#78387);
#71767=AXIS2_PLACEMENT_3D('',#96199,#78388,#78389);
#71768=AXIS2_PLACEMENT_3D('',#96208,#78391,#78392);
#71769=AXIS2_PLACEMENT_3D('',#96226,#78393,#78394);
#71770=AXIS2_PLACEMENT_3D('',#96234,#78395,#78396);
#71771=AXIS2_PLACEMENT_3D('',#96236,#78398,#78399);
#71772=AXIS2_PLACEMENT_3D('',#96246,#78400,#78401);
#71773=AXIS2_PLACEMENT_3D('',#96247,#78402,#78403);
#71774=AXIS2_PLACEMENT_3D('',#96256,#78405,#78406);
#71775=AXIS2_PLACEMENT_3D('',#96274,#78407,#78408);
#71776=AXIS2_PLACEMENT_3D('',#96282,#78409,#78410);
#71777=AXIS2_PLACEMENT_3D('',#96284,#78412,#78413);
#71778=AXIS2_PLACEMENT_3D('',#96294,#78414,#78415);
#71779=AXIS2_PLACEMENT_3D('',#96295,#78416,#78417);
#71780=AXIS2_PLACEMENT_3D('',#96304,#78419,#78420);
#71781=AXIS2_PLACEMENT_3D('',#96322,#78421,#78422);
#71782=AXIS2_PLACEMENT_3D('',#96330,#78423,#78424);
#71783=AXIS2_PLACEMENT_3D('',#96332,#78426,#78427);
#71784=AXIS2_PLACEMENT_3D('',#96342,#78428,#78429);
#71785=AXIS2_PLACEMENT_3D('',#96343,#78430,#78431);
#71786=AXIS2_PLACEMENT_3D('',#96352,#78433,#78434);
#71787=AXIS2_PLACEMENT_3D('',#96370,#78435,#78436);
#71788=AXIS2_PLACEMENT_3D('',#96378,#78437,#78438);
#71789=AXIS2_PLACEMENT_3D('',#96380,#78440,#78441);
#71790=AXIS2_PLACEMENT_3D('',#96390,#78442,#78443);
#71791=AXIS2_PLACEMENT_3D('',#96391,#78444,#78445);
#71792=AXIS2_PLACEMENT_3D('',#96400,#78447,#78448);
#71793=AXIS2_PLACEMENT_3D('',#96418,#78449,#78450);
#71794=AXIS2_PLACEMENT_3D('',#96426,#78451,#78452);
#71795=AXIS2_PLACEMENT_3D('',#96428,#78454,#78455);
#71796=AXIS2_PLACEMENT_3D('',#96438,#78456,#78457);
#71797=AXIS2_PLACEMENT_3D('',#96439,#78458,#78459);
#71798=AXIS2_PLACEMENT_3D('',#96448,#78461,#78462);
#71799=AXIS2_PLACEMENT_3D('',#96466,#78463,#78464);
#71800=AXIS2_PLACEMENT_3D('',#96474,#78465,#78466);
#71801=AXIS2_PLACEMENT_3D('',#96476,#78468,#78469);
#71802=AXIS2_PLACEMENT_3D('',#96486,#78470,#78471);
#71803=AXIS2_PLACEMENT_3D('',#96487,#78472,#78473);
#71804=AXIS2_PLACEMENT_3D('',#96496,#78475,#78476);
#71805=AXIS2_PLACEMENT_3D('',#96514,#78477,#78478);
#71806=AXIS2_PLACEMENT_3D('',#96522,#78479,#78480);
#71807=AXIS2_PLACEMENT_3D('',#96524,#78482,#78483);
#71808=AXIS2_PLACEMENT_3D('',#96534,#78484,#78485);
#71809=AXIS2_PLACEMENT_3D('',#96535,#78486,#78487);
#71810=AXIS2_PLACEMENT_3D('',#96544,#78489,#78490);
#71811=AXIS2_PLACEMENT_3D('',#96562,#78491,#78492);
#71812=AXIS2_PLACEMENT_3D('',#96570,#78493,#78494);
#71813=AXIS2_PLACEMENT_3D('',#96572,#78496,#78497);
#71814=AXIS2_PLACEMENT_3D('',#96582,#78498,#78499);
#71815=AXIS2_PLACEMENT_3D('',#96583,#78500,#78501);
#71816=AXIS2_PLACEMENT_3D('',#96592,#78503,#78504);
#71817=AXIS2_PLACEMENT_3D('',#96610,#78505,#78506);
#71818=AXIS2_PLACEMENT_3D('',#96618,#78507,#78508);
#71819=AXIS2_PLACEMENT_3D('',#96620,#78510,#78511);
#71820=AXIS2_PLACEMENT_3D('',#96630,#78512,#78513);
#71821=AXIS2_PLACEMENT_3D('',#96631,#78514,#78515);
#71822=AXIS2_PLACEMENT_3D('',#96640,#78517,#78518);
#71823=AXIS2_PLACEMENT_3D('',#96658,#78519,#78520);
#71824=AXIS2_PLACEMENT_3D('',#96666,#78521,#78522);
#71825=AXIS2_PLACEMENT_3D('',#96668,#78524,#78525);
#71826=AXIS2_PLACEMENT_3D('',#96678,#78526,#78527);
#71827=AXIS2_PLACEMENT_3D('',#96679,#78528,#78529);
#71828=AXIS2_PLACEMENT_3D('',#96688,#78531,#78532);
#71829=AXIS2_PLACEMENT_3D('',#96706,#78533,#78534);
#71830=AXIS2_PLACEMENT_3D('',#96714,#78535,#78536);
#71831=AXIS2_PLACEMENT_3D('',#96716,#78538,#78539);
#71832=AXIS2_PLACEMENT_3D('',#96726,#78540,#78541);
#71833=AXIS2_PLACEMENT_3D('',#96727,#78542,#78543);
#71834=AXIS2_PLACEMENT_3D('',#96736,#78545,#78546);
#71835=AXIS2_PLACEMENT_3D('',#96754,#78547,#78548);
#71836=AXIS2_PLACEMENT_3D('',#96762,#78549,#78550);
#71837=AXIS2_PLACEMENT_3D('',#96771,#78552,#78553);
#71838=AXIS2_PLACEMENT_3D('',#96774,#78555,#78556);
#71839=AXIS2_PLACEMENT_3D('',#96775,#78557,#78558);
#71840=AXIS2_PLACEMENT_3D('',#96784,#78559,#78560);
#71841=AXIS2_PLACEMENT_3D('',#96802,#78561,#78562);
#71842=AXIS2_PLACEMENT_3D('',#96810,#78563,#78564);
#71843=AXIS2_PLACEMENT_3D('',#96812,#78566,#78567);
#71844=AXIS2_PLACEMENT_3D('',#96814,#78568,#78569);
#71845=AXIS2_PLACEMENT_3D('',#96823,#78570,#78571);
#71846=AXIS2_PLACEMENT_3D('',#96831,#78572,#78573);
#71847=AXIS2_PLACEMENT_3D('',#96850,#78575,#78576);
#71848=AXIS2_PLACEMENT_3D('',#96858,#78577,#78578);
#71849=AXIS2_PLACEMENT_3D('',#96860,#78580,#78581);
#71850=AXIS2_PLACEMENT_3D('',#96870,#78582,#78583);
#71851=AXIS2_PLACEMENT_3D('',#96871,#78584,#78585);
#71852=AXIS2_PLACEMENT_3D('',#96880,#78587,#78588);
#71853=AXIS2_PLACEMENT_3D('',#96898,#78589,#78590);
#71854=AXIS2_PLACEMENT_3D('',#96906,#78591,#78592);
#71855=AXIS2_PLACEMENT_3D('',#96908,#78594,#78595);
#71856=AXIS2_PLACEMENT_3D('',#96918,#78596,#78597);
#71857=AXIS2_PLACEMENT_3D('',#96919,#78598,#78599);
#71858=AXIS2_PLACEMENT_3D('',#96928,#78601,#78602);
#71859=AXIS2_PLACEMENT_3D('',#96929,#78603,#78604);
#71860=AXIS2_PLACEMENT_3D('',#96939,#78605,#78606);
#71861=AXIS2_PLACEMENT_3D('',#96940,#78607,#78608);
#71862=AXIS2_PLACEMENT_3D('',#96956,#78609,#78610);
#71863=AXIS2_PLACEMENT_3D('',#96976,#78612,#78613);
#71864=AXIS2_PLACEMENT_3D('',#96990,#78616,#78617);
#71865=AXIS2_PLACEMENT_3D('',#97008,#78618,#78619);
#71866=AXIS2_PLACEMENT_3D('',#97010,#78621,#78622);
#71867=AXIS2_PLACEMENT_3D('',#97012,#78623,#78624);
#71868=AXIS2_PLACEMENT_3D('',#97013,#78625,#78626);
#71869=AXIS2_PLACEMENT_3D('',#97026,#78628,#78629);
#71870=AXIS2_PLACEMENT_3D('',#97044,#78630,#78631);
#71871=AXIS2_PLACEMENT_3D('',#97046,#78633,#78634);
#71872=AXIS2_PLACEMENT_3D('',#97048,#78635,#78636);
#71873=AXIS2_PLACEMENT_3D('',#97049,#78637,#78638);
#71874=AXIS2_PLACEMENT_3D('',#97062,#78640,#78641);
#71875=AXIS2_PLACEMENT_3D('',#97080,#78642,#78643);
#71876=AXIS2_PLACEMENT_3D('',#97082,#78645,#78646);
#71877=AXIS2_PLACEMENT_3D('',#97084,#78647,#78648);
#71878=AXIS2_PLACEMENT_3D('',#97085,#78649,#78650);
#71879=AXIS2_PLACEMENT_3D('',#97098,#78652,#78653);
#71880=AXIS2_PLACEMENT_3D('',#97116,#78654,#78655);
#71881=AXIS2_PLACEMENT_3D('',#97118,#78657,#78658);
#71882=AXIS2_PLACEMENT_3D('',#97120,#78659,#78660);
#71883=AXIS2_PLACEMENT_3D('',#97121,#78661,#78662);
#71884=AXIS2_PLACEMENT_3D('',#97134,#78664,#78665);
#71885=AXIS2_PLACEMENT_3D('',#97152,#78666,#78667);
#71886=AXIS2_PLACEMENT_3D('',#97154,#78669,#78670);
#71887=AXIS2_PLACEMENT_3D('',#97156,#78671,#78672);
#71888=AXIS2_PLACEMENT_3D('',#97157,#78673,#78674);
#71889=AXIS2_PLACEMENT_3D('',#97170,#78676,#78677);
#71890=AXIS2_PLACEMENT_3D('',#97188,#78678,#78679);
#71891=AXIS2_PLACEMENT_3D('',#97190,#78681,#78682);
#71892=AXIS2_PLACEMENT_3D('',#97192,#78683,#78684);
#71893=AXIS2_PLACEMENT_3D('',#97193,#78685,#78686);
#71894=AXIS2_PLACEMENT_3D('',#97206,#78688,#78689);
#71895=AXIS2_PLACEMENT_3D('',#97224,#78690,#78691);
#71896=AXIS2_PLACEMENT_3D('',#97226,#78693,#78694);
#71897=AXIS2_PLACEMENT_3D('',#97228,#78695,#78696);
#71898=AXIS2_PLACEMENT_3D('',#97229,#78697,#78698);
#71899=AXIS2_PLACEMENT_3D('',#97242,#78700,#78701);
#71900=AXIS2_PLACEMENT_3D('',#97260,#78702,#78703);
#71901=AXIS2_PLACEMENT_3D('',#97262,#78705,#78706);
#71902=AXIS2_PLACEMENT_3D('',#97264,#78707,#78708);
#71903=AXIS2_PLACEMENT_3D('',#97265,#78709,#78710);
#71904=AXIS2_PLACEMENT_3D('',#97278,#78712,#78713);
#71905=AXIS2_PLACEMENT_3D('',#97296,#78714,#78715);
#71906=AXIS2_PLACEMENT_3D('',#97298,#78717,#78718);
#71907=AXIS2_PLACEMENT_3D('',#97300,#78719,#78720);
#71908=AXIS2_PLACEMENT_3D('',#97301,#78721,#78722);
#71909=AXIS2_PLACEMENT_3D('',#97314,#78724,#78725);
#71910=AXIS2_PLACEMENT_3D('',#97332,#78726,#78727);
#71911=AXIS2_PLACEMENT_3D('',#97334,#78729,#78730);
#71912=AXIS2_PLACEMENT_3D('',#97336,#78731,#78732);
#71913=AXIS2_PLACEMENT_3D('',#97337,#78733,#78734);
#71914=AXIS2_PLACEMENT_3D('',#97350,#78736,#78737);
#71915=AXIS2_PLACEMENT_3D('',#97368,#78738,#78739);
#71916=AXIS2_PLACEMENT_3D('',#97370,#78741,#78742);
#71917=AXIS2_PLACEMENT_3D('',#97372,#78743,#78744);
#71918=AXIS2_PLACEMENT_3D('',#97373,#78745,#78746);
#71919=AXIS2_PLACEMENT_3D('',#97386,#78748,#78749);
#71920=AXIS2_PLACEMENT_3D('',#97404,#78750,#78751);
#71921=AXIS2_PLACEMENT_3D('',#97406,#78753,#78754);
#71922=AXIS2_PLACEMENT_3D('',#97408,#78755,#78756);
#71923=AXIS2_PLACEMENT_3D('',#97409,#78757,#78758);
#71924=AXIS2_PLACEMENT_3D('',#97422,#78760,#78761);
#71925=AXIS2_PLACEMENT_3D('',#97440,#78762,#78763);
#71926=AXIS2_PLACEMENT_3D('',#97442,#78765,#78766);
#71927=AXIS2_PLACEMENT_3D('',#97444,#78767,#78768);
#71928=AXIS2_PLACEMENT_3D('',#97445,#78769,#78770);
#71929=AXIS2_PLACEMENT_3D('',#97485,#78774,#78775);
#71930=AXIS2_PLACEMENT_3D('',#97503,#78776,#78777);
#71931=AXIS2_PLACEMENT_3D('',#97505,#78779,#78780);
#71932=AXIS2_PLACEMENT_3D('',#97507,#78781,#78782);
#71933=AXIS2_PLACEMENT_3D('',#97508,#78783,#78784);
#71934=AXIS2_PLACEMENT_3D('',#97521,#78786,#78787);
#71935=AXIS2_PLACEMENT_3D('',#97539,#78788,#78789);
#71936=AXIS2_PLACEMENT_3D('',#97541,#78791,#78792);
#71937=AXIS2_PLACEMENT_3D('',#97543,#78793,#78794);
#71938=AXIS2_PLACEMENT_3D('',#97544,#78795,#78796);
#71939=AXIS2_PLACEMENT_3D('',#97557,#78798,#78799);
#71940=AXIS2_PLACEMENT_3D('',#97575,#78800,#78801);
#71941=AXIS2_PLACEMENT_3D('',#97577,#78803,#78804);
#71942=AXIS2_PLACEMENT_3D('',#97579,#78805,#78806);
#71943=AXIS2_PLACEMENT_3D('',#97580,#78807,#78808);
#71944=AXIS2_PLACEMENT_3D('',#97593,#78810,#78811);
#71945=AXIS2_PLACEMENT_3D('',#97611,#78812,#78813);
#71946=AXIS2_PLACEMENT_3D('',#97613,#78815,#78816);
#71947=AXIS2_PLACEMENT_3D('',#97615,#78817,#78818);
#71948=AXIS2_PLACEMENT_3D('',#97616,#78819,#78820);
#71949=AXIS2_PLACEMENT_3D('',#97629,#78822,#78823);
#71950=AXIS2_PLACEMENT_3D('',#97647,#78824,#78825);
#71951=AXIS2_PLACEMENT_3D('',#97649,#78827,#78828);
#71952=AXIS2_PLACEMENT_3D('',#97651,#78829,#78830);
#71953=AXIS2_PLACEMENT_3D('',#97652,#78831,#78832);
#71954=AXIS2_PLACEMENT_3D('',#97665,#78834,#78835);
#71955=AXIS2_PLACEMENT_3D('',#97683,#78836,#78837);
#71956=AXIS2_PLACEMENT_3D('',#97685,#78839,#78840);
#71957=AXIS2_PLACEMENT_3D('',#97687,#78841,#78842);
#71958=AXIS2_PLACEMENT_3D('',#97688,#78843,#78844);
#71959=AXIS2_PLACEMENT_3D('',#97701,#78846,#78847);
#71960=AXIS2_PLACEMENT_3D('',#97719,#78848,#78849);
#71961=AXIS2_PLACEMENT_3D('',#97721,#78851,#78852);
#71962=AXIS2_PLACEMENT_3D('',#97723,#78853,#78854);
#71963=AXIS2_PLACEMENT_3D('',#97724,#78855,#78856);
#71964=AXIS2_PLACEMENT_3D('',#97737,#78858,#78859);
#71965=AXIS2_PLACEMENT_3D('',#97755,#78860,#78861);
#71966=AXIS2_PLACEMENT_3D('',#97757,#78863,#78864);
#71967=AXIS2_PLACEMENT_3D('',#97759,#78865,#78866);
#71968=AXIS2_PLACEMENT_3D('',#97760,#78867,#78868);
#71969=AXIS2_PLACEMENT_3D('',#97773,#78870,#78871);
#71970=AXIS2_PLACEMENT_3D('',#97791,#78872,#78873);
#71971=AXIS2_PLACEMENT_3D('',#97793,#78875,#78876);
#71972=AXIS2_PLACEMENT_3D('',#97795,#78877,#78878);
#71973=AXIS2_PLACEMENT_3D('',#97796,#78879,#78880);
#71974=AXIS2_PLACEMENT_3D('',#97809,#78882,#78883);
#71975=AXIS2_PLACEMENT_3D('',#97827,#78884,#78885);
#71976=AXIS2_PLACEMENT_3D('',#97829,#78887,#78888);
#71977=AXIS2_PLACEMENT_3D('',#97831,#78889,#78890);
#71978=AXIS2_PLACEMENT_3D('',#97832,#78891,#78892);
#71979=AXIS2_PLACEMENT_3D('',#97845,#78894,#78895);
#71980=AXIS2_PLACEMENT_3D('',#97863,#78896,#78897);
#71981=AXIS2_PLACEMENT_3D('',#97865,#78899,#78900);
#71982=AXIS2_PLACEMENT_3D('',#97867,#78901,#78902);
#71983=AXIS2_PLACEMENT_3D('',#97868,#78903,#78904);
#71984=AXIS2_PLACEMENT_3D('',#97881,#78906,#78907);
#71985=AXIS2_PLACEMENT_3D('',#97899,#78908,#78909);
#71986=AXIS2_PLACEMENT_3D('',#97901,#78911,#78912);
#71987=AXIS2_PLACEMENT_3D('',#97903,#78913,#78914);
#71988=AXIS2_PLACEMENT_3D('',#97904,#78915,#78916);
#71989=AXIS2_PLACEMENT_3D('',#97917,#78918,#78919);
#71990=AXIS2_PLACEMENT_3D('',#97935,#78920,#78921);
#71991=AXIS2_PLACEMENT_3D('',#97937,#78923,#78924);
#71992=AXIS2_PLACEMENT_3D('',#97939,#78925,#78926);
#71993=AXIS2_PLACEMENT_3D('',#97940,#78927,#78928);
#71994=AXIS2_PLACEMENT_3D('',#97953,#78930,#78931);
#71995=AXIS2_PLACEMENT_3D('',#97971,#78932,#78933);
#71996=AXIS2_PLACEMENT_3D('',#97973,#78935,#78936);
#71997=AXIS2_PLACEMENT_3D('',#97975,#78937,#78938);
#71998=AXIS2_PLACEMENT_3D('',#97976,#78939,#78940);
#71999=AXIS2_PLACEMENT_3D('',#97977,#78941,#78942);
#72000=AXIS2_PLACEMENT_3D('',#97979,#78943,#78944);
#72001=AXIS2_PLACEMENT_3D('',#97981,#78945,#78946);
#72002=AXIS2_PLACEMENT_3D('',#97982,#78947,#78948);
#72003=AXIS2_PLACEMENT_3D('',#98000,#78950,#78951);
#72004=AXIS2_PLACEMENT_3D('',#98039,#78952,#78953);
#72005=AXIS2_PLACEMENT_3D('',#98072,#78954,#78955);
#72006=AXIS2_PLACEMENT_3D('',#98105,#78956,#78957);
#72007=AXIS2_PLACEMENT_3D('',#98138,#78958,#78959);
#72008=AXIS2_PLACEMENT_3D('',#98171,#78960,#78961);
#72009=AXIS2_PLACEMENT_3D('',#98204,#78962,#78963);
#72010=AXIS2_PLACEMENT_3D('',#98237,#78964,#78965);
#72011=AXIS2_PLACEMENT_3D('',#98272,#78966,#78967);
#72012=AXIS2_PLACEMENT_3D('',#98305,#78968,#78969);
#72013=AXIS2_PLACEMENT_3D('',#98338,#78970,#78971);
#72014=AXIS2_PLACEMENT_3D('',#98371,#78972,#78973);
#72015=AXIS2_PLACEMENT_3D('',#98404,#78974,#78975);
#72016=AXIS2_PLACEMENT_3D('',#98439,#78976,#78977);
#72017=AXIS2_PLACEMENT_3D('',#98474,#78978,#78979);
#72018=AXIS2_PLACEMENT_3D('',#98507,#78980,#78981);
#72019=AXIS2_PLACEMENT_3D('',#98540,#78982,#78983);
#72020=AXIS2_PLACEMENT_3D('',#98575,#78984,#78985);
#72021=AXIS2_PLACEMENT_3D('',#98608,#78986,#78987);
#72022=AXIS2_PLACEMENT_3D('',#98641,#78988,#78989);
#72023=AXIS2_PLACEMENT_3D('',#98674,#78990,#78991);
#72024=AXIS2_PLACEMENT_3D('',#98707,#78992,#78993);
#72025=AXIS2_PLACEMENT_3D('',#98740,#78994,#78995);
#72026=AXIS2_PLACEMENT_3D('',#98775,#78996,#78997);
#72027=AXIS2_PLACEMENT_3D('',#98810,#78998,#78999);
#72028=AXIS2_PLACEMENT_3D('',#98845,#79000,#79001);
#72029=AXIS2_PLACEMENT_3D('',#98878,#79002,#79003);
#72030=AXIS2_PLACEMENT_3D('',#98911,#79004,#79005);
#72031=AXIS2_PLACEMENT_3D('',#98944,#79006,#79007);
#72032=AXIS2_PLACEMENT_3D('',#98983,#79008,#79009);
#72033=AXIS2_PLACEMENT_3D('',#98991,#79010,#79011);
#72034=AXIS2_PLACEMENT_3D('',#99008,#79012,#79013);
#72035=AXIS2_PLACEMENT_3D('',#99016,#79014,#79015);
#72036=AXIS2_PLACEMENT_3D('',#99033,#79016,#79017);
#72037=AXIS2_PLACEMENT_3D('',#99041,#79018,#79019);
#72038=AXIS2_PLACEMENT_3D('',#99058,#79020,#79021);
#72039=AXIS2_PLACEMENT_3D('',#99066,#79022,#79023);
#72040=AXIS2_PLACEMENT_3D('',#99083,#79024,#79025);
#72041=AXIS2_PLACEMENT_3D('',#99091,#79026,#79027);
#72042=AXIS2_PLACEMENT_3D('',#99108,#79028,#79029);
#72043=AXIS2_PLACEMENT_3D('',#99116,#79030,#79031);
#72044=AXIS2_PLACEMENT_3D('',#99133,#79032,#79033);
#72045=AXIS2_PLACEMENT_3D('',#99141,#79034,#79035);
#72046=AXIS2_PLACEMENT_3D('',#99158,#79036,#79037);
#72047=AXIS2_PLACEMENT_3D('',#99166,#79038,#79039);
#72048=AXIS2_PLACEMENT_3D('',#99183,#79040,#79041);
#72049=AXIS2_PLACEMENT_3D('',#99191,#79042,#79043);
#72050=AXIS2_PLACEMENT_3D('',#99208,#79044,#79045);
#72051=AXIS2_PLACEMENT_3D('',#99216,#79046,#79047);
#72052=AXIS2_PLACEMENT_3D('',#99233,#79048,#79049);
#72053=AXIS2_PLACEMENT_3D('',#99241,#79050,#79051);
#72054=AXIS2_PLACEMENT_3D('',#99258,#79052,#79053);
#72055=AXIS2_PLACEMENT_3D('',#99266,#79054,#79055);
#72056=AXIS2_PLACEMENT_3D('',#99283,#79056,#79057);
#72057=AXIS2_PLACEMENT_3D('',#99291,#79058,#79059);
#72058=AXIS2_PLACEMENT_3D('',#99308,#79060,#79061);
#72059=AXIS2_PLACEMENT_3D('',#99316,#79062,#79063);
#72060=AXIS2_PLACEMENT_3D('',#99333,#79064,#79065);
#72061=AXIS2_PLACEMENT_3D('',#99341,#79066,#79067);
#72062=AXIS2_PLACEMENT_3D('',#99358,#79068,#79069);
#72063=AXIS2_PLACEMENT_3D('',#99366,#79070,#79071);
#72064=AXIS2_PLACEMENT_3D('',#99383,#79072,#79073);
#72065=AXIS2_PLACEMENT_3D('',#99391,#79074,#79075);
#72066=AXIS2_PLACEMENT_3D('',#99408,#79076,#79077);
#72067=AXIS2_PLACEMENT_3D('',#99416,#79078,#79079);
#72068=AXIS2_PLACEMENT_3D('',#99433,#79080,#79081);
#72069=AXIS2_PLACEMENT_3D('',#99441,#79082,#79083);
#72070=AXIS2_PLACEMENT_3D('',#99458,#79084,#79085);
#72071=AXIS2_PLACEMENT_3D('',#99466,#79086,#79087);
#72072=AXIS2_PLACEMENT_3D('',#99483,#79088,#79089);
#72073=AXIS2_PLACEMENT_3D('',#99491,#79090,#79091);
#72074=AXIS2_PLACEMENT_3D('',#99508,#79092,#79093);
#72075=AXIS2_PLACEMENT_3D('',#99516,#79094,#79095);
#72076=AXIS2_PLACEMENT_3D('',#99533,#79096,#79097);
#72077=AXIS2_PLACEMENT_3D('',#99541,#79098,#79099);
#72078=AXIS2_PLACEMENT_3D('',#99558,#79100,#79101);
#72079=AXIS2_PLACEMENT_3D('',#99566,#79102,#79103);
#72080=AXIS2_PLACEMENT_3D('',#99583,#79104,#79105);
#72081=AXIS2_PLACEMENT_3D('',#99591,#79106,#79107);
#72082=AXIS2_PLACEMENT_3D('',#99608,#79108,#79109);
#72083=AXIS2_PLACEMENT_3D('',#99616,#79110,#79111);
#72084=AXIS2_PLACEMENT_3D('',#99633,#79112,#79113);
#72085=AXIS2_PLACEMENT_3D('',#99641,#79114,#79115);
#72086=AXIS2_PLACEMENT_3D('',#99658,#79116,#79117);
#72087=AXIS2_PLACEMENT_3D('',#99666,#79118,#79119);
#72088=AXIS2_PLACEMENT_3D('',#99683,#79120,#79121);
#72089=AXIS2_PLACEMENT_3D('',#99690,#79122,#79123);
#72090=AXIS2_PLACEMENT_3D('',#99699,#79124,#79125);
#72091=AXIS2_PLACEMENT_3D('',#99707,#79127,#79128);
#72092=AXIS2_PLACEMENT_3D('',#99709,#79129,#79130);
#72093=AXIS2_PLACEMENT_3D('',#99748,#79132,#79133);
#72094=AXIS2_PLACEMENT_3D('',#99756,#79135,#79136);
#72095=AXIS2_PLACEMENT_3D('',#99758,#79137,#79138);
#72096=AXIS2_PLACEMENT_3D('',#99797,#79140,#79141);
#72097=AXIS2_PLACEMENT_3D('',#99805,#79143,#79144);
#72098=AXIS2_PLACEMENT_3D('',#99807,#79145,#79146);
#72099=AXIS2_PLACEMENT_3D('',#99846,#79148,#79149);
#72100=AXIS2_PLACEMENT_3D('',#99854,#79151,#79152);
#72101=AXIS2_PLACEMENT_3D('',#99856,#79153,#79154);
#72102=AXIS2_PLACEMENT_3D('',#99895,#79156,#79157);
#72103=AXIS2_PLACEMENT_3D('',#99903,#79159,#79160);
#72104=AXIS2_PLACEMENT_3D('',#99905,#79161,#79162);
#72105=AXIS2_PLACEMENT_3D('',#99944,#79164,#79165);
#72106=AXIS2_PLACEMENT_3D('',#99952,#79167,#79168);
#72107=AXIS2_PLACEMENT_3D('',#99954,#79169,#79170);
#72108=AXIS2_PLACEMENT_3D('',#99993,#79172,#79173);
#72109=AXIS2_PLACEMENT_3D('',#100001,#79175,#79176);
#72110=AXIS2_PLACEMENT_3D('',#100003,#79177,#79178);
#72111=AXIS2_PLACEMENT_3D('',#100042,#79180,#79181);
#72112=AXIS2_PLACEMENT_3D('',#100050,#79183,#79184);
#72113=AXIS2_PLACEMENT_3D('',#100052,#79185,#79186);
#72114=AXIS2_PLACEMENT_3D('',#100091,#79188,#79189);
#72115=AXIS2_PLACEMENT_3D('',#100099,#79191,#79192);
#72116=AXIS2_PLACEMENT_3D('',#100101,#79193,#79194);
#72117=AXIS2_PLACEMENT_3D('',#100140,#79196,#79197);
#72118=AXIS2_PLACEMENT_3D('',#100148,#79199,#79200);
#72119=AXIS2_PLACEMENT_3D('',#100150,#79201,#79202);
#72120=AXIS2_PLACEMENT_3D('',#100189,#79204,#79205);
#72121=AXIS2_PLACEMENT_3D('',#100197,#79207,#79208);
#72122=AXIS2_PLACEMENT_3D('',#100199,#79209,#79210);
#72123=AXIS2_PLACEMENT_3D('',#100238,#79212,#79213);
#72124=AXIS2_PLACEMENT_3D('',#100246,#79215,#79216);
#72125=AXIS2_PLACEMENT_3D('',#100248,#79217,#79218);
#72126=AXIS2_PLACEMENT_3D('',#100287,#79220,#79221);
#72127=AXIS2_PLACEMENT_3D('',#100295,#79223,#79224);
#72128=AXIS2_PLACEMENT_3D('',#100297,#79225,#79226);
#72129=AXIS2_PLACEMENT_3D('',#100336,#79228,#79229);
#72130=AXIS2_PLACEMENT_3D('',#100344,#79231,#79232);
#72131=AXIS2_PLACEMENT_3D('',#100346,#79233,#79234);
#72132=AXIS2_PLACEMENT_3D('',#100413,#79238,#79239);
#72133=AXIS2_PLACEMENT_3D('',#100421,#79241,#79242);
#72134=AXIS2_PLACEMENT_3D('',#100423,#79243,#79244);
#72135=AXIS2_PLACEMENT_3D('',#100462,#79246,#79247);
#72136=AXIS2_PLACEMENT_3D('',#100470,#79249,#79250);
#72137=AXIS2_PLACEMENT_3D('',#100472,#79251,#79252);
#72138=AXIS2_PLACEMENT_3D('',#100511,#79254,#79255);
#72139=AXIS2_PLACEMENT_3D('',#100519,#79257,#79258);
#72140=AXIS2_PLACEMENT_3D('',#100521,#79259,#79260);
#72141=AXIS2_PLACEMENT_3D('',#100560,#79262,#79263);
#72142=AXIS2_PLACEMENT_3D('',#100568,#79265,#79266);
#72143=AXIS2_PLACEMENT_3D('',#100570,#79267,#79268);
#72144=AXIS2_PLACEMENT_3D('',#100609,#79270,#79271);
#72145=AXIS2_PLACEMENT_3D('',#100617,#79273,#79274);
#72146=AXIS2_PLACEMENT_3D('',#100619,#79275,#79276);
#72147=AXIS2_PLACEMENT_3D('',#100658,#79278,#79279);
#72148=AXIS2_PLACEMENT_3D('',#100666,#79281,#79282);
#72149=AXIS2_PLACEMENT_3D('',#100668,#79283,#79284);
#72150=AXIS2_PLACEMENT_3D('',#100707,#79286,#79287);
#72151=AXIS2_PLACEMENT_3D('',#100715,#79289,#79290);
#72152=AXIS2_PLACEMENT_3D('',#100717,#79291,#79292);
#72153=AXIS2_PLACEMENT_3D('',#100756,#79294,#79295);
#72154=AXIS2_PLACEMENT_3D('',#100764,#79297,#79298);
#72155=AXIS2_PLACEMENT_3D('',#100766,#79299,#79300);
#72156=AXIS2_PLACEMENT_3D('',#100805,#79302,#79303);
#72157=AXIS2_PLACEMENT_3D('',#100813,#79305,#79306);
#72158=AXIS2_PLACEMENT_3D('',#100815,#79307,#79308);
#72159=AXIS2_PLACEMENT_3D('',#100854,#79310,#79311);
#72160=AXIS2_PLACEMENT_3D('',#100885,#79314,#79315);
#72161=AXIS2_PLACEMENT_3D('',#100887,#79316,#79317);
#72162=AXIS2_PLACEMENT_3D('',#100904,#79319,#79320);
#72163=AXIS2_PLACEMENT_3D('',#100911,#79321,#79322);
#72164=AXIS2_PLACEMENT_3D('',#100921,#79323,#79324);
#72165=AXIS2_PLACEMENT_3D('',#100952,#79326,#79327);
#72166=AXIS2_PLACEMENT_3D('',#100960,#79329,#79330);
#72167=AXIS2_PLACEMENT_3D('',#100962,#79331,#79332);
#72168=AXIS2_PLACEMENT_3D('',#101001,#79334,#79335);
#72169=AXIS2_PLACEMENT_3D('',#101009,#79337,#79338);
#72170=AXIS2_PLACEMENT_3D('',#101011,#79339,#79340);
#72171=AXIS2_PLACEMENT_3D('',#101050,#79342,#79343);
#72172=AXIS2_PLACEMENT_3D('',#101058,#79345,#79346);
#72173=AXIS2_PLACEMENT_3D('',#101060,#79347,#79348);
#72174=AXIS2_PLACEMENT_3D('',#101104,#79351,#79352);
#72175=AXIS2_PLACEMENT_3D('',#101122,#79353,#79354);
#72176=AXIS2_PLACEMENT_3D('',#101124,#79356,#79357);
#72177=AXIS2_PLACEMENT_3D('',#101126,#79358,#79359);
#72178=AXIS2_PLACEMENT_3D('',#101145,#79361,#79362);
#72179=AXIS2_PLACEMENT_3D('',#101163,#79363,#79364);
#72180=AXIS2_PLACEMENT_3D('',#101165,#79366,#79367);
#72181=AXIS2_PLACEMENT_3D('',#101167,#79368,#79369);
#72182=AXIS2_PLACEMENT_3D('',#101186,#79371,#79372);
#72183=AXIS2_PLACEMENT_3D('',#101204,#79373,#79374);
#72184=AXIS2_PLACEMENT_3D('',#101206,#79376,#79377);
#72185=AXIS2_PLACEMENT_3D('',#101208,#79378,#79379);
#72186=AXIS2_PLACEMENT_3D('',#101227,#79381,#79382);
#72187=AXIS2_PLACEMENT_3D('',#101245,#79383,#79384);
#72188=AXIS2_PLACEMENT_3D('',#101247,#79386,#79387);
#72189=AXIS2_PLACEMENT_3D('',#101249,#79388,#79389);
#72190=AXIS2_PLACEMENT_3D('',#101268,#79391,#79392);
#72191=AXIS2_PLACEMENT_3D('',#101286,#79393,#79394);
#72192=AXIS2_PLACEMENT_3D('',#101288,#79396,#79397);
#72193=AXIS2_PLACEMENT_3D('',#101290,#79398,#79399);
#72194=AXIS2_PLACEMENT_3D('',#101309,#79401,#79402);
#72195=AXIS2_PLACEMENT_3D('',#101327,#79403,#79404);
#72196=AXIS2_PLACEMENT_3D('',#101329,#79406,#79407);
#72197=AXIS2_PLACEMENT_3D('',#101331,#79408,#79409);
#72198=AXIS2_PLACEMENT_3D('',#101350,#79411,#79412);
#72199=AXIS2_PLACEMENT_3D('',#101368,#79413,#79414);
#72200=AXIS2_PLACEMENT_3D('',#101370,#79416,#79417);
#72201=AXIS2_PLACEMENT_3D('',#101372,#79418,#79419);
#72202=AXIS2_PLACEMENT_3D('',#101391,#79421,#79422);
#72203=AXIS2_PLACEMENT_3D('',#101409,#79423,#79424);
#72204=AXIS2_PLACEMENT_3D('',#101411,#79426,#79427);
#72205=AXIS2_PLACEMENT_3D('',#101413,#79428,#79429);
#72206=AXIS2_PLACEMENT_3D('',#101432,#79431,#79432);
#72207=AXIS2_PLACEMENT_3D('',#101450,#79433,#79434);
#72208=AXIS2_PLACEMENT_3D('',#101452,#79436,#79437);
#72209=AXIS2_PLACEMENT_3D('',#101454,#79438,#79439);
#72210=AXIS2_PLACEMENT_3D('',#101473,#79441,#79442);
#72211=AXIS2_PLACEMENT_3D('',#101491,#79443,#79444);
#72212=AXIS2_PLACEMENT_3D('',#101493,#79446,#79447);
#72213=AXIS2_PLACEMENT_3D('',#101495,#79448,#79449);
#72214=AXIS2_PLACEMENT_3D('',#101514,#79451,#79452);
#72215=AXIS2_PLACEMENT_3D('',#101532,#79453,#79454);
#72216=AXIS2_PLACEMENT_3D('',#101534,#79456,#79457);
#72217=AXIS2_PLACEMENT_3D('',#101536,#79458,#79459);
#72218=AXIS2_PLACEMENT_3D('',#101555,#79461,#79462);
#72219=AXIS2_PLACEMENT_3D('',#101573,#79463,#79464);
#72220=AXIS2_PLACEMENT_3D('',#101575,#79466,#79467);
#72221=AXIS2_PLACEMENT_3D('',#101577,#79468,#79469);
#72222=AXIS2_PLACEMENT_3D('',#101596,#79471,#79472);
#72223=AXIS2_PLACEMENT_3D('',#101614,#79473,#79474);
#72224=AXIS2_PLACEMENT_3D('',#101616,#79476,#79477);
#72225=AXIS2_PLACEMENT_3D('',#101618,#79478,#79479);
#72226=AXIS2_PLACEMENT_3D('',#101637,#79481,#79482);
#72227=AXIS2_PLACEMENT_3D('',#101655,#79483,#79484);
#72228=AXIS2_PLACEMENT_3D('',#101657,#79486,#79487);
#72229=AXIS2_PLACEMENT_3D('',#101659,#79488,#79489);
#72230=AXIS2_PLACEMENT_3D('',#101678,#79491,#79492);
#72231=AXIS2_PLACEMENT_3D('',#101696,#79493,#79494);
#72232=AXIS2_PLACEMENT_3D('',#101698,#79496,#79497);
#72233=AXIS2_PLACEMENT_3D('',#101700,#79498,#79499);
#72234=AXIS2_PLACEMENT_3D('',#101719,#79501,#79502);
#72235=AXIS2_PLACEMENT_3D('',#101737,#79503,#79504);
#72236=AXIS2_PLACEMENT_3D('',#101739,#79506,#79507);
#72237=AXIS2_PLACEMENT_3D('',#101741,#79508,#79509);
#72238=AXIS2_PLACEMENT_3D('',#101760,#79511,#79512);
#72239=AXIS2_PLACEMENT_3D('',#101778,#79513,#79514);
#72240=AXIS2_PLACEMENT_3D('',#101780,#79516,#79517);
#72241=AXIS2_PLACEMENT_3D('',#101782,#79518,#79519);
#72242=AXIS2_PLACEMENT_3D('',#101801,#79521,#79522);
#72243=AXIS2_PLACEMENT_3D('',#101819,#79523,#79524);
#72244=AXIS2_PLACEMENT_3D('',#101821,#79526,#79527);
#72245=AXIS2_PLACEMENT_3D('',#101823,#79528,#79529);
#72246=AXIS2_PLACEMENT_3D('',#101842,#79531,#79532);
#72247=AXIS2_PLACEMENT_3D('',#101860,#79533,#79534);
#72248=AXIS2_PLACEMENT_3D('',#101862,#79536,#79537);
#72249=AXIS2_PLACEMENT_3D('',#101864,#79538,#79539);
#72250=AXIS2_PLACEMENT_3D('',#101883,#79541,#79542);
#72251=AXIS2_PLACEMENT_3D('',#101901,#79543,#79544);
#72252=AXIS2_PLACEMENT_3D('',#101903,#79546,#79547);
#72253=AXIS2_PLACEMENT_3D('',#101905,#79548,#79549);
#72254=AXIS2_PLACEMENT_3D('',#101924,#79551,#79552);
#72255=AXIS2_PLACEMENT_3D('',#101942,#79553,#79554);
#72256=AXIS2_PLACEMENT_3D('',#101944,#79556,#79557);
#72257=AXIS2_PLACEMENT_3D('',#101946,#79558,#79559);
#72258=AXIS2_PLACEMENT_3D('',#101993,#79563,#79564);
#72259=AXIS2_PLACEMENT_3D('',#102011,#79565,#79566);
#72260=AXIS2_PLACEMENT_3D('',#102013,#79568,#79569);
#72261=AXIS2_PLACEMENT_3D('',#102015,#79570,#79571);
#72262=AXIS2_PLACEMENT_3D('',#102034,#79573,#79574);
#72263=AXIS2_PLACEMENT_3D('',#102052,#79575,#79576);
#72264=AXIS2_PLACEMENT_3D('',#102054,#79578,#79579);
#72265=AXIS2_PLACEMENT_3D('',#102056,#79580,#79581);
#72266=AXIS2_PLACEMENT_3D('',#102075,#79583,#79584);
#72267=AXIS2_PLACEMENT_3D('',#102093,#79585,#79586);
#72268=AXIS2_PLACEMENT_3D('',#102095,#79588,#79589);
#72269=AXIS2_PLACEMENT_3D('',#102097,#79590,#79591);
#72270=AXIS2_PLACEMENT_3D('',#102116,#79593,#79594);
#72271=AXIS2_PLACEMENT_3D('',#102134,#79595,#79596);
#72272=AXIS2_PLACEMENT_3D('',#102136,#79598,#79599);
#72273=AXIS2_PLACEMENT_3D('',#102138,#79600,#79601);
#72274=AXIS2_PLACEMENT_3D('',#102157,#79603,#79604);
#72275=AXIS2_PLACEMENT_3D('',#102175,#79605,#79606);
#72276=AXIS2_PLACEMENT_3D('',#102177,#79608,#79609);
#72277=AXIS2_PLACEMENT_3D('',#102179,#79610,#79611);
#72278=AXIS2_PLACEMENT_3D('',#102198,#79613,#79614);
#72279=AXIS2_PLACEMENT_3D('',#102216,#79615,#79616);
#72280=AXIS2_PLACEMENT_3D('',#102218,#79618,#79619);
#72281=AXIS2_PLACEMENT_3D('',#102220,#79620,#79621);
#72282=AXIS2_PLACEMENT_3D('',#102239,#79623,#79624);
#72283=AXIS2_PLACEMENT_3D('',#102257,#79625,#79626);
#72284=AXIS2_PLACEMENT_3D('',#102259,#79628,#79629);
#72285=AXIS2_PLACEMENT_3D('',#102261,#79630,#79631);
#72286=AXIS2_PLACEMENT_3D('',#102274,#79632,#79633);
#72287=AXIS2_PLACEMENT_3D('',#102309,#79634,#79635);
#72288=AXIS2_PLACEMENT_3D('',#102344,#79636,#79637);
#72289=AXIS2_PLACEMENT_3D('',#102379,#79638,#79639);
#72290=AXIS2_PLACEMENT_3D('',#102414,#79640,#79641);
#72291=AXIS2_PLACEMENT_3D('',#102449,#79642,#79643);
#72292=AXIS2_PLACEMENT_3D('',#102484,#79644,#79645);
#72293=AXIS2_PLACEMENT_3D('',#102519,#79646,#79647);
#72294=AXIS2_PLACEMENT_3D('',#102554,#79648,#79649);
#72295=AXIS2_PLACEMENT_3D('',#102589,#79650,#79651);
#72296=AXIS2_PLACEMENT_3D('',#102624,#79652,#79653);
#72297=AXIS2_PLACEMENT_3D('',#102659,#79654,#79655);
#72298=AXIS2_PLACEMENT_3D('',#102694,#79656,#79657);
#72299=AXIS2_PLACEMENT_3D('',#102729,#79658,#79659);
#72300=AXIS2_PLACEMENT_3D('',#102764,#79660,#79661);
#72301=AXIS2_PLACEMENT_3D('',#102799,#79662,#79663);
#72302=AXIS2_PLACEMENT_3D('',#102834,#79664,#79665);
#72303=AXIS2_PLACEMENT_3D('',#102869,#79666,#79667);
#72304=AXIS2_PLACEMENT_3D('',#102904,#79668,#79669);
#72305=AXIS2_PLACEMENT_3D('',#102939,#79670,#79671);
#72306=AXIS2_PLACEMENT_3D('',#102974,#79672,#79673);
#72307=AXIS2_PLACEMENT_3D('',#103009,#79674,#79675);
#72308=AXIS2_PLACEMENT_3D('',#103044,#79676,#79677);
#72309=AXIS2_PLACEMENT_3D('',#103079,#79678,#79679);
#72310=AXIS2_PLACEMENT_3D('',#103114,#79680,#79681);
#72311=AXIS2_PLACEMENT_3D('',#103149,#79682,#79683);
#72312=AXIS2_PLACEMENT_3D('',#103184,#79684,#79685);
#72313=AXIS2_PLACEMENT_3D('',#103219,#79686,#79687);
#72314=AXIS2_PLACEMENT_3D('',#103254,#79688,#79689);
#72315=AXIS2_PLACEMENT_3D('',#103289,#79690,#79691);
#72316=AXIS2_PLACEMENT_3D('',#103320,#79692,#79693);
#72317=AXIS2_PLACEMENT_3D('',#103351,#79694,#79695);
#72318=AXIS2_PLACEMENT_3D('',#103382,#79696,#79697);
#72319=AXIS2_PLACEMENT_3D('',#103413,#79698,#79699);
#72320=AXIS2_PLACEMENT_3D('',#103444,#79700,#79701);
#72321=AXIS2_PLACEMENT_3D('',#103475,#79702,#79703);
#72322=AXIS2_PLACEMENT_3D('',#103506,#79704,#79705);
#72323=AXIS2_PLACEMENT_3D('',#103537,#79706,#79707);
#72324=AXIS2_PLACEMENT_3D('',#103568,#79708,#79709);
#72325=AXIS2_PLACEMENT_3D('',#103599,#79710,#79711);
#72326=AXIS2_PLACEMENT_3D('',#103630,#79712,#79713);
#72327=AXIS2_PLACEMENT_3D('',#103661,#79714,#79715);
#72328=AXIS2_PLACEMENT_3D('',#103692,#79716,#79717);
#72329=AXIS2_PLACEMENT_3D('',#103723,#79718,#79719);
#72330=AXIS2_PLACEMENT_3D('',#103754,#79720,#79721);
#72331=AXIS2_PLACEMENT_3D('',#103785,#79722,#79723);
#72332=AXIS2_PLACEMENT_3D('',#103816,#79724,#79725);
#72333=AXIS2_PLACEMENT_3D('',#103847,#79726,#79727);
#72334=AXIS2_PLACEMENT_3D('',#103878,#79728,#79729);
#72335=AXIS2_PLACEMENT_3D('',#103909,#79730,#79731);
#72336=AXIS2_PLACEMENT_3D('',#103940,#79732,#79733);
#72337=AXIS2_PLACEMENT_3D('',#103971,#79734,#79735);
#72338=AXIS2_PLACEMENT_3D('',#104002,#79736,#79737);
#72339=AXIS2_PLACEMENT_3D('',#104033,#79738,#79739);
#72340=AXIS2_PLACEMENT_3D('',#104064,#79740,#79741);
#72341=AXIS2_PLACEMENT_3D('',#104095,#79742,#79743);
#72342=AXIS2_PLACEMENT_3D('',#104126,#79744,#79745);
#72343=AXIS2_PLACEMENT_3D('',#104157,#79746,#79747);
#72344=AXIS2_PLACEMENT_3D('',#104189,#79748,#79749);
#72345=AXIS2_PLACEMENT_3D('',#104227,#79752,#79753);
#72346=AXIS2_PLACEMENT_3D('',#104229,#79754,#79755);
#72347=AXIS2_PLACEMENT_3D('',#104231,#79756,#79757);
#72348=AXIS2_PLACEMENT_3D('',#104232,#79758,#79759);
#72349=AXIS2_PLACEMENT_3D('',#104270,#79762,#79763);
#72350=AXIS2_PLACEMENT_3D('',#104272,#79764,#79765);
#72351=AXIS2_PLACEMENT_3D('',#104274,#79766,#79767);
#72352=AXIS2_PLACEMENT_3D('',#104275,#79768,#79769);
#72353=AXIS2_PLACEMENT_3D('',#104313,#79772,#79773);
#72354=AXIS2_PLACEMENT_3D('',#104315,#79774,#79775);
#72355=AXIS2_PLACEMENT_3D('',#104317,#79776,#79777);
#72356=AXIS2_PLACEMENT_3D('',#104318,#79778,#79779);
#72357=AXIS2_PLACEMENT_3D('',#104356,#79782,#79783);
#72358=AXIS2_PLACEMENT_3D('',#104358,#79784,#79785);
#72359=AXIS2_PLACEMENT_3D('',#104360,#79786,#79787);
#72360=AXIS2_PLACEMENT_3D('',#104361,#79788,#79789);
#72361=AXIS2_PLACEMENT_3D('',#104399,#79792,#79793);
#72362=AXIS2_PLACEMENT_3D('',#104401,#79794,#79795);
#72363=AXIS2_PLACEMENT_3D('',#104403,#79796,#79797);
#72364=AXIS2_PLACEMENT_3D('',#104404,#79798,#79799);
#72365=AXIS2_PLACEMENT_3D('',#104442,#79802,#79803);
#72366=AXIS2_PLACEMENT_3D('',#104444,#79804,#79805);
#72367=AXIS2_PLACEMENT_3D('',#104446,#79806,#79807);
#72368=AXIS2_PLACEMENT_3D('',#104447,#79808,#79809);
#72369=AXIS2_PLACEMENT_3D('',#104513,#79814,#79815);
#72370=AXIS2_PLACEMENT_3D('',#104515,#79816,#79817);
#72371=AXIS2_PLACEMENT_3D('',#104517,#79818,#79819);
#72372=AXIS2_PLACEMENT_3D('',#104518,#79820,#79821);
#72373=AXIS2_PLACEMENT_3D('',#104556,#79824,#79825);
#72374=AXIS2_PLACEMENT_3D('',#104558,#79826,#79827);
#72375=AXIS2_PLACEMENT_3D('',#104560,#79828,#79829);
#72376=AXIS2_PLACEMENT_3D('',#104561,#79830,#79831);
#72377=AXIS2_PLACEMENT_3D('',#104599,#79834,#79835);
#72378=AXIS2_PLACEMENT_3D('',#104601,#79836,#79837);
#72379=AXIS2_PLACEMENT_3D('',#104603,#79838,#79839);
#72380=AXIS2_PLACEMENT_3D('',#104604,#79840,#79841);
#72381=AXIS2_PLACEMENT_3D('',#104642,#79844,#79845);
#72382=AXIS2_PLACEMENT_3D('',#104644,#79846,#79847);
#72383=AXIS2_PLACEMENT_3D('',#104646,#79848,#79849);
#72384=AXIS2_PLACEMENT_3D('',#104647,#79850,#79851);
#72385=AXIS2_PLACEMENT_3D('',#104685,#79854,#79855);
#72386=AXIS2_PLACEMENT_3D('',#104687,#79856,#79857);
#72387=AXIS2_PLACEMENT_3D('',#104689,#79858,#79859);
#72388=AXIS2_PLACEMENT_3D('',#104690,#79860,#79861);
#72389=AXIS2_PLACEMENT_3D('',#104728,#79864,#79865);
#72390=AXIS2_PLACEMENT_3D('',#104730,#79866,#79867);
#72391=AXIS2_PLACEMENT_3D('',#104732,#79868,#79869);
#72392=AXIS2_PLACEMENT_3D('',#104733,#79870,#79871);
#72393=AXIS2_PLACEMENT_3D('',#104771,#79874,#79875);
#72394=AXIS2_PLACEMENT_3D('',#104773,#79876,#79877);
#72395=AXIS2_PLACEMENT_3D('',#104775,#79878,#79879);
#72396=AXIS2_PLACEMENT_3D('',#104776,#79880,#79881);
#72397=AXIS2_PLACEMENT_3D('',#104814,#79884,#79885);
#72398=AXIS2_PLACEMENT_3D('',#104816,#79886,#79887);
#72399=AXIS2_PLACEMENT_3D('',#104818,#79888,#79889);
#72400=AXIS2_PLACEMENT_3D('',#104819,#79890,#79891);
#72401=AXIS2_PLACEMENT_3D('',#104857,#79894,#79895);
#72402=AXIS2_PLACEMENT_3D('',#104859,#79896,#79897);
#72403=AXIS2_PLACEMENT_3D('',#104861,#79898,#79899);
#72404=AXIS2_PLACEMENT_3D('',#104862,#79900,#79901);
#72405=AXIS2_PLACEMENT_3D('',#104900,#79904,#79905);
#72406=AXIS2_PLACEMENT_3D('',#104902,#79906,#79907);
#72407=AXIS2_PLACEMENT_3D('',#104904,#79908,#79909);
#72408=AXIS2_PLACEMENT_3D('',#104905,#79910,#79911);
#72409=AXIS2_PLACEMENT_3D('',#104943,#79914,#79915);
#72410=AXIS2_PLACEMENT_3D('',#104945,#79916,#79917);
#72411=AXIS2_PLACEMENT_3D('',#104947,#79918,#79919);
#72412=AXIS2_PLACEMENT_3D('',#104948,#79920,#79921);
#72413=AXIS2_PLACEMENT_3D('',#104986,#79924,#79925);
#72414=AXIS2_PLACEMENT_3D('',#104988,#79926,#79927);
#72415=AXIS2_PLACEMENT_3D('',#104990,#79928,#79929);
#72416=AXIS2_PLACEMENT_3D('',#104991,#79930,#79931);
#72417=AXIS2_PLACEMENT_3D('',#105029,#79934,#79935);
#72418=AXIS2_PLACEMENT_3D('',#105031,#79936,#79937);
#72419=AXIS2_PLACEMENT_3D('',#105033,#79938,#79939);
#72420=AXIS2_PLACEMENT_3D('',#105034,#79940,#79941);
#72421=AXIS2_PLACEMENT_3D('',#105072,#79944,#79945);
#72422=AXIS2_PLACEMENT_3D('',#105074,#79946,#79947);
#72423=AXIS2_PLACEMENT_3D('',#105076,#79948,#79949);
#72424=AXIS2_PLACEMENT_3D('',#105077,#79950,#79951);
#72425=AXIS2_PLACEMENT_3D('',#105115,#79954,#79955);
#72426=AXIS2_PLACEMENT_3D('',#105117,#79956,#79957);
#72427=AXIS2_PLACEMENT_3D('',#105119,#79958,#79959);
#72428=AXIS2_PLACEMENT_3D('',#105120,#79960,#79961);
#72429=AXIS2_PLACEMENT_3D('',#105158,#79964,#79965);
#72430=AXIS2_PLACEMENT_3D('',#105160,#79966,#79967);
#72431=AXIS2_PLACEMENT_3D('',#105162,#79968,#79969);
#72432=AXIS2_PLACEMENT_3D('',#105163,#79970,#79971);
#72433=AXIS2_PLACEMENT_3D('',#105208,#79974,#79975);
#72434=AXIS2_PLACEMENT_3D('',#105210,#79977,#79978);
#72435=AXIS2_PLACEMENT_3D('',#105212,#79979,#79980);
#72436=AXIS2_PLACEMENT_3D('',#105213,#79981,#79982);
#72437=AXIS2_PLACEMENT_3D('',#105244,#79984,#79985);
#72438=AXIS2_PLACEMENT_3D('',#105246,#79986,#79987);
#72439=AXIS2_PLACEMENT_3D('',#105248,#79988,#79989);
#72440=AXIS2_PLACEMENT_3D('',#105249,#79990,#79991);
#72441=AXIS2_PLACEMENT_3D('',#105287,#79994,#79995);
#72442=AXIS2_PLACEMENT_3D('',#105289,#79996,#79997);
#72443=AXIS2_PLACEMENT_3D('',#105291,#79998,#79999);
#72444=AXIS2_PLACEMENT_3D('',#105292,#80000,#80001);
#72445=AXIS2_PLACEMENT_3D('',#105330,#80004,#80005);
#72446=AXIS2_PLACEMENT_3D('',#105332,#80006,#80007);
#72447=AXIS2_PLACEMENT_3D('',#105334,#80008,#80009);
#72448=AXIS2_PLACEMENT_3D('',#105335,#80010,#80011);
#72449=AXIS2_PLACEMENT_3D('',#105373,#80014,#80015);
#72450=AXIS2_PLACEMENT_3D('',#105375,#80016,#80017);
#72451=AXIS2_PLACEMENT_3D('',#105377,#80018,#80019);
#72452=AXIS2_PLACEMENT_3D('',#105378,#80020,#80021);
#72453=AXIS2_PLACEMENT_3D('',#105386,#80023,#80024);
#72454=AXIS2_PLACEMENT_3D('',#105389,#80025,#80026);
#72455=AXIS2_PLACEMENT_3D('',#105390,#80027,#80028);
#72456=AXIS2_PLACEMENT_3D('',#105431,#80030,#80031);
#72457=AXIS2_PLACEMENT_3D('',#105474,#80034,#80035);
#72458=AXIS2_PLACEMENT_3D('',#105476,#80037,#80038);
#72459=AXIS2_PLACEMENT_3D('',#105478,#80039,#80040);
#72460=AXIS2_PLACEMENT_3D('',#105479,#80041,#80042);
#72461=AXIS2_PLACEMENT_3D('',#105521,#80044,#80045);
#72462=AXIS2_PLACEMENT_3D('',#105523,#80047,#80048);
#72463=AXIS2_PLACEMENT_3D('',#105525,#80049,#80050);
#72464=AXIS2_PLACEMENT_3D('',#105526,#80051,#80052);
#72465=AXIS2_PLACEMENT_3D('',#105568,#80054,#80055);
#72466=AXIS2_PLACEMENT_3D('',#105570,#80057,#80058);
#72467=AXIS2_PLACEMENT_3D('',#105572,#80059,#80060);
#72468=AXIS2_PLACEMENT_3D('',#105573,#80061,#80062);
#72469=AXIS2_PLACEMENT_3D('',#105615,#80064,#80065);
#72470=AXIS2_PLACEMENT_3D('',#105617,#80067,#80068);
#72471=AXIS2_PLACEMENT_3D('',#105619,#80069,#80070);
#72472=AXIS2_PLACEMENT_3D('',#105620,#80071,#80072);
#72473=AXIS2_PLACEMENT_3D('',#105662,#80074,#80075);
#72474=AXIS2_PLACEMENT_3D('',#105664,#80077,#80078);
#72475=AXIS2_PLACEMENT_3D('',#105666,#80079,#80080);
#72476=AXIS2_PLACEMENT_3D('',#105667,#80081,#80082);
#72477=AXIS2_PLACEMENT_3D('',#105709,#80084,#80085);
#72478=AXIS2_PLACEMENT_3D('',#105711,#80087,#80088);
#72479=AXIS2_PLACEMENT_3D('',#105713,#80089,#80090);
#72480=AXIS2_PLACEMENT_3D('',#105714,#80091,#80092);
#72481=AXIS2_PLACEMENT_3D('',#105756,#80094,#80095);
#72482=AXIS2_PLACEMENT_3D('',#105758,#80097,#80098);
#72483=AXIS2_PLACEMENT_3D('',#105760,#80099,#80100);
#72484=AXIS2_PLACEMENT_3D('',#105761,#80101,#80102);
#72485=AXIS2_PLACEMENT_3D('',#105803,#80104,#80105);
#72486=AXIS2_PLACEMENT_3D('',#105805,#80107,#80108);
#72487=AXIS2_PLACEMENT_3D('',#105807,#80109,#80110);
#72488=AXIS2_PLACEMENT_3D('',#105808,#80111,#80112);
#72489=AXIS2_PLACEMENT_3D('',#105850,#80114,#80115);
#72490=AXIS2_PLACEMENT_3D('',#105852,#80117,#80118);
#72491=AXIS2_PLACEMENT_3D('',#105854,#80119,#80120);
#72492=AXIS2_PLACEMENT_3D('',#105855,#80121,#80122);
#72493=AXIS2_PLACEMENT_3D('',#105897,#80124,#80125);
#72494=AXIS2_PLACEMENT_3D('',#105899,#80127,#80128);
#72495=AXIS2_PLACEMENT_3D('',#105901,#80129,#80130);
#72496=AXIS2_PLACEMENT_3D('',#105902,#80131,#80132);
#72497=AXIS2_PLACEMENT_3D('',#105944,#80134,#80135);
#72498=AXIS2_PLACEMENT_3D('',#105946,#80137,#80138);
#72499=AXIS2_PLACEMENT_3D('',#105948,#80139,#80140);
#72500=AXIS2_PLACEMENT_3D('',#105949,#80141,#80142);
#72501=AXIS2_PLACEMENT_3D('',#105991,#80144,#80145);
#72502=AXIS2_PLACEMENT_3D('',#105993,#80147,#80148);
#72503=AXIS2_PLACEMENT_3D('',#105995,#80149,#80150);
#72504=AXIS2_PLACEMENT_3D('',#105996,#80151,#80152);
#72505=AXIS2_PLACEMENT_3D('',#106038,#80154,#80155);
#72506=AXIS2_PLACEMENT_3D('',#106040,#80157,#80158);
#72507=AXIS2_PLACEMENT_3D('',#106042,#80159,#80160);
#72508=AXIS2_PLACEMENT_3D('',#106043,#80161,#80162);
#72509=AXIS2_PLACEMENT_3D('',#106117,#80166,#80167);
#72510=AXIS2_PLACEMENT_3D('',#106119,#80169,#80170);
#72511=AXIS2_PLACEMENT_3D('',#106121,#80171,#80172);
#72512=AXIS2_PLACEMENT_3D('',#106122,#80173,#80174);
#72513=AXIS2_PLACEMENT_3D('',#106164,#80176,#80177);
#72514=AXIS2_PLACEMENT_3D('',#106166,#80179,#80180);
#72515=AXIS2_PLACEMENT_3D('',#106168,#80181,#80182);
#72516=AXIS2_PLACEMENT_3D('',#106169,#80183,#80184);
#72517=AXIS2_PLACEMENT_3D('',#106211,#80186,#80187);
#72518=AXIS2_PLACEMENT_3D('',#106213,#80189,#80190);
#72519=AXIS2_PLACEMENT_3D('',#106215,#80191,#80192);
#72520=AXIS2_PLACEMENT_3D('',#106216,#80193,#80194);
#72521=AXIS2_PLACEMENT_3D('',#106258,#80196,#80197);
#72522=AXIS2_PLACEMENT_3D('',#106260,#80199,#80200);
#72523=AXIS2_PLACEMENT_3D('',#106262,#80201,#80202);
#72524=AXIS2_PLACEMENT_3D('',#106263,#80203,#80204);
#72525=AXIS2_PLACEMENT_3D('',#106305,#80206,#80207);
#72526=AXIS2_PLACEMENT_3D('',#106307,#80209,#80210);
#72527=AXIS2_PLACEMENT_3D('',#106309,#80211,#80212);
#72528=AXIS2_PLACEMENT_3D('',#106310,#80213,#80214);
#72529=AXIS2_PLACEMENT_3D('',#106352,#80216,#80217);
#72530=AXIS2_PLACEMENT_3D('',#106354,#80219,#80220);
#72531=AXIS2_PLACEMENT_3D('',#106356,#80221,#80222);
#72532=AXIS2_PLACEMENT_3D('',#106357,#80223,#80224);
#72533=AXIS2_PLACEMENT_3D('',#106399,#80226,#80227);
#72534=AXIS2_PLACEMENT_3D('',#106401,#80229,#80230);
#72535=AXIS2_PLACEMENT_3D('',#106403,#80231,#80232);
#72536=AXIS2_PLACEMENT_3D('',#106404,#80233,#80234);
#72537=AXIS2_PLACEMENT_3D('',#106446,#80236,#80237);
#72538=AXIS2_PLACEMENT_3D('',#106448,#80239,#80240);
#72539=AXIS2_PLACEMENT_3D('',#106450,#80241,#80242);
#72540=AXIS2_PLACEMENT_3D('',#106451,#80243,#80244);
#72541=AXIS2_PLACEMENT_3D('',#106493,#80246,#80247);
#72542=AXIS2_PLACEMENT_3D('',#106495,#80249,#80250);
#72543=AXIS2_PLACEMENT_3D('',#106497,#80251,#80252);
#72544=AXIS2_PLACEMENT_3D('',#106498,#80253,#80254);
#72545=AXIS2_PLACEMENT_3D('',#106540,#80256,#80257);
#72546=AXIS2_PLACEMENT_3D('',#106542,#80259,#80260);
#72547=AXIS2_PLACEMENT_3D('',#106544,#80261,#80262);
#72548=AXIS2_PLACEMENT_3D('',#106545,#80263,#80264);
#72549=AXIS2_PLACEMENT_3D('',#106587,#80266,#80267);
#72550=AXIS2_PLACEMENT_3D('',#106589,#80269,#80270);
#72551=AXIS2_PLACEMENT_3D('',#106591,#80271,#80272);
#72552=AXIS2_PLACEMENT_3D('',#106592,#80273,#80274);
#72553=AXIS2_PLACEMENT_3D('',#106634,#80276,#80277);
#72554=AXIS2_PLACEMENT_3D('',#106636,#80279,#80280);
#72555=AXIS2_PLACEMENT_3D('',#106638,#80281,#80282);
#72556=AXIS2_PLACEMENT_3D('',#106639,#80283,#80284);
#72557=AXIS2_PLACEMENT_3D('',#106681,#80286,#80287);
#72558=AXIS2_PLACEMENT_3D('',#106683,#80289,#80290);
#72559=AXIS2_PLACEMENT_3D('',#106685,#80291,#80292);
#72560=AXIS2_PLACEMENT_3D('',#106686,#80293,#80294);
#72561=AXIS2_PLACEMENT_3D('',#106728,#80296,#80297);
#72562=AXIS2_PLACEMENT_3D('',#106730,#80299,#80300);
#72563=AXIS2_PLACEMENT_3D('',#106732,#80301,#80302);
#72564=AXIS2_PLACEMENT_3D('',#106733,#80303,#80304);
#72565=AXIS2_PLACEMENT_3D('',#106734,#80305,#80306);
#72566=AXIS2_PLACEMENT_3D('',#106744,#80307,#80308);
#72567=AXIS2_PLACEMENT_3D('',#106745,#80309,#80310);
#72568=AXIS2_PLACEMENT_3D('',#106768,#80312,#80313);
#72569=AXIS2_PLACEMENT_3D('',#106791,#80314,#80315);
#72570=AXIS2_PLACEMENT_3D('',#106804,#80316,#80317);
#72571=AXIS2_PLACEMENT_3D('',#106821,#80318,#80319);
#72572=AXIS2_PLACEMENT_3D('',#106834,#80320,#80321);
#72573=AXIS2_PLACEMENT_3D('',#106851,#80322,#80323);
#72574=AXIS2_PLACEMENT_3D('',#106864,#80324,#80325);
#72575=AXIS2_PLACEMENT_3D('',#106881,#80326,#80327);
#72576=AXIS2_PLACEMENT_3D('',#106894,#80328,#80329);
#72577=AXIS2_PLACEMENT_3D('',#106911,#80330,#80331);
#72578=AXIS2_PLACEMENT_3D('',#106924,#80332,#80333);
#72579=AXIS2_PLACEMENT_3D('',#106941,#80334,#80335);
#72580=AXIS2_PLACEMENT_3D('',#106954,#80336,#80337);
#72581=AXIS2_PLACEMENT_3D('',#106971,#80338,#80339);
#72582=AXIS2_PLACEMENT_3D('',#106984,#80340,#80341);
#72583=AXIS2_PLACEMENT_3D('',#107001,#80342,#80343);
#72584=AXIS2_PLACEMENT_3D('',#107014,#80344,#80345);
#72585=AXIS2_PLACEMENT_3D('',#107031,#80346,#80347);
#72586=AXIS2_PLACEMENT_3D('',#107044,#80348,#80349);
#72587=AXIS2_PLACEMENT_3D('',#107061,#80350,#80351);
#72588=AXIS2_PLACEMENT_3D('',#107074,#80352,#80353);
#72589=AXIS2_PLACEMENT_3D('',#107091,#80354,#80355);
#72590=AXIS2_PLACEMENT_3D('',#107104,#80356,#80357);
#72591=AXIS2_PLACEMENT_3D('',#107121,#80358,#80359);
#72592=AXIS2_PLACEMENT_3D('',#107134,#80360,#80361);
#72593=AXIS2_PLACEMENT_3D('',#107151,#80362,#80363);
#72594=AXIS2_PLACEMENT_3D('',#107164,#80364,#80365);
#72595=AXIS2_PLACEMENT_3D('',#107181,#80366,#80367);
#72596=AXIS2_PLACEMENT_3D('',#107194,#80368,#80369);
#72597=AXIS2_PLACEMENT_3D('',#107211,#80370,#80371);
#72598=AXIS2_PLACEMENT_3D('',#107224,#80372,#80373);
#72599=AXIS2_PLACEMENT_3D('',#107241,#80374,#80375);
#72600=AXIS2_PLACEMENT_3D('',#107254,#80376,#80377);
#72601=AXIS2_PLACEMENT_3D('',#107271,#80378,#80379);
#72602=AXIS2_PLACEMENT_3D('',#107284,#80380,#80381);
#72603=AXIS2_PLACEMENT_3D('',#107301,#80382,#80383);
#72604=AXIS2_PLACEMENT_3D('',#107314,#80384,#80385);
#72605=AXIS2_PLACEMENT_3D('',#107331,#80386,#80387);
#72606=AXIS2_PLACEMENT_3D('',#107344,#80388,#80389);
#72607=AXIS2_PLACEMENT_3D('',#107361,#80390,#80391);
#72608=AXIS2_PLACEMENT_3D('',#107374,#80392,#80393);
#72609=AXIS2_PLACEMENT_3D('',#107391,#80394,#80395);
#72610=AXIS2_PLACEMENT_3D('',#107404,#80396,#80397);
#72611=AXIS2_PLACEMENT_3D('',#107421,#80398,#80399);
#72612=AXIS2_PLACEMENT_3D('',#107434,#80400,#80401);
#72613=AXIS2_PLACEMENT_3D('',#107451,#80402,#80403);
#72614=AXIS2_PLACEMENT_3D('',#107464,#80404,#80405);
#72615=AXIS2_PLACEMENT_3D('',#107481,#80406,#80407);
#72616=AXIS2_PLACEMENT_3D('',#107494,#80408,#80409);
#72617=AXIS2_PLACEMENT_3D('',#107511,#80410,#80411);
#72618=AXIS2_PLACEMENT_3D('',#107524,#80412,#80413);
#72619=AXIS2_PLACEMENT_3D('',#107541,#80414,#80415);
#72620=AXIS2_PLACEMENT_3D('',#107554,#80416,#80417);
#72621=AXIS2_PLACEMENT_3D('',#107571,#80418,#80419);
#72622=AXIS2_PLACEMENT_3D('',#107584,#80420,#80421);
#72623=AXIS2_PLACEMENT_3D('',#107601,#80422,#80423);
#72624=AXIS2_PLACEMENT_3D('',#107614,#80424,#80425);
#72625=AXIS2_PLACEMENT_3D('',#107630,#80426,#80427);
#72626=AXIS2_PLACEMENT_3D('',#107644,#80428,#80429);
#72627=AXIS2_PLACEMENT_3D('',#107678,#80430,#80431);
#72628=AXIS2_PLACEMENT_3D('',#107712,#80432,#80433);
#72629=AXIS2_PLACEMENT_3D('',#107746,#80434,#80435);
#72630=AXIS2_PLACEMENT_3D('',#107780,#80436,#80437);
#72631=AXIS2_PLACEMENT_3D('',#107814,#80438,#80439);
#72632=AXIS2_PLACEMENT_3D('',#107848,#80440,#80441);
#72633=AXIS2_PLACEMENT_3D('',#107882,#80442,#80443);
#72634=AXIS2_PLACEMENT_3D('',#107916,#80444,#80445);
#72635=AXIS2_PLACEMENT_3D('',#107950,#80446,#80447);
#72636=AXIS2_PLACEMENT_3D('',#107984,#80448,#80449);
#72637=AXIS2_PLACEMENT_3D('',#108018,#80450,#80451);
#72638=AXIS2_PLACEMENT_3D('',#108052,#80452,#80453);
#72639=AXIS2_PLACEMENT_3D('',#108086,#80454,#80455);
#72640=AXIS2_PLACEMENT_3D('',#108120,#80456,#80457);
#72641=AXIS2_PLACEMENT_3D('',#108154,#80458,#80459);
#72642=AXIS2_PLACEMENT_3D('',#108188,#80460,#80461);
#72643=AXIS2_PLACEMENT_3D('',#108222,#80462,#80463);
#72644=AXIS2_PLACEMENT_3D('',#108256,#80464,#80465);
#72645=AXIS2_PLACEMENT_3D('',#108290,#80466,#80467);
#72646=AXIS2_PLACEMENT_3D('',#108324,#80468,#80469);
#72647=AXIS2_PLACEMENT_3D('',#108358,#80470,#80471);
#72648=AXIS2_PLACEMENT_3D('',#108392,#80472,#80473);
#72649=AXIS2_PLACEMENT_3D('',#108426,#80474,#80475);
#72650=AXIS2_PLACEMENT_3D('',#108460,#80476,#80477);
#72651=AXIS2_PLACEMENT_3D('',#108494,#80478,#80479);
#72652=AXIS2_PLACEMENT_3D('',#108528,#80480,#80481);
#72653=AXIS2_PLACEMENT_3D('',#108562,#80482,#80483);
#72654=AXIS2_PLACEMENT_3D('',#108596,#80484,#80485);
#72655=AXIS2_PLACEMENT_3D('',#108624,#80486,#80487);
#72656=AXIS2_PLACEMENT_3D('',#108632,#80489,#80490);
#72657=AXIS2_PLACEMENT_3D('',#108634,#80491,#80492);
#72658=AXIS2_PLACEMENT_3D('',#108636,#80493,#80494);
#72659=AXIS2_PLACEMENT_3D('',#108637,#80495,#80496);
#72660=AXIS2_PLACEMENT_3D('',#108660,#80498,#80499);
#72661=AXIS2_PLACEMENT_3D('',#108668,#80501,#80502);
#72662=AXIS2_PLACEMENT_3D('',#108670,#80503,#80504);
#72663=AXIS2_PLACEMENT_3D('',#108672,#80505,#80506);
#72664=AXIS2_PLACEMENT_3D('',#108673,#80507,#80508);
#72665=AXIS2_PLACEMENT_3D('',#108696,#80510,#80511);
#72666=AXIS2_PLACEMENT_3D('',#108704,#80513,#80514);
#72667=AXIS2_PLACEMENT_3D('',#108706,#80515,#80516);
#72668=AXIS2_PLACEMENT_3D('',#108708,#80517,#80518);
#72669=AXIS2_PLACEMENT_3D('',#108709,#80519,#80520);
#72670=AXIS2_PLACEMENT_3D('',#108732,#80522,#80523);
#72671=AXIS2_PLACEMENT_3D('',#108740,#80525,#80526);
#72672=AXIS2_PLACEMENT_3D('',#108742,#80527,#80528);
#72673=AXIS2_PLACEMENT_3D('',#108744,#80529,#80530);
#72674=AXIS2_PLACEMENT_3D('',#108745,#80531,#80532);
#72675=AXIS2_PLACEMENT_3D('',#108768,#80534,#80535);
#72676=AXIS2_PLACEMENT_3D('',#108776,#80537,#80538);
#72677=AXIS2_PLACEMENT_3D('',#108778,#80539,#80540);
#72678=AXIS2_PLACEMENT_3D('',#108780,#80541,#80542);
#72679=AXIS2_PLACEMENT_3D('',#108781,#80543,#80544);
#72680=AXIS2_PLACEMENT_3D('',#108804,#80546,#80547);
#72681=AXIS2_PLACEMENT_3D('',#108812,#80549,#80550);
#72682=AXIS2_PLACEMENT_3D('',#108814,#80551,#80552);
#72683=AXIS2_PLACEMENT_3D('',#108816,#80553,#80554);
#72684=AXIS2_PLACEMENT_3D('',#108817,#80555,#80556);
#72685=AXIS2_PLACEMENT_3D('',#108840,#80558,#80559);
#72686=AXIS2_PLACEMENT_3D('',#108848,#80561,#80562);
#72687=AXIS2_PLACEMENT_3D('',#108850,#80563,#80564);
#72688=AXIS2_PLACEMENT_3D('',#108852,#80565,#80566);
#72689=AXIS2_PLACEMENT_3D('',#108853,#80567,#80568);
#72690=AXIS2_PLACEMENT_3D('',#108876,#80570,#80571);
#72691=AXIS2_PLACEMENT_3D('',#108884,#80573,#80574);
#72692=AXIS2_PLACEMENT_3D('',#108886,#80575,#80576);
#72693=AXIS2_PLACEMENT_3D('',#108888,#80577,#80578);
#72694=AXIS2_PLACEMENT_3D('',#108889,#80579,#80580);
#72695=AXIS2_PLACEMENT_3D('',#108912,#80582,#80583);
#72696=AXIS2_PLACEMENT_3D('',#108920,#80585,#80586);
#72697=AXIS2_PLACEMENT_3D('',#108922,#80587,#80588);
#72698=AXIS2_PLACEMENT_3D('',#108924,#80589,#80590);
#72699=AXIS2_PLACEMENT_3D('',#108925,#80591,#80592);
#72700=AXIS2_PLACEMENT_3D('',#108948,#80594,#80595);
#72701=AXIS2_PLACEMENT_3D('',#108956,#80597,#80598);
#72702=AXIS2_PLACEMENT_3D('',#108958,#80599,#80600);
#72703=AXIS2_PLACEMENT_3D('',#108960,#80601,#80602);
#72704=AXIS2_PLACEMENT_3D('',#108961,#80603,#80604);
#72705=AXIS2_PLACEMENT_3D('',#108984,#80606,#80607);
#72706=AXIS2_PLACEMENT_3D('',#108992,#80609,#80610);
#72707=AXIS2_PLACEMENT_3D('',#108994,#80611,#80612);
#72708=AXIS2_PLACEMENT_3D('',#108996,#80613,#80614);
#72709=AXIS2_PLACEMENT_3D('',#108997,#80615,#80616);
#72710=AXIS2_PLACEMENT_3D('',#109020,#80618,#80619);
#72711=AXIS2_PLACEMENT_3D('',#109028,#80621,#80622);
#72712=AXIS2_PLACEMENT_3D('',#109030,#80623,#80624);
#72713=AXIS2_PLACEMENT_3D('',#109032,#80625,#80626);
#72714=AXIS2_PLACEMENT_3D('',#109033,#80627,#80628);
#72715=AXIS2_PLACEMENT_3D('',#109056,#80630,#80631);
#72716=AXIS2_PLACEMENT_3D('',#109064,#80633,#80634);
#72717=AXIS2_PLACEMENT_3D('',#109066,#80635,#80636);
#72718=AXIS2_PLACEMENT_3D('',#109068,#80637,#80638);
#72719=AXIS2_PLACEMENT_3D('',#109069,#80639,#80640);
#72720=AXIS2_PLACEMENT_3D('',#109092,#80642,#80643);
#72721=AXIS2_PLACEMENT_3D('',#109100,#80645,#80646);
#72722=AXIS2_PLACEMENT_3D('',#109102,#80647,#80648);
#72723=AXIS2_PLACEMENT_3D('',#109104,#80649,#80650);
#72724=AXIS2_PLACEMENT_3D('',#109105,#80651,#80652);
#72725=AXIS2_PLACEMENT_3D('',#109155,#80656,#80657);
#72726=AXIS2_PLACEMENT_3D('',#109163,#80659,#80660);
#72727=AXIS2_PLACEMENT_3D('',#109165,#80661,#80662);
#72728=AXIS2_PLACEMENT_3D('',#109167,#80663,#80664);
#72729=AXIS2_PLACEMENT_3D('',#109168,#80665,#80666);
#72730=AXIS2_PLACEMENT_3D('',#109191,#80668,#80669);
#72731=AXIS2_PLACEMENT_3D('',#109199,#80671,#80672);
#72732=AXIS2_PLACEMENT_3D('',#109201,#80673,#80674);
#72733=AXIS2_PLACEMENT_3D('',#109203,#80675,#80676);
#72734=AXIS2_PLACEMENT_3D('',#109204,#80677,#80678);
#72735=AXIS2_PLACEMENT_3D('',#109227,#80680,#80681);
#72736=AXIS2_PLACEMENT_3D('',#109235,#80683,#80684);
#72737=AXIS2_PLACEMENT_3D('',#109237,#80685,#80686);
#72738=AXIS2_PLACEMENT_3D('',#109239,#80687,#80688);
#72739=AXIS2_PLACEMENT_3D('',#109240,#80689,#80690);
#72740=AXIS2_PLACEMENT_3D('',#109263,#80692,#80693);
#72741=AXIS2_PLACEMENT_3D('',#109271,#80695,#80696);
#72742=AXIS2_PLACEMENT_3D('',#109273,#80697,#80698);
#72743=AXIS2_PLACEMENT_3D('',#109275,#80699,#80700);
#72744=AXIS2_PLACEMENT_3D('',#109276,#80701,#80702);
#72745=AXIS2_PLACEMENT_3D('',#109299,#80704,#80705);
#72746=AXIS2_PLACEMENT_3D('',#109307,#80707,#80708);
#72747=AXIS2_PLACEMENT_3D('',#109309,#80709,#80710);
#72748=AXIS2_PLACEMENT_3D('',#109311,#80711,#80712);
#72749=AXIS2_PLACEMENT_3D('',#109312,#80713,#80714);
#72750=AXIS2_PLACEMENT_3D('',#109335,#80716,#80717);
#72751=AXIS2_PLACEMENT_3D('',#109343,#80719,#80720);
#72752=AXIS2_PLACEMENT_3D('',#109345,#80721,#80722);
#72753=AXIS2_PLACEMENT_3D('',#109347,#80723,#80724);
#72754=AXIS2_PLACEMENT_3D('',#109348,#80725,#80726);
#72755=AXIS2_PLACEMENT_3D('',#109371,#80728,#80729);
#72756=AXIS2_PLACEMENT_3D('',#109379,#80731,#80732);
#72757=AXIS2_PLACEMENT_3D('',#109381,#80733,#80734);
#72758=AXIS2_PLACEMENT_3D('',#109383,#80735,#80736);
#72759=AXIS2_PLACEMENT_3D('',#109384,#80737,#80738);
#72760=AXIS2_PLACEMENT_3D('',#109407,#80740,#80741);
#72761=AXIS2_PLACEMENT_3D('',#109415,#80743,#80744);
#72762=AXIS2_PLACEMENT_3D('',#109417,#80745,#80746);
#72763=AXIS2_PLACEMENT_3D('',#109419,#80747,#80748);
#72764=AXIS2_PLACEMENT_3D('',#109420,#80749,#80750);
#72765=AXIS2_PLACEMENT_3D('',#109443,#80752,#80753);
#72766=AXIS2_PLACEMENT_3D('',#109461,#80755,#80756);
#72767=AXIS2_PLACEMENT_3D('',#109463,#80758,#80759);
#72768=AXIS2_PLACEMENT_3D('',#109465,#80760,#80761);
#72769=AXIS2_PLACEMENT_3D('',#109466,#80762,#80763);
#72770=AXIS2_PLACEMENT_3D('',#109480,#80765,#80766);
#72771=AXIS2_PLACEMENT_3D('',#109487,#80767,#80768);
#72772=AXIS2_PLACEMENT_3D('',#109489,#80769,#80770);
#72773=AXIS2_PLACEMENT_3D('',#109491,#80771,#80772);
#72774=AXIS2_PLACEMENT_3D('',#109492,#80773,#80774);
#72775=AXIS2_PLACEMENT_3D('',#109515,#80776,#80777);
#72776=AXIS2_PLACEMENT_3D('',#109523,#80779,#80780);
#72777=AXIS2_PLACEMENT_3D('',#109525,#80781,#80782);
#72778=AXIS2_PLACEMENT_3D('',#109527,#80783,#80784);
#72779=AXIS2_PLACEMENT_3D('',#109528,#80785,#80786);
#72780=AXIS2_PLACEMENT_3D('',#109551,#80788,#80789);
#72781=AXIS2_PLACEMENT_3D('',#109559,#80791,#80792);
#72782=AXIS2_PLACEMENT_3D('',#109561,#80793,#80794);
#72783=AXIS2_PLACEMENT_3D('',#109563,#80795,#80796);
#72784=AXIS2_PLACEMENT_3D('',#109564,#80797,#80798);
#72785=AXIS2_PLACEMENT_3D('',#109587,#80800,#80801);
#72786=AXIS2_PLACEMENT_3D('',#109595,#80803,#80804);
#72787=AXIS2_PLACEMENT_3D('',#109597,#80805,#80806);
#72788=AXIS2_PLACEMENT_3D('',#109599,#80807,#80808);
#72789=AXIS2_PLACEMENT_3D('',#109600,#80809,#80810);
#72790=AXIS2_PLACEMENT_3D('',#109623,#80812,#80813);
#72791=AXIS2_PLACEMENT_3D('',#109631,#80815,#80816);
#72792=AXIS2_PLACEMENT_3D('',#109633,#80817,#80818);
#72793=AXIS2_PLACEMENT_3D('',#109635,#80819,#80820);
#72794=AXIS2_PLACEMENT_3D('',#109636,#80821,#80822);
#72795=AXIS2_PLACEMENT_3D('',#109656,#80825,#80826);
#72796=AXIS2_PLACEMENT_3D('',#109686,#80828,#80829);
#72797=AXIS2_PLACEMENT_3D('',#109688,#80830,#80831);
#72798=AXIS2_PLACEMENT_3D('',#109689,#80832,#80833);
#72799=AXIS2_PLACEMENT_3D('',#109699,#80835,#80836);
#72800=AXIS2_PLACEMENT_3D('',#109729,#80838,#80839);
#72801=AXIS2_PLACEMENT_3D('',#109731,#80840,#80841);
#72802=AXIS2_PLACEMENT_3D('',#109732,#80842,#80843);
#72803=AXIS2_PLACEMENT_3D('',#109742,#80845,#80846);
#72804=AXIS2_PLACEMENT_3D('',#109772,#80848,#80849);
#72805=AXIS2_PLACEMENT_3D('',#109774,#80850,#80851);
#72806=AXIS2_PLACEMENT_3D('',#109775,#80852,#80853);
#72807=AXIS2_PLACEMENT_3D('',#109785,#80855,#80856);
#72808=AXIS2_PLACEMENT_3D('',#109815,#80858,#80859);
#72809=AXIS2_PLACEMENT_3D('',#109817,#80860,#80861);
#72810=AXIS2_PLACEMENT_3D('',#109818,#80862,#80863);
#72811=AXIS2_PLACEMENT_3D('',#109828,#80865,#80866);
#72812=AXIS2_PLACEMENT_3D('',#109858,#80868,#80869);
#72813=AXIS2_PLACEMENT_3D('',#109860,#80870,#80871);
#72814=AXIS2_PLACEMENT_3D('',#109861,#80872,#80873);
#72815=AXIS2_PLACEMENT_3D('',#109871,#80875,#80876);
#72816=AXIS2_PLACEMENT_3D('',#109901,#80878,#80879);
#72817=AXIS2_PLACEMENT_3D('',#109903,#80880,#80881);
#72818=AXIS2_PLACEMENT_3D('',#109904,#80882,#80883);
#72819=AXIS2_PLACEMENT_3D('',#109914,#80885,#80886);
#72820=AXIS2_PLACEMENT_3D('',#109944,#80888,#80889);
#72821=AXIS2_PLACEMENT_3D('',#109946,#80890,#80891);
#72822=AXIS2_PLACEMENT_3D('',#109947,#80892,#80893);
#72823=AXIS2_PLACEMENT_3D('',#109957,#80895,#80896);
#72824=AXIS2_PLACEMENT_3D('',#109987,#80898,#80899);
#72825=AXIS2_PLACEMENT_3D('',#109989,#80900,#80901);
#72826=AXIS2_PLACEMENT_3D('',#109990,#80902,#80903);
#72827=AXIS2_PLACEMENT_3D('',#110000,#80905,#80906);
#72828=AXIS2_PLACEMENT_3D('',#110030,#80908,#80909);
#72829=AXIS2_PLACEMENT_3D('',#110032,#80910,#80911);
#72830=AXIS2_PLACEMENT_3D('',#110033,#80912,#80913);
#72831=AXIS2_PLACEMENT_3D('',#110043,#80915,#80916);
#72832=AXIS2_PLACEMENT_3D('',#110073,#80918,#80919);
#72833=AXIS2_PLACEMENT_3D('',#110075,#80920,#80921);
#72834=AXIS2_PLACEMENT_3D('',#110076,#80922,#80923);
#72835=AXIS2_PLACEMENT_3D('',#110086,#80925,#80926);
#72836=AXIS2_PLACEMENT_3D('',#110116,#80928,#80929);
#72837=AXIS2_PLACEMENT_3D('',#110118,#80930,#80931);
#72838=AXIS2_PLACEMENT_3D('',#110119,#80932,#80933);
#72839=AXIS2_PLACEMENT_3D('',#110129,#80935,#80936);
#72840=AXIS2_PLACEMENT_3D('',#110159,#80938,#80939);
#72841=AXIS2_PLACEMENT_3D('',#110161,#80940,#80941);
#72842=AXIS2_PLACEMENT_3D('',#110162,#80942,#80943);
#72843=AXIS2_PLACEMENT_3D('',#110172,#80945,#80946);
#72844=AXIS2_PLACEMENT_3D('',#110202,#80948,#80949);
#72845=AXIS2_PLACEMENT_3D('',#110204,#80950,#80951);
#72846=AXIS2_PLACEMENT_3D('',#110205,#80952,#80953);
#72847=AXIS2_PLACEMENT_3D('',#110215,#80955,#80956);
#72848=AXIS2_PLACEMENT_3D('',#110245,#80958,#80959);
#72849=AXIS2_PLACEMENT_3D('',#110247,#80960,#80961);
#72850=AXIS2_PLACEMENT_3D('',#110248,#80962,#80963);
#72851=AXIS2_PLACEMENT_3D('',#110258,#80965,#80966);
#72852=AXIS2_PLACEMENT_3D('',#110288,#80968,#80969);
#72853=AXIS2_PLACEMENT_3D('',#110290,#80970,#80971);
#72854=AXIS2_PLACEMENT_3D('',#110291,#80972,#80973);
#72855=AXIS2_PLACEMENT_3D('',#110301,#80975,#80976);
#72856=AXIS2_PLACEMENT_3D('',#110331,#80978,#80979);
#72857=AXIS2_PLACEMENT_3D('',#110333,#80980,#80981);
#72858=AXIS2_PLACEMENT_3D('',#110334,#80982,#80983);
#72859=AXIS2_PLACEMENT_3D('',#110344,#80985,#80986);
#72860=AXIS2_PLACEMENT_3D('',#110374,#80988,#80989);
#72861=AXIS2_PLACEMENT_3D('',#110376,#80990,#80991);
#72862=AXIS2_PLACEMENT_3D('',#110377,#80992,#80993);
#72863=AXIS2_PLACEMENT_3D('',#110387,#80995,#80996);
#72864=AXIS2_PLACEMENT_3D('',#110417,#80998,#80999);
#72865=AXIS2_PLACEMENT_3D('',#110419,#81000,#81001);
#72866=AXIS2_PLACEMENT_3D('',#110420,#81002,#81003);
#72867=AXIS2_PLACEMENT_3D('',#110430,#81005,#81006);
#72868=AXIS2_PLACEMENT_3D('',#110460,#81008,#81009);
#72869=AXIS2_PLACEMENT_3D('',#110462,#81010,#81011);
#72870=AXIS2_PLACEMENT_3D('',#110463,#81012,#81013);
#72871=AXIS2_PLACEMENT_3D('',#110473,#81015,#81016);
#72872=AXIS2_PLACEMENT_3D('',#110503,#81018,#81019);
#72873=AXIS2_PLACEMENT_3D('',#110505,#81020,#81021);
#72874=AXIS2_PLACEMENT_3D('',#110506,#81022,#81023);
#72875=AXIS2_PLACEMENT_3D('',#110516,#81025,#81026);
#72876=AXIS2_PLACEMENT_3D('',#110546,#81028,#81029);
#72877=AXIS2_PLACEMENT_3D('',#110548,#81030,#81031);
#72878=AXIS2_PLACEMENT_3D('',#110549,#81032,#81033);
#72879=AXIS2_PLACEMENT_3D('',#110559,#81035,#81036);
#72880=AXIS2_PLACEMENT_3D('',#110589,#81038,#81039);
#72881=AXIS2_PLACEMENT_3D('',#110591,#81040,#81041);
#72882=AXIS2_PLACEMENT_3D('',#110592,#81042,#81043);
#72883=AXIS2_PLACEMENT_3D('',#110602,#81045,#81046);
#72884=AXIS2_PLACEMENT_3D('',#110632,#81048,#81049);
#72885=AXIS2_PLACEMENT_3D('',#110634,#81050,#81051);
#72886=AXIS2_PLACEMENT_3D('',#110635,#81052,#81053);
#72887=AXIS2_PLACEMENT_3D('',#110645,#81055,#81056);
#72888=AXIS2_PLACEMENT_3D('',#110675,#81058,#81059);
#72889=AXIS2_PLACEMENT_3D('',#110677,#81060,#81061);
#72890=AXIS2_PLACEMENT_3D('',#110678,#81062,#81063);
#72891=AXIS2_PLACEMENT_3D('',#110688,#81065,#81066);
#72892=AXIS2_PLACEMENT_3D('',#110718,#81068,#81069);
#72893=AXIS2_PLACEMENT_3D('',#110720,#81070,#81071);
#72894=AXIS2_PLACEMENT_3D('',#110721,#81072,#81073);
#72895=AXIS2_PLACEMENT_3D('',#110731,#81075,#81076);
#72896=AXIS2_PLACEMENT_3D('',#110761,#81078,#81079);
#72897=AXIS2_PLACEMENT_3D('',#110763,#81080,#81081);
#72898=AXIS2_PLACEMENT_3D('',#110764,#81082,#81083);
#72899=AXIS2_PLACEMENT_3D('',#110774,#81085,#81086);
#72900=AXIS2_PLACEMENT_3D('',#110804,#81088,#81089);
#72901=AXIS2_PLACEMENT_3D('',#110806,#81090,#81091);
#72902=AXIS2_PLACEMENT_3D('',#110807,#81092,#81093);
#72903=AXIS2_PLACEMENT_3D('',#110817,#81095,#81096);
#72904=AXIS2_PLACEMENT_3D('',#110847,#81098,#81099);
#72905=AXIS2_PLACEMENT_3D('',#110849,#81100,#81101);
#72906=AXIS2_PLACEMENT_3D('',#110850,#81102,#81103);
#72907=AXIS2_PLACEMENT_3D('',#110860,#81105,#81106);
#72908=AXIS2_PLACEMENT_3D('',#110890,#81108,#81109);
#72909=AXIS2_PLACEMENT_3D('',#110892,#81110,#81111);
#72910=AXIS2_PLACEMENT_3D('',#110893,#81112,#81113);
#72911=AXIS2_PLACEMENT_3D('',#110905,#81114,#81115);
#72912=AXIS2_PLACEMENT_3D('',#110918,#81116,#81117);
#72913=AXIS2_PLACEMENT_3D('',#110930,#81118,#81119);
#72914=AXIS2_PLACEMENT_3D('',#110943,#81120,#81121);
#72915=AXIS2_PLACEMENT_3D('',#110955,#81122,#81123);
#72916=AXIS2_PLACEMENT_3D('',#110968,#81124,#81125);
#72917=AXIS2_PLACEMENT_3D('',#110980,#81126,#81127);
#72918=AXIS2_PLACEMENT_3D('',#110993,#81128,#81129);
#72919=AXIS2_PLACEMENT_3D('',#111005,#81130,#81131);
#72920=AXIS2_PLACEMENT_3D('',#111018,#81132,#81133);
#72921=AXIS2_PLACEMENT_3D('',#111030,#81134,#81135);
#72922=AXIS2_PLACEMENT_3D('',#111043,#81136,#81137);
#72923=AXIS2_PLACEMENT_3D('',#111055,#81138,#81139);
#72924=AXIS2_PLACEMENT_3D('',#111068,#81140,#81141);
#72925=AXIS2_PLACEMENT_3D('',#111080,#81142,#81143);
#72926=AXIS2_PLACEMENT_3D('',#111093,#81144,#81145);
#72927=AXIS2_PLACEMENT_3D('',#111105,#81146,#81147);
#72928=AXIS2_PLACEMENT_3D('',#111118,#81148,#81149);
#72929=AXIS2_PLACEMENT_3D('',#111130,#81150,#81151);
#72930=AXIS2_PLACEMENT_3D('',#111143,#81152,#81153);
#72931=AXIS2_PLACEMENT_3D('',#111155,#81154,#81155);
#72932=AXIS2_PLACEMENT_3D('',#111168,#81156,#81157);
#72933=AXIS2_PLACEMENT_3D('',#111180,#81158,#81159);
#72934=AXIS2_PLACEMENT_3D('',#111193,#81160,#81161);
#72935=AXIS2_PLACEMENT_3D('',#111205,#81162,#81163);
#72936=AXIS2_PLACEMENT_3D('',#111218,#81164,#81165);
#72937=AXIS2_PLACEMENT_3D('',#111230,#81166,#81167);
#72938=AXIS2_PLACEMENT_3D('',#111243,#81168,#81169);
#72939=AXIS2_PLACEMENT_3D('',#111255,#81170,#81171);
#72940=AXIS2_PLACEMENT_3D('',#111268,#81172,#81173);
#72941=AXIS2_PLACEMENT_3D('',#111280,#81174,#81175);
#72942=AXIS2_PLACEMENT_3D('',#111293,#81176,#81177);
#72943=AXIS2_PLACEMENT_3D('',#111305,#81178,#81179);
#72944=AXIS2_PLACEMENT_3D('',#111318,#81180,#81181);
#72945=AXIS2_PLACEMENT_3D('',#111330,#81182,#81183);
#72946=AXIS2_PLACEMENT_3D('',#111343,#81184,#81185);
#72947=AXIS2_PLACEMENT_3D('',#111355,#81186,#81187);
#72948=AXIS2_PLACEMENT_3D('',#111368,#81188,#81189);
#72949=AXIS2_PLACEMENT_3D('',#111380,#81190,#81191);
#72950=AXIS2_PLACEMENT_3D('',#111393,#81192,#81193);
#72951=AXIS2_PLACEMENT_3D('',#111405,#81194,#81195);
#72952=AXIS2_PLACEMENT_3D('',#111418,#81196,#81197);
#72953=AXIS2_PLACEMENT_3D('',#111430,#81198,#81199);
#72954=AXIS2_PLACEMENT_3D('',#111443,#81200,#81201);
#72955=AXIS2_PLACEMENT_3D('',#111455,#81202,#81203);
#72956=AXIS2_PLACEMENT_3D('',#111468,#81204,#81205);
#72957=AXIS2_PLACEMENT_3D('',#111480,#81206,#81207);
#72958=AXIS2_PLACEMENT_3D('',#111493,#81208,#81209);
#72959=AXIS2_PLACEMENT_3D('',#111505,#81210,#81211);
#72960=AXIS2_PLACEMENT_3D('',#111518,#81212,#81213);
#72961=AXIS2_PLACEMENT_3D('',#111530,#81214,#81215);
#72962=AXIS2_PLACEMENT_3D('',#111543,#81216,#81217);
#72963=AXIS2_PLACEMENT_3D('',#111555,#81218,#81219);
#72964=AXIS2_PLACEMENT_3D('',#111568,#81220,#81221);
#72965=AXIS2_PLACEMENT_3D('',#111580,#81222,#81223);
#72966=AXIS2_PLACEMENT_3D('',#111593,#81224,#81225);
#72967=AXIS2_PLACEMENT_3D('',#111605,#81226,#81227);
#72968=AXIS2_PLACEMENT_3D('',#111618,#81228,#81229);
#72969=AXIS2_PLACEMENT_3D('',#111626,#81230,#81231);
#72970=AXIS2_PLACEMENT_3D('',#111643,#81232,#81233);
#72971=AXIS2_PLACEMENT_3D('',#111651,#81234,#81235);
#72972=AXIS2_PLACEMENT_3D('',#111668,#81236,#81237);
#72973=AXIS2_PLACEMENT_3D('',#111676,#81238,#81239);
#72974=AXIS2_PLACEMENT_3D('',#111693,#81240,#81241);
#72975=AXIS2_PLACEMENT_3D('',#111701,#81242,#81243);
#72976=AXIS2_PLACEMENT_3D('',#111718,#81244,#81245);
#72977=AXIS2_PLACEMENT_3D('',#111726,#81246,#81247);
#72978=AXIS2_PLACEMENT_3D('',#111743,#81248,#81249);
#72979=AXIS2_PLACEMENT_3D('',#111751,#81250,#81251);
#72980=AXIS2_PLACEMENT_3D('',#111768,#81252,#81253);
#72981=AXIS2_PLACEMENT_3D('',#111776,#81254,#81255);
#72982=AXIS2_PLACEMENT_3D('',#111793,#81256,#81257);
#72983=AXIS2_PLACEMENT_3D('',#111801,#81258,#81259);
#72984=AXIS2_PLACEMENT_3D('',#111818,#81260,#81261);
#72985=AXIS2_PLACEMENT_3D('',#111826,#81262,#81263);
#72986=AXIS2_PLACEMENT_3D('',#111843,#81264,#81265);
#72987=AXIS2_PLACEMENT_3D('',#111851,#81266,#81267);
#72988=AXIS2_PLACEMENT_3D('',#111868,#81268,#81269);
#72989=AXIS2_PLACEMENT_3D('',#111876,#81270,#81271);
#72990=AXIS2_PLACEMENT_3D('',#111893,#81272,#81273);
#72991=AXIS2_PLACEMENT_3D('',#111901,#81274,#81275);
#72992=AXIS2_PLACEMENT_3D('',#111918,#81276,#81277);
#72993=AXIS2_PLACEMENT_3D('',#111926,#81278,#81279);
#72994=AXIS2_PLACEMENT_3D('',#111943,#81280,#81281);
#72995=AXIS2_PLACEMENT_3D('',#111951,#81282,#81283);
#72996=AXIS2_PLACEMENT_3D('',#111968,#81284,#81285);
#72997=AXIS2_PLACEMENT_3D('',#111976,#81286,#81287);
#72998=AXIS2_PLACEMENT_3D('',#111993,#81288,#81289);
#72999=AXIS2_PLACEMENT_3D('',#112001,#81290,#81291);
#73000=AXIS2_PLACEMENT_3D('',#112018,#81292,#81293);
#73001=AXIS2_PLACEMENT_3D('',#112026,#81294,#81295);
#73002=AXIS2_PLACEMENT_3D('',#112043,#81296,#81297);
#73003=AXIS2_PLACEMENT_3D('',#112051,#81298,#81299);
#73004=AXIS2_PLACEMENT_3D('',#112068,#81300,#81301);
#73005=AXIS2_PLACEMENT_3D('',#112076,#81302,#81303);
#73006=AXIS2_PLACEMENT_3D('',#112093,#81304,#81305);
#73007=AXIS2_PLACEMENT_3D('',#112101,#81306,#81307);
#73008=AXIS2_PLACEMENT_3D('',#112118,#81308,#81309);
#73009=AXIS2_PLACEMENT_3D('',#112126,#81310,#81311);
#73010=AXIS2_PLACEMENT_3D('',#112143,#81312,#81313);
#73011=AXIS2_PLACEMENT_3D('',#112151,#81314,#81315);
#73012=AXIS2_PLACEMENT_3D('',#112168,#81316,#81317);
#73013=AXIS2_PLACEMENT_3D('',#112176,#81318,#81319);
#73014=AXIS2_PLACEMENT_3D('',#112193,#81320,#81321);
#73015=AXIS2_PLACEMENT_3D('',#112201,#81322,#81323);
#73016=AXIS2_PLACEMENT_3D('',#112218,#81324,#81325);
#73017=AXIS2_PLACEMENT_3D('',#112226,#81326,#81327);
#73018=AXIS2_PLACEMENT_3D('',#112243,#81328,#81329);
#73019=AXIS2_PLACEMENT_3D('',#112251,#81330,#81331);
#73020=AXIS2_PLACEMENT_3D('',#112268,#81332,#81333);
#73021=AXIS2_PLACEMENT_3D('',#112276,#81334,#81335);
#73022=AXIS2_PLACEMENT_3D('',#112293,#81336,#81337);
#73023=AXIS2_PLACEMENT_3D('',#112301,#81338,#81339);
#73024=AXIS2_PLACEMENT_3D('',#112318,#81340,#81341);
#73025=AXIS2_PLACEMENT_3D('',#112326,#81342,#81343);
#73026=AXIS2_PLACEMENT_3D('',#112343,#81344,#81345);
#73027=AXIS2_PLACEMENT_3D('',#112356,#81346,#81347);
#73028=AXIS2_PLACEMENT_3D('',#112376,#81349,#81350);
#73029=AXIS2_PLACEMENT_3D('',#112384,#81352,#81353);
#73030=AXIS2_PLACEMENT_3D('',#112397,#81354,#81355);
#73031=AXIS2_PLACEMENT_3D('',#112398,#81356,#81357);
#73032=AXIS2_PLACEMENT_3D('',#112422,#81359,#81360);
#73033=AXIS2_PLACEMENT_3D('',#112430,#81362,#81363);
#73034=AXIS2_PLACEMENT_3D('',#112443,#81364,#81365);
#73035=AXIS2_PLACEMENT_3D('',#112444,#81366,#81367);
#73036=AXIS2_PLACEMENT_3D('',#112468,#81369,#81370);
#73037=AXIS2_PLACEMENT_3D('',#112476,#81372,#81373);
#73038=AXIS2_PLACEMENT_3D('',#112489,#81374,#81375);
#73039=AXIS2_PLACEMENT_3D('',#112490,#81376,#81377);
#73040=AXIS2_PLACEMENT_3D('',#112514,#81379,#81380);
#73041=AXIS2_PLACEMENT_3D('',#112522,#81382,#81383);
#73042=AXIS2_PLACEMENT_3D('',#112535,#81384,#81385);
#73043=AXIS2_PLACEMENT_3D('',#112536,#81386,#81387);
#73044=AXIS2_PLACEMENT_3D('',#112560,#81389,#81390);
#73045=AXIS2_PLACEMENT_3D('',#112568,#81392,#81393);
#73046=AXIS2_PLACEMENT_3D('',#112581,#81394,#81395);
#73047=AXIS2_PLACEMENT_3D('',#112582,#81396,#81397);
#73048=AXIS2_PLACEMENT_3D('',#112606,#81399,#81400);
#73049=AXIS2_PLACEMENT_3D('',#112614,#81402,#81403);
#73050=AXIS2_PLACEMENT_3D('',#112627,#81404,#81405);
#73051=AXIS2_PLACEMENT_3D('',#112628,#81406,#81407);
#73052=AXIS2_PLACEMENT_3D('',#112680,#81411,#81412);
#73053=AXIS2_PLACEMENT_3D('',#112688,#81414,#81415);
#73054=AXIS2_PLACEMENT_3D('',#112701,#81416,#81417);
#73055=AXIS2_PLACEMENT_3D('',#112702,#81418,#81419);
#73056=AXIS2_PLACEMENT_3D('',#112726,#81421,#81422);
#73057=AXIS2_PLACEMENT_3D('',#112734,#81424,#81425);
#73058=AXIS2_PLACEMENT_3D('',#112747,#81426,#81427);
#73059=AXIS2_PLACEMENT_3D('',#112748,#81428,#81429);
#73060=AXIS2_PLACEMENT_3D('',#112772,#81431,#81432);
#73061=AXIS2_PLACEMENT_3D('',#112780,#81434,#81435);
#73062=AXIS2_PLACEMENT_3D('',#112793,#81436,#81437);
#73063=AXIS2_PLACEMENT_3D('',#112794,#81438,#81439);
#73064=AXIS2_PLACEMENT_3D('',#112818,#81441,#81442);
#73065=AXIS2_PLACEMENT_3D('',#112826,#81444,#81445);
#73066=AXIS2_PLACEMENT_3D('',#112839,#81446,#81447);
#73067=AXIS2_PLACEMENT_3D('',#112840,#81448,#81449);
#73068=AXIS2_PLACEMENT_3D('',#112864,#81451,#81452);
#73069=AXIS2_PLACEMENT_3D('',#112872,#81454,#81455);
#73070=AXIS2_PLACEMENT_3D('',#112885,#81456,#81457);
#73071=AXIS2_PLACEMENT_3D('',#112886,#81458,#81459);
#73072=AXIS2_PLACEMENT_3D('',#112910,#81461,#81462);
#73073=AXIS2_PLACEMENT_3D('',#112918,#81464,#81465);
#73074=AXIS2_PLACEMENT_3D('',#112931,#81466,#81467);
#73075=AXIS2_PLACEMENT_3D('',#112932,#81468,#81469);
#73076=AXIS2_PLACEMENT_3D('',#112956,#81471,#81472);
#73077=AXIS2_PLACEMENT_3D('',#112964,#81474,#81475);
#73078=AXIS2_PLACEMENT_3D('',#112977,#81476,#81477);
#73079=AXIS2_PLACEMENT_3D('',#112978,#81478,#81479);
#73080=AXIS2_PLACEMENT_3D('',#113002,#81481,#81482);
#73081=AXIS2_PLACEMENT_3D('',#113010,#81484,#81485);
#73082=AXIS2_PLACEMENT_3D('',#113023,#81486,#81487);
#73083=AXIS2_PLACEMENT_3D('',#113024,#81488,#81489);
#73084=AXIS2_PLACEMENT_3D('',#113048,#81491,#81492);
#73085=AXIS2_PLACEMENT_3D('',#113056,#81494,#81495);
#73086=AXIS2_PLACEMENT_3D('',#113069,#81496,#81497);
#73087=AXIS2_PLACEMENT_3D('',#113070,#81498,#81499);
#73088=AXIS2_PLACEMENT_3D('',#113094,#81501,#81502);
#73089=AXIS2_PLACEMENT_3D('',#113102,#81504,#81505);
#73090=AXIS2_PLACEMENT_3D('',#113115,#81506,#81507);
#73091=AXIS2_PLACEMENT_3D('',#113116,#81508,#81509);
#73092=AXIS2_PLACEMENT_3D('',#113140,#81511,#81512);
#73093=AXIS2_PLACEMENT_3D('',#113148,#81514,#81515);
#73094=AXIS2_PLACEMENT_3D('',#113161,#81516,#81517);
#73095=AXIS2_PLACEMENT_3D('',#113162,#81518,#81519);
#73096=AXIS2_PLACEMENT_3D('',#113186,#81521,#81522);
#73097=AXIS2_PLACEMENT_3D('',#113194,#81524,#81525);
#73098=AXIS2_PLACEMENT_3D('',#113207,#81526,#81527);
#73099=AXIS2_PLACEMENT_3D('',#113208,#81528,#81529);
#73100=AXIS2_PLACEMENT_3D('',#113232,#81531,#81532);
#73101=AXIS2_PLACEMENT_3D('',#113240,#81534,#81535);
#73102=AXIS2_PLACEMENT_3D('',#113253,#81536,#81537);
#73103=AXIS2_PLACEMENT_3D('',#113254,#81538,#81539);
#73104=AXIS2_PLACEMENT_3D('',#113278,#81541,#81542);
#73105=AXIS2_PLACEMENT_3D('',#113286,#81544,#81545);
#73106=AXIS2_PLACEMENT_3D('',#113299,#81546,#81547);
#73107=AXIS2_PLACEMENT_3D('',#113300,#81548,#81549);
#73108=AXIS2_PLACEMENT_3D('',#113324,#81551,#81552);
#73109=AXIS2_PLACEMENT_3D('',#113332,#81554,#81555);
#73110=AXIS2_PLACEMENT_3D('',#113345,#81556,#81557);
#73111=AXIS2_PLACEMENT_3D('',#113346,#81558,#81559);
#73112=AXIS2_PLACEMENT_3D('',#113370,#81561,#81562);
#73113=AXIS2_PLACEMENT_3D('',#113389,#81564,#81565);
#73114=AXIS2_PLACEMENT_3D('',#113391,#81567,#81568);
#73115=AXIS2_PLACEMENT_3D('',#113403,#81569,#81570);
#73116=AXIS2_PLACEMENT_3D('',#113417,#81572,#81573);
#73117=AXIS2_PLACEMENT_3D('',#113424,#81574,#81575);
#73118=AXIS2_PLACEMENT_3D('',#113426,#81576,#81577);
#73119=AXIS2_PLACEMENT_3D('',#113438,#81578,#81579);
#73120=AXIS2_PLACEMENT_3D('',#113462,#81581,#81582);
#73121=AXIS2_PLACEMENT_3D('',#113470,#81584,#81585);
#73122=AXIS2_PLACEMENT_3D('',#113483,#81586,#81587);
#73123=AXIS2_PLACEMENT_3D('',#113484,#81588,#81589);
#73124=AXIS2_PLACEMENT_3D('',#113508,#81591,#81592);
#73125=AXIS2_PLACEMENT_3D('',#113516,#81594,#81595);
#73126=AXIS2_PLACEMENT_3D('',#113529,#81596,#81597);
#73127=AXIS2_PLACEMENT_3D('',#113530,#81598,#81599);
#73128=AXIS2_PLACEMENT_3D('',#113554,#81601,#81602);
#73129=AXIS2_PLACEMENT_3D('',#113562,#81604,#81605);
#73130=AXIS2_PLACEMENT_3D('',#113575,#81606,#81607);
#73131=AXIS2_PLACEMENT_3D('',#113576,#81608,#81609);
#73132=AXIS2_PLACEMENT_3D('',#113600,#81611,#81612);
#73133=AXIS2_PLACEMENT_3D('',#113608,#81614,#81615);
#73134=AXIS2_PLACEMENT_3D('',#113621,#81616,#81617);
#73135=AXIS2_PLACEMENT_3D('',#113622,#81618,#81619);
#73136=AXIS2_PLACEMENT_3D('',#113634,#81621,#81622);
#73137=AXIS2_PLACEMENT_3D('',#113647,#81623,#81624);
#73138=AXIS2_PLACEMENT_3D('',#113648,#81625,#81626);
#73139=AXIS2_PLACEMENT_3D('',#113672,#81628,#81629);
#73140=AXIS2_PLACEMENT_3D('',#113689,#81632,#81633);
#73141=AXIS2_PLACEMENT_3D('',#113707,#81634,#81635);
#73142=AXIS2_PLACEMENT_3D('',#113709,#81637,#81638);
#73143=AXIS2_PLACEMENT_3D('',#113711,#81639,#81640);
#73144=AXIS2_PLACEMENT_3D('',#113712,#81641,#81642);
#73145=AXIS2_PLACEMENT_3D('',#113722,#81644,#81645);
#73146=AXIS2_PLACEMENT_3D('',#113740,#81646,#81647);
#73147=AXIS2_PLACEMENT_3D('',#113742,#81649,#81650);
#73148=AXIS2_PLACEMENT_3D('',#113744,#81651,#81652);
#73149=AXIS2_PLACEMENT_3D('',#113745,#81653,#81654);
#73150=AXIS2_PLACEMENT_3D('',#113755,#81656,#81657);
#73151=AXIS2_PLACEMENT_3D('',#113773,#81658,#81659);
#73152=AXIS2_PLACEMENT_3D('',#113775,#81661,#81662);
#73153=AXIS2_PLACEMENT_3D('',#113777,#81663,#81664);
#73154=AXIS2_PLACEMENT_3D('',#113778,#81665,#81666);
#73155=AXIS2_PLACEMENT_3D('',#113788,#81668,#81669);
#73156=AXIS2_PLACEMENT_3D('',#113806,#81670,#81671);
#73157=AXIS2_PLACEMENT_3D('',#113808,#81673,#81674);
#73158=AXIS2_PLACEMENT_3D('',#113810,#81675,#81676);
#73159=AXIS2_PLACEMENT_3D('',#113811,#81677,#81678);
#73160=AXIS2_PLACEMENT_3D('',#113821,#81680,#81681);
#73161=AXIS2_PLACEMENT_3D('',#113839,#81682,#81683);
#73162=AXIS2_PLACEMENT_3D('',#113841,#81685,#81686);
#73163=AXIS2_PLACEMENT_3D('',#113843,#81687,#81688);
#73164=AXIS2_PLACEMENT_3D('',#113844,#81689,#81690);
#73165=AXIS2_PLACEMENT_3D('',#113854,#81692,#81693);
#73166=AXIS2_PLACEMENT_3D('',#113872,#81694,#81695);
#73167=AXIS2_PLACEMENT_3D('',#113874,#81697,#81698);
#73168=AXIS2_PLACEMENT_3D('',#113876,#81699,#81700);
#73169=AXIS2_PLACEMENT_3D('',#113877,#81701,#81702);
#73170=AXIS2_PLACEMENT_3D('',#113887,#81704,#81705);
#73171=AXIS2_PLACEMENT_3D('',#113905,#81706,#81707);
#73172=AXIS2_PLACEMENT_3D('',#113907,#81709,#81710);
#73173=AXIS2_PLACEMENT_3D('',#113909,#81711,#81712);
#73174=AXIS2_PLACEMENT_3D('',#113910,#81713,#81714);
#73175=AXIS2_PLACEMENT_3D('',#113920,#81716,#81717);
#73176=AXIS2_PLACEMENT_3D('',#113938,#81718,#81719);
#73177=AXIS2_PLACEMENT_3D('',#113940,#81721,#81722);
#73178=AXIS2_PLACEMENT_3D('',#113942,#81723,#81724);
#73179=AXIS2_PLACEMENT_3D('',#113943,#81725,#81726);
#73180=AXIS2_PLACEMENT_3D('',#113953,#81728,#81729);
#73181=AXIS2_PLACEMENT_3D('',#113971,#81730,#81731);
#73182=AXIS2_PLACEMENT_3D('',#113973,#81733,#81734);
#73183=AXIS2_PLACEMENT_3D('',#113975,#81735,#81736);
#73184=AXIS2_PLACEMENT_3D('',#113976,#81737,#81738);
#73185=AXIS2_PLACEMENT_3D('',#113986,#81740,#81741);
#73186=AXIS2_PLACEMENT_3D('',#114004,#81742,#81743);
#73187=AXIS2_PLACEMENT_3D('',#114006,#81745,#81746);
#73188=AXIS2_PLACEMENT_3D('',#114008,#81747,#81748);
#73189=AXIS2_PLACEMENT_3D('',#114009,#81749,#81750);
#73190=AXIS2_PLACEMENT_3D('',#114019,#81752,#81753);
#73191=AXIS2_PLACEMENT_3D('',#114037,#81754,#81755);
#73192=AXIS2_PLACEMENT_3D('',#114039,#81757,#81758);
#73193=AXIS2_PLACEMENT_3D('',#114041,#81759,#81760);
#73194=AXIS2_PLACEMENT_3D('',#114042,#81761,#81762);
#73195=AXIS2_PLACEMENT_3D('',#114052,#81764,#81765);
#73196=AXIS2_PLACEMENT_3D('',#114070,#81766,#81767);
#73197=AXIS2_PLACEMENT_3D('',#114072,#81769,#81770);
#73198=AXIS2_PLACEMENT_3D('',#114074,#81771,#81772);
#73199=AXIS2_PLACEMENT_3D('',#114075,#81773,#81774);
#73200=AXIS2_PLACEMENT_3D('',#114085,#81776,#81777);
#73201=AXIS2_PLACEMENT_3D('',#114103,#81778,#81779);
#73202=AXIS2_PLACEMENT_3D('',#114105,#81781,#81782);
#73203=AXIS2_PLACEMENT_3D('',#114107,#81783,#81784);
#73204=AXIS2_PLACEMENT_3D('',#114108,#81785,#81786);
#73205=AXIS2_PLACEMENT_3D('',#114142,#81790,#81791);
#73206=AXIS2_PLACEMENT_3D('',#114160,#81792,#81793);
#73207=AXIS2_PLACEMENT_3D('',#114162,#81795,#81796);
#73208=AXIS2_PLACEMENT_3D('',#114164,#81797,#81798);
#73209=AXIS2_PLACEMENT_3D('',#114165,#81799,#81800);
#73210=AXIS2_PLACEMENT_3D('',#114175,#81802,#81803);
#73211=AXIS2_PLACEMENT_3D('',#114193,#81804,#81805);
#73212=AXIS2_PLACEMENT_3D('',#114195,#81807,#81808);
#73213=AXIS2_PLACEMENT_3D('',#114197,#81809,#81810);
#73214=AXIS2_PLACEMENT_3D('',#114198,#81811,#81812);
#73215=AXIS2_PLACEMENT_3D('',#114208,#81814,#81815);
#73216=AXIS2_PLACEMENT_3D('',#114226,#81816,#81817);
#73217=AXIS2_PLACEMENT_3D('',#114228,#81819,#81820);
#73218=AXIS2_PLACEMENT_3D('',#114230,#81821,#81822);
#73219=AXIS2_PLACEMENT_3D('',#114231,#81823,#81824);
#73220=AXIS2_PLACEMENT_3D('',#114241,#81826,#81827);
#73221=AXIS2_PLACEMENT_3D('',#114259,#81828,#81829);
#73222=AXIS2_PLACEMENT_3D('',#114261,#81831,#81832);
#73223=AXIS2_PLACEMENT_3D('',#114263,#81833,#81834);
#73224=AXIS2_PLACEMENT_3D('',#114264,#81835,#81836);
#73225=AXIS2_PLACEMENT_3D('',#114274,#81838,#81839);
#73226=AXIS2_PLACEMENT_3D('',#114292,#81840,#81841);
#73227=AXIS2_PLACEMENT_3D('',#114294,#81843,#81844);
#73228=AXIS2_PLACEMENT_3D('',#114296,#81845,#81846);
#73229=AXIS2_PLACEMENT_3D('',#114297,#81847,#81848);
#73230=AXIS2_PLACEMENT_3D('',#114307,#81850,#81851);
#73231=AXIS2_PLACEMENT_3D('',#114325,#81852,#81853);
#73232=AXIS2_PLACEMENT_3D('',#114327,#81855,#81856);
#73233=AXIS2_PLACEMENT_3D('',#114329,#81857,#81858);
#73234=AXIS2_PLACEMENT_3D('',#114330,#81859,#81860);
#73235=AXIS2_PLACEMENT_3D('',#114340,#81862,#81863);
#73236=AXIS2_PLACEMENT_3D('',#114358,#81864,#81865);
#73237=AXIS2_PLACEMENT_3D('',#114360,#81867,#81868);
#73238=AXIS2_PLACEMENT_3D('',#114362,#81869,#81870);
#73239=AXIS2_PLACEMENT_3D('',#114363,#81871,#81872);
#73240=AXIS2_PLACEMENT_3D('',#114373,#81874,#81875);
#73241=AXIS2_PLACEMENT_3D('',#114391,#81876,#81877);
#73242=AXIS2_PLACEMENT_3D('',#114393,#81879,#81880);
#73243=AXIS2_PLACEMENT_3D('',#114395,#81881,#81882);
#73244=AXIS2_PLACEMENT_3D('',#114396,#81883,#81884);
#73245=AXIS2_PLACEMENT_3D('',#114406,#81886,#81887);
#73246=AXIS2_PLACEMENT_3D('',#114424,#81888,#81889);
#73247=AXIS2_PLACEMENT_3D('',#114426,#81891,#81892);
#73248=AXIS2_PLACEMENT_3D('',#114428,#81893,#81894);
#73249=AXIS2_PLACEMENT_3D('',#114429,#81895,#81896);
#73250=AXIS2_PLACEMENT_3D('',#114439,#81898,#81899);
#73251=AXIS2_PLACEMENT_3D('',#114457,#81900,#81901);
#73252=AXIS2_PLACEMENT_3D('',#114459,#81903,#81904);
#73253=AXIS2_PLACEMENT_3D('',#114461,#81905,#81906);
#73254=AXIS2_PLACEMENT_3D('',#114462,#81907,#81908);
#73255=AXIS2_PLACEMENT_3D('',#114472,#81910,#81911);
#73256=AXIS2_PLACEMENT_3D('',#114490,#81912,#81913);
#73257=AXIS2_PLACEMENT_3D('',#114492,#81915,#81916);
#73258=AXIS2_PLACEMENT_3D('',#114494,#81917,#81918);
#73259=AXIS2_PLACEMENT_3D('',#114495,#81919,#81920);
#73260=AXIS2_PLACEMENT_3D('',#114505,#81922,#81923);
#73261=AXIS2_PLACEMENT_3D('',#114523,#81924,#81925);
#73262=AXIS2_PLACEMENT_3D('',#114525,#81927,#81928);
#73263=AXIS2_PLACEMENT_3D('',#114527,#81929,#81930);
#73264=AXIS2_PLACEMENT_3D('',#114528,#81931,#81932);
#73265=AXIS2_PLACEMENT_3D('',#114538,#81934,#81935);
#73266=AXIS2_PLACEMENT_3D('',#114556,#81936,#81937);
#73267=AXIS2_PLACEMENT_3D('',#114558,#81939,#81940);
#73268=AXIS2_PLACEMENT_3D('',#114560,#81941,#81942);
#73269=AXIS2_PLACEMENT_3D('',#114561,#81943,#81944);
#73270=AXIS2_PLACEMENT_3D('',#114571,#81946,#81947);
#73271=AXIS2_PLACEMENT_3D('',#114589,#81948,#81949);
#73272=AXIS2_PLACEMENT_3D('',#114591,#81951,#81952);
#73273=AXIS2_PLACEMENT_3D('',#114593,#81953,#81954);
#73274=AXIS2_PLACEMENT_3D('',#114594,#81955,#81956);
#73275=AXIS2_PLACEMENT_3D('',#114595,#81957,#81958);
#73276=AXIS2_PLACEMENT_3D('',#114598,#81959,#81960);
#73277=AXIS2_PLACEMENT_3D('',#114599,#81961,#81962);
#73278=AXIS2_PLACEMENT_3D('',#114600,#81963,#81964);
#73279=AXIS2_PLACEMENT_3D('',#114615,#81966,#81967);
#73280=AXIS2_PLACEMENT_3D('',#114652,#81968,#81969);
#73281=AXIS2_PLACEMENT_3D('',#114683,#81970,#81971);
#73282=AXIS2_PLACEMENT_3D('',#114714,#81972,#81973);
#73283=AXIS2_PLACEMENT_3D('',#114745,#81974,#81975);
#73284=AXIS2_PLACEMENT_3D('',#114776,#81976,#81977);
#73285=AXIS2_PLACEMENT_3D('',#114807,#81978,#81979);
#73286=AXIS2_PLACEMENT_3D('',#114838,#81980,#81981);
#73287=AXIS2_PLACEMENT_3D('',#114869,#81982,#81983);
#73288=AXIS2_PLACEMENT_3D('',#114900,#81984,#81985);
#73289=AXIS2_PLACEMENT_3D('',#114931,#81986,#81987);
#73290=AXIS2_PLACEMENT_3D('',#114962,#81988,#81989);
#73291=AXIS2_PLACEMENT_3D('',#114993,#81990,#81991);
#73292=AXIS2_PLACEMENT_3D('',#115024,#81992,#81993);
#73293=AXIS2_PLACEMENT_3D('',#115055,#81994,#81995);
#73294=AXIS2_PLACEMENT_3D('',#115086,#81996,#81997);
#73295=AXIS2_PLACEMENT_3D('',#115117,#81998,#81999);
#73296=AXIS2_PLACEMENT_3D('',#115148,#82000,#82001);
#73297=AXIS2_PLACEMENT_3D('',#115179,#82002,#82003);
#73298=AXIS2_PLACEMENT_3D('',#115210,#82004,#82005);
#73299=AXIS2_PLACEMENT_3D('',#115241,#82006,#82007);
#73300=AXIS2_PLACEMENT_3D('',#115272,#82008,#82009);
#73301=AXIS2_PLACEMENT_3D('',#115303,#82010,#82011);
#73302=AXIS2_PLACEMENT_3D('',#115334,#82012,#82013);
#73303=AXIS2_PLACEMENT_3D('',#115365,#82014,#82015);
#73304=AXIS2_PLACEMENT_3D('',#115396,#82016,#82017);
#73305=AXIS2_PLACEMENT_3D('',#115427,#82018,#82019);
#73306=AXIS2_PLACEMENT_3D('',#115458,#82020,#82021);
#73307=AXIS2_PLACEMENT_3D('',#115489,#82022,#82023);
#73308=AXIS2_PLACEMENT_3D('',#115524,#82024,#82025);
#73309=AXIS2_PLACEMENT_3D('',#115532,#82026,#82027);
#73310=AXIS2_PLACEMENT_3D('',#115549,#82028,#82029);
#73311=AXIS2_PLACEMENT_3D('',#115557,#82030,#82031);
#73312=AXIS2_PLACEMENT_3D('',#115574,#82032,#82033);
#73313=AXIS2_PLACEMENT_3D('',#115582,#82034,#82035);
#73314=AXIS2_PLACEMENT_3D('',#115599,#82036,#82037);
#73315=AXIS2_PLACEMENT_3D('',#115607,#82038,#82039);
#73316=AXIS2_PLACEMENT_3D('',#115624,#82040,#82041);
#73317=AXIS2_PLACEMENT_3D('',#115632,#82042,#82043);
#73318=AXIS2_PLACEMENT_3D('',#115649,#82044,#82045);
#73319=AXIS2_PLACEMENT_3D('',#115657,#82046,#82047);
#73320=AXIS2_PLACEMENT_3D('',#115674,#82048,#82049);
#73321=AXIS2_PLACEMENT_3D('',#115682,#82050,#82051);
#73322=AXIS2_PLACEMENT_3D('',#115699,#82052,#82053);
#73323=AXIS2_PLACEMENT_3D('',#115707,#82054,#82055);
#73324=AXIS2_PLACEMENT_3D('',#115724,#82056,#82057);
#73325=AXIS2_PLACEMENT_3D('',#115732,#82058,#82059);
#73326=AXIS2_PLACEMENT_3D('',#115749,#82060,#82061);
#73327=AXIS2_PLACEMENT_3D('',#115757,#82062,#82063);
#73328=AXIS2_PLACEMENT_3D('',#115774,#82064,#82065);
#73329=AXIS2_PLACEMENT_3D('',#115782,#82066,#82067);
#73330=AXIS2_PLACEMENT_3D('',#115799,#82068,#82069);
#73331=AXIS2_PLACEMENT_3D('',#115807,#82070,#82071);
#73332=AXIS2_PLACEMENT_3D('',#115824,#82072,#82073);
#73333=AXIS2_PLACEMENT_3D('',#115832,#82074,#82075);
#73334=AXIS2_PLACEMENT_3D('',#115849,#82076,#82077);
#73335=AXIS2_PLACEMENT_3D('',#115857,#82078,#82079);
#73336=AXIS2_PLACEMENT_3D('',#115874,#82080,#82081);
#73337=AXIS2_PLACEMENT_3D('',#115882,#82082,#82083);
#73338=AXIS2_PLACEMENT_3D('',#115899,#82084,#82085);
#73339=AXIS2_PLACEMENT_3D('',#115907,#82086,#82087);
#73340=AXIS2_PLACEMENT_3D('',#115924,#82088,#82089);
#73341=AXIS2_PLACEMENT_3D('',#115932,#82090,#82091);
#73342=AXIS2_PLACEMENT_3D('',#115949,#82092,#82093);
#73343=AXIS2_PLACEMENT_3D('',#115957,#82094,#82095);
#73344=AXIS2_PLACEMENT_3D('',#115974,#82096,#82097);
#73345=AXIS2_PLACEMENT_3D('',#115982,#82098,#82099);
#73346=AXIS2_PLACEMENT_3D('',#115999,#82100,#82101);
#73347=AXIS2_PLACEMENT_3D('',#116007,#82102,#82103);
#73348=AXIS2_PLACEMENT_3D('',#116024,#82104,#82105);
#73349=AXIS2_PLACEMENT_3D('',#116032,#82106,#82107);
#73350=AXIS2_PLACEMENT_3D('',#116049,#82108,#82109);
#73351=AXIS2_PLACEMENT_3D('',#116057,#82110,#82111);
#73352=AXIS2_PLACEMENT_3D('',#116074,#82112,#82113);
#73353=AXIS2_PLACEMENT_3D('',#116082,#82114,#82115);
#73354=AXIS2_PLACEMENT_3D('',#116099,#82116,#82117);
#73355=AXIS2_PLACEMENT_3D('',#116107,#82118,#82119);
#73356=AXIS2_PLACEMENT_3D('',#116124,#82120,#82121);
#73357=AXIS2_PLACEMENT_3D('',#116132,#82122,#82123);
#73358=AXIS2_PLACEMENT_3D('',#116149,#82124,#82125);
#73359=AXIS2_PLACEMENT_3D('',#116157,#82126,#82127);
#73360=AXIS2_PLACEMENT_3D('',#116174,#82128,#82129);
#73361=AXIS2_PLACEMENT_3D('',#116182,#82130,#82131);
#73362=AXIS2_PLACEMENT_3D('',#116199,#82132,#82133);
#73363=AXIS2_PLACEMENT_3D('',#116207,#82134,#82135);
#73364=AXIS2_PLACEMENT_3D('',#116224,#82136,#82137);
#73365=AXIS2_PLACEMENT_3D('',#116231,#82138,#82139);
#73366=AXIS2_PLACEMENT_3D('',#116244,#82140,#82141);
#73367=AXIS2_PLACEMENT_3D('',#116252,#82143,#82144);
#73368=AXIS2_PLACEMENT_3D('',#116254,#82145,#82146);
#73369=AXIS2_PLACEMENT_3D('',#116256,#82147,#82148);
#73370=AXIS2_PLACEMENT_3D('',#116291,#82150,#82151);
#73371=AXIS2_PLACEMENT_3D('',#116299,#82153,#82154);
#73372=AXIS2_PLACEMENT_3D('',#116301,#82155,#82156);
#73373=AXIS2_PLACEMENT_3D('',#116303,#82157,#82158);
#73374=AXIS2_PLACEMENT_3D('',#116338,#82160,#82161);
#73375=AXIS2_PLACEMENT_3D('',#116346,#82163,#82164);
#73376=AXIS2_PLACEMENT_3D('',#116348,#82165,#82166);
#73377=AXIS2_PLACEMENT_3D('',#116350,#82167,#82168);
#73378=AXIS2_PLACEMENT_3D('',#116385,#82170,#82171);
#73379=AXIS2_PLACEMENT_3D('',#116393,#82173,#82174);
#73380=AXIS2_PLACEMENT_3D('',#116395,#82175,#82176);
#73381=AXIS2_PLACEMENT_3D('',#116397,#82177,#82178);
#73382=AXIS2_PLACEMENT_3D('',#116432,#82180,#82181);
#73383=AXIS2_PLACEMENT_3D('',#116440,#82183,#82184);
#73384=AXIS2_PLACEMENT_3D('',#116442,#82185,#82186);
#73385=AXIS2_PLACEMENT_3D('',#116444,#82187,#82188);
#73386=AXIS2_PLACEMENT_3D('',#116479,#82190,#82191);
#73387=AXIS2_PLACEMENT_3D('',#116487,#82193,#82194);
#73388=AXIS2_PLACEMENT_3D('',#116489,#82195,#82196);
#73389=AXIS2_PLACEMENT_3D('',#116491,#82197,#82198);
#73390=AXIS2_PLACEMENT_3D('',#116526,#82200,#82201);
#73391=AXIS2_PLACEMENT_3D('',#116534,#82203,#82204);
#73392=AXIS2_PLACEMENT_3D('',#116536,#82205,#82206);
#73393=AXIS2_PLACEMENT_3D('',#116538,#82207,#82208);
#73394=AXIS2_PLACEMENT_3D('',#116573,#82210,#82211);
#73395=AXIS2_PLACEMENT_3D('',#116581,#82213,#82214);
#73396=AXIS2_PLACEMENT_3D('',#116583,#82215,#82216);
#73397=AXIS2_PLACEMENT_3D('',#116585,#82217,#82218);
#73398=AXIS2_PLACEMENT_3D('',#116620,#82220,#82221);
#73399=AXIS2_PLACEMENT_3D('',#116628,#82223,#82224);
#73400=AXIS2_PLACEMENT_3D('',#116630,#82225,#82226);
#73401=AXIS2_PLACEMENT_3D('',#116632,#82227,#82228);
#73402=AXIS2_PLACEMENT_3D('',#116667,#82230,#82231);
#73403=AXIS2_PLACEMENT_3D('',#116675,#82233,#82234);
#73404=AXIS2_PLACEMENT_3D('',#116677,#82235,#82236);
#73405=AXIS2_PLACEMENT_3D('',#116679,#82237,#82238);
#73406=AXIS2_PLACEMENT_3D('',#116714,#82240,#82241);
#73407=AXIS2_PLACEMENT_3D('',#116722,#82243,#82244);
#73408=AXIS2_PLACEMENT_3D('',#116724,#82245,#82246);
#73409=AXIS2_PLACEMENT_3D('',#116726,#82247,#82248);
#73410=AXIS2_PLACEMENT_3D('',#116761,#82250,#82251);
#73411=AXIS2_PLACEMENT_3D('',#116769,#82253,#82254);
#73412=AXIS2_PLACEMENT_3D('',#116771,#82255,#82256);
#73413=AXIS2_PLACEMENT_3D('',#116773,#82257,#82258);
#73414=AXIS2_PLACEMENT_3D('',#116808,#82260,#82261);
#73415=AXIS2_PLACEMENT_3D('',#116816,#82263,#82264);
#73416=AXIS2_PLACEMENT_3D('',#116818,#82265,#82266);
#73417=AXIS2_PLACEMENT_3D('',#116820,#82267,#82268);
#73418=AXIS2_PLACEMENT_3D('',#116855,#82270,#82271);
#73419=AXIS2_PLACEMENT_3D('',#116863,#82273,#82274);
#73420=AXIS2_PLACEMENT_3D('',#116865,#82275,#82276);
#73421=AXIS2_PLACEMENT_3D('',#116867,#82277,#82278);
#73422=AXIS2_PLACEMENT_3D('',#116934,#82282,#82283);
#73423=AXIS2_PLACEMENT_3D('',#116942,#82285,#82286);
#73424=AXIS2_PLACEMENT_3D('',#116944,#82287,#82288);
#73425=AXIS2_PLACEMENT_3D('',#116946,#82289,#82290);
#73426=AXIS2_PLACEMENT_3D('',#116981,#82292,#82293);
#73427=AXIS2_PLACEMENT_3D('',#116989,#82295,#82296);
#73428=AXIS2_PLACEMENT_3D('',#116991,#82297,#82298);
#73429=AXIS2_PLACEMENT_3D('',#116993,#82299,#82300);
#73430=AXIS2_PLACEMENT_3D('',#117028,#82302,#82303);
#73431=AXIS2_PLACEMENT_3D('',#117036,#82305,#82306);
#73432=AXIS2_PLACEMENT_3D('',#117038,#82307,#82308);
#73433=AXIS2_PLACEMENT_3D('',#117040,#82309,#82310);
#73434=AXIS2_PLACEMENT_3D('',#117075,#82312,#82313);
#73435=AXIS2_PLACEMENT_3D('',#117083,#82315,#82316);
#73436=AXIS2_PLACEMENT_3D('',#117085,#82317,#82318);
#73437=AXIS2_PLACEMENT_3D('',#117087,#82319,#82320);
#73438=AXIS2_PLACEMENT_3D('',#117122,#82322,#82323);
#73439=AXIS2_PLACEMENT_3D('',#117130,#82325,#82326);
#73440=AXIS2_PLACEMENT_3D('',#117132,#82327,#82328);
#73441=AXIS2_PLACEMENT_3D('',#117134,#82329,#82330);
#73442=AXIS2_PLACEMENT_3D('',#117169,#82332,#82333);
#73443=AXIS2_PLACEMENT_3D('',#117177,#82335,#82336);
#73444=AXIS2_PLACEMENT_3D('',#117179,#82337,#82338);
#73445=AXIS2_PLACEMENT_3D('',#117181,#82339,#82340);
#73446=AXIS2_PLACEMENT_3D('',#117216,#82342,#82343);
#73447=AXIS2_PLACEMENT_3D('',#117224,#82345,#82346);
#73448=AXIS2_PLACEMENT_3D('',#117226,#82347,#82348);
#73449=AXIS2_PLACEMENT_3D('',#117228,#82349,#82350);
#73450=AXIS2_PLACEMENT_3D('',#117263,#82352,#82353);
#73451=AXIS2_PLACEMENT_3D('',#117294,#82356,#82357);
#73452=AXIS2_PLACEMENT_3D('',#117296,#82358,#82359);
#73453=AXIS2_PLACEMENT_3D('',#117297,#82360,#82361);
#73454=AXIS2_PLACEMENT_3D('',#117311,#82363,#82364);
#73455=AXIS2_PLACEMENT_3D('',#117318,#82365,#82366);
#73456=AXIS2_PLACEMENT_3D('',#117328,#82367,#82368);
#73457=AXIS2_PLACEMENT_3D('',#117329,#82369,#82370);
#73458=AXIS2_PLACEMENT_3D('',#117357,#82372,#82373);
#73459=AXIS2_PLACEMENT_3D('',#117365,#82375,#82376);
#73460=AXIS2_PLACEMENT_3D('',#117367,#82377,#82378);
#73461=AXIS2_PLACEMENT_3D('',#117369,#82379,#82380);
#73462=AXIS2_PLACEMENT_3D('',#117404,#82382,#82383);
#73463=AXIS2_PLACEMENT_3D('',#117412,#82385,#82386);
#73464=AXIS2_PLACEMENT_3D('',#117414,#82387,#82388);
#73465=AXIS2_PLACEMENT_3D('',#117416,#82389,#82390);
#73466=AXIS2_PLACEMENT_3D('',#117451,#82392,#82393);
#73467=AXIS2_PLACEMENT_3D('',#117459,#82395,#82396);
#73468=AXIS2_PLACEMENT_3D('',#117461,#82397,#82398);
#73469=AXIS2_PLACEMENT_3D('',#117463,#82399,#82400);
#73470=AXIS2_PLACEMENT_3D('',#117498,#82402,#82403);
#73471=AXIS2_PLACEMENT_3D('',#117506,#82405,#82406);
#73472=AXIS2_PLACEMENT_3D('',#117508,#82407,#82408);
#73473=AXIS2_PLACEMENT_3D('',#117510,#82409,#82410);
#73474=AXIS2_PLACEMENT_3D('',#117545,#82412,#82413);
#73475=AXIS2_PLACEMENT_3D('',#117553,#82415,#82416);
#73476=AXIS2_PLACEMENT_3D('',#117555,#82417,#82418);
#73477=AXIS2_PLACEMENT_3D('',#117557,#82419,#82420);
#73478=AXIS2_PLACEMENT_3D('',#117593,#82423,#82424);
#73479=AXIS2_PLACEMENT_3D('',#117611,#82425,#82426);
#73480=AXIS2_PLACEMENT_3D('',#117613,#82428,#82429);
#73481=AXIS2_PLACEMENT_3D('',#117615,#82430,#82431);
#73482=AXIS2_PLACEMENT_3D('',#117616,#82432,#82433);
#73483=AXIS2_PLACEMENT_3D('',#117630,#82435,#82436);
#73484=AXIS2_PLACEMENT_3D('',#117648,#82437,#82438);
#73485=AXIS2_PLACEMENT_3D('',#117650,#82440,#82441);
#73486=AXIS2_PLACEMENT_3D('',#117652,#82442,#82443);
#73487=AXIS2_PLACEMENT_3D('',#117653,#82444,#82445);
#73488=AXIS2_PLACEMENT_3D('',#117667,#82447,#82448);
#73489=AXIS2_PLACEMENT_3D('',#117685,#82449,#82450);
#73490=AXIS2_PLACEMENT_3D('',#117687,#82452,#82453);
#73491=AXIS2_PLACEMENT_3D('',#117689,#82454,#82455);
#73492=AXIS2_PLACEMENT_3D('',#117690,#82456,#82457);
#73493=AXIS2_PLACEMENT_3D('',#117704,#82459,#82460);
#73494=AXIS2_PLACEMENT_3D('',#117722,#82461,#82462);
#73495=AXIS2_PLACEMENT_3D('',#117724,#82464,#82465);
#73496=AXIS2_PLACEMENT_3D('',#117726,#82466,#82467);
#73497=AXIS2_PLACEMENT_3D('',#117727,#82468,#82469);
#73498=AXIS2_PLACEMENT_3D('',#117741,#82471,#82472);
#73499=AXIS2_PLACEMENT_3D('',#117759,#82473,#82474);
#73500=AXIS2_PLACEMENT_3D('',#117761,#82476,#82477);
#73501=AXIS2_PLACEMENT_3D('',#117763,#82478,#82479);
#73502=AXIS2_PLACEMENT_3D('',#117764,#82480,#82481);
#73503=AXIS2_PLACEMENT_3D('',#117778,#82483,#82484);
#73504=AXIS2_PLACEMENT_3D('',#117796,#82485,#82486);
#73505=AXIS2_PLACEMENT_3D('',#117798,#82488,#82489);
#73506=AXIS2_PLACEMENT_3D('',#117800,#82490,#82491);
#73507=AXIS2_PLACEMENT_3D('',#117801,#82492,#82493);
#73508=AXIS2_PLACEMENT_3D('',#117815,#82495,#82496);
#73509=AXIS2_PLACEMENT_3D('',#117833,#82497,#82498);
#73510=AXIS2_PLACEMENT_3D('',#117835,#82500,#82501);
#73511=AXIS2_PLACEMENT_3D('',#117837,#82502,#82503);
#73512=AXIS2_PLACEMENT_3D('',#117838,#82504,#82505);
#73513=AXIS2_PLACEMENT_3D('',#117852,#82507,#82508);
#73514=AXIS2_PLACEMENT_3D('',#117870,#82509,#82510);
#73515=AXIS2_PLACEMENT_3D('',#117872,#82512,#82513);
#73516=AXIS2_PLACEMENT_3D('',#117874,#82514,#82515);
#73517=AXIS2_PLACEMENT_3D('',#117875,#82516,#82517);
#73518=AXIS2_PLACEMENT_3D('',#117889,#82519,#82520);
#73519=AXIS2_PLACEMENT_3D('',#117907,#82521,#82522);
#73520=AXIS2_PLACEMENT_3D('',#117909,#82524,#82525);
#73521=AXIS2_PLACEMENT_3D('',#117911,#82526,#82527);
#73522=AXIS2_PLACEMENT_3D('',#117912,#82528,#82529);
#73523=AXIS2_PLACEMENT_3D('',#117926,#82531,#82532);
#73524=AXIS2_PLACEMENT_3D('',#117944,#82533,#82534);
#73525=AXIS2_PLACEMENT_3D('',#117946,#82536,#82537);
#73526=AXIS2_PLACEMENT_3D('',#117948,#82538,#82539);
#73527=AXIS2_PLACEMENT_3D('',#117949,#82540,#82541);
#73528=AXIS2_PLACEMENT_3D('',#117963,#82543,#82544);
#73529=AXIS2_PLACEMENT_3D('',#117981,#82545,#82546);
#73530=AXIS2_PLACEMENT_3D('',#117983,#82548,#82549);
#73531=AXIS2_PLACEMENT_3D('',#117985,#82550,#82551);
#73532=AXIS2_PLACEMENT_3D('',#117986,#82552,#82553);
#73533=AXIS2_PLACEMENT_3D('',#118000,#82555,#82556);
#73534=AXIS2_PLACEMENT_3D('',#118018,#82557,#82558);
#73535=AXIS2_PLACEMENT_3D('',#118020,#82560,#82561);
#73536=AXIS2_PLACEMENT_3D('',#118022,#82562,#82563);
#73537=AXIS2_PLACEMENT_3D('',#118023,#82564,#82565);
#73538=AXIS2_PLACEMENT_3D('',#118037,#82567,#82568);
#73539=AXIS2_PLACEMENT_3D('',#118055,#82569,#82570);
#73540=AXIS2_PLACEMENT_3D('',#118057,#82572,#82573);
#73541=AXIS2_PLACEMENT_3D('',#118059,#82574,#82575);
#73542=AXIS2_PLACEMENT_3D('',#118060,#82576,#82577);
#73543=AXIS2_PLACEMENT_3D('',#118074,#82579,#82580);
#73544=AXIS2_PLACEMENT_3D('',#118092,#82581,#82582);
#73545=AXIS2_PLACEMENT_3D('',#118094,#82584,#82585);
#73546=AXIS2_PLACEMENT_3D('',#118096,#82586,#82587);
#73547=AXIS2_PLACEMENT_3D('',#118097,#82588,#82589);
#73548=AXIS2_PLACEMENT_3D('',#118111,#82591,#82592);
#73549=AXIS2_PLACEMENT_3D('',#118129,#82593,#82594);
#73550=AXIS2_PLACEMENT_3D('',#118131,#82596,#82597);
#73551=AXIS2_PLACEMENT_3D('',#118133,#82598,#82599);
#73552=AXIS2_PLACEMENT_3D('',#118134,#82600,#82601);
#73553=AXIS2_PLACEMENT_3D('',#118148,#82603,#82604);
#73554=AXIS2_PLACEMENT_3D('',#118166,#82605,#82606);
#73555=AXIS2_PLACEMENT_3D('',#118168,#82608,#82609);
#73556=AXIS2_PLACEMENT_3D('',#118170,#82610,#82611);
#73557=AXIS2_PLACEMENT_3D('',#118171,#82612,#82613);
#73558=AXIS2_PLACEMENT_3D('',#118185,#82615,#82616);
#73559=AXIS2_PLACEMENT_3D('',#118203,#82617,#82618);
#73560=AXIS2_PLACEMENT_3D('',#118205,#82620,#82621);
#73561=AXIS2_PLACEMENT_3D('',#118207,#82622,#82623);
#73562=AXIS2_PLACEMENT_3D('',#118208,#82624,#82625);
#73563=AXIS2_PLACEMENT_3D('',#118222,#82627,#82628);
#73564=AXIS2_PLACEMENT_3D('',#118240,#82629,#82630);
#73565=AXIS2_PLACEMENT_3D('',#118242,#82632,#82633);
#73566=AXIS2_PLACEMENT_3D('',#118244,#82634,#82635);
#73567=AXIS2_PLACEMENT_3D('',#118245,#82636,#82637);
#73568=AXIS2_PLACEMENT_3D('',#118259,#82639,#82640);
#73569=AXIS2_PLACEMENT_3D('',#118277,#82641,#82642);
#73570=AXIS2_PLACEMENT_3D('',#118279,#82644,#82645);
#73571=AXIS2_PLACEMENT_3D('',#118281,#82646,#82647);
#73572=AXIS2_PLACEMENT_3D('',#118282,#82648,#82649);
#73573=AXIS2_PLACEMENT_3D('',#118296,#82651,#82652);
#73574=AXIS2_PLACEMENT_3D('',#118314,#82653,#82654);
#73575=AXIS2_PLACEMENT_3D('',#118316,#82656,#82657);
#73576=AXIS2_PLACEMENT_3D('',#118318,#82658,#82659);
#73577=AXIS2_PLACEMENT_3D('',#118319,#82660,#82661);
#73578=AXIS2_PLACEMENT_3D('',#118333,#82663,#82664);
#73579=AXIS2_PLACEMENT_3D('',#118351,#82665,#82666);
#73580=AXIS2_PLACEMENT_3D('',#118353,#82668,#82669);
#73581=AXIS2_PLACEMENT_3D('',#118355,#82670,#82671);
#73582=AXIS2_PLACEMENT_3D('',#118356,#82672,#82673);
#73583=AXIS2_PLACEMENT_3D('',#118398,#82677,#82678);
#73584=AXIS2_PLACEMENT_3D('',#118416,#82679,#82680);
#73585=AXIS2_PLACEMENT_3D('',#118418,#82682,#82683);
#73586=AXIS2_PLACEMENT_3D('',#118420,#82684,#82685);
#73587=AXIS2_PLACEMENT_3D('',#118421,#82686,#82687);
#73588=AXIS2_PLACEMENT_3D('',#118435,#82689,#82690);
#73589=AXIS2_PLACEMENT_3D('',#118453,#82691,#82692);
#73590=AXIS2_PLACEMENT_3D('',#118455,#82694,#82695);
#73591=AXIS2_PLACEMENT_3D('',#118457,#82696,#82697);
#73592=AXIS2_PLACEMENT_3D('',#118458,#82698,#82699);
#73593=AXIS2_PLACEMENT_3D('',#118472,#82701,#82702);
#73594=AXIS2_PLACEMENT_3D('',#118490,#82703,#82704);
#73595=AXIS2_PLACEMENT_3D('',#118492,#82706,#82707);
#73596=AXIS2_PLACEMENT_3D('',#118494,#82708,#82709);
#73597=AXIS2_PLACEMENT_3D('',#118495,#82710,#82711);
#73598=AXIS2_PLACEMENT_3D('',#118509,#82713,#82714);
#73599=AXIS2_PLACEMENT_3D('',#118527,#82715,#82716);
#73600=AXIS2_PLACEMENT_3D('',#118529,#82718,#82719);
#73601=AXIS2_PLACEMENT_3D('',#118531,#82720,#82721);
#73602=AXIS2_PLACEMENT_3D('',#118532,#82722,#82723);
#73603=AXIS2_PLACEMENT_3D('',#118546,#82725,#82726);
#73604=AXIS2_PLACEMENT_3D('',#118564,#82727,#82728);
#73605=AXIS2_PLACEMENT_3D('',#118566,#82730,#82731);
#73606=AXIS2_PLACEMENT_3D('',#118568,#82732,#82733);
#73607=AXIS2_PLACEMENT_3D('',#118569,#82734,#82735);
#73608=AXIS2_PLACEMENT_3D('',#118583,#82737,#82738);
#73609=AXIS2_PLACEMENT_3D('',#118601,#82739,#82740);
#73610=AXIS2_PLACEMENT_3D('',#118603,#82742,#82743);
#73611=AXIS2_PLACEMENT_3D('',#118605,#82744,#82745);
#73612=AXIS2_PLACEMENT_3D('',#118606,#82746,#82747);
#73613=AXIS2_PLACEMENT_3D('',#118620,#82749,#82750);
#73614=AXIS2_PLACEMENT_3D('',#118638,#82751,#82752);
#73615=AXIS2_PLACEMENT_3D('',#118640,#82754,#82755);
#73616=AXIS2_PLACEMENT_3D('',#118642,#82756,#82757);
#73617=AXIS2_PLACEMENT_3D('',#118643,#82758,#82759);
#73618=AXIS2_PLACEMENT_3D('',#118651,#82760,#82761);
#73619=AXIS2_PLACEMENT_3D('',#118685,#82762,#82763);
#73620=AXIS2_PLACEMENT_3D('',#118719,#82764,#82765);
#73621=AXIS2_PLACEMENT_3D('',#118753,#82766,#82767);
#73622=AXIS2_PLACEMENT_3D('',#118787,#82768,#82769);
#73623=AXIS2_PLACEMENT_3D('',#118821,#82770,#82771);
#73624=AXIS2_PLACEMENT_3D('',#118855,#82772,#82773);
#73625=AXIS2_PLACEMENT_3D('',#118889,#82774,#82775);
#73626=AXIS2_PLACEMENT_3D('',#118923,#82776,#82777);
#73627=AXIS2_PLACEMENT_3D('',#118957,#82778,#82779);
#73628=AXIS2_PLACEMENT_3D('',#118991,#82780,#82781);
#73629=AXIS2_PLACEMENT_3D('',#119025,#82782,#82783);
#73630=AXIS2_PLACEMENT_3D('',#119059,#82784,#82785);
#73631=AXIS2_PLACEMENT_3D('',#119093,#82786,#82787);
#73632=AXIS2_PLACEMENT_3D('',#119127,#82788,#82789);
#73633=AXIS2_PLACEMENT_3D('',#119161,#82790,#82791);
#73634=AXIS2_PLACEMENT_3D('',#119195,#82792,#82793);
#73635=AXIS2_PLACEMENT_3D('',#119229,#82794,#82795);
#73636=AXIS2_PLACEMENT_3D('',#119263,#82796,#82797);
#73637=AXIS2_PLACEMENT_3D('',#119297,#82798,#82799);
#73638=AXIS2_PLACEMENT_3D('',#119331,#82800,#82801);
#73639=AXIS2_PLACEMENT_3D('',#119365,#82802,#82803);
#73640=AXIS2_PLACEMENT_3D('',#119399,#82804,#82805);
#73641=AXIS2_PLACEMENT_3D('',#119433,#82806,#82807);
#73642=AXIS2_PLACEMENT_3D('',#119467,#82808,#82809);
#73643=AXIS2_PLACEMENT_3D('',#119501,#82810,#82811);
#73644=AXIS2_PLACEMENT_3D('',#119535,#82812,#82813);
#73645=AXIS2_PLACEMENT_3D('',#119569,#82814,#82815);
#73646=AXIS2_PLACEMENT_3D('',#119603,#82816,#82817);
#73647=AXIS2_PLACEMENT_3D('',#119637,#82818,#82819);
#73648=AXIS2_PLACEMENT_3D('',#119675,#82820,#82821);
#73649=AXIS2_PLACEMENT_3D('',#119713,#82822,#82823);
#73650=AXIS2_PLACEMENT_3D('',#119751,#82824,#82825);
#73651=AXIS2_PLACEMENT_3D('',#119789,#82826,#82827);
#73652=AXIS2_PLACEMENT_3D('',#119827,#82828,#82829);
#73653=AXIS2_PLACEMENT_3D('',#119865,#82830,#82831);
#73654=AXIS2_PLACEMENT_3D('',#119903,#82832,#82833);
#73655=AXIS2_PLACEMENT_3D('',#119941,#82834,#82835);
#73656=AXIS2_PLACEMENT_3D('',#119979,#82836,#82837);
#73657=AXIS2_PLACEMENT_3D('',#120017,#82838,#82839);
#73658=AXIS2_PLACEMENT_3D('',#120055,#82840,#82841);
#73659=AXIS2_PLACEMENT_3D('',#120093,#82842,#82843);
#73660=AXIS2_PLACEMENT_3D('',#120131,#82844,#82845);
#73661=AXIS2_PLACEMENT_3D('',#120169,#82846,#82847);
#73662=AXIS2_PLACEMENT_3D('',#120207,#82848,#82849);
#73663=AXIS2_PLACEMENT_3D('',#120245,#82850,#82851);
#73664=AXIS2_PLACEMENT_3D('',#120283,#82852,#82853);
#73665=AXIS2_PLACEMENT_3D('',#120321,#82854,#82855);
#73666=AXIS2_PLACEMENT_3D('',#120359,#82856,#82857);
#73667=AXIS2_PLACEMENT_3D('',#120397,#82858,#82859);
#73668=AXIS2_PLACEMENT_3D('',#120435,#82860,#82861);
#73669=AXIS2_PLACEMENT_3D('',#120473,#82862,#82863);
#73670=AXIS2_PLACEMENT_3D('',#120511,#82864,#82865);
#73671=AXIS2_PLACEMENT_3D('',#120549,#82866,#82867);
#73672=AXIS2_PLACEMENT_3D('',#120587,#82868,#82869);
#73673=AXIS2_PLACEMENT_3D('',#120625,#82870,#82871);
#73674=AXIS2_PLACEMENT_3D('',#120663,#82872,#82873);
#73675=AXIS2_PLACEMENT_3D('',#120701,#82874,#82875);
#73676=AXIS2_PLACEMENT_3D('',#120740,#82876,#82877);
#73677=AXIS2_PLACEMENT_3D('',#120778,#82880,#82881);
#73678=AXIS2_PLACEMENT_3D('',#120780,#82882,#82883);
#73679=AXIS2_PLACEMENT_3D('',#120782,#82884,#82885);
#73680=AXIS2_PLACEMENT_3D('',#120783,#82886,#82887);
#73681=AXIS2_PLACEMENT_3D('',#120821,#82890,#82891);
#73682=AXIS2_PLACEMENT_3D('',#120823,#82892,#82893);
#73683=AXIS2_PLACEMENT_3D('',#120825,#82894,#82895);
#73684=AXIS2_PLACEMENT_3D('',#120826,#82896,#82897);
#73685=AXIS2_PLACEMENT_3D('',#120864,#82900,#82901);
#73686=AXIS2_PLACEMENT_3D('',#120866,#82902,#82903);
#73687=AXIS2_PLACEMENT_3D('',#120868,#82904,#82905);
#73688=AXIS2_PLACEMENT_3D('',#120869,#82906,#82907);
#73689=AXIS2_PLACEMENT_3D('',#120907,#82910,#82911);
#73690=AXIS2_PLACEMENT_3D('',#120909,#82912,#82913);
#73691=AXIS2_PLACEMENT_3D('',#120911,#82914,#82915);
#73692=AXIS2_PLACEMENT_3D('',#120912,#82916,#82917);
#73693=AXIS2_PLACEMENT_3D('',#120950,#82920,#82921);
#73694=AXIS2_PLACEMENT_3D('',#120952,#82922,#82923);
#73695=AXIS2_PLACEMENT_3D('',#120954,#82924,#82925);
#73696=AXIS2_PLACEMENT_3D('',#120955,#82926,#82927);
#73697=AXIS2_PLACEMENT_3D('',#120993,#82930,#82931);
#73698=AXIS2_PLACEMENT_3D('',#120995,#82932,#82933);
#73699=AXIS2_PLACEMENT_3D('',#120997,#82934,#82935);
#73700=AXIS2_PLACEMENT_3D('',#120998,#82936,#82937);
#73701=AXIS2_PLACEMENT_3D('',#121064,#82942,#82943);
#73702=AXIS2_PLACEMENT_3D('',#121066,#82944,#82945);
#73703=AXIS2_PLACEMENT_3D('',#121068,#82946,#82947);
#73704=AXIS2_PLACEMENT_3D('',#121069,#82948,#82949);
#73705=AXIS2_PLACEMENT_3D('',#121107,#82952,#82953);
#73706=AXIS2_PLACEMENT_3D('',#121109,#82954,#82955);
#73707=AXIS2_PLACEMENT_3D('',#121111,#82956,#82957);
#73708=AXIS2_PLACEMENT_3D('',#121112,#82958,#82959);
#73709=AXIS2_PLACEMENT_3D('',#121150,#82962,#82963);
#73710=AXIS2_PLACEMENT_3D('',#121152,#82964,#82965);
#73711=AXIS2_PLACEMENT_3D('',#121154,#82966,#82967);
#73712=AXIS2_PLACEMENT_3D('',#121155,#82968,#82969);
#73713=AXIS2_PLACEMENT_3D('',#121193,#82972,#82973);
#73714=AXIS2_PLACEMENT_3D('',#121195,#82974,#82975);
#73715=AXIS2_PLACEMENT_3D('',#121197,#82976,#82977);
#73716=AXIS2_PLACEMENT_3D('',#121198,#82978,#82979);
#73717=AXIS2_PLACEMENT_3D('',#121236,#82982,#82983);
#73718=AXIS2_PLACEMENT_3D('',#121238,#82984,#82985);
#73719=AXIS2_PLACEMENT_3D('',#121240,#82986,#82987);
#73720=AXIS2_PLACEMENT_3D('',#121241,#82988,#82989);
#73721=AXIS2_PLACEMENT_3D('',#121279,#82992,#82993);
#73722=AXIS2_PLACEMENT_3D('',#121281,#82994,#82995);
#73723=AXIS2_PLACEMENT_3D('',#121283,#82996,#82997);
#73724=AXIS2_PLACEMENT_3D('',#121284,#82998,#82999);
#73725=AXIS2_PLACEMENT_3D('',#121322,#83002,#83003);
#73726=AXIS2_PLACEMENT_3D('',#121324,#83004,#83005);
#73727=AXIS2_PLACEMENT_3D('',#121326,#83006,#83007);
#73728=AXIS2_PLACEMENT_3D('',#121327,#83008,#83009);
#73729=AXIS2_PLACEMENT_3D('',#121365,#83012,#83013);
#73730=AXIS2_PLACEMENT_3D('',#121367,#83014,#83015);
#73731=AXIS2_PLACEMENT_3D('',#121369,#83016,#83017);
#73732=AXIS2_PLACEMENT_3D('',#121370,#83018,#83019);
#73733=AXIS2_PLACEMENT_3D('',#121408,#83022,#83023);
#73734=AXIS2_PLACEMENT_3D('',#121410,#83024,#83025);
#73735=AXIS2_PLACEMENT_3D('',#121412,#83026,#83027);
#73736=AXIS2_PLACEMENT_3D('',#121413,#83028,#83029);
#73737=AXIS2_PLACEMENT_3D('',#121451,#83032,#83033);
#73738=AXIS2_PLACEMENT_3D('',#121453,#83034,#83035);
#73739=AXIS2_PLACEMENT_3D('',#121455,#83036,#83037);
#73740=AXIS2_PLACEMENT_3D('',#121456,#83038,#83039);
#73741=AXIS2_PLACEMENT_3D('',#121494,#83042,#83043);
#73742=AXIS2_PLACEMENT_3D('',#121496,#83044,#83045);
#73743=AXIS2_PLACEMENT_3D('',#121498,#83046,#83047);
#73744=AXIS2_PLACEMENT_3D('',#121499,#83048,#83049);
#73745=AXIS2_PLACEMENT_3D('',#121537,#83052,#83053);
#73746=AXIS2_PLACEMENT_3D('',#121539,#83054,#83055);
#73747=AXIS2_PLACEMENT_3D('',#121541,#83056,#83057);
#73748=AXIS2_PLACEMENT_3D('',#121542,#83058,#83059);
#73749=AXIS2_PLACEMENT_3D('',#121580,#83062,#83063);
#73750=AXIS2_PLACEMENT_3D('',#121582,#83064,#83065);
#73751=AXIS2_PLACEMENT_3D('',#121584,#83066,#83067);
#73752=AXIS2_PLACEMENT_3D('',#121585,#83068,#83069);
#73753=AXIS2_PLACEMENT_3D('',#121623,#83072,#83073);
#73754=AXIS2_PLACEMENT_3D('',#121625,#83074,#83075);
#73755=AXIS2_PLACEMENT_3D('',#121627,#83076,#83077);
#73756=AXIS2_PLACEMENT_3D('',#121628,#83078,#83079);
#73757=AXIS2_PLACEMENT_3D('',#121673,#83082,#83083);
#73758=AXIS2_PLACEMENT_3D('',#121675,#83085,#83086);
#73759=AXIS2_PLACEMENT_3D('',#121677,#83087,#83088);
#73760=AXIS2_PLACEMENT_3D('',#121678,#83089,#83090);
#73761=AXIS2_PLACEMENT_3D('',#121709,#83092,#83093);
#73762=AXIS2_PLACEMENT_3D('',#121711,#83094,#83095);
#73763=AXIS2_PLACEMENT_3D('',#121713,#83096,#83097);
#73764=AXIS2_PLACEMENT_3D('',#121714,#83098,#83099);
#73765=AXIS2_PLACEMENT_3D('',#121752,#83102,#83103);
#73766=AXIS2_PLACEMENT_3D('',#121754,#83104,#83105);
#73767=AXIS2_PLACEMENT_3D('',#121756,#83106,#83107);
#73768=AXIS2_PLACEMENT_3D('',#121757,#83108,#83109);
#73769=AXIS2_PLACEMENT_3D('',#121795,#83112,#83113);
#73770=AXIS2_PLACEMENT_3D('',#121797,#83114,#83115);
#73771=AXIS2_PLACEMENT_3D('',#121799,#83116,#83117);
#73772=AXIS2_PLACEMENT_3D('',#121800,#83118,#83119);
#73773=AXIS2_PLACEMENT_3D('',#121838,#83122,#83123);
#73774=AXIS2_PLACEMENT_3D('',#121840,#83124,#83125);
#73775=AXIS2_PLACEMENT_3D('',#121842,#83126,#83127);
#73776=AXIS2_PLACEMENT_3D('',#121843,#83128,#83129);
#73777=AXIS2_PLACEMENT_3D('',#121881,#83132,#83133);
#73778=AXIS2_PLACEMENT_3D('',#121883,#83134,#83135);
#73779=AXIS2_PLACEMENT_3D('',#121885,#83136,#83137);
#73780=AXIS2_PLACEMENT_3D('',#121886,#83138,#83139);
#73781=AXIS2_PLACEMENT_3D('',#121924,#83142,#83143);
#73782=AXIS2_PLACEMENT_3D('',#121926,#83144,#83145);
#73783=AXIS2_PLACEMENT_3D('',#121928,#83146,#83147);
#73784=AXIS2_PLACEMENT_3D('',#121929,#83148,#83149);
#73785=AXIS2_PLACEMENT_3D('',#121937,#83151,#83152);
#73786=AXIS2_PLACEMENT_3D('',#121940,#83153,#83154);
#73787=AXIS2_PLACEMENT_3D('',#121941,#83155,#83156);
#73788=AXIS2_PLACEMENT_3D('',#121978,#83158,#83159);
#73789=AXIS2_PLACEMENT_3D('',#122013,#83162,#83163);
#73790=AXIS2_PLACEMENT_3D('',#122015,#83165,#83166);
#73791=AXIS2_PLACEMENT_3D('',#122017,#83167,#83168);
#73792=AXIS2_PLACEMENT_3D('',#122018,#83169,#83170);
#73793=AXIS2_PLACEMENT_3D('',#122052,#83172,#83173);
#73794=AXIS2_PLACEMENT_3D('',#122054,#83175,#83176);
#73795=AXIS2_PLACEMENT_3D('',#122056,#83177,#83178);
#73796=AXIS2_PLACEMENT_3D('',#122057,#83179,#83180);
#73797=AXIS2_PLACEMENT_3D('',#122091,#83182,#83183);
#73798=AXIS2_PLACEMENT_3D('',#122093,#83185,#83186);
#73799=AXIS2_PLACEMENT_3D('',#122095,#83187,#83188);
#73800=AXIS2_PLACEMENT_3D('',#122096,#83189,#83190);
#73801=AXIS2_PLACEMENT_3D('',#122130,#83192,#83193);
#73802=AXIS2_PLACEMENT_3D('',#122132,#83195,#83196);
#73803=AXIS2_PLACEMENT_3D('',#122134,#83197,#83198);
#73804=AXIS2_PLACEMENT_3D('',#122135,#83199,#83200);
#73805=AXIS2_PLACEMENT_3D('',#122169,#83202,#83203);
#73806=AXIS2_PLACEMENT_3D('',#122171,#83205,#83206);
#73807=AXIS2_PLACEMENT_3D('',#122173,#83207,#83208);
#73808=AXIS2_PLACEMENT_3D('',#122174,#83209,#83210);
#73809=AXIS2_PLACEMENT_3D('',#122208,#83212,#83213);
#73810=AXIS2_PLACEMENT_3D('',#122210,#83215,#83216);
#73811=AXIS2_PLACEMENT_3D('',#122212,#83217,#83218);
#73812=AXIS2_PLACEMENT_3D('',#122213,#83219,#83220);
#73813=AXIS2_PLACEMENT_3D('',#122247,#83222,#83223);
#73814=AXIS2_PLACEMENT_3D('',#122249,#83225,#83226);
#73815=AXIS2_PLACEMENT_3D('',#122251,#83227,#83228);
#73816=AXIS2_PLACEMENT_3D('',#122252,#83229,#83230);
#73817=AXIS2_PLACEMENT_3D('',#122286,#83232,#83233);
#73818=AXIS2_PLACEMENT_3D('',#122288,#83235,#83236);
#73819=AXIS2_PLACEMENT_3D('',#122290,#83237,#83238);
#73820=AXIS2_PLACEMENT_3D('',#122291,#83239,#83240);
#73821=AXIS2_PLACEMENT_3D('',#122325,#83242,#83243);
#73822=AXIS2_PLACEMENT_3D('',#122327,#83245,#83246);
#73823=AXIS2_PLACEMENT_3D('',#122329,#83247,#83248);
#73824=AXIS2_PLACEMENT_3D('',#122330,#83249,#83250);
#73825=AXIS2_PLACEMENT_3D('',#122364,#83252,#83253);
#73826=AXIS2_PLACEMENT_3D('',#122366,#83255,#83256);
#73827=AXIS2_PLACEMENT_3D('',#122368,#83257,#83258);
#73828=AXIS2_PLACEMENT_3D('',#122369,#83259,#83260);
#73829=AXIS2_PLACEMENT_3D('',#122403,#83262,#83263);
#73830=AXIS2_PLACEMENT_3D('',#122405,#83265,#83266);
#73831=AXIS2_PLACEMENT_3D('',#122407,#83267,#83268);
#73832=AXIS2_PLACEMENT_3D('',#122408,#83269,#83270);
#73833=AXIS2_PLACEMENT_3D('',#122442,#83272,#83273);
#73834=AXIS2_PLACEMENT_3D('',#122444,#83275,#83276);
#73835=AXIS2_PLACEMENT_3D('',#122446,#83277,#83278);
#73836=AXIS2_PLACEMENT_3D('',#122447,#83279,#83280);
#73837=AXIS2_PLACEMENT_3D('',#122481,#83282,#83283);
#73838=AXIS2_PLACEMENT_3D('',#122483,#83285,#83286);
#73839=AXIS2_PLACEMENT_3D('',#122485,#83287,#83288);
#73840=AXIS2_PLACEMENT_3D('',#122486,#83289,#83290);
#73841=AXIS2_PLACEMENT_3D('',#122544,#83294,#83295);
#73842=AXIS2_PLACEMENT_3D('',#122546,#83297,#83298);
#73843=AXIS2_PLACEMENT_3D('',#122548,#83299,#83300);
#73844=AXIS2_PLACEMENT_3D('',#122549,#83301,#83302);
#73845=AXIS2_PLACEMENT_3D('',#122583,#83304,#83305);
#73846=AXIS2_PLACEMENT_3D('',#122585,#83307,#83308);
#73847=AXIS2_PLACEMENT_3D('',#122587,#83309,#83310);
#73848=AXIS2_PLACEMENT_3D('',#122588,#83311,#83312);
#73849=AXIS2_PLACEMENT_3D('',#122622,#83314,#83315);
#73850=AXIS2_PLACEMENT_3D('',#122624,#83317,#83318);
#73851=AXIS2_PLACEMENT_3D('',#122626,#83319,#83320);
#73852=AXIS2_PLACEMENT_3D('',#122627,#83321,#83322);
#73853=AXIS2_PLACEMENT_3D('',#122661,#83324,#83325);
#73854=AXIS2_PLACEMENT_3D('',#122663,#83327,#83328);
#73855=AXIS2_PLACEMENT_3D('',#122665,#83329,#83330);
#73856=AXIS2_PLACEMENT_3D('',#122666,#83331,#83332);
#73857=AXIS2_PLACEMENT_3D('',#122700,#83334,#83335);
#73858=AXIS2_PLACEMENT_3D('',#122702,#83337,#83338);
#73859=AXIS2_PLACEMENT_3D('',#122704,#83339,#83340);
#73860=AXIS2_PLACEMENT_3D('',#122705,#83341,#83342);
#73861=AXIS2_PLACEMENT_3D('',#122739,#83344,#83345);
#73862=AXIS2_PLACEMENT_3D('',#122741,#83347,#83348);
#73863=AXIS2_PLACEMENT_3D('',#122743,#83349,#83350);
#73864=AXIS2_PLACEMENT_3D('',#122744,#83351,#83352);
#73865=AXIS2_PLACEMENT_3D('',#122778,#83354,#83355);
#73866=AXIS2_PLACEMENT_3D('',#122780,#83357,#83358);
#73867=AXIS2_PLACEMENT_3D('',#122782,#83359,#83360);
#73868=AXIS2_PLACEMENT_3D('',#122783,#83361,#83362);
#73869=AXIS2_PLACEMENT_3D('',#122817,#83364,#83365);
#73870=AXIS2_PLACEMENT_3D('',#122819,#83367,#83368);
#73871=AXIS2_PLACEMENT_3D('',#122821,#83369,#83370);
#73872=AXIS2_PLACEMENT_3D('',#122822,#83371,#83372);
#73873=AXIS2_PLACEMENT_3D('',#122856,#83374,#83375);
#73874=AXIS2_PLACEMENT_3D('',#122858,#83377,#83378);
#73875=AXIS2_PLACEMENT_3D('',#122860,#83379,#83380);
#73876=AXIS2_PLACEMENT_3D('',#122861,#83381,#83382);
#73877=AXIS2_PLACEMENT_3D('',#122895,#83384,#83385);
#73878=AXIS2_PLACEMENT_3D('',#122897,#83387,#83388);
#73879=AXIS2_PLACEMENT_3D('',#122899,#83389,#83390);
#73880=AXIS2_PLACEMENT_3D('',#122900,#83391,#83392);
#73881=AXIS2_PLACEMENT_3D('',#122934,#83394,#83395);
#73882=AXIS2_PLACEMENT_3D('',#122936,#83397,#83398);
#73883=AXIS2_PLACEMENT_3D('',#122938,#83399,#83400);
#73884=AXIS2_PLACEMENT_3D('',#122939,#83401,#83402);
#73885=AXIS2_PLACEMENT_3D('',#122973,#83404,#83405);
#73886=AXIS2_PLACEMENT_3D('',#122975,#83407,#83408);
#73887=AXIS2_PLACEMENT_3D('',#122977,#83409,#83410);
#73888=AXIS2_PLACEMENT_3D('',#122978,#83411,#83412);
#73889=AXIS2_PLACEMENT_3D('',#123012,#83414,#83415);
#73890=AXIS2_PLACEMENT_3D('',#123014,#83417,#83418);
#73891=AXIS2_PLACEMENT_3D('',#123016,#83419,#83420);
#73892=AXIS2_PLACEMENT_3D('',#123017,#83421,#83422);
#73893=AXIS2_PLACEMENT_3D('',#123051,#83424,#83425);
#73894=AXIS2_PLACEMENT_3D('',#123053,#83427,#83428);
#73895=AXIS2_PLACEMENT_3D('',#123055,#83429,#83430);
#73896=AXIS2_PLACEMENT_3D('',#123056,#83431,#83432);
#73897=AXIS2_PLACEMENT_3D('',#123057,#83433,#83434);
#73898=AXIS2_PLACEMENT_3D('',#123067,#83435,#83436);
#73899=AXIS2_PLACEMENT_3D('',#123068,#83437,#83438);
#73900=AXIS2_PLACEMENT_3D('',#123087,#83440,#83441);
#73901=AXIS2_PLACEMENT_3D('',#123105,#83442,#83443);
#73902=AXIS2_PLACEMENT_3D('',#123118,#83444,#83445);
#73903=AXIS2_PLACEMENT_3D('',#123130,#83446,#83447);
#73904=AXIS2_PLACEMENT_3D('',#123143,#83448,#83449);
#73905=AXIS2_PLACEMENT_3D('',#123155,#83450,#83451);
#73906=AXIS2_PLACEMENT_3D('',#123168,#83452,#83453);
#73907=AXIS2_PLACEMENT_3D('',#123180,#83454,#83455);
#73908=AXIS2_PLACEMENT_3D('',#123193,#83456,#83457);
#73909=AXIS2_PLACEMENT_3D('',#123205,#83458,#83459);
#73910=AXIS2_PLACEMENT_3D('',#123218,#83460,#83461);
#73911=AXIS2_PLACEMENT_3D('',#123230,#83462,#83463);
#73912=AXIS2_PLACEMENT_3D('',#123243,#83464,#83465);
#73913=AXIS2_PLACEMENT_3D('',#123255,#83466,#83467);
#73914=AXIS2_PLACEMENT_3D('',#123268,#83468,#83469);
#73915=AXIS2_PLACEMENT_3D('',#123280,#83470,#83471);
#73916=AXIS2_PLACEMENT_3D('',#123293,#83472,#83473);
#73917=AXIS2_PLACEMENT_3D('',#123305,#83474,#83475);
#73918=AXIS2_PLACEMENT_3D('',#123318,#83476,#83477);
#73919=AXIS2_PLACEMENT_3D('',#123330,#83478,#83479);
#73920=AXIS2_PLACEMENT_3D('',#123343,#83480,#83481);
#73921=AXIS2_PLACEMENT_3D('',#123355,#83482,#83483);
#73922=AXIS2_PLACEMENT_3D('',#123368,#83484,#83485);
#73923=AXIS2_PLACEMENT_3D('',#123380,#83486,#83487);
#73924=AXIS2_PLACEMENT_3D('',#123393,#83488,#83489);
#73925=AXIS2_PLACEMENT_3D('',#123405,#83490,#83491);
#73926=AXIS2_PLACEMENT_3D('',#123418,#83492,#83493);
#73927=AXIS2_PLACEMENT_3D('',#123430,#83494,#83495);
#73928=AXIS2_PLACEMENT_3D('',#123443,#83496,#83497);
#73929=AXIS2_PLACEMENT_3D('',#123455,#83498,#83499);
#73930=AXIS2_PLACEMENT_3D('',#123468,#83500,#83501);
#73931=AXIS2_PLACEMENT_3D('',#123480,#83502,#83503);
#73932=AXIS2_PLACEMENT_3D('',#123493,#83504,#83505);
#73933=AXIS2_PLACEMENT_3D('',#123505,#83506,#83507);
#73934=AXIS2_PLACEMENT_3D('',#123518,#83508,#83509);
#73935=AXIS2_PLACEMENT_3D('',#123530,#83510,#83511);
#73936=AXIS2_PLACEMENT_3D('',#123543,#83512,#83513);
#73937=AXIS2_PLACEMENT_3D('',#123555,#83514,#83515);
#73938=AXIS2_PLACEMENT_3D('',#123568,#83516,#83517);
#73939=AXIS2_PLACEMENT_3D('',#123580,#83518,#83519);
#73940=AXIS2_PLACEMENT_3D('',#123593,#83520,#83521);
#73941=AXIS2_PLACEMENT_3D('',#123605,#83522,#83523);
#73942=AXIS2_PLACEMENT_3D('',#123618,#83524,#83525);
#73943=AXIS2_PLACEMENT_3D('',#123630,#83526,#83527);
#73944=AXIS2_PLACEMENT_3D('',#123643,#83528,#83529);
#73945=AXIS2_PLACEMENT_3D('',#123655,#83530,#83531);
#73946=AXIS2_PLACEMENT_3D('',#123668,#83532,#83533);
#73947=AXIS2_PLACEMENT_3D('',#123680,#83534,#83535);
#73948=AXIS2_PLACEMENT_3D('',#123693,#83536,#83537);
#73949=AXIS2_PLACEMENT_3D('',#123705,#83538,#83539);
#73950=AXIS2_PLACEMENT_3D('',#123718,#83540,#83541);
#73951=AXIS2_PLACEMENT_3D('',#123730,#83542,#83543);
#73952=AXIS2_PLACEMENT_3D('',#123743,#83544,#83545);
#73953=AXIS2_PLACEMENT_3D('',#123755,#83546,#83547);
#73954=AXIS2_PLACEMENT_3D('',#123768,#83548,#83549);
#73955=AXIS2_PLACEMENT_3D('',#123780,#83550,#83551);
#73956=AXIS2_PLACEMENT_3D('',#123793,#83552,#83553);
#73957=AXIS2_PLACEMENT_3D('',#123804,#83554,#83555);
#73958=AXIS2_PLACEMENT_3D('',#123826,#83556,#83557);
#73959=AXIS2_PLACEMENT_3D('',#123872,#83558,#83559);
#73960=AXIS2_PLACEMENT_3D('',#123913,#83560,#83561);
#73961=AXIS2_PLACEMENT_3D('',#123954,#83562,#83563);
#73962=AXIS2_PLACEMENT_3D('',#124000,#83564,#83565);
#73963=AXIS2_PLACEMENT_3D('',#124046,#83566,#83567);
#73964=AXIS2_PLACEMENT_3D('',#124087,#83568,#83569);
#73965=AXIS2_PLACEMENT_3D('',#124128,#83570,#83571);
#73966=AXIS2_PLACEMENT_3D('',#124169,#83572,#83573);
#73967=AXIS2_PLACEMENT_3D('',#124210,#83574,#83575);
#73968=AXIS2_PLACEMENT_3D('',#124256,#83576,#83577);
#73969=AXIS2_PLACEMENT_3D('',#124297,#83578,#83579);
#73970=AXIS2_PLACEMENT_3D('',#124338,#83580,#83581);
#73971=AXIS2_PLACEMENT_3D('',#124379,#83582,#83583);
#73972=AXIS2_PLACEMENT_3D('',#124429,#83584,#83585);
#73973=AXIS2_PLACEMENT_3D('',#124479,#83586,#83587);
#73974=AXIS2_PLACEMENT_3D('',#124529,#83588,#83589);
#73975=AXIS2_PLACEMENT_3D('',#124570,#83590,#83591);
#73976=AXIS2_PLACEMENT_3D('',#124611,#83592,#83593);
#73977=AXIS2_PLACEMENT_3D('',#124657,#83594,#83595);
#73978=AXIS2_PLACEMENT_3D('',#124698,#83596,#83597);
#73979=AXIS2_PLACEMENT_3D('',#124739,#83598,#83599);
#73980=AXIS2_PLACEMENT_3D('',#124785,#83600,#83601);
#73981=AXIS2_PLACEMENT_3D('',#124835,#83602,#83603);
#73982=AXIS2_PLACEMENT_3D('',#124876,#83604,#83605);
#73983=AXIS2_PLACEMENT_3D('',#124917,#83606,#83607);
#73984=AXIS2_PLACEMENT_3D('',#124958,#83608,#83609);
#73985=AXIS2_PLACEMENT_3D('',#125004,#83610,#83611);
#73986=AXIS2_PLACEMENT_3D('',#125050,#83612,#83613);
#73987=AXIS2_PLACEMENT_3D('',#125091,#83614,#83615);
#73988=AXIS2_PLACEMENT_3D('',#125099,#83617,#83618);
#73989=AXIS2_PLACEMENT_3D('',#125101,#83619,#83620);
#73990=AXIS2_PLACEMENT_3D('',#125103,#83621,#83622);
#73991=AXIS2_PLACEMENT_3D('',#125104,#83623,#83624);
#73992=AXIS2_PLACEMENT_3D('',#125124,#83626,#83627);
#73993=AXIS2_PLACEMENT_3D('',#125132,#83629,#83630);
#73994=AXIS2_PLACEMENT_3D('',#125134,#83631,#83632);
#73995=AXIS2_PLACEMENT_3D('',#125136,#83633,#83634);
#73996=AXIS2_PLACEMENT_3D('',#125137,#83635,#83636);
#73997=AXIS2_PLACEMENT_3D('',#125157,#83638,#83639);
#73998=AXIS2_PLACEMENT_3D('',#125165,#83641,#83642);
#73999=AXIS2_PLACEMENT_3D('',#125167,#83643,#83644);
#74000=AXIS2_PLACEMENT_3D('',#125169,#83645,#83646);
#74001=AXIS2_PLACEMENT_3D('',#125170,#83647,#83648);
#74002=AXIS2_PLACEMENT_3D('',#125190,#83650,#83651);
#74003=AXIS2_PLACEMENT_3D('',#125198,#83653,#83654);
#74004=AXIS2_PLACEMENT_3D('',#125200,#83655,#83656);
#74005=AXIS2_PLACEMENT_3D('',#125202,#83657,#83658);
#74006=AXIS2_PLACEMENT_3D('',#125203,#83659,#83660);
#74007=AXIS2_PLACEMENT_3D('',#125223,#83662,#83663);
#74008=AXIS2_PLACEMENT_3D('',#125231,#83665,#83666);
#74009=AXIS2_PLACEMENT_3D('',#125233,#83667,#83668);
#74010=AXIS2_PLACEMENT_3D('',#125235,#83669,#83670);
#74011=AXIS2_PLACEMENT_3D('',#125236,#83671,#83672);
#74012=AXIS2_PLACEMENT_3D('',#125256,#83674,#83675);
#74013=AXIS2_PLACEMENT_3D('',#125264,#83677,#83678);
#74014=AXIS2_PLACEMENT_3D('',#125266,#83679,#83680);
#74015=AXIS2_PLACEMENT_3D('',#125268,#83681,#83682);
#74016=AXIS2_PLACEMENT_3D('',#125269,#83683,#83684);
#74017=AXIS2_PLACEMENT_3D('',#125289,#83686,#83687);
#74018=AXIS2_PLACEMENT_3D('',#125297,#83689,#83690);
#74019=AXIS2_PLACEMENT_3D('',#125299,#83691,#83692);
#74020=AXIS2_PLACEMENT_3D('',#125301,#83693,#83694);
#74021=AXIS2_PLACEMENT_3D('',#125302,#83695,#83696);
#74022=AXIS2_PLACEMENT_3D('',#125322,#83698,#83699);
#74023=AXIS2_PLACEMENT_3D('',#125330,#83701,#83702);
#74024=AXIS2_PLACEMENT_3D('',#125332,#83703,#83704);
#74025=AXIS2_PLACEMENT_3D('',#125334,#83705,#83706);
#74026=AXIS2_PLACEMENT_3D('',#125335,#83707,#83708);
#74027=AXIS2_PLACEMENT_3D('',#125355,#83710,#83711);
#74028=AXIS2_PLACEMENT_3D('',#125363,#83713,#83714);
#74029=AXIS2_PLACEMENT_3D('',#125365,#83715,#83716);
#74030=AXIS2_PLACEMENT_3D('',#125367,#83717,#83718);
#74031=AXIS2_PLACEMENT_3D('',#125368,#83719,#83720);
#74032=AXIS2_PLACEMENT_3D('',#125388,#83722,#83723);
#74033=AXIS2_PLACEMENT_3D('',#125396,#83725,#83726);
#74034=AXIS2_PLACEMENT_3D('',#125398,#83727,#83728);
#74035=AXIS2_PLACEMENT_3D('',#125400,#83729,#83730);
#74036=AXIS2_PLACEMENT_3D('',#125401,#83731,#83732);
#74037=AXIS2_PLACEMENT_3D('',#125421,#83734,#83735);
#74038=AXIS2_PLACEMENT_3D('',#125429,#83737,#83738);
#74039=AXIS2_PLACEMENT_3D('',#125431,#83739,#83740);
#74040=AXIS2_PLACEMENT_3D('',#125433,#83741,#83742);
#74041=AXIS2_PLACEMENT_3D('',#125434,#83743,#83744);
#74042=AXIS2_PLACEMENT_3D('',#125454,#83746,#83747);
#74043=AXIS2_PLACEMENT_3D('',#125462,#83749,#83750);
#74044=AXIS2_PLACEMENT_3D('',#125464,#83751,#83752);
#74045=AXIS2_PLACEMENT_3D('',#125466,#83753,#83754);
#74046=AXIS2_PLACEMENT_3D('',#125467,#83755,#83756);
#74047=AXIS2_PLACEMENT_3D('',#125487,#83758,#83759);
#74048=AXIS2_PLACEMENT_3D('',#125495,#83761,#83762);
#74049=AXIS2_PLACEMENT_3D('',#125497,#83763,#83764);
#74050=AXIS2_PLACEMENT_3D('',#125499,#83765,#83766);
#74051=AXIS2_PLACEMENT_3D('',#125500,#83767,#83768);
#74052=AXIS2_PLACEMENT_3D('',#125520,#83770,#83771);
#74053=AXIS2_PLACEMENT_3D('',#125528,#83773,#83774);
#74054=AXIS2_PLACEMENT_3D('',#125530,#83775,#83776);
#74055=AXIS2_PLACEMENT_3D('',#125532,#83777,#83778);
#74056=AXIS2_PLACEMENT_3D('',#125533,#83779,#83780);
#74057=AXIS2_PLACEMENT_3D('',#125577,#83784,#83785);
#74058=AXIS2_PLACEMENT_3D('',#125585,#83787,#83788);
#74059=AXIS2_PLACEMENT_3D('',#125587,#83789,#83790);
#74060=AXIS2_PLACEMENT_3D('',#125589,#83791,#83792);
#74061=AXIS2_PLACEMENT_3D('',#125590,#83793,#83794);
#74062=AXIS2_PLACEMENT_3D('',#125610,#83796,#83797);
#74063=AXIS2_PLACEMENT_3D('',#125618,#83799,#83800);
#74064=AXIS2_PLACEMENT_3D('',#125620,#83801,#83802);
#74065=AXIS2_PLACEMENT_3D('',#125622,#83803,#83804);
#74066=AXIS2_PLACEMENT_3D('',#125623,#83805,#83806);
#74067=AXIS2_PLACEMENT_3D('',#125643,#83808,#83809);
#74068=AXIS2_PLACEMENT_3D('',#125651,#83811,#83812);
#74069=AXIS2_PLACEMENT_3D('',#125653,#83813,#83814);
#74070=AXIS2_PLACEMENT_3D('',#125655,#83815,#83816);
#74071=AXIS2_PLACEMENT_3D('',#125656,#83817,#83818);
#74072=AXIS2_PLACEMENT_3D('',#125676,#83820,#83821);
#74073=AXIS2_PLACEMENT_3D('',#125684,#83823,#83824);
#74074=AXIS2_PLACEMENT_3D('',#125686,#83825,#83826);
#74075=AXIS2_PLACEMENT_3D('',#125688,#83827,#83828);
#74076=AXIS2_PLACEMENT_3D('',#125689,#83829,#83830);
#74077=AXIS2_PLACEMENT_3D('',#125709,#83832,#83833);
#74078=AXIS2_PLACEMENT_3D('',#125717,#83835,#83836);
#74079=AXIS2_PLACEMENT_3D('',#125719,#83837,#83838);
#74080=AXIS2_PLACEMENT_3D('',#125721,#83839,#83840);
#74081=AXIS2_PLACEMENT_3D('',#125722,#83841,#83842);
#74082=AXIS2_PLACEMENT_3D('',#125742,#83844,#83845);
#74083=AXIS2_PLACEMENT_3D('',#125750,#83847,#83848);
#74084=AXIS2_PLACEMENT_3D('',#125752,#83849,#83850);
#74085=AXIS2_PLACEMENT_3D('',#125754,#83851,#83852);
#74086=AXIS2_PLACEMENT_3D('',#125755,#83853,#83854);
#74087=AXIS2_PLACEMENT_3D('',#125775,#83856,#83857);
#74088=AXIS2_PLACEMENT_3D('',#125790,#83859,#83860);
#74089=AXIS2_PLACEMENT_3D('',#125792,#83862,#83863);
#74090=AXIS2_PLACEMENT_3D('',#125794,#83864,#83865);
#74091=AXIS2_PLACEMENT_3D('',#125795,#83866,#83867);
#74092=AXIS2_PLACEMENT_3D('',#125809,#83869,#83870);
#74093=AXIS2_PLACEMENT_3D('',#125816,#83871,#83872);
#74094=AXIS2_PLACEMENT_3D('',#125818,#83873,#83874);
#74095=AXIS2_PLACEMENT_3D('',#125820,#83875,#83876);
#74096=AXIS2_PLACEMENT_3D('',#125821,#83877,#83878);
#74097=AXIS2_PLACEMENT_3D('',#125841,#83880,#83881);
#74098=AXIS2_PLACEMENT_3D('',#125849,#83883,#83884);
#74099=AXIS2_PLACEMENT_3D('',#125851,#83885,#83886);
#74100=AXIS2_PLACEMENT_3D('',#125853,#83887,#83888);
#74101=AXIS2_PLACEMENT_3D('',#125854,#83889,#83890);
#74102=AXIS2_PLACEMENT_3D('',#125874,#83892,#83893);
#74103=AXIS2_PLACEMENT_3D('',#125882,#83895,#83896);
#74104=AXIS2_PLACEMENT_3D('',#125884,#83897,#83898);
#74105=AXIS2_PLACEMENT_3D('',#125886,#83899,#83900);
#74106=AXIS2_PLACEMENT_3D('',#125887,#83901,#83902);
#74107=AXIS2_PLACEMENT_3D('',#125907,#83904,#83905);
#74108=AXIS2_PLACEMENT_3D('',#125915,#83907,#83908);
#74109=AXIS2_PLACEMENT_3D('',#125917,#83909,#83910);
#74110=AXIS2_PLACEMENT_3D('',#125919,#83911,#83912);
#74111=AXIS2_PLACEMENT_3D('',#125920,#83913,#83914);
#74112=AXIS2_PLACEMENT_3D('',#125940,#83916,#83917);
#74113=AXIS2_PLACEMENT_3D('',#125948,#83919,#83920);
#74114=AXIS2_PLACEMENT_3D('',#125950,#83921,#83922);
#74115=AXIS2_PLACEMENT_3D('',#125952,#83923,#83924);
#74116=AXIS2_PLACEMENT_3D('',#125953,#83925,#83926);
#74117=AXIS2_PLACEMENT_3D('',#125973,#83928,#83929);
#74118=AXIS2_PLACEMENT_3D('',#125981,#83931,#83932);
#74119=AXIS2_PLACEMENT_3D('',#125983,#83933,#83934);
#74120=AXIS2_PLACEMENT_3D('',#125985,#83935,#83936);
#74121=AXIS2_PLACEMENT_3D('',#125986,#83937,#83938);
#74122=AXIS2_PLACEMENT_3D('',#126006,#83940,#83941);
#74123=AXIS2_PLACEMENT_3D('',#126014,#83943,#83944);
#74124=AXIS2_PLACEMENT_3D('',#126016,#83945,#83946);
#74125=AXIS2_PLACEMENT_3D('',#126018,#83947,#83948);
#74126=AXIS2_PLACEMENT_3D('',#126019,#83949,#83950);
#74127=AXIS2_PLACEMENT_3D('',#126040,#83953,#83954);
#74128=AXIS2_PLACEMENT_3D('',#126066,#83956,#83957);
#74129=AXIS2_PLACEMENT_3D('',#126068,#83958,#83959);
#74130=AXIS2_PLACEMENT_3D('',#126069,#83960,#83961);
#74131=AXIS2_PLACEMENT_3D('',#126083,#83963,#83964);
#74132=AXIS2_PLACEMENT_3D('',#126109,#83966,#83967);
#74133=AXIS2_PLACEMENT_3D('',#126111,#83968,#83969);
#74134=AXIS2_PLACEMENT_3D('',#126112,#83970,#83971);
#74135=AXIS2_PLACEMENT_3D('',#126126,#83973,#83974);
#74136=AXIS2_PLACEMENT_3D('',#126152,#83976,#83977);
#74137=AXIS2_PLACEMENT_3D('',#126154,#83978,#83979);
#74138=AXIS2_PLACEMENT_3D('',#126155,#83980,#83981);
#74139=AXIS2_PLACEMENT_3D('',#126169,#83983,#83984);
#74140=AXIS2_PLACEMENT_3D('',#126195,#83986,#83987);
#74141=AXIS2_PLACEMENT_3D('',#126197,#83988,#83989);
#74142=AXIS2_PLACEMENT_3D('',#126198,#83990,#83991);
#74143=AXIS2_PLACEMENT_3D('',#126212,#83993,#83994);
#74144=AXIS2_PLACEMENT_3D('',#126238,#83996,#83997);
#74145=AXIS2_PLACEMENT_3D('',#126240,#83998,#83999);
#74146=AXIS2_PLACEMENT_3D('',#126241,#84000,#84001);
#74147=AXIS2_PLACEMENT_3D('',#126255,#84003,#84004);
#74148=AXIS2_PLACEMENT_3D('',#126281,#84006,#84007);
#74149=AXIS2_PLACEMENT_3D('',#126283,#84008,#84009);
#74150=AXIS2_PLACEMENT_3D('',#126284,#84010,#84011);
#74151=AXIS2_PLACEMENT_3D('',#126298,#84013,#84014);
#74152=AXIS2_PLACEMENT_3D('',#126324,#84016,#84017);
#74153=AXIS2_PLACEMENT_3D('',#126326,#84018,#84019);
#74154=AXIS2_PLACEMENT_3D('',#126327,#84020,#84021);
#74155=AXIS2_PLACEMENT_3D('',#126341,#84023,#84024);
#74156=AXIS2_PLACEMENT_3D('',#126367,#84026,#84027);
#74157=AXIS2_PLACEMENT_3D('',#126369,#84028,#84029);
#74158=AXIS2_PLACEMENT_3D('',#126370,#84030,#84031);
#74159=AXIS2_PLACEMENT_3D('',#126384,#84033,#84034);
#74160=AXIS2_PLACEMENT_3D('',#126410,#84036,#84037);
#74161=AXIS2_PLACEMENT_3D('',#126412,#84038,#84039);
#74162=AXIS2_PLACEMENT_3D('',#126413,#84040,#84041);
#74163=AXIS2_PLACEMENT_3D('',#126427,#84043,#84044);
#74164=AXIS2_PLACEMENT_3D('',#126453,#84046,#84047);
#74165=AXIS2_PLACEMENT_3D('',#126455,#84048,#84049);
#74166=AXIS2_PLACEMENT_3D('',#126456,#84050,#84051);
#74167=AXIS2_PLACEMENT_3D('',#126470,#84053,#84054);
#74168=AXIS2_PLACEMENT_3D('',#126496,#84056,#84057);
#74169=AXIS2_PLACEMENT_3D('',#126498,#84058,#84059);
#74170=AXIS2_PLACEMENT_3D('',#126499,#84060,#84061);
#74171=AXIS2_PLACEMENT_3D('',#126513,#84063,#84064);
#74172=AXIS2_PLACEMENT_3D('',#126539,#84066,#84067);
#74173=AXIS2_PLACEMENT_3D('',#126541,#84068,#84069);
#74174=AXIS2_PLACEMENT_3D('',#126542,#84070,#84071);
#74175=AXIS2_PLACEMENT_3D('',#126556,#84073,#84074);
#74176=AXIS2_PLACEMENT_3D('',#126582,#84076,#84077);
#74177=AXIS2_PLACEMENT_3D('',#126584,#84078,#84079);
#74178=AXIS2_PLACEMENT_3D('',#126585,#84080,#84081);
#74179=AXIS2_PLACEMENT_3D('',#126599,#84083,#84084);
#74180=AXIS2_PLACEMENT_3D('',#126625,#84086,#84087);
#74181=AXIS2_PLACEMENT_3D('',#126627,#84088,#84089);
#74182=AXIS2_PLACEMENT_3D('',#126628,#84090,#84091);
#74183=AXIS2_PLACEMENT_3D('',#126642,#84093,#84094);
#74184=AXIS2_PLACEMENT_3D('',#126668,#84096,#84097);
#74185=AXIS2_PLACEMENT_3D('',#126670,#84098,#84099);
#74186=AXIS2_PLACEMENT_3D('',#126671,#84100,#84101);
#74187=AXIS2_PLACEMENT_3D('',#126685,#84103,#84104);
#74188=AXIS2_PLACEMENT_3D('',#126711,#84106,#84107);
#74189=AXIS2_PLACEMENT_3D('',#126713,#84108,#84109);
#74190=AXIS2_PLACEMENT_3D('',#126714,#84110,#84111);
#74191=AXIS2_PLACEMENT_3D('',#126728,#84113,#84114);
#74192=AXIS2_PLACEMENT_3D('',#126754,#84116,#84117);
#74193=AXIS2_PLACEMENT_3D('',#126756,#84118,#84119);
#74194=AXIS2_PLACEMENT_3D('',#126757,#84120,#84121);
#74195=AXIS2_PLACEMENT_3D('',#126771,#84123,#84124);
#74196=AXIS2_PLACEMENT_3D('',#126797,#84126,#84127);
#74197=AXIS2_PLACEMENT_3D('',#126799,#84128,#84129);
#74198=AXIS2_PLACEMENT_3D('',#126800,#84130,#84131);
#74199=AXIS2_PLACEMENT_3D('',#126814,#84133,#84134);
#74200=AXIS2_PLACEMENT_3D('',#126840,#84136,#84137);
#74201=AXIS2_PLACEMENT_3D('',#126842,#84138,#84139);
#74202=AXIS2_PLACEMENT_3D('',#126843,#84140,#84141);
#74203=AXIS2_PLACEMENT_3D('',#126857,#84143,#84144);
#74204=AXIS2_PLACEMENT_3D('',#126883,#84146,#84147);
#74205=AXIS2_PLACEMENT_3D('',#126885,#84148,#84149);
#74206=AXIS2_PLACEMENT_3D('',#126886,#84150,#84151);
#74207=AXIS2_PLACEMENT_3D('',#126900,#84153,#84154);
#74208=AXIS2_PLACEMENT_3D('',#126926,#84156,#84157);
#74209=AXIS2_PLACEMENT_3D('',#126928,#84158,#84159);
#74210=AXIS2_PLACEMENT_3D('',#126929,#84160,#84161);
#74211=AXIS2_PLACEMENT_3D('',#126971,#84165,#84166);
#74212=AXIS2_PLACEMENT_3D('',#126997,#84168,#84169);
#74213=AXIS2_PLACEMENT_3D('',#126999,#84170,#84171);
#74214=AXIS2_PLACEMENT_3D('',#127000,#84172,#84173);
#74215=AXIS2_PLACEMENT_3D('',#127014,#84175,#84176);
#74216=AXIS2_PLACEMENT_3D('',#127040,#84178,#84179);
#74217=AXIS2_PLACEMENT_3D('',#127042,#84180,#84181);
#74218=AXIS2_PLACEMENT_3D('',#127043,#84182,#84183);
#74219=AXIS2_PLACEMENT_3D('',#127057,#84185,#84186);
#74220=AXIS2_PLACEMENT_3D('',#127083,#84188,#84189);
#74221=AXIS2_PLACEMENT_3D('',#127085,#84190,#84191);
#74222=AXIS2_PLACEMENT_3D('',#127086,#84192,#84193);
#74223=AXIS2_PLACEMENT_3D('',#127100,#84195,#84196);
#74224=AXIS2_PLACEMENT_3D('',#127126,#84198,#84199);
#74225=AXIS2_PLACEMENT_3D('',#127128,#84200,#84201);
#74226=AXIS2_PLACEMENT_3D('',#127129,#84202,#84203);
#74227=AXIS2_PLACEMENT_3D('',#127143,#84205,#84206);
#74228=AXIS2_PLACEMENT_3D('',#127169,#84208,#84209);
#74229=AXIS2_PLACEMENT_3D('',#127171,#84210,#84211);
#74230=AXIS2_PLACEMENT_3D('',#127172,#84212,#84213);
#74231=AXIS2_PLACEMENT_3D('',#127186,#84215,#84216);
#74232=AXIS2_PLACEMENT_3D('',#127212,#84218,#84219);
#74233=AXIS2_PLACEMENT_3D('',#127214,#84220,#84221);
#74234=AXIS2_PLACEMENT_3D('',#127215,#84222,#84223);
#74235=AXIS2_PLACEMENT_3D('',#127229,#84225,#84226);
#74236=AXIS2_PLACEMENT_3D('',#127255,#84228,#84229);
#74237=AXIS2_PLACEMENT_3D('',#127257,#84230,#84231);
#74238=AXIS2_PLACEMENT_3D('',#127258,#84232,#84233);
#74239=AXIS2_PLACEMENT_3D('',#127270,#84234,#84235);
#74240=AXIS2_PLACEMENT_3D('',#127283,#84236,#84237);
#74241=AXIS2_PLACEMENT_3D('',#127295,#84238,#84239);
#74242=AXIS2_PLACEMENT_3D('',#127308,#84240,#84241);
#74243=AXIS2_PLACEMENT_3D('',#127320,#84242,#84243);
#74244=AXIS2_PLACEMENT_3D('',#127333,#84244,#84245);
#74245=AXIS2_PLACEMENT_3D('',#127345,#84246,#84247);
#74246=AXIS2_PLACEMENT_3D('',#127358,#84248,#84249);
#74247=AXIS2_PLACEMENT_3D('',#127370,#84250,#84251);
#74248=AXIS2_PLACEMENT_3D('',#127383,#84252,#84253);
#74249=AXIS2_PLACEMENT_3D('',#127395,#84254,#84255);
#74250=AXIS2_PLACEMENT_3D('',#127408,#84256,#84257);
#74251=AXIS2_PLACEMENT_3D('',#127420,#84258,#84259);
#74252=AXIS2_PLACEMENT_3D('',#127433,#84260,#84261);
#74253=AXIS2_PLACEMENT_3D('',#127445,#84262,#84263);
#74254=AXIS2_PLACEMENT_3D('',#127458,#84264,#84265);
#74255=AXIS2_PLACEMENT_3D('',#127470,#84266,#84267);
#74256=AXIS2_PLACEMENT_3D('',#127483,#84268,#84269);
#74257=AXIS2_PLACEMENT_3D('',#127495,#84270,#84271);
#74258=AXIS2_PLACEMENT_3D('',#127508,#84272,#84273);
#74259=AXIS2_PLACEMENT_3D('',#127520,#84274,#84275);
#74260=AXIS2_PLACEMENT_3D('',#127533,#84276,#84277);
#74261=AXIS2_PLACEMENT_3D('',#127545,#84278,#84279);
#74262=AXIS2_PLACEMENT_3D('',#127558,#84280,#84281);
#74263=AXIS2_PLACEMENT_3D('',#127570,#84282,#84283);
#74264=AXIS2_PLACEMENT_3D('',#127583,#84284,#84285);
#74265=AXIS2_PLACEMENT_3D('',#127595,#84286,#84287);
#74266=AXIS2_PLACEMENT_3D('',#127608,#84288,#84289);
#74267=AXIS2_PLACEMENT_3D('',#127620,#84290,#84291);
#74268=AXIS2_PLACEMENT_3D('',#127633,#84292,#84293);
#74269=AXIS2_PLACEMENT_3D('',#127645,#84294,#84295);
#74270=AXIS2_PLACEMENT_3D('',#127658,#84296,#84297);
#74271=AXIS2_PLACEMENT_3D('',#127670,#84298,#84299);
#74272=AXIS2_PLACEMENT_3D('',#127683,#84300,#84301);
#74273=AXIS2_PLACEMENT_3D('',#127695,#84302,#84303);
#74274=AXIS2_PLACEMENT_3D('',#127708,#84304,#84305);
#74275=AXIS2_PLACEMENT_3D('',#127720,#84306,#84307);
#74276=AXIS2_PLACEMENT_3D('',#127733,#84308,#84309);
#74277=AXIS2_PLACEMENT_3D('',#127745,#84310,#84311);
#74278=AXIS2_PLACEMENT_3D('',#127758,#84312,#84313);
#74279=AXIS2_PLACEMENT_3D('',#127770,#84314,#84315);
#74280=AXIS2_PLACEMENT_3D('',#127783,#84316,#84317);
#74281=AXIS2_PLACEMENT_3D('',#127795,#84318,#84319);
#74282=AXIS2_PLACEMENT_3D('',#127808,#84320,#84321);
#74283=AXIS2_PLACEMENT_3D('',#127820,#84322,#84323);
#74284=AXIS2_PLACEMENT_3D('',#127833,#84324,#84325);
#74285=AXIS2_PLACEMENT_3D('',#127845,#84326,#84327);
#74286=AXIS2_PLACEMENT_3D('',#127858,#84328,#84329);
#74287=AXIS2_PLACEMENT_3D('',#127870,#84330,#84331);
#74288=AXIS2_PLACEMENT_3D('',#127883,#84332,#84333);
#74289=AXIS2_PLACEMENT_3D('',#127895,#84334,#84335);
#74290=AXIS2_PLACEMENT_3D('',#127908,#84336,#84337);
#74291=AXIS2_PLACEMENT_3D('',#127920,#84338,#84339);
#74292=AXIS2_PLACEMENT_3D('',#127933,#84340,#84341);
#74293=AXIS2_PLACEMENT_3D('',#127945,#84342,#84343);
#74294=AXIS2_PLACEMENT_3D('',#127958,#84344,#84345);
#74295=AXIS2_PLACEMENT_3D('',#127970,#84346,#84347);
#74296=AXIS2_PLACEMENT_3D('',#127983,#84348,#84349);
#74297=AXIS2_PLACEMENT_3D('',#127995,#84350,#84351);
#74298=AXIS2_PLACEMENT_3D('',#128008,#84352,#84353);
#74299=AXIS2_PLACEMENT_3D('',#128020,#84354,#84355);
#74300=AXIS2_PLACEMENT_3D('',#128033,#84356,#84357);
#74301=AXIS2_PLACEMENT_3D('',#128045,#84358,#84359);
#74302=AXIS2_PLACEMENT_3D('',#128058,#84360,#84361);
#74303=AXIS2_PLACEMENT_3D('',#128070,#84362,#84363);
#74304=AXIS2_PLACEMENT_3D('',#128083,#84364,#84365);
#74305=AXIS2_PLACEMENT_3D('',#128095,#84366,#84367);
#74306=AXIS2_PLACEMENT_3D('',#128108,#84368,#84369);
#74307=AXIS2_PLACEMENT_3D('',#128120,#84370,#84371);
#74308=AXIS2_PLACEMENT_3D('',#128133,#84372,#84373);
#74309=AXIS2_PLACEMENT_3D('',#128145,#84374,#84375);
#74310=AXIS2_PLACEMENT_3D('',#128158,#84376,#84377);
#74311=AXIS2_PLACEMENT_3D('',#128170,#84378,#84379);
#74312=AXIS2_PLACEMENT_3D('',#128183,#84380,#84381);
#74313=AXIS2_PLACEMENT_3D('',#128195,#84382,#84383);
#74314=AXIS2_PLACEMENT_3D('',#128208,#84384,#84385);
#74315=AXIS2_PLACEMENT_3D('',#128220,#84386,#84387);
#74316=AXIS2_PLACEMENT_3D('',#128233,#84388,#84389);
#74317=AXIS2_PLACEMENT_3D('',#128245,#84390,#84391);
#74318=AXIS2_PLACEMENT_3D('',#128258,#84392,#84393);
#74319=AXIS2_PLACEMENT_3D('',#128270,#84394,#84395);
#74320=AXIS2_PLACEMENT_3D('',#128283,#84396,#84397);
#74321=AXIS2_PLACEMENT_3D('',#128295,#84398,#84399);
#74322=AXIS2_PLACEMENT_3D('',#128308,#84400,#84401);
#74323=AXIS2_PLACEMENT_3D('',#128320,#84402,#84403);
#74324=AXIS2_PLACEMENT_3D('',#128333,#84404,#84405);
#74325=AXIS2_PLACEMENT_3D('',#128345,#84406,#84407);
#74326=AXIS2_PLACEMENT_3D('',#128358,#84408,#84409);
#74327=AXIS2_PLACEMENT_3D('',#128370,#84410,#84411);
#74328=AXIS2_PLACEMENT_3D('',#128383,#84412,#84413);
#74329=AXIS2_PLACEMENT_3D('',#128395,#84414,#84415);
#74330=AXIS2_PLACEMENT_3D('',#128408,#84416,#84417);
#74331=AXIS2_PLACEMENT_3D('',#128420,#84418,#84419);
#74332=AXIS2_PLACEMENT_3D('',#128433,#84420,#84421);
#74333=AXIS2_PLACEMENT_3D('',#128445,#84422,#84423);
#74334=AXIS2_PLACEMENT_3D('',#128458,#84424,#84425);
#74335=AXIS2_PLACEMENT_3D('',#128470,#84426,#84427);
#74336=AXIS2_PLACEMENT_3D('',#128483,#84428,#84429);
#74337=AXIS2_PLACEMENT_3D('',#128495,#84430,#84431);
#74338=AXIS2_PLACEMENT_3D('',#128508,#84432,#84433);
#74339=AXIS2_PLACEMENT_3D('',#128520,#84434,#84435);
#74340=AXIS2_PLACEMENT_3D('',#128533,#84436,#84437);
#74341=AXIS2_PLACEMENT_3D('',#128545,#84438,#84439);
#74342=AXIS2_PLACEMENT_3D('',#128558,#84440,#84441);
#74343=AXIS2_PLACEMENT_3D('',#128570,#84442,#84443);
#74344=AXIS2_PLACEMENT_3D('',#128583,#84444,#84445);
#74345=AXIS2_PLACEMENT_3D('',#128595,#84446,#84447);
#74346=AXIS2_PLACEMENT_3D('',#128608,#84448,#84449);
#74347=AXIS2_PLACEMENT_3D('',#128620,#84450,#84451);
#74348=AXIS2_PLACEMENT_3D('',#128633,#84452,#84453);
#74349=AXIS2_PLACEMENT_3D('',#128645,#84454,#84455);
#74350=AXIS2_PLACEMENT_3D('',#128658,#84456,#84457);
#74351=AXIS2_PLACEMENT_3D('',#128670,#84458,#84459);
#74352=AXIS2_PLACEMENT_3D('',#128683,#84460,#84461);
#74353=AXIS2_PLACEMENT_3D('',#128695,#84462,#84463);
#74354=AXIS2_PLACEMENT_3D('',#128708,#84464,#84465);
#74355=AXIS2_PLACEMENT_3D('',#128721,#84466,#84467);
#74356=AXIS2_PLACEMENT_3D('',#128741,#84469,#84470);
#74357=AXIS2_PLACEMENT_3D('',#128749,#84472,#84473);
#74358=AXIS2_PLACEMENT_3D('',#128751,#84474,#84475);
#74359=AXIS2_PLACEMENT_3D('',#128753,#84476,#84477);
#74360=AXIS2_PLACEMENT_3D('',#128754,#84478,#84479);
#74361=AXIS2_PLACEMENT_3D('',#128778,#84481,#84482);
#74362=AXIS2_PLACEMENT_3D('',#128786,#84484,#84485);
#74363=AXIS2_PLACEMENT_3D('',#128788,#84486,#84487);
#74364=AXIS2_PLACEMENT_3D('',#128790,#84488,#84489);
#74365=AXIS2_PLACEMENT_3D('',#128791,#84490,#84491);
#74366=AXIS2_PLACEMENT_3D('',#128815,#84493,#84494);
#74367=AXIS2_PLACEMENT_3D('',#128823,#84496,#84497);
#74368=AXIS2_PLACEMENT_3D('',#128825,#84498,#84499);
#74369=AXIS2_PLACEMENT_3D('',#128827,#84500,#84501);
#74370=AXIS2_PLACEMENT_3D('',#128828,#84502,#84503);
#74371=AXIS2_PLACEMENT_3D('',#128852,#84505,#84506);
#74372=AXIS2_PLACEMENT_3D('',#128860,#84508,#84509);
#74373=AXIS2_PLACEMENT_3D('',#128862,#84510,#84511);
#74374=AXIS2_PLACEMENT_3D('',#128864,#84512,#84513);
#74375=AXIS2_PLACEMENT_3D('',#128865,#84514,#84515);
#74376=AXIS2_PLACEMENT_3D('',#128889,#84517,#84518);
#74377=AXIS2_PLACEMENT_3D('',#128897,#84520,#84521);
#74378=AXIS2_PLACEMENT_3D('',#128899,#84522,#84523);
#74379=AXIS2_PLACEMENT_3D('',#128901,#84524,#84525);
#74380=AXIS2_PLACEMENT_3D('',#128902,#84526,#84527);
#74381=AXIS2_PLACEMENT_3D('',#128926,#84529,#84530);
#74382=AXIS2_PLACEMENT_3D('',#128934,#84532,#84533);
#74383=AXIS2_PLACEMENT_3D('',#128936,#84534,#84535);
#74384=AXIS2_PLACEMENT_3D('',#128938,#84536,#84537);
#74385=AXIS2_PLACEMENT_3D('',#128939,#84538,#84539);
#74386=AXIS2_PLACEMENT_3D('',#128991,#84543,#84544);
#74387=AXIS2_PLACEMENT_3D('',#128999,#84546,#84547);
#74388=AXIS2_PLACEMENT_3D('',#129001,#84548,#84549);
#74389=AXIS2_PLACEMENT_3D('',#129003,#84550,#84551);
#74390=AXIS2_PLACEMENT_3D('',#129004,#84552,#84553);
#74391=AXIS2_PLACEMENT_3D('',#129028,#84555,#84556);
#74392=AXIS2_PLACEMENT_3D('',#129036,#84558,#84559);
#74393=AXIS2_PLACEMENT_3D('',#129038,#84560,#84561);
#74394=AXIS2_PLACEMENT_3D('',#129040,#84562,#84563);
#74395=AXIS2_PLACEMENT_3D('',#129041,#84564,#84565);
#74396=AXIS2_PLACEMENT_3D('',#129065,#84567,#84568);
#74397=AXIS2_PLACEMENT_3D('',#129073,#84570,#84571);
#74398=AXIS2_PLACEMENT_3D('',#129075,#84572,#84573);
#74399=AXIS2_PLACEMENT_3D('',#129077,#84574,#84575);
#74400=AXIS2_PLACEMENT_3D('',#129078,#84576,#84577);
#74401=AXIS2_PLACEMENT_3D('',#129102,#84579,#84580);
#74402=AXIS2_PLACEMENT_3D('',#129110,#84582,#84583);
#74403=AXIS2_PLACEMENT_3D('',#129112,#84584,#84585);
#74404=AXIS2_PLACEMENT_3D('',#129114,#84586,#84587);
#74405=AXIS2_PLACEMENT_3D('',#129115,#84588,#84589);
#74406=AXIS2_PLACEMENT_3D('',#129139,#84591,#84592);
#74407=AXIS2_PLACEMENT_3D('',#129147,#84594,#84595);
#74408=AXIS2_PLACEMENT_3D('',#129149,#84596,#84597);
#74409=AXIS2_PLACEMENT_3D('',#129151,#84598,#84599);
#74410=AXIS2_PLACEMENT_3D('',#129152,#84600,#84601);
#74411=AXIS2_PLACEMENT_3D('',#129176,#84603,#84604);
#74412=AXIS2_PLACEMENT_3D('',#129184,#84606,#84607);
#74413=AXIS2_PLACEMENT_3D('',#129186,#84608,#84609);
#74414=AXIS2_PLACEMENT_3D('',#129188,#84610,#84611);
#74415=AXIS2_PLACEMENT_3D('',#129189,#84612,#84613);
#74416=AXIS2_PLACEMENT_3D('',#129213,#84615,#84616);
#74417=AXIS2_PLACEMENT_3D('',#129221,#84618,#84619);
#74418=AXIS2_PLACEMENT_3D('',#129223,#84620,#84621);
#74419=AXIS2_PLACEMENT_3D('',#129225,#84622,#84623);
#74420=AXIS2_PLACEMENT_3D('',#129226,#84624,#84625);
#74421=AXIS2_PLACEMENT_3D('',#129250,#84627,#84628);
#74422=AXIS2_PLACEMENT_3D('',#129258,#84630,#84631);
#74423=AXIS2_PLACEMENT_3D('',#129260,#84632,#84633);
#74424=AXIS2_PLACEMENT_3D('',#129262,#84634,#84635);
#74425=AXIS2_PLACEMENT_3D('',#129263,#84636,#84637);
#74426=AXIS2_PLACEMENT_3D('',#129287,#84639,#84640);
#74427=AXIS2_PLACEMENT_3D('',#129295,#84642,#84643);
#74428=AXIS2_PLACEMENT_3D('',#129297,#84644,#84645);
#74429=AXIS2_PLACEMENT_3D('',#129299,#84646,#84647);
#74430=AXIS2_PLACEMENT_3D('',#129300,#84648,#84649);
#74431=AXIS2_PLACEMENT_3D('',#129324,#84651,#84652);
#74432=AXIS2_PLACEMENT_3D('',#129332,#84654,#84655);
#74433=AXIS2_PLACEMENT_3D('',#129334,#84656,#84657);
#74434=AXIS2_PLACEMENT_3D('',#129336,#84658,#84659);
#74435=AXIS2_PLACEMENT_3D('',#129337,#84660,#84661);
#74436=AXIS2_PLACEMENT_3D('',#129361,#84663,#84664);
#74437=AXIS2_PLACEMENT_3D('',#129369,#84666,#84667);
#74438=AXIS2_PLACEMENT_3D('',#129371,#84668,#84669);
#74439=AXIS2_PLACEMENT_3D('',#129373,#84670,#84671);
#74440=AXIS2_PLACEMENT_3D('',#129374,#84672,#84673);
#74441=AXIS2_PLACEMENT_3D('',#129398,#84675,#84676);
#74442=AXIS2_PLACEMENT_3D('',#129406,#84678,#84679);
#74443=AXIS2_PLACEMENT_3D('',#129408,#84680,#84681);
#74444=AXIS2_PLACEMENT_3D('',#129410,#84682,#84683);
#74445=AXIS2_PLACEMENT_3D('',#129411,#84684,#84685);
#74446=AXIS2_PLACEMENT_3D('',#129435,#84687,#84688);
#74447=AXIS2_PLACEMENT_3D('',#129443,#84690,#84691);
#74448=AXIS2_PLACEMENT_3D('',#129445,#84692,#84693);
#74449=AXIS2_PLACEMENT_3D('',#129447,#84694,#84695);
#74450=AXIS2_PLACEMENT_3D('',#129448,#84696,#84697);
#74451=AXIS2_PLACEMENT_3D('',#129472,#84699,#84700);
#74452=AXIS2_PLACEMENT_3D('',#129491,#84702,#84703);
#74453=AXIS2_PLACEMENT_3D('',#129493,#84705,#84706);
#74454=AXIS2_PLACEMENT_3D('',#129495,#84707,#84708);
#74455=AXIS2_PLACEMENT_3D('',#129496,#84709,#84710);
#74456=AXIS2_PLACEMENT_3D('',#129510,#84712,#84713);
#74457=AXIS2_PLACEMENT_3D('',#129517,#84714,#84715);
#74458=AXIS2_PLACEMENT_3D('',#129519,#84716,#84717);
#74459=AXIS2_PLACEMENT_3D('',#129521,#84718,#84719);
#74460=AXIS2_PLACEMENT_3D('',#129522,#84720,#84721);
#74461=AXIS2_PLACEMENT_3D('',#129546,#84723,#84724);
#74462=AXIS2_PLACEMENT_3D('',#129554,#84726,#84727);
#74463=AXIS2_PLACEMENT_3D('',#129556,#84728,#84729);
#74464=AXIS2_PLACEMENT_3D('',#129558,#84730,#84731);
#74465=AXIS2_PLACEMENT_3D('',#129559,#84732,#84733);
#74466=AXIS2_PLACEMENT_3D('',#129583,#84735,#84736);
#74467=AXIS2_PLACEMENT_3D('',#129591,#84738,#84739);
#74468=AXIS2_PLACEMENT_3D('',#129593,#84740,#84741);
#74469=AXIS2_PLACEMENT_3D('',#129595,#84742,#84743);
#74470=AXIS2_PLACEMENT_3D('',#129596,#84744,#84745);
#74471=AXIS2_PLACEMENT_3D('',#129620,#84747,#84748);
#74472=AXIS2_PLACEMENT_3D('',#129628,#84750,#84751);
#74473=AXIS2_PLACEMENT_3D('',#129630,#84752,#84753);
#74474=AXIS2_PLACEMENT_3D('',#129632,#84754,#84755);
#74475=AXIS2_PLACEMENT_3D('',#129633,#84756,#84757);
#74476=AXIS2_PLACEMENT_3D('',#129657,#84759,#84760);
#74477=AXIS2_PLACEMENT_3D('',#129665,#84762,#84763);
#74478=AXIS2_PLACEMENT_3D('',#129667,#84764,#84765);
#74479=AXIS2_PLACEMENT_3D('',#129669,#84766,#84767);
#74480=AXIS2_PLACEMENT_3D('',#129670,#84768,#84769);
#74481=AXIS2_PLACEMENT_3D('',#129694,#84771,#84772);
#74482=AXIS2_PLACEMENT_3D('',#129702,#84774,#84775);
#74483=AXIS2_PLACEMENT_3D('',#129704,#84776,#84777);
#74484=AXIS2_PLACEMENT_3D('',#129706,#84778,#84779);
#74485=AXIS2_PLACEMENT_3D('',#129707,#84780,#84781);
#74486=AXIS2_PLACEMENT_3D('',#129731,#84783,#84784);
#74487=AXIS2_PLACEMENT_3D('',#129739,#84786,#84787);
#74488=AXIS2_PLACEMENT_3D('',#129741,#84788,#84789);
#74489=AXIS2_PLACEMENT_3D('',#129743,#84790,#84791);
#74490=AXIS2_PLACEMENT_3D('',#129744,#84792,#84793);
#74491=AXIS2_PLACEMENT_3D('',#129756,#84795,#84796);
#74492=AXIS2_PLACEMENT_3D('',#129759,#84797,#84798);
#74493=AXIS2_PLACEMENT_3D('',#129760,#84799,#84800);
#74494=AXIS2_PLACEMENT_3D('',#129761,#84801,#84802);
#74495=AXIS2_PLACEMENT_3D('',#129787,#84804,#84805);
#74496=AXIS2_PLACEMENT_3D('',#129802,#84808,#84809);
#74497=AXIS2_PLACEMENT_3D('',#129816,#84810,#84811);
#74498=AXIS2_PLACEMENT_3D('',#129818,#84813,#84814);
#74499=AXIS2_PLACEMENT_3D('',#129820,#84815,#84816);
#74500=AXIS2_PLACEMENT_3D('',#129821,#84817,#84818);
#74501=AXIS2_PLACEMENT_3D('',#129835,#84820,#84821);
#74502=AXIS2_PLACEMENT_3D('',#129849,#84822,#84823);
#74503=AXIS2_PLACEMENT_3D('',#129851,#84825,#84826);
#74504=AXIS2_PLACEMENT_3D('',#129853,#84827,#84828);
#74505=AXIS2_PLACEMENT_3D('',#129854,#84829,#84830);
#74506=AXIS2_PLACEMENT_3D('',#129868,#84832,#84833);
#74507=AXIS2_PLACEMENT_3D('',#129882,#84834,#84835);
#74508=AXIS2_PLACEMENT_3D('',#129884,#84837,#84838);
#74509=AXIS2_PLACEMENT_3D('',#129886,#84839,#84840);
#74510=AXIS2_PLACEMENT_3D('',#129887,#84841,#84842);
#74511=AXIS2_PLACEMENT_3D('',#129901,#84844,#84845);
#74512=AXIS2_PLACEMENT_3D('',#129915,#84846,#84847);
#74513=AXIS2_PLACEMENT_3D('',#129917,#84849,#84850);
#74514=AXIS2_PLACEMENT_3D('',#129919,#84851,#84852);
#74515=AXIS2_PLACEMENT_3D('',#129920,#84853,#84854);
#74516=AXIS2_PLACEMENT_3D('',#129934,#84856,#84857);
#74517=AXIS2_PLACEMENT_3D('',#129948,#84858,#84859);
#74518=AXIS2_PLACEMENT_3D('',#129950,#84861,#84862);
#74519=AXIS2_PLACEMENT_3D('',#129952,#84863,#84864);
#74520=AXIS2_PLACEMENT_3D('',#129953,#84865,#84866);
#74521=AXIS2_PLACEMENT_3D('',#129967,#84868,#84869);
#74522=AXIS2_PLACEMENT_3D('',#129981,#84870,#84871);
#74523=AXIS2_PLACEMENT_3D('',#129983,#84873,#84874);
#74524=AXIS2_PLACEMENT_3D('',#129985,#84875,#84876);
#74525=AXIS2_PLACEMENT_3D('',#129986,#84877,#84878);
#74526=AXIS2_PLACEMENT_3D('',#130000,#84880,#84881);
#74527=AXIS2_PLACEMENT_3D('',#130014,#84882,#84883);
#74528=AXIS2_PLACEMENT_3D('',#130016,#84885,#84886);
#74529=AXIS2_PLACEMENT_3D('',#130018,#84887,#84888);
#74530=AXIS2_PLACEMENT_3D('',#130019,#84889,#84890);
#74531=AXIS2_PLACEMENT_3D('',#130033,#84892,#84893);
#74532=AXIS2_PLACEMENT_3D('',#130047,#84894,#84895);
#74533=AXIS2_PLACEMENT_3D('',#130049,#84897,#84898);
#74534=AXIS2_PLACEMENT_3D('',#130051,#84899,#84900);
#74535=AXIS2_PLACEMENT_3D('',#130052,#84901,#84902);
#74536=AXIS2_PLACEMENT_3D('',#130066,#84904,#84905);
#74537=AXIS2_PLACEMENT_3D('',#130080,#84906,#84907);
#74538=AXIS2_PLACEMENT_3D('',#130082,#84909,#84910);
#74539=AXIS2_PLACEMENT_3D('',#130084,#84911,#84912);
#74540=AXIS2_PLACEMENT_3D('',#130085,#84913,#84914);
#74541=AXIS2_PLACEMENT_3D('',#130099,#84916,#84917);
#74542=AXIS2_PLACEMENT_3D('',#130113,#84918,#84919);
#74543=AXIS2_PLACEMENT_3D('',#130115,#84921,#84922);
#74544=AXIS2_PLACEMENT_3D('',#130117,#84923,#84924);
#74545=AXIS2_PLACEMENT_3D('',#130118,#84925,#84926);
#74546=AXIS2_PLACEMENT_3D('',#130132,#84928,#84929);
#74547=AXIS2_PLACEMENT_3D('',#130146,#84930,#84931);
#74548=AXIS2_PLACEMENT_3D('',#130148,#84933,#84934);
#74549=AXIS2_PLACEMENT_3D('',#130150,#84935,#84936);
#74550=AXIS2_PLACEMENT_3D('',#130151,#84937,#84938);
#74551=AXIS2_PLACEMENT_3D('',#130165,#84940,#84941);
#74552=AXIS2_PLACEMENT_3D('',#130179,#84942,#84943);
#74553=AXIS2_PLACEMENT_3D('',#130181,#84945,#84946);
#74554=AXIS2_PLACEMENT_3D('',#130183,#84947,#84948);
#74555=AXIS2_PLACEMENT_3D('',#130184,#84949,#84950);
#74556=AXIS2_PLACEMENT_3D('',#130198,#84952,#84953);
#74557=AXIS2_PLACEMENT_3D('',#130212,#84954,#84955);
#74558=AXIS2_PLACEMENT_3D('',#130214,#84957,#84958);
#74559=AXIS2_PLACEMENT_3D('',#130216,#84959,#84960);
#74560=AXIS2_PLACEMENT_3D('',#130217,#84961,#84962);
#74561=AXIS2_PLACEMENT_3D('',#130255,#84966,#84967);
#74562=AXIS2_PLACEMENT_3D('',#130269,#84968,#84969);
#74563=AXIS2_PLACEMENT_3D('',#130271,#84971,#84972);
#74564=AXIS2_PLACEMENT_3D('',#130273,#84973,#84974);
#74565=AXIS2_PLACEMENT_3D('',#130274,#84975,#84976);
#74566=AXIS2_PLACEMENT_3D('',#130288,#84978,#84979);
#74567=AXIS2_PLACEMENT_3D('',#130302,#84980,#84981);
#74568=AXIS2_PLACEMENT_3D('',#130304,#84983,#84984);
#74569=AXIS2_PLACEMENT_3D('',#130306,#84985,#84986);
#74570=AXIS2_PLACEMENT_3D('',#130307,#84987,#84988);
#74571=AXIS2_PLACEMENT_3D('',#130321,#84990,#84991);
#74572=AXIS2_PLACEMENT_3D('',#130335,#84992,#84993);
#74573=AXIS2_PLACEMENT_3D('',#130337,#84995,#84996);
#74574=AXIS2_PLACEMENT_3D('',#130339,#84997,#84998);
#74575=AXIS2_PLACEMENT_3D('',#130340,#84999,#85000);
#74576=AXIS2_PLACEMENT_3D('',#130354,#85002,#85003);
#74577=AXIS2_PLACEMENT_3D('',#130368,#85004,#85005);
#74578=AXIS2_PLACEMENT_3D('',#130370,#85007,#85008);
#74579=AXIS2_PLACEMENT_3D('',#130372,#85009,#85010);
#74580=AXIS2_PLACEMENT_3D('',#130373,#85011,#85012);
#74581=AXIS2_PLACEMENT_3D('',#130387,#85014,#85015);
#74582=AXIS2_PLACEMENT_3D('',#130401,#85016,#85017);
#74583=AXIS2_PLACEMENT_3D('',#130403,#85019,#85020);
#74584=AXIS2_PLACEMENT_3D('',#130405,#85021,#85022);
#74585=AXIS2_PLACEMENT_3D('',#130406,#85023,#85024);
#74586=AXIS2_PLACEMENT_3D('',#130420,#85026,#85027);
#74587=AXIS2_PLACEMENT_3D('',#130434,#85028,#85029);
#74588=AXIS2_PLACEMENT_3D('',#130436,#85031,#85032);
#74589=AXIS2_PLACEMENT_3D('',#130438,#85033,#85034);
#74590=AXIS2_PLACEMENT_3D('',#130439,#85035,#85036);
#74591=AXIS2_PLACEMENT_3D('',#130453,#85038,#85039);
#74592=AXIS2_PLACEMENT_3D('',#130467,#85040,#85041);
#74593=AXIS2_PLACEMENT_3D('',#130469,#85043,#85044);
#74594=AXIS2_PLACEMENT_3D('',#130471,#85045,#85046);
#74595=AXIS2_PLACEMENT_3D('',#130472,#85047,#85048);
#74596=AXIS2_PLACEMENT_3D('',#130486,#85050,#85051);
#74597=AXIS2_PLACEMENT_3D('',#130500,#85052,#85053);
#74598=AXIS2_PLACEMENT_3D('',#130502,#85055,#85056);
#74599=AXIS2_PLACEMENT_3D('',#130504,#85057,#85058);
#74600=AXIS2_PLACEMENT_3D('',#130505,#85059,#85060);
#74601=AXIS2_PLACEMENT_3D('',#130519,#85062,#85063);
#74602=AXIS2_PLACEMENT_3D('',#130533,#85064,#85065);
#74603=AXIS2_PLACEMENT_3D('',#130535,#85067,#85068);
#74604=AXIS2_PLACEMENT_3D('',#130537,#85069,#85070);
#74605=AXIS2_PLACEMENT_3D('',#130538,#85071,#85072);
#74606=AXIS2_PLACEMENT_3D('',#130552,#85074,#85075);
#74607=AXIS2_PLACEMENT_3D('',#130566,#85076,#85077);
#74608=AXIS2_PLACEMENT_3D('',#130568,#85079,#85080);
#74609=AXIS2_PLACEMENT_3D('',#130570,#85081,#85082);
#74610=AXIS2_PLACEMENT_3D('',#130571,#85083,#85084);
#74611=AXIS2_PLACEMENT_3D('',#130585,#85086,#85087);
#74612=AXIS2_PLACEMENT_3D('',#130599,#85088,#85089);
#74613=AXIS2_PLACEMENT_3D('',#130601,#85091,#85092);
#74614=AXIS2_PLACEMENT_3D('',#130603,#85093,#85094);
#74615=AXIS2_PLACEMENT_3D('',#130604,#85095,#85096);
#74616=AXIS2_PLACEMENT_3D('',#130618,#85098,#85099);
#74617=AXIS2_PLACEMENT_3D('',#130632,#85100,#85101);
#74618=AXIS2_PLACEMENT_3D('',#130634,#85103,#85104);
#74619=AXIS2_PLACEMENT_3D('',#130636,#85105,#85106);
#74620=AXIS2_PLACEMENT_3D('',#130637,#85107,#85108);
#74621=AXIS2_PLACEMENT_3D('',#130651,#85110,#85111);
#74622=AXIS2_PLACEMENT_3D('',#130665,#85112,#85113);
#74623=AXIS2_PLACEMENT_3D('',#130667,#85115,#85116);
#74624=AXIS2_PLACEMENT_3D('',#130669,#85117,#85118);
#74625=AXIS2_PLACEMENT_3D('',#130670,#85119,#85120);
#74626=AXIS2_PLACEMENT_3D('',#130684,#85122,#85123);
#74627=AXIS2_PLACEMENT_3D('',#130698,#85124,#85125);
#74628=AXIS2_PLACEMENT_3D('',#130700,#85127,#85128);
#74629=AXIS2_PLACEMENT_3D('',#130702,#85129,#85130);
#74630=AXIS2_PLACEMENT_3D('',#130703,#85131,#85132);
#74631=AXIS2_PLACEMENT_3D('',#130704,#85133,#85134);
#74632=AXIS2_PLACEMENT_3D('',#130706,#85135,#85136);
#74633=AXIS2_PLACEMENT_3D('',#130708,#85137,#85138);
#74634=AXIS2_PLACEMENT_3D('',#130709,#85139,#85140);
#74635=AXIS2_PLACEMENT_3D('',#130728,#85142,#85143);
#74636=AXIS2_PLACEMENT_3D('',#130776,#85144,#85145);
#74637=AXIS2_PLACEMENT_3D('',#130814,#85146,#85147);
#74638=AXIS2_PLACEMENT_3D('',#130852,#85148,#85149);
#74639=AXIS2_PLACEMENT_3D('',#130890,#85150,#85151);
#74640=AXIS2_PLACEMENT_3D('',#130928,#85152,#85153);
#74641=AXIS2_PLACEMENT_3D('',#130966,#85154,#85155);
#74642=AXIS2_PLACEMENT_3D('',#131004,#85156,#85157);
#74643=AXIS2_PLACEMENT_3D('',#131042,#85158,#85159);
#74644=AXIS2_PLACEMENT_3D('',#131080,#85160,#85161);
#74645=AXIS2_PLACEMENT_3D('',#131118,#85162,#85163);
#74646=AXIS2_PLACEMENT_3D('',#131156,#85164,#85165);
#74647=AXIS2_PLACEMENT_3D('',#131194,#85166,#85167);
#74648=AXIS2_PLACEMENT_3D('',#131232,#85168,#85169);
#74649=AXIS2_PLACEMENT_3D('',#131270,#85170,#85171);
#74650=AXIS2_PLACEMENT_3D('',#131308,#85172,#85173);
#74651=AXIS2_PLACEMENT_3D('',#131346,#85174,#85175);
#74652=AXIS2_PLACEMENT_3D('',#131384,#85176,#85177);
#74653=AXIS2_PLACEMENT_3D('',#131422,#85178,#85179);
#74654=AXIS2_PLACEMENT_3D('',#131460,#85180,#85181);
#74655=AXIS2_PLACEMENT_3D('',#131498,#85182,#85183);
#74656=AXIS2_PLACEMENT_3D('',#131536,#85184,#85185);
#74657=AXIS2_PLACEMENT_3D('',#131574,#85186,#85187);
#74658=AXIS2_PLACEMENT_3D('',#131612,#85188,#85189);
#74659=AXIS2_PLACEMENT_3D('',#131650,#85190,#85191);
#74660=AXIS2_PLACEMENT_3D('',#131688,#85192,#85193);
#74661=AXIS2_PLACEMENT_3D('',#131726,#85194,#85195);
#74662=AXIS2_PLACEMENT_3D('',#131764,#85196,#85197);
#74663=AXIS2_PLACEMENT_3D('',#131802,#85198,#85199);
#74664=AXIS2_PLACEMENT_3D('',#131836,#85200,#85201);
#74665=AXIS2_PLACEMENT_3D('',#131848,#85202,#85203);
#74666=AXIS2_PLACEMENT_3D('',#131864,#85204,#85205);
#74667=AXIS2_PLACEMENT_3D('',#131876,#85206,#85207);
#74668=AXIS2_PLACEMENT_3D('',#131892,#85208,#85209);
#74669=AXIS2_PLACEMENT_3D('',#131904,#85210,#85211);
#74670=AXIS2_PLACEMENT_3D('',#131920,#85212,#85213);
#74671=AXIS2_PLACEMENT_3D('',#131932,#85214,#85215);
#74672=AXIS2_PLACEMENT_3D('',#131948,#85216,#85217);
#74673=AXIS2_PLACEMENT_3D('',#131960,#85218,#85219);
#74674=AXIS2_PLACEMENT_3D('',#131976,#85220,#85221);
#74675=AXIS2_PLACEMENT_3D('',#131988,#85222,#85223);
#74676=AXIS2_PLACEMENT_3D('',#132004,#85224,#85225);
#74677=AXIS2_PLACEMENT_3D('',#132016,#85226,#85227);
#74678=AXIS2_PLACEMENT_3D('',#132032,#85228,#85229);
#74679=AXIS2_PLACEMENT_3D('',#132044,#85230,#85231);
#74680=AXIS2_PLACEMENT_3D('',#132060,#85232,#85233);
#74681=AXIS2_PLACEMENT_3D('',#132072,#85234,#85235);
#74682=AXIS2_PLACEMENT_3D('',#132088,#85236,#85237);
#74683=AXIS2_PLACEMENT_3D('',#132100,#85238,#85239);
#74684=AXIS2_PLACEMENT_3D('',#132116,#85240,#85241);
#74685=AXIS2_PLACEMENT_3D('',#132128,#85242,#85243);
#74686=AXIS2_PLACEMENT_3D('',#132144,#85244,#85245);
#74687=AXIS2_PLACEMENT_3D('',#132156,#85246,#85247);
#74688=AXIS2_PLACEMENT_3D('',#132172,#85248,#85249);
#74689=AXIS2_PLACEMENT_3D('',#132184,#85250,#85251);
#74690=AXIS2_PLACEMENT_3D('',#132200,#85252,#85253);
#74691=AXIS2_PLACEMENT_3D('',#132212,#85254,#85255);
#74692=AXIS2_PLACEMENT_3D('',#132228,#85256,#85257);
#74693=AXIS2_PLACEMENT_3D('',#132240,#85258,#85259);
#74694=AXIS2_PLACEMENT_3D('',#132256,#85260,#85261);
#74695=AXIS2_PLACEMENT_3D('',#132268,#85262,#85263);
#74696=AXIS2_PLACEMENT_3D('',#132284,#85264,#85265);
#74697=AXIS2_PLACEMENT_3D('',#132296,#85266,#85267);
#74698=AXIS2_PLACEMENT_3D('',#132312,#85268,#85269);
#74699=AXIS2_PLACEMENT_3D('',#132324,#85270,#85271);
#74700=AXIS2_PLACEMENT_3D('',#132340,#85272,#85273);
#74701=AXIS2_PLACEMENT_3D('',#132352,#85274,#85275);
#74702=AXIS2_PLACEMENT_3D('',#132368,#85276,#85277);
#74703=AXIS2_PLACEMENT_3D('',#132380,#85278,#85279);
#74704=AXIS2_PLACEMENT_3D('',#132396,#85280,#85281);
#74705=AXIS2_PLACEMENT_3D('',#132408,#85282,#85283);
#74706=AXIS2_PLACEMENT_3D('',#132424,#85284,#85285);
#74707=AXIS2_PLACEMENT_3D('',#132436,#85286,#85287);
#74708=AXIS2_PLACEMENT_3D('',#132452,#85288,#85289);
#74709=AXIS2_PLACEMENT_3D('',#132464,#85290,#85291);
#74710=AXIS2_PLACEMENT_3D('',#132480,#85292,#85293);
#74711=AXIS2_PLACEMENT_3D('',#132492,#85294,#85295);
#74712=AXIS2_PLACEMENT_3D('',#132508,#85296,#85297);
#74713=AXIS2_PLACEMENT_3D('',#132520,#85298,#85299);
#74714=AXIS2_PLACEMENT_3D('',#132536,#85300,#85301);
#74715=AXIS2_PLACEMENT_3D('',#132548,#85302,#85303);
#74716=AXIS2_PLACEMENT_3D('',#132564,#85304,#85305);
#74717=AXIS2_PLACEMENT_3D('',#132576,#85306,#85307);
#74718=AXIS2_PLACEMENT_3D('',#132592,#85308,#85309);
#74719=AXIS2_PLACEMENT_3D('',#132604,#85310,#85311);
#74720=AXIS2_PLACEMENT_3D('',#132620,#85312,#85313);
#74721=AXIS2_PLACEMENT_3D('',#132636,#85314,#85315);
#74722=AXIS2_PLACEMENT_3D('',#132645,#85316,#85317);
#74723=AXIS2_PLACEMENT_3D('',#132653,#85319,#85320);
#74724=AXIS2_PLACEMENT_3D('',#132655,#85321,#85322);
#74725=AXIS2_PLACEMENT_3D('',#132657,#85323,#85324);
#74726=AXIS2_PLACEMENT_3D('',#132684,#85326,#85327);
#74727=AXIS2_PLACEMENT_3D('',#132692,#85329,#85330);
#74728=AXIS2_PLACEMENT_3D('',#132694,#85331,#85332);
#74729=AXIS2_PLACEMENT_3D('',#132696,#85333,#85334);
#74730=AXIS2_PLACEMENT_3D('',#132723,#85336,#85337);
#74731=AXIS2_PLACEMENT_3D('',#132731,#85339,#85340);
#74732=AXIS2_PLACEMENT_3D('',#132733,#85341,#85342);
#74733=AXIS2_PLACEMENT_3D('',#132735,#85343,#85344);
#74734=AXIS2_PLACEMENT_3D('',#132762,#85346,#85347);
#74735=AXIS2_PLACEMENT_3D('',#132770,#85349,#85350);
#74736=AXIS2_PLACEMENT_3D('',#132772,#85351,#85352);
#74737=AXIS2_PLACEMENT_3D('',#132774,#85353,#85354);
#74738=AXIS2_PLACEMENT_3D('',#132801,#85356,#85357);
#74739=AXIS2_PLACEMENT_3D('',#132809,#85359,#85360);
#74740=AXIS2_PLACEMENT_3D('',#132811,#85361,#85362);
#74741=AXIS2_PLACEMENT_3D('',#132813,#85363,#85364);
#74742=AXIS2_PLACEMENT_3D('',#132840,#85366,#85367);
#74743=AXIS2_PLACEMENT_3D('',#132848,#85369,#85370);
#74744=AXIS2_PLACEMENT_3D('',#132850,#85371,#85372);
#74745=AXIS2_PLACEMENT_3D('',#132852,#85373,#85374);
#74746=AXIS2_PLACEMENT_3D('',#132879,#85376,#85377);
#74747=AXIS2_PLACEMENT_3D('',#132887,#85379,#85380);
#74748=AXIS2_PLACEMENT_3D('',#132889,#85381,#85382);
#74749=AXIS2_PLACEMENT_3D('',#132891,#85383,#85384);
#74750=AXIS2_PLACEMENT_3D('',#132918,#85386,#85387);
#74751=AXIS2_PLACEMENT_3D('',#132926,#85389,#85390);
#74752=AXIS2_PLACEMENT_3D('',#132928,#85391,#85392);
#74753=AXIS2_PLACEMENT_3D('',#132930,#85393,#85394);
#74754=AXIS2_PLACEMENT_3D('',#132957,#85396,#85397);
#74755=AXIS2_PLACEMENT_3D('',#132965,#85399,#85400);
#74756=AXIS2_PLACEMENT_3D('',#132967,#85401,#85402);
#74757=AXIS2_PLACEMENT_3D('',#132969,#85403,#85404);
#74758=AXIS2_PLACEMENT_3D('',#132994,#85406,#85407);
#74759=AXIS2_PLACEMENT_3D('',#133002,#85409,#85410);
#74760=AXIS2_PLACEMENT_3D('',#133004,#85411,#85412);
#74761=AXIS2_PLACEMENT_3D('',#133006,#85413,#85414);
#74762=AXIS2_PLACEMENT_3D('',#133033,#85416,#85417);
#74763=AXIS2_PLACEMENT_3D('',#133041,#85419,#85420);
#74764=AXIS2_PLACEMENT_3D('',#133043,#85421,#85422);
#74765=AXIS2_PLACEMENT_3D('',#133045,#85423,#85424);
#74766=AXIS2_PLACEMENT_3D('',#133072,#85426,#85427);
#74767=AXIS2_PLACEMENT_3D('',#133080,#85429,#85430);
#74768=AXIS2_PLACEMENT_3D('',#133082,#85431,#85432);
#74769=AXIS2_PLACEMENT_3D('',#133084,#85433,#85434);
#74770=AXIS2_PLACEMENT_3D('',#133111,#85436,#85437);
#74771=AXIS2_PLACEMENT_3D('',#133119,#85439,#85440);
#74772=AXIS2_PLACEMENT_3D('',#133121,#85441,#85442);
#74773=AXIS2_PLACEMENT_3D('',#133123,#85443,#85444);
#74774=AXIS2_PLACEMENT_3D('',#133150,#85446,#85447);
#74775=AXIS2_PLACEMENT_3D('',#133158,#85449,#85450);
#74776=AXIS2_PLACEMENT_3D('',#133160,#85451,#85452);
#74777=AXIS2_PLACEMENT_3D('',#133162,#85453,#85454);
#74778=AXIS2_PLACEMENT_3D('',#133213,#85458,#85459);
#74779=AXIS2_PLACEMENT_3D('',#133221,#85461,#85462);
#74780=AXIS2_PLACEMENT_3D('',#133223,#85463,#85464);
#74781=AXIS2_PLACEMENT_3D('',#133225,#85465,#85466);
#74782=AXIS2_PLACEMENT_3D('',#133252,#85468,#85469);
#74783=AXIS2_PLACEMENT_3D('',#133260,#85471,#85472);
#74784=AXIS2_PLACEMENT_3D('',#133262,#85473,#85474);
#74785=AXIS2_PLACEMENT_3D('',#133264,#85475,#85476);
#74786=AXIS2_PLACEMENT_3D('',#133291,#85478,#85479);
#74787=AXIS2_PLACEMENT_3D('',#133299,#85481,#85482);
#74788=AXIS2_PLACEMENT_3D('',#133301,#85483,#85484);
#74789=AXIS2_PLACEMENT_3D('',#133303,#85485,#85486);
#74790=AXIS2_PLACEMENT_3D('',#133330,#85488,#85489);
#74791=AXIS2_PLACEMENT_3D('',#133338,#85491,#85492);
#74792=AXIS2_PLACEMENT_3D('',#133340,#85493,#85494);
#74793=AXIS2_PLACEMENT_3D('',#133342,#85495,#85496);
#74794=AXIS2_PLACEMENT_3D('',#133369,#85498,#85499);
#74795=AXIS2_PLACEMENT_3D('',#133377,#85501,#85502);
#74796=AXIS2_PLACEMENT_3D('',#133379,#85503,#85504);
#74797=AXIS2_PLACEMENT_3D('',#133381,#85505,#85506);
#74798=AXIS2_PLACEMENT_3D('',#133408,#85508,#85509);
#74799=AXIS2_PLACEMENT_3D('',#133435,#85512,#85513);
#74800=AXIS2_PLACEMENT_3D('',#133437,#85514,#85515);
#74801=AXIS2_PLACEMENT_3D('',#133438,#85516,#85517);
#74802=AXIS2_PLACEMENT_3D('',#133448,#85519,#85520);
#74803=AXIS2_PLACEMENT_3D('',#133455,#85521,#85522);
#74804=AXIS2_PLACEMENT_3D('',#133465,#85523,#85524);
#74805=AXIS2_PLACEMENT_3D('',#133466,#85525,#85526);
#74806=AXIS2_PLACEMENT_3D('',#133486,#85528,#85529);
#74807=AXIS2_PLACEMENT_3D('',#133494,#85531,#85532);
#74808=AXIS2_PLACEMENT_3D('',#133496,#85533,#85534);
#74809=AXIS2_PLACEMENT_3D('',#133498,#85535,#85536);
#74810=AXIS2_PLACEMENT_3D('',#133525,#85538,#85539);
#74811=AXIS2_PLACEMENT_3D('',#133533,#85541,#85542);
#74812=AXIS2_PLACEMENT_3D('',#133535,#85543,#85544);
#74813=AXIS2_PLACEMENT_3D('',#133537,#85545,#85546);
#74814=AXIS2_PLACEMENT_3D('',#133564,#85548,#85549);
#74815=AXIS2_PLACEMENT_3D('',#133572,#85551,#85552);
#74816=AXIS2_PLACEMENT_3D('',#133574,#85553,#85554);
#74817=AXIS2_PLACEMENT_3D('',#133576,#85555,#85556);
#74818=AXIS2_PLACEMENT_3D('',#133603,#85558,#85559);
#74819=AXIS2_PLACEMENT_3D('',#133611,#85561,#85562);
#74820=AXIS2_PLACEMENT_3D('',#133613,#85563,#85564);
#74821=AXIS2_PLACEMENT_3D('',#133615,#85565,#85566);
#74822=AXIS2_PLACEMENT_3D('',#133642,#85568,#85569);
#74823=AXIS2_PLACEMENT_3D('',#133650,#85571,#85572);
#74824=AXIS2_PLACEMENT_3D('',#133652,#85573,#85574);
#74825=AXIS2_PLACEMENT_3D('',#133654,#85575,#85576);
#74826=AXIS2_PLACEMENT_3D('',#133681,#85578,#85579);
#74827=AXIS2_PLACEMENT_3D('',#133689,#85581,#85582);
#74828=AXIS2_PLACEMENT_3D('',#133691,#85583,#85584);
#74829=AXIS2_PLACEMENT_3D('',#133693,#85585,#85586);
#74830=AXIS2_PLACEMENT_3D('',#133720,#85588,#85589);
#74831=AXIS2_PLACEMENT_3D('',#133728,#85591,#85592);
#74832=AXIS2_PLACEMENT_3D('',#133730,#85593,#85594);
#74833=AXIS2_PLACEMENT_3D('',#133732,#85595,#85596);
#74834=AXIS2_PLACEMENT_3D('',#133760,#85599,#85600);
#74835=AXIS2_PLACEMENT_3D('',#133774,#85601,#85602);
#74836=AXIS2_PLACEMENT_3D('',#133776,#85604,#85605);
#74837=AXIS2_PLACEMENT_3D('',#133778,#85606,#85607);
#74838=AXIS2_PLACEMENT_3D('',#133779,#85608,#85609);
#74839=AXIS2_PLACEMENT_3D('',#133789,#85611,#85612);
#74840=AXIS2_PLACEMENT_3D('',#133803,#85613,#85614);
#74841=AXIS2_PLACEMENT_3D('',#133805,#85616,#85617);
#74842=AXIS2_PLACEMENT_3D('',#133807,#85618,#85619);
#74843=AXIS2_PLACEMENT_3D('',#133808,#85620,#85621);
#74844=AXIS2_PLACEMENT_3D('',#133818,#85623,#85624);
#74845=AXIS2_PLACEMENT_3D('',#133832,#85625,#85626);
#74846=AXIS2_PLACEMENT_3D('',#133834,#85628,#85629);
#74847=AXIS2_PLACEMENT_3D('',#133836,#85630,#85631);
#74848=AXIS2_PLACEMENT_3D('',#133837,#85632,#85633);
#74849=AXIS2_PLACEMENT_3D('',#133847,#85635,#85636);
#74850=AXIS2_PLACEMENT_3D('',#133861,#85637,#85638);
#74851=AXIS2_PLACEMENT_3D('',#133863,#85640,#85641);
#74852=AXIS2_PLACEMENT_3D('',#133865,#85642,#85643);
#74853=AXIS2_PLACEMENT_3D('',#133866,#85644,#85645);
#74854=AXIS2_PLACEMENT_3D('',#133876,#85647,#85648);
#74855=AXIS2_PLACEMENT_3D('',#133890,#85649,#85650);
#74856=AXIS2_PLACEMENT_3D('',#133892,#85652,#85653);
#74857=AXIS2_PLACEMENT_3D('',#133894,#85654,#85655);
#74858=AXIS2_PLACEMENT_3D('',#133895,#85656,#85657);
#74859=AXIS2_PLACEMENT_3D('',#133905,#85659,#85660);
#74860=AXIS2_PLACEMENT_3D('',#133919,#85661,#85662);
#74861=AXIS2_PLACEMENT_3D('',#133921,#85664,#85665);
#74862=AXIS2_PLACEMENT_3D('',#133923,#85666,#85667);
#74863=AXIS2_PLACEMENT_3D('',#133924,#85668,#85669);
#74864=AXIS2_PLACEMENT_3D('',#133934,#85671,#85672);
#74865=AXIS2_PLACEMENT_3D('',#133948,#85673,#85674);
#74866=AXIS2_PLACEMENT_3D('',#133950,#85676,#85677);
#74867=AXIS2_PLACEMENT_3D('',#133952,#85678,#85679);
#74868=AXIS2_PLACEMENT_3D('',#133953,#85680,#85681);
#74869=AXIS2_PLACEMENT_3D('',#133963,#85683,#85684);
#74870=AXIS2_PLACEMENT_3D('',#133977,#85685,#85686);
#74871=AXIS2_PLACEMENT_3D('',#133979,#85688,#85689);
#74872=AXIS2_PLACEMENT_3D('',#133981,#85690,#85691);
#74873=AXIS2_PLACEMENT_3D('',#133982,#85692,#85693);
#74874=AXIS2_PLACEMENT_3D('',#133992,#85695,#85696);
#74875=AXIS2_PLACEMENT_3D('',#134006,#85697,#85698);
#74876=AXIS2_PLACEMENT_3D('',#134008,#85700,#85701);
#74877=AXIS2_PLACEMENT_3D('',#134010,#85702,#85703);
#74878=AXIS2_PLACEMENT_3D('',#134011,#85704,#85705);
#74879=AXIS2_PLACEMENT_3D('',#134021,#85707,#85708);
#74880=AXIS2_PLACEMENT_3D('',#134035,#85709,#85710);
#74881=AXIS2_PLACEMENT_3D('',#134037,#85712,#85713);
#74882=AXIS2_PLACEMENT_3D('',#134039,#85714,#85715);
#74883=AXIS2_PLACEMENT_3D('',#134040,#85716,#85717);
#74884=AXIS2_PLACEMENT_3D('',#134050,#85719,#85720);
#74885=AXIS2_PLACEMENT_3D('',#134064,#85721,#85722);
#74886=AXIS2_PLACEMENT_3D('',#134066,#85724,#85725);
#74887=AXIS2_PLACEMENT_3D('',#134068,#85726,#85727);
#74888=AXIS2_PLACEMENT_3D('',#134069,#85728,#85729);
#74889=AXIS2_PLACEMENT_3D('',#134079,#85731,#85732);
#74890=AXIS2_PLACEMENT_3D('',#134093,#85733,#85734);
#74891=AXIS2_PLACEMENT_3D('',#134095,#85736,#85737);
#74892=AXIS2_PLACEMENT_3D('',#134097,#85738,#85739);
#74893=AXIS2_PLACEMENT_3D('',#134098,#85740,#85741);
#74894=AXIS2_PLACEMENT_3D('',#134108,#85743,#85744);
#74895=AXIS2_PLACEMENT_3D('',#134122,#85745,#85746);
#74896=AXIS2_PLACEMENT_3D('',#134124,#85748,#85749);
#74897=AXIS2_PLACEMENT_3D('',#134126,#85750,#85751);
#74898=AXIS2_PLACEMENT_3D('',#134127,#85752,#85753);
#74899=AXIS2_PLACEMENT_3D('',#134137,#85755,#85756);
#74900=AXIS2_PLACEMENT_3D('',#134151,#85757,#85758);
#74901=AXIS2_PLACEMENT_3D('',#134153,#85760,#85761);
#74902=AXIS2_PLACEMENT_3D('',#134155,#85762,#85763);
#74903=AXIS2_PLACEMENT_3D('',#134156,#85764,#85765);
#74904=AXIS2_PLACEMENT_3D('',#134166,#85767,#85768);
#74905=AXIS2_PLACEMENT_3D('',#134180,#85769,#85770);
#74906=AXIS2_PLACEMENT_3D('',#134182,#85772,#85773);
#74907=AXIS2_PLACEMENT_3D('',#134184,#85774,#85775);
#74908=AXIS2_PLACEMENT_3D('',#134185,#85776,#85777);
#74909=AXIS2_PLACEMENT_3D('',#134195,#85779,#85780);
#74910=AXIS2_PLACEMENT_3D('',#134209,#85781,#85782);
#74911=AXIS2_PLACEMENT_3D('',#134211,#85784,#85785);
#74912=AXIS2_PLACEMENT_3D('',#134213,#85786,#85787);
#74913=AXIS2_PLACEMENT_3D('',#134214,#85788,#85789);
#74914=AXIS2_PLACEMENT_3D('',#134224,#85791,#85792);
#74915=AXIS2_PLACEMENT_3D('',#134238,#85793,#85794);
#74916=AXIS2_PLACEMENT_3D('',#134240,#85796,#85797);
#74917=AXIS2_PLACEMENT_3D('',#134242,#85798,#85799);
#74918=AXIS2_PLACEMENT_3D('',#134243,#85800,#85801);
#74919=AXIS2_PLACEMENT_3D('',#134253,#85803,#85804);
#74920=AXIS2_PLACEMENT_3D('',#134267,#85805,#85806);
#74921=AXIS2_PLACEMENT_3D('',#134269,#85808,#85809);
#74922=AXIS2_PLACEMENT_3D('',#134271,#85810,#85811);
#74923=AXIS2_PLACEMENT_3D('',#134272,#85812,#85813);
#74924=AXIS2_PLACEMENT_3D('',#134282,#85815,#85816);
#74925=AXIS2_PLACEMENT_3D('',#134296,#85817,#85818);
#74926=AXIS2_PLACEMENT_3D('',#134298,#85820,#85821);
#74927=AXIS2_PLACEMENT_3D('',#134300,#85822,#85823);
#74928=AXIS2_PLACEMENT_3D('',#134301,#85824,#85825);
#74929=AXIS2_PLACEMENT_3D('',#134311,#85827,#85828);
#74930=AXIS2_PLACEMENT_3D('',#134325,#85829,#85830);
#74931=AXIS2_PLACEMENT_3D('',#134327,#85832,#85833);
#74932=AXIS2_PLACEMENT_3D('',#134329,#85834,#85835);
#74933=AXIS2_PLACEMENT_3D('',#134330,#85836,#85837);
#74934=AXIS2_PLACEMENT_3D('',#134340,#85839,#85840);
#74935=AXIS2_PLACEMENT_3D('',#134354,#85841,#85842);
#74936=AXIS2_PLACEMENT_3D('',#134356,#85844,#85845);
#74937=AXIS2_PLACEMENT_3D('',#134358,#85846,#85847);
#74938=AXIS2_PLACEMENT_3D('',#134359,#85848,#85849);
#74939=AXIS2_PLACEMENT_3D('',#134369,#85851,#85852);
#74940=AXIS2_PLACEMENT_3D('',#134383,#85853,#85854);
#74941=AXIS2_PLACEMENT_3D('',#134385,#85856,#85857);
#74942=AXIS2_PLACEMENT_3D('',#134387,#85858,#85859);
#74943=AXIS2_PLACEMENT_3D('',#134388,#85860,#85861);
#74944=AXIS2_PLACEMENT_3D('',#134398,#85863,#85864);
#74945=AXIS2_PLACEMENT_3D('',#134412,#85865,#85866);
#74946=AXIS2_PLACEMENT_3D('',#134414,#85868,#85869);
#74947=AXIS2_PLACEMENT_3D('',#134416,#85870,#85871);
#74948=AXIS2_PLACEMENT_3D('',#134417,#85872,#85873);
#74949=AXIS2_PLACEMENT_3D('',#134427,#85875,#85876);
#74950=AXIS2_PLACEMENT_3D('',#134441,#85877,#85878);
#74951=AXIS2_PLACEMENT_3D('',#134443,#85880,#85881);
#74952=AXIS2_PLACEMENT_3D('',#134445,#85882,#85883);
#74953=AXIS2_PLACEMENT_3D('',#134446,#85884,#85885);
#74954=AXIS2_PLACEMENT_3D('',#134456,#85887,#85888);
#74955=AXIS2_PLACEMENT_3D('',#134470,#85889,#85890);
#74956=AXIS2_PLACEMENT_3D('',#134472,#85892,#85893);
#74957=AXIS2_PLACEMENT_3D('',#134474,#85894,#85895);
#74958=AXIS2_PLACEMENT_3D('',#134475,#85896,#85897);
#74959=AXIS2_PLACEMENT_3D('',#134485,#85899,#85900);
#74960=AXIS2_PLACEMENT_3D('',#134499,#85901,#85902);
#74961=AXIS2_PLACEMENT_3D('',#134501,#85904,#85905);
#74962=AXIS2_PLACEMENT_3D('',#134503,#85906,#85907);
#74963=AXIS2_PLACEMENT_3D('',#134504,#85908,#85909);
#74964=AXIS2_PLACEMENT_3D('',#134514,#85911,#85912);
#74965=AXIS2_PLACEMENT_3D('',#134528,#85913,#85914);
#74966=AXIS2_PLACEMENT_3D('',#134530,#85916,#85917);
#74967=AXIS2_PLACEMENT_3D('',#134532,#85918,#85919);
#74968=AXIS2_PLACEMENT_3D('',#134533,#85920,#85921);
#74969=AXIS2_PLACEMENT_3D('',#134543,#85923,#85924);
#74970=AXIS2_PLACEMENT_3D('',#134557,#85925,#85926);
#74971=AXIS2_PLACEMENT_3D('',#134559,#85928,#85929);
#74972=AXIS2_PLACEMENT_3D('',#134561,#85930,#85931);
#74973=AXIS2_PLACEMENT_3D('',#134562,#85932,#85933);
#74974=AXIS2_PLACEMENT_3D('',#134572,#85935,#85936);
#74975=AXIS2_PLACEMENT_3D('',#134586,#85937,#85938);
#74976=AXIS2_PLACEMENT_3D('',#134588,#85940,#85941);
#74977=AXIS2_PLACEMENT_3D('',#134590,#85942,#85943);
#74978=AXIS2_PLACEMENT_3D('',#134591,#85944,#85945);
#74979=AXIS2_PLACEMENT_3D('',#134603,#85946,#85947);
#74980=AXIS2_PLACEMENT_3D('',#134649,#85948,#85949);
#74981=AXIS2_PLACEMENT_3D('',#134695,#85950,#85951);
#74982=AXIS2_PLACEMENT_3D('',#134741,#85952,#85953);
#74983=AXIS2_PLACEMENT_3D('',#134787,#85954,#85955);
#74984=AXIS2_PLACEMENT_3D('',#134833,#85956,#85957);
#74985=AXIS2_PLACEMENT_3D('',#134883,#85958,#85959);
#74986=AXIS2_PLACEMENT_3D('',#134929,#85960,#85961);
#74987=AXIS2_PLACEMENT_3D('',#134975,#85962,#85963);
#74988=AXIS2_PLACEMENT_3D('',#135021,#85964,#85965);
#74989=AXIS2_PLACEMENT_3D('',#135067,#85966,#85967);
#74990=AXIS2_PLACEMENT_3D('',#135113,#85968,#85969);
#74991=AXIS2_PLACEMENT_3D('',#135159,#85970,#85971);
#74992=AXIS2_PLACEMENT_3D('',#135209,#85972,#85973);
#74993=AXIS2_PLACEMENT_3D('',#135259,#85974,#85975);
#74994=AXIS2_PLACEMENT_3D('',#135309,#85976,#85977);
#74995=AXIS2_PLACEMENT_3D('',#135355,#85978,#85979);
#74996=AXIS2_PLACEMENT_3D('',#135401,#85980,#85981);
#74997=AXIS2_PLACEMENT_3D('',#135447,#85982,#85983);
#74998=AXIS2_PLACEMENT_3D('',#135493,#85984,#85985);
#74999=AXIS2_PLACEMENT_3D('',#135539,#85986,#85987);
#75000=AXIS2_PLACEMENT_3D('',#135585,#85988,#85989);
#75001=AXIS2_PLACEMENT_3D('',#135631,#85990,#85991);
#75002=AXIS2_PLACEMENT_3D('',#135677,#85992,#85993);
#75003=AXIS2_PLACEMENT_3D('',#135723,#85994,#85995);
#75004=AXIS2_PLACEMENT_3D('',#135769,#85996,#85997);
#75005=AXIS2_PLACEMENT_3D('',#135815,#85998,#85999);
#75006=AXIS2_PLACEMENT_3D('',#135861,#86000,#86001);
#75007=AXIS2_PLACEMENT_3D('',#135907,#86002,#86003);
#75008=AXIS2_PLACEMENT_3D('',#135957,#86004,#86005);
#75009=AXIS2_PLACEMENT_3D('',#136007,#86006,#86007);
#75010=AXIS2_PLACEMENT_3D('',#136053,#86008,#86009);
#75011=AXIS2_PLACEMENT_3D('',#136103,#86010,#86011);
#75012=AXIS2_PLACEMENT_3D('',#136152,#86012,#86013);
#75013=AXIS2_PLACEMENT_3D('',#136202,#86014,#86015);
#75014=AXIS2_PLACEMENT_3D('',#136248,#86016,#86017);
#75015=AXIS2_PLACEMENT_3D('',#136298,#86018,#86019);
#75016=AXIS2_PLACEMENT_3D('',#136344,#86020,#86021);
#75017=AXIS2_PLACEMENT_3D('',#136390,#86022,#86023);
#75018=AXIS2_PLACEMENT_3D('',#136440,#86024,#86025);
#75019=AXIS2_PLACEMENT_3D('',#136481,#86026,#86027);
#75020=AXIS2_PLACEMENT_3D('',#136522,#86028,#86029);
#75021=AXIS2_PLACEMENT_3D('',#136568,#86030,#86031);
#75022=AXIS2_PLACEMENT_3D('',#136618,#86032,#86033);
#75023=AXIS2_PLACEMENT_3D('',#136664,#86034,#86035);
#75024=AXIS2_PLACEMENT_3D('',#136708,#86036,#86037);
#75025=AXIS2_PLACEMENT_3D('',#136758,#86038,#86039);
#75026=AXIS2_PLACEMENT_3D('',#136799,#86040,#86041);
#75027=AXIS2_PLACEMENT_3D('',#136849,#86042,#86043);
#75028=AXIS2_PLACEMENT_3D('',#136898,#86044,#86045);
#75029=AXIS2_PLACEMENT_3D('',#136947,#86046,#86047);
#75030=AXIS2_PLACEMENT_3D('',#136997,#86048,#86049);
#75031=AXIS2_PLACEMENT_3D('',#137047,#86050,#86051);
#75032=AXIS2_PLACEMENT_3D('',#137088,#86052,#86053);
#75033=AXIS2_PLACEMENT_3D('',#137129,#86054,#86055);
#75034=AXIS2_PLACEMENT_3D('',#137179,#86056,#86057);
#75035=AXIS2_PLACEMENT_3D('',#137220,#86058,#86059);
#75036=AXIS2_PLACEMENT_3D('',#137266,#86060,#86061);
#75037=AXIS2_PLACEMENT_3D('',#137320,#86062,#86063);
#75038=AXIS2_PLACEMENT_3D('',#137354,#86066,#86067);
#75039=AXIS2_PLACEMENT_3D('',#137356,#86068,#86069);
#75040=AXIS2_PLACEMENT_3D('',#137358,#86070,#86071);
#75041=AXIS2_PLACEMENT_3D('',#137359,#86072,#86073);
#75042=AXIS2_PLACEMENT_3D('',#137397,#86076,#86077);
#75043=AXIS2_PLACEMENT_3D('',#137399,#86078,#86079);
#75044=AXIS2_PLACEMENT_3D('',#137401,#86080,#86081);
#75045=AXIS2_PLACEMENT_3D('',#137402,#86082,#86083);
#75046=AXIS2_PLACEMENT_3D('',#137440,#86086,#86087);
#75047=AXIS2_PLACEMENT_3D('',#137442,#86088,#86089);
#75048=AXIS2_PLACEMENT_3D('',#137444,#86090,#86091);
#75049=AXIS2_PLACEMENT_3D('',#137445,#86092,#86093);
#75050=AXIS2_PLACEMENT_3D('',#137483,#86096,#86097);
#75051=AXIS2_PLACEMENT_3D('',#137485,#86098,#86099);
#75052=AXIS2_PLACEMENT_3D('',#137487,#86100,#86101);
#75053=AXIS2_PLACEMENT_3D('',#137488,#86102,#86103);
#75054=AXIS2_PLACEMENT_3D('',#137526,#86106,#86107);
#75055=AXIS2_PLACEMENT_3D('',#137528,#86108,#86109);
#75056=AXIS2_PLACEMENT_3D('',#137530,#86110,#86111);
#75057=AXIS2_PLACEMENT_3D('',#137531,#86112,#86113);
#75058=AXIS2_PLACEMENT_3D('',#137569,#86116,#86117);
#75059=AXIS2_PLACEMENT_3D('',#137571,#86118,#86119);
#75060=AXIS2_PLACEMENT_3D('',#137573,#86120,#86121);
#75061=AXIS2_PLACEMENT_3D('',#137574,#86122,#86123);
#75062=AXIS2_PLACEMENT_3D('',#137640,#86128,#86129);
#75063=AXIS2_PLACEMENT_3D('',#137642,#86130,#86131);
#75064=AXIS2_PLACEMENT_3D('',#137644,#86132,#86133);
#75065=AXIS2_PLACEMENT_3D('',#137645,#86134,#86135);
#75066=AXIS2_PLACEMENT_3D('',#137683,#86138,#86139);
#75067=AXIS2_PLACEMENT_3D('',#137685,#86140,#86141);
#75068=AXIS2_PLACEMENT_3D('',#137687,#86142,#86143);
#75069=AXIS2_PLACEMENT_3D('',#137688,#86144,#86145);
#75070=AXIS2_PLACEMENT_3D('',#137726,#86148,#86149);
#75071=AXIS2_PLACEMENT_3D('',#137728,#86150,#86151);
#75072=AXIS2_PLACEMENT_3D('',#137730,#86152,#86153);
#75073=AXIS2_PLACEMENT_3D('',#137731,#86154,#86155);
#75074=AXIS2_PLACEMENT_3D('',#137769,#86158,#86159);
#75075=AXIS2_PLACEMENT_3D('',#137771,#86160,#86161);
#75076=AXIS2_PLACEMENT_3D('',#137773,#86162,#86163);
#75077=AXIS2_PLACEMENT_3D('',#137774,#86164,#86165);
#75078=AXIS2_PLACEMENT_3D('',#137812,#86168,#86169);
#75079=AXIS2_PLACEMENT_3D('',#137814,#86170,#86171);
#75080=AXIS2_PLACEMENT_3D('',#137816,#86172,#86173);
#75081=AXIS2_PLACEMENT_3D('',#137817,#86174,#86175);
#75082=AXIS2_PLACEMENT_3D('',#137855,#86178,#86179);
#75083=AXIS2_PLACEMENT_3D('',#137857,#86180,#86181);
#75084=AXIS2_PLACEMENT_3D('',#137859,#86182,#86183);
#75085=AXIS2_PLACEMENT_3D('',#137860,#86184,#86185);
#75086=AXIS2_PLACEMENT_3D('',#137898,#86188,#86189);
#75087=AXIS2_PLACEMENT_3D('',#137900,#86190,#86191);
#75088=AXIS2_PLACEMENT_3D('',#137902,#86192,#86193);
#75089=AXIS2_PLACEMENT_3D('',#137903,#86194,#86195);
#75090=AXIS2_PLACEMENT_3D('',#137941,#86198,#86199);
#75091=AXIS2_PLACEMENT_3D('',#137943,#86200,#86201);
#75092=AXIS2_PLACEMENT_3D('',#137945,#86202,#86203);
#75093=AXIS2_PLACEMENT_3D('',#137946,#86204,#86205);
#75094=AXIS2_PLACEMENT_3D('',#137984,#86208,#86209);
#75095=AXIS2_PLACEMENT_3D('',#137986,#86210,#86211);
#75096=AXIS2_PLACEMENT_3D('',#137988,#86212,#86213);
#75097=AXIS2_PLACEMENT_3D('',#137989,#86214,#86215);
#75098=AXIS2_PLACEMENT_3D('',#138027,#86218,#86219);
#75099=AXIS2_PLACEMENT_3D('',#138029,#86220,#86221);
#75100=AXIS2_PLACEMENT_3D('',#138031,#86222,#86223);
#75101=AXIS2_PLACEMENT_3D('',#138032,#86224,#86225);
#75102=AXIS2_PLACEMENT_3D('',#138070,#86228,#86229);
#75103=AXIS2_PLACEMENT_3D('',#138072,#86230,#86231);
#75104=AXIS2_PLACEMENT_3D('',#138074,#86232,#86233);
#75105=AXIS2_PLACEMENT_3D('',#138075,#86234,#86235);
#75106=AXIS2_PLACEMENT_3D('',#138113,#86238,#86239);
#75107=AXIS2_PLACEMENT_3D('',#138115,#86240,#86241);
#75108=AXIS2_PLACEMENT_3D('',#138117,#86242,#86243);
#75109=AXIS2_PLACEMENT_3D('',#138118,#86244,#86245);
#75110=AXIS2_PLACEMENT_3D('',#138167,#86248,#86249);
#75111=AXIS2_PLACEMENT_3D('',#138169,#86251,#86252);
#75112=AXIS2_PLACEMENT_3D('',#138171,#86253,#86254);
#75113=AXIS2_PLACEMENT_3D('',#138172,#86255,#86256);
#75114=AXIS2_PLACEMENT_3D('',#138199,#86258,#86259);
#75115=AXIS2_PLACEMENT_3D('',#138201,#86260,#86261);
#75116=AXIS2_PLACEMENT_3D('',#138203,#86262,#86263);
#75117=AXIS2_PLACEMENT_3D('',#138204,#86264,#86265);
#75118=AXIS2_PLACEMENT_3D('',#138242,#86268,#86269);
#75119=AXIS2_PLACEMENT_3D('',#138244,#86270,#86271);
#75120=AXIS2_PLACEMENT_3D('',#138246,#86272,#86273);
#75121=AXIS2_PLACEMENT_3D('',#138247,#86274,#86275);
#75122=AXIS2_PLACEMENT_3D('',#138285,#86278,#86279);
#75123=AXIS2_PLACEMENT_3D('',#138287,#86280,#86281);
#75124=AXIS2_PLACEMENT_3D('',#138289,#86282,#86283);
#75125=AXIS2_PLACEMENT_3D('',#138290,#86284,#86285);
#75126=AXIS2_PLACEMENT_3D('',#138328,#86288,#86289);
#75127=AXIS2_PLACEMENT_3D('',#138330,#86290,#86291);
#75128=AXIS2_PLACEMENT_3D('',#138332,#86292,#86293);
#75129=AXIS2_PLACEMENT_3D('',#138333,#86294,#86295);
#75130=AXIS2_PLACEMENT_3D('',#138371,#86298,#86299);
#75131=AXIS2_PLACEMENT_3D('',#138373,#86300,#86301);
#75132=AXIS2_PLACEMENT_3D('',#138375,#86302,#86303);
#75133=AXIS2_PLACEMENT_3D('',#138376,#86304,#86305);
#75134=AXIS2_PLACEMENT_3D('',#138414,#86308,#86309);
#75135=AXIS2_PLACEMENT_3D('',#138416,#86310,#86311);
#75136=AXIS2_PLACEMENT_3D('',#138418,#86312,#86313);
#75137=AXIS2_PLACEMENT_3D('',#138419,#86314,#86315);
#75138=AXIS2_PLACEMENT_3D('',#138457,#86318,#86319);
#75139=AXIS2_PLACEMENT_3D('',#138459,#86320,#86321);
#75140=AXIS2_PLACEMENT_3D('',#138461,#86322,#86323);
#75141=AXIS2_PLACEMENT_3D('',#138462,#86324,#86325);
#75142=AXIS2_PLACEMENT_3D('',#138500,#86328,#86329);
#75143=AXIS2_PLACEMENT_3D('',#138502,#86330,#86331);
#75144=AXIS2_PLACEMENT_3D('',#138504,#86332,#86333);
#75145=AXIS2_PLACEMENT_3D('',#138505,#86334,#86335);
#75146=AXIS2_PLACEMENT_3D('',#138517,#86337,#86338);
#75147=AXIS2_PLACEMENT_3D('',#138520,#86339,#86340);
#75148=AXIS2_PLACEMENT_3D('',#138521,#86341,#86342);
#75149=AXIS2_PLACEMENT_3D('',#138558,#86344,#86345);
#75150=AXIS2_PLACEMENT_3D('',#138597,#86348,#86349);
#75151=AXIS2_PLACEMENT_3D('',#138599,#86351,#86352);
#75152=AXIS2_PLACEMENT_3D('',#138601,#86353,#86354);
#75153=AXIS2_PLACEMENT_3D('',#138602,#86355,#86356);
#75154=AXIS2_PLACEMENT_3D('',#138640,#86358,#86359);
#75155=AXIS2_PLACEMENT_3D('',#138642,#86361,#86362);
#75156=AXIS2_PLACEMENT_3D('',#138644,#86363,#86364);
#75157=AXIS2_PLACEMENT_3D('',#138645,#86365,#86366);
#75158=AXIS2_PLACEMENT_3D('',#138683,#86368,#86369);
#75159=AXIS2_PLACEMENT_3D('',#138685,#86371,#86372);
#75160=AXIS2_PLACEMENT_3D('',#138687,#86373,#86374);
#75161=AXIS2_PLACEMENT_3D('',#138688,#86375,#86376);
#75162=AXIS2_PLACEMENT_3D('',#138726,#86378,#86379);
#75163=AXIS2_PLACEMENT_3D('',#138728,#86381,#86382);
#75164=AXIS2_PLACEMENT_3D('',#138730,#86383,#86384);
#75165=AXIS2_PLACEMENT_3D('',#138731,#86385,#86386);
#75166=AXIS2_PLACEMENT_3D('',#138769,#86388,#86389);
#75167=AXIS2_PLACEMENT_3D('',#138771,#86391,#86392);
#75168=AXIS2_PLACEMENT_3D('',#138773,#86393,#86394);
#75169=AXIS2_PLACEMENT_3D('',#138774,#86395,#86396);
#75170=AXIS2_PLACEMENT_3D('',#138812,#86398,#86399);
#75171=AXIS2_PLACEMENT_3D('',#138814,#86401,#86402);
#75172=AXIS2_PLACEMENT_3D('',#138816,#86403,#86404);
#75173=AXIS2_PLACEMENT_3D('',#138817,#86405,#86406);
#75174=AXIS2_PLACEMENT_3D('',#138855,#86408,#86409);
#75175=AXIS2_PLACEMENT_3D('',#138857,#86411,#86412);
#75176=AXIS2_PLACEMENT_3D('',#138859,#86413,#86414);
#75177=AXIS2_PLACEMENT_3D('',#138860,#86415,#86416);
#75178=AXIS2_PLACEMENT_3D('',#138898,#86418,#86419);
#75179=AXIS2_PLACEMENT_3D('',#138900,#86421,#86422);
#75180=AXIS2_PLACEMENT_3D('',#138902,#86423,#86424);
#75181=AXIS2_PLACEMENT_3D('',#138903,#86425,#86426);
#75182=AXIS2_PLACEMENT_3D('',#138941,#86428,#86429);
#75183=AXIS2_PLACEMENT_3D('',#138943,#86431,#86432);
#75184=AXIS2_PLACEMENT_3D('',#138945,#86433,#86434);
#75185=AXIS2_PLACEMENT_3D('',#138946,#86435,#86436);
#75186=AXIS2_PLACEMENT_3D('',#138984,#86438,#86439);
#75187=AXIS2_PLACEMENT_3D('',#138986,#86441,#86442);
#75188=AXIS2_PLACEMENT_3D('',#138988,#86443,#86444);
#75189=AXIS2_PLACEMENT_3D('',#138989,#86445,#86446);
#75190=AXIS2_PLACEMENT_3D('',#139027,#86448,#86449);
#75191=AXIS2_PLACEMENT_3D('',#139029,#86451,#86452);
#75192=AXIS2_PLACEMENT_3D('',#139031,#86453,#86454);
#75193=AXIS2_PLACEMENT_3D('',#139032,#86455,#86456);
#75194=AXIS2_PLACEMENT_3D('',#139070,#86458,#86459);
#75195=AXIS2_PLACEMENT_3D('',#139072,#86461,#86462);
#75196=AXIS2_PLACEMENT_3D('',#139074,#86463,#86464);
#75197=AXIS2_PLACEMENT_3D('',#139075,#86465,#86466);
#75198=AXIS2_PLACEMENT_3D('',#139113,#86468,#86469);
#75199=AXIS2_PLACEMENT_3D('',#139115,#86471,#86472);
#75200=AXIS2_PLACEMENT_3D('',#139117,#86473,#86474);
#75201=AXIS2_PLACEMENT_3D('',#139118,#86475,#86476);
#75202=AXIS2_PLACEMENT_3D('',#139184,#86480,#86481);
#75203=AXIS2_PLACEMENT_3D('',#139186,#86483,#86484);
#75204=AXIS2_PLACEMENT_3D('',#139188,#86485,#86486);
#75205=AXIS2_PLACEMENT_3D('',#139189,#86487,#86488);
#75206=AXIS2_PLACEMENT_3D('',#139227,#86490,#86491);
#75207=AXIS2_PLACEMENT_3D('',#139229,#86493,#86494);
#75208=AXIS2_PLACEMENT_3D('',#139231,#86495,#86496);
#75209=AXIS2_PLACEMENT_3D('',#139232,#86497,#86498);
#75210=AXIS2_PLACEMENT_3D('',#139270,#86500,#86501);
#75211=AXIS2_PLACEMENT_3D('',#139272,#86503,#86504);
#75212=AXIS2_PLACEMENT_3D('',#139274,#86505,#86506);
#75213=AXIS2_PLACEMENT_3D('',#139275,#86507,#86508);
#75214=AXIS2_PLACEMENT_3D('',#139313,#86510,#86511);
#75215=AXIS2_PLACEMENT_3D('',#139315,#86513,#86514);
#75216=AXIS2_PLACEMENT_3D('',#139317,#86515,#86516);
#75217=AXIS2_PLACEMENT_3D('',#139318,#86517,#86518);
#75218=AXIS2_PLACEMENT_3D('',#139356,#86520,#86521);
#75219=AXIS2_PLACEMENT_3D('',#139358,#86523,#86524);
#75220=AXIS2_PLACEMENT_3D('',#139360,#86525,#86526);
#75221=AXIS2_PLACEMENT_3D('',#139361,#86527,#86528);
#75222=AXIS2_PLACEMENT_3D('',#139399,#86530,#86531);
#75223=AXIS2_PLACEMENT_3D('',#139401,#86533,#86534);
#75224=AXIS2_PLACEMENT_3D('',#139403,#86535,#86536);
#75225=AXIS2_PLACEMENT_3D('',#139404,#86537,#86538);
#75226=AXIS2_PLACEMENT_3D('',#139442,#86540,#86541);
#75227=AXIS2_PLACEMENT_3D('',#139444,#86543,#86544);
#75228=AXIS2_PLACEMENT_3D('',#139446,#86545,#86546);
#75229=AXIS2_PLACEMENT_3D('',#139447,#86547,#86548);
#75230=AXIS2_PLACEMENT_3D('',#139485,#86550,#86551);
#75231=AXIS2_PLACEMENT_3D('',#139487,#86553,#86554);
#75232=AXIS2_PLACEMENT_3D('',#139489,#86555,#86556);
#75233=AXIS2_PLACEMENT_3D('',#139490,#86557,#86558);
#75234=AXIS2_PLACEMENT_3D('',#139528,#86560,#86561);
#75235=AXIS2_PLACEMENT_3D('',#139530,#86563,#86564);
#75236=AXIS2_PLACEMENT_3D('',#139532,#86565,#86566);
#75237=AXIS2_PLACEMENT_3D('',#139533,#86567,#86568);
#75238=AXIS2_PLACEMENT_3D('',#139571,#86570,#86571);
#75239=AXIS2_PLACEMENT_3D('',#139573,#86573,#86574);
#75240=AXIS2_PLACEMENT_3D('',#139575,#86575,#86576);
#75241=AXIS2_PLACEMENT_3D('',#139576,#86577,#86578);
#75242=AXIS2_PLACEMENT_3D('',#139614,#86580,#86581);
#75243=AXIS2_PLACEMENT_3D('',#139616,#86583,#86584);
#75244=AXIS2_PLACEMENT_3D('',#139618,#86585,#86586);
#75245=AXIS2_PLACEMENT_3D('',#139619,#86587,#86588);
#75246=AXIS2_PLACEMENT_3D('',#139657,#86590,#86591);
#75247=AXIS2_PLACEMENT_3D('',#139659,#86593,#86594);
#75248=AXIS2_PLACEMENT_3D('',#139661,#86595,#86596);
#75249=AXIS2_PLACEMENT_3D('',#139662,#86597,#86598);
#75250=AXIS2_PLACEMENT_3D('',#139700,#86600,#86601);
#75251=AXIS2_PLACEMENT_3D('',#139702,#86603,#86604);
#75252=AXIS2_PLACEMENT_3D('',#139704,#86605,#86606);
#75253=AXIS2_PLACEMENT_3D('',#139705,#86607,#86608);
#75254=AXIS2_PLACEMENT_3D('',#139743,#86610,#86611);
#75255=AXIS2_PLACEMENT_3D('',#139745,#86613,#86614);
#75256=AXIS2_PLACEMENT_3D('',#139747,#86615,#86616);
#75257=AXIS2_PLACEMENT_3D('',#139748,#86617,#86618);
#75258=AXIS2_PLACEMENT_3D('',#139749,#86619,#86620);
#75259=AXIS2_PLACEMENT_3D('',#139759,#86621,#86622);
#75260=AXIS2_PLACEMENT_3D('',#139760,#86623,#86624);
#75261=AXIS2_PLACEMENT_3D('',#139783,#86626,#86627);
#75262=AXIS2_PLACEMENT_3D('',#139797,#86628,#86629);
#75263=AXIS2_PLACEMENT_3D('',#139814,#86630,#86631);
#75264=AXIS2_PLACEMENT_3D('',#139822,#86632,#86633);
#75265=AXIS2_PLACEMENT_3D('',#139839,#86634,#86635);
#75266=AXIS2_PLACEMENT_3D('',#139847,#86636,#86637);
#75267=AXIS2_PLACEMENT_3D('',#139864,#86638,#86639);
#75268=AXIS2_PLACEMENT_3D('',#139872,#86640,#86641);
#75269=AXIS2_PLACEMENT_3D('',#139889,#86642,#86643);
#75270=AXIS2_PLACEMENT_3D('',#139897,#86644,#86645);
#75271=AXIS2_PLACEMENT_3D('',#139914,#86646,#86647);
#75272=AXIS2_PLACEMENT_3D('',#139922,#86648,#86649);
#75273=AXIS2_PLACEMENT_3D('',#139939,#86650,#86651);
#75274=AXIS2_PLACEMENT_3D('',#139947,#86652,#86653);
#75275=AXIS2_PLACEMENT_3D('',#139964,#86654,#86655);
#75276=AXIS2_PLACEMENT_3D('',#139972,#86656,#86657);
#75277=AXIS2_PLACEMENT_3D('',#139989,#86658,#86659);
#75278=AXIS2_PLACEMENT_3D('',#139997,#86660,#86661);
#75279=AXIS2_PLACEMENT_3D('',#140014,#86662,#86663);
#75280=AXIS2_PLACEMENT_3D('',#140022,#86664,#86665);
#75281=AXIS2_PLACEMENT_3D('',#140039,#86666,#86667);
#75282=AXIS2_PLACEMENT_3D('',#140047,#86668,#86669);
#75283=AXIS2_PLACEMENT_3D('',#140064,#86670,#86671);
#75284=AXIS2_PLACEMENT_3D('',#140072,#86672,#86673);
#75285=AXIS2_PLACEMENT_3D('',#140089,#86674,#86675);
#75286=AXIS2_PLACEMENT_3D('',#140097,#86676,#86677);
#75287=AXIS2_PLACEMENT_3D('',#140114,#86678,#86679);
#75288=AXIS2_PLACEMENT_3D('',#140122,#86680,#86681);
#75289=AXIS2_PLACEMENT_3D('',#140139,#86682,#86683);
#75290=AXIS2_PLACEMENT_3D('',#140147,#86684,#86685);
#75291=AXIS2_PLACEMENT_3D('',#140164,#86686,#86687);
#75292=AXIS2_PLACEMENT_3D('',#140172,#86688,#86689);
#75293=AXIS2_PLACEMENT_3D('',#140189,#86690,#86691);
#75294=AXIS2_PLACEMENT_3D('',#140197,#86692,#86693);
#75295=AXIS2_PLACEMENT_3D('',#140214,#86694,#86695);
#75296=AXIS2_PLACEMENT_3D('',#140222,#86696,#86697);
#75297=AXIS2_PLACEMENT_3D('',#140239,#86698,#86699);
#75298=AXIS2_PLACEMENT_3D('',#140247,#86700,#86701);
#75299=AXIS2_PLACEMENT_3D('',#140264,#86702,#86703);
#75300=AXIS2_PLACEMENT_3D('',#140272,#86704,#86705);
#75301=AXIS2_PLACEMENT_3D('',#140289,#86706,#86707);
#75302=AXIS2_PLACEMENT_3D('',#140297,#86708,#86709);
#75303=AXIS2_PLACEMENT_3D('',#140314,#86710,#86711);
#75304=AXIS2_PLACEMENT_3D('',#140322,#86712,#86713);
#75305=AXIS2_PLACEMENT_3D('',#140339,#86714,#86715);
#75306=AXIS2_PLACEMENT_3D('',#140347,#86716,#86717);
#75307=AXIS2_PLACEMENT_3D('',#140364,#86718,#86719);
#75308=AXIS2_PLACEMENT_3D('',#140372,#86720,#86721);
#75309=AXIS2_PLACEMENT_3D('',#140389,#86722,#86723);
#75310=AXIS2_PLACEMENT_3D('',#140397,#86724,#86725);
#75311=AXIS2_PLACEMENT_3D('',#140414,#86726,#86727);
#75312=AXIS2_PLACEMENT_3D('',#140422,#86728,#86729);
#75313=AXIS2_PLACEMENT_3D('',#140439,#86730,#86731);
#75314=AXIS2_PLACEMENT_3D('',#140447,#86732,#86733);
#75315=AXIS2_PLACEMENT_3D('',#140464,#86734,#86735);
#75316=AXIS2_PLACEMENT_3D('',#140472,#86736,#86737);
#75317=AXIS2_PLACEMENT_3D('',#140489,#86738,#86739);
#75318=AXIS2_PLACEMENT_3D('',#140496,#86740,#86741);
#75319=AXIS2_PLACEMENT_3D('',#140514,#86742,#86743);
#75320=AXIS2_PLACEMENT_3D('',#140526,#86744,#86745);
#75321=AXIS2_PLACEMENT_3D('',#140543,#86746,#86747);
#75322=AXIS2_PLACEMENT_3D('',#140555,#86748,#86749);
#75323=AXIS2_PLACEMENT_3D('',#140572,#86750,#86751);
#75324=AXIS2_PLACEMENT_3D('',#140584,#86752,#86753);
#75325=AXIS2_PLACEMENT_3D('',#140601,#86754,#86755);
#75326=AXIS2_PLACEMENT_3D('',#140613,#86756,#86757);
#75327=AXIS2_PLACEMENT_3D('',#140630,#86758,#86759);
#75328=AXIS2_PLACEMENT_3D('',#140647,#86760,#86761);
#75329=AXIS2_PLACEMENT_3D('',#140664,#86762,#86763);
#75330=AXIS2_PLACEMENT_3D('',#140676,#86764,#86765);
#75331=AXIS2_PLACEMENT_3D('',#140693,#86766,#86767);
#75332=AXIS2_PLACEMENT_3D('',#140705,#86768,#86769);
#75333=AXIS2_PLACEMENT_3D('',#140722,#86770,#86771);
#75334=AXIS2_PLACEMENT_3D('',#140734,#86772,#86773);
#75335=AXIS2_PLACEMENT_3D('',#140751,#86774,#86775);
#75336=AXIS2_PLACEMENT_3D('',#140763,#86776,#86777);
#75337=AXIS2_PLACEMENT_3D('',#140780,#86778,#86779);
#75338=AXIS2_PLACEMENT_3D('',#140792,#86780,#86781);
#75339=AXIS2_PLACEMENT_3D('',#140809,#86782,#86783);
#75340=AXIS2_PLACEMENT_3D('',#140821,#86784,#86785);
#75341=AXIS2_PLACEMENT_3D('',#140838,#86786,#86787);
#75342=AXIS2_PLACEMENT_3D('',#140850,#86788,#86789);
#75343=AXIS2_PLACEMENT_3D('',#140867,#86790,#86791);
#75344=AXIS2_PLACEMENT_3D('',#140879,#86792,#86793);
#75345=AXIS2_PLACEMENT_3D('',#140896,#86794,#86795);
#75346=AXIS2_PLACEMENT_3D('',#140913,#86796,#86797);
#75347=AXIS2_PLACEMENT_3D('',#140930,#86798,#86799);
#75348=AXIS2_PLACEMENT_3D('',#140942,#86800,#86801);
#75349=AXIS2_PLACEMENT_3D('',#140959,#86802,#86803);
#75350=AXIS2_PLACEMENT_3D('',#140971,#86804,#86805);
#75351=AXIS2_PLACEMENT_3D('',#140988,#86806,#86807);
#75352=AXIS2_PLACEMENT_3D('',#141000,#86808,#86809);
#75353=AXIS2_PLACEMENT_3D('',#141017,#86810,#86811);
#75354=AXIS2_PLACEMENT_3D('',#141034,#86812,#86813);
#75355=AXIS2_PLACEMENT_3D('',#141051,#86814,#86815);
#75356=AXIS2_PLACEMENT_3D('',#141063,#86816,#86817);
#75357=AXIS2_PLACEMENT_3D('',#141080,#86818,#86819);
#75358=AXIS2_PLACEMENT_3D('',#141092,#86820,#86821);
#75359=AXIS2_PLACEMENT_3D('',#141109,#86822,#86823);
#75360=AXIS2_PLACEMENT_3D('',#141121,#86824,#86825);
#75361=AXIS2_PLACEMENT_3D('',#141138,#86826,#86827);
#75362=AXIS2_PLACEMENT_3D('',#141150,#86828,#86829);
#75363=AXIS2_PLACEMENT_3D('',#141167,#86830,#86831);
#75364=AXIS2_PLACEMENT_3D('',#141179,#86832,#86833);
#75365=AXIS2_PLACEMENT_3D('',#141196,#86834,#86835);
#75366=AXIS2_PLACEMENT_3D('',#141213,#86836,#86837);
#75367=AXIS2_PLACEMENT_3D('',#141230,#86838,#86839);
#75368=AXIS2_PLACEMENT_3D('',#141247,#86840,#86841);
#75369=AXIS2_PLACEMENT_3D('',#141264,#86842,#86843);
#75370=AXIS2_PLACEMENT_3D('',#141276,#86844,#86845);
#75371=AXIS2_PLACEMENT_3D('',#141293,#86846,#86847);
#75372=AXIS2_PLACEMENT_3D('',#141305,#86848,#86849);
#75373=AXIS2_PLACEMENT_3D('',#141322,#86850,#86851);
#75374=AXIS2_PLACEMENT_3D('',#141334,#86852,#86853);
#75375=AXIS2_PLACEMENT_3D('',#141351,#86854,#86855);
#75376=AXIS2_PLACEMENT_3D('',#141367,#86856,#86857);
#75377=AXIS2_PLACEMENT_3D('',#141376,#86858,#86859);
#75378=AXIS2_PLACEMENT_3D('',#141384,#86861,#86862);
#75379=AXIS2_PLACEMENT_3D('',#141386,#86863,#86864);
#75380=AXIS2_PLACEMENT_3D('',#141388,#86865,#86866);
#75381=AXIS2_PLACEMENT_3D('',#141389,#86867,#86868);
#75382=AXIS2_PLACEMENT_3D('',#141409,#86870,#86871);
#75383=AXIS2_PLACEMENT_3D('',#141417,#86873,#86874);
#75384=AXIS2_PLACEMENT_3D('',#141419,#86875,#86876);
#75385=AXIS2_PLACEMENT_3D('',#141421,#86877,#86878);
#75386=AXIS2_PLACEMENT_3D('',#141422,#86879,#86880);
#75387=AXIS2_PLACEMENT_3D('',#141442,#86882,#86883);
#75388=AXIS2_PLACEMENT_3D('',#141450,#86885,#86886);
#75389=AXIS2_PLACEMENT_3D('',#141452,#86887,#86888);
#75390=AXIS2_PLACEMENT_3D('',#141454,#86889,#86890);
#75391=AXIS2_PLACEMENT_3D('',#141455,#86891,#86892);
#75392=AXIS2_PLACEMENT_3D('',#141475,#86894,#86895);
#75393=AXIS2_PLACEMENT_3D('',#141483,#86897,#86898);
#75394=AXIS2_PLACEMENT_3D('',#141485,#86899,#86900);
#75395=AXIS2_PLACEMENT_3D('',#141487,#86901,#86902);
#75396=AXIS2_PLACEMENT_3D('',#141488,#86903,#86904);
#75397=AXIS2_PLACEMENT_3D('',#141508,#86906,#86907);
#75398=AXIS2_PLACEMENT_3D('',#141516,#86909,#86910);
#75399=AXIS2_PLACEMENT_3D('',#141518,#86911,#86912);
#75400=AXIS2_PLACEMENT_3D('',#141520,#86913,#86914);
#75401=AXIS2_PLACEMENT_3D('',#141521,#86915,#86916);
#75402=AXIS2_PLACEMENT_3D('',#141541,#86918,#86919);
#75403=AXIS2_PLACEMENT_3D('',#141549,#86921,#86922);
#75404=AXIS2_PLACEMENT_3D('',#141551,#86923,#86924);
#75405=AXIS2_PLACEMENT_3D('',#141553,#86925,#86926);
#75406=AXIS2_PLACEMENT_3D('',#141554,#86927,#86928);
#75407=AXIS2_PLACEMENT_3D('',#141574,#86930,#86931);
#75408=AXIS2_PLACEMENT_3D('',#141582,#86933,#86934);
#75409=AXIS2_PLACEMENT_3D('',#141584,#86935,#86936);
#75410=AXIS2_PLACEMENT_3D('',#141586,#86937,#86938);
#75411=AXIS2_PLACEMENT_3D('',#141587,#86939,#86940);
#75412=AXIS2_PLACEMENT_3D('',#141607,#86942,#86943);
#75413=AXIS2_PLACEMENT_3D('',#141615,#86945,#86946);
#75414=AXIS2_PLACEMENT_3D('',#141617,#86947,#86948);
#75415=AXIS2_PLACEMENT_3D('',#141619,#86949,#86950);
#75416=AXIS2_PLACEMENT_3D('',#141620,#86951,#86952);
#75417=AXIS2_PLACEMENT_3D('',#141640,#86954,#86955);
#75418=AXIS2_PLACEMENT_3D('',#141648,#86957,#86958);
#75419=AXIS2_PLACEMENT_3D('',#141650,#86959,#86960);
#75420=AXIS2_PLACEMENT_3D('',#141652,#86961,#86962);
#75421=AXIS2_PLACEMENT_3D('',#141653,#86963,#86964);
#75422=AXIS2_PLACEMENT_3D('',#141673,#86966,#86967);
#75423=AXIS2_PLACEMENT_3D('',#141681,#86969,#86970);
#75424=AXIS2_PLACEMENT_3D('',#141683,#86971,#86972);
#75425=AXIS2_PLACEMENT_3D('',#141685,#86973,#86974);
#75426=AXIS2_PLACEMENT_3D('',#141686,#86975,#86976);
#75427=AXIS2_PLACEMENT_3D('',#141706,#86978,#86979);
#75428=AXIS2_PLACEMENT_3D('',#141714,#86981,#86982);
#75429=AXIS2_PLACEMENT_3D('',#141716,#86983,#86984);
#75430=AXIS2_PLACEMENT_3D('',#141718,#86985,#86986);
#75431=AXIS2_PLACEMENT_3D('',#141719,#86987,#86988);
#75432=AXIS2_PLACEMENT_3D('',#141739,#86990,#86991);
#75433=AXIS2_PLACEMENT_3D('',#141747,#86993,#86994);
#75434=AXIS2_PLACEMENT_3D('',#141749,#86995,#86996);
#75435=AXIS2_PLACEMENT_3D('',#141751,#86997,#86998);
#75436=AXIS2_PLACEMENT_3D('',#141752,#86999,#87000);
#75437=AXIS2_PLACEMENT_3D('',#141772,#87002,#87003);
#75438=AXIS2_PLACEMENT_3D('',#141780,#87005,#87006);
#75439=AXIS2_PLACEMENT_3D('',#141782,#87007,#87008);
#75440=AXIS2_PLACEMENT_3D('',#141784,#87009,#87010);
#75441=AXIS2_PLACEMENT_3D('',#141785,#87011,#87012);
#75442=AXIS2_PLACEMENT_3D('',#141805,#87014,#87015);
#75443=AXIS2_PLACEMENT_3D('',#141813,#87017,#87018);
#75444=AXIS2_PLACEMENT_3D('',#141815,#87019,#87020);
#75445=AXIS2_PLACEMENT_3D('',#141817,#87021,#87022);
#75446=AXIS2_PLACEMENT_3D('',#141818,#87023,#87024);
#75447=AXIS2_PLACEMENT_3D('',#141862,#87028,#87029);
#75448=AXIS2_PLACEMENT_3D('',#141870,#87031,#87032);
#75449=AXIS2_PLACEMENT_3D('',#141872,#87033,#87034);
#75450=AXIS2_PLACEMENT_3D('',#141874,#87035,#87036);
#75451=AXIS2_PLACEMENT_3D('',#141875,#87037,#87038);
#75452=AXIS2_PLACEMENT_3D('',#141895,#87040,#87041);
#75453=AXIS2_PLACEMENT_3D('',#141903,#87043,#87044);
#75454=AXIS2_PLACEMENT_3D('',#141905,#87045,#87046);
#75455=AXIS2_PLACEMENT_3D('',#141907,#87047,#87048);
#75456=AXIS2_PLACEMENT_3D('',#141908,#87049,#87050);
#75457=AXIS2_PLACEMENT_3D('',#141928,#87052,#87053);
#75458=AXIS2_PLACEMENT_3D('',#141936,#87055,#87056);
#75459=AXIS2_PLACEMENT_3D('',#141938,#87057,#87058);
#75460=AXIS2_PLACEMENT_3D('',#141940,#87059,#87060);
#75461=AXIS2_PLACEMENT_3D('',#141941,#87061,#87062);
#75462=AXIS2_PLACEMENT_3D('',#141961,#87064,#87065);
#75463=AXIS2_PLACEMENT_3D('',#141969,#87067,#87068);
#75464=AXIS2_PLACEMENT_3D('',#141971,#87069,#87070);
#75465=AXIS2_PLACEMENT_3D('',#141973,#87071,#87072);
#75466=AXIS2_PLACEMENT_3D('',#141974,#87073,#87074);
#75467=AXIS2_PLACEMENT_3D('',#141994,#87076,#87077);
#75468=AXIS2_PLACEMENT_3D('',#142013,#87079,#87080);
#75469=AXIS2_PLACEMENT_3D('',#142015,#87082,#87083);
#75470=AXIS2_PLACEMENT_3D('',#142017,#87084,#87085);
#75471=AXIS2_PLACEMENT_3D('',#142018,#87086,#87087);
#75472=AXIS2_PLACEMENT_3D('',#142028,#87089,#87090);
#75473=AXIS2_PLACEMENT_3D('',#142035,#87091,#87092);
#75474=AXIS2_PLACEMENT_3D('',#142037,#87093,#87094);
#75475=AXIS2_PLACEMENT_3D('',#142039,#87095,#87096);
#75476=AXIS2_PLACEMENT_3D('',#142040,#87097,#87098);
#75477=AXIS2_PLACEMENT_3D('',#142060,#87100,#87101);
#75478=AXIS2_PLACEMENT_3D('',#142068,#87103,#87104);
#75479=AXIS2_PLACEMENT_3D('',#142070,#87105,#87106);
#75480=AXIS2_PLACEMENT_3D('',#142072,#87107,#87108);
#75481=AXIS2_PLACEMENT_3D('',#142073,#87109,#87110);
#75482=AXIS2_PLACEMENT_3D('',#142093,#87112,#87113);
#75483=AXIS2_PLACEMENT_3D('',#142101,#87115,#87116);
#75484=AXIS2_PLACEMENT_3D('',#142103,#87117,#87118);
#75485=AXIS2_PLACEMENT_3D('',#142105,#87119,#87120);
#75486=AXIS2_PLACEMENT_3D('',#142106,#87121,#87122);
#75487=AXIS2_PLACEMENT_3D('',#142126,#87124,#87125);
#75488=AXIS2_PLACEMENT_3D('',#142134,#87127,#87128);
#75489=AXIS2_PLACEMENT_3D('',#142136,#87129,#87130);
#75490=AXIS2_PLACEMENT_3D('',#142138,#87131,#87132);
#75491=AXIS2_PLACEMENT_3D('',#142139,#87133,#87134);
#75492=AXIS2_PLACEMENT_3D('',#142159,#87136,#87137);
#75493=AXIS2_PLACEMENT_3D('',#142167,#87139,#87140);
#75494=AXIS2_PLACEMENT_3D('',#142169,#87141,#87142);
#75495=AXIS2_PLACEMENT_3D('',#142171,#87143,#87144);
#75496=AXIS2_PLACEMENT_3D('',#142172,#87145,#87146);
#75497=AXIS2_PLACEMENT_3D('',#142192,#87148,#87149);
#75498=AXIS2_PLACEMENT_3D('',#142200,#87151,#87152);
#75499=AXIS2_PLACEMENT_3D('',#142202,#87153,#87154);
#75500=AXIS2_PLACEMENT_3D('',#142204,#87155,#87156);
#75501=AXIS2_PLACEMENT_3D('',#142205,#87157,#87158);
#75502=AXIS2_PLACEMENT_3D('',#142225,#87160,#87161);
#75503=AXIS2_PLACEMENT_3D('',#142233,#87163,#87164);
#75504=AXIS2_PLACEMENT_3D('',#142235,#87165,#87166);
#75505=AXIS2_PLACEMENT_3D('',#142237,#87167,#87168);
#75506=AXIS2_PLACEMENT_3D('',#142238,#87169,#87170);
#75507=AXIS2_PLACEMENT_3D('',#142258,#87172,#87173);
#75508=AXIS2_PLACEMENT_3D('',#142266,#87175,#87176);
#75509=AXIS2_PLACEMENT_3D('',#142268,#87177,#87178);
#75510=AXIS2_PLACEMENT_3D('',#142270,#87179,#87180);
#75511=AXIS2_PLACEMENT_3D('',#142271,#87181,#87182);
#75512=AXIS2_PLACEMENT_3D('',#142291,#87184,#87185);
#75513=AXIS2_PLACEMENT_3D('',#142299,#87187,#87188);
#75514=AXIS2_PLACEMENT_3D('',#142301,#87189,#87190);
#75515=AXIS2_PLACEMENT_3D('',#142303,#87191,#87192);
#75516=AXIS2_PLACEMENT_3D('',#142304,#87193,#87194);
#75517=AXIS2_PLACEMENT_3D('',#142329,#87197,#87198);
#75518=AXIS2_PLACEMENT_3D('',#142351,#87199,#87200);
#75519=AXIS2_PLACEMENT_3D('',#142353,#87202,#87203);
#75520=AXIS2_PLACEMENT_3D('',#142355,#87204,#87205);
#75521=AXIS2_PLACEMENT_3D('',#142356,#87206,#87207);
#75522=AXIS2_PLACEMENT_3D('',#142370,#87209,#87210);
#75523=AXIS2_PLACEMENT_3D('',#142392,#87211,#87212);
#75524=AXIS2_PLACEMENT_3D('',#142394,#87214,#87215);
#75525=AXIS2_PLACEMENT_3D('',#142396,#87216,#87217);
#75526=AXIS2_PLACEMENT_3D('',#142397,#87218,#87219);
#75527=AXIS2_PLACEMENT_3D('',#142411,#87221,#87222);
#75528=AXIS2_PLACEMENT_3D('',#142433,#87223,#87224);
#75529=AXIS2_PLACEMENT_3D('',#142435,#87226,#87227);
#75530=AXIS2_PLACEMENT_3D('',#142437,#87228,#87229);
#75531=AXIS2_PLACEMENT_3D('',#142438,#87230,#87231);
#75532=AXIS2_PLACEMENT_3D('',#142452,#87233,#87234);
#75533=AXIS2_PLACEMENT_3D('',#142474,#87235,#87236);
#75534=AXIS2_PLACEMENT_3D('',#142476,#87238,#87239);
#75535=AXIS2_PLACEMENT_3D('',#142478,#87240,#87241);
#75536=AXIS2_PLACEMENT_3D('',#142479,#87242,#87243);
#75537=AXIS2_PLACEMENT_3D('',#142493,#87245,#87246);
#75538=AXIS2_PLACEMENT_3D('',#142515,#87247,#87248);
#75539=AXIS2_PLACEMENT_3D('',#142517,#87250,#87251);
#75540=AXIS2_PLACEMENT_3D('',#142519,#87252,#87253);
#75541=AXIS2_PLACEMENT_3D('',#142520,#87254,#87255);
#75542=AXIS2_PLACEMENT_3D('',#142534,#87257,#87258);
#75543=AXIS2_PLACEMENT_3D('',#142556,#87259,#87260);
#75544=AXIS2_PLACEMENT_3D('',#142558,#87262,#87263);
#75545=AXIS2_PLACEMENT_3D('',#142560,#87264,#87265);
#75546=AXIS2_PLACEMENT_3D('',#142561,#87266,#87267);
#75547=AXIS2_PLACEMENT_3D('',#142575,#87269,#87270);
#75548=AXIS2_PLACEMENT_3D('',#142597,#87271,#87272);
#75549=AXIS2_PLACEMENT_3D('',#142599,#87274,#87275);
#75550=AXIS2_PLACEMENT_3D('',#142601,#87276,#87277);
#75551=AXIS2_PLACEMENT_3D('',#142602,#87278,#87279);
#75552=AXIS2_PLACEMENT_3D('',#142616,#87281,#87282);
#75553=AXIS2_PLACEMENT_3D('',#142638,#87283,#87284);
#75554=AXIS2_PLACEMENT_3D('',#142640,#87286,#87287);
#75555=AXIS2_PLACEMENT_3D('',#142642,#87288,#87289);
#75556=AXIS2_PLACEMENT_3D('',#142643,#87290,#87291);
#75557=AXIS2_PLACEMENT_3D('',#142657,#87293,#87294);
#75558=AXIS2_PLACEMENT_3D('',#142679,#87295,#87296);
#75559=AXIS2_PLACEMENT_3D('',#142681,#87298,#87299);
#75560=AXIS2_PLACEMENT_3D('',#142683,#87300,#87301);
#75561=AXIS2_PLACEMENT_3D('',#142684,#87302,#87303);
#75562=AXIS2_PLACEMENT_3D('',#142698,#87305,#87306);
#75563=AXIS2_PLACEMENT_3D('',#142720,#87307,#87308);
#75564=AXIS2_PLACEMENT_3D('',#142722,#87310,#87311);
#75565=AXIS2_PLACEMENT_3D('',#142724,#87312,#87313);
#75566=AXIS2_PLACEMENT_3D('',#142725,#87314,#87315);
#75567=AXIS2_PLACEMENT_3D('',#142739,#87317,#87318);
#75568=AXIS2_PLACEMENT_3D('',#142761,#87319,#87320);
#75569=AXIS2_PLACEMENT_3D('',#142763,#87322,#87323);
#75570=AXIS2_PLACEMENT_3D('',#142765,#87324,#87325);
#75571=AXIS2_PLACEMENT_3D('',#142766,#87326,#87327);
#75572=AXIS2_PLACEMENT_3D('',#142780,#87329,#87330);
#75573=AXIS2_PLACEMENT_3D('',#142802,#87331,#87332);
#75574=AXIS2_PLACEMENT_3D('',#142804,#87334,#87335);
#75575=AXIS2_PLACEMENT_3D('',#142806,#87336,#87337);
#75576=AXIS2_PLACEMENT_3D('',#142807,#87338,#87339);
#75577=AXIS2_PLACEMENT_3D('',#142821,#87341,#87342);
#75578=AXIS2_PLACEMENT_3D('',#142843,#87343,#87344);
#75579=AXIS2_PLACEMENT_3D('',#142845,#87346,#87347);
#75580=AXIS2_PLACEMENT_3D('',#142847,#87348,#87349);
#75581=AXIS2_PLACEMENT_3D('',#142848,#87350,#87351);
#75582=AXIS2_PLACEMENT_3D('',#142862,#87353,#87354);
#75583=AXIS2_PLACEMENT_3D('',#142884,#87355,#87356);
#75584=AXIS2_PLACEMENT_3D('',#142886,#87358,#87359);
#75585=AXIS2_PLACEMENT_3D('',#142888,#87360,#87361);
#75586=AXIS2_PLACEMENT_3D('',#142889,#87362,#87363);
#75587=AXIS2_PLACEMENT_3D('',#142903,#87365,#87366);
#75588=AXIS2_PLACEMENT_3D('',#142925,#87367,#87368);
#75589=AXIS2_PLACEMENT_3D('',#142927,#87370,#87371);
#75590=AXIS2_PLACEMENT_3D('',#142929,#87372,#87373);
#75591=AXIS2_PLACEMENT_3D('',#142930,#87374,#87375);
#75592=AXIS2_PLACEMENT_3D('',#142944,#87377,#87378);
#75593=AXIS2_PLACEMENT_3D('',#142966,#87379,#87380);
#75594=AXIS2_PLACEMENT_3D('',#142968,#87382,#87383);
#75595=AXIS2_PLACEMENT_3D('',#142970,#87384,#87385);
#75596=AXIS2_PLACEMENT_3D('',#142971,#87386,#87387);
#75597=AXIS2_PLACEMENT_3D('',#142985,#87389,#87390);
#75598=AXIS2_PLACEMENT_3D('',#143007,#87391,#87392);
#75599=AXIS2_PLACEMENT_3D('',#143009,#87394,#87395);
#75600=AXIS2_PLACEMENT_3D('',#143011,#87396,#87397);
#75601=AXIS2_PLACEMENT_3D('',#143012,#87398,#87399);
#75602=AXIS2_PLACEMENT_3D('',#143026,#87401,#87402);
#75603=AXIS2_PLACEMENT_3D('',#143048,#87403,#87404);
#75604=AXIS2_PLACEMENT_3D('',#143050,#87406,#87407);
#75605=AXIS2_PLACEMENT_3D('',#143052,#87408,#87409);
#75606=AXIS2_PLACEMENT_3D('',#143053,#87410,#87411);
#75607=AXIS2_PLACEMENT_3D('',#143067,#87413,#87414);
#75608=AXIS2_PLACEMENT_3D('',#143089,#87415,#87416);
#75609=AXIS2_PLACEMENT_3D('',#143091,#87418,#87419);
#75610=AXIS2_PLACEMENT_3D('',#143093,#87420,#87421);
#75611=AXIS2_PLACEMENT_3D('',#143094,#87422,#87423);
#75612=AXIS2_PLACEMENT_3D('',#143108,#87425,#87426);
#75613=AXIS2_PLACEMENT_3D('',#143130,#87427,#87428);
#75614=AXIS2_PLACEMENT_3D('',#143132,#87430,#87431);
#75615=AXIS2_PLACEMENT_3D('',#143134,#87432,#87433);
#75616=AXIS2_PLACEMENT_3D('',#143135,#87434,#87435);
#75617=AXIS2_PLACEMENT_3D('',#143149,#87437,#87438);
#75618=AXIS2_PLACEMENT_3D('',#143171,#87439,#87440);
#75619=AXIS2_PLACEMENT_3D('',#143173,#87442,#87443);
#75620=AXIS2_PLACEMENT_3D('',#143175,#87444,#87445);
#75621=AXIS2_PLACEMENT_3D('',#143176,#87446,#87447);
#75622=AXIS2_PLACEMENT_3D('',#143222,#87451,#87452);
#75623=AXIS2_PLACEMENT_3D('',#143244,#87453,#87454);
#75624=AXIS2_PLACEMENT_3D('',#143246,#87456,#87457);
#75625=AXIS2_PLACEMENT_3D('',#143248,#87458,#87459);
#75626=AXIS2_PLACEMENT_3D('',#143249,#87460,#87461);
#75627=AXIS2_PLACEMENT_3D('',#143263,#87463,#87464);
#75628=AXIS2_PLACEMENT_3D('',#143285,#87465,#87466);
#75629=AXIS2_PLACEMENT_3D('',#143287,#87468,#87469);
#75630=AXIS2_PLACEMENT_3D('',#143289,#87470,#87471);
#75631=AXIS2_PLACEMENT_3D('',#143290,#87472,#87473);
#75632=AXIS2_PLACEMENT_3D('',#143304,#87475,#87476);
#75633=AXIS2_PLACEMENT_3D('',#143326,#87477,#87478);
#75634=AXIS2_PLACEMENT_3D('',#143328,#87480,#87481);
#75635=AXIS2_PLACEMENT_3D('',#143330,#87482,#87483);
#75636=AXIS2_PLACEMENT_3D('',#143331,#87484,#87485);
#75637=AXIS2_PLACEMENT_3D('',#143345,#87487,#87488);
#75638=AXIS2_PLACEMENT_3D('',#143367,#87489,#87490);
#75639=AXIS2_PLACEMENT_3D('',#143369,#87492,#87493);
#75640=AXIS2_PLACEMENT_3D('',#143371,#87494,#87495);
#75641=AXIS2_PLACEMENT_3D('',#143372,#87496,#87497);
#75642=AXIS2_PLACEMENT_3D('',#143386,#87499,#87500);
#75643=AXIS2_PLACEMENT_3D('',#143408,#87501,#87502);
#75644=AXIS2_PLACEMENT_3D('',#143410,#87504,#87505);
#75645=AXIS2_PLACEMENT_3D('',#143412,#87506,#87507);
#75646=AXIS2_PLACEMENT_3D('',#143413,#87508,#87509);
#75647=AXIS2_PLACEMENT_3D('',#143427,#87511,#87512);
#75648=AXIS2_PLACEMENT_3D('',#143449,#87513,#87514);
#75649=AXIS2_PLACEMENT_3D('',#143451,#87516,#87517);
#75650=AXIS2_PLACEMENT_3D('',#143453,#87518,#87519);
#75651=AXIS2_PLACEMENT_3D('',#143454,#87520,#87521);
#75652=AXIS2_PLACEMENT_3D('',#143468,#87523,#87524);
#75653=AXIS2_PLACEMENT_3D('',#143490,#87525,#87526);
#75654=AXIS2_PLACEMENT_3D('',#143492,#87528,#87529);
#75655=AXIS2_PLACEMENT_3D('',#143494,#87530,#87531);
#75656=AXIS2_PLACEMENT_3D('',#143495,#87532,#87533);
#75657=AXIS2_PLACEMENT_3D('',#143503,#87534,#87535);
#75658=AXIS2_PLACEMENT_3D('',#143520,#87536,#87537);
#75659=AXIS2_PLACEMENT_3D('',#143528,#87538,#87539);
#75660=AXIS2_PLACEMENT_3D('',#143545,#87540,#87541);
#75661=AXIS2_PLACEMENT_3D('',#143553,#87542,#87543);
#75662=AXIS2_PLACEMENT_3D('',#143570,#87544,#87545);
#75663=AXIS2_PLACEMENT_3D('',#143578,#87546,#87547);
#75664=AXIS2_PLACEMENT_3D('',#143595,#87548,#87549);
#75665=AXIS2_PLACEMENT_3D('',#143603,#87550,#87551);
#75666=AXIS2_PLACEMENT_3D('',#143620,#87552,#87553);
#75667=AXIS2_PLACEMENT_3D('',#143628,#87554,#87555);
#75668=AXIS2_PLACEMENT_3D('',#143645,#87556,#87557);
#75669=AXIS2_PLACEMENT_3D('',#143653,#87558,#87559);
#75670=AXIS2_PLACEMENT_3D('',#143670,#87560,#87561);
#75671=AXIS2_PLACEMENT_3D('',#143678,#87562,#87563);
#75672=AXIS2_PLACEMENT_3D('',#143695,#87564,#87565);
#75673=AXIS2_PLACEMENT_3D('',#143703,#87566,#87567);
#75674=AXIS2_PLACEMENT_3D('',#143720,#87568,#87569);
#75675=AXIS2_PLACEMENT_3D('',#143728,#87570,#87571);
#75676=AXIS2_PLACEMENT_3D('',#143745,#87572,#87573);
#75677=AXIS2_PLACEMENT_3D('',#143753,#87574,#87575);
#75678=AXIS2_PLACEMENT_3D('',#143770,#87576,#87577);
#75679=AXIS2_PLACEMENT_3D('',#143778,#87578,#87579);
#75680=AXIS2_PLACEMENT_3D('',#143795,#87580,#87581);
#75681=AXIS2_PLACEMENT_3D('',#143803,#87582,#87583);
#75682=AXIS2_PLACEMENT_3D('',#143820,#87584,#87585);
#75683=AXIS2_PLACEMENT_3D('',#143828,#87586,#87587);
#75684=AXIS2_PLACEMENT_3D('',#143845,#87588,#87589);
#75685=AXIS2_PLACEMENT_3D('',#143853,#87590,#87591);
#75686=AXIS2_PLACEMENT_3D('',#143870,#87592,#87593);
#75687=AXIS2_PLACEMENT_3D('',#143878,#87594,#87595);
#75688=AXIS2_PLACEMENT_3D('',#143895,#87596,#87597);
#75689=AXIS2_PLACEMENT_3D('',#143903,#87598,#87599);
#75690=AXIS2_PLACEMENT_3D('',#143920,#87600,#87601);
#75691=AXIS2_PLACEMENT_3D('',#143928,#87602,#87603);
#75692=AXIS2_PLACEMENT_3D('',#143945,#87604,#87605);
#75693=AXIS2_PLACEMENT_3D('',#143953,#87606,#87607);
#75694=AXIS2_PLACEMENT_3D('',#143970,#87608,#87609);
#75695=AXIS2_PLACEMENT_3D('',#143978,#87610,#87611);
#75696=AXIS2_PLACEMENT_3D('',#143995,#87612,#87613);
#75697=AXIS2_PLACEMENT_3D('',#144003,#87614,#87615);
#75698=AXIS2_PLACEMENT_3D('',#144020,#87616,#87617);
#75699=AXIS2_PLACEMENT_3D('',#144028,#87618,#87619);
#75700=AXIS2_PLACEMENT_3D('',#144045,#87620,#87621);
#75701=AXIS2_PLACEMENT_3D('',#144053,#87622,#87623);
#75702=AXIS2_PLACEMENT_3D('',#144070,#87624,#87625);
#75703=AXIS2_PLACEMENT_3D('',#144078,#87626,#87627);
#75704=AXIS2_PLACEMENT_3D('',#144095,#87628,#87629);
#75705=AXIS2_PLACEMENT_3D('',#144103,#87630,#87631);
#75706=AXIS2_PLACEMENT_3D('',#144120,#87632,#87633);
#75707=AXIS2_PLACEMENT_3D('',#144128,#87634,#87635);
#75708=AXIS2_PLACEMENT_3D('',#144145,#87636,#87637);
#75709=AXIS2_PLACEMENT_3D('',#144153,#87638,#87639);
#75710=AXIS2_PLACEMENT_3D('',#144170,#87640,#87641);
#75711=AXIS2_PLACEMENT_3D('',#144178,#87642,#87643);
#75712=AXIS2_PLACEMENT_3D('',#144195,#87644,#87645);
#75713=AXIS2_PLACEMENT_3D('',#144203,#87646,#87647);
#75714=AXIS2_PLACEMENT_3D('',#144220,#87648,#87649);
#75715=AXIS2_PLACEMENT_3D('',#144228,#87650,#87651);
#75716=AXIS2_PLACEMENT_3D('',#144241,#87652,#87653);
#75717=AXIS2_PLACEMENT_3D('',#144249,#87654,#87655);
#75718=AXIS2_PLACEMENT_3D('',#144262,#87656,#87657);
#75719=AXIS2_PLACEMENT_3D('',#144270,#87658,#87659);
#75720=AXIS2_PLACEMENT_3D('',#144283,#87660,#87661);
#75721=AXIS2_PLACEMENT_3D('',#144291,#87662,#87663);
#75722=AXIS2_PLACEMENT_3D('',#144304,#87664,#87665);
#75723=AXIS2_PLACEMENT_3D('',#144312,#87666,#87667);
#75724=AXIS2_PLACEMENT_3D('',#144325,#87668,#87669);
#75725=AXIS2_PLACEMENT_3D('',#144333,#87670,#87671);
#75726=AXIS2_PLACEMENT_3D('',#144346,#87672,#87673);
#75727=AXIS2_PLACEMENT_3D('',#144354,#87674,#87675);
#75728=AXIS2_PLACEMENT_3D('',#144367,#87676,#87677);
#75729=AXIS2_PLACEMENT_3D('',#144375,#87678,#87679);
#75730=AXIS2_PLACEMENT_3D('',#144388,#87680,#87681);
#75731=AXIS2_PLACEMENT_3D('',#144396,#87682,#87683);
#75732=AXIS2_PLACEMENT_3D('',#144409,#87684,#87685);
#75733=AXIS2_PLACEMENT_3D('',#144417,#87686,#87687);
#75734=AXIS2_PLACEMENT_3D('',#144430,#87688,#87689);
#75735=AXIS2_PLACEMENT_3D('',#144438,#87690,#87691);
#75736=AXIS2_PLACEMENT_3D('',#144451,#87692,#87693);
#75737=AXIS2_PLACEMENT_3D('',#144459,#87694,#87695);
#75738=AXIS2_PLACEMENT_3D('',#144472,#87696,#87697);
#75739=AXIS2_PLACEMENT_3D('',#144480,#87698,#87699);
#75740=AXIS2_PLACEMENT_3D('',#144493,#87700,#87701);
#75741=AXIS2_PLACEMENT_3D('',#144501,#87702,#87703);
#75742=AXIS2_PLACEMENT_3D('',#144514,#87704,#87705);
#75743=AXIS2_PLACEMENT_3D('',#144522,#87706,#87707);
#75744=AXIS2_PLACEMENT_3D('',#144535,#87708,#87709);
#75745=AXIS2_PLACEMENT_3D('',#144543,#87710,#87711);
#75746=AXIS2_PLACEMENT_3D('',#144556,#87712,#87713);
#75747=AXIS2_PLACEMENT_3D('',#144564,#87714,#87715);
#75748=AXIS2_PLACEMENT_3D('',#144577,#87716,#87717);
#75749=AXIS2_PLACEMENT_3D('',#144585,#87718,#87719);
#75750=AXIS2_PLACEMENT_3D('',#144598,#87720,#87721);
#75751=AXIS2_PLACEMENT_3D('',#144606,#87722,#87723);
#75752=AXIS2_PLACEMENT_3D('',#144619,#87724,#87725);
#75753=AXIS2_PLACEMENT_3D('',#144627,#87726,#87727);
#75754=AXIS2_PLACEMENT_3D('',#144640,#87728,#87729);
#75755=AXIS2_PLACEMENT_3D('',#144648,#87730,#87731);
#75756=AXIS2_PLACEMENT_3D('',#144661,#87732,#87733);
#75757=AXIS2_PLACEMENT_3D('',#144669,#87734,#87735);
#75758=AXIS2_PLACEMENT_3D('',#144682,#87736,#87737);
#75759=AXIS2_PLACEMENT_3D('',#144690,#87738,#87739);
#75760=AXIS2_PLACEMENT_3D('',#144703,#87740,#87741);
#75761=AXIS2_PLACEMENT_3D('',#144711,#87742,#87743);
#75762=AXIS2_PLACEMENT_3D('',#144724,#87744,#87745);
#75763=AXIS2_PLACEMENT_3D('',#144732,#87746,#87747);
#75764=AXIS2_PLACEMENT_3D('',#144745,#87748,#87749);
#75765=AXIS2_PLACEMENT_3D('',#144753,#87750,#87751);
#75766=AXIS2_PLACEMENT_3D('',#144766,#87752,#87753);
#75767=AXIS2_PLACEMENT_3D('',#144774,#87754,#87755);
#75768=AXIS2_PLACEMENT_3D('',#144787,#87756,#87757);
#75769=AXIS2_PLACEMENT_3D('',#144795,#87758,#87759);
#75770=AXIS2_PLACEMENT_3D('',#144808,#87760,#87761);
#75771=AXIS2_PLACEMENT_3D('',#144816,#87762,#87763);
#75772=AXIS2_PLACEMENT_3D('',#144829,#87764,#87765);
#75773=AXIS2_PLACEMENT_3D('',#144838,#87766,#87767);
#75774=AXIS2_PLACEMENT_3D('',#144854,#87769,#87770);
#75775=AXIS2_PLACEMENT_3D('',#144862,#87772,#87773);
#75776=AXIS2_PLACEMENT_3D('',#144864,#87774,#87775);
#75777=AXIS2_PLACEMENT_3D('',#144866,#87776,#87777);
#75778=AXIS2_PLACEMENT_3D('',#144867,#87778,#87779);
#75779=AXIS2_PLACEMENT_3D('',#144883,#87781,#87782);
#75780=AXIS2_PLACEMENT_3D('',#144891,#87784,#87785);
#75781=AXIS2_PLACEMENT_3D('',#144893,#87786,#87787);
#75782=AXIS2_PLACEMENT_3D('',#144895,#87788,#87789);
#75783=AXIS2_PLACEMENT_3D('',#144896,#87790,#87791);
#75784=AXIS2_PLACEMENT_3D('',#144912,#87793,#87794);
#75785=AXIS2_PLACEMENT_3D('',#144920,#87796,#87797);
#75786=AXIS2_PLACEMENT_3D('',#144922,#87798,#87799);
#75787=AXIS2_PLACEMENT_3D('',#144924,#87800,#87801);
#75788=AXIS2_PLACEMENT_3D('',#144925,#87802,#87803);
#75789=AXIS2_PLACEMENT_3D('',#144941,#87805,#87806);
#75790=AXIS2_PLACEMENT_3D('',#144949,#87808,#87809);
#75791=AXIS2_PLACEMENT_3D('',#144951,#87810,#87811);
#75792=AXIS2_PLACEMENT_3D('',#144953,#87812,#87813);
#75793=AXIS2_PLACEMENT_3D('',#144954,#87814,#87815);
#75794=AXIS2_PLACEMENT_3D('',#144970,#87817,#87818);
#75795=AXIS2_PLACEMENT_3D('',#144978,#87820,#87821);
#75796=AXIS2_PLACEMENT_3D('',#144980,#87822,#87823);
#75797=AXIS2_PLACEMENT_3D('',#144982,#87824,#87825);
#75798=AXIS2_PLACEMENT_3D('',#144983,#87826,#87827);
#75799=AXIS2_PLACEMENT_3D('',#144999,#87829,#87830);
#75800=AXIS2_PLACEMENT_3D('',#145007,#87832,#87833);
#75801=AXIS2_PLACEMENT_3D('',#145009,#87834,#87835);
#75802=AXIS2_PLACEMENT_3D('',#145011,#87836,#87837);
#75803=AXIS2_PLACEMENT_3D('',#145012,#87838,#87839);
#75804=AXIS2_PLACEMENT_3D('',#145048,#87843,#87844);
#75805=AXIS2_PLACEMENT_3D('',#145056,#87846,#87847);
#75806=AXIS2_PLACEMENT_3D('',#145058,#87848,#87849);
#75807=AXIS2_PLACEMENT_3D('',#145060,#87850,#87851);
#75808=AXIS2_PLACEMENT_3D('',#145061,#87852,#87853);
#75809=AXIS2_PLACEMENT_3D('',#145077,#87855,#87856);
#75810=AXIS2_PLACEMENT_3D('',#145085,#87858,#87859);
#75811=AXIS2_PLACEMENT_3D('',#145087,#87860,#87861);
#75812=AXIS2_PLACEMENT_3D('',#145089,#87862,#87863);
#75813=AXIS2_PLACEMENT_3D('',#145090,#87864,#87865);
#75814=AXIS2_PLACEMENT_3D('',#145106,#87867,#87868);
#75815=AXIS2_PLACEMENT_3D('',#145114,#87870,#87871);
#75816=AXIS2_PLACEMENT_3D('',#145116,#87872,#87873);
#75817=AXIS2_PLACEMENT_3D('',#145118,#87874,#87875);
#75818=AXIS2_PLACEMENT_3D('',#145119,#87876,#87877);
#75819=AXIS2_PLACEMENT_3D('',#145135,#87879,#87880);
#75820=AXIS2_PLACEMENT_3D('',#145143,#87882,#87883);
#75821=AXIS2_PLACEMENT_3D('',#145145,#87884,#87885);
#75822=AXIS2_PLACEMENT_3D('',#145147,#87886,#87887);
#75823=AXIS2_PLACEMENT_3D('',#145148,#87888,#87889);
#75824=AXIS2_PLACEMENT_3D('',#145164,#87891,#87892);
#75825=AXIS2_PLACEMENT_3D('',#145172,#87894,#87895);
#75826=AXIS2_PLACEMENT_3D('',#145174,#87896,#87897);
#75827=AXIS2_PLACEMENT_3D('',#145176,#87898,#87899);
#75828=AXIS2_PLACEMENT_3D('',#145177,#87900,#87901);
#75829=AXIS2_PLACEMENT_3D('',#145193,#87903,#87904);
#75830=AXIS2_PLACEMENT_3D('',#145201,#87906,#87907);
#75831=AXIS2_PLACEMENT_3D('',#145203,#87908,#87909);
#75832=AXIS2_PLACEMENT_3D('',#145205,#87910,#87911);
#75833=AXIS2_PLACEMENT_3D('',#145206,#87912,#87913);
#75834=AXIS2_PLACEMENT_3D('',#145222,#87915,#87916);
#75835=AXIS2_PLACEMENT_3D('',#145230,#87918,#87919);
#75836=AXIS2_PLACEMENT_3D('',#145232,#87920,#87921);
#75837=AXIS2_PLACEMENT_3D('',#145234,#87922,#87923);
#75838=AXIS2_PLACEMENT_3D('',#145235,#87924,#87925);
#75839=AXIS2_PLACEMENT_3D('',#145251,#87927,#87928);
#75840=AXIS2_PLACEMENT_3D('',#145259,#87930,#87931);
#75841=AXIS2_PLACEMENT_3D('',#145261,#87932,#87933);
#75842=AXIS2_PLACEMENT_3D('',#145263,#87934,#87935);
#75843=AXIS2_PLACEMENT_3D('',#145264,#87936,#87937);
#75844=AXIS2_PLACEMENT_3D('',#145280,#87939,#87940);
#75845=AXIS2_PLACEMENT_3D('',#145288,#87942,#87943);
#75846=AXIS2_PLACEMENT_3D('',#145290,#87944,#87945);
#75847=AXIS2_PLACEMENT_3D('',#145292,#87946,#87947);
#75848=AXIS2_PLACEMENT_3D('',#145293,#87948,#87949);
#75849=AXIS2_PLACEMENT_3D('',#145309,#87951,#87952);
#75850=AXIS2_PLACEMENT_3D('',#145317,#87954,#87955);
#75851=AXIS2_PLACEMENT_3D('',#145319,#87956,#87957);
#75852=AXIS2_PLACEMENT_3D('',#145321,#87958,#87959);
#75853=AXIS2_PLACEMENT_3D('',#145322,#87960,#87961);
#75854=AXIS2_PLACEMENT_3D('',#145338,#87963,#87964);
#75855=AXIS2_PLACEMENT_3D('',#145346,#87966,#87967);
#75856=AXIS2_PLACEMENT_3D('',#145348,#87968,#87969);
#75857=AXIS2_PLACEMENT_3D('',#145350,#87970,#87971);
#75858=AXIS2_PLACEMENT_3D('',#145351,#87972,#87973);
#75859=AXIS2_PLACEMENT_3D('',#145367,#87975,#87976);
#75860=AXIS2_PLACEMENT_3D('',#145382,#87978,#87979);
#75861=AXIS2_PLACEMENT_3D('',#145384,#87981,#87982);
#75862=AXIS2_PLACEMENT_3D('',#145386,#87983,#87984);
#75863=AXIS2_PLACEMENT_3D('',#145387,#87985,#87986);
#75864=AXIS2_PLACEMENT_3D('',#145397,#87988,#87989);
#75865=AXIS2_PLACEMENT_3D('',#145404,#87990,#87991);
#75866=AXIS2_PLACEMENT_3D('',#145406,#87992,#87993);
#75867=AXIS2_PLACEMENT_3D('',#145408,#87994,#87995);
#75868=AXIS2_PLACEMENT_3D('',#145409,#87996,#87997);
#75869=AXIS2_PLACEMENT_3D('',#145425,#87999,#88000);
#75870=AXIS2_PLACEMENT_3D('',#145433,#88002,#88003);
#75871=AXIS2_PLACEMENT_3D('',#145435,#88004,#88005);
#75872=AXIS2_PLACEMENT_3D('',#145437,#88006,#88007);
#75873=AXIS2_PLACEMENT_3D('',#145438,#88008,#88009);
#75874=AXIS2_PLACEMENT_3D('',#145454,#88011,#88012);
#75875=AXIS2_PLACEMENT_3D('',#145462,#88014,#88015);
#75876=AXIS2_PLACEMENT_3D('',#145464,#88016,#88017);
#75877=AXIS2_PLACEMENT_3D('',#145466,#88018,#88019);
#75878=AXIS2_PLACEMENT_3D('',#145467,#88020,#88021);
#75879=AXIS2_PLACEMENT_3D('',#145483,#88023,#88024);
#75880=AXIS2_PLACEMENT_3D('',#145491,#88026,#88027);
#75881=AXIS2_PLACEMENT_3D('',#145493,#88028,#88029);
#75882=AXIS2_PLACEMENT_3D('',#145495,#88030,#88031);
#75883=AXIS2_PLACEMENT_3D('',#145496,#88032,#88033);
#75884=AXIS2_PLACEMENT_3D('',#145512,#88035,#88036);
#75885=AXIS2_PLACEMENT_3D('',#145520,#88038,#88039);
#75886=AXIS2_PLACEMENT_3D('',#145522,#88040,#88041);
#75887=AXIS2_PLACEMENT_3D('',#145524,#88042,#88043);
#75888=AXIS2_PLACEMENT_3D('',#145525,#88044,#88045);
#75889=AXIS2_PLACEMENT_3D('',#145541,#88047,#88048);
#75890=AXIS2_PLACEMENT_3D('',#145549,#88050,#88051);
#75891=AXIS2_PLACEMENT_3D('',#145551,#88052,#88053);
#75892=AXIS2_PLACEMENT_3D('',#145553,#88054,#88055);
#75893=AXIS2_PLACEMENT_3D('',#145554,#88056,#88057);
#75894=AXIS2_PLACEMENT_3D('',#145570,#88059,#88060);
#75895=AXIS2_PLACEMENT_3D('',#145578,#88062,#88063);
#75896=AXIS2_PLACEMENT_3D('',#145580,#88064,#88065);
#75897=AXIS2_PLACEMENT_3D('',#145582,#88066,#88067);
#75898=AXIS2_PLACEMENT_3D('',#145583,#88068,#88069);
#75899=AXIS2_PLACEMENT_3D('',#145599,#88071,#88072);
#75900=AXIS2_PLACEMENT_3D('',#145607,#88074,#88075);
#75901=AXIS2_PLACEMENT_3D('',#145609,#88076,#88077);
#75902=AXIS2_PLACEMENT_3D('',#145611,#88078,#88079);
#75903=AXIS2_PLACEMENT_3D('',#145612,#88080,#88081);
#75904=AXIS2_PLACEMENT_3D('',#145628,#88083,#88084);
#75905=AXIS2_PLACEMENT_3D('',#145636,#88086,#88087);
#75906=AXIS2_PLACEMENT_3D('',#145638,#88088,#88089);
#75907=AXIS2_PLACEMENT_3D('',#145640,#88090,#88091);
#75908=AXIS2_PLACEMENT_3D('',#145641,#88092,#88093);
#75909=AXIS2_PLACEMENT_3D('',#145649,#88095,#88096);
#75910=AXIS2_PLACEMENT_3D('',#145652,#88097,#88098);
#75911=AXIS2_PLACEMENT_3D('',#145653,#88099,#88100);
#75912=AXIS2_PLACEMENT_3D('',#145654,#88101,#88102);
#75913=AXIS2_PLACEMENT_3D('',#145676,#88104,#88105);
#75914=AXIS2_PLACEMENT_3D('',#145691,#88108,#88109);
#75915=AXIS2_PLACEMENT_3D('',#145705,#88110,#88111);
#75916=AXIS2_PLACEMENT_3D('',#145707,#88113,#88114);
#75917=AXIS2_PLACEMENT_3D('',#145709,#88115,#88116);
#75918=AXIS2_PLACEMENT_3D('',#145710,#88117,#88118);
#75919=AXIS2_PLACEMENT_3D('',#145724,#88120,#88121);
#75920=AXIS2_PLACEMENT_3D('',#145738,#88122,#88123);
#75921=AXIS2_PLACEMENT_3D('',#145740,#88125,#88126);
#75922=AXIS2_PLACEMENT_3D('',#145742,#88127,#88128);
#75923=AXIS2_PLACEMENT_3D('',#145743,#88129,#88130);
#75924=AXIS2_PLACEMENT_3D('',#145757,#88132,#88133);
#75925=AXIS2_PLACEMENT_3D('',#145771,#88134,#88135);
#75926=AXIS2_PLACEMENT_3D('',#145773,#88137,#88138);
#75927=AXIS2_PLACEMENT_3D('',#145775,#88139,#88140);
#75928=AXIS2_PLACEMENT_3D('',#145776,#88141,#88142);
#75929=AXIS2_PLACEMENT_3D('',#145790,#88144,#88145);
#75930=AXIS2_PLACEMENT_3D('',#145804,#88146,#88147);
#75931=AXIS2_PLACEMENT_3D('',#145806,#88149,#88150);
#75932=AXIS2_PLACEMENT_3D('',#145808,#88151,#88152);
#75933=AXIS2_PLACEMENT_3D('',#145809,#88153,#88154);
#75934=AXIS2_PLACEMENT_3D('',#145823,#88156,#88157);
#75935=AXIS2_PLACEMENT_3D('',#145837,#88158,#88159);
#75936=AXIS2_PLACEMENT_3D('',#145839,#88161,#88162);
#75937=AXIS2_PLACEMENT_3D('',#145841,#88163,#88164);
#75938=AXIS2_PLACEMENT_3D('',#145842,#88165,#88166);
#75939=AXIS2_PLACEMENT_3D('',#145856,#88168,#88169);
#75940=AXIS2_PLACEMENT_3D('',#145870,#88170,#88171);
#75941=AXIS2_PLACEMENT_3D('',#145872,#88173,#88174);
#75942=AXIS2_PLACEMENT_3D('',#145874,#88175,#88176);
#75943=AXIS2_PLACEMENT_3D('',#145875,#88177,#88178);
#75944=AXIS2_PLACEMENT_3D('',#145889,#88180,#88181);
#75945=AXIS2_PLACEMENT_3D('',#145903,#88182,#88183);
#75946=AXIS2_PLACEMENT_3D('',#145905,#88185,#88186);
#75947=AXIS2_PLACEMENT_3D('',#145907,#88187,#88188);
#75948=AXIS2_PLACEMENT_3D('',#145908,#88189,#88190);
#75949=AXIS2_PLACEMENT_3D('',#145922,#88192,#88193);
#75950=AXIS2_PLACEMENT_3D('',#145936,#88194,#88195);
#75951=AXIS2_PLACEMENT_3D('',#145938,#88197,#88198);
#75952=AXIS2_PLACEMENT_3D('',#145940,#88199,#88200);
#75953=AXIS2_PLACEMENT_3D('',#145941,#88201,#88202);
#75954=AXIS2_PLACEMENT_3D('',#145955,#88204,#88205);
#75955=AXIS2_PLACEMENT_3D('',#145969,#88206,#88207);
#75956=AXIS2_PLACEMENT_3D('',#145971,#88209,#88210);
#75957=AXIS2_PLACEMENT_3D('',#145973,#88211,#88212);
#75958=AXIS2_PLACEMENT_3D('',#145974,#88213,#88214);
#75959=AXIS2_PLACEMENT_3D('',#145988,#88216,#88217);
#75960=AXIS2_PLACEMENT_3D('',#146002,#88218,#88219);
#75961=AXIS2_PLACEMENT_3D('',#146004,#88221,#88222);
#75962=AXIS2_PLACEMENT_3D('',#146006,#88223,#88224);
#75963=AXIS2_PLACEMENT_3D('',#146007,#88225,#88226);
#75964=AXIS2_PLACEMENT_3D('',#146021,#88228,#88229);
#75965=AXIS2_PLACEMENT_3D('',#146035,#88230,#88231);
#75966=AXIS2_PLACEMENT_3D('',#146037,#88233,#88234);
#75967=AXIS2_PLACEMENT_3D('',#146039,#88235,#88236);
#75968=AXIS2_PLACEMENT_3D('',#146040,#88237,#88238);
#75969=AXIS2_PLACEMENT_3D('',#146054,#88240,#88241);
#75970=AXIS2_PLACEMENT_3D('',#146068,#88242,#88243);
#75971=AXIS2_PLACEMENT_3D('',#146070,#88245,#88246);
#75972=AXIS2_PLACEMENT_3D('',#146072,#88247,#88248);
#75973=AXIS2_PLACEMENT_3D('',#146073,#88249,#88250);
#75974=AXIS2_PLACEMENT_3D('',#146087,#88252,#88253);
#75975=AXIS2_PLACEMENT_3D('',#146101,#88254,#88255);
#75976=AXIS2_PLACEMENT_3D('',#146103,#88257,#88258);
#75977=AXIS2_PLACEMENT_3D('',#146105,#88259,#88260);
#75978=AXIS2_PLACEMENT_3D('',#146106,#88261,#88262);
#75979=AXIS2_PLACEMENT_3D('',#146144,#88266,#88267);
#75980=AXIS2_PLACEMENT_3D('',#146158,#88268,#88269);
#75981=AXIS2_PLACEMENT_3D('',#146160,#88271,#88272);
#75982=AXIS2_PLACEMENT_3D('',#146162,#88273,#88274);
#75983=AXIS2_PLACEMENT_3D('',#146163,#88275,#88276);
#75984=AXIS2_PLACEMENT_3D('',#146177,#88278,#88279);
#75985=AXIS2_PLACEMENT_3D('',#146191,#88280,#88281);
#75986=AXIS2_PLACEMENT_3D('',#146193,#88283,#88284);
#75987=AXIS2_PLACEMENT_3D('',#146195,#88285,#88286);
#75988=AXIS2_PLACEMENT_3D('',#146196,#88287,#88288);
#75989=AXIS2_PLACEMENT_3D('',#146210,#88290,#88291);
#75990=AXIS2_PLACEMENT_3D('',#146224,#88292,#88293);
#75991=AXIS2_PLACEMENT_3D('',#146226,#88295,#88296);
#75992=AXIS2_PLACEMENT_3D('',#146228,#88297,#88298);
#75993=AXIS2_PLACEMENT_3D('',#146229,#88299,#88300);
#75994=AXIS2_PLACEMENT_3D('',#146243,#88302,#88303);
#75995=AXIS2_PLACEMENT_3D('',#146257,#88304,#88305);
#75996=AXIS2_PLACEMENT_3D('',#146259,#88307,#88308);
#75997=AXIS2_PLACEMENT_3D('',#146261,#88309,#88310);
#75998=AXIS2_PLACEMENT_3D('',#146262,#88311,#88312);
#75999=AXIS2_PLACEMENT_3D('',#146276,#88314,#88315);
#76000=AXIS2_PLACEMENT_3D('',#146290,#88316,#88317);
#76001=AXIS2_PLACEMENT_3D('',#146292,#88319,#88320);
#76002=AXIS2_PLACEMENT_3D('',#146294,#88321,#88322);
#76003=AXIS2_PLACEMENT_3D('',#146295,#88323,#88324);
#76004=AXIS2_PLACEMENT_3D('',#146309,#88326,#88327);
#76005=AXIS2_PLACEMENT_3D('',#146323,#88328,#88329);
#76006=AXIS2_PLACEMENT_3D('',#146325,#88331,#88332);
#76007=AXIS2_PLACEMENT_3D('',#146327,#88333,#88334);
#76008=AXIS2_PLACEMENT_3D('',#146328,#88335,#88336);
#76009=AXIS2_PLACEMENT_3D('',#146342,#88338,#88339);
#76010=AXIS2_PLACEMENT_3D('',#146356,#88340,#88341);
#76011=AXIS2_PLACEMENT_3D('',#146358,#88343,#88344);
#76012=AXIS2_PLACEMENT_3D('',#146360,#88345,#88346);
#76013=AXIS2_PLACEMENT_3D('',#146361,#88347,#88348);
#76014=AXIS2_PLACEMENT_3D('',#146375,#88350,#88351);
#76015=AXIS2_PLACEMENT_3D('',#146389,#88352,#88353);
#76016=AXIS2_PLACEMENT_3D('',#146391,#88355,#88356);
#76017=AXIS2_PLACEMENT_3D('',#146393,#88357,#88358);
#76018=AXIS2_PLACEMENT_3D('',#146394,#88359,#88360);
#76019=AXIS2_PLACEMENT_3D('',#146408,#88362,#88363);
#76020=AXIS2_PLACEMENT_3D('',#146422,#88364,#88365);
#76021=AXIS2_PLACEMENT_3D('',#146424,#88367,#88368);
#76022=AXIS2_PLACEMENT_3D('',#146426,#88369,#88370);
#76023=AXIS2_PLACEMENT_3D('',#146427,#88371,#88372);
#76024=AXIS2_PLACEMENT_3D('',#146441,#88374,#88375);
#76025=AXIS2_PLACEMENT_3D('',#146455,#88376,#88377);
#76026=AXIS2_PLACEMENT_3D('',#146457,#88379,#88380);
#76027=AXIS2_PLACEMENT_3D('',#146459,#88381,#88382);
#76028=AXIS2_PLACEMENT_3D('',#146460,#88383,#88384);
#76029=AXIS2_PLACEMENT_3D('',#146474,#88386,#88387);
#76030=AXIS2_PLACEMENT_3D('',#146488,#88388,#88389);
#76031=AXIS2_PLACEMENT_3D('',#146490,#88391,#88392);
#76032=AXIS2_PLACEMENT_3D('',#146492,#88393,#88394);
#76033=AXIS2_PLACEMENT_3D('',#146493,#88395,#88396);
#76034=AXIS2_PLACEMENT_3D('',#146507,#88398,#88399);
#76035=AXIS2_PLACEMENT_3D('',#146521,#88400,#88401);
#76036=AXIS2_PLACEMENT_3D('',#146523,#88403,#88404);
#76037=AXIS2_PLACEMENT_3D('',#146525,#88405,#88406);
#76038=AXIS2_PLACEMENT_3D('',#146526,#88407,#88408);
#76039=AXIS2_PLACEMENT_3D('',#146540,#88410,#88411);
#76040=AXIS2_PLACEMENT_3D('',#146554,#88412,#88413);
#76041=AXIS2_PLACEMENT_3D('',#146556,#88415,#88416);
#76042=AXIS2_PLACEMENT_3D('',#146558,#88417,#88418);
#76043=AXIS2_PLACEMENT_3D('',#146559,#88419,#88420);
#76044=AXIS2_PLACEMENT_3D('',#146573,#88422,#88423);
#76045=AXIS2_PLACEMENT_3D('',#146587,#88424,#88425);
#76046=AXIS2_PLACEMENT_3D('',#146589,#88427,#88428);
#76047=AXIS2_PLACEMENT_3D('',#146591,#88429,#88430);
#76048=AXIS2_PLACEMENT_3D('',#146592,#88431,#88432);
#76049=AXIS2_PLACEMENT_3D('',#146593,#88433,#88434);
#76050=AXIS2_PLACEMENT_3D('',#146595,#88435,#88436);
#76051=AXIS2_PLACEMENT_3D('',#146597,#88437,#88438);
#76052=AXIS2_PLACEMENT_3D('',#146598,#88439,#88440);
#76053=AXIS2_PLACEMENT_3D('',#146621,#88442,#88443);
#76054=AXIS2_PLACEMENT_3D('',#146680,#88444,#88445);
#76055=AXIS2_PLACEMENT_3D('',#146721,#88446,#88447);
#76056=AXIS2_PLACEMENT_3D('',#146771,#88448,#88449);
#76057=AXIS2_PLACEMENT_3D('',#146812,#88450,#88451);
#76058=AXIS2_PLACEMENT_3D('',#146853,#88452,#88453);
#76059=AXIS2_PLACEMENT_3D('',#146903,#88454,#88455);
#76060=AXIS2_PLACEMENT_3D('',#146953,#88456,#88457);
#76061=AXIS2_PLACEMENT_3D('',#147002,#88458,#88459);
#76062=AXIS2_PLACEMENT_3D('',#147051,#88460,#88461);
#76063=AXIS2_PLACEMENT_3D('',#147101,#88462,#88463);
#76064=AXIS2_PLACEMENT_3D('',#147142,#88464,#88465);
#76065=AXIS2_PLACEMENT_3D('',#147192,#88466,#88467);
#76066=AXIS2_PLACEMENT_3D('',#147236,#88468,#88469);
#76067=AXIS2_PLACEMENT_3D('',#147282,#88470,#88471);
#76068=AXIS2_PLACEMENT_3D('',#147332,#88472,#88473);
#76069=AXIS2_PLACEMENT_3D('',#147378,#88474,#88475);
#76070=AXIS2_PLACEMENT_3D('',#147419,#88476,#88477);
#76071=AXIS2_PLACEMENT_3D('',#147465,#88478,#88479);
#76072=AXIS2_PLACEMENT_3D('',#147515,#88480,#88481);
#76073=AXIS2_PLACEMENT_3D('',#147561,#88482,#88483);
#76074=AXIS2_PLACEMENT_3D('',#147607,#88484,#88485);
#76075=AXIS2_PLACEMENT_3D('',#147657,#88486,#88487);
#76076=AXIS2_PLACEMENT_3D('',#147703,#88488,#88489);
#76077=AXIS2_PLACEMENT_3D('',#147753,#88490,#88491);
#76078=AXIS2_PLACEMENT_3D('',#147802,#88492,#88493);
#76079=AXIS2_PLACEMENT_3D('',#147852,#88494,#88495);
#76080=AXIS2_PLACEMENT_3D('',#147898,#88496,#88497);
#76081=AXIS2_PLACEMENT_3D('',#147948,#88498,#88499);
#76082=AXIS2_PLACEMENT_3D('',#147990,#88500,#88501);
#76083=AXIS2_PLACEMENT_3D('',#148002,#88502,#88503);
#76084=AXIS2_PLACEMENT_3D('',#148015,#88504,#88505);
#76085=AXIS2_PLACEMENT_3D('',#148027,#88506,#88507);
#76086=AXIS2_PLACEMENT_3D('',#148040,#88508,#88509);
#76087=AXIS2_PLACEMENT_3D('',#148052,#88510,#88511);
#76088=AXIS2_PLACEMENT_3D('',#148065,#88512,#88513);
#76089=AXIS2_PLACEMENT_3D('',#148077,#88514,#88515);
#76090=AXIS2_PLACEMENT_3D('',#148090,#88516,#88517);
#76091=AXIS2_PLACEMENT_3D('',#148102,#88518,#88519);
#76092=AXIS2_PLACEMENT_3D('',#148115,#88520,#88521);
#76093=AXIS2_PLACEMENT_3D('',#148127,#88522,#88523);
#76094=AXIS2_PLACEMENT_3D('',#148140,#88524,#88525);
#76095=AXIS2_PLACEMENT_3D('',#148152,#88526,#88527);
#76096=AXIS2_PLACEMENT_3D('',#148165,#88528,#88529);
#76097=AXIS2_PLACEMENT_3D('',#148177,#88530,#88531);
#76098=AXIS2_PLACEMENT_3D('',#148190,#88532,#88533);
#76099=AXIS2_PLACEMENT_3D('',#148202,#88534,#88535);
#76100=AXIS2_PLACEMENT_3D('',#148215,#88536,#88537);
#76101=AXIS2_PLACEMENT_3D('',#148227,#88538,#88539);
#76102=AXIS2_PLACEMENT_3D('',#148240,#88540,#88541);
#76103=AXIS2_PLACEMENT_3D('',#148252,#88542,#88543);
#76104=AXIS2_PLACEMENT_3D('',#148265,#88544,#88545);
#76105=AXIS2_PLACEMENT_3D('',#148277,#88546,#88547);
#76106=AXIS2_PLACEMENT_3D('',#148290,#88548,#88549);
#76107=AXIS2_PLACEMENT_3D('',#148302,#88550,#88551);
#76108=AXIS2_PLACEMENT_3D('',#148315,#88552,#88553);
#76109=AXIS2_PLACEMENT_3D('',#148327,#88554,#88555);
#76110=AXIS2_PLACEMENT_3D('',#148340,#88556,#88557);
#76111=AXIS2_PLACEMENT_3D('',#148352,#88558,#88559);
#76112=AXIS2_PLACEMENT_3D('',#148365,#88560,#88561);
#76113=AXIS2_PLACEMENT_3D('',#148377,#88562,#88563);
#76114=AXIS2_PLACEMENT_3D('',#148390,#88564,#88565);
#76115=AXIS2_PLACEMENT_3D('',#148402,#88566,#88567);
#76116=AXIS2_PLACEMENT_3D('',#148415,#88568,#88569);
#76117=AXIS2_PLACEMENT_3D('',#148427,#88570,#88571);
#76118=AXIS2_PLACEMENT_3D('',#148440,#88572,#88573);
#76119=AXIS2_PLACEMENT_3D('',#148452,#88574,#88575);
#76120=AXIS2_PLACEMENT_3D('',#148465,#88576,#88577);
#76121=AXIS2_PLACEMENT_3D('',#148477,#88578,#88579);
#76122=AXIS2_PLACEMENT_3D('',#148490,#88580,#88581);
#76123=AXIS2_PLACEMENT_3D('',#148502,#88582,#88583);
#76124=AXIS2_PLACEMENT_3D('',#148515,#88584,#88585);
#76125=AXIS2_PLACEMENT_3D('',#148527,#88586,#88587);
#76126=AXIS2_PLACEMENT_3D('',#148540,#88588,#88589);
#76127=AXIS2_PLACEMENT_3D('',#148552,#88590,#88591);
#76128=AXIS2_PLACEMENT_3D('',#148565,#88592,#88593);
#76129=AXIS2_PLACEMENT_3D('',#148577,#88594,#88595);
#76130=AXIS2_PLACEMENT_3D('',#148590,#88596,#88597);
#76131=AXIS2_PLACEMENT_3D('',#148602,#88598,#88599);
#76132=AXIS2_PLACEMENT_3D('',#148615,#88600,#88601);
#76133=AXIS2_PLACEMENT_3D('',#148627,#88602,#88603);
#76134=AXIS2_PLACEMENT_3D('',#148640,#88604,#88605);
#76135=AXIS2_PLACEMENT_3D('',#148652,#88606,#88607);
#76136=AXIS2_PLACEMENT_3D('',#148665,#88608,#88609);
#76137=AXIS2_PLACEMENT_3D('',#148677,#88610,#88611);
#76138=AXIS2_PLACEMENT_3D('',#148690,#88612,#88613);
#76139=AXIS2_PLACEMENT_3D('',#148701,#88614,#88615);
#76140=AXIS2_PLACEMENT_3D('',#148714,#88616,#88617);
#76141=AXIS2_PLACEMENT_3D('',#148722,#88619,#88620);
#76142=AXIS2_PLACEMENT_3D('',#148724,#88621,#88622);
#76143=AXIS2_PLACEMENT_3D('',#148726,#88623,#88624);
#76144=AXIS2_PLACEMENT_3D('',#148757,#88626,#88627);
#76145=AXIS2_PLACEMENT_3D('',#148765,#88629,#88630);
#76146=AXIS2_PLACEMENT_3D('',#148767,#88631,#88632);
#76147=AXIS2_PLACEMENT_3D('',#148769,#88633,#88634);
#76148=AXIS2_PLACEMENT_3D('',#148800,#88636,#88637);
#76149=AXIS2_PLACEMENT_3D('',#148808,#88639,#88640);
#76150=AXIS2_PLACEMENT_3D('',#148810,#88641,#88642);
#76151=AXIS2_PLACEMENT_3D('',#148812,#88643,#88644);
#76152=AXIS2_PLACEMENT_3D('',#148843,#88646,#88647);
#76153=AXIS2_PLACEMENT_3D('',#148851,#88649,#88650);
#76154=AXIS2_PLACEMENT_3D('',#148853,#88651,#88652);
#76155=AXIS2_PLACEMENT_3D('',#148855,#88653,#88654);
#76156=AXIS2_PLACEMENT_3D('',#148886,#88656,#88657);
#76157=AXIS2_PLACEMENT_3D('',#148894,#88659,#88660);
#76158=AXIS2_PLACEMENT_3D('',#148896,#88661,#88662);
#76159=AXIS2_PLACEMENT_3D('',#148898,#88663,#88664);
#76160=AXIS2_PLACEMENT_3D('',#148929,#88666,#88667);
#76161=AXIS2_PLACEMENT_3D('',#148937,#88669,#88670);
#76162=AXIS2_PLACEMENT_3D('',#148939,#88671,#88672);
#76163=AXIS2_PLACEMENT_3D('',#148941,#88673,#88674);
#76164=AXIS2_PLACEMENT_3D('',#148972,#88676,#88677);
#76165=AXIS2_PLACEMENT_3D('',#148980,#88679,#88680);
#76166=AXIS2_PLACEMENT_3D('',#148982,#88681,#88682);
#76167=AXIS2_PLACEMENT_3D('',#148984,#88683,#88684);
#76168=AXIS2_PLACEMENT_3D('',#149015,#88686,#88687);
#76169=AXIS2_PLACEMENT_3D('',#149023,#88689,#88690);
#76170=AXIS2_PLACEMENT_3D('',#149025,#88691,#88692);
#76171=AXIS2_PLACEMENT_3D('',#149027,#88693,#88694);
#76172=AXIS2_PLACEMENT_3D('',#149058,#88696,#88697);
#76173=AXIS2_PLACEMENT_3D('',#149066,#88699,#88700);
#76174=AXIS2_PLACEMENT_3D('',#149068,#88701,#88702);
#76175=AXIS2_PLACEMENT_3D('',#149070,#88703,#88704);
#76176=AXIS2_PLACEMENT_3D('',#149101,#88706,#88707);
#76177=AXIS2_PLACEMENT_3D('',#149109,#88709,#88710);
#76178=AXIS2_PLACEMENT_3D('',#149111,#88711,#88712);
#76179=AXIS2_PLACEMENT_3D('',#149113,#88713,#88714);
#76180=AXIS2_PLACEMENT_3D('',#149144,#88716,#88717);
#76181=AXIS2_PLACEMENT_3D('',#149152,#88719,#88720);
#76182=AXIS2_PLACEMENT_3D('',#149154,#88721,#88722);
#76183=AXIS2_PLACEMENT_3D('',#149156,#88723,#88724);
#76184=AXIS2_PLACEMENT_3D('',#149187,#88726,#88727);
#76185=AXIS2_PLACEMENT_3D('',#149195,#88729,#88730);
#76186=AXIS2_PLACEMENT_3D('',#149197,#88731,#88732);
#76187=AXIS2_PLACEMENT_3D('',#149199,#88733,#88734);
#76188=AXIS2_PLACEMENT_3D('',#149230,#88736,#88737);
#76189=AXIS2_PLACEMENT_3D('',#149238,#88739,#88740);
#76190=AXIS2_PLACEMENT_3D('',#149240,#88741,#88742);
#76191=AXIS2_PLACEMENT_3D('',#149242,#88743,#88744);
#76192=AXIS2_PLACEMENT_3D('',#149273,#88746,#88747);
#76193=AXIS2_PLACEMENT_3D('',#149281,#88749,#88750);
#76194=AXIS2_PLACEMENT_3D('',#149283,#88751,#88752);
#76195=AXIS2_PLACEMENT_3D('',#149285,#88753,#88754);
#76196=AXIS2_PLACEMENT_3D('',#149344,#88758,#88759);
#76197=AXIS2_PLACEMENT_3D('',#149352,#88761,#88762);
#76198=AXIS2_PLACEMENT_3D('',#149354,#88763,#88764);
#76199=AXIS2_PLACEMENT_3D('',#149356,#88765,#88766);
#76200=AXIS2_PLACEMENT_3D('',#149387,#88768,#88769);
#76201=AXIS2_PLACEMENT_3D('',#149395,#88771,#88772);
#76202=AXIS2_PLACEMENT_3D('',#149397,#88773,#88774);
#76203=AXIS2_PLACEMENT_3D('',#149399,#88775,#88776);
#76204=AXIS2_PLACEMENT_3D('',#149430,#88778,#88779);
#76205=AXIS2_PLACEMENT_3D('',#149438,#88781,#88782);
#76206=AXIS2_PLACEMENT_3D('',#149440,#88783,#88784);
#76207=AXIS2_PLACEMENT_3D('',#149442,#88785,#88786);
#76208=AXIS2_PLACEMENT_3D('',#149473,#88788,#88789);
#76209=AXIS2_PLACEMENT_3D('',#149500,#88792,#88793);
#76210=AXIS2_PLACEMENT_3D('',#149502,#88794,#88795);
#76211=AXIS2_PLACEMENT_3D('',#149503,#88796,#88797);
#76212=AXIS2_PLACEMENT_3D('',#149517,#88799,#88800);
#76213=AXIS2_PLACEMENT_3D('',#149524,#88801,#88802);
#76214=AXIS2_PLACEMENT_3D('',#149534,#88803,#88804);
#76215=AXIS2_PLACEMENT_3D('',#149535,#88805,#88806);
#76216=AXIS2_PLACEMENT_3D('',#149559,#88808,#88809);
#76217=AXIS2_PLACEMENT_3D('',#149567,#88811,#88812);
#76218=AXIS2_PLACEMENT_3D('',#149569,#88813,#88814);
#76219=AXIS2_PLACEMENT_3D('',#149571,#88815,#88816);
#76220=AXIS2_PLACEMENT_3D('',#149602,#88818,#88819);
#76221=AXIS2_PLACEMENT_3D('',#149610,#88821,#88822);
#76222=AXIS2_PLACEMENT_3D('',#149612,#88823,#88824);
#76223=AXIS2_PLACEMENT_3D('',#149614,#88825,#88826);
#76224=AXIS2_PLACEMENT_3D('',#149645,#88828,#88829);
#76225=AXIS2_PLACEMENT_3D('',#149653,#88831,#88832);
#76226=AXIS2_PLACEMENT_3D('',#149655,#88833,#88834);
#76227=AXIS2_PLACEMENT_3D('',#149657,#88835,#88836);
#76228=AXIS2_PLACEMENT_3D('',#149688,#88838,#88839);
#76229=AXIS2_PLACEMENT_3D('',#149696,#88841,#88842);
#76230=AXIS2_PLACEMENT_3D('',#149698,#88843,#88844);
#76231=AXIS2_PLACEMENT_3D('',#149700,#88845,#88846);
#76232=AXIS2_PLACEMENT_3D('',#149731,#88848,#88849);
#76233=AXIS2_PLACEMENT_3D('',#149739,#88851,#88852);
#76234=AXIS2_PLACEMENT_3D('',#149741,#88853,#88854);
#76235=AXIS2_PLACEMENT_3D('',#149743,#88855,#88856);
#76236=AXIS2_PLACEMENT_3D('',#149774,#88858,#88859);
#76237=AXIS2_PLACEMENT_3D('',#149782,#88861,#88862);
#76238=AXIS2_PLACEMENT_3D('',#149784,#88863,#88864);
#76239=AXIS2_PLACEMENT_3D('',#149786,#88865,#88866);
#76240=AXIS2_PLACEMENT_3D('',#149817,#88868,#88869);
#76241=AXIS2_PLACEMENT_3D('',#149825,#88871,#88872);
#76242=AXIS2_PLACEMENT_3D('',#149827,#88873,#88874);
#76243=AXIS2_PLACEMENT_3D('',#149829,#88875,#88876);
#76244=AXIS2_PLACEMENT_3D('',#149860,#88878,#88879);
#76245=AXIS2_PLACEMENT_3D('',#149868,#88881,#88882);
#76246=AXIS2_PLACEMENT_3D('',#149870,#88883,#88884);
#76247=AXIS2_PLACEMENT_3D('',#149872,#88885,#88886);
#76248=AXIS2_PLACEMENT_3D('',#149903,#88888,#88889);
#76249=AXIS2_PLACEMENT_3D('',#149911,#88891,#88892);
#76250=AXIS2_PLACEMENT_3D('',#149913,#88893,#88894);
#76251=AXIS2_PLACEMENT_3D('',#149915,#88895,#88896);
#76252=AXIS2_PLACEMENT_3D('',#149947,#88899,#88900);
#76253=AXIS2_PLACEMENT_3D('',#149954,#88901,#88902);
#76254=AXIS2_PLACEMENT_3D('',#149957,#88903,#88904);
#76255=AXIS2_PLACEMENT_3D('',#149959,#88905,#88906);
#76256=AXIS2_PLACEMENT_3D('',#149960,#88907,#88908);
#76257=AXIS2_PLACEMENT_3D('',#149968,#88909,#88910);
#76258=AXIS2_PLACEMENT_3D('',#149970,#88912,#88913);
#76259=AXIS2_PLACEMENT_3D('',#149971,#88914,#88915);
#76260=AXIS2_PLACEMENT_3D('',#149972,#88916,#88917);
#76261=AXIS2_PLACEMENT_3D('',#149986,#88919,#88920);
#76262=AXIS2_PLACEMENT_3D('',#149993,#88921,#88922);
#76263=AXIS2_PLACEMENT_3D('',#149996,#88923,#88924);
#76264=AXIS2_PLACEMENT_3D('',#149998,#88925,#88926);
#76265=AXIS2_PLACEMENT_3D('',#149999,#88927,#88928);
#76266=AXIS2_PLACEMENT_3D('',#150007,#88929,#88930);
#76267=AXIS2_PLACEMENT_3D('',#150009,#88932,#88933);
#76268=AXIS2_PLACEMENT_3D('',#150010,#88934,#88935);
#76269=AXIS2_PLACEMENT_3D('',#150011,#88936,#88937);
#76270=AXIS2_PLACEMENT_3D('',#150025,#88939,#88940);
#76271=AXIS2_PLACEMENT_3D('',#150032,#88941,#88942);
#76272=AXIS2_PLACEMENT_3D('',#150035,#88943,#88944);
#76273=AXIS2_PLACEMENT_3D('',#150037,#88945,#88946);
#76274=AXIS2_PLACEMENT_3D('',#150038,#88947,#88948);
#76275=AXIS2_PLACEMENT_3D('',#150046,#88949,#88950);
#76276=AXIS2_PLACEMENT_3D('',#150048,#88952,#88953);
#76277=AXIS2_PLACEMENT_3D('',#150049,#88954,#88955);
#76278=AXIS2_PLACEMENT_3D('',#150050,#88956,#88957);
#76279=AXIS2_PLACEMENT_3D('',#150064,#88959,#88960);
#76280=AXIS2_PLACEMENT_3D('',#150071,#88961,#88962);
#76281=AXIS2_PLACEMENT_3D('',#150074,#88963,#88964);
#76282=AXIS2_PLACEMENT_3D('',#150076,#88965,#88966);
#76283=AXIS2_PLACEMENT_3D('',#150077,#88967,#88968);
#76284=AXIS2_PLACEMENT_3D('',#150085,#88969,#88970);
#76285=AXIS2_PLACEMENT_3D('',#150087,#88972,#88973);
#76286=AXIS2_PLACEMENT_3D('',#150088,#88974,#88975);
#76287=AXIS2_PLACEMENT_3D('',#150089,#88976,#88977);
#76288=AXIS2_PLACEMENT_3D('',#150103,#88979,#88980);
#76289=AXIS2_PLACEMENT_3D('',#150110,#88981,#88982);
#76290=AXIS2_PLACEMENT_3D('',#150113,#88983,#88984);
#76291=AXIS2_PLACEMENT_3D('',#150115,#88985,#88986);
#76292=AXIS2_PLACEMENT_3D('',#150116,#88987,#88988);
#76293=AXIS2_PLACEMENT_3D('',#150124,#88989,#88990);
#76294=AXIS2_PLACEMENT_3D('',#150126,#88992,#88993);
#76295=AXIS2_PLACEMENT_3D('',#150127,#88994,#88995);
#76296=AXIS2_PLACEMENT_3D('',#150128,#88996,#88997);
#76297=AXIS2_PLACEMENT_3D('',#150142,#88999,#89000);
#76298=AXIS2_PLACEMENT_3D('',#150149,#89001,#89002);
#76299=AXIS2_PLACEMENT_3D('',#150152,#89003,#89004);
#76300=AXIS2_PLACEMENT_3D('',#150154,#89005,#89006);
#76301=AXIS2_PLACEMENT_3D('',#150155,#89007,#89008);
#76302=AXIS2_PLACEMENT_3D('',#150163,#89009,#89010);
#76303=AXIS2_PLACEMENT_3D('',#150165,#89012,#89013);
#76304=AXIS2_PLACEMENT_3D('',#150166,#89014,#89015);
#76305=AXIS2_PLACEMENT_3D('',#150167,#89016,#89017);
#76306=AXIS2_PLACEMENT_3D('',#150181,#89019,#89020);
#76307=AXIS2_PLACEMENT_3D('',#150188,#89021,#89022);
#76308=AXIS2_PLACEMENT_3D('',#150191,#89023,#89024);
#76309=AXIS2_PLACEMENT_3D('',#150193,#89025,#89026);
#76310=AXIS2_PLACEMENT_3D('',#150194,#89027,#89028);
#76311=AXIS2_PLACEMENT_3D('',#150202,#89029,#89030);
#76312=AXIS2_PLACEMENT_3D('',#150204,#89032,#89033);
#76313=AXIS2_PLACEMENT_3D('',#150205,#89034,#89035);
#76314=AXIS2_PLACEMENT_3D('',#150206,#89036,#89037);
#76315=AXIS2_PLACEMENT_3D('',#150220,#89039,#89040);
#76316=AXIS2_PLACEMENT_3D('',#150227,#89041,#89042);
#76317=AXIS2_PLACEMENT_3D('',#150230,#89043,#89044);
#76318=AXIS2_PLACEMENT_3D('',#150232,#89045,#89046);
#76319=AXIS2_PLACEMENT_3D('',#150233,#89047,#89048);
#76320=AXIS2_PLACEMENT_3D('',#150241,#89049,#89050);
#76321=AXIS2_PLACEMENT_3D('',#150243,#89052,#89053);
#76322=AXIS2_PLACEMENT_3D('',#150244,#89054,#89055);
#76323=AXIS2_PLACEMENT_3D('',#150245,#89056,#89057);
#76324=AXIS2_PLACEMENT_3D('',#150259,#89059,#89060);
#76325=AXIS2_PLACEMENT_3D('',#150266,#89061,#89062);
#76326=AXIS2_PLACEMENT_3D('',#150269,#89063,#89064);
#76327=AXIS2_PLACEMENT_3D('',#150271,#89065,#89066);
#76328=AXIS2_PLACEMENT_3D('',#150272,#89067,#89068);
#76329=AXIS2_PLACEMENT_3D('',#150280,#89069,#89070);
#76330=AXIS2_PLACEMENT_3D('',#150282,#89072,#89073);
#76331=AXIS2_PLACEMENT_3D('',#150283,#89074,#89075);
#76332=AXIS2_PLACEMENT_3D('',#150284,#89076,#89077);
#76333=AXIS2_PLACEMENT_3D('',#150298,#89079,#89080);
#76334=AXIS2_PLACEMENT_3D('',#150305,#89081,#89082);
#76335=AXIS2_PLACEMENT_3D('',#150308,#89083,#89084);
#76336=AXIS2_PLACEMENT_3D('',#150310,#89085,#89086);
#76337=AXIS2_PLACEMENT_3D('',#150311,#89087,#89088);
#76338=AXIS2_PLACEMENT_3D('',#150319,#89089,#89090);
#76339=AXIS2_PLACEMENT_3D('',#150321,#89092,#89093);
#76340=AXIS2_PLACEMENT_3D('',#150322,#89094,#89095);
#76341=AXIS2_PLACEMENT_3D('',#150323,#89096,#89097);
#76342=AXIS2_PLACEMENT_3D('',#150337,#89099,#89100);
#76343=AXIS2_PLACEMENT_3D('',#150344,#89101,#89102);
#76344=AXIS2_PLACEMENT_3D('',#150347,#89103,#89104);
#76345=AXIS2_PLACEMENT_3D('',#150349,#89105,#89106);
#76346=AXIS2_PLACEMENT_3D('',#150350,#89107,#89108);
#76347=AXIS2_PLACEMENT_3D('',#150358,#89109,#89110);
#76348=AXIS2_PLACEMENT_3D('',#150360,#89112,#89113);
#76349=AXIS2_PLACEMENT_3D('',#150361,#89114,#89115);
#76350=AXIS2_PLACEMENT_3D('',#150362,#89116,#89117);
#76351=AXIS2_PLACEMENT_3D('',#150376,#89119,#89120);
#76352=AXIS2_PLACEMENT_3D('',#150383,#89121,#89122);
#76353=AXIS2_PLACEMENT_3D('',#150386,#89123,#89124);
#76354=AXIS2_PLACEMENT_3D('',#150388,#89125,#89126);
#76355=AXIS2_PLACEMENT_3D('',#150389,#89127,#89128);
#76356=AXIS2_PLACEMENT_3D('',#150397,#89129,#89130);
#76357=AXIS2_PLACEMENT_3D('',#150399,#89132,#89133);
#76358=AXIS2_PLACEMENT_3D('',#150400,#89134,#89135);
#76359=AXIS2_PLACEMENT_3D('',#150401,#89136,#89137);
#76360=AXIS2_PLACEMENT_3D('',#150415,#89139,#89140);
#76361=AXIS2_PLACEMENT_3D('',#150422,#89141,#89142);
#76362=AXIS2_PLACEMENT_3D('',#150425,#89143,#89144);
#76363=AXIS2_PLACEMENT_3D('',#150427,#89145,#89146);
#76364=AXIS2_PLACEMENT_3D('',#150428,#89147,#89148);
#76365=AXIS2_PLACEMENT_3D('',#150436,#89149,#89150);
#76366=AXIS2_PLACEMENT_3D('',#150438,#89152,#89153);
#76367=AXIS2_PLACEMENT_3D('',#150439,#89154,#89155);
#76368=AXIS2_PLACEMENT_3D('',#150440,#89156,#89157);
#76369=AXIS2_PLACEMENT_3D('',#150454,#89159,#89160);
#76370=AXIS2_PLACEMENT_3D('',#150461,#89161,#89162);
#76371=AXIS2_PLACEMENT_3D('',#150464,#89163,#89164);
#76372=AXIS2_PLACEMENT_3D('',#150466,#89165,#89166);
#76373=AXIS2_PLACEMENT_3D('',#150467,#89167,#89168);
#76374=AXIS2_PLACEMENT_3D('',#150475,#89169,#89170);
#76375=AXIS2_PLACEMENT_3D('',#150477,#89172,#89173);
#76376=AXIS2_PLACEMENT_3D('',#150478,#89174,#89175);
#76377=AXIS2_PLACEMENT_3D('',#150479,#89176,#89177);
#76378=AXIS2_PLACEMENT_3D('',#150493,#89179,#89180);
#76379=AXIS2_PLACEMENT_3D('',#150500,#89181,#89182);
#76380=AXIS2_PLACEMENT_3D('',#150503,#89183,#89184);
#76381=AXIS2_PLACEMENT_3D('',#150505,#89185,#89186);
#76382=AXIS2_PLACEMENT_3D('',#150506,#89187,#89188);
#76383=AXIS2_PLACEMENT_3D('',#150514,#89189,#89190);
#76384=AXIS2_PLACEMENT_3D('',#150516,#89192,#89193);
#76385=AXIS2_PLACEMENT_3D('',#150517,#89194,#89195);
#76386=AXIS2_PLACEMENT_3D('',#150518,#89196,#89197);
#76387=AXIS2_PLACEMENT_3D('',#150532,#89199,#89200);
#76388=AXIS2_PLACEMENT_3D('',#150539,#89201,#89202);
#76389=AXIS2_PLACEMENT_3D('',#150542,#89203,#89204);
#76390=AXIS2_PLACEMENT_3D('',#150544,#89205,#89206);
#76391=AXIS2_PLACEMENT_3D('',#150545,#89207,#89208);
#76392=AXIS2_PLACEMENT_3D('',#150553,#89209,#89210);
#76393=AXIS2_PLACEMENT_3D('',#150555,#89212,#89213);
#76394=AXIS2_PLACEMENT_3D('',#150556,#89214,#89215);
#76395=AXIS2_PLACEMENT_3D('',#150557,#89216,#89217);
#76396=AXIS2_PLACEMENT_3D('',#150571,#89219,#89220);
#76397=AXIS2_PLACEMENT_3D('',#150578,#89221,#89222);
#76398=AXIS2_PLACEMENT_3D('',#150581,#89223,#89224);
#76399=AXIS2_PLACEMENT_3D('',#150583,#89225,#89226);
#76400=AXIS2_PLACEMENT_3D('',#150584,#89227,#89228);
#76401=AXIS2_PLACEMENT_3D('',#150592,#89229,#89230);
#76402=AXIS2_PLACEMENT_3D('',#150594,#89232,#89233);
#76403=AXIS2_PLACEMENT_3D('',#150595,#89234,#89235);
#76404=AXIS2_PLACEMENT_3D('',#150596,#89236,#89237);
#76405=AXIS2_PLACEMENT_3D('',#150610,#89239,#89240);
#76406=AXIS2_PLACEMENT_3D('',#150617,#89241,#89242);
#76407=AXIS2_PLACEMENT_3D('',#150620,#89243,#89244);
#76408=AXIS2_PLACEMENT_3D('',#150622,#89245,#89246);
#76409=AXIS2_PLACEMENT_3D('',#150623,#89247,#89248);
#76410=AXIS2_PLACEMENT_3D('',#150631,#89249,#89250);
#76411=AXIS2_PLACEMENT_3D('',#150633,#89252,#89253);
#76412=AXIS2_PLACEMENT_3D('',#150634,#89254,#89255);
#76413=AXIS2_PLACEMENT_3D('',#150635,#89256,#89257);
#76414=AXIS2_PLACEMENT_3D('',#150649,#89259,#89260);
#76415=AXIS2_PLACEMENT_3D('',#150656,#89261,#89262);
#76416=AXIS2_PLACEMENT_3D('',#150659,#89263,#89264);
#76417=AXIS2_PLACEMENT_3D('',#150661,#89265,#89266);
#76418=AXIS2_PLACEMENT_3D('',#150662,#89267,#89268);
#76419=AXIS2_PLACEMENT_3D('',#150670,#89269,#89270);
#76420=AXIS2_PLACEMENT_3D('',#150672,#89272,#89273);
#76421=AXIS2_PLACEMENT_3D('',#150673,#89274,#89275);
#76422=AXIS2_PLACEMENT_3D('',#150674,#89276,#89277);
#76423=AXIS2_PLACEMENT_3D('',#150688,#89279,#89280);
#76424=AXIS2_PLACEMENT_3D('',#150695,#89281,#89282);
#76425=AXIS2_PLACEMENT_3D('',#150698,#89283,#89284);
#76426=AXIS2_PLACEMENT_3D('',#150700,#89285,#89286);
#76427=AXIS2_PLACEMENT_3D('',#150701,#89287,#89288);
#76428=AXIS2_PLACEMENT_3D('',#150709,#89289,#89290);
#76429=AXIS2_PLACEMENT_3D('',#150711,#89292,#89293);
#76430=AXIS2_PLACEMENT_3D('',#150712,#89294,#89295);
#76431=AXIS2_PLACEMENT_3D('',#150713,#89296,#89297);
#76432=AXIS2_PLACEMENT_3D('',#150727,#89299,#89300);
#76433=AXIS2_PLACEMENT_3D('',#150734,#89301,#89302);
#76434=AXIS2_PLACEMENT_3D('',#150737,#89303,#89304);
#76435=AXIS2_PLACEMENT_3D('',#150739,#89305,#89306);
#76436=AXIS2_PLACEMENT_3D('',#150740,#89307,#89308);
#76437=AXIS2_PLACEMENT_3D('',#150748,#89309,#89310);
#76438=AXIS2_PLACEMENT_3D('',#150750,#89312,#89313);
#76439=AXIS2_PLACEMENT_3D('',#150751,#89314,#89315);
#76440=AXIS2_PLACEMENT_3D('',#150752,#89316,#89317);
#76441=AXIS2_PLACEMENT_3D('',#150790,#89321,#89322);
#76442=AXIS2_PLACEMENT_3D('',#150797,#89323,#89324);
#76443=AXIS2_PLACEMENT_3D('',#150800,#89325,#89326);
#76444=AXIS2_PLACEMENT_3D('',#150802,#89327,#89328);
#76445=AXIS2_PLACEMENT_3D('',#150803,#89329,#89330);
#76446=AXIS2_PLACEMENT_3D('',#150811,#89331,#89332);
#76447=AXIS2_PLACEMENT_3D('',#150813,#89334,#89335);
#76448=AXIS2_PLACEMENT_3D('',#150814,#89336,#89337);
#76449=AXIS2_PLACEMENT_3D('',#150815,#89338,#89339);
#76450=AXIS2_PLACEMENT_3D('',#150829,#89341,#89342);
#76451=AXIS2_PLACEMENT_3D('',#150836,#89343,#89344);
#76452=AXIS2_PLACEMENT_3D('',#150839,#89345,#89346);
#76453=AXIS2_PLACEMENT_3D('',#150841,#89347,#89348);
#76454=AXIS2_PLACEMENT_3D('',#150842,#89349,#89350);
#76455=AXIS2_PLACEMENT_3D('',#150850,#89351,#89352);
#76456=AXIS2_PLACEMENT_3D('',#150852,#89354,#89355);
#76457=AXIS2_PLACEMENT_3D('',#150853,#89356,#89357);
#76458=AXIS2_PLACEMENT_3D('',#150854,#89358,#89359);
#76459=AXIS2_PLACEMENT_3D('',#150868,#89361,#89362);
#76460=AXIS2_PLACEMENT_3D('',#150875,#89363,#89364);
#76461=AXIS2_PLACEMENT_3D('',#150878,#89365,#89366);
#76462=AXIS2_PLACEMENT_3D('',#150880,#89367,#89368);
#76463=AXIS2_PLACEMENT_3D('',#150881,#89369,#89370);
#76464=AXIS2_PLACEMENT_3D('',#150889,#89371,#89372);
#76465=AXIS2_PLACEMENT_3D('',#150891,#89374,#89375);
#76466=AXIS2_PLACEMENT_3D('',#150892,#89376,#89377);
#76467=AXIS2_PLACEMENT_3D('',#150893,#89378,#89379);
#76468=AXIS2_PLACEMENT_3D('',#150907,#89381,#89382);
#76469=AXIS2_PLACEMENT_3D('',#150914,#89383,#89384);
#76470=AXIS2_PLACEMENT_3D('',#150917,#89385,#89386);
#76471=AXIS2_PLACEMENT_3D('',#150919,#89387,#89388);
#76472=AXIS2_PLACEMENT_3D('',#150920,#89389,#89390);
#76473=AXIS2_PLACEMENT_3D('',#150928,#89391,#89392);
#76474=AXIS2_PLACEMENT_3D('',#150930,#89394,#89395);
#76475=AXIS2_PLACEMENT_3D('',#150931,#89396,#89397);
#76476=AXIS2_PLACEMENT_3D('',#150932,#89398,#89399);
#76477=AXIS2_PLACEMENT_3D('',#150946,#89401,#89402);
#76478=AXIS2_PLACEMENT_3D('',#150953,#89403,#89404);
#76479=AXIS2_PLACEMENT_3D('',#150956,#89405,#89406);
#76480=AXIS2_PLACEMENT_3D('',#150958,#89407,#89408);
#76481=AXIS2_PLACEMENT_3D('',#150959,#89409,#89410);
#76482=AXIS2_PLACEMENT_3D('',#150967,#89411,#89412);
#76483=AXIS2_PLACEMENT_3D('',#150969,#89414,#89415);
#76484=AXIS2_PLACEMENT_3D('',#150970,#89416,#89417);
#76485=AXIS2_PLACEMENT_3D('',#150971,#89418,#89419);
#76486=AXIS2_PLACEMENT_3D('',#150985,#89421,#89422);
#76487=AXIS2_PLACEMENT_3D('',#150992,#89423,#89424);
#76488=AXIS2_PLACEMENT_3D('',#150995,#89425,#89426);
#76489=AXIS2_PLACEMENT_3D('',#150997,#89427,#89428);
#76490=AXIS2_PLACEMENT_3D('',#150998,#89429,#89430);
#76491=AXIS2_PLACEMENT_3D('',#151006,#89431,#89432);
#76492=AXIS2_PLACEMENT_3D('',#151008,#89434,#89435);
#76493=AXIS2_PLACEMENT_3D('',#151009,#89436,#89437);
#76494=AXIS2_PLACEMENT_3D('',#151010,#89438,#89439);
#76495=AXIS2_PLACEMENT_3D('',#151024,#89441,#89442);
#76496=AXIS2_PLACEMENT_3D('',#151031,#89443,#89444);
#76497=AXIS2_PLACEMENT_3D('',#151034,#89445,#89446);
#76498=AXIS2_PLACEMENT_3D('',#151036,#89447,#89448);
#76499=AXIS2_PLACEMENT_3D('',#151037,#89449,#89450);
#76500=AXIS2_PLACEMENT_3D('',#151045,#89451,#89452);
#76501=AXIS2_PLACEMENT_3D('',#151047,#89454,#89455);
#76502=AXIS2_PLACEMENT_3D('',#151048,#89456,#89457);
#76503=AXIS2_PLACEMENT_3D('',#151049,#89458,#89459);
#76504=AXIS2_PLACEMENT_3D('',#151061,#89460,#89461);
#76505=AXIS2_PLACEMENT_3D('',#151078,#89462,#89463);
#76506=AXIS2_PLACEMENT_3D('',#151090,#89464,#89465);
#76507=AXIS2_PLACEMENT_3D('',#151107,#89466,#89467);
#76508=AXIS2_PLACEMENT_3D('',#151119,#89468,#89469);
#76509=AXIS2_PLACEMENT_3D('',#151136,#89470,#89471);
#76510=AXIS2_PLACEMENT_3D('',#151148,#89472,#89473);
#76511=AXIS2_PLACEMENT_3D('',#151170,#89474,#89475);
#76512=AXIS2_PLACEMENT_3D('',#151182,#89476,#89477);
#76513=AXIS2_PLACEMENT_3D('',#151204,#89478,#89479);
#76514=AXIS2_PLACEMENT_3D('',#151216,#89480,#89481);
#76515=AXIS2_PLACEMENT_3D('',#151233,#89482,#89483);
#76516=AXIS2_PLACEMENT_3D('',#151245,#89484,#89485);
#76517=AXIS2_PLACEMENT_3D('',#151262,#89486,#89487);
#76518=AXIS2_PLACEMENT_3D('',#151274,#89488,#89489);
#76519=AXIS2_PLACEMENT_3D('',#151291,#89490,#89491);
#76520=AXIS2_PLACEMENT_3D('',#151303,#89492,#89493);
#76521=AXIS2_PLACEMENT_3D('',#151320,#89494,#89495);
#76522=AXIS2_PLACEMENT_3D('',#151332,#89496,#89497);
#76523=AXIS2_PLACEMENT_3D('',#151349,#89498,#89499);
#76524=AXIS2_PLACEMENT_3D('',#151361,#89500,#89501);
#76525=AXIS2_PLACEMENT_3D('',#151383,#89502,#89503);
#76526=AXIS2_PLACEMENT_3D('',#151395,#89504,#89505);
#76527=AXIS2_PLACEMENT_3D('',#151412,#89506,#89507);
#76528=AXIS2_PLACEMENT_3D('',#151424,#89508,#89509);
#76529=AXIS2_PLACEMENT_3D('',#151441,#89510,#89511);
#76530=AXIS2_PLACEMENT_3D('',#151453,#89512,#89513);
#76531=AXIS2_PLACEMENT_3D('',#151470,#89514,#89515);
#76532=AXIS2_PLACEMENT_3D('',#151482,#89516,#89517);
#76533=AXIS2_PLACEMENT_3D('',#151504,#89518,#89519);
#76534=AXIS2_PLACEMENT_3D('',#151516,#89520,#89521);
#76535=AXIS2_PLACEMENT_3D('',#151533,#89522,#89523);
#76536=AXIS2_PLACEMENT_3D('',#151545,#89524,#89525);
#76537=AXIS2_PLACEMENT_3D('',#151562,#89526,#89527);
#76538=AXIS2_PLACEMENT_3D('',#151574,#89528,#89529);
#76539=AXIS2_PLACEMENT_3D('',#151591,#89530,#89531);
#76540=AXIS2_PLACEMENT_3D('',#151603,#89532,#89533);
#76541=AXIS2_PLACEMENT_3D('',#151620,#89534,#89535);
#76542=AXIS2_PLACEMENT_3D('',#151632,#89536,#89537);
#76543=AXIS2_PLACEMENT_3D('',#151649,#89538,#89539);
#76544=AXIS2_PLACEMENT_3D('',#151661,#89540,#89541);
#76545=AXIS2_PLACEMENT_3D('',#151678,#89542,#89543);
#76546=AXIS2_PLACEMENT_3D('',#151690,#89544,#89545);
#76547=AXIS2_PLACEMENT_3D('',#151707,#89546,#89547);
#76548=AXIS2_PLACEMENT_3D('',#151719,#89548,#89549);
#76549=AXIS2_PLACEMENT_3D('',#151736,#89550,#89551);
#76550=AXIS2_PLACEMENT_3D('',#151748,#89552,#89553);
#76551=AXIS2_PLACEMENT_3D('',#151770,#89554,#89555);
#76552=AXIS2_PLACEMENT_3D('',#151782,#89556,#89557);
#76553=AXIS2_PLACEMENT_3D('',#151799,#89558,#89559);
#76554=AXIS2_PLACEMENT_3D('',#151811,#89560,#89561);
#76555=AXIS2_PLACEMENT_3D('',#151828,#89562,#89563);
#76556=AXIS2_PLACEMENT_3D('',#151840,#89564,#89565);
#76557=AXIS2_PLACEMENT_3D('',#151857,#89566,#89567);
#76558=AXIS2_PLACEMENT_3D('',#151869,#89568,#89569);
#76559=AXIS2_PLACEMENT_3D('',#151886,#89570,#89571);
#76560=AXIS2_PLACEMENT_3D('',#151898,#89572,#89573);
#76561=AXIS2_PLACEMENT_3D('',#151920,#89574,#89575);
#76562=AXIS2_PLACEMENT_3D('',#151932,#89576,#89577);
#76563=AXIS2_PLACEMENT_3D('',#151933,#89578,#89579);
#76564=AXIS2_PLACEMENT_3D('',#151940,#89580,#89581);
#76565=AXIS2_PLACEMENT_3D('',#151952,#89582,#89583);
#76566=AXIS2_PLACEMENT_3D('',#151953,#89584,#89585);
#76567=AXIS2_PLACEMENT_3D('',#151960,#89586,#89587);
#76568=AXIS2_PLACEMENT_3D('',#151972,#89588,#89589);
#76569=AXIS2_PLACEMENT_3D('',#151973,#89590,#89591);
#76570=AXIS2_PLACEMENT_3D('',#151980,#89592,#89593);
#76571=AXIS2_PLACEMENT_3D('',#151992,#89594,#89595);
#76572=AXIS2_PLACEMENT_3D('',#151993,#89596,#89597);
#76573=AXIS2_PLACEMENT_3D('',#152000,#89598,#89599);
#76574=AXIS2_PLACEMENT_3D('',#152012,#89600,#89601);
#76575=AXIS2_PLACEMENT_3D('',#152013,#89602,#89603);
#76576=AXIS2_PLACEMENT_3D('',#152020,#89604,#89605);
#76577=AXIS2_PLACEMENT_3D('',#152032,#89606,#89607);
#76578=AXIS2_PLACEMENT_3D('',#152033,#89608,#89609);
#76579=AXIS2_PLACEMENT_3D('',#152040,#89610,#89611);
#76580=AXIS2_PLACEMENT_3D('',#152052,#89612,#89613);
#76581=AXIS2_PLACEMENT_3D('',#152053,#89614,#89615);
#76582=AXIS2_PLACEMENT_3D('',#152060,#89616,#89617);
#76583=AXIS2_PLACEMENT_3D('',#152072,#89618,#89619);
#76584=AXIS2_PLACEMENT_3D('',#152073,#89620,#89621);
#76585=AXIS2_PLACEMENT_3D('',#152080,#89622,#89623);
#76586=AXIS2_PLACEMENT_3D('',#152092,#89624,#89625);
#76587=AXIS2_PLACEMENT_3D('',#152093,#89626,#89627);
#76588=AXIS2_PLACEMENT_3D('',#152100,#89628,#89629);
#76589=AXIS2_PLACEMENT_3D('',#152112,#89630,#89631);
#76590=AXIS2_PLACEMENT_3D('',#152113,#89632,#89633);
#76591=AXIS2_PLACEMENT_3D('',#152120,#89634,#89635);
#76592=AXIS2_PLACEMENT_3D('',#152132,#89636,#89637);
#76593=AXIS2_PLACEMENT_3D('',#152133,#89638,#89639);
#76594=AXIS2_PLACEMENT_3D('',#152140,#89640,#89641);
#76595=AXIS2_PLACEMENT_3D('',#152152,#89642,#89643);
#76596=AXIS2_PLACEMENT_3D('',#152153,#89644,#89645);
#76597=AXIS2_PLACEMENT_3D('',#152160,#89646,#89647);
#76598=AXIS2_PLACEMENT_3D('',#152172,#89648,#89649);
#76599=AXIS2_PLACEMENT_3D('',#152173,#89650,#89651);
#76600=AXIS2_PLACEMENT_3D('',#152180,#89652,#89653);
#76601=AXIS2_PLACEMENT_3D('',#152192,#89654,#89655);
#76602=AXIS2_PLACEMENT_3D('',#152193,#89656,#89657);
#76603=AXIS2_PLACEMENT_3D('',#152200,#89658,#89659);
#76604=AXIS2_PLACEMENT_3D('',#152212,#89660,#89661);
#76605=AXIS2_PLACEMENT_3D('',#152213,#89662,#89663);
#76606=AXIS2_PLACEMENT_3D('',#152220,#89664,#89665);
#76607=AXIS2_PLACEMENT_3D('',#152232,#89666,#89667);
#76608=AXIS2_PLACEMENT_3D('',#152233,#89668,#89669);
#76609=AXIS2_PLACEMENT_3D('',#152240,#89670,#89671);
#76610=AXIS2_PLACEMENT_3D('',#152252,#89672,#89673);
#76611=AXIS2_PLACEMENT_3D('',#152253,#89674,#89675);
#76612=AXIS2_PLACEMENT_3D('',#152260,#89676,#89677);
#76613=AXIS2_PLACEMENT_3D('',#152272,#89678,#89679);
#76614=AXIS2_PLACEMENT_3D('',#152273,#89680,#89681);
#76615=AXIS2_PLACEMENT_3D('',#152280,#89682,#89683);
#76616=AXIS2_PLACEMENT_3D('',#152292,#89684,#89685);
#76617=AXIS2_PLACEMENT_3D('',#152293,#89686,#89687);
#76618=AXIS2_PLACEMENT_3D('',#152300,#89688,#89689);
#76619=AXIS2_PLACEMENT_3D('',#152312,#89690,#89691);
#76620=AXIS2_PLACEMENT_3D('',#152313,#89692,#89693);
#76621=AXIS2_PLACEMENT_3D('',#152320,#89694,#89695);
#76622=AXIS2_PLACEMENT_3D('',#152332,#89696,#89697);
#76623=AXIS2_PLACEMENT_3D('',#152333,#89698,#89699);
#76624=AXIS2_PLACEMENT_3D('',#152340,#89700,#89701);
#76625=AXIS2_PLACEMENT_3D('',#152352,#89702,#89703);
#76626=AXIS2_PLACEMENT_3D('',#152353,#89704,#89705);
#76627=AXIS2_PLACEMENT_3D('',#152360,#89706,#89707);
#76628=AXIS2_PLACEMENT_3D('',#152372,#89708,#89709);
#76629=AXIS2_PLACEMENT_3D('',#152373,#89710,#89711);
#76630=AXIS2_PLACEMENT_3D('',#152380,#89712,#89713);
#76631=AXIS2_PLACEMENT_3D('',#152392,#89714,#89715);
#76632=AXIS2_PLACEMENT_3D('',#152393,#89716,#89717);
#76633=AXIS2_PLACEMENT_3D('',#152400,#89718,#89719);
#76634=AXIS2_PLACEMENT_3D('',#152412,#89720,#89721);
#76635=AXIS2_PLACEMENT_3D('',#152413,#89722,#89723);
#76636=AXIS2_PLACEMENT_3D('',#152420,#89724,#89725);
#76637=AXIS2_PLACEMENT_3D('',#152432,#89726,#89727);
#76638=AXIS2_PLACEMENT_3D('',#152433,#89728,#89729);
#76639=AXIS2_PLACEMENT_3D('',#152440,#89730,#89731);
#76640=AXIS2_PLACEMENT_3D('',#152452,#89732,#89733);
#76641=AXIS2_PLACEMENT_3D('',#152453,#89734,#89735);
#76642=AXIS2_PLACEMENT_3D('',#152460,#89736,#89737);
#76643=AXIS2_PLACEMENT_3D('',#152472,#89738,#89739);
#76644=AXIS2_PLACEMENT_3D('',#152473,#89740,#89741);
#76645=AXIS2_PLACEMENT_3D('',#152480,#89742,#89743);
#76646=AXIS2_PLACEMENT_3D('',#152492,#89744,#89745);
#76647=AXIS2_PLACEMENT_3D('',#152493,#89746,#89747);
#76648=AXIS2_PLACEMENT_3D('',#152500,#89748,#89749);
#76649=AXIS2_PLACEMENT_3D('',#152513,#89750,#89751);
#76650=AXIS2_PLACEMENT_3D('',#152537,#89753,#89754);
#76651=AXIS2_PLACEMENT_3D('',#152545,#89756,#89757);
#76652=AXIS2_PLACEMENT_3D('',#152547,#89758,#89759);
#76653=AXIS2_PLACEMENT_3D('',#152549,#89760,#89761);
#76654=AXIS2_PLACEMENT_3D('',#152550,#89762,#89763);
#76655=AXIS2_PLACEMENT_3D('',#152578,#89765,#89766);
#76656=AXIS2_PLACEMENT_3D('',#152586,#89768,#89769);
#76657=AXIS2_PLACEMENT_3D('',#152588,#89770,#89771);
#76658=AXIS2_PLACEMENT_3D('',#152590,#89772,#89773);
#76659=AXIS2_PLACEMENT_3D('',#152591,#89774,#89775);
#76660=AXIS2_PLACEMENT_3D('',#152619,#89777,#89778);
#76661=AXIS2_PLACEMENT_3D('',#152627,#89780,#89781);
#76662=AXIS2_PLACEMENT_3D('',#152629,#89782,#89783);
#76663=AXIS2_PLACEMENT_3D('',#152631,#89784,#89785);
#76664=AXIS2_PLACEMENT_3D('',#152632,#89786,#89787);
#76665=AXIS2_PLACEMENT_3D('',#152660,#89789,#89790);
#76666=AXIS2_PLACEMENT_3D('',#152668,#89792,#89793);
#76667=AXIS2_PLACEMENT_3D('',#152670,#89794,#89795);
#76668=AXIS2_PLACEMENT_3D('',#152672,#89796,#89797);
#76669=AXIS2_PLACEMENT_3D('',#152673,#89798,#89799);
#76670=AXIS2_PLACEMENT_3D('',#152701,#89801,#89802);
#76671=AXIS2_PLACEMENT_3D('',#152709,#89804,#89805);
#76672=AXIS2_PLACEMENT_3D('',#152711,#89806,#89807);
#76673=AXIS2_PLACEMENT_3D('',#152713,#89808,#89809);
#76674=AXIS2_PLACEMENT_3D('',#152714,#89810,#89811);
#76675=AXIS2_PLACEMENT_3D('',#152742,#89813,#89814);
#76676=AXIS2_PLACEMENT_3D('',#152750,#89816,#89817);
#76677=AXIS2_PLACEMENT_3D('',#152752,#89818,#89819);
#76678=AXIS2_PLACEMENT_3D('',#152754,#89820,#89821);
#76679=AXIS2_PLACEMENT_3D('',#152755,#89822,#89823);
#76680=AXIS2_PLACEMENT_3D('',#152815,#89827,#89828);
#76681=AXIS2_PLACEMENT_3D('',#152823,#89830,#89831);
#76682=AXIS2_PLACEMENT_3D('',#152825,#89832,#89833);
#76683=AXIS2_PLACEMENT_3D('',#152827,#89834,#89835);
#76684=AXIS2_PLACEMENT_3D('',#152828,#89836,#89837);
#76685=AXIS2_PLACEMENT_3D('',#152856,#89839,#89840);
#76686=AXIS2_PLACEMENT_3D('',#152864,#89842,#89843);
#76687=AXIS2_PLACEMENT_3D('',#152866,#89844,#89845);
#76688=AXIS2_PLACEMENT_3D('',#152868,#89846,#89847);
#76689=AXIS2_PLACEMENT_3D('',#152869,#89848,#89849);
#76690=AXIS2_PLACEMENT_3D('',#152897,#89851,#89852);
#76691=AXIS2_PLACEMENT_3D('',#152905,#89854,#89855);
#76692=AXIS2_PLACEMENT_3D('',#152907,#89856,#89857);
#76693=AXIS2_PLACEMENT_3D('',#152909,#89858,#89859);
#76694=AXIS2_PLACEMENT_3D('',#152910,#89860,#89861);
#76695=AXIS2_PLACEMENT_3D('',#152938,#89863,#89864);
#76696=AXIS2_PLACEMENT_3D('',#152946,#89866,#89867);
#76697=AXIS2_PLACEMENT_3D('',#152948,#89868,#89869);
#76698=AXIS2_PLACEMENT_3D('',#152950,#89870,#89871);
#76699=AXIS2_PLACEMENT_3D('',#152951,#89872,#89873);
#76700=AXIS2_PLACEMENT_3D('',#152979,#89875,#89876);
#76701=AXIS2_PLACEMENT_3D('',#152987,#89878,#89879);
#76702=AXIS2_PLACEMENT_3D('',#152989,#89880,#89881);
#76703=AXIS2_PLACEMENT_3D('',#152991,#89882,#89883);
#76704=AXIS2_PLACEMENT_3D('',#152992,#89884,#89885);
#76705=AXIS2_PLACEMENT_3D('',#153020,#89887,#89888);
#76706=AXIS2_PLACEMENT_3D('',#153028,#89890,#89891);
#76707=AXIS2_PLACEMENT_3D('',#153030,#89892,#89893);
#76708=AXIS2_PLACEMENT_3D('',#153032,#89894,#89895);
#76709=AXIS2_PLACEMENT_3D('',#153033,#89896,#89897);
#76710=AXIS2_PLACEMENT_3D('',#153061,#89899,#89900);
#76711=AXIS2_PLACEMENT_3D('',#153069,#89902,#89903);
#76712=AXIS2_PLACEMENT_3D('',#153071,#89904,#89905);
#76713=AXIS2_PLACEMENT_3D('',#153073,#89906,#89907);
#76714=AXIS2_PLACEMENT_3D('',#153074,#89908,#89909);
#76715=AXIS2_PLACEMENT_3D('',#153102,#89911,#89912);
#76716=AXIS2_PLACEMENT_3D('',#153110,#89914,#89915);
#76717=AXIS2_PLACEMENT_3D('',#153112,#89916,#89917);
#76718=AXIS2_PLACEMENT_3D('',#153114,#89918,#89919);
#76719=AXIS2_PLACEMENT_3D('',#153115,#89920,#89921);
#76720=AXIS2_PLACEMENT_3D('',#153143,#89923,#89924);
#76721=AXIS2_PLACEMENT_3D('',#153151,#89926,#89927);
#76722=AXIS2_PLACEMENT_3D('',#153153,#89928,#89929);
#76723=AXIS2_PLACEMENT_3D('',#153155,#89930,#89931);
#76724=AXIS2_PLACEMENT_3D('',#153156,#89932,#89933);
#76725=AXIS2_PLACEMENT_3D('',#153184,#89935,#89936);
#76726=AXIS2_PLACEMENT_3D('',#153192,#89938,#89939);
#76727=AXIS2_PLACEMENT_3D('',#153194,#89940,#89941);
#76728=AXIS2_PLACEMENT_3D('',#153196,#89942,#89943);
#76729=AXIS2_PLACEMENT_3D('',#153197,#89944,#89945);
#76730=AXIS2_PLACEMENT_3D('',#153225,#89947,#89948);
#76731=AXIS2_PLACEMENT_3D('',#153244,#89950,#89951);
#76732=AXIS2_PLACEMENT_3D('',#153246,#89953,#89954);
#76733=AXIS2_PLACEMENT_3D('',#153248,#89955,#89956);
#76734=AXIS2_PLACEMENT_3D('',#153249,#89957,#89958);
#76735=AXIS2_PLACEMENT_3D('',#153267,#89960,#89961);
#76736=AXIS2_PLACEMENT_3D('',#153274,#89962,#89963);
#76737=AXIS2_PLACEMENT_3D('',#153276,#89964,#89965);
#76738=AXIS2_PLACEMENT_3D('',#153278,#89966,#89967);
#76739=AXIS2_PLACEMENT_3D('',#153279,#89968,#89969);
#76740=AXIS2_PLACEMENT_3D('',#153307,#89971,#89972);
#76741=AXIS2_PLACEMENT_3D('',#153315,#89974,#89975);
#76742=AXIS2_PLACEMENT_3D('',#153317,#89976,#89977);
#76743=AXIS2_PLACEMENT_3D('',#153319,#89978,#89979);
#76744=AXIS2_PLACEMENT_3D('',#153320,#89980,#89981);
#76745=AXIS2_PLACEMENT_3D('',#153348,#89983,#89984);
#76746=AXIS2_PLACEMENT_3D('',#153356,#89986,#89987);
#76747=AXIS2_PLACEMENT_3D('',#153358,#89988,#89989);
#76748=AXIS2_PLACEMENT_3D('',#153360,#89990,#89991);
#76749=AXIS2_PLACEMENT_3D('',#153361,#89992,#89993);
#76750=AXIS2_PLACEMENT_3D('',#153389,#89995,#89996);
#76751=AXIS2_PLACEMENT_3D('',#153397,#89998,#89999);
#76752=AXIS2_PLACEMENT_3D('',#153399,#90000,#90001);
#76753=AXIS2_PLACEMENT_3D('',#153401,#90002,#90003);
#76754=AXIS2_PLACEMENT_3D('',#153402,#90004,#90005);
#76755=AXIS2_PLACEMENT_3D('',#153430,#90007,#90008);
#76756=AXIS2_PLACEMENT_3D('',#153438,#90010,#90011);
#76757=AXIS2_PLACEMENT_3D('',#153440,#90012,#90013);
#76758=AXIS2_PLACEMENT_3D('',#153442,#90014,#90015);
#76759=AXIS2_PLACEMENT_3D('',#153443,#90016,#90017);
#76760=AXIS2_PLACEMENT_3D('',#153471,#90019,#90020);
#76761=AXIS2_PLACEMENT_3D('',#153479,#90022,#90023);
#76762=AXIS2_PLACEMENT_3D('',#153481,#90024,#90025);
#76763=AXIS2_PLACEMENT_3D('',#153483,#90026,#90027);
#76764=AXIS2_PLACEMENT_3D('',#153484,#90028,#90029);
#76765=AXIS2_PLACEMENT_3D('',#153512,#90031,#90032);
#76766=AXIS2_PLACEMENT_3D('',#153520,#90034,#90035);
#76767=AXIS2_PLACEMENT_3D('',#153522,#90036,#90037);
#76768=AXIS2_PLACEMENT_3D('',#153524,#90038,#90039);
#76769=AXIS2_PLACEMENT_3D('',#153525,#90040,#90041);
#76770=AXIS2_PLACEMENT_3D('',#153553,#90043,#90044);
#76771=AXIS2_PLACEMENT_3D('',#153561,#90046,#90047);
#76772=AXIS2_PLACEMENT_3D('',#153563,#90048,#90049);
#76773=AXIS2_PLACEMENT_3D('',#153565,#90050,#90051);
#76774=AXIS2_PLACEMENT_3D('',#153566,#90052,#90053);
#76775=AXIS2_PLACEMENT_3D('',#153594,#90055,#90056);
#76776=AXIS2_PLACEMENT_3D('',#153602,#90058,#90059);
#76777=AXIS2_PLACEMENT_3D('',#153604,#90060,#90061);
#76778=AXIS2_PLACEMENT_3D('',#153606,#90062,#90063);
#76779=AXIS2_PLACEMENT_3D('',#153607,#90064,#90065);
#76780=AXIS2_PLACEMENT_3D('',#153635,#90067,#90068);
#76781=AXIS2_PLACEMENT_3D('',#153643,#90070,#90071);
#76782=AXIS2_PLACEMENT_3D('',#153645,#90072,#90073);
#76783=AXIS2_PLACEMENT_3D('',#153647,#90074,#90075);
#76784=AXIS2_PLACEMENT_3D('',#153648,#90076,#90077);
#76785=AXIS2_PLACEMENT_3D('',#153660,#90079,#90080);
#76786=AXIS2_PLACEMENT_3D('',#153663,#90081,#90082);
#76787=AXIS2_PLACEMENT_3D('',#153664,#90083,#90084);
#76788=AXIS2_PLACEMENT_3D('',#153665,#90085,#90086);
#76789=AXIS2_PLACEMENT_3D('',#153729,#90090,#90091);
#76790=AXIS2_PLACEMENT_3D('',#153788,#90094,#90095);
#76791=AXIS2_PLACEMENT_3D('',#153847,#90098,#90099);
#76792=AXIS2_PLACEMENT_3D('',#153906,#90102,#90103);
#76793=AXIS2_PLACEMENT_3D('',#153965,#90106,#90107);
#76794=AXIS2_PLACEMENT_3D('',#154024,#90110,#90111);
#76795=AXIS2_PLACEMENT_3D('',#154083,#90114,#90115);
#76796=AXIS2_PLACEMENT_3D('',#154142,#90118,#90119);
#76797=AXIS2_PLACEMENT_3D('',#154201,#90122,#90123);
#76798=AXIS2_PLACEMENT_3D('',#154260,#90126,#90127);
#76799=AXIS2_PLACEMENT_3D('',#154319,#90130,#90131);
#76800=AXIS2_PLACEMENT_3D('',#154378,#90134,#90135);
#76801=AXIS2_PLACEMENT_3D('',#154437,#90138,#90139);
#76802=AXIS2_PLACEMENT_3D('',#154522,#90144,#90145);
#76803=AXIS2_PLACEMENT_3D('',#154581,#90148,#90149);
#76804=AXIS2_PLACEMENT_3D('',#154640,#90152,#90153);
#76805=AXIS2_PLACEMENT_3D('',#154699,#90156,#90157);
#76806=AXIS2_PLACEMENT_3D('',#154758,#90160,#90161);
#76807=AXIS2_PLACEMENT_3D('',#154817,#90164,#90165);
#76808=AXIS2_PLACEMENT_3D('',#154902,#90170,#90171);
#76809=AXIS2_PLACEMENT_3D('',#154961,#90174,#90175);
#76810=AXIS2_PLACEMENT_3D('',#155020,#90178,#90179);
#76811=AXIS2_PLACEMENT_3D('',#155079,#90182,#90183);
#76812=AXIS2_PLACEMENT_3D('',#155138,#90186,#90187);
#76813=AXIS2_PLACEMENT_3D('',#155197,#90190,#90191);
#76814=AXIS2_PLACEMENT_3D('',#155256,#90194,#90195);
#76815=AXIS2_PLACEMENT_3D('',#155291,#90197,#90198);
#76816=AXIS2_PLACEMENT_3D('',#155333,#90200,#90201);
#76817=AXIS2_PLACEMENT_3D('',#155347,#90202,#90203);
#76818=AXIS2_PLACEMENT_3D('',#155360,#90204,#90205);
#76819=AXIS2_PLACEMENT_3D('',#155368,#90206,#90207);
#76820=AXIS2_PLACEMENT_3D('',#155381,#90208,#90209);
#76821=AXIS2_PLACEMENT_3D('',#155389,#90210,#90211);
#76822=AXIS2_PLACEMENT_3D('',#155402,#90212,#90213);
#76823=AXIS2_PLACEMENT_3D('',#155410,#90214,#90215);
#76824=AXIS2_PLACEMENT_3D('',#155423,#90216,#90217);
#76825=AXIS2_PLACEMENT_3D('',#155431,#90218,#90219);
#76826=AXIS2_PLACEMENT_3D('',#155444,#90220,#90221);
#76827=AXIS2_PLACEMENT_3D('',#155452,#90222,#90223);
#76828=AXIS2_PLACEMENT_3D('',#155465,#90224,#90225);
#76829=AXIS2_PLACEMENT_3D('',#155473,#90226,#90227);
#76830=AXIS2_PLACEMENT_3D('',#155486,#90228,#90229);
#76831=AXIS2_PLACEMENT_3D('',#155494,#90230,#90231);
#76832=AXIS2_PLACEMENT_3D('',#155507,#90232,#90233);
#76833=AXIS2_PLACEMENT_3D('',#155515,#90234,#90235);
#76834=AXIS2_PLACEMENT_3D('',#155528,#90236,#90237);
#76835=AXIS2_PLACEMENT_3D('',#155536,#90238,#90239);
#76836=AXIS2_PLACEMENT_3D('',#155549,#90240,#90241);
#76837=AXIS2_PLACEMENT_3D('',#155557,#90242,#90243);
#76838=AXIS2_PLACEMENT_3D('',#155570,#90244,#90245);
#76839=AXIS2_PLACEMENT_3D('',#155578,#90246,#90247);
#76840=AXIS2_PLACEMENT_3D('',#155591,#90248,#90249);
#76841=AXIS2_PLACEMENT_3D('',#155599,#90250,#90251);
#76842=AXIS2_PLACEMENT_3D('',#155612,#90252,#90253);
#76843=AXIS2_PLACEMENT_3D('',#155620,#90254,#90255);
#76844=AXIS2_PLACEMENT_3D('',#155633,#90256,#90257);
#76845=AXIS2_PLACEMENT_3D('',#155641,#90258,#90259);
#76846=AXIS2_PLACEMENT_3D('',#155654,#90260,#90261);
#76847=AXIS2_PLACEMENT_3D('',#155662,#90262,#90263);
#76848=AXIS2_PLACEMENT_3D('',#155675,#90264,#90265);
#76849=AXIS2_PLACEMENT_3D('',#155683,#90266,#90267);
#76850=AXIS2_PLACEMENT_3D('',#155696,#90268,#90269);
#76851=AXIS2_PLACEMENT_3D('',#155704,#90270,#90271);
#76852=AXIS2_PLACEMENT_3D('',#155717,#90272,#90273);
#76853=AXIS2_PLACEMENT_3D('',#155725,#90274,#90275);
#76854=AXIS2_PLACEMENT_3D('',#155738,#90276,#90277);
#76855=AXIS2_PLACEMENT_3D('',#155746,#90278,#90279);
#76856=AXIS2_PLACEMENT_3D('',#155759,#90280,#90281);
#76857=AXIS2_PLACEMENT_3D('',#155767,#90282,#90283);
#76858=AXIS2_PLACEMENT_3D('',#155780,#90284,#90285);
#76859=AXIS2_PLACEMENT_3D('',#155788,#90286,#90287);
#76860=AXIS2_PLACEMENT_3D('',#155801,#90288,#90289);
#76861=AXIS2_PLACEMENT_3D('',#155809,#90290,#90291);
#76862=AXIS2_PLACEMENT_3D('',#155822,#90292,#90293);
#76863=AXIS2_PLACEMENT_3D('',#155830,#90294,#90295);
#76864=AXIS2_PLACEMENT_3D('',#155843,#90296,#90297);
#76865=AXIS2_PLACEMENT_3D('',#155851,#90298,#90299);
#76866=AXIS2_PLACEMENT_3D('',#155864,#90300,#90301);
#76867=AXIS2_PLACEMENT_3D('',#155872,#90302,#90303);
#76868=AXIS2_PLACEMENT_3D('',#155885,#90304,#90305);
#76869=AXIS2_PLACEMENT_3D('',#155893,#90306,#90307);
#76870=AXIS2_PLACEMENT_3D('',#155906,#90308,#90309);
#76871=AXIS2_PLACEMENT_3D('',#155914,#90310,#90311);
#76872=AXIS2_PLACEMENT_3D('',#155927,#90312,#90313);
#76873=AXIS2_PLACEMENT_3D('',#155934,#90314,#90315);
#76874=AXIS2_PLACEMENT_3D('',#155950,#90316,#90317);
#76875=AXIS2_PLACEMENT_3D('',#155971,#90318,#90319);
#76876=AXIS2_PLACEMENT_3D('',#155997,#90320,#90321);
#76877=AXIS2_PLACEMENT_3D('',#156014,#90322,#90323);
#76878=AXIS2_PLACEMENT_3D('',#156040,#90324,#90325);
#76879=AXIS2_PLACEMENT_3D('',#156057,#90326,#90327);
#76880=AXIS2_PLACEMENT_3D('',#156083,#90328,#90329);
#76881=AXIS2_PLACEMENT_3D('',#156100,#90330,#90331);
#76882=AXIS2_PLACEMENT_3D('',#156126,#90332,#90333);
#76883=AXIS2_PLACEMENT_3D('',#156143,#90334,#90335);
#76884=AXIS2_PLACEMENT_3D('',#156169,#90336,#90337);
#76885=AXIS2_PLACEMENT_3D('',#156186,#90338,#90339);
#76886=AXIS2_PLACEMENT_3D('',#156212,#90340,#90341);
#76887=AXIS2_PLACEMENT_3D('',#156229,#90342,#90343);
#76888=AXIS2_PLACEMENT_3D('',#156255,#90344,#90345);
#76889=AXIS2_PLACEMENT_3D('',#156272,#90346,#90347);
#76890=AXIS2_PLACEMENT_3D('',#156298,#90348,#90349);
#76891=AXIS2_PLACEMENT_3D('',#156315,#90350,#90351);
#76892=AXIS2_PLACEMENT_3D('',#156341,#90352,#90353);
#76893=AXIS2_PLACEMENT_3D('',#156358,#90354,#90355);
#76894=AXIS2_PLACEMENT_3D('',#156384,#90356,#90357);
#76895=AXIS2_PLACEMENT_3D('',#156401,#90358,#90359);
#76896=AXIS2_PLACEMENT_3D('',#156427,#90360,#90361);
#76897=AXIS2_PLACEMENT_3D('',#156444,#90362,#90363);
#76898=AXIS2_PLACEMENT_3D('',#156470,#90364,#90365);
#76899=AXIS2_PLACEMENT_3D('',#156487,#90366,#90367);
#76900=AXIS2_PLACEMENT_3D('',#156513,#90368,#90369);
#76901=AXIS2_PLACEMENT_3D('',#156530,#90370,#90371);
#76902=AXIS2_PLACEMENT_3D('',#156556,#90372,#90373);
#76903=AXIS2_PLACEMENT_3D('',#156573,#90374,#90375);
#76904=AXIS2_PLACEMENT_3D('',#156599,#90376,#90377);
#76905=AXIS2_PLACEMENT_3D('',#156616,#90378,#90379);
#76906=AXIS2_PLACEMENT_3D('',#156642,#90380,#90381);
#76907=AXIS2_PLACEMENT_3D('',#156659,#90382,#90383);
#76908=AXIS2_PLACEMENT_3D('',#156685,#90384,#90385);
#76909=AXIS2_PLACEMENT_3D('',#156702,#90386,#90387);
#76910=AXIS2_PLACEMENT_3D('',#156728,#90388,#90389);
#76911=AXIS2_PLACEMENT_3D('',#156745,#90390,#90391);
#76912=AXIS2_PLACEMENT_3D('',#156771,#90392,#90393);
#76913=AXIS2_PLACEMENT_3D('',#156788,#90394,#90395);
#76914=AXIS2_PLACEMENT_3D('',#156814,#90396,#90397);
#76915=AXIS2_PLACEMENT_3D('',#156831,#90398,#90399);
#76916=AXIS2_PLACEMENT_3D('',#156857,#90400,#90401);
#76917=AXIS2_PLACEMENT_3D('',#156874,#90402,#90403);
#76918=AXIS2_PLACEMENT_3D('',#156900,#90404,#90405);
#76919=AXIS2_PLACEMENT_3D('',#156917,#90406,#90407);
#76920=AXIS2_PLACEMENT_3D('',#156943,#90408,#90409);
#76921=AXIS2_PLACEMENT_3D('',#156960,#90410,#90411);
#76922=AXIS2_PLACEMENT_3D('',#156986,#90412,#90413);
#76923=AXIS2_PLACEMENT_3D('',#157003,#90414,#90415);
#76924=AXIS2_PLACEMENT_3D('',#157029,#90416,#90417);
#76925=AXIS2_PLACEMENT_3D('',#157046,#90418,#90419);
#76926=AXIS2_PLACEMENT_3D('',#157072,#90420,#90421);
#76927=AXIS2_PLACEMENT_3D('',#157089,#90422,#90423);
#76928=AXIS2_PLACEMENT_3D('',#157115,#90424,#90425);
#76929=AXIS2_PLACEMENT_3D('',#157132,#90426,#90427);
#76930=AXIS2_PLACEMENT_3D('',#157158,#90428,#90429);
#76931=AXIS2_PLACEMENT_3D('',#157169,#90430,#90431);
#76932=AXIS2_PLACEMENT_3D('',#157178,#90432,#90433);
#76933=AXIS2_PLACEMENT_3D('',#157186,#90435,#90436);
#76934=AXIS2_PLACEMENT_3D('',#157188,#90437,#90438);
#76935=AXIS2_PLACEMENT_3D('',#157190,#90439,#90440);
#76936=AXIS2_PLACEMENT_3D('',#157191,#90441,#90442);
#76937=AXIS2_PLACEMENT_3D('',#157211,#90444,#90445);
#76938=AXIS2_PLACEMENT_3D('',#157219,#90447,#90448);
#76939=AXIS2_PLACEMENT_3D('',#157221,#90449,#90450);
#76940=AXIS2_PLACEMENT_3D('',#157223,#90451,#90452);
#76941=AXIS2_PLACEMENT_3D('',#157224,#90453,#90454);
#76942=AXIS2_PLACEMENT_3D('',#157244,#90456,#90457);
#76943=AXIS2_PLACEMENT_3D('',#157252,#90459,#90460);
#76944=AXIS2_PLACEMENT_3D('',#157254,#90461,#90462);
#76945=AXIS2_PLACEMENT_3D('',#157256,#90463,#90464);
#76946=AXIS2_PLACEMENT_3D('',#157257,#90465,#90466);
#76947=AXIS2_PLACEMENT_3D('',#157277,#90468,#90469);
#76948=AXIS2_PLACEMENT_3D('',#157285,#90471,#90472);
#76949=AXIS2_PLACEMENT_3D('',#157287,#90473,#90474);
#76950=AXIS2_PLACEMENT_3D('',#157289,#90475,#90476);
#76951=AXIS2_PLACEMENT_3D('',#157290,#90477,#90478);
#76952=AXIS2_PLACEMENT_3D('',#157310,#90480,#90481);
#76953=AXIS2_PLACEMENT_3D('',#157318,#90483,#90484);
#76954=AXIS2_PLACEMENT_3D('',#157320,#90485,#90486);
#76955=AXIS2_PLACEMENT_3D('',#157322,#90487,#90488);
#76956=AXIS2_PLACEMENT_3D('',#157323,#90489,#90490);
#76957=AXIS2_PLACEMENT_3D('',#157343,#90492,#90493);
#76958=AXIS2_PLACEMENT_3D('',#157351,#90495,#90496);
#76959=AXIS2_PLACEMENT_3D('',#157353,#90497,#90498);
#76960=AXIS2_PLACEMENT_3D('',#157355,#90499,#90500);
#76961=AXIS2_PLACEMENT_3D('',#157356,#90501,#90502);
#76962=AXIS2_PLACEMENT_3D('',#157376,#90504,#90505);
#76963=AXIS2_PLACEMENT_3D('',#157384,#90507,#90508);
#76964=AXIS2_PLACEMENT_3D('',#157386,#90509,#90510);
#76965=AXIS2_PLACEMENT_3D('',#157388,#90511,#90512);
#76966=AXIS2_PLACEMENT_3D('',#157389,#90513,#90514);
#76967=AXIS2_PLACEMENT_3D('',#157409,#90516,#90517);
#76968=AXIS2_PLACEMENT_3D('',#157417,#90519,#90520);
#76969=AXIS2_PLACEMENT_3D('',#157419,#90521,#90522);
#76970=AXIS2_PLACEMENT_3D('',#157421,#90523,#90524);
#76971=AXIS2_PLACEMENT_3D('',#157422,#90525,#90526);
#76972=AXIS2_PLACEMENT_3D('',#157442,#90528,#90529);
#76973=AXIS2_PLACEMENT_3D('',#157450,#90531,#90532);
#76974=AXIS2_PLACEMENT_3D('',#157452,#90533,#90534);
#76975=AXIS2_PLACEMENT_3D('',#157454,#90535,#90536);
#76976=AXIS2_PLACEMENT_3D('',#157455,#90537,#90538);
#76977=AXIS2_PLACEMENT_3D('',#157475,#90540,#90541);
#76978=AXIS2_PLACEMENT_3D('',#157483,#90543,#90544);
#76979=AXIS2_PLACEMENT_3D('',#157485,#90545,#90546);
#76980=AXIS2_PLACEMENT_3D('',#157487,#90547,#90548);
#76981=AXIS2_PLACEMENT_3D('',#157488,#90549,#90550);
#76982=AXIS2_PLACEMENT_3D('',#157508,#90552,#90553);
#76983=AXIS2_PLACEMENT_3D('',#157516,#90555,#90556);
#76984=AXIS2_PLACEMENT_3D('',#157518,#90557,#90558);
#76985=AXIS2_PLACEMENT_3D('',#157520,#90559,#90560);
#76986=AXIS2_PLACEMENT_3D('',#157521,#90561,#90562);
#76987=AXIS2_PLACEMENT_3D('',#157541,#90564,#90565);
#76988=AXIS2_PLACEMENT_3D('',#157549,#90567,#90568);
#76989=AXIS2_PLACEMENT_3D('',#157551,#90569,#90570);
#76990=AXIS2_PLACEMENT_3D('',#157553,#90571,#90572);
#76991=AXIS2_PLACEMENT_3D('',#157554,#90573,#90574);
#76992=AXIS2_PLACEMENT_3D('',#157574,#90576,#90577);
#76993=AXIS2_PLACEMENT_3D('',#157582,#90579,#90580);
#76994=AXIS2_PLACEMENT_3D('',#157584,#90581,#90582);
#76995=AXIS2_PLACEMENT_3D('',#157586,#90583,#90584);
#76996=AXIS2_PLACEMENT_3D('',#157587,#90585,#90586);
#76997=AXIS2_PLACEMENT_3D('',#157607,#90588,#90589);
#76998=AXIS2_PLACEMENT_3D('',#157615,#90591,#90592);
#76999=AXIS2_PLACEMENT_3D('',#157617,#90593,#90594);
#77000=AXIS2_PLACEMENT_3D('',#157619,#90595,#90596);
#77001=AXIS2_PLACEMENT_3D('',#157620,#90597,#90598);
#77002=AXIS2_PLACEMENT_3D('',#157664,#90602,#90603);
#77003=AXIS2_PLACEMENT_3D('',#157672,#90605,#90606);
#77004=AXIS2_PLACEMENT_3D('',#157674,#90607,#90608);
#77005=AXIS2_PLACEMENT_3D('',#157676,#90609,#90610);
#77006=AXIS2_PLACEMENT_3D('',#157677,#90611,#90612);
#77007=AXIS2_PLACEMENT_3D('',#157697,#90614,#90615);
#77008=AXIS2_PLACEMENT_3D('',#157705,#90617,#90618);
#77009=AXIS2_PLACEMENT_3D('',#157707,#90619,#90620);
#77010=AXIS2_PLACEMENT_3D('',#157709,#90621,#90622);
#77011=AXIS2_PLACEMENT_3D('',#157710,#90623,#90624);
#77012=AXIS2_PLACEMENT_3D('',#157730,#90626,#90627);
#77013=AXIS2_PLACEMENT_3D('',#157749,#90629,#90630);
#77014=AXIS2_PLACEMENT_3D('',#157751,#90632,#90633);
#77015=AXIS2_PLACEMENT_3D('',#157753,#90634,#90635);
#77016=AXIS2_PLACEMENT_3D('',#157754,#90636,#90637);
#77017=AXIS2_PLACEMENT_3D('',#157764,#90639,#90640);
#77018=AXIS2_PLACEMENT_3D('',#157771,#90641,#90642);
#77019=AXIS2_PLACEMENT_3D('',#157773,#90643,#90644);
#77020=AXIS2_PLACEMENT_3D('',#157775,#90645,#90646);
#77021=AXIS2_PLACEMENT_3D('',#157776,#90647,#90648);
#77022=AXIS2_PLACEMENT_3D('',#157796,#90650,#90651);
#77023=AXIS2_PLACEMENT_3D('',#157804,#90653,#90654);
#77024=AXIS2_PLACEMENT_3D('',#157806,#90655,#90656);
#77025=AXIS2_PLACEMENT_3D('',#157808,#90657,#90658);
#77026=AXIS2_PLACEMENT_3D('',#157809,#90659,#90660);
#77027=AXIS2_PLACEMENT_3D('',#157829,#90662,#90663);
#77028=AXIS2_PLACEMENT_3D('',#157837,#90665,#90666);
#77029=AXIS2_PLACEMENT_3D('',#157839,#90667,#90668);
#77030=AXIS2_PLACEMENT_3D('',#157841,#90669,#90670);
#77031=AXIS2_PLACEMENT_3D('',#157842,#90671,#90672);
#77032=AXIS2_PLACEMENT_3D('',#157862,#90674,#90675);
#77033=AXIS2_PLACEMENT_3D('',#157870,#90677,#90678);
#77034=AXIS2_PLACEMENT_3D('',#157872,#90679,#90680);
#77035=AXIS2_PLACEMENT_3D('',#157874,#90681,#90682);
#77036=AXIS2_PLACEMENT_3D('',#157875,#90683,#90684);
#77037=AXIS2_PLACEMENT_3D('',#157895,#90686,#90687);
#77038=AXIS2_PLACEMENT_3D('',#157903,#90689,#90690);
#77039=AXIS2_PLACEMENT_3D('',#157905,#90691,#90692);
#77040=AXIS2_PLACEMENT_3D('',#157907,#90693,#90694);
#77041=AXIS2_PLACEMENT_3D('',#157908,#90695,#90696);
#77042=AXIS2_PLACEMENT_3D('',#157928,#90698,#90699);
#77043=AXIS2_PLACEMENT_3D('',#157936,#90701,#90702);
#77044=AXIS2_PLACEMENT_3D('',#157938,#90703,#90704);
#77045=AXIS2_PLACEMENT_3D('',#157940,#90705,#90706);
#77046=AXIS2_PLACEMENT_3D('',#157941,#90707,#90708);
#77047=AXIS2_PLACEMENT_3D('',#157961,#90710,#90711);
#77048=AXIS2_PLACEMENT_3D('',#157969,#90713,#90714);
#77049=AXIS2_PLACEMENT_3D('',#157971,#90715,#90716);
#77050=AXIS2_PLACEMENT_3D('',#157973,#90717,#90718);
#77051=AXIS2_PLACEMENT_3D('',#157974,#90719,#90720);
#77052=AXIS2_PLACEMENT_3D('',#157994,#90722,#90723);
#77053=AXIS2_PLACEMENT_3D('',#158002,#90725,#90726);
#77054=AXIS2_PLACEMENT_3D('',#158004,#90727,#90728);
#77055=AXIS2_PLACEMENT_3D('',#158006,#90729,#90730);
#77056=AXIS2_PLACEMENT_3D('',#158007,#90731,#90732);
#77057=AXIS2_PLACEMENT_3D('',#158027,#90734,#90735);
#77058=AXIS2_PLACEMENT_3D('',#158035,#90737,#90738);
#77059=AXIS2_PLACEMENT_3D('',#158037,#90739,#90740);
#77060=AXIS2_PLACEMENT_3D('',#158039,#90741,#90742);
#77061=AXIS2_PLACEMENT_3D('',#158040,#90743,#90744);
#77062=AXIS2_PLACEMENT_3D('',#158060,#90746,#90747);
#77063=AXIS2_PLACEMENT_3D('',#158068,#90749,#90750);
#77064=AXIS2_PLACEMENT_3D('',#158070,#90751,#90752);
#77065=AXIS2_PLACEMENT_3D('',#158072,#90753,#90754);
#77066=AXIS2_PLACEMENT_3D('',#158073,#90755,#90756);
#77067=AXIS2_PLACEMENT_3D('',#158093,#90758,#90759);
#77068=AXIS2_PLACEMENT_3D('',#158101,#90761,#90762);
#77069=AXIS2_PLACEMENT_3D('',#158103,#90763,#90764);
#77070=AXIS2_PLACEMENT_3D('',#158105,#90765,#90766);
#77071=AXIS2_PLACEMENT_3D('',#158106,#90767,#90768);
#77072=AXIS2_PLACEMENT_3D('',#158128,#90770,#90771);
#77073=AXIS2_PLACEMENT_3D('',#158215,#90775,#90776);
#77074=AXIS2_PLACEMENT_3D('',#158301,#90779,#90780);
#77075=AXIS2_PLACEMENT_3D('',#158386,#90783,#90784);
#77076=AXIS2_PLACEMENT_3D('',#158472,#90787,#90788);
#77077=AXIS2_PLACEMENT_3D('',#158556,#90791,#90792);
#77078=AXIS2_PLACEMENT_3D('',#158642,#90795,#90796);
#77079=AXIS2_PLACEMENT_3D('',#158727,#90799,#90800);
#77080=AXIS2_PLACEMENT_3D('',#158813,#90803,#90804);
#77081=AXIS2_PLACEMENT_3D('',#158898,#90807,#90808);
#77082=AXIS2_PLACEMENT_3D('',#158984,#90811,#90812);
#77083=AXIS2_PLACEMENT_3D('',#159070,#90815,#90816);
#77084=AXIS2_PLACEMENT_3D('',#159156,#90819,#90820);
#77085=AXIS2_PLACEMENT_3D('',#159241,#90823,#90824);
#77086=AXIS2_PLACEMENT_3D('',#159326,#90827,#90828);
#77087=AXIS2_PLACEMENT_3D('',#159412,#90831,#90832);
#77088=AXIS2_PLACEMENT_3D('',#159498,#90835,#90836);
#77089=AXIS2_PLACEMENT_3D('',#159583,#90839,#90840);
#77090=AXIS2_PLACEMENT_3D('',#159668,#90843,#90844);
#77091=AXIS2_PLACEMENT_3D('',#159754,#90847,#90848);
#77092=AXIS2_PLACEMENT_3D('',#159839,#90851,#90852);
#77093=AXIS2_PLACEMENT_3D('',#159925,#90855,#90856);
#77094=AXIS2_PLACEMENT_3D('',#160011,#90859,#90860);
#77095=AXIS2_PLACEMENT_3D('',#160097,#90863,#90864);
#77096=AXIS2_PLACEMENT_3D('',#160183,#90867,#90868);
#77097=AXIS2_PLACEMENT_3D('',#160268,#90871,#90872);
#77098=AXIS2_PLACEMENT_3D('',#160354,#90875,#90876);
#77099=AXIS2_PLACEMENT_3D('',#160440,#90879,#90880);
#77100=AXIS2_PLACEMENT_3D('',#160526,#90883,#90884);
#77101=AXIS2_PLACEMENT_3D('',#160608,#90886,#90887);
#77102=AXIS2_PLACEMENT_3D('',#160625,#90888,#90889);
#77103=AXIS2_PLACEMENT_3D('',#160633,#90890,#90891);
#77104=AXIS2_PLACEMENT_3D('',#160650,#90892,#90893);
#77105=AXIS2_PLACEMENT_3D('',#160658,#90894,#90895);
#77106=AXIS2_PLACEMENT_3D('',#160675,#90896,#90897);
#77107=AXIS2_PLACEMENT_3D('',#160683,#90898,#90899);
#77108=AXIS2_PLACEMENT_3D('',#160700,#90900,#90901);
#77109=AXIS2_PLACEMENT_3D('',#160708,#90902,#90903);
#77110=AXIS2_PLACEMENT_3D('',#160725,#90904,#90905);
#77111=AXIS2_PLACEMENT_3D('',#160733,#90906,#90907);
#77112=AXIS2_PLACEMENT_3D('',#160750,#90908,#90909);
#77113=AXIS2_PLACEMENT_3D('',#160758,#90910,#90911);
#77114=AXIS2_PLACEMENT_3D('',#160775,#90912,#90913);
#77115=AXIS2_PLACEMENT_3D('',#160783,#90914,#90915);
#77116=AXIS2_PLACEMENT_3D('',#160800,#90916,#90917);
#77117=AXIS2_PLACEMENT_3D('',#160808,#90918,#90919);
#77118=AXIS2_PLACEMENT_3D('',#160825,#90920,#90921);
#77119=AXIS2_PLACEMENT_3D('',#160833,#90922,#90923);
#77120=AXIS2_PLACEMENT_3D('',#160850,#90924,#90925);
#77121=AXIS2_PLACEMENT_3D('',#160858,#90926,#90927);
#77122=AXIS2_PLACEMENT_3D('',#160875,#90928,#90929);
#77123=AXIS2_PLACEMENT_3D('',#160883,#90930,#90931);
#77124=AXIS2_PLACEMENT_3D('',#160900,#90932,#90933);
#77125=AXIS2_PLACEMENT_3D('',#160908,#90934,#90935);
#77126=AXIS2_PLACEMENT_3D('',#160925,#90936,#90937);
#77127=AXIS2_PLACEMENT_3D('',#160933,#90938,#90939);
#77128=AXIS2_PLACEMENT_3D('',#160950,#90940,#90941);
#77129=AXIS2_PLACEMENT_3D('',#160958,#90942,#90943);
#77130=AXIS2_PLACEMENT_3D('',#160975,#90944,#90945);
#77131=AXIS2_PLACEMENT_3D('',#160983,#90946,#90947);
#77132=AXIS2_PLACEMENT_3D('',#161000,#90948,#90949);
#77133=AXIS2_PLACEMENT_3D('',#161008,#90950,#90951);
#77134=AXIS2_PLACEMENT_3D('',#161025,#90952,#90953);
#77135=AXIS2_PLACEMENT_3D('',#161033,#90954,#90955);
#77136=AXIS2_PLACEMENT_3D('',#161050,#90956,#90957);
#77137=AXIS2_PLACEMENT_3D('',#161058,#90958,#90959);
#77138=AXIS2_PLACEMENT_3D('',#161075,#90960,#90961);
#77139=AXIS2_PLACEMENT_3D('',#161083,#90962,#90963);
#77140=AXIS2_PLACEMENT_3D('',#161100,#90964,#90965);
#77141=AXIS2_PLACEMENT_3D('',#161108,#90966,#90967);
#77142=AXIS2_PLACEMENT_3D('',#161125,#90968,#90969);
#77143=AXIS2_PLACEMENT_3D('',#161133,#90970,#90971);
#77144=AXIS2_PLACEMENT_3D('',#161150,#90972,#90973);
#77145=AXIS2_PLACEMENT_3D('',#161158,#90974,#90975);
#77146=AXIS2_PLACEMENT_3D('',#161175,#90976,#90977);
#77147=AXIS2_PLACEMENT_3D('',#161183,#90978,#90979);
#77148=AXIS2_PLACEMENT_3D('',#161200,#90980,#90981);
#77149=AXIS2_PLACEMENT_3D('',#161208,#90982,#90983);
#77150=AXIS2_PLACEMENT_3D('',#161225,#90984,#90985);
#77151=AXIS2_PLACEMENT_3D('',#161233,#90986,#90987);
#77152=AXIS2_PLACEMENT_3D('',#161250,#90988,#90989);
#77153=AXIS2_PLACEMENT_3D('',#161258,#90990,#90991);
#77154=AXIS2_PLACEMENT_3D('',#161275,#90992,#90993);
#77155=AXIS2_PLACEMENT_3D('',#161283,#90994,#90995);
#77156=AXIS2_PLACEMENT_3D('',#161300,#90996,#90997);
#77157=AXIS2_PLACEMENT_3D('',#161308,#90998,#90999);
#77158=AXIS2_PLACEMENT_3D('',#161325,#91000,#91001);
#77159=AXIS2_PLACEMENT_3D('',#161338,#91002,#91003);
#77160=AXIS2_PLACEMENT_3D('',#161354,#91005,#91006);
#77161=AXIS2_PLACEMENT_3D('',#161362,#91008,#91009);
#77162=AXIS2_PLACEMENT_3D('',#161365,#91010,#91011);
#77163=AXIS2_PLACEMENT_3D('',#161367,#91012,#91013);
#77164=AXIS2_PLACEMENT_3D('',#161368,#91014,#91015);
#77165=AXIS2_PLACEMENT_3D('',#161380,#91016,#91017);
#77166=AXIS2_PLACEMENT_3D('',#161382,#91019,#91020);
#77167=AXIS2_PLACEMENT_3D('',#161383,#91021,#91022);
#77168=AXIS2_PLACEMENT_3D('',#161384,#91023,#91024);
#77169=AXIS2_PLACEMENT_3D('',#161393,#91025,#91026);
#77170=AXIS2_PLACEMENT_3D('',#161401,#91028,#91029);
#77171=AXIS2_PLACEMENT_3D('',#161404,#91030,#91031);
#77172=AXIS2_PLACEMENT_3D('',#161406,#91032,#91033);
#77173=AXIS2_PLACEMENT_3D('',#161407,#91034,#91035);
#77174=AXIS2_PLACEMENT_3D('',#161419,#91036,#91037);
#77175=AXIS2_PLACEMENT_3D('',#161421,#91039,#91040);
#77176=AXIS2_PLACEMENT_3D('',#161422,#91041,#91042);
#77177=AXIS2_PLACEMENT_3D('',#161423,#91043,#91044);
#77178=AXIS2_PLACEMENT_3D('',#161432,#91045,#91046);
#77179=AXIS2_PLACEMENT_3D('',#161440,#91048,#91049);
#77180=AXIS2_PLACEMENT_3D('',#161443,#91050,#91051);
#77181=AXIS2_PLACEMENT_3D('',#161445,#91052,#91053);
#77182=AXIS2_PLACEMENT_3D('',#161446,#91054,#91055);
#77183=AXIS2_PLACEMENT_3D('',#161458,#91056,#91057);
#77184=AXIS2_PLACEMENT_3D('',#161460,#91059,#91060);
#77185=AXIS2_PLACEMENT_3D('',#161461,#91061,#91062);
#77186=AXIS2_PLACEMENT_3D('',#161462,#91063,#91064);
#77187=AXIS2_PLACEMENT_3D('',#161471,#91065,#91066);
#77188=AXIS2_PLACEMENT_3D('',#161479,#91068,#91069);
#77189=AXIS2_PLACEMENT_3D('',#161482,#91070,#91071);
#77190=AXIS2_PLACEMENT_3D('',#161484,#91072,#91073);
#77191=AXIS2_PLACEMENT_3D('',#161485,#91074,#91075);
#77192=AXIS2_PLACEMENT_3D('',#161497,#91076,#91077);
#77193=AXIS2_PLACEMENT_3D('',#161499,#91079,#91080);
#77194=AXIS2_PLACEMENT_3D('',#161500,#91081,#91082);
#77195=AXIS2_PLACEMENT_3D('',#161501,#91083,#91084);
#77196=AXIS2_PLACEMENT_3D('',#161510,#91085,#91086);
#77197=AXIS2_PLACEMENT_3D('',#161518,#91088,#91089);
#77198=AXIS2_PLACEMENT_3D('',#161521,#91090,#91091);
#77199=AXIS2_PLACEMENT_3D('',#161523,#91092,#91093);
#77200=AXIS2_PLACEMENT_3D('',#161524,#91094,#91095);
#77201=AXIS2_PLACEMENT_3D('',#161536,#91096,#91097);
#77202=AXIS2_PLACEMENT_3D('',#161538,#91099,#91100);
#77203=AXIS2_PLACEMENT_3D('',#161539,#91101,#91102);
#77204=AXIS2_PLACEMENT_3D('',#161540,#91103,#91104);
#77205=AXIS2_PLACEMENT_3D('',#161549,#91105,#91106);
#77206=AXIS2_PLACEMENT_3D('',#161557,#91108,#91109);
#77207=AXIS2_PLACEMENT_3D('',#161560,#91110,#91111);
#77208=AXIS2_PLACEMENT_3D('',#161562,#91112,#91113);
#77209=AXIS2_PLACEMENT_3D('',#161563,#91114,#91115);
#77210=AXIS2_PLACEMENT_3D('',#161575,#91116,#91117);
#77211=AXIS2_PLACEMENT_3D('',#161577,#91119,#91120);
#77212=AXIS2_PLACEMENT_3D('',#161578,#91121,#91122);
#77213=AXIS2_PLACEMENT_3D('',#161579,#91123,#91124);
#77214=AXIS2_PLACEMENT_3D('',#161593,#91126,#91127);
#77215=AXIS2_PLACEMENT_3D('',#161595,#91128,#91129);
#77216=AXIS2_PLACEMENT_3D('',#161596,#91130,#91131);
#77217=AXIS2_PLACEMENT_3D('',#161616,#91133,#91134);
#77218=AXIS2_PLACEMENT_3D('',#161624,#91136,#91137);
#77219=AXIS2_PLACEMENT_3D('',#161627,#91138,#91139);
#77220=AXIS2_PLACEMENT_3D('',#161629,#91140,#91141);
#77221=AXIS2_PLACEMENT_3D('',#161630,#91142,#91143);
#77222=AXIS2_PLACEMENT_3D('',#161642,#91144,#91145);
#77223=AXIS2_PLACEMENT_3D('',#161644,#91147,#91148);
#77224=AXIS2_PLACEMENT_3D('',#161645,#91149,#91150);
#77225=AXIS2_PLACEMENT_3D('',#161646,#91151,#91152);
#77226=AXIS2_PLACEMENT_3D('',#161655,#91153,#91154);
#77227=AXIS2_PLACEMENT_3D('',#161663,#91156,#91157);
#77228=AXIS2_PLACEMENT_3D('',#161666,#91158,#91159);
#77229=AXIS2_PLACEMENT_3D('',#161668,#91160,#91161);
#77230=AXIS2_PLACEMENT_3D('',#161669,#91162,#91163);
#77231=AXIS2_PLACEMENT_3D('',#161681,#91164,#91165);
#77232=AXIS2_PLACEMENT_3D('',#161683,#91167,#91168);
#77233=AXIS2_PLACEMENT_3D('',#161684,#91169,#91170);
#77234=AXIS2_PLACEMENT_3D('',#161685,#91171,#91172);
#77235=AXIS2_PLACEMENT_3D('',#161694,#91173,#91174);
#77236=AXIS2_PLACEMENT_3D('',#161702,#91176,#91177);
#77237=AXIS2_PLACEMENT_3D('',#161705,#91178,#91179);
#77238=AXIS2_PLACEMENT_3D('',#161707,#91180,#91181);
#77239=AXIS2_PLACEMENT_3D('',#161708,#91182,#91183);
#77240=AXIS2_PLACEMENT_3D('',#161720,#91184,#91185);
#77241=AXIS2_PLACEMENT_3D('',#161722,#91187,#91188);
#77242=AXIS2_PLACEMENT_3D('',#161723,#91189,#91190);
#77243=AXIS2_PLACEMENT_3D('',#161724,#91191,#91192);
#77244=AXIS2_PLACEMENT_3D('',#161733,#91193,#91194);
#77245=AXIS2_PLACEMENT_3D('',#161741,#91196,#91197);
#77246=AXIS2_PLACEMENT_3D('',#161744,#91198,#91199);
#77247=AXIS2_PLACEMENT_3D('',#161746,#91200,#91201);
#77248=AXIS2_PLACEMENT_3D('',#161747,#91202,#91203);
#77249=AXIS2_PLACEMENT_3D('',#161759,#91204,#91205);
#77250=AXIS2_PLACEMENT_3D('',#161761,#91207,#91208);
#77251=AXIS2_PLACEMENT_3D('',#161762,#91209,#91210);
#77252=AXIS2_PLACEMENT_3D('',#161763,#91211,#91212);
#77253=AXIS2_PLACEMENT_3D('',#161772,#91213,#91214);
#77254=AXIS2_PLACEMENT_3D('',#161780,#91216,#91217);
#77255=AXIS2_PLACEMENT_3D('',#161783,#91218,#91219);
#77256=AXIS2_PLACEMENT_3D('',#161785,#91220,#91221);
#77257=AXIS2_PLACEMENT_3D('',#161786,#91222,#91223);
#77258=AXIS2_PLACEMENT_3D('',#161798,#91224,#91225);
#77259=AXIS2_PLACEMENT_3D('',#161800,#91227,#91228);
#77260=AXIS2_PLACEMENT_3D('',#161801,#91229,#91230);
#77261=AXIS2_PLACEMENT_3D('',#161802,#91231,#91232);
#77262=AXIS2_PLACEMENT_3D('',#161811,#91233,#91234);
#77263=AXIS2_PLACEMENT_3D('',#161819,#91236,#91237);
#77264=AXIS2_PLACEMENT_3D('',#161822,#91238,#91239);
#77265=AXIS2_PLACEMENT_3D('',#161824,#91240,#91241);
#77266=AXIS2_PLACEMENT_3D('',#161825,#91242,#91243);
#77267=AXIS2_PLACEMENT_3D('',#161837,#91244,#91245);
#77268=AXIS2_PLACEMENT_3D('',#161839,#91247,#91248);
#77269=AXIS2_PLACEMENT_3D('',#161840,#91249,#91250);
#77270=AXIS2_PLACEMENT_3D('',#161841,#91251,#91252);
#77271=AXIS2_PLACEMENT_3D('',#161850,#91253,#91254);
#77272=AXIS2_PLACEMENT_3D('',#161858,#91256,#91257);
#77273=AXIS2_PLACEMENT_3D('',#161861,#91258,#91259);
#77274=AXIS2_PLACEMENT_3D('',#161863,#91260,#91261);
#77275=AXIS2_PLACEMENT_3D('',#161864,#91262,#91263);
#77276=AXIS2_PLACEMENT_3D('',#161876,#91264,#91265);
#77277=AXIS2_PLACEMENT_3D('',#161878,#91267,#91268);
#77278=AXIS2_PLACEMENT_3D('',#161879,#91269,#91270);
#77279=AXIS2_PLACEMENT_3D('',#161880,#91271,#91272);
#77280=AXIS2_PLACEMENT_3D('',#161889,#91273,#91274);
#77281=AXIS2_PLACEMENT_3D('',#161897,#91276,#91277);
#77282=AXIS2_PLACEMENT_3D('',#161900,#91278,#91279);
#77283=AXIS2_PLACEMENT_3D('',#161902,#91280,#91281);
#77284=AXIS2_PLACEMENT_3D('',#161903,#91282,#91283);
#77285=AXIS2_PLACEMENT_3D('',#161915,#91284,#91285);
#77286=AXIS2_PLACEMENT_3D('',#161917,#91287,#91288);
#77287=AXIS2_PLACEMENT_3D('',#161918,#91289,#91290);
#77288=AXIS2_PLACEMENT_3D('',#161919,#91291,#91292);
#77289=AXIS2_PLACEMENT_3D('',#161928,#91293,#91294);
#77290=AXIS2_PLACEMENT_3D('',#161936,#91296,#91297);
#77291=AXIS2_PLACEMENT_3D('',#161939,#91298,#91299);
#77292=AXIS2_PLACEMENT_3D('',#161941,#91300,#91301);
#77293=AXIS2_PLACEMENT_3D('',#161942,#91302,#91303);
#77294=AXIS2_PLACEMENT_3D('',#161954,#91304,#91305);
#77295=AXIS2_PLACEMENT_3D('',#161956,#91307,#91308);
#77296=AXIS2_PLACEMENT_3D('',#161957,#91309,#91310);
#77297=AXIS2_PLACEMENT_3D('',#161958,#91311,#91312);
#77298=AXIS2_PLACEMENT_3D('',#161967,#91313,#91314);
#77299=AXIS2_PLACEMENT_3D('',#161975,#91316,#91317);
#77300=AXIS2_PLACEMENT_3D('',#161978,#91318,#91319);
#77301=AXIS2_PLACEMENT_3D('',#161980,#91320,#91321);
#77302=AXIS2_PLACEMENT_3D('',#161981,#91322,#91323);
#77303=AXIS2_PLACEMENT_3D('',#161993,#91324,#91325);
#77304=AXIS2_PLACEMENT_3D('',#161995,#91327,#91328);
#77305=AXIS2_PLACEMENT_3D('',#161996,#91329,#91330);
#77306=AXIS2_PLACEMENT_3D('',#161997,#91331,#91332);
#77307=AXIS2_PLACEMENT_3D('',#162007,#91334,#91335);
#77308=AXIS2_PLACEMENT_3D('',#162014,#91336,#91337);
#77309=AXIS2_PLACEMENT_3D('',#162017,#91338,#91339);
#77310=AXIS2_PLACEMENT_3D('',#162019,#91340,#91341);
#77311=AXIS2_PLACEMENT_3D('',#162020,#91342,#91343);
#77312=AXIS2_PLACEMENT_3D('',#162032,#91344,#91345);
#77313=AXIS2_PLACEMENT_3D('',#162034,#91347,#91348);
#77314=AXIS2_PLACEMENT_3D('',#162035,#91349,#91350);
#77315=AXIS2_PLACEMENT_3D('',#162036,#91351,#91352);
#77316=AXIS2_PLACEMENT_3D('',#162045,#91353,#91354);
#77317=AXIS2_PLACEMENT_3D('',#162053,#91356,#91357);
#77318=AXIS2_PLACEMENT_3D('',#162056,#91358,#91359);
#77319=AXIS2_PLACEMENT_3D('',#162058,#91360,#91361);
#77320=AXIS2_PLACEMENT_3D('',#162059,#91362,#91363);
#77321=AXIS2_PLACEMENT_3D('',#162071,#91364,#91365);
#77322=AXIS2_PLACEMENT_3D('',#162073,#91367,#91368);
#77323=AXIS2_PLACEMENT_3D('',#162074,#91369,#91370);
#77324=AXIS2_PLACEMENT_3D('',#162075,#91371,#91372);
#77325=AXIS2_PLACEMENT_3D('',#162084,#91373,#91374);
#77326=AXIS2_PLACEMENT_3D('',#162092,#91376,#91377);
#77327=AXIS2_PLACEMENT_3D('',#162095,#91378,#91379);
#77328=AXIS2_PLACEMENT_3D('',#162097,#91380,#91381);
#77329=AXIS2_PLACEMENT_3D('',#162098,#91382,#91383);
#77330=AXIS2_PLACEMENT_3D('',#162110,#91384,#91385);
#77331=AXIS2_PLACEMENT_3D('',#162112,#91387,#91388);
#77332=AXIS2_PLACEMENT_3D('',#162113,#91389,#91390);
#77333=AXIS2_PLACEMENT_3D('',#162114,#91391,#91392);
#77334=AXIS2_PLACEMENT_3D('',#162123,#91393,#91394);
#77335=AXIS2_PLACEMENT_3D('',#162131,#91396,#91397);
#77336=AXIS2_PLACEMENT_3D('',#162134,#91398,#91399);
#77337=AXIS2_PLACEMENT_3D('',#162136,#91400,#91401);
#77338=AXIS2_PLACEMENT_3D('',#162137,#91402,#91403);
#77339=AXIS2_PLACEMENT_3D('',#162149,#91404,#91405);
#77340=AXIS2_PLACEMENT_3D('',#162151,#91407,#91408);
#77341=AXIS2_PLACEMENT_3D('',#162152,#91409,#91410);
#77342=AXIS2_PLACEMENT_3D('',#162153,#91411,#91412);
#77343=AXIS2_PLACEMENT_3D('',#162162,#91413,#91414);
#77344=AXIS2_PLACEMENT_3D('',#162170,#91416,#91417);
#77345=AXIS2_PLACEMENT_3D('',#162173,#91418,#91419);
#77346=AXIS2_PLACEMENT_3D('',#162175,#91420,#91421);
#77347=AXIS2_PLACEMENT_3D('',#162176,#91422,#91423);
#77348=AXIS2_PLACEMENT_3D('',#162188,#91424,#91425);
#77349=AXIS2_PLACEMENT_3D('',#162190,#91427,#91428);
#77350=AXIS2_PLACEMENT_3D('',#162191,#91429,#91430);
#77351=AXIS2_PLACEMENT_3D('',#162192,#91431,#91432);
#77352=AXIS2_PLACEMENT_3D('',#162201,#91433,#91434);
#77353=AXIS2_PLACEMENT_3D('',#162209,#91436,#91437);
#77354=AXIS2_PLACEMENT_3D('',#162212,#91438,#91439);
#77355=AXIS2_PLACEMENT_3D('',#162214,#91440,#91441);
#77356=AXIS2_PLACEMENT_3D('',#162215,#91442,#91443);
#77357=AXIS2_PLACEMENT_3D('',#162227,#91444,#91445);
#77358=AXIS2_PLACEMENT_3D('',#162229,#91447,#91448);
#77359=AXIS2_PLACEMENT_3D('',#162230,#91449,#91450);
#77360=AXIS2_PLACEMENT_3D('',#162231,#91451,#91452);
#77361=AXIS2_PLACEMENT_3D('',#162240,#91453,#91454);
#77362=AXIS2_PLACEMENT_3D('',#162248,#91456,#91457);
#77363=AXIS2_PLACEMENT_3D('',#162251,#91458,#91459);
#77364=AXIS2_PLACEMENT_3D('',#162253,#91460,#91461);
#77365=AXIS2_PLACEMENT_3D('',#162254,#91462,#91463);
#77366=AXIS2_PLACEMENT_3D('',#162266,#91464,#91465);
#77367=AXIS2_PLACEMENT_3D('',#162268,#91467,#91468);
#77368=AXIS2_PLACEMENT_3D('',#162269,#91469,#91470);
#77369=AXIS2_PLACEMENT_3D('',#162270,#91471,#91472);
#77370=AXIS2_PLACEMENT_3D('',#162279,#91473,#91474);
#77371=AXIS2_PLACEMENT_3D('',#162287,#91476,#91477);
#77372=AXIS2_PLACEMENT_3D('',#162290,#91478,#91479);
#77373=AXIS2_PLACEMENT_3D('',#162292,#91480,#91481);
#77374=AXIS2_PLACEMENT_3D('',#162293,#91482,#91483);
#77375=AXIS2_PLACEMENT_3D('',#162305,#91484,#91485);
#77376=AXIS2_PLACEMENT_3D('',#162307,#91487,#91488);
#77377=AXIS2_PLACEMENT_3D('',#162308,#91489,#91490);
#77378=AXIS2_PLACEMENT_3D('',#162309,#91491,#91492);
#77379=AXIS2_PLACEMENT_3D('',#162318,#91493,#91494);
#77380=AXIS2_PLACEMENT_3D('',#162326,#91496,#91497);
#77381=AXIS2_PLACEMENT_3D('',#162329,#91498,#91499);
#77382=AXIS2_PLACEMENT_3D('',#162331,#91500,#91501);
#77383=AXIS2_PLACEMENT_3D('',#162332,#91502,#91503);
#77384=AXIS2_PLACEMENT_3D('',#162344,#91504,#91505);
#77385=AXIS2_PLACEMENT_3D('',#162346,#91507,#91508);
#77386=AXIS2_PLACEMENT_3D('',#162347,#91509,#91510);
#77387=AXIS2_PLACEMENT_3D('',#162348,#91511,#91512);
#77388=AXIS2_PLACEMENT_3D('',#162357,#91513,#91514);
#77389=AXIS2_PLACEMENT_3D('',#162365,#91516,#91517);
#77390=AXIS2_PLACEMENT_3D('',#162368,#91518,#91519);
#77391=AXIS2_PLACEMENT_3D('',#162370,#91520,#91521);
#77392=AXIS2_PLACEMENT_3D('',#162371,#91522,#91523);
#77393=AXIS2_PLACEMENT_3D('',#162383,#91524,#91525);
#77394=AXIS2_PLACEMENT_3D('',#162385,#91527,#91528);
#77395=AXIS2_PLACEMENT_3D('',#162386,#91529,#91530);
#77396=AXIS2_PLACEMENT_3D('',#162387,#91531,#91532);
#77397=AXIS2_PLACEMENT_3D('',#162396,#91533,#91534);
#77398=AXIS2_PLACEMENT_3D('',#162404,#91536,#91537);
#77399=AXIS2_PLACEMENT_3D('',#162407,#91538,#91539);
#77400=AXIS2_PLACEMENT_3D('',#162409,#91540,#91541);
#77401=AXIS2_PLACEMENT_3D('',#162410,#91542,#91543);
#77402=AXIS2_PLACEMENT_3D('',#162422,#91544,#91545);
#77403=AXIS2_PLACEMENT_3D('',#162424,#91547,#91548);
#77404=AXIS2_PLACEMENT_3D('',#162425,#91549,#91550);
#77405=AXIS2_PLACEMENT_3D('',#162426,#91551,#91552);
#77406=AXIS2_PLACEMENT_3D('',#162427,#91553,#91554);
#77407=AXIS2_PLACEMENT_3D('',#162430,#91555,#91556);
#77408=AXIS2_PLACEMENT_3D('',#162432,#91557,#91558);
#77409=AXIS2_PLACEMENT_3D('',#162433,#91559,#91560);
#77410=AXIS2_PLACEMENT_3D('',#162434,#91561,#91562);
#77411=AXIS2_PLACEMENT_3D('',#162435,#91563,#91564);
#77412=AXIS2_PLACEMENT_3D('',#162437,#91565,#91566);
#77413=AXIS2_PLACEMENT_3D('',#162438,#91567,#91568);
#77414=AXIS2_PLACEMENT_3D('',#162446,#91570,#91571);
#77415=AXIS2_PLACEMENT_3D('',#162458,#91572,#91573);
#77416=AXIS2_PLACEMENT_3D('',#162459,#91574,#91575);
#77417=AXIS2_PLACEMENT_3D('',#162467,#91576,#91577);
#77418=AXIS2_PLACEMENT_3D('',#162468,#91578,#91579);
#77419=AXIS2_PLACEMENT_3D('',#162479,#91580,#91581);
#77420=AXIS2_PLACEMENT_3D('',#162487,#91582,#91583);
#77421=AXIS2_PLACEMENT_3D('',#162488,#91584,#91585);
#77422=AXIS2_PLACEMENT_3D('',#162499,#91586,#91587);
#77423=AXIS2_PLACEMENT_3D('',#162507,#91588,#91589);
#77424=AXIS2_PLACEMENT_3D('',#162508,#91590,#91591);
#77425=AXIS2_PLACEMENT_3D('',#162519,#91592,#91593);
#77426=AXIS2_PLACEMENT_3D('',#162527,#91594,#91595);
#77427=AXIS2_PLACEMENT_3D('',#162528,#91596,#91597);
#77428=AXIS2_PLACEMENT_3D('',#162539,#91598,#91599);
#77429=AXIS2_PLACEMENT_3D('',#162547,#91600,#91601);
#77430=AXIS2_PLACEMENT_3D('',#162548,#91602,#91603);
#77431=AXIS2_PLACEMENT_3D('',#162559,#91604,#91605);
#77432=AXIS2_PLACEMENT_3D('',#162567,#91606,#91607);
#77433=AXIS2_PLACEMENT_3D('',#162568,#91608,#91609);
#77434=AXIS2_PLACEMENT_3D('',#162579,#91610,#91611);
#77435=AXIS2_PLACEMENT_3D('',#162587,#91612,#91613);
#77436=AXIS2_PLACEMENT_3D('',#162588,#91614,#91615);
#77437=AXIS2_PLACEMENT_3D('',#162599,#91616,#91617);
#77438=AXIS2_PLACEMENT_3D('',#162607,#91618,#91619);
#77439=AXIS2_PLACEMENT_3D('',#162608,#91620,#91621);
#77440=AXIS2_PLACEMENT_3D('',#162619,#91622,#91623);
#77441=AXIS2_PLACEMENT_3D('',#162627,#91624,#91625);
#77442=AXIS2_PLACEMENT_3D('',#162628,#91626,#91627);
#77443=AXIS2_PLACEMENT_3D('',#162639,#91628,#91629);
#77444=AXIS2_PLACEMENT_3D('',#162647,#91630,#91631);
#77445=AXIS2_PLACEMENT_3D('',#162648,#91632,#91633);
#77446=AXIS2_PLACEMENT_3D('',#162659,#91634,#91635);
#77447=AXIS2_PLACEMENT_3D('',#162667,#91636,#91637);
#77448=AXIS2_PLACEMENT_3D('',#162668,#91638,#91639);
#77449=AXIS2_PLACEMENT_3D('',#162679,#91640,#91641);
#77450=AXIS2_PLACEMENT_3D('',#162687,#91642,#91643);
#77451=AXIS2_PLACEMENT_3D('',#162688,#91644,#91645);
#77452=AXIS2_PLACEMENT_3D('',#162699,#91646,#91647);
#77453=AXIS2_PLACEMENT_3D('',#162707,#91648,#91649);
#77454=AXIS2_PLACEMENT_3D('',#162708,#91650,#91651);
#77455=AXIS2_PLACEMENT_3D('',#162719,#91652,#91653);
#77456=AXIS2_PLACEMENT_3D('',#162727,#91654,#91655);
#77457=AXIS2_PLACEMENT_3D('',#162728,#91656,#91657);
#77458=AXIS2_PLACEMENT_3D('',#162739,#91658,#91659);
#77459=AXIS2_PLACEMENT_3D('',#162747,#91660,#91661);
#77460=AXIS2_PLACEMENT_3D('',#162748,#91662,#91663);
#77461=AXIS2_PLACEMENT_3D('',#162759,#91664,#91665);
#77462=AXIS2_PLACEMENT_3D('',#162767,#91666,#91667);
#77463=AXIS2_PLACEMENT_3D('',#162768,#91668,#91669);
#77464=AXIS2_PLACEMENT_3D('',#162779,#91670,#91671);
#77465=AXIS2_PLACEMENT_3D('',#162787,#91672,#91673);
#77466=AXIS2_PLACEMENT_3D('',#162788,#91674,#91675);
#77467=AXIS2_PLACEMENT_3D('',#162799,#91676,#91677);
#77468=AXIS2_PLACEMENT_3D('',#162807,#91678,#91679);
#77469=AXIS2_PLACEMENT_3D('',#162808,#91680,#91681);
#77470=AXIS2_PLACEMENT_3D('',#162819,#91682,#91683);
#77471=AXIS2_PLACEMENT_3D('',#162827,#91684,#91685);
#77472=AXIS2_PLACEMENT_3D('',#162828,#91686,#91687);
#77473=AXIS2_PLACEMENT_3D('',#162839,#91688,#91689);
#77474=AXIS2_PLACEMENT_3D('',#162847,#91690,#91691);
#77475=AXIS2_PLACEMENT_3D('',#162848,#91692,#91693);
#77476=AXIS2_PLACEMENT_3D('',#162859,#91694,#91695);
#77477=AXIS2_PLACEMENT_3D('',#162867,#91696,#91697);
#77478=AXIS2_PLACEMENT_3D('',#162868,#91698,#91699);
#77479=AXIS2_PLACEMENT_3D('',#162879,#91700,#91701);
#77480=AXIS2_PLACEMENT_3D('',#162887,#91702,#91703);
#77481=AXIS2_PLACEMENT_3D('',#162888,#91704,#91705);
#77482=AXIS2_PLACEMENT_3D('',#162899,#91706,#91707);
#77483=AXIS2_PLACEMENT_3D('',#162907,#91708,#91709);
#77484=AXIS2_PLACEMENT_3D('',#162908,#91710,#91711);
#77485=AXIS2_PLACEMENT_3D('',#162919,#91712,#91713);
#77486=AXIS2_PLACEMENT_3D('',#162927,#91714,#91715);
#77487=AXIS2_PLACEMENT_3D('',#162928,#91716,#91717);
#77488=AXIS2_PLACEMENT_3D('',#162939,#91718,#91719);
#77489=AXIS2_PLACEMENT_3D('',#162947,#91720,#91721);
#77490=AXIS2_PLACEMENT_3D('',#162948,#91722,#91723);
#77491=AXIS2_PLACEMENT_3D('',#162959,#91724,#91725);
#77492=AXIS2_PLACEMENT_3D('',#162967,#91726,#91727);
#77493=AXIS2_PLACEMENT_3D('',#162968,#91728,#91729);
#77494=AXIS2_PLACEMENT_3D('',#162979,#91730,#91731);
#77495=AXIS2_PLACEMENT_3D('',#162987,#91732,#91733);
#77496=AXIS2_PLACEMENT_3D('',#162988,#91734,#91735);
#77497=AXIS2_PLACEMENT_3D('',#162999,#91736,#91737);
#77498=AXIS2_PLACEMENT_3D('',#163007,#91738,#91739);
#77499=AXIS2_PLACEMENT_3D('',#163008,#91740,#91741);
#77500=AXIS2_PLACEMENT_3D('',#163019,#91742,#91743);
#77501=AXIS2_PLACEMENT_3D('',#163026,#91744,#91745);
#77502=AXIS2_PLACEMENT_3D('',#163051,#91747,#91748);
#77503=AXIS2_PLACEMENT_3D('',#163110,#91751,#91752);
#77504=AXIS2_PLACEMENT_3D('',#163169,#91755,#91756);
#77505=AXIS2_PLACEMENT_3D('',#163228,#91759,#91760);
#77506=AXIS2_PLACEMENT_3D('',#163287,#91763,#91764);
#77507=AXIS2_PLACEMENT_3D('',#163346,#91767,#91768);
#77508=AXIS2_PLACEMENT_3D('',#163405,#91771,#91772);
#77509=AXIS2_PLACEMENT_3D('',#163464,#91775,#91776);
#77510=AXIS2_PLACEMENT_3D('',#163523,#91779,#91780);
#77511=AXIS2_PLACEMENT_3D('',#163582,#91783,#91784);
#77512=AXIS2_PLACEMENT_3D('',#163641,#91787,#91788);
#77513=AXIS2_PLACEMENT_3D('',#163700,#91791,#91792);
#77514=AXIS2_PLACEMENT_3D('',#163759,#91795,#91796);
#77515=AXIS2_PLACEMENT_3D('',#163818,#91799,#91800);
#77516=AXIS2_PLACEMENT_3D('',#163877,#91803,#91804);
#77517=AXIS2_PLACEMENT_3D('',#163936,#91807,#91808);
#77518=AXIS2_PLACEMENT_3D('',#163995,#91811,#91812);
#77519=AXIS2_PLACEMENT_3D('',#164054,#91815,#91816);
#77520=AXIS2_PLACEMENT_3D('',#164113,#91819,#91820);
#77521=AXIS2_PLACEMENT_3D('',#164172,#91823,#91824);
#77522=AXIS2_PLACEMENT_3D('',#164231,#91827,#91828);
#77523=AXIS2_PLACEMENT_3D('',#164316,#91833,#91834);
#77524=AXIS2_PLACEMENT_3D('',#164375,#91837,#91838);
#77525=AXIS2_PLACEMENT_3D('',#164434,#91841,#91842);
#77526=AXIS2_PLACEMENT_3D('',#164493,#91845,#91846);
#77527=AXIS2_PLACEMENT_3D('',#164552,#91849,#91850);
#77528=AXIS2_PLACEMENT_3D('',#164611,#91853,#91854);
#77529=AXIS2_PLACEMENT_3D('',#164687,#91858,#91859);
#77530=AXIS2_PLACEMENT_3D('',#164688,#91860,#91861);
#77531=AXIS2_PLACEMENT_3D('',#164699,#91862,#91863);
#77532=AXIS2_PLACEMENT_3D('',#164722,#91864,#91865);
#77533=AXIS2_PLACEMENT_3D('',#164737,#91866,#91867);
#77534=AXIS2_PLACEMENT_3D('',#164753,#91868,#91869);
#77535=AXIS2_PLACEMENT_3D('',#164754,#91870,#91871);
#77536=AXIS2_PLACEMENT_3D('',#164765,#91872,#91873);
#77537=AXIS2_PLACEMENT_3D('',#164781,#91874,#91875);
#77538=AXIS2_PLACEMENT_3D('',#164782,#91876,#91877);
#77539=AXIS2_PLACEMENT_3D('',#164793,#91878,#91879);
#77540=AXIS2_PLACEMENT_3D('',#164809,#91880,#91881);
#77541=AXIS2_PLACEMENT_3D('',#164810,#91882,#91883);
#77542=AXIS2_PLACEMENT_3D('',#164821,#91884,#91885);
#77543=AXIS2_PLACEMENT_3D('',#164837,#91886,#91887);
#77544=AXIS2_PLACEMENT_3D('',#164838,#91888,#91889);
#77545=AXIS2_PLACEMENT_3D('',#164849,#91890,#91891);
#77546=AXIS2_PLACEMENT_3D('',#164865,#91892,#91893);
#77547=AXIS2_PLACEMENT_3D('',#164866,#91894,#91895);
#77548=AXIS2_PLACEMENT_3D('',#164877,#91896,#91897);
#77549=AXIS2_PLACEMENT_3D('',#164900,#91898,#91899);
#77550=AXIS2_PLACEMENT_3D('',#164915,#91900,#91901);
#77551=AXIS2_PLACEMENT_3D('',#164931,#91902,#91903);
#77552=AXIS2_PLACEMENT_3D('',#164932,#91904,#91905);
#77553=AXIS2_PLACEMENT_3D('',#164943,#91906,#91907);
#77554=AXIS2_PLACEMENT_3D('',#164959,#91908,#91909);
#77555=AXIS2_PLACEMENT_3D('',#164960,#91910,#91911);
#77556=AXIS2_PLACEMENT_3D('',#164971,#91912,#91913);
#77557=AXIS2_PLACEMENT_3D('',#164987,#91914,#91915);
#77558=AXIS2_PLACEMENT_3D('',#164988,#91916,#91917);
#77559=AXIS2_PLACEMENT_3D('',#164999,#91918,#91919);
#77560=AXIS2_PLACEMENT_3D('',#165015,#91920,#91921);
#77561=AXIS2_PLACEMENT_3D('',#165016,#91922,#91923);
#77562=AXIS2_PLACEMENT_3D('',#165027,#91924,#91925);
#77563=AXIS2_PLACEMENT_3D('',#165050,#91926,#91927);
#77564=AXIS2_PLACEMENT_3D('',#165065,#91928,#91929);
#77565=AXIS2_PLACEMENT_3D('',#165081,#91930,#91931);
#77566=AXIS2_PLACEMENT_3D('',#165082,#91932,#91933);
#77567=AXIS2_PLACEMENT_3D('',#165093,#91934,#91935);
#77568=AXIS2_PLACEMENT_3D('',#165109,#91936,#91937);
#77569=AXIS2_PLACEMENT_3D('',#165110,#91938,#91939);
#77570=AXIS2_PLACEMENT_3D('',#165121,#91940,#91941);
#77571=AXIS2_PLACEMENT_3D('',#165144,#91942,#91943);
#77572=AXIS2_PLACEMENT_3D('',#165159,#91944,#91945);
#77573=AXIS2_PLACEMENT_3D('',#165175,#91946,#91947);
#77574=AXIS2_PLACEMENT_3D('',#165176,#91948,#91949);
#77575=AXIS2_PLACEMENT_3D('',#165187,#91950,#91951);
#77576=AXIS2_PLACEMENT_3D('',#165210,#91952,#91953);
#77577=AXIS2_PLACEMENT_3D('',#165225,#91954,#91955);
#77578=AXIS2_PLACEMENT_3D('',#165241,#91956,#91957);
#77579=AXIS2_PLACEMENT_3D('',#165242,#91958,#91959);
#77580=AXIS2_PLACEMENT_3D('',#165253,#91960,#91961);
#77581=AXIS2_PLACEMENT_3D('',#165269,#91962,#91963);
#77582=AXIS2_PLACEMENT_3D('',#165270,#91964,#91965);
#77583=AXIS2_PLACEMENT_3D('',#165281,#91966,#91967);
#77584=AXIS2_PLACEMENT_3D('',#165304,#91968,#91969);
#77585=AXIS2_PLACEMENT_3D('',#165319,#91970,#91971);
#77586=AXIS2_PLACEMENT_3D('',#165342,#91972,#91973);
#77587=AXIS2_PLACEMENT_3D('',#165357,#91974,#91975);
#77588=AXIS2_PLACEMENT_3D('',#165373,#91976,#91977);
#77589=AXIS2_PLACEMENT_3D('',#165374,#91978,#91979);
#77590=AXIS2_PLACEMENT_3D('',#165385,#91980,#91981);
#77591=AXIS2_PLACEMENT_3D('',#165401,#91982,#91983);
#77592=AXIS2_PLACEMENT_3D('',#165402,#91984,#91985);
#77593=AXIS2_PLACEMENT_3D('',#165413,#91986,#91987);
#77594=AXIS2_PLACEMENT_3D('',#165429,#91988,#91989);
#77595=AXIS2_PLACEMENT_3D('',#165430,#91990,#91991);
#77596=AXIS2_PLACEMENT_3D('',#165441,#91992,#91993);
#77597=AXIS2_PLACEMENT_3D('',#165457,#91994,#91995);
#77598=AXIS2_PLACEMENT_3D('',#165458,#91996,#91997);
#77599=AXIS2_PLACEMENT_3D('',#165469,#91998,#91999);
#77600=AXIS2_PLACEMENT_3D('',#165485,#92000,#92001);
#77601=AXIS2_PLACEMENT_3D('',#165486,#92002,#92003);
#77602=AXIS2_PLACEMENT_3D('',#165497,#92004,#92005);
#77603=AXIS2_PLACEMENT_3D('',#165513,#92006,#92007);
#77604=AXIS2_PLACEMENT_3D('',#165514,#92008,#92009);
#77605=AXIS2_PLACEMENT_3D('',#165525,#92010,#92011);
#77606=AXIS2_PLACEMENT_3D('',#165541,#92012,#92013);
#77607=AXIS2_PLACEMENT_3D('',#165542,#92014,#92015);
#77608=AXIS2_PLACEMENT_3D('',#165558,#92016,#92017);
#77609=AXIS2_PLACEMENT_3D('',#165559,#92018,#92019);
#77610=AXIS2_PLACEMENT_3D('',#165624,#92021,#92022);
#77611=AXIS2_PLACEMENT_3D('',#165710,#92025,#92026);
#77612=AXIS2_PLACEMENT_3D('',#165796,#92029,#92030);
#77613=AXIS2_PLACEMENT_3D('',#165882,#92033,#92034);
#77614=AXIS2_PLACEMENT_3D('',#165967,#92037,#92038);
#77615=AXIS2_PLACEMENT_3D('',#166053,#92041,#92042);
#77616=AXIS2_PLACEMENT_3D('',#166139,#92045,#92046);
#77617=AXIS2_PLACEMENT_3D('',#166225,#92049,#92050);
#77618=AXIS2_PLACEMENT_3D('',#166311,#92053,#92054);
#77619=AXIS2_PLACEMENT_3D('',#166396,#92057,#92058);
#77620=AXIS2_PLACEMENT_3D('',#166482,#92061,#92062);
#77621=AXIS2_PLACEMENT_3D('',#166567,#92065,#92066);
#77622=AXIS2_PLACEMENT_3D('',#166652,#92069,#92070);
#77623=AXIS2_PLACEMENT_3D('',#166738,#92073,#92074);
#77624=AXIS2_PLACEMENT_3D('',#166824,#92077,#92078);
#77625=AXIS2_PLACEMENT_3D('',#166909,#92081,#92082);
#77626=AXIS2_PLACEMENT_3D('',#166994,#92085,#92086);
#77627=AXIS2_PLACEMENT_3D('',#167080,#92089,#92090);
#77628=AXIS2_PLACEMENT_3D('',#167166,#92093,#92094);
#77629=AXIS2_PLACEMENT_3D('',#167252,#92097,#92098);
#77630=AXIS2_PLACEMENT_3D('',#167337,#92101,#92102);
#77631=AXIS2_PLACEMENT_3D('',#167423,#92105,#92106);
#77632=AXIS2_PLACEMENT_3D('',#167508,#92109,#92110);
#77633=AXIS2_PLACEMENT_3D('',#167594,#92113,#92114);
#77634=AXIS2_PLACEMENT_3D('',#167678,#92117,#92118);
#77635=AXIS2_PLACEMENT_3D('',#167764,#92121,#92122);
#77636=AXIS2_PLACEMENT_3D('',#167849,#92125,#92126);
#77637=AXIS2_PLACEMENT_3D('',#167935,#92129,#92130);
#77638=AXIS2_PLACEMENT_3D('',#168021,#92133,#92134);
#77639=AXIS2_PLACEMENT_3D('',#168043,#92136,#92137);
#77640=AXIS2_PLACEMENT_3D('',#168044,#92138,#92139);
#77765=DIRECTION('axis',(0.,0.,1.));
#77766=DIRECTION('refdir',(1.,0.,0.));
#77767=DIRECTION('center_axis',(0.,1.,0.));
#77768=DIRECTION('ref_axis',(0.,0.,1.));
#77769=DIRECTION('',(8.65956056235494E-17,-0.707106781186547,0.707106781186548));
#77770=DIRECTION('center_axis',(0.186577261580871,-0.979058294102434,-0.0814480338020183));
#77771=DIRECTION('ref_axis',(-0.0274385629108201,0.0776784846658033,-0.996600811902847));
#77772=DIRECTION('center_axis',(-0.139289712626125,0.990111866841247,0.0166393238045287));
#77773=DIRECTION('ref_axis',(0.000407580413638487,0.0168604472915263,-0.999857769482908));
#77774=DIRECTION('center_axis',(0.199724107407254,-0.979058294675158,-0.0394352196411607));
#77775=DIRECTION('ref_axis',(0.187442652303081,0.077678476402867,-0.979199319036383));
#77776=DIRECTION('center_axis',(-0.139610153019225,0.990111867364969,-0.0136928914770513));
#77777=DIRECTION('ref_axis',(0.215337916268728,0.0168604199747552,-0.976394033193217));
#77778=DIRECTION('center_axis',(0.203532073931734,-0.979058294942538,0.00442153652667557));
#77779=DIRECTION('ref_axis',(0.393559261674466,0.0776784739001359,-0.916011551369738));
#77780=DIRECTION('center_axis',(-0.133402545882498,0.990111868926104,-0.043384879436559));
#77781=DIRECTION('ref_axis',(0.420199294087297,0.0168603479300273,-0.907275196352361));
#77782=DIRECTION('center_axis',(0.197823135310267,-0.979058291315529,0.0480715023931239));
#77783=DIRECTION('ref_axis',(0.581273459592952,0.077678521741375,-0.809992106401609));
#77784=DIRECTION('center_axis',(-0.120957256826932,0.990111867075851,-0.0710481012869155));
#77785=DIRECTION('ref_axis',(0.605412613918703,0.01686043573858,-0.795733179284883));
#77786=DIRECTION('center_axis',(0.182864205781083,-0.97905828956084,0.0894737273519817));
#77787=DIRECTION('ref_axis',(0.741807964226493,0.077678545281379,-0.666098331939898));
#77788=DIRECTION('center_axis',(-0.102856105182436,0.990111866931577,-0.0953892687253966));
#77789=DIRECTION('ref_axis',(0.762317512889428,0.0168604392837559,-0.646983566351754));
#77790=DIRECTION('center_axis',(0.159354699494,-0.97905829268383,0.126692301566439));
#77791=DIRECTION('ref_axis',(0.867656361984456,0.07767850292466,-0.491058537947649));
#77792=DIRECTION('center_axis',(-0.0799455264710559,0.990111866694433,-0.115270135890139));
#77793=DIRECTION('ref_axis',(0.88357729515684,0.0168604542072331,-0.467981718197676));
#77794=DIRECTION('center_axis',(0.128393954075586,-0.97905829431996,0.157986862998561));
#77795=DIRECTION('ref_axis',(0.952934112137038,0.0776784814458654,-0.293057385926133));
#77796=DIRECTION('center_axis',(-0.0532967709437696,0.990111866732091,-0.129761109594753));
#77797=DIRECTION('ref_axis',(0.963521984490172,0.0168604521778205,-0.267097567485144));
#77798=DIRECTION('center_axis',(0.0914296854463454,-0.979058293066137,0.181894121393751));
#77799=DIRECTION('ref_axis',(0.993653715773841,0.0776784969359244,-0.0813532067137727));
#77800=DIRECTION('center_axis',(-0.024155886086191,0.990111867373155,-0.138184598469708));
#77801=DIRECTION('ref_axis',(0.998413458662092,0.0168604200989514,-0.0537242198313367));
#77802=DIRECTION('center_axis',(0.0501902985567214,-0.979058289631927,0.197296222553278));
#77803=DIRECTION('ref_axis',(0.987911176146774,0.0776785442102777,0.134154954487968));
#77804=DIRECTION('center_axis',(0.00611445816865162,0.990111867197787,-0.140146722528269));
#77805=DIRECTION('ref_axis',(0.986620226468745,0.016860430695643,0.16216119942674));
#77806=DIRECTION('center_axis',(0.00660393563905987,-0.979058296281141,
0.203472947875497));
#77807=DIRECTION('ref_axis',(0.935975012728166,0.0776784552944495,0.343390205351839));
#77808=DIRECTION('center_axis',(0.036098924614116,0.990111867548585,-0.135555735331111));
#77809=DIRECTION('ref_axis',(0.928693728838714,0.0168604130010006,0.370464147373373));
#77810=DIRECTION('center_axis',(-0.0372910827158735,-0.9790582921264,0.200135543490943));
#77811=DIRECTION('ref_axis',(0.840273696303755,0.0776785094363429,0.536568881385953));
#77812=DIRECTION('center_axis',(0.0643953951618964,0.990111866740033,-0.124626339200465));
#77813=DIRECTION('ref_axis',(0.827342546146425,0.0168604531079493,0.561444597851778));
#77814=DIRECTION('center_axis',(-0.0794425096188056,-0.979058296902983,
0.187439960869863));
#77815=DIRECTION('ref_axis',(0.705282109548452,0.0776784470943857,0.70465821843493));
#77816=DIRECTION('center_axis',(0.0896808834567414,0.990111867832051,-0.107869496710356));
#77817=DIRECTION('ref_axis',(0.68730574403223,0.0168603966824033,0.726172528566053));
#77818=DIRECTION('center_axis',(-0.117879200938036,-0.979058291676625,0.165979985195381));
#77819=DIRECTION('ref_axis',(0.537312326052278,0.0776785149589982,0.839798495227311));
#77820=DIRECTION('center_axis',(0.110772921824695,0.990111866779734,-0.0860688738881277));
#77821=DIRECTION('ref_axis',(0.515131290854236,0.0168604487200701,0.85694543493259));
#77822=DIRECTION('center_axis',(-0.150804071311457,-0.979058298006792,0.136758843150757));
#77823=DIRECTION('ref_axis',(0.344218397227483,0.077678432474775,0.935670751994741));
#77824=DIRECTION('center_axis',(0.126685382972232,0.990111867284263,-0.0602437050989526));
#77825=DIRECTION('ref_axis',(0.318869870343511,0.0168604249104656,0.947648527598155));
#77826=DIRECTION('center_axis',(-0.176677455944571,-0.979058293932153,0.101143134436385));
#77827=DIRECTION('ref_axis',(0.135029217419843,0.0776784870269465,0.987792064706024));
#77828=DIRECTION('center_axis',(0.136674164628418,0.990111867169371,-0.031601633082882));
#77829=DIRECTION('ref_axis',(0.107698451602077,0.0168604294462928,0.994040627661366));
#77830=DIRECTION('center_axis',(-0.194289620685681,-0.979058292355819,0.060798054764296));
#77831=DIRECTION('ref_axis',(-0.0804737766854639,0.0776785068362268,0.993725324645434));
#77832=DIRECTION('center_axis',(0.140272217526581,0.990111866870354,-0.00148191520592742));
#77833=DIRECTION('ref_axis',(-0.108508833586371,0.0168604463599934,0.993952493020802));
#77834=DIRECTION('center_axis',(-0.202817020749949,-0.979058292691228,0.0176100995639517));
#77835=DIRECTION('ref_axis',(-0.29221392042967,0.0776785025208492,0.953193094264347));
#77836=DIRECTION('center_axis',(0.137311299111617,0.990111866871472,0.0287071109059762));
#77837=DIRECTION('ref_axis',(-0.319642362401726,0.0168604469759247,0.947388244325427));
#77838=DIRECTION('center_axis',(-0.2018608999098,-0.979058296179043,-0.0264013213797263));
#77839=DIRECTION('ref_axis',(-0.490290465295145,0.0776784543904377,0.868090615871513));
#77840=DIRECTION('center_axis',(0.12792986861175,0.990111866429095,0.0575538067661467));
#77841=DIRECTION('ref_axis',(-0.515829767335335,0.0168604685026887,0.856525175189056));
#77842=DIRECTION('center_axis',(-0.191466007942769,-0.979058295381442,-0.0691781905461903));
#77843=DIRECTION('ref_axis',(-0.665441568100258,0.0776784663688145,0.742397181639895));
#77844=DIRECTION('center_axis',(0.112566545125586,0.990111867161873,0.0837093986582129));
#77845=DIRECTION('ref_axis',(-0.687897551371201,0.0168604299311094,0.72561193810469));
#77846=DIRECTION('center_axis',(-0.172118434479679,-0.979058289748096,-0.108720328309829));
#77847=DIRECTION('ref_axis',(-0.809477352939237,0.0776785431668268,0.581990084975651));
#77848=DIRECTION('center_axis',(0.0919397456149225,0.990111867405625,0.105950805559984));
#77849=DIRECTION('ref_axis',(-0.827800004343528,0.0168604173753996,0.560769898563378));
#77850=DIRECTION('center_axis',(-0.144722724094128,-0.979058291373611,-0.143178892380688));
#77851=DIRECTION('ref_axis',(-0.915662888444695,0.0776785204361908,0.394369778492169));
#77852=DIRECTION('center_axis',(0.067013950564489,0.990111867470249,0.123238063618005));
#77853=DIRECTION('ref_axis',(-0.928995453990013,0.0168604141435253,0.369706874294756));
#77854=DIRECTION('center_axis',(-0.110559921260368,-0.979058294096825,-0.170942565123831));
#77855=DIRECTION('ref_axis',(-0.979033047708099,0.07767848352851,0.188309173149113));
#77856=DIRECTION('center_axis',(0.0389546925791882,0.990111866893729,0.134762839693577));
#77857=DIRECTION('ref_axis',(-0.986752105339078,0.0168604464197057,0.161356772263904));
#77858=DIRECTION('center_axis',(-0.071227498148321,-0.979058293753717,-0.190713137826399));
#77859=DIRECTION('ref_axis',(-0.996624704500865,0.0776784888229868,-0.0265565576221803));
#77860=DIRECTION('center_axis',(0.00907392544468187,0.990111866858401,0.139986267123585));
#77861=DIRECTION('ref_axis',(-0.998369325900615,0.0168604452007894,-0.0545381929328624));
#77862=DIRECTION('center_axis',(-0.0285645023421519,-0.979058297482466,
-0.20156616615067));
#77863=DIRECTION('ref_axis',(-0.967615298794827,0.0776784396145497,-0.240180543669228));
#77864=DIRECTION('center_axis',(-0.021231159700138,0.990111867542855,0.138664081897897));
#77865=DIRECTION('ref_axis',(-0.963303907751991,0.0168604107174527,-0.267883011518427));
#77866=DIRECTION('center_axis',(0.0154340398695587,-0.979058293642597,-0.202994206968947));
#77867=DIRECTION('ref_axis',(-0.893361276330957,0.0776784901989675,-0.442573928415053));
#77868=DIRECTION('center_axis',(-0.0505434286098618,0.99011186673401,0.130858141423657));
#77869=DIRECTION('ref_axis',(-0.883195468264391,0.0168604534636805,-0.468701920143541));
#77870=DIRECTION('center_axis',(0.058710979286812,-0.979058295945962,-0.194930433874684));
#77871=DIRECTION('ref_axis',(-0.777334668183151,0.0776784608195143,-0.624273073554595));
#77872=DIRECTION('center_axis',(-0.0774924111311011,0.990111867436745,0.11693338350535));
#77873=DIRECTION('ref_axis',(-0.761789790422962,0.0168604166683029,-0.647604849856077));
#77874=DIRECTION('center_axis',(0.0992425885922905,-0.979058291277952,-0.177751992645369));
#77875=DIRECTION('ref_axis',(-0.624960765663839,0.0776785237983946,-0.77678187950117));
#77876=DIRECTION('center_axis',(-0.100817900230145,0.990111867381094,0.0975409712085529));
#77877=DIRECTION('ref_axis',(-0.60476366781866,0.0168604206335193,-0.796226495604474));
#77878=DIRECTION('center_axis',(0.135133781652856,-0.979058291913772,-0.152262017887209));
#77879=DIRECTION('ref_axis',(-0.443364387932586,0.0776785131344228,-0.89296924253324));
#77880=DIRECTION('center_axis',(-0.119429263971459,0.990111867544092,0.0735876392853213));
#77881=DIRECTION('ref_axis',(-0.419459468051624,0.0168604098023566,-0.907617475175057));
#77882=DIRECTION('center_axis',(0.164706260161333,-0.979058291532398,-0.119652453570032));
#77883=DIRECTION('ref_axis',(-0.24103677993988,0.077678519808337,-0.96740235593914));
#77884=DIRECTION('center_axis',(-0.132456237944713,0.990111867284881,0.0461934550686622));
#77885=DIRECTION('ref_axis',(-0.214541811918642,0.016860425481317,-0.976569268916064));
#77886=DIRECTION('',(8.65956056235494E-17,-0.707106781186547,0.707106781186548));
#77887=DIRECTION('center_axis',(0.,-1.,0.));
#77888=DIRECTION('ref_axis',(0.,0.,1.));
#77889=DIRECTION('center_axis',(1.00080200537124E-16,-1.,0.));
#77890=DIRECTION('ref_axis',(1.,1.00080200537124E-16,0.));
#77891=DIRECTION('center_axis',(-1.00080200537124E-16,1.,0.));
#77892=DIRECTION('ref_axis',(1.,1.00080200537124E-16,0.));
#77893=DIRECTION('',(1.00080200537124E-16,-1.,0.));
#77894=DIRECTION('center_axis',(1.00080200537124E-16,-1.,0.));
#77895=DIRECTION('ref_axis',(1.,1.00080200537124E-16,0.));
#77896=DIRECTION('center_axis',(0.,1.,0.));
#77897=DIRECTION('ref_axis',(0.,0.,1.));
#77898=DIRECTION('center_axis',(0.,-1.,0.));
#77899=DIRECTION('ref_axis',(0.,0.,-1.));
#77900=DIRECTION('center_axis',(0.,1.,0.));
#77901=DIRECTION('ref_axis',(0.,0.,-1.));
#77902=DIRECTION('',(0.,-1.,0.));
#77903=DIRECTION('center_axis',(0.,1.,0.));
#77904=DIRECTION('ref_axis',(0.,0.,-1.));
#77905=DIRECTION('center_axis',(-1.41610079671576E-16,-1.,0.));
#77906=DIRECTION('ref_axis',(1.,-1.41610079671576E-16,0.));
#77907=DIRECTION('center_axis',(0.,1.,0.));
#77908=DIRECTION('ref_axis',(0.,0.,-1.));
#77909=DIRECTION('',(-1.41610079671576E-16,-1.,0.));
#77910=DIRECTION('center_axis',(1.41610079671576E-16,1.,0.));
#77911=DIRECTION('ref_axis',(1.,-1.41610079671576E-16,0.));
#77912=DIRECTION('center_axis',(0.,1.,0.));
#77913=DIRECTION('ref_axis',(0.,0.,-1.));
#77914=DIRECTION('center_axis',(1.41610079671576E-16,1.,0.));
#77915=DIRECTION('ref_axis',(-1.,1.41610079671576E-16,0.));
#77916=DIRECTION('',(0.707106781186548,0.707106781186547,-8.65956056235493E-17));
#77917=DIRECTION('center_axis',(0.,1.,0.));
#77918=DIRECTION('ref_axis',(0.,0.,1.));
#77919=DIRECTION('center_axis',(-2.19359866955191E-16,-1.,2.19359867215408E-16));
#77920=DIRECTION('ref_axis',(8.25587254851516E-33,-2.19359867215408E-16,
-1.));
#77921=DIRECTION('center_axis',(-0.132456237432219,-0.990111867233412,0.0461934576413813));
#77922=DIRECTION('ref_axis',(-0.17180492619258,-0.0229646841998517,-0.984863285240933));
#77923=DIRECTION('center_axis',(0.164706267778703,0.979058293558939,-0.119652426502217));
#77924=DIRECTION('ref_axis',(-0.277967410339795,-0.0703182237971854,-0.958013291239217));
#77925=DIRECTION('center_axis',(-0.119429259911198,-0.990111867327141,0.0735876487939799));
#77926=DIRECTION('ref_axis',(-0.379504716404044,-0.0229646761552871,-0.92490474854234));
#77927=DIRECTION('center_axis',(0.135133794647117,0.97905829393374,-0.152261993366125));
#77928=DIRECTION('ref_axis',(-0.477413223582112,-0.0703182187181641,-0.875860697865386));
#77929=DIRECTION('center_axis',(-0.100817898675726,-0.990111867329304,0.0975409733409004));
#77930=DIRECTION('ref_axis',(-0.569459287429209,-0.0229646794472329,-0.821698693840086));
#77931=DIRECTION('center_axis',(0.0992426063939419,0.979058293251314,-0.177751971837055));
#77932=DIRECTION('ref_axis',(-0.654535729064363,-0.0703182292933112,-0.752753828291319));
#77933=DIRECTION('center_axis',(-0.0774924094683679,-0.990111867394032,
0.116933384968924));
#77934=DIRECTION('ref_axis',(-0.732786575137973,-0.0229646753529087,-0.680070922024678));
#77935=DIRECTION('center_axis',(0.0587110024176738,0.979058298035316,-0.194930416413916));
#77936=DIRECTION('ref_axis',(-0.801052866818017,-0.0703181640084746,-0.594449039340728));
#77937=DIRECTION('center_axis',(-0.0505434261743817,-0.990111866679012,
0.130858142780482));
#77938=DIRECTION('ref_axis',(-0.861849579756916,-0.0229647121534493,-0.506643784002663));
#77939=DIRECTION('center_axis',(0.0154340585899416,0.97905829512376,-0.202994198401821));
#77940=DIRECTION('ref_axis',(-0.910113666004715,-0.0703182038275187,-0.408348460462299));
#77941=DIRECTION('center_axis',(-0.0212311576904246,-0.990111867502716,
0.138664082492217));
#77942=DIRECTION('ref_axis',(-0.950613451622889,-0.0229646696475091,-0.309526557086138));
#77943=DIRECTION('center_axis',(-0.0285644827311666,0.979058298926961,-0.201566161913518));
#77944=DIRECTION('ref_axis',(-0.976618566039829,-0.0703181511606769,-0.20315396644824));
#77945=DIRECTION('center_axis',(0.00907392867735618,-0.990111866793656,
0.139986267371983));
#77946=DIRECTION('ref_axis',(-0.994927697509577,-0.0229647039748019,-0.097936199128008));
#77947=DIRECTION('center_axis',(-0.0712274703710536,0.979058295754626,-0.19071313792864));
#77948=DIRECTION('ref_axis',(-0.997457861197093,-0.0703181955432002,0.011539779532913));
#77949=DIRECTION('center_axis',(0.0389546957459753,-0.990111866829932,0.134762839246897));
#77950=DIRECTION('ref_axis',(-0.992720228666671,-0.0229647050205448,0.118233539739415));
#77951=DIRECTION('center_axis',(-0.11055990363582,0.979058295394851,-0.17094256908847));
#77952=DIRECTION('ref_axis',(-0.9716571385588,-0.0703182001743572,0.225693942789707));
#77953=DIRECTION('center_axis',(0.067013960412375,-0.99011186725026,0.123238060030383));
#77954=DIRECTION('ref_axis',(-0.94409426681622,-0.0229646803965615,0.328874807212452));
#77955=DIRECTION('center_axis',(-0.144722697903038,0.979058293473277,-0.143178904496649));
#77956=DIRECTION('ref_axis',(-0.900422803742289,-0.0703182258289589,0.42929491217244));
#77957=DIRECTION('center_axis',(0.0919397473787764,-0.990111867365221,0.105950804406956));
#77958=DIRECTION('ref_axis',(-0.851323506878691,-0.0229646761936634,0.524138254931929));
#77959=DIRECTION('center_axis',(-0.172118405928228,0.979058292352157,-0.10872035006016));
#77960=DIRECTION('ref_axis',(-0.787085695174323,-0.0703182391658995,0.612822530340196));
#77961=DIRECTION('center_axis',(0.112566547260454,-0.990111867101572,0.0837093965006225));
#77962=DIRECTION('ref_axis',(-0.718745802161697,-0.0229646885380385,0.694893585346195));
#77963=DIRECTION('center_axis',(-0.191465991434706,0.979058297226015,-0.0691782101302217));
#77964=DIRECTION('ref_axis',(-0.636945360128415,-0.0703181754281751,0.767695227558004));
#77965=DIRECTION('center_axis',(0.127929874677976,-0.990111866193421,0.0575537973365679));
#77966=DIRECTION('ref_axis',(-0.552560338942516,-0.0229647350323582,0.833156463560492));
#77967=DIRECTION('center_axis',(-0.201860887006352,0.979058298183124,-0.0264013457190201));
#77968=DIRECTION('ref_axis',(-0.457022157547164,-0.0703181629482099,0.886671361593755));
#77969=DIRECTION('center_axis',(0.137311300220315,-0.990111866806451,0.0287071078454626));
#77970=DIRECTION('ref_axis',(-0.360537777972085,-0.022964705770711,0.932461866750494));
#77971=DIRECTION('center_axis',(-0.202817012634927,0.979058294905287,0.017610069931631));
#77972=DIRECTION('ref_axis',(-0.25572908737288,-0.0703182060782421,0.964187732635804));
#77973=DIRECTION('center_axis',(0.140272217935505,-0.990111866807758,-0.00148191832138533));
#77974=DIRECTION('ref_axis',(-0.151656867142916,-0.0229647050615583,0.988166391337932));
#77975=DIRECTION('center_axis',(-0.194289619523623,0.979058294022983,0.0607980316307452));
#77976=DIRECTION('ref_axis',(-0.0424784197587449,-0.0703182187381587,0.996619752949084));
#77977=DIRECTION('center_axis',(0.136674163840837,-0.990111866959273,-0.0316016430716887));
#77978=DIRECTION('ref_axis',(0.064315347849392,-0.0229646960050964,0.99766535409846));
#77979=DIRECTION('center_axis',(-0.176677458323459,0.979058295023467,0.101143119717087));
#77980=DIRECTION('ref_axis',(0.172758496808971,-0.0703182041316549,0.982450941242362));
#77981=DIRECTION('',(2.41706455067744E-16,0.707106781186547,-0.707106781186548));
#77982=DIRECTION('center_axis',(0.,1.,0.));
#77983=DIRECTION('ref_axis',(0.,0.,-1.));
#77984=DIRECTION('center_axis',(0.126685420716261,-0.990111870073335,-0.0602435798888724));
#77985=DIRECTION('ref_axis',(0.277280230621252,-0.0229645520370101,0.960514603249927));
#77986=DIRECTION('center_axis',(-0.150804080106185,0.979058299695095,0.136758821366216));
#77987=DIRECTION('ref_axis',(0.379917397187823,-0.0703181421635682,0.922343824285008));
#77988=DIRECTION('center_axis',(0.110772920956554,-0.990111866747598,-0.0860688753751264));
#77989=DIRECTION('ref_axis',(0.477279840221599,-0.0229647061293327,0.878451237343564));
#77990=DIRECTION('center_axis',(-0.117879212274808,0.979058293114798,0.165979968660709));
#77991=DIRECTION('ref_axis',(0.569311805615098,-0.0703182285970028,0.81910891504992));
#77992=DIRECTION('center_axis',(0.0896809564689254,-0.990111870174351,-0.107869414509709));
#77993=DIRECTION('ref_axis',(0.654962335239065,-0.0229645446167437,0.755312497651625));
#77994=DIRECTION('center_axis',(-0.079442525689017,0.979058298513707,0.18743994564552));
#77995=DIRECTION('ref_axis',(0.732085813543258,-0.0703181579044715,0.677573404346442));
#77996=DIRECTION('center_axis',(0.0643953874484482,-0.990111866540803,-0.124626344768881));
#77997=DIRECTION('ref_axis',(0.802019552937378,-0.0229647181121548,0.596856145505898));
#77998=DIRECTION('center_axis',(-0.0372911082222741,0.979058294286732,0.200135528170063));
#77999=DIRECTION('ref_axis',(0.860628304192011,-0.0703182148874076,0.504355302022922));
#78000=DIRECTION('center_axis',(0.0360989233961526,-0.99011186752518,-0.135555735826411));
#78001=DIRECTION('ref_axis',(0.911575207860454,-0.0229646702411923,0.41049149118451));
#78002=DIRECTION('center_axis',(0.00660391626934577,0.979058297745836,0.203472941456433));
#78003=DIRECTION('ref_axis',(0.948928776319299,-0.0703181684385485,0.307554113385929));
#78004=DIRECTION('center_axis',(0.00611444907722728,-0.990111867003953,
-0.140146724294321));
#78005=DIRECTION('ref_axis',(0.978506622816256,-0.0229646957655209,0.204932700790093));
#78006=DIRECTION('center_axis',(0.0501902716064893,0.979058291601222,0.197296219636775));
#78007=DIRECTION('ref_axis',(0.992858387487948,-0.0703182513499916,0.0963720183554905));
#78008=DIRECTION('center_axis',(-0.0241558955906642,-0.990111867174055,
-0.138184598234822));
#78009=DIRECTION('ref_axis',(0.99968415489381,-0.0229646848998216,-0.0102085112382318));
#78010=DIRECTION('center_axis',(0.0914296553058276,0.979058295267563,0.181894124694642));
#78011=DIRECTION('ref_axis',(0.990363050457822,-0.0703182019202536,-0.119316297154157));
#78012=DIRECTION('center_axis',(-0.0532966435780096,-0.990111869527684,
-0.129761140576499));
#78013=DIRECTION('ref_axis',(0.974117573573207,-0.022964579190007,-0.224872365928926));
#78014=DIRECTION('center_axis',(0.128393931794312,0.979058296012373,0.157986870618246));
#78015=DIRECTION('ref_axis',(0.941559434212215,-0.07031819095881,-0.329425536147783));
#78016=DIRECTION('center_axis',(-0.0799455276086676,-0.990111866671711,
-0.115270135296317));
#78017=DIRECTION('ref_axis',(0.903002322585386,-0.0229647115823865,-0.429021476650454));
#78018=DIRECTION('center_axis',(0.159354683412349,0.979058294034251,0.126692311358236));
#78019=DIRECTION('ref_axis',(0.848729542341873,-0.0703182181081923,-0.52413119746705));
#78020=DIRECTION('center_axis',(-0.102856112067682,-0.990111866747235,-0.0953892632146105));
#78021=DIRECTION('ref_axis',(0.789663694904801,-0.0229647044494264,-0.613109999346649));
#78022=DIRECTION('center_axis',(0.182864183474596,0.979058291793841,0.0894737485070039));
#78023=DIRECTION('ref_axis',(0.716213996241899,-0.0703182473574262,-0.694329068724469));
#78024=DIRECTION('center_axis',(-0.120957257720643,-0.990111867049381,-0.0710481001342749));
#78025=DIRECTION('ref_axis',(0.639401271429582,-0.0229646931575987,-0.768530179604166));
#78026=DIRECTION('center_axis',(0.197823121059548,0.979058293153051,0.0480715236131955));
#78027=DIRECTION('ref_axis',(0.550209090024204,-0.0703182290405912,-0.832060877532006));
#78028=DIRECTION('center_axis',(-0.133402538460898,-0.990111869283228,-0.0433848941068217));
#78029=DIRECTION('ref_axis',(0.459241170939672,-0.0229645894669955,-0.888014737796942));
#78030=DIRECTION('center_axis',(0.20353206298097,0.979058297093515,0.0044215643223696));
#78031=DIRECTION('ref_axis',(0.358477019304043,-0.0703181752952904,-0.930886448958212));
#78032=DIRECTION('center_axis',(-0.139610155127693,-0.990111867183911,-0.0136928830715721));
#78033=DIRECTION('ref_axis',(0.25760743208348,-0.0229646850592621,-0.965976725483324));
#78034=DIRECTION('center_axis',(0.199724103311477,0.979058296518537,-0.0394351946191106));
#78035=DIRECTION('ref_axis',(0.149982958526831,-0.0703181840904617,-0.98618480273109));
#78036=DIRECTION('center_axis',(-0.139289712644573,-0.990111866811864,0.0166393253985151));
#78037=DIRECTION('ref_axis',(0.0439282684083753,-0.0229647047719847,-0.998770709206761));
#78038=DIRECTION('center_axis',(0.186577263105276,0.979058295973938,-0.0814480078132881));
#78039=DIRECTION('ref_axis',(-0.0655241373408622,-0.0703181926540497,-0.995370252322021));
#78040=DIRECTION('center_axis',(-7.60853361304994E-16,1.,9.435877229074E-15));
#78041=DIRECTION('ref_axis',(3.09497666338474E-33,-9.435877229074E-15,1.));
#78042=DIRECTION('center_axis',(-0.176808658942607,0.98271042847198,-0.0549446257183899));
#78043=DIRECTION('ref_axis',(-0.186626169750472,0.0213383782231432,0.982199239655109));
#78044=DIRECTION('center_axis',(-0.135281219501057,-0.990789414020337,0.00594379639156948));
#78045=DIRECTION('ref_axis',(0.057133312143485,-0.00181167293401717,0.998364914490035));
#78046=DIRECTION('center_axis',(3.05467988155942E-15,1.,7.62291531082259E-17));
#78047=DIRECTION('ref_axis',(-1.,3.05467988155942E-15,-2.11360725830771E-35));
#78048=DIRECTION('center_axis',(-0.0132749943721122,-0.990789503434023,
-0.134758800860587));
#78049=DIRECTION('ref_axis',(-0.993807435046363,-0.00179566446072954,0.111101564506143));
#78050=DIRECTION('center_axis',(-1.85512445524357E-14,-1.,-4.76054075061197E-16));
#78051=DIRECTION('ref_axis',(1.,-1.85512445524357E-14,-1.98009382376506E-33));
#78052=DIRECTION('center_axis',(-0.0168422547262398,0.987363722175752,0.157572899278335));
#78053=DIRECTION('ref_axis',(0.999535337253718,0.0126220396434726,0.0277451562679874));
#78054=DIRECTION('center_axis',(-0.0337801347625192,-0.987363722337789,
0.15482823484976));
#78055=DIRECTION('ref_axis',(0.994438499473259,-0.0177432088148472,0.103813531422087));
#78056=DIRECTION('center_axis',(-2.55442508253129E-28,-1.,1.25044650541671E-14));
#78057=DIRECTION('ref_axis',(-2.04281036531029E-14,1.25044650541671E-14,
1.));
#78058=DIRECTION('center_axis',(-0.00706164953990097,-0.987363724136274,
-0.158313010727242));
#78059=DIRECTION('ref_axis',(0.99876285352069,0.000828878792820405,-0.0497199697018763));
#78060=DIRECTION('center_axis',(2.48501675249087E-15,-1.,4.74426298407864E-14));
#78061=DIRECTION('ref_axis',(-5.11224396500914E-33,-4.74426298407864E-14,
-1.));
#78062=DIRECTION('center_axis',(-0.158463153814555,-0.987363722560973,-0.0015192938104477));
#78063=DIRECTION('ref_axis',(-0.0274754674163315,0.00594769935929276,-0.999604783683324));
#78064=DIRECTION('center_axis',(-0.15769850577066,0.987363722272492,0.0156224587664822));
#78065=DIRECTION('ref_axis',(-0.103719826367577,-0.00082873932965462,-0.99460620891356));
#78066=DIRECTION('center_axis',(9.74404812678745E-14,-1.,-8.14357426664195E-15));
#78067=DIRECTION('ref_axis',(1.,9.74404812678745E-14,3.07580761015643E-31));
#78068=DIRECTION('center_axis',(0.0182306309460133,0.990568175243044,-0.135802556275557));
#78069=DIRECTION('ref_axis',(0.998320981674736,-0.010565373254294,0.0569525279156969));
#78070=DIRECTION('center_axis',(6.38404008822679E-15,-1.,-2.3030484033016E-13));
#78071=DIRECTION('ref_axis',(-2.77453764336849E-31,2.3030484033016E-13,
-1.));
#78072=DIRECTION('center_axis',(-0.134616404784531,0.990568175273701,-0.0255560892512512));
#78073=DIRECTION('ref_axis',(0.110917009834759,-0.0105653661152137,-0.9937735103977));
#78074=DIRECTION('center_axis',(-2.22618915808562E-14,-1.,-5.55542708669342E-16));
#78075=DIRECTION('ref_axis',(1.,-2.22618915808562E-14,2.18343570758325E-34));
#78076=DIRECTION('center_axis',(0.0197674306362294,0.987366228452097,0.157216982537903));
#78077=DIRECTION('ref_axis',(0.999508415206963,-0.0233430450078669,0.0209291705575077));
#78078=DIRECTION('center_axis',(0.000293086686366353,-0.987363722527596,
0.158470166077536));
#78079=DIRECTION('ref_axis',(0.995082110070574,0.0159849159468142,0.097755187482131));
#78080=DIRECTION('center_axis',(1.18727964638572E-13,-1.,3.04674604886636E-15));
#78081=DIRECTION('ref_axis',(1.,1.18727964638572E-13,1.30307348022364E-31));
#78082=DIRECTION('center_axis',(0.,1.,1.27213054916354E-15));
#78083=DIRECTION('ref_axis',(0.,1.27213054916354E-15,-1.));
#78084=DIRECTION('center_axis',(-0.0337729883191399,0.987363878725217,0.154828796574441));
#78085=DIRECTION('ref_axis',(0.998165425040037,0.0255338649981846,0.0548981419803683));
#78086=DIRECTION('center_axis',(-0.0168421293105201,-0.98736372378855,0.157572902577489));
#78087=DIRECTION('ref_axis',(0.994871215031476,-0.000828295926089754,0.101146326812457));
#78088=DIRECTION('center_axis',(-0.00706160151274273,0.987363724410389,
-0.158313011159923));
#78089=DIRECTION('ref_axis',(0.99997506488799,0.00696332996270449,-0.00117543102288484));
#78090=DIRECTION('center_axis',(-7.86340814423373E-13,-1.,-1.99922748743582E-14));
#78091=DIRECTION('ref_axis',(1.,-7.86340814423373E-13,4.46218307380314E-31));
#78092=DIRECTION('center_axis',(0.0312919785426607,0.983673454219395,0.177221182545905));
#78093=DIRECTION('ref_axis',(0.987338299412827,-0.00283415220946001,-0.158603436576389));
#78094=DIRECTION('center_axis',(-4.10830010678278E-15,-1.,-7.78005123770473E-14));
#78095=DIRECTION('ref_axis',(-7.54086921167661E-33,7.78005123770473E-14,
-1.));
#78096=DIRECTION('center_axis',(-0.154562215376398,-0.987363722188387,0.0349771594649241));
#78097=DIRECTION('ref_axis',(-0.0341799369672018,-0.0300375664419585,-0.998964201816643));
#78098=DIRECTION('center_axis',(0.,-1.,0.));
#78099=DIRECTION('ref_axis',(0.,0.,-1.));
#78100=DIRECTION('center_axis',(-0.15769850569658,-0.987363722272805,0.0156224594944755));
#78101=DIRECTION('ref_axis',(-0.030668260820034,-0.0109157756374432,-0.999470011366278));
#78102=DIRECTION('center_axis',(-0.158463153814891,0.987363722560907,-0.00151929381848589));
#78103=DIRECTION('ref_axis',(-0.101017486121261,-0.0177430370825393,-0.994726420747347));
#78104=DIRECTION('center_axis',(-1.48410173663198E-14,-1.,-3.79995350315268E-16));
#78105=DIRECTION('ref_axis',(1.,-1.48410173663198E-14,-3.46998329439956E-33));
#78106=DIRECTION('center_axis',(-0.0144017677944871,0.987363722001651,0.157814668391251));
#78107=DIRECTION('ref_axis',(0.999573197091345,0.010204689755033,0.0273731248415481));
#78108=DIRECTION('center_axis',(-0.0361720565029735,-0.987363723272852,
0.154286941421227));
#78109=DIRECTION('ref_axis',(0.994359178185766,-0.0201564605092843,0.104132328589471));
#78110=DIRECTION('center_axis',(1.48412610539896E-13,-1.,3.70361805778659E-15));
#78111=DIRECTION('ref_axis',(1.,1.48412610539896E-13,-1.33068137671809E-31));
#78112=DIRECTION('center_axis',(0.000293086690297423,0.987363722527305,
0.158470166079342));
#78113=DIRECTION('ref_axis',(0.999682616725007,-0.00428129299861851,0.0248261222929015));
#78114=DIRECTION('center_axis',(0.019767304632634,-0.987366232852948,0.157216970742152));
#78115=DIRECTION('ref_axis',(0.994881286324056,0.0350112846596324,0.0947915400691157));
#78116=DIRECTION('center_axis',(4.9720804442767E-15,-1.,9.49634653907226E-14));
#78117=DIRECTION('ref_axis',(-6.2871554490736E-32,-9.49634653907226E-14,
-1.));
#78118=DIRECTION('center_axis',(-0.158467690148794,-0.98736372246051,0.000933138698494708));
#78119=DIRECTION('ref_axis',(-0.0278902213647363,0.00353155478491395,-0.999604753726705));
#78120=DIRECTION('center_axis',(-0.157921387631135,0.98736372262811,0.0131800821931044));
#78121=DIRECTION('ref_axis',(-0.0301712582658057,0.00851653398384107,-0.999508461106538));
#78122=DIRECTION('center_axis',(-6.57328045624156E-15,-1.,-1.24480823416616E-13));
#78123=DIRECTION('ref_axis',(2.84794430263569E-31,1.24480823416616E-13,
-1.));
#78124=DIRECTION('center_axis',(-0.154562215376524,0.987363722188496,0.0349771594612696));
#78125=DIRECTION('ref_axis',(-0.107590663502521,0.0183708777819135,-0.994025532859498));
#78126=DIRECTION('center_axis',(2.96824138671882E-14,-1.,7.45035423054637E-16));
#78127=DIRECTION('ref_axis',(1.,2.96824138671882E-14,7.65123809267896E-33));
#78128=DIRECTION('center_axis',(-0.0021592520811022,-0.987363722029701,
0.158455728991117));
#78129=DIRECTION('ref_axis',(0.995065899253389,0.0135962687787092,0.0982801995233089));
#78130=DIRECTION('center_axis',(-1.64176650023047E-15,-1.,-3.10613620490506E-14));
#78131=DIRECTION('ref_axis',(1.6108732260432E-32,3.10613620490506E-14,-1.));
#78132=DIRECTION('center_axis',(-0.154002427947643,-0.987363722886881,0.0373648352490626));
#78133=DIRECTION('ref_axis',(-0.0344441834552631,-0.0324282855855283,-0.998880375480509));
#78134=DIRECTION('center_axis',(0.,-1.,0.));
#78135=DIRECTION('ref_axis',(0.,0.,-1.));
#78136=DIRECTION('center_axis',(-0.157921391999,-0.987363722490913,0.0131800401359445));
#78137=DIRECTION('ref_axis',(-0.103290603183284,0.00324330582810751,-0.994645933114563));
#78138=DIRECTION('center_axis',(-0.158467690148881,0.9873637224605,0.000933138694840477));
#78139=DIRECTION('ref_axis',(-0.101358811973182,-0.0153275572955993,-0.994731851919267));
#78140=DIRECTION('center_axis',(7.42052235095029E-15,-1.,1.89466780213044E-16));
#78141=DIRECTION('ref_axis',(1.,7.42052235095029E-15,1.87127582003944E-33));
#78142=DIRECTION('center_axis',(-0.0119578465267453,0.987363721826008,0.158018640445792));
#78143=DIRECTION('ref_axis',(0.994954618366562,-0.00399376455237794,0.100246482410856));
#78144=DIRECTION('center_axis',(-0.0385553989335021,-0.987363721912245,
0.153708691571677));
#78145=DIRECTION('ref_axis',(0.994276083765525,-0.0225679920880593,0.104430622831643));
#78146=DIRECTION('center_axis',(-8.90472416013529E-14,-1.,-2.23510626916282E-15));
#78147=DIRECTION('ref_axis',(1.,-8.90472416013529E-14,4.2396213639188E-33));
#78148=DIRECTION('center_axis',(-0.0021592520907733,0.987363722029776,0.158455728990515));
#78149=DIRECTION('ref_axis',(0.999678494100297,-0.00187187841216595,0.0252864490305052));
#78150=DIRECTION('center_axis',(3.31562974260561E-15,-1.,6.33437378569497E-14));
#78151=DIRECTION('ref_axis',(8.73037930690793E-32,-6.33437378569497E-14,
-1.));
#78152=DIRECTION('center_axis',(-0.158434275571817,-0.987363722236215,0.00338531178472703));
#78153=DIRECTION('ref_axis',(-0.0283192539122514,0.00111690203907079,-0.999598305514614));
#78154=DIRECTION('center_axis',(-0.158106451168979,0.9873637206975,0.0107346704253699));
#78155=DIRECTION('ref_axis',(-0.0296886063097194,0.00611302356839794,-0.999540503230479));
#78156=DIRECTION('center_axis',(-1.31341320018242E-14,-1.,-2.48490896391667E-13));
#78157=DIRECTION('ref_axis',(2.71489283531412E-31,2.48490896391667E-13,
-1.));
#78158=DIRECTION('center_axis',(-0.154002427947475,0.987363722886904,0.0373648352491493));
#78159=DIRECTION('ref_axis',(-0.108056979266439,0.0207592358981631,-0.993927936702021));
#78160=DIRECTION('center_axis',(-8.90469496711449E-14,-1.,-2.24670375016886E-15));
#78161=DIRECTION('ref_axis',(1.,-8.90469496711449E-14,4.9175005361357E-33));
#78162=DIRECTION('center_axis',(-0.00461116000528831,-0.987363722279733,
0.158403336862949));
#78163=DIRECTION('ref_axis',(0.995045043403193,0.0112022349341195,0.0987920620860687));
#78164=DIRECTION('center_axis',(-1.48410446953476E-14,-1.,-3.7893356050524E-16));
#78165=DIRECTION('ref_axis',(1.,-1.48410446953476E-14,7.48510576451842E-33));
#78166=DIRECTION('center_axis',(-0.0385554684073366,0.987363720853985,0.153708680943092));
#78167=DIRECTION('ref_axis',(0.998951850321529,0.0342871341096827,0.0303247947023321));
#78168=DIRECTION('center_axis',(-0.0119578595718116,-0.987363721877783,
0.158018639135111));
#78169=DIRECTION('ref_axis',(0.99960551080179,-0.00778744826191416,0.0269847813454248));
#78170=DIRECTION('center_axis',(-1.64083644641347E-15,-1.,-3.1026163518096E-14));
#78171=DIRECTION('ref_axis',(-4.16554257031589E-32,3.1026163518096E-14,
-1.));
#78172=DIRECTION('center_axis',(-0.153405755446833,-0.987363722291718,0.0397436044921545));
#78173=DIRECTION('ref_axis',(-0.0346645641532703,-0.0348178308286464,-0.998792314071575));
#78174=DIRECTION('center_axis',(-8.28907435649917E-15,-1.,-1.58359344641865E-13));
#78175=DIRECTION('ref_axis',(-1.73313891738106E-31,1.58359344641865E-13,
-1.));
#78176=DIRECTION('center_axis',(-0.158106468985132,-0.987363719717749,0.0107344981337491));
#78177=DIRECTION('ref_axis',(-0.102875893860418,0.00565948901390946,-0.994678099008177));
#78178=DIRECTION('center_axis',(-0.158434275572002,0.987363722236204,0.00338531177914169));
#78179=DIRECTION('ref_axis',(-0.101715674405555,-0.0129109249611921,-0.994729726909209));
#78180=DIRECTION('center_axis',(1.0388754068593E-13,-1.,2.64359607576203E-15));
#78181=DIRECTION('ref_axis',(1.,1.0388754068593E-13,5.92047222134529E-32));
#78182=DIRECTION('center_axis',(-0.00951105075573686,0.987363721760132,
0.158184768121028));
#78183=DIRECTION('ref_axis',(0.994989346787542,-0.00640051446526875,0.099775914898743));
#78184=DIRECTION('center_axis',(-1.65804226685395E-15,-1.,-3.16805598989081E-14));
#78185=DIRECTION('ref_axis',(-1.16984757162064E-32,3.16805598989081E-14,
-1.));
#78186=DIRECTION('center_axis',(-0.158362916658971,-0.987363722017152,0.0058367004121401));
#78187=DIRECTION('ref_axis',(-0.0287622556155261,-0.00129577990078118,-0.999585440873543));
#78188=DIRECTION('center_axis',(-0.158253626805769,0.987363722312596,0.00828670403938214));
#78189=DIRECTION('ref_axis',(0.00319663291263429,0.00890473459932685,-0.999955242618257));
#78190=DIRECTION('center_axis',(8.20418223212712E-15,-1.,1.55130817591217E-13));
#78191=DIRECTION('ref_axis',(-9.2586468910808E-32,-1.55130817591217E-13,
-1.));
#78192=DIRECTION('center_axis',(-0.15340575544681,0.987363722291716,0.0397436044922978));
#78193=DIRECTION('ref_axis',(-0.108481104460266,0.0231492387674881,-0.993828940371313));
#78194=DIRECTION('center_axis',(8.90466898519274E-14,-1.,2.25697728440651E-15));
#78195=DIRECTION('ref_axis',(1.,8.90466898519274E-14,5.52639293368189E-33));
#78196=DIRECTION('center_axis',(-0.00706194294935648,-0.987363722357662,
0.158313008732074));
#78197=DIRECTION('ref_axis',(0.995019539373588,0.00880345907900943,0.0992905603419373));
#78198=DIRECTION('center_axis',(1.48410772232726E-14,-1.,3.77656582478035E-16));
#78199=DIRECTION('ref_axis',(1.,1.48410772232726E-14,7.44759712696477E-33));
#78200=DIRECTION('center_axis',(-0.00951107056456808,-0.987363721886882,
0.158184766138841));
#78201=DIRECTION('ref_axis',(0.999632196233728,-0.00537048632003542,0.0265825154870454));
#78202=DIRECTION('center_axis',(-4.92158011612943E-15,-1.,-9.30433417784878E-14));
#78203=DIRECTION('ref_axis',(2.13564600095701E-32,9.30433417784878E-14,
-1.));
#78204=DIRECTION('center_axis',(0.,-1.,0.));
#78205=DIRECTION('ref_axis',(0.,0.,-1.));
#78206=DIRECTION('center_axis',(-0.158253626805765,-0.987363722312595,0.00828670403948867));
#78207=DIRECTION('ref_axis',(0.00319663291261748,-0.00890473459943204,-0.999955242618256));
#78208=DIRECTION('center_axis',(-0.158362916658982,0.987363722017151,0.00583670041201556));
#78209=DIRECTION('ref_axis',(-0.102087694185998,-0.0104936223845458,-0.994720054379641));
#78210=DIRECTION('center_axis',(-4.45233449258842E-14,-1.,-1.12848864220478E-15));
#78211=DIRECTION('ref_axis',(1.,-4.45233449258842E-14,1.38159831301423E-33));
#78212=DIRECTION('center_axis',(-0.00706194293192785,0.987363722357751,
0.158313008732295));
#78213=DIRECTION('ref_axis',(0.999653270055242,0.00295455998075385,0.026165057675858));
#78214=DIRECTION('center_axis',(0.158065644955521,0.987363722085681,0.0113195491917563));
#78215=DIRECTION('ref_axis',(0.0998162412145389,-0.0273822810115699,0.994629040736497));
#78216=DIRECTION('',(-0.60378640685546,0.,0.797146144001571));
#78217=DIRECTION('center_axis',(0.163668137701704,0.986495111192551,0.00633532117995019));
#78218=DIRECTION('ref_axis',(0.132080328024876,-0.0282764738460143,0.990835621067227));
#78219=DIRECTION('center_axis',(-0.154431767589658,0.98736372233359,0.0355486846267493));
#78220=DIRECTION('ref_axis',(0.242224239385166,0.0029545567318824,0.970215794784231));
#78221=DIRECTION('center_axis',(-0.160735572549779,0.986495109335916,0.0314876955875371));
#78222=DIRECTION('ref_axis',(0.137589022940416,-0.00919562022103512,0.990446718069706));
#78223=DIRECTION('',(-0.797146142410778,0.,-0.603786408955697));
#78224=DIRECTION('center_axis',(0.,-1.,0.));
#78225=DIRECTION('ref_axis',(0.,0.,-1.));
#78226=DIRECTION('center_axis',(0.147323595598226,-0.987363722485679,-0.0583835396257596));
#78227=DIRECTION('ref_axis',(0.246739261558621,-0.0204740031818272,0.968865600586179));
#78228=DIRECTION('center_axis',(0.156803524253748,0.987363722273868,-0.022924544032473));
#78229=DIRECTION('ref_axis',(0.311298434824083,-0.0273822732473687,0.94991762568545));
#78230=DIRECTION('',(-0.418307357430237,0.,0.908305540399117));
#78231=DIRECTION('center_axis',(0.161203576074765,0.986495111042672,-0.0289966023805347));
#78232=DIRECTION('ref_axis',(0.341992730746353,-0.0282764781824217,0.939277069292257));
#78233=DIRECTION('center_axis',(-0.14317932188315,0.987363722364015,0.0679158416318081));
#78234=DIRECTION('ref_axis',(0.445128886337906,0.0029545558905593,0.895461638009728));
#78235=DIRECTION('center_axis',(-0.150208740836956,0.986495109342673,0.0653049264540071));
#78236=DIRECTION('ref_axis',(0.347289035836765,-0.00919561888430754,0.937713051088074));
#78237=DIRECTION('',(-0.908305540023097,0.,-0.41830735824672));
#78238=DIRECTION('center_axis',(-1.9858077270038E-14,-1.,-3.9865505118548E-14));
#78239=DIRECTION('ref_axis',(4.90281767980684E-31,3.9865505118548E-14,-1.));
#78240=DIRECTION('center_axis',(0.131328515638144,-0.987363722452359,-0.0886887848902167));
#78241=DIRECTION('ref_axis',(0.449248100299316,-0.0204740050587526,0.893172413084008));
#78242=DIRECTION('center_axis',(0.148209449218898,0.987363722079822,-0.0560966976114605));
#78243=DIRECTION('ref_axis',(0.508224662243416,-0.0273822805924994,0.860789116681385));
#78244=DIRECTION('',(-0.213268722699965,0.,0.976993578237813));
#78245=DIRECTION('center_axis',(0.151201315284718,0.986495110967627,-0.062972678942065));
#78246=DIRECTION('ref_axis',(0.535913937257938,-0.0282764816587319,0.843798964468254));
#78247=DIRECTION('center_axis',(-0.125231968802575,0.987363722355346,0.0971073311672561));
#78248=DIRECTION('ref_axis',(0.627219803047757,0.00295455300416013,0.778836689737508));
#78249=DIRECTION('center_axis',(-0.132658313610852,0.986495109357093,0.0960685746977785));
#78250=DIRECTION('ref_axis',(0.540750198857879,-0.00919562137031807,0.841132963914016));
#78251=DIRECTION('',(-0.976993578046234,0.,-0.213268723577597));
#78252=DIRECTION('center_axis',(9.32123720376161E-15,-1.,1.15548573698919E-14));
#78253=DIRECTION('ref_axis',(-9.28936163875297E-32,-1.15548573698919E-14,
-1.));
#78254=DIRECTION('center_axis',(0.109192661680426,-0.987363722508771,-0.114847037875455));
#78255=DIRECTION('ref_axis',(0.630750596642655,-0.0204740033599842,0.775715476203324));
#78256=DIRECTION('center_axis',(0.132685264177728,0.987363722067609,-0.086645836685236));
#78257=DIRECTION('ref_axis',(0.681386866923425,-0.0273822827640736,0.731411066483757));
#78258=DIRECTION('',(0.00174211966764608,0.,0.99999848250838));
#78259=DIRECTION('center_axis',(0.134129050998668,0.986495110882551,-0.0940042226871755));
#78260=DIRECTION('ref_axis',(0.704776399762923,-0.0282764856453087,0.708865760702803));
#78261=DIRECTION('center_axis',(-0.101428913882394,0.987363722346396,0.121758183391945));
#78262=DIRECTION('ref_axis',(0.77998261856607,0.00295455906396604,0.6257942036449));
#78263=DIRECTION('center_axis',(-0.108904931346361,0.986495109325205,0.122340161868036));
#78264=DIRECTION('ref_axis',(0.708926482606278,-0.00919562280969778,0.705222434966893));
#78265=DIRECTION('',(-0.999998482504938,0.,0.00174212164352577));
#78266=DIRECTION('center_axis',(-3.47617938933741E-14,-1.,-2.78427622754031E-14));
#78267=DIRECTION('ref_axis',(1.,-3.47617938933741E-14,-2.64513424347123E-31));
#78268=DIRECTION('center_axis',(0.0819510840896689,-0.98736372258218,-0.135635169278427));
#78269=DIRECTION('ref_axis',(0.782759894667927,-0.020473998065395,0.621986947373233));
#78270=DIRECTION('center_axis',(0.110956859400106,0.987363722163423,-0.113143517302827));
#78271=DIRECTION('ref_axis',(0.822688179932599,-0.0273822785974938,0.567833047134452));
#78272=DIRECTION('',(0.216671507230176,0.,0.976244568719644));
#78273=DIRECTION('center_axis',(0.110785051961001,0.986495111067726,-0.120640242462761));
#78274=DIRECTION('ref_axis',(0.840684304897729,-0.0282764769411339,0.540786779008529));
#78275=DIRECTION('center_axis',(-0.072883154065608,0.987363722339465,0.140715761950835));
#78276=DIRECTION('ref_axis',(0.896274313951706,0.00295456149316253,0.443490275786045));
#78277=DIRECTION('center_axis',(-0.0800592741231056,0.986495109329499,0.142891258990401));
#78278=DIRECTION('ref_axis',(0.843954154358251,-0.00919562458937126,0.536336485641114));
#78279=DIRECTION('',(-0.976244569049372,0.,0.21667150574454));
#78280=DIRECTION('center_axis',(-1.19803360132752E-13,-1.,-5.9157167556196E-14));
#78281=DIRECTION('ref_axis',(1.,-1.19803360132752E-13,4.85558563358209E-31));
#78282=DIRECTION('center_axis',(0.0508775535853363,-0.987363722440403,-0.150081158543641));
#78283=DIRECTION('ref_axis',(0.898168212197172,-0.0204740061785341,0.439174996635211));
#78284=DIRECTION('center_axis',(0.0840402415547244,0.987363722072807,-0.134350728073787));
#78285=DIRECTION('ref_axis',(0.925521507090383,-0.0273822824049576,0.377703786747554));
#78286=DIRECTION('',(0.421469570788822,0.,0.906842544711642));
#78287=DIRECTION('center_axis',(0.0822608827577467,0.986495110858974,-0.14163524779961));
#78288=DIRECTION('ref_axis',(0.937282744975115,-0.0282764878537391,0.347421208630923));
#78289=DIRECTION('center_axis',(-0.0409294558523139,0.98736372233825,0.153093629697608));
#78290=DIRECTION('ref_axis',(0.970657218166449,0.00295456000537552,0.240449236631237));
#78291=DIRECTION('center_axis',(-0.0474701448626713,0.986495109347408,0.156760915346788));
#78292=DIRECTION('ref_axis',(0.939519464582124,-0.00919561566235212,0.342372043724235));
#78293=DIRECTION('',(-0.906842545090482,0.,0.421469569973702));
#78294=DIRECTION('center_axis',(-4.32398221734478E-14,-1.,-1.06733082637491E-14));
#78295=DIRECTION('ref_axis',(1.,-4.32398221734478E-14,1.34659732169751E-31));
#78296=DIRECTION('center_axis',(0.0174250529774224,-0.987363722464747,-0.157509514281813));
#78297=DIRECTION('ref_axis',(0.971579180580289,-0.0204740052995073,0.235827714592517));
#78298=DIRECTION('center_axis',(0.0531939918666645,0.987363722074045,-0.149275850563239));
#78299=DIRECTION('ref_axis',(0.985078477924935,-0.0273822820278065,0.169913516119356));
#78300=DIRECTION('',(0.606560188090453,0.,0.795037570322104));
#78301=DIRECTION('center_axis',(0.0498902720504715,0.986495110970026,-0.156007553621502));
#78302=DIRECTION('ref_axis',(0.99005488546476,-0.0282764821508358,0.13781061034817));
#78303=DIRECTION('center_axis',(-0.0126613523898977,0.986495109360025,0.163300610422653));
#78304=DIRECTION('ref_axis',(0.99115389070861,-0.00919561936268709,0.132398661313931));
#78305=DIRECTION('',(-0.795037570867346,0.,0.606560187375787));
#78306=DIRECTION('',(0.763288723126606,0.,0.646057524642935));
#78307=DIRECTION('center_axis',(0.0151868509194036,0.986495111011435,-0.163085117376443));
#78308=DIRECTION('ref_axis',(0.996533160031484,-0.0282764803465164,-0.0782438599308505));
#78309=DIRECTION('center_axis',(0.0271357814650671,0.987363722366795,0.156129846980859));
#78310=DIRECTION('ref_axis',(0.981906645777785,0.00295455723886698,-0.189342571993048));
#78311=DIRECTION('center_axis',(0.0227394687727759,0.986495109360623,0.162204549157858));
#78312=DIRECTION('ref_axis',(0.996443062115878,-0.00919562124639705,-0.0837655329537448));
#78313=DIRECTION('',(-0.646057525329045,0.,0.763288722545873));
#78314=DIRECTION('center_axis',(-7.28750092129755E-14,-1.,1.4115163077016E-14));
#78315=DIRECTION('ref_axis',(1.,-7.28750092129755E-14,2.34639488711829E-31));
#78316=DIRECTION('center_axis',(-0.0503219761482737,-0.987363722498344,
-0.150268353989605));
#78317=DIRECTION('ref_axis',(0.980802869726446,-0.0204740025985538,-0.193924072652061));
#78318=DIRECTION('center_axis',(-0.014401744385676,0.987363722089047,-0.157814669980683));
#78319=DIRECTION('ref_axis',(0.96537784684984,-0.0273822807921186,-0.25941438570401));
#78320=DIRECTION('',(0.884326726957381,0.,0.466868546797539));
#78321=DIRECTION('center_axis',(-0.0202266860130407,0.986495110995933,-0.162537002414993));
#78322=DIRECTION('ref_axis',(0.956414651573567,-0.0282764829956247,-0.290639733630504));
#78323=DIRECTION('center_axis',(0.0600646626950177,0.987363722325613,0.146646227809116));
#78324=DIRECTION('ref_axis',(0.918247158172296,0.00295455860910801,-0.395996751365372));
#78325=DIRECTION('center_axis',(0.0570770171919397,0.986495109334282,0.153523983038531));
#78326=DIRECTION('ref_axis',(0.955139663050738,-0.00919562223710471,-0.296012946674627));
#78327=DIRECTION('',(-0.466868545344239,0.,0.884326727724632));
#78328=DIRECTION('center_axis',(-2.72547556736019E-14,-1.,1.17804524909488E-14));
#78329=DIRECTION('ref_axis',(1.,-2.7254755673602E-14,2.30862714510734E-31));
#78330=DIRECTION('center_axis',(-0.0814487304934385,-0.987363722500416,
-0.135937426013325));
#78331=DIRECTION('ref_axis',(0.916184300434874,-0.0204740025869863,-0.400233860205166));
#78332=DIRECTION('center_axis',(-0.04799053510301,0.987363722266212,-0.151029098166998));
#78333=DIRECTION('ref_axis',(0.887041423826419,-0.027382273844073,-0.46087712407444));
#78334=DIRECTION('',(0.9640145970433,0.,0.26584931199355));
#78335=DIRECTION('center_axis',(-0.0546944500572356,0.986495111027636,-0.154388837198514));
#78336=DIRECTION('ref_axis',(0.871575256307171,-0.028276481282656,-0.489445618224703));
#78337=DIRECTION('center_axis',(0.0901849869939468,0.98736372233563,0.130305594417243));
#78338=DIRECTION('ref_axis',(0.811651454559872,0.00295456013056681,-0.584134562310158));
#78339=DIRECTION('center_axis',(0.0887457096272254,0.986495109349921,0.137664803967637));
#78340=DIRECTION('ref_axis',(0.869174995589528,-0.00919562629084827,-0.494419121291909));
#78341=DIRECTION('',(-0.265849312860113,0.,0.964014596804325));
#78342=DIRECTION('center_axis',(-2.40851055933823E-14,-1.,1.7363998897165E-14));
#78343=DIRECTION('ref_axis',(1.,-2.40851055933823E-14,-4.78390718535403E-31));
#78344=DIRECTION('center_axis',(-0.108767033401082,-0.987363722485907,-0.115250214593728));
#78345=DIRECTION('ref_axis',(0.808725971271374,-0.0204740033547571,-0.587829157645146));
#78346=DIRECTION('center_axis',(-0.0793353310092768,0.987363722158247,-0.137181578280253));
#78347=DIRECTION('ref_axis',(0.767227931430855,-0.0273822783229919,-0.640789756524068));
#78348=DIRECTION('',(0.998626215091659,0.,0.0523992607935185));
#78349=DIRECTION('center_axis',(-0.086604758281656,0.986495110914412,-0.139021624163072));
#78350=DIRECTION('ref_axis',(0.745981973061737,-0.0282764839575028,-0.665365565927422));
#78351=DIRECTION('center_axis',(0.116088364954327,0.987363722346356,0.10787201359286));
#78352=DIRECTION('ref_axis',(0.667103830154567,0.00295455740629755,-0.744958891740772));
#78353=DIRECTION('center_axis',(0.116264741557208,0.986495109322745,0.115368579574079));
#78354=DIRECTION('ref_axis',(0.742568672016664,-0.00919561744090605,-0.669706807460764));
#78355=DIRECTION('',(-0.0523992616912084,0.,0.998626215044556));
#78356=DIRECTION('center_axis',(-9.89463135438162E-15,-1.,1.10678119935376E-14));
#78357=DIRECTION('ref_axis',(-2.31592387427123E-31,-1.10678119935376E-14,
-1.));
#78358=DIRECTION('center_axis',(-0.130999510963508,-0.987363722459965,-0.0891740303974366));
#78359=DIRECTION('ref_axis',(0.663452515084082,-0.0204740050005565,-0.747938216263779));
#78360=DIRECTION('center_axis',(-0.106970499870904,0.987363722142363,-0.116919597820675));
#78361=DIRECTION('ref_axis',(0.611539710180093,-0.0273822782045853,-0.790739776230571));
#78362=DIRECTION('',(0.9865431813915,0.,-0.163500921251039));
#78363=DIRECTION('center_axis',(-0.114465528537602,0.986495111025307,-0.117153910305101));
#78364=DIRECTION('ref_axis',(0.58550739818458,-0.028276481381445,-0.810173763628401));
#78365=DIRECTION('center_axis',(0.136563576370328,0.98736372234371,0.0803944613049864));
#78366=DIRECTION('ref_axis',(0.49136317195317,0.00295456025843987,-0.870949771124488));
#78367=DIRECTION('center_axis',(0.138347373964644,0.986495109335736,0.0876778385554841));
#78368=DIRECTION('ref_axis',(0.581240659621152,-0.00919562299664161,-0.813679750344613));
#78369=DIRECTION('',(0.163500920364212,0.,0.986543181538475));
#78370=DIRECTION('center_axis',(2.18521438712326E-14,-1.,-3.88083178875241E-14));
#78371=DIRECTION('ref_axis',(-1.82162563614679E-31,3.88083178875241E-14,
-1.));
#78372=DIRECTION('center_axis',(-0.147106595225137,-0.987363722492263,-0.058928169388586));
#78373=DIRECTION('ref_axis',(0.487156755321014,-0.0204740038282639,-0.873074516242652));
#78374=DIRECTION('center_axis',(-0.129603845053748,0.987363722128369,-0.0911905892737636));
#78375=DIRECTION('ref_axis',(0.427256576207141,-0.027382280323163,-0.903715679189011));
#78376=DIRECTION('',(0.928330484082491,0.,-0.371755984919097));
#78377=DIRECTION('center_axis',(-0.136974018842237,0.986495111137968,-0.0898082059897402));
#78378=DIRECTION('ref_axis',(0.397655150255994,-0.0282764745849969,-0.917099134477799));
#78379=DIRECTION('center_axis',(0.150653229591986,0.987363722340574,0.0491577483136696));
#78380=DIRECTION('ref_axis',(0.292646918554997,0.0029545569875937,-0.956216006796201));
#78381=DIRECTION('center_axis',(0.153961033449543,0.98649510932601,0.0558873818944154));
#78382=DIRECTION('ref_axis',(0.392734481097539,-0.00919562464313007,-0.919605930735807));
#78383=DIRECTION('',(0.371755983092481,0.,0.928330484813971));
#78384=DIRECTION('center_axis',(4.33287056654286E-15,-1.,-1.41995219769621E-14));
#78385=DIRECTION('ref_axis',(1.09233946293455E-31,1.41995219769621E-14,
-1.));
#78386=DIRECTION('center_axis',(-0.156335138791017,-0.987363722512377,-0.0259268942547021));
#78387=DIRECTION('ref_axis',(0.288082088867567,-0.0204740016392568,-0.957386821159857));
#78388=DIRECTION('center_axis',(-0.146177060289827,0.987363722117319,-0.0611976085452475));
#78389=DIRECTION('ref_axis',(0.222995395855195,-0.0273822807870121,-0.974434843448389));
#78390=DIRECTION('',(0.826710085934478,0.,-0.562628148792973));
#78391=DIRECTION('center_axis',(-0.153077751184681,0.986495111055157,-0.0582631783935128));
#78392=DIRECTION('ref_axis',(0.191208989636266,-0.0282764781182431,-0.981141968864602));
#78393=DIRECTION('center_axis',(0.157698503409577,0.987363722348828,0.0156224777754914));
#78394=DIRECTION('ref_axis',(0.0802468205327068,0.0029545583644425,-0.996770644822199));
#78395=DIRECTION('center_axis',(0.162375644751385,0.986495109354807,0.0214836963909733));
#78396=DIRECTION('ref_axis',(0.185864477196135,-0.00919562331167665,-0.982532359074508));
#78397=DIRECTION('',(0.562628148677447,0.,0.826710086013101));
#78398=DIRECTION('center_axis',(5.89546486710796E-15,-1.,-7.39949208706086E-14));
#78399=DIRECTION('ref_axis',(1.17599418447442E-31,7.39949208706086E-14,
-1.));
#78400=DIRECTION('center_axis',(-0.158253626200997,-0.987363722455385,0.00828669857543342));
#78401=DIRECTION('ref_axis',(0.0755370232536191,-0.0204740045161776,-0.996932782717598));
#78402=DIRECTION('center_axis',(-0.155915199182761,0.98736372221274,-0.0283430894929197));
#78403=DIRECTION('ref_axis',(0.00830720070699266,-0.0273822746524882,-0.999590516887425));
#78404=DIRECTION('',(0.686433642056073,0.,-0.72719244705486));
#78405=DIRECTION('center_axis',(-0.162023739702991,0.986495110930413,-0.0239938301038143));
#78406=DIRECTION('ref_axis',(-0.0241778909692891,-0.0282764821330522,-0.99930769543042));
#78407=DIRECTION('center_axis',(0.157369971048538,0.987363722346775,-0.0186432831256345));
#78408=DIRECTION('ref_axis',(-0.135905529982305,0.00295455904762982,-0.990717395376231));
#78409=DIRECTION('center_axis',(0.163197752475911,0.986495109366373,-0.0139245388806963));
#78410=DIRECTION('ref_axis',(-0.0296963431688327,-0.00919561804706838,-0.99951666710022));
#78411=DIRECTION('',(0.727192446437817,0.,0.686433642709755));
#78412=DIRECTION('center_axis',(-1.21789062324421E-14,-1.,-8.8238773580434E-14));
#78413=DIRECTION('ref_axis',(-1.00747679306799E-32,8.8238773580434E-14,
-1.));
#78414=DIRECTION('center_axis',(-0.15277234939578,-0.98736372254509,0.0421128087640363));
#78415=DIRECTION('ref_axis',(-0.140540068186091,-0.020474001593977,-0.989863275656279));
#78416=DIRECTION('center_axis',(-0.158362915039067,0.987363722199346,0.00583671354287932));
#78417=DIRECTION('ref_axis',(-0.206769430856227,-0.0273822763792333,-0.978006448549131));
#78418=DIRECTION('',(0.514060324983116,0.,-0.85775403367064));
#78419=DIRECTION('center_axis',(-0.163393677467838,0.986495111106532,0.0113974526297502));
#78420=DIRECTION('ref_axis',(-0.238434241820558,-0.0282764764144799,-0.970746904815584));
#78421=DIRECTION('center_axis',(0.149682992843389,0.987363722367546,-0.0520373078276564));
#78422=DIRECTION('ref_axis',(-0.34570308938674,0.00295455657717342,-0.938339301417081));
#78423=DIRECTION('center_axis',(0.156388914161816,0.986495109361921,-0.0486816878538454));
#78424=DIRECTION('ref_axis',(-0.243868596486215,-0.00919562266043916,-0.969764687010066));
#78425=DIRECTION('',(0.85775403194092,0.,0.514060327869303));
#78426=DIRECTION('center_axis',(-2.05752654287162E-14,-1.,-5.57051301330842E-14));
#78427=DIRECTION('ref_axis',(4.21927796480682E-31,5.57051301330842E-14,
-1.));
#78428=DIRECTION('center_axis',(-0.140147605924149,-0.987363722434189,0.0739697787926336));
#78429=DIRECTION('ref_axis',(-0.350045664256259,-0.0204740067575522,-0.936508861667996));
#78430=DIRECTION('center_axis',(-0.153405758249488,0.987363722140234,0.0397435974376149));
#78431=DIRECTION('ref_axis',(-0.412177752017299,-0.0273822789533092,-0.910691886172974));
#78432=DIRECTION('',(0.317650120667855,0.,-0.948207994503156));
#78433=DIRECTION('center_axis',(-0.157123509264922,0.986495111084634,0.0462557957708086));
#78434=DIRECTION('ref_axis',(-0.441541669900457,-0.0282764778254351,-0.896795068308978));
#78435=DIRECTION('center_axis',(0.134997006587638,0.987363722345089,-0.0829981205162371));
#78436=DIRECTION('ref_axis',(-0.539335955073032,0.00295455986961746,-0.84208550524364));
#78437=DIRECTION('center_axis',(0.142267503246296,0.986495109321295,-0.081162533260312));
#78438=DIRECTION('ref_axis',(-0.446637828743161,-0.00919562490853365,-0.894667586547169));
#78439=DIRECTION('',(0.948207994217622,0.,0.317650121520194));
#78440=DIRECTION('center_axis',(0.,-1.,0.));
#78441=DIRECTION('ref_axis',(0.,0.,-1.));
#78442=DIRECTION('center_axis',(-0.120969720836266,-0.987363722540217,0.102367993300253));
#78443=DIRECTION('ref_axis',(-0.543183512539008,-0.020473999900492,-0.839364335097614));
#78444=DIRECTION('center_axis',(-0.141275518361541,0.987363722123742,0.0717921175730828));
#78445=DIRECTION('ref_axis',(-0.598313102465493,-0.0273822793619485,-0.800794381970216));
#78446=DIRECTION('',(0.106386947436074,0.,-0.994324804787266));
#78447=DIRECTION('center_axis',(-0.143506420757269,0.98649511106524,0.0789512700709557));
#78448=DIRECTION('ref_axis',(-0.624003101326521,-0.028276478820293,-0.780910091035075));
#78449=DIRECTION('center_axis',(0.113998708813961,0.987363722364336,-0.11007803662671));
#78450=DIRECTION('ref_axis',(-0.7077500725784,0.00295455974303667,-0.706456725739089));
#78451=DIRECTION('center_axis',(0.121493827765142,0.98649510934329,-0.109848300199615));
#78452=DIRECTION('ref_axis',(-0.628522767255286,-0.00919561739573514,-0.777736826736698));
#78453=DIRECTION('',(0.994324804659096,0.,0.106386948633988));
#78454=DIRECTION('center_axis',(-3.15476866325682E-14,-1.,-3.14379578369509E-14));
#78455=DIRECTION('ref_axis',(1.,-3.15476866325682E-14,7.63333428802623E-31));
#78456=DIRECTION('center_axis',(-0.0961354199646547,-0.987363722474464,
0.125979603784065));
#78457=DIRECTION('ref_axis',(-0.710922705002381,-0.0204740044788156,-0.702972063920537));
#78458=DIRECTION('center_axis',(-0.12253939143678,0.987363722160225,0.100483718622524));
#78459=DIRECTION('ref_axis',(-0.756471994289161,-0.0273822782236257,-0.653452624675625));
#78460=DIRECTION('',(-0.109850764109878,0.,-0.993948092017121));
#78461=DIRECTION('center_axis',(-0.123179134229024,0.986495110939119,0.107955069282568));
#78462=DIRECTION('ref_axis',(-0.777286841805984,-0.02827648289046,-0.6285106252647));
#78463=DIRECTION('center_axis',(0.0876699555529006,0.987363722327402,-0.132010828060165));
#78464=DIRECTION('ref_axis',(-0.843070582388619,0.00295455614116526,-0.537794815621091));
#78465=DIRECTION('center_axis',(0.0950392295741619,0.986495109351144,-0.133397691390157));
#78466=DIRECTION('ref_axis',(-0.78101868357015,-0.00919562018639328,-0.62443995426601));
#78467=DIRECTION('',(0.993948092429756,0.,-0.10985076037629));
#78468=DIRECTION('center_axis',(6.26139182359859E-14,-1.,3.98685596779503E-14));
#78469=DIRECTION('ref_axis',(1.,6.26139182359859E-14,3.82708143198835E-31));
#78470=DIRECTION('center_axis',(-0.0668059353666372,-0.98736372243687,0.143700544937714));
#78471=DIRECTION('ref_axis',(-0.845419941715254,-0.0204740056074118,-0.533709600105305));
#78472=DIRECTION('center_axis',(-0.0980734572566049,0.987363722206714,0.124476813310113));
#78473=DIRECTION('ref_axis',(-0.879259097639604,-0.0273822756801386,-0.475556148311181));
#78474=DIRECTION('',(-0.320951972736834,0.,-0.947095471004024));
#78475=DIRECTION('center_axis',(-0.0970921254666728,0.986495110935384,0.131911012705338));
#78476=DIRECTION('ref_axis',(-0.894225513091188,-0.0282764824828937,-0.446722701768331));
#78477=DIRECTION('center_axis',(0.0572418589335363,0.987363722345491,-0.147770935511318));
#78478=DIRECTION('ref_axis',(-0.938970048578615,0.00295456041420517,-0.343986218394039));
#78479=DIRECTION('center_axis',(0.0641407031162536,0.986495109342319,-0.150709553271978));
#78480=DIRECTION('ref_axis',(-0.896995032092022,-0.0091956222124549,-0.441944965956575));
#78481=DIRECTION('',(0.947095471292532,0.,-0.320951971885478));
#78482=DIRECTION('center_axis',(-1.39441202957605E-14,-1.,-5.09526267024949E-15));
#78483=DIRECTION('ref_axis',(1.,-1.39441202957605E-14,-4.33523906590216E-32));
#78484=DIRECTION('center_axis',(-0.0343526833148809,-0.987363722490136,
0.1547022063821));
#78485=DIRECTION('ref_axis',(-0.940386280729254,-0.0204740025468243,-0.339491470048825));
#78486=DIRECTION('center_axis',(-0.0690217183976504,0.987363722198575,0.142649509202135));
#78487=DIRECTION('ref_axis',(-0.960933023633175,-0.027382275329481,-0.275423192721647));
#78488=DIRECTION('',(-0.517045822704402,0.,-0.855957719296887));
#78489=DIRECTION('center_axis',(-0.0664652025269315,0.986495110851481,0.149698941610083));
#78490=DIRECTION('ref_axis',(-0.969351193563916,-0.0282764885549299,-0.244046519604798));
#78491=DIRECTION('center_axis',(0.0241371926176063,0.98736372236658,-0.156621440700023));
#78492=DIRECTION('ref_axis',(-0.990964319395181,0.002954559969109,-0.134093207363515));
#78493=DIRECTION('center_axis',(0.0302430298729286,0.986495109332971,-0.160974402953495));
#78494=DIRECTION('ref_axis',(-0.971028890904806,-0.00919562225302405,-0.238785120054752));
#78495=DIRECTION('',(0.855957719761673,0.,-0.51704582193496));
#78496=DIRECTION('center_axis',(-8.82806721608986E-14,-1.,-1.1871387483534E-14));
#78497=DIRECTION('ref_axis',(1.,-8.82806721608986E-14,1.9887858054574E-31));
#78498=DIRECTION('center_axis',(-0.000293134981233076,-0.987363722491244,
0.158470166214708));
#78499=DIRECTION('ref_axis',(-0.991381202856231,-0.0204740027916695,-0.129399095178518));
#78500=DIRECTION('center_axis',(-0.0367426028752615,0.987363722166916,0.154152071937562));
#78501=DIRECTION('ref_axis',(-0.997674788534383,-0.0273822772005084,-0.0624117554487041));
#78502=DIRECTION('',(-0.688963187756883,0.,-0.724796334093843));
#78503=DIRECTION('center_axis',(-0.0327304188065948,0.986495111201851,0.160487118671852));
#78504=DIRECTION('ref_axis',(-0.99915108956692,-0.0282764714310698,-0.0299589949872197));
#78505=DIRECTION('center_axis',(-0.0100961008866114,0.987363722319459,-0.158148501713896));
#78506=DIRECTION('ref_axis',(-0.996622199995403,0.00295456092772905,0.0820698546729972));
#78507=DIRECTION('center_axis',(-0.00506877082020845,0.986495109324231,
-0.16371226845214));
#78508=DIRECTION('ref_axis',(-0.999658517458994,-0.00919561933260429,-0.0244599480125288));
#78509=DIRECTION('',(0.724796334642181,0.,-0.688963187180026));
#78510=DIRECTION('center_axis',(8.87687165924134E-14,-1.,-7.38389392493213E-15));
#78511=DIRECTION('ref_axis',(1.,8.87687165924134E-14,6.42305605932119E-32));
#78512=DIRECTION('center_axis',(0.0337801256786956,-0.987363722407571,0.154828236386635));
#78513=DIRECTION('ref_axis',(-0.996020241549457,-0.020474008779607,0.0867438377537795));
#78514=DIRECTION('center_axis',(-0.00274544497597346,0.98736372213281,0.158446655843306));
#78515=DIRECTION('ref_axis',(-0.987766389444261,-0.0273822791546761,0.153517981593504));
#78516=DIRECTION('',(-0.828665397705427,0.,-0.559744279690027));
#78517=DIRECTION('center_axis',(0.00253477441076304,0.986495110962286,0.16377109319472));
#78518=DIRECTION('ref_axis',(-0.982231790619155,-0.0282764837612161,0.185529377628423));
#78519=DIRECTION('center_axis',(-0.0438573179899566,0.987363722349411,-0.152280712656075));
#78520=DIRECTION('ref_axis',(-0.95567913422659,0.00295455517364751,0.294395419474627));
#78521=DIRECTION('center_axis',(-0.0401435654911374,0.986495109322325,-0.158795130381233));
#78522=DIRECTION('ref_axis',(-0.981545222756637,-0.00919562080500803,0.191008942831572));
#78523=DIRECTION('',(0.559744278460836,0.,-0.828665398535717));
#78524=DIRECTION('center_axis',(2.83686781064125E-14,-1.,-8.76463754737558E-15));
#78525=DIRECTION('ref_axis',(1.,2.83686781064125E-14,-2.01260476590519E-31));
#78526=DIRECTION('center_axis',(0.0662738583278151,-0.987363722418306,0.143946710120834));
#78527=DIRECTION('ref_axis',(-0.954086480895184,-0.0204740078213297,0.298830724619768));
#78528=DIRECTION('center_axis',(0.0313800915092737,0.987363722164569,0.155332449958781));
#78529=DIRECTION('ref_axis',(-0.931671131181227,-0.0273822773082007,0.362269394529693));
#78530=DIRECTION('',(-0.929620135502299,0.,-0.36851920393473));
#78531=DIRECTION('center_axis',(0.0376814580230275,0.986495110934236,0.159397314356638));
#78532=DIRECTION('ref_axis',(-0.919384425301451,-0.0282764825435261,0.392342604171514));
#78533=DIRECTION('center_axis',(-0.0755678077734676,0.987363722339704,-0.139292448595736));
#78534=DIRECTION('ref_axis',(-0.87004957346559,0.00295455813711103,0.492955383679455));
#78535=DIRECTION('center_axis',(-0.0733412931473506,0.986495109333737,-0.146452907038722));
#78536=DIRECTION('ref_axis',(-0.917535964181013,-0.00919562396521216,0.397546468899309));
#78537=DIRECTION('',(0.3685192037855,0.,-0.929620135561457));
#78538=DIRECTION('center_axis',(2.58212961952919E-14,-1.,-1.46581524198925E-14));
#78539=DIRECTION('ref_axis',(1.,2.58212961952919E-14,-3.82337337017993E-31));
#78540=DIRECTION('center_axis',(0.0956686992681182,-0.987363722428569,0.126334395998662));
#78541=DIRECTION('ref_axis',(-0.86754069645364,-0.0204740068519684,0.496944619691328));
#78542=DIRECTION('center_axis',(0.0640383226550879,0.987363722055881,0.144955074417834));
#78543=DIRECTION('ref_axis',(-0.832011966724281,-0.0273822830093003,0.55408149022034));
#78544=DIRECTION('',(-0.987106868581237,0.,-0.160062581510308));
#78545=DIRECTION('center_axis',(0.071066195202264,0.986495110975005,0.147570294849225));
#78546=DIRECTION('ref_axis',(-0.813547665355053,-0.0282764848871257,0.580810327557776));
#78547=DIRECTION('center_axis',(-0.103744832799726,0.987363722346279,-0.119791024128924));
#78548=DIRECTION('ref_axis',(-0.743737463193152,0.00295455866069842,0.668465299343305));
#78549=DIRECTION('center_axis',(-0.103109658554765,0.98649510935733,-0.127262710668878));
#78550=DIRECTION('ref_axis',(-0.810623745170262,-0.00919562209827842,0.585495161637023));
#78551=DIRECTION('',(0.160062579596475,0.,-0.987106868891572));
#78552=DIRECTION('center_axis',(0.0937021734286871,0.98736372160279,0.127799780740929));
#78553=DIRECTION('ref_axis',(-0.693448832647947,-0.0273823195503969,0.719985364486834));
#78554=DIRECTION('',(-0.998437581939004,0.,0.0558783944990723));
#78555=DIRECTION('center_axis',(0.101127960417461,0.986495110941819,0.128843050684517));
#78556=DIRECTION('ref_axis',(-0.669670322268832,-0.028276482174131,0.742120003791984));
#78557=DIRECTION('center_axis',(-2.20665391377616E-14,-1.,1.98662683520469E-14));
#78558=DIRECTION('ref_axis',(1.,-2.20665391377616E-14,-4.42483838814686E-31));
#78559=DIRECTION('center_axis',(0.120590140483329,-0.987363723519774,0.102814860284774));
#78560=DIRECTION('ref_axis',(-0.740429679278794,-0.0204739556178617,0.671821931157699));
#78561=DIRECTION('center_axis',(-0.127070866310374,0.987363722339884,-0.0946883030910327));
#78562=DIRECTION('ref_axis',(-0.582649014492189,0.00295455734858739,0.812718522307788));
#78563=DIRECTION('center_axis',(-0.128056733023664,0.986495109359135,-0.102121850442573));
#78564=DIRECTION('ref_axis',(-0.665807659368209,-0.00919562209053125,0.746066753890692));
#78565=DIRECTION('',(-0.0558783934411736,0.,-0.99843758199821));
#78566=DIRECTION('center_axis',(3.45599505596096E-14,-1.,-4.82909193868955E-14));
#78567=DIRECTION('ref_axis',(-2.68967614992597E-31,4.82909193868955E-14,
-1.));
#78568=DIRECTION('center_axis',(0.118984666368161,0.987363722173452,0.10466866438932));
#78569=DIRECTION('ref_axis',(-0.5224608308728,-0.0273822777464371,0.852223498308467));
#78570=DIRECTION('center_axis',(0.139872995331646,-0.987363722448005,0.0744877491307953));
#78571=DIRECTION('ref_axis',(-0.57869698151077,-0.0204740057536221,0.815285605587836));
#78572=DIRECTION('center_axis',(0.12646109336356,0.986495110980928,0.104091247835831));
#78573=DIRECTION('ref_axis',(-0.494479938320355,-0.0282764800739962,0.868728974579139));
#78574=DIRECTION('',(-0.963082463535534,0.,0.269206553468387));
#78575=DIRECTION('center_axis',(-0.144455208030673,0.987363722350675,-0.0651580590459365));
#78576=DIRECTION('ref_axis',(-0.394316546242898,0.00295455278274242,0.918969929854577));
#78577=DIRECTION('center_axis',(-0.147016018399682,0.986495109320743,-0.0722058835563958));
#78578=DIRECTION('ref_axis',(-0.489859148114179,-0.00919562510734571,0.871753093190805));
#78579=DIRECTION('',(-0.269206552602653,0.,-0.963082463777529));
#78580=DIRECTION('center_axis',(-1.75281284135584E-14,-1.,4.09434541677049E-14));
#78581=DIRECTION('ref_axis',(-6.97643112798884E-32,-4.09434541677049E-14,
-1.));
#78582=DIRECTION('center_axis',(0.152615505806413,-0.987363722502889,0.0426777093186988));
#78583=DIRECTION('ref_axis',(-0.389905061888299,-0.0204740037428501,0.920627426207051));
#78584=DIRECTION('center_axis',(0.138703539562874,0.987363722143939,0.0766433839727627));
#78585=DIRECTION('ref_axis',(-0.327043125582336,-0.0273822788356535,0.94461262156246));
#78586=DIRECTION('',(-0.882694679781319,0.,0.469946914327305));
#78587=DIRECTION('center_axis',(0.145881043013491,0.986495110952259,0.0744722589733021));
#78588=DIRECTION('ref_axis',(-0.296168221911397,-0.0282764840435662,0.954717143859885));
#78589=DIRECTION('center_axis',(-0.155084980925954,0.9873637223546,-0.0325811060166102));
#78590=DIRECTION('ref_axis',(-0.187546275077728,0.00295455868251791,0.982251324910005));
#78591=DIRECTION('center_axis',(-0.159100996390971,0.986495109339711,-0.0389136505127861));
#78592=DIRECTION('ref_axis',(-0.291005366268943,-0.00919562638014897,0.956677227312407));
#78593=DIRECTION('',(-0.469946915773758,0.,-0.882694679011227));
#78594=DIRECTION('center_axis',(-1.94056290405287E-14,-1.,1.02093246551329E-13));
#78595=DIRECTION('ref_axis',(4.6849201298372E-31,-1.02093246551329E-13,
-1.));
#78596=DIRECTION('center_axis',(0.158221886231727,-0.987363722470914,0.00887210604393224));
#78597=DIRECTION('ref_axis',(-0.182881616600238,-0.0204740036971804,0.982921731106954));
#78598=DIRECTION('center_axis',(0.151936789673059,0.987363722123935,0.0450343444208377));
#78599=DIRECTION('ref_axis',(-0.116333249189989,-0.0273822798023598,0.992832707904874));
#78600=DIRECTION('',(-0.761033074141649,0.,0.648713079922481));
#78601=DIRECTION('center_axis',(0.158479759458568,0.986495110935801,0.0413710278058995));
#78602=DIRECTION('ref_axis',(-0.0840080098883409,-0.0282764847776318,0.996063800508391));
#78603=DIRECTION('center_axis',(2.56722337042868E-15,-1.,8.90382855340933E-14));
#78604=DIRECTION('ref_axis',(0.0288208255552056,8.90752879685742E-14,0.999584593725972));
#78605=DIRECTION('center_axis',(0.156429986789619,-0.987363722430428,-0.0253483502683913));
#78606=DIRECTION('ref_axis',(0.0326931712220302,-0.0204740066028789,0.999255708819856));
#78607=DIRECTION('center_axis',(-0.158463154907314,0.987363722361481,0.00151930948189432));
#78608=DIRECTION('ref_axis',(0.0279934535704983,0.00295455814615585,0.999603740060709));
#78609=DIRECTION('center_axis',(-0.163746588080473,0.986495109318213,-0.0038018657591047));
#78610=DIRECTION('ref_axis',(-0.0785444998839504,-0.0091956206558518,0.996868196954208));
#78611=DIRECTION('',(-0.648713080657652,0.,-0.761033073514981));
#78612=DIRECTION('center_axis',(-0.154562212825867,-0.987363722400022,-0.0349771647613762));
#78613=DIRECTION('ref_axis',(-0.156465939823782,-0.0104932879265436,0.987627612303115));
#78614=DIRECTION('',(0.562296676496711,-6.23377071775851E-15,0.826935576451245));
#78615=DIRECTION('',(0.826935573288472,0.,-0.562296681148009));
#78616=DIRECTION('center_axis',(0.152615509258216,-0.987363722350212,0.0426777005072813));
#78617=DIRECTION('ref_axis',(-0.32231653707131,-0.00890473778974789,0.94659006733393));
#78618=DIRECTION('center_axis',(-0.14342957841421,-0.987363722441753,-0.0673857228341938));
#78619=DIRECTION('ref_axis',(-0.36511859464289,-0.0104932857748454,0.930901876031866));
#78620=DIRECTION('',(0.371383789246354,0.,0.928479445698729));
#78621=DIRECTION('center_axis',(8.67712559411096E-15,-1.,-2.83955679719989E-14));
#78622=DIRECTION('ref_axis',(-3.40757823733139E-32,2.83955679719989E-14,
-1.));
#78623=DIRECTION('center_axis',(0.151936786270519,0.987363722024958,0.0450343580703467));
#78624=DIRECTION('ref_axis',(-0.220871911237121,-0.0104936262509378,0.975246370223733));
#78625=DIRECTION('center_axis',(-0.144455200951618,0.987363721612747,-0.0651580859222701));
#78626=DIRECTION('ref_axis',(-0.295080326269699,0.0198684700496971,0.955265850403149));
#78627=DIRECTION('',(0.928479445093011,0.,-0.371383790760683));
#78628=DIRECTION('center_axis',(0.139872999273741,-0.987363722338544,0.0744877431792839));
#78629=DIRECTION('ref_axis',(-0.518269837796488,-0.00890473716144612,0.855170790477836));
#78630=DIRECTION('center_axis',(-0.125590335269879,-0.987363722391106,-0.096643403255366));
#78631=DIRECTION('ref_axis',(-0.556698710963746,-0.0104932875265685,0.830648202386659));
#78632=DIRECTION('',(0.163105405539061,0.,0.986608649203897));
#78633=DIRECTION('center_axis',(-5.10246344398526E-14,-1.,9.0532294620924E-14));
#78634=DIRECTION('ref_axis',(1.03431144013726E-30,-9.0532294620924E-14,
-1.));
#78635=DIRECTION('center_axis',(0.138703533836429,0.987363721999689,0.0766433961943712));
#78636=DIRECTION('ref_axis',(-0.425357189232499,-0.0104936246872304,0.904964720532879));
#78637=DIRECTION('center_axis',(-0.127070856969211,0.987363721618719,-0.0946883231467527));
#78638=DIRECTION('ref_axis',(-0.493535432378174,0.0198684687691836,0.869498718191152));
#78639=DIRECTION('',(0.98660864901436,0.,-0.163105406685554));
#78640=DIRECTION('center_axis',(0.120590183957813,-0.987363722329175,0.102814820727838));
#78641=DIRECTION('ref_axis',(-0.689989418966707,-0.00890473821475343,0.723764676777827));
#78642=DIRECTION('center_axis',(-0.101878628092225,-0.987363722385251,-0.121382143891048));
#78643=DIRECTION('ref_axis',(-0.722248213566424,-0.0104932876907897,0.691554342704569));
#78644=DIRECTION('',(-0.0527996037021425,0.,0.998605128090627));
#78645=DIRECTION('center_axis',(2.9697203196646E-14,-1.,-3.31915336355735E-14));
#78646=DIRECTION('ref_axis',(-1.45851444347016E-32,3.31915336355735E-14,
-1.));
#78647=DIRECTION('center_axis',(0.118984659539348,0.987363722014647,0.104668673650181));
#78648=DIRECTION('ref_axis',(-0.609953239450716,-0.0104936216088402,0.792367925643831));
#78649=DIRECTION('center_axis',(-0.103744818751068,0.987363721575649,-0.119791042647572));
#78650=DIRECTION('ref_axis',(-0.668913370904801,0.0198684711732498,0.743074791712123));
#78651=DIRECTION('',(0.99860512817674,0.,0.052799602073472));
#78652=DIRECTION('center_axis',(0.0956687012151709,-0.987363722323065,0.126334395348786));
#78653=DIRECTION('ref_axis',(-0.829445861762146,-0.00890473335574096,0.558516130590258));
#78654=DIRECTION('center_axis',(-0.0734031899540221,-0.987363722401994,
-0.140445189981899));
#78655=DIRECTION('ref_axis',(-0.854026193536076,-0.0104932869748259,0.520124169485272));
#78656=DIRECTION('',(-0.266235760272642,0.,0.963907941637607));
#78657=DIRECTION('center_axis',(2.4092065114801E-14,-1.,-1.73543421154282E-14));
#78658=DIRECTION('ref_axis',(1.,2.4092065114801E-14,-3.57346751578377E-31));
#78659=DIRECTION('center_axis',(0.0937021908558792,0.987363722013814,0.127799764787879));
#78660=DIRECTION('ref_axis',(-0.766028551888797,-0.0104936252703983,0.642720889282305));
#78661=DIRECTION('center_axis',(-0.0755677888343809,0.987363721559842,-0.139292464398404));
#78662=DIRECTION('ref_axis',(-0.81301366345872,0.0198684717500299,0.581905513687359));
#78663=DIRECTION('',(0.963907941868057,0.,0.266235759438296));
#78664=DIRECTION('center_axis',(0.0662738630982961,-0.987363722324091,0.14394670857072));
#78665=DIRECTION('ref_axis',(-0.930118336104504,-0.00890473695803777,0.367151993732701));
#78666=DIRECTION('center_axis',(-0.04149549491575,-0.987363722304536,-0.152941177511578));
#78667=DIRECTION('ref_axis',(-0.945870857771692,-0.0104932921380493,0.324373567416256));
#78668=DIRECTION('',(-0.467223032247448,6.23377071131938E-15,0.88413949020361));
#78669=DIRECTION('center_axis',(-5.45189531984744E-14,-1.,2.35390508043942E-14));
#78670=DIRECTION('ref_axis',(1.,-5.45189531984744E-14,-2.16278283367938E-31));
#78671=DIRECTION('center_axis',(0.0640383165993706,0.987363721994225,0.144955077513102));
#78672=DIRECTION('ref_axis',(-0.886285223091077,-0.0104936222903732,0.463020936051089));
#78673=DIRECTION('center_axis',(-0.0438572993335235,0.987363721632358,-0.152280722678445));
#78674=DIRECTION('ref_axis',(-0.919098339570757,0.0198684658176202,0.393526982892318));
#78675=DIRECTION('',(0.884139492153187,0.,0.467223028558209));
#78676=DIRECTION('center_axis',(0.0337801291775882,-0.98736372232979,0.154828236119277));
#78677=DIRECTION('ref_axis',(-0.987299512398125,-0.00890473682484817,0.158620233515478));
#78678=DIRECTION('center_axis',(-0.00764752125946903,-0.987363722329066,
-0.158285802417894));
#78679=DIRECTION('ref_axis',(-0.993487651528559,-0.0104932916296771,0.113455617274087));
#78680=DIRECTION('',(-0.646363471935384,-6.23377071920573E-15,0.763029660070718));
#78681=DIRECTION('center_axis',(1.16609060841453E-13,-1.,-2.25375149943799E-14));
#78682=DIRECTION('ref_axis',(1.,1.16609060841453E-13,-4.9990146629533E-31));
#78683=DIRECTION('center_axis',(0.0313800754377996,0.987363722013489,0.155332454165855));
#78684=DIRECTION('ref_axis',(-0.965100182175857,-0.0104936260553598,0.261670636824878));
#78685=DIRECTION('center_axis',(-0.0100960862249963,0.987363721665325,-0.158148506733817));
#78686=DIRECTION('ref_axis',(-0.98220699998696,0.0198684655322117,0.186747565590591));
#78687=DIRECTION('',(0.76302966112491,0.,0.646363470690915));
#78688=DIRECTION('center_axis',(-0.000293120077939613,-0.987363722326222,
0.158470167270458));
#78689=DIRECTION('ref_axis',(-0.998315660024052,-0.00890474181677815,-0.0573284268397199));
#78690=DIRECTION('center_axis',(0.0265580433165256,-0.987363722271751,-0.156229159496141));
#78691=DIRECTION('ref_axis',(-0.994650066459442,-0.0104932930201555,-0.102767388279653));
#78692=DIRECTION('',(-0.795280674871628,-6.23377070532254E-15,0.606241410805735));
#78693=DIRECTION('center_axis',(1.48409631970856E-14,-1.,3.82112591215294E-16));
#78694=DIRECTION('ref_axis',(-0.999668706672101,-1.48458815383128E-14,-0.0257386266247645));
#78695=DIRECTION('center_axis',(-0.00274545648219705,0.987363722011251,
0.158446656401429));
#78696=DIRECTION('ref_axis',(-0.998788128182702,-0.0104936233898283,0.0480849131167593));
#78697=DIRECTION('center_axis',(0.0241372137388688,0.987363721561804,-0.156621442518411));
#78698=DIRECTION('ref_axis',(-0.999388752406702,0.0198684703996675,-0.0287639609051392));
#78699=DIRECTION('',(0.606241413488844,0.,0.795280672826298));
#78700=DIRECTION('center_axis',(-0.0343526754374226,-0.987363722316263,
0.15470220924106));
#78701=DIRECTION('ref_axis',(-0.96265167765723,-0.00890473481808807,-0.270596476698311));
#78702=DIRECTION('center_axis',(0.0595217799933164,-0.98736372233658,-0.14686741476611));
#78703=DIRECTION('ref_axis',(-0.949303750074943,-0.0104932907929634,-0.314185106174663));
#78704=DIRECTION('',(-0.907011438172325,6.23377072148099E-15,0.421105985500765));
#78705=DIRECTION('center_axis',(5.76473871287922E-14,-1.,1.42541895811654E-14));
#78706=DIRECTION('ref_axis',(1.,5.76473871287922E-14,4.64171933072534E-32));
#78707=DIRECTION('center_axis',(-0.0367426193503058,0.98736372202171,0.154152068940748));
#78708=DIRECTION('ref_axis',(-0.985773851402552,-0.0104936258606393,-0.167749210750086));
#78709=DIRECTION('center_axis',(0.0572418783879038,0.987363721619137,-0.147770932828589));
#78710=DIRECTION('ref_axis',(-0.969840197166203,0.0198684690771466,-0.24293051660331));
#78711=DIRECTION('',(0.421105986980064,0.,0.907011437485518));
#78712=DIRECTION('center_axis',(-0.0668059282074712,-0.987363722329631,
0.143700549002825));
#78713=DIRECTION('ref_axis',(-0.881975171793276,-0.00890473817601859,-0.471211737946157));
#78714=DIRECTION('center_axis',(0.0897023443099469,-0.987363722380802,-0.130638314255909));
#78715=DIRECTION('ref_axis',(-0.859569045297417,-0.0104932880608984,-0.510911878186598));
#78716=DIRECTION('',(-0.9763313539579,0.,0.216280112998708));
#78717=DIRECTION('center_axis',(3.99265454288478E-14,-1.,1.97350640766554E-14));
#78718=DIRECTION('ref_axis',(1.,3.99265454288478E-14,-5.50716463294474E-31));
#78719=DIRECTION('center_axis',(-0.0690217288582187,0.987363722016548,0.142649505400653));
#78720=DIRECTION('ref_axis',(-0.926665886657474,-0.0104936191794018,-0.375739562013153));
#78721=DIRECTION('center_axis',(0.0876699778602928,0.987363721604882,-0.132010818649586));
#78722=DIRECTION('ref_axis',(-0.894942993070415,0.0198684697000682,-0.445737908491016));
#78723=DIRECTION('',(0.216280117331436,0.,0.9763313529981));
#78724=DIRECTION('center_axis',(-0.0961354113898672,-0.987363722329987,
0.125979611459841));
#78725=DIRECTION('ref_axis',(-0.760058487094592,-0.00890474036864194,-0.649793660937414));
#78726=DIRECTION('center_axis',(0.115688529063399,-0.987363722404488,-0.108300710628786));
#78727=DIRECTION('ref_axis',(-0.729641847515942,-0.0104932879451102,-0.683748978252709));
#78728=DIRECTION('',(-0.99999910056149,0.,0.00134122190962044));
#78729=DIRECTION('center_axis',(3.47506295206373E-14,-1.,2.78566962532615E-14));
#78730=DIRECTION('ref_axis',(1.,3.47506295206373E-14,4.63567395073469E-32));
#78731=DIRECTION('center_axis',(-0.0980734723655976,0.987363721986029,0.124476803156453));
#78732=DIRECTION('ref_axis',(-0.824228051317188,-0.0104936262373712,-0.566160757409291));
#78733=DIRECTION('center_axis',(0.113998724386721,0.987363721657003,-0.11007802684384));
#78734=DIRECTION('ref_axis',(-0.778199249123463,0.0198684673062269,-0.627703092768053));
#78735=DIRECTION('',(0.00134122641155386,0.,0.999999100555452));
#78736=DIRECTION('center_axis',(-0.120969711832683,-0.987363722336904,0.10236800590092));
#78737=DIRECTION('ref_axis',(-0.602602313497403,-0.00890473952231705,-0.797991953206057));
#78738=DIRECTION('center_axis',(0.136265247370615,-0.987363722378472,-0.0808990858412706));
#78739=DIRECTION('ref_axis',(-0.565597408134151,-0.010493288525919,-0.824614735987565));
#78740=DIRECTION('',(-0.976908000747675,0.,-0.213660380218656));
#78741=DIRECTION('center_axis',(-1.86332085823107E-14,-1.,-2.31171868766338E-14));
#78742=DIRECTION('ref_axis',(-2.32159898207252E-31,2.31171868766338E-14,
-1.));
#78743=DIRECTION('center_axis',(-0.122539404214814,0.987363722008592,0.10048370452973));
#78744=DIRECTION('ref_axis',(-0.683250231372573,-0.0104936297776743,-0.730108899455016));
#78745=DIRECTION('center_axis',(0.134997021813067,0.987363721562226,-0.0829981050650767));
#78746=DIRECTION('ref_axis',(-0.625067771768455,0.0198684707171492,-0.78031757930203));
#78747=DIRECTION('',(-0.213660376481803,0.,0.976908001564965));
#78748=DIRECTION('center_axis',(-0.140147603738312,-0.987363722333548,0.0739697842774299));
#78749=DIRECTION('ref_axis',(-0.416969124659213,-0.00890473688030596,-0.908877029494102));
#78750=DIRECTION('center_axis',(0.150470353718179,-0.987363722377245,-0.0497147099486297));
#78751=DIRECTION('ref_axis',(-0.37510626190524,-0.0104932884810437,-0.926922425651862));
#78752=DIRECTION('',(-0.908137769272627,0.,-0.418671460718947));
#78753=DIRECTION('center_axis',(3.96841880413548E-14,-1.,7.9746926833596E-14));
#78754=DIRECTION('ref_axis',(2.96482732682133E-31,-7.9746926833596E-14,
-1.));
#78755=DIRECTION('center_axis',(-0.141275524388681,0.987363722030692,0.0717921069923499));
#78756=DIRECTION('ref_axis',(-0.510324391310211,-0.0104936240876129,-0.859917960905208));
#78757=DIRECTION('center_axis',(0.149683006307519,0.987363721553883,-0.052037284537236));
#78758=DIRECTION('ref_axis',(-0.442708819693711,0.0198684723546586,-0.896445282642334));
#78759=DIRECTION('',(-0.41867146160869,0.,0.908137768862436));
#78760=DIRECTION('center_axis',(-0.152772346323565,-0.987363722329941,0.0421128249534124));
#78761=DIRECTION('ref_axis',(-0.211838925404988,-0.00890474194811866,-0.977264025355532));
#78762=DIRECTION('center_axis',(0.157639633326776,-0.987363722396684,-0.0162057304544932));
#78763=DIRECTION('ref_axis',(-0.167075565562151,-0.0104932877122433,-0.985888252442981));
#78764=DIRECTION('',(-0.796904023488092,-6.23377073564162E-15,-0.604105932224218));
#78765=DIRECTION('center_axis',(-1.08065809005894E-14,-1.,-4.32067076774285E-14));
#78766=DIRECTION('ref_axis',(1.3068534013106E-31,4.32067076774285E-14,-1.));
#78767=DIRECTION('center_axis',(-0.153405762942741,0.987363721993324,0.0397435829719167));
#78768=DIRECTION('ref_axis',(-0.313536345948425,-0.0104936267221054,-0.949518216553809));
#78769=DIRECTION('center_axis',(0.157369977170714,0.98736372166309,-0.0186432676562037));
#78770=DIRECTION('ref_axis',(-0.239649298886824,0.0198684648167131,-0.970656199510867));
#78771=DIRECTION('',(-0.604105932750183,0.,0.796904023089375));
#78772=DIRECTION('',(-0.64840793185587,0.,-0.761293080164527));
#78773=DIRECTION('',(-0.761293077687916,0.,0.648407934763649));
#78774=DIRECTION('center_axis',(-0.156335141249768,-0.987363722339936,-0.0259268859958497));
#78775=DIRECTION('ref_axis',(0.218082714256779,-0.00890473458450209,-0.975889663560577));
#78776=DIRECTION('center_axis',(0.149874466705301,-0.987363722477481,0.0514832377110639));
#78777=DIRECTION('ref_axis',(0.26233005865523,-0.0104932834881059,-0.964921152907108));
#78778=DIRECTION('',(-0.469593007892373,0.,-0.882883008636248));
#78779=DIRECTION('center_axis',(2.77807948950603E-15,-1.,-1.45836371277071E-14));
#78780=DIRECTION('ref_axis',(-3.32256348487704E-32,1.45836371277071E-14,
-1.));
#78781=DIRECTION('center_axis',(-0.155915196790434,0.987363722007201,-0.0283431098132548));
#78782=DIRECTION('ref_axis',(0.114134469893609,-0.0104936276209515,-0.993409888495911));
#78783=DIRECTION('center_axis',(0.150653227138706,0.987363721651154,0.0491577696796259));
#78784=DIRECTION('ref_axis',(0.190068147031143,0.0198684676975153,-0.981569836270197));
#78785=DIRECTION('',(-0.882883007870352,0.,0.469593009332337));
#78786=DIRECTION('center_axis',(-0.147106599459758,-0.987363722334265,-0.0589281614647145));
#78787=DIRECTION('ref_axis',(0.422771490401481,-0.00890473699181164,-0.906192569249394));
#78788=DIRECTION('center_axis',(0.135303108094111,-0.98736372235854,0.0824981739819796));
#78789=DIRECTION('ref_axis',(0.463626451505004,-0.0104932900032102,-0.885968624912749));
#78790=DIRECTION('',(-0.268820435286404,0.,-0.963190310152894));
#78791=DIRECTION('center_axis',(2.92409021633132E-14,-1.,-6.82273741811819E-14));
#78792=DIRECTION('ref_axis',(1.48618071870625E-31,6.82273741811819E-14,
-1.));
#78793=DIRECTION('center_axis',(-0.146177057117787,0.98736372202545,-0.0611976176042204));
#78794=DIRECTION('ref_axis',(0.325019829443857,-0.010493622859718,-0.94564898051421));
#78795=DIRECTION('center_axis',(0.136563571725779,0.987363721650438,0.0803944777089522));
#78796=DIRECTION('ref_axis',(0.396632959753101,0.019868466210324,-0.91776224551239));
#78797=DIRECTION('',(-0.963190309714461,0.,0.26882043685732));
#78798=DIRECTION('center_axis',(-0.130999516830709,-0.987363722332075,-0.0891740231943641));
#78799=DIRECTION('ref_axis',(0.607691945400389,-0.00890473868258867,-0.794122915627352));
#78800=DIRECTION('center_axis',(0.114405126201655,-0.98736372230861,0.10965558338575));
#78801=DIRECTION('ref_axis',(0.643244187693094,-0.0104932928074988,-0.765589188667857));
#78802=DIRECTION('',(-0.0554781176097352,0.,-0.998459903284293));
#78803=DIRECTION('center_axis',(-2.59344808506195E-14,-1.,3.62077958619679E-14));
#78804=DIRECTION('ref_axis',(-2.56733982118683E-31,-3.62077958619679E-14,
-1.));
#78805=DIRECTION('center_axis',(-0.129603838858743,0.987363722017638,-0.0911905992773047));
#78806=DIRECTION('ref_axis',(0.520707624190231,-0.0104936248398,-0.853670576948677));
#78807=DIRECTION('center_axis',(0.116088352443771,0.987363721593397,0.107872033948232));
#78808=DIRECTION('ref_axis',(0.584651655468008,0.0198684704736681,-0.811041112175921));
#78809=DIRECTION('',(-0.998459903193811,0.,0.0554781192381759));
#78810=DIRECTION('center_axis',(-0.108767041434347,-0.987363722333227,-0.115250208320386));
#78811=DIRECTION('ref_axis',(0.764197398165907,-0.00890473803429298,-0.644920958162315));
#78812=DIRECTION('center_axis',(0.0881576937942685,-0.987363722413996,0.131685613054932));
#78813=DIRECTION('ref_axis',(0.792784541219236,-0.0104932863050875,-0.60941165245368));
#78814=DIRECTION('',(0.160458295775008,0.,-0.987042620820894));
#78815=DIRECTION('center_axis',(0.,-1.,0.));
#78816=DIRECTION('ref_axis',(0.,0.,-1.));
#78817=DIRECTION('center_axis',(-0.106970493768576,0.987363722044527,-0.116919604229933));
#78818=DIRECTION('ref_axis',(0.692047709918238,-0.0104936191287768,-0.721775485282302));
#78819=DIRECTION('center_axis',(0.0901849707939082,0.987363721562147,0.130305611490251));
#78820=DIRECTION('ref_axis',(0.74533268947275,0.0198684729177045,-0.666396597970935));
#78821=DIRECTION('',(-0.987042621082596,0.,-0.160458294165178));
#78822=DIRECTION('center_axis',(-0.0814487385773337,-0.987363722310449,
-0.135937422549555));
#78823=DIRECTION('ref_axis',(0.884969829016091,-0.00890473544370706,-0.465563215275765));
#78824=DIRECTION('center_axis',(0.0577880997168462,-0.987363722387455,0.147558175796212));
#78825=DIRECTION('ref_axis',(0.905255170761543,-0.0104932883859293,-0.424738704038541));
#78826=DIRECTION('',(0.368891856208119,0.,-0.929472322569816));
#78827=DIRECTION('center_axis',(-1.03308683298469E-13,-1.,5.85911991188191E-14));
#78828=DIRECTION('ref_axis',(1.,-1.03308683298469E-13,-1.34828625307809E-30));
#78829=DIRECTION('center_axis',(-0.0793353189734799,0.987363722004231,-0.137181586349362));
#78830=DIRECTION('ref_axis',(0.831028411874342,-0.0104936257469269,-0.556130976008612));
#78831=DIRECTION('center_axis',(0.0600646425439804,0.987363721585129,0.146646241048408));
#78832=DIRECTION('ref_axis',(0.87116279556875,0.0198684718001344,-0.49059211922448));
#78833=DIRECTION('',(-0.929472323171464,0.,-0.368891854692188));
#78834=DIRECTION('center_axis',(-0.0503219877413936,-0.987363722316605,
-0.150268351301444));
#78835=DIRECTION('ref_axis',(0.964362055625502,-0.0089047387008506,-0.264436251861248));
#78836=DIRECTION('center_axis',(0.0247164004782463,-0.98736372239089,0.156531080791658));
#78837=DIRECTION('ref_axis',(0.975397074152575,-0.0104932879170649,-0.220205446443284));
#78838=DIRECTION('',(0.560076443596158,0.,-0.828440931707674));
#78839=DIRECTION('center_axis',(0.,-1.,0.));
#78840=DIRECTION('ref_axis',(0.,0.,-1.));
#78841=DIRECTION('center_axis',(-0.0479905184903675,0.987363721986371,-0.151029105275263));
#78842=DIRECTION('ref_axis',(0.93115115039746,-0.0104936244188649,-0.36448239869717));
#78843=DIRECTION('center_axis',(0.0271357589007339,0.987363721594987,0.156129855783506));
#78844=DIRECTION('ref_axis',(0.956258297310921,0.0198684704798575,-0.291848098682876));
#78845=DIRECTION('',(-0.828440931287221,0.,-0.560076444218074));
#78846=DIRECTION('center_axis',(-0.0168422317619783,-0.987363722303815,
-0.157572900930427));
#78847=DIRECTION('ref_axis',(0.9986617842021,-0.00890473654938958,-0.0509445428015999));
#78848=DIRECTION('center_axis',(-0.0095110139153878,-0.987363722326397,
0.158184766801555));
#78849=DIRECTION('ref_axis',(0.999930494315556,-0.0104932914060547,-0.00537562771357042));
#78850=DIRECTION('',(0.725072479416806,0.,-0.688672563409031));
#78851=DIRECTION('center_axis',(1.47952784583182E-14,-1.,-1.2247177407368E-15));
#78852=DIRECTION('ref_axis',(1.,1.47952784583182E-14,-9.42445205896519E-33));
#78853=DIRECTION('center_axis',(-0.0144017381581264,0.98736372201421,-0.157814671017212));
#78854=DIRECTION('ref_axis',(0.987734295571055,-0.0104936198849398,-0.155791030853714));
#78855=DIRECTION('center_axis',(-0.00706196206119799,0.987363721631619,
0.158313012407715));
#78856=DIRECTION('ref_axis',(0.99664022404459,0.0198684685501518,-0.0794575847469598));
#78857=DIRECTION('',(-0.688672563156092,0.,-0.725072479657047));
#78858=DIRECTION('center_axis',(0.0174250494756407,-0.987363722319657,-0.157509515578722));
#78859=DIRECTION('ref_axis',(0.986265197685238,-0.00890473293355562,0.164929274436897));
#78860=DIRECTION('center_axis',(-0.0432936989265123,-0.987363722380122,
0.152441908151695));
#78861=DIRECTION('ref_axis',(0.977708276320475,-0.0104932898364058,0.209705549003491));
#78862=DIRECTION('',(0.85616493303156,-6.23377073251911E-15,-0.516702629611138));
#78863=DIRECTION('center_axis',(0.,-1.,0.));
#78864=DIRECTION('ref_axis',(0.,0.,-1.));
#78865=DIRECTION('center_axis',(0.0198604574059867,0.98736372203083,-0.157220999389557));
#78866=DIRECTION('ref_axis',(0.998132083080332,-0.0104936214945499,0.0601849535485897));
#78867=DIRECTION('center_axis',(-0.0409294756228172,0.987363721602464,0.153093629157369));
#78868=DIRECTION('ref_axis',(0.99042036160996,0.0198684691135502,0.136648275669615));
#78869=DIRECTION('',(-0.516702631843025,0.,-0.856164931684597));
#78870=DIRECTION('center_axis',(0.0508775475539415,-0.987363722317753,-0.150081161395184));
#78871=DIRECTION('ref_axis',(0.927751945958094,-0.00890473735616938,0.373091185132519));
#78872=DIRECTION('center_axis',(-0.075052025203131,-0.987363722271263,0.139571033726721));
#78873=DIRECTION('ref_axis',(0.909769504880944,-0.0104932946190869,0.414981130603211));
#78874=DIRECTION('',(0.947224063311177,-6.23377072438015E-15,-0.320572260004298));
#78875=DIRECTION('center_axis',(1.11536613512245E-13,-1.,4.08068196962375E-14));
#78876=DIRECTION('ref_axis',(1.,1.11536613512245E-13,2.49166158235023E-31));
#78877=DIRECTION('center_axis',(0.0531940004054215,0.987363721999169,-0.149275848015733));
#78878=DIRECTION('ref_axis',(0.961858323093725,-0.0104936232507952,0.273346758104787));
#78879=DIRECTION('center_axis',(-0.0728831743619325,0.987363721576898,0.140715756789161));
#78880=DIRECTION('ref_axis',(0.937889543295604,0.019868471341455,0.346364617741648));
#78881=DIRECTION('',(-0.320572261549173,0.,-0.94722406278834));
#78882=DIRECTION('center_axis',(0.0819510725694303,-0.987363722321963,-0.135635178133246));
#78883=DIRECTION('ref_axis',(0.825858045362124,-0.00890473659940747,0.563807763849299));
#78884=DIRECTION('center_axis',(-0.10330099281142,-0.987363722350749,0.120173976674849));
#78885=DIRECTION('ref_axis',(0.799290923600527,-0.0104932893936424,0.600852652758992));
#78886=DIRECTION('',(0.993992051028923,6.23377071783232E-15,-0.109452284084504));
#78887=DIRECTION('center_axis',(0.,-1.,0.));
#78888=DIRECTION('ref_axis',(0.,0.,-1.));
#78889=DIRECTION('center_axis',(0.0840402479765716,0.987363722025755,-0.134350724402526));
#78890=DIRECTION('ref_axis',(0.880609137464754,-0.0104936222499426,0.473727169271151));
#78891=DIRECTION('center_axis',(-0.101428934845169,0.98736372155012,0.121758172386384));
#78892=DIRECTION('ref_axis',(0.841504053053872,0.0198684718986061,0.539885332749762));
#78893=DIRECTION('',(-0.109452286018412,0.,-0.993992050815973));
#78894=DIRECTION('center_axis',(0.109192655757424,-0.987363722338937,-0.114847044966942));
#78895=DIRECTION('ref_axis',(0.685347939677887,-0.00890473688215913,0.728161319516723));
#78896=DIRECTION('center_axis',(-0.126719726918145,-0.987363722313106,0.0951577147150889));
#78897=DIRECTION('ref_axis',(0.651438386396749,-0.0104932911252255,0.758628973589963));
#78898=DIRECTION('',(0.994282074768413,0.,0.106785559858154));
#78899=DIRECTION('center_axis',(0.,-1.,0.));
#78900=DIRECTION('ref_axis',(0.,0.,-1.));
#78901=DIRECTION('center_axis',(0.110956868842276,0.987363722031638,-0.113143509193188));
#78902=DIRECTION('ref_axis',(0.758183647957641,-0.0104936236265723,0.651956624195834));
#78903=DIRECTION('center_axis',(-0.125231991823691,0.987363721532925,0.0971073098408352));
#78904=DIRECTION('ref_axis',(0.705770767641394,0.0198684735905038,0.708161611004198));
#78905=DIRECTION('',(0.106785558236532,0.,-0.994282074942575));
#78906=DIRECTION('center_axis',(0.131328513345731,-0.987363722333514,-0.0886887896078565));
#78907=DIRECTION('ref_axis',(0.512791724826996,-0.00890473470600238,0.858466861706828));
#78908=DIRECTION('center_axis',(-0.14421318479626,-0.987363722360672,0.0656919865508537));
#78909=DIRECTION('ref_axis',(0.473125316803008,-0.0104932893774458,0.880932645256205));
#78910=DIRECTION('',(0.948080573707217,0.,0.318030227744147));
#78911=DIRECTION('center_axis',(1.60245723675726E-14,-1.,2.49962771693286E-14));
#78912=DIRECTION('ref_axis',(2.60545369112877E-31,-2.49962771693286E-14,
-1.));
#78913=DIRECTION('center_axis',(0.132685267518363,0.987363722025376,-0.0866458320508048));
#78914=DIRECTION('ref_axis',(0.600306333746986,-0.0104936211668166,0.799701312727483));
#78915=DIRECTION('center_axis',(-0.143179334653652,0.987363721650584,0.0679158250810903));
#78916=DIRECTION('ref_axis',(0.537036428165803,0.0198684662055829,0.843325037499512));
#78917=DIRECTION('',(0.318030226197875,0.,-0.948080574225908));
#78918=DIRECTION('center_axis',(0.147323593750354,-0.987363722328393,-0.058383546948617));
#78919=DIRECTION('ref_axis',(0.316257941884461,-0.00890473470053631,0.948631445765382));
#78920=DIRECTION('center_axis',(-0.154963396007214,-0.987363722357769,0.0331545723803159));
#78921=DIRECTION('ref_axis',(0.272689429059446,-0.0104932892324504,0.962044887809461));
#78922=DIRECTION('',(0.857547878362251,0.,0.514404156589351));
#78923=DIRECTION('center_axis',(-2.56911651515087E-14,-1.,-6.96417186706459E-14));
#78924=DIRECTION('ref_axis',(5.51927619771536E-31,6.96417186706459E-14,
-1.));
#78925=DIRECTION('center_axis',(0.148209454900643,0.987363721999609,-0.0560966840119264));
#78926=DIRECTION('ref_axis',(0.414359359374223,-0.0104936275490271,0.910052858398811));
#78927=DIRECTION('center_axis',(-0.154431776622887,0.987363721630883,0.0355486649019513));
#78928=DIRECTION('ref_axis',(0.343190859386594,0.0198684674577238,0.939055524468267));
#78929=DIRECTION('',(0.514404155190728,0.,-0.857547879201222));
#78930=DIRECTION('center_axis',(0.156429986048551,-0.987363722317835,-0.0253483592273561));
#78931=DIRECTION('ref_axis',(0.104936288763443,-0.00890473956698211,0.994439078533119));
#78932=DIRECTION('center_axis',(-0.158467691048673,-0.987363722338777,-0.000933114686009084));
#78933=DIRECTION('ref_axis',(0.0595028880774467,-0.0104932912931376,0.998172979572319));
#78934=DIRECTION('',(0.726917198560946,0.,0.686725117085655));
#78935=DIRECTION('center_axis',(-6.07176543710283E-15,-1.,-4.41218250330748E-14));
#78936=DIRECTION('ref_axis',(1.229306260954E-32,4.41218250330748E-14,-1.));
#78937=DIRECTION('center_axis',(0.156803528780516,0.987363722000409,-0.0229245248473604));
#78938=DIRECTION('ref_axis',(0.209037406064962,-0.0104936259099717,0.977851341810653));
#78939=DIRECTION('center_axis',(-0.158463159546821,0.987363721647528,0.00151928956512539));
#78940=DIRECTION('ref_axis',(0.133298067969916,0.0198684676897788,0.990876818311513));
#78941=DIRECTION('center_axis',(1.18502573726487E-15,-1.,-1.47985104495617E-14));
#78942=DIRECTION('ref_axis',(5.2890212177402E-33,1.47985104495617E-14,-1.));
#78943=DIRECTION('center_axis',(0.15822188745822,-0.987363722342132,0.00887209850308879));
#78944=DIRECTION('ref_axis',(-0.111292072300084,-0.00890473567894903,0.993747845444528));
#78945=DIRECTION('center_axis',(0.158065644488417,0.987363722016583,0.0113195617415647));
#78946=DIRECTION('ref_axis',(-0.00605890847863349,-0.01049362580408,0.999926584027813));
#78947=DIRECTION('center_axis',(-0.155084981185087,0.987363721609556,-0.032581127361534));
#78948=DIRECTION('ref_axis',(-0.082827591604534,0.0198684694891143,0.99636581333823));
#78949=DIRECTION('',(0.686725115900101,0.,-0.726917199680949));
#78950=DIRECTION('center_axis',(0.160735571009733,-0.986495108236408,-0.0314877378961024));
#78951=DIRECTION('ref_axis',(0.0338459065175243,-0.026374683548954,0.999078991211255));
#78952=DIRECTION('center_axis',(0.150208716674817,-0.98649510778408,-0.0653050055736983));
#78953=DIRECTION('ref_axis',(0.247827082207865,-0.0263747191535445,0.968445203154989));
#78954=DIRECTION('center_axis',(0.132658271716979,-0.986495107714006,-0.09606864942007));
#78955=DIRECTION('ref_axis',(0.450220114874771,-0.026374724543006,0.89252799511692));
#78956=DIRECTION('center_axis',(0.108904879252692,-0.986495107784954,-0.122340220660702));
#78957=DIRECTION('ref_axis',(0.631561354084168,-0.026374718820451,0.774877171062946));
#78958=DIRECTION('center_axis',(0.0800592132564947,-0.986495107789174,-0.142891303726913));
#78959=DIRECTION('ref_axis',(0.78337148772173,-0.0263747179124343,0.620993950437267));
#78960=DIRECTION('center_axis',(0.0474700634140202,-0.986495107779111,-0.156760949880223));
#78961=DIRECTION('ref_axis',(0.898552041178325,-0.0263747212958625,0.438073741932602));
#78962=DIRECTION('center_axis',(0.0126612724730868,-0.986495107813198,-0.163300625963248));
#78963=DIRECTION('ref_axis',(0.971717298672813,-0.0263747183100887,0.234669694877874));
#78964=DIRECTION('center_axis',(-0.0227395414182952,-0.986495107969959,
-0.162204547431399));
#78965=DIRECTION('ref_axis',(0.999446135984411,-0.0263747114092139,0.0202927539755223));
#78966=DIRECTION('center_axis',(-0.057077088049556,-0.986495107936662,-0.153523965675774));
#78967=DIRECTION('ref_axis',(0.980441982767649,-0.0263747128260375,-0.195033056044317));
#78968=DIRECTION('center_axis',(-0.0887457768143703,-0.986495107851645,
-0.137664771391902));
#78969=DIRECTION('ref_axis',(0.915593452045644,-0.0263747184035609,-0.401239336058012));
#78970=DIRECTION('center_axis',(-0.11626480563914,-0.986495107850101,-0.115368527586643));
#78971=DIRECTION('ref_axis',(0.807932787678787,-0.0263747169054886,-0.588684113002669));
#78972=DIRECTION('center_axis',(-0.138347424378308,-0.986495107799886,-0.0876777762878373));
#78973=DIRECTION('ref_axis',(0.662494084335353,-0.0263747202768151,-0.748602673219233));
#78974=DIRECTION('center_axis',(-0.153961068298618,-0.986495107760049,-0.0558873135321256));
#78975=DIRECTION('ref_axis',(0.48607789980036,-0.0263747196220043,-0.873517400794358));
#78976=DIRECTION('center_axis',(-0.16237566480624,-0.986495107781903,-0.0214836170395995));
#78977=DIRECTION('ref_axis',(0.28693324431429,-0.0263747224425676,-0.957587430641899));
#78978=DIRECTION('center_axis',(-0.163197754870596,-0.986495107694381,0.0139246292679042));
#78979=DIRECTION('ref_axis',(0.0743719117694134,-0.0263747254297085,-0.9968817345093));
#78980=DIRECTION('center_axis',(-0.156388898490704,-0.986495107734565,0.0486817711739611));
#78981=DIRECTION('ref_axis',(-0.14166696604054,-0.026374724445378,-0.989562956381906));
#78982=DIRECTION('center_axis',(-0.14226747115853,-0.986495107737351,0.0811626087581541));
#78983=DIRECTION('ref_axis',(-0.351081656040152,-0.0263747243360462,-0.935973314100515));
#78984=DIRECTION('center_axis',(-0.121493781342904,-0.986495107917773,0.109848364345144));
#78985=DIRECTION('ref_axis',(-0.544080153780647,-0.0263747142436309,-0.838618602649974));
#78986=DIRECTION('center_axis',(-0.0950391693815611,-0.986495107856857,
0.133397745324843));
#78987=DIRECTION('ref_axis',(-0.711638074696993,-0.0263747184469962,-0.702051013010022));
#78988=DIRECTION('center_axis',(-0.0641406289410978,-0.986495107726884,
0.150709595414372));
#78989=DIRECTION('ref_axis',(-0.84592058827809,-0.0263747244747136,-0.532656298410273));
#78990=DIRECTION('center_axis',(-0.0302429488762457,-0.986495107736434,
0.160974427954722));
#78991=DIRECTION('ref_axis',(-0.940648794174339,-0.0263747240848742,-0.338355168348007));
#78992=DIRECTION('center_axis',(0.00506885405486264,-0.986495107766302,
0.163712275262799));
#78993=DIRECTION('ref_axis',(-0.991393307475592,-0.0263747202754443,-0.128232928778058));
#78994=DIRECTION('center_axis',(0.0401436540411063,-0.986495107671852,0.158795118249051));
#78995=DIRECTION('ref_axis',(-0.99578137173735,-0.026374727357795,0.0878853426783058));
#78996=DIRECTION('center_axis',(0.0733413717326372,-0.986495107710258,0.146452878620057));
#78997=DIRECTION('ref_axis',(-0.95360780588139,-0.0263747246785699,0.29989419210817));
#78998=DIRECTION('center_axis',(0.103109727120042,-0.986495107818647,0.127262667043824));
#78999=DIRECTION('ref_axis',(-0.866844599765875,-0.0263747203806475,0.497880320942274));
#79000=DIRECTION('center_axis',(0.128056786609181,-0.986495107867452,0.102121797658064));
#79001=DIRECTION('ref_axis',(-0.739548704901369,-0.0263747148151698,0.672586119019064));
#79002=DIRECTION('center_axis',(0.147016061558686,-0.986495107750468,0.0722058171352182));
#79003=DIRECTION('ref_axis',(-0.577672332535789,-0.0263747217122836,0.815842540124784));
#79004=DIRECTION('center_axis',(0.159101024800094,-0.986495107740196,0.0389135749092782));
#79005=DIRECTION('ref_axis',(-0.388784639613202,-0.0263747238453144,0.92095107250218));
#79006=DIRECTION('center_axis',(0.163746574337308,-0.986495111251671,0.00380195599009181));
#79007=DIRECTION('ref_axis',(-0.181717844385214,-0.0263745487091407,0.982996952290484));
#79008=DIRECTION('center_axis',(-0.159100997357643,0.98649510752794,-0.0389136924904468));
#79009=DIRECTION('ref_axis',(-0.0837188756473344,0.02579266142082,0.996155554357439));
#79010=DIRECTION('center_axis',(0.158479747774604,0.986495108552522,0.0413711293929183));
#79011=DIRECTION('ref_axis',(-0.188882155795407,-0.0108363123862134,0.981939970444196));
#79012=DIRECTION('center_axis',(-0.147016016485829,0.986495108226829,-0.0722059023984579));
#79013=DIRECTION('ref_axis',(-0.295905551411954,0.0257926430848816,0.954868914671686));
#79014=DIRECTION('center_axis',(0.145881036647377,0.98649510866697,0.0744723017156756));
#79015=DIRECTION('ref_axis',(-0.395554272691206,-0.0108362488831137,0.918378676290927));
#79016=DIRECTION('center_axis',(-0.12805672646284,0.986495108187664,-0.102121869985965));
#79017=DIRECTION('ref_axis',(-0.49425603816082,0.0257926470332549,0.868933661507361));
#79018=DIRECTION('center_axis',(0.126461036348405,0.986495108605843,0.104091339613025));
#79019=DIRECTION('ref_axis',(-0.583730693143186,-0.0108363135264812,0.811875022519927));
#79020=DIRECTION('center_axis',(-0.103109645269706,0.986495108091246,-0.127262731246802));
#79021=DIRECTION('ref_axis',(-0.669495658588641,0.0257926510703653,0.742368036947796));
#79022=DIRECTION('center_axis',(0.101127884369277,0.98649510856977,0.128843128535876));
#79023=DIRECTION('ref_axis',(-0.744612526030204,-0.0108363161639954,0.667408990298237));
#79024=DIRECTION('center_axis',(-0.0733412770708288,0.986495108148242,-0.146452923074984));
#79025=DIRECTION('ref_axis',(-0.813430404670402,0.0257926474265038,0.581090110134803));
#79026=DIRECTION('center_axis',(0.0710661069826356,0.986495108527701,0.147570353693592));
#79027=DIRECTION('ref_axis',(-0.870677103550572,-0.0108363157948494,0.491735656234914));
#79028=DIRECTION('center_axis',(-0.0401435546289612,0.986495108250283,-0.15879513978713));
#79029=DIRECTION('ref_axis',(-0.919330050714222,0.0257926418184515,0.392641054249057));
#79030=DIRECTION('center_axis',(0.0376813611744201,0.986495108564832,0.15939735191559));
#79031=DIRECTION('ref_axis',(-0.956029786695043,-0.0108363116963436,0.293069311427605));
#79032=DIRECTION('center_axis',(-0.00506877383917619,0.986495109538723,
-0.163712267066185));
#79033=DIRECTION('ref_axis',(-0.982242845537332,0.0257926261277419,0.18583253974522));
#79034=DIRECTION('center_axis',(0.00253467411141179,0.986495108531174,0.163771109391173));
#79035=DIRECTION('ref_axis',(-0.996679580402424,-0.010836310684072,0.0806993703792479));
#79036=DIRECTION('center_axis',(0.030243052772592,0.986495108131346,-0.160974406015112));
#79037=DIRECTION('ref_axis',(-0.999227055883883,0.0257926494833967,-0.0296652999690604));
#79038=DIRECTION('center_axis',(-0.0327304788680687,0.98649510864271,0.160487122153385));
#79039=DIRECTION('ref_axis',(-0.990725744073173,-0.0108362535714797,-0.13544399447444));
#79040=DIRECTION('center_axis',(0.0641407249324134,0.986495108138678,-0.150709551865841));
#79041=DIRECTION('ref_axis',(-0.969488520532474,0.0257926487542448,-0.24377601979275));
#79042=DIRECTION('center_axis',(-0.066465247725591,0.986495108659402,0.149698935987706));
#79043=DIRECTION('ref_axis',(-0.938446671669539,-0.0108362558229288,-0.345254138269339));
#79044=DIRECTION('center_axis',(0.0950392464485186,0.986495108205489,-0.133397687840304));
#79045=DIRECTION('ref_axis',(-0.894417778304127,0.0257926452473245,-0.446488048333497));
#79046=DIRECTION('center_axis',(-0.0970922211053784,0.986495108544631,0.131910960190357));
#79047=DIRECTION('ref_axis',(-0.842286880175986,-0.0108363168256393,-0.538920574594308));
#79048=DIRECTION('center_axis',(0.121493846397364,0.986495108098352,-0.109848290772291));
#79049=DIRECTION('ref_axis',(-0.77752505341967,0.0257926516741728,-0.628322791584353));
#79050=DIRECTION('center_axis',(-0.123179214736194,0.98649510858114,0.10795499896929));
#79051=DIRECTION('ref_axis',(-0.706742688013733,-0.0108363149944035,-0.707387692299255));
#79052=DIRECTION('center_axis',(0.142267519731351,0.986495108183289,-0.0811625181960835));
#79053=DIRECTION('ref_axis',(-0.624276124919574,0.0257926459277216,-0.78077785526451));
#79054=DIRECTION('center_axis',(-0.143506486862139,0.986495108529785,0.0789511815953027));
#79055=DIRECTION('ref_axis',(-0.538151993297995,-0.0108363146180653,-0.842778147791513));
#79056=DIRECTION('center_axis',(0.156388927828418,0.986495108133772,-0.0486816688376107));
#79057=DIRECTION('ref_axis',(-0.441836737174637,0.025792649754231,-0.896724615978354));
#79058=DIRECTION('center_axis',(-0.157123555131713,0.986495108582043,0.046255693341188));
#79059=DIRECTION('ref_axis',(-0.344397908228475,-0.0108363152052421,-0.938761234329914));
#79060=DIRECTION('center_axis',(0.163197761691791,0.98649510810079,-0.0139245205303402));
#79061=DIRECTION('ref_axis',(-0.238737553542187,0.0257926509570806,-0.97074153083367));
#79062=DIRECTION('center_axis',(-0.163393695748629,0.986495108696646,0.0113973991417967));
#79063=DIRECTION('ref_axis',(-0.134540152524605,-0.0108362549029294,-0.990848890062624));
#79064=DIRECTION('center_axis',(0.162375649064761,0.986495108153596,0.0214837189476841));
#79065=DIRECTION('ref_axis',(-0.0244752698996862,0.0257926484885163,-0.999367650290565));
#79066=DIRECTION('center_axis',(-0.162023738619945,0.986495108586251,-0.0239939337962111));
#79067=DIRECTION('ref_axis',(0.0816085326334352,-0.0108363112271417,-0.996605549733898));
#79068=DIRECTION('center_axis',(0.153961032422443,0.986495108170358,0.0558874051228876));
#79069=DIRECTION('ref_axis',(0.190931452696257,0.0257926471489565,-0.98126444943468));
#79070=DIRECTION('center_axis',(-0.153077727573336,0.986495108555797,-0.0582632827471033));
#79071=DIRECTION('ref_axis',(0.293941306053273,-0.0108363101764777,-0.955762043072153));
#79072=DIRECTION('center_axis',(0.138347370174831,0.986495108190401,0.0876778574220337));
#79073=DIRECTION('ref_axis',(0.397410430852247,0.0257926448954982,-0.917278414070192));
#79074=DIRECTION('center_axis',(-0.136973968593323,0.986495108545223,-0.0898083111084));
#79075=DIRECTION('ref_axis',(0.492529708452136,-0.0108363163076087,-0.870228165793854));
#79076=DIRECTION('center_axis',(0.116264737376085,0.986495108195573,0.115368593425922));
#79077=DIRECTION('ref_axis',(0.585306940258781,0.0257926456565238,-0.810401459225574));
#79078=DIRECTION('center_axis',(-0.114465461008113,0.98649510855171,-0.117153997113845));
#79079=DIRECTION('ref_axis',(0.668087970700035,-0.010836316193007,-0.744003385514659));
#79080=DIRECTION('center_axis',(0.0887457396433074,0.986495110261859,0.137664778082866));
#79081=DIRECTION('ref_axis',(0.745835155355629,0.0257925810343138,-0.665631026770261));
#79082=DIRECTION('center_axis',(-0.0866046781088066,0.986495108574076,-0.139021690714405));
#79083=DIRECTION('ref_axis',(0.812407179532708,-0.0108363136409741,-0.582989836060959));
#79084=DIRECTION('center_axis',(0.0570770025958331,0.986495108207936,0.153523995702587));
#79085=DIRECTION('ref_axis',(0.871488933067144,0.0257926456383099,-0.489736438273146));
#79086=DIRECTION('center_axis',(-0.0546943527508883,0.986495108539707,-0.154388887567706));
#79087=DIRECTION('ref_axis',(0.918739133301432,-0.0108363157338381,-0.394716327508567));
#79088=DIRECTION('center_axis',(0.0227394532199647,0.986495108204772,0.162204558367862));
#79089=DIRECTION('ref_axis',(0.956392864428311,0.0257926451466668,-0.290942310994721));
#79090=DIRECTION('center_axis',(-0.0202265838329727,0.986495108564546,-0.162537029887571));
#79091=DIRECTION('ref_axis',(0.982111865497668,-0.0108363139982903,-0.187986323831341));
#79092=DIRECTION('center_axis',(-0.0126613696931214,0.986495108187824,0.1633006161623));
#79093=DIRECTION('ref_axis',(0.996576927422038,0.0257926468525222,-0.0785440455947577));
#79094=DIRECTION('center_axis',(0.0151869637456814,0.986495108589766,-0.163085121518345));
#79095=DIRECTION('ref_axis',(0.999562138566932,-0.0108363183416792,0.0275337129406814));
#79096=DIRECTION('center_axis',(-0.0474701574982222,0.986495108181291,0.156760918858867));
#79097=DIRECTION('ref_axis',(0.990162161023867,0.0257926453276796,0.137526849464193));
#79098=DIRECTION('center_axis',(0.0498903833976718,0.986495108560806,-0.156007533247715));
#79099=DIRECTION('ref_axis',(0.970273996606324,-0.0108363203371629,0.241766303837284));
#79100=DIRECTION('center_axis',(-0.0800592947092413,0.98649510820446,0.142891255223438));
#79101=DIRECTION('ref_axis',(0.93744851294225,0.0257926448400367,0.347167142821033));
#79102=DIRECTION('center_axis',(0.082260972070614,0.986495108556871,-0.141635211961453));
#79103=DIRECTION('ref_axis',(0.895616922134147,-0.0108363090296816,0.444694168157815));
#79104=DIRECTION('center_axis',(-0.1089049496773,0.986495108205681,0.122340154577497));
#79105=DIRECTION('ref_axis',(0.840900814631357,0.0257926460076625,0.540574286628807));
#79106=DIRECTION('center_axis',(0.110785147588489,0.986495108531122,-0.120640175389326));
#79107=DIRECTION('ref_axis',(0.779081793886847,-0.0108363188476222,0.626828630989272));
#79108=DIRECTION('center_axis',(-0.1326583321652,0.986495108139982,0.0960685615747012));
#79109=DIRECTION('ref_axis',(0.705033525947712,0.025792649733389,0.70870478092748));
#79110=DIRECTION('center_axis',(0.1341291247422,0.986495108557981,-0.0940041418612458));
#79111=DIRECTION('ref_axis',(0.626117669612743,-0.0108363207540363,0.779653280600565));
#79112=DIRECTION('center_axis',(-0.150208754328115,0.986495108142209,0.0653049135570062));
#79113=DIRECTION('ref_axis',(0.536199657697366,0.0257926484359865,0.843697022853515));
#79114=DIRECTION('center_axis',(0.151201369427729,0.986495108577346,-0.0629725863860636));
#79115=DIRECTION('ref_axis',(0.443876975459743,-0.0108363136168601,0.896022212316139));
#79116=DIRECTION('center_axis',(-0.160735582317945,0.986495108181445,0.0314876818929413));
#79117=DIRECTION('ref_axis',(0.342293688451243,0.0257926455307577,0.939238931413604));
#79118=DIRECTION('center_axis',(0.161203610189716,0.986495108559943,-0.0289964971868899));
#79119=DIRECTION('ref_axis',(0.240881089900806,-0.0108363139760407,0.970494139512245));
#79120=DIRECTION('center_axis',(-0.16374658310287,0.986495110327121,-0.00380181835653959));
#79121=DIRECTION('ref_axis',(0.132382437034705,0.0257925790892707,0.990863074914327));
#79122=DIRECTION('center_axis',(0.163668141680259,0.986495109676435,0.00633545447533204));
#79123=DIRECTION('ref_axis',(0.0266218532422533,-0.0108363296107072,0.999586840094704));
#79124=DIRECTION('center_axis',(-0.154431767361342,0.987363722573609,0.0355486789520771));
#79125=DIRECTION('ref_axis',(0.139174517129888,-0.0138817019862933,0.990170567191141));
#79126=DIRECTION('',(-0.727678230552677,0.,-0.68591864880591));
#79127=DIRECTION('center_axis',(8.16091499892112E-15,-1.,5.88200858810152E-14));
#79128=DIRECTION('ref_axis',(1.05765828811544E-31,-5.88200858810152E-14,
-1.));
#79129=DIRECTION('center_axis',(-0.154431767361249,-0.987363722573576,0.0355486789533851));
#79130=DIRECTION('ref_axis',(0.0663140400757799,0.0255405502863858,0.99747186846542));
#79131=DIRECTION('',(-0.513452942861744,0.,0.858117751515848));
#79132=DIRECTION('center_axis',(-0.1431793235287,0.987363722550876,0.0679158354460898));
#79133=DIRECTION('ref_axis',(0.348778095876434,-0.0138817019407607,0.937102522773275));
#79134=DIRECTION('',(-0.858117752273735,0.,-0.513452941595112));
#79135=DIRECTION('center_axis',(1.54610228332736E-14,-1.,4.17679121291167E-14));
#79136=DIRECTION('ref_axis',(2.92220659082831E-31,-4.17679121291167E-14,
-1.));
#79137=DIRECTION('center_axis',(-0.143179323527856,-0.9873637225508,0.0679158354489722));
#79138=DIRECTION('ref_axis',(0.279190622005061,0.0255405499579519,0.959895971911682));
#79139=DIRECTION('',(-0.316978747916834,0.,0.948432640396289));
#79140=DIRECTION('center_axis',(-0.125231975596325,0.987363722629922,0.0971073196140432));
#79141=DIRECTION('ref_axis',(0.542073198201638,-0.0138816980343954,0.840216606745623));
#79142=DIRECTION('',(-0.948432641260561,0.,-0.316978745330844));
#79143=DIRECTION('center_axis',(-8.02613972714816E-15,-1.,-1.24892462308838E-14));
#79144=DIRECTION('ref_axis',(-6.1223084794885E-33,1.24892462308838E-14,
-1.));
#79145=DIRECTION('center_axis',(-0.125231975595508,-0.987363722629879,0.0971073196155321));
#79146=DIRECTION('ref_axis',(0.479012558830294,0.0255405459996456,0.877436407378275));
#79147=DIRECTION('',(-0.105682979626772,0.,0.994399873198507));
#79148=DIRECTION('center_axis',(-0.101428915968318,0.987363722535096,0.121758180124088));
#79149=DIRECTION('ref_axis',(0.710021563218345,-0.0138817014069173,0.704043093944559));
#79150=DIRECTION('',(-0.994399873500629,0.,-0.10568297678403));
#79151=DIRECTION('center_axis',(1.05233118009756E-14,-1.,1.04718718035991E-14));
#79152=DIRECTION('ref_axis',(1.,1.05233118009756E-14,7.09245862821757E-33));
#79153=DIRECTION('center_axis',(-0.1014289159663,-0.987363722535019,0.121758180126395));
#79154=DIRECTION('ref_axis',(0.656436402981568,0.0255405495051092,0.753948890291376));
#79155=DIRECTION('',(0.110554410161169,0.,0.993870073195645));
#79156=DIRECTION('center_axis',(-0.072883153345059,0.987363722527268,0.140715761006283));
#79157=DIRECTION('ref_axis',(0.844770107743317,-0.01388170288603,0.53494930917642));
#79158=DIRECTION('',(-0.993870073195645,0.,0.110554410161163));
#79159=DIRECTION('center_axis',(8.76989783374246E-14,-1.,5.57539098784638E-14));
#79160=DIRECTION('ref_axis',(1.,8.76989783374246E-14,1.1265317878891E-30));
#79161=DIRECTION('center_axis',(-0.0728831533423562,-0.987363722527182,
0.140715761008282));
#79162=DIRECTION('ref_axis',(0.803166008716124,0.025540551261839,0.595207562690741));
#79163=DIRECTION('',(0.321622397477402,0.,0.946868012682279));
#79164=DIRECTION('center_axis',(-0.0409294572073719,0.98736372258034,0.153093627773999));
#79165=DIRECTION('ref_axis',(0.940018140150174,-0.013881702361494,0.340841890805919));
#79166=DIRECTION('',(-0.946868013557757,0.,0.321622394899963));
#79167=DIRECTION('center_axis',(-6.97386197287161E-14,-1.,-2.54269475096828E-14));
#79168=DIRECTION('ref_axis',(1.,-6.9738619728716E-14,-6.95679877401685E-32));
#79169=DIRECTION('center_axis',(-0.040929457207014,-0.987363722580331,0.153093627774153));
#79170=DIRECTION('ref_axis',(0.912340465561708,0.0255405505164363,0.408634990153761));
#79171=DIRECTION('',(0.517651677844017,0.,0.855591456493854));
#79172=DIRECTION('center_axis',(-0.00706194783320453,0.987363722614641,
0.158313006911495));
#79173=DIRECTION('ref_axis',(0.991311969812551,-0.0138816990973224,0.130797083058193));
#79174=DIRECTION('',(-0.855591457767102,0.,0.517651675739552));
#79175=DIRECTION('center_axis',(0.,-1.,0.));
#79176=DIRECTION('ref_axis',(0.,0.,-1.));
#79177=DIRECTION('center_axis',(-0.00706194783100147,-0.987363722614584,
0.158313006911947));
#79178=DIRECTION('ref_axis',(0.97885489623469,0.0255405473561743,0.202955099857384));
#79179=DIRECTION('',(0.689476142154167,0.,0.724308393849061));
#79180=DIRECTION('center_axis',(0.027135771312802,0.987363722645229,0.156129846984537));
#79181=DIRECTION('ref_axis',(0.996253153475163,-0.0138816971664084,-0.0853636496090367));
#79182=DIRECTION('',(-0.724308395215675,0.,0.689476140718513));
#79183=DIRECTION('center_axis',(1.47939110561966E-14,-1.,-1.24112276742186E-15));
#79184=DIRECTION('ref_axis',(1.,1.47939110561966E-14,-1.12478059837392E-32));
#79185=DIRECTION('center_axis',(0.0271357713158418,-0.987363722645153,0.156129846984491));
#79186=DIRECTION('ref_axis',(0.999599159917687,0.0255405449786543,-0.0122147474000547));
#79187=DIRECTION('',(0.829061466833223,0.,0.559157477113867));
#79188=DIRECTION('center_axis',(0.0600646555848615,0.98736372261194,0.146646228793531));
#79189=DIRECTION('ref_axis',(0.954610646786095,-0.0138816987062048,-0.297532874626762));
#79190=DIRECTION('',(-0.559157478446539,0.,0.829061465934407));
#79191=DIRECTION('center_axis',(4.25436987427772E-14,-1.,-1.31770787232342E-14));
#79192=DIRECTION('ref_axis',(1.,4.25436987427772E-14,-1.95686662459851E-31));
#79193=DIRECTION('center_axis',(0.0600646555883885,-0.987363722611848,0.146646228792703));
#79194=DIRECTION('ref_axis',(0.973603277803162,0.0255405469455389,-0.226813442971669));
#79195=DIRECTION('',(0.929880799447459,0.,0.36786097757027));
#79196=DIRECTION('center_axis',(0.0901849880419648,0.987363722479871,0.130305592598951));
#79197=DIRECTION('ref_axis',(0.868331607406681,-0.0138817060745571,-0.495789791963276));
#79198=DIRECTION('',(-0.367860977570298,0.,0.929880799447448));
#79199=DIRECTION('center_axis',(1.2905456100855E-14,-1.,-7.33821453172643E-15));
#79200=DIRECTION('ref_axis',(1.,1.2905456100855E-14,7.8359382974112E-32));
#79201=DIRECTION('center_axis',(0.0901849880425129,-0.987363722479855,0.130305592598688));
#79202=DIRECTION('ref_axis',(0.902082787661463,0.0255405539856764,-0.430806597334615));
#79203=DIRECTION('',(0.987219939393379,0.,0.15936370748741));
#79204=DIRECTION('center_axis',(0.116088358724509,0.98736372258947,0.107872018071949));
#79205=DIRECTION('ref_axis',(0.741450347498087,-0.0138816993904279,-0.670864129773682));
#79206=DIRECTION('',(-0.159363707939627,0.,0.987219939320379));
#79207=DIRECTION('center_axis',(-6.615740706242E-14,-1.,5.96456564476805E-14));
#79208=DIRECTION('ref_axis',(1.,-6.615740706242E-14,3.94765483631823E-31));
#79209=DIRECTION('center_axis',(0.116088358724872,-0.987363722589458,0.107872018071664));
#79210=DIRECTION('ref_axis',(0.788381910992222,0.0255405475942004,-0.614655710824231));
#79211=DIRECTION('',(0.998397772228337,0.,-0.0565852313726192));
#79212=DIRECTION('center_axis',(0.136563571478651,0.987363722650077,0.0803944658516843));
#79213=DIRECTION('ref_axis',(0.579899693448114,-0.0138816977980671,-0.814569606605247));
#79214=DIRECTION('',(0.0565852313726899,0.,0.998397772228333));
#79215=DIRECTION('center_axis',(-8.63143843731526E-15,-1.,1.20788435100477E-14));
#79216=DIRECTION('ref_axis',(5.52127733821679E-32,-1.20788435100477E-14,
-1.));
#79217=DIRECTION('center_axis',(0.136563571478661,-0.987363722650076,0.0803944658516745));
#79218=DIRECTION('ref_axis',(0.637817169827513,0.0255405456164728,-0.769764209614109));
#79219=DIRECTION('',(0.962891634602509,0.,-0.269888310255389));
#79220=DIRECTION('center_axis',(0.150653224778143,0.987363722643224,0.0491577569876829));
#79221=DIRECTION('ref_axis',(0.391233574762388,-0.0138816977976142,-0.920186713903705));
#79222=DIRECTION('',(0.269888310255455,0.,0.96289163460249));
#79223=DIRECTION('center_axis',(-5.83304589634749E-15,-1.,1.36519509804903E-14));
#79224=DIRECTION('ref_axis',(-3.18463081696841E-32,-1.36519509804903E-14,
-1.));
#79225=DIRECTION('center_axis',(0.150653224778077,-0.987363722643228,0.0491577569878172));
#79226=DIRECTION('ref_axis',(0.457428808928521,0.0255405456747179,-0.888879387368653));
#79227=DIRECTION('',(0.882361755339619,0.,-0.470571708365458));
#79228=DIRECTION('center_axis',(0.157698501629331,0.987363722576351,0.0156224813661074));
#79229=DIRECTION('ref_axis',(0.184273806832079,-0.0138817022434584,-0.982776913881496));
#79230=DIRECTION('',(0.470571708365521,0.,0.882361755339586));
#79231=DIRECTION('center_axis',(-1.10476264533498E-14,-1.,5.8346833597847E-14));
#79232=DIRECTION('ref_axis',(-2.5417154544527E-32,-5.8346833597847E-14,
-1.));
#79233=DIRECTION('center_axis',(0.15769850162929,-0.987363722576355,0.015622481366281));
#79234=DIRECTION('ref_axis',(0.255651581918147,0.0255405499347531,-0.966431554209495));
#79235=DIRECTION('',(0.760573620677732,0.,-0.649251698133447));
#79236=DIRECTION('',(0.649251699553084,0.,0.760573619465882));
#79237=DIRECTION('',(0.603221906321608,0.,-0.797573402097716));
#79238=DIRECTION('center_axis',(0.14968299370784,0.987363722548993,-0.0520373018982967));
#79239=DIRECTION('ref_axis',(-0.245414938382434,-0.0138817019099837,-0.96931873311663));
#79240=DIRECTION('',(0.797573400714641,0.,0.603221908150295));
#79241=DIRECTION('center_axis',(1.08544839876594E-14,-1.,4.31946974113953E-14));
#79242=DIRECTION('ref_axis',(8.99397962473849E-34,-4.31946974113953E-14,
-1.));
#79243=DIRECTION('center_axis',(0.149682993707841,-0.987363722548993,-0.0520373018982921));
#79244=DIRECTION('ref_axis',(-0.173770985052446,0.025540549741825,-0.984454836481993));
#79245=DIRECTION('',(0.417664210217885,0.,-0.908601456912254));
#79246=DIRECTION('center_axis',(0.134997008782224,0.987363722631273,-0.08299811354222));
#79247=DIRECTION('ref_axis',(-0.448052147183188,-0.0138816974014571,-0.893899643070624));
#79248=DIRECTION('',(0.908601457413776,0.,0.417664209126856));
#79249=DIRECTION('center_axis',(-3.97725906070439E-14,-1.,-7.97028723859732E-14));
#79250=DIRECTION('ref_axis',(8.44798570949651E-31,7.97028723859732E-14,
-1.));
#79251=DIRECTION('center_axis',(0.134997008782151,-0.987363722631268,-0.0829981135423979));
#79252=DIRECTION('ref_axis',(-0.381337005043723,0.0255405451368106,-0.924083204662003));
#79253=DIRECTION('',(0.212576996304382,0.,-0.977144319249826));
#79254=DIRECTION('center_axis',(0.113998711847197,0.987363722595133,-0.110078031415265));
#79255=DIRECTION('ref_axis',(-0.629738937334439,-0.0138816988167137,-0.776682798343605));
#79256=DIRECTION('',(0.977144319379751,0.,0.212576995707162));
#79257=DIRECTION('center_axis',(-9.32941520012954E-15,-1.,-1.1548255390224E-14));
#79258=DIRECTION('ref_axis',(-1.54567726138217E-31,1.1548255390224E-14,
-1.));
#79259=DIRECTION('center_axis',(0.113998711845088,-0.987363722595039,-0.110078031418294));
#79260=DIRECTION('ref_axis',(-0.571072129830343,0.0255405469171674,-0.820502469828219));
#79261=DIRECTION('',(-0.00245007782715285,0.,-0.999996998554816));
#79262=DIRECTION('center_axis',(0.0876699563048406,0.987363722480806,-0.132010826413413));
#79263=DIRECTION('ref_axis',(-0.781979834526339,-0.0138817066334,-0.623149128712464));
#79264=DIRECTION('',(0.999996998554795,0.,-0.00245007783568496));
#79265=DIRECTION('center_axis',(3.47814965074125E-14,-1.,2.78181452331395E-14));
#79266=DIRECTION('ref_axis',(1.,3.47814965074125E-14,7.96189918324429E-31));
#79267=DIRECTION('center_axis',(0.0876699563044266,-0.98736372248079,-0.13201082641381));
#79268=DIRECTION('ref_axis',(-0.734104558096312,0.025540554789388,-0.678555950414753));
#79269=DIRECTION('',(-0.217362592525063,0.,-0.976090929868106));
#79270=DIRECTION('center_axis',(0.0572418589303205,0.987363722536242,-0.147770934238016));
#79271=DIRECTION('ref_axis',(-0.897656223127401,-0.0138817032674184,-0.440477699089346));
#79272=DIRECTION('',(0.9760909303422,0.,-0.217362590396092));
#79273=DIRECTION('center_axis',(-2.66322689534313E-14,-1.,-1.31271859147942E-14));
#79274=DIRECTION('ref_axis',(1.,-2.66322689534313E-14,3.23564926775337E-31));
#79275=DIRECTION('center_axis',(0.0572418589303068,-0.987363722536242,-0.147770934238022));
#79276=DIRECTION('ref_axis',(-0.86281107255647,0.0255405515494598,-0.504880910017901));
#79277=DIRECTION('',(-0.422111470626519,0.,-0.906543935154561));
#79278=DIRECTION('center_axis',(0.0241371946610542,0.987363722568252,-0.15662143911374));
#79279=DIRECTION('ref_axis',(-0.97135920429933,-0.0138817018667561,-0.237210022082234));
#79280=DIRECTION('',(0.906543934642298,0.,-0.422111471726677));
#79281=DIRECTION('center_axis',(-1.44157891168532E-14,-1.,-3.54756450935383E-15));
#79282=DIRECTION('ref_axis',(1.,-1.44157891168532E-14,-6.23813188579977E-32));
#79283=DIRECTION('center_axis',(0.0241371946612772,-0.987363722568257,-0.156621439113674));
#79284=DIRECTION('ref_axis',(-0.951173500802478,0.0255405500367738,-0.307598198426091));
#79285=DIRECTION('',(-0.607122889070729,0.,-0.79460795211627));
#79286=DIRECTION('center_axis',(-0.0100960958892223,0.987363722611222,-0.158148500211367));
#79287=DIRECTION('ref_axis',(-0.99964250877371,-0.0138816987180042,-0.0228506694279372));
#79288=DIRECTION('',(0.794607951056583,0.,-0.607122890457656));
#79289=DIRECTION('center_axis',(7.42068874433645E-14,-1.,1.82827944841588E-15));
#79290=DIRECTION('ref_axis',(-0.99969663250782,-7.42294062334711E-14,-0.0246301228686554));
#79291=DIRECTION('center_axis',(-0.0100960958892171,-0.987363722611223,
-0.158148500211366));
#79292=DIRECTION('ref_axis',(-0.995060113131406,0.0255405466605858,-0.0959325373957782));
#79293=DIRECTION('',(-0.763745915082458,0.,-0.645516984435622));
#79294=DIRECTION('center_axis',(-0.0438573087936048,0.987363722583665,-0.15228071378579));
#79295=DIRECTION('ref_axis',(-0.981183640694819,-0.0138816999014745,0.192577157629626));
#79296=DIRECTION('',(0.645516984435563,0.,-0.763745915082508));
#79297=DIRECTION('center_axis',(7.28649976714645E-14,-1.,-1.41667519678132E-14));
#79298=DIRECTION('ref_axis',(1.,7.28649976714645E-14,9.36660370336697E-32));
#79299=DIRECTION('center_axis',(-0.0438573087934124,-0.987363722583669,
-0.152280713785819));
#79300=DIRECTION('ref_axis',(-0.992418820392299,0.0255405479708334,0.120218822737984));
#79301=DIRECTION('',(-0.884657030427525,0.,-0.466242360275376));
#79302=DIRECTION('center_axis',(-0.0755677988336853,0.987363722655466,-0.139292451207418));
#79303=DIRECTION('ref_axis',(-0.916845716143399,-0.0138816972143508,0.399000289814364));
#79304=DIRECTION('',(0.466242360275311,0.,-0.884657030427559));
#79305=DIRECTION('center_axis',(1.36232043304539E-14,-1.,-5.89987236371338E-15));
#79306=DIRECTION('ref_axis',(1.,1.36232043304539E-14,-1.37390409739643E-31));
#79307=DIRECTION('center_axis',(-0.0755677988336818,-0.987363722655467,
-0.139292451207416));
#79308=DIRECTION('ref_axis',(-0.943373127031503,0.0255405454300251,0.330748883193792));
#79309=DIRECTION('',(-0.964202566256142,0.,-0.265166761161859));
#79310=DIRECTION('center_axis',(-0.103744835240006,0.987363722371026,-0.119791021811549));
#79311=DIRECTION('ref_axis',(-0.809637102056546,-0.013881708435082,0.586766615567383));
#79312=DIRECTION('',(0.265166763834479,0.,-0.964202565521141));
#79313=DIRECTION('',(-0.998663061429463,0.,-0.0516922599267325));
#79314=DIRECTION('center_axis',(-3.61092096369038E-14,-1.,2.60715685497971E-14));
#79315=DIRECTION('ref_axis',(1.,-3.61092096369038E-14,7.02924335103244E-31));
#79316=DIRECTION('center_axis',(-0.103744831159682,-0.987363722491922,-0.119791024348835));
#79317=DIRECTION('ref_axis',(-0.850216353240246,0.0255405521846307,0.525813496286432));
#79318=DIRECTION('',(0.0516922599267204,0.,-0.998663061429463));
#79319=DIRECTION('center_axis',(-0.127070861066288,0.9873637225882,-0.0946883075392291));
#79320=DIRECTION('ref_axis',(-0.664570762150803,-0.0138817002430436,0.747096379654368));
#79321=DIRECTION('center_axis',(1.97735865367437E-14,-1.,-2.21496282986849E-14));
#79322=DIRECTION('ref_axis',(-5.91610294980431E-32,2.21496282986849E-14,
-1.));
#79323=DIRECTION('center_axis',(-0.12707086106538,-0.987363722588226,-0.0946883075401802));
#79324=DIRECTION('ref_axis',(-0.717304409962752,0.0255405484483746,0.696291651416951));
#79325=DIRECTION('',(-0.986427181731827,0.,0.164199315286653));
#79326=DIRECTION('center_axis',(-0.144455203317022,0.987363722518218,-0.0651580669572451));
#79327=DIRECTION('ref_axis',(-0.488429827499476,-0.0138817019329595,0.872492751809593));
#79328=DIRECTION('',(-0.164199314821143,0.,-0.986427181809315));
#79329=DIRECTION('center_axis',(0.,-1.,0.));
#79330=DIRECTION('ref_axis',(0.,0.,-1.));
#79331=DIRECTION('center_axis',(-0.144455203317624,-0.987363722518189,-0.0651580669563533));
#79332=DIRECTION('ref_axis',(-0.550852108221544,0.0255405504288338,0.834211984540904));
#79333=DIRECTION('',(-0.928067064308992,0.,0.372413109523401));
#79334=DIRECTION('center_axis',(-0.155084978924344,0.987363722546342,-0.0325811097334957));
#79335=DIRECTION('ref_axis',(-0.289450459918619,-0.0138817012506714,0.95709233077237));
#79336=DIRECTION('',(-0.372413110516999,0.,-0.928067063910283));
#79337=DIRECTION('center_axis',(0.,-1.,0.));
#79338=DIRECTION('ref_axis',(0.,0.,-1.));
#79339=DIRECTION('center_axis',(-0.155084978924618,-0.987363722546322,-0.0325811097327927));
#79340=DIRECTION('ref_axis',(-0.358642575991151,0.0255405497773031,0.933125491562365));
#79341=DIRECTION('',(-0.826311561170158,0.,0.563213284534852));
#79342=DIRECTION('center_axis',(-0.158463154019127,0.987363722508337,0.00151930668065768));
#79343=DIRECTION('ref_axis',(-0.0769367093312951,-0.0138817032695296,0.996939336705904));
#79344=DIRECTION('',(-0.563213284534842,0.,-0.826311561170165));
#79345=DIRECTION('center_axis',(-2.33723120489955E-15,-1.,2.95996302335738E-14));
#79346=DIRECTION('ref_axis',(1.47644993132475E-32,-2.95996302335738E-14,
-1.));
#79347=DIRECTION('center_axis',(-0.158463154019238,-0.987363722508318,0.00151930668137857));
#79348=DIRECTION('ref_axis',(-0.149663313270426,0.0255405516534839,0.988407088644226));
#79349=DIRECTION('',(-0.685918647283643,0.,0.727678231987585));
#79350=DIRECTION('',(0.761098361889465,0.,-0.648636480263925));
#79351=DIRECTION('center_axis',(0.152615509638427,-0.987363721954313,0.0426777083069028));
#79352=DIRECTION('ref_axis',(-0.189172281343434,0.0131994979521353,0.981855193613158));
#79353=DIRECTION('center_axis',(-0.15456220255018,-0.987363721855482,-0.0349772255407453));
#79354=DIRECTION('ref_axis',(-0.187954824318923,-0.0053704878227672,0.982162991501812));
#79355=DIRECTION('',(0.469858074213424,0.,0.882741972547161));
#79356=DIRECTION('center_axis',(-2.77370063757617E-15,-1.,1.45844706016369E-14));
#79357=DIRECTION('ref_axis',(-3.54850712574642E-32,-1.45844706016369E-14,
-1.));
#79358=DIRECTION('center_axis',(0.158065641712032,0.987363722473557,0.0113195606506649));
#79359=DIRECTION('ref_axis',(-0.111146690329742,0.0064001555740922,0.993783402576926));
#79360=DIRECTION('',(0.882741973773695,0.,-0.469858071909084));
#79361=DIRECTION('center_axis',(0.139872998404444,-0.987363721993328,0.074487749387615));
#79362=DIRECTION('ref_axis',(-0.395819382646154,0.0131994966388906,0.918233515839025));
#79363=DIRECTION('center_axis',(-0.143429555557831,-0.987363721894278,-0.0673857795054785));
#79364=DIRECTION('ref_axis',(-0.394696555489278,-0.00537048497618321,0.918795835306201));
#79365=DIRECTION('',(0.26910962254562,0.,0.963109552986239));
#79366=DIRECTION('center_axis',(1.75322493495858E-14,-1.,-4.09416903538788E-14));
#79367=DIRECTION('ref_axis',(-3.88570892755786E-32,4.09416903538788E-14,
-1.));
#79368=DIRECTION('center_axis',(0.151936786191382,0.987363722382829,0.0450343504911405));
#79369=DIRECTION('ref_axis',(-0.322182197946835,0.00640016177914806,0.946656045908622));
#79370=DIRECTION('',(0.963109553688447,0.,-0.269109620032506));
#79371=DIRECTION('center_axis',(0.120590181104626,-0.987363721999251,0.102814827242669));
#79372=DIRECTION('ref_axis',(-0.583958407758862,0.0131994968264676,0.811676260150106));
#79373=DIRECTION('center_axis',(-0.125590297867976,-0.987363721894042,-0.0966434569382695));
#79374=DIRECTION('ref_axis',(-0.582982714666456,-0.00537049109331535,0.812466806845391));
#79375=DIRECTION('',(0.055777904388787,0.,0.998443200879247));
#79376=DIRECTION('center_axis',(3.45648110535867E-14,-1.,-4.82874413478829E-14));
#79377=DIRECTION('ref_axis',(-1.4878768112405E-31,4.82874413478829E-14,
-1.));
#79378=DIRECTION('center_axis',(0.138703532219836,0.987363722447253,0.076643393354187));
#79379=DIRECTION('ref_axis',(-0.518152824713272,0.00640015801778179,0.855264104367186));
#79380=DIRECTION('',(0.998443201024793,0.,-0.0557779017834631));
#79381=DIRECTION('center_axis',(0.095668705435196,-0.987363722100653,0.126334393891365));
#79382=DIRECTION('ref_axis',(-0.744792187180435,0.0131994908163985,0.667165924907119));
#79383=DIRECTION('center_axis',(-0.10187858278201,-0.987363721875608,-0.121382186066478));
#79384=DIRECTION('ref_axis',(-0.74400924970769,-0.00537048758462738,0.66814773382277));
#79385=DIRECTION('',(-0.160161927182448,0.,0.987090754227393));
#79386=DIRECTION('center_axis',(-4.41370775386657E-14,-1.,3.9728095186524E-14));
#79387=DIRECTION('ref_axis',(1.,-4.41370775386657E-14,6.86387583734043E-31));
#79388=DIRECTION('center_axis',(0.118984656681779,0.987363722441671,0.104668672870372));
#79389=DIRECTION('ref_axis',(-0.689895198735468,0.00640015752131604,0.723880965867629));
#79390=DIRECTION('',(0.987090754263963,0.,0.160161926957068));
#79391=DIRECTION('center_axis',(0.0662738593681364,-0.987363721996382,0.143946712535936));
#79392=DIRECTION('ref_axis',(-0.870800313020862,0.0131994960636845,0.491459650578187));
#79393=DIRECTION('center_axis',(-0.0734031336639462,-0.987363721877004,
-0.140445223092502));
#79394=DIRECTION('ref_axis',(-0.870246739706229,-0.00537049031533164,0.492586814545874));
#79395=DIRECTION('',(-0.368612762585142,0.,0.929583041615621));
#79396=DIRECTION('center_axis',(-9.03797007523297E-14,-1.,5.129443795653E-14));
#79397=DIRECTION('ref_axis',(1.,-9.03797007523297E-14,3.11692668887943E-32));
#79398=DIRECTION('center_axis',(0.0937021887534254,0.987363722499088,0.127799762580223));
#79399=DIRECTION('ref_axis',(-0.829378843888429,0.00640015560929818,0.558649954191773));
#79400=DIRECTION('',(0.929583040653769,0.,0.368612765010781));
#79401=DIRECTION('center_axis',(0.0337801242911014,-0.987363721967948,0.154828239492928));
#79402=DIRECTION('ref_axis',(-0.956090783052351,0.0131994970506592,0.292773270364546));
#79403=DIRECTION('center_axis',(-0.0414954358906202,-0.987363721863099,
-0.152941196375913));
#79404=DIRECTION('ref_axis',(-0.955792459128537,-0.00537049216965758,0.293993083059585));
#79405=DIRECTION('',(-0.559827676809204,0.,0.828609058771632));
#79406=DIRECTION('center_axis',(-5.67391208751526E-14,-1.,1.7523564833116E-14));
#79407=DIRECTION('ref_axis',(1.,-5.67391208751526E-14,2.39428158731835E-31));
#79408=DIRECTION('center_axis',(0.0640383186167767,0.987363722391337,0.144955073916917));
#79409=DIRECTION('ref_axis',(-0.930081653875991,0.00640016214797504,0.367297093709957));
#79410=DIRECTION('',(0.828609057310836,0.,0.559827678971349));
#79411=DIRECTION('center_axis',(-0.000293130042014416,-0.987363722005209,
0.158470169252131));
#79412=DIRECTION('ref_axis',(-0.996675510595413,0.0131994961838119,0.0803971385054558));
#79413=DIRECTION('center_axis',(-0.00764746068325912,-0.987363721888245,
-0.158285808094381));
#79414=DIRECTION('ref_axis',(-0.996646385061109,-0.00537049081886417,0.0816525625622804));
#79415=DIRECTION('',(-0.72486567039439,0.,0.688890237907094));
#79416=DIRECTION('center_axis',(7.39745501415128E-14,-1.,-6.14579978269866E-15));
#79417=DIRECTION('ref_axis',(1.,7.39745501415128E-14,1.07588057771275E-31));
#79418=DIRECTION('center_axis',(0.0313800724017027,0.987363722539182,0.155332451437662));
#79419=DIRECTION('ref_axis',(-0.987294879630409,0.00640015209656239,0.1587698293402));
#79420=DIRECTION('',(0.688890236015648,0.,0.724865672191962));
#79421=DIRECTION('center_axis',(-0.0343526804446576,-0.98736372198438,0.154702210247363));
#79422=DIRECTION('ref_axis',(-0.990656799336339,0.0131994978913179,-0.13573827457316));
#79423=DIRECTION('center_axis',(0.0265580987606778,-0.987363721867808,-0.156229152623856));
#79424=DIRECTION('ref_axis',(-0.990898233870037,-0.00537048704539685,-0.134505940322863));
#79425=DIRECTION('',(-0.856009751718059,0.,0.516959674407576));
#79426=DIRECTION('center_axis',(-5.8852985332957E-14,-1.,-7.9201817788065E-15));
#79427=DIRECTION('ref_axis',(1.,-5.8852985332957E-14,9.47619536544115E-32));
#79428=DIRECTION('center_axis',(-0.00274545651990735,0.987363722462837,
0.158446653586713));
#79429=DIRECTION('ref_axis',(-0.998343294030884,0.00640015748189069,-0.0571813365336253));
#79430=DIRECTION('',(0.516959673446092,0.,0.856009752298717));
#79431=DIRECTION('center_axis',(-0.0668059398504362,-0.987363721922213,
0.143700546389407));
#79432=DIRECTION('ref_axis',(-0.938316076633506,0.0131995016487155,-0.345526718919579));
#79433=DIRECTION('center_axis',(0.0595218347697124,-0.987363721868324,-0.146867395714565));
#79434=DIRECTION('ref_axis',(-0.9388167823789,-0.00537048681305594,-0.344375096363137));
#79435=DIRECTION('',(-0.947127767923488,0.,0.320856652149012));
#79436=DIRECTION('center_axis',(-2.7887215127273E-14,-1.,-1.01933322424768E-14));
#79437=DIRECTION('ref_axis',(1.,-2.7887215127273E-14,-1.63004429102285E-31));
#79438=DIRECTION('center_axis',(-0.0367426203518148,0.987363722519173,0.154152065515721));
#79439=DIRECTION('ref_axis',(-0.962710285131315,0.00640015325057946,-0.270458767542763));
#79440=DIRECTION('',(0.320856647098721,0.,0.947127769634365));
#79441=DIRECTION('center_axis',(-0.0961354192454943,-0.987363721975525,
0.125979608243283));
#79442=DIRECTION('ref_axis',(-0.842100737714532,0.0131994961709445,-0.539158715817035));
#79443=DIRECTION('center_axis',(0.0897023972641109,-0.987363721874223,-0.130638281723827));
#79444=DIRECTION('ref_axis',(-0.842837302056352,-0.00537048843902798,-0.538141654321886));
#79445=DIRECTION('',(-0.993959142840391,0.,0.109750728307355));
#79446=DIRECTION('center_axis',(5.00879248534494E-14,-1.,3.18998894380968E-14));
#79447=DIRECTION('ref_axis',(1.,5.00879248534494E-14,-3.90471029974449E-31));
#79448=DIRECTION('center_axis',(-0.069021730874996,0.987363722442924,0.142649501473623));
#79449=DIRECTION('ref_axis',(-0.88206201520754,0.0064001582682407,-0.471089842070655));
#79450=DIRECTION('',(0.109750725713721,0.,0.993959143126774));
#79451=DIRECTION('center_axis',(-0.120969721135708,-0.987363721902305,0.102367999099214));
#79452=DIRECTION('ref_axis',(-0.706509702519059,0.0131994996103268,-0.707580252308152));
#79453=DIRECTION('center_axis',(0.115688572607768,-0.98736372188139,-0.108300668883003));
#79454=DIRECTION('ref_axis',(-0.707447686309035,-0.00537048650344094,-0.70674530703126));
#79455=DIRECTION('',(-0.994314092728476,0.,-0.10648701799538));
#79456=DIRECTION('center_axis',(6.30890455641618E-14,-1.,6.28822664835682E-14));
#79457=DIRECTION('ref_axis',(1.,6.30890455641618E-14,-1.84569166322532E-31));
#79458=DIRECTION('center_axis',(-0.0980734667158721,0.987363722423218,0.124476804139958));
#79459=DIRECTION('ref_axis',(-0.760169502183937,0.00640015973960987,-0.649693286024054));
#79460=DIRECTION('',(-0.106487020589929,0.,0.99431409245061));
#79461=DIRECTION('center_axis',(-0.140147609432002,-0.987363721938444,0.0739697787637499));
#79462=DIRECTION('ref_axis',(-0.537883061423971,0.0131994988325246,-0.842916120064));
#79463=DIRECTION('center_axis',(0.136265278239864,-0.987363721884388,-0.0808990398757652));
#79464=DIRECTION('ref_axis',(-0.538978603059603,-0.00537048203791794,-0.842302334893237));
#79465=DIRECTION('',(-0.948176020641203,0.,-0.317745548955471));
#79466=DIRECTION('center_axis',(4.00801918488179E-14,-1.,6.24786615949557E-14));
#79467=DIRECTION('ref_axis',(1.14695319878951E-30,-6.24786615949557E-14,
-1.));
#79468=DIRECTION('center_axis',(-0.122539399999212,0.987363722490082,0.100483704939462));
#79469=DIRECTION('ref_axis',(-0.602732310836473,0.00640015416421709,-0.797917789938537));
#79470=DIRECTION('',(-0.317745554014208,0.,0.948176018945957));
#79471=DIRECTION('center_axis',(-0.152772350424458,-0.987363722024416,0.0421128172398611));
#79472=DIRECTION('ref_axis',(-0.344105606166508,0.0131994945560806,-0.93883816770956));
#79473=DIRECTION('center_axis',(0.150470376064837,-0.987363721904127,-0.0497146517088959));
#79474=DIRECTION('ref_axis',(-0.345307478360847,-0.00537048903212129,-0.938474242180162));
#79475=DIRECTION('',(-0.857702290213478,0.,-0.51414665355573));
#79476=DIRECTION('center_axis',(-2.05696590877686E-14,-1.,-5.57072013831238E-14));
#79477=DIRECTION('ref_axis',(4.64417736689475E-31,5.57072013831238E-14,
-1.));
#79478=DIRECTION('center_axis',(-0.141275521246512,0.987363722413862,0.0717921079058763));
#79479=DIRECTION('ref_axis',(-0.41711202824178,0.00640015907852063,-0.908832544454586));
#79480=DIRECTION('',(-0.514146654526059,0.,0.857702289631817));
#79481=DIRECTION('center_axis',(-0.158253628125781,-0.9873637220816,0.00828670635390313));
#79482=DIRECTION('ref_axis',(-0.134238153215872,0.0131994915295978,-0.990861186869559));
#79483=DIRECTION('center_axis',(0.15763964250658,-0.987363721893091,-0.0162056718410967));
#79484=DIRECTION('ref_axis',(-0.135490161169236,-0.00537048504490039,-0.990764136470794));
#79485=DIRECTION('',(-0.727123357294462,0.,-0.686506826824636));
#79486=DIRECTION('center_axis',(2.02833757196093E-15,-1.,1.47066666659893E-14));
#79487=DIRECTION('ref_axis',(3.92305557744363E-32,-1.47066666659893E-14,
-1.));
#79488=DIRECTION('center_axis',(-0.153405759751366,0.987363722449018,0.0397435839693078));
#79489=DIRECTION('ref_axis',(-0.211988047664614,0.00640015578210116,-0.977251301177599));
#79490=DIRECTION('',(-0.686506828721979,0.,0.727123355503103));
#79491=DIRECTION('center_axis',(-0.156335142838038,-0.987363722080833,-0.0259268862861391));
#79492=DIRECTION('ref_axis',(0.081906124669614,0.0131994936921692,-0.996552637901218));
#79493=DIRECTION('center_axis',(0.157437855226706,-0.987363721871608,0.0180610761988493));
#79494=DIRECTION('ref_axis',(0.0806625276050987,-0.00537048997581514,-0.996727000977588));
#79495=DIRECTION('',(-0.562544940564676,0.,-0.826766708234605));
#79496=DIRECTION('center_axis',(-1.18058243820127E-15,-1.,1.47988655758512E-14));
#79497=DIRECTION('ref_axis',(4.8499339749902E-33,-1.47988655758512E-14,
-1.));
#79498=DIRECTION('center_axis',(-0.158362913987084,0.987363722452981,0.00583669917957237));
#79499=DIRECTION('ref_axis',(0.00304825895565919,0.00640015786115479,-0.999974872732656));
#79500=DIRECTION('',(-0.826766709702496,0.,0.562544938407333));
#79501=DIRECTION('center_axis',(-0.14710660094675,-0.987363722108276,-0.0589281615391628));
#79502=DIRECTION('ref_axis',(0.294220564215013,0.0131994904617581,-0.95564639540185));
#79503=DIRECTION('center_axis',(0.149874448064302,-0.987363721871317,0.0514833036026376));
#79504=DIRECTION('ref_axis',(0.293043523486218,-0.00537049048421785,-0.956084018888895));
#79505=DIRECTION('',(-0.371662549274472,0.,-0.928367895538617));
#79506=DIRECTION('center_axis',(-1.73371989163566E-14,-1.,5.67963440396674E-14));
#79507=DIRECTION('ref_axis',(-2.26462988917793E-31,-5.67963440396674E-14,
-1.));
#79508=DIRECTION('center_axis',(-0.155915195724226,0.987363722398576,-0.0283431020444865));
#79509=DIRECTION('ref_axis',(0.217942029486368,0.00640016067289282,-0.97594073064235));
#79510=DIRECTION('',(-0.928367895516495,0.,0.371662549329729));
#79511=DIRECTION('center_axis',(-0.130999513940044,-0.987363721968695,-0.0891740314643088));
#79512=DIRECTION('ref_axis',(0.492777578093553,0.0131994981102028,-0.870055188926479));
#79513=DIRECTION('center_axis',(0.135303080594625,-0.98736372187151,0.0824982249120781));
#79514=DIRECTION('ref_axis',(0.491722131566428,-0.00537048598229784,-0.870735610393926));
#79515=DIRECTION('',(-0.163401630169058,0.,-0.986559631881466));
#79516=DIRECTION('center_axis',(-2.91413998726486E-14,-1.,5.17414917161749E-14));
#79517=DIRECTION('ref_axis',(3.23235934945798E-31,-5.17414917161749E-14,
-1.));
#79518=DIRECTION('center_axis',(-0.146177052628152,0.987363722526871,-0.061197620238264));
#79519=DIRECTION('ref_axis',(0.422645075236517,0.00640015395770225,-0.90627268435479));
#79520=DIRECTION('',(-0.986559631844411,0.,0.163401630392784));
#79521=DIRECTION('center_axis',(-0.108767037567511,-0.987363721988378,-0.115250214924069));
#79522=DIRECTION('ref_axis',(0.668292860223129,0.0131994973818557,-0.743781168250216));
#79523=DIRECTION('center_axis',(0.114405086728576,-0.987363721852231,0.109655628677866));
#79524=DIRECTION('ref_axis',(0.667408358630309,-0.00537049099330845,-0.744672572784098));
#79525=DIRECTION('',(0.0524997650266615,0.,-0.998620936427905));
#79526=DIRECTION('center_axis',(6.92702175257193E-14,-1.,-7.74677135725862E-14));
#79527=DIRECTION('ref_axis',(1.15000252023255E-30,7.74677135725862E-14,
-1.));
#79528=DIRECTION('center_axis',(-0.129603834006118,0.98736372253409,-0.0911906005821871));
#79529=DIRECTION('ref_axis',(0.60758570602415,0.00640015223266166,-0.794228334854992));
#79530=DIRECTION('',(-0.998620936282989,0.,-0.0524997677831598));
#79531=DIRECTION('center_axis',(-0.0814487376935129,-0.987363722005638,
-0.135937425293063));
#79532=DIRECTION('ref_axis',(0.812559508457631,0.0131994947613375,-0.582728769285624));
#79533=DIRECTION('center_axis',(0.088157642749355,-0.987363721858716,0.131685651390657));
#79534=DIRECTION('ref_axis',(0.811887313110997,-0.0053704882952763,-0.583789472896588));
#79535=DIRECTION('',(0.265946332280708,0.,-0.963987836202532));
#79536=DIRECTION('center_axis',(1.20434266953032E-13,-1.,-8.68078747800019E-14));
#79537=DIRECTION('ref_axis',(1.,1.20434266953032E-13,-1.16030839842935E-30));
#79538=DIRECTION('center_axis',(-0.106970488036622,0.987363722454154,-0.116919606014916));
#79539=DIRECTION('ref_axis',(0.764116305563639,0.00640015641498283,-0.645046749910144));
#79540=DIRECTION('',(-0.96398783550857,0.,-0.265946334796144));
#79541=DIRECTION('center_axis',(-0.0503219807087614,-0.987363721983654,
-0.150268355844243));
#79542=DIRECTION('ref_axis',(0.918831778987382,0.0131994974814984,-0.394428618623343));
#79543=DIRECTION('center_axis',(0.0577880427271561,-0.987363721860299,0.147558201642413));
#79544=DIRECTION('ref_axis',(0.918403318689976,-0.00537048931959254,-0.395609026772275));
#79545=DIRECTION('',(0.466957545975081,0.,-0.884279735296999));
#79546=DIRECTION('center_axis',(-2.72559415313569E-14,-1.,1.17777094957016E-14));
#79547=DIRECTION('ref_axis',(1.,-2.72559415313569E-14,2.44775647909051E-31));
#79548=DIRECTION('center_axis',(-0.0793353163545417,0.987363722508187,-0.137181584236734));
#79549=DIRECTION('ref_axis',(0.884917674707086,0.00640015430844893,-0.465703496890276));
#79550=DIRECTION('',(-0.884279734078536,-3.74026243169963E-15,-0.466957548282489));
#79551=DIRECTION('center_axis',(-0.0168422275713211,-0.987363722000351,
-0.15757290327988));
#79552=DIRECTION('ref_axis',(0.982140496261105,0.013199496140424,-0.187685425394804));
#79553=DIRECTION('center_axis',(0.0247163358735517,-0.987363721874109,0.156531094252524));
#79554=DIRECTION('ref_axis',(0.981975806292579,-0.00537049216555821,-0.188930340787122));
#79555=DIRECTION('',(0.646134340612186,0.,-0.763223698453904));
#79556=DIRECTION('center_axis',(-1.45752860926422E-14,-1.,2.82156572357862E-15));
#79557=DIRECTION('ref_axis',(1.,-1.45752860926422E-14,1.01827328463709E-32));
#79558=DIRECTION('center_axis',(-0.0479905205829132,0.987363722406498,-0.151029101863734));
#79559=DIRECTION('ref_axis',(0.964341276427462,0.00640015954765453,-0.264584467677182));
#79560=DIRECTION('',(-0.763223696767415,0.,-0.646134342604292));
#79561=DIRECTION('',(0.795098614022376,0.,-0.606480167837084));
#79562=DIRECTION('',(-0.606480167148637,0.,-0.795098614547505));
#79563=DIRECTION('center_axis',(0.050877555165117,-0.987363721972948,-0.150081161083423));
#79564=DIRECTION('ref_axis',(0.970173637559078,0.0131994982843853,0.24205141237024));
#79565=DIRECTION('center_axis',(-0.0432937565932917,-0.987363721878708,
0.152441895021893));
#79566=DIRECTION('ref_axis',(0.970546895646585,-0.00537048691830518,0.240852405470729));
#79567=DIRECTION('',(0.906884959783822,0.,-0.421378297635148));
#79568=DIRECTION('center_axis',(1.4412916073023E-14,-1.,3.55922008307402E-15));
#79569=DIRECTION('ref_axis',(1.,1.4412916073023E-14,-5.23604782595645E-32));
#79570=DIRECTION('center_axis',(0.0198604640484954,0.987363722513242,-0.157220995520868));
#79571=DIRECTION('ref_axis',(0.98630857283147,0.00640015256345255,0.164786034621606));
#79572=DIRECTION('',(-0.421378297633106,0.,-0.906884959784771));
#79573=DIRECTION('center_axis',(0.0819510773744515,-0.987363722025524,-0.135635177387983));
#79574=DIRECTION('ref_axis',(0.895457618754654,0.0131994961189737,0.444951038111443));
#79575=DIRECTION('center_axis',(-0.0750520708927661,-0.987363721878045,
0.139571011939592));
#79576=DIRECTION('ref_axis',(0.896079901408113,-0.00537048362115263,0.443860302570642));
#79577=DIRECTION('',(0.976266370926292,0.,-0.21657325088387));
#79578=DIRECTION('center_axis',(-5.32432919859296E-14,-1.,-2.62974336310652E-14));
#79579=DIRECTION('ref_axis',(1.,-5.32432919859296E-14,3.34469867477409E-31));
#79580=DIRECTION('center_axis',(0.0531939969984103,0.987363722423736,-0.14927584642157));
#79581=DIRECTION('ref_axis',(0.927825100680265,0.00640016009637148,0.37296061521077));
#79582=DIRECTION('',(-0.216573248336411,0.,-0.976266371491416));
#79583=DIRECTION('center_axis',(0.109192663323288,-0.987363721947468,-0.114847041139118));
#79584=DIRECTION('ref_axis',(0.778870996263127,0.013199499495899,0.627045249079476));
#79585=DIRECTION('center_axis',(-0.103301042454407,-0.987363721854847,0.120173938076346));
#79586=DIRECTION('ref_axis',(0.779713205798433,-0.00537049049308058,0.626113787210754));
#79587=DIRECTION('',(0.999998652775296,0.,-0.00164147725930846));
#79588=DIRECTION('center_axis',(-5.79316531842594E-14,-1.,-4.64104352224614E-14));
#79589=DIRECTION('ref_axis',(1.,-5.79316531842594E-14,3.76431018964206E-31));
#79590=DIRECTION('center_axis',(0.0840402488511352,0.987363722495072,-0.134350720406385));
#79591=DIRECTION('ref_axis',(0.825957557940463,0.00640015555580381,0.563695973455451));
#79592=DIRECTION('',(-0.00164147464991938,0.,-0.999998652779579));
#79593=DIRECTION('center_axis',(0.131328515370216,-0.987363722033873,-0.0886887899459243));
#79594=DIRECTION('ref_axis',(0.625865231966009,0.0131994945570568,0.779819520632545));
#79595=DIRECTION('center_axis',(-0.126719763793783,-0.987363721877416,0.0951576701292319));
#79596=DIRECTION('ref_axis',(0.626887989061991,-0.00537048743991487,0.779090884964309));
#79597=DIRECTION('',(0.976972108935026,0.,0.213367050790528));
#79598=DIRECTION('center_axis',(-6.52405203017506E-14,-1.,-8.08905692541282E-14));
#79599=DIRECTION('ref_axis',(-3.50266061336804E-31,8.08905692541282E-14,
-1.));
#79600=DIRECTION('center_axis',(0.110956869526365,0.987363722511827,-0.113143504331872));
#79601=DIRECTION('ref_axis',(0.685469157120961,0.00640015346900311,0.728073535208809));
#79602=DIRECTION('',(0.213367053339806,0.,-0.976972108378273));
#79603=DIRECTION('center_axis',(0.147323596858144,-0.987363721972992,-0.0583835451169203));
#79604=DIRECTION('ref_axis',(0.443594705445403,0.0131994963886616,0.896130297778114));
#79605=DIRECTION('center_axis',(-0.14421321305761,-0.987363721863186,0.0656919319861826));
#79606=DIRECTION('ref_axis',(0.444750185379517,-0.00537048885387717,0.895638560164956));
#79607=DIRECTION('',(0.908263435453809,0.,0.418398771290792));
#79608=DIRECTION('center_axis',(3.97081302317317E-14,-1.,7.97350081058221E-14));
#79609=DIRECTION('ref_axis',(-1.76608788499542E-31,-7.97350081058221E-14,
-1.));
#79610=DIRECTION('center_axis',(0.132685266333161,0.987363722430977,-0.0866458292437882));
#79611=DIRECTION('ref_axis',(0.51292898068897,0.00640015831316843,0.858407187028942));
#79612=DIRECTION('',(0.418398773660791,0.,-0.90826343436205));
#79613=DIRECTION('center_axis',(0.156429989965125,-0.987363721958195,-0.0253483490659727));
#79614=DIRECTION('ref_axis',(0.240582182111676,0.013199499044569,0.970539018728952));
#79615=DIRECTION('center_axis',(-0.154963411925007,-0.987363721875536,0.0331545123422059));
#79616=DIRECTION('ref_axis',(0.241816356527403,-0.00537048956491149,0.970307171754205));
#79617=DIRECTION('',(0.797085373092917,0.,0.603866630971877));
#79618=DIRECTION('center_axis',(3.24586596311348E-14,-1.,1.29610383251507E-13));
#79619=DIRECTION('ref_axis',(8.61439714851782E-31,-1.29610383251507E-13,
-1.));
#79620=DIRECTION('center_axis',(0.148209450383187,0.987363722419937,-0.0560966885489541));
#79621=DIRECTION('ref_axis',(0.316404815531485,0.00640015906571002,0.948602672709929));
#79622=DIRECTION('',(0.603866633051783,0.,-0.797085371517194));
#79623=DIRECTION('center_axis',(0.158221889636225,-0.987363721921636,0.00887210645764376));
#79624=DIRECTION('ref_axis',(0.0263203038047064,0.0131995003924017,0.99956641339984));
#79625=DIRECTION('center_axis',(-0.158467693619661,-0.987363721870234,-0.000933173844636907));
#79626=DIRECTION('ref_axis',(0.0275754654179984,-0.00537048891585742,0.999605297883012));
#79627=DIRECTION('',(0.648636483669163,0.,0.761098358987394));
#79628=DIRECTION('center_axis',(4.26377006545449E-16,-1.,1.48397574152667E-14));
#79629=DIRECTION('ref_axis',(0.0287202210588392,1.48458814994488E-14,0.999587489368655));
#79630=DIRECTION('center_axis',(0.156803525494413,0.987363722442391,-0.0229245282880083));
#79631=DIRECTION('ref_axis',(0.105085911959256,0.00640015912441032,0.994442551920861));
#79632=DIRECTION('center_axis',(-0.160735572208841,-0.986495109500315,0.0314876921774008));
#79633=DIRECTION('ref_axis',(0.0338459003609357,0.026374638220109,0.999078992616458));
#79634=DIRECTION('center_axis',(-0.150208729944758,-0.986495109192071,0.0653049537822887));
#79635=DIRECTION('ref_axis',(0.247827073369561,0.0263746665288115,0.968445206849914));
#79636=DIRECTION('center_axis',(-0.132658295477633,-0.986495109084167,0.0960686025399893));
#79637=DIRECTION('ref_axis',(0.450220106754815,0.0263746728872703,0.892528000739345));
#79638=DIRECTION('center_axis',(-0.108904912105237,-0.986495109156878,0.12234018035343));
#79639=DIRECTION('ref_axis',(0.631561347853854,0.026374667624227,0.774877177883525));
#79640=DIRECTION('center_axis',(-0.0800592540170044,-0.986495109155527,
0.142891271456541));
#79641=DIRECTION('ref_axis',(0.783371482987673,0.0263746667580228,0.620993958581802));
#79642=DIRECTION('center_axis',(-0.0474701058253641,-0.986495109083009,
0.156760928831869));
#79643=DIRECTION('ref_axis',(0.898552039413217,0.0263746743925295,0.438073748376956));
#79644=DIRECTION('center_axis',(-0.0126613186995483,-0.986495109111999,
0.163300614533115));
#79645=DIRECTION('ref_axis',(0.971717298236084,0.0263746712037161,0.234669701980597));
#79646=DIRECTION('center_axis',(0.0227394998600456,-0.986495109150332,0.162204546078675));
#79647=DIRECTION('ref_axis',(0.999446136981731,0.0263746700344972,0.0202927586312497));
#79648=DIRECTION('center_axis',(0.0570770466086315,-0.986495109126712,0.153523973435789));
#79649=DIRECTION('ref_axis',(0.980441984811844,0.0263746709087561,-0.195033051436586));
#79650=DIRECTION('center_axis',(0.0887457320211409,-0.986495109141813,0.137664791022663));
#79651=DIRECTION('ref_axis',(0.915593456668965,0.0263746702572848,-0.401239328672796));
#79652=DIRECTION('center_axis',(0.116264768310826,-0.986495109125943,0.115368554295456));
#79653=DIRECTION('ref_axis',(0.807932792175151,0.0263746713744888,-0.588684108871601));
#79654=DIRECTION('center_axis',(0.138347388597019,-0.986495109217853,0.0876778167933158));
#79655=DIRECTION('ref_axis',(0.662494092566996,0.0263746671072638,-0.748602667807706));
#79656=DIRECTION('center_axis',(0.153961044274636,-0.986495109084597,0.0558873563342683));
#79657=DIRECTION('ref_axis',(0.486077907132691,0.0263746711415175,-0.87351739817801));
#79658=DIRECTION('center_axis',(0.162375650580194,-0.98649510910325,0.0214836638873636));
#79659=DIRECTION('ref_axis',(0.2869332520124,0.0263746740827948,-0.95758742966719));
#79660=DIRECTION('center_axis',(0.163197750937941,-0.986495109091353,-0.0139245763898883));
#79661=DIRECTION('ref_axis',(0.0743719212258115,0.0263746732350422,-0.996881735184734));
#79662=DIRECTION('center_axis',(0.156388905548954,-0.986495109083077,-0.0486817211730238));
#79663=DIRECTION('ref_axis',(-0.141666957958585,0.0263746746431137,-0.989562958866302));
#79664=DIRECTION('center_axis',(0.142267491681255,-0.986495109182172,-0.0811625552233208));
#79665=DIRECTION('ref_axis',(-0.35108164507487,0.0263746682502834,-0.935973319794005));
#79666=DIRECTION('center_axis',(0.121493807280624,-0.986495109226014,-0.109848323908989));
#79667=DIRECTION('ref_axis',(-0.544080148475943,0.0263746667314525,-0.838618607585833));
#79668=DIRECTION('center_axis',(0.0950392032811796,-0.986495109159665,-0.133397711538612));
#79669=DIRECTION('ref_axis',(-0.71163807058147,0.0263746711143374,-0.702051018959942));
#79670=DIRECTION('center_axis',(0.0641406724996807,-0.986495109097894,-0.150709567902049));
#79671=DIRECTION('ref_axis',(-0.84592058478901,0.0263746736888512,-0.532656306466023));
#79672=DIRECTION('center_axis',(0.0302430011311341,-0.986495109169532,-0.16097440935495));
#79673=DIRECTION('ref_axis',(-0.940648791899366,0.0263746696350386,-0.338355178916926));
#79674=DIRECTION('center_axis',(-0.00506880138706661,-0.986495109150829,
-0.163712268550626));
#79675=DIRECTION('ref_axis',(-0.991393307574693,0.0263746680911805,-0.12823293874504));
#79676=DIRECTION('center_axis',(-0.0401436004710594,-0.986495109078913,
-0.15879512305044));
#79677=DIRECTION('ref_axis',(-0.995781373991902,0.0263746744667969,0.0878853330059665));
#79678=DIRECTION('center_axis',(-0.0733413264079324,-0.986495109008859,
-0.1464528925707));
#79679=DIRECTION('ref_axis',(-0.953607809106848,0.0263746777387383,0.299894185980015));
#79680=DIRECTION('center_axis',(-0.103109683648256,-0.986495109146731,-0.127262691970334));
#79681=DIRECTION('ref_axis',(-0.8668446051852,0.0263746710119367,0.497880314122105));
#79682=DIRECTION('center_axis',(-0.128056752441364,-0.986495109121959,-0.102121828384661));
#79683=DIRECTION('ref_axis',(-0.739548710327857,0.0263746693552898,0.672586114834972));
#79684=DIRECTION('center_axis',(-0.147016031601871,-0.986495109109258,-0.0722058595652089));
#79685=DIRECTION('ref_axis',(-0.577672341080192,0.0263746706390861,0.815842535725866));
#79686=DIRECTION('center_axis',(-0.159101004976774,-0.986495109093066,-0.0389136216618427));
#79687=DIRECTION('ref_axis',(-0.388784647961224,0.0263746737791896,0.920951070411837));
#79688=DIRECTION('center_axis',(-0.163746589679106,-0.986495109177042,-0.00380183353643957));
#79689=DIRECTION('ref_axis',(-0.181717824059167,0.0263746702342777,0.98299695278736));
#79690=DIRECTION('center_axis',(0.163668143187915,0.98649510955974,0.00633543369766243));
#79691=DIRECTION('ref_axis',(-0.0784216555462039,0.00660859149372386,0.996898375191705));
#79692=DIRECTION('center_axis',(0.158479742656236,0.986495109491893,0.0413711266004603));
#79693=DIRECTION('ref_axis',(-0.290891882249892,0.00660859243598289,0.956733107688414));
#79694=DIRECTION('center_axis',(0.14588100613144,0.986495109481366,0.074472350704314));
#79695=DIRECTION('ref_axis',(-0.489760328703683,0.00660859467570009,0.871832063475801));
#79696=DIRECTION('center_axis',(0.126461037299186,0.986495109425709,0.104091330687878));
#79697=DIRECTION('ref_axis',(-0.665728126384466,0.00660859742232058,0.746165121257177));
#79698=DIRECTION('center_axis',(0.101127890716206,0.98649510939482,0.128843117237175));
#79699=DIRECTION('ref_axis',(-0.810567217647311,0.00660859914361863,0.585608326522818));
#79700=DIRECTION('center_axis',(0.0710661119071067,0.986495109452163,0.147570345142143));
#79701=DIRECTION('ref_axis',(-0.917505087153752,0.0066085959530382,0.397669135722796));
#79702=DIRECTION('center_axis',(0.0376813607638582,0.986495109493467,0.159397346265416));
#79703=DIRECTION('ref_axis',(-0.981541437170374,0.00660859291907783,0.19113538033851));
#79704=DIRECTION('center_axis',(0.00253467983119023,0.986495109399991,0.163771104069227));
#79705=DIRECTION('ref_axis',(-0.999682000665267,0.00660859883572792,-0.0243356521859752));
#79706=DIRECTION('center_axis',(-0.0327305250144651,0.986495109396022,0.160487108111548));
#79707=DIRECTION('ref_axis',(-0.971078545498027,0.0066085995295211,-0.238668776520294));
#79708=DIRECTION('center_axis',(-0.0664652930897966,0.986495109464134,0.149698910543241));
#79709=DIRECTION('ref_axis',(-0.89706853564046,0.00660859391791874,-0.441842017977364));
#79710=DIRECTION('center_axis',(-0.0970922137686021,0.986495109509118,0.131910958377629));
#79711=DIRECTION('ref_axis',(-0.781112598468359,0.00660859175496055,-0.624355215425501));
#79712=DIRECTION('center_axis',(-0.123179205476025,0.986495109422879,0.107955001843537));
#79713=DIRECTION('ref_axis',(-0.628632706297494,0.00660859671899613,-0.777674255085312));
#79714=DIRECTION('center_axis',(-0.143506479071122,0.986495109469043,0.0789511840207048));
#79715=DIRECTION('ref_axis',(-0.446758644581469,0.006608594994134,-0.894630113490448));
#79716=DIRECTION('center_axis',(-0.157123548631729,0.98649510949616,0.0462556959252781));
#79717=DIRECTION('ref_axis',(-0.2439946456178,0.00660859273657448,-0.969754061302084));
#79718=DIRECTION('center_axis',(-0.163393694811817,0.98649510941163,0.0113973506868681));
#79719=DIRECTION('ref_axis',(-0.0298217307358154,0.00660859815402411,-0.999533386539119));
#79720=DIRECTION('center_axis',(-0.162023734603462,0.98649510942972,-0.0239939262396024));
#79721=DIRECTION('ref_axis',(0.185745616396384,0.0066085993854543,-0.982575642077336));
#79722=DIRECTION('center_axis',(-0.153077721679699,0.986495109522431,-0.0582632818649898));
#79723=DIRECTION('ref_axis',(0.392627706962826,0.00660859212269046,-0.919673752063888));
#79724=DIRECTION('center_axis',(-0.136973968951122,0.986495109442921,-0.089808300701981));
#79725=DIRECTION('ref_axis',(0.581150960023441,0.00660859623492829,-0.813768940252475));
#79726=DIRECTION('center_axis',(-0.114465467592361,0.986495109370403,-0.117153983786893));
#79727=DIRECTION('ref_axis',(0.742500239708373,0.00660860100223232,-0.669813198157368));
#79728=DIRECTION('center_axis',(-0.0866046785300646,0.986495109478629,-0.139021684033288));
#79729=DIRECTION('ref_axis',(0.869131036238581,0.00660859401759509,-0.494537731959819));
#79730=DIRECTION('center_axis',(-0.0546943599861106,0.986495109488404,-0.154388878942662));
#79731=DIRECTION('ref_axis',(0.955122228521663,0.00660859705495355,-0.296138236350488));
#79732=DIRECTION('center_axis',(-0.020226587168411,0.986495109469708,-0.162537023978744));
#79733=DIRECTION('ref_axis',(0.996452968940974,0.00660859375025051,-0.0838916394962136));
#79734=DIRECTION('center_axis',(0.0151869523181353,0.986495109436306,-0.163085117461823));
#79735=DIRECTION('ref_axis',(0.99119067534219,0.00660859577406016,0.132277630673472));
#79736=DIRECTION('center_axis',(0.0498903736231824,0.986495109518188,-0.156007530319653));
#79737=DIRECTION('ref_axis',(0.939581407019408,0.0066085913316494,0.342261750863341));
#79738=DIRECTION('center_axis',(0.0822609667229837,0.986495109465284,-0.14163520874019));
#79739=DIRECTION('ref_axis',(0.844038356618601,0.00660859756009447,0.536242089913558));
#79740=DIRECTION('center_axis',(0.110785139185442,0.98649510953755,-0.1206401748762));
#79741=DIRECTION('ref_axis',(0.709029009947545,0.00660859048807991,0.705148345800062));
#79742=DIRECTION('center_axis',(0.134129115877841,0.986495109511418,-0.0940041445037607));
#79743=DIRECTION('ref_axis',(0.540866255489018,0.00660859038340004,0.841082647666942));
#79744=DIRECTION('center_axis',(0.151201360818737,0.986495109387669,-0.0629725943627227));
#79745=DIRECTION('ref_axis',(0.347413197746676,0.00660860031970175,0.93768885907493));
#79746=DIRECTION('center_axis',(0.161203604303846,0.986495109502081,-0.0289964978562238));
#79747=DIRECTION('ref_axis',(0.137715482655985,0.00660859113228861,0.990449782856292));
#79748=DIRECTION('center_axis',(0.156429986790059,0.987363722430518,-0.0253483502621767));
#79749=DIRECTION('ref_axis',(0.105566785065707,0.00880314965778774,0.994373249060429));
#79750=DIRECTION('',(-0.60378640757203,0.,0.797146143458816));
#79751=DIRECTION('',(-0.797146142953525,0.,-0.603786408239137));
#79752=DIRECTION('center_axis',(7.21593417373741E-15,-1.,2.88015808780585E-14));
#79753=DIRECTION('ref_axis',(3.73148717172395E-32,-2.88015808780585E-14,
-1.));
#79754=DIRECTION('center_axis',(-0.154431767592391,-0.987363722333479,0.0355486846179549));
#79755=DIRECTION('ref_axis',(0.170524506140172,0.00880346257917287,0.985314108217409));
#79756=DIRECTION('center_axis',(0.156803524252501,-0.987363722273954,-0.0229245440372688));
#79757=DIRECTION('ref_axis',(0.240230849202258,0.015616035248029,0.970590170223609));
#79758=DIRECTION('center_axis',(0.147323595591869,0.987363722485576,-0.0583835396435483));
#79759=DIRECTION('ref_axis',(0.316859547487647,0.00880314606301053,0.9484316168208));
#79760=DIRECTION('',(-0.418307358246727,0.,0.908305540023094));
#79761=DIRECTION('',(-0.908305540399124,0.,-0.418307357430222));
#79762=DIRECTION('center_axis',(1.98580772700459E-14,-1.,3.98655051185617E-14));
#79763=DIRECTION('ref_axis',(4.90281768277353E-31,-3.98655051185617E-14,
-1.));
#79764=DIRECTION('center_axis',(-0.143179321891756,-0.987363722363956,0.0679158416145226));
#79765=DIRECTION('ref_axis',(0.378351146654384,0.00880346294309428,0.925620283304943));
#79766=DIRECTION('center_axis',(0.148209449214943,-0.987363722079989,-0.0560966976189729));
#79767=DIRECTION('ref_axis',(0.443262580240077,0.0156160420103856,0.896255780562022));
#79768=DIRECTION('center_axis',(0.131328515651695,0.987363722452776,-0.0886887848655015));
#79769=DIRECTION('ref_axis',(0.513336310721137,0.00880314782965812,0.858142375531882));
#79770=DIRECTION('',(-0.213268723577629,0.,0.976993578046227));
#79771=DIRECTION('',(-0.976993578237944,0.,-0.213268722699364));
#79772=DIRECTION('center_axis',(-1.8642474407541E-14,-1.,-2.31097147398058E-14));
#79773=DIRECTION('ref_axis',(-3.71574464986128E-31,2.31097147398058E-14,
-1.));
#79774=DIRECTION('center_axis',(-0.125231968813796,-0.987363722355263,0.0971073311536195));
#79775=DIRECTION('ref_axis',(0.568486505809193,0.00880346607357507,0.822645483606363));
#79776=DIRECTION('center_axis',(0.13268526417301,-0.98736372206775,-0.0866458366908468));
#79777=DIRECTION('ref_axis',(0.625567847037377,0.0156160442834527,0.780013466495264));
#79778=DIRECTION('center_axis',(0.109192661699068,0.987363722509184,-0.114847037854183));
#79779=DIRECTION('ref_axis',(0.685810037120877,0.00880314627001295,0.727727351141903));
#79780=DIRECTION('',(0.00174211876870894,0.,0.999998482509946));
#79781=DIRECTION('',(-0.999998482503372,0.,0.00174212254246539));
#79782=DIRECTION('center_axis',(5.7936323155652E-14,-1.,4.64046037923618E-14));
#79783=DIRECTION('ref_axis',(1.,5.7936323155652E-14,1.59675549687847E-31));
#79784=DIRECTION('center_axis',(-0.101428913894775,-0.987363722346308,0.12175818338235));
#79785=DIRECTION('ref_axis',(0.732040068171316,0.00880346020649426,0.681204695873515));
#79786=DIRECTION('center_axis',(0.110956859394232,-0.987363722163564,-0.113143517307362));
#79787=DIRECTION('ref_axis',(0.778622256538946,0.0156160399944578,0.627298589921173));
#79788=DIRECTION('center_axis',(0.0819510841136594,0.98736372258261,-0.135635169260802));
#79789=DIRECTION('ref_axis',(0.826216048340669,0.00880314079029221,0.563284604952554));
#79790=DIRECTION('',(0.216671506352657,0.,0.976244568914404));
#79791=DIRECTION('',(-0.976244568854602,0.,0.216671506622102));
#79792=DIRECTION('center_axis',(-2.66229689183797E-14,-1.,-1.31460372347046E-14));
#79793=DIRECTION('ref_axis',(1.,-2.66229689183797E-14,-3.13869790383516E-31));
#79794=DIRECTION('center_axis',(-0.0728831540845708,-0.987363722339392,
0.14071576194153));
#79795=DIRECTION('ref_axis',(0.861364251543031,0.00880345782593299,0.507911532940552));
#79796=DIRECTION('center_axis',(0.0840402415482007,-0.987363722072949,-0.134350728076821));
#79797=DIRECTION('ref_axis',(0.895269154764806,0.0156160439371077,0.445251928348957));
#79798=DIRECTION('center_axis',(0.0508775536079316,0.987363722440774,-0.150081158533545));
#79799=DIRECTION('ref_axis',(0.927989115978238,0.00880314919346329,0.372503295542745));
#79800=DIRECTION('',(0.421469569973658,0.,0.906842545090502));
#79801=DIRECTION('',(-0.906842544711597,0.,0.421469570788919));
#79802=DIRECTION('center_axis',(5.76530962313139E-14,-1.,1.42310776850099E-14));
#79803=DIRECTION('ref_axis',(1.,5.76530962313139E-14,-3.49047495775741E-32));
#79804=DIRECTION('center_axis',(-0.0409294558697067,-0.987363722338178,
0.153093629693422));
#79805=DIRECTION('ref_axis',(0.950411999976481,0.00880345909517113,0.310868990747977));
#79806=DIRECTION('center_axis',(0.0531939918611952,-0.987363722074152,-0.149275850564478));
#79807=DIRECTION('ref_axis',(0.97005426217788,0.0156160433238334,0.242385782630575));
#79808=DIRECTION('center_axis',(0.0174250530024264,0.987363722465118,-0.157509514276718));
#79809=DIRECTION('ref_axis',(0.986370443252028,0.00880314841710919,0.16430414862913));
#79810=DIRECTION('',(0.606560187375799,0.,0.795037570867337));
#79811=DIRECTION('',(-0.795037570322038,0.,0.60656018809054));
#79812=DIRECTION('',(0.763288722545863,0.,0.646057525329057));
#79813=DIRECTION('',(-0.646057524642841,0.,0.763288723126685));
#79814=DIRECTION('center_axis',(1.02025012898349E-13,-1.,-1.97612283078631E-14));
#79815=DIRECTION('ref_axis',(1.,1.02025012898349E-13,4.59893401350721E-31));
#79816=DIRECTION('center_axis',(0.0271357814488703,-0.987363722366704,0.156129846984253));
#79817=DIRECTION('ref_axis',(0.993101070891819,0.00880346203509836,-0.116930586459314));
#79818=DIRECTION('center_axis',(-0.0144017443938191,-0.987363722089207,
-0.15781466997894));
#79819=DIRECTION('ref_axis',(0.982172552118582,0.0156160426088595,-0.187331836797992));
#79820=DIRECTION('center_axis',(-0.0503219761172802,0.987363722498807,-0.150268353996944));
#79821=DIRECTION('ref_axis',(0.96419509013843,0.00880314564673555,-0.265047793387659));
#79822=DIRECTION('',(0.884326726537715,0.,0.466868547592457));
#79823=DIRECTION('',(-0.466868544549227,0.,0.884326728144347));
#79824=DIRECTION('center_axis',(-8.1764267020795E-14,-1.,3.5341357472854E-14));
#79825=DIRECTION('ref_axis',(1.,-8.1764267020795E-14,3.41816808687732E-32));
#79826=DIRECTION('center_axis',(0.0600646626700829,-0.987363722325553,0.146646227819738));
#79827=DIRECTION('ref_axis',(0.944746300203437,0.00880346065774608,-0.327684188407626));
#79828=DIRECTION('center_axis',(-0.0479905351096277,-0.987363722266364,
-0.1510290981639));
#79829=DIRECTION('ref_axis',(0.918939096098908,0.0156160354520983,-0.394090189040125));
#79830=DIRECTION('center_axis',(-0.0814487305111112,0.987363722500292,-0.135937426003639));
#79831=DIRECTION('ref_axis',(0.884675303833306,0.00880314564771947,-0.466124566413477));
#79832=DIRECTION('',(0.964014596804326,0.,0.265849312860112));
#79833=DIRECTION('',(-0.265849311993547,0.,0.964014597043301));
#79834=DIRECTION('center_axis',(-3.61276583900821E-14,-1.,2.60459983457543E-14));
#79835=DIRECTION('ref_axis',(1.,-3.61276583900821E-14,-3.2333570323359E-31));
#79836=DIRECTION('center_axis',(0.0901849869769349,-0.987363722335554,0.130305594429595));
#79837=DIRECTION('ref_axis',(0.852216242175415,0.00880345886951841,-0.52311564274484));
#79838=DIRECTION('center_axis',(-0.0793353310103516,-0.987363722158274,
-0.137181578279438));
#79839=DIRECTION('ref_axis',(0.812737069336137,0.0156160402722304,-0.582421321221264));
#79840=DIRECTION('center_axis',(-0.108767033422489,0.987363722485668,-0.115250214575575));
#79841=DIRECTION('ref_axis',(0.763789083031293,0.0088031463387518,-0.64540587327414));
#79842=DIRECTION('',(0.998626215044556,0.,0.0523992616912134));
#79843=DIRECTION('',(-0.0523992607935246,0.,0.998626215091659));
#79844=DIRECTION('center_axis',(1.97892627087603E-14,-1.,-2.2135623987073E-14));
#79845=DIRECTION('ref_axis',(2.17927070130815E-31,2.2135623987073E-14,-1.));
#79846=DIRECTION('center_axis',(0.116088364939715,-0.987363722346286,0.107872013609233));
#79847=DIRECTION('ref_axis',(0.719837499788847,0.00880346163078833,-0.694086790654495));
#79848=DIRECTION('center_axis',(-0.106970499871311,-0.987363722142377,-0.116919597820181));
#79849=DIRECTION('ref_axis',(0.668532361216325,0.0156160394805405,-0.743519079323098));
#79850=DIRECTION('center_axis',(-0.130999510954202,0.987363722460183,-0.0891740304086968));
#79851=DIRECTION('ref_axis',(0.607188933706365,0.00880314778993197,-0.794508718248904));
#79852=DIRECTION('',(0.986543181538475,0.,-0.16350092036421));
#79853=DIRECTION('',(0.163500921251019,0.,0.986543181391503));
#79854=DIRECTION('center_axis',(-7.28404795707868E-15,-1.,1.29361059625103E-14));
#79855=DIRECTION('ref_axis',(1.20157592816024E-31,-1.29361059625103E-14,
-1.));
#79856=DIRECTION('center_axis',(0.136563576359677,-0.987363722343636,0.0803944613239859));
#79857=DIRECTION('ref_axis',(0.553799956712619,0.00880345897931285,-0.8326032110526));
#79858=DIRECTION('center_axis',(-0.129603845053638,-0.987363722128365,-0.0911905892739679));
#79859=DIRECTION('ref_axis',(0.493067823026643,0.0156160419141663,-0.869850711979189));
#79860=DIRECTION('center_axis',(-0.14710659521871,0.987363722492469,-0.0589281694011677));
#79861=DIRECTION('ref_axis',(0.422197307061374,0.00880314719321597,-0.906461217322406));
#79862=DIRECTION('',(0.928330484416674,0.,-0.371755984084592));
#79863=DIRECTION('',(0.37175598392696,0.,0.928330484479799));
#79864=DIRECTION('center_axis',(-1.73314822661811E-14,-1.,5.67980879078818E-14));
#79865=DIRECTION('ref_axis',(-2.56612137703982E-31,-5.67980879078818E-14,
-1.));
#79866=DIRECTION('center_axis',(0.150653229585631,-0.987363722340501,0.0491577483346112));
#79867=DIRECTION('ref_axis',(0.361867341872136,0.00880346207617823,-0.932188031430284));
#79868=DIRECTION('center_axis',(-0.146177060289818,-0.987363722117319,-0.0611976085452662));
#79869=DIRECTION('ref_axis',(0.294547980804413,0.0156160421158191,-0.955509092700158));
#79870=DIRECTION('center_axis',(-0.156335138797612,0.987363722512107,-0.0259268942252293));
#79871=DIRECTION('ref_axis',(0.217464201437641,0.00880314485374298,-0.976028598829856));
#79872=DIRECTION('',(0.826710086440232,0.,-0.562628148049833));
#79873=DIRECTION('',(0.562628149420581,0.,0.826710085507351));
#79874=DIRECTION('center_axis',(9.43274378737716E-15,-1.,-1.1839187339302E-13));
#79875=DIRECTION('ref_axis',(-2.44385558762843E-31,1.1839187339302E-13,
-1.));
#79876=DIRECTION('center_axis',(0.157698503408068,-0.98736372234875,0.015622477795658));
#79877=DIRECTION('ref_axis',(0.15301421202466,0.00880346049852462,-0.988184775232711));
#79878=DIRECTION('center_axis',(-0.155915199182802,-0.987363722212749,-0.028343089492366));
#79879=DIRECTION('ref_axis',(0.0822554028362943,0.0156160359799182,-0.996488930256886));
#79880=DIRECTION('center_axis',(-0.158253626201034,0.987363722455138,0.00828669860420722));
#79881=DIRECTION('ref_axis',(0.00256271212569272,0.00880314780058656,-0.999957967664322));
#79882=DIRECTION('',(0.686433642709764,0.,-0.727192446437808));
#79883=DIRECTION('',(0.727192447054856,0.,0.686433642056077));
#79884=DIRECTION('center_axis',(-4.05963541081443E-15,-1.,-2.94129245268148E-14));
#79885=DIRECTION('ref_axis',(-7.93676947716632E-32,2.94129245268148E-14,
-1.));
#79886=DIRECTION('center_axis',(0.157369971051554,-0.987363722346701,-0.0186432831041112));
#79887=DIRECTION('ref_axis',(-0.0629936888030954,0.0088034602491171,-0.997975097013258));
#79888=DIRECTION('center_axis',(-0.158362915039063,-0.987363722199347,0.00583671354289517));
#79889=DIRECTION('ref_axis',(-0.133883348256068,0.0156160378949963,-0.990874052753531));
#79890=DIRECTION('center_axis',(-0.152772349398299,0.9873637225453,0.0421128087499838));
#79891=DIRECTION('ref_axis',(-0.212458609616509,0.00880314423507185,-0.977130412919072));
#79892=DIRECTION('',(0.514060325754162,0.,-0.857754033208544));
#79893=DIRECTION('',(0.857754032403029,0.,0.514060327098234));
#79894=DIRECTION('center_axis',(2.05752654287224E-14,-1.,5.57051301331E-14));
#79895=DIRECTION('ref_axis',(4.21927796756254E-31,-5.57051301331E-14,-1.));
#79896=DIRECTION('center_axis',(0.149682992850515,-0.987363722367468,-0.0520373078086402));
#79897=DIRECTION('ref_axis',(-0.276056079899396,0.0088034623672994,-0.961101212048411));
#79898=DIRECTION('center_axis',(-0.15340575824948,-0.987363722140233,0.0397435974376586));
#79899=DIRECTION('ref_axis',(-0.343761860804829,0.01561604059786,-0.938927005859373));
#79900=DIRECTION('center_axis',(-0.140147605930203,0.987363722434418,0.0739697787781123));
#79901=DIRECTION('ref_axis',(-0.417545600877838,0.00880314941097575,-0.908613325759651));
#79902=DIRECTION('',(0.317650121520213,0.,-0.948207994217616));
#79903=DIRECTION('',(0.948207994503158,0.,0.317650120667848));
#79904=DIRECTION('center_axis',(-4.00864794192018E-14,-1.,-6.24746266568276E-14));
#79905=DIRECTION('ref_axis',(9.85386662136157E-31,6.24746266568276E-14,
-1.));
#79906=DIRECTION('center_axis',(0.134997006595335,-0.987363722344993,-0.0829981205048595));
#79907=DIRECTION('ref_axis',(-0.476210392871911,0.00880345891853127,-0.87928730278098));
#79908=DIRECTION('center_axis',(-0.141275518359591,-0.9873637221238,0.0717921175761243));
#79909=DIRECTION('ref_axis',(-0.537566450769722,0.0156160405828081,-0.843076776031318));
#79910=DIRECTION('center_axis',(-0.120969720854335,0.987363722540651,0.102367993274716));
#79911=DIRECTION('ref_axis',(-0.603108622345235,0.00880314257524947,-0.797610490360823));
#79912=DIRECTION('',(0.106386948329893,0.,-0.994324804691632));
#79913=DIRECTION('',(0.994324804754728,0.,0.106386947740181));
#79914=DIRECTION('center_axis',(-7.36112688092222E-14,-1.,-7.33552349527714E-14));
#79915=DIRECTION('ref_axis',(1.,-7.36112688092222E-14,-8.57751515811246E-32));
#79916=DIRECTION('center_axis',(0.113998708832555,-0.987363722364275,-0.110078036608008));
#79917=DIRECTION('ref_axis',(-0.654097634895031,0.00880345963371462,-0.756358898356596));
#79918=DIRECTION('center_axis',(-0.122539391431094,-0.987363722160386,0.100483718627868));
#79919=DIRECTION('ref_axis',(-0.706235031996309,0.0156160398271936,-0.707805212527633));
#79920=DIRECTION('center_axis',(-0.0961354199797208,0.987363722474785,0.125979603770045));
#79921=DIRECTION('ref_axis',(-0.760470956138659,0.00880314729218524,-0.64931227423121));
#79922=DIRECTION('',(-0.109850763216409,0.,-0.993948092115867));
#79923=DIRECTION('',(0.993948092331009,0.,-0.109850761269768));
#79924=DIRECTION('center_axis',(-6.26139182359717E-14,-1.,-3.986855967794E-14));
#79925=DIRECTION('ref_axis',(1.,-6.26139182359717E-14,3.82708143775318E-31));
#79926=DIRECTION('center_axis',(0.0876699555725528,-0.987363722327332,-0.132010828047633));
#79927=DIRECTION('ref_axis',(-0.80140000250608,0.00880346280796036,-0.598063989072946));
#79928=DIRECTION('center_axis',(-0.0980734572555049,-0.987363722206742,
0.124476813310756));
#79929=DIRECTION('ref_axis',(-0.841880847839118,0.0156160374502623,-0.539437463860307));
#79930=DIRECTION('center_axis',(-0.066805935379289,0.98736372243709,0.143700544930325));
#79931=DIRECTION('ref_axis',(-0.882274512475655,0.00880314880506724,-0.470652939231194));
#79932=DIRECTION('',(-0.320951971885479,0.,-0.947095471292532));
#79933=DIRECTION('',(0.947095471004021,0.,-0.320951972736843));
#79934=DIRECTION('center_axis',(1.39441202957586E-14,-1.,5.09526267024895E-15));
#79935=DIRECTION('ref_axis',(1.,1.39441202957586E-14,-4.33523906184624E-32));
#79936=DIRECTION('center_axis',(0.0572418589532895,-0.987363722345415,-0.147770935504174));
#79937=DIRECTION('ref_axis',(-0.91122979430671,0.00880345858023634,-0.411804275214303));
#79938=DIRECTION('center_axis',(-0.0690217183973883,-0.98736372219858,0.142649509202227));
#79939=DIRECTION('ref_axis',(-0.938161250680476,0.0156160368527398,-0.34584621888154));
#79940=DIRECTION('center_axis',(-0.0343526832863041,0.987363722489873,0.154702206390121));
#79941=DIRECTION('ref_axis',(-0.962823895055901,0.00880314516105514,-0.269986391776803));
#79942=DIRECTION('',(-0.517045821934947,0.,-0.85595771976168));
#79943=DIRECTION('',(0.855957719296903,0.,-0.517045822704376));
#79944=DIRECTION('center_axis',(1.32421008241407E-13,-1.,1.78070812253087E-14));
#79945=DIRECTION('ref_axis',(1.,1.32421008241407E-13,-6.73625595346913E-32));
#79946=DIRECTION('center_axis',(0.0241371926388202,-0.987363722366506,-0.156621440697221));
#79947=DIRECTION('ref_axis',(-0.978451494625342,0.00880345880616111,-0.206289049099757));
#79948=DIRECTION('center_axis',(-0.0367426028754845,-0.987363722166912,
0.154152071937536));
#79949=DIRECTION('ref_axis',(-0.990574275756191,0.0156160384287705,-0.136083590318191));
#79950=DIRECTION('center_axis',(-0.000293134950792496,0.98736372249097,
0.15847016621647));
#79951=DIRECTION('ref_axis',(-0.998352700893353,0.00880314554373982,-0.0566955840209985));
#79952=DIRECTION('',(-0.688963187105363,0.,-0.724796334713153));
#79953=DIRECTION('',(0.724796334022858,0.,-0.68896318783156));
#79954=DIRECTION('center_axis',(-8.87687165924439E-14,-1.,7.38389392493327E-15));
#79955=DIRECTION('ref_axis',(1.,-8.87687165924439E-14,6.42305608760724E-32));
#79956=DIRECTION('center_axis',(-0.0100961008658548,-0.987363722319383,
-0.158148501715697));
#79957=DIRECTION('ref_axis',(-0.999921890126576,0.00880345827309538,0.00887202164842416));
#79958=DIRECTION('center_axis',(-0.00274544497606824,-0.987363722132808,
0.158446655843319));
#79959=DIRECTION('ref_axis',(-0.996669148956917,0.0156160409304335,0.0800421562875077));
#79960=DIRECTION('center_axis',(0.0337801256632999,0.987363722407798,0.154828236388552));
#79961=DIRECTION('ref_axis',(-0.987199644128115,0.00880315153869502,0.159246246914358));
#79962=DIRECTION('',(-0.828665397202258,0.,-0.559744280434935));
#79963=DIRECTION('',(0.559744277715943,0.,-0.828665399038875));
#79964=DIRECTION('center_axis',(2.83686781064228E-14,-1.,-8.76463754737869E-15));
#79965=DIRECTION('ref_axis',(1.,2.83686781064229E-14,-2.01260476470523E-31));
#79966=DIRECTION('center_axis',(-0.0438573179697657,-0.987363722349336,
-0.152280712662379));
#79967=DIRECTION('ref_axis',(-0.974637049721441,0.00880346401316108,0.223618246866515));
#79968=DIRECTION('center_axis',(0.0313800915095481,-0.987363722164575,0.155332449958691));
#79969=DIRECTION('ref_axis',(-0.95616088060051,0.0156160386448679,0.292425220776696));
#79970=DIRECTION('center_axis',(0.0662738583554316,0.987363722418044,0.143946710109916));
#79971=DIRECTION('ref_axis',(-0.929886229135973,0.00880315053968251,0.367741900527878));
#79972=DIRECTION('',(-0.929620135171039,0.,-0.36851920477036));
#79973=DIRECTION('',(0.36851920294983,0.,-0.929620135892732));
#79974=DIRECTION('center_axis',(0.0956686246027889,0.987363724192392,0.126334438754998));
#79975=DIRECTION('ref_axis',(-0.829092352089055,0.0088030580832515,0.559042375742503));
#79976=DIRECTION('',(-0.987106868437356,0.,-0.160062582397625));
#79977=DIRECTION('center_axis',(1.29106480976479E-14,-1.,-7.32907620994719E-15));
#79978=DIRECTION('ref_axis',(1.,1.29106480976479E-14,1.16314341729505E-31));
#79979=DIRECTION('center_axis',(-0.0755678077550528,-0.987363722339629,
-0.139292448606257));
#79980=DIRECTION('ref_axis',(-0.903779263376947,0.00880346100684245,0.427908333833455));
#79981=DIRECTION('center_axis',(0.0640381965992371,-0.987363718774048,0.14495515246103));
#79982=DIRECTION('ref_axis',(-0.87094360115238,0.0156161908311511,0.491134786179566));
#79983=DIRECTION('',(0.160062578709125,0.,-0.987106869035458));
#79984=DIRECTION('center_axis',(-4.41330782755392E-14,-1.,3.97325367041087E-14));
#79985=DIRECTION('ref_axis',(1.,-4.41330782755392E-14,5.27563451808919E-31));
#79986=DIRECTION('center_axis',(0.120590177674939,0.987363722471961,0.102814826725719));
#79987=DIRECTION('ref_axis',(-0.68953106913893,0.00880314808545024,0.724202602367534));
#79988=DIRECTION('center_axis',(-0.103744832782692,-0.987363722346209,-0.119791024144255));
#79989=DIRECTION('ref_axis',(-0.790661764724653,0.00880346052475684,0.612189899365619));
#79990=DIRECTION('center_axis',(0.0937021981459183,-0.98736372205965,0.127799759088729));
#79991=DIRECTION('ref_axis',(-0.745001950293547,0.0156160444667243,0.666879474278542));
#79992=DIRECTION('',(-0.998437581989233,-7.4805248799978E-15,0.0558783936015749));
#79993=DIRECTION('',(-0.0558783943386867,0.,-0.99843758194798));
#79994=DIRECTION('center_axis',(-4.31999381995619E-14,-1.,6.03636492336854E-14));
#79995=DIRECTION('ref_axis',(2.04237656696525E-31,-6.03636492336854E-14,
-1.));
#79996=DIRECTION('center_axis',(-0.127070866296767,-0.987363722339815,-0.0946883031100116));
#79997=DIRECTION('ref_axis',(-0.640573800107769,0.00880346197464888,0.76784614713675));
#79998=DIRECTION('center_axis',(0.118984666370147,-0.987363722173514,0.104668664386479));
#79999=DIRECTION('ref_axis',(-0.584224842185945,0.0156160393644823,0.811441601772657));
#80000=DIRECTION('center_axis',(0.139872995317343,0.987363722448375,0.0744877491527499));
#80001=DIRECTION('ref_axis',(-0.517728064119055,0.00880314880339182,0.855499945175148));
#80002=DIRECTION('',(-0.963082463777524,0.,0.269206552602669));
#80003=DIRECTION('',(-0.269206553468368,0.,-0.963082463535539));
#80004=DIRECTION('center_axis',(-3.5056256827116E-14,-1.,8.18869083354101E-14));
#80005=DIRECTION('ref_axis',(-2.79057244880545E-31,-8.18869083354101E-14,
-1.));
#80006=DIRECTION('center_axis',(-0.144455208023086,-0.987363722350595,-0.0651580590639688));
#80007=DIRECTION('ref_axis',(-0.460533315515677,0.0088034663068353,0.887598763113786));
#80008=DIRECTION('center_axis',(0.138703539564003,-0.987363722143998,0.0766433839699575));
#80009=DIRECTION('ref_axis',(-0.396130032146719,0.0156160402368145,0.918061619347395));
#80010=DIRECTION('center_axis',(0.152615505799362,0.987363722503179,0.0426777093371941));
#80011=DIRECTION('ref_axis',(-0.321716670115856,0.00880314689765988,0.946795061654983));
#80012=DIRECTION('',(-0.88269468020377,0.,0.469946913533821));
#80013=DIRECTION('',(-0.469946916567211,0.,-0.882694678588792));
#80014=DIRECTION('center_axis',(5.54446544015125E-15,-1.,-2.91694990146662E-14));
#80015=DIRECTION('ref_axis',(-1.44957932349112E-31,2.91694990146662E-14,
-1.));
#80016=DIRECTION('center_axis',(-0.15508498092205,-0.987363722354531,-0.0325811060372834));
#80017=DIRECTION('ref_axis',(-0.258958805904553,0.00880346029549782,0.965848246843837));
#80018=DIRECTION('center_axis',(0.151936789673519,-0.987363722123989,0.0450343444180885));
#80019=DIRECTION('ref_axis',(-0.189512623029802,0.015616041182101,0.981754095978297));
#80020=DIRECTION('center_axis',(0.158221886234408,0.987363722470712,0.00887210601856122));
#80021=DIRECTION('ref_axis',(-0.110662161816853,0.00880314662070804,0.99381909347305));
#80022=DIRECTION('',(-0.761033074724776,0.,0.64871307923839));
#80023=DIRECTION('center_axis',(-2.99509393216772E-15,-1.,-1.03877999789806E-13));
#80024=DIRECTION('ref_axis',(0.0288208256144518,-1.03921169296701E-13,0.999584593724264));
#80025=DIRECTION('center_axis',(-0.158463154906743,-0.987363722361537,0.00151930950452709));
#80026=DIRECTION('ref_axis',(-0.0452756706492831,0.00880346115518785,0.998935740034837));
#80027=DIRECTION('center_axis',(0.158065644955419,-0.987363722085724,0.0113195491894476));
#80028=DIRECTION('ref_axis',(0.0259661867516164,0.0156160424447702,0.99954084276929));
#80029=DIRECTION('',(-0.648713081341758,0.,-0.761033072931841));
#80030=DIRECTION('center_axis',(-0.158467695620547,-0.987363721671432,-0.000933044400132078));
#80031=DIRECTION('ref_axis',(-0.150057930269645,0.023149632801892,0.988406147322207));
#80032=DIRECTION('',(0.563196917554046,0.,0.826322716653501));
#80033=DIRECTION('',(0.826322717534269,0.,-0.563196916261782));
#80034=DIRECTION('center_axis',(-0.154562233296029,-0.987363721596047,-0.0349770970000011));
#80035=DIRECTION('ref_axis',(-0.359027761721998,0.0231496363467189,0.933039742267127));
#80036=DIRECTION('',(0.372394728026814,0.,0.928074440192076));
#80037=DIRECTION('center_axis',(2.16154908660597E-14,-1.,-7.10125017377928E-14));
#80038=DIRECTION('ref_axis',(-9.69985311778293E-32,7.10125017377928E-14,
-1.));
#80039=DIRECTION('center_axis',(0.158065646374123,0.987363722077051,0.0113195301352506));
#80040=DIRECTION('ref_axis',(-0.214528637032064,0.0231492483173103,0.976443329740906));
#80041=DIRECTION('center_axis',(-0.155570612698608,0.987363722813212,-0.0301771989590363));
#80042=DIRECTION('ref_axis',(-0.288936904074014,-0.0162697674035493,0.957209883010387));
#80043=DIRECTION('',(0.928074440978588,0.,-0.372394726066685));
#80044=DIRECTION('center_axis',(-0.14342960823569,-0.987363721719631,-0.0673856699403972));
#80045=DIRECTION('ref_axis',(-0.551209858073525,0.0231496287762393,0.834045434643753));
#80046=DIRECTION('',(0.164179775258774,0.,0.986430434139163));
#80047=DIRECTION('center_axis',(1.45502885892669E-14,-1.,-2.58822309381055E-14));
#80048=DIRECTION('ref_axis',(3.34263340561198E-31,2.58822309381055E-14,
-1.));
#80049=DIRECTION('center_axis',(0.151936792278081,0.98736372224679,0.0450343329384399));
#80050=DIRECTION('ref_axis',(-0.419419530467412,0.0231492422746426,0.907497311315359));
#80051=DIRECTION('center_axis',(-0.145446249712898,0.987363722931636,-0.0629147604543809));
#80052=DIRECTION('ref_axis',(-0.487953552939853,-0.0162697625976409,0.872717952719199));
#80053=DIRECTION('',(0.986430434661683,0.,-0.164179772119355));
#80054=DIRECTION('center_axis',(-0.125590380613658,-0.987363721619889,-0.096643352209241));
#80055=DIRECTION('ref_axis',(-0.717617991607929,0.0231496346007728,0.696052090391555));
#80056=DIRECTION('',(-0.0517120410961091,0.,0.998662037330785));
#80057=DIRECTION('center_axis',(4.94350637840417E-14,-1.,-5.53730920682456E-14));
#80058=DIRECTION('ref_axis',(1.10788581713826E-30,5.53730920682456E-14,
-1.));
#80059=DIRECTION('center_axis',(0.138703544670118,0.987363722225615,0.076643373677849));
#80060=DIRECTION('ref_axis',(-0.604698830638238,0.023149243016814,0.796117727960191));
#80061=DIRECTION('center_axis',(-0.128520985285773,0.98736372286041,-0.0927104908864498));
#80062=DIRECTION('ref_axis',(-0.664154030955957,-0.0162697648243992,0.747418703216285));
#80063=DIRECTION('',(0.998662037017743,0.,0.0517120471415683));
#80064=DIRECTION('center_axis',(-0.101878684209459,-0.987363721630791,-0.121382102927672));
#80065=DIRECTION('ref_axis',(-0.850471105103065,0.023149635510488,0.525512125226909));
#80066=DIRECTION('',(-0.265185861602725,0.,0.964197313212405));
#80067=DIRECTION('center_axis',(-1.20365754886992E-14,-1.,8.69028450318463E-15));
#80068=DIRECTION('ref_axis',(1.,-1.20365754886992E-14,7.95976927521444E-32));
#80069=DIRECTION('center_axis',(0.118984673112717,0.987363722197058,0.104668656499597));
#80070=DIRECTION('ref_axis',(-0.761703085973765,0.0231492427474054,0.647512564648954));
#80071=DIRECTION('center_axis',(-0.105586217923025,0.987363722968099,-0.118171185791153));
#80072=DIRECTION('ref_axis',(-0.809299406389199,-0.0162697611307288,0.587170985055324));
#80073=DIRECTION('',(0.964197312368427,0.,0.265185864671369));
#80074=DIRECTION('center_axis',(-0.0734032480289828,-0.987363721695065,
-0.140445164599092));
#80075=DIRECTION('ref_axis',(-0.943557136986267,0.0231496302779127,0.330399793977349));
#80076=DIRECTION('',(-0.46625988377264,0.,0.884647794765987));
#80077=DIRECTION('center_axis',(-1.36233213274569E-14,-1.,5.89960255031437E-15));
#80078=DIRECTION('ref_axis',(1.,-1.36233213274569E-14,-1.3669389075937E-31));
#80079=DIRECTION('center_axis',(0.0937022060756123,0.98736372236211,0.127799750937949));
#80080=DIRECTION('ref_axis',(-0.883090952952439,0.023149238195361,0.468630431773832));
#80081=DIRECTION('center_axis',(-0.0777143651771768,0.987363722808187,-0.138106322547035));
#80082=DIRECTION('ref_axis',(-0.91660284094264,-0.0162697677780348,0.399467804250018));
#80083=DIRECTION('',(0.884647793282078,0.,0.466259886588103));
#80084=DIRECTION('center_axis',(-0.0414955664543414,-0.987363721630556,
-0.152941162453053));
#80085=DIRECTION('ref_axis',(-0.992523484580295,0.023149634910543,0.119838336771237));
#80086=DIRECTION('',(-0.64553211208243,0.,0.763733128959585));
#80087=DIRECTION('center_axis',(1.0201139073888E-13,-1.,-1.9831432186191E-14));
#80088=DIRECTION('ref_axis',(1.,1.0201139073888E-13,1.91380290558237E-31));
#80089=DIRECTION('center_axis',(0.0640383411138823,0.987363722029649,0.144955066441778));
#80090=DIRECTION('ref_axis',(-0.963186466508821,0.023149247304864,0.267835664323237));
#80091=DIRECTION('center_axis',(-0.0462086656340887,0.98736372290792,-0.151583765310571));
#80092=DIRECTION('ref_axis',(-0.981046945841421,-0.016269763912773,0.193085951942246));
#80093=DIRECTION('',(0.763733125487799,0.,0.645532116189921));
#80094=DIRECTION('center_axis',(-0.00764758997613864,-0.987363721700575,
-0.158285803018297));
#80095=DIRECTION('ref_axis',(-0.995080537351366,0.0231496303981934,-0.0963266255868246));
#80096=DIRECTION('',(-0.794619977419008,0.,0.607107149922166));
#80097=DIRECTION('center_axis',(-1.48413703996974E-14,-1.,-3.65949892926735E-16));
#80098=DIRECTION('ref_axis',(-0.999696144378386,1.48458814041184E-14,-0.0246499272816014));
#80099=DIRECTION('center_axis',(0.0313800969967225,0.987363722278217,0.155332448127816));
#80100=DIRECTION('ref_axis',(-0.998244453125112,0.0231492385997883,0.054517195059875));
#80101=DIRECTION('center_axis',(-0.0125422991360817,0.987363723013676,-0.157973318028564));
#80102=DIRECTION('ref_axis',(-0.999618385591608,-0.0162697590345936,-0.0223243841613663));
#80103=DIRECTION('',(0.6071071473932,0.,0.794619979351194));
#80104=DIRECTION('center_axis',(0.0265579739516111,-0.987363721673672,-0.156229175067596));
#80105=DIRECTION('ref_axis',(-0.951108729662977,0.0231496319897582,-0.30798746548783));
#80106=DIRECTION('',(-0.906552294984449,0.,0.422093516247796));
#80107=DIRECTION('center_axis',(-1.44157189798803E-14,-1.,-3.54785011149324E-15));
#80108=DIRECTION('ref_axis',(1.,-1.44157189798803E-14,-6.21375054833169E-32));
#80109=DIRECTION('center_axis',(-0.00274543728995823,0.987363722329316,
0.158446654751954));
#80110=DIRECTION('ref_axis',(-0.986625637587546,0.0231492386145962,-0.16135043850741));
#80111=DIRECTION('center_axis',(0.0217105186266266,0.987363722833723,-0.156976215436906));
#80112=DIRECTION('ref_axis',(-0.971448780790989,-0.01626976712843,-0.236690855288682));
#80113=DIRECTION('',(0.422093512262599,0.,0.906552296839969));
#80114=DIRECTION('center_axis',(0.059521713817587,-0.987363721611479,-0.146867446460227));
#80115=DIRECTION('ref_axis',(-0.862664136105473,0.0231496361748456,-0.505247150038839));
#80116=DIRECTION('',(-0.976095235356397,0.,0.217343257347773));
#80117=DIRECTION('center_axis',(-5.32640183211155E-14,-1.,-2.62554272104013E-14));
#80118=DIRECTION('ref_axis',(1.,-5.32640183211155E-14,-2.10243185391532E-31));
#80119=DIRECTION('center_axis',(-0.0367425905234397,0.987363722095349,0.154152075340054));
#80120=DIRECTION('ref_axis',(-0.928873303691505,0.0231492463964906,-0.369673501999405));
#80121=DIRECTION('center_axis',(0.0549481854235957,0.987363722864592,-0.148639078608649));
#80122=DIRECTION('ref_axis',(-0.897855310311268,-0.0162697666496942,-0.439989927656328));
#80123=DIRECTION('',(0.217343253631377,0.,0.976095236183912));
#80124=DIRECTION('center_axis',(0.0897022905136939,-0.987363721638354,-0.130638356806321));
#80125=DIRECTION('ref_axis',(-0.733882324749335,0.0231496342440029,-0.678882042666382));
#80126=DIRECTION('',(-0.999997046887668,0.,0.00243027075520032));
#80127=DIRECTION('center_axis',(8.11555403438022E-14,-1.,6.49106139899144E-14));
#80128=DIRECTION('ref_axis',(1.,8.11555403438022E-14,-1.83734581581371E-30));
#80129=DIRECTION('center_axis',(-0.0690217128897,0.987363722232311,0.142649511633679));
#80130=DIRECTION('ref_axis',(-0.82768788739491,0.0231492409593687,-0.560711042964873));
#80131=DIRECTION('center_axis',(0.0856165363963591,0.987363722869809,-0.13335174335629));
#80132=DIRECTION('ref_axis',(-0.782279123826205,-0.0162697655685773,-0.62271555878591));
#80133=DIRECTION('',(0.00243026757266593,0.,0.999997046895402));
#80134=DIRECTION('center_axis',(0.115688484628851,-0.987363721599696,-0.108300765431633));
#80135=DIRECTION('ref_axis',(-0.570784992354785,0.0231496363486892,-0.82077316405903));
#80136=DIRECTION('',(-0.977140108330193,0.,-0.212596351550206));
#80137=DIRECTION('center_axis',(-2.79875595292076E-14,-1.,-3.46453208693661E-14));
#80138=DIRECTION('ref_axis',(2.42805112830695E-31,3.46453208693661E-14,
-1.));
#80139=DIRECTION('center_axis',(-0.0980734510975878,0.98736372225289,0.124476817796436));
#80140=DIRECTION('ref_axis',(-0.687800705810551,0.0231492416525541,-0.725530358908171));
#80141=DIRECTION('center_axis',(0.112281552464805,0.98736372285531,-0.111829029171298));
#80142=DIRECTION('ref_axis',(-0.630124435048572,-0.0162697654267482,-0.776323702515695));
#80143=DIRECTION('',(-0.212596357404932,0.,0.97714010705638));
#80144=DIRECTION('center_axis',(0.136265218706276,-0.987363721707863,-0.0808991423077467));
#80145=DIRECTION('ref_axis',(-0.380998386991564,0.0231496287520599,-0.924285845287305));
#80146=DIRECTION('',(-0.908593184668933,0.,-0.417682205478239));
#80147=DIRECTION('center_axis',(-5.96565182927404E-14,-1.,-1.19555491768862E-13));
#80148=DIRECTION('ref_axis',(-1.47827908722308E-30,1.19555491768862E-13,
-1.));
#80149=DIRECTION('center_axis',(-0.122539383910873,0.987363722169366,0.100483727710508));
#80150=DIRECTION('ref_axis',(-0.51575272537891,0.0231492437747636,-0.856424683656936));
#80151=DIRECTION('center_axis',(0.133696406656168,0.987363722782425,-0.0850773164859957));
#80152=DIRECTION('ref_axis',(-0.448505827915095,-0.0162697683111609,-0.893631812865509));
#80153=DIRECTION('',(-0.417682210743198,0.,0.90859318224862));
#80154=DIRECTION('center_axis',(0.150470336690132,-0.987363721658464,-0.0497147757623953));
#80155=DIRECTION('ref_axis',(-0.173396723049576,0.0231496331670833,-0.984579946433959));
#80156=DIRECTION('',(-0.797561452045313,0.,-0.603237706224812));
#80157=DIRECTION('center_axis',(-7.23575228850367E-15,-1.,-2.87966085777709E-14));
#80158=DIRECTION('ref_axis',(1.43902150932921E-33,2.87966085777709E-14,
-1.));
#80159=DIRECTION('center_axis',(-0.141275515075797,0.987363722429278,0.0717921198368483));
#80160=DIRECTION('ref_axis',(-0.319588720183942,0.0231492347253357,-0.947273541730593));
#80161=DIRECTION('center_axis',(0.148859768603231,0.987363722988668,-0.0543474729619374));
#80162=DIRECTION('ref_axis',(-0.245915584978653,-0.016269760627855,-0.969154693510648));
#80163=DIRECTION('',(-0.60323770876311,0.,0.797561450125464));
#80164=DIRECTION('',(-0.649236632677518,0.,-0.760586480809091));
#80165=DIRECTION('',(-0.760586482875992,0.,0.649236630256125));
#80166=DIRECTION('center_axis',(0.15743787146309,-0.987363721659547,0.0180609462592491));
#80167=DIRECTION('ref_axis',(0.256043784428875,0.0231496327469448,-0.966387952614798));
#80168=DIRECTION('',(-0.470554230370041,0.,-0.882371076294355));
#80169=DIRECTION('center_axis',(0.,-1.,0.));
#80170=DIRECTION('ref_axis',(0.,0.,-1.));
#80171=DIRECTION('center_axis',(-0.158362914256764,0.987363722293322,0.00583671887102137));
#80172=DIRECTION('ref_axis',(0.107698968169371,0.0231492392945268,-0.993914002806751));
#80173=DIRECTION('center_axis',(0.157921378608865,0.987363722987877,0.0131801633447803));
#80174=DIRECTION('ref_axis',(0.183750552646889,-0.0162697611016185,-0.982838251837839));
#80175=DIRECTION('',(-0.882371077791938,0.,0.470554227561812));
#80176=DIRECTION('center_axis',(0.149874493682656,-0.987363721587329,0.0514831762480454));
#80177=DIRECTION('ref_axis',(0.457802465965002,0.0231496367329827,-0.888752494497481));
#80178=DIRECTION('',(-0.269869235978793,0.,-0.962896980716121));
#80179=DIRECTION('center_axis',(-3.49998983126278E-14,-1.,8.19110133354615E-14));
#80180=DIRECTION('ref_axis',(9.01557008337089E-31,-8.19110133354614E-14,
-1.));
#80181=DIRECTION('center_axis',(-0.155915201154255,0.987363722160555,-0.0283430804656613));
#80182=DIRECTION('ref_axis',(0.318843156646597,0.023149244932748,-0.947524751084993));
#80183=DIRECTION('center_axis',(0.151395920224427,0.987363722911968,0.0468204444320834));
#80184=DIRECTION('ref_axis',(0.390735738541771,-0.0162697637311714,-0.920359102423803));
#80185=DIRECTION('',(-0.962896981574999,0.,0.269869232914305));
#80186=DIRECTION('center_axis',(0.135303149199466,-0.987363721625002,0.0824981153453359));
#80187=DIRECTION('ref_axis',(0.638154814540316,0.0231496352403355,-0.769559956772216));
#80188=DIRECTION('',(-0.0565654558858671,0.,-0.998398892828124));
#80189=DIRECTION('center_axis',(-3.45267111776215E-14,-1.,4.83146905674551E-14));
#80190=DIRECTION('ref_axis',(9.07026936983547E-31,-4.83146905674551E-14,
-1.));
#80191=DIRECTION('center_axis',(-0.14617706594016,0.987363722148467,-0.06119759454628));
#80192=DIRECTION('ref_axis',(0.515078592760366,0.0231492446704375,-0.856830295771099));
#80193=DIRECTION('center_axis',(0.137791354900117,0.987363722950062,0.0782714578692801));
#80194=DIRECTION('ref_axis',(0.579450554843935,-0.0162697613589407,-0.814844984862998));
#80195=DIRECTION('',(-0.998398893008149,0.,0.0565654527083613));
#80196=DIRECTION('center_axis',(0.114405181244365,-0.987363721617109,0.109655532185364));
#80197=DIRECTION('ref_axis',(0.78866775356503,0.0231496364833883,-0.614383649536163));
#80198=DIRECTION('',(0.159383264798036,0.,-0.987216782121495));
#80199=DIRECTION('center_axis',(7.7185020740154E-14,-1.,-6.95850708510898E-14));
#80200=DIRECTION('ref_axis',(1.,7.7185020740154E-14,-7.07954392306507E-31));
#80201=DIRECTION('center_axis',(-0.129603858059397,0.987363721960499,-0.0911905726072057));
#80202=DIRECTION('ref_axis',(0.687229526331659,0.0231492508551655,-0.726071408556217));
#80203=DIRECTION('center_axis',(0.117743826010255,0.987363722792658,0.10606257751672));
#80204=DIRECTION('ref_axis',(0.741070908158961,-0.0162697697172345,-0.671229620676711));
#80205=DIRECTION('',(-0.987216781687272,0.,-0.159383267487605));
#80206=DIRECTION('center_axis',(0.0881577516901096,-0.987363721641326,0.131685580089599));
#80207=DIRECTION('ref_axis',(0.902303462413274,0.0231496338228235,-0.430479449185309));
#80208=DIRECTION('',(0.367879397950885,0.,-0.929873512131244));
#80209=DIRECTION('center_axis',(7.74336096465508E-14,-1.,-4.40277537714319E-14));
#80210=DIRECTION('ref_axis',(1.,7.74336096465508E-14,3.13411658643789E-31));
#80211=DIRECTION('center_axis',(-0.106970507172761,0.98736372217698,-0.116919590847819));
#80212=DIRECTION('ref_axis',(0.827246372683671,0.0231492422380706,-0.561362228392249));
#80213=DIRECTION('center_axis',(0.092190715571351,0.987363722946451,0.128894338788664));
#80214=DIRECTION('ref_axis',(0.868039608686221,-0.016269762386131,-0.496228306915044));
#80215=DIRECTION('',(-0.929873511942708,0.,-0.36787939842744));
#80216=DIRECTION('center_axis',(0.0577881631569067,-0.987363721669339,0.147558155756379));
#80217=DIRECTION('ref_axis',(0.973748465835437,0.0231496316831997,-0.226446505462252));
#80218=DIRECTION('',(0.55917389836542,0.,-0.829050391343505));
#80219=DIRECTION('center_axis',(0.,-1.,0.));
#80220=DIRECTION('ref_axis',(0.,0.,-1.));
#80221=DIRECTION('center_axis',(-0.0793353368678561,0.987363722342691,-0.137181573564561));
#80222=DIRECTION('ref_axis',(0.928582098048572,0.0231492389550655,-0.370404373515639));
#80223=DIRECTION('center_axis',(0.0623268761099373,0.987363722900334,0.145699139375525));
#80224=DIRECTION('ref_axis',(0.954419742951362,-0.0162697635743861,-0.298023906856295));
#80225=DIRECTION('',(-0.829050388663707,0.,-0.559173902338581));
#80226=DIRECTION('center_axis',(0.024716470913478,-0.987363721605843,0.156531074621758));
#80227=DIRECTION('ref_axis',(0.999662072669057,0.0231496360950727,-0.011825177194063));
#80228=DIRECTION('',(0.724322051650169,0.,-0.689461794078026));
#80229=DIRECTION('center_axis',(4.438180735115E-14,-1.,-3.72248916065518E-15));
#80230=DIRECTION('ref_axis',(1.,4.438180735115E-14,-1.00930208127364E-31));
#80231=DIRECTION('center_axis',(-0.0479905464206515,0.987363722052463,-0.151029095968143));
#80232=DIRECTION('ref_axis',(0.986498355424332,0.0231492477827189,-0.162126824036563));
#80233=DIRECTION('center_axis',(0.0295487005393224,0.987363722907453,0.155691210358106));
#80234=DIRECTION('ref_axis',(0.996172270241457,-0.0162697639762549,-0.0858842405924241));
#80235=DIRECTION('',(-0.689461790264558,0.,-0.724322055280102));
#80236=DIRECTION('center_axis',(-0.00951094462361416,-0.987363721678243,
0.15818477501345));
#80237=DIRECTION('ref_axis',(0.978832592072294,0.0231496322092273,0.203349087102972));
#80238=DIRECTION('',(0.855601711026882,0.,-0.517634728440695));
#80239=DIRECTION('center_axis',(8.82888209575531E-14,-1.,1.18106344614963E-14));
#80240=DIRECTION('ref_axis',(1.,8.82888209575531E-14,1.01618340658559E-31));
#80241=DIRECTION('center_axis',(-0.0144017553818927,0.98736372226706,-0.157814667863467));
#80242=DIRECTION('ref_axis',(0.998287046995834,0.0231492401613689,0.0537315966661112));
#80243=DIRECTION('center_axis',(-0.00461113702491368,0.987363722854809,
0.15840333394733));
#80244=DIRECTION('ref_axis',(0.991344889319113,-0.0162697664504085,0.130271275116678));
#80245=DIRECTION('',(-0.517634729095432,0.,-0.855601710630769));
#80246=DIRECTION('center_axis',(-0.0432936350148198,-0.987363721689003,
0.152441930779051));
#80247=DIRECTION('ref_axis',(0.912233988122506,0.0231496315622569,0.409014969741498));
#80248=DIRECTION('',(0.946874383847733,0.,-0.321603639924949));
#80249=DIRECTION('center_axis',(1.3947623333974E-14,-1.,5.08566584326984E-15));
#80250=DIRECTION('ref_axis',(1.,1.3947623333974E-14,-6.10860190589621E-32));
#80251=DIRECTION('center_axis',(0.0198604347480238,0.987363722186016,-0.157221001277166));
#80252=DIRECTION('ref_axis',(0.963396944726995,0.0231492443313783,0.267077590556711));
#80253=DIRECTION('center_axis',(-0.0385553678039905,0.987363722908173,0.153708692982577));
#80254=DIRECTION('ref_axis',(0.940163323192753,-0.0162697641668067,0.340335452894809));
#80255=DIRECTION('',(-0.321603636911446,0.,-0.946874384871262));
#80256=DIRECTION('center_axis',(-0.0750519575388816,-0.987363721595131,
0.139571074895176));
#80257=DIRECTION('ref_axis',(0.802980336676752,0.0231496378805331,0.595555768317704));
#80258=DIRECTION('',(0.993872262844379,0.,-0.110534723723333));
#80259=DIRECTION('center_axis',(-1.2528267825801E-14,-1.,-7.96509253005815E-15));
#80260=DIRECTION('ref_axis',(1.,-1.2528267825801E-14,1.55839561051282E-31));
#80261=DIRECTION('center_axis',(0.0531939794798619,0.987363722280913,-0.149275853608936));
#80262=DIRECTION('ref_axis',(0.883459473117363,0.023149240803084,0.467935328875084));
#80263=DIRECTION('center_axis',(-0.0706967919103074,0.987363722959237,0.141826803523406));
#80264=DIRECTION('ref_axis',(0.845020764817006,-0.0162697620358347,0.534485922987107));
#80265=DIRECTION('',(-0.110534720558305,0.,-0.993872263196381));
#80266=DIRECTION('center_axis',(-0.103300941109169,-0.987363721578903,0.120174027459422));
#80267=DIRECTION('ref_axis',(0.65618021622441,0.0231496365281075,0.754249042534562));
#80268=DIRECTION('',(0.994397779862904,0.,0.105702674534415));
#80269=DIRECTION('center_axis',(-2.1046208900298E-14,-1.,-2.09441607063673E-14));
#80270=DIRECTION('ref_axis',(1.,-2.1046208900298E-14,3.70559775903116E-32));
#80271=DIRECTION('center_axis',(0.0840402285537729,0.987363722249449,-0.134350734908083));
#80272=DIRECTION('ref_axis',(0.762212418662718,0.0231492422016354,0.646912931870913));
#80273=DIRECTION('center_axis',(-0.0995325095569162,0.987363722892599,0.123313252560172));
#80274=DIRECTION('ref_axis',(0.710365975348149,-0.0162697636185344,0.70364442430781));
#80275=DIRECTION('',(0.105702677699157,0.,-0.994397779526497));
#80276=DIRECTION('center_axis',(-0.126719690076456,-0.987363721725139,0.0951577698772395));
#80277=DIRECTION('ref_axis',(0.478697837936382,0.023149628695089,0.877674469633425));
#80278=DIRECTION('',(0.948426361813909,0.,0.316997533454809));
#80279=DIRECTION('center_axis',(2.40776771854987E-14,-1.,3.74682160055375E-14));
#80280=DIRECTION('ref_axis',(-4.36064925888224E-32,-3.74682160055375E-14,
-1.));
#80281=DIRECTION('center_axis',(0.110956844829281,0.987363721895544,-0.113143533929734));
#80282=DIRECTION('ref_axis',(0.605325158041782,0.023149253813639,0.795641605931693));
#80283=DIRECTION('center_axis',(-0.123714196260695,0.987363722788117,0.0990337142874071));
#80284=DIRECTION('ref_axis',(0.542495262034564,-0.0162697688673487,0.839901294969268));
#80285=DIRECTION('',(0.316997534753807,0.,-0.948426361379738));
#80286=DIRECTION('center_axis',(-0.144213159817898,-0.987363721644968,0.0656920521428219));
#80287=DIRECTION('ref_axis',(0.278832083128177,0.0231496344178445,0.960060812576329));
#80288=DIRECTION('',(0.858107580390881,0.,0.513469941160831));
#80289=DIRECTION('center_axis',(-3.09203911029191E-14,-1.,-8.35364374290109E-14));
#80290=DIRECTION('ref_axis',(-6.00164705136111E-31,8.35364374290109E-14,
-1.));
#80291=DIRECTION('center_axis',(0.132685252824541,0.987363722069219,-0.0866458540526028));
#80292=DIRECTION('ref_axis',(0.420133565785062,0.0231492482371895,0.907166963246999));
#80293=DIRECTION('center_axis',(-0.142111149096565,0.987363722895652,0.0701234626362136));
#80294=DIRECTION('ref_axis',(0.349258074078322,-0.0162697653671039,0.936885314446758));
#80295=DIRECTION('',(0.513469942625881,0.,-0.858107579514232));
#80296=DIRECTION('center_axis',(-0.154963385615948,-0.987363721624743,0.0331546427786408));
#80297=DIRECTION('ref_axis',(0.0659284479281176,0.0231496352727361,0.997555779964473));
#80298=DIRECTION('',(0.727664643914042,0.,0.685933062330028));
#80299=DIRECTION('center_axis',(1.22396248333418E-14,-1.,8.82303721717431E-14));
#80300=DIRECTION('ref_axis',(-1.12955086660186E-31,-8.82303721717431E-14,
-1.));
#80301=DIRECTION('center_axis',(0.148209443903507,0.987363722200597,-0.0560967095291348));
#80302=DIRECTION('ref_axis',(0.215296994344091,0.0231492427667388,0.976274201638928));
#80303=DIRECTION('center_axis',(-0.153863141406208,0.987363722919929,0.0379343166316623));
#80304=DIRECTION('ref_axis',(0.139689965561605,-0.0162697632310827,0.990061618448974));
#80305=DIRECTION('center_axis',(-2.33781757796594E-15,-1.,2.95995842083303E-14));
#80306=DIRECTION('ref_axis',(1.48758021322455E-32,-2.95995842083303E-14,
-1.));
#80307=DIRECTION('center_axis',(0.156803523942189,0.987363722029914,-0.0229245566706625));
#80308=DIRECTION('ref_axis',(0.000393374217064282,0.0231492494663704,0.99973194282561));
#80309=DIRECTION('center_axis',(-0.158420663823298,0.987363722839941,0.00397140950277908));
#80310=DIRECTION('ref_axis',(-0.0764098928436923,-0.0162697670803354,0.996943741118207));
#80311=DIRECTION('',(0.68593306312575,0.,-0.727664643163955));
#80312=DIRECTION('center_axis',(0.163668138515803,-0.986495110831716,0.00633535633501474));
#80313=DIRECTION('ref_axis',(0.0266156894481207,0.0108352085748758,0.999587016387438));
#80314=DIRECTION('center_axis',(-0.160735572549809,-0.986495109335916,0.0314876955873914));
#80315=DIRECTION('ref_axis',(0.137589022940409,0.00919562022088586,0.990446718069709));
#80316=DIRECTION('center_axis',(0.161203584621629,-0.986495110673399,-0.0289965674281651));
#80317=DIRECTION('ref_axis',(0.240875086954021,0.0108352135078831,0.97049564173835));
#80318=DIRECTION('center_axis',(-0.150208740836978,-0.986495109342673,0.0653049264539607));
#80319=DIRECTION('ref_axis',(0.347289035836757,0.0091956188842569,0.937713051088077));
#80320=DIRECTION('center_axis',(0.151201330251114,-0.986495110631542,-0.0629726482717326));
#80321=DIRECTION('ref_axis',(0.443871436852541,0.0108352148540632,0.896024969331507));
#80322=DIRECTION('center_axis',(-0.132658313610887,-0.986495109357092,0.0960685746977337));
#80323=DIRECTION('ref_axis',(0.540750198857872,0.00919562137026215,0.841132963914022));
#80324=DIRECTION('center_axis',(0.134129071901824,-0.98649511055174,-0.0940041963332786));
#80325=DIRECTION('ref_axis',(0.626112849827963,0.0108352185265547,0.779657166528846));
#80326=DIRECTION('center_axis',(-0.108904931346394,-0.986495109325204,0.122340161868011));
#80327=DIRECTION('ref_axis',(0.708926482606273,0.00919562280965737,0.705222434966898));
#80328=DIRECTION('center_axis',(0.11078507982091,-0.986495110702303,-0.120640219866864));
#80329=DIRECTION('ref_axis',(0.779077926113261,0.0108352124652135,0.626833457318524));
#80330=DIRECTION('center_axis',(-0.0800592741231365,-0.986495109329498,
0.142891258990387));
#80331=DIRECTION('ref_axis',(0.843954154358249,0.00919562458933819,0.536336485641118));
#80332=DIRECTION('center_axis',(0.0822609122539169,-0.986495110548935,-0.141635232827848));
#80333=DIRECTION('ref_axis',(0.895614180534253,0.0108352201189312,0.444699716247866));
#80334=DIRECTION('center_axis',(-0.0474701448624736,-0.986495109347409,
0.156760915346842));
#80335=DIRECTION('ref_axis',(0.939519464582128,0.00919561566255652,0.342372043724219));
#80336=DIRECTION('center_axis',(0.0498903044633597,-0.986495110644867,-0.156007545312159));
#80337=DIRECTION('ref_axis',(0.970272512659709,0.0108352150321386,0.241772308778781));
#80338=DIRECTION('center_axis',(-0.0126613523898467,-0.986495109360026,
0.163300610422653));
#80339=DIRECTION('ref_axis',(0.991153890708611,0.00919561936273666,0.132398661313921));
#80340=DIRECTION('center_axis',(0.0151868873866259,-0.986495110617347,-0.163085116364352));
#80341=DIRECTION('ref_axis',(0.999561980115019,0.0108352160970614,0.0275398983417428));
#80342=DIRECTION('center_axis',(0.0227394687730209,-0.986495109360623,0.162204549157824));
#80343=DIRECTION('ref_axis',(0.996443062115871,0.00919562124663718,-0.083765532953806));
#80344=DIRECTION('center_axis',(-0.0202266525106009,-0.986495110648347,
-0.162537008693776));
#80345=DIRECTION('ref_axis',(0.982113040696751,0.0108352162892002,-0.187980247316966));
#80346=DIRECTION('center_axis',(0.0570770171920215,-0.986495109334282,0.153523983038496));
#80347=DIRECTION('ref_axis',(0.955139663050732,0.0091956222371918,-0.296012946674642));
#80348=DIRECTION('center_axis',(-0.0546944187067478,-0.986495110682322,
-0.154388850511314));
#80349=DIRECTION('ref_axis',(0.918741586296566,0.0108352146166071,-0.394710648112616));
#80350=DIRECTION('center_axis',(0.0887457096270632,-0.986495109349921,0.13766480396774));
#80351=DIRECTION('ref_axis',(0.869174995589545,0.00919562629065882,-0.494419121291882));
#80352=DIRECTION('center_axis',(-0.0866047287783385,-0.986495110539464,
-0.139021645203043));
#80353=DIRECTION('ref_axis',(0.812410797887989,0.0108352196224996,-0.582984814116744));
#80354=DIRECTION('center_axis',(0.116264741557142,-0.986495109322745,0.115368579574145));
#80355=DIRECTION('ref_axis',(0.742568672016674,0.00919561744081361,-0.669706807460754));
#80356=DIRECTION('center_axis',(-0.11446550582471,-0.986495110697102,-0.11715393526043));
#80357=DIRECTION('ref_axis',(0.668092580575766,0.0108352145780534,-0.743999262032336));
#80358=DIRECTION('center_axis',(0.138347373964608,-0.986495109335736,0.0876778385555427));
#80359=DIRECTION('ref_axis',(0.581240659621162,0.00919562299657433,-0.813679750344607));
#80360=DIRECTION('center_axis',(-0.136974001509193,-0.986495110784133,-0.0898082363124904));
#80361=DIRECTION('ref_axis',(0.492535098370621,0.0108352090189169,-0.870225128985919));
#80362=DIRECTION('center_axis',(0.153961033449504,-0.98649510932601,0.0558873818945187));
#80363=DIRECTION('ref_axis',(0.392734481097556,0.00919562464302147,-0.919605930735801));
#80364=DIRECTION('center_axis',(-0.153077740706661,-0.986495110692389,-0.0582632120652054));
#80365=DIRECTION('ref_axis',(0.293947223383176,0.0108352127995201,-0.955760235639101));
#80366=DIRECTION('center_axis',(0.162375644751377,-0.986495109354807,0.0214836963910421));
#80367=DIRECTION('ref_axis',(0.185864477196147,0.0091956233116086,-0.982532359074506));
#80368=DIRECTION('center_axis',(-0.162023736642693,-0.986495110541471,-0.0239938667602651));
#80369=DIRECTION('ref_axis',(0.0816147053940807,0.0108352178154801,-0.996605056137249));
#80370=DIRECTION('center_axis',(0.163197752475919,-0.986495109366373,-0.0139245388805864));
#80371=DIRECTION('ref_axis',(-0.0296963431688148,0.0091956180469598,-0.999516667100221));
#80372=DIRECTION('center_axis',(-0.163393682065958,-0.986495110747374,0.0113974177977136));
#80373=DIRECTION('ref_axis',(-0.134534032791039,0.0108352109294644,-0.9908497324141));
#80374=DIRECTION('center_axis',(0.156388914161848,-0.986495109361921,-0.04868168785374));
#80375=DIRECTION('ref_axis',(-0.243868596486197,0.00919562266033067,-0.969764687010071));
#80376=DIRECTION('center_axis',(-0.157123521961374,-0.98649511068723,0.0462557611184147));
#80377=DIRECTION('ref_axis',(-0.344392104001794,0.0108352142003043,-0.938763376381105));
#80378=DIRECTION('center_axis',(0.14226750324635,-0.986495109321295,-0.0811625332602162));
#80379=DIRECTION('ref_axis',(-0.446637828743146,0.00919562490842527,-0.894667586547178));
#80380=DIRECTION('center_axis',(-0.143506439863672,-0.986495110699152,0.0789512399163027));
#80381=DIRECTION('ref_axis',(-0.538146784719012,0.0108352141235931,-0.842781487831505));
#80382=DIRECTION('center_axis',(0.121493827765215,-0.98649510934329,-0.109848300199533));
#80383=DIRECTION('ref_axis',(-0.628522767255273,0.00919561739562644,-0.77773682673671));
#80384=DIRECTION('center_axis',(-0.123179159947951,-0.986495110553911,0.107955043456728));
#80385=DIRECTION('ref_axis',(-0.706738317361023,0.0108352183847782,-0.707392075737539));
#80386=DIRECTION('center_axis',(0.0950392295742507,-0.986495109351144,-0.133397691390092));
#80387=DIRECTION('ref_axis',(-0.78101868357014,0.00919562018628519,-0.624439954266025));
#80388=DIRECTION('center_axis',(-0.0970921547944209,-0.986495110583613,
0.131910993749582));
#80389=DIRECTION('ref_axis',(-0.842283554826315,0.0108352166558452,-0.538925793917091));
#80390=DIRECTION('center_axis',(0.0641407031163179,-0.986495109342318,-0.150709553271953));
#80391=DIRECTION('ref_axis',(-0.896995032092018,0.00919562221238664,-0.441944965956585));
#80392=DIRECTION('center_axis',(-0.0664652338195093,-0.986495110523081,
0.149698929880515));
#80393=DIRECTION('ref_axis',(-0.93844454810202,0.0108352208023414,-0.345259942836929));
#80394=DIRECTION('center_axis',(0.0302430298729998,-0.986495109332971,-0.160974402953483));
#80395=DIRECTION('ref_axis',(-0.971028890904804,0.00919562225295301,-0.238785120054764));
#80396=DIRECTION('center_axis',(-0.0327304542696101,-0.986495110838626,
0.160487113672068));
#80397=DIRECTION('ref_axis',(-0.990724918720199,0.0108352068721514,-0.135450115241342));
#80398=DIRECTION('center_axis',(-0.0050687708200986,-0.986495109324231,
-0.163712268452142));
#80399=DIRECTION('ref_axis',(-0.999658517458995,0.00919561933249602,-0.0244599480125467));
#80400=DIRECTION('center_axis',(0.00253474197814183,-0.986495110653344,
0.163771095557642));
#80401=DIRECTION('ref_axis',(-0.996680091659884,0.0108352157596983,0.0806932028629744));
#80402=DIRECTION('center_axis',(-0.0401435654910706,-0.986495109322325,
-0.158795130381252));
#80403=DIRECTION('ref_axis',(-0.98154522275664,0.00919562080493988,0.191008942831561));
#80404=DIRECTION('center_axis',(0.0376814241786472,-0.986495110573158,0.159397324592106));
#80405=DIRECTION('ref_axis',(-0.956031612134756,0.0108352171239012,0.293063397013166));
#80406=DIRECTION('center_axis',(-0.0733412931472915,-0.986495109333737,
-0.146452907038753));
#80407=DIRECTION('ref_axis',(-0.917535964181018,0.00919562396514639,0.397546468899299));
#80408=DIRECTION('center_axis',(0.0710661668584858,-0.986495110657146,0.14757031062374));
#80409=DIRECTION('ref_axis',(-0.870680155667432,0.0108352167935401,0.491730276273461));
#80410=DIRECTION('center_axis',(-0.103109658554887,-0.98649510935733,-0.127262710668778));
#80411=DIRECTION('ref_axis',(-0.810623745170238,0.00919562209843176,0.585495161637054));
#80412=DIRECTION('center_axis',(0.101127933530792,-0.986495110572645,0.128843074614264));
#80413=DIRECTION('ref_axis',(-0.744616664928424,0.0108352174921367,0.667404390435641));
#80414=DIRECTION('center_axis',(-0.128056733023712,-0.986495109359134,-0.102121850442517));
#80415=DIRECTION('ref_axis',(-0.665807659368194,0.00919562209060315,0.746066753890705));
#80416=DIRECTION('center_axis',(0.126461072293326,-0.986495110609015,0.104091276958878));
#80417=DIRECTION('ref_axis',(-0.583735724868433,0.0108352154539179,0.811871419387573));
#80418=DIRECTION('center_axis',(-0.147016018399577,-0.986495109320743,-0.072205883556608));
#80419=DIRECTION('ref_axis',(-0.489859148114204,0.00919562510711065,0.871753093190793));
#80420=DIRECTION('center_axis',(0.145881029487065,-0.986495110618633,0.0744722898890882));
#80421=DIRECTION('ref_axis',(-0.395559949617682,0.0108352175612732,0.91837624333323));
#80422=DIRECTION('center_axis',(-0.159100996125728,-0.986495109348092,-0.0389136513847887));
#80423=DIRECTION('ref_axis',(-0.291005366413958,0.00919562548096839,0.956677227276939));
#80424=DIRECTION('center_axis',(0.158479752759108,-0.986495110571815,0.0413710621487411));
#80425=DIRECTION('ref_axis',(-0.188888235368966,0.0108352192583513,0.981938813044286));
#80426=DIRECTION('center_axis',(-0.163746588080474,-0.986495109318213,-0.00380186575922749));
#80427=DIRECTION('ref_axis',(-0.078544499883981,0.00919562065573288,0.996868196954207));
#80428=DIRECTION('center_axis',(-0.163785826049748,0.986495107503612,-0.00126730289954508));
#80429=DIRECTION('ref_axis',(-0.0773835475264423,-0.0115671232882696,0.996934294841469));
#80430=DIRECTION('center_axis',(-0.15968413796074,0.986495109554075,-0.0364468779133307));
#80431=DIRECTION('ref_axis',(-0.289885795065082,-0.0115670281141406,0.956991342531421));
#80432=DIRECTION('center_axis',(-0.148115829760526,0.986495109166574,-0.0699221035494464));
#80433=DIRECTION('ref_axis',(-0.488833270659318,-0.0115670686396249,0.872300542484986));
#80434=DIRECTION('center_axis',(-0.129621778541751,0.986495109136216,-0.100127889111863));
#80435=DIRECTION('ref_axis',(-0.66492345234669,-0.0115670683985371,0.746821936908673));
#80436=DIRECTION('center_axis',(-0.105066761514118,0.986495109034855,-0.125651802514903));
#80437=DIRECTION('ref_axis',(-0.809922550492909,-0.0115670734541557,0.586422769863831));
#80438=DIRECTION('center_axis',(-0.0755989299477404,0.986495109165786,-0.14530038328491));
#80439=DIRECTION('ref_axis',(-0.917050572988009,-0.0115670674832961,0.398603122832976));
#80440=DIRECTION('center_axis',(-0.0425961838796048,0.986495109110088,-0.158154876057523));
#80441=DIRECTION('ref_axis',(-0.981298328950922,-0.0115670697713018,0.192145238023309));
#80442=DIRECTION('center_axis',(-0.00760168522970371,0.986495109123514,
-0.163614223272475));
#80443=DIRECTION('ref_axis',(-0.999661665709804,-0.0115670697656513,-0.0232971459054031));
#80444=DIRECTION('center_axis',(0.027748260597412,0.986495109147497,-0.161423150947704));
#80445=DIRECTION('ref_axis',(-0.971281934258545,-0.0115670683292826,-0.237650178020647));
#80446=DIRECTION('center_axis',(0.0618007301690269,0.986495109234294,-0.151684109937044));
#80447=DIRECTION('ref_axis',(-0.897486138513145,-0.0115670653616409,-0.440890954971502));
#80448=DIRECTION('center_axis',(0.0929634596254936,0.986495109112267,-0.134852493013792));
#80449=DIRECTION('ref_axis',(-0.78172489008437,-0.0115670700835441,-0.623516157859813));
#80450=DIRECTION('center_axis',(0.119779323731273,0.986495109049208,-0.111715323158778));
#80451=DIRECTION('ref_axis',(-0.629411051229153,-0.01156707348397,-0.776986442225107));
#80452=DIRECTION('center_axis',(0.140994442093736,0.98649510906358,-0.0833544665408682));
#80453=DIRECTION('ref_axis',(-0.447666654717905,-0.0115670726511384,-0.894125700941407));
#80454=DIRECTION('center_axis',(0.155616817660157,0.98649510916704,-0.0510960433970798));
#80455=DIRECTION('ref_axis',(-0.244989860530128,-0.0115670679347961,-0.969456637079153));
#80456=DIRECTION('center_axis',(0.162962722044672,0.986495109086415,-0.0164484337361611));
#80457=DIRECTION('ref_axis',(-0.0308576148295037,-0.0115670710205182,-0.999456857735761));
#80458=DIRECTION('center_axis',(0.162688670639839,0.986495109142254,0.0189682915375994));
#80459=DIRECTION('ref_axis',(0.184717500858052,-0.0115670691724926,-0.982723586664894));
#80460=DIRECTION('center_axis',(0.154807480106536,0.986495109045727,0.0534980740954653));
#80461=DIRECTION('ref_axis',(0.391655430727299,-0.0115670742698257,-0.920039252627109));
#80462=DIRECTION('center_axis',(0.139687659558307,0.986495109146884,0.0855263549813787));
#80463=DIRECTION('ref_axis',(0.580279987484035,-0.0115670691065026,-0.81433490594338));
#80464=DIRECTION('center_axis',(0.118036205631609,0.986495109050785,0.113555510561892));
#80465=DIRECTION('ref_axis',(0.741771295505608,-0.0115670741590964,-0.670553165647087));
#80466=DIRECTION('center_axis',(0.0908655060555755,0.986495109046781,0.13627494133568));
#80467=DIRECTION('ref_axis',(0.868578204792008,-0.0115670736825183,-0.495417102012755));
#80468=DIRECTION('center_axis',(0.0594460303999144,0.98649510918911,0.152622308381373));
#80469=DIRECTION('ref_axis',(0.954771361534156,-0.0115670668654126,-0.297115886748495));
#80470=DIRECTION('center_axis',(0.0252469304063644,0.986495109178945,0.161833223013932));
#80471=DIRECTION('ref_axis',(0.996320470721413,-0.0115670669916884,-0.0849218616298022));
#80472=DIRECTION('center_axis',(-0.0101326829954701,0.986495109072926,0.16347699688491));
#80473=DIRECTION('ref_axis',(0.991282741819984,-0.0115670719871803,0.131243013587384));
#80474=DIRECTION('center_axis',(-0.0450385103095808,0.986495109124808,0.157476767371973));
#80475=DIRECTION('ref_axis',(0.939893734132406,-0.0115670697918787,0.341271111339756));
#80476=DIRECTION('center_axis',(-0.0778383841323234,0.986495109096431,0.144113100322244));
#80477=DIRECTION('ref_axis',(0.844556339406886,-0.0115670710113924,0.535341752935316));
#80478=DIRECTION('center_axis',(-0.106998623258878,0.98649510911199,0.124010863712931));
#80479=DIRECTION('ref_axis',(0.709728428982206,-0.0115670700803942,0.704380408574944));
#80480=DIRECTION('center_axis',(-0.131155746156512,0.986495109479997,0.0981099853336883));
#80481=DIRECTION('ref_axis',(0.541714399859645,-0.0115670322937331,0.840483023474371));
#80482=DIRECTION('center_axis',(-0.149180131415552,0.986495109199563,0.0676216527170227));
#80483=DIRECTION('ref_axis',(0.348370418284784,-0.0115670670447902,0.937285577945199));
#80484=DIRECTION('center_axis',(-0.160229038678211,0.986495109002492,0.0339713861715604));
#80485=DIRECTION('ref_axis',(0.138737020809764,-0.0115670753660123,0.990261703704787));
#80486=DIRECTION('center_axis',(-0.158467690734171,0.987363722391381,-0.000933112434262052));
#80487=DIRECTION('ref_axis',(0.132986651957032,0.0222802173076005,0.990867368681594));
#80488=DIRECTION('',(-0.726917198560946,0.,-0.686725117085655));
#80489=DIRECTION('center_axis',(-6.0717653292393E-15,-1.,-4.41218244212294E-14));
#80490=DIRECTION('ref_axis',(1.22893474481546E-32,4.41218244212294E-14,
-1.));
#80491=DIRECTION('center_axis',(-0.158463159478122,-0.987363721657774,0.00151929007160298));
#80492=DIRECTION('ref_axis',(0.0598900529342102,-0.00807590308752957,0.998172310449883));
#80493=DIRECTION('center_axis',(0.156803528780472,-0.98736372200041,-0.0229245248475905));
#80494=DIRECTION('ref_axis',(0.136667846576374,-0.00129577614547245,0.990616081373787));
#80495=DIRECTION('center_axis',(0.156429986048559,0.987363722317839,-0.0253483592271716));
#80496=DIRECTION('ref_axis',(0.104936288763291,0.00890473956681993,0.994439078533137));
#80497=DIRECTION('',(-0.514404155191573,0.,0.857547879200715));
#80498=DIRECTION('center_axis',(-0.154963395216921,0.987363722410324,0.0331545745089898));
#80499=DIRECTION('ref_axis',(0.342884692245767,0.0222802151330409,0.939113241221287));
#80500=DIRECTION('',(-0.857547878362246,0.,-0.514404156589359));
#80501=DIRECTION('center_axis',(-2.05529318053831E-14,-1.,-5.5713374170716E-14));
#80502=DIRECTION('ref_axis',(5.90908953540761E-31,5.5713374170716E-14,-1.));
#80503=DIRECTION('center_axis',(-0.154431776448159,-0.987363721641073,0.0355486653779795));
#80504=DIRECTION('ref_axis',(0.273067397311036,-0.00807590271631994,0.961961005613582));
#80505=DIRECTION('center_axis',(0.148209454900557,-0.98736372199961,-0.0560966840121288));
#80506=DIRECTION('ref_axis',(0.346425803548562,-0.00129577417114879,0.93807648068003));
#80507=DIRECTION('center_axis',(0.147323593750353,0.987363722328396,-0.0583835469485666));
#80508=DIRECTION('ref_axis',(0.316257941884345,0.00890473470050748,0.94863144576542));
#80509=DIRECTION('',(-0.318030226197861,0.,0.948080574225913));
#80510=DIRECTION('center_axis',(-0.144213183568975,0.987363722413158,0.0656919884562336));
#80511=DIRECTION('ref_axis',(0.536749825063267,0.0222802148207466,0.843447222606189));
#80512=DIRECTION('',(-0.948080573707219,0.,-0.318030227744142));
#80513=DIRECTION('center_axis',(-4.0061430327584E-14,-1.,-6.24906920732847E-14));
#80514=DIRECTION('ref_axis',(-6.88142309551226E-31,6.24906920732847E-14,
-1.));
#80515=DIRECTION('center_axis',(-0.143179334387656,-0.987363721660589,0.0679158254964088));
#80516=DIRECTION('ref_axis',(0.473476414686258,-0.00807590141090528,0.880769472990662));
#80517=DIRECTION('center_axis',(0.132685267518502,-0.987363722025356,-0.0866458320508252));
#80518=DIRECTION('ref_axis',(0.539985276142485,-0.00129578075687071,0.841673465485015));
#80519=DIRECTION('center_axis',(0.131328513345755,0.987363722333517,-0.088688789607791));
#80520=DIRECTION('ref_axis',(0.512791724826885,0.00890473470595383,0.858466861706895));
#80521=DIRECTION('',(-0.106785558236527,0.,0.994282074942575));
#80522=DIRECTION('center_axis',(-0.126719725305287,0.987363722365704,0.0951577163171387));
#80523=DIRECTION('ref_axis',(0.705517132930511,0.0222802169333673,0.70834254924783));
#80524=DIRECTION('',(-0.994282074768412,0.,-0.106785559858167));
#80525=DIRECTION('center_axis',(-3.15350807326005E-14,-1.,-3.14506026353153E-14));
#80526=DIRECTION('ref_axis',(1.,-3.15350807326005E-14,-6.58499687751044E-31));
#80527=DIRECTION('center_axis',(-0.125231991468926,-0.98736372154303,0.097107310195598));
#80528=DIRECTION('ref_axis',(0.651746198497286,-0.00807590874348845,0.758394140564326));
#80529=DIRECTION('center_axis',(0.110956868842192,-0.987363722031639,-0.113143509193262));
#80530=DIRECTION('ref_axis',(0.708295635388373,-0.00129577826698679,0.705914735537136));
#80531=DIRECTION('center_axis',(0.109192655757456,0.98736372233894,-0.114847044966885));
#80532=DIRECTION('ref_axis',(0.685347939677784,0.00890473688211755,0.72816131951682));
#80533=DIRECTION('',(0.109452286018412,0.,0.993992050815973));
#80534=DIRECTION('center_axis',(-0.103300990893775,0.98736372240331,0.120173977891405));
#80535=DIRECTION('ref_axis',(0.841295244695768,0.0222802153147481,0.540116564509751));
#80536=DIRECTION('',(-0.993992051028922,-7.48052486139887E-15,0.10945228408451));
#80537=DIRECTION('center_axis',(-2.50391719930817E-14,-1.,-1.59574632360699E-14));
#80538=DIRECTION('ref_axis',(1.,-2.50391719930817E-14,-2.12206039582561E-32));
#80539=DIRECTION('center_axis',(-0.101428934423903,-0.987363721560199,0.121758172655575));
#80540=DIRECTION('ref_axis',(0.799541057122385,-0.0080759069910923,0.600557139414636));
#80541=DIRECTION('center_axis',(0.0840402479765299,-0.987363722025756,-0.134350724402548));
#80542=DIRECTION('ref_axis',(0.843486878181686,-0.00129577952144824,0.537148217246176));
#80543=DIRECTION('center_axis',(0.0819510725694751,0.987363722321965,-0.135635178133206));
#80544=DIRECTION('ref_axis',(0.825858045362074,0.00890473659936113,0.563807763849373));
#80545=DIRECTION('',(0.320572261549181,0.,0.947224062788337));
#80546=DIRECTION('center_axis',(-0.0750520230763435,0.987363722323689,0.139571034499487));
#80547=DIRECTION('ref_axis',(0.937735324337171,0.022280220396402,0.346635331824884));
#80548=DIRECTION('',(-0.947224063311177,0.,0.320572260004299));
#80549=DIRECTION('center_axis',(5.57683059679842E-14,-1.,2.04034095930511E-14));
#80550=DIRECTION('ref_axis',(1.,5.57683059679842E-14,-5.27596941019497E-31));
#80551=DIRECTION('center_axis',(-0.0728831738933898,-0.987363721586963,
0.140715756961213));
#80552=DIRECTION('ref_axis',(0.909950264086116,-0.00807590654910975,0.414638754367001));
#80553=DIRECTION('center_axis',(0.053194000405138,-0.987363721999171,-0.149275848015821));
#80554=DIRECTION('ref_axis',(0.939237612569815,-0.00129577834127603,0.343265244516022));
#80555=DIRECTION('center_axis',(0.0508775475537803,0.987363722317756,-0.150081161395219));
#80556=DIRECTION('ref_axis',(0.927751945958066,0.00890473735634552,0.373091185132585));
#80557=DIRECTION('',(0.516702631843025,0.,0.856164931684597));
#80558=DIRECTION('center_axis',(-0.0432936966707817,0.987363722432758,0.152441908451404));
#80559=DIRECTION('ref_axis',(0.99032794366912,0.0222802153308313,0.136945814075875));
#80560=DIRECTION('',(-0.85616493303156,8.72727902552676E-15,0.516702629611138));
#80561=DIRECTION('center_axis',(0.,-1.,0.));
#80562=DIRECTION('ref_axis',(0.,0.,-1.));
#80563=DIRECTION('center_axis',(-0.040929475115219,-0.987363721612732,0.153093629226847));
#80564=DIRECTION('ref_axis',(0.977811208330937,-0.00807590414837374,0.209332321046173));
#80565=DIRECTION('center_axis',(0.0198604574058036,-0.987363722030831,-0.157220999389572));
#80566=DIRECTION('ref_axis',(0.991070639694408,-0.0012957806161101,0.133331571986204));
#80567=DIRECTION('center_axis',(0.0174250494756002,0.98736372231966,-0.157509515578703));
#80568=DIRECTION('ref_axis',(0.986265197685215,0.00890473293361446,0.16492927443703));
#80569=DIRECTION('',(0.688672563156092,0.,0.725072479657047));
#80570=DIRECTION('center_axis',(-0.00951101165175448,0.98736372237897,0.158184766609506));
#80571=DIRECTION('ref_axis',(0.99661392865015,0.0222802169467632,-0.0791471361030735));
#80572=DIRECTION('',(-0.725072479416792,0.,0.688672563409046));
#80573=DIRECTION('center_axis',(-5.91811130109693E-14,-1.,4.89887086351612E-15));
#80574=DIRECTION('ref_axis',(1.,-5.91811130109693E-14,1.32477618157157E-31));
#80575=DIRECTION('center_axis',(-0.00706196155846046,-0.98736372164178,
0.158313012366767));
#80576=DIRECTION('ref_axis',(0.999950786861993,-0.00807590397254324,-0.00576225902811757));
#80577=DIRECTION('center_axis',(-0.0144017381581722,-0.987363722014211,
-0.1578146710172));
#80578=DIRECTION('ref_axis',(0.996562305425301,-0.00129578193788791,-0.0828365399722749));
#80579=DIRECTION('center_axis',(-0.016842231762191,0.987363722303819,-0.15757290093038));
#80580=DIRECTION('ref_axis',(0.998661784202103,0.00890473654962193,-0.0509445428015075));
#80581=DIRECTION('',(0.828440931287242,0.,0.560076444218043));
#80582=DIRECTION('center_axis',(0.0247164028032826,0.987363722445006,0.156531080083181));
#80583=DIRECTION('ref_axis',(0.956299353761225,0.0222802136408306,-0.291539256492126));
#80584=DIRECTION('',(-0.560076443596154,0.,0.828440931707677));
#80585=DIRECTION('center_axis',(1.41860947647529E-14,-1.,-4.37663197613812E-15));
#80586=DIRECTION('ref_axis',(1.,1.41860947647529E-14,8.39717137422895E-32));
#80587=DIRECTION('center_axis',(0.0271357593812573,-0.987363721605125,0.156129855635876));
#80588=DIRECTION('ref_axis',(0.975333777955869,-0.00807590569621869,-0.220587400649986));
#80589=DIRECTION('center_axis',(-0.0479905184904216,-0.987363721986366,
-0.151029105275279));
#80590=DIRECTION('ref_axis',(0.955455825497261,-0.00129577751323549,-0.295131303802195));
#80591=DIRECTION('center_axis',(-0.0503219877413723,0.987363722316606,-0.150268351301443));
#80592=DIRECTION('ref_axis',(0.964362055625514,0.00890473870083696,-0.264436251861207));
#80593=DIRECTION('',(0.929472323171464,0.,0.368891854692188));
#80594=DIRECTION('center_axis',(0.0577881016916056,0.987363722440046,0.147558174670931));
#80595=DIRECTION('ref_axis',(0.871269283997801,0.0222802142335214,-0.490299323694892));
#80596=DIRECTION('',(-0.368891856208104,0.,0.929472322569822));
#80597=DIRECTION('center_axis',(0.,-1.,0.));
#80598=DIRECTION('ref_axis',(0.,0.,-1.));
#80599=DIRECTION('center_axis',(0.0600646429832507,-0.987363721595286,0.146646240800101));
#80600=DIRECTION('ref_axis',(0.905111246041376,-0.00807590689066388,-0.425098120458466));
#80601=DIRECTION('center_axis',(-0.0793353189735047,-0.987363722004232,
-0.13718158634934));
#80602=DIRECTION('ref_axis',(0.869673293108132,-0.00129577632919989,-0.493626057069682));
#80603=DIRECTION('center_axis',(-0.0814487385771656,0.98736372231045,-0.13593742254965));
#80604=DIRECTION('ref_axis',(0.884969829016108,0.00890473544351639,-0.465563215275737));
#80605=DIRECTION('',(0.987042621082438,0.,0.160458294166147));
#80606=DIRECTION('center_axis',(0.0881576954790623,0.987363722466547,0.131685611533014));
#80607=DIRECTION('ref_axis',(0.74549963072673,0.0222802120580983,-0.666133539717793));
#80608=DIRECTION('',(-0.160458295774993,0.,0.987042620820897));
#80609=DIRECTION('center_axis',(-5.51862541569629E-14,-1.,4.96435508966708E-14));
#80610=DIRECTION('ref_axis',(1.,-5.51862541569629E-14,1.09452219029166E-30));
#80611=DIRECTION('center_axis',(0.0901849711692664,-0.987363721572303,0.130305611153511));
#80612=DIRECTION('ref_axis',(0.792566717847699,-0.00807590799570002,-0.609731725818963));
#80613=DIRECTION('center_axis',(-0.10697049376863,-0.987363722044528,-0.116919604229878));
#80614=DIRECTION('ref_axis',(0.743225803750709,-0.0012957826187869,-0.66903940510744));
#80615=DIRECTION('center_axis',(-0.108767041434322,0.987363722333227,-0.115250208320414));
#80616=DIRECTION('ref_axis',(0.764197398165913,0.00890473803425694,-0.644920958162309));
#80617=DIRECTION('',(0.998459903193811,0.,-0.055478119238171));
#80618=DIRECTION('center_axis',(0.114405127522865,0.987363722361241,0.109655581533414));
#80619=DIRECTION('ref_axis',(0.584871244104147,0.0222802183373292,-0.810820090828358));
#80620=DIRECTION('',(0.0554781176097552,0.,0.998459903284292));
#80621=DIRECTION('center_axis',(3.45793073442067E-14,-1.,-4.82770604581073E-14));
#80622=DIRECTION('ref_axis',(2.10113896538771E-31,4.82770604581073E-14,
-1.));
#80623=DIRECTION('center_axis',(0.11608835273895,-0.987363721603576,0.107872033537397));
#80624=DIRECTION('ref_axis',(0.642962649087655,-0.00807590594756614,-0.765854954688753));
#80625=DIRECTION('center_axis',(-0.129603838858782,-0.987363722017638,-0.0911905992772433));
#80626=DIRECTION('ref_axis',(0.582025902704371,-0.00129577722766678,-0.813169213351402));
#80627=DIRECTION('center_axis',(-0.130999516830708,0.987363722332075,-0.0891740231943745));
#80628=DIRECTION('ref_axis',(0.60769194540039,0.00890473868257953,-0.794122915627351));
#80629=DIRECTION('',(0.963190309714462,0.,-0.268820436857317));
#80630=DIRECTION('center_axis',(0.135303108987166,0.987363722411206,0.0824981718869856));
#80631=DIRECTION('ref_axis',(0.396894927700357,0.0222802155771096,-0.917593596511858));
#80632=DIRECTION('',(0.268820435286404,0.,0.963190310152894));
#80633=DIRECTION('center_axis',(0.,-1.,0.));
#80634=DIRECTION('ref_axis',(0.,0.,-1.));
#80635=DIRECTION('center_axis',(0.136563571924955,-0.987363721660594,0.0803944772458867));
#80636=DIRECTION('ref_axis',(0.463294363871762,-0.00807590150730855,-0.886167654690411));
#80637=DIRECTION('center_axis',(-0.146177057117807,-0.987363722025451,-0.0611976176041577));
#80638=DIRECTION('ref_axis',(0.393611115932371,-0.0012957790850932,-0.919276133907019));
#80639=DIRECTION('center_axis',(-0.147106599459718,0.987363722334265,-0.058928161464812));
#80640=DIRECTION('ref_axis',(0.422771490401496,0.00890473699170785,-0.906192569249388));
#80641=DIRECTION('',(0.882883007870352,0.,-0.469593009332337));
#80642=DIRECTION('center_axis',(0.149874467126569,0.987363722530107,0.0514832354754118));
#80643=DIRECTION('ref_axis',(0.190360243209039,0.0222802096345352,-0.981461446040565));
#80644=DIRECTION('',(0.469593007892378,-7.4805248730079E-15,0.882883008636246));
#80645=DIRECTION('center_axis',(5.55615891691316E-15,-1.,-2.91672738458947E-14));
#80646=DIRECTION('ref_axis',(-1.32900262527756E-31,2.91672738458947E-14,
-1.));
#80647=DIRECTION('center_axis',(0.150653224989841,-0.987363721911679,0.0491577710324375));
#80648=DIRECTION('ref_axis',(0.26196294939556,-0.0080759051180692,-0.965044140389704));
#80649=DIRECTION('center_axis',(-0.155915196790453,-0.987363722007203,-0.0283431098131091));
#80650=DIRECTION('ref_axis',(0.186791512180786,-0.00129577424341934,-0.982398723506055));
#80651=DIRECTION('center_axis',(-0.156335141249754,0.987363722339936,-0.0259268859959211));
#80652=DIRECTION('ref_axis',(0.218082714256815,0.0089047345844343,-0.975889663560569));
#80653=DIRECTION('',(0.761293077687916,0.,-0.648407934763649));
#80654=DIRECTION('',(0.648407931855868,0.,0.761293080164529));
#80655=DIRECTION('',(0.604105932750183,0.,-0.796904023089375));
#80656=DIRECTION('center_axis',(0.157639632770391,0.98736372244931,-0.0162057326603608));
#80657=DIRECTION('ref_axis',(-0.239338686253989,0.022280213284518,-0.970680475418256));
#80658=DIRECTION('',(0.796904023488083,-8.72727902989815E-15,0.60410593222423));
#80659=DIRECTION('center_axis',(3.60219357573548E-15,-1.,1.44022356936135E-14));
#80660=DIRECTION('ref_axis',(1.45198767877956E-32,-1.44022356936135E-14,
-1.));
#80661=DIRECTION('center_axis',(0.157369977048825,-0.987363721673261,-0.0186432681464133));
#80662=DIRECTION('ref_axis',(-0.16746038604,-0.00807590017643478,-0.985845727760523));
#80663=DIRECTION('center_axis',(-0.153405762942724,-0.987363721993325,0.039743582971959));
#80664=DIRECTION('ref_axis',(-0.242971131641253,-0.00129577523006141,-0.970032654169705));
#80665=DIRECTION('center_axis',(-0.152772346323586,0.987363722329941,0.0421128249533245));
#80666=DIRECTION('ref_axis',(-0.211838925404961,0.00890474194803155,-0.977264025355538));
#80667=DIRECTION('',(0.418671461608696,0.,-0.908137768862433));
#80668=DIRECTION('center_axis',(0.150470352701532,0.987363722429834,-0.0497147119812497));
#80669=DIRECTION('ref_axis',(-0.442410689753908,0.0222802142789809,-0.896535762612487));
#80670=DIRECTION('',(0.908137769272627,0.,0.418671460718947));
#80671=DIRECTION('center_axis',(3.30701562051688E-14,-1.,6.64557714523879E-14));
#80672=DIRECTION('ref_axis',(5.24569482125142E-31,-6.6455771452388E-14,
-1.));
#80673=DIRECTION('center_axis',(0.1496830060805,-0.987363721564142,-0.0520372849955869));
#80674=DIRECTION('ref_axis',(-0.375472943297379,-0.00807590774965808,-0.926798170350817));
#80675=DIRECTION('center_axis',(-0.141275524388632,-0.987363722030693,0.0717921069924385));
#80676=DIRECTION('ref_axis',(-0.445818949253545,-0.0012957780307353,-0.895122218161163));
#80677=DIRECTION('center_axis',(-0.140147603738348,0.987363722333552,0.0739697842773073));
#80678=DIRECTION('ref_axis',(-0.41696912465906,0.00890473688020523,-0.908877029494173));
#80679=DIRECTION('',(0.21366037648181,0.,-0.976908001564964));
#80680=DIRECTION('center_axis',(0.136265245926737,0.987363722431167,-0.0808990876301783));
#80681=DIRECTION('ref_axis',(-0.624796061376071,0.0222802142679187,-0.780470033852117));
#80682=DIRECTION('',(0.976908000747675,0.,0.213660380218656));
#80683=DIRECTION('center_axis',(4.65830207759487E-14,-1.,5.77929664104324E-14));
#80684=DIRECTION('ref_axis',(1.2425862598362E-30,-5.77929664104324E-14,
-1.));
#80685=DIRECTION('center_axis',(0.134997021497864,-0.987363721572367,-0.0829981054571122));
#80686=DIRECTION('ref_axis',(-0.565928805917978,-0.00807590600271466,-0.824414559778323));
#80687=DIRECTION('center_axis',(-0.122539404214696,-0.987363722008594,0.100483704529859));
#80688=DIRECTION('ref_axis',(-0.627820766522833,-0.00129577208819613,-0.778356862947439));
#80689=DIRECTION('center_axis',(-0.120969711832747,0.987363722336905,0.102368005900832));
#80690=DIRECTION('ref_axis',(-0.602602313497365,0.00890473952221489,-0.797991953206087));
#80691=DIRECTION('',(-0.00134122641154887,0.,-0.999999100555452));
#80692=DIRECTION('center_axis',(0.115688527292004,0.987363722456973,-0.108300712042521));
#80693=DIRECTION('ref_axis',(-0.777966662680144,0.0222802135997342,-0.627910394754115));
#80694=DIRECTION('',(0.99999910056149,0.,-0.00134122190964533));
#80695=DIRECTION('center_axis',(-6.95012580428984E-14,-1.,-5.57133917663028E-14));
#80696=DIRECTION('ref_axis',(1.,-6.95012580428984E-14,1.85482578544888E-31));
#80697=DIRECTION('center_axis',(0.113998724849479,-0.987363721657277,-0.110078026362143));
#80698=DIRECTION('ref_axis',(-0.729922464896629,-0.00807590335540471,-0.683482241923097));
#80699=DIRECTION('center_axis',(-0.0980734700468536,-0.987363722015549,
0.124476804749198));
#80700=DIRECTION('ref_axis',(-0.78046638447579,-0.00129577794930648,-0.625196404070588));
#80701=DIRECTION('center_axis',(-0.0961354113899496,0.987363722329988,0.125979611459777));
#80702=DIRECTION('ref_axis',(-0.760058487094582,0.00890474036853936,-0.649793660937427));
#80703=DIRECTION('',(-0.216280117331432,0.,-0.976331352998101));
#80704=DIRECTION('center_axis',(0.0897023422704652,0.987363722433392,-0.130638315258841));
#80705=DIRECTION('ref_axis',(-0.894760409380084,0.0222802141144841,-0.445990360731033));
#80706=DIRECTION('',(0.976331353957897,0.,-0.216280112998722));
#80707=DIRECTION('center_axis',(0.,-1.,0.));
#80708=DIRECTION('ref_axis',(0.,0.,-1.));
#80709=DIRECTION('center_axis',(0.087669977412081,-0.987363721614985,-0.132010818871684));
#80710=DIRECTION('ref_axis',(-0.859785762310091,-0.00807590481960915,-0.510591052301351));
#80711=DIRECTION('center_axis',(-0.0690217288581476,-0.987363722016549,
0.142649505400682));
#80712=DIRECTION('ref_axis',(-0.896618260249722,-0.00129578297260527,-0.442802457460716));
#80713=DIRECTION('center_axis',(-0.0668059282075274,0.987363722329631,0.143700549002799));
#80714=DIRECTION('ref_axis',(-0.881975171793268,0.00890473817595887,-0.471211737946173));
#80715=DIRECTION('',(-0.421105986980058,0.,-0.907011437485521));
#80716=DIRECTION('center_axis',(0.0595217777845465,0.987363722389193,-0.146867415307565));
#80717=DIRECTION('ref_axis',(-0.969716151761567,0.0222802164264929,-0.243216317233707));
#80718=DIRECTION('',(0.907011438172321,0.,-0.421105985500774));
#80719=DIRECTION('center_axis',(1.44118465794018E-14,-1.,3.56354735319859E-15));
#80720=DIRECTION('ref_axis',(1.,1.44118465794018E-14,-4.86129465338419E-32));
#80721=DIRECTION('center_axis',(0.0572418778963929,-0.987363721629328,-0.147770932950893));
#80722=DIRECTION('ref_axis',(-0.949446432501417,-0.00807590462824617,-0.313825192702509));
#80723=DIRECTION('center_axis',(-0.0367426193502507,-0.987363722021711,
0.154152068940755));
#80724=DIRECTION('ref_axis',(-0.970845262562338,-0.00129577570246486,-0.239703560936405));
#80725=DIRECTION('center_axis',(-0.0343526754374338,0.987363722316262,0.154702209241063));
#80726=DIRECTION('ref_axis',(-0.96265167765723,0.00890473481807808,-0.270596476698312));
#80727=DIRECTION('',(-0.606241413488836,0.,-0.795280672826304));
#80728=DIRECTION('center_axis',(0.0265580410445182,0.987363722324339,-0.156229159550013));
#80729=DIRECTION('ref_axis',(-0.999329045759756,0.0222802188112533,-0.0290697463115691));
#80730=DIRECTION('',(0.795280674871624,0.,-0.60624141080574));
#80731=DIRECTION('center_axis',(-5.93638519600052E-14,-1.,-1.52845037480549E-15));
#80732=DIRECTION('ref_axis',(-0.999668706664393,5.9383525325444E-14,-0.025738626924135));
#80733=DIRECTION('center_axis',(0.0241372132342312,-0.987363721571971,-0.156621442532088));
#80734=DIRECTION('ref_axis',(-0.994712042298421,-0.00807590568879488,-0.102385216969101));
#80735=DIRECTION('center_axis',(-0.00274545648193553,-0.987363722011253,
0.158446656401424));
#80736=DIRECTION('ref_axis',(-0.99967661984729,-0.00129577844027622,-0.0253963912580066));
#80737=DIRECTION('center_axis',(-0.000293120077989504,0.987363722326222,
0.158470167270459));
#80738=DIRECTION('ref_axis',(-0.998315660024052,0.0089047418167306,-0.0573284268397376));
#80739=DIRECTION('',(-0.763029661124908,0.,-0.646363470690918));
#80740=DIRECTION('center_axis',(-0.00764752348920133,0.987363722381642,
-0.158285801982208));
#80741=DIRECTION('ref_axis',(-0.982214424081302,0.0222802177426303,0.18643609367281));
#80742=DIRECTION('',(0.646363471935383,0.,-0.76302966007072));
#80743=DIRECTION('center_axis',(0.,-1.,0.));
#80744=DIRECTION('ref_axis',(0.,0.,-1.));
#80745=DIRECTION('center_axis',(-0.010096086717736,-0.98736372167545,-0.158148506639151));
#80746=DIRECTION('ref_axis',(-0.993466022793342,-0.00807590057927945,0.113842177531057));
#80747=DIRECTION('center_axis',(0.0313800754379938,-0.98736372201349,0.155332454165809));
#80748=DIRECTION('ref_axis',(-0.981764209494793,-0.00129577561140111,0.190098284896603));
#80749=DIRECTION('center_axis',(0.033780129177532,0.98736372232979,0.15482823611929));
#80750=DIRECTION('ref_axis',(-0.987299512398128,0.0089047368247926,0.158620233515461));
#80751=DIRECTION('',(-0.884139492153183,0.,-0.467223028558216));
#80752=DIRECTION('center_axis',(-0.0414954970019995,0.987363722357152,-0.152941176605865));
#80753=DIRECTION('ref_axis',(-0.919172548808744,0.0222802174733878,0.393224385593997));
#80754=DIRECTION('',(0.46722303224745,0.,-0.884139490203609));
#80755=DIRECTION('center_axis',(0.0662738630982185,0.987363722324091,0.143946708570755));
#80756=DIRECTION('ref_axis',(-0.930118336104512,0.00890473695795505,0.367151993732682));
#80757=DIRECTION('',(-0.963907941868057,0.,-0.266235759438296));
#80758=DIRECTION('center_axis',(-5.45189523126693E-14,-1.,2.35390503939764E-14));
#80759=DIRECTION('ref_axis',(1.,-5.45189523126693E-14,-2.16299130535504E-31));
#80760=DIRECTION('center_axis',(-0.0438572997935655,-0.98736372164247,-0.152280722480383));
#80761=DIRECTION('ref_axis',(-0.945766635917038,-0.00807590093282602,0.324746439873159));
#80762=DIRECTION('center_axis',(0.0640383176205965,-0.987363721999432,0.144955077026479));
#80763=DIRECTION('ref_axis',(-0.917945595484297,-0.00129578079888721,0.396704177798899));
#80764=DIRECTION('',(0.266235760272643,0.,-0.963907941637607));
#80765=DIRECTION('center_axis',(-0.0734031917968273,0.987363722454611,-0.140445188648852));
#80766=DIRECTION('ref_axis',(-0.813151184179084,0.0222802126576441,0.581625948348321));
#80767=DIRECTION('center_axis',(4.81841295761272E-14,-1.,-3.47086837216053E-14));
#80768=DIRECTION('ref_axis',(1.,4.81841295761272E-14,5.77589282990628E-31));
#80769=DIRECTION('center_axis',(0.0956687012153076,0.987363722323065,0.126334395348684));
#80770=DIRECTION('ref_axis',(-0.829445861762144,0.00890473335591326,0.558516130590259));
#80771=DIRECTION('center_axis',(-0.0755677892436326,-0.987363721569997,
-0.139292464104397));
#80772=DIRECTION('ref_axis',(-0.853844253208445,-0.00807590692743719,0.520465917222456));
#80773=DIRECTION('center_axis',(0.0937021908559942,-0.98736372201381,0.12779976478782));
#80774=DIRECTION('ref_axis',(-0.811204865945284,-0.00129577686847123,0.584760623186104));
#80775=DIRECTION('',(-0.998605128176721,0.,-0.0527996020738229));
#80776=DIRECTION('center_axis',(-0.101878629601441,0.987363722437774,-0.121382142197087));
#80777=DIRECTION('ref_axis',(-0.669107775438933,0.0222802132234434,0.742831324693487));
#80778=DIRECTION('',(0.0527996037021322,0.,-0.998605128090627));
#80779=DIRECTION('center_axis',(-7.919254080032E-14,-1.,8.85107550859449E-14));
#80780=DIRECTION('ref_axis',(1.42279732145531E-30,-8.85107550859449E-14,
-1.));
#80781=DIRECTION('center_axis',(-0.103744819083784,-0.98736372158572,-0.119791042276414));
#80782=DIRECTION('ref_axis',(-0.721997061657015,-0.00807590627316386,0.691848988361264));
#80783=DIRECTION('center_axis',(0.118984659539436,-0.987363722014648,0.104668673650071));
#80784=DIRECTION('ref_axis',(-0.666533097641615,-0.00129577999390995,0.745474312570514));
#80785=DIRECTION('center_axis',(0.120590183957815,0.987363722329175,0.102814820727838));
#80786=DIRECTION('ref_axis',(-0.689989418966709,0.008904738214755,0.723764676777825));
#80787=DIRECTION('',(-0.986608649014418,0.,0.163105406685201));
#80788=DIRECTION('center_axis',(-0.125590336384488,0.98736372244378,-0.0966434012687544));
#80789=DIRECTION('ref_axis',(-0.49377763077791,0.0222802131608028,0.869302734060387));
#80790=DIRECTION('',(-0.163105405539067,0.,-0.986608649203896));
#80791=DIRECTION('center_axis',(7.28923339660516E-15,-1.,-1.29331847617228E-14));
#80792=DIRECTION('ref_axis',(1.41536446124868E-31,1.29331847617228E-14,
-1.));
#80793=DIRECTION('center_axis',(-0.127070857216169,-0.987363721628838,-0.0946883227098194));
#80794=DIRECTION('ref_axis',(-0.556390090292438,-0.00807590370700494,0.830881969478029));
#80795=DIRECTION('center_axis',(0.138703533836467,-0.98736372199969,0.0766433961942858));
#80796=DIRECTION('ref_axis',(-0.490694984314965,-0.00129577725624227,0.871330450133265));
#80797=DIRECTION('center_axis',(0.13987299927364,0.987363722338545,0.0744877431794555));
#80798=DIRECTION('ref_axis',(-0.518269837796568,0.00890473716125946,0.85517079047779));
#80799=DIRECTION('',(-0.928479445093385,0.,0.371383790759748));
#80800=DIRECTION('center_axis',(-0.143429579074395,0.987363722494363,-0.0673857206581365));
#80801=DIRECTION('ref_axis',(-0.295358993677058,0.0222802112338344,0.955126513631284));
#80802=DIRECTION('',(-0.371383789246356,0.,-0.928479445698729));
#80803=DIRECTION('center_axis',(1.73542509762026E-14,-1.,-5.67911351432082E-14));
#80804=DIRECTION('ref_axis',(-1.36289230963929E-31,5.67911351432082E-14,
-1.));
#80805=DIRECTION('center_axis',(-0.144455201097379,-0.987363721622812,-0.0651580854466019));
#80806=DIRECTION('ref_axis',(-0.364766936905548,-0.00807590495895753,0.931063833203523));
#80807=DIRECTION('center_axis',(0.15193678627059,-0.987363722024951,0.0450343580702607));
#80808=DIRECTION('ref_axis',(-0.291912518475211,-0.00129577560950907,0.95644414500954));
#80809=DIRECTION('center_axis',(0.152615509258198,0.987363722350212,0.042677700507334));
#80810=DIRECTION('ref_axis',(-0.32231653707135,0.00890473778969789,0.946590067333917));
#80811=DIRECTION('',(-0.826935574625762,0.,0.562296679181339));
#80812=DIRECTION('center_axis',(-0.154562213002855,0.987363722452636,-0.0349771624940467));
#80813=DIRECTION('ref_axis',(-0.0831296955738956,0.0222802138641302,0.996289639504477));
#80814=DIRECTION('',(-0.562296676496723,0.,-0.826935576451237));
#80815=DIRECTION('center_axis',(5.92512864267629E-15,-1.,-7.3992551213235E-14));
#80816=DIRECTION('ref_axis',(1.32231659479589E-31,7.3992551213235E-14,-1.));
#80817=DIRECTION('center_axis',(-0.155084981226389,-0.987363721619744,-0.032581126856186));
#80818=DIRECTION('ref_axis',(-0.156087686465311,-0.00807590435685906,0.987710187202058));
#80819=DIRECTION('center_axis',(0.158065644439664,-0.987363722011343,0.0113195628794571));
#80820=DIRECTION('ref_axis',(-0.0794805468680407,-0.00129577465791448,0.996835575026089));
#80821=DIRECTION('center_axis',(0.158221887458208,0.987363722342132,0.00887209850323346));
#80822=DIRECTION('ref_axis',(-0.111292072300149,0.00890473567881247,0.993747845444522));
#80823=DIRECTION('',(-0.686725115900806,0.,0.726917199680283));
#80824=DIRECTION('',(0.760958224664095,0.,-0.648800878787991));
#80825=DIRECTION('center_axis',(0.158340241420988,-0.987363721978348,0.00642249700707894));
#80826=DIRECTION('ref_axis',(-0.182442184061493,-0.0228638555270408,0.982950707607106));
#80827=DIRECTION('',(0.470048751153951,0.,0.882640454283969));
#80828=DIRECTION('center_axis',(1.9393850192807E-14,-1.,-1.02095484779451E-13));
#80829=DIRECTION('ref_axis',(4.24799785959656E-31,1.02095484779451E-13,
-1.));
#80830=DIRECTION('center_axis',(0.151221680423885,0.98736372206301,0.0473802039216277));
#80831=DIRECTION('ref_axis',(-0.116574944043651,-0.0297836931839635,0.992735218495618));
#80832=DIRECTION('center_axis',(-0.155570611822151,0.987363722257103,-0.0301772216726333));
#80833=DIRECTION('ref_axis',(-0.187122270954565,0.000540286809661816,0.982336481966831));
#80834=DIRECTION('',(0.882640455447344,0.,-0.470048748969407));
#80835=DIRECTION('center_axis',(0.153257689134951,-0.987363721885547,0.0403108102788267));
#80836=DIRECTION('ref_axis',(-0.389482131659896,-0.022863859304535,0.920750190364013));
#80837=DIRECTION('',(0.269317664813194,0.,0.963051398119315));
#80838=DIRECTION('center_axis',(1.16822697290887E-14,-1.,-2.72969841571987E-14));
#80839=DIRECTION('ref_axis',(-4.67462342555635E-32,2.72969841571987E-14,
-1.));
#80840=DIRECTION('center_axis',(0.137500857422994,0.987363722012776,0.0787806744133277));
#80841=DIRECTION('ref_axis',(-0.327258211259482,-0.0297836958742307,0.944465454436167));
#80842=DIRECTION('center_axis',(-0.145446246378588,0.987363722270834,-0.0629147785330536));
#80843=DIRECTION('ref_axis',(-0.393920760901921,0.000540287765887657,0.919144244512025));
#80844=DIRECTION('',(0.963051398102499,0.,-0.269317664873326));
#80845=DIRECTION('center_axis',(0.141008974677269,-0.9873637219592,0.0723142421611428));
#80846=DIRECTION('ref_axis',(-0.578310330469618,-0.0228638554140194,0.815496416784113));
#80847=DIRECTION('',(0.055993585129981,0.,0.998431128533306));
#80848=DIRECTION('center_axis',(-5.18315684147911E-14,-1.,7.24423595823463E-14));
#80849=DIRECTION('ref_axis',(5.83498941382284E-31,-7.24423595823463E-14,
-1.));
#80850=DIRECTION('center_axis',(0.117350647804882,0.987363722042521,0.106497445293839));
#80851=DIRECTION('ref_axis',(-0.522639253324542,-0.0297836947345418,0.852033533619613));
#80852=DIRECTION('center_axis',(-0.128520974775072,0.987363722243296,-0.0927105120292627));
#80853=DIRECTION('ref_axis',(-0.582299955948521,0.000540290561766755,0.812973842991556));
#80854=DIRECTION('',(0.998431128681518,0.,-0.0559935824872008));
#80855=DIRECTION('center_axis',(0.122166839683711,-0.987363721945433,0.100936335715917));
#80856=DIRECTION('ref_axis',(-0.740097379992076,-0.0228638568074939,0.672110937405984));
#80857=DIRECTION('',(-0.159948692818663,0.,0.987125329259462));
#80858=DIRECTION('center_axis',(3.30963705216048E-14,-1.,-2.98032211797663E-14));
#80859=DIRECTION('ref_axis',(1.,3.30963705216048E-14,6.25159708608419E-31));
#80860=DIRECTION('center_axis',(0.0917132492495926,0.987363721931247,0.129234517549131));
#80861=DIRECTION('ref_axis',(-0.693582260141972,-0.0297836992689342,0.719761474152521));
#80862=DIRECTION('center_axis',(-0.105586206860168,0.98736372225967,-0.118171201595023));
#80863=DIRECTION('ref_axis',(-0.743451451729584,0.000540289541825534,0.66878968817438));
#80864=DIRECTION('',(0.9871253291959,0.,0.159948693210935));
#80865=DIRECTION('center_axis',(0.0976123117887723,-0.987363722077454,0.124838763661801));
#80866=DIRECTION('ref_axis',(-0.867278299557125,-0.0228638492548932,0.497298296311731));
#80867=DIRECTION('',(-0.368411947167087,0.,0.929662646977147));
#80868=DIRECTION('center_axis',(-3.87294073426819E-14,-1.,2.19916970886201E-14));
#80869=DIRECTION('ref_axis',(1.,-3.87294073426819E-14,-2.80400459788044E-31));
#80870=DIRECTION('center_axis',(0.0617874476087296,0.987363722074324,0.145928721126229));
#80871=DIRECTION('ref_axis',(-0.832094133351182,-0.0297836941084912,0.55383416724485));
#80872=DIRECTION('center_axis',(-0.0777143454300615,0.987363722242749,-0.138106337701498));
#80873=DIRECTION('ref_axis',(-0.869839983855047,0.000540288780145893,0.493333670627787));
#80874=DIRECTION('',(0.929662646609954,0.,0.368411948093674));
#80875=DIRECTION('center_axis',(0.0684935522830534,-0.987363721953246,0.14290386232108));
#80876=DIRECTION('ref_axis',(-0.953906248045583,-0.0228638555599683,0.299232541760637));
#80877=DIRECTION('',(-0.559648669545669,0.,0.8287299721114));
#80878=DIRECTION('center_axis',(-4.25515000991007E-14,-1.,1.31518656770642E-14));
#80879=DIRECTION('ref_axis',(1.,-4.25515000991007E-14,-9.27098447437634E-32));
#80880=DIRECTION('center_axis',(0.0289725294669247,0.987363722077741,0.155799463609725));
#80881=DIRECTION('ref_axis',(-0.931698210467539,-0.0297836942824951,0.362010187931876));
#80882=DIRECTION('center_axis',(-0.0462086544522591,0.987363722215039,-0.151583773232412));
#80883=DIRECTION('ref_axis',(-0.955555764032208,0.000540281349776698,0.294809921679862));
#80884=DIRECTION('',(0.828729971245935,0.,0.559648670827254));
#80885=DIRECTION('center_axis',(0.0361721042068151,-0.987363721965724,0.154286938602218));
#80886=DIRECTION('ref_axis',(-0.995930601319451,-0.0228638548777849,0.0871750049934288));
#80887=DIRECTION('',(-0.724716840964423,0.,0.689046805683437));
#80888=DIRECTION('center_axis',(5.91785760991902E-14,-1.,-4.92942355256591E-15));
#80889=DIRECTION('ref_axis',(1.,5.91785760991902E-14,1.20798325998743E-31));
#80890=DIRECTION('center_axis',(-0.00519711437170142,0.98736372197901,0.158385196662958));
#80891=DIRECTION('ref_axis',(-0.987737113176826,-0.0297836975432815,0.153259018050357));
#80892=DIRECTION('center_axis',(-0.0125422848273878,0.987363722246296,-0.157973323960879));
#80893=DIRECTION('ref_axis',(-0.996590820051855,0.000540287682197817,0.0825011847041714));
#80894=DIRECTION('',(0.68904680421877,0.,0.724716842357));
#80895=DIRECTION('center_axis',(0.00215929339199061,-0.987363721902053,
0.158455729223565));
#80896=DIRECTION('ref_axis',(-0.991386346590728,-0.0228638587196378,-0.128958736648343));
#80897=DIRECTION('',(-0.855898060460215,0.,0.517144573693317));
#80898=DIRECTION('center_axis',(2.94273471123754E-14,-1.,3.95373409499303E-15));
#80899=DIRECTION('ref_axis',(1.,2.94273471123754E-14,2.02742082198128E-32));
#80900=DIRECTION('center_axis',(-0.0391237393995077,0.987363722089514,0.153565013323152));
#80901=DIRECTION('ref_axis',(-0.997590527089144,-0.029783692692005,-0.0626583746328627));
#80902=DIRECTION('center_axis',(0.0217105382769153,0.987363722231686,-0.156976216505932));
#80903=DIRECTION('ref_axis',(-0.991026396674851,0.000540284273519458,-0.133665213075668));
#80904=DIRECTION('',(0.517144572474294,0.,0.855898061196764));
#80905=DIRECTION('center_axis',(-0.0319544928798145,-0.987363721986839,
0.155215304944744));
#80906=DIRECTION('ref_axis',(-0.940485968153084,-0.0228638532295288,-0.33906251329608));
#80907=DIRECTION('',(-0.947058436717489,0.,0.32106123628091));
#80908=DIRECTION('center_axis',(-5.57788322291163E-14,-1.,-2.03746154928163E-14));
#80909=DIRECTION('ref_axis',(1.,-5.57788322291163E-14,4.36823228791738E-31));
#80910=DIRECTION('center_axis',(-0.0712209830271485,0.987363722192202,0.141564302263692));
#80911=DIRECTION('ref_axis',(-0.96079771655334,-0.0297836888147394,-0.27564593185185));
#80912=DIRECTION('center_axis',(0.0549482066376669,0.987363722243729,-0.148639074890527));
#80913=DIRECTION('ref_axis',(-0.939122680647031,0.00054028684886553,-0.343581575152767));
#80914=DIRECTION('',(0.321061238918488,0.,0.947058435823326));
#80915=DIRECTION('center_axis',(-0.0645741168328686,-0.987363722016858,
0.144717185849752));
#80916=DIRECTION('ref_axis',(-0.845609510466505,-0.0228638535199251,-0.533312103754282));
#80917=DIRECTION('',(-0.993935411981185,0.,0.109965434613753));
#80918=DIRECTION('center_axis',(0.,-1.,0.));
#80919=DIRECTION('ref_axis',(0.,0.,-1.));
#80920=DIRECTION('center_axis',(-0.0999880255367153,0.987363721948417,0.122944195997362));
#80921=DIRECTION('ref_axis',(-0.879079071420455,-0.0297836993029511,-0.475744592661212));
#80922=DIRECTION('center_axis',(0.0856165537158678,0.987363722249874,-0.133351736826677));
#80923=DIRECTION('ref_axis',(-0.843306631655252,0.000540284728342988,-0.537432445148862));
#80924=DIRECTION('',(0.109965437515861,0.,0.993935411660106));
#80925=DIRECTION('center_axis',(-0.0941743252867184,-0.9873637219706,0.127452253778252));
#80926=DIRECTION('ref_axis',(-0.711193292549383,-0.0228638558648281,-0.702624611530054));
#80927=DIRECTION('',(-0.994337072346781,0.,-0.106272228530468));
#80928=DIRECTION('center_axis',(4.20684180271517E-14,-1.,4.19124239078833E-14));
#80929=DIRECTION('ref_axis',(1.,4.20684180271517E-14,1.15419787652154E-30));
#80930=DIRECTION('center_axis',(-0.124079726667146,0.987363722011638,0.0985753614527047));
#80931=DIRECTION('ref_axis',(-0.756255667861176,-0.0297836962498653,-0.653597962256265));
#80932=DIRECTION('center_axis',(0.11228156877962,0.98736372228335,-0.111829017840426));
#80933=DIRECTION('ref_axis',(-0.708058500491322,0.000540285967795188,-0.706153572513128));
#80934=DIRECTION('',(-0.106272228164584,0.,0.994337072385886));
#80935=DIRECTION('center_axis',(-0.119371047568695,-0.987363721916357,0.104227796896177));
#80936=DIRECTION('ref_axis',(-0.543522466694485,-0.0228638584411881,-0.839083173574303));
#80937=DIRECTION('',(-0.948244636544391,0.,-0.317540720640354));
#80938=DIRECTION('center_axis',(6.41498992470956E-14,-1.,9.99520022934591E-14));
#80939=DIRECTION('ref_axis',(-1.66109997065748E-30,-9.99520022934592E-14,
-1.));
#80940=DIRECTION('center_axis',(-0.142369599811967,0.987363722034372,0.069597251812215));
#80941=DIRECTION('ref_axis',(-0.598070588946222,-0.0297836950516744,-0.800889818980481));
#80942=DIRECTION('center_axis',(0.133696423493094,0.98736372226897,-0.0850772959861791));
#80943=DIRECTION('ref_axis',(-0.539702340761982,0.000540289765636053,-0.84185574266795));
#80944=DIRECTION('',(-0.317540722300475,0.,0.948244635988463));
#80945=DIRECTION('center_axis',(-0.13898611473656,-0.987363721915582,0.076129761299015));
#80946=DIRECTION('ref_axis',(-0.350437134000453,-0.0228638573645295,-0.936307139319125));
#80947=DIRECTION('',(-0.857813335121565,0.,-0.513961362446262));
#80948=DIRECTION('center_axis',(-2.57271152087778E-14,-1.,-6.96284450963471E-14));
#80949=DIRECTION('ref_axis',(2.11209165460069E-31,6.96284450963471E-14,
-1.));
#80950=DIRECTION('center_axis',(-0.154002428756816,0.987363722073544,0.0373648534063824));
#80951=DIRECTION('ref_axis',(-0.411920395828391,-0.0297836930004011,-0.910732957091067));
#80952=DIRECTION('center_axis',(0.148859778365135,0.987363722268598,-0.0543474593056635));
#80953=DIRECTION('ref_axis',(-0.346110301969915,0.000540287633313102,-0.938193672415012));
#80954=DIRECTION('',(-0.513961362392703,0.,0.857813335153655));
#80955=DIRECTION('center_axis',(-0.152102345152299,-0.987363721974116,0.0444719813882001));
#80956=DIRECTION('ref_axis',(-0.140965751559213,-0.022863855048196,-0.989750423601668));
#80957=DIRECTION('',(-0.727271635232519,0.,-0.686349742176842));
#80958=DIRECTION('center_axis',(-1.42206008573881E-14,-1.,-1.0294359583756E-13));
#80959=DIRECTION('ref_axis',(2.37051675250879E-31,1.0294359583756E-13,-1.));
#80960=DIRECTION('center_axis',(-0.158434276437426,0.987363722091202,0.00338531356859956));
#80961=DIRECTION('ref_axis',(-0.206509259301968,-0.029783693097487,-0.977991235874855));
#80962=DIRECTION('center_axis',(0.157062616400018,0.987363722260677,-0.0210763965876856));
#80963=DIRECTION('ref_axis',(-0.1363345302832,0.000540285074681563,-0.990662709475075));
#80964=DIRECTION('',(-0.686349742131425,0.,0.727271635275381));
#80965=DIRECTION('center_axis',(-0.158106438275909,-0.987363721978957,0.0107347424546262));
#80966=DIRECTION('ref_axis',(0.0750970332009502,-0.0228638543459592,-0.996914078428458));
#80967=DIRECTION('',(-0.562723523285499,0.,-0.826645169550488));
#80968=DIRECTION('center_axis',(1.17738557350016E-15,-1.,-1.47991200996898E-14));
#80969=DIRECTION('ref_axis',(4.53712827619466E-33,1.47991200996898E-14,
-1.));
#80970=DIRECTION('center_axis',(-0.15545791360717,0.987363722140864,-0.030752516922108));
#80971=DIRECTION('ref_axis',(0.00855801734471834,-0.0297836909058287,-0.999519730718285));
#80972=DIRECTION('center_axis',(0.157921382458744,0.987363722227175,0.0131801742028564));
#80973=DIRECTION('ref_axis',(0.0798160940080673,0.000540281567541906,-0.996809459843316));
#80974=DIRECTION('',(-0.826645169515347,0.,0.562723523337121));
#80975=DIRECTION('center_axis',(-0.156717651053432,-0.987363721910341,-0.0235044358292781));
#80976=DIRECTION('ref_axis',(0.287648364605956,-0.0228638592072449,-0.957463138863147));
#80977=DIRECTION('',(-0.37186308447585,0.,-0.928287588198887));
#80978=DIRECTION('center_axis',(-8.66246462967909E-15,-1.,2.84000436037034E-14));
#80979=DIRECTION('ref_axis',(-7.27882089572718E-32,-2.84000436037034E-14,
-1.));
#80980=DIRECTION('center_axis',(-0.145212510328833,0.987363722018922,-0.0634524017271248));
#80981=DIRECTION('ref_axis',(0.223225132689914,-0.0297836965305611,-0.974311793809634));
#80982=DIRECTION('center_axis',(0.151395919725379,0.987363722225758,0.0468204605167725));
#80983=DIRECTION('ref_axis',(0.292234606692641,0.000540284026219369,-0.95634650767615));
#80984=DIRECTION('',(-0.928287587778145,0.,0.371863085526155));
#80985=DIRECTION('center_axis',(-0.148000920052496,-0.987363721900531,-0.0566445790728921));
#80986=DIRECTION('ref_axis',(0.486749578565709,-0.0228638577531011,-0.873242286982685));
#80987=DIRECTION('',(-0.163614740740223,0.,-0.986524311212101));
#80988=DIRECTION('center_axis',(-2.18476663765354E-14,-1.,3.88108388533404E-14));
#80989=DIRECTION('ref_axis',(-2.37202458671487E-31,-3.88108388533404E-14,
-1.));
#80990=DIRECTION('center_axis',(-0.128177133113144,0.987363722071159,-0.0931853147479977));
#80991=DIRECTION('ref_axis',(0.427454489836029,-0.0297836935546327,-0.903546119861772));
#80992=DIRECTION('center_axis',(0.137791350316563,0.987363722237745,0.0782714749239015));
#80993=DIRECTION('ref_axis',(0.490988553554454,0.0005402878828289,-0.871165855832004));
#80994=DIRECTION('',(-0.986524311201882,0.,0.163614740801838));
#80995=DIRECTION('center_axis',(-0.132363832496354,-0.987363721865011,-0.0871360808835846));
#80996=DIRECTION('ref_axis',(0.663090921521998,-0.0228638604900558,-0.74818959741405));
#80997=DIRECTION('',(0.0522840469698041,0.,-0.998632253851466));
#80998=DIRECTION('center_axis',(9.89335438426233E-15,-1.,-1.10689535020008E-14));
#80999=DIRECTION('ref_axis',(-2.42855846616023E-31,1.10689535020008E-14,
-1.));
#81000=DIRECTION('center_axis',(-0.105148334450947,0.987363722064401,-0.118560989002812));
#81001=DIRECTION('ref_axis',(0.611696547757108,-0.0297836942674327,-0.790531634419408));
#81002=DIRECTION('center_axis',(0.117743810833585,0.987363722264892,0.106062599277983));
#81003=DIRECTION('ref_axis',(0.666784422275534,0.000540288842422262,-0.745250456087515));
#81004=DIRECTION('',(-0.99863225400483,0.,-0.0522840440405324));
#81005=DIRECTION('center_axis',(-0.110537553796009,-0.987363721965769,-0.113553202274082));
#81006=DIRECTION('ref_axis',(0.808426872685382,-0.022863855483925,-0.588152391504569));
#81007=DIRECTION('',(0.265738088458527,0.,-0.964045262600469));
#81008=DIRECTION('center_axis',(1.20415510587402E-14,-1.,-8.68338877012913E-15));
#81009=DIRECTION('ref_axis',(1.,1.20415510587402E-14,1.22739341060735E-31));
#81010=DIRECTION('center_axis',(-0.0772029162671188,0.987363722049365,-0.13839288312871));
#81011=DIRECTION('ref_axis',(0.767336357098404,-0.0297836946635119,-0.640552766450307));
#81012=DIRECTION('center_axis',(0.0921907025089084,0.987363722255374,0.128894353425302));
#81013=DIRECTION('ref_axis',(0.811402191745447,0.000540288608632149,-0.584487973630685));
#81014=DIRECTION('',(-0.964045262617061,0.,-0.265738088398336));
#81015=DIRECTION('center_axis',(-0.0835426669511802,-0.987363721945072,
-0.134660697255953));
#81016=DIRECTION('ref_axis',(0.915961679953268,-0.0228638572586547,-0.400613835118612));
#81017=DIRECTION('',(0.466766516185184,0.,-0.884380585137613));
#81018=DIRECTION('center_axis',(4.08800946221569E-14,-1.,-1.76753953209365E-14));
#81019=DIRECTION('ref_axis',(1.,4.08800946221569E-14,-2.74904545746926E-32));
#81020=DIRECTION('center_axis',(-0.045647575810467,0.987363722013861,-0.151753679604688));
#81021=DIRECTION('ref_axis',(0.887096369051805,-0.0297836951534783,-0.460622365412393));
#81022=DIRECTION('center_axis',(0.0623268615180566,0.987363722252623,0.14569915000697));
#81023=DIRECTION('ref_axis',(0.918079696437692,0.000540286067284419,-0.396395483172854));
#81024=DIRECTION('',(-0.884380585166462,0.,-0.466766516130523));
#81025=DIRECTION('center_axis',(-0.0526414158310298,-0.987363721922956,
-0.149471609243201));
#81026=DIRECTION('ref_axis',(0.980667137396743,-0.0228638565726862,-0.1943430206946));
#81027=DIRECTION('',(0.645969457690815,0.,-0.763363255423415));
#81028=DIRECTION('center_axis',(0.,-1.,0.));
#81029=DIRECTION('ref_axis',(0.,0.,-1.));
#81030=DIRECTION('center_axis',(-0.011957812984655,0.987363722205697,-0.158018640611592));
#81031=DIRECTION('ref_axis',(0.965376741456017,-0.0297836876240715,-0.259153774827367));
#81032=DIRECTION('center_axis',(0.0295486796979486,0.987363722245942,0.155691218508769));
#81033=DIRECTION('ref_axis',(0.981828814775111,0.00054029026758487,-0.189767980870663));
#81034=DIRECTION('',(-0.763363255462685,0.,-0.645969457644409));
#81035=DIRECTION('center_axis',(-0.0192787124909096,-0.987363721914727,
-0.157293394303103));
#81036=DIRECTION('ref_axis',(0.999517689362401,-0.0228638579857241,0.021015057688609));
#81037=DIRECTION('',(0.794967585437563,0.,-0.606651908513911));
#81038=DIRECTION('center_axis',(0.,-1.,0.));
#81039=DIRECTION('ref_axis',(0.,0.,-1.));
#81040=DIRECTION('center_axis',(0.0222910985942386,0.987363722043707,-0.156894828835942));
#81041=DIRECTION('ref_axis',(0.998517170574893,-0.0297836953944212,-0.0455674396445725));
#81042=DIRECTION('center_axis',(-0.00461116002007661,0.987363722279684,
0.15840333686282));
#81043=DIRECTION('ref_axis',(0.999668709074289,0.00054028841285584,0.0257328619895947));
#81044=DIRECTION('',(-0.606651908563567,0.,-0.79496758539967));
#81045=DIRECTION('center_axis',(0.0149854418475902,-0.987363721860772,-0.157760315941228));
#81046=DIRECTION('ref_axis',(0.971631905064919,-0.0228638594886714,0.23539049468744));
#81047=DIRECTION('',(0.906793913166479,0.,-0.421574191624944));
#81048=DIRECTION('center_axis',(1.44136844525623E-14,-1.,3.55610651202243E-15));
#81049=DIRECTION('ref_axis',(1.,1.44136844525623E-14,-5.50471133143517E-32));
#81050=DIRECTION('center_axis',(0.0554976904766439,0.987363722124659,-0.148434788994693));
#81051=DIRECTION('ref_axis',(0.984968046763139,-0.0297836901696709,0.170149577300337));
#81052=DIRECTION('center_axis',(-0.0385553889347902,0.987363722263352,0.153708691824324));
#81053=DIRECTION('ref_axis',(0.970765205310708,0.000540288479386633,0.240030465246431));
#81054=DIRECTION('',(-0.421574190582567,0.,-0.906793913651086));
#81055=DIRECTION('center_axis',(0.048548891846868,-0.987363721815495,-0.150850541739481));
#81056=DIRECTION('ref_axis',(0.898313693186332,-0.0228638628925394,0.438759333128726));
#81057=DIRECTION('',(0.976219564475212,0.,-0.216784136725517));
#81058=DIRECTION('center_axis',(1.33122427314128E-14,-1.,6.57148280683985E-15));
#81059=DIRECTION('ref_axis',(1.,1.33122427314128E-14,-8.34320862855221E-32));
#81060=DIRECTION('center_axis',(0.0861092826875015,0.987363721992229,-0.133034100623476));
#81061=DIRECTION('ref_axis',(0.925362911146449,-0.0297836960963146,0.377910590115454));
#81062=DIRECTION('center_axis',(-0.0706968106702072,0.987363722284384,0.141826798870266));
#81063=DIRECTION('ref_axis',(0.896469799427748,0.000540288698301344,0.443104510022292));
#81064=DIRECTION('',(-0.216784133438348,0.,-0.976219565205177));
#81065=DIRECTION('center_axis',(0.0798422585918534,-0.987363721936398,-0.136887159174463));
#81066=DIRECTION('ref_axis',(0.78299133001524,-0.0228638563166837,0.621612275615029));
#81067=DIRECTION('',(0.999998274855759,0.,-0.00185749441591979));
#81068=DIRECTION('center_axis',(-5.79416767742965E-14,-1.,-4.63979194031601E-14));
#81069=DIRECTION('ref_axis',(1.,-5.79416767742965E-14,-8.87442181665929E-32));
#81070=DIRECTION('center_axis',(0.11269449223574,0.987363722076581,-0.111412888602755));
#81071=DIRECTION('ref_axis',(0.822488835150569,-0.0297836931952023,0.568000922246007));
#81072=DIRECTION('center_axis',(-0.0995325279600817,0.987363722252021,0.123313242835106));
#81073=DIRECTION('ref_axis',(0.780256462409246,0.000540288674050379,0.625459479868007));
#81074=DIRECTION('',(-0.00185749160357402,0.,-0.999998274860983));
#81075=DIRECTION('center_axis',(0.107402284445999,-0.987363721972997,-0.116523087100419));
#81076=DIRECTION('ref_axis',(0.631057164088596,-0.022863855066005,0.775399316342218));
#81077=DIRECTION('',(0.977018176875493,0.,0.213156004031993));
#81078=DIRECTION('center_axis',(-9.3225702735687E-15,-1.,-1.15537819071333E-14));
#81079=DIRECTION('ref_axis',(-1.02932978610097E-31,1.15537819071333E-14,
-1.));
#81080=DIRECTION('center_axis',(0.134010238812352,0.987363721952771,-0.084582128520313));
#81081=DIRECTION('ref_axis',(0.681156094834938,-0.0297836985911217,0.731532163180438));
#81082=DIRECTION('center_axis',(-0.123714212040058,0.987363722232974,0.0990337001103841));
#81083=DIRECTION('ref_axis',(0.627559201727512,0.000540284264199704,0.778568658770722));
#81084=DIRECTION('',(0.213156003970963,0.,-0.977018176888808));
#81085=DIRECTION('center_axis',(0.129940297562282,-0.987363721916974,-0.0907105270169139));
#81086=DIRECTION('ref_axis',(0.449615466022523,-0.0228638564463816,0.892929547490589));
#81087=DIRECTION('',(0.908353794958554,0.,0.41820256238382));
#81088=DIRECTION('center_axis',(0.,-1.,0.));
#81089=DIRECTION('ref_axis',(0.,0.,-1.));
#81090=DIRECTION('center_axis',(0.14905980749689,0.987363722127537,-0.053796412663352));
#81091=DIRECTION('ref_axis',(0.507973253116063,-0.0297836902908456,0.860857773335029));
#81092=DIRECTION('center_axis',(-0.142111161646279,0.987363722248888,0.0701234463098179));
#81093=DIRECTION('ref_axis',(0.445517968814157,0.000540286778625937,0.895272834142701));
#81094=DIRECTION('',(0.418202564699209,0.,-0.908353793892558));
#81095=DIRECTION('center_axis',(0.146402447495151,-0.987363721952896,-0.0606564418570101));
#81096=DIRECTION('ref_axis',(0.247150249152909,-0.0228638558610294,0.96870738535371));
#81097=DIRECTION('',(0.797215799077901,0.,0.603694434048041));
#81098=DIRECTION('center_axis',(-2.16577711357467E-14,-1.,-8.64022447059934E-14));
#81099=DIRECTION('ref_axis',(2.81888937165628E-31,8.64022447059934E-14,
-1.));
#81100=DIRECTION('center_axis',(0.157139511605707,0.987363722043768,-0.0204952258879351));
#81101=DIRECTION('ref_axis',(0.311038146206098,-0.0297836945747142,0.949930630700028));
#81102=DIRECTION('center_axis',(-0.153863149848971,0.987363722253108,0.0379342997436371));
#81103=DIRECTION('ref_axis',(0.242644810113474,0.000540287020636909,0.970115046896465));
#81104=DIRECTION('',(0.603694433998265,0.,-0.797215799115594));
#81105=DIRECTION('center_axis',(0.15601898153659,-0.987363721893832,-0.0277661320360645));
#81106=DIRECTION('ref_axis',(0.0331285598677343,-0.0228638586816274,0.999189542823221));
#81107=DIRECTION('',(0.648800877075795,0.,0.760958226123931));
#81108=DIRECTION('center_axis',(3.00707855221535E-15,-1.,1.03877653670037E-13));
#81109=DIRECTION('ref_axis',(0.0289361498648771,1.03921169418994E-13,0.999581261944719));
#81110=DIRECTION('center_axis',(0.157871544748138,0.987363722095124,0.0137642889136518));
#81111=DIRECTION('ref_axis',(0.0995592420306967,-0.0297836924791192,0.994585787646587));
#81112=DIRECTION('center_axis',(-0.158420668071144,0.987363722255966,0.003971385241346));
#81113=DIRECTION('ref_axis',(0.0284258509567777,0.000540289709918792,0.999595757836343));
#81114=DIRECTION('center_axis',(-0.163746583102855,-0.986495110327124,-0.00380181835644106));
#81115=DIRECTION('ref_axis',(0.0270297015237054,-0.00833893471375523,0.999599848641135));
#81116=DIRECTION('center_axis',(0.161203610189502,-0.986495108559966,-0.0289964971872927));
#81117=DIRECTION('ref_axis',(0.137709438928237,-0.00660960175535,0.990450616434109));
#81118=DIRECTION('center_axis',(-0.160735582317879,-0.986495108181465,0.0314876818926446));
#81119=DIRECTION('ref_axis',(0.241282154885155,-0.00833899447686017,0.970419178966023));
#81120=DIRECTION('center_axis',(0.151201369427675,-0.986495108577346,-0.0629725863861876));
#81121=DIRECTION('ref_axis',(0.347407475820122,-0.00660960159429159,0.937690971968407));
#81122=DIRECTION('center_axis',(-0.150208754328077,-0.986495108142209,0.0653049135570864));
#81123=DIRECTION('ref_axis',(0.444252549571252,-0.00833899746620968,0.895862787105649));
#81124=DIRECTION('center_axis',(0.134129124742108,-0.986495108557985,-0.0940041418613364));
#81125=DIRECTION('ref_axis',(0.540861120534035,-0.00660959535685714,0.841085941829898));
#81126=DIRECTION('center_axis',(-0.132658332165123,-0.986495108139988,0.0960685615747535));
#81127=DIRECTION('ref_axis',(0.626450190063033,-0.0083389993819398,0.779416846404604));
#81128=DIRECTION('center_axis',(0.110785147588717,-0.986495108531098,-0.120640175389312));
#81129=DIRECTION('ref_axis',(0.709024704301451,-0.00660959663965462,0.705152665684886));
#81130=DIRECTION('center_axis',(-0.108904949677008,-0.986495108205661,0.122340154577923));
#81131=DIRECTION('ref_axis',(0.779355715649713,-0.00833899514876089,0.626526240187938));
#81132=DIRECTION('center_axis',(0.0822609720701449,-0.986495108556898,-0.141635211961534));
#81133=DIRECTION('ref_axis',(0.844035079541172,-0.00660960678430646,0.536247235519293));
#81134=DIRECTION('center_axis',(-0.0800592947095578,-0.986495108204483,
0.142891255223105));
#81135=DIRECTION('ref_axis',(0.895819434046711,-0.00833899422620221,0.444339963045781));
#81136=DIRECTION('center_axis',(0.0498903833975317,-0.986495108560805,-0.156007533247763));
#81137=DIRECTION('ref_axis',(0.939579312919432,-0.00660959500260434,0.342267480178513));
#81138=DIRECTION('center_axis',(-0.0474701574982248,-0.986495108181289,
0.156760918858883));
#81139=DIRECTION('ref_axis',(0.97039563113366,-0.00833899500264603,0.241376842797838));
#81140=DIRECTION('center_axis',(0.0151869637452026,-0.986495108589794,-0.163085121518218));
#81141=DIRECTION('ref_axis',(0.991189861386224,-0.00660959737962207,0.132283679672277));
#81142=DIRECTION('center_axis',(-0.0126613696933789,-0.986495108187851,
0.163300616162116));
#81143=DIRECTION('ref_axis',(0.999597206674059,-0.00833899686580644,0.027127210337405));
#81144=DIRECTION('center_axis',(-0.0202265838329378,-0.986495108564548,
-0.162537029887563));
#81145=DIRECTION('ref_axis',(0.996453473854886,-0.00660960148140599,-0.0838855625884892));
#81146=DIRECTION('center_axis',(0.0227394532200513,-0.986495108204774,0.162204558367835));
#81147=DIRECTION('ref_axis',(0.982058727938165,-0.00833899493008264,-0.188390859767746));
#81148=DIRECTION('center_axis',(-0.0546943527513138,-0.986495108539734,
-0.154388887567379));
#81149=DIRECTION('ref_axis',(0.955124029393475,-0.00660959983514798,-0.296132405631656));
#81150=DIRECTION('center_axis',(0.0570770025954627,-0.98649510820796,0.153523995702568));
#81151=DIRECTION('ref_axis',(0.918600274496498,-0.00833899512343136,-0.395099983365338));
#81152=DIRECTION('center_axis',(-0.0866046781089558,-0.986495108574079,
-0.139021690714295));
#81153=DIRECTION('ref_axis',(0.869134046575717,-0.00660960205580594,-0.494532427898903));
#81154=DIRECTION('center_axis',(0.0887457396431603,-0.986495110261855,0.137664778082992));
#81155=DIRECTION('ref_axis',(0.812189079529727,-0.00833893655201375,-0.583334690576377));
#81156=DIRECTION('center_axis',(-0.114465461008326,-0.986495108551733,-0.117153997113444));
#81157=DIRECTION('ref_axis',(0.742504322941052,-0.00660959950258174,-0.669808661938815));
#81158=DIRECTION('center_axis',(0.116264737375798,-0.986495108195593,0.11536859342604));
#81159=DIRECTION('ref_axis',(0.66780085302811,-0.00833899486530625,-0.744293276779768));
#81160=DIRECTION('center_axis',(-0.136973968593365,-0.986495108545222,-0.0898083111083468));
#81161=DIRECTION('ref_axis',(0.581155923333125,-0.00660960002778809,-0.813765387542562));
#81162=DIRECTION('center_axis',(0.138347370174825,-0.986495108190397,0.0876778574220828));
#81163=DIRECTION('ref_axis',(0.492186987026872,-0.00833899405968922,-0.870449556826518));
#81164=DIRECTION('center_axis',(-0.153077727573361,-0.986495108555823,-0.0582632827466133));
#81165=DIRECTION('ref_axis',(0.392633313565955,-0.00660960544614752,-0.919671351186969));
#81166=DIRECTION('center_axis',(0.153961032422214,-0.986495108170381,0.0558874051231136));
#81167=DIRECTION('ref_axis',(0.293559004575771,-0.00833899651873737,-0.955904583088471));
#81168=DIRECTION('center_axis',(-0.162023738619957,-0.98649510858625,-0.0239939337961682));
#81169=DIRECTION('ref_axis',(0.185751609571843,-0.0066096046717047,-0.982574502349595));
#81170=DIRECTION('center_axis',(0.162375649064777,-0.986495108153596,0.0214837189475607));
#81171=DIRECTION('ref_axis',(0.0812045315127966,-0.00833899735817754,-0.996662573384216));
#81172=DIRECTION('center_axis',(-0.163393695748669,-0.986495108696664,0.0113973991396275));
#81173=DIRECTION('ref_axis',(-0.0298156589858182,-0.00660965490275117,-0.999533560687838));
#81174=DIRECTION('center_axis',(0.163197761691683,-0.986495108100812,-0.0139245205300664));
#81175=DIRECTION('ref_axis',(-0.134946979285497,-0.00833900044466913,-0.990817729884414));
#81176=DIRECTION('center_axis',(-0.157123555131692,-0.986495108582043,0.0462556933412782));
#81177=DIRECTION('ref_axis',(-0.243988729791768,-0.00660960030427146,-0.969755542865529));
#81178=DIRECTION('center_axis',(0.156388927828435,-0.98649510813377,-0.0486816688376119));
#81179=DIRECTION('ref_axis',(-0.344788517321524,-0.00833899908727815,-0.938643350489123));
#81180=DIRECTION('center_axis',(-0.143506486861752,-0.986495108529812,0.0789511815956736));
#81181=DIRECTION('ref_axis',(-0.446753182602872,-0.0066096015307531,-0.894632833626069));
#81182=DIRECTION('center_axis',(0.142267519731386,-0.986495108183313,-0.0811625181957401));
#81183=DIRECTION('ref_axis',(-0.538508128428602,-0.00833899548032144,-0.842579050754707));
#81184=DIRECTION('center_axis',(-0.123179214736077,-0.986495108581144,0.107954998969391));
#81185=DIRECTION('ref_axis',(-0.628627956656191,-0.00660960084133648,-0.777678085898645));
#81186=DIRECTION('center_axis',(0.121493846397304,-0.986495108098356,-0.109848290772327));
#81187=DIRECTION('ref_axis',(-0.707047696569409,-0.00833900158626248,-0.707116691804428));
#81188=DIRECTION('center_axis',(-0.0970922211053125,-0.986495108544632,
0.131910960190395));
#81189=DIRECTION('ref_axis',(-0.781108784594513,-0.00660959905628847,-0.624359976159265));
#81190=DIRECTION('center_axis',(0.0950392464483762,-0.986495108205492,-0.133397687840383));
#81191=DIRECTION('ref_axis',(-0.842526501061776,-0.00833899471871473,-0.538590341702934));
#81192=DIRECTION('center_axis',(-0.0664652477252153,-0.986495108659401,
0.149698935987874));
#81193=DIRECTION('ref_axis',(-0.897065845627383,-0.00660965417426619,-0.441847463589557));
#81194=DIRECTION('center_axis',(0.0641407249323982,-0.986495108138676,-0.150709551865859));
#81195=DIRECTION('ref_axis',(-0.938609701908453,-0.00833899750784452,-0.344880107579271));
#81196=DIRECTION('center_axis',(-0.0327304788701568,-0.986495108642727,
0.160487122152853));
#81197=DIRECTION('ref_axis',(-0.971077088526604,-0.00660965631685087,-0.238674675200505));
#81198=DIRECTION('center_axis',(0.0302430527726786,-0.986495108131369,-0.160974406014955));
#81199=DIRECTION('ref_axis',(-0.990804557523789,-0.00833899897663459,-0.1350436591853));
#81200=DIRECTION('center_axis',(0.00253467411159349,-0.986495108531176,
0.16377110939116));
#81201=DIRECTION('ref_axis',(-0.999681845517634,-0.00660960532316903,-0.0243417513735121));
#81202=DIRECTION('center_axis',(-0.00506877383906692,-0.98649510953872,
-0.163712267066205));
#81203=DIRECTION('ref_axis',(-0.9966704924382,-0.00833897643643672,0.0811072806533985));
#81204=DIRECTION('center_axis',(0.0376813611748462,-0.986495108564858,0.159397351915329));
#81205=DIRECTION('ref_axis',(-0.981542596263219,-0.00660960394970318,0.19112939296845));
#81206=DIRECTION('center_axis',(-0.0401435546287142,-0.986495108250307,
-0.158795139787041));
#81207=DIRECTION('ref_axis',(-0.955933222817366,-0.00833899125541052,0.293465730092707));
#81208=DIRECTION('center_axis',(0.071066106982771,-0.986495108527701,0.14757035369353));
#81209=DIRECTION('ref_axis',(-0.917507506499398,-0.00660959972608852,0.397663537062072));
#81210=DIRECTION('center_axis',(-0.0733412770709218,-0.986495108148242,
-0.146452923074941));
#81211=DIRECTION('ref_axis',(-0.870497578451788,-0.00833899674706999,0.492102049419454));
#81212=DIRECTION('center_axis',(0.101127884369458,-0.986495108569774,0.128843128535705));
#81213=DIRECTION('ref_axis',(-0.810570785291136,-0.00660959938835658,0.585603377063722));
#81214=DIRECTION('center_axis',(-0.103109645269805,-0.986495108091252,-0.127262731246679));
#81215=DIRECTION('ref_axis',(-0.744358435177321,-0.00833900060649908,0.667728223942387));
#81216=DIRECTION('center_axis',(0.126461036348525,-0.986495108605844,0.104091339612869));
#81217=DIRECTION('ref_axis',(-0.665732675140154,-0.00660960231984546,0.746161053934007));
#81218=DIRECTION('center_axis',(-0.128056726462949,-0.986495108187667,-0.102121869985805));
#81219=DIRECTION('ref_axis',(-0.583413917845377,-0.0083389966343753,0.81213217003111));
#81220=DIRECTION('center_axis',(0.145881036647334,-0.986495108666972,0.0744723017157289));
#81221=DIRECTION('ref_axis',(-0.489765620838123,-0.00660966075859189,0.871829082463819));
#81222=DIRECTION('center_axis',(-0.147016016485838,-0.986495108226831,-0.0722059023984096));
#81223=DIRECTION('ref_axis',(-0.395189612230243,-0.0083389924723117,0.918561718987819));
#81224=DIRECTION('center_axis',(0.158479747416599,-0.986495108589863,0.0413711298739316));
#81225=DIRECTION('ref_axis',(-0.290897714801348,-0.00660960233039995,0.95673132732256));
#81226=DIRECTION('center_axis',(-0.159100997820152,-0.986495108218158,-0.0389136731018442));
#81227=DIRECTION('ref_axis',(-0.188486684529742,-0.00833899442689887,0.982040340783887));
#81228=DIRECTION('center_axis',(0.163668149216442,-0.986495108539713,0.00633543678716717));
#81229=DIRECTION('ref_axis',(-0.0784277380083555,-0.00660960110726281,0.996897889998818));
#81230=DIRECTION('center_axis',(0.157820536375367,0.986495107342785,0.0438187344287677));
#81231=DIRECTION('ref_axis',(-0.0842779456589509,-0.0307566094543304,0.9959674988926));
#81232=DIRECTION('center_axis',(-0.159684149326762,0.986495109228651,-0.0364468369236698));
#81233=DIRECTION('ref_axis',(-0.188062917200979,0.00584413918467036,0.982139595582546));
#81234=DIRECTION('center_axis',(0.144711044901561,0.986495107184974,0.0767210335149689));
#81235=DIRECTION('ref_axis',(-0.296411159314078,-0.0307566142160131,0.954565060808351));
#81236=DIRECTION('center_axis',(-0.148115826717113,0.986495109262762,-0.0699221086392466));
#81237=DIRECTION('ref_axis',(-0.394797092742267,0.0058441465540804,0.918749749122855));
#81238=DIRECTION('center_axis',(0.124835029133822,0.986495107315147,0.106035931383823));
#81239=DIRECTION('ref_axis',(-0.49468450248903,-0.0307566094782253,0.86852822289813));
#81240=DIRECTION('center_axis',(-0.129621774237926,0.986495109274237,-0.100127893323603));
#81241=DIRECTION('ref_axis',(-0.583070994334214,0.00584414688962944,0.81240018556943));
#81242=DIRECTION('center_axis',(0.0991218622187246,0.986495107224221,0.130392713956586));
#81243=DIRECTION('ref_axis',(-0.669826947539466,-0.0307566131833028,0.741879970814319));
#81244=DIRECTION('center_axis',(-0.105066754479679,0.986495109268846,-0.125651806559855));
#81245=DIRECTION('ref_axis',(-0.744081144306829,0.00584414342332145,0.668063692079347));
#81246=DIRECTION('center_axis',(0.0687738742096104,0.986495107341322,0.148652471953324));
#81247=DIRECTION('ref_axis',(-0.813649029250165,-0.0307566072135042,0.580542236459138));
#81248=DIRECTION('center_axis',(-0.0755989235215173,0.986495109243414,-0.145300386101388));
#81249=DIRECTION('ref_axis',(-0.870298887517183,0.0058441482875633,0.492489281423613));
#81250=DIRECTION('center_axis',(0.0352100904666574,0.986495107332255,0.159961410155238));
#81251=DIRECTION('ref_axis',(-0.919425787446233,-0.0307566086054127,0.392058990977081));
#81252=DIRECTION('center_axis',(-0.0425961788887042,0.98649510923347,-0.158154876632134));
#81253=DIRECTION('ref_axis',(-0.955822420196878,0.00584414429733773,0.293886622741517));
#81254=DIRECTION('center_axis',(-8.08933777940142E-8,0.986495107233467,
0.163790730520455));
#81255=DIRECTION('ref_axis',(-0.982211217362213,-0.0307566128273725,0.185243502599218));
#81256=DIRECTION('center_axis',(-0.00760168005488907,0.986495109258893,
-0.163614222696645));
#81257=DIRECTION('ref_axis',(-0.996652759685361,0.00584414497927649,0.0815421521730635));
#81258=DIRECTION('center_axis',(-0.0352102396399392,0.986495107333701,0.1599613773108));
#81259=DIRECTION('ref_axis',(-0.999069542386125,-0.0307566080214822,-0.0302337648894542));
#81260=DIRECTION('center_axis',(0.0277482648205711,0.986495109259409,-0.161423149537834));
#81261=DIRECTION('ref_axis',(-0.990880723998028,0.00584414488177559,-0.134615143203669));
#81262=DIRECTION('center_axis',(-0.068774016277597,0.986495107239889,0.14865240689881));
#81263=DIRECTION('ref_axis',(-0.969212485547708,-0.0307566129481366,-0.244297336494674));
#81264=DIRECTION('center_axis',(0.0618007367032491,0.986495109255772,-0.151684107135118));
#81265=DIRECTION('ref_axis',(-0.938776207478608,0.00584415113812403,-0.344477979222993));
#81266=DIRECTION('center_axis',(-0.0991219940639645,0.98649510717573,0.130392614097306));
#81267=DIRECTION('ref_axis',(-0.894036130325223,-0.0307566161811387,-0.446937834865417));
#81268=DIRECTION('center_axis',(0.0929634643369069,0.986495109244732,-0.134852488796849));
#81269=DIRECTION('ref_axis',(-0.84277555735421,0.00584414483275066,-0.538233412096903));
#81270=DIRECTION('center_axis',(-0.124835129047348,0.986495107325627,0.106035813659025));
#81271=DIRECTION('ref_axis',(-0.777055640426787,-0.0307566088079032,-0.628680016141403));
#81272=DIRECTION('center_axis',(0.119779331592666,0.986495109281869,-0.111715312675426));
#81273=DIRECTION('ref_axis',(-0.70736765939202,0.00584414874542795,-0.706821646790544));
#81274=DIRECTION('center_axis',(-0.144711118947382,0.986495107322158,0.0767208920857999));
#81275=DIRECTION('ref_axis',(-0.623740890245506,-0.0307566091489452,-0.78102582084679));
#81276=DIRECTION('center_axis',(0.14099444508826,0.986495109264767,-0.0833544590945802));
#81277=DIRECTION('ref_axis',(-0.538884035681307,0.00584414404218474,-0.842359686872682));
#81278=DIRECTION('center_axis',(-0.157820578861477,0.986495107231569,0.0438185839114293));
#81279=DIRECTION('ref_axis',(-0.441260710694636,-0.0307566129997595,-0.8968517246201));
#81280=DIRECTION('center_axis',(0.15561681786306,0.986495109242456,-0.0510960413230788));
#81281=DIRECTION('ref_axis',(-0.3452027953793,0.00584414322937402,-0.938509923257198));
#81282=DIRECTION('center_axis',(-0.163550521074303,0.986495107310167,0.00886737331046764));
#81283=DIRECTION('ref_axis',(-0.238147671140176,-0.0307566101542153,-0.970741838833751));
#81284=DIRECTION('center_axis',(0.162962721877935,0.986495109263591,-0.0164484247619832));
#81285=DIRECTION('ref_axis',(-0.135380253335906,0.00584414675128041,-0.99077647981543));
#81286=DIRECTION('center_axis',(-0.161633023909072,0.986495107269765,-0.0264984700468796));
#81287=DIRECTION('ref_axis',(-0.023899110607332,-0.0307566117760031,-0.999241143740708));
#81288=DIRECTION('center_axis',(0.162688669256186,0.98649510925121,0.0189682977384475));
#81289=DIRECTION('ref_axis',(0.0807725185426244,0.00584414601514746,-0.996715428899159));
#81290=DIRECTION('center_axis',(-0.152157746672938,0.986495107328072,-0.060625269856628));
#81291=DIRECTION('ref_axis',(0.191466946290586,-0.0307566085800032,-0.981017043433402));
#81292=DIRECTION('center_axis',(0.15480747712726,0.986495109248499,0.0534980789775261));
#81293=DIRECTION('ref_axis',(0.293148453799504,0.00584414074149075,-0.956049073036502));
#81294=DIRECTION('center_axis',(-0.135567741492699,0.986495107298358,-0.0919173038277894));
#81295=DIRECTION('ref_axis',(0.397880222564963,-0.0307566098130572,-0.916921675741425));
#81296=DIRECTION('center_axis',(0.139687655736703,0.986495109271076,0.0855263597906008));
#81297=DIRECTION('ref_axis',(0.491817096867627,0.00584414618293675,-0.870678924279261));
#81298=DIRECTION('center_axis',(-0.112638738693271,0.98649510727198,-0.118911386645828));
#81299=DIRECTION('ref_axis',(0.585689058392209,-0.0307566118478401,-0.809952071240816));
#81300=DIRECTION('center_axis',(0.118036198596492,0.986495109232562,0.113555516295446));
#81301=DIRECTION('ref_axis',(0.667488917242194,0.00584414393862002,-0.744596797831194));
#81302=DIRECTION('center_axis',(-0.0844428742116338,0.98649510726281,-0.140345303952126));
#81303=DIRECTION('ref_axis',(0.746111727528467,-0.0307566120268138,-0.665110006586217));
#81304=DIRECTION('center_axis',(0.0908654951821626,0.986495109267407,0.136274946988751));
#81305=DIRECTION('ref_axis',(0.811949699492863,0.00584414764719881,-0.583698150957948));
#81306=DIRECTION('center_axis',(-0.0522985590070483,0.986495107345266,-0.155216828693408));
#81307=DIRECTION('ref_axis',(0.871647040461356,-0.030756607696321,-0.489168138719167));
#81308=DIRECTION('center_axis',(0.0594460241246673,0.986495109265874,0.152622310329388));
#81309=DIRECTION('ref_axis',(0.918444615884464,0.00584414837009446,-0.39550642660097));
#81310=DIRECTION('center_axis',(-0.0177088158045688,0.986495107315265,-0.162830590141542));
#81311=DIRECTION('ref_axis',(0.95642510724864,-0.0307566096312886,-0.290353310965133));
#81312=DIRECTION('center_axis',(0.0252469209161744,0.986495109272428,0.161833223924607));
#81313=DIRECTION('ref_axis',(0.981994082020776,0.00584415117907665,-0.188821261443645));
#81314=DIRECTION('center_axis',(0.0177089703130797,0.986495107305418,-0.162830573397388));
#81315=DIRECTION('ref_axis',(0.996481798831909,-0.0307566097856968,-0.0779618852466596));
#81316=DIRECTION('center_axis',(-0.0101326912774383,0.98649510925592,0.163476995267305));
#81317=DIRECTION('ref_axis',(0.999626595924691,0.00584414560012706,0.0266929706518109));
#81318=DIRECTION('center_axis',(0.0522987062482193,0.986495107258488,-0.155216779633607));
#81319=DIRECTION('ref_axis',(0.989944108838892,-0.030756611577791,0.138074951455448));
#81320=DIRECTION('center_axis',(-0.0450385179583478,0.9864951092558,0.157476764363833));
#81321=DIRECTION('ref_axis',(0.97051768183973,0.00584414735009744,0.240959073658137));
#81322=DIRECTION('center_axis',(0.0844430093711828,0.986495107287759,-0.140345222453955));
#81323=DIRECTION('ref_axis',(0.937117733008439,-0.0307566099217808,0.347655555726129));
#81324=DIRECTION('center_axis',(-0.0778383928847949,0.986495109242354,0.144113094595974));
#81325=DIRECTION('ref_axis',(0.896028439172403,0.00584414839521296,0.443958198622125));
#81326=DIRECTION('center_axis',(0.112638853167697,0.98649510728676,-0.118911278087279));
#81327=DIRECTION('ref_axis',(0.840472772307255,-0.0307566098546537,0.540980175200909));
#81328=DIRECTION('center_axis',(-0.106998624069058,0.986495109229354,0.124010862080276));
#81329=DIRECTION('ref_axis',(0.779641903689181,0.00584414075326297,0.626198329629492));
#81330=DIRECTION('center_axis',(0.135567830575905,0.986495107258612,-0.0919171728664588));
#81331=DIRECTION('ref_axis',(0.704528239345761,-0.0307566120938428,0.709009161278521));
#81332=DIRECTION('center_axis',(-0.131155729272352,0.986495109286854,0.0981100098468817));
#81333=DIRECTION('ref_axis',(0.626800178425283,0.00584414786553591,0.779158124042713));
#81334=DIRECTION('center_axis',(0.15215780302399,0.986495107357182,-0.0606251279524845));
#81335=DIRECTION('ref_axis',(0.535640750317832,-0.03075660797491,0.843885666227854));
#81336=DIRECTION('center_axis',(-0.149180133269989,0.986495109263725,0.0676216476899283));
#81337=DIRECTION('ref_axis',(0.444649973888181,0.00584414774400711,0.895685350253305));
#81338=DIRECTION('center_axis',(0.161633050323747,0.986495107231132,-0.0264983103627146));
#81339=DIRECTION('ref_axis',(0.341707291870125,-0.0307566138101899,0.939303016810718));
#81340=DIRECTION('center_axis',(-0.160229039203752,0.986495109251109,0.0339713764732204));
#81341=DIRECTION('ref_axis',(0.241708429149031,0.00584414312165487,0.970331325511797));
#81342=DIRECTION('center_axis',(0.163550512813746,0.986495107277076,0.00886752934879879));
#81343=DIRECTION('ref_axis',(0.131795983805801,-0.0307566099985574,0.990799601127321));
#81344=DIRECTION('center_axis',(-0.163785815013084,0.986495109257399,-0.00126736408796769));
#81345=DIRECTION('ref_axis',(0.0274648691190149,0.0058441448589071,0.999605685725698));
#81346=DIRECTION('center_axis',(0.158221889598354,0.987363721928435,0.00887210637637829));
#81347=DIRECTION('ref_axis',(0.100091036882028,-0.0249769803935397,0.994664734866126));
#81348=DIRECTION('',(-0.603866633051807,0.,0.797085371517176));
#81349=DIRECTION('center_axis',(-0.154963408409918,0.987363721744034,0.0331545326878635));
#81350=DIRECTION('ref_axis',(0.170048762550982,-0.00640051209031499,0.985414862786157));
#81351=DIRECTION('',(-0.797085373092917,0.,-0.603866630971877));
#81352=DIRECTION('center_axis',(1.08195532252148E-14,-1.,4.32034611348363E-14));
#81353=DIRECTION('ref_axis',(9.57160757280875E-32,-4.32034611348363E-14,
-1.));
#81354=DIRECTION('center_axis',(0.148209450383285,-0.987363722419923,-0.0560966885489519));
#81355=DIRECTION('ref_axis',(0.246286329386107,-0.0180858580271892,0.96902835133805));
#81356=DIRECTION('center_axis',(0.156429989972518,0.987363721957276,-0.0253483490561554));
#81357=DIRECTION('ref_axis',(0.31157448071377,-0.0249769791829524,0.949893411640927));
#81358=DIRECTION('',(-0.418398773660791,0.,0.90826343436205));
#81359=DIRECTION('center_axis',(-0.144213205978919,0.987363721743852,0.0656919493196141));
#81360=DIRECTION('ref_axis',(0.377908184227036,-0.00640051097435485,0.925820953399464));
#81361=DIRECTION('',(-0.908263435453809,0.,-0.418398771290792));
#81362=DIRECTION('center_axis',(4.63261519963882E-14,-1.,9.30241762321944E-14));
#81363=DIRECTION('ref_axis',(-6.86840611318753E-31,-9.30241762321944E-14,
-1.));
#81364=DIRECTION('center_axis',(0.132685266333269,-0.987363722430966,-0.0866458292437413));
#81365=DIRECTION('ref_axis',(0.448840743760145,-0.0180858571215153,0.893428726039755));
#81366=DIRECTION('center_axis',(0.14732359669216,0.987363721989446,-0.0583835452574898));
#81367=DIRECTION('ref_axis',(0.508489047823086,-0.0249769762377366,0.860706128072753));
#81368=DIRECTION('',(-0.213367053339806,0.,0.976972108378273));
#81369=DIRECTION('center_axis',(-0.126719752544101,0.98736372175126,0.0951576864192368));
#81370=DIRECTION('ref_axis',(0.568097038624291,-0.00640051356442193,0.822936685372831));
#81371=DIRECTION('',(-0.976972108935031,0.,-0.213367050790503));
#81372=DIRECTION('center_axis',(3.72802973617033E-14,-1.,4.62231824842334E-14));
#81373=DIRECTION('ref_axis',(8.09500923725542E-31,-4.62231824842334E-14,
-1.));
#81374=DIRECTION('center_axis',(0.110956869526437,-0.987363722511827,-0.113143504331802));
#81375=DIRECTION('ref_axis',(0.63040786220677,-0.0180858524826944,0.776053367499854));
#81376=DIRECTION('center_axis',(0.131328515273723,0.98736372204213,-0.0886887899968879));
#81377=DIRECTION('ref_axis',(0.681627231977705,-0.0249769746314516,0.73127318244598));
#81378=DIRECTION('',(0.00164147464992936,0.,0.999998652779579));
#81379=DIRECTION('center_axis',(-0.103301029362936,0.987363721740793,0.120173950266803));
#81380=DIRECTION('ref_axis',(0.731722307361928,-0.00640050828832963,0.681572812253091));
#81381=DIRECTION('',(-0.999998652775296,0.,0.00164147725929106));
#81382=DIRECTION('center_axis',(6.95179839064118E-14,-1.,5.56925223301725E-14));
#81383=DIRECTION('ref_axis',(1.,6.95179839064117E-14,-7.46092427407147E-31));
#81384=DIRECTION('center_axis',(0.0840402488509648,-0.987363722495071,-0.134350720406496));
#81385=DIRECTION('ref_axis',(0.782497810464355,-0.0180858547525612,0.62239061567183));
#81386=DIRECTION('center_axis',(0.109192663208195,0.987363721956499,-0.114847041170904));
#81387=DIRECTION('ref_axis',(0.822893282784237,-0.0249769792256637,0.567646717296367));
#81388=DIRECTION('',(0.216573248336246,0.,0.976266371491452));
#81389=DIRECTION('center_axis',(-0.0750520550117979,0.987363721760651,0.139571021309803));
#81390=DIRECTION('ref_axis',(0.861133053975587,-0.00640051588460806,0.508339351956043));
#81391=DIRECTION('',(-0.976266370926293,0.,0.216573250883864));
#81392=DIRECTION('center_axis',(1.06486584100908E-13,-1.,5.25948673199192E-14));
#81393=DIRECTION('ref_axis',(1.,1.06486584100907E-13,1.33787268438141E-30));
#81394=DIRECTION('center_axis',(0.0531939969983551,-0.987363722423737,-0.149275846421587));
#81395=DIRECTION('ref_axis',(0.897999032444012,-0.0180858587656301,0.439625567321019));
#81396=DIRECTION('center_axis',(0.0819510774520538,0.987363722019657,-0.135635177383809));
#81397=DIRECTION('ref_axis',(0.925681760845532,-0.0249769763290022,0.377477718933682));
#81398=DIRECTION('',(0.421378297633106,0.,0.906884959784771));
#81399=DIRECTION('center_axis',(-0.04329373942725,0.987363721763552,0.152441900642943));
#81400=DIRECTION('ref_axis',(0.950278176164913,-0.00640051196046937,0.311336508221136));
#81401=DIRECTION('',(-0.906884959783822,0.,0.421378297635148));
#81402=DIRECTION('center_axis',(-4.32387482710148E-14,-1.,-1.06776602599891E-14));
#81403=DIRECTION('ref_axis',(1.,-4.32387482710148E-14,1.46181404460457E-31));
#81404=DIRECTION('center_axis',(0.0198604640486852,-0.987363722513244,-0.157220995520829));
#81405=DIRECTION('ref_axis',(0.971510815298322,-0.0180858514112591,0.236304121286785));
#81406=DIRECTION('center_axis',(0.0508775551859789,0.987363721971355,-0.150081161086825));
#81407=DIRECTION('ref_axis',(0.985186386900731,-0.0249769784355612,0.169658284836645));
#81408=DIRECTION('',(0.606480167148637,0.,0.795098614547505));
#81409=DIRECTION('',(-0.795098614022376,0.,0.606480167837084));
#81410=DIRECTION('',(0.763223696767892,0.,0.646134342603729));
#81411=DIRECTION('center_axis',(0.0247163556944388,0.987363721746886,0.156531091925291));
#81412=DIRECTION('ref_axis',(0.993175921563928,-0.0064005089879201,-0.116450085059387));
#81413=DIRECTION('',(-0.646134340612186,0.,0.763223698453904));
#81414=DIRECTION('center_axis',(5.83011444394288E-14,-1.,-1.12862629103633E-14));
#81415=DIRECTION('ref_axis',(1.,5.83011444394288E-14,1.62924502720985E-31));
#81416=DIRECTION('center_axis',(-0.0479905205830286,-0.987363722406496,
-0.151029101863708));
#81417=DIRECTION('ref_axis',(0.98094086059819,-0.0180858583824029,-0.19346299319367));
#81418=DIRECTION('center_axis',(-0.0168422276470354,0.987363722007276,-0.157572903228392));
#81419=DIRECTION('ref_axis',(0.965368612718929,-0.0249769765126249,-0.259691340289618));
#81420=DIRECTION('',(0.884279734078537,0.,0.466957548282488));
#81421=DIRECTION('center_axis',(0.0577880595905376,0.987363721746732,0.147558195798141));
#81422=DIRECTION('ref_axis',(0.944922693933094,-0.00640050965701902,-0.327231013148746));
#81423=DIRECTION('',(-0.466957545975081,0.,0.884279735296999));
#81424=DIRECTION('center_axis',(9.53957954715973E-14,-1.,-4.12219832883748E-14));
#81425=DIRECTION('ref_axis',(1.,9.53957954715972E-14,-5.76930804743858E-31));
#81426=DIRECTION('center_axis',(-0.079335316354445,-0.987363722508174,-0.137181584236888));
#81427=DIRECTION('ref_axis',(0.916418183908204,-0.0180858529151483,-0.399813224051833));
#81428=DIRECTION('center_axis',(-0.0503219807862601,0.987363721992186,-0.150268355762234));
#81429=DIRECTION('ref_axis',(0.886972870654081,-0.0249769774602344,-0.461145614009946));
#81430=DIRECTION('',(0.96398783550857,0.,0.265946334796144));
#81431=DIRECTION('center_axis',(0.0881576574204831,0.987363721749088,0.131685642390972));
#81432=DIRECTION('ref_axis',(0.852485931692217,-0.00640051001953579,-0.522710981076868));
#81433=DIRECTION('',(-0.265946332280708,0.,0.963987836202532));
#81434=DIRECTION('center_axis',(-1.20434267092608E-14,-1.,8.68078748888327E-15));
#81435=DIRECTION('ref_axis',(1.,-1.20434267092608E-14,1.38984695640427E-31));
#81436=DIRECTION('center_axis',(-0.106970488036425,-0.987363722454144,-0.116919606015178));
#81437=DIRECTION('ref_axis',(0.80904481124605,-0.0180858550211184,-0.587468633412881));
#81438=DIRECTION('center_axis',(-0.0814487377651023,0.98736372201617,-0.135937425173668));
#81439=DIRECTION('ref_axis',(0.767103261833128,-0.0249769747251451,-0.641037234814449));
#81440=DIRECTION('',(0.998620936282989,0.,0.0524997677831598));
#81441=DIRECTION('center_axis',(0.11440510064347,0.987363721729216,0.109655615267929));
#81442=DIRECTION('ref_axis',(0.720187874107375,-0.006400509403508,-0.693749565382261));
#81443=DIRECTION('',(-0.0524997650266615,0.,0.998620936427905));
#81444=DIRECTION('center_axis',(3.95829814884668E-14,-1.,-4.42672649531729E-14));
#81445=DIRECTION('ref_axis',(1.02946627009731E-30,4.42672649531729E-14,
-1.));
#81446=DIRECTION('center_axis',(-0.129603834006006,-0.987363722534076,-0.0911906005824955));
#81447=DIRECTION('ref_axis',(0.663841403133051,-0.0180858512043145,-0.747654661907861));
#81448=DIRECTION('center_axis',(-0.10876703762367,0.987363722001739,-0.115250214756607));
#81449=DIRECTION('ref_axis',(0.611364755852421,-0.0249769779150519,-0.790954667396141));
#81450=DIRECTION('',(0.986559631844411,0.,-0.163401630392784));
#81451=DIRECTION('center_axis',(0.135303090156659,0.987363721761573,0.0824982105454026));
#81452=DIRECTION('ref_axis',(0.554214631875562,-0.00640051217383139,-0.832349190700002));
#81453=DIRECTION('',(0.163401630169058,0.,0.986559631881466));
#81454=DIRECTION('center_axis',(0.,-1.,0.));
#81455=DIRECTION('ref_axis',(0.,0.,-1.));
#81456=DIRECTION('center_axis',(-0.14617705262823,-0.987363722526724,-0.0611976202404424));
#81457=DIRECTION('ref_axis',(0.487597508052115,-0.0180858528629753,-0.872881190121305));
#81458=DIRECTION('center_axis',(-0.130999513960469,0.987363721983204,-0.0891740312736589));
#81459=DIRECTION('ref_axis',(0.427039517577206,-0.0249769778724014,-0.903887936087096));
#81460=DIRECTION('',(0.928367895516495,0.,-0.371662549329729));
#81461=DIRECTION('center_axis',(0.149874454652235,0.987363721755551,0.0514832866445296));
#81462=DIRECTION('ref_axis',(0.362326932246914,-0.00640050910465206,-0.932029091633808));
#81463=DIRECTION('',(0.371662549274472,0.,0.928367895538617));
#81464=DIRECTION('center_axis',(-8.66859946722313E-15,-1.,2.8398172054035E-14));
#81465=DIRECTION('ref_axis',(-5.66160437743644E-32,-2.8398172054035E-14,
-1.));
#81466=DIRECTION('center_axis',(-0.155915195724191,-0.987363722398575,-0.0283431020447134));
#81467=DIRECTION('ref_axis',(0.288554093317215,-0.0180858593659295,-0.957292764477449));
#81468=DIRECTION('center_axis',(-0.147106600945047,0.987363722109429,-0.0589281615240848));
#81469=DIRECTION('ref_axis',(0.222746379323286,-0.0249769709087309,-0.974556412642486));
#81470=DIRECTION('',(0.826766709702495,0.,-0.562544938407333));
#81471=DIRECTION('center_axis',(0.157437857984951,0.987363721756996,0.0180610584209056));
#81472=DIRECTION('ref_axis',(0.153497224345565,-0.00640050896740749,-0.988128349761895));
#81473=DIRECTION('',(0.562544940564669,0.,0.82676670823461));
#81474=DIRECTION('center_axis',(5.90291219470682E-15,-1.,-7.39943279675939E-14));
#81475=DIRECTION('ref_axis',(1.21247827875496E-31,7.39943279675939E-14,
-1.));
#81476=DIRECTION('center_axis',(-0.158362913987082,-0.987363722452981,0.00583669917960967));
#81477=DIRECTION('ref_axis',(0.0760182140121149,-0.0180858566325272,-0.996942391980738));
#81478=DIRECTION('center_axis',(-0.156335142857511,0.987363722076235,-0.025926886343826));
#81479=DIRECTION('ref_axis',(0.00803787335697108,-0.0249769739436616,-0.999655712415287));
#81480=DIRECTION('',(0.686506828721979,0.,-0.727123355503103));
#81481=DIRECTION('center_axis',(0.157639641237614,0.987363721764162,-0.0162056920401103));
#81482=DIRECTION('ref_axis',(-0.0625098404813812,-0.00640051662167854,-0.998023823979151));
#81483=DIRECTION('',(0.727123357294462,0.,0.686506826824636));
#81484=DIRECTION('center_axis',(2.02833757503951E-15,-1.,1.47066666834218E-14));
#81485=DIRECTION('ref_axis',(3.92305911876007E-32,-1.47066666834218E-14,
-1.));
#81486=DIRECTION('center_axis',(-0.15340575975138,-0.987363722449015,0.0397435839693258));
#81487=DIRECTION('ref_axis',(-0.140072193470226,-0.0180858549598506,-0.989976101967523));
#81488=DIRECTION('center_axis',(-0.158253628115571,0.987363722083096,0.00828670637064815));
#81489=DIRECTION('ref_axis',(-0.207046477588685,-0.0249769721149615,-0.978012222307107));
#81490=DIRECTION('',(0.514146654526065,0.,-0.857702289631814));
#81491=DIRECTION('center_axis',(0.150470370386449,0.987363721772875,-0.0497146715022924));
#81492=DIRECTION('ref_axis',(-0.275594018979377,-0.00640051236263403,-0.961252812814761));
#81493=DIRECTION('',(0.857702290213478,0.,0.51414665355573));
#81494=DIRECTION('center_axis',(1.02848295574032E-14,-1.,2.78536007243207E-14));
#81495=DIRECTION('ref_axis',(-1.81250816775491E-31,-2.78536007243207E-14,
-1.));
#81496=DIRECTION('center_axis',(-0.141275521246826,-0.987363722413841,0.071792107905542));
#81497=DIRECTION('ref_axis',(-0.349612983833228,-0.0180858580766434,-0.936719628956743));
#81498=DIRECTION('center_axis',(-0.152772350370556,0.987363722030341,0.0421128172965009));
#81499=DIRECTION('ref_axis',(-0.412449562440443,-0.0249769746789723,-0.910637968228084));
#81500=DIRECTION('',(0.317745554014209,0.,-0.948176018945957));
#81501=DIRECTION('center_axis',(0.136265268983339,0.987363721760609,-0.0808990569780495));
#81502=DIRECTION('ref_axis',(-0.475791723949279,-0.00640051838988543,-0.87953468879045));
#81503=DIRECTION('',(0.948176020641203,0.,0.317745548955471));
#81504=DIRECTION('center_axis',(-4.00801918993373E-14,-1.,-6.2478661667528E-14));
#81505=DIRECTION('ref_axis',(1.14695610830292E-30,6.2478661667528E-14,-1.));
#81506=DIRECTION('center_axis',(-0.122539399999297,-0.987363722490077,0.100483704939411));
#81507=DIRECTION('ref_axis',(-0.542806256612586,-0.0180858529120981,-0.83966318825269));
#81508=DIRECTION('center_axis',(-0.140147609257795,0.987363721954357,0.0739697788814082));
#81509=DIRECTION('ref_axis',(-0.598566966055042,-0.0249769790975152,-0.800683294232385));
#81510=DIRECTION('',(0.106487020589929,0.,-0.99431409245061));
#81511=DIRECTION('center_axis',(0.115688560696546,0.987363721765323,-0.108300682664935));
#81512=DIRECTION('ref_axis',(-0.653741935995577,-0.00640051286148278,-0.756690501166669));
#81513=DIRECTION('',(0.994314092728476,0.,0.10648701799538));
#81514=DIRECTION('center_axis',(-4.20593637613534E-14,-1.,-4.19215110370194E-14));
#81515=DIRECTION('ref_axis',(1.,-4.20593637613534E-14,-8.90057686802853E-31));
#81516=DIRECTION('center_axis',(-0.0980734667160037,-0.987363722423222,
0.124476804139819));
#81517=DIRECTION('ref_axis',(-0.710618513547246,-0.0180858582164273,-0.703345029083506));
#81518=DIRECTION('center_axis',(-0.120969720893936,0.987363721921982,0.102367999195127));
#81519=DIRECTION('ref_axis',(-0.756696041964833,-0.0249769798023517,-0.653289561033014));
#81520=DIRECTION('',(-0.109750725713721,0.,-0.993959143126774));
#81521=DIRECTION('center_axis',(0.0897023821862004,0.987363721754206,-0.130638292984115));
#81522=DIRECTION('ref_axis',(-0.801123903692137,-0.00640051127421329,-0.598464305024535));
#81523=DIRECTION('',(0.993959142840391,0.,-0.109750728307355));
#81524=DIRECTION('center_axis',(-1.25219812285885E-14,-1.,-7.97497236843094E-15));
#81525=DIRECTION('ref_axis',(1.,-1.25219812285885E-14,2.06168302278434E-31));
#81526=DIRECTION('center_axis',(-0.0690217308745455,-0.987363722442943,
0.142649501473708));
#81527=DIRECTION('ref_axis',(-0.845203037920175,-0.0180858574324823,-0.53413923882396));
#81528=DIRECTION('center_axis',(-0.0961354190219717,0.987363721992652,0.125979608279625));
#81529=DIRECTION('ref_axis',(-0.879442854871605,-0.0249769765036889,-0.47534873057579));
#81530=DIRECTION('',(-0.320856647098721,0.,-0.947127769634365));
#81531=DIRECTION('center_axis',(0.05952181604836,0.987363721737319,-0.146867404182599));
#81532=DIRECTION('ref_axis',(-0.911046207097607,-0.00640051453204226,-0.412254583900276));
#81533=DIRECTION('',(0.947127767923488,0.,-0.320856652149012));
#81534=DIRECTION('center_axis',(2.78872151609101E-14,-1.,1.01933322533513E-14));
#81535=DIRECTION('ref_axis',(1.,2.78872151609101E-14,-1.63004772219339E-31));
#81536=DIRECTION('center_axis',(-0.0367426203520342,-0.987363722519182,
0.154152065515615));
#81537=DIRECTION('ref_axis',(-0.940266807613487,-0.0180858519364689,-0.339957692161941));
#81538=DIRECTION('center_axis',(-0.0668059397156617,0.987363721932429,0.143700546381871));
#81539=DIRECTION('ref_axis',(-0.961067894383304,-0.0249769815637861,-0.275181127219154));
#81540=DIRECTION('',(-0.516959673446092,0.,-0.856009752298717));
#81541=DIRECTION('center_axis',(0.0265580802596591,0.98736372174745,-0.156229156529586));
#81542=DIRECTION('ref_axis',(-0.978369002212705,-0.00640051292843176,-0.20676829772373));
#81543=DIRECTION('',(0.856009751718059,0.,-0.516959674407576));
#81544=DIRECTION('center_axis',(-7.35662317542014E-14,-1.,-9.90022723198433E-15));
#81545=DIRECTION('ref_axis',(1.,-7.35662317542014E-14,-1.38171261729452E-31));
#81546=DIRECTION('center_axis',(-0.00274545652003569,-0.987363722462837,
0.158446653586706));
#81547=DIRECTION('ref_axis',(-0.991364746987655,-0.018085856216804,-0.129880099457186));
#81548=DIRECTION('center_axis',(-0.034352680445948,0.987363721984285,0.154702210247681));
#81549=DIRECTION('ref_axis',(-0.997754469338468,-0.02497697794916,-0.0621463553850053));
#81550=DIRECTION('',(-0.688890236015648,0.,-0.724865672191962));
#81551=DIRECTION('center_axis',(-0.00764747800342432,0.987363721777915,
-0.15828580794579));
#81552=DIRECTION('ref_axis',(-0.999944350655294,-0.00640050754420234,0.00838624443593926));
#81553=DIRECTION('',(0.72486567039439,0.,-0.688890237907094));
#81554=DIRECTION('center_axis',(-4.43847301375668E-14,-1.,3.68747987600371E-15));
#81555=DIRECTION('ref_axis',(1.,-4.43847301375668E-14,-8.92032631172152E-32));
#81556=DIRECTION('center_axis',(0.0313800724015774,-0.987363722539182,0.155332451437688));
#81557=DIRECTION('ref_axis',(-0.996107572444681,-0.0180858510767603,0.0862705402161922));
#81558=DIRECTION('center_axis',(-0.000293129977269768,0.987363722010763,
0.158470169217646));
#81559=DIRECTION('ref_axis',(-0.987787153673095,-0.0249769763228967,0.153794309687225));
#81560=DIRECTION('',(-0.828609057310836,0.,-0.559827678971349));
#81561=DIRECTION('center_axis',(-0.0414954703147962,0.987363721637735,-0.152941188490987));
#81562=DIRECTION('ref_axis',(-0.974763412214174,-0.00640052409804163,0.22314865784909));
#81563=DIRECTION('',(0.559827676809204,0.,-0.828609058771632));
#81564=DIRECTION('center_axis',(0.0337800681979452,0.987363721247363,0.154828256326492));
#81565=DIRECTION('ref_axis',(-0.931631996025623,-0.0249770413045674,0.36254375099977));
#81566=DIRECTION('',(-0.929583040653769,0.,-0.368612765010781));
#81567=DIRECTION('center_axis',(-2.83695604196629E-14,-1.,8.76178241451945E-15));
#81568=DIRECTION('ref_axis',(1.,-2.83695604196629E-14,-1.9346427804638E-31));
#81569=DIRECTION('center_axis',(0.0640383594408077,-0.987363723068623,0.144955051268308));
#81570=DIRECTION('ref_axis',(-0.95427351150155,-0.0180859060603392,0.298387273938547));
#81571=DIRECTION('',(0.368612762585142,0.,-0.929583041615621));
#81572=DIRECTION('center_axis',(-0.0734031508739946,0.987363721755664,-0.140445214950786));
#81573=DIRECTION('ref_axis',(-0.904003620306502,-0.00640050963073223,0.427476885865428));
#81574=DIRECTION('center_axis',(-5.16455433471228E-14,-1.,2.93111074408959E-14));
#81575=DIRECTION('ref_axis',(1.,-5.16455433471228E-14,2.52306462361569E-31));
#81576=DIRECTION('center_axis',(0.0662738594893761,0.987363722011568,0.143946712375955));
#81577=DIRECTION('ref_axis',(-0.831914785709354,-0.0249769763266405,0.554340996113167));
#81578=DIRECTION('center_axis',(0.0937021887535035,-0.987363722499099,0.12779976258008));
#81579=DIRECTION('ref_axis',(-0.867818688045048,-0.0180858544134419,0.49655173602547));
#81580=DIRECTION('',(-0.987090754263963,0.,-0.160161926957068));
#81581=DIRECTION('center_axis',(-0.101878596556153,0.987363721764728,-0.121382175407489));
#81582=DIRECTION('ref_axis',(-0.79097362430467,-0.00640051099472303,0.611816769231884));
#81583=DIRECTION('',(0.160161927182448,0.,-0.987090754227393));
#81584=DIRECTION('center_axis',(-5.51713469867962E-14,-1.,4.96601190447716E-14));
#81585=DIRECTION('ref_axis',(1.,-5.51713469867962E-14,3.54595632905444E-31));
#81586=DIRECTION('center_axis',(0.118984656681206,-0.987363722441525,0.104668672872408));
#81587=DIRECTION('ref_axis',(-0.740785623688482,-0.018085856711078,0.671497998153005));
#81588=DIRECTION('center_axis',(0.0956687054159054,0.987363722097152,0.126334393933332));
#81589=DIRECTION('ref_axis',(-0.693298151125857,-0.0249769713557858,0.720217900740714));
#81590=DIRECTION('',(-0.998443201024793,0.,0.0557779017834631));
#81591=DIRECTION('center_axis',(-0.125590310399083,0.987363721769394,-0.0966434419272879));
#81592=DIRECTION('ref_axis',(-0.640958581238794,-0.00640050978831664,0.767548780606681));
#81593=DIRECTION('',(-0.0557779043887846,0.,-0.998443200879247));
#81594=DIRECTION('center_axis',(-6.04884194119145E-14,-1.,8.45030224620041E-14));
#81595=DIRECTION('ref_axis',(-1.33009085890558E-30,-8.45030224620041E-14,
-1.));
#81596=DIRECTION('center_axis',(0.1387035322197,-0.987363722447262,0.0766433933543153));
#81597=DIRECTION('ref_axis',(-0.579114246483947,-0.0180858566454766,0.815045760254434));
#81598=DIRECTION('center_axis',(0.120590181118975,0.987363722004324,0.102814827177119));
#81599=DIRECTION('ref_axis',(-0.522263667215958,-0.0249769772189026,0.852418214560872));
#81600=DIRECTION('',(-0.963109553688447,0.,0.269109620032506));
#81601=DIRECTION('center_axis',(-0.1434295647149,0.987363721767691,-0.0673857618696123));
#81602=DIRECTION('ref_axis',(-0.460973024805055,-0.00640051594299878,0.887391065876675));
#81603=DIRECTION('',(-0.26910962254562,0.,-0.963109552986239));
#81604=DIRECTION('center_axis',(3.50644987367232E-14,-1.,-8.18833808057458E-14));
#81605=DIRECTION('ref_axis',(-1.55431794060648E-31,8.18833808057458E-14,
-1.));
#81606=DIRECTION('center_axis',(0.151936786191621,-0.987363722382686,0.0450343504934522));
#81607=DIRECTION('ref_axis',(-0.390364131367923,-0.0180858605302077,0.920482887722661));
#81608=DIRECTION('center_axis',(0.139872998404293,0.987363721998246,0.0744877493227145));
#81609=DIRECTION('ref_axis',(-0.326808714331911,-0.0249769771506971,0.944760400762615));
#81610=DIRECTION('',(-0.882741973773198,0.,0.469858071910016));
#81611=DIRECTION('center_axis',(-0.154562207340053,0.987363721737865,-0.0349772076947687));
#81612=DIRECTION('ref_axis',(-0.259432884589524,-0.00640051184677438,0.965739929712787));
#81613=DIRECTION('',(-0.469858074213424,0.,-0.882741972547161));
#81614=DIRECTION('center_axis',(1.10948025608841E-14,-1.,-5.83378824764552E-14));
#81615=DIRECTION('ref_axis',(7.37852326003163E-32,5.83378824764552E-14,
-1.));
#81616=DIRECTION('center_axis',(0.158065641712028,-0.987363722473558,0.0113195606506427));
#81617=DIRECTION('ref_axis',(-0.183361024325124,-0.0180858544734437,0.982879258417028));
#81618=DIRECTION('center_axis',(0.152615509613344,0.987363721963071,0.0426777081939762));
#81619=DIRECTION('ref_axis',(-0.11607254932281,-0.0249769782048113,0.992926640720985));
#81620=DIRECTION('',(-0.761098361889465,0.,0.648636480263925));
#81621=DIRECTION('center_axis',(8.52754015441823E-16,-1.,2.96795148658844E-14));
#81622=DIRECTION('ref_axis',(0.0287202214020975,2.96917630343014E-14,0.999587489358793));
#81623=DIRECTION('center_axis',(0.156803525494539,-0.987363722442378,-0.0229245282877005));
#81624=DIRECTION('ref_axis',(0.0322158416459406,-0.0180858578001288,0.999317287599227));
#81625=DIRECTION('center_axis',(-0.158467694455886,0.98736372175334,-0.000933155522557501));
#81626=DIRECTION('ref_axis',(-0.0457619486551963,-0.00640051033716772,0.998931868308697));
#81627=DIRECTION('',(-0.648636483669163,0.,-0.761098358987394));
#81628=DIRECTION('center_axis',(-0.154002425234077,-0.987363721934798,-0.0373648715919747));
#81629=DIRECTION('ref_axis',(-0.156828000124788,-0.0129106125839618,0.987541540624781));
#81630=DIRECTION('',(0.562308454249505,0.,0.826927567734643));
#81631=DIRECTION('',(0.826927567205404,0.,-0.562308455027801));
#81632=DIRECTION('center_axis',(0.153257640420856,-0.987363719698522,0.0403110490527193));
#81633=DIRECTION('ref_axis',(-0.22011157129971,0.00565948153778567,0.97545828534525));
#81634=DIRECTION('center_axis',(-0.142369591901464,-0.987363721987792,-0.0695972686549175));
#81635=DIRECTION('ref_axis',(-0.365453688647701,-0.0129106102549393,0.930739983881983));
#81636=DIRECTION('',(0.371397010878143,0.,0.928474157050578));
#81637=DIRECTION('center_axis',(-1.73534424515167E-14,-1.,5.67913830243607E-14));
#81638=DIRECTION('ref_axis',(-1.40584472586084E-31,-5.67913830243607E-14,
-1.));
#81639=DIRECTION('center_axis',(0.151221679661691,0.987363722237908,0.0473802027095796));
#81640=DIRECTION('ref_axis',(-0.22122754271641,-0.0129109223179644,0.975136750629653));
#81641=DIRECTION('center_axis',(-0.145446249487498,0.987363722234589,-0.0629147719146933));
#81642=DIRECTION('ref_axis',(-0.294783644363712,0.0174544460973992,0.955404597710876));
#81643=DIRECTION('',(0.928474157301366,0.,-0.371397010251184));
#81644=DIRECTION('center_axis',(0.141008876239464,-0.987363719704729,0.0723144648913742));
#81645=DIRECTION('ref_axis',(-0.424660181785132,0.00565948540464467,0.905335131446457));
#81646=DIRECTION('center_axis',(-0.124079714504303,-0.98736372202158,-0.098575376662847));
#81647=DIRECTION('ref_axis',(-0.55699116933223,-0.0129106097786204,0.830418059438172));
#81648=DIRECTION('',(0.163119455793019,0.,0.98660632632362));
#81649=DIRECTION('center_axis',(-1.45780985909293E-14,-1.,2.58665774076789E-14));
#81650=DIRECTION('ref_axis',(-2.79864733334849E-31,-2.58665774076789E-14,
-1.));
#81651=DIRECTION('center_axis',(0.137500856816951,0.987363722241852,0.0787806726000697));
#81652=DIRECTION('ref_axis',(-0.425680940306143,-0.0129109245961234,0.904781213933043));
#81653=DIRECTION('center_axis',(-0.128520982733433,0.987363722311966,-0.0927105002655624));
#81654=DIRECTION('ref_axis',(-0.493275513135145,0.0174544420981305,0.869697999648328));
#81655=DIRECTION('',(0.98660632651026,0.,-0.163119454664154));
#81656=DIRECTION('center_axis',(0.122166697612528,-0.98736371968855,0.10093652974637));
#81657=DIRECTION('ref_axis',(-0.609352153792431,0.00565948107801637,0.792879513509116));
#81658=DIRECTION('center_axis',(-0.0999880073936607,-0.987363722004062,
-0.122944210305859));
#81659=DIRECTION('ref_axis',(-0.722484361105512,-0.0129106101685073,0.691266709818314));
#81660=DIRECTION('',(-0.052785381049886,0.,0.998605879988406));
#81661=DIRECTION('center_axis',(2.9696730449051E-14,-1.,-3.31919564300345E-14));
#81662=DIRECTION('ref_axis',(-2.71405253502507E-32,3.31919564300345E-14,
-1.));
#81663=DIRECTION('center_axis',(0.11735064596239,0.987363722220979,0.106497445669567));
#81664=DIRECTION('ref_axis',(-0.610229972424937,-0.0129109267773616,0.79211911271223));
#81665=DIRECTION('center_axis',(-0.105586214396424,0.9873637222575,-0.118171194879493));
#81666=DIRECTION('ref_axis',(-0.668702368113783,0.0174544451919355,0.743325288969816));
#81667=DIRECTION('',(0.998605879960773,0.,0.0527853815726573));
#81668=DIRECTION('center_axis',(0.0976121372020436,-0.987363719722958,0.124838918794155));
#81669=DIRECTION('ref_axis',(-0.765551498855408,0.00565948133520904,0.643349728274797));
#81670=DIRECTION('center_axis',(-0.0712209754792646,-0.987363722077632,
-0.141564306860121));
#81671=DIRECTION('ref_axis',(-0.854194986236279,-0.0129106066366808,0.519792498719515));
#81672=DIRECTION('',(-0.266222032663715,0.,0.963911733160459));
#81673=DIRECTION('center_axis',(9.63672715364679E-14,-1.,-6.94187404808866E-14));
#81674=DIRECTION('ref_axis',(1.,9.63672715364678E-14,-1.77223350769445E-30));
#81675=DIRECTION('center_axis',(0.0917132479702667,0.987363722209605,0.129234516330349));
#81676=DIRECTION('ref_axis',(-0.766245330217187,-0.0129109294373159,0.642418400905063));
#81677=DIRECTION('center_axis',(-0.0777143582214746,0.987363722327266,-0.138106329899358));
#81678=DIRECTION('ref_axis',(-0.812861441870596,0.0174544398692866,0.582195515998624));
#81679=DIRECTION('',(0.96391173298069,0.,0.266222033314604));
#81680=DIRECTION('center_axis',(0.068493335254789,-0.98736371970251,0.142903981893081));
#81681=DIRECTION('ref_axis',(-0.885954504802779,0.00565948925795247,0.463737625819819));
#81682=DIRECTION('center_axis',(-0.03912372399873,-0.98736372203281,-0.153565017611393));
#81683=DIRECTION('ref_axis',(-0.945964404768215,-0.012910609960063,0.324013365560705));
#81684=DIRECTION('',(-0.467210440327732,0.,0.884146144282022));
#81685=DIRECTION('center_axis',(-1.36296544362407E-14,-1.,5.8849567649498E-15));
#81686=DIRECTION('ref_axis',(1.,-1.36296544362407E-14,-9.90844762885813E-32));
#81687=DIRECTION('center_axis',(0.061787444507619,0.987363722220606,0.145928721449507));
#81688=DIRECTION('ref_axis',(-0.886431907160726,-0.012910926851988,0.462678918835968));
#81689=DIRECTION('center_axis',(-0.0462086621742918,0.987363722352972,-0.151583769979986));
#81690=DIRECTION('ref_axis',(-0.919012019491634,0.0174544387401066,0.393842926302068));
#81691=DIRECTION('',(0.884146145154076,0.,0.467210438677464));
#81692=DIRECTION('center_axis',(0.0361718722602125,-0.987363719711651,0.154287007406209));
#81693=DIRECTION('ref_axis',(-0.964931262274253,0.00565948410852384,0.262441668424515));
#81694=DIRECTION('center_axis',(-0.00519709259350015,-0.987363721985343,
-0.15838519733809));
#81695=DIRECTION('ref_axis',(-0.993501578246324,-0.0129106113742557,0.113083730642412));
#81696=DIRECTION('',(-0.64635260602278,0.,0.763038864467309));
#81697=DIRECTION('center_axis',(-8.74565546649098E-14,-1.,1.69043816072292E-14));
#81698=DIRECTION('ref_axis',(1.,-8.74565546649098E-14,4.47822014116462E-31));
#81699=DIRECTION('center_axis',(0.0289725258709897,0.987363722235357,0.155799463279547));
#81700=DIRECTION('ref_axis',(-0.965169912231812,-0.0129109281183902,0.261305086933948));
#81701=DIRECTION('center_axis',(-0.0125422923522538,0.987363722231902,-0.157973323453408));
#81702=DIRECTION('ref_axis',(-0.982190616805527,0.0174544457418185,0.187074676487826));
#81703=DIRECTION('',(0.763038865448696,0.,0.646352604864224));
#81704=DIRECTION('center_axis',(0.00215905541530509,-0.987363719712137,
0.15845574611205));
#81705=DIRECTION('ref_axis',(-0.998788906524019,0.00565947699061602,0.0488742317049259));
#81706=DIRECTION('center_axis',(0.0289725475431906,-0.987363722006681,-0.155799460698588));
#81707=DIRECTION('ref_axis',(-0.994583722670036,-0.0129106105555476,-0.103133577145834));
#81708=DIRECTION('',(-0.795272041985628,0.,0.606252735446208));
#81709=DIRECTION('center_axis',(0.,-1.,0.));
#81710=DIRECTION('ref_axis',(0.,0.,-1.));
#81711=DIRECTION('center_axis',(-0.00519711222669223,0.987363722216384,
0.158385195253569));
#81712=DIRECTION('ref_axis',(-0.998777645603758,-0.0129109255541131,0.0477129190424396));
#81713=DIRECTION('center_axis',(0.0217105317550711,0.987363722287536,-0.156976217056641));
#81714=DIRECTION('ref_axis',(-0.99944307160964,0.0174544431624296,-0.028440974409791));
#81715=DIRECTION('',(0.606252735341353,0.,0.795272042065561));
#81716=DIRECTION('center_axis',(-0.0319547269489774,-0.987363719689367,
0.155215271371064));
#81717=DIRECTION('ref_axis',(-0.985944291779663,0.00565948020654221,-0.166978512961669));
#81718=DIRECTION('center_axis',(0.061787468866819,-0.987363721901482,-0.145928713294833));
#81719=DIRECTION('ref_axis',(-0.949160236890853,-0.0129106152611583,-0.314528473621829));
#81720=DIRECTION('',(-0.907005440776329,0.,0.421118902926641));
#81721=DIRECTION('center_axis',(-4.32356925031948E-14,-1.,-1.06900264805193E-14));
#81722=DIRECTION('ref_axis',(1.,-4.32356925031948E-14,1.79016941821345E-31));
#81723=DIRECTION('center_axis',(-0.0391237430712795,0.987363722200939,0.15356501167128));
#81724=DIRECTION('ref_axis',(-0.985683646016057,-0.0129109264441407,-0.168110255352985));
#81725=DIRECTION('center_axis',(0.0549482001638952,0.987363722238535,-0.148639077318224));
#81726=DIRECTION('ref_axis',(-0.969962679413179,0.0174544454904423,-0.242626756311474));
#81727=DIRECTION('',(0.421118902314201,0.,0.907005441060682));
#81728=DIRECTION('center_axis',(-0.064574338796006,-0.987363719700537,0.144717102611194));
#81729=DIRECTION('ref_axis',(-0.926998018391755,0.00565948096684053,-0.375023524826038));
#81730=DIRECTION('center_axis',(0.0917132688626462,-0.987363721970692,-0.129234503329062));
#81731=DIRECTION('ref_axis',(-0.859355073458652,-0.0129106117045736,-0.511216366938979));
#81732=DIRECTION('',(-0.9763282731838,0.,0.216294019755377));
#81733=DIRECTION('center_axis',(-1.33089421047624E-14,-1.,-6.57816514610932E-15));
#81734=DIRECTION('ref_axis',(1.,-1.33089421047624E-14,-6.18048586043692E-32));
#81735=DIRECTION('center_axis',(-0.0712209911166728,0.987363722215975,0.141564298028046));
#81736=DIRECTION('ref_axis',(-0.926500175100293,-0.0129109281555154,-0.37607277683088));
#81737=DIRECTION('center_axis',(0.0856165460212759,0.987363722297612,-0.133351741413418));
#81738=DIRECTION('ref_axis',(-0.895127910167366,0.0174544412333558,-0.445467582345378));
#81739=DIRECTION('',(0.216294019096123,0.,0.97632827332985));
#81740=DIRECTION('center_axis',(-0.0941745270390424,-0.987363719687872,
0.127452122387594));
#81741=DIRECTION('ref_axis',(-0.82470634699939,0.00565948217092306,-0.565532856234258));
#81742=DIRECTION('center_axis',(0.117350661423251,-0.987363721986634,-0.106497430805754));
#81743=DIRECTION('ref_axis',(-0.729367422684911,-0.0129106116023004,-0.684000350024783));
#81744=DIRECTION('',(-0.999999081357214,0.,0.00135546476455657));
#81745=DIRECTION('center_axis',(1.15836753776633E-14,-1.,9.28540044415546E-15));
#81746=DIRECTION('ref_axis',(1.,1.15836753776633E-14,-1.75050267875677E-31));
#81747=DIRECTION('center_axis',(-0.0999880263442184,0.987363722188352,0.122944193413724));
#81748=DIRECTION('ref_axis',(-0.823994584277942,-0.0129109315438825,-0.566450556471869));
#81749=DIRECTION('center_axis',(0.112281563017468,0.987363722285881,-0.111829023603552));
#81750=DIRECTION('ref_axis',(-0.778437954930438,0.0174544436516842,-0.627478838464317));
#81751=DIRECTION('',(0.00135546408934942,0.,0.999999081358129));
#81752=DIRECTION('center_axis',(-0.119371216758459,-0.987363719705103,0.10422762407207));
#81753=DIRECTION('ref_axis',(-0.683852325090944,0.00565948098279108,-0.729598497629152));
#81754=DIRECTION('center_axis',(0.137500865949824,-0.987363722045799,-0.0787806591170389));
#81755=DIRECTION('ref_axis',(-0.565275361749489,-0.0129106086395355,-0.82480123762246));
#81756=DIRECTION('',(-0.976911043828257,0.,-0.213646466028307));
#81757=DIRECTION('center_axis',(-2.7950306566047E-14,-1.,-3.4675382181889E-14));
#81758=DIRECTION('ref_axis',(-5.33496938660793E-31,3.4675382181889E-14,
-1.));
#81759=DIRECTION('center_axis',(-0.12407972669933,0.987363722202763,0.0985753594978235));
#81760=DIRECTION('ref_axis',(-0.682959926175101,-0.0129109281602422,-0.730341733144794));
#81761=DIRECTION('center_axis',(0.133696416719564,0.987363722290334,-0.0850773063826399));
#81762=DIRECTION('ref_axis',(-0.625349106696063,0.0174544434909131,-0.780149881213128));
#81763=DIRECTION('',(-0.213646469431568,0.,0.976911043083978));
#81764=DIRECTION('center_axis',(-0.138986243896786,-0.987363719681023,0.0761295544786478));
#81765=DIRECTION('ref_axis',(-0.511022127211816,0.00565948406729928,-0.859548925739543));
#81766=DIRECTION('center_axis',(0.151221685925258,-0.987363722020143,-0.0473801872564035));
#81767=DIRECTION('ref_axis',(-0.374751652353903,-0.0129106109021625,-0.92703533653478));
#81768=DIRECTION('',(-0.908143731209353,0.,-0.418658528475361));
#81769=DIRECTION('center_axis',(6.61422058830698E-15,-1.,1.32910602459398E-14));
#81770=DIRECTION('ref_axis',(-5.61309428634172E-32,-1.32910602459398E-14,
-1.));
#81771=DIRECTION('center_axis',(-0.142369597806779,0.987363722223232,0.0695972532347455));
#81772=DIRECTION('ref_axis',(-0.509990818251875,-0.0129109231207067,-0.860082945629637));
#81773=DIRECTION('center_axis',(0.148859773252513,0.987363722335809,-0.0543474720882764));
#81774=DIRECTION('ref_axis',(-0.443019628618916,0.017454439684933,-0.896341983393416));
#81775=DIRECTION('',(-0.418658529088568,0.,0.908143730926662));
#81776=DIRECTION('center_axis',(-0.152102425325803,-0.987363719696516,0.0444717577465602));
#81777=DIRECTION('ref_axis',(-0.314297103910649,0.00565948000699346,-0.94930780085251));
#81778=DIRECTION('center_axis',(0.157871546545998,-0.987363722028207,-0.0137642730931085));
#81779=DIRECTION('ref_axis',(-0.166704973938361,-0.0129106104254692,-0.985922292983911));
#81780=DIRECTION('',(-0.796912626680255,0.,-0.604094583188408));
#81781=DIRECTION('center_axis',(-1.08071961368061E-14,-1.,-4.32065536369259E-14));
#81782=DIRECTION('ref_axis',(1.29028034373309E-31,4.32065536369259E-14,
-1.));
#81783=DIRECTION('center_axis',(-0.154002427753715,0.987363722237364,0.0373648532117916));
#81784=DIRECTION('ref_axis',(-0.313175106282416,-0.0129109227870478,-0.949607635225088));
#81785=DIRECTION('center_axis',(0.157062615356744,0.987363722285769,-0.0210764031867505));
#81786=DIRECTION('ref_axis',(-0.239975045778217,0.0174544441542665,-0.970622130276766));
#81787=DIRECTION('',(-0.60409458190082,0.,0.796912627656303));
#81788=DIRECTION('',(-0.648418775400067,0.,-0.761283844376509));
#81789=DIRECTION('',(-0.761283846233458,0.,0.648418773219895));
#81790=DIRECTION('center_axis',(-0.156717628096624,-0.987363719703207,-0.0235046816106097));
#81791=DIRECTION('ref_axis',(0.113355675865131,0.00565948486422126,-0.993538354055962));
#81792=DIRECTION('center_axis',(0.14905980269933,-0.987363721901566,0.0537964301038988));
#81793=DIRECTION('ref_axis',(0.262680691146538,-0.0129106143644342,-0.964796439947573));
#81794=DIRECTION('',(-0.469605582630858,0.,-0.882876320195492));
#81795=DIRECTION('center_axis',(2.22229744853242E-14,-1.,-1.16669413356185E-13));
#81796=DIRECTION('ref_axis',(4.36736143566875E-31,1.16669413356185E-13,
-1.));
#81797=DIRECTION('center_axis',(-0.155457912814063,0.987363722264946,-0.0307525169474946));
#81798=DIRECTION('ref_axis',(0.114499868445593,-0.0129109209841225,-0.99333936207385));
#81799=DIRECTION('center_axis',(0.151395920500974,0.987363722202361,0.0468204585022689));
#81800=DIRECTION('ref_axis',(0.189758203180646,0.0174544474591918,-0.981675693184642));
#81801=DIRECTION('',(-0.8828763217045,0.,0.469605579793865));
#81802=DIRECTION('center_axis',(-0.148000847497835,-0.987363719703838,-0.0566448069334213));
#81803=DIRECTION('ref_axis',(0.324286860420664,0.00565947861214943,-0.945941859978903));
#81804=DIRECTION('center_axis',(0.134010224920062,-0.987363721885144,0.0845821513204255));
#81805=DIRECTION('ref_axis',(0.463942076602047,-0.0129106150950262,-0.885771452224584));
#81806=DIRECTION('',(-0.268834151573639,0.,-0.963186481917018));
#81807=DIRECTION('center_axis',(-1.75439583158224E-14,-1.,4.09366742645534E-14));
#81808=DIRECTION('ref_axis',(4.91190218677542E-32,-4.09366742645534E-14,
-1.));
#81809=DIRECTION('center_axis',(-0.145212510191229,0.987363722233914,-0.0634523986965965));
#81810=DIRECTION('ref_axis',(0.325361525070664,-0.0129109237299263,-0.945501552643956));
#81811=DIRECTION('center_axis',(0.137791354159373,0.987363722222338,0.0782714683532711));
#81812=DIRECTION('ref_axis',(0.396353016518055,0.0174544459680833,-0.917932257093619));
#81813=DIRECTION('',(-0.963186482098545,0.,0.268834150923259));
#81814=DIRECTION('center_axis',(-0.132363709699744,-0.987363719708208,-0.0871362918564599));
#81815=DIRECTION('ref_axis',(0.520054751302658,0.00565948078914774,-0.854114176164245));
#81816=DIRECTION('center_axis',(0.1126944776794,-0.987363721924488,0.111412904674414));
#81817=DIRECTION('ref_axis',(0.643510048271339,-0.0129106152021611,-0.765328774964669));
#81818=DIRECTION('',(-0.0554923374905852,0.,-0.998459113073656));
#81819=DIRECTION('center_axis',(4.32232752686131E-14,-1.,-6.03469417671824E-14));
#81820=DIRECTION('ref_axis',(9.26499412064615E-31,6.03469417671824E-14,
-1.));
#81821=DIRECTION('center_axis',(-0.128177131858304,0.987363722255328,-0.0931853145226321));
#81822=DIRECTION('ref_axis',(0.521009637840492,-0.0129109244303183,-0.85345314183479));
#81823=DIRECTION('center_axis',(0.117743818984395,0.987363722290477,0.106062589991308));
#81824=DIRECTION('ref_axis',(0.584414805440217,0.0174544421071706,-0.811267328094137));
#81825=DIRECTION('',(-0.998459113111129,0.,0.0554923368163326));
#81826=DIRECTION('center_axis',(-0.110537393066309,-0.987363719709225,-0.113553378356029));
#81827=DIRECTION('ref_axis',(0.691505459935205,0.00565948043168418,-0.722349063238157));
#81828=DIRECTION('center_axis',(0.0861092664287607,-0.987363721999118,0.133034111096177));
#81829=DIRECTION('ref_axis',(0.792988204586121,-0.0129106098602343,-0.609100175291649));
#81830=DIRECTION('',(0.160444237331189,0.,-0.987044906124951));
#81831=DIRECTION('center_axis',(0.,-1.,0.));
#81832=DIRECTION('ref_axis',(0.,0.,-1.));
#81833=DIRECTION('center_axis',(-0.105148331973208,0.987363722223282,-0.118560989877104));
#81834=DIRECTION('ref_axis',(0.692295920183945,-0.0129109267763575,-0.721498209884432));
#81835=DIRECTION('center_axis',(0.0921907102839049,0.987363722266113,0.128894347782028));
#81836=DIRECTION('ref_axis',(0.74515000645914,0.0174544447381545,-0.666668441005592));
#81837=DIRECTION('',(-0.987044905635345,0.,-0.160444240343221));
#81838=DIRECTION('center_axis',(-0.0835424717653903,-0.987363719700328,
-0.134660834806788));
#81839=DIRECTION('ref_axis',(0.83062214417687,0.00565947854203068,-0.556807708195255));
#81840=DIRECTION('center_axis',(0.0554976762857084,-0.987363721959145,0.148434795401454));
#81841=DIRECTION('ref_axis',(0.905387113396104,-0.0129106122046947,-0.424390729150356));
#81842=DIRECTION('',(0.36887861981684,0.,-0.929477575760719));
#81843=DIRECTION('center_axis',(9.03943676094093E-14,-1.,-5.12685863601807E-14));
#81844=DIRECTION('ref_axis',(1.,9.03943676094093E-14,7.83102586053432E-31));
#81845=DIRECTION('center_axis',(-0.0772029158233061,0.987363722218407,-0.138392882170259));
#81846=DIRECTION('ref_axis',(0.831211213975916,-0.012910924975103,-0.555806824154734));
#81847=DIRECTION('center_axis',(0.0623268682590145,0.987363722274991,0.145699146971756));
#81848=DIRECTION('ref_axis',(0.871042822047256,0.0174544443199294,-0.490896877697786));
#81849=DIRECTION('',(-0.929477575511641,0.,-0.368878620444452));
#81850=DIRECTION('center_axis',(-0.0526411923994217,-0.987363719715787,
-0.149471702511788));
#81851=DIRECTION('ref_axis',(0.930899857264182,0.00565948303979362,-0.365230647669728));
#81852=DIRECTION('center_axis',(0.0222910793373077,-0.987363722001288,0.15689483183885));
#81853=DIRECTION('ref_axis',(0.97545112806071,-0.012910610669765,-0.219837241834094));
#81854=DIRECTION('',(0.56006464518858,0.,-0.828448908026192));
#81855=DIRECTION('center_axis',(2.8372065137431E-14,-1.,-8.75366807693456E-15));
#81856=DIRECTION('ref_axis',(1.,2.8372065137431E-14,-1.7135964172008E-31));
#81857=DIRECTION('center_axis',(-0.045647571293492,0.987363722194643,-0.151753679787165));
#81858=DIRECTION('ref_axis',(0.931259995085496,-0.0129109298287278,-0.36412652944316));
#81859=DIRECTION('center_axis',(0.0295486889639333,0.987363722256726,0.15569121668179));
#81860=DIRECTION('ref_axis',(0.956206642880283,0.0174544463351347,-0.292171522251491));
#81861=DIRECTION('',(-0.82844890631414,0.,-0.560064647721052));
#81862=DIRECTION('center_axis',(-0.0192784774288681,-0.987363719716235,
-0.157293436913768));
#81863=DIRECTION('ref_axis',(0.987649729086615,0.00565947836576162,-0.156575805729248));
#81864=DIRECTION('center_axis',(-0.0119578245152855,-0.98736372200228,0.158018641010057));
#81865=DIRECTION('ref_axis',(0.999904131400371,-0.0129106106213219,-0.00500441223858307));
#81866=DIRECTION('',(0.725062671623472,0.,-0.688682889447845));
#81867=DIRECTION('center_axis',(-1.47952609495248E-14,-1.,1.2249284241146E-15));
#81868=DIRECTION('ref_axis',(1.,-1.47952609495248E-14,-9.44752033172559E-33));
#81869=DIRECTION('center_axis',(-0.0119578035856478,0.987363722219315,-0.158018641237758));
#81870=DIRECTION('ref_axis',(0.9877640942684,-0.0129109272861874,-0.155420082456347));
#81871=DIRECTION('center_axis',(-0.0046111468982762,0.987363722325162,0.158403336961328));
#81872=DIRECTION('ref_axis',(0.996659303735564,0.0174544409252697,-0.0797845521973175));
#81873=DIRECTION('',(-0.688682888958241,0.,-0.725062672088511));
#81874=DIRECTION('center_axis',(0.0149856872273682,-0.987363719693288,-0.157760306198226));
#81875=DIRECTION('ref_axis',(0.998218197100463,0.00565948357705208,0.0594003469951372));
#81876=DIRECTION('center_axis',(-0.0456475956634642,-0.987363721979248,
0.151753673858105));
#81877=DIRECTION('ref_axis',(0.977602729074026,-0.0129106122427607,0.210062419767398));
#81878=DIRECTION('',(0.856157573483628,0.,-0.516714824024457));
#81879=DIRECTION('center_axis',(1.32414114458036E-13,-1.,1.78582813416022E-14));
#81880=DIRECTION('ref_axis',(1.,1.32414114458036E-13,5.55548786246673E-32));
#81881=DIRECTION('center_axis',(0.0222911022848482,0.987363722208355,-0.156894827275438));
#81882=DIRECTION('ref_axis',(0.998081442094801,-0.012910929320345,0.0605536361422535));
#81883=DIRECTION('center_axis',(-0.0385553754235707,0.987363722312957,0.15370869489476));
#81884=DIRECTION('ref_axis',(0.990509283694734,0.0174544407656422,0.136333053263337));
#81885=DIRECTION('',(-0.516714824718151,0.,-0.856157573064965));
#81886=DIRECTION('center_axis',(0.0485491287704313,-0.987363719723607,-0.150850479181189));
#81887=DIRECTION('ref_axis',(0.962111091449422,0.00565947937755026,0.272599005873419));
#81888=DIRECTION('center_axis',(-0.0772029342179146,-0.987363721959937,
0.138392873752822));
#81889=DIRECTION('ref_axis',(0.90958970992946,-0.0129106121656763,0.415306965609714));
#81890=DIRECTION('',(0.947219498157893,0.,-0.32058574876234));
#81891=DIRECTION('center_axis',(5.57685970606299E-14,-1.,2.04026155986365E-14));
#81892=DIRECTION('ref_axis',(1.,5.57685970606299E-14,-5.33515460699669E-31));
#81893=DIRECTION('center_axis',(0.0554976970957135,0.9873637222177,-0.148434785901016));
#81894=DIRECTION('ref_axis',(0.961729611179224,-0.0129109277223155,0.273695931512342));
#81895=DIRECTION('center_axis',(-0.0706968022411019,0.987363722240037,0.14182680338068));
#81896=DIRECTION('ref_axis',(0.938044149622633,0.01745444496317,0.346075881433219));
#81897=DIRECTION('',(-0.320585748995687,0.,-0.947219498078916));
#81898=DIRECTION('center_axis',(0.0798424772113265,-0.987363719686393,-0.136887047889156));
#81899=DIRECTION('ref_axis',(0.881016739713925,0.00565948623402568,0.473051238830861));
#81900=DIRECTION('center_axis',(-0.105148351657736,-0.987363721915906,0.118560974979252));
#81901=DIRECTION('ref_axis',(0.799045286445946,-0.0129106147625576,0.60113222026021));
#81902=DIRECTION('',(0.993990492096634,0.,-0.109466440617618));
#81903=DIRECTION('center_axis',(1.00157598129628E-13,-1.,6.38284273780134E-14));
#81904=DIRECTION('ref_axis',(1.,1.00157598129628E-13,-3.97615990582066E-31));
#81905=DIRECTION('center_axis',(0.0861092789791971,0.987363722241669,-0.133034101172438));
#81906=DIRECTION('ref_axis',(0.880408371952486,-0.0129109227373763,0.474040511633807));
#81907=DIRECTION('center_axis',(-0.0995325171218021,0.98736372227733,0.123313251380591));
#81908=DIRECTION('ref_axis',(0.841717114861623,0.0174544407701366,0.539636582383391));
#81909=DIRECTION('',(-0.109466440259225,0.,-0.993990492136104));
#81910=DIRECTION('center_axis',(0.107402471327209,-0.987363719708752,-0.116522934033203));
#81911=DIRECTION('ref_axis',(0.758727025472456,0.00565948363991874,0.651384119443089));
#81912=DIRECTION('center_axis',(-0.128177146079023,-0.987363721938031,0.0931852983239097));
#81913=DIRECTION('ref_axis',(0.651138393509337,-0.0129106139935096,0.75884920013425));
#81914=DIRECTION('',(0.994283595393051,0.,0.106771400347975));
#81915=DIRECTION('center_axis',(5.25592149427991E-14,-1.,5.24169231671855E-14));
#81916=DIRECTION('ref_axis',(1.,5.25592149427991E-14,1.52343460007419E-31));
#81917=DIRECTION('center_axis',(0.112694496580979,0.987363722214069,-0.111412882989084));
#81918=DIRECTION('ref_axis',(0.757920215591527,-0.012910930245521,0.652219483516008));
#81919=DIRECTION('center_axis',(-0.12371420854767,0.987363722261302,0.0990337041906916));
#81920=DIRECTION('ref_axis',(0.706032321934242,0.0174544443873073,0.707964478455857));
#81921=DIRECTION('',(0.106771401019337,0.,-0.994283595320957));
#81922=DIRECTION('center_axis',(0.129940445222184,-0.987363719718547,-0.0907103394273005));
#81923=DIRECTION('ref_axis',(0.600960079687005,0.00565947968915366,0.799259002396743));
#81924=DIRECTION('center_axis',(-0.145212520372231,-0.987363721945181,0.0634523798899918));
#81925=DIRECTION('ref_axis',(0.472784992661812,-0.0129106143584673,0.8810832348596));
#81926=DIRECTION('',(0.948085102432835,0.,0.318016726831972));
#81927=DIRECTION('center_axis',(0.,-1.,0.));
#81928=DIRECTION('ref_axis',(0.,0.,-1.));
#81929=DIRECTION('center_axis',(0.134010234072352,0.987363722256383,-0.0845821324860878));
#81930=DIRECTION('ref_axis',(0.599992554262842,-0.0129109228150569,0.799901395736508));
#81931=DIRECTION('center_axis',(-0.142111155988232,0.987363722341574,0.0701234564712802));
#81932=DIRECTION('ref_axis',(0.537334244319765,0.0174544408201278,0.843188740660692));
#81933=DIRECTION('',(0.318016724021307,0.,-0.948085103375618));
#81934=DIRECTION('center_axis',(0.14640255189611,-0.987363719719664,-0.0606562262233358));
#81935=DIRECTION('ref_axis',(0.415092905252734,0.00565948058615717,0.909761424928722));
#81936=DIRECTION('center_axis',(-0.155457917085905,-0.987363722019786,0.0307525032240912));
#81937=DIRECTION('ref_axis',(0.272324693801645,-0.0129106103601986,0.962118795828232));
#81938=DIRECTION('',(0.857555204217401,0.,0.514391943676854));
#81939=DIRECTION('center_axis',(2.56921567550482E-14,-1.,6.96413525208238E-14));
#81940=DIRECTION('ref_axis',(5.42541743807951E-31,-6.96413525208238E-14,
-1.));
#81941=DIRECTION('center_axis',(0.149059810145022,0.987363722194985,-0.0537964040879616));
#81942=DIRECTION('ref_axis',(0.414009904232867,-0.0129109291564851,0.910180810117094));
#81943=DIRECTION('center_axis',(-0.153863147665941,0.987363722279557,0.03793430790968));
#81944=DIRECTION('ref_axis',(0.343511013224812,0.0174544443899348,0.938986435559269));
#81945=DIRECTION('',(0.514391942141765,0.,-0.857555205138202));
#81946=DIRECTION('center_axis',(0.156019037498486,-0.987363719708581,-0.027765895290473));
#81947=DIRECTION('ref_axis',(0.209816451605885,0.00565948196952231,0.97772441255159));
#81948=DIRECTION('center_axis',(-0.158434276356287,-0.987363722051535,-0.0033853289351005));
#81949=DIRECTION('ref_axis',(0.0591307919551479,-0.0129106090674337,0.998166752409769));
#81950=DIRECTION('',(0.72692697915402,0.,0.686714763914401));
#81951=DIRECTION('center_axis',(0.,-1.,0.));
#81952=DIRECTION('ref_axis',(0.,0.,-1.));
#81953=DIRECTION('center_axis',(0.157139511089208,0.987363722227819,-0.0204952209812866));
#81954=DIRECTION('ref_axis',(0.208668612810206,-0.0129109291001378,0.977901180047164));
#81955=DIRECTION('center_axis',(-0.158420667613503,0.987363722279252,0.00397139770759942));
#81956=DIRECTION('ref_axis',(0.133625589541009,0.0174544430089088,0.990878168211949));
#81957=DIRECTION('center_axis',(-2.36962999805567E-15,-1.,2.95970545814484E-14));
#81958=DIRECTION('ref_axis',(2.10725079438871E-32,-2.95970545814484E-14,
-1.));
#81959=DIRECTION('center_axis',(0.157871543355326,0.987363722242725,0.0137642943007882));
#81960=DIRECTION('ref_axis',(-0.00642978887167585,-0.0129109278822441,0.999895977467799));
#81961=DIRECTION('center_axis',(-0.155570614016615,0.98736372228924,-0.0301772093081879));
#81962=DIRECTION('ref_axis',(-0.082508018693808,0.0174544402047945,0.996437539120421));
#81963=DIRECTION('center_axis',(0.158340246542571,-0.987363720697896,0.00642256758979644));
#81964=DIRECTION('ref_axis',(-0.00527076112834019,0.0056593145872632,0.999970095170616));
#81965=DIRECTION('',(0.686714765840337,0.,-0.726926977334623));
#81966=DIRECTION('center_axis',(0.161203604208133,-0.986495109513923,-0.0289964979854629));
#81967=DIRECTION('ref_axis',(0.0334320569963806,-0.0239054702440692,0.999155056063573));
#81968=DIRECTION('center_axis',(0.151201360906316,-0.986495109379104,-0.0629725942866305));
#81969=DIRECTION('ref_axis',(0.247439236341897,-0.0239054792976647,0.968608461855505));
#81970=DIRECTION('center_axis',(0.13412911587782,-0.986495109511419,-0.0940041445037833));
#81971=DIRECTION('ref_axis',(0.449876430650253,-0.0239054694228749,0.892770813634194));
#81972=DIRECTION('center_axis',(0.110785139185501,-0.986495109537552,-0.120640174876129));
#81973=DIRECTION('ref_axis',(0.631277905258259,-0.0239054693349842,0.7751881931948));
#81974=DIRECTION('center_axis',(0.0822609672332386,-0.986495109427629,-0.141635208706104));
#81975=DIRECTION('ref_axis',(0.783161525338651,-0.0239054762326219,0.621358635117699));
#81976=DIRECTION('center_axis',(0.0498903701130608,-0.986495109459145,-0.156007531815523));
#81977=DIRECTION('ref_axis',(0.898425384303044,-0.0239054739893283,0.43847503595219));
#81978=DIRECTION('center_axis',(0.0151869524931169,-0.986495109422531,-0.163085117528855));
#81979=DIRECTION('ref_axis',(0.971679868827215,-0.0239054752549652,0.235088835908386));
#81980=DIRECTION('center_axis',(-0.0202265870975381,-0.986495109463458,
-0.162537024025499));
#81981=DIRECTION('ref_axis',(0.999499684133882,-0.0239054723659645,0.0207101377887582));
#81982=DIRECTION('center_axis',(-0.054694359581535,-0.986495109445661,-0.154388879359104));
#81983=DIRECTION('ref_axis',(0.980584004496004,-0.023905475956201,-0.194636939828719));
#81984=DIRECTION('center_axis',(-0.0866046785300437,-0.98649510947863,-0.1390216840333));
#81985=DIRECTION('ref_axis',(0.915817306663047,-0.0239054728221509,-0.400883011844594));
#81986=DIRECTION('center_axis',(-0.114465467498151,-0.986495109349503,-0.117153984054926));
#81987=DIRECTION('ref_axis',(0.808228009920007,-0.0239054802132403,-0.588384238399126));
#81988=DIRECTION('center_axis',(-0.136973968945314,-0.986495109439412,-0.0898083007493744));
#81989=DIRECTION('ref_axis',(0.662846868214859,-0.0239054750836998,-0.748373274214663));
#81990=DIRECTION('center_axis',(-0.153077721692645,-0.986495109512432,-0.0582632820002848));
#81991=DIRECTION('ref_axis',(0.486471746056184,-0.0239054710243431,-0.87336920528729));
#81992=DIRECTION('center_axis',(-0.162023734697267,-0.986495109407243,-0.0239939265302789));
#81993=DIRECTION('ref_axis',(0.287349742887533,-0.023905478144174,-0.957527364296795));
#81994=DIRECTION('center_axis',(-0.16339369481978,-0.986495109410467,0.01139735067332));
#81995=DIRECTION('ref_axis',(0.0747915872978661,-0.0239054772206403,-0.996912607317371));
#81996=DIRECTION('center_axis',(-0.157123548484063,-0.986495109484464,0.0462556966763247));
#81997=DIRECTION('ref_axis',(-0.141263742161791,-0.0239054720233515,-0.989683324886192));
#81998=DIRECTION('center_axis',(-0.143506479156584,-0.986495109461388,0.0789511839610127));
#81999=DIRECTION('ref_axis',(-0.350713731644889,-0.0239054740284668,-0.936177550866924));
#82000=DIRECTION('center_axis',(-0.123179205476089,-0.98649510942288,0.107955001843448));
#82001=DIRECTION('ref_axis',(-0.54376474062529,-0.0239054759324562,-0.838897154049979));
#82002=DIRECTION('center_axis',(-0.0970922114149732,-0.986495109447443,
0.131910960571241));
#82003=DIRECTION('ref_axis',(-0.711389914873902,-0.0239054735609438,-0.702390857962666));
#82004=DIRECTION('center_axis',(-0.0664652930898098,-0.986495109464134,
0.149698910543234));
#82005=DIRECTION('ref_axis',(-0.845751284614566,-0.0239054729384704,-0.533041548977562));
#82006=DIRECTION('center_axis',(-0.0327305254113617,-0.986495109365823,
0.160487108216234));
#82007=DIRECTION('ref_axis',(-0.940566265756416,-0.0239054786927108,-0.338767808106827));
#82008=DIRECTION('center_axis',(0.00253467972596253,-0.986495109391286,
0.163771104123291));
#82009=DIRECTION('ref_axis',(-0.991401414099233,-0.0239054778873439,-0.128653660068495));
#82010=DIRECTION('center_axis',(0.0376813603758679,-0.986495109487736,0.159397346392603));
#82011=DIRECTION('ref_axis',(-0.995879734001976,-0.0239054713375422,0.0874761901564217));
#82012=DIRECTION('center_axis',(0.0710661117949504,-0.986495109438756,0.14757034528578));
#82013=DIRECTION('ref_axis',(-0.953791823912064,-0.0239054744511443,0.299515750720665));
#82014=DIRECTION('center_axis',(0.10112789063694,-0.986495109381306,0.12884311740286));
#82015=DIRECTION('ref_axis',(-0.867105668209388,-0.0239054779846499,0.497550287188617));
#82016=DIRECTION('center_axis',(0.126461037271181,-0.986495109416645,0.104091330807796));
#82017=DIRECTION('ref_axis',(-0.739874616419024,-0.023905476675434,0.672319923967542));
#82018=DIRECTION('center_axis',(0.14588100612832,-0.986495109464053,0.0744723509397584));
#82019=DIRECTION('ref_axis',(-0.578047850450362,-0.0239054740051813,0.815652628820813));
#82020=DIRECTION('center_axis',(0.158479742656197,-0.986495109491895,0.0413711266005706));
#82021=DIRECTION('ref_axis',(-0.389192206378908,-0.023905471580982,0.920846325356413));
#82022=DIRECTION('center_axis',(0.163668143341035,-0.986495109532137,0.00633543404000669));
#82023=DIRECTION('ref_axis',(-0.182138368827764,-0.0239054700782205,0.982982269983086));
#82024=DIRECTION('center_axis',(-0.15968414742932,0.986495108980163,-0.0364468519626609));
#82025=DIRECTION('ref_axis',(-0.0834110839114267,0.0233052156986855,0.996242670237507));
#82026=DIRECTION('center_axis',(0.157820544757278,0.986495109280205,0.0438186606225335));
#82027=DIRECTION('ref_axis',(-0.189267235091296,-0.0133324946527578,0.981835097308723));
#82028=DIRECTION('center_axis',(-0.148115819742677,0.98649510925013,-0.0699221235913883));
#82029=DIRECTION('ref_axis',(-0.295623702609842,0.02330522464751,0.955020153169229));
#82030=DIRECTION('center_axis',(0.144711069366068,0.986495109279994,0.0767209604318213));
#82031=DIRECTION('ref_axis',(-0.395907796897688,-0.0133324986804576,0.918193476798085));
#82032=DIRECTION('center_axis',(-0.129621765649933,0.986495109247231,-0.100127904707367));
#82033=DIRECTION('ref_axis',(-0.49401328476561,0.0233052232947627,0.869141956783973));
#82034=DIRECTION('center_axis',(0.124835066434606,0.986495109301351,0.106035868991504));
#82035=DIRECTION('ref_axis',(-0.584036148783592,-0.0133324983230549,0.811618149995733));
#82036=DIRECTION('center_axis',(-0.105066742164848,0.986495109264697,-0.125651816889763));
#82037=DIRECTION('ref_axis',(-0.669303358386494,0.0233052215977236,0.742623647010275));
#82038=DIRECTION('center_axis',(0.0991219123680177,0.986495109264719,0.130392660396576));
#82039=DIRECTION('ref_axis',(-0.744855620159144,-0.0133325009867863,0.667092459509755));
#82040=DIRECTION('center_axis',(-0.0755989173091877,0.986495109354151,-0.145300388581793));
#82041=DIRECTION('ref_axis',(-0.813297549159958,0.0233052174831723,0.581381082740458));
#82042=DIRECTION('center_axis',(0.0687739335327272,0.986495109263157,0.148652431753765));
#82043=DIRECTION('ref_axis',(-0.870846468817089,-0.0133324967428771,0.491374269044899));
#82044=DIRECTION('center_axis',(-0.0425961641668376,0.986495109300106,-0.15815488018156));
#82045=DIRECTION('ref_axis',(-0.919262851645652,0.0233052217291667,0.392953783827639));
#82046=DIRECTION('center_axis',(0.0352101565309262,0.986495109262151,0.159961383711587));
#82047=DIRECTION('ref_axis',(-0.956117505325965,-0.0133324987105083,0.292679962565576));
#82048=DIRECTION('center_axis',(-0.00760166424791377,0.986495109286655,
-0.163614223263664));
#82049=DIRECTION('ref_axis',(-0.982244445249597,0.0233052224913856,0.186152400953997));
#82050=DIRECTION('center_axis',(-4.18661250280414E-9,0.986495109267288,
0.163790718270974));
#82051=DIRECTION('ref_axis',(-0.996681549668706,-0.0133324966986084,0.0803002682546456));
#82052=DIRECTION('center_axis',(0.0277482857855902,0.986495109197101,-0.161423146314772));
#82053=DIRECTION('ref_axis',(-0.999297379399636,0.0233052282832678,-0.0293532597795325));
#82054=DIRECTION('center_axis',(-0.0352101726580663,0.986495109258677,0.159961380183158));
#82055=DIRECTION('ref_axis',(-0.990641872508763,-0.0133325022384921,-0.135834181325586));
#82056=DIRECTION('center_axis',(0.0618007488839688,0.986495109226498,-0.151684102362711));
#82057=DIRECTION('ref_axis',(-0.969624278718342,0.0233052258209236,-0.243486395039581));
#82058=DIRECTION('center_axis',(-0.0687739426532382,0.986495109277808,0.148652427436938));
#82059=DIRECTION('ref_axis',(-0.938280882830305,-0.0133324980118305,-0.345617171755035));
#82060=DIRECTION('center_axis',(0.0929634778324112,0.986495109264974,-0.134852479345355));
#82061=DIRECTION('ref_axis',(-0.89461262460464,0.0233052233982638,-0.446234376152661));
#82062=DIRECTION('center_axis',(-0.0991219242755312,0.986495109247182,0.130392651477402));
#82063=DIRECTION('ref_axis',(-0.84204692162246,-0.0133324984111526,-0.539239488791627));
#82064=DIRECTION('center_axis',(0.119779342921852,0.98649510919913,-0.111715301259079));
#82065=DIRECTION('ref_axis',(-0.777769877304456,0.0233052267413185,-0.62811693526313));
#82066=DIRECTION('center_axis',(-0.124835075987954,0.986495109277209,0.106035857969037));
#82067=DIRECTION('ref_axis',(-0.706439782054066,-0.0133325009604519,-0.70764756676579));
#82068=DIRECTION('center_axis',(0.140994452051711,0.986495109320719,-0.0833544466536714));
#82069=DIRECTION('ref_axis',(-0.624559478487569,0.023305220786728,-0.780629441230228));
#82070=DIRECTION('center_axis',(-0.144711073722138,0.986495109289194,0.0767209520971159));
#82071=DIRECTION('ref_axis',(-0.537800303819866,-0.0133324954651747,-0.842966830768525));
#82072=DIRECTION('center_axis',(0.155616822593003,0.986495109297831,-0.0510960258485798));
#82073=DIRECTION('ref_axis',(-0.442145367329196,0.0233052210821708,-0.896640586199198));
#82074=DIRECTION('center_axis',(-0.157820545741181,0.986495109287339,0.043818656918217));
#82075=DIRECTION('ref_axis',(-0.344013881227021,-0.0133324941993633,-0.938869902660398));
#82076=DIRECTION('center_axis',(0.162962722649269,0.986495109321916,-0.0164484136219705));
#82077=DIRECTION('ref_axis',(-0.239057033921903,0.0233052199010562,-0.97072581157494));
#82078=DIRECTION('center_axis',(-0.163550504854886,0.986495109300725,0.00886745101273296));
#82079=DIRECTION('ref_axis',(-0.134141752519128,-0.0133324921844451,-0.990872461461741));
#82080=DIRECTION('center_axis',(0.162688667483949,0.986495109300975,0.0189683103505219));
#82081=DIRECTION('ref_axis',(-0.0247906600931756,0.0233052211894522,-0.999420977285076));
#82082=DIRECTION('center_axis',(-0.161633024216997,0.986495109294657,-0.02649839278503));
#82083=DIRECTION('ref_axis',(0.0820026983652642,-0.0133324956280381,-0.996542925327928));
#82084=DIRECTION('center_axis',(0.154807469423538,0.986495109257914,0.053498101096184));
#82085=DIRECTION('ref_axis',(0.190634902087668,0.0233052257812496,-0.981384328669105));
#82086=DIRECTION('center_axis',(-0.152157762777711,0.986495109280064,-0.0606251976738774));
#82087=DIRECTION('ref_axis',(0.294312792599874,-0.0133324957669015,-0.955616149229746));
#82088=DIRECTION('center_axis',(0.139687648469914,0.986495109284146,0.0855263715084811));
#82089=DIRECTION('ref_axis',(0.397146585108484,0.0233052216819088,-0.917459239737127));
#82090=DIRECTION('center_axis',(-0.135567769450184,0.986495109256001,-0.091917241583357));
#82091=DIRECTION('ref_axis',(0.49286114707,-0.0133325031596082,-0.870005824157714));
#82092=DIRECTION('center_axis',(0.118036188482416,0.986495109330827,0.113555525954939));
#82093=DIRECTION('ref_axis',(0.585088132697792,0.0233052199382875,-0.810634778244703));
#82094=DIRECTION('center_axis',(-0.112638782506801,0.986495109231987,-0.118911328883146));
#82095=DIRECTION('ref_axis',(0.668363861819259,-0.0133325005712271,-0.743714994230024));
#82096=DIRECTION('center_axis',(0.0908654815662987,0.98649510920376,0.136274956528284));
#82097=DIRECTION('ref_axis',(0.745671613248655,0.0233052263820281,-0.665905933010384));
#82098=DIRECTION('center_axis',(-0.0844429344226583,0.986495109307055,-0.140345253355262));
#82099=DIRECTION('ref_axis',(0.81261462650057,-0.0133324944657728,-0.582648876587486));
#82100=DIRECTION('center_axis',(0.0594460085246961,0.986495109207123,0.152622316785285));
#82101=DIRECTION('ref_axis',(0.871388316849539,0.0233052276412447,-0.490040067364615));
#82102=DIRECTION('center_axis',(-0.052298619937897,0.986495109270013,-0.155216795930522));
#82103=DIRECTION('ref_axis',(0.918868433255501,-0.0133324996967874,-0.39433874628093));
#82104=DIRECTION('center_axis',(0.025246910107844,0.986495109231267,0.16183322586168));
#82105=DIRECTION('ref_axis',(0.956359871910885,0.0233052243661917,-0.291260470911925));
#82106=DIRECTION('center_axis',(-0.0177088862318153,0.986495109292059,-0.162830570505903));
#82107=DIRECTION('ref_axis',(0.982156973931475,-0.0133324976255219,-0.18758977334821));
#82108=DIRECTION('center_axis',(-0.0101327025401918,0.986495109345222,0.163476994030323));
#82109=DIRECTION('ref_axis',(0.99661310121068,0.0233052186751277,-0.0788618619976393));
#82110=DIRECTION('center_axis',(0.0177088989246918,0.986495109263363,-0.16283056929932));
#82111=DIRECTION('ref_axis',(0.999520945806007,-0.0133324994616411,0.0279306883762481));
#82112=DIRECTION('center_axis',(-0.045038534560328,0.986495109243709,0.157476759691396));
#82113=DIRECTION('ref_axis',(0.99026580966141,0.023305226422398,0.137224242162354));
#82114=DIRECTION('center_axis',(0.0522986285573802,0.986495109283445,-0.155216792940907));
#82115=DIRECTION('ref_axis',(0.970148429509415,-0.0133324940184864,0.242145141028396));
#82116=DIRECTION('center_axis',(-0.0778384024322311,0.98649510932681,0.144113088861088));
#82117=DIRECTION('ref_axis',(0.937614789438134,0.0233052212853708,0.346893893413713));
#82118=DIRECTION('center_axis',(0.0844429366349048,0.986495109286383,-0.140345252169504));
#82119=DIRECTION('ref_axis',(0.895412851334178,-0.0133324926260604,0.445037156095953));
#82120=DIRECTION('center_axis',(-0.106998637769303,0.986495109310485,0.124010849614086));
#82121=DIRECTION('ref_axis',(0.841121944973973,0.0233052212986492,0.540343169054095));
#82122=DIRECTION('center_axis',(0.112638793408809,0.986495109254256,-0.118911318371472));
#82123=DIRECTION('ref_axis',(0.778808761715822,-0.0133324991579478,0.627119731104731));
#82124=DIRECTION('center_axis',(-0.131155737577945,0.98649510924389,0.0981099991757735));
#82125=DIRECTION('ref_axis',(0.705299172575773,0.0233052234911864,0.70852660057471));
#82126=DIRECTION('center_axis',(0.135567778586344,0.986495109306674,-0.0919172275646806));
#82127=DIRECTION('ref_axis',(0.625788442491835,-0.0133324983270567,0.779878881450192));
#82128=DIRECTION('center_axis',(-0.149180137288326,0.986495109329306,0.0676216378683425));
#82129=DIRECTION('ref_axis',(0.536497393132868,0.0233052200227967,0.843580117049546));
#82130=DIRECTION('center_axis',(0.152157765743977,0.986495109271346,-0.0606251903709633));
#82131=DIRECTION('ref_axis',(0.443506950190524,-0.0133324967788789,0.896171763481946));
#82132=DIRECTION('center_axis',(-0.1602290428339,0.986495109287375,0.0339713582981541));
#82133=DIRECTION('ref_axis',(0.342609592811973,0.0233052236259752,0.939188763489511));
#82134=DIRECTION('center_axis',(0.161633025665583,0.98649510926358,-0.0264983851059975));
#82135=DIRECTION('ref_axis',(0.240487563639497,-0.0133324965701397,0.970560650485041));
#82136=DIRECTION('center_axis',(-0.163785814321667,0.986495109358156,-0.00126737501506783));
#82137=DIRECTION('ref_axis',(0.13270175267014,0.0233052181179322,0.990881986740474));
#82138=DIRECTION('center_axis',(0.163550504525506,0.986495109354549,0.00886745109988042));
#82139=DIRECTION('ref_axis',(0.0262232508807231,-0.0133324930323418,0.999567199213134));
#82140=DIRECTION('center_axis',(-0.154963399779559,0.987363722743152,0.0331545432715526));
#82141=DIRECTION('ref_axis',(0.138670756052496,-0.0114882900478161,0.990271902361976));
#82142=DIRECTION('',(-0.72766464391209,0.,-0.685933062332099));
#82143=DIRECTION('center_axis',(1.22396249182026E-14,-1.,8.82303726500718E-14));
#82144=DIRECTION('ref_axis',(-1.12949232739023E-31,-8.82303726500718E-14,
-1.));
#82145=DIRECTION('center_axis',(-0.153863150617874,-0.987363722405381,0.0379342926615524));
#82146=DIRECTION('ref_axis',(0.0666568490087253,0.0279320151284881,0.997384914168592));
#82147=DIRECTION('center_axis',(0.148209443903646,-0.987363722200592,-0.0560967095288448));
#82148=DIRECTION('ref_axis',(0.142449801462467,-0.0348178353517325,0.989189452230827));
#82149=DIRECTION('',(-0.513469942625881,0.,0.858107579514232));
#82150=DIRECTION('center_axis',(-0.144213195008524,0.987363722762328,0.065691958094963));
#82151=DIRECTION('ref_axis',(0.34830789812865,-0.0114882892894636,0.937309781934662));
#82152=DIRECTION('',(-0.858107580390448,0.,-0.513469941161556));
#82153=DIRECTION('center_axis',(5.15339854808296E-15,-1.,1.39227396462689E-14));
#82154=DIRECTION('ref_axis',(-6.63359757292675E-32,-1.39227396462689E-14,
-1.));
#82155=DIRECTION('center_axis',(-0.142111163603627,-0.98736372241876,0.070123439951227));
#82156=DIRECTION('ref_axis',(0.279506722704434,0.0279320160327722,0.959737357011475));
#82157=DIRECTION('center_axis',(0.132685252824785,-0.987363722069216,-0.0866458540522629));
#82158=DIRECTION('ref_axis',(0.351765899733318,-0.0348178403340402,0.935440254521518));
#82159=DIRECTION('',(-0.316997534753803,0.,0.948426361379739));
#82160=DIRECTION('center_axis',(-0.126719744698157,0.98736372284324,0.0951576855370697));
#82161=DIRECTION('ref_axis',(0.541658548276654,-0.0114882834278289,0.840520098761897));
#82162=DIRECTION('',(-0.94842636181411,0.,-0.316997533454207));
#82163=DIRECTION('center_axis',(4.8155354648782E-14,-1.,7.49364324094566E-14));
#82164=DIRECTION('ref_axis',(-1.74406787356792E-31,-7.49364324094566E-14,
-1.));
#82165=DIRECTION('center_axis',(-0.123714216968241,-0.987363722393222,0.0990336923563706));
#82166=DIRECTION('ref_axis',(0.479287174540691,0.0279320157356044,0.877213546873136));
#82167=DIRECTION('center_axis',(0.110956844829601,-0.987363721895533,-0.11314353392952));
#82168=DIRECTION('ref_axis',(0.5446338136483,-0.0348178455852978,0.837950909456937));
#82169=DIRECTION('',(-0.105702677699157,0.,0.994397779526497));
#82170=DIRECTION('center_axis',(-0.103301012505807,0.987363722695783,0.120173956910803));
#82171=DIRECTION('ref_axis',(0.709681848697047,-0.0114882913682037,0.704428628600074));
#82172=DIRECTION('',(-0.994397779862904,0.,-0.105702674534415));
#82173=DIRECTION('center_axis',(6.31386270573628E-14,-1.,6.28324824480148E-14));
#82174=DIRECTION('ref_axis',(1.,6.31386270573628E-14,3.33481401827685E-31));
#82175=DIRECTION('center_axis',(-0.0995325333667008,-0.98736372246363,0.123313236776796));
#82176=DIRECTION('ref_axis',(0.656656687002873,0.0279320125704962,0.75367220864788));
#82177=DIRECTION('center_axis',(0.0840402285537813,-0.987363722249468,-0.134350734907943));
#82178=DIRECTION('ref_axis',(0.712035251163724,-0.034817834568617,0.701279915223704));
#82179=DIRECTION('',(0.110534720558305,0.,0.993872263196381));
#82180=DIRECTION('center_axis',(-0.0750520425157905,0.987363722713108,0.139571021291385));
#82181=DIRECTION('ref_axis',(0.844521214338555,-0.0114882926440067,0.535398858482401));
#82182=DIRECTION('',(-0.993872263160416,0.,0.110534720881691));
#82183=DIRECTION('center_axis',(8.76978752697669E-14,-1.,5.57556479960677E-14));
#82184=DIRECTION('ref_axis',(1.,8.76978752697669E-14,1.18806915830677E-30));
#82185=DIRECTION('center_axis',(-0.0706968179443026,-0.987363722496075,
0.141826793770582));
#82186=DIRECTION('ref_axis',(0.803321666208873,0.0279320113621636,0.594889992637852));
#82187=DIRECTION('center_axis',(0.0531939794800717,-0.987363722280923,-0.149275853608792));
#82188=DIRECTION('ref_axis',(0.846142716066501,-0.0348178326291315,0.531817847179478));
#82189=DIRECTION('',(0.321603636911446,0.,0.946874384871262));
#82190=DIRECTION('center_axis',(-0.0432937294344491,0.987363722805861,0.15244189672989));
#82191=DIRECTION('ref_axis',(0.939871705575629,-0.0114882864976855,0.34133443472891));
#82192=DIRECTION('',(-0.946874383847733,0.,0.321603639924949));
#82193=DIRECTION('center_axis',(8.36857404655723E-14,-1.,3.05139952084908E-14));
#82194=DIRECTION('ref_axis',(1.,8.36857404655723E-14,-4.34665991130318E-31));
#82195=DIRECTION('center_axis',(-0.0385553939103757,-0.987363722414026,
0.153708689608408));
#82196=DIRECTION('ref_axis',(0.912424215593072,0.0279320150912321,0.408291382877855));
#82197=DIRECTION('center_axis',(0.0198604347482932,-0.987363722186018,-0.15722100127712));
#82198=DIRECTION('ref_axis',(0.940685486343554,-0.0348178358371948,0.337488568828939));
#82199=DIRECTION('',(0.517634729095432,0.,0.855601710630769));
#82200=DIRECTION('center_axis',(-0.00951104415543458,0.987363722795096,
0.158184762057801));
#82201=DIRECTION('ref_axis',(0.991274841117851,-0.0114882867674769,0.131309590791865));
#82202=DIRECTION('',(-0.855601711026882,0.,0.517634728440695));
#82203=DIRECTION('center_axis',(7.35740178671048E-14,-1.,9.84219542303022E-15));
#82204=DIRECTION('ref_axis',(1.,7.35740178671048E-14,-2.13993793218284E-31));
#82205=DIRECTION('center_axis',(-0.00461116285625835,-0.987363722349456,
0.158403336345352));
#82206=DIRECTION('ref_axis',(0.978862822739999,0.0279320178453563,0.202601521802199));
#82207=DIRECTION('center_axis',(-0.0144017553816479,-0.98736372226706,-0.157814667863491));
#82208=DIRECTION('ref_axis',(0.991242848386679,-0.0348178325842814,0.127378703307875));
#82209=DIRECTION('',(0.689461790264558,0.,0.724322055280102));
#82210=DIRECTION('center_axis',(0.0247163709221402,0.987363722722755,0.156531083365262));
#82211=DIRECTION('ref_axis',(0.99632706671758,-0.0114882911099796,-0.0848551429986193));
#82212=DIRECTION('',(-0.724322051650169,0.,0.689461794078026));
#82213=DIRECTION('center_axis',(7.39696793198838E-14,-1.,-6.20414865005964E-15));
#82214=DIRECTION('ref_axis',(1.,7.39696793198838E-14,7.83902087019578E-32));
#82215=DIRECTION('center_axis',(0.0295486732720129,-0.987363722463355,0.155691218349561));
#82216=DIRECTION('ref_axis',(0.999530892382157,0.0279320124645528,-0.0125617615567688));
#82217=DIRECTION('center_axis',(-0.04799054642031,-0.987363722052468,-0.151029095968217));
#82218=DIRECTION('ref_axis',(0.995450796857855,-0.0348178397390494,-0.08868725427573));
#82219=DIRECTION('',(0.829050388663707,0.,0.559173902338581));
#82220=DIRECTION('center_axis',(0.0577880672762993,0.987363722787464,0.147558185824273));
#82221=DIRECTION('ref_axis',(0.954792146314158,-0.0114882864052091,-0.297052144601374));
#82222=DIRECTION('',(-0.559173898367332,0.,0.829050391342216));
#82223=DIRECTION('center_axis',(-2.83626402819203E-14,-1.,8.78415744494621E-15));
#82224=DIRECTION('ref_axis',(1.,-2.83626402819203E-14,2.53190229195437E-31));
#82225=DIRECTION('center_axis',(0.0623268522204319,-0.987363722435415,0.145699152745555));
#82226=DIRECTION('ref_axis',(0.973462008503631,0.0279320135103828,-0.227137668873598));
#82227=DIRECTION('center_axis',(-0.0793353368674458,-0.987363722342688,
-0.13718157356482));
#82228=DIRECTION('ref_axis',(0.953112573469767,-0.0348178311350821,-0.300606288904418));
#82229=DIRECTION('',(0.929873511942708,0.,0.36787939842744));
#82230=DIRECTION('center_axis',(0.0881576644780861,0.987363722759926,0.13168563008707));
#82231=DIRECTION('ref_axis',(0.868612205916541,-0.0114882885629135,-0.495359319038914));
#82232=DIRECTION('',(-0.367879397953789,0.,0.929873512130095));
#82233=DIRECTION('center_axis',(5.16224067063556E-14,-1.,-2.93518360182265E-14));
#82234=DIRECTION('ref_axis',(1.,5.16224067063556E-14,-4.26445836114867E-31));
#82235=DIRECTION('center_axis',(0.0921906971087603,-0.987363722419199,0.128894356032774));
#82236=DIRECTION('ref_axis',(0.901875122927973,0.027932014716579,-0.431092873053506));
#82237=DIRECTION('center_axis',(-0.10697050717258,-0.987363722176988,-0.116919590847921));
#82238=DIRECTION('ref_axis',(0.866207865215385,-0.0348178347625664,-0.498469309608377));
#82239=DIRECTION('',(0.987216781687272,0.,0.159383267487605));
#82240=DIRECTION('center_axis',(0.114405106934006,0.98736372273398,0.109655599657815));
#82241=DIRECTION('ref_axis',(0.741816923184193,-0.0114882907434627,-0.6705040429806));
#82242=DIRECTION('',(-0.159383264798036,0.,0.987216782121495));
#82243=DIRECTION('center_axis',(-6.61585895537706E-14,-1.,5.96443467821074E-14));
#82244=DIRECTION('ref_axis',(1.,-6.61585895537706E-14,4.65285739771408E-31));
#82245=DIRECTION('center_axis',(0.117743809112344,-0.987363722349516,0.106062600401007));
#82246=DIRECTION('ref_axis',(0.788117558174073,0.0279320182998367,-0.614890654386155));
#82247=DIRECTION('center_axis',(-0.129603858059164,-0.987363721960494,-0.0911905726075923));
#82248=DIRECTION('ref_axis',(0.738800236790062,-0.0348178427955682,-0.673024463108149));
#82249=DIRECTION('',(0.998398893008149,0.,-0.0565654527083613));
#82250=DIRECTION('center_axis',(0.135303091130996,0.987363722741908,0.0824981972144672));
#82251=DIRECTION('ref_axis',(0.580335108423646,-0.0114882902169116,-0.814296740211335));
#82252=DIRECTION('',(0.0565654558858671,0.,0.998398892828124));
#82253=DIRECTION('center_axis',(4.31583891944395E-14,-1.,-6.03933635467864E-14));
#82254=DIRECTION('ref_axis',(-1.07838066469352E-30,6.03933635467864E-14,
-1.));
#82255=DIRECTION('center_axis',(0.13779134444909,-0.987363722465363,0.0782714823818561));
#82256=DIRECTION('ref_axis',(0.637508495489619,0.0279320123949856,-0.769936829137384));
#82257=DIRECTION('center_axis',(-0.146177065940087,-0.987363722148474,-0.0611975945463366));
#82258=DIRECTION('ref_axis',(0.57684713562104,-0.0348178369452184,-0.816109735486753));
#82259=DIRECTION('',(0.962896981574999,0.,-0.269869232914305));
#82260=DIRECTION('center_axis',(0.149874454570686,0.987363722704243,0.0514832686875784));
#82261=DIRECTION('ref_axis',(0.391717465649994,-0.0114882915735154,-0.920013829385987));
#82262=DIRECTION('',(0.269869235978793,0.,0.962896980716121));
#82263=DIRECTION('center_axis',(5.83331641438036E-15,-1.,-1.36518356314104E-14));
#82264=DIRECTION('ref_axis',(-3.1174917420091E-32,1.36518356314104E-14,
-1.));
#82265=DIRECTION('center_axis',(0.151395914356882,-0.98736372247739,0.0468204725695329));
#82266=DIRECTION('ref_axis',(0.457090239152709,0.0279320119247548,-0.88898161734715));
#82267=DIRECTION('center_axis',(-0.155915201154234,-0.987363722160554,-0.0283430804658039));
#82268=DIRECTION('ref_axis',(0.38792129719992,-0.0348178363740269,-0.921034627714378));
#82269=DIRECTION('',(0.882371077791938,0.,-0.470554227561812));
#82270=DIRECTION('center_axis',(0.15743785313733,0.987363722776465,0.0180610449450756));
#82271=DIRECTION('ref_axis',(0.184783553077732,-0.0114882878011365,-0.9827120930137));
#82272=DIRECTION('',(0.470554230370041,0.,0.882371076294355));
#82273=DIRECTION('center_axis',(8.28658681025308E-15,-1.,-4.37599616907709E-14));
#82274=DIRECTION('ref_axis',(1.06847413692382E-31,4.37599616907709E-14,
-1.));
#82275=DIRECTION('center_axis',(0.15792137988059,-0.987363722452379,0.0131801882229025));
#82276=DIRECTION('ref_axis',(0.25529895511123,0.0279320135506513,-0.966458610669966));
#82277=DIRECTION('center_axis',(-0.158362914256743,-0.987363722293327,0.00583671887090705));
#82278=DIRECTION('ref_axis',(0.180856695325737,-0.0348178310148215,-0.982892961822027));
#82279=DIRECTION('',(0.760586482875992,0.,-0.649236630256125));
#82280=DIRECTION('',(0.649236632676749,0.,0.760586480809747));
#82281=DIRECTION('',(0.60323770876311,0.,-0.797561450125464));
#82282=DIRECTION('center_axis',(0.150470361495174,0.987363722775319,-0.0497146785041838));
#82283=DIRECTION('ref_axis',(-0.244925087799148,-0.0114882879430562,-0.969473940138009));
#82284=DIRECTION('',(0.797561452045313,0.,0.603237706224812));
#82285=DIRECTION('center_axis',(1.80893808345559E-14,-1.,7.19915218327124E-14));
#82286=DIRECTION('ref_axis',(9.00090843414257E-33,-7.19915218327125E-14,
-1.));
#82287=DIRECTION('center_axis',(0.148859780283991,-0.987363722466057,-0.0543474504624917));
#82288=DIRECTION('ref_axis',(-0.174102381956169,0.0279320124232198,-0.984331327998442));
#82289=DIRECTION('center_axis',(-0.141275515076049,-0.987363722429259,0.0717921198366065));
#82290=DIRECTION('ref_axis',(-0.248564947590659,-0.0348178268732931,-0.967989248783825));
#82291=DIRECTION('',(0.417682210743198,0.,-0.90859318224862));
#82292=DIRECTION('center_axis',(0.136265263839099,0.987363722824759,-0.0808990526551015));
#82293=DIRECTION('ref_axis',(-0.447607114670165,-0.0114882833099783,-0.89415652446495));
#82294=DIRECTION('',(0.908593184668933,0.,0.417682205478239));
#82295=DIRECTION('center_axis',(-6.62850207133685E-15,-1.,-1.32839436008182E-14));
#82296=DIRECTION('ref_axis',(-1.03424838227994E-31,1.32839436008182E-14,
-1.));
#82297=DIRECTION('center_axis',(0.13369642391556,-0.987363722333989,-0.0850772945677055));
#82298=DIRECTION('ref_axis',(-0.381634103862487,0.0279320177142337,-0.923891342721366));
#82299=DIRECTION('center_axis',(-0.122539383911072,-0.987363722169357,0.10048372771035));
#82300=DIRECTION('ref_axis',(-0.450842714588386,-0.0348178357828447,-0.891924080297182));
#82301=DIRECTION('',(0.212596357404932,0.,-0.97714010705638));
#82302=DIRECTION('center_axis',(0.115688547978383,0.987363722716593,-0.108300687578074));
#82303=DIRECTION('ref_axis',(-0.629359530672324,-0.0114882911178694,-0.777029343280615));
#82304=DIRECTION('',(0.977140108330193,0.,0.212596351550206));
#82305=DIRECTION('center_axis',(-9.32918656287232E-15,-1.,-1.15484403507104E-14));
#82306=DIRECTION('ref_axis',(-1.52838407231594E-31,1.15484403507104E-14,
-1.));
#82307=DIRECTION('center_axis',(0.112281573151259,-0.987363722364002,-0.111829012739007));
#82308=DIRECTION('ref_axis',(-0.571321039142443,0.0279320163939665,-0.820251225353164));
#82309=DIRECTION('center_axis',(-0.0980734510977039,-0.987363722252895,
0.124476817796301));
#82310=DIRECTION('ref_axis',(-0.632039572503668,-0.0348178343586433,-0.774153535934542));
#82311=DIRECTION('',(-0.00243026757266593,0.,-0.999997046895402));
#82312=DIRECTION('center_axis',(0.0897023691207246,0.98736372275528,-0.130638294389373));
#82313=DIRECTION('ref_axis',(-0.781683795070389,-0.0114882888628608,-0.623569133090596));
#82314=DIRECTION('',(0.999997046887668,0.,-0.00243027075520032));
#82315=DIRECTION('center_axis',(-6.95618921132794E-14,-1.,-5.56376694227202E-14));
#82316=DIRECTION('ref_axis',(1.,-6.95618921132794E-14,2.8891161799313E-32));
#82317=DIRECTION('center_axis',(0.0856165603819998,-0.987363722387814,-0.133351731525449));
#82318=DIRECTION('ref_axis',(-0.734293637815565,0.0279320161221314,-0.678257072162861));
#82319=DIRECTION('center_axis',(-0.0690217128897348,-0.987363722232314,
0.142649511633647));
#82320=DIRECTION('ref_axis',(-0.783682965940413,-0.0348178332220065,-0.620184430137167));
#82321=DIRECTION('',(-0.217343253631377,0.,-0.976095236183912));
#82322=DIRECTION('center_axis',(0.0595218040036869,0.987363722728397,-0.146867402401171));
#82323=DIRECTION('ref_axis',(-0.897457392777709,-0.0114882912460929,-0.440951524901414));
#82324=DIRECTION('',(0.976095235356397,0.,-0.217343257347773));
#82325=DIRECTION('center_axis',(-1.06528037232494E-13,-1.,-5.25108546845533E-14));
#82326=DIRECTION('ref_axis',(1.,-1.06528037232494E-13,-8.41003740475711E-31));
#82327=DIRECTION('center_axis',(0.0549482133195925,-0.98736372243382,-0.14863907115767));
#82328=DIRECTION('ref_axis',(-0.862931481368871,0.0279320151382408,-0.504548373293229));
#82329=DIRECTION('center_axis',(-0.0367425905234866,-0.987363722095364,
0.154152075339946));
#82330=DIRECTION('ref_axis',(-0.898682215257586,-0.0348178378225455,-0.437216186970566));
#82331=DIRECTION('',(-0.422093512262599,0.,-0.906552296839969));
#82332=DIRECTION('center_axis',(0.0265580714999559,0.987363722790579,-0.156229151426141));
#82333=DIRECTION('ref_axis',(-0.971266881255812,-0.0114882866172744,-0.237715512001651));
#82334=DIRECTION('',(0.906552294984449,0.,-0.422093516247796));
#82335=DIRECTION('center_axis',(1.44157190590594E-14,-1.,3.54785012783786E-15));
#82336=DIRECTION('ref_axis',(1.,1.44157190590594E-14,-6.21377867058364E-32));
#82337=DIRECTION('center_axis',(0.0217105441157315,-0.987363722315354,-0.156976215172135));
#82338=DIRECTION('ref_axis',(-0.951219608639794,0.0279320193667842,-0.307247552363319));
#82339=DIRECTION('center_axis',(-0.00274543728998556,-0.987363722329321,
0.158446654751922));
#82340=DIRECTION('ref_axis',(-0.97166008011877,-0.0348178304814863,-0.233804207370502));
#82341=DIRECTION('',(-0.6071071473932,0.,-0.794619979351194));
#82342=DIRECTION('center_axis',(-0.0076474896256404,0.987363722817488,-0.158285800899564));
#82343=DIRECTION('ref_axis',(-0.999661009578761,-0.0114882853853447,-0.0233641868439042));
#82344=DIRECTION('',(0.794619977419008,0.,-0.607107149922166));
#82345=DIRECTION('center_axis',(-7.42068524027303E-14,-1.,-1.82974945934095E-15));
#82346=DIRECTION('ref_axis',(-0.99969614439276,7.42294074245818E-14,-0.0246499266986752));
#82347=DIRECTION('center_axis',(-0.0125422745102943,-0.987363722475656,
-0.157973323346459));
#82348=DIRECTION('ref_axis',(-0.995029764692228,0.0279320112165366,-0.0955801764275887));
#82349=DIRECTION('center_axis',(0.0313800969965281,-0.987363722278222,0.155332448127826));
#82350=DIRECTION('ref_axis',(-0.999204200729344,-0.0348178311476597,-0.0194598016178513));
#82351=DIRECTION('',(-0.763733125487799,0.,-0.645532116189921));
#82352=DIRECTION('center_axis',(-0.0414954679937745,0.987363722747479,-0.152941181956391));
#82353=DIRECTION('ref_axis',(-0.981312099500299,-0.0114882890458985,0.192079625648099));
#82354=DIRECTION('',(0.64553211208243,0.,-0.763733128959585));
#82355=DIRECTION('',(-0.884647793282078,0.,-0.466259886588103));
#82356=DIRECTION('center_axis',(0.,-1.,0.));
#82357=DIRECTION('ref_axis',(0.,0.,-1.));
#82358=DIRECTION('center_axis',(-0.0462086416140792,-0.987363722411243,
-0.151583775867986));
#82359=DIRECTION('ref_axis',(-0.992313434186013,0.0279320148958749,0.120556421968377));
#82360=DIRECTION('center_axis',(0.0640383411135482,-0.987363722029644,0.144955066441962));
#82361=DIRECTION('ref_axis',(-0.980026643477236,-0.0348178399924535,0.19579452518649));
#82362=DIRECTION('',(0.46625988377264,0.,-0.884647794765987));
#82363=DIRECTION('center_axis',(-0.0734031560636246,0.98736372281198,-0.140445204812293));
#82364=DIRECTION('ref_axis',(-0.917078127633942,-0.0114882850235305,0.398542001704515));
#82365=DIRECTION('center_axis',(0.,-1.,0.));
#82366=DIRECTION('ref_axis',(0.,0.,-1.));
#82367=DIRECTION('center_axis',(-0.077714340139779,-0.98736372241589,-0.138106339440582));
#82368=DIRECTION('ref_axis',(-0.943197630236814,0.0279320146514098,0.331055936169662));
#82369=DIRECTION('center_axis',(0.093702206075612,-0.98736372236211,0.12779975093795));
#82370=DIRECTION('ref_axis',(-0.915024129431169,-0.0348178301339077,0.401893718865446));
#82371=DIRECTION('',(-0.964197312368427,0.,-0.265185864671369));
#82372=DIRECTION('center_axis',(-0.101878603038959,0.987363722747707,-0.121382161970443));
#82373=DIRECTION('ref_axis',(-0.809962599989905,-0.0114882903200018,0.586369001400241));
#82374=DIRECTION('',(0.265185861599813,0.,-0.964197313213206));
#82375=DIRECTION('center_axis',(-3.61097266571981E-14,-1.,2.60708536588153E-14));
#82376=DIRECTION('ref_axis',(1.,-3.61097266571981E-14,7.16384221097358E-31));
#82377=DIRECTION('center_axis',(-0.105586200624493,-0.987363722469058,-0.118171205417098));
#82378=DIRECTION('ref_axis',(-0.849978954034902,0.027932012352796,0.526075641313735));
#82379=DIRECTION('center_axis',(0.118984673112858,-0.987363722197065,0.104668656499369));
#82380=DIRECTION('ref_axis',(-0.807236104611648,-0.0348178350983758,0.589200805982541));
#82381=DIRECTION('',(-0.998662037017743,0.,-0.0517120471415683));
#82382=DIRECTION('center_axis',(-0.125590314053738,0.987363722735068,-0.0966434273121139));
#82383=DIRECTION('ref_axis',(-0.664974122526173,-0.0114882892188372,0.746778036354425));
#82384=DIRECTION('',(0.0517120410961091,0.,-0.998662037330785));
#82385=DIRECTION('center_axis',(5.93220768500817E-14,-1.,-6.64477108557578E-14));
#82386=DIRECTION('ref_axis',(-4.62814580839856E-31,6.64477108557578E-14,
-1.));
#82387=DIRECTION('center_axis',(-0.12852097045819,-0.987363722436845,-0.0927105159523013));
#82388=DIRECTION('ref_axis',(-0.71701620639877,0.0279320129697168,0.696496634889915));
#82389=DIRECTION('center_axis',(0.138703544670002,-0.98736372222561,0.0766433736781297));
#82390=DIRECTION('ref_axis',(-0.661702615127607,-0.0348178349574889,0.748957520492423));
#82391=DIRECTION('',(-0.986430434661682,0.,0.164179772119362));
#82392=DIRECTION('center_axis',(-0.143429559359027,0.987363722836541,-0.0673857576082798));
#82393=DIRECTION('ref_axis',(-0.488892194469872,-0.0114882833766482,0.872268560439668));
#82394=DIRECTION('',(-0.164179775258991,0.,-0.986430434139127));
#82395=DIRECTION('center_axis',(1.45502886631244E-14,-1.,-2.58822310819358E-14));
#82396=DIRECTION('ref_axis',(3.34261249505911E-31,2.58822310819358E-14,
-1.));
#82397=DIRECTION('center_axis',(-0.145446240355865,-0.987363722521506,-0.0629147885223953));
#82398=DIRECTION('ref_axis',(-0.550526577599503,0.0279320098890628,0.834350220339238));
#82399=DIRECTION('center_axis',(0.151936792278092,-0.987363722246792,0.0450343329383656));
#82400=DIRECTION('ref_axis',(-0.485228646736117,-0.0348178338663002,0.873693812975401));
#82401=DIRECTION('',(-0.928074440978592,0.,0.372394726066675));
#82402=DIRECTION('center_axis',(-0.154562204409905,0.987363722712876,-0.0349771931195304));
#82403=DIRECTION('ref_axis',(-0.289950209006206,-0.0114882910818072,0.956972776762891));
#82404=DIRECTION('',(-0.372394728026814,0.,-0.928074440192076));
#82405=DIRECTION('center_axis',(8.64619638763411E-15,-1.,-2.84050008514506E-14));
#82406=DIRECTION('ref_axis',(-1.15512849116693E-31,2.84050008514506E-14,
-1.));
#82407=DIRECTION('center_axis',(-0.155570610176543,-0.987363722363232,-0.0301772266837314));
#82408=DIRECTION('ref_axis',(-0.358294937629885,0.0279320170368305,0.933190516504026));
#82409=DIRECTION('center_axis',(0.158065646374136,-0.987363722077046,0.0113195301354719));
#82410=DIRECTION('ref_axis',(-0.286065929346506,-0.0348178405079036,0.957577152008905));
#82411=DIRECTION('',(-0.826322717534286,0.,0.563196916261757));
#82412=DIRECTION('center_axis',(-0.158467688071278,0.987363722788458,-0.000933144502251157));
#82413=DIRECTION('ref_axis',(-0.0774504756911478,-0.0114882872480132,0.99693000911364));
#82414=DIRECTION('',(-0.563196917553715,0.,-0.826322716653726));
#82415=DIRECTION('center_axis',(-9.3512703384342E-15,-1.,1.18398337479732E-13));
#82416=DIRECTION('ref_axis',(2.38006789847537E-31,-1.18398337479732E-13,
-1.));
#82417=DIRECTION('center_axis',(-0.158420667211256,-0.987363722412121,0.00397138071973608));
#82418=DIRECTION('ref_axis',(-0.149309823991232,0.0279320148995181,0.988395861486358));
#82419=DIRECTION('center_axis',(0.15680352394228,-0.987363722029905,-0.0229245566704076));
#82420=DIRECTION('ref_axis',(-0.073527080722506,-0.0348178407589832,0.996685249396874));
#82421=DIRECTION('',(-0.68593306312575,0.,0.727664643163955));
#82422=DIRECTION('',(0.761154167860895,0.,-0.648570992835779));
#82423=DIRECTION('center_axis',(0.153257689897193,-0.987363722734368,0.0403107865900156));
#82424=DIRECTION('ref_axis',(-0.18881520529075,0.0107821800906864,0.98195344229933));
#82425=DIRECTION('center_axis',(-0.154002417765247,-0.987363721883716,-0.0373649037252043));
#82426=DIRECTION('ref_axis',(-0.188347474697552,-0.00778744783873706,0.982071578058959));
#82427=DIRECTION('',(0.46978211759282,0.,0.882782397870509));
#82428=DIRECTION('center_axis',(1.1099822106242E-14,-1.,-5.83369275286436E-14));
#82429=DIRECTION('ref_axis',(8.44183654759075E-32,5.83369275286436E-14,
-1.));
#82430=DIRECTION('center_axis',(0.157871543102446,0.98736372238965,0.0137642866617665));
#82431=DIRECTION('ref_axis',(-0.111617347157657,0.0039934990218299,0.9937432363438));
#82432=DIRECTION('center_axis',(-0.145446222113249,0.98736372086277,-0.0629148567272404));
#82433=DIRECTION('ref_axis',(-0.191537738360655,0.0342871344957478,0.980886174431955));
#82434=DIRECTION('',(0.88278239777599,0.,-0.469782117770433));
#82435=DIRECTION('center_axis',(0.141008981378088,-0.987363722661823,0.072314219501428));
#82436=DIRECTION('ref_axis',(-0.395491774985701,0.0107821839268003,0.918406228435124));
#82437=DIRECTION('center_axis',(-0.14236957508107,-0.987363721868668,-0.0695973047530321));
#82438=DIRECTION('ref_axis',(-0.395060375331871,-0.00778745240990678,0.918622150520879));
#82439=DIRECTION('',(0.269026752423883,0.,0.96313270450144));
#82440=DIRECTION('center_axis',(1.75357720831305E-14,-1.,-4.09401817359017E-14));
#82441=DIRECTION('ref_axis',(-1.24101159417695E-32,4.09401817359017E-14,
-1.));
#82442=DIRECTION('center_axis',(0.151221679088276,0.98736372240244,0.0473802011110068));
#82443=DIRECTION('ref_axis',(-0.322633218628695,0.0039934985935031,0.946515640761563));
#82444=DIRECTION('center_axis',(-0.128520934758922,0.987363720788093,-0.0927105829999236));
#82445=DIRECTION('ref_axis',(-0.397921226436083,0.0342871368088993,0.916778648203072));
#82446=DIRECTION('',(0.963132705018708,0.,-0.269026750572033));
#82447=DIRECTION('center_axis',(0.122166850775448,-0.987363722682965,0.100936315076614));
#82448=DIRECTION('ref_axis',(-0.583675588839591,0.010782182662631,0.811915359831175));
#82449=DIRECTION('center_axis',(-0.124079693435435,-0.987363721896849,-0.0985754044321944));
#82450=DIRECTION('ref_axis',(-0.583300690181401,-0.0077874473065718,0.812218973244499));
#82451=DIRECTION('',(0.0556919954647298,0.,0.998447996463089));
#82452=DIRECTION('center_axis',(-4.32112072582799E-14,-1.,6.03555839612015E-14));
#82453=DIRECTION('ref_axis',(5.52801095037507E-31,-6.03555839612015E-14,
-1.));
#82454=DIRECTION('center_axis',(0.137500857919074,0.987363722378521,0.0787806689635775));
#82455=DIRECTION('ref_axis',(-0.518563117419946,0.00399349906777367,0.855030025915408));
#82456=DIRECTION('center_axis',(-0.10558615361227,0.987363720860938,-0.118171260859017));
#82457=DIRECTION('ref_axis',(-0.585698356105705,0.0342871345631837,0.809803573750154));
#82458=DIRECTION('',(0.998447996527099,0.,-0.05569199431715));
#82459=DIRECTION('center_axis',(0.0976123324921318,-0.987363722657208,0.124838742888357));
#82460=DIRECTION('ref_axis',(-0.744567380952206,0.0107821840596194,0.66746023082194));
#82461=DIRECTION('center_axis',(-0.0999879825042087,-0.987363721894786,
-0.122944231425527));
#82462=DIRECTION('ref_axis',(-0.744266513551164,-0.00778744565864629,0.66783733984894));
#82463=DIRECTION('',(-0.160246858747463,0.,0.987076969775696));
#82464=DIRECTION('center_axis',(-5.51756196524937E-14,-1.,4.96553716611219E-14));
#82465=DIRECTION('ref_axis',(1.,-5.51756196524937E-14,5.66722537932442E-31));
#82466=DIRECTION('center_axis',(0.117350647949358,0.987363722424568,0.10649744159259));
#82467=DIRECTION('ref_axis',(-0.690245581144517,0.0039934975576326,0.723564157271299));
#82468=DIRECTION('center_axis',(-0.0777142754592605,0.98736372070586,-0.138106388062694));
#82469=DIRECTION('ref_axis',(-0.746088886902966,0.0342871399768338,0.664962980076412));
#82470=DIRECTION('',(0.987076969591517,0.,0.160246859881955));
#82471=DIRECTION('center_axis',(0.0684935700481875,-0.987363722645525,0.142903849023131));
#82472=DIRECTION('ref_axis',(-0.870644028746578,0.0107821851182117,0.491795404301427));
#82473=DIRECTION('center_axis',(-0.0712209419243646,-0.987363721889244,
-0.141564325055521));
#82474=DIRECTION('ref_axis',(-0.870431263362817,-0.0077874473242738,0.492228373242321));
#82475=DIRECTION('',(-0.368692746674862,0.,0.929551321094939));
#82476=DIRECTION('center_axis',(-9.03841140943282E-14,-1.,5.12866612338516E-14));
#82477=DIRECTION('ref_axis',(1.,-9.03841140943282E-14,2.57510117333047E-31));
#82478=DIRECTION('center_axis',(0.0917132551111147,0.987363722365359,0.129234510072762));
#82479=DIRECTION('ref_axis',(-0.829652928099899,0.00399349968643042,0.558265233428985));
#82480=DIRECTION('center_axis',(-0.0462085670591155,0.987363720688045,-0.151583809819533));
#82481=DIRECTION('ref_axis',(-0.871593127806196,0.0342871408666792,0.489029458757037));
#82482=DIRECTION('',(0.929551320671185,0.,0.368692747743234));
#82483=DIRECTION('center_axis',(0.036172125985831,-0.987363722634944,0.154286929213499));
#82484=DIRECTION('ref_axis',(-0.956010329767849,0.0107821842182488,0.293134770848927));
#82485=DIRECTION('center_axis',(-0.0391236905722506,-0.98736372188221,-0.153565027095745));
#82486=DIRECTION('ref_axis',(-0.955895614537263,-0.00778744719550599,0.293603354501621));
#82487=DIRECTION('',(-0.559898972904418,0.,0.828560884993117));
#82488=DIRECTION('center_axis',(8.51109427279946E-14,-1.,-2.62780241083103E-14));
#82489=DIRECTION('ref_axis',(1.,8.51109427279946E-14,-1.61762959713368E-31));
#82490=DIRECTION('center_axis',(0.0617874444496923,0.987363722445373,0.145928719953246));
#82491=DIRECTION('ref_axis',(-0.930266626826431,0.00399349312500233,0.366862447009278));
#82492=DIRECTION('center_axis',(-0.0125422004180125,0.987363720749498,-0.157973340017808));
#82493=DIRECTION('ref_axis',(-0.956342642361099,0.0342871387732709,0.290229465279688));
#82494=DIRECTION('',(0.82856088525082,0.,0.55989897252306));
#82495=DIRECTION('center_axis',(0.00215930871990054,-0.987363722594613,
0.15845572469924));
#82496=DIRECTION('ref_axis',(-0.996674650224871,0.0107821882209069,0.0807674811808595));
#82497=DIRECTION('center_axis',(-0.00519705505445424,-0.987363721855407,
-0.158385199379862));
#82498=DIRECTION('ref_axis',(-0.99666334859478,-0.00778745117250021,0.0812497702893763));
#82499=DIRECTION('',(-0.724924943069254,0.,0.6888278645032));
#82500=DIRECTION('center_axis',(0.,-1.,0.));
#82501=DIRECTION('ref_axis',(0.,0.,-1.));
#82502=DIRECTION('center_axis',(0.0289725338065441,0.987363722367401,0.155799460967034));
#82503=DIRECTION('ref_axis',(-0.987382091802038,0.00399349993332521,0.158305580277241));
#82504=DIRECTION('center_axis',(0.0217106310419858,0.987363720643665,-0.156976213664544));
#82505=DIRECTION('ref_axis',(-0.996374638587734,0.0342871422369901,0.0778586633354473));
#82506=DIRECTION('',(0.688827863670013,0.,0.724924943860953));
#82507=DIRECTION('center_axis',(-0.0319544657509305,-0.987363722688464,
0.15521530606661));
#82508=DIRECTION('ref_axis',(-0.99073557192863,0.0107821823962816,-0.13537640510083));
#82509=DIRECTION('center_axis',(0.0289725837152514,-0.987363721882134,-0.155799454761312));
#82510=DIRECTION('ref_axis',(-0.990828212218113,-0.00778744957994967,-0.134902963279899));
#82511=DIRECTION('',(-0.856054231466657,0.,0.516886015276125));
#82512=DIRECTION('center_axis',(-1.47130759122275E-14,-1.,-1.9813114182039E-15));
#82513=DIRECTION('ref_axis',(1.,-1.47130759122275E-14,-5.10197245919429E-32));
#82514=DIRECTION('center_axis',(-0.00519711077038148,0.987363722453804,
0.158385193821289));
#82515=DIRECTION('ref_axis',(-0.998328667570516,0.00399349550016951,-0.057653477783817));
#82516=DIRECTION('center_axis',(0.0549482872906021,0.987363720830978,-0.148639054459575));
#82517=DIRECTION('ref_axis',(-0.989817264642019,0.0342871350541035,-0.138152723412795));
#82518=DIRECTION('',(0.516886016398843,0.,0.85605423078876));
#82519=DIRECTION('center_axis',(-0.0645740904836284,-0.987363722683157,
0.144717193061053));
#82520=DIRECTION('ref_axis',(-0.938470799614058,0.0107821821538341,-0.34519024148975));
#82521=DIRECTION('center_axis',(0.061787500539433,-0.987363721862154,-0.145928700150466));
#82522=DIRECTION('ref_axis',(-0.938663049981464,-0.00778745220173615,-0.344747783441317));
#82523=DIRECTION('',(-0.947155372266923,0.,0.320775156123267));
#82524=DIRECTION('center_axis',(-6.97158450332253E-14,-1.,-2.54893293604934E-14));
#82525=DIRECTION('ref_axis',(1.,-6.97158450332253E-14,5.10773051084881E-31));
#82526=DIRECTION('center_axis',(-0.0391237406597983,0.987363722421879,0.15356501086509));
#82527=DIRECTION('ref_axis',(-0.96259450430855,0.00399349509328662,-0.270916725714593));
#82528=DIRECTION('center_axis',(0.0856166299241214,0.987363720838917,-0.133351698345259));
#82529=DIRECTION('ref_axis',(-0.936977134491496,0.0342871348173222,-0.347704244762878));
#82530=DIRECTION('',(0.320775152455668,0.,0.947155373509037));
#82531=DIRECTION('center_axis',(-0.0941743021688814,-0.987363722710651,
0.127452265126865));
#82532=DIRECTION('ref_axis',(-0.842324175661386,0.0107821814342959,-0.538863366411083));
#82533=DIRECTION('center_axis',(0.0917132966142065,-0.98736372187387,-0.129234484374461));
#82534=DIRECTION('ref_axis',(-0.842607046355374,-0.00778744790203565,-0.538472581555872));
#82535=DIRECTION('',(-0.993968582433906,0.,0.10966520475671));
#82536=DIRECTION('center_axis',(0.,-1.,0.));
#82537=DIRECTION('ref_axis',(0.,0.,-1.));
#82538=DIRECTION('center_axis',(-0.0712209816399244,0.987363722372652,0.141564301703027));
#82539=DIRECTION('ref_axis',(-0.881850493045238,0.00399350132227135,-0.471512205423211));
#82540=DIRECTION('center_axis',(0.112281636624268,0.987363720745417,-0.111828963299954));
#82541=DIRECTION('ref_axis',(-0.840324996204307,0.0342871383705696,-0.540997498050211));
#82542=DIRECTION('',(0.109665200774071,0.,0.993968582873313));
#82543=DIRECTION('center_axis',(-0.11937103403139,-0.987363722603769,0.104227805888375));
#82544=DIRECTION('ref_axis',(-0.706791409383475,0.0107821886588213,-0.707339839136356));
#82545=DIRECTION('center_axis',(0.117350683385862,-0.987363721880914,-0.106497407585072));
#82546=DIRECTION('ref_axis',(-0.707151675129846,-0.00778744623160996,-0.707018998360188));
#82547=DIRECTION('',(-0.994304926390161,0.,-0.106572573189616));
#82548=DIRECTION('center_axis',(7.3597573916883E-14,-1.,7.33689771798346E-14));
#82549=DIRECTION('ref_axis',(1.,7.3597573916883E-14,9.18989021195146E-31));
#82550=DIRECTION('center_axis',(-0.0999880192034275,0.987363722417957,0.122944197377228));
#82551=DIRECTION('ref_axis',(-0.759872130882321,0.00399349582696179,-0.650060302356205));
#82552=DIRECTION('center_axis',(0.133696477668497,0.987363720680591,-0.0850772292850251));
#82553=DIRECTION('ref_axis',(-0.704380193370113,0.0342871409978466,-0.708994312494872));
#82554=DIRECTION('',(-0.106572574332393,0.,0.994304926267675));
#82555=DIRECTION('center_axis',(-0.138986101728336,-0.987363722614939,0.0761297759771471));
#82556=DIRECTION('ref_axis',(-0.538209861740386,0.0107821861776475,-0.842741887642133));
#82557=DIRECTION('center_axis',(0.137500887126174,-0.987363721858741,-0.0787806245010161));
#82558=DIRECTION('ref_axis',(-0.538630675840616,-0.00778745178170863,-0.842505994422728));
#82559=DIRECTION('',(-0.94814867668019,0.,-0.317827133690004));
#82560=DIRECTION('center_axis',(6.41197054336129E-14,-1.,9.99713762191257E-14));
#82561=DIRECTION('ref_axis',(-4.18067723980065E-31,-9.99713762191257E-14,
-1.));
#82562=DIRECTION('center_axis',(-0.124079723161249,0.987363722414627,0.0985753618292045));
#82563=DIRECTION('ref_axis',(-0.602362992892309,0.00399349586706796,-0.798212300572085));
#82564=DIRECTION('center_axis',(0.148859815873385,0.987363720773916,-0.054347383723873));
#82565=DIRECTION('ref_axis',(-0.535499356440476,0.0342871370330924,-0.8438393398544));
#82566=DIRECTION('',(-0.317827133913437,0.,0.948148676605294));
#82567=DIRECTION('center_axis',(-0.152102334827415,-0.987363722642613,0.0444720018592623));
#82568=DIRECTION('ref_axis',(-0.344462219111818,0.0107821847411895,-0.938738261762441));
#82569=DIRECTION('center_axis',(0.151221697237912,-0.987363721876949,-0.0473801541342403));
#82570=DIRECTION('ref_axis',(-0.344923905103641,-0.00778744840236856,-0.938598346117995));
#82571=DIRECTION('',(-0.85765804862894,0.,-0.514220450412077));
#82572=DIRECTION('center_axis',(1.5423649336475E-14,-1.,4.17817283315104E-14));
#82573=DIRECTION('ref_axis',(-3.87248343031339E-31,-4.17817283315104E-14,
-1.));
#82574=DIRECTION('center_axis',(-0.142369594341165,0.987363722348721,0.0695972585437816));
#82575=DIRECTION('ref_axis',(-0.416688032452796,0.00399350289763168,-0.909040777713092));
#82576=DIRECTION('center_axis',(0.157062637484616,0.987363720750114,-0.021076310228941));
#82577=DIRECTION('ref_axis',(-0.341579164027156,0.0342871386853031,-0.939227377594629));
#82578=DIRECTION('',(-0.514220451397814,0.,0.857658048037928));
#82579=DIRECTION('center_axis',(-0.158106432739376,-0.987363722622455,0.0107347648114259));
#82580=DIRECTION('ref_axis',(-0.134607907972329,0.0107821854895616,-0.990840277535881));
#82581=DIRECTION('center_axis',(0.157871551018963,-0.98736372185081,-0.0137642345149945));
#82582=DIRECTION('ref_axis',(-0.135088876457087,-0.00778745163005778,-0.990802882037932));
#82583=DIRECTION('',(-0.727064283330936,0.,-0.686569390451156));
#82584=DIRECTION('center_axis',(1.21624329307288E-14,-1.,8.82410470081755E-14));
#82585=DIRECTION('ref_axis',(1.75892719290299E-32,-8.82410470081755E-14,
-1.));
#82586=DIRECTION('center_axis',(-0.154002425721275,0.987363722322915,0.0373648593279877));
#82587=DIRECTION('ref_axis',(-0.211529202855841,0.00399350306266881,-0.977363519000203));
#82588=DIRECTION('center_axis',(0.157921384382321,0.987363720665047,0.0131802681780967));
#82589=DIRECTION('ref_axis',(-0.131687111262305,0.0342871405833779,-0.990698186491731));
#82590=DIRECTION('',(-0.686569391286805,0.,0.72706428254183));
#82591=DIRECTION('center_axis',(-0.156717649183816,-0.987363722713147,-0.0235044145711971));
#82592=DIRECTION('ref_axis',(0.0815405202994448,0.0107821826469929,-0.996611703767652));
#82593=DIRECTION('center_axis',(0.157139505704567,-0.987363721919153,0.0204952771360236));
#82594=DIRECTION('ref_axis',(0.0810627569208432,-0.00778744642864526,-0.996678576632664));
#82595=DIRECTION('',(-0.562473799699905,0.,-0.826815109109135));
#82596=DIRECTION('center_axis',(7.09113469916638E-15,-1.,-8.8792583730072E-14));
#82597=DIRECTION('ref_axis',(1.79109581697142E-31,8.8792583730072E-14,-1.));
#82598=DIRECTION('center_axis',(-0.158434274586989,0.987363722374258,0.00338531761353594));
#82599=DIRECTION('ref_axis',(0.00352049925138151,0.00399350036430735,-0.999985828919521));
#82600=DIRECTION('center_axis',(0.151395902272578,0.987363720784873,0.0468205473368705));
#82601=DIRECTION('ref_axis',(0.0843624842551672,0.034287137723654,-0.995845049913397));
#82602=DIRECTION('',(-0.826815108418627,0.,0.562473800714926));
#82603=DIRECTION('center_axis',(-0.148000923743781,-0.98736372267634,-0.0566445559052908));
#82604=DIRECTION('ref_axis',(0.293876205497284,0.0107821818853998,-0.955782674249909));
#82605=DIRECTION('center_axis',(0.149059792165184,-0.987363721865846,0.0537964599476181));
#82606=DIRECTION('ref_axis',(0.293423987027018,-0.00778744878999118,-0.955950688832071));
#82607=DIRECTION('',(-0.371582668334801,0.,-0.928399871064828));
#82608=DIRECTION('center_axis',(0.,-1.,0.));
#82609=DIRECTION('ref_axis',(0.,0.,-1.));
#82610=DIRECTION('center_axis',(-0.155457912687852,0.987363722342951,-0.0307525150810125));
#82611=DIRECTION('ref_axis',(0.218405587602123,0.00399350060691493,-0.975849912259603));
#82612=DIRECTION('center_axis',(0.137791315732748,0.987363720667919,0.0782715556089313));
#82613=DIRECTION('ref_axis',(0.296467386930115,0.0342871404434376,-0.954427304977724));
#82614=DIRECTION('',(-0.928399871491895,0.,0.371582667267774));
#82615=DIRECTION('center_axis',(-0.132363838760895,-0.987363722668939,-0.0871360622579147));
#82616=DIRECTION('ref_axis',(0.492470564867695,0.0107821829897946,-0.870262309461273));
#82617=DIRECTION('center_axis',(0.134010209521018,-0.987363721882876,0.0845821757448213));
#82618=DIRECTION('ref_axis',(0.492065037535445,-0.00778744648125535,-0.870523609394107));
#82619=DIRECTION('',(-0.163316741957422,0.,-0.986573687970854));
#82620=DIRECTION('center_axis',(-4.37187777539197E-14,-1.,7.76084762604717E-14));
#82621=DIRECTION('ref_axis',(-3.72167831404108E-31,-7.76084762604717E-14,
-1.));
#82622=DIRECTION('center_axis',(-0.145212512392347,0.987363722361678,-0.0634523916711932));
#82623=DIRECTION('ref_axis',(0.423078269486658,0.00399350308370285,-0.906084339242929));
#82624=DIRECTION('center_axis',(0.117743765163003,0.98736372094914,0.106062662227139));
#82625=DIRECTION('ref_axis',(0.494709800043066,0.0342871317601711,-0.868381601795553));
#82626=DIRECTION('',(-0.986573688235236,0.,0.16331674036033));
#82627=DIRECTION('center_axis',(-0.110537568239643,-0.987363722654522,-0.113553182225208));
#82628=DIRECTION('ref_axis',(0.668037549826968,0.0107821826083705,-0.744049444969473));
#82629=DIRECTION('center_axis',(0.112694458303171,-0.987363721903264,0.111412924461612));
#82630=DIRECTION('ref_axis',(0.667697674265223,-0.00778744546243803,-0.74439181314277));
#82631=DIRECTION('',(0.0525856941427118,0.,-0.99861641523236));
#82632=DIRECTION('center_axis',(-2.96900927039073E-14,-1.,3.31978941985153E-14));
#82633=DIRECTION('ref_axis',(-2.03427355717816E-31,-3.31978941985153E-14,
-1.));
#82634=DIRECTION('center_axis',(-0.128177133532957,0.987363722358752,-0.0931853111232876));
#82635=DIRECTION('ref_axis',(0.607968284882378,0.00399349903820969,-0.793951268367657));
#82636=DIRECTION('center_axis',(0.0921906441866638,0.987363720942169,0.128894405199308));
#82637=DIRECTION('ref_axis',(0.669820133955363,0.0342871320156405,-0.741731339991888));
#82638=DIRECTION('',(-0.998616415322888,0.,-0.0525856924235507));
#82639=DIRECTION('center_axis',(-0.0835426829196343,-0.987363722641279,
-0.134660682244467));
#82640=DIRECTION('ref_axis',(0.812367839804286,0.0107821836697777,-0.5830456563315));
#82641=DIRECTION('center_axis',(0.086109234869091,-0.987363721866257,0.133034132509938));
#82642=DIRECTION('ref_axis',(0.812109509998393,-0.00778745053491031,-0.583453082419088));
#82643=DIRECTION('',(0.266029277211529,0.,-0.963964949397182));
#82644=DIRECTION('center_axis',(-2.40883471761575E-14,-1.,1.73595023882834E-14));
#82645=DIRECTION('ref_axis',(1.,-2.40883471761575E-14,-4.21994572424516E-31));
#82646=DIRECTION('center_axis',(-0.105148334878442,0.98736372239929,-0.118560985834753));
#82647=DIRECTION('ref_axis',(0.76443037844203,0.00399349783751838,-0.644693918452777));
#82648=DIRECTION('center_axis',(0.0623267879409281,0.987363720822469,0.145699191173377));
#82649=DIRECTION('ref_axis',(0.813610424532457,0.0342871357841829,-0.580398543598993));
#82650=DIRECTION('',(-0.96396494909142,0.,-0.266029278319467));
#82651=DIRECTION('center_axis',(-0.0526414310432203,-0.987363722597889,
-0.149471599427316));
#82652=DIRECTION('ref_axis',(0.918712712274094,0.0107821884151984,-0.394779301279786));
#82653=DIRECTION('center_axis',(0.0554976459794082,-0.987363721875457,0.148434807289226));
#82654=DIRECTION('ref_axis',(0.918548006720365,-0.00778744714791775,-0.395232735254764));
#82655=DIRECTION('',(0.467033631299099,0.,-0.884239553082522));
#82656=DIRECTION('center_axis',(4.08854323012095E-14,-1.,-1.76630464062346E-14));
#82657=DIRECTION('ref_axis',(1.,4.08854323012095E-14,6.6808424631127E-32));
#82658=DIRECTION('center_axis',(-0.0772029153070789,0.987363722443365,-0.138392880853279));
#82659=DIRECTION('ref_axis',(0.885148556303636,0.00399349489836831,-0.46529139823565));
#82660=DIRECTION('center_axis',(0.0295485949190189,0.987363720562215,0.155691245276839));
#82661=DIRECTION('ref_axis',(0.919357195679558,0.0342871443428298,-0.391926955547883));
#82662=DIRECTION('',(-0.884239552545753,0.,-0.467033632315368));
#82663=DIRECTION('center_axis',(-0.0192787361679484,-0.98736372270696,-0.157293386428101));
#82664=DIRECTION('ref_axis',(0.982099599572674,0.0107821803329207,-0.18805350596695));
#82665=DIRECTION('center_axis',(0.0222910451404309,-0.987363721898582,0.156894837343769));
#82666=DIRECTION('ref_axis',(0.982036219967827,-0.00778744788706836,-0.188531743551871));
#82667=DIRECTION('',(0.6462000100523,0.,-0.763168098788469));
#82668=DIRECTION('center_axis',(-5.83021152723025E-14,-1.,1.12812464120419E-14));
#82669=DIRECTION('ref_axis',(1.,-5.83021152723025E-14,1.73804291370917E-31));
#82670=DIRECTION('center_axis',(-0.0456475817544446,0.987363722372612,-0.151753675482572));
#82671=DIRECTION('ref_axis',(0.964478171007239,0.00399350098066409,-0.264132371360362));
#82672=DIRECTION('center_axis',(-0.00461124735747092,0.987363720695088,
0.158403344197525));
#82673=DIRECTION('ref_axis',(0.98211584554125,0.0342871412890047,-0.185129300433572));
#82674=DIRECTION('',(-0.763168097828485,0.,-0.646200011186051));
#82675=DIRECTION('',(0.795150795057726,0.,-0.606411752128096));
#82676=DIRECTION('',(-0.606411752600396,0.,-0.795150794697532));
#82677=DIRECTION('center_axis',(0.0485488734866696,-0.987363722705137,-0.150850541825439));
#82678=DIRECTION('ref_axis',(0.970291073781123,0.0107821822196579,0.241700179328144));
#82679=DIRECTION('center_axis',(-0.0456476284023987,-0.9873637218804,0.151753664653351));
#82680=DIRECTION('ref_axis',(0.97043435862057,-0.00778744848726708,0.241239530870754));
#82681=DIRECTION('',(0.906921212507855,0.,-0.421300266203668));
#82682=DIRECTION('center_axis',(1.15300878293867E-13,-1.,2.84836816942017E-14));
#82683=DIRECTION('ref_axis',(1.,1.15300878293867E-13,1.16424979269799E-32));
#82684=DIRECTION('center_axis',(0.0222910902114904,0.987363722384019,-0.156894827885296));
#82685=DIRECTION('ref_axis',(0.986242984785856,0.00399350219507649,0.165253825677056));
#82686=DIRECTION('center_axis',(-0.070696892983569,0.987363720655471,0.141826769179359));
#82687=DIRECTION('ref_axis',(0.969077975887884,0.0342871413349356,0.244360939161972));
#82688=DIRECTION('',(-0.421300264062887,0.,-0.906921213502331));
#82689=DIRECTION('center_axis',(0.0798422345229059,-0.987363722715342,-0.136887167594668));
#82690=DIRECTION('ref_axis',(0.895647813564768,0.0107821814158304,0.444633263061331));
#82691=DIRECTION('center_axis',(-0.0772029647371953,-0.987363721887239,
0.138392857246199));
#82692=DIRECTION('ref_axis',(0.895886775400287,-0.00778744934797183,0.444214184032353));
#82693=DIRECTION('',(0.976285002225685,0.,-0.216489247837379));
#82694=DIRECTION('center_axis',(-5.32410291125588E-14,-1.,-2.6302014804238E-14));
#82695=DIRECTION('ref_axis',(1.,-5.32410291125588E-14,3.94046262851656E-31));
#82696=DIRECTION('center_axis',(0.0554976885389505,0.987363722365366,-0.148434788118024));
#82697=DIRECTION('ref_axis',(0.927660483796157,0.00399350089771891,0.373403372713291));
#82698=DIRECTION('center_axis',(-0.0995325946957576,0.98736372090704,0.123313199738447));
#82699=DIRECTION('ref_axis',(0.893891093343772,0.0342871332184858,0.446971034560779));
#82700=DIRECTION('',(-0.216489246715314,0.,-0.976285002474501));
#82701=DIRECTION('center_axis',(0.107402265541574,-0.987363722643892,-0.11652309884024));
#82702=DIRECTION('ref_axis',(0.779125057181291,0.0107821857526969,0.626775789052708));
#82703=DIRECTION('center_axis',(-0.105148378018556,-0.987363721868306,0.118560951996997));
#82704=DIRECTION('ref_axis',(0.779448521139954,-0.0077874521372006,0.626417878482047));
#82705=DIRECTION('',(0.999998790317524,0.,-0.00155543032291784));
#82706=DIRECTION('center_axis',(8.10987235823951E-14,-1.,6.49815876441424E-14));
#82707=DIRECTION('ref_axis',(1.,8.10987235823951E-14,1.85268858048969E-30));
#82708=DIRECTION('center_axis',(0.0861092731979058,0.987363722354393,-0.133034104077886));
#82709=DIRECTION('ref_axis',(0.825701610179814,0.00399350320383623,0.564092991339747));
#82710=DIRECTION('center_axis',(-0.123714279183475,0.987363720576037,0.0990336327535193));
#82711=DIRECTION('ref_axis',(0.776906855088247,0.0342871442005448,0.628681262850628));
#82712=DIRECTION('',(-0.00155543204838868,0.,-0.99999879031484));
#82713=DIRECTION('center_axis',(0.129940280794788,-0.987363722678062,-0.0907105427516035));
#82714=DIRECTION('ref_axis',(0.626171278679668,0.0107821836502577,0.779610976239048));
#82715=DIRECTION('center_axis',(-0.128177166241555,-0.987363721875366,0.0931852712541492));
#82716=DIRECTION('ref_axis',(0.626564120888356,-0.00778745019988622,0.779330968225173));
#82717=DIRECTION('',(0.976953746694739,0.,0.213451111074907));
#82718=DIRECTION('center_axis',(-5.591447997912E-14,-1.,-6.93395850183567E-14));
#82719=DIRECTION('ref_axis',(4.73600965494586E-31,6.93395850183567E-14,
-1.));
#82720=DIRECTION('center_axis',(0.11269449106455,0.987363722439772,-0.11141288656874));
#82721=DIRECTION('ref_axis',(0.685133845045221,0.00399349595334245,0.728406250909218));
#82722=DIRECTION('center_axis',(-0.142111207537177,0.987363720768343,0.0701233741545532));
#82723=DIRECTION('ref_axis',(0.623595318461725,0.0342871373290877,0.780995051845014));
#82724=DIRECTION('',(0.213451112797233,0.,-0.976953746318434));
#82725=DIRECTION('center_axis',(0.146402435956436,-0.987363722636331,-0.0606564585823214));
#82726=DIRECTION('ref_axis',(0.443938426367657,0.0107821865755688,0.895992420753021));
#82727=DIRECTION('center_axis',(-0.145212533291427,-0.987363721887346,0.0634523512239978));
#82728=DIRECTION('ref_axis',(0.44438227874412,-0.00778744832990127,0.895803408112903));
#82729=DIRECTION('',(0.908227431050156,0.,0.418476921093665));
#82730=DIRECTION('center_axis',(6.6168782348743E-15,-1.,1.32897374105932E-14));
#82731=DIRECTION('ref_axis',(-6.49065371568284E-32,-1.32897374105932E-14,
-1.));
#82732=DIRECTION('center_axis',(0.134010233686802,0.987363722422075,-0.0845821311627522));
#82733=DIRECTION('ref_axis',(0.512529985759116,0.00399349595654121,0.858660040812314));
#82734=DIRECTION('center_axis',(-0.153863177968342,0.987363720847149,0.0379342222848389));
#82735=DIRECTION('ref_axis',(0.441125156119624,0.0342871345160342,0.896790381887047));
#82736=DIRECTION('',(0.418476923230167,0.,-0.908227430065737));
#82737=DIRECTION('center_axis',(0.156018974614436,-0.987363722571497,-0.0277661468341567));
#82738=DIRECTION('ref_axis',(0.24094750808905,0.0107821881505182,0.970478254658168));
#82739=DIRECTION('center_axis',(-0.155457924575797,-0.987363721898907,0.0307524692427131));
#82740=DIRECTION('ref_axis',(0.241421615051718,-0.00778744735097303,0.970389076324325));
#82741=DIRECTION('',(0.797033410730777,0.,0.603935213560912));
#82742=DIRECTION('center_axis',(1.08158357943823E-14,-1.,4.32043918942849E-14));
#82743=DIRECTION('ref_axis',(1.05750130502512E-31,-4.32043918942849E-14,
-1.));
#82744=DIRECTION('center_axis',(0.14905980619695,0.987363722366931,-0.053796411871477));
#82745=DIRECTION('ref_axis',(0.315960793488531,0.00399349875883481,0.948763842558179));
#82746=DIRECTION('center_axis',(-0.15842068050042,0.9873637206152,0.00397129735636706));
#82747=DIRECTION('ref_axis',(0.238028470805658,0.0342871433874741,0.970652790076991));
#82748=DIRECTION('',(0.603935214477023,0.,-0.797033410036613));
#82749=DIRECTION('center_axis',(0.158340237993581,-0.987363722683899,0.00642247303839128));
#82750=DIRECTION('ref_axis',(0.0266901526908901,0.0107821833814529,0.999585604273524));
#82751=DIRECTION('center_axis',(-0.158434276660815,-0.987363721875677,-0.00338536597356439));
#82752=DIRECTION('ref_axis',(0.0271723456231515,-0.00778744857226169,0.999600429810867));
#82753=DIRECTION('',(0.648570992291408,0.,0.761154168324748));
#82754=DIRECTION('center_axis',(-2.55060083723739E-15,-1.,-8.90387643367751E-14));
#82755=DIRECTION('ref_axis',(0.0286342148928776,-8.90752890494927E-14,0.999589956801022));
#82756=DIRECTION('center_axis',(0.157139508999401,0.987363722409248,-0.0204952282636888));
#82757=DIRECTION('ref_axis',(0.1046176245841,0.0039934975627731,0.994504502052955));
#82758=DIRECTION('center_axis',(-0.155570604572091,0.987363720558139,-0.0301773146363916));
#82759=DIRECTION('ref_axis',(0.0238018383267625,0.0342871450113978,0.999128552379139));
#82760=DIRECTION('center_axis',(-0.160229038939383,-0.986495109024279,0.0339713843070435));
#82761=DIRECTION('ref_axis',(0.0342169345737296,0.0288443415490679,0.998998100773459));
#82762=DIRECTION('center_axis',(-0.149180144518476,-0.986495109463456,0.0676216199608588));
#82763=DIRECTION('ref_axis',(0.248172015499022,0.0288443005917729,0.968286454024079));
#82764=DIRECTION('center_axis',(-0.131155746156479,-0.986495109479995,0.0981099853337623));
#82765=DIRECTION('ref_axis',(0.450522855937786,0.0288443007497549,0.892298807906813));
#82766=DIRECTION('center_axis',(-0.106998655483312,-0.98649510960293,0.12401083200377));
#82767=DIRECTION('ref_axis',(0.631807747640335,0.0288442944302163,0.774588262692168));
#82768=DIRECTION('center_axis',(-0.077838417858667,-0.986495109440658,0.144113079749635));
#82769=DIRECTION('ref_axis',(0.783550014359944,0.0288443009343881,0.620658828423585));
#82770=DIRECTION('center_axis',(-0.0450385499786022,-0.986495109516865,
0.157476753570594));
#82771=DIRECTION('ref_axis',(0.898654352338061,0.0288442972480577,0.437708077992771));
#82772=DIRECTION('center_axis',(-0.0101327280341518,-0.986495109574413,
0.163476991067101));
#82773=DIRECTION('ref_axis',(0.971738610638713,0.0288442962006352,0.234290587029514));
#82774=DIRECTION('center_axis',(0.0252468906766347,-0.986495109565086,0.161833226858181));
#82775=DIRECTION('ref_axis',(0.999385452589112,0.0288442963429899,0.0199179246341851));
#82776=DIRECTION('center_axis',(0.0594459960109537,-0.986495109493425,0.152622319808805));
#82777=DIRECTION('ref_axis',(0.980302140845566,0.0288442999651713,-0.195386076814905));
#82778=DIRECTION('center_axis',(0.0908654655990513,-0.986495109564504,0.136274964563505));
#82779=DIRECTION('ref_axis',(0.915380991535049,0.0288442965137984,-0.40155403981897));
#82780=DIRECTION('center_axis',(0.118036175066675,-0.986495109414409,0.113555539173929));
#82781=DIRECTION('ref_axis',(0.807657643449368,0.0288443020225124,-0.588945784617437));
#82782=DIRECTION('center_axis',(0.139687636476012,-0.986495109540251,0.0855263881437399));
#82783=DIRECTION('ref_axis',(0.66216912185642,0.0288442980024015,-0.748799078880741));
#82784=DIRECTION('center_axis',(0.15480746285218,-0.986495109521674,0.0534981152480289));
#82785=DIRECTION('ref_axis',(0.485718306482793,0.028844298557354,-0.87363936105708));
#82786=DIRECTION('center_axis',(0.162688663862699,-0.986495109497723,0.0189683311771181));
#82787=DIRECTION('ref_axis',(0.286555844169295,0.0288442979926773,-0.957629236524101));
#82788=DIRECTION('center_axis',(0.162962723698444,-0.986495109521754,-0.0164483912419118));
#82789=DIRECTION('ref_axis',(0.0739943517728547,0.0288442980844734,-0.996841432913846));
#82790=DIRECTION('center_axis',(0.155616827733293,-0.986495109507004,-0.0510960061549885));
#82791=DIRECTION('ref_axis',(-0.14202703735263,0.028844298707668,-0.989442432429951));
#82792=DIRECTION('center_axis',(0.140994460789364,-0.986495109453923,-0.0833544302974347));
#82793=DIRECTION('ref_axis',(-0.351407401293269,0.028844301034906,-0.935778202681661));
#82794=DIRECTION('center_axis',(0.119779354035356,-0.986495109626686,-0.111715285567845));
#82795=DIRECTION('ref_axis',(-0.544356342929197,0.0288442941149483,-0.838358025314818));
#82796=DIRECTION('center_axis',(0.0929634932824821,-0.986495109537122,-0.134852466703655));
#82797=DIRECTION('ref_axis',(-0.711851787185283,0.0288442970362033,-0.70173715849284));
#82798=DIRECTION('center_axis',(0.0618007632488235,-0.986495109509818,-0.151684094667419));
#82799=DIRECTION('ref_axis',(-0.846061833762455,0.0288442983264773,-0.532303841715017));
#82800=DIRECTION('center_axis',(0.0277482946305678,-0.986495109406112,-0.161423143517025));
#82801=DIRECTION('ref_axis',(-0.940710969996221,0.0288443027818726,-0.3379805869067));
#82802=DIRECTION('center_axis',(-0.00760164176617008,-0.986495109582979,
-0.16361422252153));
#82803=DIRECTION('ref_axis',(-0.991373505862717,0.0288442953495626,-0.127853738698767));
#82804=DIRECTION('center_axis',(-0.0425961448445734,-0.986495109496576,
-0.158154884160174));
#82805=DIRECTION('ref_axis',(-0.995680518590945,0.0288442992254162,0.0882514096242231));
#82806=DIRECTION('center_axis',(-0.0755988954940555,-0.986495109515445,
-0.145300398836991));
#82807=DIRECTION('ref_axis',(-0.953430617566002,0.0288442993207796,0.300230018293316));
#82808=DIRECTION('center_axis',(-0.105066729765575,-0.986495109402435,-0.125651826176323));
#82809=DIRECTION('ref_axis',(-0.866599358686841,0.0288443032152825,0.498170209562536));
#82810=DIRECTION('center_axis',(-0.129621749359243,-0.986495109613201,-0.100127922191002));
#82811=DIRECTION('ref_axis',(-0.73924687943124,0.0288442934410548,0.672816511381119));
#82812=DIRECTION('center_axis',(-0.148115811053804,-0.986495109518648,-0.069922138208617));
#82813=DIRECTION('ref_axis',(-0.577328035667357,0.0288442983711295,0.816002662792192));
#82814=DIRECTION('center_axis',(-0.159684137960783,-0.98649510955407,-0.0364468779132737));
#82815=DIRECTION('ref_axis',(-0.38841397670723,0.0288442969363252,0.921033435458629));
#82816=DIRECTION('center_axis',(-0.163785812747736,-0.986495109585999,-0.00126740106956708));
#82817=DIRECTION('ref_axis',(-0.181338109777202,0.0288442964058661,0.982997709309275));
#82818=DIRECTION('center_axis',(0.163550499649484,0.986495109843996,0.00886748658227992));
#82819=DIRECTION('ref_axis',(-0.0789203331419368,0.00412339327425965,0.996872398376378));
#82820=DIRECTION('center_axis',(0.157820545689508,0.986495109373187,0.043818655171623));
#82821=DIRECTION('ref_axis',(-0.291373304723066,0.00412343120499991,0.956600540774391));
#82822=DIRECTION('center_axis',(0.14471107203118,0.986495109447332,0.0767209532532179));
#82823=DIRECTION('ref_axis',(-0.490202001414802,0.00412342961885999,0.871599102303978));
#82824=DIRECTION('center_axis',(0.124835069886123,0.986495109370258,0.106035864286994));
#82825=DIRECTION('ref_axis',(-0.666109393625256,0.00412342810459183,0.745842659724462));
#82826=DIRECTION('center_axis',(0.0991219177812932,0.986495109435623,0.130392654988527));
#82827=DIRECTION('ref_axis',(-0.81087025092018,0.00412342693382052,0.585211443431318));
#82828=DIRECTION('center_axis',(0.0687739385131564,0.986495109397187,0.148652428560119));
#82829=DIRECTION('ref_axis',(-0.917715716882505,0.00412342974764044,0.397216389785147));
#82830=DIRECTION('center_axis',(0.035210162910571,0.986495109405196,0.159961381425146));
#82831=DIRECTION('ref_axis',(-0.981649815310068,0.00412342834487012,0.190647941086164));
#82832=DIRECTION('center_axis',(-2.83305944967152E-9,0.986495109461485,
0.163790717101347));
#82833=DIRECTION('ref_axis',(-0.999683059979575,0.00412342514179896,-0.0248349945635702));
#82834=DIRECTION('center_axis',(-0.035210167842371,0.986495109484084,0.159961379853065));
#82835=DIRECTION('ref_axis',(-0.970972235526654,0.00412342273155899,-0.239156675050788));
#82836=DIRECTION('center_axis',(-0.068773934373553,0.98649510939345,0.1486524305001));
#82837=DIRECTION('ref_axis',(-0.896859828128692,0.00412343157330405,-0.442295654512945));
#82838=DIRECTION('center_axis',(-0.099121918885696,0.986495109403051,0.130392654395409));
#82839=DIRECTION('ref_axis',(-0.780811251037479,0.00412342870837165,-0.624753381414598));
#82840=DIRECTION('center_axis',(-0.124835073263289,0.986495109420972,0.106035859839273));
#82841=DIRECTION('ref_axis',(-0.628252808807675,0.00412342311877974,-0.77799833265056));
#82842=DIRECTION('center_axis',(-0.144711074072459,0.986495109433479,0.0767209495810921));
#82843=DIRECTION('ref_axis',(-0.446317964038295,0.00412342285807861,-0.894864946436413));
#82844=DIRECTION('center_axis',(-0.157820545244122,0.986495109411327,0.0438186559171042));
#82845=DIRECTION('ref_axis',(-0.243513790037603,0.00412342517897462,-0.969888669604051));
#82846=DIRECTION('center_axis',(-0.16355050422689,0.986495109393709,0.00886745225109193));
#82847=DIRECTION('ref_axis',(-0.0293231770748078,0.00412342975117166,-0.999561478155959));
#82848=DIRECTION('center_axis',(-0.161633023231499,0.986495109438459,-0.02649839344278));
#82849=DIRECTION('ref_axis',(0.18623855536835,0.00412342416576182,-0.98249590221408));
#82850=DIRECTION('center_axis',(-0.152157762655465,0.9864951094082,-0.0606251958956625));
#82851=DIRECTION('ref_axis',(0.393091977801218,0.00412342637242704,-0.919489909864854));
#82852=DIRECTION('center_axis',(-0.135567773032974,0.986495109404893,-0.0919172347011641));
#82853=DIRECTION('ref_axis',(0.581564857222371,0.00412342533892671,-0.813489590718528));
#82854=DIRECTION('center_axis',(-0.112638786693034,0.986495109457597,-0.118911323046059));
#82855=DIRECTION('ref_axis',(0.742844406071995,0.00412342655905149,-0.669451406541922));
#82856=DIRECTION('center_axis',(-0.0844429339025283,0.986495109396176,-0.140345253041778));
#82857=DIRECTION('ref_axis',(0.869389381988438,0.00412342564311634,-0.494110412607068));
#82858=DIRECTION('center_axis',(-0.0522986278065988,0.986495109418806,-0.155216792333578));
#82859=DIRECTION('ref_axis',(0.955282674023109,0.00412342940239734,-0.295665368349459));
#82860=DIRECTION('center_axis',(-0.0177088933836277,0.98649510941386,-0.162830568990174));
#82861=DIRECTION('ref_axis',(0.996508010535055,0.00412343038860525,-0.0833953371676001));
#82862=DIRECTION('center_axis',(0.0177088922524152,0.986495109402834,-0.162830569180003));
#82863=DIRECTION('ref_axis',(0.991137739773237,0.00412342739576669,0.132774162184182));
#82864=DIRECTION('center_axis',(0.0522986293653706,0.986495109470237,-0.155216791481493));
#82865=DIRECTION('ref_axis',(0.939422969947577,0.004123425151586,0.342735292755054));
#82866=DIRECTION('center_axis',(0.0844429357467301,0.986495109349537,-0.140345252259984));
#82867=DIRECTION('ref_axis',(0.843781825182108,0.00412342914002899,0.536670503031867));
#82868=DIRECTION('center_axis',(0.112638790080962,0.986495109475539,-0.118911319687998));
#82869=DIRECTION('ref_axis',(0.708686382684141,0.00412342432368572,0.705511593363223));
#82870=DIRECTION('center_axis',(0.135567776406498,0.986495109430993,-0.0919172294454673));
#82871=DIRECTION('ref_axis',(0.540453551221462,0.00412342487770254,0.841363747935094));
#82872=DIRECTION('center_axis',(0.152157764571979,0.98649510943652,-0.0606251906247457));
#82873=DIRECTION('ref_axis',(0.34694970956876,0.00412342481747551,0.937874669877552));
#82874=DIRECTION('center_axis',(0.161633024106174,0.986495109430748,-0.0264983883945512));
#82875=DIRECTION('ref_axis',(0.137222889143665,0.00412342727951331,0.990531612843596));
#82876=DIRECTION('center_axis',(0.156018981440023,0.987363721870147,-0.0277661334209345));
#82877=DIRECTION('ref_axis',(0.106060021918456,0.0112019472137412,0.9942966298491));
#82878=DIRECTION('',(-0.603694433998265,0.,0.797215799115594));
#82879=DIRECTION('',(-0.797215799077898,0.,-0.603694434048045));
#82880=DIRECTION('center_axis',(1.08288855678234E-14,-1.,4.32011223528413E-14));
#82881=DIRECTION('ref_axis',(7.04722324508856E-32,-4.32011223528413E-14,
-1.));
#82882=DIRECTION('center_axis',(-0.15386314984286,-0.98736372225306,0.0379342997696712));
#82883=DIRECTION('ref_axis',(0.171011654648654,0.0112022366990284,0.985205320665326));
#82884=DIRECTION('center_axis',(0.157139511605135,-0.987363722043811,-0.0204952258902551));
#82885=DIRECTION('ref_axis',(0.239893891223624,0.0180313431330044,0.970631645691819));
#82886=DIRECTION('center_axis',(0.146402446990452,0.987363721922409,-0.0606564435714413));
#82887=DIRECTION('ref_axis',(0.317324780468734,0.0112019451391554,0.948250758041126));
#82888=DIRECTION('',(-0.418202564699196,0.,0.908353793892564));
#82889=DIRECTION('',(-0.908353794958524,0.,-0.418202562383886));
#82890=DIRECTION('center_axis',(6.62089218032808E-15,-1.,1.32877379472513E-14));
#82891=DIRECTION('ref_axis',(-7.81841420998606E-32,-1.32877379472513E-14,
-1.));
#82892=DIRECTION('center_axis',(-0.142111161632101,-0.98736372224877,0.07012344634021));
#82893=DIRECTION('ref_axis',(0.378803518223432,0.0112022371766569,0.925409317255769));
#82894=DIRECTION('center_axis',(0.149059807495583,-0.987363722127591,-0.0537964126659872));
#82895=DIRECTION('ref_axis',(0.442942417495199,0.0180313388269867,0.89636872190166));
#82896=DIRECTION('center_axis',(0.129940297717711,0.987363721920756,-0.0907105267531021));
#82897=DIRECTION('ref_axis',(0.513751786447825,0.0112019434459527,0.85786573447405));
#82898=DIRECTION('',(-0.213156003970963,0.,0.977018176888808));
#82899=DIRECTION('',(-0.977018176875493,0.,-0.213156004031993));
#82900=DIRECTION('center_axis',(-1.86451405470691E-14,-1.,-2.3107563814193E-14));
#82901=DIRECTION('ref_axis',(-4.11731915750795E-31,2.3107563814193E-14,
-1.));
#82902=DIRECTION('center_axis',(-0.123714212024382,-0.987363722232937,0.0990337001303415));
#82903=DIRECTION('ref_axis',(0.568882952848608,0.0112022393150633,0.822342201150213));
#82904=DIRECTION('center_axis',(0.134010238811121,-0.987363721952807,-0.0845821285218517));
#82905=DIRECTION('ref_axis',(0.625279446823254,0.0180313468374548,0.780192594114833));
#82906=DIRECTION('center_axis',(0.107402283594654,0.987363721950959,-0.116523088071864));
#82907=DIRECTION('ref_axis',(0.686156328941859,0.0112019438535314,0.727367863399898));
#82908=DIRECTION('',(0.00185749160357402,0.,0.999998274860983));
#82909=DIRECTION('',(-0.999998274855759,0.,0.00185749441591979));
#82910=DIRECTION('center_axis',(4.63533414192115E-14,-1.,3.71183355223613E-14));
#82911=DIRECTION('ref_axis',(1.,4.63533414192115E-14,8.01737682443457E-31));
#82912=DIRECTION('center_axis',(-0.0995325279449254,-0.987363722252009,
0.123313242847437));
#82913=DIRECTION('ref_axis',(0.732362049748505,0.0112022347792573,0.680823279584444));
#82914=DIRECTION('center_axis',(0.112694492230308,-0.987363722076729,-0.111412888606934));
#82915=DIRECTION('ref_axis',(0.778379106755819,0.0180313415424152,0.627535526395275));
#82916=DIRECTION('center_axis',(0.0798422598236929,0.987363721944083,-0.136887158400539));
#82917=DIRECTION('ref_axis',(0.82647696532404,0.0112019420910649,0.562859078528679));
#82918=DIRECTION('',(0.216784133438348,0.,0.976219565205177));
#82919=DIRECTION('',(-0.976219564475212,0.,0.216784136725517));
#82920=DIRECTION('center_axis',(3.99367281940478E-14,-1.,1.97144484204352E-14));
#82921=DIRECTION('ref_axis',(1.,3.99367281940478E-14,3.89081776988677E-31));
#82922=DIRECTION('center_axis',(-0.0706968106498305,-0.987363722284355,
0.141826798880623));
#82923=DIRECTION('ref_axis',(0.8615967118823,0.0112022347444393,0.507469817831898));
#82924=DIRECTION('center_axis',(0.0861092826808786,-0.987363721992386,-0.133034100626598));
#82925=DIRECTION('ref_axis',(0.895082624554255,0.0180313447346119,0.445535594344748));
#82926=DIRECTION('center_axis',(0.0485488928772202,0.987363721828466,-0.150850541322981));
#82927=DIRECTION('ref_axis',(0.928152457786751,0.0112019490099345,0.372031626938884));
#82928=DIRECTION('',(0.421574190582567,0.,0.906793913651086));
#82929=DIRECTION('',(-0.906793913166479,0.,0.421574191624944));
#82930=DIRECTION('center_axis',(-1.29723160072588E-13,-1.,-3.20049586081121E-14));
#82931=DIRECTION('ref_axis',(1.,-1.29723160072588E-13,-7.57499294018975E-31));
#82932=DIRECTION('center_axis',(-0.0385553889118671,-0.987363722263305,
0.153708691830376));
#82933=DIRECTION('ref_axis',(0.950544069762331,0.0112022349597061,0.310387630828893));
#82934=DIRECTION('center_axis',(0.0554976904691863,-0.987363722124819,-0.14843478899641));
#82935=DIRECTION('ref_axis',(0.96993307281497,0.0180313384327736,0.242702915297762));
#82936=DIRECTION('center_axis',(0.01498544227234,0.987363721863414,-0.157760315884345));
#82937=DIRECTION('ref_axis',(0.986428571397858,0.0112019464713099,0.163808393940099));
#82938=DIRECTION('',(0.606651908563567,0.,0.79496758539967));
#82939=DIRECTION('',(-0.794967585437568,0.,0.606651908513905));
#82940=DIRECTION('',(0.763363255463762,0.,0.645969457643136));
#82941=DIRECTION('',(-0.645969457690815,0.,0.763363255423415));
#82942=DIRECTION('center_axis',(2.91493521777504E-14,-1.,-5.64942831183301E-15));
#82943=DIRECTION('ref_axis',(1.,2.91493521777504E-14,3.3884035720465E-32));
#82944=DIRECTION('center_axis',(0.0295486797280843,-0.987363722245854,0.155691218503611));
#82945=DIRECTION('ref_axis',(0.993018816372276,0.0112022332241641,-0.117422912165366));
#82946=DIRECTION('center_axis',(-0.0119578129886334,-0.987363722205775,
-0.158018640610806));
#82947=DIRECTION('ref_axis',(0.982195724128258,0.0180313362869311,-0.186993129327992));
#82948=DIRECTION('center_axis',(-0.0526414173739263,0.9873637218959,-0.149471608878542));
#82949=DIRECTION('ref_axis',(0.964039683787994,0.0112019454545849,-0.265522135612039));
#82950=DIRECTION('',(0.884380585166769,0.,0.466766516129941));
#82951=DIRECTION('',(-0.466766516185183,0.,0.884380585137614));
#82952=DIRECTION('center_axis',(4.08800946220324E-14,-1.,-1.76753953208713E-14));
#82953=DIRECTION('ref_axis',(1.,4.08800946220324E-14,-2.74904565889751E-32));
#82954=DIRECTION('center_axis',(0.0623268615422876,-0.987363722252581,0.145699149996891));
#82955=DIRECTION('ref_axis',(0.944560133027489,0.0112022373139612,-0.328147322058637));
#82956=DIRECTION('center_axis',(-0.0456475758122678,-0.987363722013895,
-0.151753679603923));
#82957=DIRECTION('ref_axis',(0.919034539789773,0.0180313434872257,-0.393764377928535));
#82958=DIRECTION('center_axis',(-0.0835426679191584,0.987363721926463,-0.134660696791869));
#82959=DIRECTION('ref_axis',(0.884421561891373,0.0112019458379472,-0.466554409764892));
#82960=DIRECTION('',(0.964045262617061,0.,0.265738088398336));
#82961=DIRECTION('',(-0.265738088458527,0.,0.964045262600469));
#82962=DIRECTION('center_axis',(0.,-1.,0.));
#82963=DIRECTION('ref_axis',(0.,0.,-1.));
#82964=DIRECTION('center_axis',(0.0921907025317405,-0.987363722255318,0.128894353409397));
#82965=DIRECTION('ref_axis',(0.851934869173167,0.011202235227345,-0.523527925341916));
#82966=DIRECTION('center_axis',(-0.0772029162694352,-0.987363722049419,
-0.138392883127032));
#82967=DIRECTION('ref_axis',(0.812900319838701,0.0180313436171572,-0.582123647220672));
#82968=DIRECTION('center_axis',(-0.110537555212464,0.987363721935053,-0.11355320116232));
#82969=DIRECTION('ref_axis',(0.763448870616057,0.0112019447737031,-0.645771119196542));
#82970=DIRECTION('',(0.99863225400483,0.,0.0522840440405398));
#82971=DIRECTION('',(-0.0522840469698092,0.,0.998632253851466));
#82972=DIRECTION('center_axis',(9.89335438420199E-15,-1.,-1.10689535019281E-14));
#82973=DIRECTION('ref_axis',(-2.42855845865753E-31,1.10689535019281E-14,
-1.));
#82974=DIRECTION('center_axis',(0.117743810847805,-0.987363722264918,0.106062599261951));
#82975=DIRECTION('ref_axis',(0.719474076791775,0.0112022350142792,-0.694428947233126));
#82976=DIRECTION('center_axis',(-0.105148334451143,-0.987363722064409,-0.118560989002571));
#82977=DIRECTION('ref_axis',(0.668755786226334,0.0180313427373918,-0.743263458719641));
#82978=DIRECTION('center_axis',(-0.132363832466933,0.987363721862616,-0.087136080955418));
#82979=DIRECTION('ref_axis',(0.606778157678717,0.0112019480430204,-0.79479228967326));
#82980=DIRECTION('',(0.986524311201882,0.,-0.163614740801838));
#82981=DIRECTION('',(0.163614740740217,0.,0.986524311212102));
#82982=DIRECTION('center_axis',(0.,-1.,0.));
#82983=DIRECTION('ref_axis',(0.,0.,-1.));
#82984=DIRECTION('center_axis',(0.137791350328405,-0.987363722237725,0.0782714749033058));
#82985=DIRECTION('ref_axis',(0.553371476054598,0.0112022361144345,-0.83285924344705));
#82986=DIRECTION('center_axis',(-0.128177133113773,-0.98736372207118,-0.0931853147468999));
#82987=DIRECTION('ref_axis',(0.493340974292365,0.0180313422430586,-0.869649098074145));
#82988=DIRECTION('center_axis',(-0.148000920166892,0.987363721894028,-0.0566445788873566));
#82989=DIRECTION('ref_axis',(0.421735172486176,0.0112019452194524,-0.906649855628597));
#82990=DIRECTION('',(0.928287587778145,0.,-0.371863085526155));
#82991=DIRECTION('',(0.371863084475821,0.,0.928287588198899));
#82992=DIRECTION('center_axis',(-8.66246462963213E-15,-1.,2.84000436035281E-14));
#82993=DIRECTION('ref_axis',(-7.27882073886525E-32,-2.84000436035281E-14,
-1.));
#82994=DIRECTION('center_axis',(0.151395919729731,-0.987363722225806,0.0468204605016794));
#82995=DIRECTION('ref_axis',(0.361393837408662,0.0112022394380031,-0.932345968036874));
#82996=DIRECTION('center_axis',(-0.145212510328798,-0.987363722018919,-0.0634524017272397));
#82997=DIRECTION('ref_axis',(0.294858087543414,0.0180313448874745,-0.955370911642065));
#82998=DIRECTION('center_axis',(-0.156717651463886,0.987363721882632,-0.0235044342565438));
#82999=DIRECTION('ref_axis',(0.216972319801143,0.0112019481712355,-0.976113481515997));
#83000=DIRECTION('',(0.826645169515348,0.,-0.56272352333712));
#83001=DIRECTION('',(0.56272352328549,0.,0.826645169550494));
#83002=DIRECTION('center_axis',(-2.35477114699405E-15,-1.,2.95982401992128E-14));
#83003=DIRECTION('ref_axis',(1.8148513515194E-32,-2.95982401992128E-14,
-1.));
#83004=DIRECTION('center_axis',(0.157921382460364,-0.987363722227189,0.0131801741823417));
#83005=DIRECTION('ref_axis',(0.15251782909657,0.0112022422485203,-0.988237229402068));
#83006=DIRECTION('center_axis',(-0.155457913607194,-0.987363722140868,-0.0307525169218483));
#83007=DIRECTION('ref_axis',(0.0825879624401618,0.0180313393924332,-0.99642064373421));
#83008=DIRECTION('center_axis',(-0.158106438295245,0.987363721977051,0.0107347423451855));
#83009=DIRECTION('ref_axis',(0.00206408220887537,0.0112019414720079,-0.999935125931624));
#83010=DIRECTION('',(0.686349742131425,0.,-0.727271635275381));
#83011=DIRECTION('',(0.727271635232524,0.,0.686349742176837));
#83012=DIRECTION('center_axis',(-4.06302881637799E-15,-1.,-2.94124559535081E-14));
#83013=DIRECTION('ref_axis',(-8.13378641990255E-32,2.94124559535081E-14,
-1.));
#83014=DIRECTION('center_axis',(0.157062616396446,-0.987363722260598,-0.021076396618003));
#83015=DIRECTION('ref_axis',(-0.0634897471633578,0.0112022384316609,-0.997919616932773));
#83016=DIRECTION('center_axis',(-0.158434276437026,-0.987363722091255,0.00338531357163764));
#83017=DIRECTION('ref_axis',(-0.1335438816567,0.0180313416766307,-0.990878853538313));
#83018=DIRECTION('center_axis',(-0.152102345193246,0.98736372197672,0.0444719811903379));
#83019=DIRECTION('ref_axis',(-0.212940667766901,0.0112019422303222,-0.977000915302158));
#83020=DIRECTION('',(0.513961362392701,0.,-0.857813335153656));
#83021=DIRECTION('',(0.857813335121557,0.,0.513961362446274));
#83022=DIRECTION('center_axis',(-1.54362691251806E-14,-1.,-4.17770670576077E-14));
#83023=DIRECTION('ref_axis',(4.33070742457523E-31,4.17770670576077E-14,
-1.));
#83024=DIRECTION('center_axis',(0.148859778356902,-0.987363722268594,-0.0543474593282965));
#83025=DIRECTION('ref_axis',(-0.276528610540624,0.0112022357729868,-0.960940392254462));
#83026=DIRECTION('center_axis',(-0.154002428756523,-0.987363722073559,0.0373648534071712));
#83027=DIRECTION('ref_axis',(-0.343431362720795,0.0180313411743159,-0.939004669762186));
#83028=DIRECTION('center_axis',(-0.13898611326727,0.987363721839146,0.0761297649727565));
#83029=DIRECTION('ref_axis',(-0.417988550412985,0.0112019485432832,-0.908383227538072));
#83030=DIRECTION('',(0.317540722300475,0.,-0.948244635988463));
#83031=DIRECTION('',(0.948244636544387,0.,0.317540720640366));
#83032=DIRECTION('center_axis',(4.00936870292431E-14,-1.,6.24700014331448E-14));
#83033=DIRECTION('ref_axis',(8.00121565978192E-31,-6.24700014331447E-14,
-1.));
#83034=DIRECTION('center_axis',(0.13369642348063,-0.987363722268957,-0.0850772960059203));
#83035=DIRECTION('ref_axis',(-0.476637303526556,0.011202233537974,-0.879028663270257));
#83036=DIRECTION('center_axis',(-0.142369599811224,-0.987363722034396,0.0695972518133825));
#83037=DIRECTION('ref_axis',(-0.53726037401082,0.0180313432663028,-0.84322367209286));
#83038=DIRECTION('center_axis',(-0.119371046962671,0.987363721897949,0.104227797764633));
#83039=DIRECTION('ref_axis',(-0.603491752064952,0.0112019468735407,-0.797290550286291));
#83040=DIRECTION('',(0.106272228164614,0.,-0.994337072385883));
#83041=DIRECTION('',(0.994337072346781,0.,0.10627222853047));
#83042=DIRECTION('center_axis',(-3.15513135201966E-14,-1.,-3.14343179307583E-14));
#83043=DIRECTION('ref_axis',(1.,-3.15513135201966E-14,6.49236310791174E-31));
#83044=DIRECTION('center_axis',(0.11228156876534,-0.987363722283361,-0.111829017854669));
#83045=DIRECTION('ref_axis',(-0.654458968400117,0.0112022372151143,-0.756014529332626));
#83046=DIRECTION('center_axis',(-0.12407972666712,-0.987363722011638,0.0985753614527323));
#83047=DIRECTION('ref_axis',(-0.705967689967984,0.0180313446855486,-0.708014471130428));
#83048=DIRECTION('center_axis',(-0.0941743240009238,0.98736372194084,0.127452254958871));
#83049=DIRECTION('ref_axis',(-0.760776350944052,0.0112019449395735,-0.648917452588404));
#83050=DIRECTION('',(-0.109965437515888,0.,-0.993935411660103));
#83051=DIRECTION('',(0.993935411981186,0.,-0.109965434613747));
#83052=DIRECTION('center_axis',(-5.00948140137855E-14,-1.,-3.18890683862576E-14));
#83053=DIRECTION('ref_axis',(1.,-5.00948140137855E-14,-6.10027479870061E-31));
#83054=DIRECTION('center_axis',(0.0856165536929381,-0.987363722249842,-0.133351736841637));
#83055=DIRECTION('ref_axis',(-0.801678856600124,0.0112022390584335,-0.597649998511165));
#83056=DIRECTION('center_axis',(-0.0999880255357913,-0.987363721948436,
0.122944195997963));
#83057=DIRECTION('ref_axis',(-0.841664740409905,0.0180313480723561,-0.539699300756838));
#83058=DIRECTION('center_axis',(-0.0645741169833012,0.987363722015683,0.144717185790647));
#83059=DIRECTION('ref_axis',(-0.882487893320251,0.0112019405356229,-0.470201695734311));
#83060=DIRECTION('',(-0.321061238918488,0.,-0.947058435823326));
#83061=DIRECTION('',(0.947058436717493,0.,-0.321061236280897));
#83062=DIRECTION('center_axis',(5.57788322286723E-14,-1.,2.03746154926628E-14));
#83063=DIRECTION('ref_axis',(1.,5.57788322286723E-14,4.3682323794354E-31));
#83064=DIRECTION('center_axis',(0.0549482066282451,-0.987363722243805,-0.148639074893508));
#83065=DIRECTION('ref_axis',(-0.911413133585882,0.0112022370251814,-0.411340017276212));
#83066=DIRECTION('center_axis',(-0.0712209830205846,-0.987363722192365,
0.141564302265861));
#83067=DIRECTION('ref_axis',(-0.938006483548204,0.0180313375612654,-0.346148389693329));
#83068=DIRECTION('center_axis',(-0.0319544928820863,0.987363721983359,0.155215304966415));
#83069=DIRECTION('ref_axis',(-0.962935282094827,0.0112019407089108,-0.269499831208312));
#83070=DIRECTION('',(-0.517144572474315,0.,-0.855898061196751));
#83071=DIRECTION('',(0.855898060460217,0.,-0.517144573693314));
#83072=DIRECTION('center_axis',(-5.88546942245058E-14,-1.,-7.90746818996684E-15));
#83073=DIRECTION('ref_axis',(1.,-5.88546942245058E-14,8.10968348491405E-32));
#83074=DIRECTION('center_axis',(0.0217105382537213,-0.987363722231665,-0.156976216509269));
#83075=DIRECTION('ref_axis',(-0.978530745503069,0.011202239615509,-0.20579623401026));
#83076=DIRECTION('center_axis',(-0.0391237393982408,-0.987363722089536,
0.153565013323332));
#83077=DIRECTION('ref_axis',(-0.990488084645076,0.0180313411108617,-0.136411967634343));
#83078=DIRECTION('center_axis',(0.00215929493914566,0.987363721875552,0.158455729367619));
#83079=DIRECTION('ref_axis',(-0.99835688760782,0.0112019478522475,-0.0561964530049911));
#83080=DIRECTION('',(-0.68904680421877,0.,-0.724716842357));
#83081=DIRECTION('',(0.724716840964441,0.,-0.689046805683417));
#83082=DIRECTION('center_axis',(0.0361720501024856,0.987363723226731,0.15428694321695));
#83083=DIRECTION('ref_axis',(-0.987096432090511,0.0112018841470787,0.159734628511599));
#83084=DIRECTION('',(-0.828729971245926,0.,-0.559648670827267));
#83085=DIRECTION('center_axis',(1.03562508173011E-13,-1.,-8.62649121691859E-15));
#83086=DIRECTION('ref_axis',(1.,1.03562508173011E-13,-4.16955228716423E-33));
#83087=DIRECTION('center_axis',(-0.0125422848473503,-0.987363722246317,
-0.157973323959163));
#83088=DIRECTION('ref_axis',(-0.999893347505735,0.0112022358467117,0.00937035355842204));
#83089=DIRECTION('center_axis',(-0.00519715123370011,-0.987363721335481,
0.158385199465116));
#83090=DIRECTION('ref_axis',(-0.996655564095281,0.0180313824950653,0.0797029221750023));
#83091=DIRECTION('',(0.559648669545658,0.,-0.828729972111408));
#83092=DIRECTION('center_axis',(2.8367666732571E-14,-1.,-8.76791045131834E-15));
#83093=DIRECTION('ref_axis',(1.,2.8367666732571E-14,-2.10203266835669E-31));
#83094=DIRECTION('center_axis',(0.0684935539383942,0.987363721923308,0.142903861734529));
#83095=DIRECTION('ref_axis',(-0.929680449617988,0.0112019447854592,0.368196656735391));
#83096=DIRECTION('center_axis',(-0.0462086544756258,-0.987363722215038,
-0.151583773225295));
#83097=DIRECTION('ref_axis',(-0.974502047462563,0.0112022423458931,0.224098793521289));
#83098=DIRECTION('center_axis',(0.0289725294676274,-0.987363722077757,0.155799463609492));
#83099=DIRECTION('ref_axis',(-0.956220537480874,0.0180313430440089,0.292091003572205));
#83100=DIRECTION('',(-0.929662646609954,0.,-0.368411948093674));
#83101=DIRECTION('',(0.368411947167104,0.,-0.92966264697714));
#83102=DIRECTION('center_axis',(3.87294073425063E-14,-1.,-2.19916970885083E-14));
#83103=DIRECTION('ref_axis',(1.,3.87294073425063E-14,-2.80400463742889E-31));
#83104=DIRECTION('center_axis',(-0.0777143454502976,-0.987363722242736,
-0.138106337690207));
#83105=DIRECTION('ref_axis',(-0.903544115145585,0.0112022346100321,0.428348621948903));
#83106=DIRECTION('center_axis',(0.0617874476101675,-0.987363722074356,0.145928721125403));
#83107=DIRECTION('ref_axis',(-0.87107370117854,0.0180313424742626,0.490821227947299));
#83108=DIRECTION('center_axis',(0.0976123131343119,0.987363722050419,0.124838762823539));
#83109=DIRECTION('ref_axis',(-0.828793639509073,0.0112019379749413,0.559442239820082));
#83110=DIRECTION('',(-0.987125329195886,0.,-0.159948693211022));
#83111=DIRECTION('',(0.159948692818607,0.,-0.987125329259471));
#83112=DIRECTION('center_axis',(-3.30963705214028E-14,-1.,2.9803221179575E-14));
#83113=DIRECTION('ref_axis',(1.,-3.30963705214028E-14,6.25159702479296E-31));
#83114=DIRECTION('center_axis',(-0.105586206869686,-0.987363722259735,-0.118171201585976));
#83115=DIRECTION('ref_axis',(-0.790337464271335,0.0112022339772626,0.612569345072927));
#83116=DIRECTION('center_axis',(0.0917132492516903,-0.987363721931314,0.129234517547133));
#83117=DIRECTION('ref_axis',(-0.745196427498504,0.0180313474279287,0.66660119633361));
#83118=DIRECTION('center_axis',(0.122166840284463,0.987363721930211,0.100936335137705));
#83119=DIRECTION('ref_axis',(-0.689153359040235,0.0112019447743796,0.724528925686775));
#83120=DIRECTION('',(-0.998431128681538,0.,0.0559935824868428));
#83121=DIRECTION('',(-0.0559935851300269,0.,-0.998431128533304));
#83122=DIRECTION('center_axis',(3.45543789430862E-14,-1.,-4.82949063880597E-14));
#83123=DIRECTION('ref_axis',(-4.06692601993503E-31,4.82949063880597E-14,
-1.));
#83124=DIRECTION('center_axis',(-0.128520974782549,-0.987363722243347,-0.0927105120183547));
#83125=DIRECTION('ref_axis',(-0.640175512069977,0.0112022330864055,0.768147006581306));
#83126=DIRECTION('center_axis',(0.117350647805832,-0.98736372204255,0.10649744529252));
#83127=DIRECTION('ref_axis',(-0.584474595140577,0.0180313435221755,0.811211635940981));
#83128=DIRECTION('center_axis',(0.141008974823679,0.987363721952356,0.0723142419691046));
#83129=DIRECTION('ref_axis',(-0.517289037097874,0.0112019432813125,0.85573744137152));
#83130=DIRECTION('',(-0.963051398102499,0.,0.269317664873326));
#83131=DIRECTION('',(-0.269317664813245,0.,-0.963051398119301));
#83132=DIRECTION('center_axis',(2.92056743225914E-14,-1.,-6.82424603926603E-14));
#83133=DIRECTION('ref_axis',(-2.92163954713156E-31,6.82424603926603E-14,
-1.));
#83134=DIRECTION('center_axis',(-0.145446246385829,-0.987363722270873,-0.062914778515692));
#83135=DIRECTION('ref_axis',(-0.460079663912597,0.0112022359509466,0.887806968188339));
#83136=DIRECTION('center_axis',(0.137500857423055,-0.98736372201278,0.0787806744131776));
#83137=DIRECTION('ref_axis',(-0.396423382729331,0.0180313439371385,0.917890719127966));
#83138=DIRECTION('center_axis',(0.153257689760006,0.987363721863816,0.0403108084346932));
#83139=DIRECTION('ref_axis',(-0.321236848885251,0.0112019484669408,0.946932628685282));
#83140=DIRECTION('',(-0.882640455447384,0.,0.470048748969333));
#83141=DIRECTION('',(-0.470048751153994,0.,-0.882640454283946));
#83142=DIRECTION('center_axis',(2.77055002754196E-15,-1.,-1.45850692541728E-14));
#83143=DIRECTION('ref_axis',(-3.71033610358611E-32,1.45850692541728E-14,
-1.));
#83144=DIRECTION('center_axis',(-0.155570611822742,-0.987363722257185,-0.0301772216669084));
#83145=DIRECTION('ref_axis',(-0.258471001547092,0.0112022365512323,0.965954062704585));
#83146=DIRECTION('center_axis',(0.151221680424715,-0.987363722063087,0.0473802039173925));
#83147=DIRECTION('ref_axis',(-0.189835852008218,0.0180313416813938,0.981650253404685));
#83148=DIRECTION('center_axis',(0.158340241637008,0.987363721953189,0.00642249554924032));
#83149=DIRECTION('ref_axis',(-0.110163989544152,0.0112019445036678,0.993850296496939));
#83150=DIRECTION('',(-0.760958224664093,8.72727899869762E-15,0.648800878787993));
#83151=DIRECTION('center_axis',(-3.00707855217943E-15,-1.,-1.03877653669684E-13));
#83152=DIRECTION('ref_axis',(0.0289361497150056,-1.0392116941864E-13,0.999581261949058));
#83153=DIRECTION('center_axis',(-0.158420668070115,-0.987363722255939,0.0039713852891132));
#83154=DIRECTION('ref_axis',(-0.0447765240641304,0.0112022340570488,0.998934218477306));
#83155=DIRECTION('center_axis',(0.157871544748071,-0.987363722095171,0.0137642889111219));
#83156=DIRECTION('ref_axis',(0.0256281921958917,0.0180313407672832,0.999508912674071));
#83157=DIRECTION('',(-0.64880087707579,0.,-0.760958226123935));
#83158=DIRECTION('center_axis',(-0.15843427510874,-0.987363722233975,-0.00338533411013414));
#83159=DIRECTION('ref_axis',(-0.150493176847073,0.0207595602057009,0.98839306168272));
#83160=DIRECTION('',(0.563147788029111,0.,0.826356199733456));
#83161=DIRECTION('',(0.826356198741165,0.,-0.563147789485187));
#83162=DIRECTION('center_axis',(-0.154002421975287,-0.987363722280647,-0.0373648758843351));
#83163=DIRECTION('ref_axis',(-0.359450020738448,0.0207595567062281,0.932933397084963));
#83164=DIRECTION('',(0.372339549379017,0.,0.928096579009012));
#83165=DIRECTION('center_axis',(-4.32394255814854E-15,-1.,1.42022434872714E-14));
#83166=DIRECTION('ref_axis',(9.72412122363789E-32,-1.42022434872714E-14,
-1.));
#83167=DIRECTION('center_axis',(0.157871536511912,0.98736372308643,0.0137643122702139));
#83168=DIRECTION('ref_axis',(-0.214962170603115,0.0207592293548863,0.976401720403128));
#83169=DIRECTION('center_axis',(-0.156018989066482,0.987363721752651,-0.0277660947457013));
#83170=DIRECTION('ref_axis',(-0.288435909505167,-0.0186562580954878,0.957317434366366));
#83171=DIRECTION('',(0.92809657835293,0.,-0.372339551014372));
#83172=DIRECTION('center_axis',(-0.142369586171416,-0.987363722340502,-0.0695972753725918));
#83173=DIRECTION('ref_axis',(-0.551599383034971,0.0207595554529733,0.833850802897517));
#83174=DIRECTION('',(0.164121129029902,0.,0.986440193324436));
#83175=DIRECTION('center_axis',(-1.45518274130907E-14,-1.,2.58813661411197E-14));
#83176=DIRECTION('ref_axis',(3.468830684141E-31,-2.58813661411197E-14,-1.));
#83177=DIRECTION('center_axis',(0.151221665785298,0.98736372318903,0.0473802271777533));
#83178=DIRECTION('ref_axis',(-0.41983398324885,0.0207592259088541,0.907363477912281));
#83179=DIRECTION('center_axis',(-0.146402463399386,0.987363721717716,-0.0606564072982545));
#83180=DIRECTION('ref_axis',(-0.487487389798135,-0.0186562610013775,0.872930689524231));
#83181=DIRECTION('',(0.986440193500669,0.,-0.164121127970665));
#83182=DIRECTION('center_axis',(-0.124079706088548,-0.987363722361159,-0.0985753838546666));
#83183=DIRECTION('ref_axis',(-0.717956569952352,0.0207595533658661,0.695778272588548));
#83184=DIRECTION('',(-0.0517714178151324,0.,0.998658960955846));
#83185=DIRECTION('center_axis',(-2.96630136708453E-14,-1.,3.32220921542847E-14));
#83186=DIRECTION('ref_axis',(7.94211428211299E-31,-3.32220921542847E-14,
-1.));
#83187=DIRECTION('center_axis',(0.137500844342313,0.987363722957583,0.0787806854025349));
#83188=DIRECTION('ref_axis',(-0.60507482268427,0.020759234097064,0.795897928853507));
#83189=DIRECTION('center_axis',(-0.12994032206456,0.987363721679227,-0.0907104945058956));
#83190=DIRECTION('ref_axis',(-0.66374449884885,-0.0186562630185771,0.747726677401623));
#83191=DIRECTION('',(0.998658961195707,0.,0.0517714131882863));
#83192=DIRECTION('center_axis',(-0.0999879970011825,-0.987363722364416,
-0.122944215863846));
#83193=DIRECTION('ref_axis',(-0.850742905726827,0.0207595522304107,0.525171923608515));
#83194=DIRECTION('',(-0.265243185223135,0.,0.964181545505143));
#83195=DIRECTION('center_axis',(9.62967379208464E-14,-1.,-6.95165520896173E-14));
#83196=DIRECTION('ref_axis',(1.,9.62967379208465E-14,1.36148196072087E-30));
#83197=DIRECTION('center_axis',(0.117350631393154,0.987363722976472,0.106497454719203));
#83198=DIRECTION('ref_axis',(-0.762023036778937,0.0207592324872928,0.647217077714073));
#83199=DIRECTION('center_axis',(-0.107402310027922,0.987363721799827,-0.116523064988271));
#83200=DIRECTION('ref_axis',(-0.808965654938278,-0.0186562575082339,0.587559795413258));
#83201=DIRECTION('',(0.964181545972515,0.,0.265243183524199));
#83202=DIRECTION('center_axis',(-0.0712209641401703,-0.987363722346009,
-0.141564310692975));
#83203=DIRECTION('ref_axis',(-0.943749448360311,0.0207595554677546,0.330009120444254));
#83204=DIRECTION('',(-0.466312478831761,0.,0.884620072169843));
#83205=DIRECTION('center_axis',(-1.08989377379274E-13,-1.,4.71903415295343E-14));
#83206=DIRECTION('ref_axis',(1.,-1.08989377379274E-13,-4.28536810502175E-31));
#83207=DIRECTION('center_axis',(0.0917132337655013,0.987363722983199,0.129234520500645));
#83208=DIRECTION('ref_axis',(-0.883339902800466,0.0207592324290681,0.468273072458175));
#83209=DIRECTION('center_axis',(-0.0798422878900739,0.98736372183659,-0.136887142805579));
#83210=DIRECTION('ref_axis',(-0.916360475668615,-0.0186562562932369,0.399919270270277));
#83211=DIRECTION('',(0.8846200741774,0.,0.466312475023317));
#83212=DIRECTION('center_axis',(-0.0391237163265227,-0.987363722297884,
-0.153565017861715));
#83213=DIRECTION('ref_axis',(-0.992627316897588,0.0207595568304632,0.119415453559823));
#83214=DIRECTION('',(-0.645577518758643,0.,0.763694747443921));
#83215=DIRECTION('center_axis',(-4.3719673062391E-14,-1.,8.49658617979204E-15));
#83216=DIRECTION('ref_axis',(1.,-4.3719673062391E-14,3.94366309046456E-32));
#83217=DIRECTION('center_axis',(0.0617874283049422,0.987363722959405,0.145928723311089));
#83218=DIRECTION('ref_axis',(-0.963352775381175,0.0207592332646177,0.267433140054953));
#83219=DIRECTION('center_axis',(-0.0485489300449553,0.987363721841696,-0.150850529274524));
#83220=DIRECTION('ref_axis',(-0.980907298568706,-0.018656256121526,0.193578965081882));
#83221=DIRECTION('',(0.763694749779609,0.,0.645577515995608));
#83222=DIRECTION('center_axis',(-0.00519708773014777,-0.987363722309297,
-0.158385195478159));
#83223=DIRECTION('ref_axis',(-0.995091034656455,0.0207595581066054,-0.0967619423821432));
#83224=DIRECTION('',(-0.794656070501521,0.,0.607059906117248));
#83225=DIRECTION('center_axis',(2.96826975295269E-14,-1.,7.33664433365271E-16));
#83226=DIRECTION('ref_axis',(-0.999694677174641,-2.9691763102419E-14,-0.0247093591315182));
#83227=DIRECTION('center_axis',(0.028972516634715,0.987363722781084,0.155799461538642));
#83228=DIRECTION('ref_axis',(-0.998320342515947,0.0207592391582244,0.0540883324610285));
#83229=DIRECTION('center_axis',(-0.0149854786283017,0.987363721847577,-0.157760312530055));
#83230=DIRECTION('ref_axis',(-0.999587986357288,-0.0186562564288687,-0.0218128775323698));
#83231=DIRECTION('',(0.607059907517467,0.,0.794656069431855));
#83232=DIRECTION('center_axis',(0.0289725563100853,-0.987363722322521,-0.155799457066687));
#83233=DIRECTION('ref_axis',(-0.951025401157534,0.0207595545961579,-0.308414862232871));
#83234=DIRECTION('',(-0.906577388181206,0.,0.422039618091172));
#83235=DIRECTION('center_axis',(-7.20775410205984E-14,-1.,-1.77435358103594E-14));
#83236=DIRECTION('ref_axis',(1.,-7.20775410205984E-14,-5.0910909284395E-31));
#83237=DIRECTION('center_axis',(-0.00519712986190833,0.987363722957772,
0.158385190053129));
#83238=DIRECTION('ref_axis',(-0.986607560385699,0.0207592326909068,-0.161785586650553));
#83239=DIRECTION('center_axis',(0.0192786812815472,0.987363721912878,-0.157293398139886));
#83240=DIRECTION('ref_axis',(-0.971529050833944,-0.0186562524121231,-0.236184774343376));
#83241=DIRECTION('',(0.422039619688627,0.,0.906577387437542));
#83242=DIRECTION('center_axis',(0.0617874731942246,-0.987363722350534,-0.145928708424253));
#83243=DIRECTION('ref_axis',(-0.862490877748826,0.0207595528997825,-0.505646642195377));
#83244=DIRECTION('',(-0.976108155148253,0.,0.217285226034985));
#83245=DIRECTION('center_axis',(7.9893686956293E-14,-1.,3.93878910334263E-14));
#83246=DIRECTION('ref_axis',(1.,7.9893686956293E-14,7.57869122091651E-31));
#83247=DIRECTION('center_axis',(-0.0391237546114933,0.987363722897334,0.153565004253628));
#83248=DIRECTION('ref_axis',(-0.928762104735744,0.0207592363557858,-0.370094591844781));
#83249=DIRECTION('center_axis',(0.0526413843344021,0.987363721816876,-0.149471621036518));
#83250=DIRECTION('ref_axis',(-0.898042496937889,-0.0186562558923963,-0.439512932471434));
#83251=DIRECTION('',(0.21728522775494,0.,0.976108154765385));
#83252=DIRECTION('center_axis',(0.0917132761324331,-0.987363722364209,-0.129234495163442));
#83253=DIRECTION('ref_axis',(-0.733627238879286,0.0207595515989269,-0.679234948594201));
#83254=DIRECTION('',(-0.999997189610847,0.,0.00237081640126621));
#83255=DIRECTION('center_axis',(-3.47792923060787E-14,-1.,-2.782090251181E-14));
#83256=DIRECTION('ref_axis',(1.,-3.47792923060787E-14,-7.51127384914101E-31));
#83257=DIRECTION('center_axis',(-0.0712210092506948,0.98736372322825,0.141564281844537));
#83258=DIRECTION('ref_axis',(-0.82748876612426,0.020759224011969,-0.561098384025984));
#83259=DIRECTION('center_axis',(0.0835426338265499,0.987363721708827,-0.134660719538468));
#83260=DIRECTION('ref_axis',(-0.782564473587812,-0.0186562616054858,-0.622289955391487));
#83261=DIRECTION('',(0.00237082103812565,0.,0.999997189599853));
#83262=DIRECTION('center_axis',(0.117350665271771,-0.987363722334509,-0.106497423339791));
#83263=DIRECTION('ref_axis',(-0.570460005892413,0.0207595544146053,-0.821062983319633));
#83264=DIRECTION('',(-0.977127466912818,0.,-0.212654446002285));
#83265=DIRECTION('center_axis',(-1.86570000645977E-14,-1.,-2.30979900170607E-14));
#83266=DIRECTION('ref_axis',(4.88212395773465E-31,2.30979900170607E-14,
-1.));
#83267=DIRECTION('center_axis',(-0.0999880321934036,0.987363722991602,0.122944182205804));
#83268=DIRECTION('ref_axis',(-0.687522971709477,0.0207592324695274,-0.725865839972543));
#83269=DIRECTION('center_axis',(0.110537530221466,0.987363721825394,-0.113553226443133));
#83270=DIRECTION('ref_axis',(-0.630494605257325,-0.0186562572179942,-0.775969391669559));
#83271=DIRECTION('',(-0.212654444280544,0.,0.977127467287525));
#83272=DIRECTION('center_axis',(0.137500868251949,-0.987363722272268,-0.0787806522606443));
#83273=DIRECTION('ref_axis',(-0.380618696773504,0.0207595585214019,-0.924499025633038));
#83274=DIRECTION('',(-0.908568350643389,0.,-0.417736223242793));
#83275=DIRECTION('center_axis',(-3.31385617699243E-14,-1.,-6.64216885082524E-14));
#83276=DIRECTION('ref_axis',(-6.03805196582697E-31,6.64216885082524E-14,
-1.));
#83277=DIRECTION('center_axis',(-0.12407973107399,0.987363722900487,0.0985753470026679));
#83278=DIRECTION('ref_axis',(-0.515409366918908,0.0207592357297002,-0.85669261618399));
#83279=DIRECTION('center_axis',(0.132363809458612,0.987363721692603,-0.087136117832598));
#83280=DIRECTION('ref_axis',(-0.448943511408003,-0.0186562616387398,-0.893365360569974));
#83281=DIRECTION('',(-0.41773622273295,0.,0.908568350877801));
#83282=DIRECTION('center_axis',(0.151221686204625,-0.987363722346416,-0.0473801795654959));
#83283=DIRECTION('ref_axis',(-0.172980080774042,0.0207595558008577,-0.984706520999205));
#83284=DIRECTION('',(-0.797525585226132,0.,-0.603285124058033));
#83285=DIRECTION('center_axis',(-1.08510605719282E-14,-1.,-4.31955584310798E-14));
#83286=DIRECTION('ref_axis',(1.02420910079709E-32,4.31955584310798E-14,
-1.));
#83287=DIRECTION('center_axis',(-0.142369603550258,0.987363723128988,0.069597228635955));
#83288=DIRECTION('ref_axis',(-0.319195796297111,0.0207592278209998,-0.947461396620743));
#83289=DIRECTION('center_axis',(0.148000906130631,0.987363721679453,-0.0566446193014943));
#83290=DIRECTION('ref_axis',(-0.246400316544395,-0.0186562636632086,-0.968988559185789));
#83291=DIRECTION('',(-0.603285121269556,0.,0.797525587335464));
#83292=DIRECTION('',(-0.649191412957101,3.74026243672172E-15,-0.76062507803961));
#83293=DIRECTION('',(-0.760625076895703,0.,0.64919141429736));
#83294=DIRECTION('center_axis',(0.15713950675887,-0.987363722295113,0.0204952509405883));
#83295=DIRECTION('ref_axis',(0.256475066635952,0.02075955649749,-0.966327884834186));
#83296=DIRECTION('',(-0.470501770976394,0.,-0.882399050038064));
#83297=DIRECTION('center_axis',(2.76306279419956E-15,-1.,-1.45864897414642E-14));
#83298=DIRECTION('ref_axis',(-4.09279871659108E-32,1.45864897414642E-14,
-1.));
#83299=DIRECTION('center_axis',(-0.158434270677379,0.987363723095254,0.00338529029850841));
#83300=DIRECTION('ref_axis',(0.108134457296577,0.0207592293236594,-0.993919510595834));
#83301=DIRECTION('center_axis',(0.158106442288904,0.987363721720486,0.010734707122974));
#83302=DIRECTION('ref_axis',(0.18324086639066,-0.0186562600823441,-0.982891005576987));
#83303=DIRECTION('',(-0.882399049845416,0.,0.470501771337694));
#83304=DIRECTION('center_axis',(0.149059797579392,-0.98736372234962,0.0537964360668407));
#83305=DIRECTION('ref_axis',(0.458210753203742,0.0207595523637838,-0.888601117844286));
#83306=DIRECTION('',(-0.26981198698136,0.,-0.9629130239441));
#83307=DIRECTION('center_axis',(0.,-1.,0.));
#83308=DIRECTION('ref_axis',(0.,0.,-1.));
#83309=DIRECTION('center_axis',(-0.155457905398942,0.987363722888109,-0.0307525344241237));
#83310=DIRECTION('ref_axis',(0.319269649296509,0.0207592364372728,-0.94743651245908));
#83311=DIRECTION('center_axis',(0.152102355397201,0.987363721802279,0.0444719501638507));
#83312=DIRECTION('ref_axis',(0.390249308908463,-0.0186562566933496,-0.920520190426402));
#83313=DIRECTION('',(-0.962913022721775,0.,0.26981199134363));
#83314=DIRECTION('center_axis',(0.134010221269008,-0.987363722314795,0.084582152089576));
#83315=DIRECTION('ref_axis',(0.63852101350025,0.0207595566138072,-0.769324350406128));
#83316=DIRECTION('',(-0.0565060964350291,0.,-0.998402254136916));
#83317=DIRECTION('center_axis',(-4.31619796904112E-14,-1.,6.039079790533E-14));
#83318=DIRECTION('ref_axis',(-9.67732215104448E-31,-6.039079790533E-14,
-1.));
#83319=DIRECTION('center_axis',(-0.145212496255427,0.987363723096625,-0.0634524171646621));
#83320=DIRECTION('ref_axis',(0.515476145884545,0.0207592294934855,-0.856652436764673));
#83321=DIRECTION('center_axis',(0.138986131034853,0.987363721861035,0.076129732251514));
#83322=DIRECTION('ref_axis',(0.57901012730644,-0.0186562549495507,-0.815106874359331));
#83323=DIRECTION('',(-0.998402253875163,0.,0.0565061010599261));
#83324=DIRECTION('center_axis',(0.112694472634348,-0.987363722352503,0.111412905984339));
#83325=DIRECTION('ref_axis',(0.788974741981374,0.0207595546116365,-0.614074830462665));
#83326=DIRECTION('',(0.15944195467659,0.,-0.987207305022055));
#83327=DIRECTION('center_axis',(9.92432034065362E-14,-1.,-8.9460620704829E-14));
#83328=DIRECTION('ref_axis',(1.,9.92432034065362E-14,1.52267170892412E-30));
#83329=DIRECTION('center_axis',(-0.128177111838365,0.987363723176768,-0.0931853322969094));
#83330=DIRECTION('ref_axis',(0.687579553211328,0.0207592255307392,-0.725812243325417));
#83331=DIRECTION('center_axis',(0.11937107285857,0.987363721788263,0.104227769145382));
#83332=DIRECTION('ref_axis',(0.740697075790419,-0.0186562581167305,-0.671580066670091));
#83333=DIRECTION('',(-0.987207304850248,0.,-0.159441955740358));
#83334=DIRECTION('center_axis',(0.0861092603822379,-0.987363722265456,0.133034113033189));
#83335=DIRECTION('ref_axis',(0.902536886948628,0.0207595581119766,-0.430111855735313));
#83336=DIRECTION('',(0.367934678144182,0.,-0.929851640111979));
#83337=DIRECTION('center_axis',(3.87181138908445E-14,-1.,-2.20115753669646E-14));
#83338=DIRECTION('ref_axis',(1.,3.87181138908445E-14,-5.29240579877378E-31));
#83339=DIRECTION('center_axis',(-0.105148313695901,0.987363723085993,-0.118560998902152));
#83340=DIRECTION('ref_axis',(0.827532501342244,0.0207592292772026,-0.561033879210574));
#83341=DIRECTION('center_axis',(0.0941743549645455,0.987363721723206,0.127452233765876));
#83342=DIRECTION('ref_axis',(0.867749851718935,-0.0186562587549658,-0.496650922531142));
#83343=DIRECTION('',(-0.929851640370812,0.,-0.367934677490054));
#83344=DIRECTION('center_axis',(0.0554976663461317,-0.987363722373159,0.148434796363768));
#83345=DIRECTION('ref_axis',(0.973897411717727,0.0207595527340627,-0.226037325280125));
#83346=DIRECTION('',(0.559223188237572,0.,-0.829017144417053));
#83347=DIRECTION('center_axis',(2.83631625789902E-14,-1.,-8.78247130185755E-15));
#83348=DIRECTION('ref_axis',(1.,2.83631625789902E-14,-2.50109950454817E-31));
#83349=DIRECTION('center_axis',(-0.0772028993467409,0.987363722956136,-0.138392886098437));
#83350=DIRECTION('ref_axis',(0.928790951318559,0.0207592346313163,-0.370022192478082));
#83351=DIRECTION('center_axis',(0.0645741468664167,0.987363721787944,0.144717174010324));
#83352=DIRECTION('ref_axis',(0.95422761013519,-0.0186562576921633,-0.298498931496591));
#83353=DIRECTION('',(-0.829017145402445,0.,-0.559223186776784));
#83354=DIRECTION('center_axis',(0.0222910694351928,-0.987363722348557,0.156894831060289));
#83355=DIRECTION('ref_axis',(0.999719574720903,0.0207595537623816,-0.0113935441124832));
#83356=DIRECTION('',(0.724363041874931,0.,-0.689418728760466));
#83357=DIRECTION('center_axis',(-1.47940096643841E-14,-1.,1.23995022967283E-15));
#83358=DIRECTION('ref_axis',(1.,-1.47940096643841E-14,-1.11149104892168E-32));
#83359=DIRECTION('center_axis',(-0.0456475581498243,0.987363722973727,-0.151753678671785));
#83360=DIRECTION('ref_axis',(0.986620168387057,0.0207592337038213,-0.161708681114913));
#83361=DIRECTION('center_axis',(0.0319545266572246,0.987363721747205,0.155215299515288));
#83362=DIRECTION('ref_axis',(0.996086745484081,-0.0186562596592667,-0.0863894637467843));
#83363=DIRECTION('',(-0.689418728599904,0.,-0.724363042027747));
#83364=DIRECTION('center_axis',(-0.0119578282286655,-0.987363722267693,
0.158018639070651));
#83365=DIRECTION('ref_axis',(0.978795961913238,0.0207595597848566,0.203782986581015));
#83366=DIRECTION('',(0.855632484051998,0.,-0.517583860099026));
#83367=DIRECTION('center_axis',(1.32432179419927E-13,-1.,1.77238250181088E-14));
#83368=DIRECTION('ref_axis',(1.,1.32432179419927E-13,-2.65043621295196E-31));
#83369=DIRECTION('center_axis',(-0.0119577902703965,0.987363722876856,-0.158018638136787));
#83370=DIRECTION('ref_axis',(0.998316123369291,0.0207592357518346,0.0541661513485184));
#83371=DIRECTION('center_axis',(-0.00215925399566002,0.987363721770524,
0.158455730580002));
#83372=DIRECTION('ref_axis',(0.991369971740769,-0.0186562595974695,0.129759481767379));
#83373=DIRECTION('',(-0.517583861605946,0.,-0.855632483140441));
#83374=DIRECTION('center_axis',(-0.0456476012493495,-0.987363722312714,
0.151753670008215));
#83375=DIRECTION('ref_axis',(0.912104937720815,0.0207595555807828,0.409430853059947));
#83376=DIRECTION('',(0.946893502365912,0.,-0.321547345156537));
#83377=DIRECTION('center_axis',(-9.76312478759136E-14,-1.,-3.56054655558263E-14));
#83378=DIRECTION('ref_axis',(1.,-9.76312478759136E-14,-8.59526417176721E-31));
#83379=DIRECTION('center_axis',(0.0222911163562628,0.987363723032372,-0.156894820090549));
#83380=DIRECTION('ref_axis',(0.963331926327018,0.0207592312244037,0.267508231720164));
#83381=DIRECTION('center_axis',(-0.0361720677920674,0.987363721674074,0.154286949005961));
#83382=DIRECTION('ref_axis',(0.940297840452972,-0.0186562617608721,0.339841014500292));
#83383=DIRECTION('',(-0.32154734682426,0.,-0.946893501799584));
#83384=DIRECTION('center_axis',(-0.0772029402015664,-0.987363722356275,
0.138392867587147));
#83385=DIRECTION('ref_axis',(0.802764900110338,0.0207595540381597,0.595934187697749));
#83386=DIRECTION('',(0.993878832740327,0.,-0.110475634556792));
#83387=DIRECTION('center_axis',(7.51667665024089E-14,-1.,4.77950244623643E-14));
#83388=DIRECTION('ref_axis',(1.,7.51667665024089E-14,2.19098282777113E-31));
#83389=DIRECTION('center_axis',(0.0554977124760272,0.987363723067266,-0.148434774499359));
#83390=DIRECTION('ref_axis',(0.883303398270499,0.0207592297355248,0.46834192742544));
#83391=DIRECTION('center_axis',(-0.0684935226579129,0.98736372182022,0.142903877439465));
#83392=DIRECTION('ref_axis',(0.845258426819615,-0.0186562564228737,0.534031961577875));
#83393=DIRECTION('',(-0.110475636307964,0.,-0.993878832545673));
#83394=DIRECTION('center_axis',(-0.105148352850834,-0.987363722301292,0.118560970711675));
#83395=DIRECTION('ref_axis',(0.655888469378332,0.0207595557135769,0.754572300434573));
#83396=DIRECTION('',(0.99439149393359,0.,0.105761792687731));
#83397=DIRECTION('center_axis',(2.10449639732453E-14,-1.,2.09454121104238E-14));
#83398=DIRECTION('ref_axis',(1.,2.10449639732453E-14,6.31337018212632E-32));
#83399=DIRECTION('center_axis',(0.0861092934140696,0.987363722975823,-0.133034086380344));
#83400=DIRECTION('ref_axis',(0.76197258528134,0.0207592328245021,0.647276473797873));
#83401=DIRECTION('center_axis',(-0.0976122906414578,0.987363721776479,0.124838782577484));
#83402=DIRECTION('ref_axis',(0.710695667994112,-0.0186562580397901,0.703252167810633));
#83403=DIRECTION('',(0.105761793778192,0.,-0.994391493817611));
#83404=DIRECTION('center_axis',(-0.128177146779924,-0.987363722313685,0.0931852933794923));
#83405=DIRECTION('ref_axis',(0.478343420119804,0.0207595560447544,0.87792745330176));
#83406=DIRECTION('',(0.948407514082987,0.,0.317053918491681));
#83407=DIRECTION('center_axis',(3.21005998968575E-14,-1.,4.99595303694677E-14));
#83408=DIRECTION('ref_axis',(-1.62345145347269E-32,-4.99595303694677E-14,
-1.));
#83409=DIRECTION('center_axis',(0.112694502133346,0.987363722956734,-0.111412870791198));
#83410=DIRECTION('ref_axis',(0.605012781775338,0.0207592327885922,0.7959450911605));
#83411=DIRECTION('center_axis',(-0.122166815496786,0.987363721684866,0.100936367539084));
#83412=DIRECTION('ref_axis',(0.542901569720667,-0.0186562621546152,0.839589083705388));
#83413=DIRECTION('',(0.317053919406767,0.,-0.948407513777072));
#83414=DIRECTION('center_axis',(-0.145212520777593,-0.987363722355149,0.0634523725829109));
#83415=DIRECTION('ref_axis',(0.278431566842413,0.0207595529164433,0.960231692639015));
#83416=DIRECTION('',(0.858077052116883,0.,0.51352095636926));
#83417=DIRECTION('center_axis',(2.06102834792613E-14,-1.,5.56921844170132E-14));
#83418=DIRECTION('ref_axis',(1.55831017715474E-31,-5.56921844170132E-14,
-1.));
#83419=DIRECTION('center_axis',(0.134010239663865,0.987363722853647,-0.0845821166548784));
#83420=DIRECTION('ref_axis',(0.419763252540507,0.0207592367336559,0.907396201175016));
#83421=DIRECTION('center_axis',(-0.141008959833401,0.987363721776961,0.0723142735941615));
#83422=DIRECTION('ref_axis',(0.349721999250997,-0.0186562580065864,0.936667746469941));
#83423=DIRECTION('',(0.513520954857275,0.,-0.858077053021739));
#83424=DIRECTION('center_axis',(-0.155457916612102,-0.987363722303317,0.0307524965159346));
#83425=DIRECTION('ref_axis',(0.0655005617138484,0.020759557685025,0.997636565679051));
#83426=DIRECTION('',(0.727623861282843,0.,0.685976323565068));
#83427=DIRECTION('center_axis',(-6.11718982189012E-15,-1.,-4.41155503170608E-14));
#83428=DIRECTION('ref_axis',(-2.5998598857542E-32,4.41155503170608E-14,
-1.));
#83429=DIRECTION('center_axis',(0.149059810412648,0.987363723002602,-0.0537963885236487));
#83430=DIRECTION('ref_axis',(0.214886058244713,0.0207592318881922,0.976418473946218));
#83431=DIRECTION('center_axis',(-0.153257680116604,0.987363721845255,0.0403108455525592));
#83432=DIRECTION('ref_axis',(0.140189813985162,-0.0186562558720133,0.989948867453084));
#83433=DIRECTION('center_axis',(-7.01873189011981E-15,-1.,8.87983364791519E-14));
#83434=DIRECTION('ref_axis',(1.3690381083063E-31,-8.87983364791519E-14,
-1.));
#83435=DIRECTION('center_axis',(0.157139508177808,0.987363722970567,-0.0204952075212232));
#83436=DIRECTION('ref_axis',(-3.89661523431908E-5,0.0207592334146242,0.999784503135389));
#83437=DIRECTION('center_axis',(-0.158340241192816,0.987363721799664,0.00642253010240786));
#83438=DIRECTION('ref_axis',(-0.0758974889019666,-0.018656256436268,0.996941079138662));
#83439=DIRECTION('',(0.68597632228297,0.,-0.727623862491556));
#83440=DIRECTION('center_axis',(0.163550506959679,-0.986495108643176,0.00886748534365151));
#83441=DIRECTION('ref_axis',(0.0262170039174905,0.0133314937162301,0.999567376408856));
#83442=DIRECTION('center_axis',(-0.160229039203745,-0.98649510925111,0.0339713764732357));
#83443=DIRECTION('ref_axis',(0.138731003294514,0.0115680715646117,0.990262535111358));
#83444=DIRECTION('center_axis',(0.161633050324773,-0.98649510723104,-0.0264983103598656));
#83445=DIRECTION('ref_axis',(0.240481465453549,0.0133315360443304,0.970562174680227));
#83446=DIRECTION('center_axis',(-0.149180133269807,-0.986495109263739,0.0676216476901187));
#83447=DIRECTION('ref_axis',(0.348364721933479,0.0115680673112049,0.937287682801227));
#83448=DIRECTION('center_axis',(0.152157803025431,-0.986495107357098,-0.0606251279502263));
#83449=DIRECTION('ref_axis',(0.443501319199322,0.013331529601327,0.896174564572634));
#83450=DIRECTION('center_axis',(-0.131155729272303,-0.986495109286855,0.0981100098469422));
#83451=DIRECTION('ref_axis',(0.541709293051917,0.0115680673377809,0.840486300685062));
#83452=DIRECTION('center_axis',(0.135567830578251,-0.986495107258517,-0.0919171728640135));
#83453=DIRECTION('ref_axis',(0.625783546599744,0.0133315341903691,0.779882826456114));
#83454=DIRECTION('center_axis',(-0.106998624069017,-0.986495109229355,0.124010862080306));
#83455=DIRECTION('ref_axis',(0.709724143246153,0.0115680739444168,0.704384710338556));
#83456=DIRECTION('center_axis',(0.112638853169902,-0.986495107286684,-0.11891127808582));
#83457=DIRECTION('ref_axis',(0.778804829717616,0.0133315319382028,0.627124634713624));
#83458=DIRECTION('center_axis',(-0.0778383928847543,-0.986495109242355,
0.144113094595991));
#83459=DIRECTION('ref_axis',(0.844553077683583,0.0115680663400262,0.535346877095908));
#83460=DIRECTION('center_axis',(0.0844430093730047,-0.986495107287699,-0.140345222453287));
#83461=DIRECTION('ref_axis',(0.895410064196242,0.0133315316262661,0.445042792549863));
#83462=DIRECTION('center_axis',(-0.0450385179583259,-0.986495109255801,
0.157476764363836));
#83463=DIRECTION('ref_axis',(0.939891649508408,0.0115680677193456,0.341276818717012));
#83464=DIRECTION('center_axis',(0.0522987062510939,-0.986495107258399,-0.1552167796332));
#83465=DIRECTION('ref_axis',(0.970146919221119,0.0133315332775466,0.242151244775328));
#83466=DIRECTION('center_axis',(-0.0101326912773838,-0.986495109255921,
0.163476995267303));
#83467=DIRECTION('ref_axis',(0.991281933042656,0.0115680694691132,0.131249034251579));
#83468=DIRECTION('center_axis',(0.0177089702822737,-0.986495107305781,-0.162830573398542));
#83469=DIRECTION('ref_axis',(0.999520783098335,0.0133315315275395,0.0279369723059262));
#83470=DIRECTION('center_axis',(0.0252469209161869,-0.986495109272429,0.1618332239246));
#83471=DIRECTION('ref_axis',(0.996320974931463,0.0115680629516839,-0.0849158102544182));
#83472=DIRECTION('center_axis',(-0.0177088158145139,-0.986495107315351,
-0.162830590139942));
#83473=DIRECTION('ref_axis',(0.98215816532745,0.0133315318177788,-0.187583604134287));
#83474=DIRECTION('center_axis',(0.0594460241247487,-0.986495109265875,0.152622310329353));
#83475=DIRECTION('ref_axis',(0.954773155677358,0.0115680663260198,-0.297110082359009));
#83476=DIRECTION('center_axis',(-0.0522985590052692,-0.986495107345191,
-0.155216828694483));
#83477=DIRECTION('ref_axis',(0.918870923356613,0.0133315297702083,-0.394332976713528));
#83478=DIRECTION('center_axis',(0.0908654951821714,-0.986495109267404,0.136274946988765));
#83479=DIRECTION('ref_axis',(0.868581205501574,0.0115680676184969,-0.495411817845524));
#83480=DIRECTION('center_axis',(-0.0844428741895767,-0.98649510726196,-0.140345303971376));
#83481=DIRECTION('ref_axis',(0.812618298321134,0.0133315342674835,-0.58264377747277));
#83482=DIRECTION('center_axis',(0.118036198596521,-0.986495109232563,0.113555516295406));
#83483=DIRECTION('ref_axis',(0.741775361464524,0.0115680711949706,-0.670548650623505));
#83484=DIRECTION('center_axis',(-0.11263873867622,-0.986495107271142,-0.118911386668935));
#83485=DIRECTION('ref_axis',(0.668368546867031,0.0133315334872308,-0.743710801167854));
#83486=DIRECTION('center_axis',(0.139687655736812,-0.986495109271077,0.0855263597904134));
#83487=DIRECTION('ref_axis',(0.580284927671301,0.0115680688497371,-0.814331371433399));
#83488=DIRECTION('center_axis',(-0.135567741482167,-0.986495107297552,-0.0919173038519721));
#83489=DIRECTION('ref_axis',(0.492866620788169,0.0133315323142876,-0.87000273813305));
#83490=DIRECTION('center_axis',(0.154807477127269,-0.986495109248506,0.0534980789773647));
#83491=DIRECTION('ref_axis',(0.391661014295995,0.0115680743258794,-0.920036863140289));
#83492=DIRECTION('center_axis',(-0.152157746667951,-0.98649510732727,-0.0606252698822009));
#83493=DIRECTION('ref_axis',(0.294318802411539,0.0133315306675126,-0.9556143117582));
#83494=DIRECTION('center_axis',(0.162688669256179,-0.986495109251213,0.0189682977383472));
#83495=DIRECTION('ref_axis',(0.184723468394355,0.0115680686706918,-0.982722453193978));
#83496=DIRECTION('center_axis',(-0.161633023909734,-0.98649510726897,-0.0264984700724086));
#83497=DIRECTION('ref_axis',(0.0820089640255199,0.0133315336497295,-0.996542422594245));
#83498=DIRECTION('center_axis',(0.16296272187791,-0.986495109263594,-0.0164484247620746));
#83499=DIRECTION('ref_axis',(-0.0308515416615133,0.011568068114073,-0.999457033682397));
#83500=DIRECTION('center_axis',(-0.163550521080517,-0.986495107309364,0.00886737328516426));
#83501=DIRECTION('ref_axis',(-0.134135522765056,0.0133315319656148,-0.990873317729363));
#83502=DIRECTION('center_axis',(0.155616817863015,-0.986495109242457,-0.0510960413232052));
#83503=DIRECTION('ref_axis',(-0.24498396980316,0.0115680715744787,-0.969458113721027));
#83504=DIRECTION('center_axis',(-0.157820578872764,-0.986495107230776,0.0438185838886268));
#83505=DIRECTION('ref_axis',(-0.34400798034835,0.0133315346117581,-0.938872078422585));
#83506=DIRECTION('center_axis',(0.140994445088194,-0.986495109264766,-0.0833544590946969));
#83507=DIRECTION('ref_axis',(-0.447661218276787,0.0115680704375784,-0.89412840990391));
#83508=DIRECTION('center_axis',(-0.144711118948954,-0.986495107322079,0.076720892083849));
#83509=DIRECTION('ref_axis',(-0.537795012205508,0.013331531453837,-0.842970221962777));
#83510=DIRECTION('center_axis',(0.119779331592619,-0.98649510928187,-0.111715312675464));
#83511=DIRECTION('ref_axis',(-0.629406325552992,0.0115680658336281,-0.776990255541696));
#83512=DIRECTION('center_axis',(-0.12483512904919,-0.986495107325552,0.106035813657553));
#83513=DIRECTION('ref_axis',(-0.706435342852236,0.0133315307102021,-0.707652016642479));
#83514=DIRECTION('center_axis',(0.0929634643369165,-0.986495109244733,-0.134852488796836));
#83515=DIRECTION('ref_axis',(-0.781721093297915,0.0115680696470281,-0.623520899455467));
#83516=DIRECTION('center_axis',(-0.099121994066111,-0.986495107175654,0.130392614096246));
#83517=DIRECTION('ref_axis',(-0.842043541607428,0.0133315380501615,-0.539244790545479));
#83518=DIRECTION('center_axis',(0.0618007367032678,-0.986495109255773,-0.151684107135105));
#83519=DIRECTION('ref_axis',(-0.897483449175347,0.0115680643638219,-0.440896403186959));
#83520=DIRECTION('center_axis',(-0.0687740162808509,-0.986495107239798,
0.148652406897909));
#83521=DIRECTION('ref_axis',(-0.9382787215921,0.0133315348704548,-0.345623076176191));
#83522=DIRECTION('center_axis',(0.0277482648204804,-0.986495109259417,-0.1614231495378));
#83523=DIRECTION('ref_axis',(-0.971280479329197,0.0115680697816831,-0.237656075528424));
#83524=DIRECTION('center_axis',(-0.035210239642401,-0.986495107333624,0.159961377310733));
#83525=DIRECTION('ref_axis',(-0.990641031576325,0.0133315299978489,-0.135840409544843));
#83526=DIRECTION('center_axis',(-0.00760168005493634,-0.986495109258894,
-0.163614222696638));
#83527=DIRECTION('ref_axis',(-0.999661512623984,0.0115680702645302,-0.0233032171316153));
#83528=DIRECTION('center_axis',(-8.08991190322417E-8,-0.986495107233334,
0.163790730521253));
#83529=DIRECTION('ref_axis',(-0.996682067559661,0.0133315344477418,0.080293999740133));
#83530=DIRECTION('center_axis',(-0.0425961788913145,-0.986495109233485,
-0.158154876631335));
#83531=DIRECTION('ref_axis',(-0.981299484699764,0.0115680705614484,0.192139275192408));
#83532=DIRECTION('center_axis',(0.0352100904617006,-0.986495107332138,0.159961410157052));
#83533=DIRECTION('ref_axis',(-0.956119357377107,0.0133315306025481,0.292673956375658));
#83534=DIRECTION('center_axis',(-0.0755989235215392,-0.986495109243415,
-0.145300386101373));
#83535=DIRECTION('ref_axis',(-0.917052983559382,0.0115680662317178,0.398597547895737));
#83536=DIRECTION('center_axis',(0.0687738742027003,-0.986495107341154,0.148652471957637));
#83537=DIRECTION('ref_axis',(-0.870849568622735,0.0133315291853619,0.491368801572887));
#83538=DIRECTION('center_axis',(-0.105066754479705,-0.986495109268846,-0.125651806559833));
#83539=DIRECTION('ref_axis',(-0.809926103476048,0.0115680712214746,0.586417843040541));
#83540=DIRECTION('center_axis',(0.0991218622055378,-0.986495107223832,0.130392713969553));
#83541=DIRECTION('ref_axis',(-0.744859823054238,0.0133315350752992,0.66708778595635));
#83542=DIRECTION('center_axis',(-0.129621774237956,-0.986495109274238,-0.100127893323553));
#83543=DIRECTION('ref_axis',(-0.664927980385921,0.0115680680390169,0.746817889918115));
#83544=DIRECTION('center_axis',(0.124835029130842,-0.986495107315024,0.106035931388474));
#83545=DIRECTION('ref_axis',(-0.584041259269706,0.0133315314906892,0.81161448837411));
#83546=DIRECTION('center_axis',(-0.148115826717122,-0.986495109262762,-0.0699221086392219));
#83547=DIRECTION('ref_axis',(-0.488838562437753,0.011568068288881,0.872297563718858));
#83548=DIRECTION('center_axis',(0.144711044899141,-0.986495107184836,0.076721033521315));
#83549=DIRECTION('ref_axis',(-0.395913577600531,0.0133315358117855,0.918190998226648));
#83550=DIRECTION('center_axis',(-0.159684149326762,-0.986495109228651,-0.036446836923669));
#83551=DIRECTION('ref_axis',(-0.28989159657348,0.0115680757083828,0.956989572493078));
#83552=DIRECTION('center_axis',(0.157820536374888,-0.986495107342756,0.0438187344311385));
#83553=DIRECTION('ref_axis',(-0.189273412709158,0.0133315291307049,0.981833919546715));
#83554=DIRECTION('center_axis',(-0.163785816964949,-0.986495108921018,-0.00126737367530744));
#83555=DIRECTION('ref_axis',(-0.0773896270365963,0.0115680610235149,0.996933812041348));
#83556=DIRECTION('center_axis',(-0.163785817306842,0.986495108821648,0.00126740683861602));
#83557=DIRECTION('ref_axis',(-0.0768446779811248,-0.0140392001935921,0.996944229294649));
#83558=DIRECTION('center_axis',(-0.160229061654718,0.986495107964944,-0.033971307930117));
#83559=DIRECTION('ref_axis',(-0.289361608418837,-0.0140392242780245,0.957116899733222));
#83560=DIRECTION('center_axis',(-0.149180170698907,0.986495107847839,-0.0676215857735171));
#83561=DIRECTION('ref_axis',(-0.488348336529291,-0.0140392289373408,0.872535845830943));
#83562=DIRECTION('center_axis',(-0.131155774091502,0.986495108033152,-0.0981099625375499));
#83563=DIRECTION('ref_axis',(-0.664500439371671,-0.0140392219614871,0.74715598526785));
#83564=DIRECTION('center_axis',(-0.106998686998783,0.986495107899956,-0.124010818358685));
#83565=DIRECTION('ref_axis',(-0.809581238604204,-0.0140392262583843,0.586839942596061));
#83566=DIRECTION('center_axis',(-0.0778384296784011,0.986495108808148,-0.144113077695263));
#83567=DIRECTION('ref_axis',(-0.916806922417426,-0.0140391983509365,0.399083910872326));
#83568=DIRECTION('center_axis',(-0.0450385871440512,0.986495107907963,-0.157476753020009));
#83569=DIRECTION('ref_axis',(-0.981163728413274,-0.0140392260617028,0.192667169434109));
#83570=DIRECTION('center_axis',(-0.0101327645796777,0.986495107901833,-0.163476998895024));
#83571=DIRECTION('ref_axis',(-0.999642411894656,-0.0140392275555301,-0.0227584804211519));
#83572=DIRECTION('center_axis',(0.0252468556544985,0.98649510787844,-0.161833242603198));
#83573=DIRECTION('ref_axis',(-0.971378926912717,-0.0140392284255323,-0.237119970510952));
#83574=DIRECTION('center_axis',(0.0594459620639049,0.986495107877398,-0.152622343476498));
#83575=DIRECTION('ref_axis',(-0.897694843465258,-0.0140392277430696,-0.440393991898465));
#83576=DIRECTION('center_axis',(0.0908654418332143,0.986495107903131,-0.136274992436783));
#83577=DIRECTION('ref_axis',(-0.782035544919108,-0.0140392268974693,-0.623075682875841));
#83578=DIRECTION('center_axis',(0.118036168365079,0.986495108253068,-0.113555556228917));
#83579=DIRECTION('ref_axis',(-0.629809135699137,-0.0140392025394138,-0.776623044585958));
#83580=DIRECTION('center_axis',(0.139687633297808,0.986495108711818,-0.0855264028900755));
#83581=DIRECTION('ref_axis',(-0.448133544647552,-0.0140392045032719,-0.893856379346557));
#83582=DIRECTION('center_axis',(0.154807463347207,0.986495108715876,-0.0534981286743339));
#83583=DIRECTION('ref_axis',(-0.245503734126674,-0.0140392015699084,-0.969293978805779));
#83584=DIRECTION('center_axis',(0.162688669059064,0.986495107942603,-0.0189683674864747));
#83585=DIRECTION('ref_axis',(-0.0313944450013707,-0.0140392248625478,-0.999408469540015));
#83586=DIRECTION('center_axis',(0.162962736978838,0.986495107917882,0.016448355858674));
#83587=DIRECTION('ref_axis',(0.184182820785979,-0.0140392266767644,-0.982791732078388));
#83588=DIRECTION('center_axis',(0.155616834415035,0.986495108793173,0.0510959995869567));
#83589=DIRECTION('ref_axis',(0.391147904392901,-0.0140391977490532,-0.920220744069381));
#83590=DIRECTION('center_axis',(0.140994474738935,0.986495108267932,0.0833544207377945));
#83591=DIRECTION('ref_axis',(0.579823339829956,-0.0140392019901395,-0.814621258865686));
#83592=DIRECTION('center_axis',(0.11977938301305,0.986495107934913,0.111715269437521));
#83593=DIRECTION('ref_axis',(0.741386879346129,-0.0140392247113993,-0.670930991461053));
#83594=DIRECTION('center_axis',(0.0929635116883181,0.98649510817471,0.134852463981731));
#83595=DIRECTION('ref_axis',(0.868283999279012,-0.0140392076646582,-0.495868729851151));
#83596=DIRECTION('center_axis',(0.0618007963427444,0.986495108013688,0.151684090914192));
#83597=DIRECTION('ref_axis',(0.954581119976345,-0.0140392215243303,-0.29762020368869));
#83598=DIRECTION('center_axis',(0.0277483051069888,0.986495108865338,0.16142314502095));
#83599=DIRECTION('ref_axis',(0.996243090992236,-0.0140391952154022,-0.0854552786429238));
#83600=DIRECTION('center_axis',(-0.00760161067101913,0.986495107971953,
0.163614233679749));
#83601=DIRECTION('ref_axis',(0.991321840591628,-0.0140392237424351,0.130705426676691));
#83602=DIRECTION('center_axis',(-0.0425961330144984,0.986495108686194,0.158154892401169));
#83603=DIRECTION('ref_axis',(0.940047482190855,-0.014039202231463,0.340754504045564));
#83604=DIRECTION('center_axis',(-0.0755988870791609,0.986495108778708,0.145300408217175));
#83605=DIRECTION('ref_axis',(0.844817547664969,-0.0140392009180133,0.534870275856615));
#83606=DIRECTION('center_axis',(-0.105066704035494,0.986495107904468,0.125651859451703));
#83607=DIRECTION('ref_axis',(0.710084888071399,-0.0140392256505157,0.703976101778862));
#83608=DIRECTION('center_axis',(-0.129621748001392,0.986495108655268,0.100127933386719));
#83609=DIRECTION('ref_axis',(0.542149443931951,-0.0140392038569982,0.840164794072769));
#83610=DIRECTION('center_axis',(-0.14811581037353,0.986495108721487,0.0699221508963698));
#83611=DIRECTION('ref_axis',(0.34886369311992,-0.0140392012981556,0.937068313651486));
#83612=DIRECTION('center_axis',(-0.159684140679065,0.986495108775018,0.0364468870900323));
#83613=DIRECTION('ref_axis',(0.139265465867208,-0.0140391994767074,0.990155558937505));
#83614=DIRECTION('center_axis',(-0.158434276191237,0.98736372208211,-0.00338532774206208));
#83615=DIRECTION('ref_axis',(0.13269176373348,0.0246892551673806,0.990849805226089));
#83616=DIRECTION('',(-0.72692697915403,0.,-0.68671476391439));
#83617=DIRECTION('center_axis',(-2.02413120793788E-15,-1.,-1.47072459452993E-14));
#83618=DIRECTION('ref_axis',(4.03217368274812E-32,1.47072459452993E-14,
-1.));
#83619=DIRECTION('center_axis',(-0.158420667353366,-0.987363722313518,0.00397139956531338));
#83620=DIRECTION('ref_axis',(0.0602919305233937,-0.0056588840615867,0.998164745993836));
#83621=DIRECTION('center_axis',(0.157139511088837,-0.98736372222782,-0.0204952209840727));
#83622=DIRECTION('ref_axis',(0.136228832793141,0.00111690644803579,0.990676767485644));
#83623=DIRECTION('center_axis',(0.156019001054146,0.987363720691631,-0.0277660651163378));
#83624=DIRECTION('ref_axis',(0.137583909697684,0.00611303106107622,0.990471250791029));
#83625=DIRECTION('',(-0.514391942141765,0.,0.857555205138202));
#83626=DIRECTION('center_axis',(-0.155457916667695,0.987363722050394,0.0307525043554571));
#83627=DIRECTION('ref_axis',(0.342592924413078,0.0246892566060478,0.939159479934231));
#83628=DIRECTION('',(-0.857555204217411,0.,-0.514391943676838));
#83629=DIRECTION('center_axis',(-2.05537251143393E-14,-1.,-5.57130813142657E-14));
#83630=DIRECTION('ref_axis',(5.84912470819078E-31,5.57130813142657E-14,
-1.));
#83631=DIRECTION('center_axis',(-0.153863147012197,-0.987363722313836,0.0379343096690717));
#83632=DIRECTION('ref_axis',(0.273458254901472,-0.00565888572755253,0.961867225680636));
#83633=DIRECTION('center_axis',(0.149059810143834,-0.987363722194988,-0.0537964040911902));
#83634=DIRECTION('ref_axis',(0.346010097831234,0.00111690617069978,0.938230123540822));
#83635=DIRECTION('center_axis',(0.146402480579443,0.98736372069204,-0.0606563825277796));
#83636=DIRECTION('ref_axis',(0.347289315232596,0.00611303022144713,0.93773810970163));
#83637=DIRECTION('',(-0.318016724021307,0.,0.948085103375618));
#83638=DIRECTION('center_axis',(-0.145212519477854,0.987363721982425,0.0634523813572531));
#83639=DIRECTION('ref_axis',(0.536474817340266,0.0246892601642735,0.843555102404264));
#83640=DIRECTION('',(-0.948085102432839,0.,-0.318016726831959));
#83641=DIRECTION('center_axis',(1.60249280290899E-14,-1.,2.49960485478454E-14));
#83642=DIRECTION('ref_axis',(2.56887509140615E-31,-2.49960485478454E-14,
-1.));
#83643=DIRECTION('center_axis',(-0.142111154973303,-0.987363722375813,0.0701234580460158));
#83644=DIRECTION('ref_axis',(0.473837973053062,-0.00565888198529935,0.880593863451048));
#83645=DIRECTION('center_axis',(0.134010234071191,-0.987363722256383,-0.0845821324879288));
#83646=DIRECTION('ref_axis',(0.539612318646171,0.0011168997964084,0.841912880350543));
#83647=DIRECTION('center_axis',(0.129940342043695,0.987363720690238,-0.0907104766512528));
#83648=DIRECTION('ref_axis',(0.540755859363086,0.00611303116878817,0.841157376127928));
#83649=DIRECTION('',(-0.106771401019337,0.,0.994283595320957));
#83650=DIRECTION('center_axis',(-0.128177144889255,0.987363721975308,0.0931852995654673));
#83651=DIRECTION('ref_axis',(0.705271747402913,0.0246892600517126,0.708507023785467));
#83652=DIRECTION('',(-0.994283595393053,0.,-0.106771400347955));
#83653=DIRECTION('center_axis',(3.15355285472734E-14,-1.,3.1450153513418E-14));
#83654=DIRECTION('ref_axis',(1.,3.15355285472734E-14,-6.7257412422847E-31));
#83655=DIRECTION('center_axis',(-0.1237142072212,-0.987363722295486,0.0990337055069238));
#83656=DIRECTION('ref_axis',(0.652061557236837,-0.00565888625187118,0.758144908695072));
#83657=DIRECTION('center_axis',(0.112694496579076,-0.987363722214071,-0.111412882990986));
#83658=DIRECTION('ref_axis',(0.707982863381585,0.0011169071748736,0.706228729008085));
#83659=DIRECTION('center_axis',(0.107402339291569,0.987363720693659,-0.116523047388375));
#83660=DIRECTION('ref_axis',(0.708937258694998,0.00611302945419982,0.705245059610426));
#83661=DIRECTION('',(0.109466440259237,0.,0.993990492136102));
#83662=DIRECTION('center_axis',(-0.105148350645483,0.987363721946392,0.118560975623103));
#83663=DIRECTION('ref_axis',(0.841090951872643,0.0246892610870285,0.540329946481729));
#83664=DIRECTION('',(-0.993990492096633,0.,0.10946644061763));
#83665=DIRECTION('center_axis',(7.51181976136774E-14,-1.,4.78713199577313E-14));
#83666=DIRECTION('ref_axis',(1.,7.51181976136774E-14,-2.23611908406028E-31));
#83667=DIRECTION('center_axis',(-0.0995325155372356,-0.987363722311601,
0.123313252385175));
#83668=DIRECTION('ref_axis',(0.799795464104186,-0.00565888214353483,0.600245943469221));
#83669=DIRECTION('center_axis',(0.086109278976296,-0.987363722241673,-0.13303410117429));
#83670=DIRECTION('ref_axis',(0.843248919199685,0.00111689985599072,0.53752210447876));
#83671=DIRECTION('center_axis',(0.079842323792572,0.987363720671974,-0.136887130265043));
#83672=DIRECTION('ref_axis',(0.843969540097002,0.00611302695943941,0.536356268062421));
#83673=DIRECTION('',(0.320585748995715,0.,0.947219498078907));
#83674=DIRECTION('center_axis',(-0.0772029325999934,0.987363721997434,0.138392874387865));
#83675=DIRECTION('ref_axis',(0.937581679979158,0.0246892581637656,0.34688763872295));
#83676=DIRECTION('',(-0.947219498157887,0.,0.320585748762358));
#83677=DIRECTION('center_axis',(5.57685963377941E-14,-1.,2.04026153647313E-14));
#83678=DIRECTION('ref_axis',(1.,5.57685963377941E-14,-5.33500706981931E-31));
#83679=DIRECTION('center_axis',(-0.0706968004725781,-0.98736372227437,0.141826804023219));
#83680=DIRECTION('ref_axis',(0.910131825527501,-0.00565888663633035,0.414280143337833));
#83681=DIRECTION('center_axis',(0.0554976970913057,-0.987363722217709,-0.148434785902608));
#83682=DIRECTION('ref_axis',(0.939085591280658,0.00111690456700952,0.343681545581436));
#83683=DIRECTION('center_axis',(0.0485489640099731,0.987363720692829,-0.150850525863092));
#83684=DIRECTION('ref_axis',(0.939538744720995,0.00611303092727423,0.342388051808148));
#83685=DIRECTION('',(0.516714824718151,0.,0.856157573064965));
#83686=DIRECTION('center_axis',(-0.0456475944673371,0.987363722009869,0.151753674018667));
#83687=DIRECTION('ref_axis',(0.990232129493659,0.0246892586075882,0.137225253608296));
#83688=DIRECTION('',(-0.85615757348362,0.,0.516714824024471));
#83689=DIRECTION('center_axis',(1.02988754365913E-13,-1.,1.38897742489236E-14));
#83690=DIRECTION('ref_axis',(1.,1.02988754365913E-13,-5.56147776580004E-32));
#83691=DIRECTION('center_axis',(-0.0385553735729892,-0.987363722347117,
0.153708695139513));
#83692=DIRECTION('ref_axis',(0.977911433889352,-0.00565888193743767,0.208943065268242));
#83693=DIRECTION('center_axis',(0.0222911022856109,-0.987363722208346,-0.156894827275387));
#83694=DIRECTION('ref_axis',(0.991011665082042,0.00111690628612727,0.133770819656857));
#83695=DIRECTION('center_axis',(0.014985513516289,0.987363720678149,-0.157760316535104));
#83696=DIRECTION('ref_axis',(0.991176161185229,0.00611302969020073,0.132410152050812));
#83697=DIRECTION('',(0.688682888958241,0.,0.725062672088511));
#83698=DIRECTION('center_axis',(-0.0119578233143749,0.987363722032868,0.158018640909809));
#83699=DIRECTION('ref_axis',(0.996580425785282,0.0246892569760022,-0.0788536335979417));
#83700=DIRECTION('',(-0.72506267162346,0.,0.688682889447858));
#83701=DIRECTION('center_axis',(1.4795260760968E-14,-1.,-1.22492840130852E-15));
#83702=DIRECTION('ref_axis',(1.,1.4795260760968E-14,-9.44775112401041E-33));
#83703=DIRECTION('center_axis',(-0.00461114502435709,-0.987363722359484,
0.158403336801938));
#83704=DIRECTION('ref_axis',(0.999964990721314,-0.00565888236509894,-0.00616395831436079));
#83705=DIRECTION('center_axis',(-0.011957803590877,-0.987363722219323,-0.158018641237308));
#83706=DIRECTION('ref_axis',(0.996599135032951,0.00111690409048127,-0.0823948819819873));
#83707=DIRECTION('center_axis',(-0.0192786475907753,0.987363720691356,-0.157293409936951));
#83708=DIRECTION('ref_axis',(0.996467281998849,0.00611303320384331,-0.0837590993915001));
#83709=DIRECTION('',(0.82844890631414,0.,0.560064647721052));
#83710=DIRECTION('center_axis',(0.0222910820964577,0.987363722053383,0.156894831118995));
#83711=DIRECTION('ref_axis',(0.956329728706116,0.0246892557043555,-0.291245413089463));
#83712=DIRECTION('',(-0.560064645188563,0.,0.828448908026203));
#83713=DIRECTION('center_axis',(-5.67441295577895E-14,-1.,1.75073359026152E-14));
#83714=DIRECTION('ref_axis',(1.,-5.67441295577895E-14,3.268951088727E-31));
#83715=DIRECTION('center_axis',(0.0295486907568079,-0.987363722291013,0.155691216124079));
#83716=DIRECTION('ref_axis',(0.975261296101418,-0.00565888786648576,-0.220982762483178));
#83717=DIRECTION('center_axis',(-0.0456475712957085,-0.987363722194644,
-0.151753679786494));
#83718=DIRECTION('ref_axis',(0.955586737475137,0.00111690638869429,-0.294707888733477));
#83719=DIRECTION('center_axis',(-0.05264135563157,0.987363720687697,-0.149471638604182));
#83720=DIRECTION('ref_axis',(0.955164700011649,0.00611303150036867,-0.296011869183537));
#83721=DIRECTION('',(0.929477575511641,0.,0.368878620444452));
#83722=DIRECTION('center_axis',(0.0554976773333573,0.987363721989729,0.148434794806314));
#83723=DIRECTION('ref_axis',(0.871362116748079,0.02468925852975,-0.49001887923789));
#83724=DIRECTION('',(-0.368878619816821,0.,0.929477575760727));
#83725=DIRECTION('center_axis',(-1.29134809254887E-14,-1.,7.3240836658601E-15));
#83726=DIRECTION('ref_axis',(1.,-1.29134809254887E-14,1.36982976880086E-31));
#83727=DIRECTION('center_axis',(0.0623268698928645,-0.987363722309312,0.14569914604025));
#83728=DIRECTION('ref_axis',(0.904955466281401,-0.00565888615062404,-0.425468660485055));
#83729=DIRECTION('center_axis',(-0.0772029158270658,-0.987363722218414,
-0.138392882168117));
#83730=DIRECTION('ref_axis',(0.869892165667375,0.00111690173774196,-0.493240684292194));
#83731=DIRECTION('center_axis',(-0.0835426144518167,0.987363720671955,-0.134660739161004));
#83732=DIRECTION('ref_axis',(0.869199678216931,0.00611303202809246,-0.494423452343238));
#83733=DIRECTION('',(0.9870449056352,0.,0.16044424034411));
#83734=DIRECTION('center_axis',(0.0861092673242092,0.987363722029707,0.133034110289549));
#83735=DIRECTION('ref_axis',(0.745650580592605,0.0246892563347975,-0.665879607949925));
#83736=DIRECTION('',(-0.160444237331189,0.,0.987044906124951));
#83737=DIRECTION('center_axis',(-6.62226565463095E-14,-1.,5.95732040164543E-14));
#83738=DIRECTION('ref_axis',(1.,-6.62226565463095E-14,8.3663892018305E-31));
#83739=DIRECTION('center_axis',(0.0921907116689665,-0.987363722300279,0.12889434652966));
#83740=DIRECTION('ref_axis',(0.792334927588738,-0.00565888580197279,-0.610060111410695));
#83741=DIRECTION('center_axis',(-0.105148331973004,-0.987363722223273,-0.118560989877356));
#83742=DIRECTION('ref_axis',(0.743522402554116,0.00111690374376028,-0.668710093707417));
#83743=DIRECTION('center_axis',(-0.110537512083763,0.987363720682677,-0.113553254035247));
#83744=DIRECTION('ref_axis',(0.742591847367116,0.00611303133035507,-0.669716342246363));
#83745=DIRECTION('',(0.998459113111179,0.,-0.0554923368154404));
#83746=DIRECTION('center_axis',(0.112694478378786,0.987363721955025,0.11141290369636));
#83747=DIRECTION('ref_axis',(0.585073252754729,0.0246892615105305,-0.810604545556627));
#83748=DIRECTION('',(0.05549233749058,0.,0.998459113073656));
#83749=DIRECTION('center_axis',(5.18679296940795E-14,-1.,-7.2416329169589E-14));
#83750=DIRECTION('ref_axis',(-1.06516527527658E-30,7.2416329169589E-14,
-1.));
#83751=DIRECTION('center_axis',(0.117743820074337,-0.987363722324764,0.106062588462134));
#83752=DIRECTION('ref_axis',(0.642665685848445,-0.00565888336345777,-0.766125833836731));
#83753=DIRECTION('center_axis',(-0.128177131859556,-0.987363722255328,-0.0931853145209106));
#83754=DIRECTION('ref_axis',(0.58238635873767,0.00111690127847762,-0.8129113615197));
#83755=DIRECTION('center_axis',(-0.132363799105279,0.987363720680554,-0.0871361450275937));
#83756=DIRECTION('ref_axis',(0.581261245462771,0.00611303055727861,-0.813694042856696));
#83757=DIRECTION('',(0.96318648209878,0.,-0.268834150922416));
#83758=DIRECTION('center_axis',(0.134010225449165,0.987363721917216,0.0845821501077273));
#83759=DIRECTION('ref_axis',(0.397138547751906,0.0246892614356591,-0.917426517089662));
#83760=DIRECTION('',(0.268834151573656,0.,0.963186481917013));
#83761=DIRECTION('center_axis',(2.92399301853973E-14,-1.,-6.82277895542969E-14));
#83762=DIRECTION('ref_axis',(1.3646765082506E-31,6.82277895542969E-14,-1.));
#83763=DIRECTION('center_axis',(0.13779135489011,-0.987363722256491,0.0782714666360208));
#83764=DIRECTION('ref_axis',(0.462946110105927,-0.00565888732432013,-0.886368363679595));
#83765=DIRECTION('center_axis',(-0.145212510191132,-0.987363722233906,-0.0634523986969547));
#83766=DIRECTION('ref_axis',(0.394018574864488,0.00111690088530794,-0.919101798058393));
#83767=DIRECTION('center_axis',(-0.148000903291999,0.987363720676903,-0.0566446441935525));
#83768=DIRECTION('ref_axis',(0.39275151165799,0.00611303235841334,-0.919624315101416));
#83769=DIRECTION('',(0.882876321704911,0.,-0.469605579793092));
#83770=DIRECTION('center_axis',(0.149059803058461,0.987363721938806,0.0537964284253243));
#83771=DIRECTION('ref_axis',(0.190634087994129,0.0246892603839579,-0.981350643203712));
#83772=DIRECTION('',(0.469605582630874,0.,0.882876320195483));
#83773=DIRECTION('center_axis',(-2.77787178218631E-15,-1.,1.4583676481692E-14));
#83774=DIRECTION('ref_axis',(-3.33324710125482E-32,-1.4583676481692E-14,
-1.));
#83775=DIRECTION('center_axis',(0.15139592084631,-0.987363722236557,0.0468204566644608));
#83776=DIRECTION('ref_axis',(0.261579691361806,-0.00565888879861934,-0.965165292602582));
#83777=DIRECTION('center_axis',(-0.155457912814124,-0.987363722264939,-0.0307525169473966));
#83778=DIRECTION('ref_axis',(0.187226921022217,0.00111689821087627,-0.982316055342132));
#83779=DIRECTION('center_axis',(-0.156717647683712,0.987363720680356,-0.0235045099656937));
#83780=DIRECTION('ref_axis',(0.185877157397317,0.00611302709239814,-0.982553974729969));
#83781=DIRECTION('',(0.761283846234037,0.,-0.648418773219215));
#83782=DIRECTION('',(0.648418775400083,0.,0.761283844376496));
#83783=DIRECTION('',(0.604094581901541,0.,-0.796912627655757));
#83784=DIRECTION('center_axis',(0.15787154625285,0.987363722058788,-0.013764274261669));
#83785=DIRECTION('ref_axis',(-0.239043629497269,0.0246892569315091,-0.970694897374526));
#83786=DIRECTION('',(0.796912626680266,0.,0.604094583188394));
#83787=DIRECTION('center_axis',(-1.44095946369905E-14,-1.,-5.76087374528612E-14));
#83788=DIRECTION('ref_axis',(2.29372654111249E-31,5.76087374528612E-14,
-1.));
#83789=DIRECTION('center_axis',(0.157062614897765,-0.987363722320007,-0.0210764050031671));
#83790=DIRECTION('ref_axis',(-0.16785909061338,-0.00565888540722353,-0.98579475689131));
#83791=DIRECTION('center_axis',(-0.154002427753442,-0.987363722237362,0.0373648532129905));
#83792=DIRECTION('ref_axis',(-0.242541254906398,0.00111690004499825,-0.970140449730202));
#83793=DIRECTION('center_axis',(-0.152102370896309,0.987363720676094,0.0444719221574905));
#83794=DIRECTION('ref_axis',(-0.243866167031853,0.00611303266598791,-0.969789628429185));
#83795=DIRECTION('',(0.418658529089389,0.,-0.908143730926283));
#83796=DIRECTION('center_axis',(0.151221685386099,0.987363722050727,-0.0473801883398824));
#83797=DIRECTION('ref_axis',(-0.442125629794732,0.024689257286697,-0.896613276754947));
#83798=DIRECTION('',(0.90814373120936,0.,0.418658528475346));
#83799=DIRECTION('center_axis',(-3.96853229838742E-14,-1.,-7.97463604750937E-14));
#83800=DIRECTION('ref_axis',(2.74015092108731E-31,7.97463604750937E-14,
-1.));
#83801=DIRECTION('center_axis',(0.148859772414883,-0.987363722370017,-0.0543474737610927));
#83802=DIRECTION('ref_axis',(-0.375851371087144,-0.00565888102545851,-0.926662680762236));
#83803=DIRECTION('center_axis',(-0.14236959780652,-0.987363722223227,0.0695972532353474));
#83804=DIRECTION('ref_axis',(-0.445422293864881,0.0011169001223638,-0.895319905208336));
#83805=DIRECTION('center_axis',(-0.138986155548796,0.987363720659471,0.0761297030813302));
#83806=DIRECTION('ref_axis',(-0.446640814676025,0.00611302818007946,-0.894692468701959));
#83807=DIRECTION('',(0.213646469431561,0.,-0.97691104308398));
#83808=DIRECTION('center_axis',(0.137500865192042,0.987363722076415,-0.078780660055933));
#83809=DIRECTION('ref_axis',(-0.624534330014507,0.0246892551508924,-0.780607014645286));
#83810=DIRECTION('',(0.976911043828262,0.,0.213646466028285));
#83811=DIRECTION('center_axis',(-6.52173811143766E-14,-1.,-8.09092240879132E-14));
#83812=DIRECTION('ref_axis',(8.66477572707589E-31,8.09092240879132E-14,
-1.));
#83813=DIRECTION('center_axis',(0.133696415542447,-0.987363722324532,-0.085077307835553));
#83814=DIRECTION('ref_axis',(-0.566269257745158,-0.00565888451119376,-0.824200888593817));
#83815=DIRECTION('center_axis',(-0.124079726700196,-0.987363722202752,0.0985753594968428));
#83816=DIRECTION('ref_axis',(-0.627475881044624,0.00111690481182892,-0.778635197785789));
#83817=DIRECTION('center_axis',(-0.119371098919121,0.987363720680323,0.104227749794143));
#83818=DIRECTION('ref_axis',(-0.628531034292203,0.00611303077633138,-0.777760483559239));
#83819=DIRECTION('',(-0.00135546408935191,0.,-0.999999081358129));
#83820=DIRECTION('center_axis',(0.117350660482125,0.98736372201723,-0.106497431559126));
#83821=DIRECTION('ref_axis',(-0.777740498287201,0.0246892582809723,-0.62810043611632));
#83822=DIRECTION('',(0.999999081357214,0.,-0.00135546476457403));
#83823=DIRECTION('center_axis',(1.15836752250586E-14,-1.,9.2854003310176E-15));
#83824=DIRECTION('ref_axis',(1.,1.15836752250587E-14,-1.75048848759714E-31));
#83825=DIRECTION('center_axis',(0.112281561555748,-0.987363722320076,-0.11182902476927));
#83826=DIRECTION('ref_axis',(-0.730209026605619,-0.00565888518529751,-0.683200376523707));
#83827=DIRECTION('center_axis',(-0.0999880263435284,-0.987363722188348,
0.122944193414313));
#83828=DIRECTION('ref_axis',(-0.780189394960913,0.00111690884324557,-0.625542373069291));
#83829=DIRECTION('center_axis',(-0.0941743838306357,0.987363720670641,0.127452220590891));
#83830=DIRECTION('ref_axis',(-0.781031841493226,0.00611303067508159,-0.624461282570558));
#83831=DIRECTION('',(-0.216294019096128,0.,-0.976328273329849));
#83832=DIRECTION('center_axis',(0.0917132677724629,0.987363722001367,-0.129234503868373));
#83833=DIRECTION('ref_axis',(-0.894580384647363,0.0246892584665362,-0.446224580139361));
#83834=DIRECTION('',(0.976328273183796,0.,-0.216294019755396));
#83835=DIRECTION('center_axis',(-3.99268257941694E-14,-1.,-1.97344952052439E-14));
#83836=DIRECTION('ref_axis',(1.,-3.99268257941694E-14,-5.56233456522579E-31));
#83837=DIRECTION('center_axis',(0.0856165443422947,-0.987363722331818,-0.133351742238116));
#83838=DIRECTION('ref_axis',(-0.860005031066307,-0.0056588828079528,-0.510254175471408));
#83839=DIRECTION('center_axis',(-0.0712209911176648,-0.987363722215966,
0.141564298027612));
#83840=DIRECTION('ref_axis',(-0.89642212049867,0.00111690538718566,-0.443199880869823));
#83841=DIRECTION('center_axis',(-0.0645741780897509,0.987363720681666,0.144717167625991));
#83842=DIRECTION('ref_axis',(-0.897012468634678,0.00611303148819058,-0.441962964466419));
#83843=DIRECTION('',(-0.421118902314207,0.,-0.907005441060679));
#83844=DIRECTION('center_axis',(0.0617874672746259,0.98736372193773,-0.145928713723719));
#83845=DIRECTION('ref_axis',(-0.969590686425388,0.024689261332682,-0.243483759565174));
#83846=DIRECTION('',(0.907005440776321,0.,-0.421118902926657));
#83847=DIRECTION('center_axis',(-5.76475892601268E-14,-1.,-1.42533684862447E-14));
#83848=DIRECTION('ref_axis',(1.,-5.76475892601268E-14,4.35334671275454E-32));
#83849=DIRECTION('center_axis',(0.054948198358191,-0.987363722272578,-0.148639077759611));
#83850=DIRECTION('ref_axis',(-0.949588155632919,-0.00565888675938369,-0.313449057555315));
#83851=DIRECTION('center_axis',(-0.0391237430721977,-0.987363722200919,
0.153565011671174));
#83852=DIRECTION('ref_axis',(-0.970739142604666,0.00111690367333193,-0.240133857548958));
#83853=DIRECTION('center_axis',(-0.0319545557613576,0.987363720672074,0.155215300362732));
#83854=DIRECTION('ref_axis',(-0.971049788381102,0.00611303238509471,-0.238798951672898));
#83855=DIRECTION('',(-0.60625273534136,0.,-0.795272042065556));
#83856=DIRECTION('center_axis',(0.0289725463399352,0.987363722037242,-0.155799460728673));
#83857=DIRECTION('ref_axis',(-0.999264006069101,0.0246892567636708,-0.0293579082222947));
#83858=DIRECTION('',(0.795272041985617,0.,-0.606252735446222));
#83859=DIRECTION('center_axis',(0.00215939850788328,0.987363721656155,0.158455729323336));
#83860=DIRECTION('ref_axis',(-0.999681899289745,0.00611320332131533,-0.0244689390370909));
#83861=DIRECTION('',(-0.763038865448691,0.,-0.64635260486423));
#83862=DIRECTION('center_axis',(-1.48409683524321E-14,-1.,-3.8190125160023E-16));
#83863=DIRECTION('ref_axis',(-0.999669073108583,1.48458812538651E-14,-0.0257243905705709));
#83864=DIRECTION('center_axis',(0.0217105298845489,-0.987363722321747,-0.15697621710016));
#83865=DIRECTION('ref_axis',(-0.994769594219394,-0.00565888470389273,-0.101987408244792));
#83866=DIRECTION('center_axis',(-0.00519733342331163,-0.98736372042386,
0.158385199169749));
#83867=DIRECTION('ref_axis',(-0.999665480855963,0.00111712080139465,-0.0258394741845179));
#83868=DIRECTION('',(0.64635260602278,0.,-0.763038864467309));
#83869=DIRECTION('center_axis',(-0.00519709416112407,0.987363722020954,
-0.158385197064655));
#83870=DIRECTION('ref_axis',(-0.982212851051216,0.0246892572281748,0.186140688210189));
#83871=DIRECTION('center_axis',(4.3728276777336E-14,-1.,-8.45219067440875E-15));
#83872=DIRECTION('ref_axis',(1.,4.3728276777336E-14,1.11950809907711E-31));
#83873=DIRECTION('center_axis',(0.0361720401591797,0.987363720696401,0.154286961741046));
#83874=DIRECTION('ref_axis',(-0.981569996660989,0.00611302890590471,0.191005163627955));
#83875=DIRECTION('center_axis',(-0.0125422941873798,-0.987363722266098,
-0.157973323093972));
#83876=DIRECTION('ref_axis',(-0.993436711795227,-0.00565888753205764,0.114243059523927));
#83877=DIRECTION('center_axis',(0.0289725258699401,-0.987363722235349,0.155799463279798));
#83878=DIRECTION('ref_axis',(-0.981848574517903,0.00111690498030995,0.189663199489062));
#83879=DIRECTION('',(-0.88414614515408,0.,-0.467210438677456));
#83880=DIRECTION('center_axis',(-0.0391237251010263,0.987363722063321,-0.153565017134384));
#83881=DIRECTION('ref_axis',(-0.919234514576966,0.0246892565919667,0.392935551737669));
#83882=DIRECTION('',(0.467210440327718,8.7272790084625E-15,-0.88414614428203));
#83883=DIRECTION('center_axis',(9.54075798536309E-14,-1.,-4.1194696781827E-14));
#83884=DIRECTION('ref_axis',(1.,9.54075798536309E-14,-9.10948663397066E-32));
#83885=DIRECTION('center_axis',(-0.0462086638903957,-0.987363722387185,
-0.151583769233998));
#83886=DIRECTION('ref_axis',(-0.945651833071557,-0.0056588799705953,0.325131646700044));
#83887=DIRECTION('center_axis',(0.0617874445083887,-0.987363722220602,0.145928721449209));
#83888=DIRECTION('ref_axis',(-0.918121518951185,0.00111690394803397,0.396297399643676));
#83889=DIRECTION('center_axis',(0.0684934889757973,0.987363720684482,0.142903901430361));
#83890=DIRECTION('ref_axis',(-0.917560972092285,0.00611302340973764,0.397548102042825));
#83891=DIRECTION('',(-0.963911732980681,0.,-0.266222033314638));
#83892=DIRECTION('center_axis',(-0.0712209764537815,0.987363722108156,-0.141564306156951));
#83893=DIRECTION('ref_axis',(-0.813273794121335,0.0246892530481944,0.581357185024329));
#83894=DIRECTION('',(0.266222032663698,0.,-0.963911733160464));
#83895=DIRECTION('center_axis',(2.40918175844038E-14,-1.,-1.73546848866497E-14));
#83896=DIRECTION('ref_axis',(1.,2.40918175844038E-14,-3.61649621631541E-31));
#83897=DIRECTION('center_axis',(-0.077714359735654,-0.987363722361458,-0.138106328802857));
#83898=DIRECTION('ref_axis',(-0.853649325806049,-0.00565888098702445,0.520817439816345));
#83899=DIRECTION('center_axis',(0.0917132479690571,-0.987363722209593,0.129234516331292));
#83900=DIRECTION('ref_axis',(-0.811464122170743,0.00111690621270039,0.584401172954143));
#83901=DIRECTION('center_axis',(0.0976122690732956,0.98736372069769,0.12483880797403));
#83902=DIRECTION('ref_axis',(-0.810647814349427,0.00611302973016654,0.585502136595602));
#83903=DIRECTION('',(-0.998605879960763,-8.72727900573397E-15,-0.0527853815728483));
#83904=DIRECTION('center_axis',(-0.0999880081949315,0.987363722034604,-0.122944209408914));
#83905=DIRECTION('ref_axis',(-0.669285294789748,0.024689256854248,0.742595202498768));
#83906=DIRECTION('',(0.0527853810498718,0.,-0.998605879988407));
#83907=DIRECTION('center_axis',(-8.90901902559685E-14,-1.,9.95758679737192E-14));
#83908=DIRECTION('ref_axis',(-2.44147446982783E-31,-9.95758679737192E-14,
-1.));
#83909=DIRECTION('center_axis',(-0.10558621563704,-0.98736372229164,-0.118171193485749));
#83910=DIRECTION('ref_axis',(-0.721731125798102,-0.00565888635371337,0.69215038760333));
#83911=DIRECTION('center_axis',(0.117350645962308,-0.987363722220967,0.106497445669769));
#83912=DIRECTION('ref_axis',(-0.666863563286744,0.00111690353864807,0.745178998957292));
#83913=DIRECTION('center_axis',(0.122166802887998,0.987363720666353,0.100936392763069));
#83914=DIRECTION('ref_axis',(-0.665829667603348,0.0061130311092627,0.746078738867335));
#83915=DIRECTION('',(-0.986606326510258,0.,0.163119454664165));
#83916=DIRECTION('center_axis',(-0.124079715094384,0.987363722052136,-0.0985753756140405));
#83917=DIRECTION('ref_axis',(-0.494001758384005,0.0246892565635383,0.86911029410763));
#83918=DIRECTION('',(-0.16311945579303,0.,-0.986606326323618));
#83919=DIRECTION('center_axis',(-7.28904920849601E-14,-1.,1.29332885349243E-13));
#83920=DIRECTION('ref_axis',(1.43316139478469E-30,-1.29332885349243E-13,
-1.));
#83921=DIRECTION('center_axis',(-0.128520983646098,-0.987363722346133,-0.0927104986364962));
#83922=DIRECTION('ref_axis',(-0.556065577731079,-0.00565888351541373,0.831119155296014));
#83923=DIRECTION('center_axis',(0.13750085681627,-0.987363722241842,0.0787806726013888));
#83924=DIRECTION('ref_axis',(-0.4910812059078,0.00111690141433312,0.871113082059598));
#83925=DIRECTION('center_axis',(0.141008950102571,0.987363720689102,0.0723143074221373));
#83926=DIRECTION('ref_axis',(-0.489878064606547,0.00611302773077556,0.871769529582966));
#83927=DIRECTION('',(-0.928474157301363,0.,0.371397010251191));
#83928=DIRECTION('center_axis',(-0.142369592250741,0.98736372201826,-0.0695972675081812));
#83929=DIRECTION('ref_axis',(-0.295619249946772,0.024689256796667,0.954986753656686));
#83930=DIRECTION('',(-0.371397010878169,0.,-0.928474157050567));
#83931=DIRECTION('center_axis',(-1.73534422570156E-14,-1.,5.67913822896903E-14));
#83932=DIRECTION('ref_axis',(-1.40571721593363E-31,-5.67913822896903E-14,
-1.));
#83933=DIRECTION('center_axis',(-0.145446250028888,-0.987363722268766,-0.0629147701267425));
#83934=DIRECTION('ref_axis',(-0.364399023979489,-0.0056588873821436,0.931225712873303));
#83935=DIRECTION('center_axis',(0.151221679661245,-0.987363722237896,0.0473802027112372));
#83936=DIRECTION('ref_axis',(-0.292336437731566,0.00111689942938177,0.956314885228753));
#83937=DIRECTION('center_axis',(0.153257678612783,0.98736372068058,0.0403108797971802));
#83938=DIRECTION('ref_axis',(-0.291020309763654,0.00611303139448231,0.956697345116122));
#83939=DIRECTION('',(-0.826927567205339,0.,0.562308455027896));
#83940=DIRECTION('center_axis',(-0.154002425329325,0.987363721965411,-0.0373648703904596));
#83941=DIRECTION('ref_axis',(-0.083413912942098,0.0246892591347644,0.996209094322605));
#83942=DIRECTION('',(-0.562308454249525,-8.72727898606521E-15,-0.826927567734629));
#83943=DIRECTION('center_axis',(-7.1088899461577E-15,-1.,8.87911626056644E-14));
#83944=DIRECTION('ref_axis',(1.8966066488671E-31,-8.87911626056644E-14,
-1.));
#83945=DIRECTION('center_axis',(-0.155570614161056,-0.987363722323422,-0.0301772074451632));
#83946=DIRECTION('ref_axis',(-0.155693573555354,-0.00565888170651582,0.987789192192036));
#83947=DIRECTION('center_axis',(0.157871543355574,-0.987363722242727,0.0137642942978041));
#83948=DIRECTION('ref_axis',(-0.0799223410303271,0.00111690518742693,0.996800467459278));
#83949=DIRECTION('center_axis',(0.15834024654227,0.987363720697898,0.00642256759684789));
#83950=DIRECTION('ref_axis',(-0.0785547654154159,0.00611302663392469,0.996891057104989));
#83951=DIRECTION('',(-0.686714765840337,0.,0.726926977334623));
#83952=DIRECTION('',(0.760873717902008,0.,-0.648899981049449));
#83953=DIRECTION('center_axis',(0.158420670951937,-0.987363721845357,0.00397137241051485));
#83954=DIRECTION('ref_axis',(-0.18204302254892,-0.0252547793770049,0.982966191717636));
#83955=DIRECTION('',(0.470163700157015,0.,0.882579228769103));
#83956=DIRECTION('center_axis',(1.66119026794183E-14,-1.,-8.75125797881804E-14));
#83957=DIRECTION('ref_axis',(5.50379459184303E-31,8.75125797881804E-14,
-1.));
#83958=DIRECTION('center_axis',(0.150470357297638,0.987363722706508,0.0497146925754033));
#83959=DIRECTION('ref_axis',(-0.116797137708958,-0.0321806451053153,0.992634290513682));
#83960=DIRECTION('center_axis',(-0.156018993570792,0.987363721745411,-0.027766069693188));
#83961=DIRECTION('ref_axis',(-0.186683316697925,-0.00187190037319769,0.982418360605936));
#83962=DIRECTION('',(0.882579228239459,0.,-0.470163701151249));
#83963=DIRECTION('center_axis',(0.153863155238695,-0.987363721900371,0.0379342870638276));
#83964=DIRECTION('ref_axis',(-0.389095632825037,-0.025254777427565,0.920851119743886));
#83965=DIRECTION('',(0.269443091726455,0.,0.963016313631752));
#83966=DIRECTION('center_axis',(2.33574289875519E-14,-1.,-5.45970109405145E-14));
#83967=DIRECTION('ref_axis',(-2.57995956160863E-31,5.45970109405145E-14,
-1.));
#83968=DIRECTION('center_axis',(0.136265253013163,0.987363722600581,0.0808990736262259));
#83969=DIRECTION('ref_axis',(-0.327453516387912,-0.0321806493677835,0.944319120007352));
#83970=DIRECTION('center_axis',(-0.146402464080743,0.987363721985126,-0.0606564013008222));
#83971=DIRECTION('ref_axis',(-0.393509674167322,-0.00187188349778186,0.919318569587768));
#83972=DIRECTION('',(0.963016313438966,0.,-0.269443092415491));
#83973=DIRECTION('center_axis',(0.142111166557216,-0.987363722011711,0.0701234396969183));
#83974=DIRECTION('ref_axis',(-0.577954565812851,-0.025254771821771,0.815678071518604));
#83975=DIRECTION('',(0.0561236183417539,0.,0.998423827572354));
#83976=DIRECTION('center_axis',(-5.18221330477079E-14,-1.,7.24491094435913E-14));
#83977=DIRECTION('ref_axis',(-2.76296851101971E-30,-7.24491094435913E-14,
-1.));
#83978=DIRECTION('center_axis',(0.115688539590078,0.987363722702905,0.108300696663393));
#83979=DIRECTION('ref_axis',(-0.52279853179565,-0.0321806458123467,0.851848637486387));
#83980=DIRECTION('center_axis',(-0.129940334586113,0.987363721716063,-0.0907104761681578));
#83981=DIRECTION('ref_axis',(-0.581935951137064,-0.00187190178823612,0.813232466615725));
#83982=DIRECTION('',(0.99842382757567,0.,-0.0561236182827579));
#83983=DIRECTION('center_axis',(0.123714223149916,-0.987363721940037,0.0990336891523768));
#83984=DIRECTION('ref_axis',(-0.739788982046662,-0.0252547764804811,0.672364825304897));
#83985=DIRECTION('',(-0.159820128826896,0.,0.987146152513271));
#83986=DIRECTION('center_axis',(4.41233181953626E-14,-1.,-3.97433751604223E-14));
#83987=DIRECTION('ref_axis',(1.,4.41233181953626E-14,-2.15831669479006E-30));
#83988=DIRECTION('center_axis',(0.0897023546228915,0.987363722634468,0.130638305257357));
#83989=DIRECTION('ref_axis',(-0.693698068926603,-0.0321806495628235,0.719546659335735));
#83990=DIRECTION('center_axis',(-0.107402316178315,0.987363721994519,-0.116523057669561));
#83991=DIRECTION('ref_axis',(-0.743151555138497,-0.00187188370506456,0.669120513918553));
#83992=DIRECTION('',(0.987146152503824,0.,0.159820128885249));
#83993=DIRECTION('center_axis',(0.0995325402727104,-0.987363721842449,0.123313236176365));
#83994=DIRECTION('ref_axis',(-0.867031688858854,-0.0252547794111912,0.497612546698187));
#83995=DIRECTION('',(-0.368290866546792,0.,0.929710620364322));
#83996=DIRECTION('center_axis',(-7.74530857502545E-14,-1.,4.39934820937403E-14));
#83997=DIRECTION('ref_axis',(1.,-7.74530857502545E-14,-1.3738948908618E-30));
#83998=DIRECTION('center_axis',(0.0595217899121446,0.987363722621448,0.146867408831129));
#83999=DIRECTION('ref_axis',(-0.832161056395907,-0.0321806488996472,0.553599478011356));
#84000=DIRECTION('center_axis',(-0.0798422942999397,0.987363721988568,-0.13688713797068));
#84001=DIRECTION('ref_axis',(-0.86961821732428,-0.00187188122784259,0.493721229195595));
#84002=DIRECTION('',(0.929710620732484,0.,0.368290865617407));
#84003=DIRECTION('center_axis',(0.0706968232391802,-0.987363721882445,0.141826795403174));
#84004=DIRECTION('ref_axis',(-0.953732957852313,-0.0252547784065486,0.299592458639924));
#84005=DIRECTION('',(-0.559540732515555,0.,0.828802852707419));
#84006=DIRECTION('center_axis',(8.50995737247474E-14,-1.,-2.63148149472303E-14));
#84007=DIRECTION('ref_axis',(1.,8.50995737247474E-14,-4.61162654382223E-31));
#84008=DIRECTION('center_axis',(0.0265580544804943,0.987363722702226,0.15622915487774));
#84009=DIRECTION('ref_axis',(-0.931713116916154,-0.032180646225258,0.361766601242998));
#84010=DIRECTION('center_axis',(-0.0485489594157441,0.987363721707236,-0.150850520702069));
#84011=DIRECTION('ref_axis',(-0.955422495320087,-0.00187190327627904,0.295236094362568));
#84012=DIRECTION('',(0.828802852674343,0.,0.559540732564549));
#84013=DIRECTION('center_axis',(0.0385554032256785,-0.987363721881548,0.153708690692241));
#84014=DIRECTION('ref_axis',(-0.995838733942716,-0.0252547794232253,0.0875637601731004));
#84015=DIRECTION('',(-0.724627094472956,0.,0.689141185792637));
#84016=DIRECTION('center_axis',(0.,-1.,0.));
#84017=DIRECTION('ref_axis',(0.,0.,-1.));
#84018=DIRECTION('center_axis',(-0.00764751234414346,0.987363722585381,
0.158285801249784));
#84019=DIRECTION('ref_axis',(-0.987699307272752,-0.0321806505023496,0.15301792099676));
#84020=DIRECTION('center_axis',(-0.014985482612071,0.987363722043209,-0.157760310927254));
#84021=DIRECTION('ref_axis',(-0.996552281853689,-0.00187187734051423,0.0829460403360414));
#84022=DIRECTION('',(0.689141185749805,0.,0.724627094513691));
#84023=DIRECTION('center_axis',(0.00461117065540764,-0.98736372194356,0.15840333864836));
#84024=DIRECTION('ref_axis',(-0.991380197761653,-0.0252547757806465,-0.128559323996106));
#84025=DIRECTION('',(-0.855830699792882,0.,0.517256042296294));
#84026=DIRECTION('center_axis',(5.88557235901373E-14,-1.,7.89980289289736E-15));
#84027=DIRECTION('ref_axis',(1.,5.88557235901373E-14,7.28864359769959E-32));
#84028=DIRECTION('center_axis',(-0.041495480880162,0.987363722713628,0.152941178678636));
#84029=DIRECTION('ref_axis',(-0.997501776374992,-0.0321806452263054,-0.0628857074505336));
#84030=DIRECTION('center_axis',(0.0192786467163599,0.987363721692677,-0.157293403758615));
#84031=DIRECTION('ref_axis',(-0.991084390577787,-0.00187190395811225,-0.133222470809653));
#84032=DIRECTION('',(0.51725604351836,0.,0.855830699054277));
#84033=DIRECTION('center_axis',(-0.0295486717052587,-0.987363721972233,
0.15569122176152));
#84034=DIRECTION('ref_axis',(-0.940565825156794,-0.0252547754165295,-0.338671116078387));
#84035=DIRECTION('',(-0.947016612388295,0.,0.321184582227414));
#84036=DIRECTION('center_axis',(1.11562970629401E-13,-1.,4.07347013544332E-14));
#84037=DIRECTION('ref_axis',(1.,1.11562970629401E-13,1.53052459812118E-30));
#84038=DIRECTION('center_axis',(-0.0734031763791204,0.987363722626315,0.14044519549974));
#84039=DIRECTION('ref_axis',(-0.960662170736016,-0.0321806497949105,-0.275848870752705));
#84040=DIRECTION('center_axis',(0.0526413731130204,0.987363721985208,-0.149471623876552));
#84041=DIRECTION('ref_axis',(-0.939274493787547,-0.00187188437303119,-0.343161654864061));
#84042=DIRECTION('',(0.321184582171429,0.,0.947016612407282));
#84043=DIRECTION('center_axis',(-0.0623268523181122,-0.987363721967415,
0.145699155875284));
#84044=DIRECTION('ref_axis',(-0.845771638811263,-0.0252547739760518,-0.532947024922674));
#84045=DIRECTION('',(-0.993921081291667,0.,0.110094887092924));
#84046=DIRECTION('center_axis',(7.51484503470179E-14,-1.,4.78238157380566E-14));
#84047=DIRECTION('ref_axis',(1.,7.51484503470179E-14,1.09517870617567E-30));
#84048=DIRECTION('center_axis',(-0.101878612836726,0.987363722718883,0.121382153981436));
#84049=DIRECTION('ref_axis',(-0.878903069713223,-0.0321806454471711,-0.47591364774219));
#84050=DIRECTION('center_axis',(0.0835426327950051,0.9873637220322,-0.13466071780738));
#84051=DIRECTION('ref_axis',(-0.843545165481614,-0.0018718784691315,-0.537054978436652));
#84052=DIRECTION('',(0.110094884194222,0.,0.993921081612751));
#84053=DIRECTION('center_axis',(-0.0921906923225379,-0.987363721856517,
0.12889436376637));
#84054=DIRECTION('ref_axis',(-0.711430113097762,-0.0252547796932717,-0.70230291917402));
#84055=DIRECTION('',(-0.994350904942001,0.,-0.106142723919367));
#84056=DIRECTION('center_axis',(0.,-1.,0.));
#84057=DIRECTION('ref_axis',(0.,0.,-1.));
#84058=DIRECTION('center_axis',(-0.125590323972974,0.987363722658854,0.0966434152004877));
#84059=DIRECTION('ref_axis',(-0.756047438066,-0.0321806473676782,-0.653725230757415));
#84060=DIRECTION('center_axis',(0.110537521524331,0.98736372195806,-0.113553233755737));
#84061=DIRECTION('ref_axis',(-0.708372604320887,-0.0018718853427728,-0.705836205852964));
#84062=DIRECTION('',(-0.106142721135687,0.,0.994350905239147));
#84063=DIRECTION('center_axis',(-0.117743802252636,-0.987363721835322,0.106062612802972));
#84064=DIRECTION('ref_axis',(-0.543822905209596,-0.0252547813062237,-0.838819911417564));
#84065=DIRECTION('',(-0.948285986047789,0.,-0.317417215452112));
#84066=DIRECTION('center_axis',(-4.81221873529243E-14,-1.,-7.49577349565336E-14));
#84067=DIRECTION('ref_axis',(8.50838497286474E-31,7.49577349565336E-14,
-1.));
#84068=DIRECTION('center_axis',(-0.143429568776544,0.987363722694744,0.0673857396408982));
#84069=DIRECTION('ref_axis',(-0.597839867781445,-0.0321806459674356,-0.800969349298825));
#84070=DIRECTION('center_axis',(0.132363804610462,0.987363721967653,-0.0871361220804899));
#84071=DIRECTION('ref_axis',(-0.54007732666416,-0.00187188474904035,-0.841613318140095));
#84072=DIRECTION('',(-0.317417216373473,0.,0.948285985739384));
#84073=DIRECTION('center_axis',(-0.13779134681076,-0.987363721977672,0.0782714843763365));
#84074=DIRECTION('ref_axis',(-0.350787141703557,-0.0252547743292595,-0.936114617762711));
#84075=DIRECTION('',(-0.857880267877045,0.,-0.513849633635376));
#84076=DIRECTION('center_axis',(-3.08834200477059E-14,-1.,-8.35501124920039E-14));
#84077=DIRECTION('ref_axis',(1.60869207676635E-30,8.35501124920039E-14,
-1.));
#84078=DIRECTION('center_axis',(-0.154562208249242,0.987363722638654,0.0349771782489369));
#84079=DIRECTION('ref_axis',(-0.411677971069692,-0.0321806490103536,-0.910761030109004));
#84080=DIRECTION('center_axis',(0.148000904439035,0.987363722001869,-0.0566446181013166));
#84081=DIRECTION('ref_axis',(-0.346528631681396,-0.00187188022074965,-0.938037527761794));
#84082=DIRECTION('',(-0.513849635801822,0.,0.857880266579396));
#84083=DIRECTION('center_axis',(-0.151395917147904,-0.987363721934246,0.0468204749986269));
#84084=DIRECTION('ref_axis',(-0.141348960074115,-0.0252547755188113,-0.989637644696007));
#84085=DIRECTION('',(-0.727361020504471,0.,-0.686255015173438));
#84086=DIRECTION('center_axis',(-1.22005783802258E-14,-1.,-8.82357797049569E-14));
#84087=DIRECTION('ref_axis',(-4.66197082555383E-32,8.82357797049569E-14,
-1.));
#84088=DIRECTION('center_axis',(-0.158467688440811,0.987363722742502,0.00093313037385869));
#84089=DIRECTION('ref_axis',(-0.206266469571198,-0.0321806438930113,-0.977966538123501));
#84090=DIRECTION('center_axis',(0.156717643448514,0.987363722017604,-0.0235044820297946));
#84091=DIRECTION('ref_axis',(-0.13677664582851,-0.00187188330714621,-0.990600143957584));
#84092=DIRECTION('',(-0.686255015216422,0.,0.727361020463916));
#84093=DIRECTION('center_axis',(-0.157921382952396,-0.987363721842888,0.0131801970760088));
#84094=DIRECTION('ref_axis',(0.0746985365481363,-0.0252547807219919,-0.996886314826446));
#84095=DIRECTION('',(-0.562831181859169,0.,-0.826571872692878));
#84096=DIRECTION('center_axis',(2.35091625679143E-15,-1.,-2.95985466508887E-14));
#84097=DIRECTION('ref_axis',(1.73983611715488E-32,2.95985466508887E-14,
-1.));
#84098=DIRECTION('center_axis',(-0.154963397163266,0.987363722655173,-0.0331545581200833));
#84099=DIRECTION('ref_axis',(0.00878982263912512,-0.0321806476884021,-0.999443417574165));
#84100=DIRECTION('center_axis',(0.158106440926136,0.987363722001472,0.0107347013498738));
#84101=DIRECTION('ref_axis',(0.0793708644578278,-0.00187188233847563,-0.996843398900614));
#84102=DIRECTION('',(-0.826571873636816,0.,0.562831180472905));
#84103=DIRECTION('center_axis',(-0.157062621681397,-0.987363721823588,-0.0210763777067678));
#84104=DIRECTION('ref_axis',(0.287253218042712,-0.0252547811743122,-0.957521688919861));
#84105=DIRECTION('',(-0.371983982078545,0.,-0.928239148644889));
#84106=DIRECTION('center_axis',(0.,-1.,0.));
#84107=DIRECTION('ref_axis',(0.,0.,-1.));
#84108=DIRECTION('center_axis',(-0.144213189672392,0.987363722716302,-0.0656919705011265));
#84109=DIRECTION('ref_axis',(0.223435111451264,-0.0321806456465352,-0.974187434232516));
#84110=DIRECTION('center_axis',(0.152102356220726,0.987363722015024,0.0444719426238749));
#84111=DIRECTION('ref_axis',(0.291807083291674,-0.00187188102446143,-0.956475364137643));
#84112=DIRECTION('',(-0.928239148269088,0.,0.37198398301631));
#84113=DIRECTION('center_axis',(-0.148859783533753,-0.987363721980219,-0.0543474503877802));
#84114=DIRECTION('ref_axis',(0.486376257462539,-0.0252547747120306,-0.87338441280514));
#84115=DIRECTION('',(-0.163743224263631,0.,-0.986502993663856));
#84116=DIRECTION('center_axis',(4.3685222893723E-14,-1.,-7.76273678386911E-14));
#84117=DIRECTION('ref_axis',(-1.1971649917518E-30,7.7627367838691E-14,-1.));
#84118=DIRECTION('center_axis',(-0.126719731067538,0.987363722569715,-0.0951577065268265));
#84119=DIRECTION('ref_axis',(0.42763282427826,-0.03218065124485,-0.903379528927491));
#84120=DIRECTION('center_axis',(0.138986134009488,0.987363722017502,0.0761297247915765));
#84121=DIRECTION('ref_axis',(0.490598724984633,-0.00187187968910189,-0.871383605027018));
#84122=DIRECTION('',(-0.986502993673533,0.,0.163743224205332));
#84123=DIRECTION('center_axis',(-0.133696433187651,-0.987363721844637,-0.0850772856760678));
#84124=DIRECTION('ref_axis',(0.662756881152128,-0.0252547807035617,-0.748408653435487));
#84125=DIRECTION('',(0.05215398216031,0.,-0.998639054986746));
#84126=DIRECTION('center_axis',(5.93514761815451E-14,-1.,-6.64214516128926E-14));
#84127=DIRECTION('ref_axis',(-2.33646575295403E-30,6.64214516128926E-14,
-1.));
#84128=DIRECTION('center_axis',(-0.103301005449085,0.987363722780521,-0.120173962280518));
#84129=DIRECTION('ref_axis',(0.61183490179735,-0.0321806428555542,-0.790330601184106));
#84130=DIRECTION('center_axis',(0.119371077060778,0.987363721991977,0.104227762402829));
#84131=DIRECTION('ref_axis',(0.666450517002388,-0.00187188279882516,-0.745546916325215));
#84132=DIRECTION('',(-0.998639054975845,0.,-0.0521539823690436));
#84133=DIRECTION('center_axis',(-0.112281580436837,-0.987363721918056,-0.111829009361297));
#84134=DIRECTION('ref_axis',(0.808147731523845,-0.0252547770532661,-0.588438136314136));
#84135=DIRECTION('',(0.265612528541422,0.,-0.964079864265317));
#84136=DIRECTION('center_axis',(-4.81616801158825E-14,-1.,3.47398279347916E-14));
#84137=DIRECTION('ref_axis',(1.,-4.81616801158825E-14,1.80701700499117E-30));
#84138=DIRECTION('center_axis',(-0.0750520328090775,0.987363722700972,-0.139571026596869));
#84139=DIRECTION('ref_axis',(0.767428259443635,-0.0321806464379674,-0.640326692089395));
#84140=DIRECTION('center_axis',(0.0941743565718948,0.987363722016492,0.127452230306137));
#84141=DIRECTION('ref_axis',(0.811139823184763,-0.00187187906711774,-0.584849282561371));
#84142=DIRECTION('',(-0.964079864249621,0.,-0.265612528598395));
#84143=DIRECTION('center_axis',(-0.0856165686441856,-0.987363721901408,
-0.133351729822281));
#84144=DIRECTION('ref_axis',(0.915750492197764,-0.0252547777773986,-0.400952905263157));
#84145=DIRECTION('',(0.466651329562723,0.,-0.884441369802059));
#84146=DIRECTION('center_axis',(-5.45037230112074E-14,-1.,2.35742925329346E-14));
#84147=DIRECTION('ref_axis',(1.,-5.45037230112074E-14,7.87519646691859E-31));
#84148=DIRECTION('center_axis',(-0.0432937091944434,0.987363722575924,-0.152441903967382));
#84149=DIRECTION('ref_axis',(0.887137525153124,-0.0321806502956287,-0.460381816769234));
#84150=DIRECTION('center_axis',(0.0645741461488577,0.987363722058241,0.144717172486346));
#84151=DIRECTION('ref_axis',(0.917901132754908,-0.00187187453050333,-0.396804746157349));
#84152=DIRECTION('',(-0.884441369774467,0.,-0.466651329615018));
#84153=DIRECTION('center_axis',(-0.0549482167247938,-0.987363721999776,
-0.14863907278207));
#84154=DIRECTION('ref_axis',(0.980533777242356,-0.0252547735855317,-0.194719562699746));
#84155=DIRECTION('',(0.645870029654509,0.,-0.763447381811009));
#84156=DIRECTION('center_axis',(-5.82972322439759E-14,-1.,1.1306449337716E-14));
#84157=DIRECTION('ref_axis',(1.,-5.82972322439759E-14,1.18982867353277E-31));
#84158=DIRECTION('center_axis',(-0.009511024359043,0.987363722641755,-0.158184764205208));
#84159=DIRECTION('ref_axis',(0.965365224232181,-0.0321806492226432,-0.258910003010234));
#84160=DIRECTION('center_axis',(0.0319545315579717,0.987363721993611,0.155215296938911));
#84161=DIRECTION('ref_axis',(0.981742405061269,-0.00187188183297512,-0.190206062371624));
#84162=DIRECTION('',(-0.7634473805736,0.,-0.645870031117181));
#84163=DIRECTION('',(0.794888567218867,0.,-0.606755441429854));
#84164=DIRECTION('',(-0.606755441382878,0.,-0.794888567254724));
#84165=DIRECTION('center_axis',(0.0125422740500174,-0.987363721949525,-0.157973326671421));
#84166=DIRECTION('ref_axis',(0.971668976639003,-0.0252547754455921,0.234992757663944));
#84167=DIRECTION('',(0.906738999989211,0.,-0.421692288165868));
#84168=DIRECTION('center_axis',(-2.88282949215819E-14,-1.,-7.10845848220289E-15));
#84169=DIRECTION('ref_axis',(1.,-2.88282949215819E-14,-2.26654765156684E-31));
#84170=DIRECTION('center_axis',(0.0577880837148793,0.987363722691916,-0.147558180025793));
#84171=DIRECTION('ref_axis',(0.98485523721207,-0.0321806462577187,0.170365981763946));
#84172=DIRECTION('center_axis',(-0.0361720451932298,0.987363721719128,0.15428695401586));
#84173=DIRECTION('ref_axis',(0.970870728505734,-0.00187190160635395,0.239596587027282));
#84174=DIRECTION('',(-0.421692289376655,0.,-0.906738999426117));
#84175=DIRECTION('center_axis',(0.0462086355117911,-0.987363721864621,-0.151583781288707));
#84176=DIRECTION('ref_axis',(0.89843539973103,-0.0252547783768751,0.438378864316335));
#84177=DIRECTION('',(0.976191322337168,0.,-0.216911277239362));
#84178=DIRECTION('center_axis',(7.98785909856274E-14,-1.,3.94184938248821E-14));
#84179=DIRECTION('ref_axis',(1.,7.98785909856274E-14,1.35351838227383E-30));
#84180=DIRECTION('center_axis',(0.0881576752423758,0.987363722731961,-0.131685623090541));
#84181=DIRECTION('ref_axis',(0.925206219006397,-0.0321806438492019,0.378097683771452));
#84182=DIRECTION('center_axis',(-0.0684935153894493,0.987363722021412,0.142903879533128));
#84183=DIRECTION('ref_axis',(0.896666124993326,-0.00187188095421391,0.442703463224704));
#84184=DIRECTION('',(-0.216911277181653,0.,-0.976191322349991));
#84185=DIRECTION('center_axis',(0.0777143366891166,-0.987363721914026,-0.138106344970288));
#84186=DIRECTION('ref_axis',(0.783191980717488,-0.0252547770838744,0.621266865021998));
#84187=DIRECTION('',(0.999998024453727,0.,-0.00198773455025544));
#84188=DIRECTION('center_axis',(-4.6358175241323E-14,-1.,-3.71122980948279E-14));
#84189=DIRECTION('ref_axis',(1.,-4.6358175241323E-14,6.22213030087365E-31));
#84190=DIRECTION('center_axis',(0.11440511685421,0.987363722685258,-0.10965558974664));
#84191=DIRECTION('ref_axis',(0.822295585228745,-0.0321806472280121,0.568149959480154));
#84192=DIRECTION('center_axis',(-0.0976122826722845,0.987363722002558,0.12483878702055));
#84193=DIRECTION('ref_axis',(0.780534411660532,-0.00187188378597566,0.625110012929596));
#84194=DIRECTION('',(-0.00198773449113936,0.,-0.999998024453845));
#84195=DIRECTION('center_axis',(0.105586197529413,-0.987363721824817,-0.118171213565425));
#84196=DIRECTION('ref_axis',(0.631327377166835,-0.0252547813377562,0.775105114716209));
#84197=DIRECTION('',(0.977045930400975,0.,0.213028753662255));
#84198=DIRECTION('center_axis',(5.59444497098018E-14,-1.,6.93154057869814E-14));
#84199=DIRECTION('ref_axis',(2.356099361098E-30,-6.93154057869814E-14,-1.));
#84200=DIRECTION('center_axis',(0.135303100940913,0.987363722605909,-0.0824981827531636));
#84201=DIRECTION('ref_axis',(0.680935325332856,-0.0321806500350066,0.731636172203891));
#84202=DIRECTION('center_axis',(-0.122166801575977,0.987363721726155,0.100936383984035));
#84203=DIRECTION('ref_axis',(0.627905778710353,-0.00187189998213551,0.778287112223119));
#84204=DIRECTION('',(0.213028754318377,0.,-0.977045930257918));
#84205=DIRECTION('center_axis',(0.128520970701227,-0.987363721876118,-0.0927105215871122));
#84206=DIRECTION('ref_axis',(0.449942604776546,-0.0252547776970041,0.89270031287682));
#84207=DIRECTION('',(0.908408255110064,0.,0.418084252331859));
#84208=DIRECTION('center_axis',(2.64904908668139E-14,-1.,5.31475021130798E-14));
#84209=DIRECTION('ref_axis',(-1.34265684866501E-30,-5.31475021130798E-14,
-1.));
#84210=DIRECTION('center_axis',(0.149874459411184,0.987363722638236,-0.051483255862173));
#84211=DIRECTION('ref_axis',(0.507735286740845,-0.0321806480468414,0.860911891246414));
#84212=DIRECTION('center_axis',(-0.141008954760601,0.987363721981079,0.072314280698864));
#84213=DIRECTION('ref_axis',(0.44591696457479,-0.00187188353848564,0.895072375149867));
#84214=DIRECTION('',(0.418084253477456,0.,-0.908408254582816));
#84215=DIRECTION('center_axis',(0.145446242924412,-0.987363721883228,-0.0629147926013606));
#84216=DIRECTION('ref_axis',(0.24751901900161,-0.0252547786965402,0.968553835047629));
#84217=DIRECTION('',(0.797294417685632,0.,0.603590599270175));
#84218=DIRECTION('center_axis',(-2.16690239643906E-14,-1.,-8.63994232246378E-14));
#84219=DIRECTION('ref_axis',(2.20896652263452E-31,8.63994232246378E-14,
-1.));
#84220=DIRECTION('center_axis',(0.157437855437323,0.987363722701675,-0.0180610289846971));
#84221=DIRECTION('ref_axis',(0.310794110370792,-0.032180646490395,0.949932327563542));
#84222=DIRECTION('center_axis',(-0.153257677595432,0.987363722047016,0.0403108501959122));
#84223=DIRECTION('ref_axis',(0.243077569452302,-0.00187187794105808,0.970005047049826));
#84224=DIRECTION('',(0.603590599317295,0.,-0.79729441764996));
#84225=DIRECTION('center_axis',(0.155570611632627,-0.98736372193401,-0.0301772332209221));
#84226=DIRECTION('ref_axis',(0.0335217173615916,-0.0252547750561712,0.999118857194674));
#84227=DIRECTION('',(0.648899979430102,0.,0.760873719283045));
#84228=DIRECTION('center_axis',(1.72606145034788E-15,-1.,5.93584349259378E-14));
#84229=DIRECTION('ref_axis',(0.029066335084342,5.93835253667814E-14,0.999577484822845));
#84230=DIRECTION('center_axis',(0.15763963336802,0.987363722676915,0.0162057129797262));
#84231=DIRECTION('ref_axis',(0.0993205454413462,-0.0321806464481439,0.994534984426095));
#84232=DIRECTION('center_axis',(-0.158340239529387,0.987363722011668,0.00642253852005476));
#84233=DIRECTION('ref_axis',(0.0288721401833863,-0.00187188181618428,0.999581360160191));
#84234=DIRECTION('center_axis',(-0.163785815689771,-0.986495109135139,-0.00126737180284747));
#84235=DIRECTION('ref_axis',(0.0274586618280204,-0.00584312233850029,0.999605862233687));
#84236=DIRECTION('center_axis',(0.161633025665585,-0.98649510926358,-0.026498385106));
#84237=DIRECTION('ref_axis',(0.137216842249404,-0.00412443690745434,0.990532446325358));
#84238=DIRECTION('center_axis',(-0.16022904283391,-0.986495109287375,0.0339713582981242));
#84239=DIRECTION('ref_axis',(0.241702398635757,-0.00584313045738827,0.97033283378446));
#84240=DIRECTION('center_axis',(0.152157765743994,-0.986495109271346,-0.0606251903709286));
#84241=DIRECTION('ref_axis',(0.34694398407328,-0.00412443715934191,0.937876783449446));
#84242=DIRECTION('center_axis',(-0.149180137288371,-0.986495109329304,0.0676216378682646));
#84243=DIRECTION('ref_axis',(0.444644406204661,-0.00584312659425322,0.895688120889469));
#84244=DIRECTION('center_axis',(0.135567778586396,-0.986495109306673,-0.0919172275646138));
#84245=DIRECTION('ref_axis',(0.540448409869318,-0.00412443587822252,0.84136704552675));
#84246=DIRECTION('center_axis',(-0.131155737577983,-0.986495109243889,0.0981099991757331));
#84247=DIRECTION('ref_axis',(0.626795335741588,-0.00584312953040013,0.779162027392173));
#84248=DIRECTION('center_axis',(0.11263879340883,-0.986495109254255,-0.118911318371457));
#84249=DIRECTION('ref_axis',(0.708682071585451,-0.00412443451684314,0.705515917930468));
#84250=DIRECTION('center_axis',(-0.106998637769328,-0.986495109310485,0.124010849614069));
#84251=DIRECTION('ref_axis',(0.77963801399506,-0.00584312763501283,0.62620318187732));
#84252=DIRECTION('center_axis',(0.0844429366349232,-0.986495109286381,-0.140345252169501));
#84253=DIRECTION('ref_axis',(0.843778545533548,-0.00412444154263402,0.536675651654937));
#84254=DIRECTION('center_axis',(-0.0778384024322776,-0.986495109326809,
0.14411308886107));
#84255=DIRECTION('ref_axis',(0.896025684448892,-0.00584312812733907,0.443963771789526));
#84256=DIRECTION('center_axis',(0.0522986285574558,-0.986495109283444,-0.155216792940887));
#84257=DIRECTION('ref_axis',(0.939420873422059,-0.00412443980772976,0.342741026979858));
#84258=DIRECTION('center_axis',(-0.0450385345604746,-0.986495109243706,
0.157476759691369));
#84259=DIRECTION('ref_axis',(0.970516188902198,-0.00584313285570177,0.240965111327725));
#84260=DIRECTION('center_axis',(0.0177088989246973,-0.986495109263363,-0.162830569299322));
#84261=DIRECTION('ref_axis',(0.991136924909274,-0.00412443418164394,0.132780213601537));
#84262=DIRECTION('center_axis',(-0.0101327025402808,-0.986495109345221,
0.163476994030326));
#84263=DIRECTION('ref_axis',(0.999626435896561,-0.00584312539720088,0.0266991861735747));
#84264=DIRECTION('center_axis',(-0.017708886231778,-0.986495109292058,-0.16283057050591));
#84265=DIRECTION('ref_axis',(0.996508515296202,-0.00412443589834953,-0.0833892557268596));
#84266=DIRECTION('center_axis',(0.0252469101078213,-0.986495109231266,0.161833225861687));
#84267=DIRECTION('ref_axis',(0.981995261046375,-0.0058431313974677,-0.188815161197225));
#84268=DIRECTION('center_axis',(-0.0522986199379418,-0.986495109270012,
-0.155216795930509));
#84269=DIRECTION('ref_axis',(0.955284475706084,-0.00412443434778573,-0.295659533105672));
#84270=DIRECTION('center_axis',(0.0594460085246589,-0.986495109207122,0.152622316785305));
#84271=DIRECTION('ref_axis',(0.918447080136415,-0.00584313396351778,-0.395500719056714));
#84272=DIRECTION('center_axis',(-0.0844429344225918,-0.986495109307054,
-0.140345253355305));
#84273=DIRECTION('ref_axis',(0.869392394054461,-0.00412443895913273,-0.494105104369026));
#84274=DIRECTION('center_axis',(0.0908654815661706,-0.986495109203758,0.136274956528388));
#84275=DIRECTION('ref_axis',(0.811953333948451,-0.00584313273512341,-0.583693105398577));
#84276=DIRECTION('center_axis',(-0.112638782506712,-0.986495109231985,-0.118911328883243));
#84277=DIRECTION('ref_axis',(0.742848493168704,-0.00412443353133674,-0.669446865139445));
#84278=DIRECTION('center_axis',(0.118036188482337,-0.986495109330825,0.11355552595504));
#84279=DIRECTION('ref_axis',(0.667493552315554,-0.00584312610117444,-0.744592650712138));
#84280=DIRECTION('center_axis',(-0.135567769450099,-0.986495109256,-0.0919172415834949));
#84281=DIRECTION('ref_axis',(0.581569820465018,-0.00412443070425866,-0.81348603736982));
#84282=DIRECTION('center_axis',(0.139687648469892,-0.986495109284145,0.0855263715085294));
#84283=DIRECTION('ref_axis',(0.491822512892929,-0.00584312859394028,-0.870675871757061));
#84284=DIRECTION('center_axis',(-0.152157762777686,-0.986495109280063,-0.0606251976739593));
#84285=DIRECTION('ref_axis',(0.393097587747994,-0.00412443771534683,-0.919487506995196));
#84286=DIRECTION('center_axis',(0.154807469423525,-0.986495109257913,0.0534981010962386));
#84287=DIRECTION('ref_axis',(0.293154401945519,-0.00584313246842049,-0.956047255329422));
#84288=DIRECTION('center_axis',(-0.161633024216978,-0.986495109294656,-0.0264983927851836));
#84289=DIRECTION('ref_axis',(0.186244550464229,-0.00412443791836214,-0.982494761530175));
#84290=DIRECTION('center_axis',(0.162688667483946,-0.986495109300973,0.0189683103506619));
#84291=DIRECTION('ref_axis',(0.0807787151376006,-0.00584312744504146,-0.996714932687566));
#84292=DIRECTION('center_axis',(-0.163550504854883,-0.986495109300725,0.00886745101275484));
#84293=DIRECTION('ref_axis',(-0.0293170730888086,-0.00412444202667359,-0.999561653027703));
#84294=DIRECTION('center_axis',(0.162962722649296,-0.986495109321913,-0.0164484136218403));
#84295=DIRECTION('ref_axis',(-0.135374094935768,-0.00584312658610667,-0.990777327300146));
#84296=DIRECTION('center_axis',(-0.157820545741235,-0.986495109287338,0.0438186569180516));
#84297=DIRECTION('ref_axis',(-0.243507866879218,-0.00412443949873136,-0.969890152422817));
#84298=DIRECTION('center_axis',(0.155616822593042,-0.986495109297829,-0.0510960258484943));
#84299=DIRECTION('ref_axis',(-0.34519696219726,-0.00584312798122105,-0.938512075119536));
#84300=DIRECTION('center_axis',(-0.144711073722153,-0.986495109289193,0.076720952097095));
#84301=DIRECTION('ref_axis',(-0.446312499512019,-0.00412443849907849,-0.894867667192419));
#84302=DIRECTION('center_axis',(0.140994452051794,-0.986495109320717,-0.0833544466535578));
#84303=DIRECTION('ref_axis',(-0.53887880255101,-0.00584312705756995,-0.842363041703148));
#84304=DIRECTION('center_axis',(-0.124835075987998,-0.986495109277208,0.106035857968992));
#84305=DIRECTION('ref_axis',(-0.628248057932132,-0.00412443289639802,-0.778002163723076));
#84306=DIRECTION('center_axis',(0.119779342921941,-0.986495109199128,-0.111715301258998));
#84307=DIRECTION('ref_axis',(-0.7073632684812,-0.00584313333012281,-0.706826049460884));
#84308=DIRECTION('center_axis',(-0.0991219242755701,-0.986495109247181,
0.130392651477376));
#84309=DIRECTION('ref_axis',(-0.780807435100502,-0.00412443550550682,-0.624758143863317));
#84310=DIRECTION('center_axis',(0.0929634778324503,-0.986495109264974,-0.134852479345333));
#84311=DIRECTION('ref_axis',(-0.842772215666208,-0.00584312983766792,-0.538238655556037));
#84312=DIRECTION('center_axis',(-0.0687739426533017,-0.986495109277807,
0.148652427436915));
#84313=DIRECTION('ref_axis',(-0.896857124779159,-0.00412443574213562,-0.442301126793352));
#84314=DIRECTION('center_axis',(0.0618007488840924,-0.986495109226495,-0.151684102362676));
#84315=DIRECTION('ref_axis',(-0.938774069888716,-0.00584313211839086,-0.344483821843091));
#84316=DIRECTION('center_axis',(-0.0352101726582262,-0.986495109258675,
0.159961380183131));
#84317=DIRECTION('ref_axis',(-0.970970771535139,-0.00412443128434196,-0.239162601363671));
#84318=DIRECTION('center_axis',(0.0277482857856159,-0.986495109197101,-0.161423146314771));
#84319=DIRECTION('ref_axis',(-0.990879892697005,-0.00584313456157943,-0.134621305993024));
#84320=DIRECTION('center_axis',(-4.18658415555892E-9,-0.986495109267289,
0.163790718270967));
#84321=DIRECTION('ref_axis',(-0.999682904139737,-0.00412443729868955,-0.0248410987621459));
#84322=DIRECTION('center_axis',(-0.00760166424773501,-0.986495109286652,
-0.163614223263692));
#84323=DIRECTION('ref_axis',(-0.99665327290905,-0.00584312869504784,0.0815359518662326));
#84324=DIRECTION('center_axis',(0.0352101565309749,-0.986495109262151,0.15996138371157));
#84325=DIRECTION('ref_axis',(-0.98165097512954,-0.00412443485408824,0.19064194728432));
#84326=DIRECTION('center_axis',(-0.0425961641670186,-0.986495109300108,
-0.158154880181497));
#84327=DIRECTION('ref_axis',(-0.955824253713504,-0.00584312765218506,0.29388067965122));
#84328=DIRECTION('center_axis',(0.0687739335326133,-0.986495109263156,0.148652431753823));
#84329=DIRECTION('ref_axis',(-0.917718138243298,-0.00412443719897299,0.397210785046234));
#84330=DIRECTION('center_axis',(-0.0755989173093816,-0.986495109354155,
-0.145300388581668));
#84331=DIRECTION('ref_axis',(-0.870301954080379,-0.00584312361802103,0.492483874487539));
#84332=DIRECTION('center_axis',(0.0991219123679854,-0.986495109264719,0.130392660396599));
#84333=DIRECTION('ref_axis',(-0.810873820575113,-0.00412443265964962,0.585206490190561));
#84334=DIRECTION('center_axis',(-0.105066742165034,-0.986495109264701,-0.125651816889575));
#84335=DIRECTION('ref_axis',(-0.744085303337244,-0.00584312785497444,0.668059068656651));
#84336=DIRECTION('center_axis',(0.124835066434611,-0.98649510930135,0.106035868991502));
#84337=DIRECTION('ref_axis',(-0.666113944006964,-0.0041244354640061,0.745838590200045));
#84338=DIRECTION('center_axis',(-0.129621765649896,-0.986495109247229,-0.100127904707433));
#84339=DIRECTION('ref_axis',(-0.583076051165369,-0.00584312925752157,0.812396563506936));
#84340=DIRECTION('center_axis',(0.144711069366066,-0.986495109279995,0.0767209604318137));
#84341=DIRECTION('ref_axis',(-0.490207320958835,-0.00412443533582184,0.871596105723014));
#84342=DIRECTION('center_axis',(-0.148115819742761,-0.986495109250133,-0.0699221235911587));
#84343=DIRECTION('ref_axis',(-0.394802809718104,-0.00584313123430531,0.918747298910897));
#84344=DIRECTION('center_axis',(0.157820544757281,-0.986495109280205,0.0438186606225097));
#84345=DIRECTION('ref_axis',(-0.291379146863202,-0.00412443951164448,0.956598756936254));
#84346=DIRECTION('center_axis',(-0.159684144067683,-0.986495109300543,-0.0364468580193389));
#84347=DIRECTION('ref_axis',(-0.18806902754466,-0.00584312910065061,0.982138431546551));
#84348=DIRECTION('center_axis',(0.163550506209464,-0.986495109038151,0.00886745524006982));
#84349=DIRECTION('ref_axis',(-0.0789264177712791,-0.00412443861087988,0.99687191232572));
#84350=DIRECTION('center_axis',(0.15712354266245,0.986495109435393,0.0462557174979818));
#84351=DIRECTION('ref_axis',(-0.0845282468056531,-0.0332319479630796,0.99586676474644));
#84352=DIRECTION('center_axis',(-0.160229052463087,0.986495108976718,-0.0339713219023825));
#84353=DIRECTION('ref_axis',(-0.18762955624287,0.00334931877564638,0.982234153187438));
#84354=DIRECTION('center_axis',(0.143506481236011,0.986495109925276,0.0789511743850364));
#84355=DIRECTION('ref_axis',(-0.296633918114572,-0.0332319218886669,0.954412886538936));
#84356=DIRECTION('center_axis',(-0.14918015440409,0.986495109054244,-0.067621604121956));
#84357=DIRECTION('ref_axis',(-0.394394189435828,0.00334932227517103,0.918935256358985));
#84358=DIRECTION('center_axis',(0.123179213512155,0.986495110027753,0.107954987146767));
#84359=DIRECTION('ref_axis',(-0.494869342219976,-0.0332319165515335,0.868331718787861));
#84360=DIRECTION('center_axis',(-0.131155762220521,0.986495108970641,-0.0981099689805186));
#84361=DIRECTION('ref_axis',(-0.5827173879895,0.00334931822458211,0.812667968977567));
#84362=DIRECTION('center_axis',(0.0970922175602616,0.986495109914703,0.13191095255364));
#84363=DIRECTION('ref_axis',(-0.669965224461655,-0.0332319210725802,0.741648324634979));
#84364=DIRECTION('center_axis',(-0.10699866856939,0.986495109004646,-0.12401082547217));
#84365=DIRECTION('ref_axis',(-0.743793371796284,0.00334931980664887,0.668401228401585));
#84366=DIRECTION('center_axis',(0.0664652972180845,0.986495109850739,0.149698906162635));
#84367=DIRECTION('ref_axis',(-0.813734276754544,-0.0332319242107122,0.580286279389762));
#84368=DIRECTION('center_axis',(-0.0778384347764584,0.986495109011886,-0.144113073547051));
#84369=DIRECTION('ref_axis',(-0.870090401643211,0.00334932307507521,0.492880791879025));
#84370=DIRECTION('center_axis',(0.0327305405511539,0.986495109972787,0.160487101397616));
#84371=DIRECTION('ref_axis',(-0.919454018071839,-0.0332319192853551,0.391790694366472));
#84372=DIRECTION('center_axis',(-0.0450385678146406,0.986495108996408,-0.157476751729809));
#84373=DIRECTION('ref_axis',(-0.955702972692551,0.0033493195060858,0.294313795200746));
#84374=DIRECTION('center_axis',(-0.00253465994445632,0.986495110068069,
0.16377110035276));
#84375=DIRECTION('ref_axis',(-0.982181112188289,-0.0332319150790252,0.184975411016589));
#84376=DIRECTION('center_axis',(-0.0101327460188246,0.986495108992418,-0.16347699346439));
#84377=DIRECTION('ref_axis',(-0.996627934277689,0.00334931820573886,0.081985015002393));
#84378=DIRECTION('center_axis',(-0.0376813519129768,0.986495109949854,0.159397345533218));
#84379=DIRECTION('ref_axis',(-0.998982508909587,-0.0332319202960521,-0.0304891188154647));
#84380=DIRECTION('center_axis',(0.02524687742827,0.986495109027206,-0.161833232203781));
#84381=DIRECTION('ref_axis',(-0.990951681531433,0.00334932228370334,-0.134177296552975));
#84382=DIRECTION('center_axis',(-0.0710661011878459,0.986495109933046,0.147570347089602));
#84383=DIRECTION('ref_axis',(-0.969072594036823,-0.0332319214002897,-0.244528008389197));
#84384=DIRECTION('center_axis',(0.0594459811191166,0.986495109049416,-0.152622328479048));
#84385=DIRECTION('ref_axis',(-0.93893962948678,0.00334932291028807,-0.344065624867221));
#84386=DIRECTION('center_axis',(-0.101127876712746,0.986495109938007,0.12884312406943));
#84387=DIRECTION('ref_axis',(-0.893849921483746,-0.033231920065598,-0.447133042116387));
#84388=DIRECTION('center_axis',(0.0908654531082973,0.986495109005426,-0.136274976939262));
#84389=DIRECTION('ref_axis',(-0.843023804543385,0.00334931910330392,-0.53786582623805));
#84390=DIRECTION('center_axis',(-0.126461025342994,0.986495109956393,0.104091340184102));
#84391=DIRECTION('ref_axis',(-0.776831821485583,-0.033231919097129,-0.628830629566112));
#84392=DIRECTION('center_axis',(0.118036163879419,0.986495109044257,-0.113555554018244));
#84393=DIRECTION('ref_axis',(-0.707689122394941,0.00334932327296944,-0.706516021104611));
#84394=DIRECTION('center_axis',(-0.145880998923188,0.986495109926482,0.0744723589280713));
#84395=DIRECTION('ref_axis',(-0.62348992709468,-0.0332319204812905,-0.781124798142138));
#84396=DIRECTION('center_axis',(0.13968763128992,0.986495109047707,-0.0855264022952221));
#84397=DIRECTION('ref_axis',(-0.539263682656536,0.00334932285080722,-0.842130312127613));
#84398=DIRECTION('center_axis',(-0.1584797400563,0.986495109801124,0.0413711291863717));
#84399=DIRECTION('ref_axis',(-0.440994335358874,-0.0332319254215281,-0.896894439337296));
#84400=DIRECTION('center_axis',(0.154807460333395,0.986495109016585,-0.0534981318503795));
#84401=DIRECTION('ref_axis',(-0.345622874549849,0.00334932213427141,-0.938367524283071));
#84402=DIRECTION('center_axis',(-0.163668140770195,0.986495109923557,0.00633543950617634));
#84403=DIRECTION('ref_axis',(-0.237878339260044,-0.0332319212560437,-0.970726292587419));
#84404=DIRECTION('center_axis',(0.162688664882239,0.986495109019678,-0.0189683472946007));
#84405=DIRECTION('ref_axis',(-0.135821122852929,0.00334932200186453,-0.990727714676993));
#84406=DIRECTION('center_axis',(-0.161203602974452,0.98649510998187,-0.0289964889238977));
#84407=DIRECTION('ref_axis',(-0.0236394202842747,-0.0332319187916197,-0.999168062631132));
#84408=DIRECTION('center_axis',(0.162962728442386,0.986495108997507,0.0164483756830008));
#84409=DIRECTION('ref_axis',(0.0803314697776428,0.00334932208550028,-0.996762578052031));
#84410=DIRECTION('center_axis',(-0.151201364507919,0.986495110021318,-0.0629725755783483));
#84411=DIRECTION('ref_axis',(0.191704853736926,-0.0332319178461485,-0.980889845339409));
#84412=DIRECTION('center_axis',(0.155616836747566,0.986495109020785,0.0510959880886054));
#84413=DIRECTION('ref_axis',(0.292727855798555,0.00334931856927389,-0.956189931187681));
#84414=DIRECTION('center_axis',(-0.134129119682807,0.986495110072656,-0.0940041331849542));
#84415=DIRECTION('ref_axis',(0.398085224325408,-0.0332319147272993,-0.916746308428535));
#84416=DIRECTION('center_axis',(0.140994470581048,0.986495109053583,0.083354418472747));
#84417=DIRECTION('ref_axis',(0.491436612895278,0.00334932584772274,-0.870906905198473));
#84418=DIRECTION('center_axis',(-0.110785145530079,0.986495110071087,-0.12064016468703));
#84419=DIRECTION('ref_axis',(0.585851568710888,-0.033231915064203,-0.809736734537934));
#84420=DIRECTION('center_axis',(0.11977936442388,0.986495109030295,0.111715279695832));
#84421=DIRECTION('ref_axis',(0.667166337497202,0.00334932295266879,-0.744901241874605));
#84422=DIRECTION('center_axis',(-0.0822609770536327,0.986495109954466,-0.141635199333031));
#84423=DIRECTION('ref_axis',(0.746224147227216,-0.0332319201177854,-0.66486476939322));
#84424=DIRECTION('center_axis',(0.0929635057152089,0.986495109045637,0.134852461728273));
#84425=DIRECTION('ref_axis',(0.811700106743077,0.00334932408193139,-0.584064824091875));
#84426=DIRECTION('center_axis',(-0.0498903763927356,0.986495109833051,-0.156007527442964));
#84427=DIRECTION('ref_axis',(0.871704114499594,-0.0332319238633797,-0.488904465106239));
#84428=DIRECTION('center_axis',(0.0618007766378893,0.986495109035607,0.151684092296388));
#84429=DIRECTION('ref_axis',(0.918279682544927,0.00334932473737517,-0.395918181761071));
#84430=DIRECTION('center_axis',(-0.0151869682934995,0.986495110040763,-0.163085112317817));
#84431=DIRECTION('ref_axis',(0.956424164040124,-0.0332319160599138,-0.29008353658065));
#84432=DIRECTION('center_axis',(0.0277483150289102,0.986495109025233,0.161423142338237));
#84433=DIRECTION('ref_axis',(0.98192151939393,0.0033493226463211,-0.189258848641028));
#84434=DIRECTION('center_axis',(0.0202265769072787,0.986495109950066,-0.162537022340209));
#84435=DIRECTION('ref_axis',(0.996422884216933,-0.0332319196220728,-0.0776986185658488));
#84436=DIRECTION('center_axis',(-0.0076016257944453,0.986495109024876,0.163614226628614));
#84437=DIRECTION('ref_axis',(0.999649797962388,0.00334931933611909,0.0262500189284213));
#84438=DIRECTION('center_axis',(0.0546943469278073,0.986495109914991,-0.154388880842986));
#84439=DIRECTION('ref_axis',(0.989829977359144,-0.0332319208452661,0.138319396174687));
#84440=DIRECTION('center_axis',(-0.0425961353137144,0.986495109055382,0.158154889479096));
#84441=DIRECTION('ref_axis',(0.970635562333554,0.00334932831784015,0.240531468072776));
#84442=DIRECTION('center_axis',(0.0866046692179882,0.986495109923493,-0.139021686677578));
#84443=DIRECTION('ref_axis',(0.936953721048867,-0.0332319209181787,0.347869751551886));
#84444=DIRECTION('center_axis',(-0.0755988798102178,0.986495109009909,0.145300410429456));
#84445=DIRECTION('ref_axis',(0.896235487868925,0.00334931975946973,0.443565927841058));
#84446=DIRECTION('center_axis',(0.114465449777541,0.986495110036967,-0.117153995580081));
#84447=DIRECTION('ref_axis',(0.840266549276586,-0.0332319161818368,0.541154105513118));
#84448=DIRECTION('center_axis',(-0.105066715113567,0.986495109010335,0.125651841506333));
#84449=DIRECTION('ref_axis',(0.779928436803072,0.0033493221170034,0.625859741082036));
#84450=DIRECTION('center_axis',(0.136973958783264,0.986495109992769,-0.0898083101700282));
#84451=DIRECTION('ref_axis',(0.704289448443,-0.0332319188577156,0.709134692693066));
#84452=DIRECTION('center_axis',(-0.129621746388085,0.986495109054189,0.100127931544929));
#84453=DIRECTION('ref_axis',(0.627152799867747,0.00334932424359592,0.778889047069707));
#84454=DIRECTION('center_axis',(0.153077714731913,0.98649511003431,-0.0582632914522498));
#84455=DIRECTION('ref_axis',(0.5353805562444,-0.0332319168564682,0.843956930001456));
#84456=DIRECTION('center_axis',(-0.148115806239736,0.986495109048684,0.0699221550367086));
#84457=DIRECTION('ref_axis',(0.445052195942097,0.00334932140284593,0.895498366795416));
#84458=DIRECTION('center_axis',(0.162023729773525,0.986495109914706,-0.0239939389148083));
#84459=DIRECTION('ref_axis',(0.341437862680118,-0.0332319224161379,0.939316679965261));
#84460=DIRECTION('center_axis',(-0.159684137199492,0.9864951090058,0.0364468960885444));
#84461=DIRECTION('ref_axis',(0.242141441283249,0.0033493185268396,0.970235179984047));
#84462=DIRECTION('center_axis',(0.163393692715904,0.986495109888097,0.0113973394935696));
#84463=DIRECTION('ref_axis',(0.13152991478354,-0.0332319233338571,0.990755025618628));
#84464=DIRECTION('center_axis',(-0.163785816773439,0.986495108928238,0.00126739280443092));
#84465=DIRECTION('ref_axis',(0.0279084234544092,0.00334934443904838,0.99960487283332));
#84466=DIRECTION('center_axis',(0.158340237893585,0.987363722701301,0.00642247282834522));
#84467=DIRECTION('ref_axis',(0.10038315980289,-0.0225682600917394,0.994692864589075));
#84468=DIRECTION('',(-0.603935214477145,0.,0.797033410036521));
#84469=DIRECTION('center_axis',(-0.155457922179175,0.987363721843173,0.0307524831473961));
#84470=DIRECTION('ref_axis',(0.169586056764272,-0.00399376666708634,0.985507290271845));
#84471=DIRECTION('',(-0.797033410730744,0.,-0.603935213560956));
#84472=DIRECTION('center_axis',(-1.44211143998122E-14,-1.,-5.7605855884159E-14));
#84473=DIRECTION('ref_axis',(1.88000594205393E-31,5.7605855884159E-14,-1.));
#84474=DIRECTION('center_axis',(-0.158420672394944,-0.98736372164076,0.00397136571504476));
#84475=DIRECTION('ref_axis',(0.165372899663439,-0.02256800269505,0.985972864388905));
#84476=DIRECTION('center_axis',(0.149059806197162,-0.987363722366908,-0.0537964118713228));
#84477=DIRECTION('ref_axis',(0.245793064245949,-0.0156997426146358,0.969195175210041));
#84478=DIRECTION('center_axis',(0.156018974387301,0.987363722599173,-0.027766147126286));
#84479=DIRECTION('ref_axis',(0.311865820899157,-0.0225682650208507,0.949858085804845));
#84480=DIRECTION('',(-0.418476923230307,0.,0.908227430065672));
#84481=DIRECTION('center_axis',(-0.145212528016864,0.987363721832163,0.0634523641536714));
#84482=DIRECTION('ref_axis',(0.377476166873708,-0.00399376522103734,0.926010687455437));
#84483=DIRECTION('',(-0.908227431050156,0.,-0.418476921093665));
#84484=DIRECTION('center_axis',(2.31590738330052E-14,-1.,4.65140809571269E-14));
#84485=DIRECTION('ref_axis',(-1.25528131886048E-31,-4.65140809571269E-14,
-1.));
#84486=DIRECTION('center_axis',(-0.15386315511425,-0.98736372188743,0.0379342879054026));
#84487=DIRECTION('ref_axis',(0.373461598612057,-0.0225679937784545,0.927371079999232));
#84488=DIRECTION('center_axis',(0.134010233686999,-0.987363722422057,-0.0845821311626506));
#84489=DIRECTION('ref_axis',(0.448394871139783,-0.0156997398795868,0.893697688093267));
#84490=DIRECTION('center_axis',(0.14640243582563,0.987363722649047,-0.0606564586910423));
#84491=DIRECTION('ref_axis',(0.508765982049945,-0.0225682636858441,0.86060899889727));
#84492=DIRECTION('',(-0.213451112797401,0.,0.976953746318397));
#84493=DIRECTION('center_axis',(-0.128177159307217,0.987363721827163,0.0931852813031351));
#84494=DIRECTION('ref_axis',(0.567715906841173,-0.00399376197540127,0.823214855906274));
#84495=DIRECTION('',(-0.976953746694739,0.,-0.213451111074907));
#84496=DIRECTION('center_axis',(-3.72763200032572E-14,-1.,-4.62263900319702E-14));
#84497=DIRECTION('ref_axis',(-1.48754987227568E-31,4.62263900319702E-14,
-1.));
#84498=DIRECTION('center_axis',(-0.142111171391025,-0.987363721797395,0.0701234329184363));
#84499=DIRECTION('ref_axis',(0.564087641138766,-0.0225679966417213,0.825406456627328));
#84500=DIRECTION('center_axis',(0.112694491064729,-0.987363722439752,-0.111412886568739));
#84501=DIRECTION('ref_axis',(0.630030234816697,-0.0156997393169039,0.776411889013943));
#84502=DIRECTION('center_axis',(0.129940280587677,0.987363722695499,-0.0907105428584852));
#84503=DIRECTION('ref_axis',(0.681876811644499,-0.0225682605544513,0.73111879154969));
#84504=DIRECTION('',(0.00155543204822409,0.,0.99999879031484));
#84505=DIRECTION('center_axis',(-0.105148369505461,0.987363721822415,0.118560959929194));
#84506=DIRECTION('ref_axis',(0.731409885236659,-0.00399375923834658,0.68192641074037));
#84507=DIRECTION('',(-0.999998790317524,0.,0.00155543032291784));
#84508=DIRECTION('center_axis',(-3.47565958367976E-14,-1.,-2.78492518591803E-14));
#84509=DIRECTION('ref_axis',(1.,-3.47565958367976E-14,-1.19813090436101E-31));
#84510=DIRECTION('center_axis',(-0.123714231112402,-0.98736372160937,0.0990336825022796));
#84511=DIRECTION('ref_axis',(0.728337575162783,-0.0225680037404996,0.684846743303322));
#84512=DIRECTION('center_axis',(0.0861092731980021,-0.987363722354366,-0.13303410407802));
#84513=DIRECTION('ref_axis',(0.782206083646391,-0.0156997469095425,0.622821933343352));
#84514=DIRECTION('center_axis',(0.107402265374242,0.987363722656843,-0.116523098884737));
#84515=DIRECTION('ref_axis',(0.823103837842111,-0.0225682622741833,0.567442283996806));
#84516=DIRECTION('',(0.216489246715154,0.,0.976285002474536));
#84517=DIRECTION('center_axis',(-0.077202954207757,0.987363721838984,0.138392863464355));
#84518=DIRECTION('ref_axis',(0.86090394918356,-0.0039937628012165,0.508751845341948));
#84519=DIRECTION('',(-0.976285002225685,0.,0.216489247837379));
#84520=DIRECTION('center_axis',(3.9930771852328E-14,-1.,1.97265111112018E-14));
#84521=DIRECTION('ref_axis',(1.,3.9930771852328E-14,-6.35163460405498E-32));
#84522=DIRECTION('center_axis',(-0.0995325366648503,-0.987363721950605,
0.12331323822246));
#84523=DIRECTION('ref_axis',(0.858531254097983,-0.0225679922629129,0.512264357009314));
#84524=DIRECTION('center_axis',(0.0554976885393332,-0.987363722365339,-0.148434788118059));
#84525=DIRECTION('ref_axis',(0.89780684558997,-0.0156997443940525,0.440109515959095));
#84526=DIRECTION('center_axis',(0.079842234321559,0.987363722730416,-0.13688716760338));
#84527=DIRECTION('ref_axis',(0.925843445770208,-0.0225682581826276,0.377232802983714));
#84528=DIRECTION('',(0.421300264062744,0.,0.906921213502398));
#84529=DIRECTION('center_axis',(-0.0456476172175642,0.98736372183397,0.151753668319847));
#84530=DIRECTION('ref_axis',(0.950143101272476,-0.00399376292983926,0.311788609416672));
#84531=DIRECTION('',(-0.906921212507855,0.,0.421300266203668));
#84532=DIRECTION('center_axis',(4.32378293793031E-14,-1.,1.06813806392854E-14));
#84533=DIRECTION('ref_axis',(1.,4.32378293793031E-14,-1.52773325573375E-31));
#84534=DIRECTION('center_axis',(-0.0706968279110265,-0.987363721698004,
0.14182679435842));
#84535=DIRECTION('ref_axis',(0.948580963488652,-0.0225679997999443,0.315729062792722));
#84536=DIRECTION('center_axis',(0.0222910902134773,-0.987363722383866,-0.156894827885975));
#84537=DIRECTION('ref_axis',(0.971427156744944,-0.0156997459091039,0.236818067547269));
#84538=DIRECTION('center_axis',(0.0485488733164528,0.98736372271806,-0.150850541795637));
#84539=DIRECTION('ref_axis',(0.985291642253544,-0.022568258991991,0.169384336322413));
#84540=DIRECTION('',(0.606411752600289,0.,0.795150794697614));
#84541=DIRECTION('',(-0.795150795057726,0.,0.606411752128096));
#84542=DIRECTION('',(0.763168097828372,0.,0.646200011186184));
#84543=DIRECTION('center_axis',(0.0222910563515225,0.987363721854081,0.156894836030986));
#84544=DIRECTION('ref_axis',(0.993243163244486,-0.00399376358983429,-0.115983052729596));
#84545=DIRECTION('',(-0.6462000100523,0.,0.763168098788469));
#84546=DIRECTION('center_axis',(-6.55898797099622E-14,-1.,1.26914022202139E-14));
#84547=DIRECTION('ref_axis',(1.,-6.55898797099622E-14,-1.46963136636167E-31));
#84548=DIRECTION('center_axis',(-0.00461118059927081,-0.987363721673051,
0.158403340045037));
#84549=DIRECTION('ref_axis',(0.993479958729521,-0.0225680020847444,-0.111750869726782));
#84550=DIRECTION('center_axis',(-0.0456475817526598,-0.987363722372463,
-0.151753675484082));
#84551=DIRECTION('ref_axis',(0.981080735173516,-0.0156997448954984,-0.192961418634945));
#84552=DIRECTION('center_axis',(-0.0192787363169843,0.987363722720525,-0.157293386324687));
#84553=DIRECTION('ref_axis',(0.96534911195294,-0.0225682574057377,-0.259984164535724));
#84554=DIRECTION('',(0.884239552545667,0.,0.467033632315531));
#84555=DIRECTION('center_axis',(0.0554976572498314,0.987363721828398,0.148434803388402));
#84556=DIRECTION('ref_axis',(0.945088761644806,-0.00399376484876287,-0.326789354867965));
#84557=DIRECTION('',(-0.467033631299099,0.,0.884239553082522));
#84558=DIRECTION('center_axis',(2.72569548792655E-14,-1.,-1.17753642764545E-14));
#84559=DIRECTION('ref_axis',(1.,2.72569548792655E-14,-8.37905660890704E-32));
#84560=DIRECTION('center_axis',(0.0295486617759713,-0.987363721604755,0.155691225976474));
#84561=DIRECTION('ref_axis',(0.946229815089767,-0.0225680027411708,-0.32270702237085));
#84562=DIRECTION('center_axis',(-0.0772029153070725,-0.987363722443341,
-0.13839288085345));
#84563=DIRECTION('ref_axis',(0.916662612281878,-0.01569973864484,-0.399353444270922));
#84564=DIRECTION('center_axis',(-0.0526414311335554,0.987363722607825,-0.149471599329872));
#84565=DIRECTION('ref_axis',(0.886890876746755,-0.0225682654117284,-0.461427400724835));
#84566=DIRECTION('',(0.963964949091376,0.,0.266029278319627));
#84567=DIRECTION('center_axis',(0.0861092440564124,0.98736372182379,0.133034126878435));
#84568=DIRECTION('ref_axis',(0.852743060306908,-0.00399376025843779,-0.522315348211603));
#84569=DIRECTION('',(-0.266029277211529,0.,0.963964949397182));
#84570=DIRECTION('center_axis',(-5.4198781169427E-14,-1.,3.90588803916287E-14));
#84571=DIRECTION('ref_axis',(1.,-5.4198781169427E-14,-4.4243770373351E-31));
#84572=DIRECTION('center_axis',(0.0623268493950371,-0.98736372187317,0.145699157764377));
#84573=DIRECTION('ref_axis',(0.854735017319459,-0.0225679935913295,-0.518573751585216));
#84574=DIRECTION('center_axis',(-0.105148334878449,-0.987363722399287,-0.11856098583477));
#84575=DIRECTION('ref_axis',(0.809382363103314,-0.015699741278534,-0.587072149246651));
#84576=DIRECTION('center_axis',(-0.0835426830519901,0.987363722660821,-0.134660682019068));
#84577=DIRECTION('ref_axis',(0.766962608774369,-0.0225682608416332,-0.641294807670075));
#84578=DIRECTION('',(0.99861641532288,0.,0.0525856924237102));
#84579=DIRECTION('center_axis',(0.112694467126882,0.987363721854894,0.111412915965074));
#84580=DIRECTION('ref_axis',(0.720524038701269,-0.00399376641948853,-0.693418459145268));
#84581=DIRECTION('',(-0.0525856941427118,0.,0.99861641523236));
#84582=DIRECTION('center_axis',(9.89669757213282E-15,-1.,-1.10659647378638E-14));
#84583=DIRECTION('ref_axis',(7.27748752740703E-32,1.10659647378638E-14,
-1.));
#84584=DIRECTION('center_axis',(0.0921906888296262,-0.987363721661339,0.128894367759766));
#84585=DIRECTION('ref_axis',(0.723273756993294,-0.0225680022062431,-0.690192551192219));
#84586=DIRECTION('center_axis',(-0.128177133529277,-0.987363722357498,-0.0931853111416337));
#84587=DIRECTION('ref_axis',(0.664256296123621,-0.0156997428788034,-0.747340010392637));
#84588=DIRECTION('center_axis',(-0.11053756830992,0.987363722671541,-0.113553182008812));
#84589=DIRECTION('ref_axis',(0.611172022170688,-0.0225682598153682,-0.791175981033738));
#84590=DIRECTION('',(0.986573688235263,0.,-0.163316740360169));
#84591=DIRECTION('center_axis',(0.134010214694044,0.987363721846181,0.0845821679771451));
#84592=DIRECTION('ref_axis',(0.554614118231904,-0.00399376301988119,-0.832098088998399));
#84593=DIRECTION('',(0.163316741957422,0.,0.986573687970854));
#84594=DIRECTION('center_axis',(3.64323148098048E-14,-1.,-6.46737302459633E-14));
#84595=DIRECTION('ref_axis',(9.26601293729421E-32,6.46737302459633E-14,
-1.));
#84596=DIRECTION('center_axis',(0.117743806453333,-0.987363721981412,0.106062606779642));
#84597=DIRECTION('ref_axis',(0.557993023279549,-0.0225679909028752,-0.82953871022271));
#84598=DIRECTION('center_axis',(-0.145212512392438,-0.987363722361673,-0.0634523916710614));
#84599=DIRECTION('ref_axis',(0.488070340442066,-0.0156997468238425,-0.872663085463361));
#84600=DIRECTION('center_axis',(-0.132363838781167,0.987363722684511,-0.0871360620506701));
#84601=DIRECTION('ref_axis',(0.426803711705219,-0.022568259797764,-0.904062644579649));
#84602=DIRECTION('',(0.928399871491961,0.,-0.371582667267609));
#84603=DIRECTION('center_axis',(0.149059796702993,0.987363721816425,0.0537964482812778));
#84604=DIRECTION('ref_axis',(0.362771055313395,-0.00399376382293106,-0.931869739436437));
#84605=DIRECTION('',(0.371582668334801,0.,0.928399871064828));
#84606=DIRECTION('center_axis',(-8.67104292624063E-15,-1.,2.83974261068442E-14));
#84607=DIRECTION('ref_axis',(-5.0163862275377E-32,-2.83974261068442E-14,
-1.));
#84608=DIRECTION('center_axis',(0.137791344859856,-0.987363721744609,0.0782714907507665));
#84609=DIRECTION('ref_axis',(0.366621154304528,-0.0225679980487453,-0.930096562019497));
#84610=DIRECTION('center_axis',(-0.155457912687875,-0.987363722342947,-0.0307525150810445));
#84611=DIRECTION('ref_axis',(0.289062760137001,-0.0156997441135714,-0.957181403254758));
#84612=DIRECTION('center_axis',(-0.148000923706643,0.987363722699675,-0.0566445555955659));
#84613=DIRECTION('ref_axis',(0.222478534563419,-0.0225682585023063,-0.974676343904317));
#84614=DIRECTION('',(0.826815108418725,0.,-0.562473800714782));
#84615=DIRECTION('center_axis',(0.157139507936205,0.987363721861756,0.0204952627908948));
#84616=DIRECTION('ref_axis',(0.153965220883453,-0.0039937680742605,-0.988068196317885));
#84617=DIRECTION('',(0.562473799699905,0.,0.826815109109135));
#84618=DIRECTION('center_axis',(1.18185578346938E-15,-1.,-1.47987639615482E-14));
#84619=DIRECTION('ref_axis',(4.97525843814439E-33,1.47987639615482E-14,
-1.));
#84620=DIRECTION('center_axis',(0.151395916621486,-0.987363721839513,0.0468204786985774));
#84621=DIRECTION('ref_axis',(0.158106489918185,-0.0225679957185716,-0.987164131953242));
#84622=DIRECTION('center_axis',(-0.158434274587155,-0.987363722374232,0.00338531761313504));
#84623=DIRECTION('ref_axis',(0.0765389249906997,-0.015699744021737,-0.996942982822448));
#84624=DIRECTION('center_axis',(-0.156717649159304,0.987363722718713,-0.0235044145008221));
#84625=DIRECTION('ref_axis',(0.00775050626250672,-0.0225682595442366,-0.999715261118794));
#84626=DIRECTION('',(0.686569391286906,0.,-0.727064282541735));
#84627=DIRECTION('center_axis',(0.157871550275308,0.987363721803754,-0.0137642464199764));
#84628=DIRECTION('ref_axis',(-0.0620398544850762,-0.00399376025474478,-0.998065682374912));
#84629=DIRECTION('',(0.727064283330936,0.,0.686569390451156));
#84630=DIRECTION('center_axis',(-4.05414431250584E-15,-1.,-2.94136823488773E-14));
#84631=DIRECTION('ref_axis',(4.1025633915743E-32,2.94136823488773E-14,-1.));
#84632=DIRECTION('center_axis',(0.157921383722301,-0.987363721687767,0.0131801994717713));
#84633=DIRECTION('ref_axis',(-0.0578010613898766,-0.0225680004185413,-0.998073004674163));
#84634=DIRECTION('center_axis',(-0.154002425721324,-0.987363722322906,0.0373648593280209));
#84635=DIRECTION('ref_axis',(-0.13956378452677,-0.0156997468687922,-0.990088616234336));
#84636=DIRECTION('center_axis',(-0.158106432639921,0.987363722636627,0.010734764972707));
#84637=DIRECTION('ref_axis',(-0.207339927418302,-0.0225682625965862,-0.978008603245158));
#84638=DIRECTION('',(0.514220451397935,0.,-0.857658048037856));
#84639=DIRECTION('center_axis',(0.151221694258108,0.987363721834325,-0.0473801645330356));
#84640=DIRECTION('ref_axis',(-0.275144016599707,-0.00399376225466582,-0.961394726422209));
#84641=DIRECTION('',(0.85765804862894,0.,0.514220450412077));
#84642=DIRECTION('center_axis',(-2.31354740159072E-14,-1.,-6.26725925243937E-14));
#84643=DIRECTION('ref_axis',(-2.02413979510853E-31,6.26725925243937E-14,
-1.));
#84644=DIRECTION('center_axis',(0.157062622255562,-0.98736372175739,-0.0210763765292199));
#84645=DIRECTION('ref_axis',(-0.271005896921264,-0.0225679992448247,-0.962313093147956));
#84646=DIRECTION('center_axis',(-0.142369594341273,-0.987363722348708,0.0695972585437428));
#84647=DIRECTION('ref_axis',(-0.349140646055173,-0.0156997465692948,-0.936938806555602));
#84648=DIRECTION('center_axis',(-0.152102334687275,0.987363722657685,0.0444720020039294));
#84649=DIRECTION('ref_axis',(-0.412735373600482,-0.0225682618095411,-0.910571350821981));
#84650=DIRECTION('',(0.317827133913603,0.,-0.948148676605238));
#84651=DIRECTION('center_axis',(0.137500881589967,0.987363721812837,-0.0787806347390351));
#84652=DIRECTION('ref_axis',(-0.475382749181283,-0.00399375991611874,-0.879770022029949));
#84653=DIRECTION('',(0.948148676680187,0.,0.317827133690014));
#84654=DIRECTION('center_axis',(-3.60673343231128E-14,-1.,-5.62338991472549E-14));
#84655=DIRECTION('ref_axis',(-1.93076868610309E-33,5.62338991472549E-14,
-1.));
#84656=DIRECTION('center_axis',(0.148859786500606,-0.987363721793018,-0.0543474456624563));
#84657=DIRECTION('ref_axis',(-0.471538799476592,-0.0225679970353284,-0.881556490588089));
#84658=DIRECTION('center_axis',(-0.124079723161267,-0.987363722414623,0.0985753618292251));
#84659=DIRECTION('ref_axis',(-0.542392077558857,-0.0156997396972913,-0.839978780907485));
#84660=DIRECTION('center_axis',(-0.138986101500481,0.987363722635373,0.0761297761281104));
#84661=DIRECTION('ref_axis',(-0.59883177246696,-0.0225682627670856,-0.800556794862023));
#84662=DIRECTION('',(0.10657257433255,0.,-0.994304926267658));
#84663=DIRECTION('center_axis',(0.117350675322984,0.987363721832221,-0.106497416921091));
#84664=DIRECTION('ref_axis',(-0.653393114799153,-0.00399376605342258,-0.757008247884903));
#84665=DIRECTION('',(0.994304926390161,0.,0.106572573189616));
#84666=DIRECTION('center_axis',(0.,-1.,0.));
#84667=DIRECTION('ref_axis',(0.,0.,-1.));
#84668=DIRECTION('center_axis',(0.133696435217807,-0.987363721715313,-0.0850772839866021));
#84669=DIRECTION('ref_axis',(-0.650023071279847,-0.0225680003215464,-0.759579286293012));
#84670=DIRECTION('center_axis',(-0.0999880192034972,-0.987363722417943,
0.122944197377283));
#84671=DIRECTION('ref_axis',(-0.710281861740028,-0.0156997394700075,-0.70374227886613));
#84672=DIRECTION('center_axis',(-0.119371033888332,0.987363722615232,0.104227805943629));
#84673=DIRECTION('ref_axis',(-0.756927465696326,-0.0225682653976303,-0.653109091248529));
#84674=DIRECTION('',(-0.109665200773914,0.,-0.993968582873331));
#84675=DIRECTION('center_axis',(0.0917132874572295,0.987363721828803,-0.129234491217171));
#84676=DIRECTION('ref_axis',(-0.800851542707552,-0.00399376332935696,-0.598849610835144));
#84677=DIRECTION('',(0.993968582433906,0.,-0.10966520475671));
#84678=DIRECTION('center_axis',(3.1303237468505E-14,-1.,1.99401244391312E-14));
#84679=DIRECTION('ref_axis',(1.,3.1303237468505E-14,1.69915241587248E-31));
#84680=DIRECTION('center_axis',(0.112281583312903,-0.987363721782803,-0.111829007667775));
#84681=DIRECTION('ref_axis',(-0.798112985393402,-0.0225679969923309,-0.602085000691916));
#84682=DIRECTION('center_axis',(-0.0712209816399454,-0.987363722372648,
0.141564301703048));
#84683=DIRECTION('ref_axis',(-0.844959654147784,-0.0156997452244272,-0.534599570578153));
#84684=DIRECTION('center_axis',(-0.0941743020315624,0.98736372272103,0.127452265147924));
#84685=DIRECTION('ref_axis',(-0.879630072575917,-0.0225682586684263,-0.475122730587332));
#84686=DIRECTION('',(-0.320775152455513,0.,-0.947155373509089));
#84687=DIRECTION('center_axis',(0.0617874894451126,0.987363721814091,-0.145928705173099));
#84688=DIRECTION('ref_axis',(-0.910863042776533,-0.00399376005426055,-0.41268943187887));
#84689=DIRECTION('',(0.947155372266923,0.,-0.320775156123267));
#84690=DIRECTION('center_axis',(-9.0630598583574E-14,-1.,-3.31361281817047E-14));
#84691=DIRECTION('ref_axis',(1.,-9.0630598583574E-14,2.88384923956341E-31));
#84692=DIRECTION('center_axis',(0.0856165697309439,-0.987363721841294,-0.133351729569643));
#84693=DIRECTION('ref_axis',(-0.90888402603509,-0.0225679957248545,-0.416437885869201));
#84694=DIRECTION('center_axis',(-0.0391237406600589,-0.987363722421869,
0.15356501086509));
#84695=DIRECTION('ref_axis',(-0.940128071733025,-0.0156997387927986,-0.340459581949726));
#84696=DIRECTION('center_axis',(-0.0645740902690142,0.987363722699242,0.144717193047071));
#84697=DIRECTION('ref_axis',(-0.961202152072892,-0.0225682588743498,-0.274920163941863));
#84698=DIRECTION('',(-0.516886016398843,0.,-0.85605423078876));
#84699=DIRECTION('center_axis',(0.0289725594784648,0.987363721783673,-0.155799459892387));
#84700=DIRECTION('ref_axis',(-0.978283600768689,-0.00399377459283345,-0.207232348419715));
#84701=DIRECTION('',(0.856054231466657,0.,-0.516886015276125));
#84702=DIRECTION('center_axis',(-0.0319544625179998,0.987363722921529,0.155215305249591));
#84703=DIRECTION('ref_axis',(-0.997829489240866,-0.0225682578414181,-0.0618626231202355));
#84704=DIRECTION('',(-0.688827863670013,0.,-0.724924943860953));
#84705=DIRECTION('center_axis',(-3.67826898181065E-14,-1.,-4.9532785507768E-15));
#84706=DIRECTION('ref_axis',(1.,-3.67826898181065E-14,-3.24545121082182E-32));
#84707=DIRECTION('center_axis',(0.0549482210325186,-0.987363721850913,-0.148639072178465));
#84708=DIRECTION('ref_axis',(-0.977156658219623,-0.0225679947894841,-0.211318600478614));
#84709=DIRECTION('center_axis',(-0.00519719412118699,-0.987363723144184,
0.158385186782481));
#84710=DIRECTION('ref_axis',(-0.991337145602754,-0.015699656874459,-0.130400094026839));
#84711=DIRECTION('',(0.724924943069254,0.,-0.6888278645032));
#84712=DIRECTION('center_axis',(-0.00519706731890305,0.987363721807003,
-0.158385199279182));
#84713=DIRECTION('ref_axis',(-0.999960703086363,-0.0039937612537115,0.00791467965712267));
#84714=DIRECTION('center_axis',(-7.39750789299226E-15,-1.,6.13943474870816E-16));
#84715=DIRECTION('ref_axis',(1.,-7.39750789299226E-15,-2.44284292500047E-33));
#84716=DIRECTION('center_axis',(0.00215930891104003,0.987363722610884,0.158455724595244));
#84717=DIRECTION('ref_axis',(-0.987799426921624,-0.0225682652907615,0.154087525695875));
#84718=DIRECTION('center_axis',(0.0217105622614043,-0.987363721669521,-0.15697621672472));
#84719=DIRECTION('ref_axis',(-0.999738531004337,-0.0225680011955719,0.00368170440508826));
#84720=DIRECTION('center_axis',(0.0289725338067105,-0.987363722367395,0.155799460967041));
#84721=DIRECTION('ref_axis',(-0.996192397019456,-0.0156997433330986,0.0857567850371339));
#84722=DIRECTION('',(-0.828560885250734,0.,-0.559898972523187));
#84723=DIRECTION('center_axis',(-0.0391237013701955,0.987363721838545,-0.153565024625507));
#84724=DIRECTION('ref_axis',(-0.974880754886833,-0.0039937636615464,0.222691633437574));
#84725=DIRECTION('',(0.559898972904418,0.,-0.828560884993117));
#84726=DIRECTION('center_axis',(-5.67406285099299E-14,-1.,1.7518682747499E-14));
#84727=DIRECTION('ref_axis',(1.,-5.67406285099299E-14,-2.40727941335239E-31));
#84728=DIRECTION('center_axis',(-0.0125422691398479,-0.987363721795969,
-0.15797332802102));
#84729=DIRECTION('ref_axis',(-0.975573742112354,-0.0225679969457333,0.218509860680832));
#84730=DIRECTION('center_axis',(0.0617874444497453,-0.987363722445358,0.145928719953322));
#84731=DIRECTION('ref_axis',(-0.954466799122952,-0.0156997368295077,0.297903755658552));
#84732=DIRECTION('center_axis',(0.0361721262527808,0.987363722661402,0.154286928981594));
#84733=DIRECTION('ref_axis',(-0.931580962053001,-0.0225682611666196,0.362832722791536));
#84734=DIRECTION('',(-0.929551320671124,0.,-0.368692747743386));
#84735=DIRECTION('center_axis',(-0.0712209533168093,0.987363721839486,-0.141564319671038));
#84736=DIRECTION('ref_axis',(-0.904216466082979,-0.00399376523860615,0.427055771888904));
#84737=DIRECTION('',(0.368692746674862,0.,-0.929551321094939));
#84738=DIRECTION('center_axis',(2.58240326094427E-14,-1.,-1.4653331787943E-14));
#84739=DIRECTION('ref_axis',(1.,2.58240326094427E-14,8.15439645215452E-32));
#84740=DIRECTION('center_axis',(-0.0462086316812563,-0.987363721736649,
-0.151583783289969));
#84741=DIRECTION('ref_axis',(-0.905792208218432,-0.0225679996060896,0.423120740362082));
#84742=DIRECTION('center_axis',(0.0917132551112029,-0.987363722365354,0.129234510072732));
#84743=DIRECTION('ref_axis',(-0.868111393534543,-0.0156997432445028,0.496121080460778));
#84744=DIRECTION('center_axis',(0.0684935701650493,0.987363722660185,0.142903848865823));
#84745=DIRECTION('ref_axis',(-0.831802807343454,-0.0225682620060956,0.554612263879526));
#84746=DIRECTION('',(-0.987076969591494,0.,-0.160246859882096));
#84747=DIRECTION('center_axis',(-0.0999879913543567,0.987363721850669,-0.122944224582188));
#84748=DIRECTION('ref_axis',(-0.791272019556096,-0.00399376539654314,0.611451257996559));
#84749=DIRECTION('',(0.160246858747463,0.,-0.987076969775696));
#84750=DIRECTION('center_axis',(-7.72458675462459E-14,-1.,6.95175203573688E-14));
#84751=DIRECTION('ref_axis',(1.,-7.72458675462459E-14,-4.97137208957954E-31));
#84752=DIRECTION('center_axis',(-0.0777143321985765,-0.98736372173193,-0.138106348799036));
#84753=DIRECTION('ref_axis',(-0.79365683635452,-0.0225680000081501,0.60794696436726));
#84754=DIRECTION('center_axis',(0.117350647948898,-0.987363722424414,0.106497441594521));
#84755=DIRECTION('ref_axis',(-0.741164064492037,-0.0156997409901681,0.671140333789056));
#84756=DIRECTION('center_axis',(0.0976123325991251,0.987363722676726,0.124838742650328));
#84757=DIRECTION('ref_axis',(-0.69313047612766,-0.0225682612557523,0.720458754299603));
#84758=DIRECTION('',(-0.998447996527108,0.,0.0556919943169951));
#84759=DIRECTION('center_axis',(-0.12407970139484,0.987363721847796,-0.0985753949047921));
#84760=DIRECTION('ref_axis',(-0.64132857471426,-0.0039937650622799,0.767255960612626));
#84761=DIRECTION('',(-0.0556919954647224,0.,-0.998447996463089));
#84762=DIRECTION('center_axis',(-3.8890086548536E-14,-1.,5.43200255894411E-14));
#84763=DIRECTION('ref_axis',(2.22889452794712E-31,-5.43200255894411E-14,
-1.));
#84764=DIRECTION('center_axis',(-0.105586202327676,-0.987363721951747,-0.118171208217622));
#84765=DIRECTION('ref_axis',(-0.644410957040571,-0.0225679906816595,0.764346259389452));
#84766=DIRECTION('center_axis',(0.137500857919152,-0.987363722378517,0.0787806689634994));
#84767=DIRECTION('ref_axis',(-0.579560727718488,-0.0156997425922317,0.814777810798106));
#84768=DIRECTION('center_axis',(0.122166850809071,0.987363722695286,0.100936314915398));
#84769=DIRECTION('ref_axis',(-0.522048136227153,-0.0225682595929491,0.852617391988166));
#84770=DIRECTION('',(-0.963132705018756,0.,0.269026750571861));
#84771=DIRECTION('center_axis',(-0.142369580929604,0.987363721818591,-0.0695972934995943));
#84772=DIRECTION('ref_axis',(-0.461397319791492,-0.00399376042415553,0.887184627440592));
#84773=DIRECTION('',(-0.269026752423883,0.,-0.96313270450144));
#84774=DIRECTION('center_axis',(1.75357720910963E-14,-1.,-4.09401817561554E-14));
#84775=DIRECTION('ref_axis',(-1.24104711689061E-32,4.09401817561554E-14,
-1.));
#84776=DIRECTION('center_axis',(-0.128520969011961,-0.987363721781514,-0.0927105249364065));
#84777=DIRECTION('ref_axis',(-0.465033134446565,-0.0225679979504978,0.88500557587809));
#84778=DIRECTION('center_axis',(0.151221679088339,-0.987363722402413,0.0473802011113796));
#84779=DIRECTION('ref_axis',(-0.390857774145752,-0.0156997419415777,0.920317183634423));
#84780=DIRECTION('center_axis',(0.14100898137543,0.987363722679383,0.0723142192668541));
#84781=DIRECTION('ref_axis',(-0.326555403018843,-0.0225682609843977,0.944908589417697));
#84782=DIRECTION('',(-0.882782397777927,0.,0.469782117766793));
#84783=DIRECTION('center_axis',(-0.154002420805334,0.987363721837519,-0.0373648924159926));
#84784=DIRECTION('ref_axis',(-0.259891633084747,-0.00399376345168055,0.965629529843633));
#84785=DIRECTION('',(-0.469782117592815,0.,-0.882782397870512));
#84786=DIRECTION('center_axis',(-1.38747776376638E-15,-1.,7.2921159442934E-15));
#84787=DIRECTION('ref_axis',(-8.70967686797131E-33,-7.2921159442934E-15,
-1.));
#84788=DIRECTION('center_axis',(-0.145446243500322,-0.987363721891815,-0.0629147911352066));
#84789=DIRECTION('ref_axis',(-0.263910877837491,-0.0225679941728419,0.964283015612149));
#84790=DIRECTION('center_axis',(0.157871543102428,-0.98736372238965,0.0137642866619683));
#84791=DIRECTION('ref_axis',(-0.183878747956065,-0.0156997429578689,0.982823546788113));
#84792=DIRECTION('center_axis',(0.153257689853346,0.987363722748906,0.0403107864006331));
#84793=DIRECTION('ref_axis',(-0.115793303377786,-0.0225682571521611,0.993016910561937));
#84794=DIRECTION('',(-0.761154167861,0.,0.648570992835656));
#84795=DIRECTION('center_axis',(-4.25100139972006E-16,-1.,-1.48397940626387E-14));
#84796=DIRECTION('ref_axis',(0.0286342151763591,-1.48458815147681E-14,0.999589956792901));
#84797=DIRECTION('center_axis',(-0.155570611353887,-0.987363721584867,-0.0301772460814274));
#84798=DIRECTION('ref_axis',(-0.0504484436952952,-0.0225680051134673,0.998471651913023));
#84799=DIRECTION('center_axis',(0.157139508945422,-0.98736372241605,-0.0204952283498716));
#84800=DIRECTION('ref_axis',(0.0316982446689963,-0.0156997415914642,0.999374173870261));
#84801=DIRECTION('center_axis',(-0.15843427719912,0.987363721829461,-0.00338535426014318));
#84802=DIRECTION('ref_axis',(-0.0462337054453067,-0.00399376289762505,0.998922666845995));
#84803=DIRECTION('',(-0.648570992291408,0.,-0.761154168324748));
#84804=DIRECTION('center_axis',(-0.153405773087261,-0.987363727283469,-0.0397434123899093));
#84805=DIRECTION('ref_axis',(-0.157173522146972,-0.0153270656264595,0.987452057061606));
#84806=DIRECTION('',(0.562332021776287,0.,0.82691154139061));
#84807=DIRECTION('',(0.826911541049425,0.,-0.562332022278));
#84808=DIRECTION('center_axis',(0.153863114323219,-0.987363722524759,0.0379344367667496));
#84809=DIRECTION('ref_axis',(-0.219708301913583,0.00324330723637056,0.975560220093265));
#84810=DIRECTION('center_axis',(-0.141275571303142,-0.987363727223331,-0.0717919432570488));
#84811=DIRECTION('ref_axis',(-0.365771893840048,-0.0153270694356919,0.930578316220176));
#84812=DIRECTION('',(0.371423474713531,0.,0.928463570869491));
#84813=DIRECTION('center_axis',(-1.7351823490725E-14,-1.,5.67918761022166E-14));
#84814=DIRECTION('ref_axis',(-1.49127156747896E-31,-5.67918761022166E-14,
-1.));
#84815=DIRECTION('center_axis',(0.15047035997798,0.987363722444626,0.0497146896640039));
#84816=DIRECTION('ref_axis',(-0.221566403652918,-0.0153275630368041,0.975024817419364));
#84817=DIRECTION('center_axis',(-0.146402532268554,0.987363725081384,-0.0606561863190324));
#84818=DIRECTION('ref_axis',(-0.294469331016928,0.0150385452734834,0.955542597295641));
#84819=DIRECTION('',(0.928463571527175,0.,-0.37142347306949));
#84820=DIRECTION('center_axis',(0.14211109818593,-0.987363722486231,0.0701235715756216));
#84821=DIRECTION('ref_axis',(-0.424288253350281,0.00324330658409198,0.905521374143851));
#84822=DIRECTION('center_axis',(-0.122539482670012,-0.987363727276341,-0.10048355709238));
#84823=DIRECTION('ref_axis',(-0.557267181460097,-0.015327066655971,0.830191766699263));
#84824=DIRECTION('',(0.163147578338454,0.,0.986601676302193));
#84825=DIRECTION('center_axis',(2.91547221559089E-14,-1.,-5.17339845454345E-14));
#84826=DIRECTION('ref_axis',(-1.1435928490905E-30,5.17339845454345E-14,
-1.));
#84827=DIRECTION('center_axis',(0.136265258712005,0.98736372244224,0.0808990659597058));
#84828=DIRECTION('ref_axis',(-0.425987817925329,-0.0153275614763488,0.904599051977397));
#84829=DIRECTION('center_axis',(-0.129940438600569,0.987363725138663,-0.0907102899157286));
#84830=DIRECTION('ref_axis',(-0.492998214050994,0.0150385390808293,0.869900341007431));
#84831=DIRECTION('',(0.986601676591079,0.,-0.163147576591479));
#84832=DIRECTION('center_axis',(0.123714122094534,-0.987363722509705,0.0990338097124305));
#84833=DIRECTION('ref_axis',(-0.609028958882343,0.00324331036576084,0.793141354476338));
#84834=DIRECTION('center_axis',(-0.0980735815685175,-0.987363727196121,
-0.124476675789915));
#84835=DIRECTION('ref_axis',(-0.722705274136803,-0.0153270691020051,0.690986373011502));
#84836=DIRECTION('',(-0.0527569189652392,0.,0.998607384061071));
#84837=DIRECTION('center_axis',(9.89859460105397E-14,-1.,-1.10642673273612E-13));
#84838=DIRECTION('ref_axis',(3.23530552762749E-30,1.10642673273612E-13,
-1.));
#84839=DIRECTION('center_axis',(0.115688545146719,0.987363722462374,0.10830069292059));
#84840=DIRECTION('ref_axis',(-0.610490517346357,-0.0153275606209121,0.791875238983762));
#84841=DIRECTION('center_axis',(-0.107402468389288,0.987363725040729,-0.116522891560345));
#84842=DIRECTION('ref_axis',(-0.66847504879309,0.0150385452406436,0.743582511425679));
#84843=DIRECTION('',(0.998607383967675,0.,0.052756920733087));
#84844=DIRECTION('center_axis',(0.0995324170010677,-0.987363722526679,0.123313330196635));
#84845=DIRECTION('ref_axis',(-0.765292145204351,0.00324330536830047,0.643674928406265));
#84846=DIRECTION('center_axis',(-0.0690218637930236,-0.987363727041147,
-0.142649405333328));
#84847=DIRECTION('ref_axis',(-0.854350472246275,-0.0153270762106045,0.519471222790446));
#84848=DIRECTION('',(-0.266194559677108,0.,0.963919320481912));
#84849=DIRECTION('center_axis',(0.,-1.,0.));
#84850=DIRECTION('ref_axis',(0.,0.,-1.));
#84851=DIRECTION('center_axis',(0.0897023623906408,0.987363722436819,0.130638301417487));
#84852=DIRECTION('ref_axis',(-0.766447355673877,-0.0153275625774428,0.642124222254507));
#84853=DIRECTION('center_axis',(-0.0798424829433611,0.987363725095465,-0.136887005530275));
#84854=DIRECTION('ref_axis',(-0.812694733563037,0.0150385427962143,0.582495589914181));
#84855=DIRECTION('',(0.963919320010511,0.,0.2661945613841));
#84856=DIRECTION('center_axis',(0.0706966795421928,-0.987363722499517,0.141826862736246));
#84857=DIRECTION('ref_axis',(-0.885771123801721,0.00324330962918667,0.464110975071356));
#84858=DIRECTION('center_axis',(-0.0367427722384984,-0.987363727231605,
-0.154151999129244));
#84859=DIRECTION('ref_axis',(-0.946047190512105,-0.015327068845835,0.323666177233194));
#84860=DIRECTION('',(-0.467185239535495,0.,0.884159460708396));
#84861=DIRECTION('center_axis',(-8.17769184107928E-14,-1.,3.53120703705101E-14));
#84862=DIRECTION('ref_axis',(1.,-8.17769184107928E-14,4.80900128964418E-31));
#84863=DIRECTION('center_axis',(0.0595218018669185,0.987363722479098,0.146867404943148));
#84864=DIRECTION('ref_axis',(-0.886565968493784,-0.015327558313575,0.46234819072299));
#84865=DIRECTION('center_axis',(-0.0485491517023675,0.987363725125182,-0.150850436445856));
#84866=DIRECTION('ref_axis',(-0.918913715657819,0.015038541178121,0.394171822249098));
#84867=DIRECTION('',(0.88415945988124,0.,0.467185241100908));
#84868=DIRECTION('center_axis',(0.0385552524335785,-0.987363722507462,0.153708724495363));
#84869=DIRECTION('ref_axis',(-0.964832426832062,0.00324330488953956,0.262845713502707));
#84870=DIRECTION('center_axis',(-0.00274561996653052,-0.987363727123007,
-0.15844662171458));
#84871=DIRECTION('ref_axis',(-0.99350779309227,-0.0153270730418421,0.112726864131391));
#84872=DIRECTION('',(-0.646330857894656,0.,0.763057286272242));
#84873=DIRECTION('center_axis',(5.83040472254443E-14,-1.,-1.12712490979864E-14));
#84874=DIRECTION('ref_axis',(1.,5.83040472254443E-14,1.95425793165654E-31));
#84875=DIRECTION('center_axis',(0.0265580647611155,0.987363722491237,0.156229154463538));
#84876=DIRECTION('ref_axis',(-0.96522974321078,-0.0153275578722416,0.260953269362401));
#84877=DIRECTION('center_axis',(-0.0149857128551614,0.9873637250895,-0.157760269990921));
#84878=DIRECTION('ref_axis',(-0.982165313426428,0.0150385434514299,0.187417019805635));
#84879=DIRECTION('',(0.763057286545784,0.,0.646330857571712));
#84880=DIRECTION('center_axis',(0.00461101746230197,-0.987363722509209,
0.158403339581966));
#84881=DIRECTION('ref_axis',(-0.998779239687249,0.00324330703679607,0.0492900733335472));
#84882=DIRECTION('center_axis',(0.0313799112010356,-0.987363727124713,-0.155332454855419));
#84883=DIRECTION('ref_axis',(-0.994513076466955,-0.0153270729185943,-0.103483436220397));
#84884=DIRECTION('',(-0.795254762302715,0.,0.606275401970797));
#84885=DIRECTION('center_axis',(0.,-1.,0.));
#84886=DIRECTION('ref_axis',(0.,0.,-1.));
#84887=DIRECTION('center_axis',(-0.00764750030215644,0.987363722476008,
0.158285802513836));
#84888=DIRECTION('ref_axis',(-0.998760447427132,-0.0153275598347146,0.0473564627550317));
#84889=DIRECTION('center_axis',(0.0192784397313903,0.987363725081687,-0.157293407854043));
#84890=DIRECTION('ref_axis',(-0.999491953403475,0.0150385434598007,-0.0281011973466172));
#84891=DIRECTION('',(0.606275400562902,0.,0.795254763376047));
#84892=DIRECTION('center_axis',(-0.0295488213498787,-0.987363722475921,
0.155691190166067));
#84893=DIRECTION('ref_axis',(-0.986024244800647,0.00324330709653314,-0.166570314355205));
#84894=DIRECTION('center_axis',(0.0640381510629094,-0.987363727167838,-0.144955115403629));
#84895=DIRECTION('ref_axis',(-0.949016033550402,-0.0153270713953641,-0.314854964938944));
#84896=DIRECTION('',(-0.906993438031825,0.,0.421144753460387));
#84897=DIRECTION('center_axis',(-1.15295989682027E-13,-1.,-2.8503450786955E-14));
#84898=DIRECTION('ref_axis',(1.,-1.15295989682027E-13,1.50992885536303E-31));
#84899=DIRECTION('center_axis',(-0.041495475479177,0.987363722444346,0.152941181882454));
#84900=DIRECTION('ref_axis',(-0.985590222827933,-0.0153275606837138,-0.168454678027869));
#84901=DIRECTION('center_axis',(0.0526411530319517,0.987363725091179,-0.149471680868111));
#84902=DIRECTION('ref_axis',(-0.970083460286782,0.0150385428657411,-0.242305431855127));
#84903=DIRECTION('',(0.421144752952713,0.,0.906993438267554));
#84904=DIRECTION('center_axis',(-0.0623269906669315,-0.98736372250425,0.145699093054675));
#84905=DIRECTION('ref_axis',(-0.927163852952879,0.00324330825580986,-0.374642056807736));
#84906=DIRECTION('center_axis',(0.0937020379828365,-0.987363727189288,-0.127799836888554));
#84907=DIRECTION('ref_axis',(-0.859144055829087,-0.0153270694498359,-0.511504225080914));
#84908=DIRECTION('',(-0.976322108155361,0.,0.216321846162313));
#84909=DIRECTION('center_axis',(7.98547755975139E-14,-1.,3.94667141899776E-14));
#84910=DIRECTION('ref_axis',(1.,7.98547755975138E-14,-2.26916646106724E-30));
#84911=DIRECTION('center_axis',(-0.073403164279386,0.987363722488244,0.140445202794295));
#84912=DIRECTION('ref_axis',(-0.926334895999688,-0.0153275575962674,-0.37638906258203));
#84913=DIRECTION('center_axis',(0.0835424247531459,0.987363725082729,-0.134660824507808));
#84914=DIRECTION('ref_axis',(-0.895314942855587,0.0150385423990028,-0.445179733750325));
#84915=DIRECTION('',(0.216321844433724,0.,0.976322108538361));
#84916=DIRECTION('center_axis',(-0.0921908136359495,-0.987363722493434,
0.128894272118859));
#84917=DIRECTION('ref_axis',(-0.824950308713439,0.00324330202760705,-0.565195956412959));
#84918=DIRECTION('center_axis',(0.118984524740799,-0.987363727165298,-0.104668778298292));
#84919=DIRECTION('ref_axis',(-0.729099456103866,-0.0153270708733323,-0.684236117146333));
#84920=DIRECTION('',(-0.999999042317255,0.,0.00138396696961088));
#84921=DIRECTION('center_axis',(-2.31678794544605E-14,-1.,-1.85701401945779E-14));
#84922=DIRECTION('ref_axis',(1.,-2.31678794544605E-14,-7.0999417749956E-31));
#84923=DIRECTION('center_axis',(-0.101878611122322,0.987363722418195,0.12138215786627));
#84924=DIRECTION('ref_axis',(-0.82376517608398,-0.0153275631584234,-0.566723919099021));
#84925=DIRECTION('center_axis',(0.110537343690459,0.987363725132923,-0.113553379260571));
#84926=DIRECTION('ref_axis',(-0.778682493658275,0.0150385393935025,-0.627237926470523));
#84927=DIRECTION('',(0.00138396519504415,0.,0.999999042319711));
#84928=DIRECTION('center_axis',(-0.117743905255329,-0.987363722487702,0.106062492382807));
#84929=DIRECTION('ref_axis',(-0.684163005159501,0.00324330677383027,-0.72932192023296));
#84930=DIRECTION('center_axis',(0.138703424939811,-0.987363727212438,-0.0766435261136204));
#84931=DIRECTION('ref_axis',(-0.564962976342534,-0.0153270690604205,-0.82497388826326));
#84932=DIRECTION('',(-0.97691713277092,0.,-0.213618622078332));
#84933=DIRECTION('center_axis',(1.86341961019305E-14,-1.,2.31163898898676E-14));
#84934=DIRECTION('ref_axis',(-2.47023409854845E-31,-2.31163898898676E-14,
-1.));
#84935=DIRECTION('center_axis',(-0.125590320890986,0.987363722425395,0.0966434215907506));
#84936=DIRECTION('ref_axis',(-0.682677114237897,-0.0153275619638483,-0.730559390836955));
#84937=DIRECTION('center_axis',(0.13236366662272,0.987363725051147,-0.0871362967500453));
#84938=DIRECTION('ref_axis',(-0.625639715317128,0.0150385470019746,-0.779967171566837));
#84939=DIRECTION('',(-0.213618626551051,0.,0.976917131792888));
#84940=DIRECTION('center_axis',(-0.13779142013565,-0.987363722500148,0.0782713487021446));
#84941=DIRECTION('ref_axis',(-0.511385000068983,0.00324330953190384,-0.859345601401279));
#84942=DIRECTION('center_axis',(0.151936708248103,-0.987363727213298,-0.0450345075491616));
#84943=DIRECTION('ref_axis',(-0.374409458267511,-0.0153270686067452,-0.927136796016507));
#84944=DIRECTION('',(-0.908155662980834,0.,-0.418632645401481));
#84945=DIRECTION('center_axis',(1.32291984440385E-14,-1.,2.6581742884735E-14));
#84946=DIRECTION('ref_axis',(-2.29532064287214E-31,-2.6581742884735E-14,
-1.));
#84947=DIRECTION('center_axis',(-0.143429566062224,0.987363722443134,0.0673857491049875));
#84948=DIRECTION('ref_axis',(-0.509667831387102,-0.0153275583912248,-0.860234716576198));
#84949=DIRECTION('center_axis',(0.14800080553809,0.987363725055514,-0.0566448232813552));
#84950=DIRECTION('ref_axis',(-0.443342720814214,0.0150385466523101,-0.896226017261068));
#84951=DIRECTION('',(-0.418632647009715,0.,0.908155662239486));
#84952=DIRECTION('center_axis',(-0.15139595935967,-0.987363722529884,0.0468203259439202));
#84953=DIRECTION('ref_axis',(-0.314695199533534,0.00324330913949309,-0.949187237765223));
#84954=DIRECTION('center_axis',(0.15806560158646,-0.987363727076912,-0.0113197194267311));
#84955=DIRECTION('ref_axis',(-0.166348965609218,-0.0153270737247311,-0.985947819335172));
#84956=DIRECTION('',(-0.79692984530751,0.,-0.604071867957902));
#84957=DIRECTION('center_axis',(0.,-1.,0.));
#84958=DIRECTION('ref_axis',(0.,0.,-1.));
#84959=DIRECTION('center_axis',(-0.154562207296368,0.987363722441907,0.0349771880135615));
#84960=DIRECTION('ref_axis',(-0.312827044980643,-0.0153275612519601,-0.949686424981818));
#84961=DIRECTION('center_axis',(0.156717592653502,0.987363725001226,-0.0235046953733427));
#84962=DIRECTION('ref_axis',(-0.240315511502135,0.0150385517052381,-0.97057833114802));
#84963=DIRECTION('',(-0.604071869369054,0.,0.796929844237858));
#84964=DIRECTION('',(-0.648440472711469,0.,-0.761265363293068));
#84965=DIRECTION('',(-0.761265364441084,0.,0.648440471363705));
#84966=DIRECTION('center_axis',(-0.15706259615762,-0.987363722513704,-0.0210765355813124));
#84967=DIRECTION('ref_axis',(0.11294374790137,0.00324330843188972,-0.993596090350806));
#84968=DIRECTION('center_axis',(0.148209482175692,-0.987363727203217,0.0560965203607491));
#84969=DIRECTION('ref_axis',(0.263014511757221,-0.0153270696763623,-0.964670123690086));
#84970=DIRECTION('',(-0.46963074398653,0.,-0.88286293630589));
#84971=DIRECTION('center_axis',(0.,-1.,0.));
#84972=DIRECTION('ref_axis',(0.,0.,-1.));
#84973=DIRECTION('center_axis',(-0.154963399384117,0.987363722388463,-0.0331545556826997));
#84974=DIRECTION('ref_axis',(0.114848845116973,-0.0153275664721359,-0.993264722257536));
#84975=DIRECTION('center_axis',(0.152102401169859,0.987363725054083,0.0444717214158533));
#84976=DIRECTION('ref_axis',(0.189430811856307,0.0150385476419998,-0.98177890056992));
#84977=DIRECTION('',(-0.882862937137393,0.,0.46963074242338));
#84978=DIRECTION('center_axis',(-0.148859727349044,-0.9873637225025,-0.0543475947910742));
#84979=DIRECTION('ref_axis',(0.323896974311614,0.00324331006221809,-0.946086798857072));
#84980=DIRECTION('center_axis',(0.132685333069044,-0.987363727208248,0.0866456726085828));
#84981=DIRECTION('ref_axis',(0.464240939393531,-0.0153270698761599,-0.885576327100055));
#84982=DIRECTION('',(-0.26886160500068,0.,-0.963178818992849));
#84983=DIRECTION('center_axis',(4.67807765707652E-14,-1.,-1.09165795252073E-13));
#84984=DIRECTION('ref_axis',(2.870235819188E-31,1.09165795252073E-13,-1.));
#84985=DIRECTION('center_axis',(-0.144213194894241,0.987363722466965,-0.0656919627852075));
#84986=DIRECTION('ref_axis',(0.325686296658284,-0.0153275579518285,-0.945353638664519));
#84987=DIRECTION('center_axis',(0.138986227524642,0.98736372509821,0.0761295141101926));
#84988=DIRECTION('ref_axis',(0.39605546709624,0.0150385439839594,-0.918103430544741));
#84989=DIRECTION('',(-0.963178819468904,-2.49350829358902E-15,0.268861603295241));
#84990=DIRECTION('center_axis',(-0.133696343123587,-0.987363722536948,-0.0850774191743116));
#84991=DIRECTION('ref_axis',(0.519705138598534,0.00324331000604487,-0.854339540144598));
#84992=DIRECTION('center_axis',(0.110956963422593,-0.987363727101881,0.113143372194397));
#84993=DIRECTION('ref_axis',(0.643759976556952,-0.0153270733983734,-0.765073965969587));
#84994=DIRECTION('',(-0.0555207965247666,0.,-0.998457530971275));
#84995=DIRECTION('center_axis',(-1.72886217674519E-14,-1.,2.41392688765716E-14));
#84996=DIRECTION('ref_axis',(5.39604775529338E-31,-2.41392688765716E-14,
-1.));
#84997=DIRECTION('center_axis',(-0.126719736909377,0.987363722443892,-0.0951577000529103));
#84998=DIRECTION('ref_axis',(0.521295021806607,-0.0153275636165744,-0.853238868098042));
#84999=DIRECTION('center_axis',(0.11937121039447,0.987363725046559,0.104227580760289));
#85000=DIRECTION('ref_axis',(0.584161008503692,0.0150385463260237,-0.81149846473567));
#85001=DIRECTION('',(-0.998457531228927,-2.49350828872853E-15,0.0555207918912913));
#85002=DIRECTION('center_axis',(-0.112281469383263,-0.987363722483312,-0.111829115873426));
#85003=DIRECTION('ref_axis',(0.691212468285046,0.00324330645825146,-0.722644314065026));
#85004=DIRECTION('center_axis',(0.0840403717824719,-0.987363727152753,0.134350609279183));
#85005=DIRECTION('ref_axis',(0.793177513644596,-0.0153270718563438,-0.608797595853407));
#85006=DIRECTION('',(0.160416105690236,0.,-0.987049478514213));
#85007=DIRECTION('center_axis',(2.2073652675844E-14,-1.,-1.9858363567774E-14));
#85008=DIRECTION('ref_axis',(1.,2.2073652675844E-14,-3.01044548961814E-31));
#85009=DIRECTION('center_axis',(-0.103301011992431,0.987363722464074,-0.120173959255853));
#85010=DIRECTION('ref_axis',(0.692528568071411,-0.0153275573522582,-0.721227598189763));
#85011=DIRECTION('center_axis',(0.0941745282129391,0.987363725059354,0.127452079907653));
#85012=DIRECTION('ref_axis',(0.744951831282862,0.0150385470532171,-0.666948732040806));
#85013=DIRECTION('',(-0.987049478230213,0.,-0.160416107437699));
#85014=DIRECTION('center_axis',(-0.0856164309490843,-0.987363722505332,
-0.133351813755776));
#85015=DIRECTION('ref_axis',(0.830399471803581,0.00324331317645552,-0.557159042058884));
#85016=DIRECTION('center_axis',(0.0531941425906414,-0.987363727074868,0.14927576377588));
#85017=DIRECTION('ref_axis',(0.905506951271153,-0.0153270746360375,-0.424054527133861));
#85018=DIRECTION('',(0.368852126985954,0.,-0.929488089443828));
#85019=DIRECTION('center_axis',(-2.5826544115284E-14,-1.,1.4648903240881E-14));
#85020=DIRECTION('ref_axis',(1.,-2.5826544115284E-14,5.41840065352129E-31));
#85021=DIRECTION('center_axis',(-0.075052037718006,0.987363722424622,-0.139571025912148));
#85022=DIRECTION('ref_axis',(0.831380248175949,-0.0153275636330696,-0.555492528064935));
#85023=DIRECTION('center_axis',(0.0645743547481768,0.98736372508055,0.144717058786852));
#85024=DIRECTION('ref_axis',(0.870909534039187,0.0150385421285242,-0.491213218236536));
#85025=DIRECTION('',(-0.929488088790823,0.,-0.368852128631492));
#85026=DIRECTION('center_axis',(-0.0549480768125023,-0.987363722501825,
-0.14863912116918));
#85027=DIRECTION('ref_axis',(0.93075791777958,0.0032433041339868,-0.365621634300973));
#85028=DIRECTION('center_axis',(0.0198606187809754,-0.987363727155474,0.157220946820986));
#85029=DIRECTION('ref_axis',(0.975495890339712,-0.0153270721634695,-0.219483140102441));
#85030=DIRECTION('',(0.560041033052935,0.,-0.828464870285398));
#85031=DIRECTION('center_axis',(0.,-1.,0.));
#85032=DIRECTION('ref_axis',(0.,0.,-1.));
#85033=DIRECTION('center_axis',(-0.0432937216744962,0.987363722469847,-0.152441901110088));
#85034=DIRECTION('ref_axis',(0.931357513590266,-0.0153275594589119,-0.363783242879591));
#85035=DIRECTION('center_axis',(0.0319547486199412,0.987363725072818,0.155215232664082));
#85036=DIRECTION('ref_axis',(0.956144474632417,0.0150385461158406,-0.292509120816121));
#85037=DIRECTION('',(-0.828464869293675,0.,-0.560041034519984));
#85038=DIRECTION('center_axis',(-0.0217103961479561,-0.987363722531891,
-0.156976234274701));
#85039=DIRECTION('ref_axis',(0.987595158629252,0.00324331204516959,-0.156988163818294));
#85040=DIRECTION('center_axis',(-0.0144015673470265,-0.987363727150147,
0.157814654472007));
#85041=DIRECTION('ref_axis',(0.999871725773331,-0.0153270717692356,-0.00464896440519302));
#85042=DIRECTION('',(0.725043043015264,0.,-0.688703554350612));
#85043=DIRECTION('center_axis',(-1.47952256911602E-13,-1.,1.22535004851514E-14));
#85044=DIRECTION('ref_axis',(1.,-1.47952256911602E-13,4.67698059803635E-31));
#85045=DIRECTION('center_axis',(-0.00951103288197081,0.987363722430219,
-0.158184765013131));
#85046=DIRECTION('ref_axis',(0.987785536274728,-0.0153275626069874,-0.155063858300302));
#85047=DIRECTION('center_axis',(-0.00215902604927871,0.987363725041648,
0.158455713303118));
#85048=DIRECTION('ref_axis',(0.996671162633965,0.0150385495453836,-0.0801276207149027));
#85049=DIRECTION('',(-0.688703551631228,0.,-0.725043045598351));
#85050=DIRECTION('center_axis',(0.0125424252946417,-0.987363722492876,-0.157973311267251));
#85051=DIRECTION('ref_axis',(0.998253547486997,0.00324330660448014,0.058985895703088));
#85052=DIRECTION('center_axis',(-0.0479903557107524,-0.987363727048957,
0.15102912390247));
#85053=DIRECTION('ref_axis',(0.977494670715387,-0.0153270753681568,0.210402589061247));
#85054=DIRECTION('',(0.856142845888465,0.,-0.51673922575512));
#85055=DIRECTION('center_axis',(-1.17701884843292E-13,-1.,-1.58706731088539E-14));
#85056=DIRECTION('ref_axis',(1.,-1.17701884843292E-13,4.44617853897246E-31));
#85057=DIRECTION('center_axis',(0.0247163783165966,0.987363722430302,-0.156531084042401));
#85058=DIRECTION('ref_axis',(0.998025805201912,-0.0153275624701153,0.0609061407396708));
#85059=DIRECTION('center_axis',(-0.0361718358223352,0.987363725075744,0.154286981621242));
#85060=DIRECTION('ref_axis',(0.990594614933057,0.0150385416996737,0.136000555620831));
#85061=DIRECTION('',(-0.516739224239438,0.,-0.85614284680328));
#85062=DIRECTION('center_axis',(0.0462087799976181,-0.987363722484958,-0.151583733203066));
#85063=DIRECTION('ref_axis',(0.962234710082633,0.00324330366222394,0.272201843663019));
#85064=DIRECTION('center_axis',(-0.0793351628521738,-0.987363727125316,
0.137181639778887));
#85065=DIRECTION('ref_axis',(0.909411050441021,-0.0153270726115122,0.415615955156824));
#85066=DIRECTION('',(0.94721036075467,0.,-0.320612745347106));
#85067=DIRECTION('center_axis',(8.36537658803244E-14,-1.,3.06015386714305E-14));
#85068=DIRECTION('ref_axis',(1.,8.36537658803244E-14,-1.22694844227837E-30));
#85069=DIRECTION('center_axis',(0.0577880795530927,0.987363722415614,-0.147558183504497));
#85070=DIRECTION('ref_axis',(0.961599496605368,-0.015327562862503,0.27402823567107));
#85071=DIRECTION('center_axis',(-0.06849329531904,0.987363725143355,0.142903963441803));
#85072=DIRECTION('ref_axis',(0.938198964110948,0.0150385380395308,0.345769498531576));
#85073=DIRECTION('',(-0.320612743670349,0.,-0.94721036132222));
#85074=DIRECTION('center_axis',(0.0777144716089803,-0.987363722534733,-0.138106264611323));
#85075=DIRECTION('ref_axis',(0.881222846599685,0.0032433098799736,0.472689935974704));
#85076=DIRECTION('center_axis',(-0.10697034869677,-0.987363727119017,0.11691969410384));
#85077=DIRECTION('ref_axis',(0.798804382014933,-0.0153270734635542,0.601395577047906));
#85078=DIRECTION('',(0.99398737210975,0.,-0.10949476739257));
#85079=DIRECTION('center_axis',(-5.00797073109942E-14,-1.,-3.1912785667902E-14));
#85080=DIRECTION('ref_axis',(1.,-5.00797073109942E-14,-1.28384215650724E-31));
#85081=DIRECTION('center_axis',(0.0881576724725291,0.987363722452936,-0.131685627036921));
#85082=DIRECTION('ref_axis',(0.880209864213759,-0.0153275610711369,0.474337075097874));
#85083=DIRECTION('center_axis',(-0.097612092652736,0.987363725102616,0.124838911079198));
#85084=DIRECTION('ref_axis',(0.841934171533672,0.0150385435014291,0.539370645301786));
#85085=DIRECTION('',(-0.109494768473299,0.,-0.9939873719907));
#85086=DIRECTION('center_axis',(0.105586311494449,-0.987363722473641,-0.118171106316189));
#85087=DIRECTION('ref_axis',(0.759005982455155,0.00324330483115373,0.65107557132107));
#85088=DIRECTION('center_axis',(-0.129603722111918,-0.987363727025109,0.0911907109842997));
#85089=DIRECTION('ref_axis',(0.650846506593612,-0.0153270770696368,0.759054613030836));
#85090=DIRECTION('',(0.994286638431596,0.,0.106743058961212));
#85091=DIRECTION('center_axis',(-4.20485661031268E-14,-1.,-4.19323393028766E-14));
#85092=DIRECTION('ref_axis',(1.,-4.20485661031268E-14,1.98718392696402E-30));
#85093=DIRECTION('center_axis',(0.114405110205379,0.987363722454575,-0.109655598760575));
#85094=DIRECTION('ref_axis',(0.757662596725444,-0.0153275579906525,0.652466440124931));
#85095=DIRECTION('center_axis',(-0.122166652612043,0.987363725061852,0.100936531650103));
#85096=DIRECTION('ref_axis',(0.706301474123408,0.0150385445990266,0.70775141810345));
#85097=DIRECTION('',(0.106743061026633,0.,-0.99428663820986));
#85098=DIRECTION('center_axis',(0.128521060442471,-0.987363722513769,-0.0927103903912335));
#85099=DIRECTION('ref_axis',(0.601298842027583,0.0032433111868436,0.799017636544297));
#85100=DIRECTION('center_axis',(-0.14617696274712,-0.987363727185108,0.0611977597723875));
#85101=DIRECTION('ref_axis',(0.472455772832713,-0.0153270698767051,0.881221098048633));
#85102=DIRECTION('',(0.9480941669185,0.,0.317989702121177));
#85103=DIRECTION('center_axis',(3.20512805188825E-14,-1.,4.9991183218023E-14));
#85104=DIRECTION('ref_axis',(9.98304756685787E-31,-4.9991183218023E-14,
-1.));
#85105=DIRECTION('center_axis',(0.135303096653766,0.987363722448722,-0.0824981916656709));
#85106=DIRECTION('ref_axis',(0.599687867911419,-0.0153275617382559,0.800087199579531));
#85107=DIRECTION('center_axis',(-0.141008833775221,0.987363725092081,0.0723144741365186));
#85108=DIRECTION('ref_axis',(0.537642905377994,0.0150385428868407,0.843038521376425));
#85109=DIRECTION('',(0.317989704666138,0.,-0.948094166064923));
#85110=DIRECTION('center_axis',(0.145446300746767,-0.987363722521415,-0.0629146489121133));
#85111=DIRECTION('ref_axis',(0.415475637959499,0.00324330610647331,0.909598524200456));
#85112=DIRECTION('center_axis',(-0.155915135243843,-0.987363727241485,0.0283432660379365));
#85113=DIRECTION('ref_axis',(0.271973531750121,-0.0153270677699031,0.962182664061737));
#85114=DIRECTION('',(0.857569866383666,0.,0.514367499236393));
#85115=DIRECTION('center_axis',(-1.02776563488674E-14,-1.,-2.78562474690747E-14));
#85116=DIRECTION('ref_axis',(-1.53922069392155E-31,2.78562474690747E-14,
-1.));
#85117=DIRECTION('center_axis',(0.149874458591521,0.987363722433168,-0.051483262181182));
#85118=DIRECTION('ref_axis',(0.413672401964247,-0.0153275633457503,0.910296770100286));
#85119=DIRECTION('center_axis',(-0.153257600591622,0.987363725089412,0.0403110684360965));
#85120=DIRECTION('ref_axis',(0.343844748655256,0.0150385450137742,0.938906082090255));
#85121=DIRECTION('',(0.514367502868879,0.,-0.857569864204913));
#85122=DIRECTION('center_axis',(0.155570636345677,-0.987363722485842,-0.0301770877637659));
#85123=DIRECTION('ref_axis',(0.210225250933983,0.00324330197631951,0.977647597481851));
#85124=DIRECTION('center_axis',(-0.158362890807331,-0.987363727153055,-0.00583653300974646));
#85125=DIRECTION('ref_axis',(0.0587741088908879,-0.0153270715028807,0.998153637975251));
#85126=DIRECTION('',(0.726946551156652,0.,0.686694045235176));
#85127=DIRECTION('center_axis',(-1.61964027106475E-14,-1.,-1.17657504934848E-13));
#85128=DIRECTION('ref_axis',(7.00547276313006E-31,1.17657504934848E-13,
-1.));
#85129=DIRECTION('center_axis',(0.157437856145186,0.987363722433385,-0.0180610374811915));
#85130=DIRECTION('ref_axis',(0.20831407392069,-0.0153275596268245,0.977941875840508));
#85131=DIRECTION('center_axis',(-0.158340210916804,0.987363725114748,0.00642276687656476));
#85132=DIRECTION('ref_axis',(0.133968796643142,0.0150385424311846,0.990871436548422));
#85133=DIRECTION('center_axis',(9.475145798617E-15,-1.,-1.18388485589748E-13));
#85134=DIRECTION('ref_axis',(3.34507738867976E-31,1.18388485589748E-13,
-1.));
#85135=DIRECTION('center_axis',(0.158420663065506,-0.987363722652752,0.00397148626897056));
#85136=DIRECTION('ref_axis',(-0.00485502709988203,0.00324326475489117,0.999982954827526));
#85137=DIRECTION('center_axis',(0.157639635277696,0.987363722413663,0.0162057104426415));
#85138=DIRECTION('ref_axis',(-0.0067847896129553,-0.015327565251928,0.99985950631744));
#85139=DIRECTION('center_axis',(-0.156019010174988,0.98736372512438,-0.0277658562361314));
#85140=DIRECTION('ref_axis',(-0.0821713885434937,0.0150385398846669,0.996504744204949));
#85141=DIRECTION('',(0.686694046522226,0.,-0.726946549940868));
#85142=DIRECTION('center_axis',(0.161633027721701,-0.986495109307913,-0.0264983709137736));
#85143=DIRECTION('ref_axis',(0.0329757751559212,-0.021437402364222,0.99922621864758));
#85144=DIRECTION('center_axis',(0.152157772461857,-0.986495109388684,-0.0606251716010378));
#85145=DIRECTION('ref_axis',(0.247008917377821,-0.0214373972602293,0.968776048803099));
#85146=DIRECTION('center_axis',(0.135567786644849,-0.986495109332269,-0.0919172154045821));
#85147=DIRECTION('ref_axis',(0.449492204001712,-0.0214374003032971,0.893026985264118));
#85148=DIRECTION('center_axis',(0.112638805325703,-0.986495109394101,-0.118911305923026));
#85149=DIRECTION('ref_axis',(0.630957728715546,-0.0214373968278044,0.775520974952559));
#85150=DIRECTION('center_axis',(0.0844429508784094,-0.986495109298641,-0.140345243513304));
#85151=DIRECTION('ref_axis',(0.782920372643902,-0.0214374043459836,0.621752465048624));
#85152=DIRECTION('center_axis',(0.0522986471423926,-0.986495109339015,-0.155216786325707));
#85153=DIRECTION('ref_axis',(0.898274530838002,-0.0214373995791351,0.438911500358616));
#85154=DIRECTION('center_axis',(0.0177089115152549,-0.986495109323431,-0.162830567566096));
#85155=DIRECTION('ref_axis',(0.971626369491964,-0.021437401334743,0.235547523722664));
#85156=DIRECTION('center_axis',(-0.0177088730347992,-0.986495109302549,
-0.162830571877608));
#85157=DIRECTION('ref_axis',(0.999546039841321,-0.0214374020191855,0.0211696016070285));
#85158=DIRECTION('center_axis',(-0.0522986060263791,-0.986495109352257,
-0.155216800095144));
#85159=DIRECTION('ref_axis',(0.980728047866526,-0.0214373990674815,-0.1941981824043));
#85160=DIRECTION('center_axis',(-0.0844429212236144,-0.986495109321542,
-0.140345261195033));
#85161=DIRECTION('ref_axis',(0.916052301958489,-0.0214374031897024,-0.400485477665591));
#85162=DIRECTION('center_axis',(-0.112638775583892,-0.986495109307086,-0.118911334817845));
#85163=DIRECTION('ref_axis',(0.808542968252034,-0.0214374034631445,-0.588046517057068));
#85164=DIRECTION('center_axis',(-0.135567764890909,-0.986495109299295,-0.091917247843127));
#85165=DIRECTION('ref_axis',(0.663227066358007,-0.0214374025783219,-0.748111152316851));
#85166=DIRECTION('center_axis',(-0.152157756514673,-0.986495109323669,-0.0606252126833621));
#85167=DIRECTION('ref_axis',(0.486899401442756,-0.0214374011196443,-0.873194944275287));
#85168=DIRECTION('center_axis',(-0.16163302008143,-0.986495109394794,-0.0264984142829452));
#85169=DIRECTION('ref_axis',(0.287804863568124,-0.0214373958016446,-0.957449110171281));
#85170=DIRECTION('center_axis',(-0.16355050573217,-0.986495109320764,0.00886743260276391));
#85171=DIRECTION('ref_axis',(0.0752528885113876,-0.0214374029907239,-0.996934020145619));
#85172=DIRECTION('center_axis',(-0.157820551393897,-0.986495109400653,0.0438186340079117));
#85173=DIRECTION('ref_axis',(-0.140817826880512,-0.0214373956793978,-0.989803403560088));
#85174=DIRECTION('center_axis',(-0.14471108034547,-0.986495109311796,0.0767209393135648));
#85175=DIRECTION('ref_axis',(-0.350304059732387,-0.0214374033023344,-0.936390678870022));
#85176=DIRECTION('center_axis',(-0.124835082058921,-0.986495109341509,0.106035850223527));
#85177=DIRECTION('ref_axis',(-0.543410459690549,-0.021437402805147,-0.839193368693935));
#85178=DIRECTION('center_axis',(-0.0991219325973794,-0.986495109282782,
0.130392644881959));
#85179=DIRECTION('ref_axis',(-0.711107593841883,-0.0214374044549463,-0.702756307457032));
#85180=DIRECTION('center_axis',(-0.0687739571027954,-0.986495109354319,
0.148652420244118));
#85181=DIRECTION('ref_axis',(-0.84555412615911,-0.0214373992962003,-0.533459143371561));
#85182=DIRECTION('center_axis',(-0.0352101828835034,-0.986495109356184,
0.159961377331033));
#85183=DIRECTION('ref_axis',(-0.940463487107214,-0.0214374005833562,-0.3392180232157));
#85184=DIRECTION('center_axis',(-2.29072636489518E-8,-0.986495109393899,
0.163790717508406));
#85185=DIRECTION('ref_axis',(-0.991397821399262,-0.0214373980985389,-0.129115443257425));
#85186=DIRECTION('center_axis',(0.0352101442534024,-0.986495109312445,0.159961386103901));
#85187=DIRECTION('ref_axis',(-0.995975494961977,-0.0214374023636677,0.0870244288412309));
#85188=DIRECTION('center_axis',(0.0687739176294749,-0.986495109353612,0.148652438511108));
#85189=DIRECTION('ref_axis',(-0.953982461632991,-0.0214373995559519,0.299095136698905));
#85190=DIRECTION('center_axis',(0.0991219030583523,-0.986495109317149,0.130392667076936));
#85191=DIRECTION('ref_axis',(-0.867382267681587,-0.0214374007047037,0.497180489925514));
#85192=DIRECTION('center_axis',(0.124835057371591,-0.986495109317044,0.106035879515309));
#85193=DIRECTION('ref_axis',(-0.740224245270894,-0.021437401580189,0.672018232287358));
#85194=DIRECTION('center_axis',(0.144711062094892,-0.986495109348447,0.0767209732665392));
#85195=DIRECTION('ref_axis',(-0.578454156478538,-0.0214373999808668,0.8154331528303));
#85196=DIRECTION('center_axis',(0.1578205394305,-0.986495109336992,0.0438186785293996));
#85197=DIRECTION('ref_axis',(-0.389636195492413,-0.0214374002396133,0.920719323699228));
#85198=DIRECTION('center_axis',(0.163550503166418,-0.986495109376726,0.00886747369963931));
#85199=DIRECTION('ref_axis',(-0.182599282568975,-0.0214373983432661,0.982953681491436));
#85200=DIRECTION('center_axis',(-0.160229046173638,0.986495109397072,-0.0339713393604832));
#85201=DIRECTION('ref_axis',(-0.0830851096497846,0.020814952117708,0.996325048527247));
#85202=DIRECTION('center_axis',(0.157123543110423,0.986495109271922,0.0462557194626253));
#85203=DIRECTION('ref_axis',(-0.18963547562865,-0.0158280458834692,0.981726978006923));
#85204=DIRECTION('center_axis',(-0.149180147486952,0.98649510939812,-0.0676216143652457));
#85205=DIRECTION('ref_axis',(-0.295323059389635,0.020814949454296,0.955170680282828));
#85206=DIRECTION('center_axis',(0.143506470660469,0.986495109262567,0.0789512018883271));
#85207=DIRECTION('ref_axis',(-0.396244184410726,-0.0158280437673955,0.918008725095342));
#85208=DIRECTION('center_axis',(-0.131155749138624,0.986495109406565,-0.0981099820854892));
#85209=DIRECTION('ref_axis',(-0.493752032498834,0.020814951281715,0.869353592162827));
#85210=DIRECTION('center_axis',(0.123179189100121,0.986495109195954,0.107955022602464));
#85211=DIRECTION('ref_axis',(-0.58432495687368,-0.0158280522011428,0.811365403217372));
#85212=DIRECTION('center_axis',(-0.106998655213202,0.986495109384959,-0.124010833970759));
#85213=DIRECTION('ref_axis',(-0.669093708611319,0.0208149505950684,0.742886496665861));
#85214=DIRECTION('center_axis',(0.097092189150081,0.986495109219769,0.131910978661827));
#85215=DIRECTION('ref_axis',(-0.745083340957672,-0.0158280526239247,0.666783538922106));
#85216=DIRECTION('center_axis',(-0.0778384228895612,0.986495109391339,-0.144113077369946));
#85217=DIRECTION('ref_axis',(-0.8131493056209,0.0208149504930532,0.581682855690469));
#85218=DIRECTION('center_axis',(0.066465272464082,0.986495109238995,0.149698921184551));
#85219=DIRECTION('ref_axis',(-0.871002456793015,-0.0158280462852299,0.491023617773447));
#85220=DIRECTION('center_axis',(-0.0450385516176566,0.986495109416014,-0.15747675373359));
#85221=DIRECTION('ref_axis',(-0.919182947471826,0.0208149504743908,0.393280366804337));
#85222=DIRECTION('center_axis',(0.0327305050275662,0.986495109232261,0.160487113194395));
#85223=DIRECTION('ref_axis',(-0.956194466999986,-0.0158280494827267,0.292303975560005));
#85224=DIRECTION('center_axis',(-0.0101327330925777,0.986495109448707,-0.163476991512135));
#85225=DIRECTION('ref_axis',(-0.982236614171915,0.0208149459504699,0.186488529956059));
#85226=DIRECTION('center_axis',(-0.00253469703033147,0.986495109264329,
0.163771104620211));
#85227=DIRECTION('ref_axis',(-0.996675886002857,-0.0158280452887455,0.079916526718559));
#85228=DIRECTION('center_axis',(0.0252468874683863,0.986495109426824,-0.161833228201498));
#85229=DIRECTION('ref_axis',(-0.9993619893109,0.02081494807157,-0.029023305417169));
#85230=DIRECTION('center_axis',(-0.037681384372286,0.986495109269882,0.159397342068155));
#85231=DIRECTION('ref_axis',(-0.990553848653424,-0.0158280461198542,-0.136207730595283));
#85232=DIRECTION('center_axis',(0.0594459888264633,0.986495109421206,-0.15262232307394));
#85233=DIRECTION('ref_axis',(-0.969758308850799,0.0208149474045697,-0.24317804255192));
#85234=DIRECTION('center_axis',(-0.0710661339837401,0.986495109226173,0.14757033602132));
#85235=DIRECTION('ref_axis',(-0.938114613916673,-0.015828048803026,-0.345963067432148));
#85236=DIRECTION('center_axis',(0.0908654631635529,0.98649510941151,-0.136274967294975));
#85237=DIRECTION('ref_axis',(-0.894809806919867,0.0208149477677228,-0.44596204702806));
#85238=DIRECTION('center_axis',(-0.101127910663473,0.986495109187203,0.128843103170366));
#85239=DIRECTION('ref_axis',(-0.841810182221258,-0.0158280527582371,-0.539541555261961));
#85240=DIRECTION('center_axis',(0.118036168935702,0.986495109427504,-0.113555545433062));
#85241=DIRECTION('ref_axis',(-0.778020993295535,0.0208149479903139,-0.627893360318128));
#85242=DIRECTION('center_axis',(-0.126461053175876,0.986495109247567,0.104091313087494));
#85243=DIRECTION('ref_axis',(-0.706143642576749,-0.0158280504594505,-0.70789167876667));
#85244=DIRECTION('center_axis',(0.139687634455818,0.98649510944765,-0.0855263925113603));
#85245=DIRECTION('ref_axis',(-0.624852784076839,0.0208149483880809,-0.780465076832413));
#85246=DIRECTION('center_axis',(-0.145881020994131,0.986495109214407,0.074472325126622));
#85247=DIRECTION('ref_axis',(-0.537458610002052,-0.0158280534109935,-0.843141574861471));
#85248=DIRECTION('center_axis',(0.154807460829294,0.986495109447023,-0.0534981224782106));
#85249=DIRECTION('ref_axis',(-0.442467151133643,0.0208149463326911,-0.896543115626262));
#85250=DIRECTION('center_axis',(-0.158479752553331,0.986495109210154,0.0413710954058669));
#85251=DIRECTION('ref_axis',(-0.343642610869599,-0.0158280543008508,-0.938967107353487));
#85252=DIRECTION('center_axis',(0.162688663350698,0.986495109444919,-0.018968338314703));
#85253=DIRECTION('ref_axis',(-0.239392246518749,0.0208149460742025,-0.970699794131344));
#85254=DIRECTION('center_axis',(-0.163668146516347,0.986495109199942,0.0063354037359762));
#85255=DIRECTION('ref_axis',(-0.133758266319021,-0.0158280507412877,-0.99088758141429));
#85256=DIRECTION('center_axis',(0.16296272472669,0.986495109485003,0.0164483832587217));
#85257=DIRECTION('ref_axis',(-0.025123626692503,0.0208149448285755,-0.999467629017368));
#85258=DIRECTION('center_axis',(-0.161203600904315,0.986495109252866,-0.0289965252342124));
#85259=DIRECTION('ref_axis',(0.0823804677645385,-0.0158280478511732,-0.996475253798165));
#85260=DIRECTION('center_axis',(0.155616830226651,0.986495109422284,0.0510960001969397));
#85261=DIRECTION('ref_axis',(0.190319746929274,0.0208149470435386,-0.981501468113192));
#85262=DIRECTION('center_axis',(-0.151201354025936,0.986495109218322,-0.0629726133256001));
#85263=DIRECTION('ref_axis',(0.294667181714052,-0.015828049706957,-0.955468850807378));
#85264=DIRECTION('center_axis',(0.140994463552116,0.986495109354395,0.0833544268021333));
#85265=DIRECTION('ref_axis',(0.39686397774258,0.0208149520937682,-0.917641390162667));
#85266=DIRECTION('center_axis',(-0.134129102511911,0.986495109263272,-0.0940041661789216));
#85267=DIRECTION('ref_axis',(0.493175586742465,-0.0158280447577772,-0.869785786064805));
#85268=DIRECTION('center_axis',(0.11977935520278,0.986495109416186,0.111715286174963));
#85269=DIRECTION('ref_axis',(0.584851292792108,0.0208149490328238,-0.810873419971429));
#85270=DIRECTION('center_axis',(-0.110785115663833,0.986495109186654,-0.12064019934567));
#85271=DIRECTION('ref_axis',(0.668623649731056,-0.0158280532216668,-0.743432503830398));
#85272=DIRECTION('center_axis',(0.0929634964319924,0.986495109410282,0.134852465460354));
#85273=DIRECTION('ref_axis',(0.74549160979465,0.0208149489752835,-0.66618991108012));
#85274=DIRECTION('center_axis',(-0.0822609475935,0.986495109233674,-0.14163522146366));
#85275=DIRECTION('ref_axis',(0.812807611767165,-0.0158280497325542,-0.58231714648894));
#85276=DIRECTION('center_axis',(0.0618007681567064,0.986495109400869,0.151684093376358));
#85277=DIRECTION('ref_axis',(0.871273569082446,0.0208149483613273,-0.490356100954247));
#85278=DIRECTION('center_axis',(-0.0498903480221808,0.986495109248187,-0.156007540214033));
#85279=DIRECTION('ref_axis',(0.918985594304392,-0.0158280482471485,-0.393973286340191));
#85280=DIRECTION('center_axis',(0.0277483075383048,0.986495109427382,0.161423141168227));
#85281=DIRECTION('ref_axis',(0.956315744374027,0.0208149448057552,-0.291593784458935));
#85282=DIRECTION('center_axis',(-0.0151869309708522,0.986495109262656,-0.163085120500148));
#85283=DIRECTION('ref_axis',(0.982192832897511,-0.015828046811078,-0.187207670619844));
#85284=DIRECTION('center_axis',(-0.00760163979730092,0.98649510939943,0.163614223719695));
#85285=DIRECTION('ref_axis',(0.996641657828032,0.0208149484683471,-0.0791968673752444));
#85286=DIRECTION('center_axis',(0.0202266118953025,0.986495109261528,-0.162537022165174));
#85287=DIRECTION('ref_axis',(0.999473825620694,-0.0158280474677465,0.0283115667615459));
#85288=DIRECTION('center_axis',(-0.0425961376215212,0.986495109425181,0.158154886550903));
#85289=DIRECTION('ref_axis',(0.990365715286638,0.0208149467752881,0.136903206593304));
#85290=DIRECTION('center_axis',(0.0546943881994909,0.986495109174822,-0.154388870951374));
#85291=DIRECTION('ref_axis',(0.970020532949181,-0.0158280559788013,0.24250698608683));
#85292=DIRECTION('center_axis',(-0.0755988898492081,0.986495109447872,0.14530040223275));
#85293=DIRECTION('ref_axis',(0.937781371961546,0.0208149472751966,0.34660184127014));
#85294=DIRECTION('center_axis',(0.0866047015303078,0.986495109243973,-0.139021671370213));
#85295=DIRECTION('ref_axis',(0.895210158480271,-0.0158280492832253,0.44536304854536));
#85296=DIRECTION('center_axis',(-0.105066720103058,0.986495109422893,0.12565183409525));
#85297=DIRECTION('ref_axis',(0.841347414505468,0.0208149457481815,0.54009375680382));
#85298=DIRECTION('center_axis',(0.114465482555487,0.986495109200375,-0.117153970598861));
#85299=DIRECTION('ref_axis',(0.778540752379732,-0.0158280504998284,0.62739442912842));
#85300=DIRECTION('center_axis',(-0.129621752543377,0.986495109404068,0.100127920129402));
#85301=DIRECTION('ref_axis',(0.705572987566036,0.0208149521856119,0.70833148806378));
#85302=DIRECTION('center_axis',(0.13697398323435,0.986495109207171,-0.0898082815070361));
#85303=DIRECTION('ref_axis',(0.6254676446499,-0.015828049283185,0.780089545085688));
#85304=DIRECTION('center_axis',(-0.148115809468914,0.986495109426496,0.0699221428660026));
#85305=DIRECTION('ref_axis',(0.536806752086055,0.0208149488146366,0.843448426888488));
#85306=DIRECTION('center_axis',(0.153077736248759,0.986495109159638,-0.0582632497297413));
#85307=DIRECTION('ref_axis',(0.443148364745263,-0.015828056351047,0.896308540322889));
#85308=DIRECTION('center_axis',(-0.159684136636216,0.986495109476762,0.0364468858090491));
#85309=DIRECTION('ref_axis',(0.342940027684309,0.0208149437938576,0.939126655742847));
#85310=DIRECTION('center_axis',(0.16202373838693,0.986495109239524,-0.0239939085107565));
#85311=DIRECTION('ref_axis',(0.240107962164591,-0.0158280467462338,0.970617143595437));
#85312=DIRECTION('center_axis',(-0.163785813527936,0.986495109450472,0.00126740573369946));
#85313=DIRECTION('ref_axis',(0.133037809399803,0.0208149467552055,0.990892365124326));
#85314=DIRECTION('center_axis',(0.163393698449405,0.986495108418207,0.0113973845234563));
#85315=DIRECTION('ref_axis',(0.0258403863850521,-0.0158280630558587,0.999540767978661));
#85316=DIRECTION('center_axis',(-0.155457916630874,0.987363722298953,0.0307524965611573));
#85317=DIRECTION('ref_axis',(0.138178875923994,-0.00909007846864055,0.990365573271716));
#85318=DIRECTION('',(-0.727623861284462,0.,-0.68597632356335));
#85319=DIRECTION('center_axis',(-1.12148479625166E-14,-1.,-8.08785086650414E-14));
#85320=DIRECTION('ref_axis',(1.2877591139289E-31,8.08785086650414E-14,-1.));
#85321=DIRECTION('center_axis',(-0.153257680235064,-0.987363721873262,0.0403108444161852));
#85322=DIRECTION('ref_axis',(0.0669565413129348,0.0303233739208332,0.997294998768903));
#85323=DIRECTION('center_axis',(0.149059810413061,-0.987363723002569,-0.0537963885231106));
#85324=DIRECTION('ref_axis',(0.14224023693335,-0.0324282815239169,0.989300824600157));
#85325=DIRECTION('',(-0.513520954857275,0.,0.858077053021739));
#85326=DIRECTION('center_axis',(-0.145212520775725,0.987363722362003,0.0634523724805455));
#85327=DIRECTION('ref_axis',(0.347847652333208,-0.00909007383497536,0.937507003346615));
#85328=DIRECTION('',(-0.858077052117147,0.,-0.513520956368819));
#85329=DIRECTION('center_axis',(0.,-1.,0.));
#85330=DIRECTION('ref_axis',(0.,0.,-1.));
#85331=DIRECTION('center_axis',(-0.141008960123313,-0.987363721799518,0.0723142727208516));
#85332=DIRECTION('ref_axis',(0.279780078968391,0.0303233766047821,0.959585118811107));
#85333=DIRECTION('center_axis',(0.134010239664075,-0.98736372285364,-0.0845821166546276));
#85334=DIRECTION('ref_axis',(0.351585171224556,-0.0324282869747367,0.935594075215787));
#85335=DIRECTION('',(-0.317053919406352,0.,0.948407513777211));
#85336=DIRECTION('center_axis',(-0.128177146769656,0.987363722305179,0.0931852934837393));
#85337=DIRECTION('ref_axis',(0.541251461767044,-0.00909007676524374,0.84081164694564));
#85338=DIRECTION('',(-0.948407514082987,0.,-0.317053918491681));
#85339=DIRECTION('center_axis',(6.01886246066096E-14,-1.,9.36741191559153E-14));
#85340=DIRECTION('ref_axis',(-5.70917302974635E-32,-9.36741191559153E-14,
-1.));
#85341=DIRECTION('center_axis',(-0.122166815496601,-0.987363721684859,0.100936367539379));
#85342=DIRECTION('ref_axis',(0.479521412833519,0.0303233812058827,0.877006104417973));
#85343=DIRECTION('center_axis',(0.112694502133529,-0.987363722956722,-0.111412870791117));
#85344=DIRECTION('ref_axis',(0.5444903757614,-0.032428282988734,0.838139986616563));
#85345=DIRECTION('',(-0.105761793778192,0.,0.994391493817611));
#85346=DIRECTION('center_axis',(-0.105148352898413,0.987363722309484,0.118560970601255));
#85347=DIRECTION('ref_axis',(0.709346952146409,-0.00909007678427596,0.704800873995383));
#85348=DIRECTION('',(-0.99439149393359,0.,-0.105761792687731));
#85349=DIRECTION('center_axis',(2.63062048809266E-14,-1.,2.61817650590162E-14));
#85350=DIRECTION('ref_axis',(1.,2.63062048809266E-14,9.86486506770613E-32));
#85351=DIRECTION('center_axis',(-0.0976122912519061,-0.987363721798348,
0.1248387819272));
#85352=DIRECTION('ref_axis',(0.656840855817275,0.0303233765312807,0.753419261079096));
#85353=DIRECTION('center_axis',(0.0861092934143021,-0.987363722975803,-0.133034086380336));
#85354=DIRECTION('ref_axis',(0.711935815224303,-0.0324282828974503,0.70149540374063));
#85355=DIRECTION('',(0.110475636308035,0.,0.993878832545665));
#85356=DIRECTION('center_axis',(-0.0772029402071325,0.987363722355735,0.138392867587899));
#85357=DIRECTION('ref_axis',(0.844274169030345,-0.00909007489063781,0.53583439423632));
#85358=DIRECTION('',(-0.993878832740016,0.,0.110475634559585));
#85359=DIRECTION('center_axis',(-7.51667662639805E-14,-1.,-4.77950243231242E-14));
#85360=DIRECTION('ref_axis',(1.,-7.51667662639805E-14,2.19109677680993E-31));
#85361=DIRECTION('center_axis',(-0.0684935240125511,-0.987363721860461,
0.142903876512153));
#85362=DIRECTION('ref_axis',(0.803447151474661,0.0303233744073822,0.594603370114737));
#85363=DIRECTION('center_axis',(0.0554977124764765,-0.987363723067244,-0.14843477449934));
#85364=DIRECTION('ref_axis',(0.846091927685473,-0.0324282797104404,0.532049674918143));
#85365=DIRECTION('',(0.321547346824495,0.,0.946893501799504));
#85366=DIRECTION('center_axis',(-0.0456476012935844,0.987363722316211,0.151753669972159));
#85367=DIRECTION('ref_axis',(0.939724063897283,-0.00909007638497098,0.341812893618263));
#85368=DIRECTION('',(-0.946893502365445,0.,0.32154734515791));
#85369=DIRECTION('center_axis',(-2.09209816216792E-14,-1.,-7.62974259781717E-15));
#85370=DIRECTION('ref_axis',(1.,-2.09209816216792E-14,8.65847740393996E-32));
#85371=DIRECTION('center_axis',(-0.0361720699851638,-0.98736372173205,0.15428694812078));
#85372=DIRECTION('ref_axis',(0.912485152557324,0.0303233787472675,0.407984483851759));
#85373=DIRECTION('center_axis',(0.0222911163563204,-0.987363723032363,-0.156894820090594));
#85374=DIRECTION('ref_axis',(0.940685720889932,-0.0324282816366707,0.337725896347736));
#85375=DIRECTION('',(0.517583861605946,0.,0.855632483140441));
#85376=DIRECTION('center_axis',(-0.011957828115349,0.987363722256829,0.158018639147103));
#85377=DIRECTION('ref_axis',(0.991233505649836,-0.00909008090717694,0.1318086025502));
#85378=DIRECTION('',(-0.85563248405198,0.,0.517583860099056));
#85379=DIRECTION('center_axis',(-7.35734327801556E-15,-1.,-9.84656943244725E-16));
#85380=DIRECTION('ref_axis',(1.,-7.35734327801556E-15,-1.3470661391192E-32));
#85381=DIRECTION('center_axis',(-0.00215925495983984,-0.987363721794488,
0.158455730417539));
#85382=DIRECTION('ref_axis',(0.978856360877033,0.0303233776589315,0.202288698492838));
#85383=DIRECTION('center_axis',(-0.0119577902699399,-0.987363722876836,
-0.158018638136943));
#85384=DIRECTION('ref_axis',(0.9912940961874,-0.0324282856353993,0.127610427296341));
#85385=DIRECTION('',(0.689418728599909,0.,0.724363042027743));
#85386=DIRECTION('center_axis',(0.022291069413263,0.987363722349427,0.156894831057929));
#85387=DIRECTION('ref_axis',(0.996393970420733,-0.00909007440818482,-0.0843589133195836));
#85388=DIRECTION('',(-0.724363041876131,0.,0.689418728759206));
#85389=DIRECTION('center_axis',(-6.65730432814955E-14,-1.,5.57977600812412E-15));
#85390=DIRECTION('ref_axis',(1.,-6.65730432814955E-14,-6.37552911105267E-32));
#85391=DIRECTION('center_axis',(0.0319545255018942,-0.987363721775575,0.155215299572671));
#85392=DIRECTION('ref_axis',(0.999457333683558,0.0303233778893256,-0.0128658812187456));
#85393=DIRECTION('center_axis',(-0.0456475581498333,-0.987363722973715,
-0.151753678671865));
#85394=DIRECTION('ref_axis',(0.99555066093659,-0.0324282838992063,-0.0884719611632503));
#85395=DIRECTION('',(0.829017145402445,0.,0.559223186776784));
#85396=DIRECTION('center_axis',(0.0554976664419892,0.987363722365212,0.148434796380787));
#85397=DIRECTION('ref_axis',(0.954964160800323,-0.00909007353095526,-0.296581897880058));
#85398=DIRECTION('',(-0.559223188237572,0.,0.829017144417053));
#85399=DIRECTION('center_axis',(-1.13452649964229E-13,-1.,3.51298850837732E-14));
#85400=DIRECTION('ref_axis',(1.,-1.13452649964229E-13,6.09375410996373E-32));
#85401=DIRECTION('center_axis',(0.0645741449693705,-0.987363721836154,0.144717174527881));
#85402=DIRECTION('ref_axis',(0.973324792786892,0.0303233751357475,-0.227418866118733));
#85403=DIRECTION('center_axis',(-0.0772028993465973,-0.987363722956117,
-0.138392886098657));
#85404=DIRECTION('ref_axis',(0.953256383221609,-0.0324282845561554,-0.300417499836481));
#85405=DIRECTION('',(0.929851640370812,0.,0.367934677490054));
#85406=DIRECTION('center_axis',(0.0861092603282511,0.987363722268804,0.133034113043285));
#85407=DIRECTION('ref_axis',(0.868881288000507,-0.00909007908539792,-0.494937044304426));
#85408=DIRECTION('',(-0.367934678144954,0.,0.929851640111673));
#85409=DIRECTION('center_axis',(-4.51711327338588E-14,-1.,2.56801711754637E-14));
#85410=DIRECTION('ref_axis',(1.,-4.51711327338588E-14,2.69596667039635E-31));
#85411=DIRECTION('center_axis',(0.0941743527967696,-0.987363721783213,0.127452234902771));
#85412=DIRECTION('ref_axis',(0.901680666214819,0.0303233758618026,-0.431337998616797));
#85413=DIRECTION('center_axis',(-0.105148313696102,-0.987363723085985,-0.118560998902036));
#85414=DIRECTION('ref_axis',(0.866388897096936,-0.0324282793889344,-0.498315849319514));
#85415=DIRECTION('',(0.987207304850248,0.,0.159441955740358));
#85416=DIRECTION('center_axis',(0.112694470843253,0.987363722358728,0.111412907740871));
#85417=DIRECTION('ref_axis',(0.742170492605667,-0.00909007302830182,-0.670149483680919));
#85418=DIRECTION('',(-0.159441954225668,0.,0.987207305094882));
#85419=DIRECTION('center_axis',(2.20540451644059E-14,-1.,-1.98801378983789E-14));
#85420=DIRECTION('ref_axis',(1.,2.20540451644059E-14,-1.16398971375676E-31));
#85421=DIRECTION('center_axis',(0.119371070808828,-0.987363721830502,0.104227771092797));
#85422=DIRECTION('ref_axis',(0.787874952879634,0.0303233743726265,-0.615088246995154));
#85423=DIRECTION('center_axis',(-0.128177111842097,-0.987363723177813,-0.0931853322807025));
#85424=DIRECTION('ref_axis',(0.73901002942784,-0.0324282754283277,-0.672913503622723));
#85425=DIRECTION('',(0.998402253875163,0.,-0.0565061010599261));
#85426=DIRECTION('center_axis',(0.134010221267995,0.98736372231437,0.0845821520961454));
#85427=DIRECTION('ref_axis',(0.580756628251935,-0.00909007750398461,-0.814026479441802));
#85428=DIRECTION('',(0.0565060964350291,0.,0.998402254136916));
#85429=DIRECTION('center_axis',(-3.88457816059066E-14,-1.,5.43517179396169E-14));
#85430=DIRECTION('ref_axis',(1.14632904336126E-31,-5.43517179396169E-14,
-1.));
#85431=DIRECTION('center_axis',(0.138986130481117,-0.987363721883336,0.0761297329732144));
#85432=DIRECTION('ref_axis',(0.637229084006982,0.0303233733069723,-0.770077650322946));
#85433=DIRECTION('center_axis',(-0.145212496255406,-0.987363723096613,-0.0634524171649051));
#85434=DIRECTION('ref_axis',(0.577075873870543,-0.0324282798070519,-0.816046470775595));
#85435=DIRECTION('',(0.962913022721775,0.,-0.26981199134363));
#85436=DIRECTION('center_axis',(0.149059797608916,0.98736372234626,0.0537964360466986));
#85437=DIRECTION('ref_axis',(0.392187231442824,-0.00909007338534998,-0.919840500336369));
#85438=DIRECTION('',(0.26981198698136,0.,0.9629130239441));
#85439=DIRECTION('center_axis',(1.45853200714515E-14,-1.,-3.41287221346288E-14));
#85440=DIRECTION('ref_axis',(-1.8222568904173E-31,3.41287221346288E-14,
-1.));
#85441=DIRECTION('center_axis',(0.152102354641146,-0.987363721845998,0.0444719517790476));
#85442=DIRECTION('ref_axis',(0.456787090216585,0.0303233740596595,-0.889059079700052));
#85443=DIRECTION('center_axis',(-0.15545790539908,-0.987363722888087,-0.0307525344241499));
#85444=DIRECTION('ref_axis',(0.388158288051228,-0.032428286051492,-0.921022013678773));
#85445=DIRECTION('',(0.88239904984541,0.,-0.470501771337704));
#85446=DIRECTION('center_axis',(0.157139506714322,0.987363722300695,0.0204952510132345));
#85447=DIRECTION('ref_axis',(0.185279594329072,-0.00909007741256787,-0.98264380241158));
#85448=DIRECTION('',(0.470501770976394,0.,0.882399050038064));
#85449=DIRECTION('center_axis',(-2.21045022981612E-14,-1.,1.1669191756339E-13));
#85450=DIRECTION('ref_axis',(-6.30364264290393E-32,-1.1669191756339E-13,
-1.));
#85451=DIRECTION('center_axis',(0.158106441959231,-0.987363721757333,0.0107347085894193));
#85452=DIRECTION('ref_axis',(0.254986240945197,0.0303233778593733,-0.96646909401379));
#85453=DIRECTION('center_axis',(-0.158434270677612,-0.987363723095218,0.00338529029809263));
#85454=DIRECTION('ref_axis',(0.18109085788381,-0.0324282794849182,-0.982931588606528));
#85455=DIRECTION('',(0.760625076895703,0.,-0.64919141429736));
#85456=DIRECTION('',(0.649191412957105,0.,0.760625078039607));
#85457=DIRECTION('',(0.603285121269556,0.,-0.797525587335464));
#85458=DIRECTION('center_axis',(0.151221686215521,0.987363722343238,-0.047380179596961));
#85459=DIRECTION('ref_axis',(-0.244446218187792,-0.00909007671548458,-0.969620243661916));
#85460=DIRECTION('',(0.797525585226132,0.,0.603285124058033));
#85461=DIRECTION('center_axis',(-1.80851008879526E-15,-1.,-7.19925971614798E-15));
#85462=DIRECTION('ref_axis',(2.8446207780274E-34,7.19925971614798E-15,-1.));
#85463=DIRECTION('center_axis',(0.148000906469275,-0.987363721718874,-0.0566446177295607));
#85464=DIRECTION('ref_axis',(-0.174390597605054,0.0303233811261436,-0.984209536645541));
#85465=DIRECTION('center_axis',(-0.142369603550533,-0.987363723128967,0.0695972286356919));
#85466=DIRECTION('ref_axis',(-0.24836864875715,-0.0324282784717592,-0.968122627082905));
#85467=DIRECTION('',(0.41773622273295,0.,-0.908568350877801));
#85468=DIRECTION('center_axis',(0.137500868255779,0.987363722269032,-0.0787806522945108));
#85469=DIRECTION('ref_axis',(-0.447170891372606,-0.00909007952360674,-0.894402350378891));
#85470=DIRECTION('',(0.908568350643389,0.,0.417736223242793));
#85471=DIRECTION('center_axis',(4.63939863213034E-14,-1.,9.29903636253066E-14));
#85472=DIRECTION('ref_axis',(4.26143284160394E-31,-9.29903636253066E-14,
-1.));
#85473=DIRECTION('center_axis',(0.132363810189427,-0.987363721735688,-0.0871361162342473));
#85474=DIRECTION('ref_axis',(-0.381889396612541,0.0303233795313162,-0.923710442405362));
#85475=DIRECTION('center_axis',(-0.124079731074172,-0.987363722900472,0.0985753470025941));
#85476=DIRECTION('ref_axis',(-0.450679678382106,-0.0324282853365217,-0.892096538387822));
#85477=DIRECTION('',(0.212654444280544,0.,-0.977127467287525));
#85478=DIRECTION('center_axis',(0.11735066527046,0.987363722331918,-0.10649742336526));
#85479=DIRECTION('ref_axis',(-0.628986351769033,-0.0090900753738975,-0.777363196850725));
#85480=DIRECTION('',(0.977127466912818,0.,0.212654446002285));
#85481=DIRECTION('center_axis',(5.59710000100304E-14,-1.,6.92939698404936E-14));
#85482=DIRECTION('ref_axis',(-4.60810629483416E-31,-6.92939698404935E-14,
-1.));
#85483=DIRECTION('center_axis',(0.110537530305549,-0.987363721828821,-0.11355322633148));
#85484=DIRECTION('ref_axis',(-0.571531475732816,0.0303233763923442,-0.82001967359987));
#85485=DIRECTION('center_axis',(-0.0999880321937499,-0.98736372299158,0.122944182205695));
#85486=DIRECTION('ref_axis',(-0.631917422190177,-0.0324282824640613,-0.774357009414232));
#85487=DIRECTION('',(-0.00237082103812565,0.,-0.999997189599853));
#85488=DIRECTION('center_axis',(0.0917132760761384,0.987363722355005,-0.129234495273713));
#85489=DIRECTION('ref_axis',(-0.781391109084285,-0.00909007261383878,-0.623975404342116));
#85490=DIRECTION('',(0.999997189610847,0.,-0.00237081640126621));
#85491=DIRECTION('center_axis',(1.15930973899852E-14,-1.,9.27363413703666E-15));
#85492=DIRECTION('ref_axis',(1.,1.15930973899852E-14,5.91510523815103E-33));
#85493=DIRECTION('center_axis',(0.0835426346946244,-0.987363721744513,-0.134660718738259));
#85494=DIRECTION('ref_axis',(-0.734449379788685,0.0303233792619161,-0.677985693948002));
#85495=DIRECTION('center_axis',(-0.0712210092508804,-0.987363723228234,
0.141564281844558));
#85496=DIRECTION('ref_axis',(-0.783607409986975,-0.0324282744047808,-0.620409408401124));
#85497=DIRECTION('',(-0.21728522775494,0.,-0.976108154765385));
#85498=DIRECTION('center_axis',(0.0617874731962761,0.987363722349567,-0.145928708429927));
#85499=DIRECTION('ref_axis',(-0.89725888607618,-0.00909007401268137,-0.441411216341154));
#85500=DIRECTION('',(0.976108155148254,-9.35065609140375E-15,-0.217285226034981));
#85501=DIRECTION('center_axis',(-7.98936867010663E-14,-1.,-3.93878909193784E-14));
#85502=DIRECTION('ref_axis',(1.,-7.98936867010663E-14,-3.8090581129996E-31));
#85503=DIRECTION('center_axis',(0.0526413862943957,-0.987363721871389,-0.149471619986147));
#85504=DIRECTION('ref_axis',(-0.863025242613456,0.0303233731980806,-0.504249862320135));
#85505=DIRECTION('center_axis',(-0.0391237546118326,-0.98736372289731,0.153565004253697));
#85506=DIRECTION('ref_axis',(-0.898656789348412,-0.0324282859703908,-0.437452147356745));
#85507=DIRECTION('',(-0.422039619688627,0.,-0.906577387437542));
#85508=DIRECTION('center_axis',(0.0289725558770176,0.987363722280623,-0.155799457412744));
#85509=DIRECTION('ref_axis',(-0.97117183573339,-0.00909007579519604,-0.238207128357393));
#85510=DIRECTION('',(0.906577388181206,-9.35065607453509E-15,-0.422039618091173));
#85511=DIRECTION('',(-0.607059907517467,0.,-0.794656069431855));
#85512=DIRECTION('center_axis',(-3.60387703961403E-14,-1.,-8.87176788160941E-15));
#85513=DIRECTION('ref_axis',(1.,-3.60387703961403E-14,-1.27276260034576E-31));
#85514=DIRECTION('center_axis',(0.0192786812813638,-0.987363721912874,-0.157293398139934));
#85515=DIRECTION('ref_axis',(-0.951247007159819,0.03032337171749,-0.306935863817135));
#85516=DIRECTION('center_axis',(-0.00519712986202774,-0.987363722957762,
0.158385190053192));
#85517=DIRECTION('ref_axis',(-0.97168597329991,-0.0324282827858379,-0.234040115723286));
#85518=DIRECTION('',(0.794656070501523,0.,-0.607059906117246));
#85519=DIRECTION('center_axis',(-0.00519708766551451,0.987363722313707,
-0.15838519545279));
#85520=DIRECTION('ref_axis',(-0.999673869137803,-0.0090900790429132,-0.0238647402258607));
#85521=DIRECTION('center_axis',(4.45240460760042E-14,-1.,1.10049664697024E-15));
#85522=DIRECTION('ref_axis',(-0.999694677173031,-4.45376444353329E-14,-0.0247093591966371));
#85523=DIRECTION('center_axis',(-0.0149854786284753,-0.987363721847574,
-0.157760312530061));
#85524=DIRECTION('ref_axis',(-0.994989518555826,0.0303233755014844,-0.095269884340445));
#85525=DIRECTION('center_axis',(0.0289725116530487,-0.987363722953917,0.155799461369719));
#85526=DIRECTION('ref_axis',(-0.999280201885406,-0.0324282842135005,-0.0196846260526198));
#85527=DIRECTION('',(-0.763694749702693,0.,-0.645577516086597));
#85528=DIRECTION('center_axis',(-0.0391237164597122,0.987363722286895,-0.153565017898441));
#85529=DIRECTION('ref_axis',(-0.981432263325734,-0.0090900775719372,0.191593535885382));
#85530=DIRECTION('',(0.645577518758643,0.,-0.763694747443921));
#85531=DIRECTION('center_axis',(7.28661215438116E-15,-1.,-1.41609769132671E-15));
#85532=DIRECTION('ref_axis',(1.,7.28661215438116E-15,1.09542984455334E-33));
#85533=DIRECTION('center_axis',(-0.048548929510468,-0.987363721854955,-0.150850529359757));
#85534=DIRECTION('ref_axis',(-0.992207425625152,0.0303233748037648,0.120850806678399));
#85535=DIRECTION('center_axis',(0.0617874283044647,-0.987363722959389,0.1459287233114));
#85536=DIRECTION('ref_axis',(-0.980149198894436,-0.0324282832786011,0.195591294157482));
#85537=DIRECTION('',(-0.884620074177392,0.,-0.466312475023332));
#85538=DIRECTION('center_axis',(-0.0712209641420276,0.987363722345124,-0.141564310698214));
#85539=DIRECTION('ref_axis',(-0.917299976199164,-0.0090900767457838,0.398093109925014));
#85540=DIRECTION('',(0.466312478831761,0.,-0.884620072169843));
#85541=DIRECTION('center_axis',(4.08710163910781E-14,-1.,-1.76963780131983E-14));
#85542=DIRECTION('ref_axis',(1.,4.08710163910781E-14,-1.88174897648644E-31));
#85543=DIRECTION('center_axis',(-0.0798422872074384,-0.987363721854571,
-0.136887143074045));
#85544=DIRECTION('ref_axis',(-0.943030816223802,0.0303233747598678,0.331320649213783));
#85545=DIRECTION('center_axis',(0.0917132337652694,-0.987363722983189,0.129234520500883));
#85546=DIRECTION('ref_axis',(-0.915187508710007,-0.0324282825088845,0.40172158318255));
#85547=DIRECTION('',(-0.964181545972515,0.,-0.265243183524199));
#85548=DIRECTION('center_axis',(-0.0999879970270678,0.987363722361799,-0.122944215863811));
#85549=DIRECTION('ref_axis',(-0.810275761337678,-0.00909007322328466,0.585978294100934));
#85550=DIRECTION('',(0.265243185223135,0.,-0.964181545505143));
#85551=DIRECTION('center_axis',(-6.01854610169138E-15,-1.,4.34478449126022E-15));
#85552=DIRECTION('ref_axis',(1.,-6.01854610169138E-15,2.10202917262272E-32));
#85553=DIRECTION('center_axis',(-0.107402309026535,-0.987363721829395,-0.116523065660722));
#85554=DIRECTION('ref_axis',(-0.849759133394177,0.0303233754483682,0.526298307155356));
#85555=DIRECTION('center_axis',(0.117350631392854,-0.987363722976456,0.106497454719681));
#85556=DIRECTION('ref_axis',(-0.807432667974151,-0.0324282829819871,0.589067817106812));
#85557=DIRECTION('',(-0.998658961195706,0.,-0.0517714131882922));
#85558=DIRECTION('center_axis',(-0.124079706118009,0.9873637223582,-0.0985753838472311));
#85559=DIRECTION('ref_axis',(-0.665363952244306,-0.00909007427090294,0.746463784522455));
#85560=DIRECTION('',(0.0517714178151324,0.,-0.998658960955846));
#85561=DIRECTION('center_axis',(-4.94383559695101E-14,-1.,5.5370153410865E-14));
#85562=DIRECTION('ref_axis',(-1.76122624385495E-31,-5.5370153410865E-14,
-1.));
#85563=DIRECTION('center_axis',(-0.129940320557335,-0.987363721732702,-0.0907104960828901));
#85564=DIRECTION('ref_axis',(-0.71675365861586,0.0303233802018828,0.6966668396543));
#85565=DIRECTION('center_axis',(0.137500844342104,-0.987363722957578,0.0787806854029617));
#85566=DIRECTION('ref_axis',(-0.661923171710724,-0.0324282840967445,0.748869896005278));
#85567=DIRECTION('',(-0.986440193500669,0.,0.164121127970665));
#85568=DIRECTION('center_axis',(-0.142369586162368,0.987363722340887,-0.069597275385635));
#85569=DIRECTION('ref_axis',(-0.489340464185005,-0.00909007622411355,0.872045457889348));
#85570=DIRECTION('',(-0.164121129030201,0.,-0.986440193324386));
#85571=DIRECTION('center_axis',(-3.27416115837152E-14,-1.,5.82330736311059E-14));
#85572=DIRECTION('ref_axis',(-1.3715310984991E-31,-5.82330736311059E-14,
-1.));
#85573=DIRECTION('center_axis',(-0.146402462725365,-0.987363721749518,-0.0606564084074233));
#85574=DIRECTION('ref_axis',(-0.550233578611314,0.0303233787080033,0.834460006035231));
#85575=DIRECTION('center_axis',(0.151221665785124,-0.987363723189041,0.0473802271780921));
#85576=DIRECTION('ref_axis',(-0.4854628862946,-0.032428275889997,0.873655648956337));
#85577=DIRECTION('',(-0.928096578352929,0.,0.372339551014374));
#85578=DIRECTION('center_axis',(-0.154002421996287,0.987363722277982,-0.0373648758681921));
#85579=DIRECTION('ref_axis',(-0.290435959825997,-0.009090077635243,0.956851254756212));
#85580=DIRECTION('',(-0.372339549380154,0.,-0.928096579008556));
#85581=DIRECTION('center_axis',(1.94577414584816E-14,-1.,-6.39100954909678E-14));
#85582=DIRECTION('ref_axis',(-2.8111492504619E-31,6.39100954909678E-14,
-1.));
#85583=DIRECTION('center_axis',(-0.156018988142432,-0.987363721822666,-0.0277660974482387));
#85584=DIRECTION('ref_axis',(-0.357985189673304,0.0303233746749526,0.933234749097402));
#85585=DIRECTION('center_axis',(0.157871536511976,-0.987363723086416,0.0137643122704986));
#85586=DIRECTION('ref_axis',(-0.286302893437925,-0.0324282793787185,0.957590235907618));
#85587=DIRECTION('',(-0.826356198741165,0.,0.563147789485187));
#85588=DIRECTION('center_axis',(-0.158434274704725,0.987363722287983,-0.00338533726621558));
#85589=DIRECTION('ref_axis',(-0.0779509939136845,-0.00909007789139745,0.996915750217538));
#85590=DIRECTION('',(-0.563147788031161,0.,-0.826356199732059));
#85591=DIRECTION('center_axis',(-6.4338375555057E-15,-1.,8.13984748522599E-14));
#85592=DIRECTION('ref_axis',(-7.09766227055145E-32,-8.13984748522599E-14,
-1.));
#85593=DIRECTION('center_axis',(-0.158340241063287,-0.987363721828894,0.00642252880218966));
#85594=DIRECTION('ref_axis',(-0.148997811258801,0.0303233746239653,0.98837247290255));
#85595=DIRECTION('center_axis',(0.157139508177838,-0.987363722970566,-0.0204952075210409));
#85596=DIRECTION('ref_axis',(-0.0737556956995861,-0.0324282834517269,0.996748967285266));
#85597=DIRECTION('',(-0.68597632228297,0.,0.727623862491556));
#85598=DIRECTION('',(0.761200566737339,0.,-0.648516535794388));
#85599=DIRECTION('center_axis',(0.153863152436169,-0.987363722371363,0.03793428617189));
#85600=DIRECTION('ref_axis',(-0.188441790513884,0.00836476944115453,0.982048737191855));
#85601=DIRECTION('center_axis',(-0.153405752207115,-0.987363721985033,-0.0397436246161791));
#85602=DIRECTION('ref_axis',(-0.260336356464506,0.00158397740775573,0.965516686815074));
#85603=DIRECTION('',(0.469718957703108,0.,0.882816006183795));
#85604=DIRECTION('center_axis',(-5.55199781974668E-15,-1.,2.91680662988477E-14));
#85605=DIRECTION('ref_axis',(-1.37200428465795E-31,-2.91680662988477E-14,
-1.));
#85606=DIRECTION('center_axis',(0.157639630788376,0.987363722515582,0.0162057479024672));
#85607=DIRECTION('ref_axis',(-0.112073886978174,0.00158366860756381,0.993698614194135));
#85608=DIRECTION('center_axis',(-0.14640245848675,0.987363723292207,-0.0606563935260433));
#85609=DIRECTION('ref_axis',(-0.191341517099414,0.0318943943832642,0.981005184207005));
#85610=DIRECTION('',(0.882816006173184,0.,-0.469718957723051));
#85611=DIRECTION('center_axis',(0.142111167445554,-0.987363722349851,0.0701234331354898));
#85612=DIRECTION('ref_axis',(-0.395147576306963,0.00836476911063044,0.918579568451454));
#85613=DIRECTION('center_axis',(-0.141275512893773,-0.987363722159082,-0.0717921278467529));
#85614=DIRECTION('ref_axis',(-0.461807381783311,0.00158399341620002,0.886978823363501));
#85615=DIRECTION('',(0.268957842517584,0.,0.963151950082793));
#85616=DIRECTION('center_axis',(-2.33849344727135E-14,-1.,5.45852353395005E-14));
#85617=DIRECTION('ref_axis',(1.70718886853183E-32,-5.45852353395005E-14,
-1.));
#85618=DIRECTION('center_axis',(0.150470348483635,0.987363722496377,0.0497147234258606));
#85619=DIRECTION('ref_axis',(-0.323069488553992,0.00158367253386998,0.9463739205762));
#85620=DIRECTION('center_axis',(-0.129940323503184,0.987363723619674,-0.0907104713237707));
#85621=DIRECTION('ref_axis',(-0.397755173973421,0.0318943830411897,0.916937058858347));
#85622=DIRECTION('',(0.963151949602078,0.,-0.268957844239047));
#85623=DIRECTION('center_axis',(0.123714217828372,-0.987363722263984,0.0990336925703855));
#85624=DIRECTION('ref_axis',(-0.583376700032673,0.00836477655867606,0.81215863990486));
#85625=DIRECTION('center_axis',(-0.122539376667729,-0.987363722039492,-0.100483737819634));
#85626=DIRECTION('ref_axis',(-0.641684811093609,0.00158398009810487,0.76696681428782));
#85627=DIRECTION('',(0.0556205582211182,0.,0.998451978566406));
#85628=DIRECTION('center_axis',(1.72862098727691E-14,-1.,-2.41409965901546E-14));
#85629=DIRECTION('ref_axis',(5.0966387703121E-31,2.41409965901546E-14,-1.));
#85630=DIRECTION('center_axis',(0.136265238390394,0.987363722512308,0.0808990993339642));
#85631=DIRECTION('ref_axis',(-0.518958723024964,0.00158367098874867,0.854797833281354));
#85632=DIRECTION('center_axis',(-0.107402317333303,0.98736372348291,-0.116523043993025));
#85633=DIRECTION('ref_axis',(-0.585570242472141,0.0318943888650221,0.809993974724532));
#85634=DIRECTION('',(0.99845197842399,0.,-0.0556205607776467));
#85635=DIRECTION('center_axis',(0.099532535089522,-0.987363722350104,0.123313236295216));
#85636=DIRECTION('ref_axis',(-0.744327775711308,0.00836477204862553,0.667762078058668));
#85637=DIRECTION('center_axis',(-0.0980734501969365,-0.987363722134044,
-0.124476819448742));
#85638=DIRECTION('ref_axis',(-0.791557770193034,0.00158399262243925,0.61109229042298));
#85639=DIRECTION('',(-0.160317479600256,0.,0.987065502251305));
#85640=DIRECTION('center_axis',(6.62150057297851E-14,-1.,-5.95817081362791E-14));
#85641=DIRECTION('ref_axis',(1.,6.62150057297851E-14,-3.0643499606565E-30));
#85642=DIRECTION('center_axis',(0.115688518570161,0.987363722502101,0.108300720947907));
#85643=DIRECTION('ref_axis',(-0.690582021097443,0.00158367157795096,0.723252351618233));
#85644=DIRECTION('center_axis',(-0.0798423016070618,0.987363723489339,-0.136887122883619));
#85645=DIRECTION('ref_axis',(-0.746004697532087,0.0318943877439224,0.665176472291751));
#85646=DIRECTION('',(0.987065502661801,0.,0.160317477072854));
#85647=DIRECTION('center_axis',(0.0706968123188893,-0.987363722207916,0.141826798580794));
#85648=DIRECTION('ref_axis',(-0.870474915562179,0.00836477955372812,0.492141698944556));
#85649=DIRECTION('center_axis',(-0.0690217115090215,-0.987363722152823,
-0.142649512851912));
#85650=DIRECTION('ref_axis',(-0.90441836785597,0.00158399343718549,0.42664377043329));
#85651=DIRECTION('',(-0.368759251362437,0.,0.929524940243464));
#85652=DIRECTION('center_axis',(2.58250805724881E-14,-1.,-1.46514839927069E-14));
#85653=DIRECTION('ref_axis',(1.,2.58250805724881E-14,5.20492449486746E-31));
#85654=DIRECTION('center_axis',(0.089702331649604,0.987363722499697,0.130638322050482));
#85655=DIRECTION('ref_axis',(-0.829914475268389,0.00158367205682094,0.557888390023319));
#85656=DIRECTION('center_axis',(-0.048548946371977,0.987363723458484,-0.150850513437537));
#85657=DIRECTION('ref_axis',(-0.871556800476462,0.0318943896923164,0.489256059185154));
#85658=DIRECTION('',(0.929524940202268,0.,0.368759251466278));
#85659=DIRECTION('center_axis',(0.0385553978110738,-0.987363722333291,0.15370868914859));
#85660=DIRECTION('ref_axis',(-0.95591961231219,0.00836477265671015,0.293509327578042));
#85661=DIRECTION('center_axis',(-0.0367425853322626,-0.987363722085997,
-0.154152076637289));
#85662=DIRECTION('ref_axis',(-0.97498936820771,0.00158398468336746,0.222245861321313));
#85663=DIRECTION('',(-0.559958251059163,0.,0.828520824765898));
#85664=DIRECTION('center_axis',(2.83709405267253E-14,-1.,-8.75731150790992E-15));
#85665=DIRECTION('ref_axis',(1.,2.83709405267253E-14,3.25104264459992E-31));
#85666=DIRECTION('center_axis',(0.0595217627816455,0.987363722497361,0.146867420660677));
#85667=DIRECTION('ref_axis',(-0.930441048090257,0.0015836710718016,0.36643819126101));
#85668=DIRECTION('center_axis',(-0.0149854919230227,0.987363723258614,-0.157760302436043));
#85669=DIRECTION('ref_axis',(-0.95635587745199,0.0318943956067335,0.290458573968674));
#85670=DIRECTION('',(0.828520826199677,0.,0.559958248937727));
#85671=DIRECTION('center_axis',(0.00461116712645498,-0.987363722278625,
0.158403336662551));
#85672=DIRECTION('ref_axis',(-0.996666572634082,0.00836477445303214,0.0811527790170065));
#85673=DIRECTION('center_axis',(-0.00274543282601405,-0.987363722148695,
-0.158446655954841));
#85674=DIRECTION('ref_axis',(-0.999970949214054,0.00158399315517319,0.00745598374647318));
#85675=DIRECTION('',(-0.72497422441143,0.,0.688775996924287));
#85676=DIRECTION('center_axis',(0.,-1.,0.));
#85677=DIRECTION('ref_axis',(0.,0.,-1.));
#85678=DIRECTION('center_axis',(0.0265580251225395,0.98736372248948,0.156229161212971));
#85679=DIRECTION('ref_axis',(-0.987461233018084,0.00158367357248836,0.157853746437712));
#85680=DIRECTION('center_axis',(0.0192786623139663,0.987363723283692,-0.157293391859761));
#85681=DIRECTION('ref_axis',(-0.996436816101143,0.0318943955032277,0.0780795687340866));
#85682=DIRECTION('',(0.688775998780597,0.,0.724974222647806));
#85683=DIRECTION('center_axis',(-0.0295486712570818,-0.987363722331637,
0.155691219567303));
#85684=DIRECTION('ref_axis',(-0.99081051081007,0.00836477140751204,-0.134998378759112));
#85685=DIRECTION('center_axis',(0.0313801075564329,-0.987363722072691,-0.155332447300972));
#85686=DIRECTION('ref_axis',(-0.978194999555421,0.00158398726276867,-0.207682531352836));
#85687=DIRECTION('',(-0.856091208538384,0.,0.516824769784972));
#85688=DIRECTION('center_axis',(2.94258679130039E-14,-1.,3.96472806032467E-15));
#85689=DIRECTION('ref_axis',(1.,2.94258679130039E-14,-2.03061687717273E-31));
#85690=DIRECTION('center_axis',(-0.00764753657259386,0.987363722466856,
0.158285800818532));
#85691=DIRECTION('ref_axis',(-0.998308827638998,0.00158367492915277,-0.0581117598405685));
#85692=DIRECTION('center_axis',(0.0526413609300347,0.987363723434933,-0.14947161859075));
#85693=DIRECTION('ref_axis',(-0.989925476770943,0.0318943888980207,-0.137950347577098));
#85694=DIRECTION('',(0.516824771977019,0.,0.856091207215039));
#85695=DIRECTION('center_axis',(-0.0623268468155332,-0.987363722406808,
0.145699155251516));
#85696=DIRECTION('ref_axis',(-0.938625251787949,0.00836476882371502,-0.344837160625904));
#85697=DIRECTION('center_axis',(0.0640383424309129,-0.987363722105989,-0.144955065339949));
#85698=DIRECTION('ref_axis',(-0.910679739708499,0.00158398709049708,-0.413110036999052));
#85699=DIRECTION('',(-0.947178320273382,0.,0.320707389381808));
#85700=DIRECTION('center_axis',(1.39428040580449E-13,-1.,5.09886334668116E-14));
#85701=DIRECTION('ref_axis',(1.,1.39428040580449E-13,2.22957426837468E-30));
#85702=DIRECTION('center_axis',(-0.0414955103107478,0.987363722492926,0.152941172118444));
#85703=DIRECTION('ref_axis',(-0.962476611317351,0.00158367430440513,-0.271360027717359));
#85704=DIRECTION('center_axis',(0.0835426153607864,0.987363723422421,-0.134660718430034));
#85705=DIRECTION('ref_axis',(-0.937126322349836,0.0318943895417038,-0.347529860407468));
#85706=DIRECTION('',(0.320707392680363,0.,0.947178319156516));
#85707=DIRECTION('center_axis',(-0.0921906959890649,-0.987363722318877,
0.128894357602123));
#85708=DIRECTION('ref_axis',(-0.842550917106313,0.00836477377934728,-0.538551745557408));
#85709=DIRECTION('center_axis',(0.0937022132057685,-0.987363722093186,-0.127799747787823));
#85710=DIRECTION('ref_axis',(-0.800582108000364,0.00158399010146328,-0.599220977040234));
#85711=DIRECTION('',(-0.993976426077081,-1.24675414343594E-14,0.109594089270516));
#85712=DIRECTION('center_axis',(2.50414483022948E-14,-1.,1.59538909637361E-14));
#85713=DIRECTION('ref_axis',(1.,2.50414483022948E-14,8.64987797024603E-31));
#85714=DIRECTION('center_axis',(-0.0734031997935144,0.987363722515641,0.14044518404036));
#85715=DIRECTION('ref_axis',(-0.881640057253848,0.00158367420529362,-0.47191980401488));
#85716=DIRECTION('center_axis',(0.110537511239738,0.987363723356507,-0.113553231607469));
#85717=DIRECTION('ref_axis',(-0.840508183059939,0.0318943919763055,-0.540859262627296));
#85718=DIRECTION('',(0.109594089288516,0.,0.993976426075096));
#85719=DIRECTION('center_axis',(-0.11774380657933,-0.987363722266,0.106062603990463));
#85720=DIRECTION('ref_axis',(-0.707079838374903,0.00836477484011131,-0.707084247247523));
#85721=DIRECTION('center_axis',(0.118984675664632,-0.987363722112959,-0.104668654391976));
#85722=DIRECTION('ref_axis',(-0.653050145064529,0.00158399001390786,-0.757313012569329));
#85723=DIRECTION('',(-0.994297298974217,0.,-0.106643711734809));
#85724=DIRECTION('center_axis',(-2.10263781896676E-14,-1.,-2.09640690225964E-14));
#85725=DIRECTION('ref_axis',(1.,-2.10263781896676E-14,4.52823587212026E-31));
#85726=DIRECTION('center_axis',(-0.101878638090563,0.987363722508961,0.121382134492933));
#85727=DIRECTION('ref_axis',(-0.759578996500587,0.00158367209155293,-0.650413130293253));
#85728=DIRECTION('center_axis',(0.132363795336434,0.98736372331842,-0.0871361208622546));
#85729=DIRECTION('ref_axis',(-0.704588813393261,0.0318943940108991,-0.708898689286243));
#85730=DIRECTION('',(-0.106643708884035,0.,0.994297299279978));
#85731=DIRECTION('center_axis',(-0.137791344891649,-0.987363722327925,0.0782714833364976));
#85732=DIRECTION('ref_axis',(-0.538546495051158,0.00836477267704766,-0.842554273175428));
#85733=DIRECTION('center_axis',(0.138703546279527,-0.987363722114087,-0.0766433722020272));
#85734=DIRECTION('ref_axis',(-0.474982282313184,0.00158399133528933,-0.879993933195001));
#85735=DIRECTION('',(-0.948125934970738,0.,-0.317894969189297));
#85736=DIRECTION('center_axis',(4.80844140052452E-14,-1.,7.49819715214931E-14));
#85737=DIRECTION('ref_axis',(2.0155716587825E-30,-7.49819715214931E-14,
-1.));
#85738=DIRECTION('center_axis',(-0.125590341158658,0.987363722487909,0.0966433946137617));
#85739=DIRECTION('ref_axis',(-0.602000863538362,0.00158367561643957,-0.798493864892278));
#85740=DIRECTION('center_axis',(0.148000890406933,0.987363723485712,-0.0566446288997078));
#85741=DIRECTION('ref_axis',(-0.535723656273679,0.0318943877768316,-0.843790798798554));
#85742=DIRECTION('',(-0.317894965895091,0.,0.948125936075245));
#85743=DIRECTION('center_axis',(-0.151395913665258,-0.987363722405331,0.0468204763255448));
#85744=DIRECTION('ref_axis',(-0.34483131411186,0.0083647694638503,-0.938627399685149));
#85745=DIRECTION('center_axis',(0.151936793256339,-0.987363722132207,-0.0450343321502049));
#85746=DIRECTION('ref_axis',(-0.274704778256895,0.00158399311141727,-0.961527314104312));
#85747=DIRECTION('',(-0.857621255980855,0.,-0.514281811159816));
#85748=DIRECTION('center_axis',(4.11217595969307E-14,-1.,1.11420883109922E-13));
#85749=DIRECTION('ref_axis',(2.12336121339679E-30,-1.11420883109922E-13,
-1.));
#85750=DIRECTION('center_axis',(-0.143429583022958,0.987363722493762,0.067385712262476));
#85751=DIRECTION('ref_axis',(-0.416273840057586,0.00158367279585466,-0.909237912795208));
#85752=DIRECTION('center_axis',(0.156717633017502,0.98736372345637,-0.0235044911402842));
#85753=DIRECTION('ref_axis',(-0.341808656410646,0.0318943892618742,-0.939228188640205));
#85754=DIRECTION('',(-0.514281808963847,0.,0.857621257297692));
#85755=DIRECTION('center_axis',(-0.157921381073739,-0.987363722267462,0.0131801877795928));
#85756=DIRECTION('ref_axis',(-0.134992203354449,0.00836477513405653,-0.990811352160676));
#85757=DIRECTION('center_axis',(0.158065646082108,-0.987363722122479,-0.0113195302504295));
#85758=DIRECTION('ref_axis',(-0.0615823826120716,0.00158398821891373,-0.998100746985565));
#85759=DIRECTION('',(-0.727015160077822,0.,-0.686621407339604));
#85760=DIRECTION('center_axis',(-8.10407971111379E-15,-1.,-5.88279438136482E-14));
#85761=DIRECTION('ref_axis',(-2.99900690858271E-31,5.88279438136482E-14,
-1.));
#85762=DIRECTION('center_axis',(-0.15456221444901,0.98736372244984,0.0349771561824722));
#85763=DIRECTION('ref_axis',(-0.211082316846037,0.00158367759288358,-0.977467005826893));
#85764=DIRECTION('center_axis',(0.158106432629902,0.987363723460094,0.0107346893790416));
#85765=DIRECTION('ref_axis',(-0.13191106112732,0.0318943890127931,-0.990748313095594));
#85766=DIRECTION('',(-0.686621405562463,0.,0.727015161756224));
#85767=DIRECTION('center_axis',(-0.157062618066433,-0.987363722391757,-0.0210763780287661));
#85768=DIRECTION('ref_axis',(0.0811589922647188,0.00836476649861784,-0.996666066772617));
#85769=DIRECTION('center_axis',(0.156803523454507,-0.987363722103122,0.0229245568533188));
#85770=DIRECTION('ref_axis',(0.154419534208586,0.0015839866243612,-0.988004098392905));
#85771=DIRECTION('',(-0.562414644138898,0.,-0.826855348932398));
#85772=DIRECTION('center_axis',(-9.46331629412281E-15,-1.,1.18389433539854E-13));
#85773=DIRECTION('ref_axis',(3.25119361935713E-31,-1.18389433539854E-13,
-1.));
#85774=DIRECTION('center_axis',(-0.158467690465133,0.987363722444043,0.000933102400878574));
#85775=DIRECTION('ref_axis',(0.0039791834017034,0.00158367763717511,-0.999990828990245));
#85776=DIRECTION('center_axis',(0.152102351266528,0.987363723473008,0.0444719271980735));
#85777=DIRECTION('ref_axis',(0.0841545458583856,0.0318943886797806,-0.995942147106001));
#85778=DIRECTION('',(-0.826855347492317,0.,0.562414646256087));
#85779=DIRECTION('center_axis',(-0.148859780937109,-0.987363722285066,-0.0543474519617457));
#85780=DIRECTION('ref_axis',(0.293515284482669,0.00836477446767391,-0.955917783244544));
#85781=DIRECTION('center_axis',(0.14820944281693,-0.987363722100043,0.0560967141697563));
#85782=DIRECTION('ref_axis',(0.363200967923451,0.00158398863631637,-0.93170947611338));
#85783=DIRECTION('',(-0.371516244401546,0.,-0.928426453816225));
#85784=DIRECTION('center_axis',(-1.73461489318175E-14,-1.,5.67936105665548E-14));
#85785=DIRECTION('ref_axis',(-1.79164664649797E-31,-5.67936105665548E-14,
-1.));
#85786=DIRECTION('center_axis',(-0.154963392512639,0.987363722477644,-0.0331545851438956));
#85787=DIRECTION('ref_axis',(0.218854622341282,0.00158367475091716,-0.975756192014244));
#85788=DIRECTION('center_axis',(0.138986131040637,0.987363723275524,0.0761297138957497));
#85789=DIRECTION('ref_axis',(0.296285183575623,0.0318943948969972,-0.954566832425951));
#85790=DIRECTION('',(-0.928426452468148,0.,0.371516247770418));
#85791=DIRECTION('center_axis',(-0.133696426889398,-0.987363722309465,-0.0850772901790237));
#85792=DIRECTION('ref_axis',(0.492147125907155,0.00836477331035454,-0.870471847349926));
#85793=DIRECTION('center_axis',(0.132685252704572,-0.987363722101427,0.086645853869304));
#85794=DIRECTION('ref_axis',(0.55499952682238,0.00158398787712574,-0.831849154720578));
#85795=DIRECTION('',(-0.163246158252737,-1.24675414427253E-14,-0.986585369755564));
#85796=DIRECTION('center_axis',(1.45747765284724E-14,-1.,-2.58684491063667E-14));
#85797=DIRECTION('ref_axis',(5.35693019029158E-31,2.58684491063667E-14,
-1.));
#85798=DIRECTION('center_axis',(-0.144213177993266,0.987363722497658,-0.0656919994264963));
#85799=DIRECTION('ref_axis',(0.423496662042141,0.00158367336515953,-0.905896279503253));
#85800=DIRECTION('center_axis',(0.119371075236614,0.987363723315672,0.104227751952477));
#85801=DIRECTION('ref_axis',(0.494561850446257,0.031894393766983,-0.868557035392271));
#85802=DIRECTION('',(-0.986585369800573,0.,0.163246157980722));
#85803=DIRECTION('center_axis',(-0.112281577443688,-0.9873637223284,-0.111829008743547));
#85804=DIRECTION('ref_axis',(0.667766714850343,0.0083647716155623,-0.744323615864632));
#85805=DIRECTION('center_axis',(0.110956847896642,-0.987363722081101,0.11314352930237));
#85806=DIRECTION('ref_axis',(0.720846926519561,0.00158398805948769,-0.693092489866345));
#85807=DIRECTION('',(0.0526571372340305,0.,-0.998612650579952));
#85808=DIRECTION('center_axis',(1.97949782769355E-14,-1.,-2.21305130496739E-14));
#85809=DIRECTION('ref_axis',(-8.25466210470689E-31,2.21305130496739E-14,
-1.));
#85810=DIRECTION('center_axis',(-0.126719716998718,0.987363722469099,-0.0951577263060111));
#85811=DIRECTION('ref_axis',(0.60833646652202,0.00158367463533589,-0.793677664719219));
#85812=DIRECTION('center_axis',(0.094174361865117,0.987363723369365,0.127452215914363));
#85813=DIRECTION('ref_axis',(0.669713359057949,0.0318943909699352,-0.741934474548781));
#85814=DIRECTION('',(-0.998612650714781,0.,-0.0526571346770678));
#85815=DIRECTION('center_axis',(-0.0856165661101796,-0.987363722404662,
-0.133351727723007));
#85816=DIRECTION('ref_axis',(0.812162274774787,0.00836477053525665,-0.583371639734514));
#85817=DIRECTION('center_axis',(0.0840402268233821,-0.987363722129493,0.134350736872072));
#85818=DIRECTION('ref_axis',(0.852988322579091,0.00158399112249083,-0.521927593173452));
#85819=DIRECTION('',(0.266098244580432,0.,-0.963945913540388));
#85820=DIRECTION('center_axis',(-4.81791775471634E-14,-1.,3.4715557455305E-14));
#85821=DIRECTION('ref_axis',(1.,-4.81791775471634E-14,-1.60160519362453E-30));
#85822=DIRECTION('center_axis',(-0.103300975937542,0.987363722552576,-0.120173989521323));
#85823=DIRECTION('ref_axis',(0.764731136019292,0.00158366708520907,-0.644347562733969));
#85824=DIRECTION('center_axis',(0.0645741589271399,0.987363723386845,0.144717157719871));
#85825=DIRECTION('ref_axis',(0.813549812505479,0.0318943908738347,-0.580619884608758));
#85826=DIRECTION('',(-0.963945914018185,0.,-0.266098242849603));
#85827=DIRECTION('center_axis',(-0.0549482164094863,-0.987363722325894,
-0.148639070732333));
#85828=DIRECTION('ref_axis',(0.918582031228676,0.00836477290385111,-0.395141851083971));
#85829=DIRECTION('center_axis',(0.0531939751881081,-0.987363722116085,0.149275856228521));
#85830=DIRECTION('ref_axis',(0.945244934851768,0.00158399063008826,-0.326357938636032));
#85831=DIRECTION('',(0.467096893063886,0.,-0.884206136876501));
#85832=DIRECTION('center_axis',(1.09031187632399E-13,-1.,-4.7093656008092E-14));
#85833=DIRECTION('ref_axis',(1.,1.09031187632399E-13,-1.18181014932651E-30));
#85834=DIRECTION('center_axis',(-0.0750520055291037,0.987363722501096,-0.139571042680201));
#85835=DIRECTION('ref_axis',(0.885367824820323,0.00158367152393529,-0.464888488518951));
#85836=DIRECTION('center_axis',(0.0319545399072673,0.98736372339762,0.155215286288767));
#85837=DIRECTION('ref_axis',(0.919345582593993,0.0318943906489118,-0.392156152074713));
#85838=DIRECTION('',(-0.884206138072515,0.,-0.467096890799851));
#85839=DIRECTION('center_axis',(-0.0217105585997335,-0.987363722455224,
-0.156976212289159));
#85840=DIRECTION('ref_axis',(0.982049910802658,0.00836476579291928,-0.188435674397715));
#85841=DIRECTION('center_axis',(0.0198604336684252,-0.987363722123183,0.15722100180814));
#85842=DIRECTION('ref_axis',(0.993302943375519,0.00158399135114877,-0.115528150911064));
#85843=DIRECTION('',(0.646254610502261,0.,-0.763121863403592));
#85844=DIRECTION('center_axis',(0.,-1.,0.));
#85845=DIRECTION('ref_axis',(0.,0.,-1.));
#85846=DIRECTION('center_axis',(-0.0432936835437904,0.987363722495306,-0.152441911774364));
#85847=DIRECTION('ref_axis',(0.964605700418953,0.00158367242142303,-0.263691741814041));
#85848=DIRECTION('center_axis',(-0.00215923201411667,0.987363723575172,
0.158455719634478));
#85849=DIRECTION('ref_axis',(0.982153774465284,0.0318943847097455,-0.185355635273339));
#85850=DIRECTION('',(-0.763121866258997,0.,-0.646254607130491));
#85851=DIRECTION('center_axis',(0.0125422742197993,-0.987363722351044,-0.157973324148369));
#85852=DIRECTION('ref_axis',(0.999598229358044,0.00836477189981278,0.0270815519372187));
#85853=DIRECTION('center_axis',(-0.0144017728166543,-0.987363722007407,
0.157814667896928));
#85854=DIRECTION('ref_axis',(0.994915210037057,0.00158397858048353,0.100703603951277));
#85855=DIRECTION('',(0.795194177911862,-1.2467541437894E-14,-0.606354862613534));
#85856=DIRECTION('center_axis',(0.,-1.,0.));
#85857=DIRECTION('ref_axis',(0.,0.,-1.));
#85858=DIRECTION('center_axis',(-0.0095109963087418,0.987363722509277,-0.158184766718666));
#85859=DIRECTION('ref_axis',(0.998739685024105,0.00158367240317003,-0.0501650629389698));
#85860=DIRECTION('center_axis',(-0.0361720565381791,0.98736372327208,0.154286941417914));
#85861=DIRECTION('ref_axis',(0.999037547159214,0.0318943950411722,0.0301119067987736));
#85862=DIRECTION('',(-0.606354862831809,0.,-0.795194177745422));
#85863=DIRECTION('center_axis',(0.0462086372706431,-0.987363722333362,-0.151583777699325));
#85864=DIRECTION('ref_axis',(0.970406444941592,0.00836477114710228,0.241332472368468));
#85865=DIRECTION('center_axis',(-0.0479905467177105,-0.987363722122278,
0.151029095417331));
#85866=DIRECTION('ref_axis',(0.950006347883252,0.00158398786905911,0.312226568318515));
#85867=DIRECTION('',(0.906951352788388,0.,-0.421235377995858));
#85868=DIRECTION('center_axis',(0.,-1.,0.));
#85869=DIRECTION('ref_axis',(0.,0.,-1.));
#85870=DIRECTION('center_axis',(0.0247164153185022,0.987363722501068,-0.156531077753389));
#85871=DIRECTION('ref_axis',(0.986173711967527,0.00158367140532946,0.165707277477693));
#85872=DIRECTION('center_axis',(-0.0684934961390298,0.987363723561067,0.142903878121892));
#85873=DIRECTION('ref_axis',(0.969207435188215,0.0318943852159877,0.244171447486345));
#85874=DIRECTION('',(-0.421235379219833,0.,-0.90695135221991));
#85875=DIRECTION('center_axis',(0.0777143306467572,-0.987363722433298,-0.138106344657978));
#85876=DIRECTION('ref_axis',(0.895839535150784,0.00836476526275839,0.444298951116167));
#85877=DIRECTION('center_axis',(-0.0793353440989328,-0.98736372213029,0.137181570911415));
#85878=DIRECTION('ref_axis',(0.860676244930596,0.00158398939727591,0.509150166836621));
#85879=DIRECTION('',(0.976300488927256,0.,-0.21641939682108));
#85880=DIRECTION('center_axis',(2.66195733031672E-14,-1.,1.31529117696217E-14));
#85881=DIRECTION('ref_axis',(1.,2.66195733031672E-14,-2.69371696899743E-31));
#85882=DIRECTION('center_axis',(0.0577881148440998,0.987363722518325,-0.147558168996237));
#85883=DIRECTION('ref_axis',(0.927495351769603,0.00158367058952022,0.373831331529668));
#85884=DIRECTION('center_axis',(-0.0976122735639677,0.987363723325657,0.124838783677868));
#85885=DIRECTION('ref_axis',(0.894058259712442,0.0318943939332761,0.446813804481899));
#85886=DIRECTION('',(-0.216419402668503,0.,-0.976300487631041));
#85887=DIRECTION('center_axis',(0.105586202135494,-0.987363722288055,-0.118171205579362));
#85888=DIRECTION('ref_axis',(0.779384160790386,0.00836477417458723,0.626490511071056));
#85889=DIRECTION('center_axis',(-0.106970512095575,-0.98736372209358,0.116919587048206));
#85890=DIRECTION('ref_axis',(0.73110187581061,0.00158398776783174,0.682266471526308));
#85891=DIRECTION('',(0.999998899039541,0.,-0.00148388668929281));
#85892=DIRECTION('center_axis',(-2.31697352304947E-14,-1.,-1.85678253840655E-14));
#85893=DIRECTION('ref_axis',(1.,-2.31697352304947E-14,-7.4436340050474E-31));
#85894=DIRECTION('center_axis',(0.0881577081296384,0.98736372254722,-0.131685602459135));
#85895=DIRECTION('ref_axis',(0.825448339563568,0.0015836672265046,0.564475447393299));
#85896=DIRECTION('center_axis',(-0.122166803491906,0.987363723229867,0.100936366955741));
#85897=DIRECTION('ref_axis',(0.777103913440387,0.0318943968373218,0.628563644483213));
#85898=DIRECTION('',(-0.00148388924556319,0.,-0.999998899035747));
#85899=DIRECTION('center_axis',(0.12852096790079,-0.987363722400553,-0.0927105198840292));
#85900=DIRECTION('ref_axis',(0.626485654806589,0.00836476963973098,0.779388064413636));
#85901=DIRECTION('center_axis',(-0.129603853819052,-0.987363722117569,0.0911905769330912));
#85902=DIRECTION('ref_axis',(0.567341997927538,0.00158399122592401,0.823480751662955));
#85903=DIRECTION('',(0.976938472070387,0.,0.213521010181148));
#85904=DIRECTION('center_axis',(-3.72730121926079E-14,-1.,-4.62290562453021E-14));
#85905=DIRECTION('ref_axis',(-1.12700347311895E-30,4.62290562453021E-14,
-1.));
#85906=DIRECTION('center_axis',(0.114405139984501,0.987363722521768,-0.109655567086603));
#85907=DIRECTION('ref_axis',(0.684804280432006,0.0015836701562166,0.728725318272144));
#85908=DIRECTION('center_axis',(-0.141008943767301,0.987363723370658,0.0723142831621817));
#85909=DIRECTION('ref_axis',(0.623813053134467,0.0318943919879685,0.780922545774402));
#85910=DIRECTION('',(0.21352100493591,0.,-0.976938473216793));
#85911=DIRECTION('center_axis',(0.145446241810615,-0.987363722339979,-0.0629147880081431));
#85912=DIRECTION('ref_axis',(0.444293371274801,0.00836477215045521,0.895842302432823));
#85913=DIRECTION('center_axis',(-0.146177066759276,-0.987363722116811,0.061197593100471));
#85914=DIRECTION('ref_axis',(0.377053836385937,0.00158398999577492,0.926189988848044));
#85915=DIRECTION('',(0.908197487535578,0.,0.418541901885658));
#85916=DIRECTION('center_axis',(-2.6463709296946E-14,-1.,-5.31608424195587E-14));
#85917=DIRECTION('ref_axis',(-9.88265445775187E-31,5.31608424195587E-14,
-1.));
#85918=DIRECTION('center_axis',(0.135303116346826,0.987363722522324,-0.0824981584867021));
#85919=DIRECTION('ref_axis',(0.512139533901716,0.00158367135915935,0.858900803236299));
#85920=DIRECTION('center_axis',(-0.153257664669201,0.98736372347784,0.0403108642938551));
#85921=DIRECTION('ref_axis',(0.441353388196775,0.0318943881547522,0.896766376896157));
#85922=DIRECTION('',(0.418541898467425,0.,-0.908197489110867));
#85923=DIRECTION('center_axis',(0.155570609330718,-0.987363722322886,-0.0301772323642034));
#85924=DIRECTION('ref_axis',(0.241326424552547,0.00836477233750035,0.970407948955709));
#85925=DIRECTION('center_axis',(-0.155915202237607,-0.987363722117027,0.0283430760224913));
#85926=DIRECTION('ref_axis',(0.169135057023849,0.00158398703376236,0.985591610897037));
#85927=DIRECTION('',(0.796990199392675,0.,0.603992236764699));
#85928=DIRECTION('center_axis',(-4.3250978366289E-14,-1.,-1.72820660217093E-13));
#85929=DIRECTION('ref_axis',(1.82527821333089E-30,1.72820660217093E-13,
-1.));
#85930=DIRECTION('center_axis',(0.149874468447564,0.987363722435629,-0.0514832334417587));
#85931=DIRECTION('ref_axis',(0.315527715267146,0.00158367769808369,0.94891503985512));
#85932=DIRECTION('center_axis',(-0.158340230231295,0.987363723437144,0.00642254860944178));
#85933=DIRECTION('ref_axis',(0.238256526802803,0.0318943903744065,0.970678409824031));
#85934=DIRECTION('',(0.603992234724004,0.,-0.796990200939199));
#85935=DIRECTION('center_axis',(0.158420668035202,-0.987363722286791,0.0039713790114702));
#85936=DIRECTION('ref_axis',(0.0270753218508432,0.00836477428387887,0.999598398106886));
#85937=DIRECTION('center_axis',(-0.158362914949753,-0.987363722140767,-0.00583672587568806));
#85938=DIRECTION('ref_axis',(-0.0466922879302391,0.00158399001302859,0.998908064450117));
#85939=DIRECTION('',(0.648516533598729,0.,0.761200568607965));
#85940=DIRECTION('center_axis',(1.6961537084023E-15,-1.,5.93592969796357E-14));
#85941=DIRECTION('ref_axis',(0.0285626985659955,5.93835252853779E-14,0.999592002894495));
#85942=DIRECTION('center_axis',(0.157437860183184,0.98736372253255,-0.0180609968608128));
#85943=DIRECTION('ref_axis',(0.104162167762182,0.0015836710625599,0.994559065512476));
#85944=DIRECTION('center_axis',(-0.156018981952473,0.987363723488671,-0.0277660729866842));
#85945=DIRECTION('ref_axis',(0.0240190581876539,0.0318943875855101,0.9992025985176));
#85946=DIRECTION('center_axis',(-0.159684140538363,-0.986495108818778,0.0364468865220547));
#85947=DIRECTION('ref_axis',(0.0345447361073574,0.0313138932743736,0.998912459275223));
#85948=DIRECTION('center_axis',(-0.148115809490731,-0.986495108701721,0.0699221530452668));
#85949=DIRECTION('ref_axis',(0.248473749993952,0.0313138980921802,0.968132343923193));
#85950=DIRECTION('center_axis',(-0.12962174787917,-0.986495108694425,0.100127933159151));
#85951=DIRECTION('ref_axis',(0.450784409547227,0.0313138983123357,0.892083435493364));
#85952=DIRECTION('center_axis',(-0.105066723785353,-0.986495108928782,0.125651834895487));
#85953=DIRECTION('ref_axis',(0.632016888372423,0.0313138890706075,0.774321698755313));
#85954=DIRECTION('center_axis',(-0.0755988850223349,-0.986495108721425,
0.145300409676239));
#85955=DIRECTION('ref_axis',(0.783696961325252,0.0313138975870502,0.620353538417791));
#85956=DIRECTION('center_axis',(-0.0425961334791471,-0.986495108732847,
0.158154891985026));
#85957=DIRECTION('ref_axis',(0.898732234955032,0.0313138961805359,0.43737833709356));
#85958=DIRECTION('center_axis',(-0.0076016341106203,-0.98649510878029,0.163614227716942));
#85959=DIRECTION('ref_axis',(0.97174378815581,0.0313138950000823,0.233951811620515));
#85960=DIRECTION('center_axis',(0.0277483045209817,-0.986495108911177,0.161423144841548));
#85961=DIRECTION('ref_axis',(0.999317682535591,0.0313138888934835,0.0195859575732665));
#85962=DIRECTION('center_axis',(0.06180077703097,-0.986495108727566,0.151684094139618));
#85963=DIRECTION('ref_axis',(0.980164591732371,0.0313138968610427,-0.195695715276269));
#85964=DIRECTION('center_axis',(0.0929635090524299,-0.98649510864731,0.134852462341594));
#85965=DIRECTION('ref_axis',(0.915180094010994,0.0313139006406196,-0.401826872113722));
#85966=DIRECTION('center_axis',(0.119779364643231,-0.986495108721393,0.111715282188389));
#85967=DIRECTION('ref_axis',(0.807402792437604,0.031313897487759,-0.58916905094216));
#85968=DIRECTION('center_axis',(0.140994469775086,-0.986495108843429,0.0833544223231981));
#85969=DIRECTION('ref_axis',(0.661872236306209,0.0313138927496215,-0.748962337456219));
#85970=DIRECTION('center_axis',(0.155616833928388,-0.98649510884469,0.0510960000744523));
#85971=DIRECTION('ref_axis',(0.485393267343429,0.0313138915404638,-0.873734980537155));
#85972=DIRECTION('center_axis',(0.162962728474184,-0.986495108838192,0.016448384922926));
#85973=DIRECTION('ref_axis',(0.286217849566809,0.031313891402459,-0.95765274645593));
#85974=DIRECTION('center_axis',(0.162688667007504,-0.986495108715825,-0.0189683448691279));
#85975=DIRECTION('ref_axis',(0.0736591994292219,0.0313138971291646,-0.996791734609608));
#85976=DIRECTION('center_axis',(0.154807463159199,-0.986495108750943,-0.0534981285717385));
#85977=DIRECTION('ref_axis',(-0.142343667071612,0.0313138962284748,-0.989321848716381));
#85978=DIRECTION('center_axis',(0.139687633297746,-0.986495108711815,-0.0855264028902112));
#85979=DIRECTION('ref_axis',(-0.351690706253517,0.0313138985509523,-0.935592372185902));
#85980=DIRECTION('center_axis',(0.118036166693634,-0.986495108760817,-0.113555553555324));
#85981=DIRECTION('ref_axis',(-0.544593076327316,0.031313896742111,-0.838115637061602));
#85982=DIRECTION('center_axis',(0.0908654613277357,-0.986495108803846,-0.136274972917941));
#85983=DIRECTION('ref_axis',(-0.712030880213924,0.0313138942150547,-0.701449546047949));
#85984=DIRECTION('center_axis',(0.0594459848832865,-0.986495108759378,-0.152622328887617));
#85985=DIRECTION('ref_axis',(-0.846174912151683,0.0313138958326044,-0.53198445275485));
#85986=DIRECTION('center_axis',(0.0252468845082368,-0.986495108812974,-0.161833232405173));
#85987=DIRECTION('ref_axis',(-0.940752744030153,0.0313138932274296,-0.337644361260008));
#85988=DIRECTION('center_axis',(-0.0101327382908042,-0.986495108745157,
-0.163476995435478));
#85989=DIRECTION('ref_axis',(-0.991342024823339,0.0313138963622141,-0.127516389980966));
#85990=DIRECTION('center_axis',(-0.0450385595798584,-0.98649510879385,-0.157476755353867));
#85991=DIRECTION('ref_axis',(-0.995577253951608,0.0313138940938735,0.0885741014679431));
#85992=DIRECTION('center_axis',(-0.0778384300520701,-0.986495108830986,
-0.144113077337106));
#85993=DIRECTION('ref_axis',(-0.953260397127133,0.0313138934865127,0.300522969743973));
#85994=DIRECTION('center_axis',(-0.106998666375314,-0.986495108702445,-0.124010829769242));
#85995=DIRECTION('ref_axis',(-0.866370142673745,0.0313138977871995,0.498419718398908));
#85996=DIRECTION('center_axis',(-0.131155757433405,-0.986495108791424,-0.0981099771820695));
#85997=DIRECTION('ref_axis',(-0.738969385524146,0.0313138950364302,0.673010911676559));
#85998=DIRECTION('center_axis',(-0.149180151055395,-0.986495108909675,-0.0676216136185635));
#85999=DIRECTION('ref_axis',(-0.577015238312227,0.0313138897532672,0.816132866060425));
#86000=DIRECTION('center_axis',(-0.160229051121939,-0.986495108808044,-0.033971333126167));
#86001=DIRECTION('ref_axis',(-0.38808050329743,0.0313138924109167,0.921093352002115));
#86002=DIRECTION('center_axis',(-0.163785817251066,-0.986495108829472,0.00126740795685309));
#86003=DIRECTION('ref_axis',(-0.180999553561232,0.0313138929432056,0.982984537884181));
#86004=DIRECTION('center_axis',(0.163393689063109,0.986495109768771,0.0113974021885637));
#86005=DIRECTION('ref_axis',(-0.0794050099347329,0.00163495854620576,0.996841096317671));
#86006=DIRECTION('center_axis',(0.157123533358946,0.986495109699961,0.0462557434581015));
#86007=DIRECTION('ref_axis',(-0.291839933992601,0.00163496610135612,0.956465775557621));
#86008=DIRECTION('center_axis',(0.143506452626063,0.98649510974477,0.0789512286436251));
#86009=DIRECTION('ref_axis',(-0.490628746776434,0.00163496164287221,0.871367178482763));
#86010=DIRECTION('center_axis',(0.123179172730457,0.98649510972553,0.107955036441359));
#86011=DIRECTION('ref_axis',(-0.666476305501507,0.00163496401637486,0.74552442018872));
#86012=DIRECTION('center_axis',(0.0970921703789306,0.986495109704194,0.131910988855437));
#86013=DIRECTION('ref_axis',(-0.811160172091883,0.00163496371730446,0.58482176952086));
#86014=DIRECTION('center_axis',(0.0664652449160892,0.986495109728464,0.149698930190134));
#86015=DIRECTION('ref_axis',(-0.917915092029476,0.00163496284088318,0.396773500527729));
#86016=DIRECTION('center_axis',(0.0327304761927758,0.986495109770256,0.160487115768106));
#86017=DIRECTION('ref_axis',(-0.981749320862673,0.00163495903920392,0.190172547689251));
#86018=DIRECTION('center_axis',(-0.00253472577803093,0.986495109707266,
0.163771101507191));
#86019=DIRECTION('ref_axis',(-0.999678043570141,0.00163496356549726,-0.0253206654319272));
#86020=DIRECTION('center_axis',(-0.0376814169658792,0.986495109780748,0.159397331201352));
#86021=DIRECTION('ref_axis',(-0.970862931954814,0.00163495726033712,-0.239629911052146));
#86022=DIRECTION('center_axis',(-0.0710661533304047,0.986495109669065,0.147570323743763));
#86023=DIRECTION('ref_axis',(-0.896651348677815,0.0016349660250336,-0.442734328689737));
#86024=DIRECTION('center_axis',(-0.101127924003168,0.986495109680366,0.128843088924214));
#86025=DIRECTION('ref_axis',(-0.780513344196942,0.00163496565390908,-0.625136982122972));
#86026=DIRECTION('center_axis',(-0.126461067969803,0.986495109761011,0.10409129024826));
#86027=DIRECTION('ref_axis',(-0.627879402344894,0.00163496041797718,-0.778308925180388));
#86028=DIRECTION('center_axis',(-0.145881030927093,0.986495109831703,0.0744722974923257));
#86029=DIRECTION('ref_axis',(-0.445886520492454,0.00163495483425792,-0.895088005598233));
#86030=DIRECTION('center_axis',(-0.158479755726482,0.986495109780593,0.0413710696483741));
#86031=DIRECTION('ref_axis',(-0.243044480116943,0.00163495717991353,-0.97001376670628));
#86032=DIRECTION('center_axis',(-0.163668144146346,0.986495109748637,0.00633537952423184));
#86033=DIRECTION('ref_axis',(-0.0288379486012532,0.00163496263033163,-0.999582762765379));
#86034=DIRECTION('center_axis',(-0.161203593004104,0.986495109729878,-0.0289965529262278));
#86035=DIRECTION('ref_axis',(0.186717016147342,0.00163496130242488,-0.98241237918838));
#86036=DIRECTION('center_axis',(-0.151201340427938,0.986495109738066,-0.0629726378332434));
#86037=DIRECTION('ref_axis',(0.393541296294608,0.00163496009607257,-0.919305485144217));
#86038=DIRECTION('center_axis',(-0.134129084367225,0.986495109697267,-0.0940041875141071));
#86039=DIRECTION('ref_axis',(0.581964024137621,0.00163496488445213,-0.813212888178349));
#86040=DIRECTION('center_axis',(-0.110785101103599,0.986495109684906,-0.120640208642186));
#86041=DIRECTION('ref_axis',(0.743174760527573,0.00163496707339627,-0.669095361064066));
#86042=DIRECTION('center_axis',(-0.0822609321710779,0.986495109641854,-0.141635227577926));
#86043=DIRECTION('ref_axis',(0.869635471994105,0.00163497154988837,-0.493691677788497));
#86044=DIRECTION('center_axis',(-0.0498903167228879,0.986495109779128,-0.156007546866028));
#86045=DIRECTION('ref_axis',(0.95543299508861,0.0016349575170583,-0.295203520998523));
#86046=DIRECTION('center_axis',(-0.0151869031800958,0.986495109716005,-0.163085120345806));
#86047=DIRECTION('ref_axis',(0.996555533314269,0.00163496265415759,-0.0829119769263292));
#86048=DIRECTION('center_axis',(0.0202266359325298,0.986495109692222,-0.162537016559871));
#86049=DIRECTION('ref_axis',(0.991080242650887,0.00163496541075243,0.133256442677886));
#86050=DIRECTION('center_axis',(0.0546944116456743,0.986495109801367,-0.154388858641817));
#86051=DIRECTION('ref_axis',(0.93926314036049,0.00163495565976323,0.343193939457185));
#86052=DIRECTION('center_axis',(0.0866047237704853,0.986495109744136,-0.139021653966364));
#86053=DIRECTION('ref_axis',(0.843527139657631,0.00163495989678595,0.537084063780664));
#86054=DIRECTION('center_axis',(0.114465497175955,0.986495109730546,-0.117153951849609));
#86055=DIRECTION('ref_axis',(0.708348745149213,0.00163496368711045,0.705860738488321));
#86056=DIRECTION('center_axis',(0.136973995550169,0.986495109745676,-0.0898082568079875));
#86057=DIRECTION('ref_axis',(0.5400487517329,0.00163496073983085,0.841632148064174));
#86058=DIRECTION('center_axis',(0.153077741137595,0.986495109790513,-0.0582632262032798));
#86059=DIRECTION('ref_axis',(0.34649667925581,0.00163495710657844,0.938049773828637));
#86060=DIRECTION('center_axis',(0.162023740072934,0.986495109747255,-0.0239938762505992));
#86061=DIRECTION('ref_axis',(0.136742804768779,0.00163495871085023,0.990605235325345));
#86062=DIRECTION('center_axis',(0.155570611334107,0.98736372189594,-0.0301772360054662));
#86063=DIRECTION('ref_axis',(0.10656539603492,0.0135959508125922,0.994212737038418));
#86064=DIRECTION('',(-0.603590599317291,0.,0.797294417649963));
#86065=DIRECTION('',(-0.797294417685632,0.,-0.603590599270175));
#86066=DIRECTION('center_axis',(-2.16690239644328E-14,-1.,-8.63994232248037E-14));
#86067=DIRECTION('ref_axis',(2.20896655942274E-31,8.63994232248037E-14,
-1.));
#86068=DIRECTION('center_axis',(-0.153257677595439,-0.987363722047016,0.0403108501958945));
#86069=DIRECTION('ref_axis',(0.171510441839821,0.0135962682989244,0.985088478172521));
#86070=DIRECTION('center_axis',(0.157437855436751,-0.987363722701725,-0.0180610289869838));
#86071=DIRECTION('ref_axis',(0.239571732524885,0.0204448268811709,0.970663378328875));
#86072=DIRECTION('center_axis',(0.145446242574693,0.987363721859127,-0.062914793788077));
#86073=DIRECTION('ref_axis',(0.317800305140332,0.0135959530681929,0.94806018591273));
#86074=DIRECTION('',(-0.418084253477456,0.,0.908408254582816));
#86075=DIRECTION('',(-0.908408255110073,0.,-0.418084252331839));
#86076=DIRECTION('center_axis',(0.,-1.,0.));
#86077=DIRECTION('ref_axis',(0.,0.,-1.));
#86078=DIRECTION('center_axis',(-0.141008954754318,-0.987363721980961,0.072314280712722));
#86079=DIRECTION('ref_axis',(0.379265525348352,0.0135962744649355,0.925187982305711));
#86080=DIRECTION('center_axis',(0.149874459410224,-0.98736372263828,-0.0514832558641257));
#86081=DIRECTION('ref_axis',(0.442634611781386,0.0204448284590848,0.896468967361626));
#86082=DIRECTION('center_axis',(0.128520970205328,0.987363721862734,-0.0927105224170952));
#86083=DIRECTION('ref_axis',(0.514175227362223,0.0135959513014948,0.857577393402609));
#86084=DIRECTION('',(-0.213028754318377,0.,0.977045930257918));
#86085=DIRECTION('',(-0.977045930401007,0.,-0.213028753662108));
#86086=DIRECTION('center_axis',(6.52685246616099E-14,-1.,8.08679734183554E-14));
#86087=DIRECTION('ref_axis',(6.18340889097101E-32,-8.08679734183554E-14,
-1.));
#86088=DIRECTION('center_axis',(-0.122166801556987,-0.987363721726011,0.100936384008427));
#86089=DIRECTION('ref_axis',(0.569286579566093,0.0135962907662992,0.822026721708812));
#86090=DIRECTION('center_axis',(0.135303100939358,-0.987363722605958,-0.0824981827551266));
#86091=DIRECTION('ref_axis',(0.625000388726575,0.0204448305551808,0.780356663965395));
#86092=DIRECTION('center_axis',(0.105586198250978,0.987363721838476,-0.118171212806577));
#86093=DIRECTION('ref_axis',(0.686507884976537,0.0135959534087707,0.726995236515308));
#86094=DIRECTION('',(0.00198773449113936,0.,0.999998024453845));
#86095=DIRECTION('',(-0.999998024453727,0.,0.00198773455025544));
#86096=DIRECTION('center_axis',(5.2152947146657E-14,-1.,4.17513353568119E-14));
#86097=DIRECTION('ref_axis',(1.,5.2152947146657E-14,1.83929845959689E-31));
#86098=DIRECTION('center_axis',(-0.0976122826634162,-0.987363722002467,
0.124838787028203));
#86099=DIRECTION('ref_axis',(0.732688419148167,0.0135962746535594,0.680428410460428));
#86100=DIRECTION('center_axis',(0.114405116851751,-0.987363722685321,-0.109655589748638));
#86101=DIRECTION('ref_axis',(0.778141843300161,0.020444828126451,0.627755749243532));
#86102=DIRECTION('center_axis',(0.077714336524821,0.987363721911229,-0.138106345082737));
#86103=DIRECTION('ref_axis',(0.826740198628292,0.0135959500333555,0.562419589021171));
#86104=DIRECTION('',(0.216911277181653,0.,0.976191322349991));
#86105=DIRECTION('',(-0.976191322337167,0.,0.216911277239366));
#86106=DIRECTION('center_axis',(7.32220417368825E-14,-1.,3.61336193395029E-14));
#86107=DIRECTION('ref_axis',(1.,7.32220417368825E-14,4.40866552489188E-31));
#86108=DIRECTION('center_axis',(-0.0684935153893333,-0.987363722021411,
0.142903879533191));
#86109=DIRECTION('ref_axis',(0.861830567147825,0.0135962712680681,0.507014018481997));
#86110=DIRECTION('center_axis',(0.0881576752415342,-0.987363722731981,-0.131685623090954));
#86111=DIRECTION('ref_axis',(0.894898249330239,0.0204448245006342,0.445801673950212));
#86112=DIRECTION('center_axis',(0.0462086360162934,0.987363721869846,-0.151583781100878));
#86113=DIRECTION('ref_axis',(0.928315057984613,0.0135959512476378,0.371545829244113));
#86114=DIRECTION('',(0.421692289376655,0.,0.906738999426117));
#86115=DIRECTION('',(-0.906738999989211,0.,0.421692288165868));
#86116=DIRECTION('center_axis',(-4.32424423825748E-14,-1.,-1.06626877233512E-14));
#86117=DIRECTION('ref_axis',(1.,-4.32424423825748E-14,1.06587266596841E-31));
#86118=DIRECTION('center_axis',(-0.0361720451580659,-0.987363721718911,
0.154286954025493));
#86119=DIRECTION('ref_axis',(0.950674474606201,0.0135962922486553,0.309892213792654));
#86120=DIRECTION('center_axis',(0.0577880837103379,-0.987363722692009,-0.147558180026943));
#86121=DIRECTION('ref_axis',(0.969810207301856,0.020444826699476,0.243002409194558));
#86122=DIRECTION('center_axis',(0.0125422746948997,0.987363721956659,-0.157973326575631));
#86123=DIRECTION('ref_axis',(0.986482938283097,0.0135959480903535,0.163298997767508));
#86124=DIRECTION('',(0.606755441382883,0.,0.794888567254721));
#86125=DIRECTION('',(-0.794888567218748,0.,0.60675544143001));
#86126=DIRECTION('',(0.763447380573604,0.,0.645870031117177));
#86127=DIRECTION('',(-0.645870029654529,0.,0.763447381810991));
#86128=DIRECTION('center_axis',(5.10100782136153E-14,-1.,-9.89314317053015E-15));
#86129=DIRECTION('ref_axis',(1.,5.10100782136153E-14,9.10962590624933E-32));
#86130=DIRECTION('center_axis',(0.0319545315684787,-0.987363721993528,0.155215296937275));
#86131=DIRECTION('ref_axis',(0.992929149174126,0.0135962725467901,-0.117927291553649));
#86132=DIRECTION('center_axis',(-0.009511024361953,-0.987363722641815,-0.158184764204658));
#86133=DIRECTION('ref_axis',(0.982209968780626,0.0204448300012928,-0.186669724792695));
#86134=DIRECTION('center_axis',(-0.0549482154845397,0.987363722017389,-0.148639073123564));
#86135=DIRECTION('ref_axis',(0.96387513573961,0.0135959452699276,-0.266007279928886));
#86136=DIRECTION('',(0.884441369774467,0.,0.466651329615018));
#86137=DIRECTION('',(-0.466651329562727,0.,0.884441369802057));
#86138=DIRECTION('center_axis',(5.45037230112174E-14,-1.,-2.35742925329388E-14));
#86139=DIRECTION('ref_axis',(1.,5.45037230112174E-14,1.05938335290951E-31));
#86140=DIRECTION('center_axis',(0.0645741461527722,-0.987363722058208,0.144717172484823));
#86141=DIRECTION('ref_axis',(0.944364136417791,0.0135962653503995,-0.328620631452744));
#86142=DIRECTION('center_axis',(-0.043293709194828,-0.987363722575933,-0.152441903967217));
#86143=DIRECTION('ref_axis',(0.919117972571777,0.0204448313293298,-0.393451599777483));
#86144=DIRECTION('center_axis',(-0.0856165677881559,0.987363721914613,-0.133351730274106));
#86145=DIRECTION('ref_axis',(0.884156568761363,0.0135959498463249,-0.466992839413957));
#86146=DIRECTION('',(0.964079864249621,0.,0.265612528598395));
#86147=DIRECTION('',(-0.265612528541396,0.,0.964079864265324));
#86148=DIRECTION('center_axis',(-4.21414701015372E-14,-1.,3.03973494430455E-14));
#86149=DIRECTION('ref_axis',(1.,-4.21414701015372E-14,-3.74202457519215E-31));
#86150=DIRECTION('center_axis',(0.0941743565822621,-0.987363722016396,0.127452230299223));
#86151=DIRECTION('ref_axis',(0.851641705444955,0.0135962698329562,-0.523948038447934));
#86152=DIRECTION('center_axis',(-0.0750520328118397,-0.98736372270104,-0.139571026594901));
#86153=DIRECTION('ref_axis',(0.813049042287908,0.0204448268834036,-0.581836114286852));
#86154=DIRECTION('center_axis',(-0.112281580731656,0.987363721908427,-0.111829009150301));
#86155=DIRECTION('ref_axis',(0.763095823305131,0.0135959506265528,-0.646142333066658));
#86156=DIRECTION('',(0.998639054975845,0.,0.0521539823690411));
#86157=DIRECTION('',(-0.05215398216031,0.,0.998639054986746));
#86158=DIRECTION('center_axis',(-9.8919126969435E-15,-1.,1.10702419355046E-14));
#86159=DIRECTION('ref_axis',(3.04300242946951E-32,-1.10702419355046E-14,
-1.));
#86160=DIRECTION('center_axis',(0.11937107706672,-0.98736372199191,0.104227762396657));
#86161=DIRECTION('ref_axis',(0.719097454151467,0.0135962733631525,-0.694776217773402));
#86162=DIRECTION('center_axis',(-0.103301005450512,-0.987363722780564,-0.120173962278935));
#86163=DIRECTION('ref_axis',(0.668962840739906,0.0204448234264662,-0.743014620922265));
#86164=DIRECTION('center_axis',(-0.133696432457323,0.987363721861109,-0.0850772866325803));
#86165=DIRECTION('ref_axis',(0.606353563973455,0.0135959524929253,-0.795078930378927));
#86166=DIRECTION('',(0.986502993673533,0.,-0.163743224205332));
#86167=DIRECTION('',(0.163743224263852,0.,0.986502993663819));
#86168=DIRECTION('center_axis',(1.45617409646071E-14,-1.,-2.58757892796229E-14));
#86169=DIRECTION('ref_axis',(7.31829950293539E-33,2.58757892796229E-14,
-1.));
#86170=DIRECTION('center_axis',(0.138986134014219,-0.987363722017432,0.076129724783847));
#86171=DIRECTION('ref_axis',(0.552929007076716,0.0135962705645634,-0.833117431434424));
#86172=DIRECTION('center_axis',(-0.126719731068657,-0.98736372256976,-0.0951577065248656));
#86173=DIRECTION('ref_axis',(0.493596682389456,0.0204448315520646,-0.869450587438372));
#86174=DIRECTION('center_axis',(-0.148859783585737,0.987363721978464,-0.0543474502772831));
#86175=DIRECTION('ref_axis',(0.421258887391482,0.0135959476505099,-0.906838519253111));
#86176=DIRECTION('',(0.928239148269088,0.,-0.37198398301631));
#86177=DIRECTION('',(0.371983982078545,0.,0.928239148644889));
#86178=DIRECTION('center_axis',(2.38116057765714E-14,-1.,-7.8103221770465E-14));
#86179=DIRECTION('ref_axis',(-2.79864792815286E-31,7.8103221770465E-14,
-1.));
#86180=DIRECTION('center_axis',(0.152102356226166,-0.987363722014895,0.0444719426081411));
#86181=DIRECTION('ref_axis',(0.360906212233439,0.0135962715702553,-0.932503001266323));
#86182=DIRECTION('center_axis',(-0.144213189673931,-0.987363722716407,-0.0656919704961667));
#86183=DIRECTION('ref_axis',(0.295150489684352,0.020444826116553,-0.955232012405443));
#86184=DIRECTION('center_axis',(-0.157062621723428,0.987363721820909,-0.0210763775190806));
#86185=DIRECTION('ref_axis',(0.216466612364278,0.0135959542449752,-0.976195347130738));
#86186=DIRECTION('',(0.826571873636816,0.,-0.562831180472905));
#86187=DIRECTION('',(0.562831181859169,0.,0.826571872692878));
#86188=DIRECTION('center_axis',(4.70183251359275E-15,-1.,-5.91970933019358E-14));
#86189=DIRECTION('ref_axis',(-6.63462100443905E-32,5.91970933019358E-14,
-1.));
#86190=DIRECTION('center_axis',(0.158106440927349,-0.987363722001391,0.0107347013394576));
#86191=DIRECTION('ref_axis',(0.152007846781394,0.0135962733988064,-0.988285766297658));
#86192=DIRECTION('center_axis',(-0.154963397163516,-0.987363722655234,-0.0331545581171144));
#86193=DIRECTION('ref_axis',(0.0829033887011708,0.0204448284530127,-0.996347849463926));
#86194=DIRECTION('center_axis',(-0.15792138294966,0.987363721859615,0.0131801958557069));
#86195=DIRECTION('ref_axis',(0.00155260087807025,0.0135959528525333,-0.99990636536455));
#86196=DIRECTION('',(0.686255015216422,0.,-0.727361020463916));
#86197=DIRECTION('',(0.727361020504861,0.,0.686255015173024));
#86198=DIRECTION('center_axis',(-5.08357432511528E-15,-1.,-3.67649082105399E-14));
#86199=DIRECTION('ref_axis',(-5.70858969985437E-32,3.67649082105399E-14,
-1.));
#86200=DIRECTION('center_axis',(0.156717643447317,-0.98736372201751,-0.02350448204169));
#86201=DIRECTION('ref_axis',(-0.0639982407964878,0.0135962738668925,-0.99785738786256));
#86202=DIRECTION('center_axis',(-0.158467688440349,-0.987363722742572,0.000933130377306471));
#86203=DIRECTION('ref_axis',(-0.133220182211163,0.0204448247090343,-0.990875568471764));
#86204=DIRECTION('center_axis',(-0.15139591711616,0.987363721932101,0.0468204751465142));
#86205=DIRECTION('ref_axis',(-0.213434009684826,0.0135959484370491,-0.976862873537507));
#86206=DIRECTION('',(0.513849635801822,0.,-0.857880266579396));
#86207=DIRECTION('',(0.857880267877561,0.,0.513849633634515));
#86208=DIRECTION('center_axis',(-2.05889466985223E-14,-1.,-5.57000749948014E-14));
#86209=DIRECTION('ref_axis',(-2.77140440273355E-31,5.57000749948014E-14,
-1.));
#86210=DIRECTION('center_axis',(0.148000904436245,-0.987363722001798,-0.0566446181098321));
#86211=DIRECTION('ref_axis',(-0.277011838133409,0.0135962708098426,-0.960770307073452));
#86212=DIRECTION('center_axis',(-0.154562208248359,-0.987363722638707,0.0349771782513351));
#86213=DIRECTION('ref_axis',(-0.343114525414335,0.0204448298680979,-0.939071047036038));
#86214=DIRECTION('center_axis',(-0.137791347031469,0.987363721984853,0.0782714838972129));
#86215=DIRECTION('ref_axis',(-0.418440681523933,0.0135959471253179,-0.908142360132789));
#86216=DIRECTION('',(0.317417216373473,0.,-0.948285985739384));
#86217=DIRECTION('',(0.948285986047992,0.,0.317417215451505));
#86218=DIRECTION('center_axis',(4.01018227942412E-14,-1.,6.24647791306544E-14));
#86219=DIRECTION('ref_axis',(-5.68566147680559E-31,-6.24647791306544E-14,
-1.));
#86220=DIRECTION('center_axis',(0.132363804604318,-0.98736372196756,-0.0871361220908843));
#86221=DIRECTION('ref_axis',(-0.477072672688627,0.0135962753491566,-0.878758673510743));
#86222=DIRECTION('center_axis',(-0.143429568774726,-0.987363722694813,0.0673857396437633));
#86223=DIRECTION('ref_axis',(-0.536965214303182,0.0204448268453923,-0.843356607659891));
#86224=DIRECTION('center_axis',(-0.11774380298488,0.987363721851963,0.10606261183517));
#86225=DIRECTION('ref_axis',(-0.603881533767801,0.0135959535221113,-0.796958118863264));
#86226=DIRECTION('',(0.106142721135687,0.,-0.994350905239147));
#86227=DIRECTION('',(0.994350904942087,0.,0.106142723918561));
#86228=DIRECTION('center_axis',(-3.15554073413638E-14,-1.,-3.14302085104392E-14));
#86229=DIRECTION('ref_axis',(1.,-3.15554073413638E-14,-3.88230226445637E-31));
#86230=DIRECTION('center_axis',(0.110537521518214,-0.98736372195799,-0.113553233762299));
#86231=DIRECTION('ref_axis',(-0.654826117545247,0.0135962759388342,-0.755657261634674));
#86232=DIRECTION('center_axis',(-0.125590323971213,-0.987363722658905,0.0966434152022493));
#86233=DIRECTION('ref_axis',(-0.705708007468931,0.0204448281709577,-0.708207750024872));
#86234=DIRECTION('center_axis',(-0.0921906931258788,0.98736372187097,0.128894363081076));
#86235=DIRECTION('ref_axis',(-0.761085557922345,0.0135959516747523,-0.648509000415639));
#86236=DIRECTION('',(-0.110094884194222,0.,-0.993921081612751));
#86237=DIRECTION('',(0.993921081291397,0.,-0.110094887095358));
#86238=DIRECTION('center_axis',(5.63613377604692E-14,-1.,3.58678618036695E-14));
#86239=DIRECTION('ref_axis',(1.,5.63613377604692E-14,-4.20975683792422E-31));
#86240=DIRECTION('center_axis',(0.0835426327848654,-0.987363722032105,-0.134660717814369));
#86241=DIRECTION('ref_axis',(-0.80196062057044,0.0135962689252322,-0.597222156760436));
#86242=DIRECTION('center_axis',(-0.101878612833617,-0.987363722718959,0.121382153983431));
#86243=DIRECTION('ref_axis',(-0.841452678222415,0.0204448262750383,-0.539943885409317));
#86244=DIRECTION('center_axis',(-0.0623268517272042,0.987363721958143,0.145699156190894));
#86245=DIRECTION('ref_axis',(-0.882702065230997,0.0135959474982537,-0.469736324174061));
#86246=DIRECTION('',(-0.321184582171429,0.,-0.947016612407282));
#86247=DIRECTION('',(0.947016612388014,0.,-0.321184582228242));
#86248=DIRECTION('center_axis',(-0.0295486726347458,0.98736372195704,0.15569122168146));
#86249=DIRECTION('ref_axis',(-0.963044405676187,0.0135959478040231,-0.268999299068065));
#86250=DIRECTION('',(-0.51725604351836,0.,-0.855830699054277));
#86251=DIRECTION('center_axis',(-3.48634287493128E-14,-1.,-1.27295943479517E-14));
#86252=DIRECTION('ref_axis',(1.,-3.48634287493128E-14,5.74501590485154E-32));
#86253=DIRECTION('center_axis',(0.05264137310468,-0.987363721985138,-0.149471623879952));
#86254=DIRECTION('ref_axis',(-0.911596337546528,0.0135962747113278,-0.410861605270839));
#86255=DIRECTION('center_axis',(-0.0734031758498871,-0.987363722626589,
0.140445195774421));
#86256=DIRECTION('ref_axis',(-0.937851956604742,0.0204448298265036,-0.346432845478055));
#86257=DIRECTION('',(0.855830699792872,0.,-0.517256042296312));
#86258=DIRECTION('center_axis',(-1.02997516282883E-13,-1.,-1.38246550625899E-14));
#86259=DIRECTION('ref_axis',(1.,-1.02997516282883E-13,-1.76484519791174E-31));
#86260=DIRECTION('center_axis',(0.00461117005004301,0.987363721951836,0.158403338614394));
#86261=DIRECTION('ref_axis',(-0.998355860480601,0.0135959481915025,-0.0556841632496482));
#86262=DIRECTION('center_axis',(0.0192786466928749,-0.987363721692602,-0.157293403761965));
#86263=DIRECTION('ref_axis',(-0.978606822198162,0.0135962945650253,-0.205289620588369));
#86264=DIRECTION('center_axis',(-0.0414954808748873,-0.98736372271376,0.152941178679215));
#86265=DIRECTION('ref_axis',(-0.99039832053053,0.0204448259328905,-0.136722989225951));
#86266=DIRECTION('',(-0.6891411857498,0.,-0.724627094513695));
#86267=DIRECTION('',(0.724627094472951,0.,-0.689141185792642));
#86268=DIRECTION('center_axis',(1.47944833905471E-14,-1.,-1.23428272891312E-15));
#86269=DIRECTION('ref_axis',(1.,1.47944833905471E-14,-1.04793950114792E-32));
#86270=DIRECTION('center_axis',(-0.0149854826176444,-0.987363722043136,
-0.157760310927184));
#86271=DIRECTION('ref_axis',(-0.999858739051166,0.0135962683570005,0.0098814690090491));
#86272=DIRECTION('center_axis',(-0.00764751232626353,-0.987363722585862,
0.158285801247647));
#86273=DIRECTION('ref_axis',(-0.996634759231673,0.0204448312899083,0.0793798813601607));
#86274=DIRECTION('center_axis',(0.0385554024431205,0.987363721891044,0.153708690827534));
#86275=DIRECTION('ref_axis',(-0.986985304127919,0.0135959516543579,0.16023470140432));
#86276=DIRECTION('',(-0.828802852674338,0.,-0.559540732564555));
#86277=DIRECTION('',(0.559540732515555,0.,-0.828802852707419));
#86278=DIRECTION('center_axis',(-4.96414180061546E-14,-1.,1.5350308719234E-14));
#86279=DIRECTION('ref_axis',(1.,-4.96414180061546E-14,-8.98706406991303E-33));
#86280=DIRECTION('center_axis',(-0.0485489594385595,-0.987363721707173,
-0.150850520695132));
#86281=DIRECTION('ref_axis',(-0.974358371712792,0.0135962938640854,0.224590525771589));
#86282=DIRECTION('center_axis',(0.0265580544860549,-0.987363722702375,0.156229154875853));
#86283=DIRECTION('ref_axis',(-0.956269664959881,0.0204448268694524,0.291771035114516));
#86284=DIRECTION('center_axis',(0.0706968220400096,0.987363721900133,0.14182679587779));
#86285=DIRECTION('ref_axis',(-0.929464413230009,0.0135959506144346,0.368661165117625));
#86286=DIRECTION('',(-0.929710620732484,0.,-0.368290865617407));
#86287=DIRECTION('',(0.368290866546792,0.,-0.929710620364322));
#86288=DIRECTION('center_axis',(-4.51809666877942E-14,-1.,2.56628645547669E-14));
#86289=DIRECTION('ref_axis',(1.,-4.51809666877942E-14,-2.20183821085922E-31));
#86290=DIRECTION('center_axis',(-0.0798422943103286,-0.987363721988475,
-0.136887137965287));
#86291=DIRECTION('ref_axis',(-0.903298092113965,0.0135962716534009,0.428797968955542));
#86292=DIRECTION('center_axis',(0.059521789918778,-0.987363722621634,0.146867408827195));
#86293=DIRECTION('ref_axis',(-0.871190463336196,0.0204448296496739,0.490519301896122));
#86294=DIRECTION('center_axis',(0.0995325402727057,0.987363721842399,0.123313236176773));
#86295=DIRECTION('ref_axis',(-0.82848279735365,0.0135959524090879,0.559849448126155));
#86296=DIRECTION('',(-0.987146152503824,0.,-0.159820128885245));
#86297=DIRECTION('',(0.159820128826887,0.,-0.987146152513272));
#86298=DIRECTION('center_axis',(3.86079034210145E-14,-1.,-3.47754532654341E-14));
#86299=DIRECTION('ref_axis',(1.,3.86079034210145E-14,3.58398621757385E-31));
#86300=DIRECTION('center_axis',(-0.107402316184702,-0.987363721994453,-0.116523057664233));
#86301=DIRECTION('ref_axis',(-0.790000597333135,0.0135962746960822,0.61295529814798));
#86302=DIRECTION('center_axis',(0.0897023546254517,-0.98736372263455,0.130638305254982));
#86303=DIRECTION('ref_axis',(-0.745375363963095,0.0204448301796836,0.66633143083289));
#86304=DIRECTION('center_axis',(0.123714222696916,0.987363721947433,0.0990336896445395));
#86305=DIRECTION('ref_axis',(-0.688762246509255,0.0135959484644339,0.724859791938329));
#86306=DIRECTION('',(-0.998423827575672,0.,0.0561236182827234));
#86307=DIRECTION('',(-0.0561236183417539,0.,-0.998423827572354));
#86308=DIRECTION('center_axis',(-2.59110665239106E-14,-1.,3.62245547218756E-14));
#86309=DIRECTION('ref_axis',(5.84001265530547E-32,-3.62245547218756E-14,
-1.));
#86310=DIRECTION('center_axis',(-0.129940334603434,-0.987363721715944,-0.0907104761446398));
#86311=DIRECTION('ref_axis',(-0.639763549392157,0.0135962927576524,0.768451522018402));
#86312=DIRECTION('center_axis',(0.11568853959148,-0.987363722702958,0.108300696661411));
#86313=DIRECTION('ref_axis',(-0.58470734183779,0.020444826339279,0.810986641984282));
#86314=DIRECTION('center_axis',(0.142111167041916,0.987363721998744,0.0701234388972172));
#86315=DIRECTION('ref_axis',(-0.516835941609039,0.0135959455452013,0.855976494844239));
#86316=DIRECTION('',(-0.963016313438974,0.,0.269443092415463));
#86317=DIRECTION('',(-0.269443091726455,0.,-0.963016313631752));
#86318=DIRECTION('center_axis',(-8.75903587034078E-15,-1.,2.04738791027141E-14));
#86319=DIRECTION('ref_axis',(-3.62806814991581E-32,-2.04738791027141E-14,
-1.));
#86320=DIRECTION('center_axis',(-0.14640246408389,-0.987363721985062,-0.060656401294257));
#86321=DIRECTION('ref_axis',(-0.459611873173492,0.013596274118306,0.888015803557602));
#86322=DIRECTION('center_axis',(0.136265253015123,-0.987363722600714,0.0808990736212951));
#86323=DIRECTION('ref_axis',(-0.39669905330566,0.0204448300118289,0.917721019717964));
#86324=DIRECTION('center_axis',(0.153863154833479,0.987363721917656,0.0379342882574982));
#86325=DIRECTION('ref_axis',(-0.320742961130513,0.0135959494123135,0.947068689718337));
#86326=DIRECTION('',(-0.882579228239459,0.,0.470163701151249));
#86327=DIRECTION('',(-0.470163700157015,0.,-0.882579228769103));
#86328=DIRECTION('center_axis',(1.66119026794174E-14,-1.,-8.75125797881813E-14));
#86329=DIRECTION('ref_axis',(7.00951663590181E-32,8.75125797881813E-14,
-1.));
#86330=DIRECTION('center_axis',(-0.156018993575103,-0.987363721745371,-0.0277660696704074));
#86331=DIRECTION('ref_axis',(-0.257969252019171,0.0135962909953125,0.966057454752998));
#86332=DIRECTION('center_axis',(0.150470357297635,-0.987363722706508,0.0497146925754064));
#86333=DIRECTION('ref_axis',(-0.190141558768352,0.0204448255908761,0.981543782383496));
#86334=DIRECTION('center_axis',(0.158420670878443,0.987363721854469,0.00397137307680872));
#86335=DIRECTION('ref_axis',(-0.109652395100579,0.0135959518425372,0.993877005641142));
#86336=DIRECTION('',(-0.760873717902008,0.,0.648899981049449));
#86337=DIRECTION('center_axis',(-1.51030376905466E-15,-1.,-5.19386305601871E-14));
#86338=DIRECTION('ref_axis',(0.0290663354547457,-5.19605846959252E-14,0.999577484812074));
#86339=DIRECTION('center_axis',(-0.158340239529416,-0.987363722011645,0.00642253852296898));
#86340=DIRECTION('ref_axis',(-0.0442642795989572,0.0135962721816249,0.998927332159026));
#86341=DIRECTION('center_axis',(0.157639633367977,-0.98736372267693,0.0162057129791808));
#86342=DIRECTION('ref_axis',(0.0253067453442215,0.0204448270264858,0.99947064873759));
#86343=DIRECTION('',(-0.648899979430115,0.,-0.760873719283033));
#86344=DIRECTION('center_axis',(-0.158362916807467,-0.987363722049377,-0.00583669093171205));
#86345=DIRECTION('ref_axis',(-0.150968894543394,0.018371221016767,0.988367791421138));
#86346=DIRECTION('',(0.563065840553494,0.,0.826412039603603));
#86347=DIRECTION('',(0.82641203914066,0.,-0.563065841232956));
#86348=DIRECTION('center_axis',(-0.15340576406886,-0.987363722034686,-0.039743577597651));
#86349=DIRECTION('ref_axis',(-0.359909186701557,0.0183712220704353,0.932806451268141));
#86350=DIRECTION('',(0.372247514396375,0.,0.928133496877319));
#86351=DIRECTION('center_axis',(1.73014035762452E-14,-1.,-5.68072586656539E-14));
#86352=DIRECTION('ref_axis',(-4.14833769841157E-31,5.68072586656539E-14,
-1.));
#86353=DIRECTION('center_axis',(0.157639635048058,0.987363722095099,0.0162057320855101));
#86354=DIRECTION('ref_axis',(-0.21543524078911,0.018370881756947,0.976345311726138));
#86355=DIRECTION('center_axis',(-0.156429986875914,0.987363722026089,-0.0253483654855673));
#86356=DIRECTION('ref_axis',(-0.287973013507099,-0.0210448339910764,0.957407258408838));
#86357=DIRECTION('',(0.928133496571451,0.,-0.372247515159002));
#86358=DIRECTION('center_axis',(-0.141275528519,-0.987363722023162,-0.0717920989680929));
#86359=DIRECTION('ref_axis',(-0.552020522473789,0.0183712225113625,0.8336281190982));
#86360=DIRECTION('',(0.164023306625657,0.,0.98645646375478));
#86361=DIRECTION('center_axis',(1.45543938869861E-14,-1.,-2.58799230889811E-14));
#86362=DIRECTION('ref_axis',(3.67946996634454E-31,2.58799230889811E-14,
-1.));
#86363=DIRECTION('center_axis',(0.150470353914268,0.987363722120268,0.0497147144588495));
#86364=DIRECTION('ref_axis',(-0.420283866394558,0.0183708800064232,0.907206692224121));
#86365=DIRECTION('center_axis',(-0.147323591242544,0.987363722045255,-0.0583835580650956));
#86366=DIRECTION('ref_axis',(-0.487054623391906,-0.021044833616294,0.873117923771257));
#86367=DIRECTION('',(0.98645646307743,0.,-0.164023310699326));
#86368=DIRECTION('center_axis',(-0.122539408226903,-0.987363722003608,-0.100483699685982));
#86369=DIRECTION('ref_axis',(-0.718319992977518,0.018371225795244,0.695470262305699));
#86370=DIRECTION('',(-0.0518704469154818,0.,0.998653822271155));
#86371=DIRECTION('center_axis',(1.97775386860055E-14,-1.,-2.21461003884614E-14));
#86372=DIRECTION('ref_axis',(-1.13301816167624E-30,2.21461003884614E-14,
-1.));
#86373=DIRECTION('center_axis',(0.136265247913238,0.987363722105047,0.0808990882644076));
#86374=DIRECTION('ref_axis',(-0.605480484557487,0.018370882320908,0.795648096524325));
#86375=DIRECTION('center_axis',(-0.131328506624462,0.987363722081932,-0.0886888023614173));
#86376=DIRECTION('ref_axis',(-0.66336210148133,-0.0210448308065385,0.748002565112312));
#86377=DIRECTION('',(0.998653822462692,0.,0.0518704432278523));
#86378=DIRECTION('center_axis',(-0.0980734813275416,-0.987363721991955,
-0.124476796048459));
#86379=DIRECTION('ref_axis',(-0.851031619179291,0.0183712277123154,0.524792988853144));
#86380=DIRECTION('',(-0.265338796268726,0.,0.964155238120223));
#86381=DIRECTION('center_axis',(0.,-1.,0.));
#86382=DIRECTION('ref_axis',(0.,0.,-1.));
#86383=DIRECTION('center_axis',(0.115688529441642,0.987363722089161,0.108300713099541));
#86384=DIRECTION('ref_axis',(-0.762365509257207,0.0183708822016604,0.64688587941161));
#86385=DIRECTION('center_axis',(-0.109192647626212,0.987363722133983,-0.114847054459851));
#86386=DIRECTION('ref_axis',(-0.808651505534936,-0.0210448304026786,0.587911436960877));
#86387=DIRECTION('',(0.964155239073708,0.,0.26533879280407));
#86388=DIRECTION('center_axis',(-0.0690217373890758,-0.987363722105139,
-0.142649500659764));
#86389=DIRECTION('ref_axis',(-0.943949953433183,0.0183712184221452,0.329576976967713));
#86390=DIRECTION('',(-0.466400199211432,0.,0.884573826300291));
#86391=DIRECTION('center_axis',(8.17455424435588E-14,-1.,-3.53846501850613E-14));
#86392=DIRECTION('ref_axis',(1.,8.17455424435588E-14,-6.2833906170899E-31));
#86393=DIRECTION('center_axis',(0.0897023381817425,0.987363722254612,0.130638319417566));
#86394=DIRECTION('ref_axis',(-0.883603169697384,0.0183708757720218,0.46787599791409));
#86395=DIRECTION('center_axis',(-0.0819510660883673,0.987363722030276,-0.135635184172474));
#86396=DIRECTION('ref_axis',(-0.916129262541471,-0.0210448342814313,0.400330225270697));
#86397=DIRECTION('',(0.884573827309106,0.,0.466400197298114));
#86398=DIRECTION('center_axis',(-0.0367426329069288,-0.987363721970691,
-0.154152066036269));
#86399=DIRECTION('ref_axis',(-0.992730235309415,0.0183712295096434,0.118950316640258));
#86400=DIRECTION('',(-0.645653245721451,0.,0.763630726391595));
#86401=DIRECTION('center_axis',(2.91470103242875E-14,-1.,-5.6615004967518E-15));
#86402=DIRECTION('ref_axis',(1.,2.91470103242875E-14,2.0698037467484E-32));
#86403=DIRECTION('center_axis',(0.0595217788484243,0.987363722020597,0.146867417354402));
#86404=DIRECTION('ref_axis',(-0.963524527467881,0.0183708844563654,0.266988755516199));
#86405=DIRECTION('center_axis',(-0.0508775378651978,0.987363722085364,-0.150081166208527));
#86406=DIRECTION('ref_axis',(-0.980769834430407,-0.0210448317193077,0.194030015536922));
#86407=DIRECTION('',(0.763630725504702,0.,0.645653246770403));
#86408=DIRECTION('center_axis',(-0.00274546586929473,-0.987363722062483,
-0.158446655919526));
#86409=DIRECTION('ref_axis',(-0.995091555744463,0.0183712228409193,-0.0972383353281675));
#86410=DIRECTION('',(-0.794716264791645,0.,0.606981102239283));
#86411=DIRECTION('center_axis',(2.9682624687141E-14,-1.,7.36607880923249E-16));
#86412=DIRECTION('ref_axis',(-0.999692221971624,-2.96917631589623E-14,-0.0248084930908046));
#86413=DIRECTION('center_axis',(0.026558039131714,0.98736372202967,0.15622916173748));
#86414=DIRECTION('ref_axis',(-0.998392549720632,0.0183708840716378,0.0536174158344317));
#86415=DIRECTION('center_axis',(-0.0174250346579384,0.987363722105934,-0.157509518557722));
#86416=DIRECTION('ref_axis',(-0.999550698583589,-0.0210448314459766,-0.0213428215208139));
#86417=DIRECTION('',(0.606981102892691,0.,0.794716264292592));
#86418=DIRECTION('center_axis',(0.0313800669307913,-0.987363722011099,-0.155332455899623));
#86419=DIRECTION('ref_axis',(-0.950923500765827,0.0183712248308667,-0.308880225636862));
#86420=DIRECTION('',(-0.90661923571427,0.,0.4219497143415));
#86421=DIRECTION('center_axis',(5.76606249419919E-14,-1.,1.42005465698906E-14));
#86422=DIRECTION('ref_axis',(1.,5.76606249419919E-14,6.7939237826861E-31));
#86423=DIRECTION('center_axis',(-0.00764752810225059,0.987363722126267,
0.158285803352323));
#86424=DIRECTION('ref_axis',(-0.986576846474386,0.0183708803886285,-0.162261014277621));
#86425=DIRECTION('center_axis',(0.0168422438111064,0.987363722105163,-0.157572900887325));
#86426=DIRECTION('ref_axis',(-0.971593683228542,-0.021044830978553,-0.235717690892048));
#86427=DIRECTION('',(0.421949717449873,-2.49350828777751E-15,0.906619234267602));
#86428=DIRECTION('center_axis',(0.0640383063061008,-0.987363722036451,-0.144955081772845));
#86429=DIRECTION('ref_axis',(-0.862291320331763,0.0183712229205566,-0.506079220131501));
#86430=DIRECTION('',(-0.976129697219472,0.,0.217188430184996));
#86431=DIRECTION('center_axis',(1.33149634599131E-13,-1.,6.56596890341522E-14));
#86432=DIRECTION('ref_axis',(1.,1.33149634599131E-13,-2.52920306949116E-30));
#86433=DIRECTION('center_axis',(-0.041495503895507,0.98736372218836,0.152941175825237));
#86434=DIRECTION('ref_axis',(-0.928629905547145,0.0183708786055248,-0.370552303113557));
#86435=DIRECTION('center_axis',(0.0503220003050336,0.987363722191509,-0.150268347916085));
#86436=DIRECTION('ref_axis',(-0.898206026753204,-0.0210448277626684,-0.439070664846402));
#86437=DIRECTION('',(0.217188431596517,0.,0.976129696905409));
#86438=DIRECTION('center_axis',(0.0937021797661748,-0.987363721991622,-0.127799773090246));
#86439=DIRECTION('ref_axis',(-0.733339355073252,0.018371228609779,-0.679614514456625));
#86440=DIRECTION('',(-0.99999741978848,0.,0.00227165498764559));
#86441=DIRECTION('center_axis',(6.95530666805971E-14,-1.,5.5648702500083E-14));
#86442=DIRECTION('ref_axis',(1.,6.95530666805971E-14,-2.69781625273742E-30));
#86443=DIRECTION('center_axis',(-0.0734031933831537,0.98736372216877,0.140445189829294));
#86444=DIRECTION('ref_axis',(-0.827261262436935,0.018370879413501,-0.561516976110984));
#86445=DIRECTION('center_axis',(0.0814487490481949,0.987363722058279,-0.135937418107396));
#86446=DIRECTION('ref_axis',(-0.782819254446178,-0.0210448328580041,-0.62189318204842));
#86447=DIRECTION('',(0.00227165580984504,0.,0.999997419786612));
#86448=DIRECTION('center_axis',(0.118984650603525,-0.987363722022246,-0.104668683736512));
#86449=DIRECTION('ref_axis',(-0.570097257187399,0.0183712249409984,-0.82137178880308));
#86450=DIRECTION('',(-0.97710637405149,0.,-0.212751342623141));
#86451=DIRECTION('center_axis',(5.5964128605694E-14,-1.,6.92995201892614E-14));
#86452=DIRECTION('ref_axis',(1.46790450287485E-30,-6.92995201892614E-14,
-1.));
#86453=DIRECTION('center_axis',(-0.101878629409016,0.987363722040531,0.121382145589907));
#86454=DIRECTION('ref_axis',(-0.687210802807775,0.0183708831942544,-0.726225738427767));
#86455=DIRECTION('center_axis',(0.108767048569711,0.987363722075025,-0.115250203798458));
#86456=DIRECTION('ref_axis',(-0.630828724288943,-0.0210448335494104,-0.775636664678032));
#86457=DIRECTION('',(-0.21275134122214,0.,0.977106374356539));
#86458=DIRECTION('center_axis',(0.138703528583435,-0.987363722005588,-0.0766434056248631));
#86459=DIRECTION('ref_axis',(-0.380198045567245,0.0183712251232356,-0.924722630973374));
#86460=DIRECTION('',(-0.908526921025632,0.,-0.417826320104041));
#86461=DIRECTION('center_axis',(1.32527900101837E-14,-1.,2.65699897642818E-14));
#86462=DIRECTION('ref_axis',(-3.85703025017377E-31,-2.65699897642817E-14,
-1.));
#86463=DIRECTION('center_axis',(-0.125590338476727,0.987363722139054,0.0966434016630939));
#86464=DIRECTION('ref_axis',(-0.515027128630378,0.018370879941791,-0.856976993591375));
#86465=DIRECTION('center_axis',(0.130999522454367,0.987363722018216,-0.0891740184081779));
#86466=DIRECTION('ref_axis',(-0.449341343911688,-0.0210448341519091,-0.893112239087091));
#86467=DIRECTION('',(-0.41782632044881,0.,0.908526920867075));
#86468=DIRECTION('center_axis',(0.151936783382105,-0.987363721993645,-0.0450343685017907));
#86469=DIRECTION('ref_axis',(-0.172521198272612,0.0183712264494477,-0.984834470449387));
#86470=DIRECTION('',(-0.797465757841021,0.,-0.603364205990914));
#86471=DIRECTION('center_axis',(7.23118474322659E-15,-1.,2.87977562494652E-14));
#86472=DIRECTION('ref_axis',(9.73713914984225E-33,-2.87977562494652E-14,
-1.));
#86473=DIRECTION('center_axis',(-0.143429581007702,0.987363722192312,0.0673857209688961));
#86474=DIRECTION('ref_axis',(-0.318761360374116,0.0183708783634438,-0.947656955844571));
#86475=DIRECTION('center_axis',(0.147106605348864,0.987363722149102,-0.0589281498657818));
#86476=DIRECTION('ref_axis',(-0.246843263567107,-0.0210448291783784,-0.968826877412261));
#86477=DIRECTION('',(-0.603364203506953,0.,0.797465759720391));
#86478=DIRECTION('',(-0.649115982975384,0.,-0.760689450857511));
#86479=DIRECTION('',(-0.760689450324139,0.,0.649115983600434));
#86480=DIRECTION('center_axis',(0.15680352997555,-0.987363722031627,0.0229245153287668));
#86481=DIRECTION('ref_axis',(0.256945263434263,0.0183712248304825,-0.966251328432166));
#86482=DIRECTION('',(-0.470414265591835,0.,-0.882445702991235));
#86483=DIRECTION('center_axis',(-3.31741108596706E-14,-1.,1.75034588439747E-13));
#86484=DIRECTION('ref_axis',(1.88543075864206E-30,-1.75034588439748E-13,
-1.));
#86485=DIRECTION('center_axis',(-0.158467693351964,0.987363721969067,0.000933114729498503));
#86486=DIRECTION('ref_axis',(0.108610850412292,0.0183708869075653,-0.99391458067932));
#86487=DIRECTION('center_axis',(0.158253627755301,0.987363722053648,0.00828671675958859));
#86488=DIRECTION('ref_axis',(0.182770968834695,-0.0210448325953407,-0.982930255904386));
#86489=DIRECTION('',(-0.882445701968546,0.,0.470414267510287));
#86490=DIRECTION('center_axis',(0.148209457615993,-0.98736372200383,0.0560966767635802));
#86491=DIRECTION('ref_axis',(0.458653501977566,0.0183712253838114,-0.888425271591039));
#86492=DIRECTION('',(-0.269716499743633,0.,-0.962939774734663));
#86493=DIRECTION('center_axis',(1.16709635174659E-14,-1.,-2.73018206340956E-14));
#86494=DIRECTION('ref_axis',(-1.0314733824329E-31,2.73018206340956E-14,
-1.));
#86495=DIRECTION('center_axis',(-0.154963396044541,0.987363722152497,-0.0331545783189781));
#86496=DIRECTION('ref_axis',(0.31973384434166,0.0183708788110592,-0.94732928783724));
#86497=DIRECTION('center_axis',(0.152772346968418,0.987363722044585,0.0421128293044433));
#86498=DIRECTION('ref_axis',(0.389798836580696,-0.0210448335722502,-0.920659536408683));
#86499=DIRECTION('',(-0.962939774722175,0.,0.269716499788217));
#86500=DIRECTION('center_axis',(0.132685277493759,-0.987363721998059,0.0866458170862475));
#86501=DIRECTION('ref_axis',(0.638915607237054,0.0183712283842684,-0.769057439205005));
#86502=DIRECTION('',(-0.0564070903287917,0.,-0.99840785261367));
#86503=DIRECTION('center_axis',(1.72671872884761E-14,-1.,-2.41546070876787E-14));
#86504=DIRECTION('ref_axis',(2.74088008315019E-31,2.41546070876787E-14,
-1.));
#86505=DIRECTION('center_axis',(-0.144213188967013,0.987363721902049,-0.0656919842880165));
#86506=DIRECTION('ref_axis',(0.515906438873904,0.0183708884535525,-0.856447929991003));
#86507=DIRECTION('center_axis',(0.140147600266339,0.987363722073609,0.0739697943253586));
#86508=DIRECTION('ref_axis',(0.578600140813818,-0.0210448321666288,-0.815339801609923));
#86509=DIRECTION('',(-0.998407852567306,0.,0.0564070911494373));
#86510=DIRECTION('center_axis',(0.110956879050134,-0.987363721968771,0.113143499731222));
#86511=DIRECTION('ref_axis',(0.789302732667269,0.0183712271502386,-0.613729333026356));
#86512=DIRECTION('',(0.159539850457337,0.,-0.987191489082058));
#86513=DIRECTION('center_axis',(-2.20560165650436E-14,-1.,1.98779509493039E-14));
#86514=DIRECTION('ref_axis',(1.,-2.20560165650436E-14,-6.51911231040562E-31));
#86515=DIRECTION('center_axis',(-0.126719727502218,0.987363722008613,-0.0951577170967375));
#86516=DIRECTION('ref_axis',(0.687955821391077,0.0183708850872274,-0.725520019293224));
#86517=DIRECTION('center_axis',(0.12096970734739,0.987363722095569,0.102368013528986));
#86518=DIRECTION('ref_axis',(0.740346747930026,-0.0210448314755895,-0.671895682303137));
#86519=DIRECTION('',(-0.987191489212964,0.,-0.159539849647322));
#86520=DIRECTION('center_axis',(0.0840402580818046,-0.98736372204253,0.13435071795813));
#86521=DIRECTION('ref_axis',(0.902782938705594,0.0183712241368421,-0.429703925634623));
#86522=DIRECTION('',(0.368026888566917,0.,-0.929815147914764));
#86523=DIRECTION('center_axis',(0.,-1.,0.));
#86524=DIRECTION('ref_axis',(0.,0.,-1.));
#86525=DIRECTION('center_axis',(-0.103300989412016,0.987363722147504,-0.120173981266849));
#86526=DIRECTION('ref_axis',(0.827837155414535,0.0183708794019659,-0.560667597516718));
#86527=DIRECTION('center_axis',(0.0961354049611609,0.987363722122848,0.125979617989056));
#86528=DIRECTION('ref_axis',(0.867475562994424,-0.0210448304182839,-0.497034468342159));
#86529=DIRECTION('',(-0.929815148606724,0.,-0.368026886818689));
#86530=DIRECTION('center_axis',(0.053194013979902,-0.987363721990877,0.149275843233354));
#86531=DIRECTION('ref_axis',(0.974050017223779,0.0183712276662062,-0.225586041102707));
#86532=DIRECTION('',(0.559305393715518,0.,-0.828961685821926));
#86533=DIRECTION('center_axis',(-8.5092100362368E-14,-1.,2.63389760788361E-14));
#86534=DIRECTION('ref_axis',(1.,-8.5092100362368E-14,-6.58426787095862E-31));
#86535=DIRECTION('center_axis',(-0.0750520182169393,0.98736372208175,-0.139571038824097));
#86536=DIRECTION('ref_axis',(0.929009743068865,0.0183708817694427,-0.369598982663825));
#86537=DIRECTION('center_axis',(0.0668059196099684,0.987363722094998,0.143700554611937));
#86538=DIRECTION('ref_axis',(0.954042184755361,-0.0210448313464778,-0.298932475286338));
#86539=DIRECTION('',(-0.828961684948636,0.,-0.559305395009845));
#86540=DIRECTION('center_axis',(0.0198604736064091,-0.987363721987085,0.157220997617807));
#86541=DIRECTION('ref_axis',(0.99977159965937,0.0183712272039706,-0.0109200057492469));
#86542=DIRECTION('',(0.724431404105314,0.,-0.689346894347108));
#86543=DIRECTION('center_axis',(8.87647956210514E-14,-1.,-7.43089918185425E-15));
#86544=DIRECTION('ref_axis',(1.,8.87647956210513E-14,-3.94182071300882E-31));
#86545=DIRECTION('center_axis',(-0.0432936985365139,0.98736372200008,-0.152441910723981));
#86546=DIRECTION('ref_axis',(0.986742867208569,0.0183708839620664,-0.161248332194369));
#86547=DIRECTION('center_axis',(0.0343526625781289,0.987363722125914,0.154702213311425));
#86548=DIRECTION('ref_axis',(0.995998854493829,-0.0210448311515057,-0.0868527312684218));
#86549=DIRECTION('',(-0.689346896451424,0.,-0.724431402102911));
#86550=DIRECTION('center_axis',(-0.014401724422129,-0.987363722031899,0.157814672160051));
#86551=DIRECTION('ref_axis',(0.978744973309671,0.0183712233283643,0.204256640955612));
#86552=DIRECTION('',(0.855683805531922,0.,-0.517499009612973));
#86553=DIRECTION('center_axis',(2.94289825351575E-14,-1.,3.94154609637067E-15));
#86554=DIRECTION('ref_axis',(1.,2.94289825351575E-14,-2.14150802636011E-31));
#86555=DIRECTION('center_axis',(-0.00951100661057945,0.987363722136511,
-0.158184768426005));
#86556=DIRECTION('ref_axis',(0.998336992161528,0.0183708797645671,0.0546421161609756));
#86557=DIRECTION('center_axis',(0.000293112974508184,0.987363722118915,
0.158470168575244));
#86558=DIRECTION('ref_axis',(0.991383724636723,-0.0210448306235249,0.129288149609488));
#86559=DIRECTION('',(-0.517499010316405,0.,-0.855683805106501));
#86560=DIRECTION('center_axis',(-0.0479905100827411,-0.987363722040683,
0.151029107591772));
#86561=DIRECTION('ref_axis',(0.911953320089083,0.0183712227089235,0.409882471148349));
#86562=DIRECTION('',(0.946925383165727,0.,-0.321453447199499));
#86563=DIRECTION('center_axis',(2.78936333747509E-14,-1.,1.01757562670739E-14));
#86564=DIRECTION('ref_axis',(1.,2.78936333747509E-14,-2.28033888729291E-31));
#86565=DIRECTION('center_axis',(0.0247164011025826,0.987363722070318,-0.156531082715173));
#86566=DIRECTION('ref_axis',(0.963249988847597,0.0183708832253758,0.267977554348538));
#86567=DIRECTION('center_axis',(-0.0337801386902987,0.987363722008994,0.154828236089577));
#86568=DIRECTION('ref_axis',(0.940412594373351,-0.0210448336306716,0.339383658005864));
#86569=DIRECTION('',(-0.321453447977455,0.,-0.946925382901634));
#86570=DIRECTION('center_axis',(-0.0793353132184248,-0.987363722067417,
0.137181589222863));
#86571=DIRECTION('ref_axis',(0.802519742299411,0.018371221794083,0.596342654377062));
#86572=DIRECTION('',(0.993889783075419,0.,-0.110377076869685));
#86573=DIRECTION('center_axis',(-7.51620268031192E-14,-1.,-4.78024781847107E-14));
#86574=DIRECTION('ref_axis',(1.,-7.51620268031192E-14,4.45701823373997E-31));
#86575=DIRECTION('center_axis',(0.057788096969252,0.987363721938313,-0.147558179877612));
#86576=DIRECTION('ref_axis',(0.883122486736232,0.0183708880663981,0.468782661680726));
#86577=DIRECTION('center_axis',(-0.0662738728966525,0.987363722051591,0.143946705928643));
#86578=DIRECTION('ref_axis',(0.845468815551909,-0.0210448325433083,0.53360996706628));
#86579=DIRECTION('',(-0.110377077686295,0.,-0.99388978298473));
#86580=DIRECTION('center_axis',(-0.106970483905427,-0.987363722071512,0.116919613025908));
#86581=DIRECTION('ref_axis',(0.655561234390894,0.0183712221816143,0.754918516238303));
#86582=DIRECTION('',(0.994381001052632,0.,0.105860402160414));
#86583=DIRECTION('center_axis',(-4.20857737396286E-14,-1.,-4.18949978672253E-14));
#86584=DIRECTION('ref_axis',(1.,-4.20857737396286E-14,4.26600455538985E-31));
#86585=DIRECTION('center_axis',(0.0881576982960553,0.987363722200972,-0.131685611638414));
#86586=DIRECTION('ref_axis',(0.761701158200427,0.0183708771844214,0.647668014084069));
#86587=DIRECTION('center_axis',(-0.0956687127568795,0.987363722041466,0.126334388809476));
#86588=DIRECTION('ref_axis',(0.710991853905636,-0.0210448335406359,0.702885267067872));
#86589=DIRECTION('',(0.105860401342926,0.,-0.994381001139661));
#86590=DIRECTION('center_axis',(-0.129603830352234,-0.987363721976718,0.0911906118101647));
#86591=DIRECTION('ref_axis',(0.477949413275875,0.0183712293018593,0.878195226748122));
#86592=DIRECTION('',(0.948376068001928,0.,0.317147968054664));
#86593=DIRECTION('center_axis',(0.,-1.,0.));
#86594=DIRECTION('ref_axis',(0.,0.,-1.));
#86595=DIRECTION('center_axis',(0.114405130916887,0.987363722064272,-0.109655580666363));
#86596=DIRECTION('ref_axis',(0.60466353119606,0.0183708827655051,0.79626912831525));
#86597=DIRECTION('center_axis',(-0.120590190775855,0.987363722103883,0.102814814894587));
#86598=DIRECTION('ref_axis',(0.543269704745646,-0.0210448326431497,0.839294431605858));
#86599=DIRECTION('',(0.317147963824605,0.,-0.948376069416509));
#86600=DIRECTION('center_axis',(-0.14617705182175,-0.987363722017283,0.0611976303861404));
#86601=DIRECTION('ref_axis',(0.277989205306797,0.0183712262658596,0.960408506719086));
#86602=DIRECTION('',(0.85802612362603,0.,0.513606046669321));
#86603=DIRECTION('center_axis',(-4.12095214699751E-14,-1.,-1.11388455919924E-13));
#86604=DIRECTION('ref_axis',(7.91583898807535E-31,1.11388455919924E-13,
-1.));
#86605=DIRECTION('center_axis',(0.135303109888205,0.987363721994031,-0.0824981754020864));
#86606=DIRECTION('ref_axis',(0.419352507557114,0.0183708858640293,0.907637584588767));
#86607=DIRECTION('center_axis',(-0.139873004629083,0.987363722041037,0.0744877370666017));
#86608=DIRECTION('ref_axis',(0.35014486756981,-0.0210448345286272,0.936459121720848));
#86609=DIRECTION('',(0.513606044697418,0.,-0.858026124806392));
#86610=DIRECTION('center_axis',(-0.155915195768687,-0.987363722021331,0.028343114941639));
#86611=DIRECTION('ref_axis',(0.0650305337710549,0.0183712223399492,0.997714151381641));
#86612=DIRECTION('',(0.727555834386069,0.,0.686048473397318));
#86613=DIRECTION('center_axis',(0.,-1.,0.));
#86614=DIRECTION('ref_axis',(0.,0.,-1.));
#86615=DIRECTION('center_axis',(0.14987446749451,0.987363722004551,-0.0514832444835786));
#86616=DIRECTION('ref_axis',(0.214433030125156,0.0183708851604601,0.976565914912949));
#86617=DIRECTION('center_axis',(-0.152615514008743,0.987363722134678,0.0426776885058355));
#86618=DIRECTION('ref_axis',(0.140647645910758,-0.0210448290467592,0.989836024233385));
#86619=DIRECTION('center_axis',(-2.34251248529641E-15,-1.,2.95992134304517E-14));
#86620=DIRECTION('ref_axis',(1.57742281693884E-32,-2.95992134304517E-14,
-1.));
#86621=DIRECTION('center_axis',(0.157437861538929,0.987363721967134,-0.0180610159530712));
#86622=DIRECTION('ref_axis',(-0.000513102483762423,0.0183708870102229,0.999831109356125));
#86623=DIRECTION('center_axis',(-0.158221889080688,0.987363722241387,0.00887208078028815));
#86624=DIRECTION('ref_axis',(-0.0754261047720061,-0.0210448262853796,0.996929294386287));
#86625=DIRECTION('',(0.686048471277825,0.,-0.727555836384645));
#86626=DIRECTION('center_axis',(0.163393692715905,-0.986495109888097,0.0113973394935624));
#86627=DIRECTION('ref_axis',(0.0258341094970031,0.0158269796852664,0.999540947385618));
#86628=DIRECTION('center_axis',(-0.1596841371995,-0.986495109005799,0.0364468960885218));
#86629=DIRECTION('ref_axis',(0.139259431844732,0.0140402165467154,0.99015639318322));
#86630=DIRECTION('center_axis',(0.162023729773524,-0.986495109914706,-0.0239939389148123));
#86631=DIRECTION('ref_axis',(0.240101877481402,0.0158269783313953,0.970618666205634));
#86632=DIRECTION('center_axis',(-0.148115806239777,-0.986495109048686,0.0699221550366034));
#86633=DIRECTION('ref_axis',(0.348857978478882,0.0140402144241546,0.937070425971576));
#86634=DIRECTION('center_axis',(0.15307771473187,-0.986495110034312,-0.0582632914523267));
#86635=DIRECTION('ref_axis',(0.443142750284692,0.0158269724739011,0.896311335314035));
#86636=DIRECTION('center_axis',(-0.129621746388249,-0.986495109054191,0.100127931544702));
#86637=DIRECTION('ref_axis',(0.542144315518207,0.0140402112031747,0.840168086528324));
#86638=DIRECTION('center_axis',(0.136973958783133,-0.986495109992773,-0.0898083101701765));
#86639=DIRECTION('ref_axis',(0.625462761400192,0.0158269746406774,0.780093482202851));
#86640=DIRECTION('center_axis',(-0.105066715113658,-0.986495109010335,0.125651841506255));
#86641=DIRECTION('ref_axis',(0.710080586202779,0.0140402132056087,0.703980421255491));
#86642=DIRECTION('center_axis',(0.114465449777524,-0.986495110036968,-0.117153995580092));
#86643=DIRECTION('ref_axis',(0.778536828715126,0.0158269720084483,0.627399325223767));
#86644=DIRECTION('center_axis',(-0.0755988798103096,-0.986495109009909,
0.145300410429407));
#86645=DIRECTION('ref_axis',(0.844814278286775,0.014040215547775,0.534875413110537));
#86646=DIRECTION('center_axis',(0.0866046692179544,-0.986495109923494,-0.139021686677592));
#86647=DIRECTION('ref_axis',(0.89520737956913,0.0158269765333149,0.445368672426323));
#86648=DIRECTION('center_axis',(-0.0425961353136749,-0.986495109055382,
0.158154889479112));
#86649=DIRECTION('ref_axis',(0.940045392205716,0.0140402069799854,0.340760228284876));
#86650=DIRECTION('center_axis',(0.0546943469278652,-0.98649510991499,-0.154388880842975));
#86651=DIRECTION('ref_axis',(0.970019027659476,0.015826976159292,0.242513077594213));
#86652=DIRECTION('center_axis',(-0.00760162579462577,-0.986495109024877,
0.163614226628601));
#86653=DIRECTION('ref_axis',(0.991321029569393,0.0140402163257876,0.13071147103068));
#86654=DIRECTION('center_axis',(0.0202265769071983,-0.986495109950068,-0.162537022340207));
#86655=DIRECTION('ref_axis',(0.999473664960509,0.0158269756080494,0.0283178370203542));
#86656=DIRECTION('center_axis',(0.0277483150287501,-0.986495109025233,0.161423142338262));
#86657=DIRECTION('ref_axis',(0.996243597198247,0.0140402127555468,-0.0854492098692269));
#86658=DIRECTION('center_axis',(-0.015186968293509,-0.986495110040764,-0.163085112317813));
#86659=DIRECTION('ref_axis',(0.982194024074973,0.0158269715953397,-0.187201511856963));
#86660=DIRECTION('center_axis',(0.0618007766378345,-0.986495109035607,0.151684092296411));
#86661=DIRECTION('ref_axis',(0.954582921692536,0.0140402106311878,-0.297614378178163));
#86662=DIRECTION('center_axis',(-0.0498903763927462,-0.986495109833052,
-0.156007527442959));
#86663=DIRECTION('ref_axis',(0.918988082572133,0.0158269797608328,-0.393967525060181));
#86664=DIRECTION('center_axis',(0.0929635057152368,-0.986495109045637,0.134852461728253));
#86665=DIRECTION('ref_axis',(0.868287009737066,0.0140402117084069,-0.495863429965397));
#86666=DIRECTION('center_axis',(-0.0822609770536424,-0.986495109954466,
-0.141635199333024));
#86667=DIRECTION('ref_axis',(0.8128112796066,0.0158269756738695,-0.582312056019194));
#86668=DIRECTION('center_axis',(0.119779364423865,-0.986495109030295,0.11171527969585));
#86669=DIRECTION('ref_axis',(0.741390961601542,0.014040212596467,-0.670926459819395));
#86670=DIRECTION('center_axis',(-0.110785145530173,-0.986495110071091,-0.120640164686907));
#86671=DIRECTION('ref_axis',(0.668628322217801,0.0158269710235375,-0.743428324531981));
#86672=DIRECTION('center_axis',(0.140994470581036,-0.986495109053583,0.0833544184727661));
#86673=DIRECTION('ref_axis',(0.579828297438555,0.0140402095968446,-0.81461771279784));
#86674=DIRECTION('center_axis',(-0.134129119682768,-0.986495110072653,-0.0940041331850318));
#86675=DIRECTION('ref_axis',(0.493181049503002,0.0158269710266419,-0.869782708151432));
#86676=DIRECTION('center_axis',(0.155616836747567,-0.986495109020785,0.051095988088611));
#86677=DIRECTION('ref_axis',(0.391153502999558,0.0140402166268495,-0.920218348767425));
#86678=DIRECTION('center_axis',(-0.151201364507911,-0.986495110021318,-0.0629725755783759));
#86679=DIRECTION('ref_axis',(0.294673181296257,0.0158269734645186,-0.955467018340087));
#86680=DIRECTION('center_axis',(0.162962728442398,-0.986495108997506,0.0164483756829379));
#86681=DIRECTION('ref_axis',(0.184188810225888,0.0140402136861454,-0.982790595491847));
#86682=DIRECTION('center_axis',(-0.161203602974457,-0.986495109981873,-0.0289964889237524));
#86683=DIRECTION('ref_axis',(0.0823867191797638,0.0158269747516762,-0.996474754006846));
#86684=DIRECTION('center_axis',(0.16268866488224,-0.986495109019677,-0.0189683472946162));
#86685=DIRECTION('ref_axis',(-0.031388350063932,0.0140402130897802,-0.999408647099202));
#86686=DIRECTION('center_axis',(-0.163668140770209,-0.986495109923555,0.00633543950610209));
#86687=DIRECTION('ref_axis',(-0.133752052438717,0.0158269775873577,-0.990888437337362));
#86688=DIRECTION('center_axis',(0.154807460333412,-0.986495109016584,-0.05349813185034));
#86689=DIRECTION('ref_axis',(-0.245497824500102,0.0140402131910535,-0.969295460929879));
#86690=DIRECTION('center_axis',(-0.158479740056268,-0.986495109801126,0.0413711291864477));
#86691=DIRECTION('ref_axis',(-0.343636726738424,0.0158269814347735,-0.938969278887848));
#86692=DIRECTION('center_axis',(0.139687631289941,-0.986495109047706,-0.0855264022951965));
#86693=DIRECTION('ref_axis',(-0.448128094060664,0.0140402122128746,-0.893859096141318));
#86694=DIRECTION('center_axis',(-0.145880998923126,-0.986495109926484,0.0744723589281599));
#86695=DIRECTION('ref_axis',(-0.537453330319667,0.0158269761416644,-0.843144960581815));
#86696=DIRECTION('center_axis',(0.118036163879493,-0.986495109044257,-0.113555554018166));
#86697=DIRECTION('ref_axis',(-0.629804389132666,0.0140402125730394,-0.776626875571618));
#86698=DIRECTION('center_axis',(-0.126461025342854,-0.986495109956398,0.10409134018423));
#86699=DIRECTION('ref_axis',(-0.70613921349188,0.0158269745844066,-0.707896120941889));
#86700=DIRECTION('center_axis',(0.0908654531084785,-0.986495109005427,-0.136274976939132));
#86701=DIRECTION('ref_axis',(-0.782031736374587,0.0140402162115408,-0.623080440739141));
#86702=DIRECTION('center_axis',(-0.101127876712809,-0.986495109938006,0.128843124069392));
#86703=DIRECTION('ref_axis',(-0.841806811906979,0.0158269759318603,-0.539546845287655));
#86704=DIRECTION('center_axis',(0.0594459811192609,-0.986495109049417,-0.152622328478988));
#86705=DIRECTION('ref_axis',(-0.897692144812778,0.0140402125023846,-0.440399461369247));
#86706=DIRECTION('center_axis',(-0.0710661011877669,-0.986495109933049,
0.147570347089622));
#86707=DIRECTION('ref_axis',(-0.93811245894817,0.0158269770340597,-0.345968959827586));
#86708=DIRECTION('center_axis',(0.0252468774281873,-0.986495109027206,-0.161833232203796));
#86709=DIRECTION('ref_axis',(-0.971377467360531,0.0140402131190302,-0.237125891289441));
#86710=DIRECTION('center_axis',(-0.0376813519130728,-0.986495109949852,
0.159397345533208));
#86711=DIRECTION('ref_axis',(-0.990553010817809,0.0158269764618599,-0.13621394780216));
#86712=DIRECTION('center_axis',(-0.0101327460188599,-0.986495108992418,
-0.163476993464387));
#86713=DIRECTION('ref_axis',(-0.99964225913962,0.0140402175746079,-0.0227645784651067));
#86714=DIRECTION('center_axis',(-0.0025346599444412,-0.98649511006807,0.163771100352759));
#86715=DIRECTION('ref_axis',(-0.99667640424643,0.0158269710860104,0.0799102759640404));
#86716=DIRECTION('center_axis',(-0.0450385678145862,-0.986495108996407,
-0.157476751729825));
#86717=DIRECTION('ref_axis',(-0.981164889711611,0.0140402156784061,0.192661183274957));
#86718=DIRECTION('center_axis',(0.0327305405511363,-0.986495109972786,0.160487101397622));
#86719=DIRECTION('ref_axis',(-0.956196316558089,0.0158269753346832,0.292297983319246));
#86720=DIRECTION('center_axis',(-0.0778384347764789,-0.986495109011886,
-0.144113073547044));
#86721=DIRECTION('ref_axis',(-0.916809341545154,0.0140402127225352,0.399078317730051));
#86722=DIRECTION('center_axis',(0.0664652972180809,-0.986495109850739,0.149698906162638));
#86723=DIRECTION('ref_axis',(-0.871005552933621,0.0158269801331046,0.491018160009041));
#86724=DIRECTION('center_axis',(-0.106998668569342,-0.986495109004646,-0.124010825472212));
#86725=DIRECTION('ref_axis',(-0.809584805429825,0.0140402153031817,0.586834998250269));
#86726=DIRECTION('center_axis',(0.0970922175602582,-0.986495109914703,0.131910952553644));
#86727=DIRECTION('ref_axis',(-0.745087536041886,0.0158269772062907,0.66677887671067));
#86728=DIRECTION('center_axis',(-0.131155762220523,-0.98649510897064,-0.0981099689805202));
#86729=DIRECTION('ref_axis',(-0.664504985384022,0.0140402174317722,0.74715192343609));
#86730=DIRECTION('center_axis',(0.123179213512161,-0.986495110027753,0.107954987146756));
#86731=DIRECTION('ref_axis',(-0.584330053200728,0.0158269728669726,0.811361754001446));
#86732=DIRECTION('center_axis',(-0.149180154404103,-0.986495109054244,-0.0676216041219363));
#86733=DIRECTION('ref_axis',(-0.48835365175152,0.0140402134121568,0.872532855099621));
#86734=DIRECTION('center_axis',(0.143506481236003,-0.986495109925275,0.0789511743850581));
#86735=DIRECTION('ref_axis',(-0.396249950523607,0.0158269773943524,0.918006254606469));
#86736=DIRECTION('center_axis',(-0.160229052463089,-0.986495108976717,-0.0339713219023875));
#86737=DIRECTION('ref_axis',(-0.28936744084067,0.014040216551562,0.957115121863878));
#86738=DIRECTION('center_axis',(0.157123548865898,-0.986495109968347,0.0462556850595121));
#86739=DIRECTION('ref_axis',(-0.189641636534491,0.0158269742616208,0.981725805191165));
#86740=DIRECTION('center_axis',(-0.163785816046288,-0.986495109021849,0.0012674139114061));
#86741=DIRECTION('ref_axis',(-0.0768507322934788,0.0140402118077792,0.996943748362137));
#86742=DIRECTION('center_axis',(-0.163746589113265,0.986495109212932,0.00380184859464142));
#86743=DIRECTION('ref_axis',(-0.0762928037604484,-0.0165058445169965,0.996948827769585));
#86744=DIRECTION('center_axis',(0.163385855644741,0.986495983400253,0.0114340242435876));
#86745=DIRECTION('ref_axis',(-0.183100330941314,0.0189330377687653,0.982911902914004));
#86746=DIRECTION('center_axis',(-0.160735569747077,0.986495109243657,-0.031487712784955));
#86747=DIRECTION('ref_axis',(-0.288823649385265,-0.0165058446405764,0.957240020396389));
#86748=DIRECTION('center_axis',(0.157107995693868,0.98649598417733,0.0462898573237903));
#86749=DIRECTION('ref_axis',(-0.390116547996733,0.0189330090465228,0.920570812131015));
#86750=DIRECTION('center_axis',(-0.150208734751245,0.986495109188334,-0.0653049427832729));
#86751=DIRECTION('ref_axis',(-0.487849419977123,-0.0165058455838431,0.872771734469871));
#86752=DIRECTION('center_axis',(0.143483944818749,0.98649598426314,0.0789812041687666));
#86753=DIRECTION('ref_axis',(-0.57889135101082,0.0189330049272192,0.815184853299724));
#86754=DIRECTION('center_axis',(-0.132658304626714,0.986495109226924,-0.0960685884403693));
#86755=DIRECTION('ref_axis',(-0.664063896654305,-0.0165058442549272,0.747493610852783));
#86756=DIRECTION('center_axis',(0.123150816988761,0.986495981727044,0.107979416146764));
#86757=DIRECTION('ref_axis',(-0.740597844773079,0.0189330996251722,0.671681747597814));
#86758=DIRECTION('center_axis',(-0.108904925617282,0.986495109062018,-0.122340169090171));
#86759=DIRECTION('ref_axis',(-0.809227481863439,-0.0165058503434508,0.58726351793841));
#86760=DIRECTION('center_axis',(0.0970592346619194,0.986495982026364,0.131928702004838));
#86761=DIRECTION('ref_axis',(-0.867674800138622,0.0189330983424895,0.49677155614181));
#86762=DIRECTION('center_axis',(-0.0800592635376213,0.986495109206599,-0.142891265769723));
#86763=DIRECTION('ref_axis',(-0.916552489471739,-0.0165058442070702,0.399573636705639));
#86764=DIRECTION('center_axis',(0.0664292055707529,0.986495983699788,0.149709167359338));
#86765=DIRECTION('ref_axis',(-0.954180245093614,0.0189330269066743,0.298632885605793));
#86766=DIRECTION('center_axis',(-0.0474701296011309,0.98649510908173,-0.156760921640174));
#86767=DIRECTION('ref_axis',(-0.981020522367194,-0.0165058500441775,0.193200133562884));
#86768=DIRECTION('center_axis',(0.0326930102895807,0.986495985677644,0.160489368246307));
#86769=DIRECTION('ref_axis',(-0.996069284688432,0.018932952693861,0.0865304767267995));
#86770=DIRECTION('center_axis',(-0.0126613353093269,0.986495109225124,-0.163300612561913));
#86771=DIRECTION('ref_axis',(-0.999617125580531,-0.016505845105072,-0.0222071908057615));
#86772=DIRECTION('center_axis',(-0.00257165866145818,0.98649598158772,0.16376527373961));
#86773=DIRECTION('ref_axis',(-0.991383228009754,0.0189331052978054,-0.129618026310932));
#86774=DIRECTION('center_axis',(0.0227394843069944,0.986495109192044,-0.162204548005379));
#86775=DIRECTION('ref_axis',(-0.97147274280131,-0.0165058452943239,-0.236576133760823));
#86776=DIRECTION('center_axis',(-0.0377162304408249,0.986495981670314,0.159383700890832));
#86777=DIRECTION('ref_axis',(-0.940341195460543,0.0189331020324126,-0.339705716418294));
#86778=DIRECTION('center_axis',(0.0570770288022208,0.986495109144714,-0.153523979940172));
#86779=DIRECTION('ref_axis',(-0.897903374253699,-0.0165058476851046,-0.439883038427282));
#86780=DIRECTION('center_axis',(-0.0710972329446366,0.986495981748296,0.147549522066601));
#86781=DIRECTION('ref_axis',(-0.845329852427979,0.018933099101845,-0.53390914803222));
#86782=DIRECTION('center_axis',(0.088745716900431,0.986495109151901,-0.137664800697958));
#86783=DIRECTION('ref_axis',(-0.782349042285949,-0.0165058478410961,-0.622621500609563));
#86784=DIRECTION('center_axis',(-0.101153799510025,0.986495981517584,0.128816098739029));
#86785=DIRECTION('ref_axis',(-0.710791826200741,0.0189331070572685,-0.703147578580324));
#86786=DIRECTION('center_axis',(0.116264754633492,0.986495109150606,-0.115368567868151));
#86787=DIRECTION('ref_axis',(-0.63021293651818,-0.0165058475711234,-0.77624687544691));
#86788=DIRECTION('center_axis',(-0.126480538716153,0.986495981850945,0.104059363432665));
#86789=DIRECTION('ref_axis',(-0.543017961707908,0.0189330962803664,-0.839507612310828));
#86790=DIRECTION('center_axis',(0.138347381237138,0.986495109182418,-0.087677828805208));
#86791=DIRECTION('ref_axis',(-0.448608776393294,-0.0165058468718704,-0.893575806947544));
#86792=DIRECTION('center_axis',(-0.145893181782997,0.986495981861824,0.0744369349161404));
#86793=DIRECTION('ref_axis',(-0.349853182694279,0.0189330947671037,-0.936613201103435));
#86794=DIRECTION('center_axis',(0.153961037350114,0.986495109136802,-0.0558873744887531));
#86795=DIRECTION('ref_axis',(-0.246028168759599,-0.0165058488472811,-0.96912212704624));
#86796=DIRECTION('center_axis',(-0.158484017824289,0.986495981700585,0.0413339350034501));
#86797=DIRECTION('ref_axis',(-0.140329663760193,0.0189331099927658,-0.989923796468674));
#86798=DIRECTION('center_axis',(0.16237564746021,0.986495109135972,-0.0214836859659558));
#86799=DIRECTION('ref_axis',(-0.0319435566139225,-0.0165058480456351,-0.999353374022997));
#86800=DIRECTION('center_axis',(-0.163664315062582,0.986495983653055,0.00629811173985892));
#86801=DIRECTION('ref_axis',(0.0757555163317556,0.0189330280744371,-0.996946659652983));
#86802=DIRECTION('center_axis',(0.163197752493999,0.98649510914378,0.0139245544384616));
#86803=DIRECTION('ref_axis',(0.183634698391597,-0.0165058483007756,-0.982855968348618));
#86804=DIRECTION('center_axis',(-0.161191868054319,0.986495981535451,-0.0290320527618295));
#86805=DIRECTION('ref_axis',(0.288298462114998,0.0189331062348063,-0.957353400908164));
#86806=DIRECTION('center_axis',(0.156388911180579,0.986495109171284,0.048681701294124));
#86807=DIRECTION('ref_axis',(0.390626404147077,-0.0165058460816333,-0.920401308901858));
#86808=DIRECTION('center_axis',(-0.151182256635406,0.986495981655841,-0.0630047891473777));
#86809=DIRECTION('ref_axis',(0.487360887744349,0.0189331030435584,-0.872995362362357));
#86810=DIRECTION('center_axis',(0.142267496094813,0.986495109287409,0.0811625462078183));
#86811=DIRECTION('ref_axis',(0.579352849964745,-0.016505842071336,-0.814909708136579));
#86812=DIRECTION('center_axis',(-0.134103531952461,0.986495981849888,-0.0940314868110691));
#86813=DIRECTION('ref_axis',(0.663634858768959,0.0189331041865345,-0.747817030959155));
#86814=DIRECTION('center_axis',(0.121493814933404,0.98649510921518,0.109848315542195));
#86815=DIRECTION('ref_axis',(0.740989400275716,-0.016505844661274,-0.671313835527805));
#86816=DIRECTION('center_axis',(-0.110754275835824,0.98649598164166,-0.120661379856773));
#86817=DIRECTION('ref_axis',(0.808877999520859,0.0189331028534798,-0.587671608559979));
#86818=DIRECTION('center_axis',(0.0950392159143356,0.986495109219244,0.133397702097527));
#86819=DIRECTION('ref_axis',(0.867978110778369,-0.0165058442422676,-0.496328073269549));
#86820=DIRECTION('center_axis',(-0.0822261980276879,0.986495983852485,-0.141649307096185));
#86821=DIRECTION('ref_axis',(0.916298905042974,0.0189330215273502,-0.400047318842275));
#86822=DIRECTION('center_axis',(0.064140691289718,0.986495109175035,0.150709559400232));
#86823=DIRECTION('ref_axis',(0.954381129773572,-0.0165058468249323,-0.298134560480182));
#86824=DIRECTION('center_axis',(-0.0498534589114977,0.986495981677122,-0.156013815956958));
#86825=DIRECTION('ref_axis',(0.980874694402299,0.0189331024249501,-0.193717246299246));
#86826=DIRECTION('center_axis',(0.0302430200186192,0.986495109093,0.16097440627548));
#86827=DIRECTION('ref_axis',(0.996158346896073,-0.016505849461692,-0.0860006095491782));
#86828=DIRECTION('center_axis',(-0.0151495071665771,0.986495982983799,-0.163083316097745));
#86829=DIRECTION('ref_axis',(0.999585871964159,0.0189330533656895,0.0216708112424038));
#86830=DIRECTION('center_axis',(-0.00506879005589042,0.986495109267348,
0.163712268199342));
#86831=DIRECTION('ref_axis',(0.991356307130926,-0.0165058434051812,0.1301546366643));
#86832=DIRECTION('center_axis',(0.0202627268826977,0.986495981675467,-0.16252722860319));
#86833=DIRECTION('ref_axis',(0.971557523482164,0.0189331022783203,0.236045580774823));
#86834=DIRECTION('center_axis',(-0.0401435778617752,0.986495109147451,0.158795128340308));
#86835=DIRECTION('ref_axis',(0.940199548977773,-0.0165058484342841,0.340223992495321));
#86836=DIRECTION('center_axis',(0.054727547497996,0.986495981988391,-0.154371542279058));
#86837=DIRECTION('ref_axis',(0.898100225758627,0.0189330993522306,0.439383115562287));
#86838=DIRECTION('center_axis',(-0.0733413035779035,0.986495109199414,0.146452902720055));
#86839=DIRECTION('ref_axis',(0.845080103326574,-0.0165058468114072,0.534384857553605));
#86840=DIRECTION('center_axis',(0.0866333614647967,0.98649598183897,-0.138997620471991));
#86841=DIRECTION('ref_axis',(0.782648761242793,0.0189331052907383,0.622175581366845));
#86842=DIRECTION('center_axis',(-0.1031096704265,0.986495109194321,0.127262702313847));
#86843=DIRECTION('ref_axis',(0.710445651810553,-0.016505845860293,0.703558478646881));
#86844=DIRECTION('center_axis',(0.114488301191737,0.98649598151416,-0.117124324316706));
#86845=DIRECTION('ref_axis',(0.630601508918483,0.0189331076900093,0.775875811185612));
#86846=DIRECTION('center_axis',(-0.128056743368114,0.986495109232669,0.102121838692695));
#86847=DIRECTION('ref_axis',(0.542591550572572,-0.0165058447424131,0.839834487465591));
#86848=DIRECTION('center_axis',(0.136989899075835,0.986495981729044,-0.0897744149724316));
#86849=DIRECTION('ref_axis',(0.449068030412752,0.0189330998910831,0.893296950509586));
#86850=DIRECTION('center_axis',(-0.147016025755215,0.986495109314145,0.0722058686701834));
#86851=DIRECTION('ref_axis',(0.349366471721126,-0.0165058408723137,0.93684076856968));
#86852=DIRECTION('center_axis',(0.153085996471795,0.986495981709713,-0.0582267615004277));
#86853=DIRECTION('ref_axis',(0.246536630648454,0.0189331013475293,0.968948516393865));
#86854=DIRECTION('center_axis',(-0.159100999133471,0.986495109064463,0.0389136462776891));
#86855=DIRECTION('ref_axis',(0.139805408798706,-0.0165058509385653,0.990041415575844));
#86856=DIRECTION('center_axis',(0.162023961952645,0.986495981990121,-0.0239564870236498));
#86857=DIRECTION('ref_axis',(0.0324774513921005,0.0189331004002128,0.999293126595149));
#86858=DIRECTION('center_axis',(-0.15836291160918,0.987363722905755,-0.00583668710401735));
#86859=DIRECTION('ref_axis',(0.132413884601793,0.0270949580336305,0.990824114772051));
#86860=DIRECTION('',(-0.72694655115667,0.,-0.686694045235156));
#86861=DIRECTION('center_axis',(-2.0245503388309E-15,-1.,-1.47071881168559E-14));
#86862=DIRECTION('ref_axis',(-1.83209071492823E-32,1.47071881168559E-14,
-1.));
#86863=DIRECTION('center_axis',(-0.15834023719723,-0.987363722465014,0.00642252632184778));
#86864=DIRECTION('ref_axis',(0.0607081672435869,-0.00324287698160672,0.998150290376558));
#86865=DIRECTION('center_axis',(0.157437856145224,-0.987363722433383,-0.0180610374809706));
#86866=DIRECTION('ref_axis',(0.135803012302186,0.00353155705231592,0.990729564489946));
#86867=DIRECTION('center_axis',(0.155570627572672,0.987363722621189,-0.0301771285624221));
#86868=DIRECTION('ref_axis',(0.138060268971994,0.00851653687434142,0.990387212523995));
#86869=DIRECTION('',(-0.514367502868879,0.,0.857569864204913));
#86870=DIRECTION('center_axis',(-0.155915188834612,0.98736372298566,0.0283431194924692));
#86871=DIRECTION('ref_axis',(0.342316018190414,0.0270949546174172,0.939194126432092));
#86872=DIRECTION('',(-0.857569866383719,0.,-0.514367499236305));
#86873=DIRECTION('center_axis',(2.56941408722281E-15,-1.,6.96406186728433E-15));
#86874=DIRECTION('ref_axis',(-9.62012929511592E-33,-6.96406186728433E-15,
-1.));
#86875=DIRECTION('center_axis',(-0.153257677401923,-0.98736372244662,0.0403108411438247));
#86876=DIRECTION('ref_axis',(0.27386165228357,-0.00324287777277629,0.961763629564075));
#86877=DIRECTION('center_axis',(0.149874458590937,-0.987363722433169,-0.0514832621828552));
#86878=DIRECTION('ref_axis',(0.345605584671512,0.0035315609454342,0.938373224213666));
#86879=DIRECTION('center_axis',(0.145446283705042,0.987363722654481,-0.0629146862209245));
#86880=DIRECTION('ref_axis',(0.347736469892643,0.00851653269792382,0.937553633760442));
#86881=DIRECTION('',(-0.317989704666151,0.,0.948094166064919));
#86882=DIRECTION('center_axis',(-0.146177046567747,0.987363722929969,0.0611976282105879));
#86883=DIRECTION('ref_axis',(0.536211834736705,0.0270949566464369,0.843648464475948));
#86884=DIRECTION('',(-0.948094166918618,0.,-0.317989702120825));
#86885=DIRECTION('center_axis',(4.40705107135704E-14,-1.,6.87378769249437E-14));
#86886=DIRECTION('ref_axis',(6.13250777988043E-31,-6.87378769249437E-14,
-1.));
#86887=DIRECTION('center_axis',(-0.141008958275276,-0.987363722445226,0.0723142675080716));
#86888=DIRECTION('ref_axis',(0.474209669804676,-0.00324287656832448,0.880405970456416));
#86889=DIRECTION('center_axis',(0.13530309665382,-0.987363722448703,-0.0824981916658008));
#86890=DIRECTION('ref_axis',(0.539248023675166,0.00353155953696141,0.842139594752358));
#86891=DIRECTION('center_axis',(0.128521034514222,0.987363722653669,-0.0927104248446941));
#86892=DIRECTION('ref_axis',(0.541152901773958,0.00851652945533707,0.840881088875033));
#86893=DIRECTION('',(-0.106743061026616,0.,0.994286638209862));
#86894=DIRECTION('center_axis',(-0.129603832284082,0.9873637227692,0.0911906004839699));
#86895=DIRECTION('ref_axis',(0.705034980934041,0.02709496374429,0.708654738641485));
#86896=DIRECTION('',(-0.994286638431604,0.,-0.106743058961141));
#86897=DIRECTION('center_axis',(-6.30728491548966E-14,-1.,-6.28985089545158E-14));
#86898=DIRECTION('ref_axis',(1.,-6.30728491548966E-14,8.34113152972558E-31));
#86899=DIRECTION('center_axis',(-0.122166818764846,-0.98736372241398,0.100936356451412));
#86900=DIRECTION('ref_axis',(0.652384170649037,-0.00324287878729627,0.757881506321232));
#86901=DIRECTION('center_axis',(0.114405110202945,-0.987363722454584,-0.109655598763029));
#86902=DIRECTION('ref_axis',(0.707675823845859,0.00353155565455917,0.70652845410411));
#86903=DIRECTION('center_axis',(0.105586278763573,0.98736372261356,-0.11817113439226));
#86904=DIRECTION('ref_axis',(0.709265625848057,0.00851653576707507,0.70488987835611));
#86905=DIRECTION('',(0.109494768473299,0.,0.9939873719907));
#86906=DIRECTION('center_axis',(-0.106970480047799,0.987363722863142,0.116919609870118));
#86907=DIRECTION('ref_axis',(0.840891476130767,0.0270949599582825,0.540525104426685));
#86908=DIRECTION('',(-0.993987372109725,0.,0.109494767392795));
#86909=DIRECTION('center_axis',(6.88595975526522E-14,-1.,4.3880080293387E-14));
#86910=DIRECTION('ref_axis',(1.,6.88595975526522E-14,3.91605303123208E-31));
#86911=DIRECTION('center_axis',(-0.0976122921152477,-0.987363722456686,
0.124838776045279));
#86912=DIRECTION('ref_axis',(0.800053913492653,-0.0032428775879435,0.599919343953868));
#86913=DIRECTION('center_axis',(0.0881576724751072,-0.987363722452903,-0.131685627035442));
#86914=DIRECTION('ref_axis',(0.843013489298349,0.00353155875429685,0.537880827836229));
#86915=DIRECTION('center_axis',(0.07771443415297,0.987363722672603,-0.1381062847027));
#86916=DIRECTION('ref_axis',(0.844213877071177,0.00851653011734737,0.535938801054012));
#86917=DIRECTION('',(0.320612743670323,0.,0.947210361322229));
#86918=DIRECTION('center_axis',(-0.0793353088483608,0.987363722876107,0.137181585929636));
#86919=DIRECTION('ref_axis',(0.937428820871696,0.0270949592767233,0.347121115723165));
#86920=DIRECTION('',(-0.947210360754578,0.,0.320612745347376));
#86921=DIRECTION('center_axis',(0.,-1.,0.));
#86922=DIRECTION('ref_axis',(0.,0.,-1.));
#86923=DIRECTION('center_axis',(-0.0684935224953906,-0.987363722485225,
0.142903872922647));
#86924=DIRECTION('ref_axis',(0.910314022305051,-0.0032428753198789,0.413905622762555));
#86925=DIRECTION('center_axis',(0.0577880795527804,-0.987363722415584,-0.147558183504823));
#86926=DIRECTION('ref_axis',(0.938932780253383,0.00353156027763765,0.344082493375728));
#86927=DIRECTION('center_axis',(0.0462087395804152,0.987363722621269,-0.151583744635957));
#86928=DIRECTION('ref_axis',(0.939687625507126,0.00851653610917604,0.341927821449909));
#86929=DIRECTION('',(0.516739224239444,0.,0.856142846803276));
#86930=DIRECTION('center_axis',(-0.047990510290617,0.987363722793048,0.151029102607078));
#86931=DIRECTION('ref_axis',(0.990133034822597,0.0270949619669287,0.137486131624267));
#86932=DIRECTION('',(-0.856142845888396,0.,0.516739225755234));
#86933=DIRECTION('center_axis',(-7.35636780272307E-14,-1.,-9.91917069305592E-15));
#86934=DIRECTION('ref_axis',(1.,-7.35636780272307E-14,-1.13104790148456E-31));
#86935=DIRECTION('center_axis',(-0.0361720754548826,-0.987363722423393,
0.154286942414149));
#86936=DIRECTION('ref_axis',(0.978008860380544,-0.00324287732998205,0.208538132637109));
#86937=DIRECTION('center_axis',(0.02471637831391,-0.98736372243031,-0.156531084042774));
#86938=DIRECTION('ref_axis',(0.990948618920442,0.00353156016155522,0.134195241132066));
#86939=DIRECTION('center_axis',(0.0125423821788183,0.987363722633,-0.157973313814658));
#86940=DIRECTION('ref_axis',(0.991222625357522,0.00851653447638002,0.131928676260526));
#86941=DIRECTION('',(0.688703551631228,0.,0.725043045598351));
#86942=DIRECTION('center_axis',(-0.0144017228910838,0.987363722894221,0.15781466690467));
#86943=DIRECTION('ref_axis',(0.99653972906016,0.0270949585737063,-0.0785775516581714));
#86944=DIRECTION('',(-0.725043043015455,0.,0.688703554350411));
#86945=DIRECTION('center_axis',(-2.21928385368045E-14,-1.,1.83802507277912E-15));
#86946=DIRECTION('ref_axis',(1.,-2.21928385368045E-14,-2.13614459626393E-32));
#86947=DIRECTION('center_axis',(-0.00215926571236271,-0.987363722398442,
0.158455726507681));
#86948=DIRECTION('ref_axis',(0.999973090886145,-0.0032428822627582,-0.00658036611741906));
#86949=DIRECTION('center_axis',(-0.0095110328850321,-0.987363722430227,
-0.158184765012899));
#86950=DIRECTION('ref_axis',(0.996628801083753,0.00353155993727947,-0.0819668282585741));
#86951=DIRECTION('center_axis',(-0.0217104385133635,0.987363722671077,-0.156976227539939));
#86952=DIRECTION('ref_axis',(0.996409156842823,0.00851652826540035,-0.0842393073694228));
#86953=DIRECTION('',(0.828464869293673,1.87013121872489E-15,0.560041034519987));
#86954=DIRECTION('center_axis',(0.0198604695456076,0.987363722899584,0.157220992400195));
#86955=DIRECTION('ref_axis',(0.956349333116399,0.0270949588163081,-0.290967036371067));
#86956=DIRECTION('',(-0.560041033053189,0.,0.828464870285227));
#86957=DIRECTION('center_axis',(4.25577224838883E-14,-1.,-1.31317146727204E-14));
#86958=DIRECTION('ref_axis',(1.,4.25577224838883E-14,-1.08572151518037E-32));
#86959=DIRECTION('center_axis',(0.0319545165155947,-0.987363722426653,0.15521529728103));
#86960=DIRECTION('ref_axis',(0.975179691686365,-0.00324287950557378,-0.221391175648441));
#86961=DIRECTION('center_axis',(-0.0432937216746018,-0.987363722469846,
-0.152441901110066));
#86962=DIRECTION('ref_axis',(0.955707728024584,0.00353155703424488,-0.294296222705968));
#86963=DIRECTION('center_axis',(-0.0549481159469274,0.987363722638201,-0.148639105796278));
#86964=DIRECTION('ref_axis',(0.955004703283605,0.00851653533058213,-0.296468354689258));
#86965=DIRECTION('',(0.929488088790823,0.,0.368852128631492));
#86966=DIRECTION('center_axis',(0.0531940068768264,0.98736372282302,0.149275840260425));
#86967=DIRECTION('ref_axis',(0.871441105152733,0.0270949610725341,-0.489751225965449));
#86968=DIRECTION('',(-0.368852126985839,0.,0.929488089443874));
#86969=DIRECTION('center_axis',(-6.45663602884179E-14,-1.,3.66222581023245E-14));
#86970=DIRECTION('ref_axis',(1.,-6.45663602884179E-14,2.10025872039675E-31));
#86971=DIRECTION('center_axis',(0.0645741407431292,-0.987363722430153,0.144717172360982));
#86972=DIRECTION('ref_axis',(0.904787972919877,-0.00324287734543557,-0.425849982747519));
#86973=DIRECTION('center_axis',(-0.0750520377175071,-0.987363722424591,
-0.139571025912634));
#86974=DIRECTION('ref_axis',(0.870098824602278,0.00353156085805394,-0.492864650288129));
#86975=DIRECTION('center_axis',(-0.0856164675832888,0.987363722648476,-0.133351789175487));
#86976=DIRECTION('ref_axis',(0.868945292031076,0.00851652843073849,-0.494834869628764));
#86977=DIRECTION('',(0.987049478230213,-1.87013121704985E-15,0.160416107437701));
#86978=DIRECTION('center_axis',(0.0840402554793423,0.987363722896862,0.134350713307433));
#86979=DIRECTION('ref_axis',(0.745785259666093,0.0270949585837386,-0.66563519264243));
#86980=DIRECTION('',(-0.160416105690125,0.,0.987049478514231));
#86981=DIRECTION('center_axis',(4.96657185207468E-14,-1.,-4.46813180275799E-14));
#86982=DIRECTION('ref_axis',(1.,4.96657185207468E-14,-2.32209169568253E-31));
#86983=DIRECTION('center_axis',(0.0941743444094941,-0.987363722412064,0.127452236228457));
#86984=DIRECTION('ref_axis',(0.792089375903309,-0.00324288094989723,-0.610396514000736));
#86985=DIRECTION('center_axis',(-0.103301011994103,-0.987363722464081,-0.120173959254356));
#86986=DIRECTION('ref_axis',(0.743805065498613,0.00353155516523428,-0.668387277449773));
#86987=DIRECTION('center_axis',(-0.11228149913824,0.987363722622966,-0.111829084765048));
#86988=DIRECTION('ref_axis',(0.742254964002065,0.00851653420417142,-0.670063457487007));
#86989=DIRECTION('',(0.998457531228928,0.,-0.0555207918912755));
#86990=DIRECTION('center_axis',(0.110956872201526,0.987363722845984,0.113143498792342));
#86991=DIRECTION('ref_axis',(0.585257325062038,0.0270949599090236,-0.810394796755727));
#86992=DIRECTION('',(0.0555207965249884,0.,0.998457530971263));
#86993=DIRECTION('center_axis',(2.16107772093633E-14,-1.,-3.01740860957852E-14));
#86994=DIRECTION('ref_axis',(2.18320417523822E-31,3.01740860957852E-14,
-1.));
#86995=DIRECTION('center_axis',(0.119371065794289,-0.987363722406043,0.104227771383728));
#86996=DIRECTION('ref_axis',(0.642353557624346,-0.00324287839619577,-0.766401585819767));
#86997=DIRECTION('center_axis',(-0.126719736910895,-0.9873637224439,-0.0951577000508082));
#86998=DIRECTION('ref_axis',(0.582731810288293,0.00353156143387916,-0.812656855845054));
#86999=DIRECTION('center_axis',(-0.13369636490729,0.987363722672937,-0.0850773833637106));
#87000=DIRECTION('ref_axis',(0.580857619958026,0.00851652967266056,-0.813960621933907));
#87001=DIRECTION('',(0.9631788194689,0.,-0.268861603295255));
#87002=DIRECTION('center_axis',(0.132685271195736,0.987363722952293,0.0866458158568595));
#87003=DIRECTION('ref_axis',(0.397363406138617,0.0270949567738405,-0.917261242383728));
#87004=DIRECTION('',(0.26886160500055,0.,0.963178818992885));
#87005=DIRECTION('center_axis',(-1.46189926784329E-14,-1.,3.41143110164411E-14));
#87006=DIRECTION('ref_axis',(2.80296443029282E-32,-3.41143110164411E-14,
-1.));
#87007=DIRECTION('center_axis',(0.138986126964955,-0.987363722455319,0.0761297319741655));
#87008=DIRECTION('ref_axis',(0.462582001950055,-0.00324287689216964,-0.886570569792017));
#87009=DIRECTION('center_axis',(-0.144213194896543,-0.987363722466983,-0.0656919627798898));
#87010=DIRECTION('ref_axis',(0.394410661594976,0.00353155551480209,-0.918927504287394));
#87011=DIRECTION('center_axis',(-0.148859741286094,0.98736372264215,-0.0543475540799514));
#87012=DIRECTION('ref_axis',(0.392300018065111,0.00851653069053326,-0.919797893306519));
#87013=DIRECTION('',(0.882862937137387,1.87013121653348E-15,-0.469630742423393));
#87014=DIRECTION('center_axis',(0.148209452542795,0.987363722947302,0.0560966735609954));
#87015=DIRECTION('ref_axis',(0.19088921752838,0.0270949566362958,-0.981237570599638));
#87016=DIRECTION('',(0.469630743986495,0.,0.882862936305909));
#87017=DIRECTION('center_axis',(0.,-1.,0.));
#87018=DIRECTION('ref_axis',(0.,0.,-1.));
#87019=DIRECTION('center_axis',(0.152102349520003,-0.987363722407373,0.0444719568306875));
#87020=DIRECTION('ref_axis',(0.261180626874225,-0.00324288151993721,-0.965284498925076));
#87021=DIRECTION('center_axis',(-0.154963399384707,-0.987363722388471,-0.0331545556796895));
#87022=DIRECTION('ref_axis',(0.18764731161762,0.0035315638300726,-0.982230122985237));
#87023=DIRECTION('center_axis',(-0.15706260107623,0.987363722655006,-0.0210764923082087));
#87024=DIRECTION('ref_axis',(0.185398901952652,0.00851653249045242,-0.982626437578946));
#87025=DIRECTION('',(0.761265364441084,0.,-0.648440471363705));
#87026=DIRECTION('',(0.648440472711532,0.,0.761265363293015));
#87027=DIRECTION('',(0.604071869369054,0.,-0.796929844237858));
#87028=DIRECTION('center_axis',(0.158065638931242,0.987363722829192,-0.0113195684606789));
#87029=DIRECTION('ref_axis',(-0.238764600494895,0.0270949602251595,-0.970699401813409));
#87030=DIRECTION('',(0.796929845307366,0.,0.604071867958091));
#87031=DIRECTION('center_axis',(2.34182590397253E-14,-1.,9.36135301163808E-14));
#87032=DIRECTION('ref_axis',(-8.69630141945268E-32,-9.36135301163808E-14,
-1.));
#87033=DIRECTION('center_axis',(0.156717644371601,-0.987363722359724,-0.0235044615034313));
#87034=DIRECTION('ref_axis',(-0.168271322623861,-0.00324288391144424,-0.985735383196907));
#87035=DIRECTION('center_axis',(-0.154562207294442,-0.987363722441959,0.034977188020583));
#87036=DIRECTION('ref_axis',(-0.242123637853155,0.00353155854253617,-0.970238976792323));
#87037=DIRECTION('center_axis',(-0.151395946244086,0.987363722665093,0.0468203655024876));
#87038=DIRECTION('ref_axis',(-0.24433064533845,0.00851652983106372,-0.969654579975845));
#87039=DIRECTION('',(0.418632647009714,0.,-0.908155662239486));
#87040=DIRECTION('center_axis',(0.151936777370572,0.987363722957365,-0.0450343676542403));
#87041=DIRECTION('ref_axis',(-0.44185409481804,0.0270949552799474,-0.8966776579635));
#87042=DIRECTION('',(0.908155662980674,0.,0.418632645401827));
#87043=DIRECTION('center_axis',(9.92189883306421E-15,-1.,1.99363071636205E-14));
#87044=DIRECTION('ref_axis',(-1.29111785430247E-31,-1.99363071636205E-14,
-1.));
#87045=DIRECTION('center_axis',(0.148000906784593,-0.987363722409755,-0.0566446048630474));
#87046=DIRECTION('ref_axis',(-0.376241204684736,-0.00324288035874891,-0.926516076290292));
#87047=DIRECTION('center_axis',(-0.143429566060712,-0.987363722443142,0.0673857491080862));
#87048=DIRECTION('ref_axis',(-0.44503562198399,0.00353155572008162,-0.895505903542528));
#87049=DIRECTION('center_axis',(-0.137791397644641,0.987363722642848,0.0782713864959209));
#87050=DIRECTION('ref_axis',(-0.447065403159386,0.00851653186774189,-0.894460728027162));
#87051=DIRECTION('',(0.213618626551052,1.87013121746126E-15,-0.976917131792888));
#87052=DIRECTION('center_axis',(0.138703522518533,0.987363722956564,-0.0766434043496538));
#87053=DIRECTION('ref_axis',(-0.624282981195083,0.0270949558569211,-0.780728264351491));
#87054=DIRECTION('',(0.97691713277104,0.,0.213618622077782));
#87055=DIRECTION('center_axis',(-5.12440392804277E-14,-1.,-6.35700721972811E-14));
#87056=DIRECTION('ref_axis',(-3.8654389694051E-31,6.35700721972811E-14,
-1.));
#87057=DIRECTION('center_axis',(0.132363811790207,-0.987363722409503,-0.0871361061674017));
#87058=DIRECTION('ref_axis',(-0.56661846094771,-0.00324287919072601,-0.823973909446047));
#87059=DIRECTION('center_axis',(-0.125590320889639,-0.987363722425399,0.0966434215924563));
#87060=DIRECTION('ref_axis',(-0.627138234454523,0.00353155971536402,-0.778899969810784));
#87061=DIRECTION('center_axis',(-0.117743875713536,0.987363722627784,0.106062523874179));
#87062=DIRECTION('ref_axis',(-0.628895878264022,0.00851653394903831,-0.777442887260549));
#87063=DIRECTION('',(-0.00138396519504165,0.,-0.999999042319711));
#87064=DIRECTION('center_axis',(0.118984646214767,0.987363722909371,-0.104668680357086));
#87065=DIRECTION('ref_axis',(-0.777521090773876,0.0270949576384109,-0.628272883922563));
#87066=DIRECTION('',(0.999999042317255,0.,-0.00138396696952341));
#87067=DIRECTION('center_axis',(-2.31678794545486E-14,-1.,-1.85701401946468E-14));
#87068=DIRECTION('ref_axis',(1.,-2.31678794545486E-14,-1.73093210128079E-31));
#87069=DIRECTION('center_axis',(0.110537527352398,-0.987363722487205,-0.113553223481447));
#87070=DIRECTION('ref_axis',(-0.730501271666092,-0.00324287296146556,-0.682903635858807));
#87071=DIRECTION('center_axis',(-0.101878611119281,-0.987363722418207,0.121382157868727));
#87072=DIRECTION('ref_axis',(-0.779916560199733,0.00353156097293767,-0.625873539305913));
#87073=DIRECTION('center_axis',(-0.0921907795654185,0.987363722627442,0.128894295461047));
#87074=DIRECTION('ref_axis',(-0.781319882146542,0.00851653674625868,-0.624072680354111));
#87075=DIRECTION('',(-0.216321844433724,0.,-0.976322108538361));
#87076=DIRECTION('center_axis',(0.0937021776712861,0.987363722933383,-0.127799767350289));
#87077=DIRECTION('ref_axis',(-0.894403178552326,0.0270949561808685,-0.446440161214304));
#87078=DIRECTION('',(0.97632210815536,0.,-0.216321846162316));
#87079=DIRECTION('center_axis',(-0.0623268466247098,0.987363722160776,0.145699157000437));
#87080=DIRECTION('ref_axis',(-0.897210243280335,0.00851664566298019,-0.441521512612345));
#87081=DIRECTION('',(-0.421144752952744,0.,-0.906993438267539));
#87082=DIRECTION('center_axis',(1.996369424311E-14,-1.,9.86667873383296E-15));
#87083=DIRECTION('ref_axis',(1.,1.996369424311E-14,-1.41826297981486E-31));
#87084=DIRECTION('center_axis',(0.0835426374854572,-0.987363722437547,-0.134660711925359));
#87085=DIRECTION('ref_axis',(-0.860226652654134,-0.0032428756551188,-0.50990154914547));
#87086=DIRECTION('center_axis',(-0.0734031620397199,-0.987363722481538,
0.140445204011996));
#87087=DIRECTION('ref_axis',(-0.896226855125206,0.00353155234490209,-0.443581956678153));
#87088=DIRECTION('',(0.90699343803103,0.,-0.421144753462099));
#87089=DIRECTION('center_axis',(0.0640383013215094,0.987363722930161,-0.144955077887422));
#87090=DIRECTION('ref_axis',(-0.969463967507944,0.027094957164752,-0.243732392184538));
#87091=DIRECTION('center_axis',(-7.92659929065579E-14,-1.,-1.95961224160717E-14));
#87092=DIRECTION('ref_axis',(1.,-7.92659929065579E-14,2.13008784219506E-31));
#87093=DIRECTION('center_axis',(-0.0295487779255952,0.987363722618801,0.155691197501488));
#87094=DIRECTION('ref_axis',(-0.971148037060758,0.00851653427239421,-0.238325321267012));
#87095=DIRECTION('center_axis',(0.05264138558487,-0.987363722444023,-0.149471616453384));
#87096=DIRECTION('ref_axis',(-0.949728792505462,-0.00324287704961478,-0.313057030642274));
#87097=DIRECTION('center_axis',(-0.0414954754768436,-0.987363722444349,
0.152941181883068));
#87098=DIRECTION('ref_axis',(-0.970630577874648,0.00353155855321122,-0.240548975031929));
#87099=DIRECTION('',(-0.606275400562902,0.,-0.795254763376047));
#87100=DIRECTION('center_axis',(0.0313800671770485,0.987363722868791,-0.155332450397991));
#87101=DIRECTION('ref_axis',(-0.999193698214912,0.0270949595955448,-0.0296279700979335));
#87102=DIRECTION('',(0.795254762302624,0.,-0.606275401970917));
#87103=DIRECTION('center_axis',(-8.16253850365633E-14,-1.,-2.09813056959433E-15));
#87104=DIRECTION('ref_axis',(-0.999669805779023,8.16523461650324E-14,-0.0256959026642592));
#87105=DIRECTION('center_axis',(0.0192786812535226,-0.987363722432654,-0.157293394880581));
#87106=DIRECTION('ref_axis',(-0.994822668868896,-0.00324287838217591,-0.101574313900534));
#87107=DIRECTION('center_axis',(-0.00764750029647438,-0.987363722476038,
0.158285802513925));
#87108=DIRECTION('ref_axis',(-0.999648693396266,0.00353155762759509,-0.0262681916366585));
#87109=DIRECTION('center_axis',(0.00461105941972974,0.98736372264553,0.158403337510889));
#87110=DIRECTION('ref_axis',(-0.999676034875211,0.00851653231120432,-0.0239852866059154));
#87111=DIRECTION('',(-0.763057286545784,0.,-0.646330857571712));
#87112=DIRECTION('center_axis',(-0.00274546700816765,0.987363722872233,
-0.158446650853819));
#87113=DIRECTION('ref_axis',(-0.982202242647199,0.0270949591400856,0.185861824288935));
#87114=DIRECTION('',(0.646330857894588,0.,-0.763057286272299));
#87115=DIRECTION('center_axis',(2.91520236126574E-14,-1.,-5.63562454897997E-15));
#87116=DIRECTION('ref_axis',(1.,2.91520236126574E-14,4.88564478945882E-32));
#87117=DIRECTION('center_axis',(-0.0149854773444683,-0.987363722451026,
-0.157760308875241));
#87118=DIRECTION('ref_axis',(-0.993399742862264,-0.00324287466414407,0.114657902671822));
#87119=DIRECTION('center_axis',(0.0265580647803664,-0.987363722491441,0.156229154458978));
#87120=DIRECTION('ref_axis',(-0.981924347057675,0.00353155553646724,0.189240864431687));
#87121=DIRECTION('center_axis',(0.0385552928309168,0.98736372264335,0.15370871348947));
#87122=DIRECTION('ref_axis',(-0.981460292520777,0.00851653480253085,0.191476272263664));
#87123=DIRECTION('',(-0.88415945988124,0.,-0.467185241100908));
#87124=DIRECTION('center_axis',(-0.0367426288065956,0.987363722975676,-0.15415206057654));
#87125=DIRECTION('ref_axis',(-0.91928410143936,0.0270949559871885,0.39266092777469));
#87126=DIRECTION('',(0.467185239535493,0.,-0.884159460708398));
#87127=DIRECTION('center_axis',(-1.36294864018309E-14,-1.,5.88534506176603E-15));
#87128=DIRECTION('ref_axis',(1.,-1.36294864018309E-14,7.0077482906534E-32));
#87129=DIRECTION('center_axis',(-0.0485489273147898,-0.98736372247699,-0.150850525994987));
#87130=DIRECTION('ref_axis',(-0.945526549719031,-0.00324287530838049,0.32552884286367));
#87131=DIRECTION('center_axis',(0.0595218018727172,-0.987363722479134,0.146867404940558));
#87132=DIRECTION('ref_axis',(-0.918286310020471,0.00353155562112468,0.395901226247004));
#87133=DIRECTION('center_axis',(0.0706967180234564,0.987363722640494,0.141826842572968));
#87134=DIRECTION('ref_axis',(-0.917352557164235,0.00851653082876537,0.397984615992731));
#87135=DIRECTION('',(-0.963919320010511,0.,-0.2661945613841));
#87136=DIRECTION('center_axis',(-0.0690217369231991,0.987363722785221,-0.142649496177916));
#87137=DIRECTION('ref_axis',(-0.813381258259928,0.0270949631238604,0.581099640065981));
#87138=DIRECTION('',(0.266194559677452,0.,-0.963919320481817));
#87139=DIRECTION('center_axis',(-4.21598147701531E-14,-1.,3.03718997949049E-14));
#87140=DIRECTION('ref_axis',(1.,-4.21598147701531E-14,1.83273274081679E-31));
#87141=DIRECTION('center_axis',(-0.0798422822123721,-0.987363722443673,
-0.136887141738341));
#87142=DIRECTION('ref_axis',(-0.853441585256062,-0.00324287810098406,0.521178418871352));
#87143=DIRECTION('center_axis',(0.0897023623928398,-0.98736372243683,0.130638301415894));
#87144=DIRECTION('ref_axis',(-0.811710225602143,0.00353156010617074,0.584049687728822));
#87145=DIRECTION('center_axis',(0.0995324486587646,0.987363722660884,0.123313303569528));
#87146=DIRECTION('ref_axis',(-0.810350436308831,0.00851653338126038,0.585883639499562));
#87147=DIRECTION('',(-0.998607383967675,0.,-0.052756920733087));
#87148=DIRECTION('center_axis',(-0.0980734771944362,0.987363722940225,-0.124476791783094));
#87149=DIRECTION('ref_axis',(-0.669445610333536,0.02709495584999,0.742366781431286));
#87150=DIRECTION('',(0.0527569189650408,0.,-0.998607384061081));
#87151=DIRECTION('center_axis',(4.45436757048174E-14,-1.,-4.97892029732121E-14));
#87152=DIRECTION('ref_axis',(-1.17560233778818E-31,4.97892029732121E-14,
-1.));
#87153=DIRECTION('center_axis',(-0.107402302702658,-0.987363722394039,-0.116523066705065));
#87154=DIRECTION('ref_axis',(-0.721450640681184,-0.00324287910373861,0.692458270797474));
#87155=DIRECTION('center_axis',(0.115688545148596,-0.987363722462385,0.108300692918484));
#87156=DIRECTION('ref_axis',(-0.667179472758881,0.0035315585640653,0.744888635450488));
#87157=DIRECTION('center_axis',(0.123714148172352,0.987363722648617,0.0990337757507747));
#87158=DIRECTION('ref_axis',(-0.665457230495865,0.00851652976932358,0.746387394790039));
#87159=DIRECTION('',(-0.986601676591079,0.,0.163147576591479));
#87160=DIRECTION('center_axis',(-0.122539405670769,0.98736372302042,-0.100483692811866));
#87161=DIRECTION('ref_axis',(-0.494207430073928,0.0270949533761717,0.868921676309935));
#87162=DIRECTION('',(-0.163147578338245,0.,-0.986601676302228));
#87163=DIRECTION('center_axis',(-2.55103818864632E-14,-1.,4.52672364773351E-14));
#87164=DIRECTION('ref_axis',(2.30773181488144E-31,-4.52672364773351E-14,
-1.));
#87165=DIRECTION('center_axis',(-0.12994031340418,-0.987363722485979,-0.0907104981303418));
#87166=DIRECTION('ref_axis',(-0.555725466069267,-0.00324287493191982,0.831359543232814));
#87167=DIRECTION('center_axis',(0.136265258713363,-0.987363722442251,0.0808990659572843));
#87168=DIRECTION('ref_axis',(-0.491452149815892,0.00353155907475124,0.870897417915474));
#87169=DIRECTION('center_axis',(0.142111116604461,0.987363722627063,0.0701235322660115));
#87170=DIRECTION('ref_axis',(-0.489447982345426,0.00851653410216828,0.871990906618227));
#87171=DIRECTION('',(-0.928463571527175,0.,0.37142347306949));
#87172=DIRECTION('center_axis',(-0.141275525387784,0.987363722972098,-0.0717920920790242));
#87173=DIRECTION('ref_axis',(-0.295860660461752,0.0270949555521446,0.954846758896297));
#87174=DIRECTION('',(-0.371423474713337,0.,-0.928463570869569));
#87175=DIRECTION('center_axis',(4.33795587267854E-15,-1.,-1.41979690255456E-14));
#87176=DIRECTION('ref_axis',(-9.32044726918642E-33,1.41979690255456E-14,
-1.));
#87177=DIRECTION('center_axis',(-0.146402455491522,-0.987363722435009,-0.0606564147088839));
#87178=DIRECTION('ref_axis',(-0.364015186036907,-0.0032428792593312,0.931387367355079));
#87179=DIRECTION('center_axis',(0.150470359978484,-0.987363722444644,0.0497146896621282));
#87180=DIRECTION('ref_axis',(-0.292745071069821,0.00353156062358516,0.956184005013621));
#87181=DIRECTION('center_axis',(0.153863123526249,0.987363722660625,0.0379343959026435));
#87182=DIRECTION('ref_axis',(-0.290552692081676,0.00851653190555025,0.956821091849669));
#87183=DIRECTION('',(-0.826911541049425,0.,0.562332022278));
#87184=DIRECTION('center_axis',(-0.153405760191542,0.987363723027589,-0.0397435678966314));
#87185=DIRECTION('ref_axis',(-0.0836797723377556,0.0270949527568631,0.996124268972805));
#87186=DIRECTION('',(-0.562332021776287,0.,-0.82691154139061));
#87187=DIRECTION('center_axis',(6.51416273654917E-15,-1.,-8.13920838429517E-14));
#87188=DIRECTION('ref_axis',(-3.02306769725167E-32,8.13920838429517E-14,
-1.));
#87189=DIRECTION('center_axis',(-0.156018984352937,-0.987363722479574,-0.0277660953819161));
#87190=DIRECTION('ref_axis',(-0.155283961225101,-0.00324287333498782,0.987864553042964));
#87191=DIRECTION('center_axis',(0.157639635277682,-0.987363722413661,0.016205710442862));
#87192=DIRECTION('ref_axis',(-0.0803495567989669,0.00353156288138682,0.996760491184228));
#87193=DIRECTION('center_axis',(0.158420663065514,0.987363722652751,0.00397148626885451));
#87194=DIRECTION('ref_axis',(-0.0780714789323286,0.00851653284668103,0.996911386656603));
#87195=DIRECTION('',(-0.686694046522226,0.,0.726946549940868));
#87196=DIRECTION('',(0.760779449282709,0.,-0.64901050033809));
#87197=DIRECTION('center_axis',(0.158463151347264,-0.987363722875478,0.00151934675762116));
#87198=DIRECTION('ref_axis',(-0.181684484803401,-0.0276461711805923,0.982968177104822));
#87199=DIRECTION('center_axis',(-0.1583438731014,-0.987366232511757,-0.00592796312298457));
#87200=DIRECTION('ref_axis',(-0.254496684801816,0.0350112965860882,0.966439675580554));
#87201=DIRECTION('',(0.470291906521109,0.,0.882510919286974));
#87202=DIRECTION('center_axis',(-2.76653169601616E-14,-1.,1.45858321561486E-13));
#87203=DIRECTION('ref_axis',(-7.16568994862189E-31,-1.45858321561486E-13,
-1.));
#87204=DIRECTION('center_axis',(0.149682993082549,0.987363722771234,0.0520372994800879));
#87205=DIRECTION('ref_axis',(-0.116999345722024,-0.0345726402853016,0.992530042691062));
#87206=DIRECTION('center_axis',(-0.156429978772876,0.98736372254834,-0.0253483951484592));
#87207=DIRECTION('ref_axis',(-0.186229725703106,-0.00428129196166639,0.982496900658564));
#87208=DIRECTION('',(0.882510921618164,0.,-0.470291902146591));
#87209=DIRECTION('center_axis',(0.154431756916398,-0.987363722835662,0.0355487170488168));
#87210=DIRECTION('ref_axis',(-0.388745904643052,-0.0276461730162438,0.920930133474202));
#87211=DIRECTION('center_axis',(-0.153367540844493,-0.987366232745327,-0.0398286310286096));
#87212=DIRECTION('ref_axis',(-0.456302657595336,0.0350112876543126,0.889135588314977));
#87213=DIRECTION('',(0.269582982049911,0.,0.962977162651886));
#87214=DIRECTION('center_axis',(4.66989958556477E-14,-1.,-1.09200807760306E-13));
#87215=DIRECTION('ref_axis',(-1.34852716042978E-30,1.09200807760306E-13,
-1.));
#87216=DIRECTION('center_axis',(0.1349970075158,0.987363722840858,0.0829981131087992));
#87217=DIRECTION('ref_axis',(-0.32762858532778,-0.0345726381238089,0.944173841392187));
#87218=DIRECTION('center_axis',(-0.147323577184204,0.98736372254447,-0.0583835850969862));
#87219=DIRECTION('ref_axis',(-0.393083569634015,-0.00428129206822049,0.919492782909146));
#87220=DIRECTION('',(0.962977163988183,0.,-0.269582977276527));
#87221=DIRECTION('center_axis',(0.143179307552801,-0.987363722692721,0.0679158670641323));
#87222=DIRECTION('ref_axis',(-0.577629997206268,-0.0276461773922787,0.815830420616369));
#87223=DIRECTION('center_axis',(-0.141219909593753,-0.987366232973952,-0.0718669542777509));
#87224=DIRECTION('ref_axis',(-0.636772424978514,0.0350112793450637,0.770256508642156));
#87225=DIRECTION('',(0.0562686569827914,0.,0.998415664060492));
#87226=DIRECTION('center_axis',(0.,-1.,0.));
#87227=DIRECTION('ref_axis',(0.,0.,-1.));
#87228=DIRECTION('center_axis',(0.113998714502817,0.987363722957846,0.110078025411647));
#87229=DIRECTION('ref_axis',(-0.522938275540814,-0.0345726334276287,0.851669121779273));
#87230=DIRECTION('center_axis',(-0.131328487686392,0.987363722542039,-0.0886888252821752));
#87231=DIRECTION('ref_axis',(-0.581557263221753,-0.00428129011378238,0.81349420412747));
#87232=DIRECTION('',(0.998415664339409,0.,-0.056268652033758));
#87233=DIRECTION('center_axis',(0.125231945585741,-0.98736372287055,0.097107355869765));
#87234=DIRECTION('ref_axis',(-0.739504754353445,-0.0276461698608584,0.672583383366461));
#87235=DIRECTION('center_axis',(-0.122469001945228,-0.987366232743165,-0.100544845721249));
#87236=DIRECTION('ref_axis',(-0.787467419312884,0.0350112873268973,0.615361091783044));
#87237=DIRECTION('',(-0.159676728324535,0.,0.987169358535592));
#87238=DIRECTION('center_axis',(-6.6176317490642E-14,-1.,5.9624677248181E-14));
#87239=DIRECTION('ref_axis',(1.,-6.6176317490642E-14,1.52215481233823E-30));
#87240=DIRECTION('center_axis',(0.0876699622063549,0.987363722805222,0.132010820067707));
#87241=DIRECTION('ref_axis',(-0.693795956342581,-0.034572638888989,0.719341298413302));
#87242=DIRECTION('center_axis',(-0.109192625788737,0.987363722537062,-0.114847071756822));
#87243=DIRECTION('ref_axis',(-0.742837983763109,-0.00428129121212216,0.66945754191309));
#87244=DIRECTION('',(0.987169358123943,0.,0.159676730869475));
#87245=DIRECTION('center_axis',(0.101428888160009,-0.987363722703554,0.121758201923339));
#87246=DIRECTION('ref_axis',(-0.866801089322196,-0.0276461779428406,0.497887096031828));
#87247=DIRECTION('center_axis',(-0.097991569270547,-0.987366232948689,-0.124521381234754));
#87248=DIRECTION('ref_axis',(-0.901341314070176,0.0350112810043919,0.431692072839751));
#87249=DIRECTION('',(-0.368155805865995,0.,0.929764111270789));
#87250=DIRECTION('center_axis',(-2.58155649983822E-14,-1.,1.46682444274038E-14));
#87251=DIRECTION('ref_axis',(1.,-2.58155649983822E-14,3.81511095375126E-31));
#87252=DIRECTION('center_axis',(0.0572418606348332,0.987363722728194,0.147770932295171));
#87253=DIRECTION('ref_axis',(-0.832212508054769,-0.0345726417617727,0.553377876210102));
#87254=DIRECTION('center_axis',(-0.0819510393314511,0.987363722535972,-0.135635196657812));
#87255=DIRECTION('ref_axis',(-0.869384427205194,-0.00428129367737856,0.494117787837622));
#87256=DIRECTION('',(0.929764109056227,0.,0.368155811458791));
#87257=DIRECTION('center_axis',(0.0728831202913177,-0.987363722758493,0.140715776503882));
#87258=DIRECTION('ref_axis',(-0.953566769668903,-0.0276461750994164,0.299910161190959));
#87259=DIRECTION('center_axis',(-0.0689321668874775,-0.987366232873716,
-0.142675430782474));
#87260=DIRECTION('ref_axis',(-0.973069489809453,0.0350112832333832,0.227837613330903));
#87261=DIRECTION('',(-0.559420330169213,0.,0.828884125914696));
#87262=DIRECTION('center_axis',(8.50957512599141E-14,-1.,-2.63271769752319E-14));
#87263=DIRECTION('ref_axis',(1.,8.50957512599141E-14,-5.62014004724192E-31));
#87264=DIRECTION('center_axis',(0.0241371969399978,0.987363722764857,0.156621437523103));
#87265=DIRECTION('ref_axis',(-0.93171572713276,-0.0345726403955516,0.361539121464817));
#87266=DIRECTION('center_axis',(-0.0508775060530495,0.987363722578641,-0.150081173747645));
#87267=DIRECTION('ref_axis',(-0.955279421173268,-0.00428128798470859,0.295673634360688));
#87268=DIRECTION('',(0.828884125374412,0.,0.559420330969743));
#87269=DIRECTION('center_axis',(0.0409294185900453,-0.987363722835548,0.153093636452364));
#87270=DIRECTION('ref_axis',(-0.995744728148929,-0.0276461730218223,0.0879097575975621));
#87271=DIRECTION('center_axis',(-0.036649578451434,-0.987366232673174,-0.15415813626311));
#87272=DIRECTION('ref_axis',(-0.999298017642841,0.035011290644136,0.0133297210218571));
#87273=DIRECTION('',(-0.724526977917467,0.,0.689246442333787));
#87274=DIRECTION('center_axis',(-1.77531649047457E-13,-1.,1.48371821668093E-14));
#87275=DIRECTION('ref_axis',(1.,-1.77531649047457E-13,1.72309228978644E-31));
#87276=DIRECTION('center_axis',(-0.0100960932869904,0.98736372289332,0.158148498616284));
#87277=DIRECTION('ref_axis',(-0.987652955733019,-0.0345726365893217,0.152795195706845));
#87278=DIRECTION('center_axis',(-0.0174250066752681,0.987363722557612,-0.157509518822014));
#87279=DIRECTION('ref_axis',(-0.996506610362838,-0.00428129225189455,0.0834041128471496));
#87280=DIRECTION('',(0.689246440251503,0.,0.724526979898355));
#87281=DIRECTION('center_axis',(0.0070619071952816,-0.987363722761738,0.158313007806833));
#87282=DIRECTION('ref_axis',(-0.991362769072797,-0.0276461750575922,-0.128201205536457));
#87283=DIRECTION('center_axis',(-0.0026532898277805,-0.987366232668752,
-0.158432580735802));
#87284=DIRECTION('ref_axis',(-0.97880048130708,0.0350112911956791,-0.201801455103376));
#87285=DIRECTION('',(-0.855755550708435,0.,0.517380360500573));
#87286=DIRECTION('center_axis',(2.94284356015184E-14,-1.,3.94562661660699E-15));
#87287=DIRECTION('ref_axis',(1.,2.94284356015184E-14,-2.12214508197234E-31));
#87288=DIRECTION('center_axis',(-0.0438573043099532,0.987363722881898,0.152280713143399));
#87289=DIRECTION('ref_axis',(-0.997408629008132,-0.034572636386421,-0.0630932610776304));
#87290=DIRECTION('center_axis',(0.016842266717739,0.987363722512254,-0.157572895888073));
#87291=DIRECTION('ref_axis',(-0.991138258333607,-0.00428129664525406,-0.132765294284534));
#87292=DIRECTION('',(0.517380356258672,0.,0.855755553273042));
#87293=DIRECTION('center_axis',(-0.0271358127186797,-0.987363722769501,
0.156129839002188));
#87294=DIRECTION('ref_axis',(-0.940625789107942,-0.0276461754538182,-0.33831762272728));
#87295=DIRECTION('center_axis',(0.0314670689078621,-0.987366232801023,-0.155298892135983));
#87296=DIRECTION('ref_axis',(-0.912535322196976,0.0350112862613325,-0.407496620326093));
#87297=DIRECTION('',(-0.946969945721879,0.,0.321322146606022));
#87298=DIRECTION('center_axis',(-5.57844440175138E-14,-1.,-2.035924760324E-14));
#87299=DIRECTION('ref_axis',(1.,-5.57844440175138E-14,-8.55013534209805E-31));
#87300=DIRECTION('center_axis',(-0.0755677933535081,0.987363722995108,0.139292451772959));
#87301=DIRECTION('ref_axis',(-0.960526584060122,-0.0345726329790713,-0.276031545955689));
#87302=DIRECTION('center_axis',(0.0503220214550908,0.98736372254472,-0.150268338512501));
#87303=DIRECTION('ref_axis',(-0.939425383102902,-0.00428129350617084,-0.342726742621407));
#87304=DIRECTION('',(0.321322141912006,0.,0.946969947314634));
#87305=DIRECTION('center_axis',(-0.0600646941385593,-0.987363722798142,
0.146646211748671));
#87306=DIRECTION('ref_axis',(-0.84590619296491,-0.0276461737180322,-0.532614684159538));
#87307=DIRECTION('center_axis',(0.0641160512521902,-0.987366232586723,-0.144903604921779));
#87308=DIRECTION('ref_axis',(-0.803601026101154,0.0350112937354277,-0.594137694613079));
#87309=DIRECTION('',(-0.993905077902487,0.,0.110239267593957));
#87310=DIRECTION('center_axis',(7.51553974837504E-14,-1.,4.78128993183431E-14));
#87311=DIRECTION('ref_axis',(1.,7.51553974837504E-14,7.6276596824472E-31));
#87312=DIRECTION('center_axis',(-0.103744825459102,0.987363722817035,0.119791026606108));
#87313=DIRECTION('ref_axis',(-0.87873138215879,-0.0345726390575195,-0.47606290617722));
#87314=DIRECTION('center_axis',(0.0814487732528563,0.987363722547936,-0.135937400048282));
#87315=DIRECTION('ref_axis',(-0.843786021557471,-0.00428129117531677,-0.536662669066974));
#87316=DIRECTION('',(0.110239262352301,0.,0.993905078483866));
#87317=DIRECTION('center_axis',(-0.0901850156524691,-0.987363722797321,
0.130305571084201));
#87318=DIRECTION('ref_axis',(-0.711632962922774,-0.0276461737828286,-0.702007275715091));
#87319=DIRECTION('center_axis',(0.0937670542025258,-0.98736623292584,-0.127732774275111));
#87320=DIRECTION('ref_axis',(-0.657091237794409,0.0350112811773555,-0.752997553385223));
#87321=DIRECTION('',(-0.994366313661193,0.,-0.105998274777704));
#87322=DIRECTION('center_axis',(2.10399820468787E-14,-1.,2.09504164275063E-14));
#87323=DIRECTION('ref_axis',(1.,2.10399820468787E-14,1.6752221775065E-31));
#87324=DIRECTION('center_axis',(-0.12707085922723,0.987363722782335,0.0946883079828834));
#87325=DIRECTION('ref_axis',(-0.755847677170102,-0.0345726392425312,-0.653834093277773));
#87326=DIRECTION('center_axis',(0.108767068286513,0.98736372251492,-0.115250181422144));
#87327=DIRECTION('ref_axis',(-0.708692162259974,-0.00428129244825316,-0.705504847386788));
#87328=DIRECTION('',(-0.105998282549184,0.,0.994366312832763));
#87329=DIRECTION('center_axis',(-0.116088384586537,-0.987363722707326,0.107871989161319));
#87330=DIRECTION('ref_axis',(-0.544084566223478,-0.0276461767386126,-0.838574787189042));
#87331=DIRECTION('center_axis',(0.119033597923905,-0.987366232659441,-0.104589316706792));
#87332=DIRECTION('ref_axis',(-0.479856595381014,0.0350112912223035,-0.876648080677925));
#87333=DIRECTION('',(-0.94833208570079,0.,-0.317279459200228));
#87334=DIRECTION('center_axis',(1.12310510839231E-13,-1.,1.74885070496406E-13));
#87335=DIRECTION('ref_axis',(2.80148662775557E-30,-1.74885070496406E-13,
-1.));
#87336=DIRECTION('center_axis',(-0.144455198836148,0.987363722863726,0.0651580716557243));
#87337=DIRECTION('ref_axis',(-0.597621377110798,-0.0345726367517376,-0.801032722432876));
#87338=DIRECTION('center_axis',(0.130999534217845,0.987363722517991,-0.0891739955935754));
#87339=DIRECTION('ref_axis',(-0.540460646669499,-0.00428129707550931,-0.841358401572682));
#87340=DIRECTION('',(-0.317279463900984,0.,0.948332084128078));
#87341=DIRECTION('center_axis',(-0.136563593350214,-0.987363722837716,0.0803944263946385));
#87342=DIRECTION('ref_axis',(-0.351095380460181,-0.0276461718789811,-0.935931473453029));
#87343=DIRECTION('center_axis',(0.138734270925482,-0.987366232734516,-0.0765553690241583));
#87344=DIRECTION('ref_axis',(-0.280184390699922,0.0350112884613783,-0.959307519457858));
#87345=DIRECTION('',(-0.85795490315098,0.,-0.513725008306187));
#87346=DIRECTION('center_axis',(-2.059703798478E-14,-1.,-5.56970842119747E-14));
#87347=DIRECTION('ref_axis',(-9.34353377149569E-31,5.56970842119747E-14,
-1.));
#87348=DIRECTION('center_axis',(-0.155084976578115,0.987363722815606,0.032581112741468));
#87349=DIRECTION('ref_axis',(-0.411450964096934,-0.0345726385626235,-0.910775953133657));
#87350=DIRECTION('center_axis',(0.147106613134512,0.987363722546665,-0.0589281237685905));
#87351=DIRECTION('ref_axis',(-0.346957789155213,-0.00428129112961885,-0.937870973583675));
#87352=DIRECTION('',(-0.513725012558988,0.,0.857954900604495));
#87353=DIRECTION('center_axis',(-0.150653237000636,-0.987363722747342,0.0491577174382569));
#87354=DIRECTION('ref_axis',(-0.141689365085258,-0.0276461757563053,-0.989525044042741));
#87355=DIRECTION('center_axis',(0.151947881918142,-0.987366232725817,-0.0449417807103583));
#87356=DIRECTION('ref_axis',(-0.067411075721759,0.0350112894293617,-0.997110804515992));
#87357=DIRECTION('',(-0.727460703861421,0.,-0.686149345505369));
#87358=DIRECTION('center_axis',(-1.2213395960312E-14,-1.,-8.82340075326601E-14));
#87359=DIRECTION('ref_axis',(-6.8312927238905E-32,8.82340075326601E-14,
-1.));
#87360=DIRECTION('center_axis',(-0.158463151597563,0.987363722911698,-0.00151929711346461));
#87361=DIRECTION('ref_axis',(-0.206041562667633,-0.0345726345089346,-0.977932312277589));
#87362=DIRECTION('center_axis',(0.156335146712928,0.987363722543225,-0.0259268453120185));
#87363=DIRECTION('ref_axis',(-0.137231572949308,-0.00428129286093705,-0.990529740046859));
#87364=DIRECTION('',(-0.686149350632658,0.,0.727460699025302));
#87365=DIRECTION('center_axis',(-0.157698504326823,-0.987363722731835,0.0156224443098921));
#87366=DIRECTION('ref_axis',(0.0743418882063654,-0.0276461754851028,-0.996849523568607));
#87367=DIRECTION('center_axis',(0.158056579374827,-0.987366232721537,-0.0112267625613302));
#87368=DIRECTION('ref_axis',(0.148514306471102,0.0350112882390293,-0.988290296658452));
#87369=DIRECTION('',(-0.562951250125031,0.,-0.826490102773569));
#87370=DIRECTION('center_axis',(1.17330831551609E-14,-1.,-1.47994441068827E-13));
#87371=DIRECTION('ref_axis',(4.1412559795609E-31,1.47994441068827E-13,-1.));
#87372=DIRECTION('center_axis',(-0.154431767114463,0.987363722967678,-0.0355486690793248));
#87373=DIRECTION('ref_axis',(0.00900211458576799,-0.0345726332720927,-0.999361643731446));
#87374=DIRECTION('center_axis',(0.158253623050005,0.987363722546468,0.00828674789823349));
#87375=DIRECTION('ref_axis',(0.078911438306756,-0.00428129000922054,-0.99687243690465));
#87376=DIRECTION('',(-0.826490105990566,0.,0.562951245402036));
#87377=DIRECTION('center_axis',(-0.157369964369938,-0.987363722781335,-0.018643316485744));
#87378=DIRECTION('ref_axis',(0.28689699642415,-0.0276461754527353,-0.957562427430002));
#87379=DIRECTION('center_axis',(0.156774723284306,-0.987366233007562,0.0230132148033821));
#87380=DIRECTION('ref_axis',(0.357495326215101,0.0350112783984714,-0.933258432653712));
#87381=DIRECTION('',(-0.372118820942155,0.,-0.928185101744593));
#87382=DIRECTION('center_axis',(1.73092801111523E-14,-1.,-5.68048588197779E-14));
#87383=DIRECTION('ref_axis',(-3.73483020556181E-31,5.68048588197779E-14,
-1.));
#87384=DIRECTION('center_axis',(-0.143179323934678,0.987363722859351,-0.0679158301055866));
#87385=DIRECTION('ref_axis',(0.223624860699663,-0.0345726379955593,-0.974061935597057));
#87386=DIRECTION('center_axis',(0.152772335844917,0.987363722537645,0.04211285809693));
#87387=DIRECTION('ref_axis',(0.291364638567275,-0.00428129121433651,-0.9566024868973));
#87388=DIRECTION('',(-0.928185103589145,0.,0.372118816341243));
#87389=DIRECTION('center_axis',(-0.149682979293308,-0.987363722808054,-0.0520373384455801));
#87390=DIRECTION('ref_axis',(0.486037120909077,-0.0276461734877023,-0.873500776296108));
#87391=DIRECTION('center_axis',(0.148162258618649,-0.987366232901802,0.0561771060693289));
#87392=DIRECTION('ref_axis',(0.549760259598465,0.0350112827382477,-0.834588441716785));
#87393=DIRECTION('',(-0.163886529631915,0.,-0.986479196640866));
#87394=DIRECTION('center_axis',(-1.45579821417781E-14,-1.,2.58779046247183E-14));
#87395=DIRECTION('ref_axis',(3.97422477312386E-31,-2.58779046247183E-14,
-1.));
#87396=DIRECTION('center_axis',(-0.125231975789399,0.987363722872469,-0.097107316898887));
#87397=DIRECTION('ref_axis',(0.427791161340583,-0.034572636188313,-0.90321617296518));
#87398=DIRECTION('center_axis',(0.140147584035429,0.987363722542533,0.0739698188181151));
#87399=DIRECTION('ref_axis',(0.490193954158814,-0.00428129181852567,-0.871602867048125));
#87400=DIRECTION('',(-0.986479197453234,0.,0.16388652474204));
#87401=DIRECTION('center_axis',(-0.134996984326904,-0.987363722815423,-0.0829981511282625));
#87402=DIRECTION('ref_axis',(0.66245069095475,-0.0276461728301328,-0.748595198476066));
#87403=DIRECTION('center_axis',(0.132621887525639,-0.987366233003682,0.0867142253223539));
#87404=DIRECTION('ref_axis',(0.716319015462737,0.035011278959132,-0.696894022382271));
#87405=DIRECTION('',(0.0520089118984746,0.,-0.998646620723836));
#87406=DIRECTION('center_axis',(-5.93418274472076E-14,-1.,6.64300732659738E-14));
#87407=DIRECTION('ref_axis',(-2.84771056551696E-30,-6.64300732659738E-14,
-1.));
#87408=DIRECTION('center_axis',(-0.10142891811791,0.987363722837423,-0.121758175881763));
#87409=DIRECTION('ref_axis',(0.611954418604463,-0.0345726379864004,-0.790137027516832));
#87410=DIRECTION('center_axis',(0.120969685025489,0.987363722554852,0.102368035477193));
